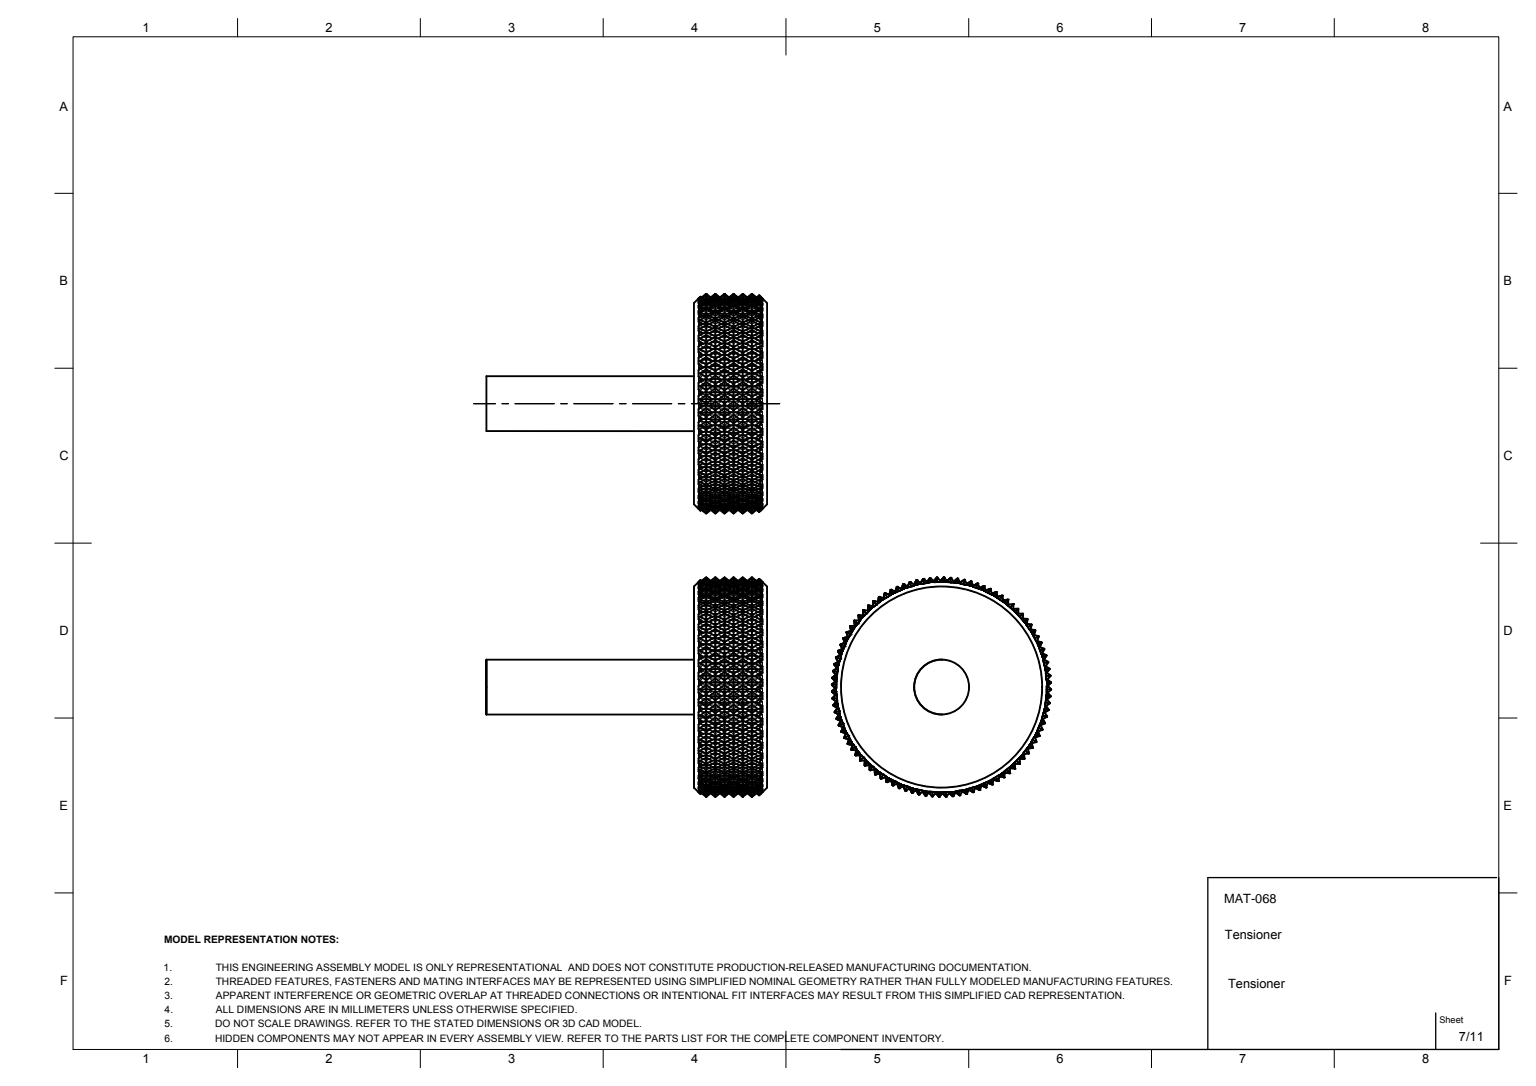
ISO-10303-21;
HEADER;
/* Generated by software containing ST-Developer
 * from STEP Tools, Inc. (www.steptools.com) 
 */

FILE_DESCRIPTION(
/* description */ ('CAx-IF Rec.Pracs.---Representation and Presentation of Product Manufa
cturing Information (PMI)---4.0---2014-10-13'),
/* implementation_level */ '2;1');

FILE_NAME(
/* name */ 'Tensioner.step',
/* time_stamp */ '2026-10-24T16:53:48-07:00',
/* author */ (''),
/* organization */ (''),
/* preprocessor_version */ 'ST-DEVELOPER v20.2',
/* originating_system */ 'Autodesk Translation Framework v15.17.0.0',
/* authorisation */ '');

FILE_SCHEMA (('AP242_MANAGED_MODEL_BASED_3D_ENGINEERING_MIM_LF { 1 0 10303 442 2 1 4 }'));
ENDSEC;

DATA;
#10=MECHANICAL_DESIGN_GEOMETRIC_PRESENTATION_REPRESENTATION('',(#3494),#107910);
#51=(
BOUNDED_CURVE()
B_SPLINE_CURVE(2,(#91091,#91092,#91093,#91094,#91095),.UNSPECIFIED.,.F.,
 .F.)
B_SPLINE_CURVE_WITH_KNOTS((3,2,3),(0.457349576892943,0.480683592164461,
0.539236617436895),.UNSPECIFIED.)
CURVE()
GEOMETRIC_REPRESENTATION_ITEM()
RATIONAL_B_SPLINE_CURVE((0.999326490452302,0.99964606396824,1.,0.999111853439226,
0.998440080679707))
REPRESENTATION_ITEM('')
);
#52=(
BOUNDED_CURVE()
B_SPLINE_CURVE(2,(#91384,#91385,#91386,#91387,#91388),.UNSPECIFIED.,.F.,
 .F.)
B_SPLINE_CURVE_WITH_KNOTS((3,2,3),(0.457349576892961,0.480683592164461,
0.539236615838568),.UNSPECIFIED.)
CURVE()
GEOMETRIC_REPRESENTATION_ITEM()
RATIONAL_B_SPLINE_CURVE((0.999326490452302,0.999646063968241,1.,0.99911185346347,
0.998440080716382))
REPRESENTATION_ITEM('')
);
#53=(
BOUNDED_CURVE()
B_SPLINE_CURVE(2,(#91904,#91905,#91906,#91907,#91908),.UNSPECIFIED.,.F.,
 .F.)
B_SPLINE_CURVE_WITH_KNOTS((3,2,3),(0.457349576892952,0.480683592164462,
0.539236618408897),.UNSPECIFIED.)
CURVE()
GEOMETRIC_REPRESENTATION_ITEM()
RATIONAL_B_SPLINE_CURVE((0.999326490452302,0.999646063968241,1.,0.999111853424483,
0.998440080657404))
REPRESENTATION_ITEM('')
);
#54=(
BOUNDED_CURVE()
B_SPLINE_CURVE(2,(#92179,#92180,#92181,#92182,#92183),.UNSPECIFIED.,.F.,
 .F.)
B_SPLINE_CURVE_WITH_KNOTS((3,2,3),(0.457349576892958,0.480683592164462,
0.539236618408893),.UNSPECIFIED.)
CURVE()
GEOMETRIC_REPRESENTATION_ITEM()
RATIONAL_B_SPLINE_CURVE((0.999326490452302,0.999646063968241,1.,0.999111853424483,
0.998440080657404))
REPRESENTATION_ITEM('')
);
#55=(
BOUNDED_CURVE()
B_SPLINE_CURVE(2,(#92403,#92404,#92405,#92406,#92407),.UNSPECIFIED.,.F.,
 .F.)
B_SPLINE_CURVE_WITH_KNOTS((3,2,3),(0.457349576892958,0.480683592164463,
0.539236618408894),.UNSPECIFIED.)
CURVE()
GEOMETRIC_REPRESENTATION_ITEM()
RATIONAL_B_SPLINE_CURVE((0.999326490452302,0.999646063968241,1.,0.999111853424483,
0.998440080657404))
REPRESENTATION_ITEM('')
);
#56=(
BOUNDED_CURVE()
B_SPLINE_CURVE(2,(#92707,#92708,#92709,#92710,#92711),.UNSPECIFIED.,.F.,
 .F.)
B_SPLINE_CURVE_WITH_KNOTS((3,2,3),(0.457349576892963,0.480683592164461,
0.539236618408894),.UNSPECIFIED.)
CURVE()
GEOMETRIC_REPRESENTATION_ITEM()
RATIONAL_B_SPLINE_CURVE((0.999326490452302,0.999646063968241,1.,0.999111853424483,
0.998440080657404))
REPRESENTATION_ITEM('')
);
#57=(
BOUNDED_CURVE()
B_SPLINE_CURVE(2,(#93011,#93012,#93013,#93014,#93015),.UNSPECIFIED.,.F.,
 .F.)
B_SPLINE_CURVE_WITH_KNOTS((3,2,3),(0.457349576892959,0.480683592164461,
0.539236618408895),.UNSPECIFIED.)
CURVE()
GEOMETRIC_REPRESENTATION_ITEM()
RATIONAL_B_SPLINE_CURVE((0.999326490452302,0.999646063968241,1.,0.999111853424483,
0.998440080657404))
REPRESENTATION_ITEM('')
);
#58=(
BOUNDED_CURVE()
B_SPLINE_CURVE(2,(#93315,#93316,#93317,#93318,#93319),.UNSPECIFIED.,.F.,
 .F.)
B_SPLINE_CURVE_WITH_KNOTS((3,2,3),(0.457349576892959,0.480683592164461,
0.539236615838582),.UNSPECIFIED.)
CURVE()
GEOMETRIC_REPRESENTATION_ITEM()
RATIONAL_B_SPLINE_CURVE((0.999326490452302,0.999646063968241,1.,0.99911185346347,
0.998440080716382))
REPRESENTATION_ITEM('')
);
#59=(
BOUNDED_CURVE()
B_SPLINE_CURVE(2,(#93619,#93620,#93621,#93622,#93623),.UNSPECIFIED.,.F.,
 .F.)
B_SPLINE_CURVE_WITH_KNOTS((3,2,3),(0.457349576892961,0.480683592164461,
0.539236618408892),.UNSPECIFIED.)
CURVE()
GEOMETRIC_REPRESENTATION_ITEM()
RATIONAL_B_SPLINE_CURVE((0.999326490452302,0.999646063968241,1.,0.999111853424483,
0.998440080657404))
REPRESENTATION_ITEM('')
);
#60=(
BOUNDED_CURVE()
B_SPLINE_CURVE(2,(#93923,#93924,#93925,#93926,#93927),.UNSPECIFIED.,.F.,
 .F.)
B_SPLINE_CURVE_WITH_KNOTS((3,2,3),(0.457349576892952,0.480683592164462,
0.539236615838583),.UNSPECIFIED.)
CURVE()
GEOMETRIC_REPRESENTATION_ITEM()
RATIONAL_B_SPLINE_CURVE((0.999326490452302,0.999646063968241,1.,0.99911185346347,
0.998440080716382))
REPRESENTATION_ITEM('')
);
#61=(
BOUNDED_CURVE()
B_SPLINE_CURVE(2,(#94227,#94228,#94229,#94230,#94231),.UNSPECIFIED.,.F.,
 .F.)
B_SPLINE_CURVE_WITH_KNOTS((3,2,3),(0.457349576892963,0.48068359216447,0.539236618408901),
 .UNSPECIFIED.)
CURVE()
GEOMETRIC_REPRESENTATION_ITEM()
RATIONAL_B_SPLINE_CURVE((0.999326490452302,0.999646063968241,1.,0.999111853424483,
0.998440080657404))
REPRESENTATION_ITEM('')
);
#62=(
BOUNDED_CURVE()
B_SPLINE_CURVE(2,(#94531,#94532,#94533,#94534,#94535),.UNSPECIFIED.,.F.,
 .F.)
B_SPLINE_CURVE_WITH_KNOTS((3,2,3),(0.457349576892948,0.48068359216446,0.539236618408892),
 .UNSPECIFIED.)
CURVE()
GEOMETRIC_REPRESENTATION_ITEM()
RATIONAL_B_SPLINE_CURVE((0.999326490452302,0.999646063968241,1.,0.999111853424483,
0.998440080657404))
REPRESENTATION_ITEM('')
);
#63=(
BOUNDED_CURVE()
B_SPLINE_CURVE(2,(#94835,#94836,#94837,#94838,#94839),.UNSPECIFIED.,.F.,
 .F.)
B_SPLINE_CURVE_WITH_KNOTS((3,2,3),(0.457349576892957,0.480683592164462,
0.539236618408896),.UNSPECIFIED.)
CURVE()
GEOMETRIC_REPRESENTATION_ITEM()
RATIONAL_B_SPLINE_CURVE((0.999326490452302,0.999646063968241,1.,0.999111853424483,
0.998440080657404))
REPRESENTATION_ITEM('')
);
#64=(
BOUNDED_CURVE()
B_SPLINE_CURVE(2,(#95139,#95140,#95141,#95142,#95143),.UNSPECIFIED.,.F.,
 .F.)
B_SPLINE_CURVE_WITH_KNOTS((3,2,3),(0.457349576892956,0.48068359216446,0.539236617436898),
 .UNSPECIFIED.)
CURVE()
GEOMETRIC_REPRESENTATION_ITEM()
RATIONAL_B_SPLINE_CURVE((0.999326490452302,0.999646063968241,1.,0.999111853439226,
0.998440080679707))
REPRESENTATION_ITEM('')
);
#65=(
BOUNDED_CURVE()
B_SPLINE_CURVE(2,(#95443,#95444,#95445,#95446,#95447),.UNSPECIFIED.,.F.,
 .F.)
B_SPLINE_CURVE_WITH_KNOTS((3,2,3),(0.457349576892961,0.480683592164473,
0.539236615838594),.UNSPECIFIED.)
CURVE()
GEOMETRIC_REPRESENTATION_ITEM()
RATIONAL_B_SPLINE_CURVE((0.999326490452302,0.999646063968241,1.,0.99911185346347,
0.998440080716382))
REPRESENTATION_ITEM('')
);
#66=(
BOUNDED_CURVE()
B_SPLINE_CURVE(2,(#95747,#95748,#95749,#95750,#95751),.UNSPECIFIED.,.F.,
 .F.)
B_SPLINE_CURVE_WITH_KNOTS((3,2,3),(0.457349576892959,0.480683592164459,
0.539236618408898),.UNSPECIFIED.)
CURVE()
GEOMETRIC_REPRESENTATION_ITEM()
RATIONAL_B_SPLINE_CURVE((0.999326490452302,0.999646063968241,1.,0.999111853424483,
0.998440080657404))
REPRESENTATION_ITEM('')
);
#67=(
BOUNDED_CURVE()
B_SPLINE_CURVE(2,(#96051,#96052,#96053,#96054,#96055),.UNSPECIFIED.,.F.,
 .F.)
B_SPLINE_CURVE_WITH_KNOTS((3,2,3),(0.457349576892962,0.480683592164469,
0.539236618408905),.UNSPECIFIED.)
CURVE()
GEOMETRIC_REPRESENTATION_ITEM()
RATIONAL_B_SPLINE_CURVE((0.999326490452302,0.999646063968241,1.,0.999111853424483,
0.998440080657404))
REPRESENTATION_ITEM('')
);
#68=(
BOUNDED_CURVE()
B_SPLINE_CURVE(2,(#96355,#96356,#96357,#96358,#96359),.UNSPECIFIED.,.F.,
 .F.)
B_SPLINE_CURVE_WITH_KNOTS((3,2,3),(0.457349576892966,0.480683592164469,
0.539236618408905),.UNSPECIFIED.)
CURVE()
GEOMETRIC_REPRESENTATION_ITEM()
RATIONAL_B_SPLINE_CURVE((0.999326490452302,0.999646063968241,1.,0.999111853424483,
0.998440080657404))
REPRESENTATION_ITEM('')
);
#69=(
BOUNDED_CURVE()
B_SPLINE_CURVE(2,(#96659,#96660,#96661,#96662,#96663),.UNSPECIFIED.,.F.,
 .F.)
B_SPLINE_CURVE_WITH_KNOTS((3,2,3),(0.457349576892951,0.48068359216446,0.539236618408896),
 .UNSPECIFIED.)
CURVE()
GEOMETRIC_REPRESENTATION_ITEM()
RATIONAL_B_SPLINE_CURVE((0.999326490452302,0.999646063968241,1.,0.999111853424483,
0.998440080657404))
REPRESENTATION_ITEM('')
);
#70=(
BOUNDED_CURVE()
B_SPLINE_CURVE(2,(#96963,#96964,#96965,#96966,#96967),.UNSPECIFIED.,.F.,
 .F.)
B_SPLINE_CURVE_WITH_KNOTS((3,2,3),(0.457349576892956,0.480683592164461,
0.539236618408896),.UNSPECIFIED.)
CURVE()
GEOMETRIC_REPRESENTATION_ITEM()
RATIONAL_B_SPLINE_CURVE((0.999326490452302,0.999646063968241,1.,0.999111853424483,
0.998440080657404))
REPRESENTATION_ITEM('')
);
#71=(
BOUNDED_CURVE()
B_SPLINE_CURVE(2,(#97267,#97268,#97269,#97270,#97271),.UNSPECIFIED.,.F.,
 .F.)
B_SPLINE_CURVE_WITH_KNOTS((3,2,3),(0.457349576892952,0.480683592164461,
0.539236618408892),.UNSPECIFIED.)
CURVE()
GEOMETRIC_REPRESENTATION_ITEM()
RATIONAL_B_SPLINE_CURVE((0.999326490452302,0.999646063968241,1.,0.999111853424483,
0.998440080657404))
REPRESENTATION_ITEM('')
);
#72=(
BOUNDED_CURVE()
B_SPLINE_CURVE(2,(#97571,#97572,#97573,#97574,#97575),.UNSPECIFIED.,.F.,
 .F.)
B_SPLINE_CURVE_WITH_KNOTS((3,2,3),(0.457349576892964,0.480683592164459,
0.539236618408898),.UNSPECIFIED.)
CURVE()
GEOMETRIC_REPRESENTATION_ITEM()
RATIONAL_B_SPLINE_CURVE((0.999326490452302,0.999646063968241,1.,0.999111853424483,
0.998440080657404))
REPRESENTATION_ITEM('')
);
#73=(
BOUNDED_CURVE()
B_SPLINE_CURVE(2,(#97875,#97876,#97877,#97878,#97879),.UNSPECIFIED.,.F.,
 .F.)
B_SPLINE_CURVE_WITH_KNOTS((3,2,3),(0.457349576892949,0.480683592164462,
0.539236618408898),.UNSPECIFIED.)
CURVE()
GEOMETRIC_REPRESENTATION_ITEM()
RATIONAL_B_SPLINE_CURVE((0.999326490452302,0.999646063968241,1.,0.999111853424483,
0.998440080657404))
REPRESENTATION_ITEM('')
);
#74=(
BOUNDED_CURVE()
B_SPLINE_CURVE(2,(#98179,#98180,#98181,#98182,#98183),.UNSPECIFIED.,.F.,
 .F.)
B_SPLINE_CURVE_WITH_KNOTS((3,2,3),(0.457349576892952,0.48068359216446,0.539236615838581),
 .UNSPECIFIED.)
CURVE()
GEOMETRIC_REPRESENTATION_ITEM()
RATIONAL_B_SPLINE_CURVE((0.999326490452302,0.999646063968241,1.,0.99911185346347,
0.998440080716382))
REPRESENTATION_ITEM('')
);
#75=(
BOUNDED_CURVE()
B_SPLINE_CURVE(2,(#98483,#98484,#98485,#98486,#98487),.UNSPECIFIED.,.F.,
 .F.)
B_SPLINE_CURVE_WITH_KNOTS((3,2,3),(0.457349576892958,0.48068359216446,0.539236618408894),
 .UNSPECIFIED.)
CURVE()
GEOMETRIC_REPRESENTATION_ITEM()
RATIONAL_B_SPLINE_CURVE((0.999326490452302,0.999646063968241,1.,0.999111853424483,
0.998440080657404))
REPRESENTATION_ITEM('')
);
#76=(
BOUNDED_CURVE()
B_SPLINE_CURVE(2,(#98787,#98788,#98789,#98790,#98791),.UNSPECIFIED.,.F.,
 .F.)
B_SPLINE_CURVE_WITH_KNOTS((3,2,3),(0.457349576892947,0.480683592164461,
0.539236617436902),.UNSPECIFIED.)
CURVE()
GEOMETRIC_REPRESENTATION_ITEM()
RATIONAL_B_SPLINE_CURVE((0.999326490452302,0.999646063968241,1.,0.999111853439226,
0.998440080679707))
REPRESENTATION_ITEM('')
);
#77=(
BOUNDED_CURVE()
B_SPLINE_CURVE(2,(#99091,#99092,#99093,#99094,#99095),.UNSPECIFIED.,.F.,
 .F.)
B_SPLINE_CURVE_WITH_KNOTS((3,2,3),(0.457349576892974,0.48068359216447,0.539236615838595),
 .UNSPECIFIED.)
CURVE()
GEOMETRIC_REPRESENTATION_ITEM()
RATIONAL_B_SPLINE_CURVE((0.999326490452302,0.999646063968241,1.,0.99911185346347,
0.998440080716382))
REPRESENTATION_ITEM('')
);
#78=(
BOUNDED_CURVE()
B_SPLINE_CURVE(2,(#99395,#99396,#99397,#99398,#99399),.UNSPECIFIED.,.F.,
 .F.)
B_SPLINE_CURVE_WITH_KNOTS((3,2,3),(0.457349576892952,0.480683592164461,
0.539236615838591),.UNSPECIFIED.)
CURVE()
GEOMETRIC_REPRESENTATION_ITEM()
RATIONAL_B_SPLINE_CURVE((0.999326490452302,0.999646063968241,1.,0.99911185346347,
0.998440080716382))
REPRESENTATION_ITEM('')
);
#79=(
BOUNDED_CURVE()
B_SPLINE_CURVE(2,(#99699,#99700,#99701,#99702,#99703),.UNSPECIFIED.,.F.,
 .F.)
B_SPLINE_CURVE_WITH_KNOTS((3,2,3),(0.457349576892966,0.480683592164471,
0.539236615838593),.UNSPECIFIED.)
CURVE()
GEOMETRIC_REPRESENTATION_ITEM()
RATIONAL_B_SPLINE_CURVE((0.999326490452302,0.999646063968241,1.,0.99911185346347,
0.998440080716382))
REPRESENTATION_ITEM('')
);
#80=(
BOUNDED_CURVE()
B_SPLINE_CURVE(2,(#100003,#100004,#100005,#100006,#100007),
 .UNSPECIFIED.,.F.,.F.)
B_SPLINE_CURVE_WITH_KNOTS((3,2,3),(0.457349576892955,0.48068359216446,0.539236618408892),
 .UNSPECIFIED.)
CURVE()
GEOMETRIC_REPRESENTATION_ITEM()
RATIONAL_B_SPLINE_CURVE((0.999326490452302,0.999646063968241,1.,0.999111853424483,
0.998440080657404))
REPRESENTATION_ITEM('')
);
#81=(
BOUNDED_CURVE()
B_SPLINE_CURVE(2,(#100307,#100308,#100309,#100310,#100311),
 .UNSPECIFIED.,.F.,.F.)
B_SPLINE_CURVE_WITH_KNOTS((3,2,3),(0.457349576892948,0.480683592164461,
0.539236618408894),.UNSPECIFIED.)
CURVE()
GEOMETRIC_REPRESENTATION_ITEM()
RATIONAL_B_SPLINE_CURVE((0.999326490452302,0.999646063968241,1.,0.999111853424483,
0.998440080657404))
REPRESENTATION_ITEM('')
);
#82=(
BOUNDED_CURVE()
B_SPLINE_CURVE(2,(#100611,#100612,#100613,#100614,#100615),
 .UNSPECIFIED.,.F.,.F.)
B_SPLINE_CURVE_WITH_KNOTS((3,2,3),(0.457349576892958,0.480683592164462,
0.539236615838579),.UNSPECIFIED.)
CURVE()
GEOMETRIC_REPRESENTATION_ITEM()
RATIONAL_B_SPLINE_CURVE((0.999326490452302,0.999646063968241,1.,0.99911185346347,
0.998440080716382))
REPRESENTATION_ITEM('')
);
#83=(
BOUNDED_CURVE()
B_SPLINE_CURVE(2,(#100915,#100916,#100917,#100918,#100919),
 .UNSPECIFIED.,.F.,.F.)
B_SPLINE_CURVE_WITH_KNOTS((3,2,3),(0.457349576892956,0.48068359216446,0.539236618408897),
 .UNSPECIFIED.)
CURVE()
GEOMETRIC_REPRESENTATION_ITEM()
RATIONAL_B_SPLINE_CURVE((0.999326490452302,0.999646063968241,1.,0.999111853424483,
0.998440080657404))
REPRESENTATION_ITEM('')
);
#84=(
BOUNDED_CURVE()
B_SPLINE_CURVE(2,(#101219,#101220,#101221,#101222,#101223),
 .UNSPECIFIED.,.F.,.F.)
B_SPLINE_CURVE_WITH_KNOTS((3,2,3),(0.457349576892958,0.480683592164462,
0.539236618408895),.UNSPECIFIED.)
CURVE()
GEOMETRIC_REPRESENTATION_ITEM()
RATIONAL_B_SPLINE_CURVE((0.999326490452302,0.999646063968241,1.,0.999111853424483,
0.998440080657404))
REPRESENTATION_ITEM('')
);
#85=(
BOUNDED_CURVE()
B_SPLINE_CURVE(2,(#101523,#101524,#101525,#101526,#101527),
 .UNSPECIFIED.,.F.,.F.)
B_SPLINE_CURVE_WITH_KNOTS((3,2,3),(0.457349576892956,0.480683592164458,
0.539236615838573),.UNSPECIFIED.)
CURVE()
GEOMETRIC_REPRESENTATION_ITEM()
RATIONAL_B_SPLINE_CURVE((0.999326490452302,0.999646063968241,1.,0.99911185346347,
0.998440080716382))
REPRESENTATION_ITEM('')
);
#86=(
BOUNDED_CURVE()
B_SPLINE_CURVE(2,(#101827,#101828,#101829,#101830,#101831),
 .UNSPECIFIED.,.F.,.F.)
B_SPLINE_CURVE_WITH_KNOTS((3,2,3),(0.457349576892953,0.48068359216446,0.539236618408898),
 .UNSPECIFIED.)
CURVE()
GEOMETRIC_REPRESENTATION_ITEM()
RATIONAL_B_SPLINE_CURVE((0.999326490452302,0.999646063968241,1.,0.999111853424483,
0.998440080657404))
REPRESENTATION_ITEM('')
);
#87=(
BOUNDED_CURVE()
B_SPLINE_CURVE(2,(#102131,#102132,#102133,#102134,#102135),
 .UNSPECIFIED.,.F.,.F.)
B_SPLINE_CURVE_WITH_KNOTS((3,2,3),(0.457349576892963,0.480683592164461,
0.539236618408896),.UNSPECIFIED.)
CURVE()
GEOMETRIC_REPRESENTATION_ITEM()
RATIONAL_B_SPLINE_CURVE((0.999326490452302,0.999646063968241,1.,0.999111853424483,
0.998440080657404))
REPRESENTATION_ITEM('')
);
#88=(
BOUNDED_CURVE()
B_SPLINE_CURVE(2,(#102435,#102436,#102437,#102438,#102439),
 .UNSPECIFIED.,.F.,.F.)
B_SPLINE_CURVE_WITH_KNOTS((3,2,3),(0.457349576892965,0.480683592164474,
0.539236615838598),.UNSPECIFIED.)
CURVE()
GEOMETRIC_REPRESENTATION_ITEM()
RATIONAL_B_SPLINE_CURVE((0.999326490452302,0.999646063968241,1.,0.99911185346347,
0.998440080716382))
REPRESENTATION_ITEM('')
);
#89=(
BOUNDED_CURVE()
B_SPLINE_CURVE(2,(#102739,#102740,#102741,#102742,#102743),
 .UNSPECIFIED.,.F.,.F.)
B_SPLINE_CURVE_WITH_KNOTS((3,2,3),(0.457349576892951,0.480683592164463,
0.5392366174369),.UNSPECIFIED.)
CURVE()
GEOMETRIC_REPRESENTATION_ITEM()
RATIONAL_B_SPLINE_CURVE((0.999326490452302,0.999646063968241,1.,0.999111853439226,
0.998440080679707))
REPRESENTATION_ITEM('')
);
#90=(
BOUNDED_CURVE()
B_SPLINE_CURVE(2,(#103043,#103044,#103045,#103046,#103047),
 .UNSPECIFIED.,.F.,.F.)
B_SPLINE_CURVE_WITH_KNOTS((3,2,3),(0.45734957689296,0.480683592164459,0.539236618408886),
 .UNSPECIFIED.)
CURVE()
GEOMETRIC_REPRESENTATION_ITEM()
RATIONAL_B_SPLINE_CURVE((0.999326490452302,0.999646063968241,1.,0.999111853424483,
0.998440080657404))
REPRESENTATION_ITEM('')
);
#91=(
BOUNDED_CURVE()
B_SPLINE_CURVE(2,(#103347,#103348,#103349,#103350,#103351),
 .UNSPECIFIED.,.F.,.F.)
B_SPLINE_CURVE_WITH_KNOTS((3,2,3),(0.457349576892963,0.48068359216447,0.5392366184089),
 .UNSPECIFIED.)
CURVE()
GEOMETRIC_REPRESENTATION_ITEM()
RATIONAL_B_SPLINE_CURVE((0.999326490452302,0.999646063968241,1.,0.999111853424483,
0.998440080657404))
REPRESENTATION_ITEM('')
);
#92=(
BOUNDED_CURVE()
B_SPLINE_CURVE(2,(#103651,#103652,#103653,#103654,#103655),
 .UNSPECIFIED.,.F.,.F.)
B_SPLINE_CURVE_WITH_KNOTS((3,2,3),(0.457349576892972,0.480683592164467,
0.539236618408904),.UNSPECIFIED.)
CURVE()
GEOMETRIC_REPRESENTATION_ITEM()
RATIONAL_B_SPLINE_CURVE((0.999326490452302,0.999646063968241,1.,0.999111853424483,
0.998440080657404))
REPRESENTATION_ITEM('')
);
#93=(
BOUNDED_CURVE()
B_SPLINE_CURVE(2,(#103955,#103956,#103957,#103958,#103959),
 .UNSPECIFIED.,.F.,.F.)
B_SPLINE_CURVE_WITH_KNOTS((3,2,3),(0.457349576892955,0.480683592164463,
0.539236618408902),.UNSPECIFIED.)
CURVE()
GEOMETRIC_REPRESENTATION_ITEM()
RATIONAL_B_SPLINE_CURVE((0.999326490452302,0.999646063968241,1.,0.999111853424483,
0.998440080657404))
REPRESENTATION_ITEM('')
);
#94=(
BOUNDED_CURVE()
B_SPLINE_CURVE(2,(#104259,#104260,#104261,#104262,#104263),
 .UNSPECIFIED.,.F.,.F.)
B_SPLINE_CURVE_WITH_KNOTS((3,2,3),(0.457349576892956,0.48068359216446,0.539236618408889),
 .UNSPECIFIED.)
CURVE()
GEOMETRIC_REPRESENTATION_ITEM()
RATIONAL_B_SPLINE_CURVE((0.999326490452302,0.999646063968241,1.,0.999111853424483,
0.998440080657404))
REPRESENTATION_ITEM('')
);
#95=(
BOUNDED_CURVE()
B_SPLINE_CURVE(2,(#104563,#104564,#104565,#104566,#104567),
 .UNSPECIFIED.,.F.,.F.)
B_SPLINE_CURVE_WITH_KNOTS((3,2,3),(0.457349576892965,0.480683592164471,
0.539236618408903),.UNSPECIFIED.)
CURVE()
GEOMETRIC_REPRESENTATION_ITEM()
RATIONAL_B_SPLINE_CURVE((0.999326490452302,0.999646063968241,1.,0.999111853424483,
0.998440080657404))
REPRESENTATION_ITEM('')
);
#96=(
BOUNDED_CURVE()
B_SPLINE_CURVE(2,(#104867,#104868,#104869,#104870,#104871),
 .UNSPECIFIED.,.F.,.F.)
B_SPLINE_CURVE_WITH_KNOTS((3,2,3),(0.457349576892956,0.480683592164462,
0.539236618408896),.UNSPECIFIED.)
CURVE()
GEOMETRIC_REPRESENTATION_ITEM()
RATIONAL_B_SPLINE_CURVE((0.999326490452302,0.999646063968241,1.,0.999111853424483,
0.998440080657404))
REPRESENTATION_ITEM('')
);
#97=(
BOUNDED_CURVE()
B_SPLINE_CURVE(2,(#105171,#105172,#105173,#105174,#105175),
 .UNSPECIFIED.,.F.,.F.)
B_SPLINE_CURVE_WITH_KNOTS((3,2,3),(0.45734957689296,0.480683592164462,0.539236618408894),
 .UNSPECIFIED.)
CURVE()
GEOMETRIC_REPRESENTATION_ITEM()
RATIONAL_B_SPLINE_CURVE((0.999326490452302,0.999646063968241,1.,0.999111853424483,
0.998440080657404))
REPRESENTATION_ITEM('')
);
#98=(
BOUNDED_CURVE()
B_SPLINE_CURVE(2,(#105475,#105476,#105477,#105478,#105479),
 .UNSPECIFIED.,.F.,.F.)
B_SPLINE_CURVE_WITH_KNOTS((3,2,3),(0.457349576892957,0.480683592164459,
0.539236618408901),.UNSPECIFIED.)
CURVE()
GEOMETRIC_REPRESENTATION_ITEM()
RATIONAL_B_SPLINE_CURVE((0.999326490452302,0.999646063968241,1.,0.999111853424483,
0.998440080657404))
REPRESENTATION_ITEM('')
);
#99=(
BOUNDED_CURVE()
B_SPLINE_CURVE(2,(#105779,#105780,#105781,#105782,#105783),
 .UNSPECIFIED.,.F.,.F.)
B_SPLINE_CURVE_WITH_KNOTS((3,2,3),(0.457349576892957,0.480683592164462,
0.539236615838586),.UNSPECIFIED.)
CURVE()
GEOMETRIC_REPRESENTATION_ITEM()
RATIONAL_B_SPLINE_CURVE((0.999326490452302,0.999646063968241,1.,0.99911185346347,
0.998440080716382))
REPRESENTATION_ITEM('')
);
#100=(
BOUNDED_CURVE()
B_SPLINE_CURVE(2,(#106083,#106084,#106085,#106086,#106087),
 .UNSPECIFIED.,.F.,.F.)
B_SPLINE_CURVE_WITH_KNOTS((3,2,3),(0.457349576892964,0.480683592164471,
0.539236615838594),.UNSPECIFIED.)
CURVE()
GEOMETRIC_REPRESENTATION_ITEM()
RATIONAL_B_SPLINE_CURVE((0.999326490452302,0.999646063968241,1.,0.99911185346347,
0.998440080716382))
REPRESENTATION_ITEM('')
);
#101=(
BOUNDED_SURFACE()
B_SPLINE_SURFACE(1,2,((#65259,#65260,#65261),(#65262,#65263,#65264)),
 .UNSPECIFIED.,.F.,.F.,.F.)
B_SPLINE_SURFACE_WITH_KNOTS((2,2),(3,3),(0.,1.),(0.0556006976418392,0.0675888856590501),
 .UNSPECIFIED.)
GEOMETRIC_REPRESENTATION_ITEM()
RATIONAL_B_SPLINE_SURFACE(((0.996397562408606,0.996150386832629,0.997319912843745),
(0.996397562408606,0.996150386832629,0.997319912843745)))
REPRESENTATION_ITEM('')
SURFACE()
);
#102=(
BOUNDED_SURFACE()
B_SPLINE_SURFACE(1,2,((#65277,#65278,#65279),(#65280,#65281,#65282),(#65283,
#65284,#65285)),.UNSPECIFIED.,.F.,.F.,.F.)
B_SPLINE_SURFACE_WITH_KNOTS((2,1,2),(3,3),(-0.000171761237665326,1.,1.00600020634817),
(0.066589869885605,0.0751324139155164),.UNSPECIFIED.)
GEOMETRIC_REPRESENTATION_ITEM()
RATIONAL_B_SPLINE_SURFACE(((0.997134830028878,0.997884084852412,0.999352698774608),
(0.997134830028878,0.997884084852412,0.999352698774608),(0.997134830028879,
0.997884084852412,0.999352698774608)))
REPRESENTATION_ITEM('')
SURFACE()
);
#103=(
BOUNDED_SURFACE()
B_SPLINE_SURFACE(1,2,((#65395,#65396,#65397),(#65398,#65399,#65400),(#65401,
#65402,#65403)),.UNSPECIFIED.,.F.,.F.,.F.)
B_SPLINE_SURFACE_WITH_KNOTS((2,1,2),(3,3),(0.,1.,1.01),(0.0456081671210044,
0.057598944781882),.UNSPECIFIED.)
GEOMETRIC_REPRESENTATION_ITEM()
RATIONAL_B_SPLINE_SURFACE(((0.997793907739636,0.996365558499688,0.996354522974128),
(0.997793907739636,0.996365558499688,0.996354522974128),(0.997793907739636,
0.996365558499688,0.996354522974128)))
REPRESENTATION_ITEM('')
SURFACE()
);
#104=(
BOUNDED_SURFACE()
B_SPLINE_SURFACE(1,2,((#65416,#65417,#65418),(#65419,#65420,#65421),(#65422,
#65423,#65424)),.UNSPECIFIED.,.F.,.F.,.F.)
B_SPLINE_SURFACE_WITH_KNOTS((2,1,2),(3,3),(0.,1.,1.01),(0.0556006976418428,
0.0675888856590486),.UNSPECIFIED.)
GEOMETRIC_REPRESENTATION_ITEM()
RATIONAL_B_SPLINE_SURFACE(((0.996397562408606,0.996150386832629,0.997319912843744),
(0.996397562408606,0.996150386832629,0.997319912843744),(0.996397562408606,
0.996150386832629,0.997319912843744)))
REPRESENTATION_ITEM('')
SURFACE()
);
#105=(
BOUNDED_SURFACE()
B_SPLINE_SURFACE(1,2,((#65482,#65483,#65484),(#65485,#65486,#65487),(#65488,
#65489,#65490)),.UNSPECIFIED.,.F.,.F.,.F.)
B_SPLINE_SURFACE_WITH_KNOTS((2,1,2),(3,3),(-0.00286810173538045,0.,0.477902879811279),
(0.0466073985929118,0.053183492915798),.UNSPECIFIED.)
GEOMETRIC_REPRESENTATION_ITEM()
RATIONAL_B_SPLINE_SURFACE(((0.997565691989291,0.996847118055594,0.996554836292953),
(0.997565691989291,0.996847118055594,0.996554836292953),(0.997565691989291,
0.996847118055594,0.996554836292953)))
REPRESENTATION_ITEM('')
SURFACE()
);
#106=(
BOUNDED_SURFACE()
B_SPLINE_SURFACE(1,2,((#65501,#65502,#65503),(#65504,#65505,#65506),(#65507,
#65508,#65509)),.UNSPECIFIED.,.F.,.F.,.F.)
B_SPLINE_SURFACE_WITH_KNOTS((2,1,2),(3,3),(-0.00286764392039102,0.,0.477902879807514),
(0.0565997133101203,0.0631721430887056),.UNSPECIFIED.)
GEOMETRIC_REPRESENTATION_ITEM()
RATIONAL_B_SPLINE_SURFACE(((0.996366204684738,0.996295417244646,0.996650447003324),
(0.996366204684738,0.996295417244646,0.996650447003324),(0.996366204684738,
0.996295417244646,0.996650447003324)))
REPRESENTATION_ITEM('')
SURFACE()
);
#107=(
BOUNDED_SURFACE()
B_SPLINE_SURFACE(1,2,((#65532,#65533,#65534,#65535,#65536),(#65537,#65538,
#65539,#65540,#65541),(#65542,#65543,#65544,#65545,#65546)),
 .UNSPECIFIED.,.F.,.F.,.F.)
B_SPLINE_SURFACE_WITH_KNOTS((2,1,2),(3,2,3),(0.,1.,1.01),(0.03559319327139,
0.0384615384615384,0.0476086899858148),.UNSPECIFIED.)
GEOMETRIC_REPRESENTATION_ITEM()
RATIONAL_B_SPLINE_SURFACE(((0.998993602249807,0.999456249886298,1.,0.9982659811314,
0.997356751596327),(0.998993602249807,0.999456249886298,1.,0.9982659811314,
0.997356751596327),(0.998993602249807,0.999456249886298,1.,0.9982659811314,
0.997356751596327)))
REPRESENTATION_ITEM('')
SURFACE()
);
#108=(
BOUNDED_SURFACE()
B_SPLINE_SURFACE(1,2,((#65572,#65573,#65574),(#65575,#65576,#65577)),
 .UNSPECIFIED.,.F.,.F.,.F.)
B_SPLINE_SURFACE_WITH_KNOTS((2,2),(3,3),(0.,1.),(0.0456081671210079,0.0575989447818804),
 .UNSPECIFIED.)
GEOMETRIC_REPRESENTATION_ITEM()
RATIONAL_B_SPLINE_SURFACE(((0.997793907739635,0.996365558499688,0.996354522974128),
(0.997793907739635,0.996365558499688,0.996354522974128)))
REPRESENTATION_ITEM('')
SURFACE()
);
#109=(
BOUNDED_SURFACE()
B_SPLINE_SURFACE(1,2,((#65635,#65636,#65637,#65638,#65639),(#65640,#65641,
#65642,#65643,#65644),(#65645,#65646,#65647,#65648,#65649)),
 .UNSPECIFIED.,.F.,.F.,.F.)
B_SPLINE_SURFACE_WITH_KNOTS((2,1,2),(3,2,3),(-0.00286743094908464,0.,0.480770297171449),
(0.0365944846643089,0.0384615384615384,0.0431859280915203),
 .UNSPECIFIED.)
GEOMETRIC_REPRESENTATION_ITEM()
RATIONAL_B_SPLINE_SURFACE(((0.999326490452167,0.999646063968166,1.,0.999104400890347,
0.9984288220563),(0.999326490452167,0.999646063968166,1.,0.999104400890347,
0.9984288220563),(0.999326490452167,0.999646063968166,1.,0.999104400890347,
0.9984288220563)))
REPRESENTATION_ITEM('')
SURFACE()
);
#110=(
BOUNDED_SURFACE()
B_SPLINE_SURFACE(1,2,((#65665,#65666,#65667),(#65668,#65669,#65670),(#65671,
#65672,#65673)),.UNSPECIFIED.,.F.,.F.,.F.)
B_SPLINE_SURFACE_WITH_KNOTS((2,1,2),(3,3),(-0.0028681017738025,0.,0.477902879812032),
(0.046607398592911,0.0531834933545499),.UNSPECIFIED.)
GEOMETRIC_REPRESENTATION_ITEM()
RATIONAL_B_SPLINE_SURFACE(((0.997565691989291,0.99684711800765,0.996554836253951),
(0.997565691989291,0.99684711800765,0.996554836253951),(0.997565691989291,
0.99684711800765,0.996554836253951)))
REPRESENTATION_ITEM('')
SURFACE()
);
#111=(
BOUNDED_SURFACE()
B_SPLINE_SURFACE(1,2,((#65701,#65702,#65703),(#65704,#65705,#65706)),
 .UNSPECIFIED.,.F.,.F.,.F.)
B_SPLINE_SURFACE_WITH_KNOTS((2,2),(3,3),(0.,1.),(0.0255903596131799,0.0375948596693886),
 .UNSPECIFIED.)
GEOMETRIC_REPRESENTATION_ITEM()
RATIONAL_B_SPLINE_SURFACE(((0.996753121755999,0.997505687613148,0.999678813023854),
(0.996753121755999,0.997505687613148,0.999678813023854)))
REPRESENTATION_ITEM('')
SURFACE()
);
#112=(
BOUNDED_SURFACE()
B_SPLINE_SURFACE(1,2,((#65719,#65720,#65721,#65722,#65723),(#65724,#65725,
#65726,#65727,#65728),(#65729,#65730,#65731,#65732,#65733)),
 .UNSPECIFIED.,.F.,.F.,.F.)
B_SPLINE_SURFACE_WITH_KNOTS((2,1,2),(3,2,3),(0.,1.,1.01),(0.0355931932713904,
0.0384615384615384,0.0476086899858121),.UNSPECIFIED.)
GEOMETRIC_REPRESENTATION_ITEM()
RATIONAL_B_SPLINE_SURFACE(((0.998993602249807,0.999456249886298,1.,0.998265981131401,
0.997356751596327),(0.998993602249807,0.999456249886298,1.,0.998265981131401,
0.997356751596327),(0.998993602249807,0.999456249886298,1.,0.998265981131401,
0.997356751596327)))
REPRESENTATION_ITEM('')
SURFACE()
);
#113=(
BOUNDED_SURFACE()
B_SPLINE_SURFACE(1,2,((#65830,#65831,#65832,#65833,#65834),(#65835,#65836,
#65837,#65838,#65839)),.UNSPECIFIED.,.F.,.F.,.F.)
B_SPLINE_SURFACE_WITH_KNOTS((2,2),(3,2,3),(0.,0.480770297146589),(0.0365944846642941,
0.0384615384615384,0.0431859280915188),.UNSPECIFIED.)
GEOMETRIC_REPRESENTATION_ITEM()
RATIONAL_B_SPLINE_SURFACE(((0.999326490452162,0.999646063968163,1.,0.999104400890347,
0.9984288220563),(0.999326490452162,0.999646063968163,1.,0.999104400890347,
0.9984288220563)))
REPRESENTATION_ITEM('')
SURFACE()
);
#114=(
BOUNDED_SURFACE()
B_SPLINE_SURFACE(1,2,((#65900,#65901,#65902),(#65903,#65904,#65905),(#65906,
#65907,#65908)),.UNSPECIFIED.,.F.,.F.,.F.)
B_SPLINE_SURFACE_WITH_KNOTS((2,1,2),(3,3),(-0.01,0.,1.),(0.0255903596131809,
0.0375948596693858),.UNSPECIFIED.)
GEOMETRIC_REPRESENTATION_ITEM()
RATIONAL_B_SPLINE_SURFACE(((0.996753121755999,0.997505687613148,0.999678813023853),
(0.996753121755999,0.997505687613148,0.999678813023853),(0.996753121755999,
0.997505687613148,0.999678813023853)))
REPRESENTATION_ITEM('')
SURFACE()
);
#115=(
BOUNDED_SURFACE()
B_SPLINE_SURFACE(1,2,((#66030,#66031,#66032),(#66033,#66034,#66035),(#66036,
#66037,#66038)),.UNSPECIFIED.,.F.,.F.,.F.)
B_SPLINE_SURFACE_WITH_KNOTS((2,1,2),(3,3),(-0.01,0.,1.00000001517992),(0.00560769168370699,
0.0176009700440532),.UNSPECIFIED.)
GEOMETRIC_REPRESENTATION_ITEM()
RATIONAL_B_SPLINE_SURFACE(((0.99818389211382,0.99657330421516,0.996380621259469),
(0.99818389211382,0.99657330421516,0.996380621259469),(0.99818389211382,
0.99657330421516,0.996380621259469)))
REPRESENTATION_ITEM('')
SURFACE()
);
#116=(
BOUNDED_SURFACE()
B_SPLINE_SURFACE(1,2,((#66180,#66181,#66182),(#66183,#66184,#66185),(#66186,
#66187,#66188)),.UNSPECIFIED.,.F.,.F.,.F.)
B_SPLINE_SURFACE_WITH_KNOTS((2,1,2),(3,3),(-0.01,0.,1.00000001523837),(0.0056076916836887,
0.0176009700440532),.UNSPECIFIED.)
GEOMETRIC_REPRESENTATION_ITEM()
RATIONAL_B_SPLINE_SURFACE(((0.998183892113825,0.99657330421516,0.996380621259469),
(0.998183892113825,0.99657330421516,0.996380621259469),(0.998183892113825,
0.99657330421516,0.996380621259469)))
REPRESENTATION_ITEM('')
SURFACE()
);
#117=(
BOUNDED_SURFACE()
B_SPLINE_SURFACE(1,2,((#66306,#66307,#66308),(#66309,#66310,#66311)),
 .UNSPECIFIED.,.F.,.F.,.F.)
B_SPLINE_SURFACE_WITH_KNOTS((2,2),(3,3),(0.,1.),(0.0556006976418416,0.0675888856590493),
 .UNSPECIFIED.)
GEOMETRIC_REPRESENTATION_ITEM()
RATIONAL_B_SPLINE_SURFACE(((0.996397562408606,0.996150386832629,0.997319912843745),
(0.996397562408606,0.996150386832629,0.997319912843745)))
REPRESENTATION_ITEM('')
SURFACE()
);
#118=(
BOUNDED_SURFACE()
B_SPLINE_SURFACE(1,2,((#66374,#66375,#66376),(#66377,#66378,#66379),(#66380,
#66381,#66382)),.UNSPECIFIED.,.F.,.F.,.F.)
B_SPLINE_SURFACE_WITH_KNOTS((2,1,2),(3,3),(0.,1.,1.01),(0.0456081671210036,
0.0575989447818809),.UNSPECIFIED.)
GEOMETRIC_REPRESENTATION_ITEM()
RATIONAL_B_SPLINE_SURFACE(((0.997793907739636,0.996365558499688,0.996354522974128),
(0.997793907739636,0.996365558499688,0.996354522974128),(0.997793907739636,
0.996365558499688,0.996354522974128)))
REPRESENTATION_ITEM('')
SURFACE()
);
#119=(
BOUNDED_SURFACE()
B_SPLINE_SURFACE(1,2,((#66394,#66395,#66396),(#66397,#66398,#66399),(#66400,
#66401,#66402)),.UNSPECIFIED.,.F.,.F.,.F.)
B_SPLINE_SURFACE_WITH_KNOTS((2,1,2),(3,3),(-0.00286810173540422,0.,0.477902879809766),
(0.0466073985929115,0.0531834929157974),.UNSPECIFIED.)
GEOMETRIC_REPRESENTATION_ITEM()
RATIONAL_B_SPLINE_SURFACE(((0.997565691989291,0.996847118055594,0.996554836292953),
(0.997565691989291,0.996847118055594,0.996554836292953),(0.997565691989291,
0.996847118055593,0.996554836292953)))
REPRESENTATION_ITEM('')
SURFACE()
);
#120=(
BOUNDED_SURFACE()
B_SPLINE_SURFACE(1,2,((#66448,#66449,#66450,#66451,#66452),(#66453,#66454,
#66455,#66456,#66457),(#66458,#66459,#66460,#66461,#66462)),
 .UNSPECIFIED.,.F.,.F.,.F.)
B_SPLINE_SURFACE_WITH_KNOTS((2,1,2),(3,2,3),(0.,1.,1.01),(0.0355931932713902,
0.0384615384615384,0.0476086899858131),.UNSPECIFIED.)
GEOMETRIC_REPRESENTATION_ITEM()
RATIONAL_B_SPLINE_SURFACE(((0.998993602249807,0.999456249886298,1.,0.998265981131401,
0.997356751596327),(0.998993602249807,0.999456249886298,1.,0.998265981131401,
0.997356751596327),(0.998993602249807,0.999456249886298,1.,0.998265981131401,
0.997356751596327)))
REPRESENTATION_ITEM('')
SURFACE()
);
#121=(
BOUNDED_SURFACE()
B_SPLINE_SURFACE(1,2,((#66510,#66511,#66512,#66513,#66514),(#66515,#66516,
#66517,#66518,#66519),(#66520,#66521,#66522,#66523,#66524)),
 .UNSPECIFIED.,.F.,.F.,.F.)
B_SPLINE_SURFACE_WITH_KNOTS((2,1,2),(3,2,3),(-0.00286743095031093,0.,0.480770297170425),
(0.0365944846643235,0.0384615384615384,0.0431859280915194),
 .UNSPECIFIED.)
GEOMETRIC_REPRESENTATION_ITEM()
RATIONAL_B_SPLINE_SURFACE(((0.999326490452172,0.999646063968169,1.,0.999104400890347,
0.9984288220563),(0.999326490452172,0.999646063968169,1.,0.999104400890347,
0.9984288220563),(0.999326490452172,0.999646063968169,1.,0.999104400890347,
0.9984288220563)))
REPRESENTATION_ITEM('')
SURFACE()
);
#122=(
BOUNDED_SURFACE()
B_SPLINE_SURFACE(1,2,((#66551,#66552,#66553),(#66554,#66555,#66556)),
 .UNSPECIFIED.,.F.,.F.,.F.)
B_SPLINE_SURFACE_WITH_KNOTS((2,2),(3,3),(0.,1.),(0.025590359613181,0.0375948596693881),
 .UNSPECIFIED.)
GEOMETRIC_REPRESENTATION_ITEM()
RATIONAL_B_SPLINE_SURFACE(((0.996753121755999,0.997505687613148,0.999678813023854),
(0.996753121755999,0.997505687613148,0.999678813023854)))
REPRESENTATION_ITEM('')
SURFACE()
);
#123=(
BOUNDED_SURFACE()
B_SPLINE_SURFACE(1,2,((#66591,#66592,#66593),(#66594,#66595,#66596),(#66597,
#66598,#66599)),.UNSPECIFIED.,.F.,.F.,.F.)
B_SPLINE_SURFACE_WITH_KNOTS((2,1,2),(3,3),(-0.00286823356222208,0.,0.477902879811012),
(0.0265907346180619,0.0331702037252919),.UNSPECIFIED.)
GEOMETRIC_REPRESENTATION_ITEM()
RATIONAL_B_SPLINE_SURFACE(((0.996888414395785,0.99736576547994,0.998269846384985),
(0.996888414395785,0.99736576547994,0.998269846384985),(0.996888414395785,
0.99736576547994,0.998269846384985)))
REPRESENTATION_ITEM('')
SURFACE()
);
#124=(
BOUNDED_SURFACE()
B_SPLINE_SURFACE(1,2,((#66698,#66699,#66700),(#66701,#66702,#66703),(#66704,
#66705,#66706),(#66707,#66708,#66709)),.UNSPECIFIED.,.F.,.F.,.F.)
B_SPLINE_SURFACE_WITH_KNOTS((2,1,1,2),(3,3),(-0.01,0.,1.,1.0101),(0.00560769168370619,
0.0176009700440517),.UNSPECIFIED.)
GEOMETRIC_REPRESENTATION_ITEM()
RATIONAL_B_SPLINE_SURFACE(((0.99818389211382,0.99657330421516,0.996380621259469),
(0.99818389211382,0.99657330421516,0.996380621259469),(0.99818389211382,
0.99657330421516,0.996380621259469),(0.99818389211382,0.99657330421516,
0.996380621259469)))
REPRESENTATION_ITEM('')
SURFACE()
);
#125=(
BOUNDED_SURFACE()
B_SPLINE_SURFACE(1,2,((#66832,#66833,#66834),(#66835,#66836,#66837)),
 .UNSPECIFIED.,.F.,.F.,.F.)
B_SPLINE_SURFACE_WITH_KNOTS((2,2),(3,3),(0.,1.),(0.0556006976418412,0.0675888856590511),
 .UNSPECIFIED.)
GEOMETRIC_REPRESENTATION_ITEM()
RATIONAL_B_SPLINE_SURFACE(((0.996397562408606,0.996150386832629,0.997319912843745),
(0.996397562408606,0.996150386832629,0.997319912843745)))
REPRESENTATION_ITEM('')
SURFACE()
);
#126=(
BOUNDED_SURFACE()
B_SPLINE_SURFACE(1,2,((#66906,#66907,#66908),(#66909,#66910,#66911),(#66912,
#66913,#66914)),.UNSPECIFIED.,.F.,.F.,.F.)
B_SPLINE_SURFACE_WITH_KNOTS((2,1,2),(3,3),(0.,1.,1.01),(0.0456081671210034,
0.0575989447818821),.UNSPECIFIED.)
GEOMETRIC_REPRESENTATION_ITEM()
RATIONAL_B_SPLINE_SURFACE(((0.997793907739636,0.996365558499688,0.996354522974128),
(0.997793907739636,0.996365558499688,0.996354522974128),(0.997793907739636,
0.996365558499688,0.996354522974128)))
REPRESENTATION_ITEM('')
SURFACE()
);
#127=(
BOUNDED_SURFACE()
B_SPLINE_SURFACE(1,2,((#66949,#66950,#66951),(#66952,#66953,#66954),(#66955,
#66956,#66957)),.UNSPECIFIED.,.F.,.F.,.F.)
B_SPLINE_SURFACE_WITH_KNOTS((2,1,2),(3,3),(-0.00286810173547451,0.,0.477902879808668),
(0.0466073985929113,0.0531834929157984),.UNSPECIFIED.)
GEOMETRIC_REPRESENTATION_ITEM()
RATIONAL_B_SPLINE_SURFACE(((0.997565691989291,0.996847118055593,0.996554836292953),
(0.997565691989291,0.996847118055593,0.996554836292953),(0.997565691989291,
0.996847118055593,0.996554836292953)))
REPRESENTATION_ITEM('')
SURFACE()
);
#128=(
BOUNDED_SURFACE()
B_SPLINE_SURFACE(1,2,((#66968,#66969,#66970,#66971,#66972),(#66973,#66974,
#66975,#66976,#66977),(#66978,#66979,#66980,#66981,#66982)),
 .UNSPECIFIED.,.F.,.F.,.F.)
B_SPLINE_SURFACE_WITH_KNOTS((2,1,2),(3,2,3),(0.,1.,1.01),(0.0355931932713904,
0.0384615384615384,0.0476086899858127),.UNSPECIFIED.)
GEOMETRIC_REPRESENTATION_ITEM()
RATIONAL_B_SPLINE_SURFACE(((0.998993602249807,0.999456249886298,1.,0.998265981131401,
0.997356751596327),(0.998993602249807,0.999456249886298,1.,0.998265981131401,
0.997356751596327),(0.998993602249807,0.999456249886298,1.,0.998265981131401,
0.997356751596327)))
REPRESENTATION_ITEM('')
SURFACE()
);
#129=(
BOUNDED_SURFACE()
B_SPLINE_SURFACE(1,2,((#67007,#67008,#67009,#67010,#67011),(#67012,#67013,
#67014,#67015,#67016),(#67017,#67018,#67019,#67020,#67021)),
 .UNSPECIFIED.,.F.,.F.,.F.)
B_SPLINE_SURFACE_WITH_KNOTS((2,1,2),(3,2,3),(-0.00141401191197287,0.,0.480770297102985),
(0.0365944846645793,0.0384615384615384,0.0431859280915182),
 .UNSPECIFIED.)
GEOMETRIC_REPRESENTATION_ITEM()
RATIONAL_B_SPLINE_SURFACE(((0.99932649045226,0.999646063968218,1.,0.999104400890347,
0.9984288220563),(0.99932649045226,0.999646063968218,1.,0.999104400890347,
0.9984288220563),(0.99932649045226,0.999646063968218,1.,0.999104400890347,
0.9984288220563)))
REPRESENTATION_ITEM('')
SURFACE()
);
#130=(
BOUNDED_SURFACE()
B_SPLINE_SURFACE(1,2,((#67077,#67078,#67079),(#67080,#67081,#67082),(#67083,
#67084,#67085)),.UNSPECIFIED.,.F.,.F.,.F.)
B_SPLINE_SURFACE_WITH_KNOTS((2,1,2),(3,3),(0.,1.,1.01),(0.0255903596131785,
0.0375948596693883),.UNSPECIFIED.)
GEOMETRIC_REPRESENTATION_ITEM()
RATIONAL_B_SPLINE_SURFACE(((0.996753121755999,0.997505687613148,0.999678813023854),
(0.996753121755999,0.997505687613148,0.999678813023854),(0.996753121755999,
0.997505687613148,0.999678813023854)))
REPRESENTATION_ITEM('')
SURFACE()
);
#131=(
BOUNDED_SURFACE()
B_SPLINE_SURFACE(1,2,((#67120,#67121,#67122),(#67123,#67124,#67125),(#67126,
#67127,#67128)),.UNSPECIFIED.,.F.,.F.,.F.)
B_SPLINE_SURFACE_WITH_KNOTS((2,1,2),(3,3),(-0.00286823356243391,0.,0.477902879809815),
(0.0265907346180619,0.0331702037252936),.UNSPECIFIED.)
GEOMETRIC_REPRESENTATION_ITEM()
RATIONAL_B_SPLINE_SURFACE(((0.996888414395785,0.997365765479939,0.998269846384985),
(0.996888414395785,0.997365765479939,0.998269846384985),(0.996888414395785,
0.997365765479939,0.998269846384985)))
REPRESENTATION_ITEM('')
SURFACE()
);
#132=(
BOUNDED_SURFACE()
B_SPLINE_SURFACE(1,2,((#67195,#67196,#67197),(#67198,#67199,#67200),(#67201,
#67202,#67203)),.UNSPECIFIED.,.F.,.F.,.F.)
B_SPLINE_SURFACE_WITH_KNOTS((2,1,2),(3,3),(-0.00286753128221124,0.,0.477902879810469),
(0.0166015299238957,0.023173678811188),.UNSPECIFIED.)
GEOMETRIC_REPRESENTATION_ITEM()
RATIONAL_B_SPLINE_SURFACE(((0.996422581660833,0.996252244737342,0.996507688616405),
(0.996422581660833,0.996252244737342,0.996507688616405),(0.996422581660833,
0.996252244737342,0.996507688616405)))
REPRESENTATION_ITEM('')
SURFACE()
);
#133=(
BOUNDED_SURFACE()
B_SPLINE_SURFACE(1,2,((#67220,#67221,#67222),(#67223,#67224,#67225),(#67226,
#67227,#67228),(#67229,#67230,#67231)),.UNSPECIFIED.,.F.,.F.,.F.)
B_SPLINE_SURFACE_WITH_KNOTS((2,1,1,2),(3,3),(-0.0101,0.,1.,1.01),(0.00560769168370512,
0.0176009700440517),.UNSPECIFIED.)
GEOMETRIC_REPRESENTATION_ITEM()
RATIONAL_B_SPLINE_SURFACE(((0.99818389211382,0.99657330421516,0.996380621259469),
(0.99818389211382,0.99657330421516,0.996380621259469),(0.99818389211382,
0.99657330421516,0.996380621259469),(0.99818389211382,0.99657330421516,
0.996380621259469)))
REPRESENTATION_ITEM('')
SURFACE()
);
#134=(
BOUNDED_SURFACE()
B_SPLINE_SURFACE(1,2,((#67354,#67355,#67356),(#67357,#67358,#67359)),
 .UNSPECIFIED.,.F.,.F.,.F.)
B_SPLINE_SURFACE_WITH_KNOTS((2,2),(3,3),(0.,1.),(0.0556006976418415,0.0675888856590488),
 .UNSPECIFIED.)
GEOMETRIC_REPRESENTATION_ITEM()
RATIONAL_B_SPLINE_SURFACE(((0.996397562408606,0.996150386832629,0.997319912843745),
(0.996397562408606,0.996150386832629,0.997319912843745)))
REPRESENTATION_ITEM('')
SURFACE()
);
#135=(
BOUNDED_SURFACE()
B_SPLINE_SURFACE(1,2,((#67428,#67429,#67430),(#67431,#67432,#67433),(#67434,
#67435,#67436)),.UNSPECIFIED.,.F.,.F.,.F.)
B_SPLINE_SURFACE_WITH_KNOTS((2,1,2),(3,3),(0.,1.,1.01),(0.0456081671210055,
0.0575989447818817),.UNSPECIFIED.)
GEOMETRIC_REPRESENTATION_ITEM()
RATIONAL_B_SPLINE_SURFACE(((0.997793907739636,0.996365558499688,0.996354522974128),
(0.997793907739636,0.996365558499688,0.996354522974128),(0.997793907739636,
0.996365558499688,0.996354522974128)))
REPRESENTATION_ITEM('')
SURFACE()
);
#136=(
BOUNDED_SURFACE()
B_SPLINE_SURFACE(1,2,((#67471,#67472,#67473),(#67474,#67475,#67476),(#67477,
#67478,#67479)),.UNSPECIFIED.,.F.,.F.,.F.)
B_SPLINE_SURFACE_WITH_KNOTS((2,1,2),(3,3),(-0.00286810173546857,0.,0.477902879806836),
(0.0466073985929116,0.0531834929157973),.UNSPECIFIED.)
GEOMETRIC_REPRESENTATION_ITEM()
RATIONAL_B_SPLINE_SURFACE(((0.997565691989291,0.996847118055594,0.996554836292953),
(0.997565691989291,0.996847118055594,0.996554836292953),(0.997565691989291,
0.996847118055594,0.996554836292953)))
REPRESENTATION_ITEM('')
SURFACE()
);
#137=(
BOUNDED_SURFACE()
B_SPLINE_SURFACE(1,2,((#67496,#67497,#67498,#67499,#67500),(#67501,#67502,
#67503,#67504,#67505),(#67506,#67507,#67508,#67509,#67510)),
 .UNSPECIFIED.,.F.,.F.,.F.)
B_SPLINE_SURFACE_WITH_KNOTS((2,1,2),(3,2,3),(0.,1.,1.01),(0.0355931932713903,
0.0384615384615384,0.0476086899858126),.UNSPECIFIED.)
GEOMETRIC_REPRESENTATION_ITEM()
RATIONAL_B_SPLINE_SURFACE(((0.998993602249807,0.999456249886298,1.,0.998265981131401,
0.997356751596327),(0.998993602249807,0.999456249886298,1.,0.998265981131401,
0.997356751596327),(0.998993602249807,0.999456249886298,1.,0.998265981131401,
0.997356751596327)))
REPRESENTATION_ITEM('')
SURFACE()
);
#138=(
BOUNDED_SURFACE()
B_SPLINE_SURFACE(1,2,((#67558,#67559,#67560,#67561,#67562),(#67563,#67564,
#67565,#67566,#67567),(#67568,#67569,#67570,#67571,#67572)),
 .UNSPECIFIED.,.F.,.F.,.F.)
B_SPLINE_SURFACE_WITH_KNOTS((2,1,2),(3,2,3),(-0.00141401191198394,0.,0.480770297101345),
(0.0365944846645757,0.0384615384615384,0.0431859280915184),
 .UNSPECIFIED.)
GEOMETRIC_REPRESENTATION_ITEM()
RATIONAL_B_SPLINE_SURFACE(((0.999326490452258,0.999646063968217,1.,0.999104400890347,
0.9984288220563),(0.999326490452258,0.999646063968217,1.,0.999104400890347,
0.9984288220563),(0.999326490452258,0.999646063968217,1.,0.999104400890347,
0.9984288220563)))
REPRESENTATION_ITEM('')
SURFACE()
);
#139=(
BOUNDED_SURFACE()
B_SPLINE_SURFACE(1,2,((#67588,#67589,#67590),(#67591,#67592,#67593),(#67594,
#67595,#67596)),.UNSPECIFIED.,.F.,.F.,.F.)
B_SPLINE_SURFACE_WITH_KNOTS((2,1,2),(3,3),(0.,1.,1.01),(0.0255903596131788,
0.0375948596693866),.UNSPECIFIED.)
GEOMETRIC_REPRESENTATION_ITEM()
RATIONAL_B_SPLINE_SURFACE(((0.996753121755999,0.997505687613147,0.999678813023853),
(0.996753121755999,0.997505687613147,0.999678813023853),(0.996753121755999,
0.997505687613147,0.999678813023853)))
REPRESENTATION_ITEM('')
SURFACE()
);
#140=(
BOUNDED_SURFACE()
B_SPLINE_SURFACE(1,2,((#67608,#67609,#67610),(#67611,#67612,#67613),(#67614,
#67615,#67616)),.UNSPECIFIED.,.F.,.F.,.F.)
B_SPLINE_SURFACE_WITH_KNOTS((2,1,2),(3,3),(-0.00286823356237821,0.,0.477902879808255),
(0.0265907346180626,0.0331702037252925),.UNSPECIFIED.)
GEOMETRIC_REPRESENTATION_ITEM()
RATIONAL_B_SPLINE_SURFACE(((0.996888414395785,0.997365765479939,0.998269846384986),
(0.996888414395785,0.997365765479939,0.998269846384986),(0.996888414395785,
0.997365765479939,0.998269846384986)))
REPRESENTATION_ITEM('')
SURFACE()
);
#141=(
BOUNDED_SURFACE()
B_SPLINE_SURFACE(1,2,((#67717,#67718,#67719),(#67720,#67721,#67722),(#67723,
#67724,#67725)),.UNSPECIFIED.,.F.,.F.,.F.)
B_SPLINE_SURFACE_WITH_KNOTS((2,1,2),(3,3),(-0.00286753128227487,0.,0.477902879809176),
(0.0166015299238962,0.0231736788111887),.UNSPECIFIED.)
GEOMETRIC_REPRESENTATION_ITEM()
RATIONAL_B_SPLINE_SURFACE(((0.996422581660833,0.996252244737342,0.996507688616405),
(0.996422581660833,0.996252244737342,0.996507688616404),(0.996422581660833,
0.996252244737342,0.996507688616404)))
REPRESENTATION_ITEM('')
SURFACE()
);
#142=(
BOUNDED_SURFACE()
B_SPLINE_SURFACE(1,2,((#67742,#67743,#67744),(#67745,#67746,#67747),(#67748,
#67749,#67750)),.UNSPECIFIED.,.F.,.F.,.F.)
B_SPLINE_SURFACE_WITH_KNOTS((2,1,2),(3,3),(-0.01,0.,1.),(0.00560769168370637,
0.0176009700440516),.UNSPECIFIED.)
GEOMETRIC_REPRESENTATION_ITEM()
RATIONAL_B_SPLINE_SURFACE(((0.99818389211382,0.99657330421516,0.996380621259469),
(0.99818389211382,0.99657330421516,0.996380621259469),(0.99818389211382,
0.99657330421516,0.996380621259469)))
REPRESENTATION_ITEM('')
SURFACE()
);
#143=(
BOUNDED_SURFACE()
B_SPLINE_SURFACE(1,2,((#67785,#67786,#67787),(#67788,#67789,#67790),(#67791,
#67792,#67793)),.UNSPECIFIED.,.F.,.F.,.F.)
B_SPLINE_SURFACE_WITH_KNOTS((2,1,2),(3,3),(-0.00206901892693671,0.,0.346769728509108),
(0.0066071315471312,0.0131849431468896),.UNSPECIFIED.)
GEOMETRIC_REPRESENTATION_ITEM()
RATIONAL_B_SPLINE_SURFACE(((0.997925307359465,0.997106772384946,0.996714752253861),
(0.997925307359465,0.997106772384946,0.996714752253861),(0.997925307359465,
0.997106772384946,0.996714752253861)))
REPRESENTATION_ITEM('')
SURFACE()
);
#144=(
BOUNDED_SURFACE()
B_SPLINE_SURFACE(1,2,((#67866,#67867,#67868),(#67869,#67870,#67871)),
 .UNSPECIFIED.,.F.,.F.,.F.)
B_SPLINE_SURFACE_WITH_KNOTS((2,2),(3,3),(0.,1.),(0.0556006976418457,0.0675888856590507),
 .UNSPECIFIED.)
GEOMETRIC_REPRESENTATION_ITEM()
RATIONAL_B_SPLINE_SURFACE(((0.996397562408606,0.996150386832629,0.997319912843745),
(0.996397562408606,0.996150386832629,0.997319912843745)))
REPRESENTATION_ITEM('')
SURFACE()
);
#145=(
BOUNDED_SURFACE()
B_SPLINE_SURFACE(1,2,((#67940,#67941,#67942),(#67943,#67944,#67945),(#67946,
#67947,#67948)),.UNSPECIFIED.,.F.,.F.,.F.)
B_SPLINE_SURFACE_WITH_KNOTS((2,1,2),(3,3),(0.,1.,1.01),(0.0456081671210043,
0.0575989447818814),.UNSPECIFIED.)
GEOMETRIC_REPRESENTATION_ITEM()
RATIONAL_B_SPLINE_SURFACE(((0.997793907739636,0.996365558499688,0.996354522974128),
(0.997793907739636,0.996365558499688,0.996354522974128),(0.997793907739636,
0.996365558499688,0.996354522974128)))
REPRESENTATION_ITEM('')
SURFACE()
);
#146=(
BOUNDED_SURFACE()
B_SPLINE_SURFACE(1,2,((#67983,#67984,#67985),(#67986,#67987,#67988),(#67989,
#67990,#67991)),.UNSPECIFIED.,.F.,.F.,.F.)
B_SPLINE_SURFACE_WITH_KNOTS((2,1,2),(3,3),(-0.00286810173237255,0.,0.477902879804808),
(0.0466073985929115,0.0531834929157976),.UNSPECIFIED.)
GEOMETRIC_REPRESENTATION_ITEM()
RATIONAL_B_SPLINE_SURFACE(((0.997565691989291,0.996847118055593,0.996554836292953),
(0.997565691989291,0.996847118055593,0.996554836292953),(0.997565691989291,
0.996847118055593,0.996554836292953)))
REPRESENTATION_ITEM('')
SURFACE()
);
#147=(
BOUNDED_SURFACE()
B_SPLINE_SURFACE(1,2,((#68008,#68009,#68010,#68011,#68012),(#68013,#68014,
#68015,#68016,#68017),(#68018,#68019,#68020,#68021,#68022)),
 .UNSPECIFIED.,.F.,.F.,.F.)
B_SPLINE_SURFACE_WITH_KNOTS((2,1,2),(3,2,3),(0.,1.,1.01),(0.0355931932713902,
0.0384615384615384,0.0476086899858139),.UNSPECIFIED.)
GEOMETRIC_REPRESENTATION_ITEM()
RATIONAL_B_SPLINE_SURFACE(((0.998993602249807,0.999456249886298,1.,0.998265981131401,
0.997356751596327),(0.998993602249807,0.999456249886298,1.,0.998265981131401,
0.997356751596327),(0.998993602249807,0.999456249886298,1.,0.998265981131401,
0.997356751596327)))
REPRESENTATION_ITEM('')
SURFACE()
);
#148=(
BOUNDED_SURFACE()
B_SPLINE_SURFACE(1,2,((#68070,#68071,#68072,#68073,#68074),(#68075,#68076,
#68077,#68078,#68079),(#68080,#68081,#68082,#68083,#68084)),
 .UNSPECIFIED.,.F.,.F.,.F.)
B_SPLINE_SURFACE_WITH_KNOTS((2,1,2),(3,2,3),(-0.00141401191198009,0.,0.480770297099536),
(0.0365944846645796,0.0384615384615384,0.0431859280915184),
 .UNSPECIFIED.)
GEOMETRIC_REPRESENTATION_ITEM()
RATIONAL_B_SPLINE_SURFACE(((0.99932649045226,0.999646063968218,1.,0.999104400890347,
0.9984288220563),(0.99932649045226,0.999646063968218,1.,0.999104400890347,
0.9984288220563),(0.99932649045226,0.999646063968218,1.,0.999104400890347,
0.9984288220563)))
REPRESENTATION_ITEM('')
SURFACE()
);
#149=(
BOUNDED_SURFACE()
B_SPLINE_SURFACE(1,2,((#68111,#68112,#68113),(#68114,#68115,#68116),(#68117,
#68118,#68119)),.UNSPECIFIED.,.F.,.F.,.F.)
B_SPLINE_SURFACE_WITH_KNOTS((2,1,2),(3,3),(0.,1.,1.01),(0.025590359613181,
0.0375948596693874),.UNSPECIFIED.)
GEOMETRIC_REPRESENTATION_ITEM()
RATIONAL_B_SPLINE_SURFACE(((0.996753121755999,0.997505687613148,0.999678813023853),
(0.996753121755999,0.997505687613148,0.999678813023853),(0.996753121755999,
0.997505687613148,0.999678813023853)))
REPRESENTATION_ITEM('')
SURFACE()
);
#150=(
BOUNDED_SURFACE()
B_SPLINE_SURFACE(1,2,((#68154,#68155,#68156),(#68157,#68158,#68159),(#68160,
#68161,#68162)),.UNSPECIFIED.,.F.,.F.,.F.)
B_SPLINE_SURFACE_WITH_KNOTS((2,1,2),(3,3),(-0.00286823045912087,0.,0.477902879806536),
(0.0265907346180616,0.0331702036774538),.UNSPECIFIED.)
GEOMETRIC_REPRESENTATION_ITEM()
RATIONAL_B_SPLINE_SURFACE(((0.996888414395785,0.997365765476469,0.998269846371838),
(0.996888414395785,0.997365765476469,0.998269846371838),(0.996888414395785,
0.997365765476469,0.998269846371838)))
REPRESENTATION_ITEM('')
SURFACE()
);
#151=(
BOUNDED_SURFACE()
B_SPLINE_SURFACE(1,2,((#68200,#68201,#68202),(#68203,#68204,#68205),(#68206,
#68207,#68208)),.UNSPECIFIED.,.F.,.F.,.F.)
B_SPLINE_SURFACE_WITH_KNOTS((2,1,2),(3,3),(-0.00286753128222655,0.,0.477902879807592),
(0.0166015299238958,0.0231736788111887),.UNSPECIFIED.)
GEOMETRIC_REPRESENTATION_ITEM()
RATIONAL_B_SPLINE_SURFACE(((0.996422581660833,0.996252244737342,0.996507688616404),
(0.996422581660833,0.996252244737342,0.996507688616404),(0.996422581660833,
0.996252244737342,0.996507688616404)))
REPRESENTATION_ITEM('')
SURFACE()
);
#152=(
BOUNDED_SURFACE()
B_SPLINE_SURFACE(1,2,((#68254,#68255,#68256),(#68257,#68258,#68259),(#68260,
#68261,#68262)),.UNSPECIFIED.,.F.,.F.,.F.)
B_SPLINE_SURFACE_WITH_KNOTS((2,1,2),(3,3),(0.,1.,1.01),(0.00560769170937608,
0.0176009697616828),.UNSPECIFIED.)
GEOMETRIC_REPRESENTATION_ITEM()
RATIONAL_B_SPLINE_SURFACE(((0.998183892106926,0.996573304252667,0.996380621268542),
(0.998183892106926,0.996573304252667,0.996380621268542),(0.998183892106926,
0.996573304252667,0.996380621268542)))
REPRESENTATION_ITEM('')
SURFACE()
);
#153=(
BOUNDED_SURFACE()
B_SPLINE_SURFACE(1,2,((#68297,#68298,#68299),(#68300,#68301,#68302),(#68303,
#68304,#68305)),.UNSPECIFIED.,.F.,.F.,.F.)
B_SPLINE_SURFACE_WITH_KNOTS((2,1,2),(3,3),(-0.00206901892698856,0.,0.346769728507897),
(0.00660713154714496,0.0131849431468368),.UNSPECIFIED.)
GEOMETRIC_REPRESENTATION_ITEM()
RATIONAL_B_SPLINE_SURFACE(((0.997925307359461,0.997106772384952,0.996714752253867),
(0.997925307359461,0.997106772384952,0.996714752253867),(0.997925307359461,
0.997106772384952,0.996714752253867)))
REPRESENTATION_ITEM('')
SURFACE()
);
#154=(
BOUNDED_SURFACE()
B_SPLINE_SURFACE(1,2,((#68378,#68379,#68380),(#68381,#68382,#68383)),
 .UNSPECIFIED.,.F.,.F.,.F.)
B_SPLINE_SURFACE_WITH_KNOTS((2,2),(3,3),(0.,1.),(0.0556006976418394,0.0675888856590502),
 .UNSPECIFIED.)
GEOMETRIC_REPRESENTATION_ITEM()
RATIONAL_B_SPLINE_SURFACE(((0.996397562408606,0.996150386832629,0.997319912843745),
(0.996397562408606,0.996150386832629,0.997319912843745)))
REPRESENTATION_ITEM('')
SURFACE()
);
#155=(
BOUNDED_SURFACE()
B_SPLINE_SURFACE(1,2,((#68452,#68453,#68454),(#68455,#68456,#68457),(#68458,
#68459,#68460)),.UNSPECIFIED.,.F.,.F.,.F.)
B_SPLINE_SURFACE_WITH_KNOTS((2,1,2),(3,3),(0.,1.,1.01),(0.0456081671210063,
0.0575989447818833),.UNSPECIFIED.)
GEOMETRIC_REPRESENTATION_ITEM()
RATIONAL_B_SPLINE_SURFACE(((0.997793907739636,0.996365558499688,0.996354522974128),
(0.997793907739636,0.996365558499688,0.996354522974128),(0.997793907739636,
0.996365558499688,0.996354522974128)))
REPRESENTATION_ITEM('')
SURFACE()
);
#156=(
BOUNDED_SURFACE()
B_SPLINE_SURFACE(1,2,((#68495,#68496,#68497),(#68498,#68499,#68500),(#68501,
#68502,#68503)),.UNSPECIFIED.,.F.,.F.,.F.)
B_SPLINE_SURFACE_WITH_KNOTS((2,1,2),(3,3),(-0.00286810173241533,0.,0.477902879802667),
(0.0466073985929121,0.053183492915798),.UNSPECIFIED.)
GEOMETRIC_REPRESENTATION_ITEM()
RATIONAL_B_SPLINE_SURFACE(((0.997565691989291,0.996847118055593,0.996554836292953),
(0.997565691989291,0.996847118055593,0.996554836292953),(0.997565691989291,
0.996847118055593,0.996554836292953)))
REPRESENTATION_ITEM('')
SURFACE()
);
#157=(
BOUNDED_SURFACE()
B_SPLINE_SURFACE(1,2,((#68520,#68521,#68522,#68523,#68524),(#68525,#68526,
#68527,#68528,#68529),(#68530,#68531,#68532,#68533,#68534)),
 .UNSPECIFIED.,.F.,.F.,.F.)
B_SPLINE_SURFACE_WITH_KNOTS((2,1,2),(3,2,3),(0.,1.,1.01),(0.0355931932713904,
0.0384615384615384,0.0476086899858132),.UNSPECIFIED.)
GEOMETRIC_REPRESENTATION_ITEM()
RATIONAL_B_SPLINE_SURFACE(((0.998993602249807,0.999456249886298,1.,0.998265981131401,
0.997356751596327),(0.998993602249807,0.999456249886298,1.,0.998265981131401,
0.997356751596327),(0.998993602249807,0.999456249886298,1.,0.998265981131401,
0.997356751596327)))
REPRESENTATION_ITEM('')
SURFACE()
);
#158=(
BOUNDED_SURFACE()
B_SPLINE_SURFACE(1,2,((#68582,#68583,#68584,#68585,#68586),(#68587,#68588,
#68589,#68590,#68591),(#68592,#68593,#68594,#68595,#68596)),
 .UNSPECIFIED.,.F.,.F.,.F.)
B_SPLINE_SURFACE_WITH_KNOTS((2,1,2),(3,2,3),(-0.00141401191198431,0.,0.480770297097393),
(0.0365944846645793,0.0384615384615384,0.043185928091518),.UNSPECIFIED.)
GEOMETRIC_REPRESENTATION_ITEM()
RATIONAL_B_SPLINE_SURFACE(((0.99932649045226,0.999646063968218,1.,0.999104400890347,
0.9984288220563),(0.99932649045226,0.999646063968218,1.,0.999104400890347,
0.9984288220563),(0.99932649045226,0.999646063968218,1.,0.999104400890347,
0.9984288220563)))
REPRESENTATION_ITEM('')
SURFACE()
);
#159=(
BOUNDED_SURFACE()
B_SPLINE_SURFACE(1,2,((#68623,#68624,#68625),(#68626,#68627,#68628),(#68629,
#68630,#68631)),.UNSPECIFIED.,.F.,.F.,.F.)
B_SPLINE_SURFACE_WITH_KNOTS((2,1,2),(3,3),(0.,1.,1.01),(0.0255903596131799,
0.0375948596693881),.UNSPECIFIED.)
GEOMETRIC_REPRESENTATION_ITEM()
RATIONAL_B_SPLINE_SURFACE(((0.996753121755999,0.997505687613148,0.999678813023854),
(0.996753121755999,0.997505687613148,0.999678813023854),(0.996753121755999,
0.997505687613148,0.999678813023854)))
REPRESENTATION_ITEM('')
SURFACE()
);
#160=(
BOUNDED_SURFACE()
B_SPLINE_SURFACE(1,2,((#68666,#68667,#68668),(#68669,#68670,#68671),(#68672,
#68673,#68674)),.UNSPECIFIED.,.F.,.F.,.F.)
B_SPLINE_SURFACE_WITH_KNOTS((2,1,2),(3,3),(-0.00286823356251491,0.,0.477902879804656),
(0.0265907346180619,0.0331702037252935),.UNSPECIFIED.)
GEOMETRIC_REPRESENTATION_ITEM()
RATIONAL_B_SPLINE_SURFACE(((0.996888414395785,0.997365765479939,0.998269846384986),
(0.996888414395785,0.997365765479939,0.998269846384986),(0.996888414395785,
0.997365765479939,0.998269846384986)))
REPRESENTATION_ITEM('')
SURFACE()
);
#161=(
BOUNDED_SURFACE()
B_SPLINE_SURFACE(1,2,((#68741,#68742,#68743),(#68744,#68745,#68746),(#68747,
#68748,#68749)),.UNSPECIFIED.,.F.,.F.,.F.)
B_SPLINE_SURFACE_WITH_KNOTS((2,1,2),(3,3),(-0.00286753128226436,0.,0.477902879805871),
(0.0166015299238958,0.0231736788111887),.UNSPECIFIED.)
GEOMETRIC_REPRESENTATION_ITEM()
RATIONAL_B_SPLINE_SURFACE(((0.996422581660833,0.996252244737342,0.996507688616404),
(0.996422581660833,0.996252244737342,0.996507688616404),(0.996422581660833,
0.996252244737342,0.996507688616404)))
REPRESENTATION_ITEM('')
SURFACE()
);
#162=(
BOUNDED_SURFACE()
B_SPLINE_SURFACE(1,2,((#68760,#68761,#68762),(#68763,#68764,#68765),(#68766,
#68767,#68768),(#68769,#68770,#68771)),.UNSPECIFIED.,.F.,.F.,.F.)
B_SPLINE_SURFACE_WITH_KNOTS((2,1,1,2),(3,3),(-0.0101,0.,1.,1.01),(0.00560769168370509,
0.0176009700440523),.UNSPECIFIED.)
GEOMETRIC_REPRESENTATION_ITEM()
RATIONAL_B_SPLINE_SURFACE(((0.998183892113821,0.99657330421516,0.996380621259469),
(0.998183892113821,0.99657330421516,0.996380621259469),(0.998183892113821,
0.99657330421516,0.996380621259469),(0.998183892113821,0.99657330421516,
0.996380621259469)))
REPRESENTATION_ITEM('')
SURFACE()
);
#163=(
BOUNDED_SURFACE()
B_SPLINE_SURFACE(1,2,((#68783,#68784,#68785),(#68786,#68787,#68788),(#68789,
#68790,#68791)),.UNSPECIFIED.,.F.,.F.,.F.)
B_SPLINE_SURFACE_WITH_KNOTS((2,1,2),(3,3),(-0.00206901892703507,0.,0.346769728506472),
(0.00660713154710819,0.0131849431468896),.UNSPECIFIED.)
GEOMETRIC_REPRESENTATION_ITEM()
RATIONAL_B_SPLINE_SURFACE(((0.997925307359471,0.997106772384947,0.99671475225386),
(0.997925307359471,0.997106772384947,0.99671475225386),(0.997925307359471,
0.997106772384947,0.99671475225386)))
REPRESENTATION_ITEM('')
SURFACE()
);
#164=(
BOUNDED_SURFACE()
B_SPLINE_SURFACE(1,2,((#68893,#68894,#68895),(#68896,#68897,#68898)),
 .UNSPECIFIED.,.F.,.F.,.F.)
B_SPLINE_SURFACE_WITH_KNOTS((2,2),(3,3),(0.,1.),(0.0556006976418427,0.0675888856590493),
 .UNSPECIFIED.)
GEOMETRIC_REPRESENTATION_ITEM()
RATIONAL_B_SPLINE_SURFACE(((0.996397562408606,0.996150386832629,0.997319912843745),
(0.996397562408606,0.996150386832629,0.997319912843745)))
REPRESENTATION_ITEM('')
SURFACE()
);
#165=(
BOUNDED_SURFACE()
B_SPLINE_SURFACE(1,2,((#68967,#68968,#68969),(#68970,#68971,#68972),(#68973,
#68974,#68975)),.UNSPECIFIED.,.F.,.F.,.F.)
B_SPLINE_SURFACE_WITH_KNOTS((2,1,2),(3,3),(0.,1.,1.01),(0.0456081671210056,
0.0575989447818805),.UNSPECIFIED.)
GEOMETRIC_REPRESENTATION_ITEM()
RATIONAL_B_SPLINE_SURFACE(((0.997793907739636,0.996365558499688,0.996354522974128),
(0.997793907739636,0.996365558499688,0.996354522974128),(0.997793907739636,
0.996365558499688,0.996354522974128)))
REPRESENTATION_ITEM('')
SURFACE()
);
#166=(
BOUNDED_SURFACE()
B_SPLINE_SURFACE(1,2,((#69010,#69011,#69012),(#69013,#69014,#69015),(#69016,
#69017,#69018)),.UNSPECIFIED.,.F.,.F.,.F.)
B_SPLINE_SURFACE_WITH_KNOTS((2,1,2),(3,3),(-0.00286810173213876,0.,0.477902879800509),
(0.0466073985929119,0.0531834929157981),.UNSPECIFIED.)
GEOMETRIC_REPRESENTATION_ITEM()
RATIONAL_B_SPLINE_SURFACE(((0.997565691989292,0.996847118055594,0.996554836292953),
(0.997565691989292,0.996847118055594,0.996554836292953),(0.997565691989292,
0.996847118055594,0.996554836292953)))
REPRESENTATION_ITEM('')
SURFACE()
);
#167=(
BOUNDED_SURFACE()
B_SPLINE_SURFACE(1,2,((#69035,#69036,#69037,#69038,#69039),(#69040,#69041,
#69042,#69043,#69044),(#69045,#69046,#69047,#69048,#69049)),
 .UNSPECIFIED.,.F.,.F.,.F.)
B_SPLINE_SURFACE_WITH_KNOTS((2,1,2),(3,2,3),(0.,1.,1.01),(0.0355931932713901,
0.0384615384615384,0.0476086899858143),.UNSPECIFIED.)
GEOMETRIC_REPRESENTATION_ITEM()
RATIONAL_B_SPLINE_SURFACE(((0.998993602249807,0.999456249886298,1.,0.998265981131401,
0.997356751596327),(0.998993602249807,0.999456249886298,1.,0.998265981131401,
0.997356751596327),(0.998993602249807,0.999456249886298,1.,0.998265981131401,
0.997356751596327)))
REPRESENTATION_ITEM('')
SURFACE()
);
#168=(
BOUNDED_SURFACE()
B_SPLINE_SURFACE(1,2,((#69097,#69098,#69099,#69100,#69101),(#69102,#69103,
#69104,#69105,#69106),(#69107,#69108,#69109,#69110,#69111)),
 .UNSPECIFIED.,.F.,.F.,.F.)
B_SPLINE_SURFACE_WITH_KNOTS((2,1,2),(3,2,3),(-0.00141401191198412,0.,0.480770297095169),
(0.0365944846645757,0.0384615384615384,0.0431859280915181),
 .UNSPECIFIED.)
GEOMETRIC_REPRESENTATION_ITEM()
RATIONAL_B_SPLINE_SURFACE(((0.999326490452259,0.999646063968217,1.,0.999104400890347,
0.9984288220563),(0.999326490452259,0.999646063968217,1.,0.999104400890347,
0.9984288220563),(0.999326490452259,0.999646063968217,1.,0.999104400890347,
0.9984288220563)))
REPRESENTATION_ITEM('')
SURFACE()
);
#169=(
BOUNDED_SURFACE()
B_SPLINE_SURFACE(1,2,((#69138,#69139,#69140),(#69141,#69142,#69143),(#69144,
#69145,#69146)),.UNSPECIFIED.,.F.,.F.,.F.)
B_SPLINE_SURFACE_WITH_KNOTS((2,1,2),(3,3),(0.,1.,1.01),(0.0255903596131801,
0.0375948596693865),.UNSPECIFIED.)
GEOMETRIC_REPRESENTATION_ITEM()
RATIONAL_B_SPLINE_SURFACE(((0.996753121755999,0.997505687613148,0.999678813023853),
(0.996753121755999,0.997505687613148,0.999678813023853),(0.996753121755999,
0.997505687613148,0.999678813023853)))
REPRESENTATION_ITEM('')
SURFACE()
);
#170=(
BOUNDED_SURFACE()
B_SPLINE_SURFACE(1,2,((#69181,#69182,#69183),(#69184,#69185,#69186),(#69187,
#69188,#69189)),.UNSPECIFIED.,.F.,.F.,.F.)
B_SPLINE_SURFACE_WITH_KNOTS((2,1,2),(3,3),(-0.00286823356233756,0.,0.477902879802539),
(0.0265907346180619,0.0331702037252928),.UNSPECIFIED.)
GEOMETRIC_REPRESENTATION_ITEM()
RATIONAL_B_SPLINE_SURFACE(((0.996888414395785,0.997365765479939,0.998269846384985),
(0.996888414395785,0.997365765479939,0.998269846384985),(0.996888414395785,
0.997365765479939,0.998269846384985)))
REPRESENTATION_ITEM('')
SURFACE()
);
#171=(
BOUNDED_SURFACE()
B_SPLINE_SURFACE(1,2,((#69256,#69257,#69258),(#69259,#69260,#69261),(#69262,
#69263,#69264)),.UNSPECIFIED.,.F.,.F.,.F.)
B_SPLINE_SURFACE_WITH_KNOTS((2,1,2),(3,3),(-0.0028675312823971,0.,0.47790287980379),
(0.016601529923896,0.0231736788111898),.UNSPECIFIED.)
GEOMETRIC_REPRESENTATION_ITEM()
RATIONAL_B_SPLINE_SURFACE(((0.996422581660833,0.996252244737342,0.996507688616404),
(0.996422581660833,0.996252244737342,0.996507688616404),(0.996422581660833,
0.996252244737342,0.996507688616404)))
REPRESENTATION_ITEM('')
SURFACE()
);
#172=(
BOUNDED_SURFACE()
B_SPLINE_SURFACE(1,2,((#69281,#69282,#69283),(#69284,#69285,#69286),(#69287,
#69288,#69289),(#69290,#69291,#69292)),.UNSPECIFIED.,.F.,.F.,.F.)
B_SPLINE_SURFACE_WITH_KNOTS((2,1,1,2),(3,3),(-0.0101,0.,1.,1.01),(0.00560769168370544,
0.0176009700440511),.UNSPECIFIED.)
GEOMETRIC_REPRESENTATION_ITEM()
RATIONAL_B_SPLINE_SURFACE(((0.99818389211382,0.99657330421516,0.996380621259469),
(0.99818389211382,0.99657330421516,0.996380621259469),(0.99818389211382,
0.99657330421516,0.996380621259469),(0.99818389211382,0.99657330421516,
0.996380621259469)))
REPRESENTATION_ITEM('')
SURFACE()
);
#173=(
BOUNDED_SURFACE()
B_SPLINE_SURFACE(1,2,((#69327,#69328,#69329),(#69330,#69331,#69332),(#69333,
#69334,#69335)),.UNSPECIFIED.,.F.,.F.,.F.)
B_SPLINE_SURFACE_WITH_KNOTS((2,1,2),(3,3),(-0.00206901892705003,0.,0.346769728504996),
(0.0066071315471665,0.0131849431468897),.UNSPECIFIED.)
GEOMETRIC_REPRESENTATION_ITEM()
RATIONAL_B_SPLINE_SURFACE(((0.997925307359456,0.997106772384944,0.99671475225386),
(0.997925307359456,0.997106772384944,0.99671475225386),(0.997925307359456,
0.997106772384944,0.99671475225386)))
REPRESENTATION_ITEM('')
SURFACE()
);
#174=(
BOUNDED_SURFACE()
B_SPLINE_SURFACE(1,2,((#69408,#69409,#69410),(#69411,#69412,#69413)),
 .UNSPECIFIED.,.F.,.F.,.F.)
B_SPLINE_SURFACE_WITH_KNOTS((2,2),(3,3),(0.,1.),(0.0556006976418448,0.0675888856590502),
 .UNSPECIFIED.)
GEOMETRIC_REPRESENTATION_ITEM()
RATIONAL_B_SPLINE_SURFACE(((0.996397562408606,0.996150386832629,0.997319912843745),
(0.996397562408606,0.996150386832629,0.997319912843745)))
REPRESENTATION_ITEM('')
SURFACE()
);
#175=(
BOUNDED_SURFACE()
B_SPLINE_SURFACE(1,2,((#69482,#69483,#69484),(#69485,#69486,#69487),(#69488,
#69489,#69490)),.UNSPECIFIED.,.F.,.F.,.F.)
B_SPLINE_SURFACE_WITH_KNOTS((2,1,2),(3,3),(0.,1.,1.01),(0.0456081671210065,
0.0575989447818822),.UNSPECIFIED.)
GEOMETRIC_REPRESENTATION_ITEM()
RATIONAL_B_SPLINE_SURFACE(((0.997793907739636,0.996365558499688,0.996354522974128),
(0.997793907739636,0.996365558499688,0.996354522974128),(0.997793907739636,
0.996365558499688,0.996354522974128)))
REPRESENTATION_ITEM('')
SURFACE()
);
#176=(
BOUNDED_SURFACE()
B_SPLINE_SURFACE(1,2,((#69525,#69526,#69527),(#69528,#69529,#69530),(#69531,
#69532,#69533)),.UNSPECIFIED.,.F.,.F.,.F.)
B_SPLINE_SURFACE_WITH_KNOTS((2,1,2),(3,3),(-0.0028681017353746,0.,0.477902879797914),
(0.0466073985929116,0.0531834929157982),.UNSPECIFIED.)
GEOMETRIC_REPRESENTATION_ITEM()
RATIONAL_B_SPLINE_SURFACE(((0.997565691989291,0.996847118055594,0.996554836292953),
(0.997565691989291,0.996847118055594,0.996554836292953),(0.997565691989291,
0.996847118055594,0.996554836292953)))
REPRESENTATION_ITEM('')
SURFACE()
);
#177=(
BOUNDED_SURFACE()
B_SPLINE_SURFACE(1,2,((#69550,#69551,#69552,#69553,#69554),(#69555,#69556,
#69557,#69558,#69559),(#69560,#69561,#69562,#69563,#69564)),
 .UNSPECIFIED.,.F.,.F.,.F.)
B_SPLINE_SURFACE_WITH_KNOTS((2,1,2),(3,2,3),(0.,1.,1.01),(0.0355931932713903,
0.0384615384615384,0.0476086899858138),.UNSPECIFIED.)
GEOMETRIC_REPRESENTATION_ITEM()
RATIONAL_B_SPLINE_SURFACE(((0.998993602249807,0.999456249886298,1.,0.998265981131401,
0.997356751596327),(0.998993602249807,0.999456249886298,1.,0.998265981131401,
0.997356751596327),(0.998993602249807,0.999456249886298,1.,0.998265981131401,
0.997356751596327)))
REPRESENTATION_ITEM('')
SURFACE()
);
#178=(
BOUNDED_SURFACE()
B_SPLINE_SURFACE(1,2,((#69612,#69613,#69614,#69615,#69616),(#69617,#69618,
#69619,#69620,#69621),(#69622,#69623,#69624,#69625,#69626)),
 .UNSPECIFIED.,.F.,.F.,.F.)
B_SPLINE_SURFACE_WITH_KNOTS((2,1,2),(3,2,3),(-0.0014140119119741,0.,0.480770297092789),
(0.0365944846645798,0.0384615384615384,0.0431859280915187),
 .UNSPECIFIED.)
GEOMETRIC_REPRESENTATION_ITEM()
RATIONAL_B_SPLINE_SURFACE(((0.99932649045226,0.999646063968218,1.,0.999104400890347,
0.9984288220563),(0.99932649045226,0.999646063968218,1.,0.999104400890347,
0.9984288220563),(0.99932649045226,0.999646063968218,1.,0.999104400890347,
0.9984288220563)))
REPRESENTATION_ITEM('')
SURFACE()
);
#179=(
BOUNDED_SURFACE()
B_SPLINE_SURFACE(1,2,((#69653,#69654,#69655),(#69656,#69657,#69658),(#69659,
#69660,#69661)),.UNSPECIFIED.,.F.,.F.,.F.)
B_SPLINE_SURFACE_WITH_KNOTS((2,1,2),(3,3),(0.,1.,1.01),(0.0255903596131829,
0.0375948596693895),.UNSPECIFIED.)
GEOMETRIC_REPRESENTATION_ITEM()
RATIONAL_B_SPLINE_SURFACE(((0.996753121755999,0.997505687613148,0.999678813023854),
(0.996753121755999,0.997505687613148,0.999678813023854),(0.996753121755999,
0.997505687613148,0.999678813023854)))
REPRESENTATION_ITEM('')
SURFACE()
);
#180=(
BOUNDED_SURFACE()
B_SPLINE_SURFACE(1,2,((#69696,#69697,#69698),(#69699,#69700,#69701),(#69702,
#69703,#69704)),.UNSPECIFIED.,.F.,.F.,.F.)
B_SPLINE_SURFACE_WITH_KNOTS((2,1,2),(3,3),(-0.0028682335623885,0.,0.477902879800222),
(0.0265907346180618,0.0331702037252924),.UNSPECIFIED.)
GEOMETRIC_REPRESENTATION_ITEM()
RATIONAL_B_SPLINE_SURFACE(((0.996888414395785,0.997365765479939,0.998269846384985),
(0.996888414395785,0.997365765479939,0.998269846384985),(0.996888414395785,
0.997365765479939,0.998269846384985)))
REPRESENTATION_ITEM('')
SURFACE()
);
#181=(
BOUNDED_SURFACE()
B_SPLINE_SURFACE(1,2,((#69771,#69772,#69773),(#69774,#69775,#69776),(#69777,
#69778,#69779)),.UNSPECIFIED.,.F.,.F.,.F.)
B_SPLINE_SURFACE_WITH_KNOTS((2,1,2),(3,3),(-0.00286753128209166,0.,0.477902879801465),
(0.0166015299238953,0.0231736788111885),.UNSPECIFIED.)
GEOMETRIC_REPRESENTATION_ITEM()
RATIONAL_B_SPLINE_SURFACE(((0.996422581660833,0.996252244737341,0.996507688616404),
(0.996422581660833,0.996252244737341,0.996507688616404),(0.996422581660833,
0.996252244737341,0.996507688616404)))
REPRESENTATION_ITEM('')
SURFACE()
);
#182=(
BOUNDED_SURFACE()
B_SPLINE_SURFACE(1,2,((#69796,#69797,#69798),(#69799,#69800,#69801),(#69802,
#69803,#69804),(#69805,#69806,#69807)),.UNSPECIFIED.,.F.,.F.,.F.)
B_SPLINE_SURFACE_WITH_KNOTS((2,1,1,2),(3,3),(-0.0101,0.,1.,1.01),(0.00560769168370701,
0.0176009700440521),.UNSPECIFIED.)
GEOMETRIC_REPRESENTATION_ITEM()
RATIONAL_B_SPLINE_SURFACE(((0.99818389211382,0.99657330421516,0.996380621259469),
(0.99818389211382,0.99657330421516,0.996380621259469),(0.99818389211382,
0.99657330421516,0.996380621259469),(0.99818389211382,0.99657330421516,
0.996380621259469)))
REPRESENTATION_ITEM('')
SURFACE()
);
#183=(
BOUNDED_SURFACE()
B_SPLINE_SURFACE(1,2,((#69842,#69843,#69844),(#69845,#69846,#69847),(#69848,
#69849,#69850)),.UNSPECIFIED.,.F.,.F.,.F.)
B_SPLINE_SURFACE_WITH_KNOTS((2,1,2),(3,3),(-0.00206901892700914,0.,0.346769728503543),
(0.00660713154717611,0.0131849431468889),.UNSPECIFIED.)
GEOMETRIC_REPRESENTATION_ITEM()
RATIONAL_B_SPLINE_SURFACE(((0.997925307359454,0.997106772384943,0.99671475225386),
(0.997925307359454,0.997106772384943,0.99671475225386),(0.997925307359454,
0.997106772384943,0.99671475225386)))
REPRESENTATION_ITEM('')
SURFACE()
);
#184=(
BOUNDED_SURFACE()
B_SPLINE_SURFACE(1,2,((#69923,#69924,#69925),(#69926,#69927,#69928)),
 .UNSPECIFIED.,.F.,.F.,.F.)
B_SPLINE_SURFACE_WITH_KNOTS((2,2),(3,3),(0.,1.),(0.0556006976418403,0.0675888856590522),
 .UNSPECIFIED.)
GEOMETRIC_REPRESENTATION_ITEM()
RATIONAL_B_SPLINE_SURFACE(((0.996397562408606,0.996150386832629,0.997319912843745),
(0.996397562408606,0.996150386832629,0.997319912843745)))
REPRESENTATION_ITEM('')
SURFACE()
);
#185=(
BOUNDED_SURFACE()
B_SPLINE_SURFACE(1,2,((#69997,#69998,#69999),(#70000,#70001,#70002),(#70003,
#70004,#70005)),.UNSPECIFIED.,.F.,.F.,.F.)
B_SPLINE_SURFACE_WITH_KNOTS((2,1,2),(3,3),(0.,1.,1.01),(0.0456081671210032,
0.0575989447818836),.UNSPECIFIED.)
GEOMETRIC_REPRESENTATION_ITEM()
RATIONAL_B_SPLINE_SURFACE(((0.997793907739636,0.996365558499688,0.996354522974128),
(0.997793907739636,0.996365558499688,0.996354522974128),(0.997793907739636,
0.996365558499688,0.996354522974128)))
REPRESENTATION_ITEM('')
SURFACE()
);
#186=(
BOUNDED_SURFACE()
B_SPLINE_SURFACE(1,2,((#70040,#70041,#70042),(#70043,#70044,#70045),(#70046,
#70047,#70048)),.UNSPECIFIED.,.F.,.F.,.F.)
B_SPLINE_SURFACE_WITH_KNOTS((2,1,2),(3,3),(-0.00286810173537214,0.,0.477902879795336),
(0.0466073985929122,0.0531834929157976),.UNSPECIFIED.)
GEOMETRIC_REPRESENTATION_ITEM()
RATIONAL_B_SPLINE_SURFACE(((0.997565691989291,0.996847118055594,0.996554836292953),
(0.997565691989291,0.996847118055594,0.996554836292953),(0.997565691989291,
0.996847118055594,0.996554836292953)))
REPRESENTATION_ITEM('')
SURFACE()
);
#187=(
BOUNDED_SURFACE()
B_SPLINE_SURFACE(1,2,((#70065,#70066,#70067,#70068,#70069),(#70070,#70071,
#70072,#70073,#70074),(#70075,#70076,#70077,#70078,#70079)),
 .UNSPECIFIED.,.F.,.F.,.F.)
B_SPLINE_SURFACE_WITH_KNOTS((2,1,2),(3,2,3),(0.,1.,1.01),(0.0355931932713903,
0.0384615384615384,0.0476086899858143),.UNSPECIFIED.)
GEOMETRIC_REPRESENTATION_ITEM()
RATIONAL_B_SPLINE_SURFACE(((0.998993602249807,0.999456249886298,1.,0.998265981131401,
0.997356751596327),(0.998993602249807,0.999456249886298,1.,0.998265981131401,
0.997356751596327),(0.998993602249807,0.999456249886298,1.,0.998265981131401,
0.997356751596327)))
REPRESENTATION_ITEM('')
SURFACE()
);
#188=(
BOUNDED_SURFACE()
B_SPLINE_SURFACE(1,2,((#70127,#70128,#70129,#70130,#70131),(#70132,#70133,
#70134,#70135,#70136),(#70137,#70138,#70139,#70140,#70141)),
 .UNSPECIFIED.,.F.,.F.,.F.)
B_SPLINE_SURFACE_WITH_KNOTS((2,1,2),(3,2,3),(-0.00141401191198383,0.,0.480770297090291),
(0.0365944846645756,0.0384615384615384,0.0431859280915189),
 .UNSPECIFIED.)
GEOMETRIC_REPRESENTATION_ITEM()
RATIONAL_B_SPLINE_SURFACE(((0.999326490452258,0.999646063968217,1.,0.999104400890347,
0.9984288220563),(0.999326490452258,0.999646063968217,1.,0.999104400890347,
0.9984288220563),(0.999326490452258,0.999646063968217,1.,0.999104400890347,
0.9984288220563)))
REPRESENTATION_ITEM('')
SURFACE()
);
#189=(
BOUNDED_SURFACE()
B_SPLINE_SURFACE(1,2,((#70168,#70169,#70170),(#70171,#70172,#70173),(#70174,
#70175,#70176)),.UNSPECIFIED.,.F.,.F.,.F.)
B_SPLINE_SURFACE_WITH_KNOTS((2,1,2),(3,3),(0.,1.,1.01),(0.0255903596131799,
0.0375948596693882),.UNSPECIFIED.)
GEOMETRIC_REPRESENTATION_ITEM()
RATIONAL_B_SPLINE_SURFACE(((0.996753121755999,0.997505687613148,0.999678813023854),
(0.996753121755999,0.997505687613148,0.999678813023854),(0.996753121755999,
0.997505687613148,0.999678813023854)))
REPRESENTATION_ITEM('')
SURFACE()
);
#190=(
BOUNDED_SURFACE()
B_SPLINE_SURFACE(1,2,((#70211,#70212,#70213),(#70214,#70215,#70216),(#70217,
#70218,#70219)),.UNSPECIFIED.,.F.,.F.,.F.)
B_SPLINE_SURFACE_WITH_KNOTS((2,1,2),(3,3),(-0.00286823356229767,0.,0.477902879797869),
(0.0265907346180625,0.0331702037252934),.UNSPECIFIED.)
GEOMETRIC_REPRESENTATION_ITEM()
RATIONAL_B_SPLINE_SURFACE(((0.996888414395785,0.997365765479939,0.998269846384985),
(0.996888414395785,0.997365765479939,0.998269846384985),(0.996888414395785,
0.997365765479939,0.998269846384985)))
REPRESENTATION_ITEM('')
SURFACE()
);
#191=(
BOUNDED_SURFACE()
B_SPLINE_SURFACE(1,2,((#70286,#70287,#70288),(#70289,#70290,#70291),(#70292,
#70293,#70294)),.UNSPECIFIED.,.F.,.F.,.F.)
B_SPLINE_SURFACE_WITH_KNOTS((2,1,2),(3,3),(-0.0028675312822896,0.,0.477902879799127),
(0.0166015299238957,0.0231736788111886),.UNSPECIFIED.)
GEOMETRIC_REPRESENTATION_ITEM()
RATIONAL_B_SPLINE_SURFACE(((0.996422581660833,0.996252244737342,0.996507688616404),
(0.996422581660833,0.996252244737342,0.996507688616404),(0.996422581660833,
0.996252244737342,0.996507688616404)))
REPRESENTATION_ITEM('')
SURFACE()
);
#192=(
BOUNDED_SURFACE()
B_SPLINE_SURFACE(1,2,((#70311,#70312,#70313),(#70314,#70315,#70316),(#70317,
#70318,#70319),(#70320,#70321,#70322)),.UNSPECIFIED.,.F.,.F.,.F.)
B_SPLINE_SURFACE_WITH_KNOTS((2,1,1,2),(3,3),(-0.0101,0.,1.,1.01),(0.00560769168370382,
0.0176009700440517),.UNSPECIFIED.)
GEOMETRIC_REPRESENTATION_ITEM()
RATIONAL_B_SPLINE_SURFACE(((0.998183892113821,0.99657330421516,0.996380621259469),
(0.998183892113821,0.99657330421516,0.996380621259469),(0.998183892113821,
0.99657330421516,0.996380621259469),(0.998183892113821,0.99657330421516,
0.996380621259469)))
REPRESENTATION_ITEM('')
SURFACE()
);
#193=(
BOUNDED_SURFACE()
B_SPLINE_SURFACE(1,2,((#70357,#70358,#70359),(#70360,#70361,#70362),(#70363,
#70364,#70365)),.UNSPECIFIED.,.F.,.F.,.F.)
B_SPLINE_SURFACE_WITH_KNOTS((2,1,2),(3,3),(-0.00206901892692145,0.,0.346769728502048),
(0.0066071315471865,0.0131849431468885),.UNSPECIFIED.)
GEOMETRIC_REPRESENTATION_ITEM()
RATIONAL_B_SPLINE_SURFACE(((0.997925307359452,0.997106772384943,0.996714752253861),
(0.997925307359452,0.997106772384943,0.996714752253861),(0.997925307359452,
0.997106772384943,0.996714752253861)))
REPRESENTATION_ITEM('')
SURFACE()
);
#194=(
BOUNDED_SURFACE()
B_SPLINE_SURFACE(1,2,((#70438,#70439,#70440),(#70441,#70442,#70443)),
 .UNSPECIFIED.,.F.,.F.,.F.)
B_SPLINE_SURFACE_WITH_KNOTS((2,2),(3,3),(0.,1.),(0.0556006976418414,0.0675888856590493),
 .UNSPECIFIED.)
GEOMETRIC_REPRESENTATION_ITEM()
RATIONAL_B_SPLINE_SURFACE(((0.996397562408606,0.996150386832629,0.997319912843745),
(0.996397562408606,0.996150386832629,0.997319912843745)))
REPRESENTATION_ITEM('')
SURFACE()
);
#195=(
BOUNDED_SURFACE()
B_SPLINE_SURFACE(1,2,((#70512,#70513,#70514),(#70515,#70516,#70517),(#70518,
#70519,#70520)),.UNSPECIFIED.,.F.,.F.,.F.)
B_SPLINE_SURFACE_WITH_KNOTS((2,1,2),(3,3),(0.,1.,1.01),(0.0456081671210046,
0.0575989447818808),.UNSPECIFIED.)
GEOMETRIC_REPRESENTATION_ITEM()
RATIONAL_B_SPLINE_SURFACE(((0.997793907739636,0.996365558499688,0.996354522974128),
(0.997793907739636,0.996365558499688,0.996354522974128),(0.997793907739636,
0.996365558499688,0.996354522974128)))
REPRESENTATION_ITEM('')
SURFACE()
);
#196=(
BOUNDED_SURFACE()
B_SPLINE_SURFACE(1,2,((#70555,#70556,#70557),(#70558,#70559,#70560),(#70561,
#70562,#70563)),.UNSPECIFIED.,.F.,.F.,.F.)
B_SPLINE_SURFACE_WITH_KNOTS((2,1,2),(3,3),(-0.00286810173532013,0.,0.477902879792973),
(0.0466073985929103,0.0531834929157972),.UNSPECIFIED.)
GEOMETRIC_REPRESENTATION_ITEM()
RATIONAL_B_SPLINE_SURFACE(((0.997565691989292,0.996847118055594,0.996554836292953),
(0.997565691989292,0.996847118055594,0.996554836292953),(0.997565691989292,
0.996847118055594,0.996554836292953)))
REPRESENTATION_ITEM('')
SURFACE()
);
#197=(
BOUNDED_SURFACE()
B_SPLINE_SURFACE(1,2,((#70580,#70581,#70582,#70583,#70584),(#70585,#70586,
#70587,#70588,#70589),(#70590,#70591,#70592,#70593,#70594)),
 .UNSPECIFIED.,.F.,.F.,.F.)
B_SPLINE_SURFACE_WITH_KNOTS((2,1,2),(3,2,3),(0.,1.,1.01),(0.0355931932713892,
0.0384615384615384,0.0476086899858129),.UNSPECIFIED.)
GEOMETRIC_REPRESENTATION_ITEM()
RATIONAL_B_SPLINE_SURFACE(((0.998993602249806,0.999456249886298,1.,0.998265981131401,
0.997356751596327),(0.998993602249806,0.999456249886298,1.,0.998265981131401,
0.997356751596327),(0.998993602249806,0.999456249886298,1.,0.998265981131401,
0.997356751596327)))
REPRESENTATION_ITEM('')
SURFACE()
);
#198=(
BOUNDED_SURFACE()
B_SPLINE_SURFACE(1,2,((#70642,#70643,#70644,#70645,#70646),(#70647,#70648,
#70649,#70650,#70651),(#70652,#70653,#70654,#70655,#70656)),
 .UNSPECIFIED.,.F.,.F.,.F.)
B_SPLINE_SURFACE_WITH_KNOTS((2,1,2),(3,2,3),(-0.00141401191198409,0.,0.480770297087816),
(0.0365944846645747,0.0384615384615384,0.0431859280915185),
 .UNSPECIFIED.)
GEOMETRIC_REPRESENTATION_ITEM()
RATIONAL_B_SPLINE_SURFACE(((0.999326490452258,0.999646063968217,1.,0.999104400890347,
0.9984288220563),(0.999326490452258,0.999646063968217,1.,0.999104400890347,
0.9984288220563),(0.999326490452258,0.999646063968217,1.,0.999104400890347,
0.9984288220563)))
REPRESENTATION_ITEM('')
SURFACE()
);
#199=(
BOUNDED_SURFACE()
B_SPLINE_SURFACE(1,2,((#70683,#70684,#70685),(#70686,#70687,#70688),(#70689,
#70690,#70691)),.UNSPECIFIED.,.F.,.F.,.F.)
B_SPLINE_SURFACE_WITH_KNOTS((2,1,2),(3,3),(0.,1.,1.01),(0.0255903596131799,
0.0375948596693877),.UNSPECIFIED.)
GEOMETRIC_REPRESENTATION_ITEM()
RATIONAL_B_SPLINE_SURFACE(((0.996753121755999,0.997505687613148,0.999678813023853),
(0.996753121755999,0.997505687613148,0.999678813023853),(0.996753121755999,
0.997505687613148,0.999678813023853)))
REPRESENTATION_ITEM('')
SURFACE()
);
#200=(
BOUNDED_SURFACE()
B_SPLINE_SURFACE(1,2,((#70726,#70727,#70728),(#70729,#70730,#70731),(#70732,
#70733,#70734)),.UNSPECIFIED.,.F.,.F.,.F.)
B_SPLINE_SURFACE_WITH_KNOTS((2,1,2),(3,3),(-0.00286823356226583,0.,0.477902879795317),
(0.0265907346180613,0.0331702037252919),.UNSPECIFIED.)
GEOMETRIC_REPRESENTATION_ITEM()
RATIONAL_B_SPLINE_SURFACE(((0.996888414395785,0.997365765479939,0.998269846384985),
(0.996888414395785,0.997365765479939,0.998269846384985),(0.996888414395785,
0.997365765479939,0.998269846384985)))
REPRESENTATION_ITEM('')
SURFACE()
);
#201=(
BOUNDED_SURFACE()
B_SPLINE_SURFACE(1,2,((#70801,#70802,#70803),(#70804,#70805,#70806),(#70807,
#70808,#70809)),.UNSPECIFIED.,.F.,.F.,.F.)
B_SPLINE_SURFACE_WITH_KNOTS((2,1,2),(3,3),(-0.00286753114057915,0.,0.477902879796716),
(0.0166015299238963,0.0231736788090048),.UNSPECIFIED.)
GEOMETRIC_REPRESENTATION_ITEM()
RATIONAL_B_SPLINE_SURFACE(((0.996422581660833,0.996252244737398,0.996507688616234),
(0.996422581660833,0.996252244737398,0.996507688616234),(0.996422581660833,
0.996252244737398,0.996507688616234)))
REPRESENTATION_ITEM('')
SURFACE()
);
#202=(
BOUNDED_SURFACE()
B_SPLINE_SURFACE(1,2,((#70826,#70827,#70828),(#70829,#70830,#70831),(#70832,
#70833,#70834),(#70835,#70836,#70837)),.UNSPECIFIED.,.F.,.F.,.F.)
B_SPLINE_SURFACE_WITH_KNOTS((2,1,1,2),(3,3),(-0.0101,0.,1.,1.01),(0.00560769168370605,
0.0176009700440523),.UNSPECIFIED.)
GEOMETRIC_REPRESENTATION_ITEM()
RATIONAL_B_SPLINE_SURFACE(((0.99818389211382,0.99657330421516,0.996380621259469),
(0.99818389211382,0.99657330421516,0.996380621259469),(0.99818389211382,
0.99657330421516,0.996380621259469),(0.99818389211382,0.99657330421516,
0.996380621259469)))
REPRESENTATION_ITEM('')
SURFACE()
);
#203=(
BOUNDED_SURFACE()
B_SPLINE_SURFACE(1,2,((#70872,#70873,#70874),(#70875,#70876,#70877),(#70878,
#70879,#70880)),.UNSPECIFIED.,.F.,.F.,.F.)
B_SPLINE_SURFACE_WITH_KNOTS((2,1,2),(3,3),(-0.00206901892691817,0.,0.346769728500459),
(0.00660713154719582,0.0131849431468882),.UNSPECIFIED.)
GEOMETRIC_REPRESENTATION_ITEM()
RATIONAL_B_SPLINE_SURFACE(((0.997925307359449,0.997106772384942,0.99671475225386),
(0.997925307359449,0.997106772384942,0.996714752253861),(0.997925307359449,
0.997106772384942,0.996714752253861)))
REPRESENTATION_ITEM('')
SURFACE()
);
#204=(
BOUNDED_SURFACE()
B_SPLINE_SURFACE(1,2,((#70953,#70954,#70955),(#70956,#70957,#70958)),
 .UNSPECIFIED.,.F.,.F.,.F.)
B_SPLINE_SURFACE_WITH_KNOTS((2,2),(3,3),(0.,1.),(0.0556006976418436,0.0675888856590503),
 .UNSPECIFIED.)
GEOMETRIC_REPRESENTATION_ITEM()
RATIONAL_B_SPLINE_SURFACE(((0.996397562408606,0.996150386832629,0.997319912843745),
(0.996397562408606,0.996150386832629,0.997319912843745)))
REPRESENTATION_ITEM('')
SURFACE()
);
#205=(
BOUNDED_SURFACE()
B_SPLINE_SURFACE(1,2,((#71027,#71028,#71029),(#71030,#71031,#71032),(#71033,
#71034,#71035)),.UNSPECIFIED.,.F.,.F.,.F.)
B_SPLINE_SURFACE_WITH_KNOTS((2,1,2),(3,3),(0.,1.,1.01),(0.0456081671210056,
0.0575989447818813),.UNSPECIFIED.)
GEOMETRIC_REPRESENTATION_ITEM()
RATIONAL_B_SPLINE_SURFACE(((0.997793907739636,0.996365558499688,0.996354522974128),
(0.997793907739636,0.996365558499688,0.996354522974128),(0.997793907739636,
0.996365558499688,0.996354522974128)))
REPRESENTATION_ITEM('')
SURFACE()
);
#206=(
BOUNDED_SURFACE()
B_SPLINE_SURFACE(1,2,((#71070,#71071,#71072),(#71073,#71074,#71075),(#71076,
#71077,#71078)),.UNSPECIFIED.,.F.,.F.,.F.)
B_SPLINE_SURFACE_WITH_KNOTS((2,1,2),(3,3),(-0.00286810173524515,0.,0.477902879790257),
(0.0466073985929112,0.0531834929157974),.UNSPECIFIED.)
GEOMETRIC_REPRESENTATION_ITEM()
RATIONAL_B_SPLINE_SURFACE(((0.997565691989291,0.996847118055594,0.996554836292953),
(0.997565691989291,0.996847118055594,0.996554836292953),(0.997565691989291,
0.996847118055594,0.996554836292953)))
REPRESENTATION_ITEM('')
SURFACE()
);
#207=(
BOUNDED_SURFACE()
B_SPLINE_SURFACE(1,2,((#71095,#71096,#71097,#71098,#71099),(#71100,#71101,
#71102,#71103,#71104),(#71105,#71106,#71107,#71108,#71109)),
 .UNSPECIFIED.,.F.,.F.,.F.)
B_SPLINE_SURFACE_WITH_KNOTS((2,1,2),(3,2,3),(0.,1.,1.01),(0.0355931932713904,
0.0384615384615384,0.0476086899858132),.UNSPECIFIED.)
GEOMETRIC_REPRESENTATION_ITEM()
RATIONAL_B_SPLINE_SURFACE(((0.998993602249807,0.999456249886298,1.,0.998265981131401,
0.997356751596327),(0.998993602249807,0.999456249886298,1.,0.998265981131401,
0.997356751596327),(0.998993602249807,0.999456249886298,1.,0.998265981131401,
0.997356751596327)))
REPRESENTATION_ITEM('')
SURFACE()
);
#208=(
BOUNDED_SURFACE()
B_SPLINE_SURFACE(1,2,((#71157,#71158,#71159,#71160,#71161),(#71162,#71163,
#71164,#71165,#71166),(#71167,#71168,#71169,#71170,#71171)),
 .UNSPECIFIED.,.F.,.F.,.F.)
B_SPLINE_SURFACE_WITH_KNOTS((2,1,2),(3,2,3),(-0.00141401191198426,0.,0.480770297085224),
(0.0365944846645756,0.0384615384615384,0.0431859280915178),
 .UNSPECIFIED.)
GEOMETRIC_REPRESENTATION_ITEM()
RATIONAL_B_SPLINE_SURFACE(((0.999326490452258,0.999646063968217,1.,0.999104400890347,
0.9984288220563),(0.999326490452258,0.999646063968217,1.,0.999104400890347,
0.9984288220563),(0.999326490452258,0.999646063968217,1.,0.999104400890347,
0.9984288220563)))
REPRESENTATION_ITEM('')
SURFACE()
);
#209=(
BOUNDED_SURFACE()
B_SPLINE_SURFACE(1,2,((#71198,#71199,#71200),(#71201,#71202,#71203),(#71204,
#71205,#71206)),.UNSPECIFIED.,.F.,.F.,.F.)
B_SPLINE_SURFACE_WITH_KNOTS((2,1,2),(3,3),(0.,1.,1.01),(0.0255903596131787,
0.0375948596693877),.UNSPECIFIED.)
GEOMETRIC_REPRESENTATION_ITEM()
RATIONAL_B_SPLINE_SURFACE(((0.996753121755999,0.997505687613148,0.999678813023853),
(0.996753121755999,0.997505687613148,0.999678813023853),(0.996753121755999,
0.997505687613148,0.999678813023853)))
REPRESENTATION_ITEM('')
SURFACE()
);
#210=(
BOUNDED_SURFACE()
B_SPLINE_SURFACE(1,2,((#71241,#71242,#71243),(#71244,#71245,#71246),(#71247,
#71248,#71249)),.UNSPECIFIED.,.F.,.F.,.F.)
B_SPLINE_SURFACE_WITH_KNOTS((2,1,2),(3,3),(-0.00286823356222536,0.,0.477902879792683),
(0.0265907346180612,0.0331702037252918),.UNSPECIFIED.)
GEOMETRIC_REPRESENTATION_ITEM()
RATIONAL_B_SPLINE_SURFACE(((0.996888414395785,0.997365765479939,0.998269846384985),
(0.996888414395785,0.997365765479939,0.998269846384985),(0.996888414395785,
0.997365765479939,0.998269846384985)))
REPRESENTATION_ITEM('')
SURFACE()
);
#211=(
BOUNDED_SURFACE()
B_SPLINE_SURFACE(1,2,((#71316,#71317,#71318),(#71319,#71320,#71321),(#71322,
#71323,#71324)),.UNSPECIFIED.,.F.,.F.,.F.)
B_SPLINE_SURFACE_WITH_KNOTS((2,1,2),(3,3),(-0.00286753074374937,0.,0.477902879794037),
(0.0166015299238958,0.023173678802883),.UNSPECIFIED.)
GEOMETRIC_REPRESENTATION_ITEM()
RATIONAL_B_SPLINE_SURFACE(((0.996422581660833,0.996252244737557,0.996507688615759),
(0.996422581660833,0.996252244737557,0.996507688615759),(0.996422581660833,
0.996252244737557,0.996507688615759)))
REPRESENTATION_ITEM('')
SURFACE()
);
#212=(
BOUNDED_SURFACE()
B_SPLINE_SURFACE(1,2,((#71341,#71342,#71343),(#71344,#71345,#71346),(#71347,
#71348,#71349),(#71350,#71351,#71352)),.UNSPECIFIED.,.F.,.F.,.F.)
B_SPLINE_SURFACE_WITH_KNOTS((2,1,1,2),(3,3),(-0.0101,0.,1.,1.01),(0.00560769168370419,
0.0176009700440507),.UNSPECIFIED.)
GEOMETRIC_REPRESENTATION_ITEM()
RATIONAL_B_SPLINE_SURFACE(((0.998183892113821,0.99657330421516,0.996380621259469),
(0.998183892113821,0.99657330421516,0.996380621259469),(0.998183892113821,
0.99657330421516,0.996380621259469),(0.998183892113821,0.99657330421516,
0.996380621259469)))
REPRESENTATION_ITEM('')
SURFACE()
);
#213=(
BOUNDED_SURFACE()
B_SPLINE_SURFACE(1,2,((#71387,#71388,#71389),(#71390,#71391,#71392),(#71393,
#71394,#71395)),.UNSPECIFIED.,.F.,.F.,.F.)
B_SPLINE_SURFACE_WITH_KNOTS((2,1,2),(3,3),(-0.00206901892690419,0.,0.346769728499074),
(0.00660713154720198,0.0131849431468887),.UNSPECIFIED.)
GEOMETRIC_REPRESENTATION_ITEM()
RATIONAL_B_SPLINE_SURFACE(((0.997925307359448,0.997106772384942,0.996714752253861),
(0.997925307359448,0.997106772384942,0.996714752253861),(0.997925307359448,
0.997106772384942,0.996714752253861)))
REPRESENTATION_ITEM('')
SURFACE()
);
#214=(
BOUNDED_SURFACE()
B_SPLINE_SURFACE(1,2,((#71468,#71469,#71470),(#71471,#71472,#71473)),
 .UNSPECIFIED.,.F.,.F.,.F.)
B_SPLINE_SURFACE_WITH_KNOTS((2,2),(3,3),(0.,1.),(0.0556006976418414,0.06758888565905),
 .UNSPECIFIED.)
GEOMETRIC_REPRESENTATION_ITEM()
RATIONAL_B_SPLINE_SURFACE(((0.996397562408606,0.996150386832629,0.997319912843745),
(0.996397562408606,0.996150386832629,0.997319912843745)))
REPRESENTATION_ITEM('')
SURFACE()
);
#215=(
BOUNDED_SURFACE()
B_SPLINE_SURFACE(1,2,((#71542,#71543,#71544),(#71545,#71546,#71547),(#71548,
#71549,#71550)),.UNSPECIFIED.,.F.,.F.,.F.)
B_SPLINE_SURFACE_WITH_KNOTS((2,1,2),(3,3),(0.,1.,1.01),(0.0456081671210075,
0.0575989447818828),.UNSPECIFIED.)
GEOMETRIC_REPRESENTATION_ITEM()
RATIONAL_B_SPLINE_SURFACE(((0.997793907739635,0.996365558499688,0.996354522974128),
(0.997793907739635,0.996365558499688,0.996354522974128),(0.997793907739635,
0.996365558499688,0.996354522974128)))
REPRESENTATION_ITEM('')
SURFACE()
);
#216=(
BOUNDED_SURFACE()
B_SPLINE_SURFACE(1,2,((#71585,#71586,#71587),(#71588,#71589,#71590),(#71591,
#71592,#71593)),.UNSPECIFIED.,.F.,.F.,.F.)
B_SPLINE_SURFACE_WITH_KNOTS((2,1,2),(3,3),(-0.00286810172002,0.,0.477902879787716),
(0.0466073985929109,0.0531834927425526),.UNSPECIFIED.)
GEOMETRIC_REPRESENTATION_ITEM()
RATIONAL_B_SPLINE_SURFACE(((0.997565691989291,0.996847118074524,0.996554836308353),
(0.997565691989291,0.996847118074524,0.996554836308353),(0.997565691989291,
0.996847118074524,0.996554836308353)))
REPRESENTATION_ITEM('')
SURFACE()
);
#217=(
BOUNDED_SURFACE()
B_SPLINE_SURFACE(1,2,((#71610,#71611,#71612,#71613,#71614),(#71615,#71616,
#71617,#71618,#71619),(#71620,#71621,#71622,#71623,#71624)),
 .UNSPECIFIED.,.F.,.F.,.F.)
B_SPLINE_SURFACE_WITH_KNOTS((2,1,2),(3,2,3),(0.,1.,1.01),(0.0355931932713914,
0.0384615384615384,0.0476086899858133),.UNSPECIFIED.)
GEOMETRIC_REPRESENTATION_ITEM()
RATIONAL_B_SPLINE_SURFACE(((0.998993602249807,0.999456249886298,1.,0.998265981131401,
0.997356751596327),(0.998993602249807,0.999456249886298,1.,0.998265981131401,
0.997356751596327),(0.998993602249807,0.999456249886298,1.,0.998265981131401,
0.997356751596327)))
REPRESENTATION_ITEM('')
SURFACE()
);
#218=(
BOUNDED_SURFACE()
B_SPLINE_SURFACE(1,2,((#71672,#71673,#71674,#71675,#71676),(#71677,#71678,
#71679,#71680,#71681),(#71682,#71683,#71684,#71685,#71686)),
 .UNSPECIFIED.,.F.,.F.,.F.)
B_SPLINE_SURFACE_WITH_KNOTS((2,1,2),(3,2,3),(-0.00286742666571506,0.,0.480770297123148),
(0.0365944846644088,0.0384615384615384,0.043185928091519),.UNSPECIFIED.)
GEOMETRIC_REPRESENTATION_ITEM()
RATIONAL_B_SPLINE_SURFACE(((0.999326490452201,0.999646063968185,1.,0.999104400890347,
0.9984288220563),(0.999326490452201,0.999646063968185,1.,0.999104400890347,
0.9984288220563),(0.999326490452201,0.999646063968185,1.,0.999104400890347,
0.9984288220563)))
REPRESENTATION_ITEM('')
SURFACE()
);
#219=(
BOUNDED_SURFACE()
B_SPLINE_SURFACE(1,2,((#71713,#71714,#71715),(#71716,#71717,#71718),(#71719,
#71720,#71721)),.UNSPECIFIED.,.F.,.F.,.F.)
B_SPLINE_SURFACE_WITH_KNOTS((2,1,2),(3,3),(0.,1.,1.01),(0.025590359613181,
0.0375948596693869),.UNSPECIFIED.)
GEOMETRIC_REPRESENTATION_ITEM()
RATIONAL_B_SPLINE_SURFACE(((0.996753121755999,0.997505687613148,0.999678813023853),
(0.996753121755999,0.997505687613148,0.999678813023853),(0.996753121755999,
0.997505687613148,0.999678813023853)))
REPRESENTATION_ITEM('')
SURFACE()
);
#220=(
BOUNDED_SURFACE()
B_SPLINE_SURFACE(1,2,((#71756,#71757,#71758),(#71759,#71760,#71761),(#71762,
#71763,#71764)),.UNSPECIFIED.,.F.,.F.,.F.)
B_SPLINE_SURFACE_WITH_KNOTS((2,1,2),(3,3),(-0.00286823257317966,0.,0.477902879790169),
(0.0265907346180612,0.0331702037100437),.UNSPECIFIED.)
GEOMETRIC_REPRESENTATION_ITEM()
RATIONAL_B_SPLINE_SURFACE(((0.996888414395785,0.997365765478833,0.998269846380795),
(0.996888414395785,0.997365765478833,0.998269846380795),(0.996888414395785,
0.997365765478833,0.998269846380795)))
REPRESENTATION_ITEM('')
SURFACE()
);
#221=(
BOUNDED_SURFACE()
B_SPLINE_SURFACE(1,2,((#71831,#71832,#71833),(#71834,#71835,#71836),(#71837,
#71838,#71839)),.UNSPECIFIED.,.F.,.F.,.F.)
B_SPLINE_SURFACE_WITH_KNOTS((2,1,2),(3,3),(-0.00286753114053279,0.,0.477902879791518),
(0.0166015299238948,0.0231736788090038),.UNSPECIFIED.)
GEOMETRIC_REPRESENTATION_ITEM()
RATIONAL_B_SPLINE_SURFACE(((0.996422581660833,0.996252244737398,0.996507688616235),
(0.996422581660833,0.996252244737398,0.996507688616234),(0.996422581660833,
0.996252244737398,0.996507688616235)))
REPRESENTATION_ITEM('')
SURFACE()
);
#222=(
BOUNDED_SURFACE()
B_SPLINE_SURFACE(1,2,((#71856,#71857,#71858),(#71859,#71860,#71861),(#71862,
#71863,#71864),(#71865,#71866,#71867)),.UNSPECIFIED.,.F.,.F.,.F.)
B_SPLINE_SURFACE_WITH_KNOTS((2,1,1,2),(3,3),(-0.0101,0.,1.,1.01),(0.00560769168370626,
0.0176009700440511),.UNSPECIFIED.)
GEOMETRIC_REPRESENTATION_ITEM()
RATIONAL_B_SPLINE_SURFACE(((0.99818389211382,0.99657330421516,0.996380621259469),
(0.99818389211382,0.99657330421516,0.996380621259469),(0.99818389211382,
0.99657330421516,0.996380621259469),(0.99818389211382,0.99657330421516,
0.996380621259469)))
REPRESENTATION_ITEM('')
SURFACE()
);
#223=(
BOUNDED_SURFACE()
B_SPLINE_SURFACE(1,2,((#71902,#71903,#71904),(#71905,#71906,#71907),(#71908,
#71909,#71910)),.UNSPECIFIED.,.F.,.F.,.F.)
B_SPLINE_SURFACE_WITH_KNOTS((2,1,2),(3,3),(-0.00206901892684705,0.,0.346769728497568),
(0.00660713154720629,0.0131849431468891),.UNSPECIFIED.)
GEOMETRIC_REPRESENTATION_ITEM()
RATIONAL_B_SPLINE_SURFACE(((0.997925307359447,0.997106772384942,0.996714752253861),
(0.997925307359447,0.997106772384942,0.996714752253861),(0.997925307359447,
0.997106772384942,0.996714752253861)))
REPRESENTATION_ITEM('')
SURFACE()
);
#224=(
BOUNDED_SURFACE()
B_SPLINE_SURFACE(1,2,((#71983,#71984,#71985),(#71986,#71987,#71988)),
 .UNSPECIFIED.,.F.,.F.,.F.)
B_SPLINE_SURFACE_WITH_KNOTS((2,2),(3,3),(0.,1.),(0.0556006976418414,0.0675888856590497),
 .UNSPECIFIED.)
GEOMETRIC_REPRESENTATION_ITEM()
RATIONAL_B_SPLINE_SURFACE(((0.996397562408606,0.996150386832629,0.997319912843745),
(0.996397562408606,0.996150386832629,0.997319912843745)))
REPRESENTATION_ITEM('')
SURFACE()
);
#225=(
BOUNDED_SURFACE()
B_SPLINE_SURFACE(1,2,((#72057,#72058,#72059),(#72060,#72061,#72062),(#72063,
#72064,#72065)),.UNSPECIFIED.,.F.,.F.,.F.)
B_SPLINE_SURFACE_WITH_KNOTS((2,1,2),(3,3),(0.,1.,1.01),(0.0456081671210055,
0.0575989447818817),.UNSPECIFIED.)
GEOMETRIC_REPRESENTATION_ITEM()
RATIONAL_B_SPLINE_SURFACE(((0.997793907739636,0.996365558499688,0.996354522974128),
(0.997793907739636,0.996365558499688,0.996354522974128),(0.997793907739636,
0.996365558499688,0.996354522974128)))
REPRESENTATION_ITEM('')
SURFACE()
);
#226=(
BOUNDED_SURFACE()
B_SPLINE_SURFACE(1,2,((#72100,#72101,#72102),(#72103,#72104,#72105),(#72106,
#72107,#72108)),.UNSPECIFIED.,.F.,.F.,.F.)
B_SPLINE_SURFACE_WITH_KNOTS((2,1,2),(3,3),(-0.00286810173515641,0.,0.477902879786463),
(0.0466073985929113,0.0531834929157985),.UNSPECIFIED.)
GEOMETRIC_REPRESENTATION_ITEM()
RATIONAL_B_SPLINE_SURFACE(((0.997565691989292,0.996847118055594,0.996554836292953),
(0.997565691989292,0.996847118055594,0.996554836292953),(0.997565691989292,
0.996847118055594,0.996554836292953)))
REPRESENTATION_ITEM('')
SURFACE()
);
#227=(
BOUNDED_SURFACE()
B_SPLINE_SURFACE(1,2,((#72125,#72126,#72127,#72128,#72129),(#72130,#72131,
#72132,#72133,#72134),(#72135,#72136,#72137,#72138,#72139)),
 .UNSPECIFIED.,.F.,.F.,.F.)
B_SPLINE_SURFACE_WITH_KNOTS((2,1,2),(3,2,3),(0.,1.,1.01),(0.0355931932713902,
0.0384615384615384,0.0476086899858155),.UNSPECIFIED.)
GEOMETRIC_REPRESENTATION_ITEM()
RATIONAL_B_SPLINE_SURFACE(((0.998993602249807,0.999456249886298,1.,0.9982659811314,
0.997356751596326),(0.998993602249807,0.999456249886298,1.,0.9982659811314,
0.997356751596326),(0.998993602249807,0.999456249886298,1.,0.9982659811314,
0.997356751596326)))
REPRESENTATION_ITEM('')
SURFACE()
);
#228=(
BOUNDED_SURFACE()
B_SPLINE_SURFACE(1,2,((#72187,#72188,#72189,#72190,#72191),(#72192,#72193,
#72194,#72195,#72196),(#72197,#72198,#72199,#72200,#72201)),
 .UNSPECIFIED.,.F.,.F.,.F.)
B_SPLINE_SURFACE_WITH_KNOTS((2,1,2),(3,2,3),(-0.00286743097398646,0.,0.480770297146974),
(0.0365944846644077,0.0384615384615384,0.0431859280915196),
 .UNSPECIFIED.)
GEOMETRIC_REPRESENTATION_ITEM()
RATIONAL_B_SPLINE_SURFACE(((0.999326490452201,0.999646063968185,1.,0.999104400890347,
0.9984288220563),(0.999326490452201,0.999646063968185,1.,0.999104400890347,
0.9984288220563),(0.999326490452201,0.999646063968185,1.,0.999104400890347,
0.9984288220563)))
REPRESENTATION_ITEM('')
SURFACE()
);
#229=(
BOUNDED_SURFACE()
B_SPLINE_SURFACE(1,2,((#72228,#72229,#72230),(#72231,#72232,#72233),(#72234,
#72235,#72236)),.UNSPECIFIED.,.F.,.F.,.F.)
B_SPLINE_SURFACE_WITH_KNOTS((2,1,2),(3,3),(0.,1.,1.01),(0.0255903596131818,
0.0375948596693897),.UNSPECIFIED.)
GEOMETRIC_REPRESENTATION_ITEM()
RATIONAL_B_SPLINE_SURFACE(((0.996753121755999,0.997505687613148,0.999678813023854),
(0.996753121755999,0.997505687613148,0.999678813023854),(0.996753121755999,
0.997505687613148,0.999678813023854)))
REPRESENTATION_ITEM('')
SURFACE()
);
#230=(
BOUNDED_SURFACE()
B_SPLINE_SURFACE(1,2,((#72271,#72272,#72273),(#72274,#72275,#72276),(#72277,
#72278,#72279)),.UNSPECIFIED.,.F.,.F.,.F.)
B_SPLINE_SURFACE_WITH_KNOTS((2,1,2),(3,3),(-0.00286823045902527,0.,0.477902879787612),
(0.0265907346180616,0.0331702036774543),.UNSPECIFIED.)
GEOMETRIC_REPRESENTATION_ITEM()
RATIONAL_B_SPLINE_SURFACE(((0.996888414395785,0.997365765476469,0.998269846371839),
(0.996888414395785,0.997365765476469,0.998269846371839),(0.996888414395785,
0.997365765476469,0.998269846371839)))
REPRESENTATION_ITEM('')
SURFACE()
);
#231=(
BOUNDED_SURFACE()
B_SPLINE_SURFACE(1,2,((#72346,#72347,#72348),(#72349,#72350,#72351),(#72352,
#72353,#72354)),.UNSPECIFIED.,.F.,.F.,.F.)
B_SPLINE_SURFACE_WITH_KNOTS((2,1,2),(3,3),(-0.00286753128207188,0.,0.477902879788894),
(0.0166015299238944,0.0231736788111879),.UNSPECIFIED.)
GEOMETRIC_REPRESENTATION_ITEM()
RATIONAL_B_SPLINE_SURFACE(((0.996422581660833,0.996252244737341,0.996507688616404),
(0.996422581660833,0.996252244737341,0.996507688616404),(0.996422581660833,
0.996252244737341,0.996507688616404)))
REPRESENTATION_ITEM('')
SURFACE()
);
#232=(
BOUNDED_SURFACE()
B_SPLINE_SURFACE(1,2,((#72371,#72372,#72373),(#72374,#72375,#72376),(#72377,
#72378,#72379),(#72380,#72381,#72382)),.UNSPECIFIED.,.F.,.F.,.F.)
B_SPLINE_SURFACE_WITH_KNOTS((2,1,1,2),(3,3),(-0.0101,0.,1.,1.01),(0.00560769168370511,
0.0176009700440523),.UNSPECIFIED.)
GEOMETRIC_REPRESENTATION_ITEM()
RATIONAL_B_SPLINE_SURFACE(((0.998183892113821,0.99657330421516,0.996380621259469),
(0.998183892113821,0.99657330421516,0.996380621259469),(0.998183892113821,
0.99657330421516,0.996380621259469),(0.998183892113821,0.99657330421516,
0.996380621259469)))
REPRESENTATION_ITEM('')
SURFACE()
);
#233=(
BOUNDED_SURFACE()
B_SPLINE_SURFACE(1,2,((#72417,#72418,#72419),(#72420,#72421,#72422),(#72423,
#72424,#72425)),.UNSPECIFIED.,.F.,.F.,.F.)
B_SPLINE_SURFACE_WITH_KNOTS((2,1,2),(3,3),(-0.00206901892682504,0.,0.346769728496379),
(0.0066071315472073,0.0131849431468888),.UNSPECIFIED.)
GEOMETRIC_REPRESENTATION_ITEM()
RATIONAL_B_SPLINE_SURFACE(((0.997925307359446,0.997106772384942,0.996714752253861),
(0.997925307359446,0.997106772384942,0.996714752253861),(0.997925307359446,
0.997106772384942,0.996714752253861)))
REPRESENTATION_ITEM('')
SURFACE()
);
#234=(
BOUNDED_SURFACE()
B_SPLINE_SURFACE(1,2,((#72498,#72499,#72500),(#72501,#72502,#72503)),
 .UNSPECIFIED.,.F.,.F.,.F.)
B_SPLINE_SURFACE_WITH_KNOTS((2,2),(3,3),(0.,1.),(0.0556006976418428,0.0675888856590498),
 .UNSPECIFIED.)
GEOMETRIC_REPRESENTATION_ITEM()
RATIONAL_B_SPLINE_SURFACE(((0.996397562408606,0.996150386832629,0.997319912843745),
(0.996397562408606,0.996150386832629,0.997319912843745)))
REPRESENTATION_ITEM('')
SURFACE()
);
#235=(
BOUNDED_SURFACE()
B_SPLINE_SURFACE(1,2,((#72572,#72573,#72574),(#72575,#72576,#72577),(#72578,
#72579,#72580)),.UNSPECIFIED.,.F.,.F.,.F.)
B_SPLINE_SURFACE_WITH_KNOTS((2,1,2),(3,3),(0.,1.,1.01),(0.0456081671210033,
0.057598944781882),.UNSPECIFIED.)
GEOMETRIC_REPRESENTATION_ITEM()
RATIONAL_B_SPLINE_SURFACE(((0.997793907739636,0.996365558499688,0.996354522974128),
(0.997793907739636,0.996365558499688,0.996354522974128),(0.997793907739636,
0.996365558499688,0.996354522974128)))
REPRESENTATION_ITEM('')
SURFACE()
);
#236=(
BOUNDED_SURFACE()
B_SPLINE_SURFACE(1,2,((#72615,#72616,#72617),(#72618,#72619,#72620),(#72621,
#72622,#72623)),.UNSPECIFIED.,.F.,.F.,.F.)
B_SPLINE_SURFACE_WITH_KNOTS((2,1,2),(3,3),(-0.00286810173510994,0.,0.477902879786495),
(0.0466073985929119,0.0531834929157975),.UNSPECIFIED.)
GEOMETRIC_REPRESENTATION_ITEM()
RATIONAL_B_SPLINE_SURFACE(((0.997565691989291,0.996847118055594,0.996554836292953),
(0.997565691989291,0.996847118055594,0.996554836292953),(0.997565691989291,
0.996847118055594,0.996554836292953)))
REPRESENTATION_ITEM('')
SURFACE()
);
#237=(
BOUNDED_SURFACE()
B_SPLINE_SURFACE(1,2,((#72640,#72641,#72642,#72643,#72644),(#72645,#72646,
#72647,#72648,#72649),(#72650,#72651,#72652,#72653,#72654)),
 .UNSPECIFIED.,.F.,.F.,.F.)
B_SPLINE_SURFACE_WITH_KNOTS((2,1,2),(3,2,3),(0.,1.,1.01),(0.0355931932713904,
0.0384615384615384,0.0476086899858138),.UNSPECIFIED.)
GEOMETRIC_REPRESENTATION_ITEM()
RATIONAL_B_SPLINE_SURFACE(((0.998993602249807,0.999456249886298,1.,0.998265981131401,
0.997356751596327),(0.998993602249807,0.999456249886298,1.,0.998265981131401,
0.997356751596327),(0.998993602249807,0.999456249886298,1.,0.998265981131401,
0.997356751596327)))
REPRESENTATION_ITEM('')
SURFACE()
);
#238=(
BOUNDED_SURFACE()
B_SPLINE_SURFACE(1,2,((#72702,#72703,#72704,#72705,#72706),(#72707,#72708,
#72709,#72710,#72711),(#72712,#72713,#72714,#72715,#72716)),
 .UNSPECIFIED.,.F.,.F.,.F.)
B_SPLINE_SURFACE_WITH_KNOTS((2,1,2),(3,2,3),(-0.00141401191198139,0.,0.480770297079875),
(0.0365944846645798,0.0384615384615384,0.0431859280915183),
 .UNSPECIFIED.)
GEOMETRIC_REPRESENTATION_ITEM()
RATIONAL_B_SPLINE_SURFACE(((0.99932649045226,0.999646063968218,1.,0.999104400890347,
0.9984288220563),(0.99932649045226,0.999646063968218,1.,0.999104400890347,
0.9984288220563),(0.99932649045226,0.999646063968218,1.,0.999104400890347,
0.9984288220563)))
REPRESENTATION_ITEM('')
SURFACE()
);
#239=(
BOUNDED_SURFACE()
B_SPLINE_SURFACE(1,2,((#72743,#72744,#72745),(#72746,#72747,#72748),(#72749,
#72750,#72751)),.UNSPECIFIED.,.F.,.F.,.F.)
B_SPLINE_SURFACE_WITH_KNOTS((2,1,2),(3,3),(0.,1.,1.01),(0.0255903596131808,
0.0375948596693885),.UNSPECIFIED.)
GEOMETRIC_REPRESENTATION_ITEM()
RATIONAL_B_SPLINE_SURFACE(((0.996753121755999,0.997505687613148,0.999678813023854),
(0.996753121755999,0.997505687613148,0.999678813023854),(0.996753121755999,
0.997505687613148,0.999678813023854)))
REPRESENTATION_ITEM('')
SURFACE()
);
#240=(
BOUNDED_SURFACE()
B_SPLINE_SURFACE(1,2,((#72786,#72787,#72788),(#72789,#72790,#72791),(#72792,
#72793,#72794)),.UNSPECIFIED.,.F.,.F.,.F.)
B_SPLINE_SURFACE_WITH_KNOTS((2,1,2),(3,3),(-0.00286823356224596,0.,0.47790287978649),
(0.0265907346180609,0.0331702037252913),.UNSPECIFIED.)
GEOMETRIC_REPRESENTATION_ITEM()
RATIONAL_B_SPLINE_SURFACE(((0.996888414395785,0.997365765479939,0.998269846384985),
(0.996888414395785,0.997365765479939,0.998269846384985),(0.996888414395785,
0.997365765479939,0.998269846384985)))
REPRESENTATION_ITEM('')
SURFACE()
);
#241=(
BOUNDED_SURFACE()
B_SPLINE_SURFACE(1,2,((#72861,#72862,#72863),(#72864,#72865,#72866),(#72867,
#72868,#72869)),.UNSPECIFIED.,.F.,.F.,.F.)
B_SPLINE_SURFACE_WITH_KNOTS((2,1,2),(3,3),(-0.00286753128217537,0.,0.477902879803344),
(0.0166015299238946,0.0231736788111885),.UNSPECIFIED.)
GEOMETRIC_REPRESENTATION_ITEM()
RATIONAL_B_SPLINE_SURFACE(((0.996422581660833,0.996252244737341,0.996507688616404),
(0.996422581660833,0.996252244737341,0.996507688616404),(0.996422581660833,
0.996252244737341,0.996507688616404)))
REPRESENTATION_ITEM('')
SURFACE()
);
#242=(
BOUNDED_SURFACE()
B_SPLINE_SURFACE(1,2,((#72886,#72887,#72888),(#72889,#72890,#72891),(#72892,
#72893,#72894),(#72895,#72896,#72897)),.UNSPECIFIED.,.F.,.F.,.F.)
B_SPLINE_SURFACE_WITH_KNOTS((2,1,1,2),(3,3),(-0.0101,0.,1.,1.01),(0.0056076916837073,
0.0176009700440516),.UNSPECIFIED.)
GEOMETRIC_REPRESENTATION_ITEM()
RATIONAL_B_SPLINE_SURFACE(((0.99818389211382,0.99657330421516,0.996380621259469),
(0.99818389211382,0.99657330421516,0.996380621259469),(0.99818389211382,
0.99657330421516,0.996380621259469),(0.99818389211382,0.99657330421516,
0.996380621259469)))
REPRESENTATION_ITEM('')
SURFACE()
);
#243=(
BOUNDED_SURFACE()
B_SPLINE_SURFACE(1,2,((#72932,#72933,#72934),(#72935,#72936,#72937),(#72938,
#72939,#72940)),.UNSPECIFIED.,.F.,.F.,.F.)
B_SPLINE_SURFACE_WITH_KNOTS((2,1,2),(3,3),(-0.00206901892514686,0.,0.346769728494917),
(0.00660713154720862,0.0131849431292488),.UNSPECIFIED.)
GEOMETRIC_REPRESENTATION_ITEM()
RATIONAL_B_SPLINE_SURFACE(((0.997925307359446,0.997106772387137,0.996714752255963),
(0.997925307359446,0.997106772387137,0.996714752255963),(0.997925307359446,
0.997106772387137,0.996714752255963)))
REPRESENTATION_ITEM('')
SURFACE()
);
#244=(
BOUNDED_SURFACE()
B_SPLINE_SURFACE(1,2,((#73013,#73014,#73015),(#73016,#73017,#73018)),
 .UNSPECIFIED.,.F.,.F.,.F.)
B_SPLINE_SURFACE_WITH_KNOTS((2,2),(3,3),(0.,1.),(0.0556006976418414,0.0675888856590506),
 .UNSPECIFIED.)
GEOMETRIC_REPRESENTATION_ITEM()
RATIONAL_B_SPLINE_SURFACE(((0.996397562408606,0.996150386832629,0.997319912843745),
(0.996397562408606,0.996150386832629,0.997319912843745)))
REPRESENTATION_ITEM('')
SURFACE()
);
#245=(
BOUNDED_SURFACE()
B_SPLINE_SURFACE(1,2,((#73087,#73088,#73089),(#73090,#73091,#73092)),
 .UNSPECIFIED.,.F.,.F.,.F.)
B_SPLINE_SURFACE_WITH_KNOTS((2,2),(3,3),(0.,1.),(0.0456081671210034,0.0575989447818825),
 .UNSPECIFIED.)
GEOMETRIC_REPRESENTATION_ITEM()
RATIONAL_B_SPLINE_SURFACE(((0.997793907739636,0.996365558499688,0.996354522974128),
(0.997793907739636,0.996365558499688,0.996354522974128)))
REPRESENTATION_ITEM('')
SURFACE()
);
#246=(
BOUNDED_SURFACE()
B_SPLINE_SURFACE(1,2,((#73159,#73160,#73161,#73162,#73163),(#73164,#73165,
#73166,#73167,#73168),(#73169,#73170,#73171,#73172,#73173)),
 .UNSPECIFIED.,.F.,.F.,.F.)
B_SPLINE_SURFACE_WITH_KNOTS((2,1,2),(3,2,3),(0.,1.,1.01),(0.0355931932713903,
0.0384615384615384,0.0476086899858127),.UNSPECIFIED.)
GEOMETRIC_REPRESENTATION_ITEM()
RATIONAL_B_SPLINE_SURFACE(((0.998993602249807,0.999456249886298,1.,0.998265981131401,
0.997356751596327),(0.998993602249807,0.999456249886298,1.,0.998265981131401,
0.997356751596327),(0.998993602249807,0.999456249886298,1.,0.998265981131401,
0.997356751596327)))
REPRESENTATION_ITEM('')
SURFACE()
);
#247=(
BOUNDED_SURFACE()
B_SPLINE_SURFACE(1,2,((#73221,#73222,#73223,#73224,#73225),(#73226,#73227,
#73228,#73229,#73230),(#73231,#73232,#73233,#73234,#73235)),
 .UNSPECIFIED.,.F.,.F.,.F.)
B_SPLINE_SURFACE_WITH_KNOTS((2,1,2),(3,2,3),(-0.00141401191198094,0.,0.480770297079957),
(0.0365944846645789,0.0384615384615384,0.0431859280915187),
 .UNSPECIFIED.)
GEOMETRIC_REPRESENTATION_ITEM()
RATIONAL_B_SPLINE_SURFACE(((0.99932649045226,0.999646063968218,1.,0.999104400890347,
0.9984288220563),(0.99932649045226,0.999646063968218,1.,0.999104400890347,
0.9984288220563),(0.99932649045226,0.999646063968218,1.,0.999104400890347,
0.9984288220563)))
REPRESENTATION_ITEM('')
SURFACE()
);
#248=(
BOUNDED_SURFACE()
B_SPLINE_SURFACE(1,2,((#73262,#73263,#73264),(#73265,#73266,#73267),(#73268,
#73269,#73270)),.UNSPECIFIED.,.F.,.F.,.F.)
B_SPLINE_SURFACE_WITH_KNOTS((2,1,2),(3,3),(0.,1.,1.01),(0.0255903596131778,
0.0375948596693862),.UNSPECIFIED.)
GEOMETRIC_REPRESENTATION_ITEM()
RATIONAL_B_SPLINE_SURFACE(((0.996753121755999,0.997505687613147,0.999678813023853),
(0.996753121755999,0.997505687613147,0.999678813023853),(0.996753121755999,
0.997505687613147,0.999678813023853)))
REPRESENTATION_ITEM('')
SURFACE()
);
#249=(
BOUNDED_SURFACE()
B_SPLINE_SURFACE(1,2,((#73305,#73306,#73307),(#73308,#73309,#73310),(#73311,
#73312,#73313)),.UNSPECIFIED.,.F.,.F.,.F.)
B_SPLINE_SURFACE_WITH_KNOTS((2,1,2),(3,3),(-0.00286823045909901,0.,0.477902879786441),
(0.0265907346180619,0.0331702036774536),.UNSPECIFIED.)
GEOMETRIC_REPRESENTATION_ITEM()
RATIONAL_B_SPLINE_SURFACE(((0.996888414395785,0.997365765476469,0.998269846371839),
(0.996888414395785,0.997365765476469,0.998269846371839),(0.996888414395785,
0.997365765476469,0.998269846371839)))
REPRESENTATION_ITEM('')
SURFACE()
);
#250=(
BOUNDED_SURFACE()
B_SPLINE_SURFACE(1,2,((#73380,#73381,#73382),(#73383,#73384,#73385),(#73386,
#73387,#73388)),.UNSPECIFIED.,.F.,.F.,.F.)
B_SPLINE_SURFACE_WITH_KNOTS((2,1,2),(3,3),(-0.00286753128207195,0.,0.477902879786496),
(0.0166015299238956,0.0231736788111879),.UNSPECIFIED.)
GEOMETRIC_REPRESENTATION_ITEM()
RATIONAL_B_SPLINE_SURFACE(((0.996422581660832,0.996252244737341,0.996507688616404),
(0.996422581660832,0.996252244737341,0.996507688616404),(0.996422581660832,
0.996252244737341,0.996507688616404)))
REPRESENTATION_ITEM('')
SURFACE()
);
#251=(
BOUNDED_SURFACE()
B_SPLINE_SURFACE(1,2,((#73405,#73406,#73407),(#73408,#73409,#73410),(#73411,
#73412,#73413),(#73414,#73415,#73416)),.UNSPECIFIED.,.F.,.F.,.F.)
B_SPLINE_SURFACE_WITH_KNOTS((2,1,1,2),(3,3),(-0.0101,0.,1.,1.01),(0.00560769168370627,
0.0176009700440521),.UNSPECIFIED.)
GEOMETRIC_REPRESENTATION_ITEM()
RATIONAL_B_SPLINE_SURFACE(((0.99818389211382,0.99657330421516,0.996380621259469),
(0.99818389211382,0.99657330421516,0.996380621259469),(0.99818389211382,
0.99657330421516,0.996380621259469),(0.99818389211382,0.99657330421516,
0.996380621259469)))
REPRESENTATION_ITEM('')
SURFACE()
);
#252=(
BOUNDED_SURFACE()
B_SPLINE_SURFACE(1,2,((#73451,#73452,#73453),(#73454,#73455,#73456),(#73457,
#73458,#73459)),.UNSPECIFIED.,.F.,.F.,.F.)
B_SPLINE_SURFACE_WITH_KNOTS((2,1,2),(3,3),(-0.0020690189250989,0.,0.346769728493813),
(0.00660713154720725,0.0131849431292534),.UNSPECIFIED.)
GEOMETRIC_REPRESENTATION_ITEM()
RATIONAL_B_SPLINE_SURFACE(((0.997925307359446,0.997106772387136,0.996714752255963),
(0.997925307359446,0.997106772387136,0.996714752255963),(0.997925307359446,
0.997106772387136,0.996714752255963)))
REPRESENTATION_ITEM('')
SURFACE()
);
#253=(
BOUNDED_SURFACE()
B_SPLINE_SURFACE(1,2,((#73532,#73533,#73534),(#73535,#73536,#73537)),
 .UNSPECIFIED.,.F.,.F.,.F.)
B_SPLINE_SURFACE_WITH_KNOTS((2,2),(3,3),(0.,1.),(0.0556006976418393,0.0675888856590512),
 .UNSPECIFIED.)
GEOMETRIC_REPRESENTATION_ITEM()
RATIONAL_B_SPLINE_SURFACE(((0.996397562408606,0.996150386832629,0.997319912843745),
(0.996397562408606,0.996150386832629,0.997319912843745)))
REPRESENTATION_ITEM('')
SURFACE()
);
#254=(
BOUNDED_SURFACE()
B_SPLINE_SURFACE(1,2,((#73606,#73607,#73608),(#73609,#73610,#73611),(#73612,
#73613,#73614)),.UNSPECIFIED.,.F.,.F.,.F.)
B_SPLINE_SURFACE_WITH_KNOTS((2,1,2),(3,3),(0.,1.,1.01),(0.0456081671210001,
0.0575989447818822),.UNSPECIFIED.)
GEOMETRIC_REPRESENTATION_ITEM()
RATIONAL_B_SPLINE_SURFACE(((0.997793907739637,0.996365558499688,0.996354522974128),
(0.997793907739637,0.996365558499688,0.996354522974128),(0.997793907739637,
0.996365558499688,0.996354522974128)))
REPRESENTATION_ITEM('')
SURFACE()
);
#255=(
BOUNDED_SURFACE()
B_SPLINE_SURFACE(1,2,((#73649,#73650,#73651),(#73652,#73653,#73654),(#73655,
#73656,#73657)),.UNSPECIFIED.,.F.,.F.,.F.)
B_SPLINE_SURFACE_WITH_KNOTS((2,1,2),(3,3),(-0.0028681017350075,0.,0.47790287978652),
(0.0466073985929105,0.0531834929157979),.UNSPECIFIED.)
GEOMETRIC_REPRESENTATION_ITEM()
RATIONAL_B_SPLINE_SURFACE(((0.997565691989291,0.996847118055594,0.996554836292953),
(0.997565691989291,0.996847118055594,0.996554836292953),(0.997565691989291,
0.996847118055594,0.996554836292953)))
REPRESENTATION_ITEM('')
SURFACE()
);
#256=(
BOUNDED_SURFACE()
B_SPLINE_SURFACE(1,2,((#73674,#73675,#73676,#73677,#73678),(#73679,#73680,
#73681,#73682,#73683),(#73684,#73685,#73686,#73687,#73688)),
 .UNSPECIFIED.,.F.,.F.,.F.)
B_SPLINE_SURFACE_WITH_KNOTS((2,1,2),(3,2,3),(0.,1.,1.01),(0.0355931932713903,
0.0384615384615384,0.0476086899858126),.UNSPECIFIED.)
GEOMETRIC_REPRESENTATION_ITEM()
RATIONAL_B_SPLINE_SURFACE(((0.998993602249807,0.999456249886298,1.,0.998265981131401,
0.997356751596327),(0.998993602249807,0.999456249886298,1.,0.998265981131401,
0.997356751596327),(0.998993602249807,0.999456249886298,1.,0.998265981131401,
0.997356751596327)))
REPRESENTATION_ITEM('')
SURFACE()
);
#257=(
BOUNDED_SURFACE()
B_SPLINE_SURFACE(1,2,((#73736,#73737,#73738,#73739,#73740),(#73741,#73742,
#73743,#73744,#73745),(#73746,#73747,#73748,#73749,#73750)),
 .UNSPECIFIED.,.F.,.F.,.F.)
B_SPLINE_SURFACE_WITH_KNOTS((2,1,2),(3,2,3),(-0.00286743098086898,0.,0.480770297146936),
(0.0365944846643956,0.0384615384615384,0.0431859280915195),
 .UNSPECIFIED.)
GEOMETRIC_REPRESENTATION_ITEM()
RATIONAL_B_SPLINE_SURFACE(((0.999326490452197,0.999646063968182,1.,0.999104400890347,
0.9984288220563),(0.999326490452197,0.999646063968182,1.,0.999104400890347,
0.9984288220563),(0.999326490452197,0.999646063968182,1.,0.999104400890347,
0.9984288220563)))
REPRESENTATION_ITEM('')
SURFACE()
);
#258=(
BOUNDED_SURFACE()
B_SPLINE_SURFACE(1,2,((#73777,#73778,#73779),(#73780,#73781,#73782),(#73783,
#73784,#73785)),.UNSPECIFIED.,.F.,.F.,.F.)
B_SPLINE_SURFACE_WITH_KNOTS((2,1,2),(3,3),(0.,1.,1.01),(0.0255903596131777,
0.0375948596693867),.UNSPECIFIED.)
GEOMETRIC_REPRESENTATION_ITEM()
RATIONAL_B_SPLINE_SURFACE(((0.996753121755999,0.997505687613147,0.999678813023853),
(0.996753121755999,0.997505687613147,0.999678813023853),(0.996753121755999,
0.997505687613147,0.999678813023853)))
REPRESENTATION_ITEM('')
SURFACE()
);
#259=(
BOUNDED_SURFACE()
B_SPLINE_SURFACE(1,2,((#73820,#73821,#73822),(#73823,#73824,#73825),(#73826,
#73827,#73828)),.UNSPECIFIED.,.F.,.F.,.F.)
B_SPLINE_SURFACE_WITH_KNOTS((2,1,2),(3,3),(-0.00286823356216264,0.,0.477902879786493),
(0.0265907346180615,0.0331702037252919),.UNSPECIFIED.)
GEOMETRIC_REPRESENTATION_ITEM()
RATIONAL_B_SPLINE_SURFACE(((0.996888414395785,0.997365765479939,0.998269846384985),
(0.996888414395785,0.997365765479939,0.998269846384985),(0.996888414395785,
0.997365765479939,0.998269846384985)))
REPRESENTATION_ITEM('')
SURFACE()
);
#260=(
BOUNDED_SURFACE()
B_SPLINE_SURFACE(1,2,((#73895,#73896,#73897),(#73898,#73899,#73900),(#73901,
#73902,#73903)),.UNSPECIFIED.,.F.,.F.,.F.)
B_SPLINE_SURFACE_WITH_KNOTS((2,1,2),(3,3),(-0.00286753128208516,0.,0.47790287978643),
(0.0166015299238966,0.0231736788111885),.UNSPECIFIED.)
GEOMETRIC_REPRESENTATION_ITEM()
RATIONAL_B_SPLINE_SURFACE(((0.996422581660833,0.996252244737341,0.996507688616404),
(0.996422581660833,0.996252244737341,0.996507688616404),(0.996422581660833,
0.996252244737341,0.996507688616404)))
REPRESENTATION_ITEM('')
SURFACE()
);
#261=(
BOUNDED_SURFACE()
B_SPLINE_SURFACE(1,2,((#73920,#73921,#73922),(#73923,#73924,#73925),(#73926,
#73927,#73928),(#73929,#73930,#73931)),.UNSPECIFIED.,.F.,.F.,.F.)
B_SPLINE_SURFACE_WITH_KNOTS((2,1,1,2),(3,3),(-0.0101,0.,1.,1.01),(0.00560769168370496,
0.0176009700440518),.UNSPECIFIED.)
GEOMETRIC_REPRESENTATION_ITEM()
RATIONAL_B_SPLINE_SURFACE(((0.998183892113821,0.99657330421516,0.996380621259469),
(0.998183892113821,0.99657330421516,0.996380621259469),(0.998183892113821,
0.99657330421516,0.996380621259469),(0.998183892113821,0.99657330421516,
0.996380621259469)))
REPRESENTATION_ITEM('')
SURFACE()
);
#262=(
BOUNDED_SURFACE()
B_SPLINE_SURFACE(1,2,((#73966,#73967,#73968),(#73969,#73970,#73971),(#73972,
#73973,#73974)),.UNSPECIFIED.,.F.,.F.,.F.)
B_SPLINE_SURFACE_WITH_KNOTS((2,1,2),(3,3),(-0.00206901892662539,0.,0.346769728493036),
(0.00660713154720504,0.013184943146903),.UNSPECIFIED.)
GEOMETRIC_REPRESENTATION_ITEM()
RATIONAL_B_SPLINE_SURFACE(((0.997925307359447,0.99710677238494,0.996714752253859),
(0.997925307359447,0.99710677238494,0.996714752253859),(0.997925307359447,
0.99710677238494,0.996714752253859)))
REPRESENTATION_ITEM('')
SURFACE()
);
#263=(
BOUNDED_SURFACE()
B_SPLINE_SURFACE(1,2,((#74047,#74048,#74049),(#74050,#74051,#74052)),
 .UNSPECIFIED.,.F.,.F.,.F.)
B_SPLINE_SURFACE_WITH_KNOTS((2,2),(3,3),(0.,1.),(0.0556006976418428,0.0675888856590492),
 .UNSPECIFIED.)
GEOMETRIC_REPRESENTATION_ITEM()
RATIONAL_B_SPLINE_SURFACE(((0.996397562408606,0.996150386832629,0.997319912843745),
(0.996397562408606,0.996150386832629,0.997319912843745)))
REPRESENTATION_ITEM('')
SURFACE()
);
#264=(
BOUNDED_SURFACE()
B_SPLINE_SURFACE(1,2,((#74121,#74122,#74123),(#74124,#74125,#74126),(#74127,
#74128,#74129)),.UNSPECIFIED.,.F.,.F.,.F.)
B_SPLINE_SURFACE_WITH_KNOTS((2,1,2),(3,3),(0.,1.,1.01),(0.0456081671210057,
0.0575989447818801),.UNSPECIFIED.)
GEOMETRIC_REPRESENTATION_ITEM()
RATIONAL_B_SPLINE_SURFACE(((0.997793907739636,0.996365558499688,0.996354522974128),
(0.997793907739636,0.996365558499688,0.996354522974128),(0.997793907739636,
0.996365558499688,0.996354522974128)))
REPRESENTATION_ITEM('')
SURFACE()
);
#265=(
BOUNDED_SURFACE()
B_SPLINE_SURFACE(1,2,((#74164,#74165,#74166),(#74167,#74168,#74169),(#74170,
#74171,#74172)),.UNSPECIFIED.,.F.,.F.,.F.)
B_SPLINE_SURFACE_WITH_KNOTS((2,1,2),(3,3),(-0.00286810173496387,0.,0.477902879786524),
(0.0466073985929113,0.0531834929157973),.UNSPECIFIED.)
GEOMETRIC_REPRESENTATION_ITEM()
RATIONAL_B_SPLINE_SURFACE(((0.997565691989291,0.996847118055594,0.996554836292953),
(0.997565691989291,0.996847118055594,0.996554836292953),(0.997565691989291,
0.996847118055594,0.996554836292953)))
REPRESENTATION_ITEM('')
SURFACE()
);
#266=(
BOUNDED_SURFACE()
B_SPLINE_SURFACE(1,2,((#74189,#74190,#74191,#74192,#74193),(#74194,#74195,
#74196,#74197,#74198),(#74199,#74200,#74201,#74202,#74203)),
 .UNSPECIFIED.,.F.,.F.,.F.)
B_SPLINE_SURFACE_WITH_KNOTS((2,1,2),(3,2,3),(0.,1.,1.01),(0.0355931932713904,
0.0384615384615384,0.047608689985811),.UNSPECIFIED.)
GEOMETRIC_REPRESENTATION_ITEM()
RATIONAL_B_SPLINE_SURFACE(((0.998993602249807,0.999456249886298,1.,0.998265981131401,
0.997356751596327),(0.998993602249807,0.999456249886298,1.,0.998265981131401,
0.997356751596327),(0.998993602249807,0.999456249886298,1.,0.998265981131401,
0.997356751596327)))
REPRESENTATION_ITEM('')
SURFACE()
);
#267=(
BOUNDED_SURFACE()
B_SPLINE_SURFACE(1,2,((#74251,#74252,#74253,#74254,#74255),(#74256,#74257,
#74258,#74259,#74260),(#74261,#74262,#74263,#74264,#74265)),
 .UNSPECIFIED.,.F.,.F.,.F.)
B_SPLINE_SURFACE_WITH_KNOTS((2,1,2),(3,2,3),(-0.00141401191198245,0.,0.48077029708073),
(0.0365944846645754,0.0384615384615384,0.0431859280915184),
 .UNSPECIFIED.)
GEOMETRIC_REPRESENTATION_ITEM()
RATIONAL_B_SPLINE_SURFACE(((0.999326490452258,0.999646063968217,1.,0.999104400890347,
0.9984288220563),(0.999326490452258,0.999646063968217,1.,0.999104400890347,
0.9984288220563),(0.999326490452258,0.999646063968217,1.,0.999104400890347,
0.9984288220563)))
REPRESENTATION_ITEM('')
SURFACE()
);
#268=(
BOUNDED_SURFACE()
B_SPLINE_SURFACE(1,2,((#74292,#74293,#74294),(#74295,#74296,#74297),(#74298,
#74299,#74300)),.UNSPECIFIED.,.F.,.F.,.F.)
B_SPLINE_SURFACE_WITH_KNOTS((2,1,2),(3,3),(0.,1.,1.01),(0.025590359613179,
0.0375948596693855),.UNSPECIFIED.)
GEOMETRIC_REPRESENTATION_ITEM()
RATIONAL_B_SPLINE_SURFACE(((0.996753121755999,0.997505687613147,0.999678813023853),
(0.996753121755999,0.997505687613147,0.999678813023853),(0.996753121755999,
0.997505687613147,0.999678813023853)))
REPRESENTATION_ITEM('')
SURFACE()
);
#269=(
BOUNDED_SURFACE()
B_SPLINE_SURFACE(1,2,((#74335,#74336,#74337),(#74338,#74339,#74340),(#74341,
#74342,#74343)),.UNSPECIFIED.,.F.,.F.,.F.)
B_SPLINE_SURFACE_WITH_KNOTS((2,1,2),(3,3),(-0.00286823356219737,0.,0.477902879786498),
(0.0265907346180618,0.0331702037252923),.UNSPECIFIED.)
GEOMETRIC_REPRESENTATION_ITEM()
RATIONAL_B_SPLINE_SURFACE(((0.996888414395785,0.997365765479939,0.998269846384985),
(0.996888414395785,0.997365765479939,0.998269846384985),(0.996888414395785,
0.997365765479939,0.998269846384985)))
REPRESENTATION_ITEM('')
SURFACE()
);
#270=(
BOUNDED_SURFACE()
B_SPLINE_SURFACE(1,2,((#74410,#74411,#74412),(#74413,#74414,#74415),(#74416,
#74417,#74418)),.UNSPECIFIED.,.F.,.F.,.F.)
B_SPLINE_SURFACE_WITH_KNOTS((2,1,2),(3,3),(-0.00286753128207131,0.,0.477902879786491),
(0.0166015299238959,0.0231736788111888),.UNSPECIFIED.)
GEOMETRIC_REPRESENTATION_ITEM()
RATIONAL_B_SPLINE_SURFACE(((0.996422581660833,0.996252244737342,0.996507688616404),
(0.996422581660833,0.996252244737342,0.996507688616404),(0.996422581660833,
0.996252244737342,0.996507688616404)))
REPRESENTATION_ITEM('')
SURFACE()
);
#271=(
BOUNDED_SURFACE()
B_SPLINE_SURFACE(1,2,((#74435,#74436,#74437),(#74438,#74439,#74440),(#74441,
#74442,#74443),(#74444,#74445,#74446)),.UNSPECIFIED.,.F.,.F.,.F.)
B_SPLINE_SURFACE_WITH_KNOTS((2,1,1,2),(3,3),(-0.0101,0.,1.,1.01),(0.00560769168370524,
0.0176009700440501),.UNSPECIFIED.)
GEOMETRIC_REPRESENTATION_ITEM()
RATIONAL_B_SPLINE_SURFACE(((0.998183892113821,0.99657330421516,0.996380621259469),
(0.998183892113821,0.99657330421516,0.996380621259469),(0.998183892113821,
0.99657330421516,0.996380621259469),(0.998183892113821,0.99657330421516,
0.996380621259469)))
REPRESENTATION_ITEM('')
SURFACE()
);
#272=(
BOUNDED_SURFACE()
B_SPLINE_SURFACE(1,2,((#74481,#74482,#74483),(#74484,#74485,#74486),(#74487,
#74488,#74489)),.UNSPECIFIED.,.F.,.F.,.F.)
B_SPLINE_SURFACE_WITH_KNOTS((2,1,2),(3,3),(-0.00206901892656846,0.,0.346769728493026),
(0.00660713154720006,0.0131849431469154),.UNSPECIFIED.)
GEOMETRIC_REPRESENTATION_ITEM()
RATIONAL_B_SPLINE_SURFACE(((0.997925307359448,0.997106772384939,0.996714752253857),
(0.997925307359448,0.997106772384939,0.996714752253857),(0.997925307359448,
0.997106772384939,0.996714752253857)))
REPRESENTATION_ITEM('')
SURFACE()
);
#273=(
BOUNDED_SURFACE()
B_SPLINE_SURFACE(1,2,((#74562,#74563,#74564),(#74565,#74566,#74567)),
 .UNSPECIFIED.,.F.,.F.,.F.)
B_SPLINE_SURFACE_WITH_KNOTS((2,2),(3,3),(0.,1.),(0.0556006976418415,0.0675888856590505),
 .UNSPECIFIED.)
GEOMETRIC_REPRESENTATION_ITEM()
RATIONAL_B_SPLINE_SURFACE(((0.996397562408606,0.996150386832629,0.997319912843745),
(0.996397562408606,0.996150386832629,0.997319912843745)))
REPRESENTATION_ITEM('')
SURFACE()
);
#274=(
BOUNDED_SURFACE()
B_SPLINE_SURFACE(1,2,((#74636,#74637,#74638),(#74639,#74640,#74641),(#74642,
#74643,#74644)),.UNSPECIFIED.,.F.,.F.,.F.)
B_SPLINE_SURFACE_WITH_KNOTS((2,1,2),(3,3),(0.,1.,1.01),(0.0456081671210066,
0.0575989447818817),.UNSPECIFIED.)
GEOMETRIC_REPRESENTATION_ITEM()
RATIONAL_B_SPLINE_SURFACE(((0.997793907739636,0.996365558499688,0.996354522974128),
(0.997793907739636,0.996365558499688,0.996354522974128),(0.997793907739636,
0.996365558499688,0.996354522974128)))
REPRESENTATION_ITEM('')
SURFACE()
);
#275=(
BOUNDED_SURFACE()
B_SPLINE_SURFACE(1,2,((#74679,#74680,#74681),(#74682,#74683,#74684),(#74685,
#74686,#74687)),.UNSPECIFIED.,.F.,.F.,.F.)
B_SPLINE_SURFACE_WITH_KNOTS((2,1,2),(3,3),(-0.00286810173489828,0.,0.477902879786517),
(0.0466073985929122,0.0531834929157977),.UNSPECIFIED.)
GEOMETRIC_REPRESENTATION_ITEM()
RATIONAL_B_SPLINE_SURFACE(((0.997565691989291,0.996847118055593,0.996554836292953),
(0.997565691989291,0.996847118055593,0.996554836292953),(0.997565691989291,
0.996847118055593,0.996554836292953)))
REPRESENTATION_ITEM('')
SURFACE()
);
#276=(
BOUNDED_SURFACE()
B_SPLINE_SURFACE(1,2,((#74704,#74705,#74706,#74707,#74708),(#74709,#74710,
#74711,#74712,#74713),(#74714,#74715,#74716,#74717,#74718)),
 .UNSPECIFIED.,.F.,.F.,.F.)
B_SPLINE_SURFACE_WITH_KNOTS((2,1,2),(3,2,3),(0.,1.,1.01),(0.0355931932713902,
0.0384615384615384,0.0476086899858138),.UNSPECIFIED.)
GEOMETRIC_REPRESENTATION_ITEM()
RATIONAL_B_SPLINE_SURFACE(((0.998993602249807,0.999456249886298,1.,0.998265981131401,
0.997356751596327),(0.998993602249807,0.999456249886298,1.,0.998265981131401,
0.997356751596327),(0.998993602249807,0.999456249886298,1.,0.998265981131401,
0.997356751596327)))
REPRESENTATION_ITEM('')
SURFACE()
);
#277=(
BOUNDED_SURFACE()
B_SPLINE_SURFACE(1,2,((#74766,#74767,#74768,#74769,#74770),(#74771,#74772,
#74773,#74774,#74775),(#74776,#74777,#74778,#74779,#74780)),
 .UNSPECIFIED.,.F.,.F.,.F.)
B_SPLINE_SURFACE_WITH_KNOTS((2,1,2),(3,2,3),(-0.00141401191198367,0.,0.480770297080774),
(0.0365944846645756,0.0384615384615384,0.0431859280915187),
 .UNSPECIFIED.)
GEOMETRIC_REPRESENTATION_ITEM()
RATIONAL_B_SPLINE_SURFACE(((0.999326490452259,0.999646063968217,1.,0.999104400890347,
0.9984288220563),(0.999326490452258,0.999646063968217,1.,0.999104400890347,
0.9984288220563),(0.999326490452258,0.999646063968217,1.,0.999104400890347,
0.9984288220563)))
REPRESENTATION_ITEM('')
SURFACE()
);
#278=(
BOUNDED_SURFACE()
B_SPLINE_SURFACE(1,2,((#74807,#74808,#74809),(#74810,#74811,#74812),(#74813,
#74814,#74815)),.UNSPECIFIED.,.F.,.F.,.F.)
B_SPLINE_SURFACE_WITH_KNOTS((2,1,2),(3,3),(0.,1.,1.01),(0.0255903596131811,
0.0375948596693875),.UNSPECIFIED.)
GEOMETRIC_REPRESENTATION_ITEM()
RATIONAL_B_SPLINE_SURFACE(((0.996753121755999,0.997505687613148,0.999678813023853),
(0.996753121755999,0.997505687613148,0.999678813023853),(0.996753121755999,
0.997505687613148,0.999678813023853)))
REPRESENTATION_ITEM('')
SURFACE()
);
#279=(
BOUNDED_SURFACE()
B_SPLINE_SURFACE(1,2,((#74850,#74851,#74852),(#74853,#74854,#74855),(#74856,
#74857,#74858)),.UNSPECIFIED.,.F.,.F.,.F.)
B_SPLINE_SURFACE_WITH_KNOTS((2,1,2),(3,3),(-0.00286823356220283,0.,0.477902879786487),
(0.0265907346180614,0.0331702037252926),.UNSPECIFIED.)
GEOMETRIC_REPRESENTATION_ITEM()
RATIONAL_B_SPLINE_SURFACE(((0.996888414395785,0.997365765479939,0.998269846384985),
(0.996888414395785,0.997365765479939,0.998269846384985),(0.996888414395785,
0.997365765479939,0.998269846384985)))
REPRESENTATION_ITEM('')
SURFACE()
);
#280=(
BOUNDED_SURFACE()
B_SPLINE_SURFACE(1,2,((#74925,#74926,#74927),(#74928,#74929,#74930),(#74931,
#74932,#74933)),.UNSPECIFIED.,.F.,.F.,.F.)
B_SPLINE_SURFACE_WITH_KNOTS((2,1,2),(3,3),(-0.00286753128207528,0.,0.477902879786539),
(0.0166015299238958,0.0231736788111881),.UNSPECIFIED.)
GEOMETRIC_REPRESENTATION_ITEM()
RATIONAL_B_SPLINE_SURFACE(((0.996422581660833,0.996252244737342,0.996507688616404),
(0.996422581660833,0.996252244737342,0.996507688616404),(0.996422581660833,
0.996252244737342,0.996507688616404)))
REPRESENTATION_ITEM('')
SURFACE()
);
#281=(
BOUNDED_SURFACE()
B_SPLINE_SURFACE(1,2,((#74950,#74951,#74952),(#74953,#74954,#74955),(#74956,
#74957,#74958),(#74959,#74960,#74961)),.UNSPECIFIED.,.F.,.F.,.F.)
B_SPLINE_SURFACE_WITH_KNOTS((2,1,1,2),(3,3),(-0.0101,0.,1.,1.01),(0.00560769168370515,
0.0176009700440511),.UNSPECIFIED.)
GEOMETRIC_REPRESENTATION_ITEM()
RATIONAL_B_SPLINE_SURFACE(((0.998183892113821,0.99657330421516,0.996380621259469),
(0.998183892113821,0.99657330421516,0.996380621259469),(0.998183892113821,
0.99657330421516,0.996380621259469),(0.998183892113821,0.99657330421516,
0.996380621259469)))
REPRESENTATION_ITEM('')
SURFACE()
);
#282=(
BOUNDED_SURFACE()
B_SPLINE_SURFACE(1,2,((#74996,#74997,#74998),(#74999,#75000,#75001),(#75002,
#75003,#75004)),.UNSPECIFIED.,.F.,.F.,.F.)
B_SPLINE_SURFACE_WITH_KNOTS((2,1,2),(3,3),(-0.00206901892653575,0.,0.346769728493005),
(0.00660713154719305,0.0131849431468706),.UNSPECIFIED.)
GEOMETRIC_REPRESENTATION_ITEM()
RATIONAL_B_SPLINE_SURFACE(((0.99792530735945,0.997106772384944,0.996714752253862),
(0.99792530735945,0.997106772384944,0.996714752253862),(0.99792530735945,
0.997106772384944,0.996714752253862)))
REPRESENTATION_ITEM('')
SURFACE()
);
#283=(
BOUNDED_SURFACE()
B_SPLINE_SURFACE(1,2,((#75077,#75078,#75079),(#75080,#75081,#75082)),
 .UNSPECIFIED.,.F.,.F.,.F.)
B_SPLINE_SURFACE_WITH_KNOTS((2,2),(3,3),(0.,1.),(0.0556006976418437,0.0675888856590508),
 .UNSPECIFIED.)
GEOMETRIC_REPRESENTATION_ITEM()
RATIONAL_B_SPLINE_SURFACE(((0.996397562408606,0.996150386832629,0.997319912843745),
(0.996397562408606,0.996150386832629,0.997319912843745)))
REPRESENTATION_ITEM('')
SURFACE()
);
#284=(
BOUNDED_SURFACE()
B_SPLINE_SURFACE(1,2,((#75151,#75152,#75153),(#75154,#75155,#75156),(#75157,
#75158,#75159)),.UNSPECIFIED.,.F.,.F.,.F.)
B_SPLINE_SURFACE_WITH_KNOTS((2,1,2),(3,3),(0.,1.,1.01),(0.0456081671210055,
0.0575989447818818),.UNSPECIFIED.)
GEOMETRIC_REPRESENTATION_ITEM()
RATIONAL_B_SPLINE_SURFACE(((0.997793907739636,0.996365558499688,0.996354522974128),
(0.997793907739636,0.996365558499688,0.996354522974128),(0.997793907739636,
0.996365558499688,0.996354522974128)))
REPRESENTATION_ITEM('')
SURFACE()
);
#285=(
BOUNDED_SURFACE()
B_SPLINE_SURFACE(1,2,((#75194,#75195,#75196),(#75197,#75198,#75199),(#75200,
#75201,#75202)),.UNSPECIFIED.,.F.,.F.,.F.)
B_SPLINE_SURFACE_WITH_KNOTS((2,1,2),(3,3),(-0.00286810173486603,0.,0.477902879786523),
(0.0466073985929115,0.0531834929157976),.UNSPECIFIED.)
GEOMETRIC_REPRESENTATION_ITEM()
RATIONAL_B_SPLINE_SURFACE(((0.997565691989291,0.996847118055594,0.996554836292953),
(0.997565691989291,0.996847118055594,0.996554836292953),(0.997565691989291,
0.996847118055594,0.996554836292953)))
REPRESENTATION_ITEM('')
SURFACE()
);
#286=(
BOUNDED_SURFACE()
B_SPLINE_SURFACE(1,2,((#75219,#75220,#75221,#75222,#75223),(#75224,#75225,
#75226,#75227,#75228),(#75229,#75230,#75231,#75232,#75233)),
 .UNSPECIFIED.,.F.,.F.,.F.)
B_SPLINE_SURFACE_WITH_KNOTS((2,1,2),(3,2,3),(0.,1.,1.01),(0.0355931932713902,
0.0384615384615384,0.0476086899858144),.UNSPECIFIED.)
GEOMETRIC_REPRESENTATION_ITEM()
RATIONAL_B_SPLINE_SURFACE(((0.998993602249807,0.999456249886298,1.,0.998265981131401,
0.997356751596327),(0.998993602249807,0.999456249886298,1.,0.998265981131401,
0.997356751596327),(0.998993602249807,0.999456249886298,1.,0.998265981131401,
0.997356751596327)))
REPRESENTATION_ITEM('')
SURFACE()
);
#287=(
BOUNDED_SURFACE()
B_SPLINE_SURFACE(1,2,((#75281,#75282,#75283,#75284,#75285),(#75286,#75287,
#75288,#75289,#75290),(#75291,#75292,#75293,#75294,#75295)),
 .UNSPECIFIED.,.F.,.F.,.F.)
B_SPLINE_SURFACE_WITH_KNOTS((2,1,2),(3,2,3),(-0.00286743098587475,0.,0.480770297146967),
(0.0365944846643704,0.0384615384615384,0.0431859280915192),
 .UNSPECIFIED.)
GEOMETRIC_REPRESENTATION_ITEM()
RATIONAL_B_SPLINE_SURFACE(((0.999326490452188,0.999646063968178,1.,0.999104400890346,
0.9984288220563),(0.999326490452188,0.999646063968178,1.,0.999104400890347,
0.9984288220563),(0.999326490452188,0.999646063968178,1.,0.999104400890347,
0.9984288220563)))
REPRESENTATION_ITEM('')
SURFACE()
);
#288=(
BOUNDED_SURFACE()
B_SPLINE_SURFACE(1,2,((#75322,#75323,#75324),(#75325,#75326,#75327),(#75328,
#75329,#75330)),.UNSPECIFIED.,.F.,.F.,.F.)
B_SPLINE_SURFACE_WITH_KNOTS((2,1,2),(3,3),(0.,1.,1.01),(0.025590359613181,
0.0375948596693885),.UNSPECIFIED.)
GEOMETRIC_REPRESENTATION_ITEM()
RATIONAL_B_SPLINE_SURFACE(((0.996753121755999,0.997505687613148,0.999678813023854),
(0.996753121755999,0.997505687613148,0.999678813023854),(0.996753121755999,
0.997505687613148,0.999678813023854)))
REPRESENTATION_ITEM('')
SURFACE()
);
#289=(
BOUNDED_SURFACE()
B_SPLINE_SURFACE(1,2,((#75365,#75366,#75367),(#75368,#75369,#75370),(#75371,
#75372,#75373)),.UNSPECIFIED.,.F.,.F.,.F.)
B_SPLINE_SURFACE_WITH_KNOTS((2,1,2),(3,3),(-0.00286823356216702,0.,0.477902879786504),
(0.0265907346180616,0.0331702037252923),.UNSPECIFIED.)
GEOMETRIC_REPRESENTATION_ITEM()
RATIONAL_B_SPLINE_SURFACE(((0.996888414395785,0.997365765479939,0.998269846384985),
(0.996888414395785,0.997365765479939,0.998269846384985),(0.996888414395785,
0.997365765479939,0.998269846384985)))
REPRESENTATION_ITEM('')
SURFACE()
);
#290=(
BOUNDED_SURFACE()
B_SPLINE_SURFACE(1,2,((#75440,#75441,#75442),(#75443,#75444,#75445),(#75446,
#75447,#75448)),.UNSPECIFIED.,.F.,.F.,.F.)
B_SPLINE_SURFACE_WITH_KNOTS((2,1,2),(3,3),(-0.00286753128206841,0.,0.477902879786505),
(0.0166015299238955,0.0231736788111888),.UNSPECIFIED.)
GEOMETRIC_REPRESENTATION_ITEM()
RATIONAL_B_SPLINE_SURFACE(((0.996422581660833,0.996252244737341,0.996507688616404),
(0.996422581660833,0.996252244737341,0.996507688616404),(0.996422581660833,
0.996252244737341,0.996507688616404)))
REPRESENTATION_ITEM('')
SURFACE()
);
#291=(
BOUNDED_SURFACE()
B_SPLINE_SURFACE(1,2,((#75465,#75466,#75467),(#75468,#75469,#75470),(#75471,
#75472,#75473),(#75474,#75475,#75476)),.UNSPECIFIED.,.F.,.F.,.F.)
B_SPLINE_SURFACE_WITH_KNOTS((2,1,1,2),(3,3),(-0.0101,0.,1.,1.01),(0.00560769168370622,
0.0176009700440522),.UNSPECIFIED.)
GEOMETRIC_REPRESENTATION_ITEM()
RATIONAL_B_SPLINE_SURFACE(((0.99818389211382,0.99657330421516,0.996380621259469),
(0.99818389211382,0.99657330421516,0.996380621259469),(0.99818389211382,
0.99657330421516,0.996380621259469),(0.99818389211382,0.99657330421516,
0.996380621259469)))
REPRESENTATION_ITEM('')
SURFACE()
);
#292=(
BOUNDED_SURFACE()
B_SPLINE_SURFACE(1,2,((#75511,#75512,#75513),(#75514,#75515,#75516),(#75517,
#75518,#75519)),.UNSPECIFIED.,.F.,.F.,.F.)
B_SPLINE_SURFACE_WITH_KNOTS((2,1,2),(3,3),(-0.00206901892646732,0.,0.346769728493036),
(0.00660713154718544,0.013184943146879),.UNSPECIFIED.)
GEOMETRIC_REPRESENTATION_ITEM()
RATIONAL_B_SPLINE_SURFACE(((0.997925307359452,0.997106772384944,0.996714752253861),
(0.997925307359452,0.997106772384944,0.996714752253861),(0.997925307359452,
0.997106772384944,0.996714752253861)))
REPRESENTATION_ITEM('')
SURFACE()
);
#293=(
BOUNDED_SURFACE()
B_SPLINE_SURFACE(1,2,((#75592,#75593,#75594),(#75595,#75596,#75597)),
 .UNSPECIFIED.,.F.,.F.,.F.)
B_SPLINE_SURFACE_WITH_KNOTS((2,2),(3,3),(0.,1.),(0.0556006976418415,0.0675888856590505),
 .UNSPECIFIED.)
GEOMETRIC_REPRESENTATION_ITEM()
RATIONAL_B_SPLINE_SURFACE(((0.996397562408606,0.996150386832629,0.997319912843745),
(0.996397562408606,0.996150386832629,0.997319912843745)))
REPRESENTATION_ITEM('')
SURFACE()
);
#294=(
BOUNDED_SURFACE()
B_SPLINE_SURFACE(1,2,((#75666,#75667,#75668),(#75669,#75670,#75671)),
 .UNSPECIFIED.,.F.,.F.,.F.)
B_SPLINE_SURFACE_WITH_KNOTS((2,2),(3,3),(0.,1.),(0.0456081671210054,0.0575989447818824),
 .UNSPECIFIED.)
GEOMETRIC_REPRESENTATION_ITEM()
RATIONAL_B_SPLINE_SURFACE(((0.997793907739636,0.996365558499688,0.996354522974128),
(0.997793907739636,0.996365558499688,0.996354522974128)))
REPRESENTATION_ITEM('')
SURFACE()
);
#295=(
BOUNDED_SURFACE()
B_SPLINE_SURFACE(1,2,((#75738,#75739,#75740,#75741,#75742),(#75743,#75744,
#75745,#75746,#75747),(#75748,#75749,#75750,#75751,#75752)),
 .UNSPECIFIED.,.F.,.F.,.F.)
B_SPLINE_SURFACE_WITH_KNOTS((2,1,2),(3,2,3),(0.,1.,1.01),(0.0355931932713902,
0.0384615384615384,0.0476086899858138),.UNSPECIFIED.)
GEOMETRIC_REPRESENTATION_ITEM()
RATIONAL_B_SPLINE_SURFACE(((0.998993602249807,0.999456249886298,1.,0.998265981131401,
0.997356751596327),(0.998993602249807,0.999456249886298,1.,0.998265981131401,
0.997356751596327),(0.998993602249807,0.999456249886298,1.,0.998265981131401,
0.997356751596327)))
REPRESENTATION_ITEM('')
SURFACE()
);
#296=(
BOUNDED_SURFACE()
B_SPLINE_SURFACE(1,2,((#75800,#75801,#75802,#75803,#75804),(#75805,#75806,
#75807,#75808,#75809),(#75810,#75811,#75812,#75813,#75814)),
 .UNSPECIFIED.,.F.,.F.,.F.)
B_SPLINE_SURFACE_WITH_KNOTS((2,1,2),(3,2,3),(-0.00141401191198346,0.,0.480770297080816),
(0.0365944846645752,0.0384615384615384,0.0431859280915184),
 .UNSPECIFIED.)
GEOMETRIC_REPRESENTATION_ITEM()
RATIONAL_B_SPLINE_SURFACE(((0.999326490452258,0.999646063968217,1.,0.999104400890347,
0.9984288220563),(0.999326490452258,0.999646063968217,1.,0.999104400890347,
0.9984288220563),(0.999326490452258,0.999646063968217,1.,0.999104400890347,
0.9984288220563)))
REPRESENTATION_ITEM('')
SURFACE()
);
#297=(
BOUNDED_SURFACE()
B_SPLINE_SURFACE(1,2,((#75841,#75842,#75843),(#75844,#75845,#75846),(#75847,
#75848,#75849)),.UNSPECIFIED.,.F.,.F.,.F.)
B_SPLINE_SURFACE_WITH_KNOTS((2,1,2),(3,3),(0.,1.,1.01),(0.025590359613181,
0.0375948596693879),.UNSPECIFIED.)
GEOMETRIC_REPRESENTATION_ITEM()
RATIONAL_B_SPLINE_SURFACE(((0.996753121755999,0.997505687613148,0.999678813023854),
(0.996753121755999,0.997505687613148,0.999678813023854),(0.996753121755999,
0.997505687613148,0.999678813023854)))
REPRESENTATION_ITEM('')
SURFACE()
);
#298=(
BOUNDED_SURFACE()
B_SPLINE_SURFACE(1,2,((#75884,#75885,#75886),(#75887,#75888,#75889),(#75890,
#75891,#75892)),.UNSPECIFIED.,.F.,.F.,.F.)
B_SPLINE_SURFACE_WITH_KNOTS((2,1,2),(3,3),(-0.00286823045904505,0.,0.477902879786501),
(0.0265907346180621,0.0331702036774533),.UNSPECIFIED.)
GEOMETRIC_REPRESENTATION_ITEM()
RATIONAL_B_SPLINE_SURFACE(((0.996888414395786,0.997365765476469,0.998269846371839),
(0.996888414395786,0.997365765476469,0.998269846371839),(0.996888414395786,
0.997365765476469,0.998269846371839)))
REPRESENTATION_ITEM('')
SURFACE()
);
#299=(
BOUNDED_SURFACE()
B_SPLINE_SURFACE(1,2,((#75959,#75960,#75961),(#75962,#75963,#75964),(#75965,
#75966,#75967)),.UNSPECIFIED.,.F.,.F.,.F.)
B_SPLINE_SURFACE_WITH_KNOTS((2,1,2),(3,3),(-0.00286753128206318,0.,0.477902879786521),
(0.0166015299238956,0.0231736788111887),.UNSPECIFIED.)
GEOMETRIC_REPRESENTATION_ITEM()
RATIONAL_B_SPLINE_SURFACE(((0.996422581660833,0.996252244737341,0.996507688616404),
(0.996422581660833,0.996252244737341,0.996507688616404),(0.996422581660833,
0.996252244737341,0.996507688616404)))
REPRESENTATION_ITEM('')
SURFACE()
);
#300=(
BOUNDED_SURFACE()
B_SPLINE_SURFACE(1,2,((#75984,#75985,#75986),(#75987,#75988,#75989),(#75990,
#75991,#75992),(#75993,#75994,#75995)),.UNSPECIFIED.,.F.,.F.,.F.)
B_SPLINE_SURFACE_WITH_KNOTS((2,1,1,2),(3,3),(-0.0101,0.,1.,1.01),(0.00560769168370531,
0.0176009700440517),.UNSPECIFIED.)
GEOMETRIC_REPRESENTATION_ITEM()
RATIONAL_B_SPLINE_SURFACE(((0.998183892113821,0.99657330421516,0.996380621259469),
(0.998183892113821,0.99657330421516,0.996380621259469),(0.998183892113821,
0.99657330421516,0.996380621259469),(0.998183892113821,0.99657330421516,
0.996380621259469)))
REPRESENTATION_ITEM('')
SURFACE()
);
#301=(
BOUNDED_SURFACE()
B_SPLINE_SURFACE(1,2,((#76030,#76031,#76032),(#76033,#76034,#76035),(#76036,
#76037,#76038)),.UNSPECIFIED.,.F.,.F.,.F.)
B_SPLINE_SURFACE_WITH_KNOTS((2,1,2),(3,3),(-0.00206901892640366,0.,0.346769728493003),
(0.00660713154717563,0.013184943146939),.UNSPECIFIED.)
GEOMETRIC_REPRESENTATION_ITEM()
RATIONAL_B_SPLINE_SURFACE(((0.997925307359454,0.997106772384937,0.996714752253855),
(0.997925307359454,0.997106772384937,0.996714752253855),(0.997925307359454,
0.997106772384937,0.996714752253854)))
REPRESENTATION_ITEM('')
SURFACE()
);
#302=(
BOUNDED_SURFACE()
B_SPLINE_SURFACE(1,2,((#76111,#76112,#76113),(#76114,#76115,#76116)),
 .UNSPECIFIED.,.F.,.F.,.F.)
B_SPLINE_SURFACE_WITH_KNOTS((2,2),(3,3),(0.,1.),(0.0556006976418414,0.0675888856590511),
 .UNSPECIFIED.)
GEOMETRIC_REPRESENTATION_ITEM()
RATIONAL_B_SPLINE_SURFACE(((0.996397562408606,0.996150386832629,0.997319912843745),
(0.996397562408606,0.996150386832629,0.997319912843745)))
REPRESENTATION_ITEM('')
SURFACE()
);
#303=(
BOUNDED_SURFACE()
B_SPLINE_SURFACE(1,2,((#76185,#76186,#76187),(#76188,#76189,#76190),(#76191,
#76192,#76193)),.UNSPECIFIED.,.F.,.F.,.F.)
B_SPLINE_SURFACE_WITH_KNOTS((2,1,2),(3,3),(0.,1.,1.01),(0.0456081671210045,
0.0575989447818814),.UNSPECIFIED.)
GEOMETRIC_REPRESENTATION_ITEM()
RATIONAL_B_SPLINE_SURFACE(((0.997793907739636,0.996365558499688,0.996354522974128),
(0.997793907739636,0.996365558499688,0.996354522974128),(0.997793907739636,
0.996365558499688,0.996354522974128)))
REPRESENTATION_ITEM('')
SURFACE()
);
#304=(
BOUNDED_SURFACE()
B_SPLINE_SURFACE(1,2,((#76228,#76229,#76230),(#76231,#76232,#76233),(#76234,
#76235,#76236)),.UNSPECIFIED.,.F.,.F.,.F.)
B_SPLINE_SURFACE_WITH_KNOTS((2,1,2),(3,3),(-0.00286810173474343,0.,0.477902879786529),
(0.0466073985929116,0.0531834929157972),.UNSPECIFIED.)
GEOMETRIC_REPRESENTATION_ITEM()
RATIONAL_B_SPLINE_SURFACE(((0.997565691989291,0.996847118055594,0.996554836292953),
(0.997565691989291,0.996847118055594,0.996554836292953),(0.997565691989291,
0.996847118055594,0.996554836292953)))
REPRESENTATION_ITEM('')
SURFACE()
);
#305=(
BOUNDED_SURFACE()
B_SPLINE_SURFACE(1,2,((#76314,#76315,#76316,#76317,#76318),(#76319,#76320,
#76321,#76322,#76323)),.UNSPECIFIED.,.F.,.F.,.F.)
B_SPLINE_SURFACE_WITH_KNOTS((2,2),(3,2,3),(0.,0.480770297080784),(0.0365944846645756,
0.0384615384615384,0.0431859280915184),.UNSPECIFIED.)
GEOMETRIC_REPRESENTATION_ITEM()
RATIONAL_B_SPLINE_SURFACE(((0.999326490452258,0.999646063968217,1.,0.999104400890347,
0.9984288220563),(0.999326490452258,0.999646063968217,1.,0.999104400890347,
0.9984288220563)))
REPRESENTATION_ITEM('')
SURFACE()
);
#306=(
BOUNDED_SURFACE()
B_SPLINE_SURFACE(1,2,((#76350,#76351,#76352),(#76353,#76354,#76355),(#76356,
#76357,#76358)),.UNSPECIFIED.,.F.,.F.,.F.)
B_SPLINE_SURFACE_WITH_KNOTS((2,1,2),(3,3),(0.,1.,1.01),(0.02559035961318,
0.0375948596693876),.UNSPECIFIED.)
GEOMETRIC_REPRESENTATION_ITEM()
RATIONAL_B_SPLINE_SURFACE(((0.996753121755999,0.997505687613148,0.999678813023853),
(0.996753121755999,0.997505687613148,0.999678813023853),(0.996753121755999,
0.997505687613148,0.999678813023853)))
REPRESENTATION_ITEM('')
SURFACE()
);
#307=(
BOUNDED_SURFACE()
B_SPLINE_SURFACE(1,2,((#76393,#76394,#76395),(#76396,#76397,#76398),(#76399,
#76400,#76401)),.UNSPECIFIED.,.F.,.F.,.F.)
B_SPLINE_SURFACE_WITH_KNOTS((2,1,2),(3,3),(-0.00286823045901626,0.,0.47790287978655),
(0.0265907346180616,0.0331702036774535),.UNSPECIFIED.)
GEOMETRIC_REPRESENTATION_ITEM()
RATIONAL_B_SPLINE_SURFACE(((0.996888414395785,0.997365765476469,0.998269846371839),
(0.996888414395785,0.997365765476469,0.998269846371838),(0.996888414395785,
0.997365765476469,0.998269846371838)))
REPRESENTATION_ITEM('')
SURFACE()
);
#308=(
BOUNDED_SURFACE()
B_SPLINE_SURFACE(1,2,((#76468,#76469,#76470),(#76471,#76472,#76473),(#76474,
#76475,#76476)),.UNSPECIFIED.,.F.,.F.,.F.)
B_SPLINE_SURFACE_WITH_KNOTS((2,1,2),(3,3),(-0.00286753128201114,0.,0.477902879786504),
(0.0166015299238954,0.0231736788111883),.UNSPECIFIED.)
GEOMETRIC_REPRESENTATION_ITEM()
RATIONAL_B_SPLINE_SURFACE(((0.996422581660833,0.996252244737342,0.996507688616404),
(0.996422581660833,0.996252244737342,0.996507688616404),(0.996422581660833,
0.996252244737342,0.996507688616404)))
REPRESENTATION_ITEM('')
SURFACE()
);
#309=(
BOUNDED_SURFACE()
B_SPLINE_SURFACE(1,2,((#76493,#76494,#76495),(#76496,#76497,#76498),(#76499,
#76500,#76501),(#76502,#76503,#76504)),.UNSPECIFIED.,.F.,.F.,.F.)
B_SPLINE_SURFACE_WITH_KNOTS((2,1,1,2),(3,3),(-0.0101,0.,1.,1.01),(0.00560769168370589,
0.0176009700440522),.UNSPECIFIED.)
GEOMETRIC_REPRESENTATION_ITEM()
RATIONAL_B_SPLINE_SURFACE(((0.99818389211382,0.99657330421516,0.996380621259469),
(0.99818389211382,0.99657330421516,0.996380621259469),(0.99818389211382,
0.99657330421516,0.996380621259469),(0.99818389211382,0.99657330421516,
0.996380621259469)))
REPRESENTATION_ITEM('')
SURFACE()
);
#310=(
BOUNDED_SURFACE()
B_SPLINE_SURFACE(1,2,((#76539,#76540,#76541),(#76542,#76543,#76544),(#76545,
#76546,#76547)),.UNSPECIFIED.,.F.,.F.,.F.)
B_SPLINE_SURFACE_WITH_KNOTS((2,1,2),(3,3),(-0.00206901892635118,0.,0.346769728493102),
(0.00660713154716551,0.0131849431469464),.UNSPECIFIED.)
GEOMETRIC_REPRESENTATION_ITEM()
RATIONAL_B_SPLINE_SURFACE(((0.997925307359457,0.997106772384937,0.996714752253854),
(0.997925307359457,0.997106772384937,0.996714752253854),(0.997925307359457,
0.997106772384937,0.996714752253854)))
REPRESENTATION_ITEM('')
SURFACE()
);
#311=(
BOUNDED_SURFACE()
B_SPLINE_SURFACE(1,2,((#76620,#76621,#76622),(#76623,#76624,#76625)),
 .UNSPECIFIED.,.F.,.F.,.F.)
B_SPLINE_SURFACE_WITH_KNOTS((2,2),(3,3),(0.,1.),(0.0556006976418414,0.0675888856590506),
 .UNSPECIFIED.)
GEOMETRIC_REPRESENTATION_ITEM()
RATIONAL_B_SPLINE_SURFACE(((0.996397562408606,0.996150386832629,0.997319912843745),
(0.996397562408606,0.996150386832629,0.997319912843745)))
REPRESENTATION_ITEM('')
SURFACE()
);
#312=(
BOUNDED_SURFACE()
B_SPLINE_SURFACE(1,2,((#76694,#76695,#76696),(#76697,#76698,#76699)),
 .UNSPECIFIED.,.F.,.F.,.F.)
B_SPLINE_SURFACE_WITH_KNOTS((2,2),(3,3),(0.,1.),(0.0456081671210044,0.0575989447818824),
 .UNSPECIFIED.)
GEOMETRIC_REPRESENTATION_ITEM()
RATIONAL_B_SPLINE_SURFACE(((0.997793907739636,0.996365558499688,0.996354522974128),
(0.997793907739636,0.996365558499688,0.996354522974128)))
REPRESENTATION_ITEM('')
SURFACE()
);
#313=(
BOUNDED_SURFACE()
B_SPLINE_SURFACE(1,2,((#76766,#76767,#76768,#76769,#76770),(#76771,#76772,
#76773,#76774,#76775),(#76776,#76777,#76778,#76779,#76780)),
 .UNSPECIFIED.,.F.,.F.,.F.)
B_SPLINE_SURFACE_WITH_KNOTS((2,1,2),(3,2,3),(0.,1.,1.01),(0.0355931932713903,
0.0384615384615384,0.0476086899858133),.UNSPECIFIED.)
GEOMETRIC_REPRESENTATION_ITEM()
RATIONAL_B_SPLINE_SURFACE(((0.998993602249807,0.999456249886298,1.,0.998265981131401,
0.997356751596327),(0.998993602249807,0.999456249886298,1.,0.998265981131401,
0.997356751596327),(0.998993602249807,0.999456249886298,1.,0.998265981131401,
0.997356751596327)))
REPRESENTATION_ITEM('')
SURFACE()
);
#314=(
BOUNDED_SURFACE()
B_SPLINE_SURFACE(1,2,((#76828,#76829,#76830,#76831,#76832),(#76833,#76834,
#76835,#76836,#76837),(#76838,#76839,#76840,#76841,#76842)),
 .UNSPECIFIED.,.F.,.F.,.F.)
B_SPLINE_SURFACE_WITH_KNOTS((2,1,2),(3,2,3),(-0.00286743098833038,0.,0.480770297147049),
(0.0365944846643319,0.0384615384615384,0.0431859280915196),
 .UNSPECIFIED.)
GEOMETRIC_REPRESENTATION_ITEM()
RATIONAL_B_SPLINE_SURFACE(((0.999326490452175,0.99964606396817,1.,0.999104400890347,
0.9984288220563),(0.999326490452175,0.99964606396817,1.,0.999104400890347,
0.9984288220563),(0.999326490452175,0.99964606396817,1.,0.999104400890347,
0.9984288220563)))
REPRESENTATION_ITEM('')
SURFACE()
);
#315=(
BOUNDED_SURFACE()
B_SPLINE_SURFACE(1,2,((#76869,#76870,#76871),(#76872,#76873,#76874)),
 .UNSPECIFIED.,.F.,.F.,.F.)
B_SPLINE_SURFACE_WITH_KNOTS((2,2),(3,3),(0.,1.),(0.0255903596131787,0.0375948596693877),
 .UNSPECIFIED.)
GEOMETRIC_REPRESENTATION_ITEM()
RATIONAL_B_SPLINE_SURFACE(((0.996753121755999,0.997505687613147,0.999678813023853),
(0.996753121755999,0.997505687613147,0.999678813023853)))
REPRESENTATION_ITEM('')
SURFACE()
);
#316=(
BOUNDED_SURFACE()
B_SPLINE_SURFACE(1,2,((#76991,#76992,#76993),(#76994,#76995,#76996),(#76997,
#76998,#76999)),.UNSPECIFIED.,.F.,.F.,.F.)
B_SPLINE_SURFACE_WITH_KNOTS((2,1,2),(3,3),(-0.00286753114038783,0.,0.477902879786557),
(0.0166015299238959,0.0231736788090033),.UNSPECIFIED.)
GEOMETRIC_REPRESENTATION_ITEM()
RATIONAL_B_SPLINE_SURFACE(((0.996422581660833,0.996252244737399,0.996507688616235),
(0.996422581660833,0.996252244737399,0.996507688616235),(0.996422581660833,
0.996252244737399,0.996507688616235)))
REPRESENTATION_ITEM('')
SURFACE()
);
#317=(
BOUNDED_SURFACE()
B_SPLINE_SURFACE(1,2,((#77016,#77017,#77018),(#77019,#77020,#77021),(#77022,
#77023,#77024),(#77025,#77026,#77027)),.UNSPECIFIED.,.F.,.F.,.F.)
B_SPLINE_SURFACE_WITH_KNOTS((2,1,1,2),(3,3),(-0.0101,0.,1.,1.01),(0.00560769168370523,
0.0176009700440517),.UNSPECIFIED.)
GEOMETRIC_REPRESENTATION_ITEM()
RATIONAL_B_SPLINE_SURFACE(((0.99818389211382,0.99657330421516,0.996380621259469),
(0.99818389211382,0.99657330421516,0.996380621259469),(0.99818389211382,
0.99657330421516,0.996380621259469),(0.99818389211382,0.99657330421516,
0.996380621259469)))
REPRESENTATION_ITEM('')
SURFACE()
);
#318=(
BOUNDED_SURFACE()
B_SPLINE_SURFACE(1,2,((#77062,#77063,#77064),(#77065,#77066,#77067),(#77068,
#77069,#77070)),.UNSPECIFIED.,.F.,.F.,.F.)
B_SPLINE_SURFACE_WITH_KNOTS((2,1,2),(3,3),(-0.0020690189263002,0.,0.346769728493041),
(0.00660713154715324,0.0131849431469514),.UNSPECIFIED.)
GEOMETRIC_REPRESENTATION_ITEM()
RATIONAL_B_SPLINE_SURFACE(((0.99792530735946,0.997106772384937,0.996714752253853),
(0.99792530735946,0.997106772384937,0.996714752253853),(0.99792530735946,
0.997106772384937,0.996714752253853)))
REPRESENTATION_ITEM('')
SURFACE()
);
#319=(
BOUNDED_SURFACE()
B_SPLINE_SURFACE(1,2,((#77143,#77144,#77145),(#77146,#77147,#77148)),
 .UNSPECIFIED.,.F.,.F.,.F.)
B_SPLINE_SURFACE_WITH_KNOTS((2,2),(3,3),(0.,1.),(0.0556006976418415,0.06758888565905),
 .UNSPECIFIED.)
GEOMETRIC_REPRESENTATION_ITEM()
RATIONAL_B_SPLINE_SURFACE(((0.996397562408606,0.996150386832629,0.997319912843745),
(0.996397562408606,0.996150386832629,0.997319912843745)))
REPRESENTATION_ITEM('')
SURFACE()
);
#320=(
BOUNDED_SURFACE()
B_SPLINE_SURFACE(1,2,((#77217,#77218,#77219),(#77220,#77221,#77222),(#77223,
#77224,#77225)),.UNSPECIFIED.,.F.,.F.,.F.)
B_SPLINE_SURFACE_WITH_KNOTS((2,1,2),(3,3),(0.,1.,1.01),(0.0456081671210055,
0.0575989447818818),.UNSPECIFIED.)
GEOMETRIC_REPRESENTATION_ITEM()
RATIONAL_B_SPLINE_SURFACE(((0.997793907739636,0.996365558499688,0.996354522974128),
(0.997793907739636,0.996365558499688,0.996354522974128),(0.997793907739636,
0.996365558499688,0.996354522974128)))
REPRESENTATION_ITEM('')
SURFACE()
);
#321=(
BOUNDED_SURFACE()
B_SPLINE_SURFACE(1,2,((#77260,#77261,#77262),(#77263,#77264,#77265),(#77266,
#77267,#77268)),.UNSPECIFIED.,.F.,.F.,.F.)
B_SPLINE_SURFACE_WITH_KNOTS((2,1,2),(3,3),(-0.00286810173465011,0.,0.477902879786603),
(0.0466073985929122,0.0531834929157972),.UNSPECIFIED.)
GEOMETRIC_REPRESENTATION_ITEM()
RATIONAL_B_SPLINE_SURFACE(((0.997565691989291,0.996847118055594,0.996554836292953),
(0.997565691989291,0.996847118055594,0.996554836292953),(0.997565691989291,
0.996847118055594,0.996554836292953)))
REPRESENTATION_ITEM('')
SURFACE()
);
#322=(
BOUNDED_SURFACE()
B_SPLINE_SURFACE(1,2,((#77285,#77286,#77287,#77288,#77289),(#77290,#77291,
#77292,#77293,#77294),(#77295,#77296,#77297,#77298,#77299)),
 .UNSPECIFIED.,.F.,.F.,.F.)
B_SPLINE_SURFACE_WITH_KNOTS((2,1,2),(3,2,3),(0.,1.,1.01),(0.0355931932713912,
0.0384615384615384,0.0476086899858135),.UNSPECIFIED.)
GEOMETRIC_REPRESENTATION_ITEM()
RATIONAL_B_SPLINE_SURFACE(((0.998993602249807,0.999456249886298,1.,0.998265981131401,
0.997356751596327),(0.998993602249807,0.999456249886298,1.,0.998265981131401,
0.997356751596327),(0.998993602249807,0.999456249886298,1.,0.998265981131401,
0.997356751596327)))
REPRESENTATION_ITEM('')
SURFACE()
);
#323=(
BOUNDED_SURFACE()
B_SPLINE_SURFACE(1,2,((#77347,#77348,#77349,#77350,#77351),(#77352,#77353,
#77354,#77355,#77356),(#77357,#77358,#77359,#77360,#77361)),
 .UNSPECIFIED.,.F.,.F.,.F.)
B_SPLINE_SURFACE_WITH_KNOTS((2,1,2),(3,2,3),(-0.00286743098864766,0.,0.480770297147027),
(0.0365944846643192,0.0384615384615384,0.0431859280915204),
 .UNSPECIFIED.)
GEOMETRIC_REPRESENTATION_ITEM()
RATIONAL_B_SPLINE_SURFACE(((0.999326490452171,0.999646063968168,1.,0.999104400890346,
0.998428822056299),(0.999326490452171,0.999646063968168,1.,0.999104400890346,
0.998428822056299),(0.999326490452171,0.999646063968168,1.,0.999104400890346,
0.998428822056299)))
REPRESENTATION_ITEM('')
SURFACE()
);
#324=(
BOUNDED_SURFACE()
B_SPLINE_SURFACE(1,2,((#77388,#77389,#77390),(#77391,#77392,#77393),(#77394,
#77395,#77396)),.UNSPECIFIED.,.F.,.F.,.F.)
B_SPLINE_SURFACE_WITH_KNOTS((2,1,2),(3,3),(0.,1.,1.01),(0.02559035961318,
0.0375948596693866),.UNSPECIFIED.)
GEOMETRIC_REPRESENTATION_ITEM()
RATIONAL_B_SPLINE_SURFACE(((0.996753121755999,0.997505687613148,0.999678813023853),
(0.996753121755999,0.997505687613148,0.999678813023853),(0.996753121755999,
0.997505687613148,0.999678813023853)))
REPRESENTATION_ITEM('')
SURFACE()
);
#325=(
BOUNDED_SURFACE()
B_SPLINE_SURFACE(1,2,((#77431,#77432,#77433),(#77434,#77435,#77436),(#77437,
#77438,#77439)),.UNSPECIFIED.,.F.,.F.,.F.)
B_SPLINE_SURFACE_WITH_KNOTS((2,1,2),(3,3),(-0.00286823356211481,0.,0.477902879786507),
(0.0265907346180626,0.0331702037252924),.UNSPECIFIED.)
GEOMETRIC_REPRESENTATION_ITEM()
RATIONAL_B_SPLINE_SURFACE(((0.996888414395785,0.997365765479939,0.998269846384985),
(0.996888414395785,0.997365765479939,0.998269846384985),(0.996888414395785,
0.997365765479939,0.998269846384985)))
REPRESENTATION_ITEM('')
SURFACE()
);
#326=(
BOUNDED_SURFACE()
B_SPLINE_SURFACE(1,2,((#77538,#77539,#77540),(#77541,#77542,#77543),(#77544,
#77545,#77546),(#77547,#77548,#77549)),.UNSPECIFIED.,.F.,.F.,.F.)
B_SPLINE_SURFACE_WITH_KNOTS((2,1,1,2),(3,3),(-0.0101,0.,1.,1.01),(0.00560769168370627,
0.0176009700440506),.UNSPECIFIED.)
GEOMETRIC_REPRESENTATION_ITEM()
RATIONAL_B_SPLINE_SURFACE(((0.99818389211382,0.99657330421516,0.996380621259469),
(0.99818389211382,0.99657330421516,0.996380621259469),(0.99818389211382,
0.99657330421516,0.996380621259469),(0.99818389211382,0.99657330421516,
0.996380621259469)))
REPRESENTATION_ITEM('')
SURFACE()
);
#327=(
BOUNDED_SURFACE()
B_SPLINE_SURFACE(1,2,((#77584,#77585,#77586),(#77587,#77588,#77589),(#77590,
#77591,#77592)),.UNSPECIFIED.,.F.,.F.,.F.)
B_SPLINE_SURFACE_WITH_KNOTS((2,1,2),(3,3),(-0.00206901892627739,0.,0.346769728493106),
(0.00660713154713986,0.013184943146955),.UNSPECIFIED.)
GEOMETRIC_REPRESENTATION_ITEM()
RATIONAL_B_SPLINE_SURFACE(((0.997925307359463,0.997106772384937,0.996714752253853),
(0.997925307359463,0.997106772384937,0.996714752253853),(0.997925307359463,
0.997106772384937,0.996714752253853)))
REPRESENTATION_ITEM('')
SURFACE()
);
#328=(
BOUNDED_SURFACE()
B_SPLINE_SURFACE(1,2,((#77665,#77666,#77667),(#77668,#77669,#77670)),
 .UNSPECIFIED.,.F.,.F.,.F.)
B_SPLINE_SURFACE_WITH_KNOTS((2,2),(3,3),(0.,1.),(0.0556006976418401,0.0675888856590505),
 .UNSPECIFIED.)
GEOMETRIC_REPRESENTATION_ITEM()
RATIONAL_B_SPLINE_SURFACE(((0.996397562408606,0.996150386832629,0.997319912843745),
(0.996397562408606,0.996150386832629,0.997319912843745)))
REPRESENTATION_ITEM('')
SURFACE()
);
#329=(
BOUNDED_SURFACE()
B_SPLINE_SURFACE(1,2,((#77739,#77740,#77741),(#77742,#77743,#77744),(#77745,
#77746,#77747)),.UNSPECIFIED.,.F.,.F.,.F.)
B_SPLINE_SURFACE_WITH_KNOTS((2,1,2),(3,3),(0.,1.,1.01),(0.0456081671210034,
0.0575989447818819),.UNSPECIFIED.)
GEOMETRIC_REPRESENTATION_ITEM()
RATIONAL_B_SPLINE_SURFACE(((0.997793907739636,0.996365558499688,0.996354522974128),
(0.997793907739636,0.996365558499688,0.996354522974128),(0.997793907739636,
0.996365558499688,0.996354522974128)))
REPRESENTATION_ITEM('')
SURFACE()
);
#330=(
BOUNDED_SURFACE()
B_SPLINE_SURFACE(1,2,((#77782,#77783,#77784),(#77785,#77786,#77787),(#77788,
#77789,#77790)),.UNSPECIFIED.,.F.,.F.,.F.)
B_SPLINE_SURFACE_WITH_KNOTS((2,1,2),(3,3),(-0.00286810173460448,0.,0.477902879786547),
(0.0466073985929112,0.0531834929157984),.UNSPECIFIED.)
GEOMETRIC_REPRESENTATION_ITEM()
RATIONAL_B_SPLINE_SURFACE(((0.997565691989291,0.996847118055593,0.996554836292953),
(0.997565691989291,0.996847118055593,0.996554836292953),(0.997565691989291,
0.996847118055593,0.996554836292953)))
REPRESENTATION_ITEM('')
SURFACE()
);
#331=(
BOUNDED_SURFACE()
B_SPLINE_SURFACE(1,2,((#77807,#77808,#77809,#77810,#77811),(#77812,#77813,
#77814,#77815,#77816),(#77817,#77818,#77819,#77820,#77821)),
 .UNSPECIFIED.,.F.,.F.,.F.)
B_SPLINE_SURFACE_WITH_KNOTS((2,1,2),(3,2,3),(0.,1.,1.01),(0.0355931932713902,
0.0384615384615384,0.0476086899858139),.UNSPECIFIED.)
GEOMETRIC_REPRESENTATION_ITEM()
RATIONAL_B_SPLINE_SURFACE(((0.998993602249807,0.999456249886298,1.,0.998265981131401,
0.997356751596327),(0.998993602249807,0.999456249886298,1.,0.998265981131401,
0.997356751596327),(0.998993602249807,0.999456249886298,1.,0.998265981131401,
0.997356751596327)))
REPRESENTATION_ITEM('')
SURFACE()
);
#332=(
BOUNDED_SURFACE()
B_SPLINE_SURFACE(1,2,((#77869,#77870,#77871,#77872,#77873),(#77874,#77875,
#77876,#77877,#77878),(#77879,#77880,#77881,#77882,#77883)),
 .UNSPECIFIED.,.F.,.F.,.F.)
B_SPLINE_SURFACE_WITH_KNOTS((2,1,2),(3,2,3),(-0.00286743098852175,0.,0.480770297147094),
(0.0365944846643036,0.0384615384615384,0.04318592809152),.UNSPECIFIED.)
GEOMETRIC_REPRESENTATION_ITEM()
RATIONAL_B_SPLINE_SURFACE(((0.999326490452165,0.999646063968165,1.,0.999104400890347,
0.9984288220563),(0.999326490452165,0.999646063968165,1.,0.999104400890347,
0.9984288220563),(0.999326490452165,0.999646063968165,1.,0.999104400890347,
0.9984288220563)))
REPRESENTATION_ITEM('')
SURFACE()
);
#333=(
BOUNDED_SURFACE()
B_SPLINE_SURFACE(1,2,((#77910,#77911,#77912),(#77913,#77914,#77915),(#77916,
#77917,#77918)),.UNSPECIFIED.,.F.,.F.,.F.)
B_SPLINE_SURFACE_WITH_KNOTS((2,1,2),(3,3),(0.,1.,1.01),(0.0255903596131798,
0.0375948596693887),.UNSPECIFIED.)
GEOMETRIC_REPRESENTATION_ITEM()
RATIONAL_B_SPLINE_SURFACE(((0.996753121755999,0.997505687613148,0.999678813023854),
(0.996753121755999,0.997505687613148,0.999678813023854),(0.996753121755999,
0.997505687613148,0.999678813023854)))
REPRESENTATION_ITEM('')
SURFACE()
);
#334=(
BOUNDED_SURFACE()
B_SPLINE_SURFACE(1,2,((#77953,#77954,#77955),(#77956,#77957,#77958),(#77959,
#77960,#77961)),.UNSPECIFIED.,.F.,.F.,.F.)
B_SPLINE_SURFACE_WITH_KNOTS((2,1,2),(3,3),(-0.0028682325730164,0.,0.477902879786577),
(0.0265907346180616,0.0331702037100451),.UNSPECIFIED.)
GEOMETRIC_REPRESENTATION_ITEM()
RATIONAL_B_SPLINE_SURFACE(((0.996888414395785,0.997365765478833,0.998269846380795),
(0.996888414395785,0.997365765478833,0.998269846380795),(0.996888414395785,
0.997365765478833,0.998269846380795)))
REPRESENTATION_ITEM('')
SURFACE()
);
#335=(
BOUNDED_SURFACE()
B_SPLINE_SURFACE(1,2,((#78028,#78029,#78030),(#78031,#78032,#78033),(#78034,
#78035,#78036)),.UNSPECIFIED.,.F.,.F.,.F.)
B_SPLINE_SURFACE_WITH_KNOTS((2,1,2),(3,3),(-0.0028675311404356,0.,0.47790287978656),
(0.0166015299238945,0.023173678809005),.UNSPECIFIED.)
GEOMETRIC_REPRESENTATION_ITEM()
RATIONAL_B_SPLINE_SURFACE(((0.996422581660833,0.996252244737399,0.996507688616235),
(0.996422581660833,0.996252244737399,0.996507688616235),(0.996422581660833,
0.996252244737399,0.996507688616235)))
REPRESENTATION_ITEM('')
SURFACE()
);
#336=(
BOUNDED_SURFACE()
B_SPLINE_SURFACE(1,2,((#78053,#78054,#78055),(#78056,#78057,#78058),(#78059,
#78060,#78061)),.UNSPECIFIED.,.F.,.F.,.F.)
B_SPLINE_SURFACE_WITH_KNOTS((2,1,2),(3,3),(-0.01,0.,1.00000001523966),(0.00560769168370504,
0.0176009700440523),.UNSPECIFIED.)
GEOMETRIC_REPRESENTATION_ITEM()
RATIONAL_B_SPLINE_SURFACE(((0.998183892113821,0.99657330421516,0.996380621259469),
(0.998183892113821,0.99657330421516,0.996380621259469),(0.998183892113821,
0.99657330421516,0.996380621259469)))
REPRESENTATION_ITEM('')
SURFACE()
);
#337=(
BOUNDED_SURFACE()
B_SPLINE_SURFACE(1,2,((#78184,#78185,#78186),(#78187,#78188,#78189)),
 .UNSPECIFIED.,.F.,.F.,.F.)
B_SPLINE_SURFACE_WITH_KNOTS((2,2),(3,3),(0.,1.),(0.0556006976418415,0.0675888856590494),
 .UNSPECIFIED.)
GEOMETRIC_REPRESENTATION_ITEM()
RATIONAL_B_SPLINE_SURFACE(((0.996397562408606,0.996150386832629,0.997319912843745),
(0.996397562408606,0.996150386832629,0.997319912843745)))
REPRESENTATION_ITEM('')
SURFACE()
);
#338=(
BOUNDED_SURFACE()
B_SPLINE_SURFACE(1,2,((#78258,#78259,#78260),(#78261,#78262,#78263),(#78264,
#78265,#78266)),.UNSPECIFIED.,.F.,.F.,.F.)
B_SPLINE_SURFACE_WITH_KNOTS((2,1,2),(3,3),(0.,1.,1.01),(0.0456081671210047,
0.0575989447818808),.UNSPECIFIED.)
GEOMETRIC_REPRESENTATION_ITEM()
RATIONAL_B_SPLINE_SURFACE(((0.997793907739636,0.996365558499688,0.996354522974128),
(0.997793907739636,0.996365558499688,0.996354522974128),(0.997793907739636,
0.996365558499688,0.996354522974128)))
REPRESENTATION_ITEM('')
SURFACE()
);
#339=(
BOUNDED_SURFACE()
B_SPLINE_SURFACE(1,2,((#78301,#78302,#78303),(#78304,#78305,#78306),(#78307,
#78308,#78309)),.UNSPECIFIED.,.F.,.F.,.F.)
B_SPLINE_SURFACE_WITH_KNOTS((2,1,2),(3,3),(-0.00286810171938679,0.,0.47790287978657),
(0.0466073985929119,0.0531834927425516),.UNSPECIFIED.)
GEOMETRIC_REPRESENTATION_ITEM()
RATIONAL_B_SPLINE_SURFACE(((0.997565691989291,0.996847118074524,0.996554836308353),
(0.997565691989291,0.996847118074524,0.996554836308353),(0.997565691989291,
0.996847118074524,0.996554836308353)))
REPRESENTATION_ITEM('')
SURFACE()
);
#340=(
BOUNDED_SURFACE()
B_SPLINE_SURFACE(1,2,((#78326,#78327,#78328,#78329,#78330),(#78331,#78332,
#78333,#78334,#78335),(#78336,#78337,#78338,#78339,#78340)),
 .UNSPECIFIED.,.F.,.F.,.F.)
B_SPLINE_SURFACE_WITH_KNOTS((2,1,2),(3,2,3),(0.,1.,1.01),(0.0355931932713914,
0.0384615384615384,0.0476086899858119),.UNSPECIFIED.)
GEOMETRIC_REPRESENTATION_ITEM()
RATIONAL_B_SPLINE_SURFACE(((0.998993602249807,0.999456249886298,1.,0.998265981131401,
0.997356751596327),(0.998993602249807,0.999456249886298,1.,0.998265981131401,
0.997356751596327),(0.998993602249807,0.999456249886298,1.,0.998265981131401,
0.997356751596327)))
REPRESENTATION_ITEM('')
SURFACE()
);
#341=(
BOUNDED_SURFACE()
B_SPLINE_SURFACE(1,2,((#78388,#78389,#78390,#78391,#78392),(#78393,#78394,
#78395,#78396,#78397),(#78398,#78399,#78400,#78401,#78402)),
 .UNSPECIFIED.,.F.,.F.,.F.)
B_SPLINE_SURFACE_WITH_KNOTS((2,1,2),(3,2,3),(-0.00286742668227491,0.,0.480770297121352),
(0.03659448466429,0.0384615384615384,0.0431859280915197),.UNSPECIFIED.)
GEOMETRIC_REPRESENTATION_ITEM()
RATIONAL_B_SPLINE_SURFACE(((0.99932649045216,0.999646063968162,1.,0.999104400890347,
0.9984288220563),(0.99932649045216,0.999646063968162,1.,0.999104400890347,
0.9984288220563),(0.99932649045216,0.999646063968162,1.,0.999104400890347,
0.9984288220563)))
REPRESENTATION_ITEM('')
SURFACE()
);
#342=(
BOUNDED_SURFACE()
B_SPLINE_SURFACE(1,2,((#78429,#78430,#78431),(#78432,#78433,#78434),(#78435,
#78436,#78437)),.UNSPECIFIED.,.F.,.F.,.F.)
B_SPLINE_SURFACE_WITH_KNOTS((2,1,2),(3,3),(0.,1.,1.01),(0.02559035961318,
0.0375948596693869),.UNSPECIFIED.)
GEOMETRIC_REPRESENTATION_ITEM()
RATIONAL_B_SPLINE_SURFACE(((0.996753121755999,0.997505687613148,0.999678813023853),
(0.996753121755999,0.997505687613148,0.999678813023853),(0.996753121755999,
0.997505687613148,0.999678813023853)))
REPRESENTATION_ITEM('')
SURFACE()
);
#343=(
BOUNDED_SURFACE()
B_SPLINE_SURFACE(1,2,((#78472,#78473,#78474),(#78475,#78476,#78477),(#78478,
#78479,#78480)),.UNSPECIFIED.,.F.,.F.,.F.)
B_SPLINE_SURFACE_WITH_KNOTS((2,1,2),(3,3),(-0.00286823257304667,0.,0.477902879786519),
(0.0265907346180622,0.0331702037100437),.UNSPECIFIED.)
GEOMETRIC_REPRESENTATION_ITEM()
RATIONAL_B_SPLINE_SURFACE(((0.996888414395785,0.997365765478833,0.998269846380795),
(0.996888414395785,0.997365765478833,0.998269846380795),(0.996888414395785,
0.997365765478833,0.998269846380795)))
REPRESENTATION_ITEM('')
SURFACE()
);
#344=(
BOUNDED_SURFACE()
B_SPLINE_SURFACE(1,2,((#78547,#78548,#78549),(#78550,#78551,#78552),(#78553,
#78554,#78555)),.UNSPECIFIED.,.F.,.F.,.F.)
B_SPLINE_SURFACE_WITH_KNOTS((2,1,2),(3,3),(-0.00286753114035171,0.,0.477902879786553),
(0.0166015299238961,0.0231736788090039),.UNSPECIFIED.)
GEOMETRIC_REPRESENTATION_ITEM()
RATIONAL_B_SPLINE_SURFACE(((0.996422581660833,0.996252244737399,0.996507688616235),
(0.996422581660833,0.996252244737399,0.996507688616235),(0.996422581660833,
0.996252244737398,0.996507688616234)))
REPRESENTATION_ITEM('')
SURFACE()
);
#345=(
BOUNDED_SURFACE()
B_SPLINE_SURFACE(1,2,((#78572,#78573,#78574),(#78575,#78576,#78577),(#78578,
#78579,#78580),(#78581,#78582,#78583)),.UNSPECIFIED.,.F.,.F.,.F.)
B_SPLINE_SURFACE_WITH_KNOTS((2,1,1,2),(3,3),(-0.0101,0.,1.,1.01),(0.00560769168370619,
0.0176009700440505),.UNSPECIFIED.)
GEOMETRIC_REPRESENTATION_ITEM()
RATIONAL_B_SPLINE_SURFACE(((0.99818389211382,0.99657330421516,0.996380621259469),
(0.99818389211382,0.99657330421516,0.996380621259469),(0.99818389211382,
0.99657330421516,0.996380621259469),(0.99818389211382,0.99657330421516,
0.996380621259469)))
REPRESENTATION_ITEM('')
SURFACE()
);
#346=(
BOUNDED_SURFACE()
B_SPLINE_SURFACE(1,2,((#78618,#78619,#78620),(#78621,#78622,#78623),(#78624,
#78625,#78626)),.UNSPECIFIED.,.F.,.F.,.F.)
B_SPLINE_SURFACE_WITH_KNOTS((2,1,2),(3,3),(-0.00206901892609941,0.,0.346769728493053),
(0.00660713154711239,0.0131849431469057),.UNSPECIFIED.)
GEOMETRIC_REPRESENTATION_ITEM()
RATIONAL_B_SPLINE_SURFACE(((0.99792530735947,0.997106772384945,0.996714752253859),
(0.99792530735947,0.997106772384945,0.996714752253859),(0.99792530735947,
0.997106772384945,0.996714752253859)))
REPRESENTATION_ITEM('')
SURFACE()
);
#347=(
BOUNDED_SURFACE()
B_SPLINE_SURFACE(1,2,((#78699,#78700,#78701),(#78702,#78703,#78704)),
 .UNSPECIFIED.,.F.,.F.,.F.)
B_SPLINE_SURFACE_WITH_KNOTS((2,2),(3,3),(0.,1.),(0.0556006976418415,0.0675888856590505),
 .UNSPECIFIED.)
GEOMETRIC_REPRESENTATION_ITEM()
RATIONAL_B_SPLINE_SURFACE(((0.996397562408606,0.996150386832629,0.997319912843745),
(0.996397562408606,0.996150386832629,0.997319912843745)))
REPRESENTATION_ITEM('')
SURFACE()
);
#348=(
BOUNDED_SURFACE()
B_SPLINE_SURFACE(1,2,((#78773,#78774,#78775),(#78776,#78777,#78778),(#78779,
#78780,#78781)),.UNSPECIFIED.,.F.,.F.,.F.)
B_SPLINE_SURFACE_WITH_KNOTS((2,1,2),(3,3),(0.,1.,1.01),(0.0456081671210044,
0.0575989447818814),.UNSPECIFIED.)
GEOMETRIC_REPRESENTATION_ITEM()
RATIONAL_B_SPLINE_SURFACE(((0.997793907739636,0.996365558499688,0.996354522974128),
(0.997793907739636,0.996365558499688,0.996354522974128),(0.997793907739636,
0.996365558499688,0.996354522974128)))
REPRESENTATION_ITEM('')
SURFACE()
);
#349=(
BOUNDED_SURFACE()
B_SPLINE_SURFACE(1,2,((#78816,#78817,#78818),(#78819,#78820,#78821),(#78822,
#78823,#78824)),.UNSPECIFIED.,.F.,.F.,.F.)
B_SPLINE_SURFACE_WITH_KNOTS((2,1,2),(3,3),(-0.00286810173453871,0.,0.477902879786588),
(0.0466073985929109,0.0531834929157976),.UNSPECIFIED.)
GEOMETRIC_REPRESENTATION_ITEM()
RATIONAL_B_SPLINE_SURFACE(((0.997565691989291,0.996847118055593,0.996554836292953),
(0.997565691989291,0.996847118055593,0.996554836292953),(0.997565691989291,
0.996847118055593,0.996554836292953)))
REPRESENTATION_ITEM('')
SURFACE()
);
#350=(
BOUNDED_SURFACE()
B_SPLINE_SURFACE(1,2,((#78841,#78842,#78843,#78844,#78845),(#78846,#78847,
#78848,#78849,#78850),(#78851,#78852,#78853,#78854,#78855)),
 .UNSPECIFIED.,.F.,.F.,.F.)
B_SPLINE_SURFACE_WITH_KNOTS((2,1,2),(3,2,3),(0.,1.,1.01),(0.0355931932713903,
0.0384615384615384,0.0476086899858134),.UNSPECIFIED.)
GEOMETRIC_REPRESENTATION_ITEM()
RATIONAL_B_SPLINE_SURFACE(((0.998993602249807,0.999456249886298,1.,0.998265981131401,
0.997356751596327),(0.998993602249807,0.999456249886298,1.,0.998265981131401,
0.997356751596327),(0.998993602249807,0.999456249886298,1.,0.998265981131401,
0.997356751596327)))
REPRESENTATION_ITEM('')
SURFACE()
);
#351=(
BOUNDED_SURFACE()
B_SPLINE_SURFACE(1,2,((#78903,#78904,#78905,#78906,#78907),(#78908,#78909,
#78910,#78911,#78912),(#78913,#78914,#78915,#78916,#78917)),
 .UNSPECIFIED.,.F.,.F.,.F.)
B_SPLINE_SURFACE_WITH_KNOTS((2,1,2),(3,2,3),(-0.00141401191198416,0.,0.480770297080041),
(0.0365944846645786,0.0384615384615384,0.0431859280915184),
 .UNSPECIFIED.)
GEOMETRIC_REPRESENTATION_ITEM()
RATIONAL_B_SPLINE_SURFACE(((0.999326490452259,0.999646063968217,1.,0.999104400890347,
0.9984288220563),(0.999326490452259,0.999646063968217,1.,0.999104400890347,
0.9984288220563),(0.999326490452259,0.999646063968217,1.,0.999104400890347,
0.9984288220563)))
REPRESENTATION_ITEM('')
SURFACE()
);
#352=(
BOUNDED_SURFACE()
B_SPLINE_SURFACE(1,2,((#78944,#78945,#78946),(#78947,#78948,#78949),(#78950,
#78951,#78952)),.UNSPECIFIED.,.F.,.F.,.F.)
B_SPLINE_SURFACE_WITH_KNOTS((2,1,2),(3,3),(0.,1.,1.01),(0.0255903596131787,
0.0375948596693877),.UNSPECIFIED.)
GEOMETRIC_REPRESENTATION_ITEM()
RATIONAL_B_SPLINE_SURFACE(((0.996753121755999,0.997505687613148,0.999678813023853),
(0.996753121755999,0.997505687613148,0.999678813023853),(0.996753121755999,
0.997505687613148,0.999678813023853)))
REPRESENTATION_ITEM('')
SURFACE()
);
#353=(
BOUNDED_SURFACE()
B_SPLINE_SURFACE(1,2,((#78987,#78988,#78989),(#78990,#78991,#78992),(#78993,
#78994,#78995)),.UNSPECIFIED.,.F.,.F.,.F.)
B_SPLINE_SURFACE_WITH_KNOTS((2,1,2),(3,3),(-0.00286823356215784,0.,0.477902879786496),
(0.0265907346180615,0.0331702037252929),.UNSPECIFIED.)
GEOMETRIC_REPRESENTATION_ITEM()
RATIONAL_B_SPLINE_SURFACE(((0.996888414395785,0.997365765479939,0.998269846384985),
(0.996888414395785,0.997365765479939,0.998269846384985),(0.996888414395785,
0.997365765479939,0.998269846384985)))
REPRESENTATION_ITEM('')
SURFACE()
);
#354=(
BOUNDED_SURFACE()
B_SPLINE_SURFACE(1,2,((#79062,#79063,#79064),(#79065,#79066,#79067),(#79068,
#79069,#79070)),.UNSPECIFIED.,.F.,.F.,.F.)
B_SPLINE_SURFACE_WITH_KNOTS((2,1,2),(3,3),(-0.00286753074356712,0.,0.47790287978649),
(0.0166015299238963,0.0231736788028835),.UNSPECIFIED.)
GEOMETRIC_REPRESENTATION_ITEM()
RATIONAL_B_SPLINE_SURFACE(((0.996422581660833,0.996252244737557,0.996507688615759),
(0.996422581660833,0.996252244737557,0.996507688615759),(0.996422581660833,
0.996252244737557,0.996507688615759)))
REPRESENTATION_ITEM('')
SURFACE()
);
#355=(
BOUNDED_SURFACE()
B_SPLINE_SURFACE(1,2,((#79087,#79088,#79089),(#79090,#79091,#79092),(#79093,
#79094,#79095),(#79096,#79097,#79098)),.UNSPECIFIED.,.F.,.F.,.F.)
B_SPLINE_SURFACE_WITH_KNOTS((2,1,1,2),(3,3),(-0.0101,0.,1.,1.01),(0.00560769168370609,
0.0176009700440527),.UNSPECIFIED.)
GEOMETRIC_REPRESENTATION_ITEM()
RATIONAL_B_SPLINE_SURFACE(((0.99818389211382,0.99657330421516,0.996380621259469),
(0.99818389211382,0.99657330421516,0.996380621259469),(0.99818389211382,
0.99657330421516,0.996380621259469),(0.99818389211382,0.99657330421516,
0.996380621259469)))
REPRESENTATION_ITEM('')
SURFACE()
);
#356=(
BOUNDED_SURFACE()
B_SPLINE_SURFACE(1,2,((#79133,#79134,#79135),(#79136,#79137,#79138),(#79139,
#79140,#79141)),.UNSPECIFIED.,.F.,.F.,.F.)
B_SPLINE_SURFACE_WITH_KNOTS((2,1,2),(3,3),(-0.00206901892446915,0.,0.346769728493051),
(0.00660713154709824,0.0131849431293194),.UNSPECIFIED.)
GEOMETRIC_REPRESENTATION_ITEM()
RATIONAL_B_SPLINE_SURFACE(((0.997925307359474,0.997106772387135,0.996714752255955),
(0.997925307359474,0.997106772387135,0.996714752255955),(0.997925307359474,
0.997106772387135,0.996714752255955)))
REPRESENTATION_ITEM('')
SURFACE()
);
#357=(
BOUNDED_SURFACE()
B_SPLINE_SURFACE(1,2,((#79214,#79215,#79216),(#79217,#79218,#79219)),
 .UNSPECIFIED.,.F.,.F.,.F.)
B_SPLINE_SURFACE_WITH_KNOTS((2,2),(3,3),(0.,1.),(0.0556006976418428,0.0675888856590498),
 .UNSPECIFIED.)
GEOMETRIC_REPRESENTATION_ITEM()
RATIONAL_B_SPLINE_SURFACE(((0.996397562408606,0.996150386832629,0.997319912843745),
(0.996397562408606,0.996150386832629,0.997319912843745)))
REPRESENTATION_ITEM('')
SURFACE()
);
#358=(
BOUNDED_SURFACE()
B_SPLINE_SURFACE(1,2,((#79288,#79289,#79290),(#79291,#79292,#79293),(#79294,
#79295,#79296)),.UNSPECIFIED.,.F.,.F.,.F.)
B_SPLINE_SURFACE_WITH_KNOTS((2,1,2),(3,3),(0.,1.,1.01),(0.0456081671210055,
0.0575989447818819),.UNSPECIFIED.)
GEOMETRIC_REPRESENTATION_ITEM()
RATIONAL_B_SPLINE_SURFACE(((0.997793907739636,0.996365558499688,0.996354522974128),
(0.997793907739636,0.996365558499688,0.996354522974128),(0.997793907739636,
0.996365558499688,0.996354522974128)))
REPRESENTATION_ITEM('')
SURFACE()
);
#359=(
BOUNDED_SURFACE()
B_SPLINE_SURFACE(1,2,((#79331,#79332,#79333),(#79334,#79335,#79336),(#79337,
#79338,#79339)),.UNSPECIFIED.,.F.,.F.,.F.)
B_SPLINE_SURFACE_WITH_KNOTS((2,1,2),(3,3),(-0.00286810173451702,0.,0.47790287978659),
(0.0466073985929117,0.0531834929157972),.UNSPECIFIED.)
GEOMETRIC_REPRESENTATION_ITEM()
RATIONAL_B_SPLINE_SURFACE(((0.997565691989291,0.996847118055593,0.996554836292953),
(0.997565691989291,0.996847118055593,0.996554836292953),(0.997565691989291,
0.996847118055594,0.996554836292953)))
REPRESENTATION_ITEM('')
SURFACE()
);
#360=(
BOUNDED_SURFACE()
B_SPLINE_SURFACE(1,2,((#79356,#79357,#79358,#79359,#79360),(#79361,#79362,
#79363,#79364,#79365),(#79366,#79367,#79368,#79369,#79370)),
 .UNSPECIFIED.,.F.,.F.,.F.)
B_SPLINE_SURFACE_WITH_KNOTS((2,1,2),(3,2,3),(0.,1.,1.01),(0.0355931932713904,
0.0384615384615384,0.0476086899858127),.UNSPECIFIED.)
GEOMETRIC_REPRESENTATION_ITEM()
RATIONAL_B_SPLINE_SURFACE(((0.998993602249807,0.999456249886298,1.,0.998265981131401,
0.997356751596327),(0.998993602249807,0.999456249886298,1.,0.998265981131401,
0.997356751596327),(0.998993602249807,0.999456249886298,1.,0.998265981131401,
0.997356751596327)))
REPRESENTATION_ITEM('')
SURFACE()
);
#361=(
BOUNDED_SURFACE()
B_SPLINE_SURFACE(1,2,((#79418,#79419,#79420,#79421,#79422),(#79423,#79424,
#79425,#79426,#79427),(#79428,#79429,#79430,#79431,#79432)),
 .UNSPECIFIED.,.F.,.F.,.F.)
B_SPLINE_SURFACE_WITH_KNOTS((2,1,2),(3,2,3),(-0.00286743098642913,0.,0.480770297146903),
(0.0365944846642603,0.0384615384615384,0.0431859280915195),
 .UNSPECIFIED.)
GEOMETRIC_REPRESENTATION_ITEM()
RATIONAL_B_SPLINE_SURFACE(((0.999326490452151,0.999646063968157,1.,0.999104400890347,
0.9984288220563),(0.999326490452151,0.999646063968157,1.,0.999104400890347,
0.9984288220563),(0.999326490452151,0.999646063968157,1.,0.999104400890347,
0.9984288220563)))
REPRESENTATION_ITEM('')
SURFACE()
);
#362=(
BOUNDED_SURFACE()
B_SPLINE_SURFACE(1,2,((#79459,#79460,#79461),(#79462,#79463,#79464),(#79465,
#79466,#79467)),.UNSPECIFIED.,.F.,.F.,.F.)
B_SPLINE_SURFACE_WITH_KNOTS((2,1,2),(3,3),(0.,1.,1.01),(0.0255903596131786,
0.0375948596693872),.UNSPECIFIED.)
GEOMETRIC_REPRESENTATION_ITEM()
RATIONAL_B_SPLINE_SURFACE(((0.996753121755999,0.997505687613147,0.999678813023853),
(0.996753121755999,0.997505687613147,0.999678813023853),(0.996753121755999,
0.997505687613147,0.999678813023853)))
REPRESENTATION_ITEM('')
SURFACE()
);
#363=(
BOUNDED_SURFACE()
B_SPLINE_SURFACE(1,2,((#79502,#79503,#79504),(#79505,#79506,#79507),(#79508,
#79509,#79510)),.UNSPECIFIED.,.F.,.F.,.F.)
B_SPLINE_SURFACE_WITH_KNOTS((2,1,2),(3,3),(-0.00286823356208571,0.,0.477902879786613),
(0.0265907346180613,0.0331702037252923),.UNSPECIFIED.)
GEOMETRIC_REPRESENTATION_ITEM()
RATIONAL_B_SPLINE_SURFACE(((0.996888414395785,0.997365765479939,0.998269846384985),
(0.996888414395785,0.997365765479939,0.998269846384985),(0.996888414395785,
0.997365765479939,0.998269846384985)))
REPRESENTATION_ITEM('')
SURFACE()
);
#364=(
BOUNDED_SURFACE()
B_SPLINE_SURFACE(1,2,((#79577,#79578,#79579),(#79580,#79581,#79582),(#79583,
#79584,#79585)),.UNSPECIFIED.,.F.,.F.,.F.)
B_SPLINE_SURFACE_WITH_KNOTS((2,1,2),(3,3),(-0.00286753128194045,0.,0.477902879786441),
(0.0166015299238959,0.0231736788111881),.UNSPECIFIED.)
GEOMETRIC_REPRESENTATION_ITEM()
RATIONAL_B_SPLINE_SURFACE(((0.996422581660833,0.996252244737342,0.996507688616404),
(0.996422581660833,0.996252244737342,0.996507688616404),(0.996422581660833,
0.996252244737342,0.996507688616404)))
REPRESENTATION_ITEM('')
SURFACE()
);
#365=(
BOUNDED_SURFACE()
B_SPLINE_SURFACE(1,2,((#79602,#79603,#79604),(#79605,#79606,#79607),(#79608,
#79609,#79610),(#79611,#79612,#79613)),.UNSPECIFIED.,.F.,.F.,.F.)
B_SPLINE_SURFACE_WITH_KNOTS((2,1,1,2),(3,3),(-0.0101,0.,1.,1.01),(0.00560769168370533,
0.0176009700440512),.UNSPECIFIED.)
GEOMETRIC_REPRESENTATION_ITEM()
RATIONAL_B_SPLINE_SURFACE(((0.998183892113821,0.99657330421516,0.996380621259469),
(0.998183892113821,0.99657330421516,0.996380621259469),(0.998183892113821,
0.99657330421516,0.996380621259469),(0.998183892113821,0.99657330421516,
0.996380621259469)))
REPRESENTATION_ITEM('')
SURFACE()
);
#366=(
BOUNDED_SURFACE()
B_SPLINE_SURFACE(1,2,((#79648,#79649,#79650),(#79651,#79652,#79653),(#79654,
#79655,#79656)),.UNSPECIFIED.,.F.,.F.,.F.)
B_SPLINE_SURFACE_WITH_KNOTS((2,1,2),(3,3),(-0.00206901892451206,0.,0.346769728493621),
(0.00660713154708297,0.0131849431293158),.UNSPECIFIED.)
GEOMETRIC_REPRESENTATION_ITEM()
RATIONAL_B_SPLINE_SURFACE(((0.997925307359477,0.997106772387136,0.996714752255955),
(0.997925307359477,0.997106772387136,0.996714752255955),(0.997925307359477,
0.997106772387136,0.996714752255955)))
REPRESENTATION_ITEM('')
SURFACE()
);
#367=(
BOUNDED_SURFACE()
B_SPLINE_SURFACE(1,2,((#79729,#79730,#79731),(#79732,#79733,#79734)),
 .UNSPECIFIED.,.F.,.F.,.F.)
B_SPLINE_SURFACE_WITH_KNOTS((2,2),(3,3),(0.,1.),(0.0556006976418427,0.0675888856590503),
 .UNSPECIFIED.)
GEOMETRIC_REPRESENTATION_ITEM()
RATIONAL_B_SPLINE_SURFACE(((0.996397562408606,0.996150386832629,0.997319912843745),
(0.996397562408606,0.996150386832629,0.997319912843745)))
REPRESENTATION_ITEM('')
SURFACE()
);
#368=(
BOUNDED_SURFACE()
B_SPLINE_SURFACE(1,2,((#79803,#79804,#79805),(#79806,#79807,#79808),(#79809,
#79810,#79811)),.UNSPECIFIED.,.F.,.F.,.F.)
B_SPLINE_SURFACE_WITH_KNOTS((2,1,2),(3,3),(0.,1.,1.01),(0.0456081671210046,
0.0575989447818824),.UNSPECIFIED.)
GEOMETRIC_REPRESENTATION_ITEM()
RATIONAL_B_SPLINE_SURFACE(((0.997793907739636,0.996365558499688,0.996354522974129),
(0.997793907739636,0.996365558499688,0.996354522974129),(0.997793907739636,
0.996365558499688,0.996354522974129)))
REPRESENTATION_ITEM('')
SURFACE()
);
#369=(
BOUNDED_SURFACE()
B_SPLINE_SURFACE(1,2,((#79846,#79847,#79848),(#79849,#79850,#79851),(#79852,
#79853,#79854)),.UNSPECIFIED.,.F.,.F.,.F.)
B_SPLINE_SURFACE_WITH_KNOTS((2,1,2),(3,3),(-0.00286810173448454,0.,0.477902879786614),
(0.0466073985929115,0.0531834929157978),.UNSPECIFIED.)
GEOMETRIC_REPRESENTATION_ITEM()
RATIONAL_B_SPLINE_SURFACE(((0.997565691989291,0.996847118055593,0.996554836292953),
(0.997565691989291,0.996847118055593,0.996554836292953),(0.997565691989291,
0.996847118055593,0.996554836292953)))
REPRESENTATION_ITEM('')
SURFACE()
);
#370=(
BOUNDED_SURFACE()
B_SPLINE_SURFACE(1,2,((#79871,#79872,#79873,#79874,#79875),(#79876,#79877,
#79878,#79879,#79880),(#79881,#79882,#79883,#79884,#79885)),
 .UNSPECIFIED.,.F.,.F.,.F.)
B_SPLINE_SURFACE_WITH_KNOTS((2,1,2),(3,2,3),(0.,1.,1.01),(0.0355931932713903,
0.0384615384615384,0.0476086899858137),.UNSPECIFIED.)
GEOMETRIC_REPRESENTATION_ITEM()
RATIONAL_B_SPLINE_SURFACE(((0.998993602249807,0.999456249886298,1.,0.998265981131401,
0.997356751596327),(0.998993602249807,0.999456249886298,1.,0.998265981131401,
0.997356751596327),(0.998993602249807,0.999456249886298,1.,0.998265981131401,
0.997356751596327)))
REPRESENTATION_ITEM('')
SURFACE()
);
#371=(
BOUNDED_SURFACE()
B_SPLINE_SURFACE(1,2,((#79933,#79934,#79935,#79936,#79937),(#79938,#79939,
#79940,#79941,#79942),(#79943,#79944,#79945,#79946,#79947)),
 .UNSPECIFIED.,.F.,.F.,.F.)
B_SPLINE_SURFACE_WITH_KNOTS((2,1,2),(3,2,3),(-0.00141401191197124,0.,0.48077029708092),
(0.0365944846645755,0.0384615384615384,0.0431859280915187),
 .UNSPECIFIED.)
GEOMETRIC_REPRESENTATION_ITEM()
RATIONAL_B_SPLINE_SURFACE(((0.999326490452259,0.999646063968217,1.,0.999104400890347,
0.9984288220563),(0.999326490452259,0.999646063968217,1.,0.999104400890347,
0.9984288220563),(0.999326490452259,0.999646063968217,1.,0.999104400890347,
0.9984288220563)))
REPRESENTATION_ITEM('')
SURFACE()
);
#372=(
BOUNDED_SURFACE()
B_SPLINE_SURFACE(1,2,((#79974,#79975,#79976),(#79977,#79978,#79979),(#79980,
#79981,#79982)),.UNSPECIFIED.,.F.,.F.,.F.)
B_SPLINE_SURFACE_WITH_KNOTS((2,1,2),(3,3),(0.,1.,1.01),(0.0255903596131801,
0.037594859669387),.UNSPECIFIED.)
GEOMETRIC_REPRESENTATION_ITEM()
RATIONAL_B_SPLINE_SURFACE(((0.996753121755999,0.997505687613148,0.999678813023853),
(0.996753121755999,0.997505687613148,0.999678813023853),(0.996753121755999,
0.997505687613148,0.999678813023853)))
REPRESENTATION_ITEM('')
SURFACE()
);
#373=(
BOUNDED_SURFACE()
B_SPLINE_SURFACE(1,2,((#80017,#80018,#80019),(#80020,#80021,#80022),(#80023,
#80024,#80025)),.UNSPECIFIED.,.F.,.F.,.F.)
B_SPLINE_SURFACE_WITH_KNOTS((2,1,2),(3,3),(-0.00286823356213617,0.,0.477902879786565),
(0.0265907346180619,0.0331702037252924),.UNSPECIFIED.)
GEOMETRIC_REPRESENTATION_ITEM()
RATIONAL_B_SPLINE_SURFACE(((0.996888414395785,0.997365765479939,0.998269846384985),
(0.996888414395785,0.997365765479939,0.998269846384985),(0.996888414395785,
0.997365765479939,0.998269846384985)))
REPRESENTATION_ITEM('')
SURFACE()
);
#374=(
BOUNDED_SURFACE()
B_SPLINE_SURFACE(1,2,((#80092,#80093,#80094),(#80095,#80096,#80097),(#80098,
#80099,#80100)),.UNSPECIFIED.,.F.,.F.,.F.)
B_SPLINE_SURFACE_WITH_KNOTS((2,1,2),(3,3),(-0.00286753128190398,0.,0.477902879786596),
(0.0166015299238956,0.0231736788111882),.UNSPECIFIED.)
GEOMETRIC_REPRESENTATION_ITEM()
RATIONAL_B_SPLINE_SURFACE(((0.996422581660833,0.996252244737342,0.996507688616404),
(0.996422581660833,0.996252244737342,0.996507688616404),(0.996422581660833,
0.996252244737342,0.996507688616404)))
REPRESENTATION_ITEM('')
SURFACE()
);
#375=(
BOUNDED_SURFACE()
B_SPLINE_SURFACE(1,2,((#80117,#80118,#80119),(#80120,#80121,#80122),(#80123,
#80124,#80125),(#80126,#80127,#80128)),.UNSPECIFIED.,.F.,.F.,.F.)
B_SPLINE_SURFACE_WITH_KNOTS((2,1,1,2),(3,3),(-0.0101,0.,1.,1.01),(0.00560769168370618,
0.0176009700440517),.UNSPECIFIED.)
GEOMETRIC_REPRESENTATION_ITEM()
RATIONAL_B_SPLINE_SURFACE(((0.99818389211382,0.99657330421516,0.996380621259469),
(0.99818389211382,0.99657330421516,0.996380621259469),(0.99818389211382,
0.99657330421516,0.996380621259469),(0.99818389211382,0.99657330421516,
0.996380621259469)))
REPRESENTATION_ITEM('')
SURFACE()
);
#376=(
BOUNDED_SURFACE()
B_SPLINE_SURFACE(1,2,((#80163,#80164,#80165),(#80166,#80167,#80168),(#80169,
#80170,#80171)),.UNSPECIFIED.,.F.,.F.,.F.)
B_SPLINE_SURFACE_WITH_KNOTS((2,1,2),(3,3),(-0.00206901892603345,0.,0.346769728494672),
(0.00660713154706902,0.013184943146953),.UNSPECIFIED.)
GEOMETRIC_REPRESENTATION_ITEM()
RATIONAL_B_SPLINE_SURFACE(((0.99792530735948,0.997106772384942,0.996714752253853),
(0.99792530735948,0.997106772384942,0.996714752253853),(0.99792530735948,
0.997106772384942,0.996714752253853)))
REPRESENTATION_ITEM('')
SURFACE()
);
#377=(
BOUNDED_SURFACE()
B_SPLINE_SURFACE(1,2,((#80244,#80245,#80246),(#80247,#80248,#80249)),
 .UNSPECIFIED.,.F.,.F.,.F.)
B_SPLINE_SURFACE_WITH_KNOTS((2,2),(3,3),(0.,1.),(0.0556006976418414,0.0675888856590506),
 .UNSPECIFIED.)
GEOMETRIC_REPRESENTATION_ITEM()
RATIONAL_B_SPLINE_SURFACE(((0.996397562408606,0.996150386832629,0.997319912843745),
(0.996397562408606,0.996150386832629,0.997319912843745)))
REPRESENTATION_ITEM('')
SURFACE()
);
#378=(
BOUNDED_SURFACE()
B_SPLINE_SURFACE(1,2,((#80318,#80319,#80320),(#80321,#80322,#80323),(#80324,
#80325,#80326)),.UNSPECIFIED.,.F.,.F.,.F.)
B_SPLINE_SURFACE_WITH_KNOTS((2,1,2),(3,3),(0.,1.,1.01),(0.0456081671210044,
0.0575989447818825),.UNSPECIFIED.)
GEOMETRIC_REPRESENTATION_ITEM()
RATIONAL_B_SPLINE_SURFACE(((0.997793907739636,0.996365558499688,0.996354522974128),
(0.997793907739636,0.996365558499688,0.996354522974128),(0.997793907739636,
0.996365558499688,0.996354522974128)))
REPRESENTATION_ITEM('')
SURFACE()
);
#379=(
BOUNDED_SURFACE()
B_SPLINE_SURFACE(1,2,((#80361,#80362,#80363),(#80364,#80365,#80366),(#80367,
#80368,#80369)),.UNSPECIFIED.,.F.,.F.,.F.)
B_SPLINE_SURFACE_WITH_KNOTS((2,1,2),(3,3),(-0.00286810173447193,0.,0.4779028797867),
(0.0466073985929119,0.0531834929157973),.UNSPECIFIED.)
GEOMETRIC_REPRESENTATION_ITEM()
RATIONAL_B_SPLINE_SURFACE(((0.997565691989291,0.996847118055594,0.996554836292953),
(0.997565691989291,0.996847118055594,0.996554836292953),(0.997565691989291,
0.996847118055594,0.996554836292953)))
REPRESENTATION_ITEM('')
SURFACE()
);
#380=(
BOUNDED_SURFACE()
B_SPLINE_SURFACE(1,2,((#80386,#80387,#80388,#80389,#80390),(#80391,#80392,
#80393,#80394,#80395),(#80396,#80397,#80398,#80399,#80400)),
 .UNSPECIFIED.,.F.,.F.,.F.)
B_SPLINE_SURFACE_WITH_KNOTS((2,1,2),(3,2,3),(0.,1.,1.01),(0.0355931932713903,
0.0384615384615384,0.0476086899858133),.UNSPECIFIED.)
GEOMETRIC_REPRESENTATION_ITEM()
RATIONAL_B_SPLINE_SURFACE(((0.998993602249807,0.999456249886298,1.,0.998265981131401,
0.997356751596327),(0.998993602249807,0.999456249886298,1.,0.998265981131401,
0.997356751596327),(0.998993602249807,0.999456249886298,1.,0.998265981131401,
0.997356751596327)))
REPRESENTATION_ITEM('')
SURFACE()
);
#381=(
BOUNDED_SURFACE()
B_SPLINE_SURFACE(1,2,((#80448,#80449,#80450,#80451,#80452),(#80453,#80454,
#80455,#80456,#80457),(#80458,#80459,#80460,#80461,#80462)),
 .UNSPECIFIED.,.F.,.F.,.F.)
B_SPLINE_SURFACE_WITH_KNOTS((2,1,2),(3,2,3),(-0.00141401191198348,0.,0.480770297080689),
(0.0365944846645759,0.0384615384615384,0.0431859280915187),
 .UNSPECIFIED.)
GEOMETRIC_REPRESENTATION_ITEM()
RATIONAL_B_SPLINE_SURFACE(((0.999326490452259,0.999646063968217,1.,0.999104400890347,
0.9984288220563),(0.999326490452259,0.999646063968217,1.,0.999104400890347,
0.9984288220563),(0.999326490452259,0.999646063968217,1.,0.999104400890347,
0.9984288220563)))
REPRESENTATION_ITEM('')
SURFACE()
);
#382=(
BOUNDED_SURFACE()
B_SPLINE_SURFACE(1,2,((#80489,#80490,#80491),(#80492,#80493,#80494),(#80495,
#80496,#80497)),.UNSPECIFIED.,.F.,.F.,.F.)
B_SPLINE_SURFACE_WITH_KNOTS((2,1,2),(3,3),(0.,1.,1.01),(0.0255903596131798,
0.0375948596693881),.UNSPECIFIED.)
GEOMETRIC_REPRESENTATION_ITEM()
RATIONAL_B_SPLINE_SURFACE(((0.996753121755999,0.997505687613148,0.999678813023854),
(0.996753121755999,0.997505687613148,0.999678813023854),(0.996753121755999,
0.997505687613148,0.999678813023854)))
REPRESENTATION_ITEM('')
SURFACE()
);
#383=(
BOUNDED_SURFACE()
B_SPLINE_SURFACE(1,2,((#80532,#80533,#80534),(#80535,#80536,#80537),(#80538,
#80539,#80540)),.UNSPECIFIED.,.F.,.F.,.F.)
B_SPLINE_SURFACE_WITH_KNOTS((2,1,2),(3,3),(-0.00286823045888591,0.,0.477902879786571),
(0.0265907346180616,0.0331702036774535),.UNSPECIFIED.)
GEOMETRIC_REPRESENTATION_ITEM()
RATIONAL_B_SPLINE_SURFACE(((0.996888414395785,0.997365765476469,0.998269846371838),
(0.996888414395785,0.997365765476469,0.998269846371838),(0.996888414395785,
0.997365765476469,0.998269846371838)))
REPRESENTATION_ITEM('')
SURFACE()
);
#384=(
BOUNDED_SURFACE()
B_SPLINE_SURFACE(1,2,((#80607,#80608,#80609),(#80610,#80611,#80612),(#80613,
#80614,#80615)),.UNSPECIFIED.,.F.,.F.,.F.)
B_SPLINE_SURFACE_WITH_KNOTS((2,1,2),(3,3),(-0.00286753128209032,0.,0.477902879786622),
(0.016601529923896,0.0231736788111887),.UNSPECIFIED.)
GEOMETRIC_REPRESENTATION_ITEM()
RATIONAL_B_SPLINE_SURFACE(((0.996422581660833,0.996252244737342,0.996507688616404),
(0.996422581660833,0.996252244737342,0.996507688616404),(0.996422581660833,
0.996252244737342,0.996507688616404)))
REPRESENTATION_ITEM('')
SURFACE()
);
#385=(
BOUNDED_SURFACE()
B_SPLINE_SURFACE(1,2,((#80632,#80633,#80634),(#80635,#80636,#80637),(#80638,
#80639,#80640),(#80641,#80642,#80643)),.UNSPECIFIED.,.F.,.F.,.F.)
B_SPLINE_SURFACE_WITH_KNOTS((2,1,1,2),(3,3),(-0.0101,0.,1.,1.01),(0.00560769168370516,
0.0176009700440517),.UNSPECIFIED.)
GEOMETRIC_REPRESENTATION_ITEM()
RATIONAL_B_SPLINE_SURFACE(((0.998183892113821,0.99657330421516,0.996380621259469),
(0.998183892113821,0.99657330421516,0.996380621259469),(0.998183892113821,
0.99657330421516,0.996380621259469),(0.998183892113821,0.99657330421516,
0.996380621259469)))
REPRESENTATION_ITEM('')
SURFACE()
);
#386=(
BOUNDED_SURFACE()
B_SPLINE_SURFACE(1,2,((#80678,#80679,#80680),(#80681,#80682,#80683),(#80684,
#80685,#80686)),.UNSPECIFIED.,.F.,.F.,.F.)
B_SPLINE_SURFACE_WITH_KNOTS((2,1,2),(3,3),(-0.00206901892596923,0.,0.346769728495858),
(0.00660713154705422,0.0131849431469467),.UNSPECIFIED.)
GEOMETRIC_REPRESENTATION_ITEM()
RATIONAL_B_SPLINE_SURFACE(((0.997925307359485,0.997106772384944,0.996714752253854),
(0.997925307359485,0.997106772384944,0.996714752253854),(0.997925307359485,
0.997106772384944,0.996714752253854)))
REPRESENTATION_ITEM('')
SURFACE()
);
#387=(
BOUNDED_SURFACE()
B_SPLINE_SURFACE(1,2,((#80759,#80760,#80761),(#80762,#80763,#80764)),
 .UNSPECIFIED.,.F.,.F.,.F.)
B_SPLINE_SURFACE_WITH_KNOTS((2,2),(3,3),(0.,1.),(0.0556006976418415,0.0675888856590506),
 .UNSPECIFIED.)
GEOMETRIC_REPRESENTATION_ITEM()
RATIONAL_B_SPLINE_SURFACE(((0.996397562408606,0.996150386832629,0.997319912843745),
(0.996397562408606,0.996150386832629,0.997319912843745)))
REPRESENTATION_ITEM('')
SURFACE()
);
#388=(
BOUNDED_SURFACE()
B_SPLINE_SURFACE(1,2,((#80833,#80834,#80835),(#80836,#80837,#80838),(#80839,
#80840,#80841)),.UNSPECIFIED.,.F.,.F.,.F.)
B_SPLINE_SURFACE_WITH_KNOTS((2,1,2),(3,3),(0.,1.,1.01),(0.0456081671210032,
0.0575989447818814),.UNSPECIFIED.)
GEOMETRIC_REPRESENTATION_ITEM()
RATIONAL_B_SPLINE_SURFACE(((0.997793907739636,0.996365558499688,0.996354522974128),
(0.997793907739636,0.996365558499688,0.996354522974128),(0.997793907739636,
0.996365558499688,0.996354522974128)))
REPRESENTATION_ITEM('')
SURFACE()
);
#389=(
BOUNDED_SURFACE()
B_SPLINE_SURFACE(1,2,((#80876,#80877,#80878),(#80879,#80880,#80881),(#80882,
#80883,#80884)),.UNSPECIFIED.,.F.,.F.,.F.)
B_SPLINE_SURFACE_WITH_KNOTS((2,1,2),(3,3),(-0.00286810173442196,0.,0.477902879786453),
(0.0466073985929114,0.0531834929157971),.UNSPECIFIED.)
GEOMETRIC_REPRESENTATION_ITEM()
RATIONAL_B_SPLINE_SURFACE(((0.997565691989291,0.996847118055594,0.996554836292953),
(0.997565691989291,0.996847118055594,0.996554836292953),(0.997565691989291,
0.996847118055594,0.996554836292953)))
REPRESENTATION_ITEM('')
SURFACE()
);
#390=(
BOUNDED_SURFACE()
B_SPLINE_SURFACE(1,2,((#80901,#80902,#80903,#80904,#80905),(#80906,#80907,
#80908,#80909,#80910),(#80911,#80912,#80913,#80914,#80915)),
 .UNSPECIFIED.,.F.,.F.,.F.)
B_SPLINE_SURFACE_WITH_KNOTS((2,1,2),(3,2,3),(0.,1.,1.01),(0.0355931932713903,
0.0384615384615384,0.0476086899858133),.UNSPECIFIED.)
GEOMETRIC_REPRESENTATION_ITEM()
RATIONAL_B_SPLINE_SURFACE(((0.998993602249807,0.999456249886298,1.,0.998265981131401,
0.997356751596327),(0.998993602249807,0.999456249886298,1.,0.998265981131401,
0.997356751596327),(0.998993602249807,0.999456249886298,1.,0.998265981131401,
0.997356751596327)))
REPRESENTATION_ITEM('')
SURFACE()
);
#391=(
BOUNDED_SURFACE()
B_SPLINE_SURFACE(1,2,((#80963,#80964,#80965,#80966,#80967),(#80968,#80969,
#80970,#80971,#80972),(#80973,#80974,#80975,#80976,#80977)),
 .UNSPECIFIED.,.F.,.F.,.F.)
B_SPLINE_SURFACE_WITH_KNOTS((2,1,2),(3,2,3),(-0.0014140119119804,0.,0.480770297080892),
(0.0365944846645756,0.0384615384615384,0.0431859280915182),
 .UNSPECIFIED.)
GEOMETRIC_REPRESENTATION_ITEM()
RATIONAL_B_SPLINE_SURFACE(((0.999326490452258,0.999646063968217,1.,0.999104400890347,
0.9984288220563),(0.999326490452258,0.999646063968217,1.,0.999104400890347,
0.9984288220563),(0.999326490452258,0.999646063968217,1.,0.999104400890347,
0.9984288220563)))
REPRESENTATION_ITEM('')
SURFACE()
);
#392=(
BOUNDED_SURFACE()
B_SPLINE_SURFACE(1,2,((#81004,#81005,#81006),(#81007,#81008,#81009),(#81010,
#81011,#81012)),.UNSPECIFIED.,.F.,.F.,.F.)
B_SPLINE_SURFACE_WITH_KNOTS((2,1,2),(3,3),(0.,1.,1.01),(0.0255903596131789,
0.0375948596693871),.UNSPECIFIED.)
GEOMETRIC_REPRESENTATION_ITEM()
RATIONAL_B_SPLINE_SURFACE(((0.996753121755999,0.997505687613148,0.999678813023853),
(0.996753121755999,0.997505687613148,0.999678813023853),(0.996753121755999,
0.997505687613148,0.999678813023853)))
REPRESENTATION_ITEM('')
SURFACE()
);
#393=(
BOUNDED_SURFACE()
B_SPLINE_SURFACE(1,2,((#81047,#81048,#81049),(#81050,#81051,#81052),(#81053,
#81054,#81055)),.UNSPECIFIED.,.F.,.F.,.F.)
B_SPLINE_SURFACE_WITH_KNOTS((2,1,2),(3,3),(-0.00286823356211971,0.,0.477902879786608),
(0.0265907346180618,0.0331702037252924),.UNSPECIFIED.)
GEOMETRIC_REPRESENTATION_ITEM()
RATIONAL_B_SPLINE_SURFACE(((0.996888414395785,0.997365765479939,0.998269846384985),
(0.996888414395785,0.997365765479939,0.998269846384985),(0.996888414395785,
0.997365765479939,0.998269846384985)))
REPRESENTATION_ITEM('')
SURFACE()
);
#394=(
BOUNDED_SURFACE()
B_SPLINE_SURFACE(1,2,((#81122,#81123,#81124),(#81125,#81126,#81127),(#81128,
#81129,#81130)),.UNSPECIFIED.,.F.,.F.,.F.)
B_SPLINE_SURFACE_WITH_KNOTS((2,1,2),(3,3),(-0.00286753128194112,0.,0.477902879786505),
(0.0166015299238958,0.0231736788111885),.UNSPECIFIED.)
GEOMETRIC_REPRESENTATION_ITEM()
RATIONAL_B_SPLINE_SURFACE(((0.996422581660833,0.996252244737342,0.996507688616404),
(0.996422581660833,0.996252244737342,0.996507688616404),(0.996422581660833,
0.996252244737342,0.996507688616404)))
REPRESENTATION_ITEM('')
SURFACE()
);
#395=(
BOUNDED_SURFACE()
B_SPLINE_SURFACE(1,2,((#81147,#81148,#81149),(#81150,#81151,#81152),(#81153,
#81154,#81155),(#81156,#81157,#81158)),.UNSPECIFIED.,.F.,.F.,.F.)
B_SPLINE_SURFACE_WITH_KNOTS((2,1,1,2),(3,3),(-0.0101,0.,1.,1.01),(0.00560769168370521,
0.0176009700440511),.UNSPECIFIED.)
GEOMETRIC_REPRESENTATION_ITEM()
RATIONAL_B_SPLINE_SURFACE(((0.998183892113821,0.99657330421516,0.996380621259469),
(0.998183892113821,0.99657330421516,0.996380621259469),(0.998183892113821,
0.99657330421516,0.996380621259469),(0.998183892113821,0.99657330421516,
0.996380621259469)))
REPRESENTATION_ITEM('')
SURFACE()
);
#396=(
BOUNDED_SURFACE()
B_SPLINE_SURFACE(1,2,((#81193,#81194,#81195),(#81196,#81197,#81198),(#81199,
#81200,#81201)),.UNSPECIFIED.,.F.,.F.,.F.)
B_SPLINE_SURFACE_WITH_KNOTS((2,1,2),(3,3),(-0.00206901892602457,0.,0.346769728497025),
(0.00660713154704112,0.0131849431469406),.UNSPECIFIED.)
GEOMETRIC_REPRESENTATION_ITEM()
RATIONAL_B_SPLINE_SURFACE(((0.997925307359487,0.997106772384945,0.996714752253855),
(0.997925307359487,0.997106772384945,0.996714752253855),(0.997925307359487,
0.997106772384945,0.996714752253855)))
REPRESENTATION_ITEM('')
SURFACE()
);
#397=(
BOUNDED_SURFACE()
B_SPLINE_SURFACE(1,2,((#81274,#81275,#81276),(#81277,#81278,#81279)),
 .UNSPECIFIED.,.F.,.F.,.F.)
B_SPLINE_SURFACE_WITH_KNOTS((2,2),(3,3),(0.,1.),(0.0556006976418426,0.067588885659051),
 .UNSPECIFIED.)
GEOMETRIC_REPRESENTATION_ITEM()
RATIONAL_B_SPLINE_SURFACE(((0.996397562408606,0.996150386832629,0.997319912843745),
(0.996397562408606,0.996150386832629,0.997319912843745)))
REPRESENTATION_ITEM('')
SURFACE()
);
#398=(
BOUNDED_SURFACE()
B_SPLINE_SURFACE(1,2,((#81348,#81349,#81350),(#81351,#81352,#81353)),
 .UNSPECIFIED.,.F.,.F.,.F.)
B_SPLINE_SURFACE_WITH_KNOTS((2,2),(3,3),(0.,1.),(0.0456081671210033,0.0575989447818814),
 .UNSPECIFIED.)
GEOMETRIC_REPRESENTATION_ITEM()
RATIONAL_B_SPLINE_SURFACE(((0.997793907739636,0.996365558499688,0.996354522974128),
(0.997793907739636,0.996365558499688,0.996354522974128)))
REPRESENTATION_ITEM('')
SURFACE()
);
#399=(
BOUNDED_SURFACE()
B_SPLINE_SURFACE(1,2,((#81420,#81421,#81422,#81423,#81424),(#81425,#81426,
#81427,#81428,#81429),(#81430,#81431,#81432,#81433,#81434)),
 .UNSPECIFIED.,.F.,.F.,.F.)
B_SPLINE_SURFACE_WITH_KNOTS((2,1,2),(3,2,3),(0.,1.,1.01),(0.0355931932713904,
0.0384615384615384,0.0476086899858126),.UNSPECIFIED.)
GEOMETRIC_REPRESENTATION_ITEM()
RATIONAL_B_SPLINE_SURFACE(((0.998993602249807,0.999456249886298,1.,0.998265981131401,
0.997356751596327),(0.998993602249807,0.999456249886298,1.,0.998265981131401,
0.997356751596327),(0.998993602249807,0.999456249886298,1.,0.998265981131401,
0.997356751596327)))
REPRESENTATION_ITEM('')
SURFACE()
);
#400=(
BOUNDED_SURFACE()
B_SPLINE_SURFACE(1,2,((#81482,#81483,#81484,#81485,#81486),(#81487,#81488,
#81489,#81490,#81491),(#81492,#81493,#81494,#81495,#81496)),
 .UNSPECIFIED.,.F.,.F.,.F.)
B_SPLINE_SURFACE_WITH_KNOTS((2,1,2),(3,2,3),(-0.00141401191198374,0.,0.480770297080743),
(0.0365944846645755,0.0384615384615384,0.0431859280915181),
 .UNSPECIFIED.)
GEOMETRIC_REPRESENTATION_ITEM()
RATIONAL_B_SPLINE_SURFACE(((0.999326490452259,0.999646063968217,1.,0.999104400890347,
0.9984288220563),(0.999326490452258,0.999646063968217,1.,0.999104400890347,
0.9984288220563),(0.999326490452258,0.999646063968217,1.,0.999104400890347,
0.9984288220563)))
REPRESENTATION_ITEM('')
SURFACE()
);
#401=(
BOUNDED_SURFACE()
B_SPLINE_SURFACE(1,2,((#81523,#81524,#81525),(#81526,#81527,#81528),(#81529,
#81530,#81531)),.UNSPECIFIED.,.F.,.F.,.F.)
B_SPLINE_SURFACE_WITH_KNOTS((2,1,2),(3,3),(0.,1.,1.01),(0.0255903596131787,
0.0375948596693867),.UNSPECIFIED.)
GEOMETRIC_REPRESENTATION_ITEM()
RATIONAL_B_SPLINE_SURFACE(((0.996753121755999,0.997505687613147,0.999678813023853),
(0.996753121755999,0.997505687613147,0.999678813023853),(0.996753121755999,
0.997505687613147,0.999678813023853)))
REPRESENTATION_ITEM('')
SURFACE()
);
#402=(
BOUNDED_SURFACE()
B_SPLINE_SURFACE(1,2,((#81566,#81567,#81568),(#81569,#81570,#81571),(#81572,
#81573,#81574)),.UNSPECIFIED.,.F.,.F.,.F.)
B_SPLINE_SURFACE_WITH_KNOTS((2,1,2),(3,3),(-0.00286823356207599,0.,0.477902879786576),
(0.0265907346180618,0.0331702037252926),.UNSPECIFIED.)
GEOMETRIC_REPRESENTATION_ITEM()
RATIONAL_B_SPLINE_SURFACE(((0.996888414395785,0.997365765479939,0.998269846384985),
(0.996888414395785,0.997365765479939,0.998269846384985),(0.996888414395785,
0.997365765479939,0.998269846384985)))
REPRESENTATION_ITEM('')
SURFACE()
);
#403=(
BOUNDED_SURFACE()
B_SPLINE_SURFACE(1,2,((#81641,#81642,#81643),(#81644,#81645,#81646),(#81647,
#81648,#81649)),.UNSPECIFIED.,.F.,.F.,.F.)
B_SPLINE_SURFACE_WITH_KNOTS((2,1,2),(3,3),(-0.00286753074348226,0.,0.477902879786661),
(0.0166015299238961,0.0231736788028833),.UNSPECIFIED.)
GEOMETRIC_REPRESENTATION_ITEM()
RATIONAL_B_SPLINE_SURFACE(((0.996422581660833,0.996252244737557,0.996507688615759),
(0.996422581660833,0.996252244737557,0.996507688615759),(0.996422581660833,
0.996252244737557,0.996507688615759)))
REPRESENTATION_ITEM('')
SURFACE()
);
#404=(
BOUNDED_SURFACE()
B_SPLINE_SURFACE(1,2,((#81666,#81667,#81668),(#81669,#81670,#81671),(#81672,
#81673,#81674),(#81675,#81676,#81677)),.UNSPECIFIED.,.F.,.F.,.F.)
B_SPLINE_SURFACE_WITH_KNOTS((2,1,1,2),(3,3),(-0.0101,0.,1.,1.01),(0.0056076916837051,
0.0176009700440511),.UNSPECIFIED.)
GEOMETRIC_REPRESENTATION_ITEM()
RATIONAL_B_SPLINE_SURFACE(((0.998183892113821,0.99657330421516,0.996380621259469),
(0.998183892113821,0.99657330421516,0.996380621259469),(0.998183892113821,
0.99657330421516,0.996380621259469),(0.998183892113821,0.99657330421516,
0.996380621259469)))
REPRESENTATION_ITEM('')
SURFACE()
);
#405=(
BOUNDED_SURFACE()
B_SPLINE_SURFACE(1,2,((#81712,#81713,#81714),(#81715,#81716,#81717),(#81718,
#81719,#81720)),.UNSPECIFIED.,.F.,.F.,.F.)
B_SPLINE_SURFACE_WITH_KNOTS((2,1,2),(3,3),(-0.0020690189259847,0.,0.346769728498705),
(0.00660713154702827,0.0131849431469338),.UNSPECIFIED.)
GEOMETRIC_REPRESENTATION_ITEM()
RATIONAL_B_SPLINE_SURFACE(((0.997925307359491,0.997106772384947,0.996714752253855),
(0.997925307359491,0.997106772384947,0.996714752253855),(0.997925307359491,
0.997106772384947,0.996714752253855)))
REPRESENTATION_ITEM('')
SURFACE()
);
#406=(
BOUNDED_SURFACE()
B_SPLINE_SURFACE(1,2,((#81793,#81794,#81795),(#81796,#81797,#81798)),
 .UNSPECIFIED.,.F.,.F.,.F.)
B_SPLINE_SURFACE_WITH_KNOTS((2,2),(3,3),(0.,1.),(0.0556006976418394,0.0675888856590496),
 .UNSPECIFIED.)
GEOMETRIC_REPRESENTATION_ITEM()
RATIONAL_B_SPLINE_SURFACE(((0.996397562408606,0.996150386832629,0.997319912843745),
(0.996397562408606,0.996150386832629,0.997319912843745)))
REPRESENTATION_ITEM('')
SURFACE()
);
#407=(
BOUNDED_SURFACE()
B_SPLINE_SURFACE(1,2,((#81867,#81868,#81869),(#81870,#81871,#81872),(#81873,
#81874,#81875)),.UNSPECIFIED.,.F.,.F.,.F.)
B_SPLINE_SURFACE_WITH_KNOTS((2,1,2),(3,3),(0.,1.,1.01),(0.0456081671210036,
0.0575989447818819),.UNSPECIFIED.)
GEOMETRIC_REPRESENTATION_ITEM()
RATIONAL_B_SPLINE_SURFACE(((0.997793907739636,0.996365558499688,0.996354522974128),
(0.997793907739636,0.996365558499688,0.996354522974128),(0.997793907739636,
0.996365558499688,0.996354522974128)))
REPRESENTATION_ITEM('')
SURFACE()
);
#408=(
BOUNDED_SURFACE()
B_SPLINE_SURFACE(1,2,((#81910,#81911,#81912),(#81913,#81914,#81915),(#81916,
#81917,#81918)),.UNSPECIFIED.,.F.,.F.,.F.)
B_SPLINE_SURFACE_WITH_KNOTS((2,1,2),(3,3),(-0.00286810173449685,0.,0.477902879786636),
(0.0466073985929117,0.0531834929157983),.UNSPECIFIED.)
GEOMETRIC_REPRESENTATION_ITEM()
RATIONAL_B_SPLINE_SURFACE(((0.997565691989291,0.996847118055593,0.996554836292953),
(0.997565691989291,0.996847118055593,0.996554836292953),(0.997565691989291,
0.996847118055593,0.996554836292953)))
REPRESENTATION_ITEM('')
SURFACE()
);
#409=(
BOUNDED_SURFACE()
B_SPLINE_SURFACE(1,2,((#81996,#81997,#81998,#81999,#82000),(#82001,#82002,
#82003,#82004,#82005)),.UNSPECIFIED.,.F.,.F.,.F.)
B_SPLINE_SURFACE_WITH_KNOTS((2,2),(3,2,3),(0.,0.480770297080763),(0.0365944846645756,
0.0384615384615384,0.0431859280915182),.UNSPECIFIED.)
GEOMETRIC_REPRESENTATION_ITEM()
RATIONAL_B_SPLINE_SURFACE(((0.999326490452258,0.999646063968217,1.,0.999104400890347,
0.9984288220563),(0.999326490452258,0.999646063968217,1.,0.999104400890347,
0.9984288220563)))
REPRESENTATION_ITEM('')
SURFACE()
);
#410=(
BOUNDED_SURFACE()
B_SPLINE_SURFACE(1,2,((#82032,#82033,#82034),(#82035,#82036,#82037),(#82038,
#82039,#82040)),.UNSPECIFIED.,.F.,.F.,.F.)
B_SPLINE_SURFACE_WITH_KNOTS((2,1,2),(3,3),(0.,1.,1.01),(0.0255903596131788,
0.0375948596693871),.UNSPECIFIED.)
GEOMETRIC_REPRESENTATION_ITEM()
RATIONAL_B_SPLINE_SURFACE(((0.996753121755999,0.997505687613148,0.999678813023853),
(0.996753121755999,0.997505687613148,0.999678813023853),(0.996753121755999,
0.997505687613148,0.999678813023853)))
REPRESENTATION_ITEM('')
SURFACE()
);
#411=(
BOUNDED_SURFACE()
B_SPLINE_SURFACE(1,2,((#82075,#82076,#82077),(#82078,#82079,#82080),(#82081,
#82082,#82083)),.UNSPECIFIED.,.F.,.F.,.F.)
B_SPLINE_SURFACE_WITH_KNOTS((2,1,2),(3,3),(-0.00286823356213975,0.,0.47790287978654),
(0.0265907346180619,0.0331702037252932),.UNSPECIFIED.)
GEOMETRIC_REPRESENTATION_ITEM()
RATIONAL_B_SPLINE_SURFACE(((0.996888414395785,0.997365765479939,0.998269846384986),
(0.996888414395785,0.997365765479939,0.998269846384986),(0.996888414395785,
0.997365765479939,0.998269846384986)))
REPRESENTATION_ITEM('')
SURFACE()
);
#412=(
BOUNDED_SURFACE()
B_SPLINE_SURFACE(1,2,((#82150,#82151,#82152),(#82153,#82154,#82155),(#82156,
#82157,#82158)),.UNSPECIFIED.,.F.,.F.,.F.)
B_SPLINE_SURFACE_WITH_KNOTS((2,1,2),(3,3),(-0.00286753128198799,0.,0.477902879786589),
(0.0166015299238963,0.023173678811189),.UNSPECIFIED.)
GEOMETRIC_REPRESENTATION_ITEM()
RATIONAL_B_SPLINE_SURFACE(((0.996422581660833,0.996252244737342,0.996507688616404),
(0.996422581660833,0.996252244737342,0.996507688616404),(0.996422581660833,
0.996252244737342,0.996507688616404)))
REPRESENTATION_ITEM('')
SURFACE()
);
#413=(
BOUNDED_SURFACE()
B_SPLINE_SURFACE(1,2,((#82175,#82176,#82177),(#82178,#82179,#82180),(#82181,
#82182,#82183),(#82184,#82185,#82186)),.UNSPECIFIED.,.F.,.F.,.F.)
B_SPLINE_SURFACE_WITH_KNOTS((2,1,1,2),(3,3),(-0.0101,0.,1.,1.01),(0.00560769168370525,
0.0176009700440511),.UNSPECIFIED.)
GEOMETRIC_REPRESENTATION_ITEM()
RATIONAL_B_SPLINE_SURFACE(((0.99818389211382,0.99657330421516,0.996380621259469),
(0.99818389211382,0.99657330421516,0.996380621259469),(0.99818389211382,
0.99657330421516,0.996380621259469),(0.99818389211382,0.99657330421516,
0.996380621259469)))
REPRESENTATION_ITEM('')
SURFACE()
);
#414=(
BOUNDED_SURFACE()
B_SPLINE_SURFACE(1,2,((#82221,#82222,#82223),(#82224,#82225,#82226),(#82227,
#82228,#82229)),.UNSPECIFIED.,.F.,.F.,.F.)
B_SPLINE_SURFACE_WITH_KNOTS((2,1,2),(3,3),(-0.00206901892598934,0.,0.346769728500098),
(0.00660713154701696,0.0131849431469243),.UNSPECIFIED.)
GEOMETRIC_REPRESENTATION_ITEM()
RATIONAL_B_SPLINE_SURFACE(((0.997925307359493,0.997106772384949,0.996714752253856),
(0.997925307359493,0.997106772384949,0.996714752253856),(0.997925307359494,
0.997106772384949,0.996714752253856)))
REPRESENTATION_ITEM('')
SURFACE()
);
#415=(
BOUNDED_SURFACE()
B_SPLINE_SURFACE(1,2,((#82302,#82303,#82304),(#82305,#82306,#82307)),
 .UNSPECIFIED.,.F.,.F.,.F.)
B_SPLINE_SURFACE_WITH_KNOTS((2,2),(3,3),(0.,1.),(0.0556006976418415,0.0675888856590506),
 .UNSPECIFIED.)
GEOMETRIC_REPRESENTATION_ITEM()
RATIONAL_B_SPLINE_SURFACE(((0.996397562408606,0.996150386832629,0.997319912843745),
(0.996397562408606,0.996150386832629,0.997319912843745)))
REPRESENTATION_ITEM('')
SURFACE()
);
#416=(
BOUNDED_SURFACE()
B_SPLINE_SURFACE(1,2,((#82376,#82377,#82378),(#82379,#82380,#82381),(#82382,
#82383,#82384)),.UNSPECIFIED.,.F.,.F.,.F.)
B_SPLINE_SURFACE_WITH_KNOTS((2,1,2),(3,3),(0.,1.,1.01),(0.0456081671210023,
0.057598944781881),.UNSPECIFIED.)
GEOMETRIC_REPRESENTATION_ITEM()
RATIONAL_B_SPLINE_SURFACE(((0.997793907739637,0.996365558499688,0.996354522974128),
(0.997793907739637,0.996365558499688,0.996354522974128),(0.997793907739637,
0.996365558499688,0.996354522974128)))
REPRESENTATION_ITEM('')
SURFACE()
);
#417=(
BOUNDED_SURFACE()
B_SPLINE_SURFACE(1,2,((#82419,#82420,#82421),(#82422,#82423,#82424),(#82425,
#82426,#82427)),.UNSPECIFIED.,.F.,.F.,.F.)
B_SPLINE_SURFACE_WITH_KNOTS((2,1,2),(3,3),(-0.00286810173498889,0.,0.477902879865112),
(0.0466073985929115,0.0531834929157973),.UNSPECIFIED.)
GEOMETRIC_REPRESENTATION_ITEM()
RATIONAL_B_SPLINE_SURFACE(((0.997565691989291,0.996847118055594,0.996554836292953),
(0.997565691989291,0.996847118055594,0.996554836292953),(0.997565691989291,
0.996847118055593,0.996554836292953)))
REPRESENTATION_ITEM('')
SURFACE()
);
#418=(
BOUNDED_SURFACE()
B_SPLINE_SURFACE(1,2,((#82444,#82445,#82446,#82447,#82448),(#82449,#82450,
#82451,#82452,#82453),(#82454,#82455,#82456,#82457,#82458)),
 .UNSPECIFIED.,.F.,.F.,.F.)
B_SPLINE_SURFACE_WITH_KNOTS((2,1,2),(3,2,3),(0.,1.,1.01),(0.0355931932713904,
0.0384615384615384,0.0476086899858127),.UNSPECIFIED.)
GEOMETRIC_REPRESENTATION_ITEM()
RATIONAL_B_SPLINE_SURFACE(((0.998993602249807,0.999456249886298,1.,0.998265981131401,
0.997356751596327),(0.998993602249807,0.999456249886298,1.,0.998265981131401,
0.997356751596327),(0.998993602249807,0.999456249886298,1.,0.998265981131401,
0.997356751596327)))
REPRESENTATION_ITEM('')
SURFACE()
);
#419=(
BOUNDED_SURFACE()
B_SPLINE_SURFACE(1,2,((#82506,#82507,#82508,#82509,#82510),(#82511,#82512,
#82513,#82514,#82515),(#82516,#82517,#82518,#82519,#82520)),
 .UNSPECIFIED.,.F.,.F.,.F.)
B_SPLINE_SURFACE_WITH_KNOTS((2,1,2),(3,2,3),(-0.00141401191196798,0.,0.480770297080667),
(0.0365944846645755,0.0384615384615384,0.0431859280915186),
 .UNSPECIFIED.)
GEOMETRIC_REPRESENTATION_ITEM()
RATIONAL_B_SPLINE_SURFACE(((0.999326490452258,0.999646063968217,1.,0.999104400890347,
0.9984288220563),(0.999326490452259,0.999646063968217,1.,0.999104400890347,
0.9984288220563),(0.999326490452259,0.999646063968217,1.,0.999104400890347,
0.9984288220563)))
REPRESENTATION_ITEM('')
SURFACE()
);
#420=(
BOUNDED_SURFACE()
B_SPLINE_SURFACE(1,2,((#82547,#82548,#82549),(#82550,#82551,#82552)),
 .UNSPECIFIED.,.F.,.F.,.F.)
B_SPLINE_SURFACE_WITH_KNOTS((2,2),(3,3),(0.,1.),(0.0255903596131801,0.0375948596693865),
 .UNSPECIFIED.)
GEOMETRIC_REPRESENTATION_ITEM()
RATIONAL_B_SPLINE_SURFACE(((0.996753121755999,0.997505687613148,0.999678813023853),
(0.996753121755999,0.997505687613148,0.999678813023853)))
REPRESENTATION_ITEM('')
SURFACE()
);
#421=(
BOUNDED_SURFACE()
B_SPLINE_SURFACE(1,2,((#82669,#82670,#82671),(#82672,#82673,#82674),(#82675,
#82676,#82677)),.UNSPECIFIED.,.F.,.F.,.F.)
B_SPLINE_SURFACE_WITH_KNOTS((2,1,2),(3,3),(-0.00286753074352407,0.,0.477902879786511),
(0.0166015299238963,0.0231736788028833),.UNSPECIFIED.)
GEOMETRIC_REPRESENTATION_ITEM()
RATIONAL_B_SPLINE_SURFACE(((0.996422581660833,0.996252244737557,0.996507688615759),
(0.996422581660833,0.996252244737557,0.996507688615759),(0.996422581660833,
0.996252244737557,0.996507688615759)))
REPRESENTATION_ITEM('')
SURFACE()
);
#422=(
BOUNDED_SURFACE()
B_SPLINE_SURFACE(1,2,((#82694,#82695,#82696),(#82697,#82698,#82699),(#82700,
#82701,#82702),(#82703,#82704,#82705)),.UNSPECIFIED.,.F.,.F.,.F.)
B_SPLINE_SURFACE_WITH_KNOTS((2,1,1,2),(3,3),(-0.0101,0.,1.,1.01),(0.00560769168370406,
0.0176009700440506),.UNSPECIFIED.)
GEOMETRIC_REPRESENTATION_ITEM()
RATIONAL_B_SPLINE_SURFACE(((0.998183892113821,0.99657330421516,0.996380621259469),
(0.998183892113821,0.99657330421516,0.996380621259469),(0.998183892113821,
0.99657330421516,0.996380621259469),(0.998183892113821,0.99657330421516,
0.996380621259469)))
REPRESENTATION_ITEM('')
SURFACE()
);
#423=(
BOUNDED_SURFACE()
B_SPLINE_SURFACE(1,2,((#82740,#82741,#82742),(#82743,#82744,#82745),(#82746,
#82747,#82748)),.UNSPECIFIED.,.F.,.F.,.F.)
B_SPLINE_SURFACE_WITH_KNOTS((2,1,2),(3,3),(-0.00206901892599668,0.,0.346769728501626),
(0.0066071315470067,0.013184943146863),.UNSPECIFIED.)
GEOMETRIC_REPRESENTATION_ITEM()
RATIONAL_B_SPLINE_SURFACE(((0.997925307359496,0.997106772384957,0.996714752253863),
(0.997925307359496,0.997106772384957,0.996714752253863),(0.997925307359496,
0.997106772384957,0.996714752253863)))
REPRESENTATION_ITEM('')
SURFACE()
);
#424=(
BOUNDED_SURFACE()
B_SPLINE_SURFACE(1,2,((#82821,#82822,#82823),(#82824,#82825,#82826)),
 .UNSPECIFIED.,.F.,.F.,.F.)
B_SPLINE_SURFACE_WITH_KNOTS((2,2),(3,3),(0.,1.),(0.0556006976418438,0.0675888856590503),
 .UNSPECIFIED.)
GEOMETRIC_REPRESENTATION_ITEM()
RATIONAL_B_SPLINE_SURFACE(((0.996397562408606,0.996150386832629,0.997319912843745),
(0.996397562408606,0.996150386832629,0.997319912843745)))
REPRESENTATION_ITEM('')
SURFACE()
);
#425=(
BOUNDED_SURFACE()
B_SPLINE_SURFACE(1,2,((#82895,#82896,#82897),(#82898,#82899,#82900),(#82901,
#82902,#82903)),.UNSPECIFIED.,.F.,.F.,.F.)
B_SPLINE_SURFACE_WITH_KNOTS((2,1,2),(3,3),(0.,1.,1.01),(0.0456081671210055,
0.0575989447818814),.UNSPECIFIED.)
GEOMETRIC_REPRESENTATION_ITEM()
RATIONAL_B_SPLINE_SURFACE(((0.997793907739636,0.996365558499688,0.996354522974128),
(0.997793907739636,0.996365558499688,0.996354522974128),(0.997793907739636,
0.996365558499688,0.996354522974128)))
REPRESENTATION_ITEM('')
SURFACE()
);
#426=(
BOUNDED_SURFACE()
B_SPLINE_SURFACE(1,2,((#82938,#82939,#82940),(#82941,#82942,#82943),(#82944,
#82945,#82946)),.UNSPECIFIED.,.F.,.F.,.F.)
B_SPLINE_SURFACE_WITH_KNOTS((2,1,2),(3,3),(-0.00286810173450747,0.,0.477902879789481),
(0.046607398592912,0.0531834929157981),.UNSPECIFIED.)
GEOMETRIC_REPRESENTATION_ITEM()
RATIONAL_B_SPLINE_SURFACE(((0.997565691989291,0.996847118055593,0.996554836292953),
(0.997565691989291,0.996847118055593,0.996554836292953),(0.997565691989291,
0.996847118055593,0.996554836292953)))
REPRESENTATION_ITEM('')
SURFACE()
);
#427=(
BOUNDED_SURFACE()
B_SPLINE_SURFACE(1,2,((#82963,#82964,#82965,#82966,#82967),(#82968,#82969,
#82970,#82971,#82972),(#82973,#82974,#82975,#82976,#82977)),
 .UNSPECIFIED.,.F.,.F.,.F.)
B_SPLINE_SURFACE_WITH_KNOTS((2,1,2),(3,2,3),(0.,1.,1.01),(0.0355931932713904,
0.0384615384615384,0.0476086899858121),.UNSPECIFIED.)
GEOMETRIC_REPRESENTATION_ITEM()
RATIONAL_B_SPLINE_SURFACE(((0.998993602249807,0.999456249886298,1.,0.998265981131401,
0.997356751596327),(0.998993602249807,0.999456249886298,1.,0.998265981131401,
0.997356751596327),(0.998993602249807,0.999456249886298,1.,0.998265981131401,
0.997356751596327)))
REPRESENTATION_ITEM('')
SURFACE()
);
#428=(
BOUNDED_SURFACE()
B_SPLINE_SURFACE(1,2,((#83025,#83026,#83027,#83028,#83029),(#83030,#83031,
#83032,#83033,#83034),(#83035,#83036,#83037,#83038,#83039)),
 .UNSPECIFIED.,.F.,.F.,.F.)
B_SPLINE_SURFACE_WITH_KNOTS((2,1,2),(3,2,3),(-0.00141401191198176,0.,0.480770297081945),
(0.0365944846645797,0.0384615384615384,0.0431859280915184),
 .UNSPECIFIED.)
GEOMETRIC_REPRESENTATION_ITEM()
RATIONAL_B_SPLINE_SURFACE(((0.99932649045226,0.999646063968218,1.,0.999104400890347,
0.9984288220563),(0.99932649045226,0.999646063968218,1.,0.999104400890347,
0.9984288220563),(0.99932649045226,0.999646063968218,1.,0.999104400890347,
0.9984288220563)))
REPRESENTATION_ITEM('')
SURFACE()
);
#429=(
BOUNDED_SURFACE()
B_SPLINE_SURFACE(1,2,((#83066,#83067,#83068),(#83069,#83070,#83071),(#83072,
#83073,#83074)),.UNSPECIFIED.,.F.,.F.,.F.)
B_SPLINE_SURFACE_WITH_KNOTS((2,1,2),(3,3),(0.,1.,1.01),(0.0255903596131819,
0.0375948596693879),.UNSPECIFIED.)
GEOMETRIC_REPRESENTATION_ITEM()
RATIONAL_B_SPLINE_SURFACE(((0.996753121755999,0.997505687613148,0.999678813023854),
(0.996753121755999,0.997505687613148,0.999678813023854),(0.996753121755999,
0.997505687613148,0.999678813023854)))
REPRESENTATION_ITEM('')
SURFACE()
);
#430=(
BOUNDED_SURFACE()
B_SPLINE_SURFACE(1,2,((#83109,#83110,#83111),(#83112,#83113,#83114),(#83115,
#83116,#83117)),.UNSPECIFIED.,.F.,.F.,.F.)
B_SPLINE_SURFACE_WITH_KNOTS((2,1,2),(3,3),(-0.00286823356200407,0.,0.477902879786893),
(0.0265907346180622,0.033170203725293),.UNSPECIFIED.)
GEOMETRIC_REPRESENTATION_ITEM()
RATIONAL_B_SPLINE_SURFACE(((0.996888414395785,0.997365765479939,0.998269846384985),
(0.996888414395785,0.997365765479939,0.998269846384985),(0.996888414395785,
0.997365765479939,0.998269846384985)))
REPRESENTATION_ITEM('')
SURFACE()
);
#431=(
BOUNDED_SURFACE()
B_SPLINE_SURFACE(1,2,((#83216,#83217,#83218),(#83219,#83220,#83221),(#83222,
#83223,#83224),(#83225,#83226,#83227)),.UNSPECIFIED.,.F.,.F.,.F.)
B_SPLINE_SURFACE_WITH_KNOTS((2,1,1,2),(3,3),(-0.0101,0.,1.,1.01),(0.00560769168370728,
0.0176009700440516),.UNSPECIFIED.)
GEOMETRIC_REPRESENTATION_ITEM()
RATIONAL_B_SPLINE_SURFACE(((0.99818389211382,0.99657330421516,0.996380621259469),
(0.99818389211382,0.99657330421516,0.996380621259469),(0.99818389211382,
0.99657330421516,0.996380621259469),(0.99818389211382,0.99657330421516,
0.996380621259469)))
REPRESENTATION_ITEM('')
SURFACE()
);
#432=(
BOUNDED_SURFACE()
B_SPLINE_SURFACE(1,2,((#83262,#83263,#83264),(#83265,#83266,#83267),(#83268,
#83269,#83270)),.UNSPECIFIED.,.F.,.F.,.F.)
B_SPLINE_SURFACE_WITH_KNOTS((2,1,2),(3,3),(-0.00206901892604864,0.,0.346769728503092),
(0.00660713154699752,0.0131849431469057),.UNSPECIFIED.)
GEOMETRIC_REPRESENTATION_ITEM()
RATIONAL_B_SPLINE_SURFACE(((0.997925307359498,0.997106772384952,0.996714752253859),
(0.997925307359498,0.997106772384952,0.996714752253859),(0.997925307359498,
0.997106772384952,0.996714752253858)))
REPRESENTATION_ITEM('')
SURFACE()
);
#433=(
BOUNDED_SURFACE()
B_SPLINE_SURFACE(1,2,((#83343,#83344,#83345),(#83346,#83347,#83348)),
 .UNSPECIFIED.,.F.,.F.,.F.)
B_SPLINE_SURFACE_WITH_KNOTS((2,2),(3,3),(0.,1.),(0.0556006976418438,0.0675888856590507),
 .UNSPECIFIED.)
GEOMETRIC_REPRESENTATION_ITEM()
RATIONAL_B_SPLINE_SURFACE(((0.996397562408606,0.996150386832629,0.997319912843745),
(0.996397562408606,0.996150386832629,0.997319912843745)))
REPRESENTATION_ITEM('')
SURFACE()
);
#434=(
BOUNDED_SURFACE()
B_SPLINE_SURFACE(1,2,((#83417,#83418,#83419),(#83420,#83421,#83422),(#83423,
#83424,#83425)),.UNSPECIFIED.,.F.,.F.,.F.)
B_SPLINE_SURFACE_WITH_KNOTS((2,1,2),(3,3),(0.,1.,1.01),(0.0456081671210054,
0.0575989447818828),.UNSPECIFIED.)
GEOMETRIC_REPRESENTATION_ITEM()
RATIONAL_B_SPLINE_SURFACE(((0.997793907739636,0.996365558499688,0.996354522974128),
(0.997793907739636,0.996365558499688,0.996354522974128),(0.997793907739636,
0.996365558499688,0.996354522974128)))
REPRESENTATION_ITEM('')
SURFACE()
);
#435=(
BOUNDED_SURFACE()
B_SPLINE_SURFACE(1,2,((#83460,#83461,#83462),(#83463,#83464,#83465),(#83466,
#83467,#83468)),.UNSPECIFIED.,.F.,.F.,.F.)
B_SPLINE_SURFACE_WITH_KNOTS((2,1,2),(3,3),(-0.00286810173452563,0.,0.477902879792037),
(0.0466073985929119,0.0531834929157979),.UNSPECIFIED.)
GEOMETRIC_REPRESENTATION_ITEM()
RATIONAL_B_SPLINE_SURFACE(((0.997565691989291,0.996847118055594,0.996554836292953),
(0.997565691989291,0.996847118055594,0.996554836292953),(0.997565691989291,
0.996847118055594,0.996554836292953)))
REPRESENTATION_ITEM('')
SURFACE()
);
#436=(
BOUNDED_SURFACE()
B_SPLINE_SURFACE(1,2,((#83485,#83486,#83487,#83488,#83489),(#83490,#83491,
#83492,#83493,#83494),(#83495,#83496,#83497,#83498,#83499)),
 .UNSPECIFIED.,.F.,.F.,.F.)
B_SPLINE_SURFACE_WITH_KNOTS((2,1,2),(3,2,3),(0.,1.,1.01),(0.0355931932713903,
0.0384615384615384,0.0476086899858139),.UNSPECIFIED.)
GEOMETRIC_REPRESENTATION_ITEM()
RATIONAL_B_SPLINE_SURFACE(((0.998993602249807,0.999456249886298,1.,0.998265981131401,
0.997356751596327),(0.998993602249807,0.999456249886298,1.,0.998265981131401,
0.997356751596327),(0.998993602249807,0.999456249886298,1.,0.998265981131401,
0.997356751596327)))
REPRESENTATION_ITEM('')
SURFACE()
);
#437=(
BOUNDED_SURFACE()
B_SPLINE_SURFACE(1,2,((#83547,#83548,#83549,#83550,#83551),(#83552,#83553,
#83554,#83555,#83556),(#83557,#83558,#83559,#83560,#83561)),
 .UNSPECIFIED.,.F.,.F.,.F.)
B_SPLINE_SURFACE_WITH_KNOTS((2,1,2),(3,2,3),(-0.00141401191198388,0.,0.480770297084423),
(0.0365944846645751,0.0384615384615384,0.0431859280915186),
 .UNSPECIFIED.)
GEOMETRIC_REPRESENTATION_ITEM()
RATIONAL_B_SPLINE_SURFACE(((0.999326490452258,0.999646063968217,1.,0.999104400890347,
0.9984288220563),(0.999326490452258,0.999646063968217,1.,0.999104400890347,
0.9984288220563),(0.999326490452258,0.999646063968217,1.,0.999104400890347,
0.9984288220563)))
REPRESENTATION_ITEM('')
SURFACE()
);
#438=(
BOUNDED_SURFACE()
B_SPLINE_SURFACE(1,2,((#83588,#83589,#83590),(#83591,#83592,#83593),(#83594,
#83595,#83596)),.UNSPECIFIED.,.F.,.F.,.F.)
B_SPLINE_SURFACE_WITH_KNOTS((2,1,2),(3,3),(0.,1.,1.01),(0.0255903596131801,
0.0375948596693865),.UNSPECIFIED.)
GEOMETRIC_REPRESENTATION_ITEM()
RATIONAL_B_SPLINE_SURFACE(((0.996753121755999,0.997505687613148,0.999678813023853),
(0.996753121755999,0.997505687613148,0.999678813023853),(0.996753121755999,
0.997505687613148,0.999678813023853)))
REPRESENTATION_ITEM('')
SURFACE()
);
#439=(
BOUNDED_SURFACE()
B_SPLINE_SURFACE(1,2,((#83631,#83632,#83633),(#83634,#83635,#83636),(#83637,
#83638,#83639)),.UNSPECIFIED.,.F.,.F.,.F.)
B_SPLINE_SURFACE_WITH_KNOTS((2,1,2),(3,3),(-0.00286823045906607,0.,0.477902879789481),
(0.0265907346180612,0.0331702036774533),.UNSPECIFIED.)
GEOMETRIC_REPRESENTATION_ITEM()
RATIONAL_B_SPLINE_SURFACE(((0.996888414395785,0.997365765476469,0.998269846371838),
(0.996888414395785,0.997365765476469,0.998269846371838),(0.996888414395785,
0.997365765476469,0.998269846371838)))
REPRESENTATION_ITEM('')
SURFACE()
);
#440=(
BOUNDED_SURFACE()
B_SPLINE_SURFACE(1,2,((#83706,#83707,#83708),(#83709,#83710,#83711),(#83712,
#83713,#83714)),.UNSPECIFIED.,.F.,.F.,.F.)
B_SPLINE_SURFACE_WITH_KNOTS((2,1,2),(3,3),(-0.00286753114037982,0.,0.47790287978806),
(0.016601529923896,0.0231736788090044),.UNSPECIFIED.)
GEOMETRIC_REPRESENTATION_ITEM()
RATIONAL_B_SPLINE_SURFACE(((0.996422581660833,0.996252244737399,0.996507688616235),
(0.996422581660833,0.996252244737399,0.996507688616235),(0.996422581660833,
0.996252244737399,0.996507688616235)))
REPRESENTATION_ITEM('')
SURFACE()
);
#441=(
BOUNDED_SURFACE()
B_SPLINE_SURFACE(1,2,((#83731,#83732,#83733),(#83734,#83735,#83736),(#83737,
#83738,#83739)),.UNSPECIFIED.,.F.,.F.,.F.)
B_SPLINE_SURFACE_WITH_KNOTS((2,1,2),(3,3),(-0.01,0.,1.00000001523928),(0.0056076916837061,
0.0176009700440528),.UNSPECIFIED.)
GEOMETRIC_REPRESENTATION_ITEM()
RATIONAL_B_SPLINE_SURFACE(((0.99818389211382,0.99657330421516,0.996380621259469),
(0.99818389211382,0.99657330421516,0.996380621259469),(0.99818389211382,
0.99657330421516,0.996380621259469)))
REPRESENTATION_ITEM('')
SURFACE()
);
#442=(
BOUNDED_SURFACE()
B_SPLINE_SURFACE(1,2,((#83862,#83863,#83864),(#83865,#83866,#83867)),
 .UNSPECIFIED.,.F.,.F.,.F.)
B_SPLINE_SURFACE_WITH_KNOTS((2,2),(3,3),(0.,1.),(0.0556006976418436,0.0675888856590519),
 .UNSPECIFIED.)
GEOMETRIC_REPRESENTATION_ITEM()
RATIONAL_B_SPLINE_SURFACE(((0.996397562408606,0.996150386832629,0.997319912843745),
(0.996397562408606,0.996150386832629,0.997319912843745)))
REPRESENTATION_ITEM('')
SURFACE()
);
#443=(
BOUNDED_SURFACE()
B_SPLINE_SURFACE(1,2,((#83936,#83937,#83938),(#83939,#83940,#83941),(#83942,
#83943,#83944)),.UNSPECIFIED.,.F.,.F.,.F.)
B_SPLINE_SURFACE_WITH_KNOTS((2,1,2),(3,3),(0.,1.,1.01),(0.0456081671210043,
0.057598944781883),.UNSPECIFIED.)
GEOMETRIC_REPRESENTATION_ITEM()
RATIONAL_B_SPLINE_SURFACE(((0.997793907739636,0.996365558499688,0.996354522974128),
(0.997793907739636,0.996365558499688,0.996354522974128),(0.997793907739636,
0.996365558499688,0.996354522974128)))
REPRESENTATION_ITEM('')
SURFACE()
);
#444=(
BOUNDED_SURFACE()
B_SPLINE_SURFACE(1,2,((#83979,#83980,#83981),(#83982,#83983,#83984),(#83985,
#83986,#83987)),.UNSPECIFIED.,.F.,.F.,.F.)
B_SPLINE_SURFACE_WITH_KNOTS((2,1,2),(3,3),(-0.00286810173457896,0.,0.477902879794604),
(0.0466073985929109,0.0531834929157975),.UNSPECIFIED.)
GEOMETRIC_REPRESENTATION_ITEM()
RATIONAL_B_SPLINE_SURFACE(((0.997565691989291,0.996847118055594,0.996554836292953),
(0.997565691989291,0.996847118055594,0.996554836292953),(0.997565691989291,
0.996847118055594,0.996554836292953)))
REPRESENTATION_ITEM('')
SURFACE()
);
#445=(
BOUNDED_SURFACE()
B_SPLINE_SURFACE(1,2,((#84004,#84005,#84006,#84007,#84008),(#84009,#84010,
#84011,#84012,#84013),(#84014,#84015,#84016,#84017,#84018)),
 .UNSPECIFIED.,.F.,.F.,.F.)
B_SPLINE_SURFACE_WITH_KNOTS((2,1,2),(3,2,3),(0.,1.,1.01),(0.0355931932713903,
0.0384615384615384,0.0476086899858138),.UNSPECIFIED.)
GEOMETRIC_REPRESENTATION_ITEM()
RATIONAL_B_SPLINE_SURFACE(((0.998993602249807,0.999456249886298,1.,0.998265981131401,
0.997356751596327),(0.998993602249807,0.999456249886298,1.,0.998265981131401,
0.997356751596327),(0.998993602249807,0.999456249886298,1.,0.998265981131401,
0.997356751596327)))
REPRESENTATION_ITEM('')
SURFACE()
);
#446=(
BOUNDED_SURFACE()
B_SPLINE_SURFACE(1,2,((#84066,#84067,#84068,#84069,#84070),(#84071,#84072,
#84073,#84074,#84075),(#84076,#84077,#84078,#84079,#84080)),
 .UNSPECIFIED.,.F.,.F.,.F.)
B_SPLINE_SURFACE_WITH_KNOTS((2,1,2),(3,2,3),(-0.00286743096746644,0.,0.480770297153185),
(0.0365944846641764,0.0384615384615384,0.0431859280915206),
 .UNSPECIFIED.)
GEOMETRIC_REPRESENTATION_ITEM()
RATIONAL_B_SPLINE_SURFACE(((0.999326490452122,0.999646063968141,1.,0.999104400890346,
0.998428822056299),(0.999326490452122,0.999646063968141,1.,0.999104400890346,
0.998428822056299),(0.999326490452122,0.999646063968141,1.,0.999104400890346,
0.998428822056299)))
REPRESENTATION_ITEM('')
SURFACE()
);
#447=(
BOUNDED_SURFACE()
B_SPLINE_SURFACE(1,2,((#84107,#84108,#84109),(#84110,#84111,#84112),(#84113,
#84114,#84115)),.UNSPECIFIED.,.F.,.F.,.F.)
B_SPLINE_SURFACE_WITH_KNOTS((2,1,2),(3,3),(0.,1.,1.01),(0.0255903596131786,
0.0375948596693872),.UNSPECIFIED.)
GEOMETRIC_REPRESENTATION_ITEM()
RATIONAL_B_SPLINE_SURFACE(((0.996753121755999,0.997505687613147,0.999678813023853),
(0.996753121755999,0.997505687613147,0.999678813023853),(0.996753121755999,
0.997505687613147,0.999678813023853)))
REPRESENTATION_ITEM('')
SURFACE()
);
#448=(
BOUNDED_SURFACE()
B_SPLINE_SURFACE(1,2,((#84150,#84151,#84152),(#84153,#84154,#84155),(#84156,
#84157,#84158)),.UNSPECIFIED.,.F.,.F.,.F.)
B_SPLINE_SURFACE_WITH_KNOTS((2,1,2),(3,3),(-0.00286823356217506,0.,0.477902879792038),
(0.0265907346180622,0.0331702037252929),.UNSPECIFIED.)
GEOMETRIC_REPRESENTATION_ITEM()
RATIONAL_B_SPLINE_SURFACE(((0.996888414395785,0.997365765479939,0.998269846384985),
(0.996888414395785,0.997365765479939,0.998269846384985),(0.996888414395785,
0.997365765479939,0.998269846384985)))
REPRESENTATION_ITEM('')
SURFACE()
);
#449=(
BOUNDED_SURFACE()
B_SPLINE_SURFACE(1,2,((#84225,#84226,#84227),(#84228,#84229,#84230),(#84231,
#84232,#84233)),.UNSPECIFIED.,.F.,.F.,.F.)
B_SPLINE_SURFACE_WITH_KNOTS((2,1,2),(3,3),(-0.00286753114037473,0.,0.477902879790725),
(0.0166015299238962,0.0231736788090045),.UNSPECIFIED.)
GEOMETRIC_REPRESENTATION_ITEM()
RATIONAL_B_SPLINE_SURFACE(((0.996422581660833,0.996252244737398,0.996507688616234),
(0.996422581660833,0.996252244737398,0.996507688616234),(0.996422581660833,
0.996252244737399,0.996507688616235)))
REPRESENTATION_ITEM('')
SURFACE()
);
#450=(
BOUNDED_SURFACE()
B_SPLINE_SURFACE(1,2,((#84250,#84251,#84252),(#84253,#84254,#84255),(#84256,
#84257,#84258),(#84259,#84260,#84261)),.UNSPECIFIED.,.F.,.F.,.F.)
B_SPLINE_SURFACE_WITH_KNOTS((2,1,1,2),(3,3),(-0.0101,0.,1.,1.01),(0.00560769168370621,
0.0176009700440521),.UNSPECIFIED.)
GEOMETRIC_REPRESENTATION_ITEM()
RATIONAL_B_SPLINE_SURFACE(((0.99818389211382,0.99657330421516,0.996380621259469),
(0.99818389211382,0.99657330421516,0.996380621259469),(0.99818389211382,
0.99657330421516,0.996380621259469),(0.99818389211382,0.99657330421516,
0.996380621259469)))
REPRESENTATION_ITEM('')
SURFACE()
);
#451=(
BOUNDED_SURFACE()
B_SPLINE_SURFACE(1,2,((#84296,#84297,#84298),(#84299,#84300,#84301),(#84302,
#84303,#84304)),.UNSPECIFIED.,.F.,.F.,.F.)
B_SPLINE_SURFACE_WITH_KNOTS((2,1,2),(3,3),(-0.0020690189260231,0.,0.346769728505991),
(0.00660713154698392,0.0131849431468902),.UNSPECIFIED.)
GEOMETRIC_REPRESENTATION_ITEM()
RATIONAL_B_SPLINE_SURFACE(((0.997925307359502,0.997106772384955,0.996714752253861),
(0.997925307359502,0.997106772384955,0.996714752253861),(0.997925307359502,
0.997106772384955,0.996714752253861)))
REPRESENTATION_ITEM('')
SURFACE()
);
#452=(
BOUNDED_SURFACE()
B_SPLINE_SURFACE(1,2,((#84377,#84378,#84379),(#84380,#84381,#84382)),
 .UNSPECIFIED.,.F.,.F.,.F.)
B_SPLINE_SURFACE_WITH_KNOTS((2,2),(3,3),(0.,1.),(0.0556006976418385,0.0675888856590485),
 .UNSPECIFIED.)
GEOMETRIC_REPRESENTATION_ITEM()
RATIONAL_B_SPLINE_SURFACE(((0.996397562408606,0.996150386832629,0.997319912843744),
(0.996397562408606,0.996150386832629,0.997319912843744)))
REPRESENTATION_ITEM('')
SURFACE()
);
#453=(
BOUNDED_SURFACE()
B_SPLINE_SURFACE(1,2,((#84451,#84452,#84453),(#84454,#84455,#84456),(#84457,
#84458,#84459)),.UNSPECIFIED.,.F.,.F.,.F.)
B_SPLINE_SURFACE_WITH_KNOTS((2,1,2),(3,3),(0.,1.,1.01),(0.0456081671210087,
0.057598944781882),.UNSPECIFIED.)
GEOMETRIC_REPRESENTATION_ITEM()
RATIONAL_B_SPLINE_SURFACE(((0.997793907739635,0.996365558499688,0.996354522974128),
(0.997793907739635,0.996365558499688,0.996354522974128),(0.997793907739635,
0.996365558499688,0.996354522974128)))
REPRESENTATION_ITEM('')
SURFACE()
);
#454=(
BOUNDED_SURFACE()
B_SPLINE_SURFACE(1,2,((#84494,#84495,#84496),(#84497,#84498,#84499),(#84500,
#84501,#84502)),.UNSPECIFIED.,.F.,.F.,.F.)
B_SPLINE_SURFACE_WITH_KNOTS((2,1,2),(3,3),(-0.0028681017194608,0.,0.477902879797066),
(0.046607398592912,0.0531834927425532),.UNSPECIFIED.)
GEOMETRIC_REPRESENTATION_ITEM()
RATIONAL_B_SPLINE_SURFACE(((0.997565691989291,0.996847118074524,0.996554836308353),
(0.997565691989291,0.996847118074524,0.996554836308353),(0.997565691989291,
0.996847118074524,0.996554836308353)))
REPRESENTATION_ITEM('')
SURFACE()
);
#455=(
BOUNDED_SURFACE()
B_SPLINE_SURFACE(1,2,((#84519,#84520,#84521,#84522,#84523),(#84524,#84525,
#84526,#84527,#84528),(#84529,#84530,#84531,#84532,#84533)),
 .UNSPECIFIED.,.F.,.F.,.F.)
B_SPLINE_SURFACE_WITH_KNOTS((2,1,2),(3,2,3),(0.,1.,1.01),(0.0355931932713903,
0.0384615384615384,0.0476086899858133),.UNSPECIFIED.)
GEOMETRIC_REPRESENTATION_ITEM()
RATIONAL_B_SPLINE_SURFACE(((0.998993602249807,0.999456249886298,1.,0.998265981131401,
0.997356751596327),(0.998993602249807,0.999456249886298,1.,0.998265981131401,
0.997356751596327),(0.998993602249807,0.999456249886298,1.,0.998265981131401,
0.997356751596327)))
REPRESENTATION_ITEM('')
SURFACE()
);
#456=(
BOUNDED_SURFACE()
B_SPLINE_SURFACE(1,2,((#84581,#84582,#84583,#84584,#84585),(#84586,#84587,
#84588,#84589,#84590),(#84591,#84592,#84593,#84594,#84595)),
 .UNSPECIFIED.,.F.,.F.,.F.)
B_SPLINE_SURFACE_WITH_KNOTS((2,1,2),(3,2,3),(-0.00286742665919738,0.,0.480770297130077),
(0.036594484664175,0.0384615384615384,0.0431859280915206),.UNSPECIFIED.)
GEOMETRIC_REPRESENTATION_ITEM()
RATIONAL_B_SPLINE_SURFACE(((0.999326490452121,0.99964606396814,1.,0.999104400890346,
0.998428822056299),(0.999326490452121,0.99964606396814,1.,0.999104400890346,
0.998428822056299),(0.999326490452121,0.99964606396814,1.,0.999104400890346,
0.998428822056299)))
REPRESENTATION_ITEM('')
SURFACE()
);
#457=(
BOUNDED_SURFACE()
B_SPLINE_SURFACE(1,2,((#84622,#84623,#84624),(#84625,#84626,#84627),(#84628,
#84629,#84630)),.UNSPECIFIED.,.F.,.F.,.F.)
B_SPLINE_SURFACE_WITH_KNOTS((2,1,2),(3,3),(0.,1.,1.01),(0.02559035961318,
0.0375948596693871),.UNSPECIFIED.)
GEOMETRIC_REPRESENTATION_ITEM()
RATIONAL_B_SPLINE_SURFACE(((0.996753121755999,0.997505687613148,0.999678813023853),
(0.996753121755999,0.997505687613148,0.999678813023853),(0.996753121755999,
0.997505687613148,0.999678813023853)))
REPRESENTATION_ITEM('')
SURFACE()
);
#458=(
BOUNDED_SURFACE()
B_SPLINE_SURFACE(1,2,((#84665,#84666,#84667),(#84668,#84669,#84670),(#84671,
#84672,#84673)),.UNSPECIFIED.,.F.,.F.,.F.)
B_SPLINE_SURFACE_WITH_KNOTS((2,1,2),(3,3),(-0.00286823257315062,0.,0.477902879794566),
(0.0265907346180623,0.0331702037100443),.UNSPECIFIED.)
GEOMETRIC_REPRESENTATION_ITEM()
RATIONAL_B_SPLINE_SURFACE(((0.996888414395785,0.997365765478833,0.998269846380795),
(0.996888414395785,0.997365765478833,0.998269846380795),(0.996888414395785,
0.997365765478833,0.998269846380795)))
REPRESENTATION_ITEM('')
SURFACE()
);
#459=(
BOUNDED_SURFACE()
B_SPLINE_SURFACE(1,2,((#84740,#84741,#84742),(#84743,#84744,#84745),(#84746,
#84747,#84748)),.UNSPECIFIED.,.F.,.F.,.F.)
B_SPLINE_SURFACE_WITH_KNOTS((2,1,2),(3,3),(-0.00286753114032031,0.,0.477902879793208),
(0.0166015299238958,0.0231736788090044),.UNSPECIFIED.)
GEOMETRIC_REPRESENTATION_ITEM()
RATIONAL_B_SPLINE_SURFACE(((0.996422581660833,0.996252244737398,0.996507688616235),
(0.996422581660833,0.996252244737398,0.996507688616235),(0.996422581660833,
0.996252244737399,0.996507688616235)))
REPRESENTATION_ITEM('')
SURFACE()
);
#460=(
BOUNDED_SURFACE()
B_SPLINE_SURFACE(1,2,((#84765,#84766,#84767),(#84768,#84769,#84770),(#84771,
#84772,#84773),(#84774,#84775,#84776)),.UNSPECIFIED.,.F.,.F.,.F.)
B_SPLINE_SURFACE_WITH_KNOTS((2,1,1,2),(3,3),(-0.0101,0.,1.,1.01),(0.00560769168370516,
0.0176009700440511),.UNSPECIFIED.)
GEOMETRIC_REPRESENTATION_ITEM()
RATIONAL_B_SPLINE_SURFACE(((0.998183892113821,0.99657330421516,0.996380621259469),
(0.998183892113821,0.99657330421516,0.996380621259469),(0.998183892113821,
0.99657330421516,0.996380621259469),(0.998183892113821,0.99657330421516,
0.996380621259469)))
REPRESENTATION_ITEM('')
SURFACE()
);
#461=(
BOUNDED_SURFACE()
B_SPLINE_SURFACE(1,2,((#84811,#84812,#84813),(#84814,#84815,#84816),(#84817,
#84818,#84819)),.UNSPECIFIED.,.F.,.F.,.F.)
B_SPLINE_SURFACE_WITH_KNOTS((2,1,2),(3,3),(-0.00206901892615475,0.,0.346769728507453),
(0.00660713154697986,0.0131849431468375),.UNSPECIFIED.)
GEOMETRIC_REPRESENTATION_ITEM()
RATIONAL_B_SPLINE_SURFACE(((0.997925307359503,0.997106772384962,0.996714752253866),
(0.997925307359503,0.997106772384962,0.996714752253866),(0.997925307359503,
0.997106772384962,0.996714752253866)))
REPRESENTATION_ITEM('')
SURFACE()
);
#462=(
BOUNDED_SURFACE()
B_SPLINE_SURFACE(1,2,((#84892,#84893,#84894),(#84895,#84896,#84897)),
 .UNSPECIFIED.,.F.,.F.,.F.)
B_SPLINE_SURFACE_WITH_KNOTS((2,2),(3,3),(0.,1.),(0.0556006976418427,0.0675888856590499),
 .UNSPECIFIED.)
GEOMETRIC_REPRESENTATION_ITEM()
RATIONAL_B_SPLINE_SURFACE(((0.996397562408606,0.996150386832629,0.997319912843745),
(0.996397562408606,0.996150386832629,0.997319912843745)))
REPRESENTATION_ITEM('')
SURFACE()
);
#463=(
BOUNDED_SURFACE()
B_SPLINE_SURFACE(1,2,((#84966,#84967,#84968),(#84969,#84970,#84971),(#84972,
#84973,#84974)),.UNSPECIFIED.,.F.,.F.,.F.)
B_SPLINE_SURFACE_WITH_KNOTS((2,1,2),(3,3),(0.,1.,1.01),(0.0456081671210024,
0.0575989447818799),.UNSPECIFIED.)
GEOMETRIC_REPRESENTATION_ITEM()
RATIONAL_B_SPLINE_SURFACE(((0.997793907739637,0.996365558499689,0.996354522974128),
(0.997793907739637,0.996365558499689,0.996354522974128),(0.997793907739637,
0.996365558499689,0.996354522974128)))
REPRESENTATION_ITEM('')
SURFACE()
);
#464=(
BOUNDED_SURFACE()
B_SPLINE_SURFACE(1,2,((#85009,#85010,#85011),(#85012,#85013,#85014),(#85015,
#85016,#85017)),.UNSPECIFIED.,.F.,.F.,.F.)
B_SPLINE_SURFACE_WITH_KNOTS((2,1,2),(3,3),(-0.00286810173468854,0.,0.47790287979959),
(0.0466073985929113,0.0531834929157972),.UNSPECIFIED.)
GEOMETRIC_REPRESENTATION_ITEM()
RATIONAL_B_SPLINE_SURFACE(((0.997565691989291,0.996847118055593,0.996554836292953),
(0.997565691989291,0.996847118055593,0.996554836292953),(0.997565691989291,
0.996847118055593,0.996554836292953)))
REPRESENTATION_ITEM('')
SURFACE()
);
#465=(
BOUNDED_SURFACE()
B_SPLINE_SURFACE(1,2,((#85034,#85035,#85036,#85037,#85038),(#85039,#85040,
#85041,#85042,#85043),(#85044,#85045,#85046,#85047,#85048)),
 .UNSPECIFIED.,.F.,.F.,.F.)
B_SPLINE_SURFACE_WITH_KNOTS((2,1,2),(3,2,3),(0.,1.,1.01),(0.0355931932713903,
0.0384615384615384,0.0476086899858149),.UNSPECIFIED.)
GEOMETRIC_REPRESENTATION_ITEM()
RATIONAL_B_SPLINE_SURFACE(((0.998993602249807,0.999456249886298,1.,0.9982659811314,
0.997356751596327),(0.998993602249807,0.999456249886298,1.,0.9982659811314,
0.997356751596327),(0.998993602249807,0.999456249886298,1.,0.9982659811314,
0.997356751596327)))
REPRESENTATION_ITEM('')
SURFACE()
);
#466=(
BOUNDED_SURFACE()
B_SPLINE_SURFACE(1,2,((#85096,#85097,#85098,#85099,#85100),(#85101,#85102,
#85103,#85104,#85105),(#85106,#85107,#85108,#85109,#85110)),
 .UNSPECIFIED.,.F.,.F.,.F.)
B_SPLINE_SURFACE_WITH_KNOTS((2,1,2),(3,2,3),(-0.00141401191198397,0.,0.480770297092029),
(0.0365944846645762,0.0384615384615384,0.043185928091518),.UNSPECIFIED.)
GEOMETRIC_REPRESENTATION_ITEM()
RATIONAL_B_SPLINE_SURFACE(((0.999326490452258,0.999646063968217,1.,0.999104400890347,
0.9984288220563),(0.999326490452259,0.999646063968217,1.,0.999104400890347,
0.9984288220563),(0.999326490452259,0.999646063968217,1.,0.999104400890347,
0.9984288220563)))
REPRESENTATION_ITEM('')
SURFACE()
);
#467=(
BOUNDED_SURFACE()
B_SPLINE_SURFACE(1,2,((#85137,#85138,#85139),(#85140,#85141,#85142),(#85143,
#85144,#85145)),.UNSPECIFIED.,.F.,.F.,.F.)
B_SPLINE_SURFACE_WITH_KNOTS((2,1,2),(3,3),(0.,1.,1.01),(0.025590359613181,
0.0375948596693886),.UNSPECIFIED.)
GEOMETRIC_REPRESENTATION_ITEM()
RATIONAL_B_SPLINE_SURFACE(((0.996753121755999,0.997505687613148,0.999678813023854),
(0.996753121755999,0.997505687613148,0.999678813023854),(0.996753121755999,
0.997505687613148,0.999678813023854)))
REPRESENTATION_ITEM('')
SURFACE()
);
#468=(
BOUNDED_SURFACE()
B_SPLINE_SURFACE(1,2,((#85180,#85181,#85182),(#85183,#85184,#85185),(#85186,
#85187,#85188)),.UNSPECIFIED.,.F.,.F.,.F.)
B_SPLINE_SURFACE_WITH_KNOTS((2,1,2),(3,3),(-0.00286823356219242,0.,0.477902879797069),
(0.0265907346180625,0.0331702037252923),.UNSPECIFIED.)
GEOMETRIC_REPRESENTATION_ITEM()
RATIONAL_B_SPLINE_SURFACE(((0.996888414395785,0.997365765479939,0.998269846384986),
(0.996888414395785,0.997365765479939,0.998269846384985),(0.996888414395786,
0.997365765479939,0.998269846384985)))
REPRESENTATION_ITEM('')
SURFACE()
);
#469=(
BOUNDED_SURFACE()
B_SPLINE_SURFACE(1,2,((#85255,#85256,#85257),(#85258,#85259,#85260),(#85261,
#85262,#85263)),.UNSPECIFIED.,.F.,.F.,.F.)
B_SPLINE_SURFACE_WITH_KNOTS((2,1,2),(3,3),(-0.00286753128209527,0.,0.477902879795792),
(0.016601529923896,0.0231736788111884),.UNSPECIFIED.)
GEOMETRIC_REPRESENTATION_ITEM()
RATIONAL_B_SPLINE_SURFACE(((0.996422581660833,0.996252244737341,0.996507688616404),
(0.996422581660833,0.996252244737341,0.996507688616404),(0.996422581660833,
0.996252244737341,0.996507688616404)))
REPRESENTATION_ITEM('')
SURFACE()
);
#470=(
BOUNDED_SURFACE()
B_SPLINE_SURFACE(1,2,((#85280,#85281,#85282),(#85283,#85284,#85285),(#85286,
#85287,#85288),(#85289,#85290,#85291)),.UNSPECIFIED.,.F.,.F.,.F.)
B_SPLINE_SURFACE_WITH_KNOTS((2,1,1,2),(3,3),(-0.0101,0.,1.,1.01),(0.00560769168370618,
0.0176009700440511),.UNSPECIFIED.)
GEOMETRIC_REPRESENTATION_ITEM()
RATIONAL_B_SPLINE_SURFACE(((0.99818389211382,0.99657330421516,0.996380621259469),
(0.99818389211382,0.99657330421516,0.996380621259469),(0.99818389211382,
0.99657330421516,0.996380621259469),(0.99818389211382,0.99657330421516,
0.996380621259469)))
REPRESENTATION_ITEM('')
SURFACE()
);
#471=(
BOUNDED_SURFACE()
B_SPLINE_SURFACE(1,2,((#85326,#85327,#85328),(#85329,#85330,#85331),(#85332,
#85333,#85334)),.UNSPECIFIED.,.F.,.F.,.F.)
B_SPLINE_SURFACE_WITH_KNOTS((2,1,2),(3,3),(-0.00206901892616219,0.,0.346769728508837),
(0.0066071315469777,0.0131849431468903),.UNSPECIFIED.)
GEOMETRIC_REPRESENTATION_ITEM()
RATIONAL_B_SPLINE_SURFACE(((0.997925307359503,0.997106772384955,0.996714752253861),
(0.997925307359503,0.997106772384955,0.99671475225386),(0.997925307359504,
0.997106772384955,0.99671475225386)))
REPRESENTATION_ITEM('')
SURFACE()
);
#472=(
BOUNDED_SURFACE()
B_SPLINE_SURFACE(1,2,((#85407,#85408,#85409),(#85410,#85411,#85412)),
 .UNSPECIFIED.,.F.,.F.,.F.)
B_SPLINE_SURFACE_WITH_KNOTS((2,2),(3,3),(0.,1.),(0.0556006976418383,0.0675888856590508),
 .UNSPECIFIED.)
GEOMETRIC_REPRESENTATION_ITEM()
RATIONAL_B_SPLINE_SURFACE(((0.996397562408606,0.996150386832629,0.997319912843745),
(0.996397562408606,0.996150386832629,0.997319912843745)))
REPRESENTATION_ITEM('')
SURFACE()
);
#473=(
BOUNDED_SURFACE()
B_SPLINE_SURFACE(1,2,((#85481,#85482,#85483),(#85484,#85485,#85486),(#85487,
#85488,#85489)),.UNSPECIFIED.,.F.,.F.,.F.)
B_SPLINE_SURFACE_WITH_KNOTS((2,1,2),(3,3),(0.,1.,1.01),(0.0456081671210034,
0.057598944781882),.UNSPECIFIED.)
GEOMETRIC_REPRESENTATION_ITEM()
RATIONAL_B_SPLINE_SURFACE(((0.997793907739636,0.996365558499688,0.996354522974128),
(0.997793907739636,0.996365558499688,0.996354522974128),(0.997793907739636,
0.996365558499688,0.996354522974128)))
REPRESENTATION_ITEM('')
SURFACE()
);
#474=(
BOUNDED_SURFACE()
B_SPLINE_SURFACE(1,2,((#85524,#85525,#85526),(#85527,#85528,#85529),(#85530,
#85531,#85532)),.UNSPECIFIED.,.F.,.F.,.F.)
B_SPLINE_SURFACE_WITH_KNOTS((2,1,2),(3,3),(-0.00286810173476254,0.,0.477902879801921),
(0.0466073985929117,0.0531834929157977),.UNSPECIFIED.)
GEOMETRIC_REPRESENTATION_ITEM()
RATIONAL_B_SPLINE_SURFACE(((0.997565691989291,0.996847118055594,0.996554836292953),
(0.997565691989291,0.996847118055594,0.996554836292953),(0.997565691989291,
0.996847118055594,0.996554836292953)))
REPRESENTATION_ITEM('')
SURFACE()
);
#475=(
BOUNDED_SURFACE()
B_SPLINE_SURFACE(1,2,((#85549,#85550,#85551,#85552,#85553),(#85554,#85555,
#85556,#85557,#85558),(#85559,#85560,#85561,#85562,#85563)),
 .UNSPECIFIED.,.F.,.F.,.F.)
B_SPLINE_SURFACE_WITH_KNOTS((2,1,2),(3,2,3),(0.,1.,1.01),(0.0355931932713904,
0.0384615384615384,0.0476086899858116),.UNSPECIFIED.)
GEOMETRIC_REPRESENTATION_ITEM()
RATIONAL_B_SPLINE_SURFACE(((0.998993602249807,0.999456249886298,1.,0.998265981131401,
0.997356751596327),(0.998993602249807,0.999456249886298,1.,0.998265981131401,
0.997356751596327),(0.998993602249807,0.999456249886298,1.,0.998265981131401,
0.997356751596327)))
REPRESENTATION_ITEM('')
SURFACE()
);
#476=(
BOUNDED_SURFACE()
B_SPLINE_SURFACE(1,2,((#85611,#85612,#85613,#85614,#85615),(#85616,#85617,
#85618,#85619,#85620),(#85621,#85622,#85623,#85624,#85625)),
 .UNSPECIFIED.,.F.,.F.,.F.)
B_SPLINE_SURFACE_WITH_KNOTS((2,1,2),(3,2,3),(-0.00141401191198296,0.,0.480770297094429),
(0.0365944846645748,0.0384615384615384,0.0431859280915183),
 .UNSPECIFIED.)
GEOMETRIC_REPRESENTATION_ITEM()
RATIONAL_B_SPLINE_SURFACE(((0.999326490452258,0.999646063968217,1.,0.999104400890347,
0.9984288220563),(0.999326490452258,0.999646063968217,1.,0.999104400890347,
0.9984288220563),(0.999326490452258,0.999646063968217,1.,0.999104400890347,
0.9984288220563)))
REPRESENTATION_ITEM('')
SURFACE()
);
#477=(
BOUNDED_SURFACE()
B_SPLINE_SURFACE(1,2,((#85652,#85653,#85654),(#85655,#85656,#85657),(#85658,
#85659,#85660)),.UNSPECIFIED.,.F.,.F.,.F.)
B_SPLINE_SURFACE_WITH_KNOTS((2,1,2),(3,3),(0.,1.,1.01),(0.0255903596131811,
0.0375948596693879),.UNSPECIFIED.)
GEOMETRIC_REPRESENTATION_ITEM()
RATIONAL_B_SPLINE_SURFACE(((0.996753121755999,0.997505687613148,0.999678813023854),
(0.996753121755999,0.997505687613148,0.999678813023854),(0.996753121755999,
0.997505687613148,0.999678813023854)))
REPRESENTATION_ITEM('')
SURFACE()
);
#478=(
BOUNDED_SURFACE()
B_SPLINE_SURFACE(1,2,((#85695,#85696,#85697),(#85698,#85699,#85700),(#85701,
#85702,#85703)),.UNSPECIFIED.,.F.,.F.,.F.)
B_SPLINE_SURFACE_WITH_KNOTS((2,1,2),(3,3),(-0.00286823356221668,0.,0.477902879799528),
(0.0265907346180627,0.0331702037252926),.UNSPECIFIED.)
GEOMETRIC_REPRESENTATION_ITEM()
RATIONAL_B_SPLINE_SURFACE(((0.996888414395785,0.997365765479939,0.998269846384985),
(0.996888414395785,0.997365765479939,0.998269846384985),(0.996888414395785,
0.997365765479939,0.998269846384985)))
REPRESENTATION_ITEM('')
SURFACE()
);
#479=(
BOUNDED_SURFACE()
B_SPLINE_SURFACE(1,2,((#85770,#85771,#85772),(#85773,#85774,#85775),(#85776,
#85777,#85778)),.UNSPECIFIED.,.F.,.F.,.F.)
B_SPLINE_SURFACE_WITH_KNOTS((2,1,2),(3,3),(-0.00286753128205672,0.,0.477902879798263),
(0.0166015299238967,0.0231736788111887),.UNSPECIFIED.)
GEOMETRIC_REPRESENTATION_ITEM()
RATIONAL_B_SPLINE_SURFACE(((0.996422581660833,0.996252244737342,0.996507688616404),
(0.996422581660833,0.996252244737342,0.996507688616404),(0.996422581660833,
0.996252244737342,0.996507688616404)))
REPRESENTATION_ITEM('')
SURFACE()
);
#480=(
BOUNDED_SURFACE()
B_SPLINE_SURFACE(1,2,((#85795,#85796,#85797),(#85798,#85799,#85800),(#85801,
#85802,#85803),(#85804,#85805,#85806)),.UNSPECIFIED.,.F.,.F.,.F.)
B_SPLINE_SURFACE_WITH_KNOTS((2,1,1,2),(3,3),(-0.0101,0.,1.,1.01),(0.00560769168370501,
0.0176009700440522),.UNSPECIFIED.)
GEOMETRIC_REPRESENTATION_ITEM()
RATIONAL_B_SPLINE_SURFACE(((0.998183892113821,0.99657330421516,0.996380621259469),
(0.998183892113821,0.99657330421516,0.996380621259469),(0.998183892113821,
0.99657330421516,0.996380621259469),(0.998183892113821,0.99657330421516,
0.996380621259469)))
REPRESENTATION_ITEM('')
SURFACE()
);
#481=(
BOUNDED_SURFACE()
B_SPLINE_SURFACE(1,2,((#85841,#85842,#85843),(#85844,#85845,#85846),(#85847,
#85848,#85849)),.UNSPECIFIED.,.F.,.F.,.F.)
B_SPLINE_SURFACE_WITH_KNOTS((2,1,2),(3,3),(-0.00206901892463095,0.,0.346769728509987),
(0.00660713154697685,0.0131849431292506),.UNSPECIFIED.)
GEOMETRIC_REPRESENTATION_ITEM()
RATIONAL_B_SPLINE_SURFACE(((0.997925307359503,0.99710677238715,0.996714752255963),
(0.997925307359503,0.99710677238715,0.996714752255963),(0.997925307359503,
0.99710677238715,0.996714752255963)))
REPRESENTATION_ITEM('')
SURFACE()
);
#482=(
BOUNDED_SURFACE()
B_SPLINE_SURFACE(1,2,((#85922,#85923,#85924),(#85925,#85926,#85927)),
 .UNSPECIFIED.,.F.,.F.,.F.)
B_SPLINE_SURFACE_WITH_KNOTS((2,2),(3,3),(0.,1.),(0.0556006976418437,0.0675888856590492),
 .UNSPECIFIED.)
GEOMETRIC_REPRESENTATION_ITEM()
RATIONAL_B_SPLINE_SURFACE(((0.996397562408606,0.996150386832629,0.997319912843745),
(0.996397562408606,0.996150386832629,0.997319912843745)))
REPRESENTATION_ITEM('')
SURFACE()
);
#483=(
BOUNDED_SURFACE()
B_SPLINE_SURFACE(1,2,((#85996,#85997,#85998),(#85999,#86000,#86001),(#86002,
#86003,#86004)),.UNSPECIFIED.,.F.,.F.,.F.)
B_SPLINE_SURFACE_WITH_KNOTS((2,1,2),(3,3),(0.,1.,1.01),(0.0456081671210057,
0.0575989447818802),.UNSPECIFIED.)
GEOMETRIC_REPRESENTATION_ITEM()
RATIONAL_B_SPLINE_SURFACE(((0.997793907739636,0.996365558499688,0.996354522974128),
(0.997793907739636,0.996365558499688,0.996354522974128),(0.997793907739636,
0.996365558499688,0.996354522974128)))
REPRESENTATION_ITEM('')
SURFACE()
);
#484=(
BOUNDED_SURFACE()
B_SPLINE_SURFACE(1,2,((#86039,#86040,#86041),(#86042,#86043,#86044),(#86045,
#86046,#86047)),.UNSPECIFIED.,.F.,.F.,.F.)
B_SPLINE_SURFACE_WITH_KNOTS((2,1,2),(3,3),(-0.00286810173481973,0.,0.477902879804097),
(0.0466073985929127,0.053183492915797),.UNSPECIFIED.)
GEOMETRIC_REPRESENTATION_ITEM()
RATIONAL_B_SPLINE_SURFACE(((0.997565691989291,0.996847118055594,0.996554836292953),
(0.997565691989291,0.996847118055594,0.996554836292953),(0.997565691989291,
0.996847118055594,0.996554836292953)))
REPRESENTATION_ITEM('')
SURFACE()
);
#485=(
BOUNDED_SURFACE()
B_SPLINE_SURFACE(1,2,((#86064,#86065,#86066,#86067,#86068),(#86069,#86070,
#86071,#86072,#86073),(#86074,#86075,#86076,#86077,#86078)),
 .UNSPECIFIED.,.F.,.F.,.F.)
B_SPLINE_SURFACE_WITH_KNOTS((2,1,2),(3,2,3),(0.,1.,1.01),(0.0355931932713904,
0.0384615384615384,0.0476086899858128),.UNSPECIFIED.)
GEOMETRIC_REPRESENTATION_ITEM()
RATIONAL_B_SPLINE_SURFACE(((0.998993602249807,0.999456249886298,1.,0.998265981131401,
0.997356751596327),(0.998993602249807,0.999456249886298,1.,0.998265981131401,
0.997356751596327),(0.998993602249807,0.999456249886298,1.,0.998265981131401,
0.997356751596327)))
REPRESENTATION_ITEM('')
SURFACE()
);
#486=(
BOUNDED_SURFACE()
B_SPLINE_SURFACE(1,2,((#86126,#86127,#86128,#86129,#86130),(#86131,#86132,
#86133,#86134,#86135),(#86136,#86137,#86138,#86139,#86140)),
 .UNSPECIFIED.,.F.,.F.,.F.)
B_SPLINE_SURFACE_WITH_KNOTS((2,1,2),(3,2,3),(-0.00141401191198409,0.,0.4807702970967),
(0.0365944846645792,0.0384615384615384,0.043185928091518),.UNSPECIFIED.)
GEOMETRIC_REPRESENTATION_ITEM()
RATIONAL_B_SPLINE_SURFACE(((0.999326490452259,0.999646063968217,1.,0.999104400890347,
0.9984288220563),(0.999326490452259,0.999646063968217,1.,0.999104400890347,
0.9984288220563),(0.999326490452259,0.999646063968217,1.,0.999104400890347,
0.9984288220563)))
REPRESENTATION_ITEM('')
SURFACE()
);
#487=(
BOUNDED_SURFACE()
B_SPLINE_SURFACE(1,2,((#86167,#86168,#86169),(#86170,#86171,#86172),(#86173,
#86174,#86175)),.UNSPECIFIED.,.F.,.F.,.F.)
B_SPLINE_SURFACE_WITH_KNOTS((2,1,2),(3,3),(0.,1.,1.01),(0.0255903596131777,
0.0375948596693867),.UNSPECIFIED.)
GEOMETRIC_REPRESENTATION_ITEM()
RATIONAL_B_SPLINE_SURFACE(((0.996753121755999,0.997505687613147,0.999678813023853),
(0.996753121755999,0.997505687613147,0.999678813023853),(0.996753121755999,
0.997505687613147,0.999678813023853)))
REPRESENTATION_ITEM('')
SURFACE()
);
#488=(
BOUNDED_SURFACE()
B_SPLINE_SURFACE(1,2,((#86210,#86211,#86212),(#86213,#86214,#86215),(#86216,
#86217,#86218)),.UNSPECIFIED.,.F.,.F.,.F.)
B_SPLINE_SURFACE_WITH_KNOTS((2,1,2),(3,3),(-0.00286823356225374,0.,0.477902879801828),
(0.0265907346180626,0.0331702037252923),.UNSPECIFIED.)
GEOMETRIC_REPRESENTATION_ITEM()
RATIONAL_B_SPLINE_SURFACE(((0.996888414395785,0.997365765479939,0.998269846384985),
(0.996888414395785,0.997365765479939,0.998269846384985),(0.996888414395785,
0.997365765479939,0.998269846384985)))
REPRESENTATION_ITEM('')
SURFACE()
);
#489=(
BOUNDED_SURFACE()
B_SPLINE_SURFACE(1,2,((#86285,#86286,#86287),(#86288,#86289,#86290),(#86291,
#86292,#86293)),.UNSPECIFIED.,.F.,.F.,.F.)
B_SPLINE_SURFACE_WITH_KNOTS((2,1,2),(3,3),(-0.00286753128208184,0.,0.477902879800619),
(0.0166015299238959,0.0231736788111884),.UNSPECIFIED.)
GEOMETRIC_REPRESENTATION_ITEM()
RATIONAL_B_SPLINE_SURFACE(((0.996422581660833,0.996252244737341,0.996507688616404),
(0.996422581660833,0.996252244737341,0.996507688616404),(0.996422581660833,
0.996252244737341,0.996507688616404)))
REPRESENTATION_ITEM('')
SURFACE()
);
#490=(
BOUNDED_SURFACE()
B_SPLINE_SURFACE(1,2,((#86310,#86311,#86312),(#86313,#86314,#86315),(#86316,
#86317,#86318),(#86319,#86320,#86321)),.UNSPECIFIED.,.F.,.F.,.F.)
B_SPLINE_SURFACE_WITH_KNOTS((2,1,1,2),(3,3),(-0.0101,0.,1.,1.01),(0.00560769168370726,
0.0176009700440521),.UNSPECIFIED.)
GEOMETRIC_REPRESENTATION_ITEM()
RATIONAL_B_SPLINE_SURFACE(((0.99818389211382,0.99657330421516,0.996380621259469),
(0.99818389211382,0.99657330421516,0.996380621259469),(0.99818389211382,
0.99657330421516,0.996380621259469),(0.99818389211382,0.99657330421516,
0.996380621259469)))
REPRESENTATION_ITEM('')
SURFACE()
);
#491=(
BOUNDED_SURFACE()
B_SPLINE_SURFACE(1,2,((#86356,#86357,#86358),(#86359,#86360,#86361),(#86362,
#86363,#86364)),.UNSPECIFIED.,.F.,.F.,.F.)
B_SPLINE_SURFACE_WITH_KNOTS((2,1,2),(3,3),(-0.00206901892625295,0.,0.346769728511189),
(0.00660713154697812,0.013184943146838),.UNSPECIFIED.)
GEOMETRIC_REPRESENTATION_ITEM()
RATIONAL_B_SPLINE_SURFACE(((0.997925307359503,0.997106772384961,0.996714752253866),
(0.997925307359503,0.997106772384961,0.996714752253866),(0.997925307359503,
0.997106772384961,0.996714752253866)))
REPRESENTATION_ITEM('')
SURFACE()
);
#492=(
BOUNDED_SURFACE()
B_SPLINE_SURFACE(1,2,((#86437,#86438,#86439),(#86440,#86441,#86442)),
 .UNSPECIFIED.,.F.,.F.,.F.)
B_SPLINE_SURFACE_WITH_KNOTS((2,2),(3,3),(0.,1.),(0.0556006976418426,0.0675888856590519),
 .UNSPECIFIED.)
GEOMETRIC_REPRESENTATION_ITEM()
RATIONAL_B_SPLINE_SURFACE(((0.996397562408606,0.996150386832629,0.997319912843745),
(0.996397562408606,0.996150386832629,0.997319912843745)))
REPRESENTATION_ITEM('')
SURFACE()
);
#493=(
BOUNDED_SURFACE()
B_SPLINE_SURFACE(1,2,((#86511,#86512,#86513),(#86514,#86515,#86516),(#86517,
#86518,#86519)),.UNSPECIFIED.,.F.,.F.,.F.)
B_SPLINE_SURFACE_WITH_KNOTS((2,1,2),(3,3),(0.,1.,1.01),(0.0456081671210031,
0.0575989447818832),.UNSPECIFIED.)
GEOMETRIC_REPRESENTATION_ITEM()
RATIONAL_B_SPLINE_SURFACE(((0.997793907739636,0.996365558499688,0.996354522974128),
(0.997793907739636,0.996365558499688,0.996354522974128),(0.997793907739636,
0.996365558499688,0.996354522974128)))
REPRESENTATION_ITEM('')
SURFACE()
);
#494=(
BOUNDED_SURFACE()
B_SPLINE_SURFACE(1,2,((#86554,#86555,#86556),(#86557,#86558,#86559),(#86560,
#86561,#86562)),.UNSPECIFIED.,.F.,.F.,.F.)
B_SPLINE_SURFACE_WITH_KNOTS((2,1,2),(3,3),(-0.00286810173489927,0.,0.477902879806116),
(0.046607398592912,0.0531834929157973),.UNSPECIFIED.)
GEOMETRIC_REPRESENTATION_ITEM()
RATIONAL_B_SPLINE_SURFACE(((0.997565691989291,0.996847118055593,0.996554836292953),
(0.997565691989291,0.996847118055593,0.996554836292953),(0.997565691989291,
0.996847118055593,0.996554836292953)))
REPRESENTATION_ITEM('')
SURFACE()
);
#495=(
BOUNDED_SURFACE()
B_SPLINE_SURFACE(1,2,((#86579,#86580,#86581,#86582,#86583),(#86584,#86585,
#86586,#86587,#86588),(#86589,#86590,#86591,#86592,#86593)),
 .UNSPECIFIED.,.F.,.F.,.F.)
B_SPLINE_SURFACE_WITH_KNOTS((2,1,2),(3,2,3),(0.,1.,1.01),(0.0355931932713903,
0.0384615384615384,0.0476086899858138),.UNSPECIFIED.)
GEOMETRIC_REPRESENTATION_ITEM()
RATIONAL_B_SPLINE_SURFACE(((0.998993602249807,0.999456249886298,1.,0.998265981131401,
0.997356751596327),(0.998993602249807,0.999456249886298,1.,0.998265981131401,
0.997356751596327),(0.998993602249807,0.999456249886298,1.,0.998265981131401,
0.997356751596327)))
REPRESENTATION_ITEM('')
SURFACE()
);
#496=(
BOUNDED_SURFACE()
B_SPLINE_SURFACE(1,2,((#86641,#86642,#86643,#86644,#86645),(#86646,#86647,
#86648,#86649,#86650),(#86651,#86652,#86653,#86654,#86655)),
 .UNSPECIFIED.,.F.,.F.,.F.)
B_SPLINE_SURFACE_WITH_KNOTS((2,1,2),(3,2,3),(-0.00286743095560886,0.,0.480770297165012),
(0.0365944846641869,0.0384615384615384,0.0431859280915204),
 .UNSPECIFIED.)
GEOMETRIC_REPRESENTATION_ITEM()
RATIONAL_B_SPLINE_SURFACE(((0.999326490452125,0.999646063968143,1.,0.999104400890347,
0.9984288220563),(0.999326490452125,0.999646063968143,1.,0.999104400890347,
0.9984288220563),(0.999326490452125,0.999646063968143,1.,0.999104400890347,
0.9984288220563)))
REPRESENTATION_ITEM('')
SURFACE()
);
#497=(
BOUNDED_SURFACE()
B_SPLINE_SURFACE(1,2,((#86682,#86683,#86684),(#86685,#86686,#86687),(#86688,
#86689,#86690)),.UNSPECIFIED.,.F.,.F.,.F.)
B_SPLINE_SURFACE_WITH_KNOTS((2,1,2),(3,3),(0.,1.,1.01),(0.0255903596131801,
0.0375948596693875),.UNSPECIFIED.)
GEOMETRIC_REPRESENTATION_ITEM()
RATIONAL_B_SPLINE_SURFACE(((0.996753121755999,0.997505687613148,0.999678813023853),
(0.996753121755999,0.997505687613148,0.999678813023853),(0.996753121755999,
0.997505687613148,0.999678813023853)))
REPRESENTATION_ITEM('')
SURFACE()
);
#498=(
BOUNDED_SURFACE()
B_SPLINE_SURFACE(1,2,((#86725,#86726,#86727),(#86728,#86729,#86730),(#86731,
#86732,#86733)),.UNSPECIFIED.,.F.,.F.,.F.)
B_SPLINE_SURFACE_WITH_KNOTS((2,1,2),(3,3),(-0.00286823356225963,0.,0.477902879804001),
(0.0265907346180617,0.0331702037252925),.UNSPECIFIED.)
GEOMETRIC_REPRESENTATION_ITEM()
RATIONAL_B_SPLINE_SURFACE(((0.996888414395785,0.997365765479939,0.998269846384985),
(0.996888414395785,0.997365765479939,0.998269846384985),(0.996888414395785,
0.997365765479939,0.998269846384985)))
REPRESENTATION_ITEM('')
SURFACE()
);
#499=(
BOUNDED_SURFACE()
B_SPLINE_SURFACE(1,2,((#86800,#86801,#86802),(#86803,#86804,#86805),(#86806,
#86807,#86808)),.UNSPECIFIED.,.F.,.F.,.F.)
B_SPLINE_SURFACE_WITH_KNOTS((2,1,2),(3,3),(-0.0028675312820472,0.,0.477902879803021),
(0.0166015299238958,0.023173678811189),.UNSPECIFIED.)
GEOMETRIC_REPRESENTATION_ITEM()
RATIONAL_B_SPLINE_SURFACE(((0.996422581660833,0.996252244737342,0.996507688616404),
(0.996422581660833,0.996252244737342,0.996507688616404),(0.996422581660833,
0.996252244737342,0.996507688616404)))
REPRESENTATION_ITEM('')
SURFACE()
);
#500=(
BOUNDED_SURFACE()
B_SPLINE_SURFACE(1,2,((#86825,#86826,#86827),(#86828,#86829,#86830),(#86831,
#86832,#86833),(#86834,#86835,#86836)),.UNSPECIFIED.,.F.,.F.,.F.)
B_SPLINE_SURFACE_WITH_KNOTS((2,1,1,2),(3,3),(-0.0101,0.,1.,1.01),(0.00560769168370729,
0.0176009700440515),.UNSPECIFIED.)
GEOMETRIC_REPRESENTATION_ITEM()
RATIONAL_B_SPLINE_SURFACE(((0.99818389211382,0.99657330421516,0.996380621259469),
(0.99818389211382,0.99657330421516,0.996380621259469),(0.99818389211382,
0.99657330421516,0.996380621259469),(0.99818389211382,0.99657330421516,
0.996380621259469)))
REPRESENTATION_ITEM('')
SURFACE()
);
#501=(
BOUNDED_SURFACE()
B_SPLINE_SURFACE(1,2,((#86871,#86872,#86873),(#86874,#86875,#86876),(#86877,
#86878,#86879)),.UNSPECIFIED.,.F.,.F.,.F.)
B_SPLINE_SURFACE_WITH_KNOTS((2,1,2),(3,3),(-0.00206901892633123,0.,0.346769728512148),
(0.00660713154698074,0.0131849431468902),.UNSPECIFIED.)
GEOMETRIC_REPRESENTATION_ITEM()
RATIONAL_B_SPLINE_SURFACE(((0.997925307359502,0.997106772384955,0.99671475225386),
(0.997925307359502,0.997106772384955,0.99671475225386),(0.997925307359502,
0.997106772384955,0.99671475225386)))
REPRESENTATION_ITEM('')
SURFACE()
);
#502=(
BOUNDED_SURFACE()
B_SPLINE_SURFACE(1,2,((#86952,#86953,#86954),(#86955,#86956,#86957)),
 .UNSPECIFIED.,.F.,.F.,.F.)
B_SPLINE_SURFACE_WITH_KNOTS((2,2),(3,3),(0.,1.),(0.0556006976418428,0.0675888856590498),
 .UNSPECIFIED.)
GEOMETRIC_REPRESENTATION_ITEM()
RATIONAL_B_SPLINE_SURFACE(((0.996397562408606,0.996150386832629,0.997319912843745),
(0.996397562408606,0.996150386832629,0.997319912843745)))
REPRESENTATION_ITEM('')
SURFACE()
);
#503=(
BOUNDED_SURFACE()
B_SPLINE_SURFACE(1,2,((#87026,#87027,#87028),(#87029,#87030,#87031),(#87032,
#87033,#87034)),.UNSPECIFIED.,.F.,.F.,.F.)
B_SPLINE_SURFACE_WITH_KNOTS((2,1,2),(3,3),(0.,1.,1.01),(0.0456081671210065,
0.0575989447818823),.UNSPECIFIED.)
GEOMETRIC_REPRESENTATION_ITEM()
RATIONAL_B_SPLINE_SURFACE(((0.997793907739636,0.996365558499688,0.996354522974128),
(0.997793907739636,0.996365558499688,0.996354522974128),(0.997793907739636,
0.996365558499688,0.996354522974128)))
REPRESENTATION_ITEM('')
SURFACE()
);
#504=(
BOUNDED_SURFACE()
B_SPLINE_SURFACE(1,2,((#87069,#87070,#87071),(#87072,#87073,#87074),(#87075,
#87076,#87077)),.UNSPECIFIED.,.F.,.F.,.F.)
B_SPLINE_SURFACE_WITH_KNOTS((2,1,2),(3,3),(-0.00286810173493617,0.,0.477902879807942),
(0.046607398592912,0.0531834929157968),.UNSPECIFIED.)
GEOMETRIC_REPRESENTATION_ITEM()
RATIONAL_B_SPLINE_SURFACE(((0.997565691989291,0.996847118055594,0.996554836292953),
(0.997565691989291,0.996847118055594,0.996554836292953),(0.997565691989291,
0.996847118055594,0.996554836292953)))
REPRESENTATION_ITEM('')
SURFACE()
);
#505=(
BOUNDED_SURFACE()
B_SPLINE_SURFACE(1,2,((#87094,#87095,#87096,#87097,#87098),(#87099,#87100,
#87101,#87102,#87103),(#87104,#87105,#87106,#87107,#87108)),
 .UNSPECIFIED.,.F.,.F.,.F.)
B_SPLINE_SURFACE_WITH_KNOTS((2,1,2),(3,2,3),(0.,1.,1.01),(0.0355931932713904,
0.0384615384615384,0.0476086899858133),.UNSPECIFIED.)
GEOMETRIC_REPRESENTATION_ITEM()
RATIONAL_B_SPLINE_SURFACE(((0.998993602249807,0.999456249886298,1.,0.998265981131401,
0.997356751596327),(0.998993602249807,0.999456249886298,1.,0.998265981131401,
0.997356751596327),(0.998993602249807,0.999456249886298,1.,0.998265981131401,
0.997356751596327)))
REPRESENTATION_ITEM('')
SURFACE()
);
#506=(
BOUNDED_SURFACE()
B_SPLINE_SURFACE(1,2,((#87156,#87157,#87158,#87159,#87160),(#87161,#87162,
#87163,#87164,#87165),(#87166,#87167,#87168,#87169,#87170)),
 .UNSPECIFIED.,.F.,.F.,.F.)
B_SPLINE_SURFACE_WITH_KNOTS((2,1,2),(3,2,3),(-0.00141401191198266,0.,0.48077029710071),
(0.0365944846645759,0.0384615384615384,0.0431859280915189),
 .UNSPECIFIED.)
GEOMETRIC_REPRESENTATION_ITEM()
RATIONAL_B_SPLINE_SURFACE(((0.999326490452258,0.999646063968217,1.,0.999104400890347,
0.9984288220563),(0.999326490452258,0.999646063968217,1.,0.999104400890347,
0.9984288220563),(0.999326490452258,0.999646063968217,1.,0.999104400890347,
0.9984288220563)))
REPRESENTATION_ITEM('')
SURFACE()
);
#507=(
BOUNDED_SURFACE()
B_SPLINE_SURFACE(1,2,((#87197,#87198,#87199),(#87200,#87201,#87202),(#87203,
#87204,#87205)),.UNSPECIFIED.,.F.,.F.,.F.)
B_SPLINE_SURFACE_WITH_KNOTS((2,1,2),(3,3),(0.,1.,1.01),(0.0255903596131819,
0.0375948596693869),.UNSPECIFIED.)
GEOMETRIC_REPRESENTATION_ITEM()
RATIONAL_B_SPLINE_SURFACE(((0.996753121755999,0.997505687613148,0.999678813023853),
(0.996753121755999,0.997505687613148,0.999678813023853),(0.996753121755999,
0.997505687613148,0.999678813023853)))
REPRESENTATION_ITEM('')
SURFACE()
);
#508=(
BOUNDED_SURFACE()
B_SPLINE_SURFACE(1,2,((#87240,#87241,#87242),(#87243,#87244,#87245),(#87246,
#87247,#87248)),.UNSPECIFIED.,.F.,.F.,.F.)
B_SPLINE_SURFACE_WITH_KNOTS((2,1,2),(3,3),(-0.00286823356225022,0.,0.477902879806047),
(0.0265907346180628,0.0331702037252935),.UNSPECIFIED.)
GEOMETRIC_REPRESENTATION_ITEM()
RATIONAL_B_SPLINE_SURFACE(((0.996888414395785,0.997365765479939,0.998269846384985),
(0.996888414395785,0.997365765479939,0.998269846384985),(0.996888414395785,
0.997365765479939,0.998269846384985)))
REPRESENTATION_ITEM('')
SURFACE()
);
#509=(
BOUNDED_SURFACE()
B_SPLINE_SURFACE(1,2,((#87315,#87316,#87317),(#87318,#87319,#87320),(#87321,
#87322,#87323)),.UNSPECIFIED.,.F.,.F.,.F.)
B_SPLINE_SURFACE_WITH_KNOTS((2,1,2),(3,3),(-0.00286753074368029,0.,0.47790287980504),
(0.0166015299238948,0.0231736788028833),.UNSPECIFIED.)
GEOMETRIC_REPRESENTATION_ITEM()
RATIONAL_B_SPLINE_SURFACE(((0.996422581660833,0.996252244737556,0.996507688615758),
(0.996422581660833,0.996252244737556,0.996507688615758),(0.996422581660833,
0.996252244737556,0.996507688615758)))
REPRESENTATION_ITEM('')
SURFACE()
);
#510=(
BOUNDED_SURFACE()
B_SPLINE_SURFACE(1,2,((#87340,#87341,#87342),(#87343,#87344,#87345),(#87346,
#87347,#87348),(#87349,#87350,#87351)),.UNSPECIFIED.,.F.,.F.,.F.)
B_SPLINE_SURFACE_WITH_KNOTS((2,1,1,2),(3,3),(-0.0101,0.,1.,1.01),(0.00560769168370531,
0.0176009700440506),.UNSPECIFIED.)
GEOMETRIC_REPRESENTATION_ITEM()
RATIONAL_B_SPLINE_SURFACE(((0.99818389211382,0.99657330421516,0.996380621259469),
(0.99818389211382,0.99657330421516,0.996380621259469),(0.99818389211382,
0.99657330421516,0.996380621259469),(0.99818389211382,0.99657330421516,
0.996380621259469)))
REPRESENTATION_ITEM('')
SURFACE()
);
#511=(
BOUNDED_SURFACE()
B_SPLINE_SURFACE(1,2,((#87386,#87387,#87388),(#87389,#87390,#87391),(#87392,
#87393,#87394)),.UNSPECIFIED.,.F.,.F.,.F.)
B_SPLINE_SURFACE_WITH_KNOTS((2,1,2),(3,3),(-0.00206901892636993,0.,0.346769728513067),
(0.00660713154698595,0.0131849431468901),.UNSPECIFIED.)
GEOMETRIC_REPRESENTATION_ITEM()
RATIONAL_B_SPLINE_SURFACE(((0.997925307359501,0.997106772384955,0.99671475225386),
(0.997925307359501,0.997106772384955,0.99671475225386),(0.997925307359501,
0.997106772384955,0.99671475225386)))
REPRESENTATION_ITEM('')
SURFACE()
);
#512=(
BOUNDED_SURFACE()
B_SPLINE_SURFACE(1,2,((#87467,#87468,#87469),(#87470,#87471,#87472)),
 .UNSPECIFIED.,.F.,.F.,.F.)
B_SPLINE_SURFACE_WITH_KNOTS((2,2),(3,3),(0.,1.),(0.0556006976418437,0.0675888856590502),
 .UNSPECIFIED.)
GEOMETRIC_REPRESENTATION_ITEM()
RATIONAL_B_SPLINE_SURFACE(((0.996397562408606,0.996150386832629,0.997319912843745),
(0.996397562408606,0.996150386832629,0.997319912843745)))
REPRESENTATION_ITEM('')
SURFACE()
);
#513=(
BOUNDED_SURFACE()
B_SPLINE_SURFACE(1,2,((#87541,#87542,#87543),(#87544,#87545,#87546),(#87547,
#87548,#87549)),.UNSPECIFIED.,.F.,.F.,.F.)
B_SPLINE_SURFACE_WITH_KNOTS((2,1,2),(3,3),(0.,1.,1.01),(0.0456081671210055,
0.0575989447818823),.UNSPECIFIED.)
GEOMETRIC_REPRESENTATION_ITEM()
RATIONAL_B_SPLINE_SURFACE(((0.997793907739636,0.996365558499688,0.996354522974128),
(0.997793907739636,0.996365558499688,0.996354522974128),(0.997793907739636,
0.996365558499688,0.996354522974128)))
REPRESENTATION_ITEM('')
SURFACE()
);
#514=(
BOUNDED_SURFACE()
B_SPLINE_SURFACE(1,2,((#87584,#87585,#87586),(#87587,#87588,#87589),(#87590,
#87591,#87592)),.UNSPECIFIED.,.F.,.F.,.F.)
B_SPLINE_SURFACE_WITH_KNOTS((2,1,2),(3,3),(-0.00286810173500546,0.,0.477902879809462),
(0.0466073985929117,0.0531834929157977),.UNSPECIFIED.)
GEOMETRIC_REPRESENTATION_ITEM()
RATIONAL_B_SPLINE_SURFACE(((0.997565691989291,0.996847118055593,0.996554836292953),
(0.997565691989291,0.996847118055593,0.996554836292953),(0.997565691989291,
0.996847118055593,0.996554836292953)))
REPRESENTATION_ITEM('')
SURFACE()
);
#515=(
BOUNDED_SURFACE()
B_SPLINE_SURFACE(1,2,((#87609,#87610,#87611,#87612,#87613),(#87614,#87615,
#87616,#87617,#87618),(#87619,#87620,#87621,#87622,#87623)),
 .UNSPECIFIED.,.F.,.F.,.F.)
B_SPLINE_SURFACE_WITH_KNOTS((2,1,2),(3,2,3),(0.,1.,1.01),(0.0355931932713903,
0.0384615384615384,0.0476086899858143),.UNSPECIFIED.)
GEOMETRIC_REPRESENTATION_ITEM()
RATIONAL_B_SPLINE_SURFACE(((0.998993602249807,0.999456249886298,1.,0.998265981131401,
0.997356751596327),(0.998993602249807,0.999456249886298,1.,0.998265981131401,
0.997356751596327),(0.998993602249807,0.999456249886298,1.,0.998265981131401,
0.997356751596327)))
REPRESENTATION_ITEM('')
SURFACE()
);
#516=(
BOUNDED_SURFACE()
B_SPLINE_SURFACE(1,2,((#87671,#87672,#87673,#87674,#87675),(#87676,#87677,
#87678,#87679,#87680),(#87681,#87682,#87683,#87684,#87685)),
 .UNSPECIFIED.,.F.,.F.,.F.)
B_SPLINE_SURFACE_WITH_KNOTS((2,1,2),(3,2,3),(-0.00286743095205352,0.,0.480770297168586),
(0.0365944846642022,0.0384615384615384,0.04318592809152),.UNSPECIFIED.)
GEOMETRIC_REPRESENTATION_ITEM()
RATIONAL_B_SPLINE_SURFACE(((0.999326490452131,0.999646063968146,1.,0.999104400890347,
0.9984288220563),(0.999326490452131,0.999646063968146,1.,0.999104400890347,
0.998428822056299),(0.999326490452131,0.999646063968146,1.,0.999104400890347,
0.998428822056299)))
REPRESENTATION_ITEM('')
SURFACE()
);
#517=(
BOUNDED_SURFACE()
B_SPLINE_SURFACE(1,2,((#87712,#87713,#87714),(#87715,#87716,#87717),(#87718,
#87719,#87720)),.UNSPECIFIED.,.F.,.F.,.F.)
B_SPLINE_SURFACE_WITH_KNOTS((2,1,2),(3,3),(0.,1.,1.01),(0.025590359613181,
0.0375948596693874),.UNSPECIFIED.)
GEOMETRIC_REPRESENTATION_ITEM()
RATIONAL_B_SPLINE_SURFACE(((0.996753121755999,0.997505687613148,0.999678813023853),
(0.996753121755999,0.997505687613148,0.999678813023853),(0.996753121755999,
0.997505687613148,0.999678813023853)))
REPRESENTATION_ITEM('')
SURFACE()
);
#518=(
BOUNDED_SURFACE()
B_SPLINE_SURFACE(1,2,((#87755,#87756,#87757),(#87758,#87759,#87760),(#87761,
#87762,#87763)),.UNSPECIFIED.,.F.,.F.,.F.)
B_SPLINE_SURFACE_WITH_KNOTS((2,1,2),(3,3),(-0.00286823356227653,0.,0.477902879807841),
(0.0265907346180622,0.0331702037252924),.UNSPECIFIED.)
GEOMETRIC_REPRESENTATION_ITEM()
RATIONAL_B_SPLINE_SURFACE(((0.996888414395785,0.997365765479939,0.998269846384985),
(0.996888414395785,0.997365765479939,0.998269846384985),(0.996888414395785,
0.997365765479939,0.998269846384985)))
REPRESENTATION_ITEM('')
SURFACE()
);
#519=(
BOUNDED_SURFACE()
B_SPLINE_SURFACE(1,2,((#87830,#87831,#87832),(#87833,#87834,#87835),(#87836,
#87837,#87838)),.UNSPECIFIED.,.F.,.F.,.F.)
B_SPLINE_SURFACE_WITH_KNOTS((2,1,2),(3,3),(-0.00286753128216935,0.,0.477902879807046),
(0.0166015299238956,0.0231736788111884),.UNSPECIFIED.)
GEOMETRIC_REPRESENTATION_ITEM()
RATIONAL_B_SPLINE_SURFACE(((0.996422581660833,0.996252244737342,0.996507688616404),
(0.996422581660833,0.996252244737342,0.996507688616404),(0.996422581660833,
0.996252244737342,0.996507688616404)))
REPRESENTATION_ITEM('')
SURFACE()
);
#520=(
BOUNDED_SURFACE()
B_SPLINE_SURFACE(1,2,((#87855,#87856,#87857),(#87858,#87859,#87860),(#87861,
#87862,#87863),(#87864,#87865,#87866)),.UNSPECIFIED.,.F.,.F.,.F.)
B_SPLINE_SURFACE_WITH_KNOTS((2,1,1,2),(3,3),(-0.0101,0.,1.,1.01),(0.00560769168370714,
0.0176009700440521),.UNSPECIFIED.)
GEOMETRIC_REPRESENTATION_ITEM()
RATIONAL_B_SPLINE_SURFACE(((0.99818389211382,0.99657330421516,0.996380621259469),
(0.99818389211382,0.99657330421516,0.996380621259469),(0.99818389211382,
0.99657330421516,0.996380621259469),(0.99818389211382,0.99657330421516,
0.996380621259469)))
REPRESENTATION_ITEM('')
SURFACE()
);
#521=(
BOUNDED_SURFACE()
B_SPLINE_SURFACE(1,2,((#87901,#87902,#87903),(#87904,#87905,#87906),(#87907,
#87908,#87909)),.UNSPECIFIED.,.F.,.F.,.F.)
B_SPLINE_SURFACE_WITH_KNOTS((2,1,2),(3,3),(-0.00206901892643086,0.,0.346769728513646),
(0.00660713154699298,0.0131849431468898),.UNSPECIFIED.)
GEOMETRIC_REPRESENTATION_ITEM()
RATIONAL_B_SPLINE_SURFACE(((0.997925307359499,0.997106772384954,0.99671475225386),
(0.997925307359499,0.997106772384954,0.99671475225386),(0.997925307359499,
0.997106772384954,0.99671475225386)))
REPRESENTATION_ITEM('')
SURFACE()
);
#522=(
BOUNDED_SURFACE()
B_SPLINE_SURFACE(1,2,((#87982,#87983,#87984),(#87985,#87986,#87987)),
 .UNSPECIFIED.,.F.,.F.,.F.)
B_SPLINE_SURFACE_WITH_KNOTS((2,2),(3,3),(0.,1.),(0.0556006976418426,0.0675888856590509),
 .UNSPECIFIED.)
GEOMETRIC_REPRESENTATION_ITEM()
RATIONAL_B_SPLINE_SURFACE(((0.996397562408606,0.996150386832629,0.997319912843745),
(0.996397562408606,0.996150386832629,0.997319912843745)))
REPRESENTATION_ITEM('')
SURFACE()
);
#523=(
BOUNDED_SURFACE()
B_SPLINE_SURFACE(1,2,((#88056,#88057,#88058),(#88059,#88060,#88061),(#88062,
#88063,#88064)),.UNSPECIFIED.,.F.,.F.,.F.)
B_SPLINE_SURFACE_WITH_KNOTS((2,1,2),(3,3),(0.,1.,1.01),(0.0456081671207015,
0.0575989447852278),.UNSPECIFIED.)
GEOMETRIC_REPRESENTATION_ITEM()
RATIONAL_B_SPLINE_SURFACE(((0.997793907739708,0.99636555849929,0.996354522974122),
(0.997793907739708,0.99636555849929,0.996354522974122),(0.997793907739708,
0.99636555849929,0.996354522974122)))
REPRESENTATION_ITEM('')
SURFACE()
);
#524=(
BOUNDED_SURFACE()
B_SPLINE_SURFACE(1,2,((#88099,#88100,#88101),(#88102,#88103,#88104),(#88105,
#88106,#88107)),.UNSPECIFIED.,.F.,.F.,.F.)
B_SPLINE_SURFACE_WITH_KNOTS((2,1,2),(3,3),(-0.00286810173509,0.,0.477902879810816),
(0.0466073985929116,0.053183492915798),.UNSPECIFIED.)
GEOMETRIC_REPRESENTATION_ITEM()
RATIONAL_B_SPLINE_SURFACE(((0.997565691989291,0.996847118055594,0.996554836292953),
(0.997565691989291,0.996847118055594,0.996554836292953),(0.997565691989291,
0.996847118055594,0.996554836292953)))
REPRESENTATION_ITEM('')
SURFACE()
);
#525=(
BOUNDED_SURFACE()
B_SPLINE_SURFACE(1,2,((#88124,#88125,#88126,#88127,#88128),(#88129,#88130,
#88131,#88132,#88133),(#88134,#88135,#88136,#88137,#88138)),
 .UNSPECIFIED.,.F.,.F.,.F.)
B_SPLINE_SURFACE_WITH_KNOTS((2,1,2),(3,2,3),(0.,1.,1.01),(0.0355931932713903,
0.0384615384615384,0.0476086899858139),.UNSPECIFIED.)
GEOMETRIC_REPRESENTATION_ITEM()
RATIONAL_B_SPLINE_SURFACE(((0.998993602249807,0.999456249886298,1.,0.998265981131401,
0.997356751596327),(0.998993602249807,0.999456249886298,1.,0.998265981131401,
0.997356751596327),(0.998993602249807,0.999456249886298,1.,0.998265981131401,
0.997356751596327)))
REPRESENTATION_ITEM('')
SURFACE()
);
#526=(
BOUNDED_SURFACE()
B_SPLINE_SURFACE(1,2,((#88186,#88187,#88188,#88189,#88190),(#88191,#88192,
#88193,#88194,#88195),(#88196,#88197,#88198,#88199,#88200)),
 .UNSPECIFIED.,.F.,.F.,.F.)
B_SPLINE_SURFACE_WITH_KNOTS((2,1,2),(3,2,3),(-0.00141401191198401,0.,0.480770297103859),
(0.0365944846645752,0.0384615384615384,0.0431859280915187),
 .UNSPECIFIED.)
GEOMETRIC_REPRESENTATION_ITEM()
RATIONAL_B_SPLINE_SURFACE(((0.999326490452258,0.999646063968217,1.,0.999104400890347,
0.9984288220563),(0.999326490452258,0.999646063968217,1.,0.999104400890347,
0.9984288220563),(0.999326490452258,0.999646063968217,1.,0.999104400890347,
0.9984288220563)))
REPRESENTATION_ITEM('')
SURFACE()
);
#527=(
BOUNDED_SURFACE()
B_SPLINE_SURFACE(1,2,((#88227,#88228,#88229),(#88230,#88231,#88232),(#88233,
#88234,#88235)),.UNSPECIFIED.,.F.,.F.,.F.)
B_SPLINE_SURFACE_WITH_KNOTS((2,1,2),(3,3),(0.,1.,1.01),(0.0255903596131799,
0.0375948596693882),.UNSPECIFIED.)
GEOMETRIC_REPRESENTATION_ITEM()
RATIONAL_B_SPLINE_SURFACE(((0.996753121755999,0.997505687613148,0.999678813023854),
(0.996753121755999,0.997505687613148,0.999678813023854),(0.996753121755999,
0.997505687613148,0.999678813023854)))
REPRESENTATION_ITEM('')
SURFACE()
);
#528=(
BOUNDED_SURFACE()
B_SPLINE_SURFACE(1,2,((#88270,#88271,#88272),(#88273,#88274,#88275),(#88276,
#88277,#88278)),.UNSPECIFIED.,.F.,.F.,.F.)
B_SPLINE_SURFACE_WITH_KNOTS((2,1,2),(3,3),(-0.00286823356231214,0.,0.477902879809393),
(0.0265907346180619,0.033170203725292),.UNSPECIFIED.)
GEOMETRIC_REPRESENTATION_ITEM()
RATIONAL_B_SPLINE_SURFACE(((0.996888414395785,0.997365765479939,0.998269846384985),
(0.996888414395785,0.997365765479939,0.998269846384985),(0.996888414395785,
0.997365765479939,0.998269846384985)))
REPRESENTATION_ITEM('')
SURFACE()
);
#529=(
BOUNDED_SURFACE()
B_SPLINE_SURFACE(1,2,((#88345,#88346,#88347),(#88348,#88349,#88350),(#88351,
#88352,#88353)),.UNSPECIFIED.,.F.,.F.,.F.)
B_SPLINE_SURFACE_WITH_KNOTS((2,1,2),(3,3),(-0.00286753074372667,0.,0.477902879808682),
(0.0166015299238963,0.023173678802884),.UNSPECIFIED.)
GEOMETRIC_REPRESENTATION_ITEM()
RATIONAL_B_SPLINE_SURFACE(((0.996422581660833,0.996252244737557,0.996507688615759),
(0.996422581660833,0.996252244737557,0.996507688615759),(0.996422581660833,
0.996252244737557,0.996507688615759)))
REPRESENTATION_ITEM('')
SURFACE()
);
#530=(
BOUNDED_SURFACE()
B_SPLINE_SURFACE(1,2,((#88370,#88371,#88372),(#88373,#88374,#88375),(#88376,
#88377,#88378),(#88379,#88380,#88381)),.UNSPECIFIED.,.F.,.F.,.F.)
B_SPLINE_SURFACE_WITH_KNOTS((2,1,1,2),(3,3),(-0.0101,0.,1.,1.01),(0.00560769168370498,
0.0176009700440528),.UNSPECIFIED.)
GEOMETRIC_REPRESENTATION_ITEM()
RATIONAL_B_SPLINE_SURFACE(((0.998183892113821,0.99657330421516,0.996380621259469),
(0.998183892113821,0.99657330421516,0.996380621259469),(0.998183892113821,
0.99657330421516,0.996380621259469),(0.998183892113821,0.99657330421516,
0.996380621259469)))
REPRESENTATION_ITEM('')
SURFACE()
);
#531=(
BOUNDED_SURFACE()
B_SPLINE_SURFACE(1,2,((#88416,#88417,#88418),(#88419,#88420,#88421),(#88422,
#88423,#88424)),.UNSPECIFIED.,.F.,.F.,.F.)
B_SPLINE_SURFACE_WITH_KNOTS((2,1,2),(3,3),(-0.00206901892651131,0.,0.346769728514169),
(0.00660713154700106,0.0131849431468915),.UNSPECIFIED.)
GEOMETRIC_REPRESENTATION_ITEM()
RATIONAL_B_SPLINE_SURFACE(((0.997925307359498,0.997106772384953,0.99671475225386),
(0.997925307359498,0.997106772384953,0.99671475225386),(0.997925307359498,
0.997106772384953,0.99671475225386)))
REPRESENTATION_ITEM('')
SURFACE()
);
#532=(
BOUNDED_SURFACE()
B_SPLINE_SURFACE(1,2,((#88506,#88507,#88508),(#88509,#88510,#88511),(#88512,
#88513,#88514)),.UNSPECIFIED.,.F.,.F.,.F.)
B_SPLINE_SURFACE_WITH_KNOTS((2,1,2),(3,3),(-0.01,0.,1.),(0.0556006976418415,
0.0675888856590499),.UNSPECIFIED.)
GEOMETRIC_REPRESENTATION_ITEM()
RATIONAL_B_SPLINE_SURFACE(((0.996397562408606,0.996150386832629,0.997319912843745),
(0.996397562408606,0.996150386832629,0.997319912843745),(0.996397562408606,
0.996150386832629,0.997319912843745)))
REPRESENTATION_ITEM('')
SURFACE()
);
#533=(
BOUNDED_SURFACE()
B_SPLINE_SURFACE(1,2,((#88574,#88575,#88576),(#88577,#88578,#88579)),
 .UNSPECIFIED.,.F.,.F.,.F.)
B_SPLINE_SURFACE_WITH_KNOTS((2,2),(3,3),(0.,1.),(0.0456081671210044,0.0575989447818823),
 .UNSPECIFIED.)
GEOMETRIC_REPRESENTATION_ITEM()
RATIONAL_B_SPLINE_SURFACE(((0.997793907739636,0.996365558499688,0.996354522974128),
(0.997793907739636,0.996365558499688,0.996354522974128)))
REPRESENTATION_ITEM('')
SURFACE()
);
#534=(
BOUNDED_SURFACE()
B_SPLINE_SURFACE(1,2,((#88646,#88647,#88648,#88649,#88650),(#88651,#88652,
#88653,#88654,#88655),(#88656,#88657,#88658,#88659,#88660)),
 .UNSPECIFIED.,.F.,.F.,.F.)
B_SPLINE_SURFACE_WITH_KNOTS((2,1,2),(3,2,3),(0.,1.,1.01),(0.0355931932713903,
0.0384615384615384,0.0476086899858139),.UNSPECIFIED.)
GEOMETRIC_REPRESENTATION_ITEM()
RATIONAL_B_SPLINE_SURFACE(((0.998993602249807,0.999456249886298,1.,0.998265981131401,
0.997356751596327),(0.998993602249807,0.999456249886298,1.,0.998265981131401,
0.997356751596327),(0.998993602249807,0.999456249886298,1.,0.998265981131401,
0.997356751596327)))
REPRESENTATION_ITEM('')
SURFACE()
);
#535=(
BOUNDED_SURFACE()
B_SPLINE_SURFACE(1,2,((#88708,#88709,#88710,#88711,#88712),(#88713,#88714,
#88715,#88716,#88717),(#88718,#88719,#88720,#88721,#88722)),
 .UNSPECIFIED.,.F.,.F.,.F.)
B_SPLINE_SURFACE_WITH_KNOTS((2,1,2),(3,2,3),(-0.0014140119119827,0.,0.480770297104947),
(0.0365944846645793,0.0384615384615384,0.0431859280915189),
 .UNSPECIFIED.)
GEOMETRIC_REPRESENTATION_ITEM()
RATIONAL_B_SPLINE_SURFACE(((0.99932649045226,0.999646063968218,1.,0.999104400890347,
0.9984288220563),(0.99932649045226,0.999646063968218,1.,0.999104400890347,
0.9984288220563),(0.99932649045226,0.999646063968218,1.,0.999104400890347,
0.9984288220563)))
REPRESENTATION_ITEM('')
SURFACE()
);
#536=(
BOUNDED_SURFACE()
B_SPLINE_SURFACE(1,2,((#88749,#88750,#88751),(#88752,#88753,#88754),(#88755,
#88756,#88757)),.UNSPECIFIED.,.F.,.F.,.F.)
B_SPLINE_SURFACE_WITH_KNOTS((2,1,2),(3,3),(0.,1.,1.01),(0.0255903596131785,
0.0375948596693877),.UNSPECIFIED.)
GEOMETRIC_REPRESENTATION_ITEM()
RATIONAL_B_SPLINE_SURFACE(((0.996753121755999,0.997505687613148,0.999678813023853),
(0.996753121755999,0.997505687613148,0.999678813023853),(0.996753121755999,
0.997505687613148,0.999678813023853)))
REPRESENTATION_ITEM('')
SURFACE()
);
#537=(
BOUNDED_SURFACE()
B_SPLINE_SURFACE(1,2,((#88792,#88793,#88794),(#88795,#88796,#88797),(#88798,
#88799,#88800)),.UNSPECIFIED.,.F.,.F.,.F.)
B_SPLINE_SURFACE_WITH_KNOTS((2,1,2),(3,3),(-0.00286823356223954,0.,0.477902879810711),
(0.0265907346180618,0.0331702037252911),.UNSPECIFIED.)
GEOMETRIC_REPRESENTATION_ITEM()
RATIONAL_B_SPLINE_SURFACE(((0.996888414395785,0.997365765479939,0.998269846384985),
(0.996888414395785,0.997365765479939,0.998269846384985),(0.996888414395785,
0.997365765479939,0.998269846384985)))
REPRESENTATION_ITEM('')
SURFACE()
);
#538=(
BOUNDED_SURFACE()
B_SPLINE_SURFACE(1,2,((#88867,#88868,#88869),(#88870,#88871,#88872),(#88873,
#88874,#88875)),.UNSPECIFIED.,.F.,.F.,.F.)
B_SPLINE_SURFACE_WITH_KNOTS((2,1,2),(3,3),(-0.00286753128216343,0.,0.477902879810108),
(0.0166015299238955,0.0231736788111875),.UNSPECIFIED.)
GEOMETRIC_REPRESENTATION_ITEM()
RATIONAL_B_SPLINE_SURFACE(((0.996422581660833,0.996252244737342,0.996507688616404),
(0.996422581660833,0.996252244737342,0.996507688616404),(0.996422581660833,
0.996252244737342,0.996507688616404)))
REPRESENTATION_ITEM('')
SURFACE()
);
#539=(
BOUNDED_SURFACE()
B_SPLINE_SURFACE(1,2,((#88892,#88893,#88894),(#88895,#88896,#88897),(#88898,
#88899,#88900),(#88901,#88902,#88903)),.UNSPECIFIED.,.F.,.F.,.F.)
B_SPLINE_SURFACE_WITH_KNOTS((2,1,1,2),(3,3),(-0.0101,0.,1.,1.01),(0.00560769168370538,
0.0176009700440511),.UNSPECIFIED.)
GEOMETRIC_REPRESENTATION_ITEM()
RATIONAL_B_SPLINE_SURFACE(((0.99818389211382,0.99657330421516,0.996380621259469),
(0.99818389211382,0.99657330421516,0.996380621259469),(0.99818389211382,
0.99657330421516,0.996380621259469),(0.99818389211382,0.99657330421516,
0.996380621259469)))
REPRESENTATION_ITEM('')
SURFACE()
);
#540=(
BOUNDED_SURFACE()
B_SPLINE_SURFACE(1,2,((#88938,#88939,#88940),(#88941,#88942,#88943),(#88944,
#88945,#88946)),.UNSPECIFIED.,.F.,.F.,.F.)
B_SPLINE_SURFACE_WITH_KNOTS((2,1,2),(3,3),(-0.00206901892655097,0.,0.346769728514504),
(0.00660713154700985,0.0131849431468903),.UNSPECIFIED.)
GEOMETRIC_REPRESENTATION_ITEM()
RATIONAL_B_SPLINE_SURFACE(((0.997925307359495,0.997106772384953,0.99671475225386),
(0.997925307359495,0.997106772384953,0.99671475225386),(0.997925307359495,
0.997106772384953,0.99671475225386)))
REPRESENTATION_ITEM('')
SURFACE()
);
#541=(
BOUNDED_SURFACE()
B_SPLINE_SURFACE(1,2,((#88983,#88984,#88985),(#88986,#88987,#88988)),
 .UNSPECIFIED.,.F.,.F.,.F.)
B_SPLINE_SURFACE_WITH_KNOTS((2,2),(3,3),(0.,1.),(0.0556006976418414,0.0675888856590499),
 .UNSPECIFIED.)
GEOMETRIC_REPRESENTATION_ITEM()
RATIONAL_B_SPLINE_SURFACE(((0.996397562408606,0.996150386832629,0.997319912843745),
(0.996397562408606,0.996150386832629,0.997319912843745)))
REPRESENTATION_ITEM('')
SURFACE()
);
#542=(
BOUNDED_SURFACE()
B_SPLINE_SURFACE(1,2,((#89048,#89049,#89050),(#89051,#89052,#89053),(#89054,
#89055,#89056),(#89057,#89058,#89059)),.UNSPECIFIED.,.F.,.F.,.F.)
B_SPLINE_SURFACE_WITH_KNOTS((2,1,1,2),(3,3),(-0.01,0.,1.,1.0101),(0.0456081671210032,
0.0575989447818821),.UNSPECIFIED.)
GEOMETRIC_REPRESENTATION_ITEM()
RATIONAL_B_SPLINE_SURFACE(((0.997793907739636,0.996365558499688,0.996354522974128),
(0.997793907739636,0.996365558499688,0.996354522974128),(0.997793907739636,
0.996365558499688,0.996354522974128),(0.997793907739636,0.996365558499688,
0.996354522974128)))
REPRESENTATION_ITEM('')
SURFACE()
);
#543=(
BOUNDED_SURFACE()
B_SPLINE_SURFACE(1,2,((#89094,#89095,#89096),(#89097,#89098,#89099),(#89100,
#89101,#89102)),.UNSPECIFIED.,.F.,.F.,.F.)
B_SPLINE_SURFACE_WITH_KNOTS((2,1,2),(3,3),(-0.00286810173515549,0.,0.477902879812476),
(0.0466073985929118,0.0531834929157986),.UNSPECIFIED.)
GEOMETRIC_REPRESENTATION_ITEM()
RATIONAL_B_SPLINE_SURFACE(((0.997565691989291,0.996847118055593,0.996554836292953),
(0.997565691989291,0.996847118055593,0.996554836292953),(0.997565691989291,
0.996847118055593,0.996554836292953)))
REPRESENTATION_ITEM('')
SURFACE()
);
#544=(
BOUNDED_SURFACE()
B_SPLINE_SURFACE(1,2,((#89171,#89172,#89173,#89174,#89175),(#89176,#89177,
#89178,#89179,#89180)),.UNSPECIFIED.,.F.,.F.,.F.)
B_SPLINE_SURFACE_WITH_KNOTS((2,2),(3,2,3),(0.,0.480770297105795),(0.0365944846645799,
0.0384615384615384,0.0431859280915184),.UNSPECIFIED.)
GEOMETRIC_REPRESENTATION_ITEM()
RATIONAL_B_SPLINE_SURFACE(((0.99932649045226,0.999646063968218,1.,0.999104400890347,
0.9984288220563),(0.99932649045226,0.999646063968218,1.,0.999104400890347,
0.9984288220563)))
REPRESENTATION_ITEM('')
SURFACE()
);
#545=(
BOUNDED_SURFACE()
B_SPLINE_SURFACE(1,2,((#89196,#89197,#89198),(#89199,#89200,#89201),(#89202,
#89203,#89204)),.UNSPECIFIED.,.F.,.F.,.F.)
B_SPLINE_SURFACE_WITH_KNOTS((2,1,2),(3,3),(-0.000171761234198046,1.,1.00600020634825),
(0.066589869885604,0.0751324139120509),.UNSPECIFIED.)
GEOMETRIC_REPRESENTATION_ITEM()
RATIONAL_B_SPLINE_SURFACE(((0.997134830028879,0.997884084852109,0.999352698773416),
(0.997134830028879,0.997884084852109,0.999352698773416),(0.997134830028878,
0.997884084852109,0.999352698773416)))
REPRESENTATION_ITEM('')
SURFACE()
);
#546=(
BOUNDED_SURFACE()
B_SPLINE_SURFACE(1,2,((#89254,#89255,#89256),(#89257,#89258,#89259),(#89260,
#89261,#89262)),.UNSPECIFIED.,.F.,.F.,.F.)
B_SPLINE_SURFACE_WITH_KNOTS((2,1,2),(3,3),(0.,1.,1.01),(0.0255903596131786,
0.0375948596693877),.UNSPECIFIED.)
GEOMETRIC_REPRESENTATION_ITEM()
RATIONAL_B_SPLINE_SURFACE(((0.996753121755999,0.997505687613148,0.999678813023853),
(0.996753121755999,0.997505687613148,0.999678813023853),(0.996753121755999,
0.997505687613148,0.999678813023853)))
REPRESENTATION_ITEM('')
SURFACE()
);
#547=(
BOUNDED_SURFACE()
B_SPLINE_SURFACE(1,2,((#89297,#89298,#89299),(#89300,#89301,#89302),(#89303,
#89304,#89305)),.UNSPECIFIED.,.F.,.F.,.F.)
B_SPLINE_SURFACE_WITH_KNOTS((2,1,2),(3,3),(-0.00286823356227599,0.,0.477902879811651),
(0.0265907346180628,0.033170203725292),.UNSPECIFIED.)
GEOMETRIC_REPRESENTATION_ITEM()
RATIONAL_B_SPLINE_SURFACE(((0.996888414395785,0.997365765479939,0.998269846384985),
(0.996888414395785,0.997365765479939,0.998269846384985),(0.996888414395785,
0.997365765479939,0.998269846384985)))
REPRESENTATION_ITEM('')
SURFACE()
);
#548=(
BOUNDED_SURFACE()
B_SPLINE_SURFACE(1,2,((#89372,#89373,#89374),(#89375,#89376,#89377),(#89378,
#89379,#89380)),.UNSPECIFIED.,.F.,.F.,.F.)
B_SPLINE_SURFACE_WITH_KNOTS((2,1,2),(3,3),(-0.00286753074369785,0.,0.477902879811209),
(0.0166015299238962,0.0231736788028824),.UNSPECIFIED.)
GEOMETRIC_REPRESENTATION_ITEM()
RATIONAL_B_SPLINE_SURFACE(((0.996422581660833,0.996252244737557,0.996507688615759),
(0.996422581660833,0.996252244737557,0.996507688615759),(0.996422581660833,
0.996252244737558,0.996507688615759)))
REPRESENTATION_ITEM('')
SURFACE()
);
#549=(
BOUNDED_SURFACE()
B_SPLINE_SURFACE(1,2,((#89397,#89398,#89399),(#89400,#89401,#89402),(#89403,
#89404,#89405),(#89406,#89407,#89408)),.UNSPECIFIED.,.F.,.F.,.F.)
B_SPLINE_SURFACE_WITH_KNOTS((2,1,1,2),(3,3),(-0.0101,0.,1.,1.01),(0.00560769168370639,
0.0176009700440511),.UNSPECIFIED.)
GEOMETRIC_REPRESENTATION_ITEM()
RATIONAL_B_SPLINE_SURFACE(((0.99818389211382,0.99657330421516,0.996380621259469),
(0.99818389211382,0.99657330421516,0.996380621259469),(0.99818389211382,
0.99657330421516,0.996380621259469),(0.99818389211382,0.99657330421516,
0.996380621259469)))
REPRESENTATION_ITEM('')
SURFACE()
);
#550=(
BOUNDED_SURFACE()
B_SPLINE_SURFACE(1,2,((#89443,#89444,#89445),(#89446,#89447,#89448),(#89449,
#89450,#89451)),.UNSPECIFIED.,.F.,.F.,.F.)
B_SPLINE_SURFACE_WITH_KNOTS((2,1,2),(3,3),(-0.00206901892662418,0.,0.346769728514616),
(0.00660713154702066,0.0131849431468895),.UNSPECIFIED.)
GEOMETRIC_REPRESENTATION_ITEM()
RATIONAL_B_SPLINE_SURFACE(((0.997925307359492,0.997106772384953,0.99671475225386),
(0.997925307359492,0.997106772384953,0.99671475225386),(0.997925307359492,
0.997106772384953,0.99671475225386)))
REPRESENTATION_ITEM('')
SURFACE()
);
#551=(
BOUNDED_SURFACE()
B_SPLINE_SURFACE(1,2,((#89507,#89508,#89509),(#89510,#89511,#89512)),
 .UNSPECIFIED.,.F.,.F.,.F.)
B_SPLINE_SURFACE_WITH_KNOTS((2,2),(3,3),(0.,1.),(0.0456081671210045,0.0575989447818819),
 .UNSPECIFIED.)
GEOMETRIC_REPRESENTATION_ITEM()
RATIONAL_B_SPLINE_SURFACE(((0.997793907739636,0.996365558499688,0.996354522974128),
(0.997793907739636,0.996365558499688,0.996354522974128)))
REPRESENTATION_ITEM('')
SURFACE()
);
#552=(
BOUNDED_SURFACE()
B_SPLINE_SURFACE(1,2,((#89570,#89571,#89572,#89573,#89574),(#89575,#89576,
#89577,#89578,#89579),(#89580,#89581,#89582,#89583,#89584),(#89585,#89586,
#89587,#89588,#89589)),.UNSPECIFIED.,.F.,.F.,.F.)
B_SPLINE_SURFACE_WITH_KNOTS((2,1,1,2),(3,2,3),(-0.01,0.,1.,1.0101),(0.0355931932713904,
0.0384615384615384,0.0476086899858126),.UNSPECIFIED.)
GEOMETRIC_REPRESENTATION_ITEM()
RATIONAL_B_SPLINE_SURFACE(((0.998993602249807,0.999456249886298,1.,0.998265981131401,
0.997356751596327),(0.998993602249807,0.999456249886298,1.,0.998265981131401,
0.997356751596327),(0.998993602249807,0.999456249886298,1.,0.998265981131401,
0.997356751596327),(0.998993602249807,0.999456249886298,1.,0.998265981131401,
0.997356751596327)))
REPRESENTATION_ITEM('')
SURFACE()
);
#553=(
BOUNDED_SURFACE()
B_SPLINE_SURFACE(1,2,((#89637,#89638,#89639,#89640,#89641),(#89642,#89643,
#89644,#89645,#89646),(#89647,#89648,#89649,#89650,#89651)),
 .UNSPECIFIED.,.F.,.F.,.F.)
B_SPLINE_SURFACE_WITH_KNOTS((2,1,2),(3,2,3),(-0.00141401191197939,0.,0.480770297106305),
(0.0365944846645761,0.0384615384615384,0.0431859280915181),
 .UNSPECIFIED.)
GEOMETRIC_REPRESENTATION_ITEM()
RATIONAL_B_SPLINE_SURFACE(((0.999326490452259,0.999646063968217,1.,0.999104400890347,
0.9984288220563),(0.999326490452259,0.999646063968217,1.,0.999104400890347,
0.9984288220563),(0.999326490452259,0.999646063968217,1.,0.999104400890347,
0.9984288220563)))
REPRESENTATION_ITEM('')
SURFACE()
);
#554=(
BOUNDED_SURFACE()
B_SPLINE_SURFACE(1,2,((#89659,#89660,#89661),(#89662,#89663,#89664)),
 .UNSPECIFIED.,.F.,.F.,.F.)
B_SPLINE_SURFACE_WITH_KNOTS((2,2),(3,3),(0.,1.),(0.02559035961318,0.0375948596693869),
 .UNSPECIFIED.)
GEOMETRIC_REPRESENTATION_ITEM()
RATIONAL_B_SPLINE_SURFACE(((0.996753121755999,0.997505687613148,0.999678813023853),
(0.996753121755999,0.997505687613148,0.999678813023853)))
REPRESENTATION_ITEM('')
SURFACE()
);
#555=(
BOUNDED_SURFACE()
B_SPLINE_SURFACE(1,2,((#89725,#89726,#89727),(#89728,#89729,#89730),(#89731,
#89732,#89733)),.UNSPECIFIED.,.F.,.F.,.F.)
B_SPLINE_SURFACE_WITH_KNOTS((2,1,2),(3,3),(-0.000171761234875073,1.,1.00600020634811),
(0.0665898698856039,0.0751324139127276),.UNSPECIFIED.)
GEOMETRIC_REPRESENTATION_ITEM()
RATIONAL_B_SPLINE_SURFACE(((0.997134830028879,0.997884084852167,0.999352698773649),
(0.997134830028879,0.997884084852167,0.999352698773649),(0.997134830028879,
0.997884084852167,0.999352698773649)))
REPRESENTATION_ITEM('')
SURFACE()
);
#556=(
BOUNDED_SURFACE()
B_SPLINE_SURFACE(1,2,((#89772,#89773,#89774),(#89775,#89776,#89777),(#89778,
#89779,#89780),(#89781,#89782,#89783)),.UNSPECIFIED.,.F.,.F.,.F.)
B_SPLINE_SURFACE_WITH_KNOTS((2,1,1,2),(3,3),(-0.01,0.,1.,1.0101),(0.0556006976418396,
0.0675888856590483),.UNSPECIFIED.)
GEOMETRIC_REPRESENTATION_ITEM()
RATIONAL_B_SPLINE_SURFACE(((0.996397562408606,0.996150386832629,0.997319912843744),
(0.996397562408606,0.996150386832629,0.997319912843744),(0.996397562408606,
0.996150386832629,0.997319912843744),(0.996397562408606,0.996150386832629,
0.997319912843744)))
REPRESENTATION_ITEM('')
SURFACE()
);
#557=(
BOUNDED_SURFACE()
B_SPLINE_SURFACE(1,2,((#89899,#89900,#89901),(#89902,#89903,#89904),(#89905,
#89906,#89907)),.UNSPECIFIED.,.F.,.F.,.F.)
B_SPLINE_SURFACE_WITH_KNOTS((2,1,2),(3,3),(-0.00286753114067742,0.,0.477902879812045),
(0.0166015299238962,0.0231736788090054),.UNSPECIFIED.)
GEOMETRIC_REPRESENTATION_ITEM()
RATIONAL_B_SPLINE_SURFACE(((0.996422581660833,0.996252244737399,0.996507688616235),
(0.996422581660833,0.996252244737399,0.996507688616235),(0.996422581660833,
0.996252244737399,0.996507688616235)))
REPRESENTATION_ITEM('')
SURFACE()
);
#558=(
BOUNDED_SURFACE()
B_SPLINE_SURFACE(1,2,((#89924,#89925,#89926),(#89927,#89928,#89929),(#89930,
#89931,#89932),(#89933,#89934,#89935)),.UNSPECIFIED.,.F.,.F.,.F.)
B_SPLINE_SURFACE_WITH_KNOTS((2,1,1,2),(3,3),(-0.0101,0.,1.,1.01),(0.00560769168370519,
0.0176009700440511),.UNSPECIFIED.)
GEOMETRIC_REPRESENTATION_ITEM()
RATIONAL_B_SPLINE_SURFACE(((0.998183892113821,0.99657330421516,0.996380621259469),
(0.998183892113821,0.99657330421516,0.996380621259469),(0.998183892113821,
0.99657330421516,0.996380621259469),(0.998183892113821,0.99657330421516,
0.996380621259469)))
REPRESENTATION_ITEM('')
SURFACE()
);
#559=(
BOUNDED_SURFACE()
B_SPLINE_SURFACE(1,2,((#89970,#89971,#89972),(#89973,#89974,#89975),(#89976,
#89977,#89978)),.UNSPECIFIED.,.F.,.F.,.F.)
B_SPLINE_SURFACE_WITH_KNOTS((2,1,2),(3,3),(-0.00206901892668318,0.,0.346769728514577),
(0.00660713154703276,0.0131849431468903),.UNSPECIFIED.)
GEOMETRIC_REPRESENTATION_ITEM()
RATIONAL_B_SPLINE_SURFACE(((0.99792530735949,0.997106772384952,0.996714752253861),
(0.99792530735949,0.997106772384952,0.996714752253861),(0.99792530735949,
0.997106772384952,0.996714752253861)))
REPRESENTATION_ITEM('')
SURFACE()
);
#560=(
BOUNDED_SURFACE()
B_SPLINE_SURFACE(1,2,((#90104,#90105,#90106,#90107,#90108),(#90109,#90110,
#90111,#90112,#90113)),.UNSPECIFIED.,.F.,.F.,.F.)
B_SPLINE_SURFACE_WITH_KNOTS((2,2),(3,2,3),(0.,0.480770297106543),(0.0365944846645797,
0.0384615384615384,0.0431859280915183),.UNSPECIFIED.)
GEOMETRIC_REPRESENTATION_ITEM()
RATIONAL_B_SPLINE_SURFACE(((0.999326490452259,0.999646063968217,1.,0.999104400890347,
0.9984288220563),(0.999326490452259,0.999646063968217,1.,0.999104400890347,
0.9984288220563)))
REPRESENTATION_ITEM('')
SURFACE()
);
#561=(
BOUNDED_SURFACE()
B_SPLINE_SURFACE(1,2,((#90121,#90122,#90123),(#90124,#90125,#90126),(#90127,
#90128,#90129),(#90130,#90131,#90132)),.UNSPECIFIED.,.F.,.F.,.F.)
B_SPLINE_SURFACE_WITH_KNOTS((2,1,1,2),(3,3),(-0.01,0.,1.,1.0101),(0.0255903596131811,
0.0375948596693868),.UNSPECIFIED.)
GEOMETRIC_REPRESENTATION_ITEM()
RATIONAL_B_SPLINE_SURFACE(((0.996753121755999,0.997505687613148,0.999678813023853),
(0.996753121755999,0.997505687613148,0.999678813023853),(0.996753121755999,
0.997505687613148,0.999678813023853),(0.996753121755999,0.997505687613148,
0.999678813023853)))
REPRESENTATION_ITEM('')
SURFACE()
);
#562=(
BOUNDED_SURFACE()
B_SPLINE_SURFACE(1,2,((#90167,#90168,#90169),(#90170,#90171,#90172),(#90173,
#90174,#90175)),.UNSPECIFIED.,.F.,.F.,.F.)
B_SPLINE_SURFACE_WITH_KNOTS((2,1,2),(3,3),(-0.00286823356239707,0.,0.47790287981273),
(0.0265907346180625,0.033170203725292),.UNSPECIFIED.)
GEOMETRIC_REPRESENTATION_ITEM()
RATIONAL_B_SPLINE_SURFACE(((0.996888414395785,0.997365765479939,0.998269846384985),
(0.996888414395785,0.997365765479939,0.998269846384985),(0.996888414395785,
0.997365765479939,0.998269846384985)))
REPRESENTATION_ITEM('')
SURFACE()
);
#563=(
BOUNDED_SURFACE()
B_SPLINE_SURFACE(1,2,((#90290,#90291,#90292),(#90293,#90294,#90295),(#90296,
#90297,#90298)),.UNSPECIFIED.,.F.,.F.,.F.)
B_SPLINE_SURFACE_WITH_KNOTS((2,1,2),(3,3),(-0.00286833998609553,0.,0.477902879812572),
(0.0665898698862494,0.073171619874849),.UNSPECIFIED.)
GEOMETRIC_REPRESENTATION_ITEM()
RATIONAL_B_SPLINE_SURFACE(((0.997134830028992,0.997712106295797,0.998716408300625),
(0.997134830028992,0.997712106295797,0.998716408300625),(0.997134830028992,
0.997712106295797,0.998716408300625)))
REPRESENTATION_ITEM('')
SURFACE()
);
#564=(
BOUNDED_SURFACE()
B_SPLINE_SURFACE(1,2,((#90306,#90307,#90308),(#90309,#90310,#90311),(#90312,
#90313,#90314),(#90315,#90316,#90317)),.UNSPECIFIED.,.F.,.F.,.F.)
B_SPLINE_SURFACE_WITH_KNOTS((2,1,1,2),(3,3),(-0.0101,0.,1.,1.01),(0.0556006976418405,
0.0675888856590483),.UNSPECIFIED.)
GEOMETRIC_REPRESENTATION_ITEM()
RATIONAL_B_SPLINE_SURFACE(((0.996397562408606,0.996150386832629,0.997319912843744),
(0.996397562408606,0.996150386832629,0.997319912843744),(0.996397562408606,
0.996150386832629,0.997319912843744),(0.996397562408606,0.996150386832629,
0.997319912843744)))
REPRESENTATION_ITEM('')
SURFACE()
);
#565=(
BOUNDED_SURFACE()
B_SPLINE_SURFACE(1,2,((#90377,#90378,#90379),(#90380,#90381,#90382),(#90383,
#90384,#90385),(#90386,#90387,#90388)),.UNSPECIFIED.,.F.,.F.,.F.)
B_SPLINE_SURFACE_WITH_KNOTS((2,1,1,2),(3,3),(-0.01,0.,1.,1.0101),(0.0456081671210023,
0.0575989447818803),.UNSPECIFIED.)
GEOMETRIC_REPRESENTATION_ITEM()
RATIONAL_B_SPLINE_SURFACE(((0.997793907739637,0.996365558499688,0.996354522974128),
(0.997793907739637,0.996365558499688,0.996354522974128),(0.997793907739637,
0.996365558499688,0.996354522974128),(0.997793907739637,0.996365558499688,
0.996354522974128)))
REPRESENTATION_ITEM('')
SURFACE()
);
#566=(
BOUNDED_SURFACE()
B_SPLINE_SURFACE(1,2,((#90423,#90424,#90425),(#90426,#90427,#90428),(#90429,
#90430,#90431)),.UNSPECIFIED.,.F.,.F.,.F.)
B_SPLINE_SURFACE_WITH_KNOTS((2,1,2),(3,3),(-0.0028681017353273,0.,0.477902879815827),
(0.0466073985929115,0.0531834929157966),.UNSPECIFIED.)
GEOMETRIC_REPRESENTATION_ITEM()
RATIONAL_B_SPLINE_SURFACE(((0.997565691989291,0.996847118055594,0.996554836292953),
(0.997565691989291,0.996847118055594,0.996554836292953),(0.997565691989291,
0.996847118055594,0.996554836292953)))
REPRESENTATION_ITEM('')
SURFACE()
);
#567=(
BOUNDED_SURFACE()
B_SPLINE_SURFACE(1,2,((#90445,#90446,#90447),(#90448,#90449,#90450),(#90451,
#90452,#90453),(#90454,#90455,#90456)),.UNSPECIFIED.,.F.,.F.,.F.)
B_SPLINE_SURFACE_WITH_KNOTS((2,1,1,2),(3,3),(-0.0101,0.,1.,1.01),(0.0056076916837051,
0.0176009700440511),.UNSPECIFIED.)
GEOMETRIC_REPRESENTATION_ITEM()
RATIONAL_B_SPLINE_SURFACE(((0.998183892113821,0.99657330421516,0.996380621259469),
(0.998183892113821,0.99657330421516,0.996380621259469),(0.998183892113821,
0.99657330421516,0.996380621259469),(0.998183892113821,0.99657330421516,
0.996380621259469)))
REPRESENTATION_ITEM('')
SURFACE()
);
#568=(
BOUNDED_SURFACE()
B_SPLINE_SURFACE(1,2,((#90491,#90492,#90493),(#90494,#90495,#90496),(#90497,
#90498,#90499)),.UNSPECIFIED.,.F.,.F.,.F.)
B_SPLINE_SURFACE_WITH_KNOTS((2,1,2),(3,3),(-0.00206901892672331,0.,0.346769728514296),
(0.00660713154704671,0.0131849431468893),.UNSPECIFIED.)
GEOMETRIC_REPRESENTATION_ITEM()
RATIONAL_B_SPLINE_SURFACE(((0.997925307359486,0.997106772384951,0.99671475225386),
(0.997925307359486,0.997106772384951,0.99671475225386),(0.997925307359486,
0.997106772384951,0.99671475225386)))
REPRESENTATION_ITEM('')
SURFACE()
);
#569=(
BOUNDED_SURFACE()
B_SPLINE_SURFACE(1,2,((#90573,#90574,#90575),(#90576,#90577,#90578)),
 .UNSPECIFIED.,.F.,.F.,.F.)
B_SPLINE_SURFACE_WITH_KNOTS((2,2),(3,3),(0.,1.),(0.0255903596131799,0.0375948596693882),
 .UNSPECIFIED.)
GEOMETRIC_REPRESENTATION_ITEM()
RATIONAL_B_SPLINE_SURFACE(((0.996753121755999,0.997505687613148,0.999678813023854),
(0.996753121755999,0.997505687613148,0.999678813023854)))
REPRESENTATION_ITEM('')
SURFACE()
);
#570=(
BOUNDED_SURFACE()
B_SPLINE_SURFACE(1,2,((#90635,#90636,#90637),(#90638,#90639,#90640),(#90641,
#90642,#90643),(#90644,#90645,#90646)),.UNSPECIFIED.,.F.,.F.,.F.)
B_SPLINE_SURFACE_WITH_KNOTS((2,1,1,2),(3,3),(-0.00600004466592092,0.,1.,
1.00399715809618),(0.0166015299238287,0.0265907346180642),.UNSPECIFIED.)
GEOMETRIC_REPRESENTATION_ITEM()
RATIONAL_B_SPLINE_SURFACE(((0.996422581660836,0.996163681501244,0.996888414395786),
(0.996422581660836,0.996163681501244,0.996888414395786),(0.996422581660836,
0.996163681501244,0.996888414395786),(0.996422581660836,0.996163681501244,
0.996888414395786)))
REPRESENTATION_ITEM('')
SURFACE()
);
#571=(
BOUNDED_SURFACE()
B_SPLINE_SURFACE(1,2,((#90680,#90681,#90682),(#90683,#90684,#90685),(#90686,
#90687,#90688)),.UNSPECIFIED.,.F.,.F.,.F.)
B_SPLINE_SURFACE_WITH_KNOTS((2,1,2),(3,3),(-0.00286753114071372,0.,0.477902879812748),
(0.0166015299238963,0.0231736788090055),.UNSPECIFIED.)
GEOMETRIC_REPRESENTATION_ITEM()
RATIONAL_B_SPLINE_SURFACE(((0.996422581660833,0.996252244737399,0.996507688616235),
(0.996422581660833,0.996252244737399,0.996507688616235),(0.996422581660833,
0.996252244737399,0.996507688616235)))
REPRESENTATION_ITEM('')
SURFACE()
);
#572=(
BOUNDED_SURFACE()
B_SPLINE_SURFACE(1,2,((#90696,#90697,#90698),(#90699,#90700,#90701),(#90702,
#90703,#90704)),.UNSPECIFIED.,.F.,.F.,.F.)
B_SPLINE_SURFACE_WITH_KNOTS((2,1,2),(3,3),(-0.01,0.,1.00000001523839),(0.00560769168370637,
0.0176009700440516),.UNSPECIFIED.)
GEOMETRIC_REPRESENTATION_ITEM()
RATIONAL_B_SPLINE_SURFACE(((0.99818389211382,0.99657330421516,0.996380621259469),
(0.99818389211382,0.99657330421516,0.996380621259469),(0.99818389211382,
0.99657330421516,0.996380621259469)))
REPRESENTATION_ITEM('')
SURFACE()
);
#573=(
BOUNDED_SURFACE()
B_SPLINE_SURFACE(1,2,((#90757,#90758,#90759),(#90760,#90761,#90762),(#90763,
#90764,#90765)),.UNSPECIFIED.,.F.,.F.,.F.)
B_SPLINE_SURFACE_WITH_KNOTS((2,1,2),(3,3),(-0.000171761236754886,1.,1.00600020634818),
(0.0665898698856032,0.0751324139146066),.UNSPECIFIED.)
GEOMETRIC_REPRESENTATION_ITEM()
RATIONAL_B_SPLINE_SURFACE(((0.997134830028878,0.997884084852332,0.999352698774295),
(0.997134830028878,0.997884084852332,0.999352698774295),(0.997134830028878,
0.997884084852332,0.999352698774295)))
REPRESENTATION_ITEM('')
SURFACE()
);
#574=(
BOUNDED_SURFACE()
B_SPLINE_SURFACE(1,2,((#90780,#90781,#90782),(#90783,#90784,#90785),(#90786,
#90787,#90788)),.UNSPECIFIED.,.F.,.F.,.F.)
B_SPLINE_SURFACE_WITH_KNOTS((2,1,2),(3,3),(-0.00286833998615812,0.,0.477902879812017),
(0.0665898698862492,0.07317161987485),.UNSPECIFIED.)
GEOMETRIC_REPRESENTATION_ITEM()
RATIONAL_B_SPLINE_SURFACE(((0.997134830028992,0.997712106295797,0.998716408300625),
(0.997134830028992,0.997712106295797,0.998716408300625),(0.997134830028992,
0.997712106295797,0.998716408300625)))
REPRESENTATION_ITEM('')
SURFACE()
);
#575=(
BOUNDED_SURFACE()
B_SPLINE_SURFACE(1,2,((#90796,#90797,#90798),(#90799,#90800,#90801),(#90802,
#90803,#90804)),.UNSPECIFIED.,.F.,.F.,.F.)
B_SPLINE_SURFACE_WITH_KNOTS((2,1,2),(3,3),(-0.01,0.,1.),(0.0556006976418417,
0.0675888856590487),.UNSPECIFIED.)
GEOMETRIC_REPRESENTATION_ITEM()
RATIONAL_B_SPLINE_SURFACE(((0.996397562408606,0.996150386832629,0.997319912843744),
(0.996397562408606,0.996150386832629,0.997319912843744),(0.996397562408606,
0.996150386832629,0.997319912843744)))
REPRESENTATION_ITEM('')
SURFACE()
);
#576=(
BOUNDED_SURFACE()
B_SPLINE_SURFACE(1,2,((#90840,#90841,#90842),(#90843,#90844,#90845),(#90846,
#90847,#90848)),.UNSPECIFIED.,.F.,.F.,.F.)
B_SPLINE_SURFACE_WITH_KNOTS((2,1,2),(3,3),(-0.00286764392049501,0.,0.47790287980793),
(0.0565997133101191,0.0631721430887064),.UNSPECIFIED.)
GEOMETRIC_REPRESENTATION_ITEM()
RATIONAL_B_SPLINE_SURFACE(((0.996366204684739,0.996295417244646,0.996650447003323),
(0.996366204684739,0.996295417244646,0.996650447003323),(0.996366204684738,
0.996295417244646,0.996650447003323)))
REPRESENTATION_ITEM('')
SURFACE()
);
#577=(
BOUNDED_SURFACE()
B_SPLINE_SURFACE(1,2,((#90856,#90857,#90858),(#90859,#90860,#90861),(#90862,
#90863,#90864),(#90865,#90866,#90867)),.UNSPECIFIED.,.F.,.F.,.F.)
B_SPLINE_SURFACE_WITH_KNOTS((2,1,1,2),(3,3),(-0.0101,0.,1.,1.01),(0.0456081671210031,
0.057598944781881),.UNSPECIFIED.)
GEOMETRIC_REPRESENTATION_ITEM()
RATIONAL_B_SPLINE_SURFACE(((0.997793907739636,0.996365558499688,0.996354522974128),
(0.997793907739636,0.996365558499688,0.996354522974128),(0.997793907739636,
0.996365558499688,0.996354522974128),(0.997793907739636,0.996365558499688,
0.996354522974128)))
REPRESENTATION_ITEM('')
SURFACE()
);
#578=(
BOUNDED_SURFACE()
B_SPLINE_SURFACE(1,2,((#90901,#90902,#90903),(#90904,#90905,#90906),(#90907,
#90908,#90909)),.UNSPECIFIED.,.F.,.F.,.F.)
B_SPLINE_SURFACE_WITH_KNOTS((2,1,2),(3,3),(-0.00286810173531933,0.,0.477902879812644),
(0.046607398592911,0.0531834929157964),.UNSPECIFIED.)
GEOMETRIC_REPRESENTATION_ITEM()
RATIONAL_B_SPLINE_SURFACE(((0.997565691989291,0.996847118055594,0.996554836292953),
(0.997565691989291,0.996847118055594,0.996554836292953),(0.997565691989291,
0.996847118055594,0.996554836292953)))
REPRESENTATION_ITEM('')
SURFACE()
);
#579=(
BOUNDED_SURFACE()
B_SPLINE_SURFACE(1,2,((#90917,#90918,#90919,#90920,#90921),(#90922,#90923,
#90924,#90925,#90926),(#90927,#90928,#90929,#90930,#90931),(#90932,#90933,
#90934,#90935,#90936)),.UNSPECIFIED.,.F.,.F.,.F.)
B_SPLINE_SURFACE_WITH_KNOTS((2,1,1,2),(3,2,3),(-0.01,0.,1.,1.0101),(0.0355931932713894,
0.0384615384615384,0.0476086899858116),.UNSPECIFIED.)
GEOMETRIC_REPRESENTATION_ITEM()
RATIONAL_B_SPLINE_SURFACE(((0.998993602249806,0.999456249886298,1.,0.998265981131401,
0.997356751596327),(0.998993602249806,0.999456249886298,1.,0.998265981131401,
0.997356751596327),(0.998993602249806,0.999456249886298,1.,0.998265981131401,
0.997356751596327),(0.998993602249806,0.999456249886298,1.,0.998265981131401,
0.997356751596327)))
REPRESENTATION_ITEM('')
SURFACE()
);
#580=(
BOUNDED_SURFACE()
B_SPLINE_SURFACE(1,2,((#90983,#90984,#90985,#90986,#90987),(#90988,#90989,
#90990,#90991,#90992),(#90993,#90994,#90995,#90996,#90997)),
 .UNSPECIFIED.,.F.,.F.,.F.)
B_SPLINE_SURFACE_WITH_KNOTS((2,1,2),(3,2,3),(-0.00286743094794425,0.,0.48077029717846),
(0.0365944846642787,0.0384615384615384,0.0431859280915192),
 .UNSPECIFIED.)
GEOMETRIC_REPRESENTATION_ITEM()
RATIONAL_B_SPLINE_SURFACE(((0.999326490452157,0.99964606396816,1.,0.999104400890347,
0.998428822056299),(0.999326490452157,0.99964606396816,1.,0.999104400890347,
0.998428822056299),(0.999326490452157,0.99964606396816,1.,0.999104400890347,
0.998428822056299)))
REPRESENTATION_ITEM('')
SURFACE()
);
#581=(
BOUNDED_SURFACE()
B_SPLINE_SURFACE(1,2,((#91058,#91059,#91060),(#91061,#91062,#91063)),
 .UNSPECIFIED.,.F.,.F.,.F.)
B_SPLINE_SURFACE_WITH_KNOTS((2,2),(3,3),(0.,1.),(0.0255903596132002,0.0375948596691635),
 .UNSPECIFIED.)
GEOMETRIC_REPRESENTATION_ITEM()
RATIONAL_B_SPLINE_SURFACE(((0.996753121756002,0.997505687613137,0.999678813023772),
(0.996753121756002,0.997505687613137,0.999678813023772)))
REPRESENTATION_ITEM('')
SURFACE()
);
#582=(
BOUNDED_SURFACE()
B_SPLINE_SURFACE(1,2,((#91081,#91082,#91083,#91084,#91085),(#91086,#91087,
#91088,#91089,#91090)),.UNSPECIFIED.,.F.,.F.,.F.)
B_SPLINE_SURFACE_WITH_KNOTS((2,2),(3,2,3),(0.519229702917177,1.),(0.0365944846644287,
0.0384615384615384,0.0431859278099541),.UNSPECIFIED.)
GEOMETRIC_REPRESENTATION_ITEM()
RATIONAL_B_SPLINE_SURFACE(((0.999326490452208,0.999646063968189,1.,0.999104400943723,
0.998428822136826),(0.999326490452208,0.999646063968189,1.,0.999104400943723,
0.998428822136826)))
REPRESENTATION_ITEM('')
SURFACE()
);
#583=(
BOUNDED_SURFACE()
B_SPLINE_SURFACE(1,2,((#91146,#91147,#91148),(#91149,#91150,#91151)),
 .UNSPECIFIED.,.F.,.F.,.F.)
B_SPLINE_SURFACE_WITH_KNOTS((2,2),(3,3),(0.,1.),(0.0456081671210052,0.0575989447818612),
 .UNSPECIFIED.)
GEOMETRIC_REPRESENTATION_ITEM()
RATIONAL_B_SPLINE_SURFACE(((0.997793907739636,0.996365558499691,0.996354522974128),
(0.997793907739636,0.996365558499691,0.996354522974128)))
REPRESENTATION_ITEM('')
SURFACE()
);
#584=(
BOUNDED_SURFACE()
B_SPLINE_SURFACE(1,2,((#91186,#91187,#91188),(#91189,#91190,#91191)),
 .UNSPECIFIED.,.F.,.F.,.F.)
B_SPLINE_SURFACE_WITH_KNOTS((2,2),(3,3),(0.,1.),(0.0556006976522449,0.067588885544615),
 .UNSPECIFIED.)
GEOMETRIC_REPRESENTATION_ITEM()
RATIONAL_B_SPLINE_SURFACE(((0.996397562408177,0.996150386836003,0.997319912821417),
(0.996397562408177,0.996150386836003,0.997319912821417)))
REPRESENTATION_ITEM('')
SURFACE()
);
#585=(
BOUNDED_SURFACE()
B_SPLINE_SURFACE(1,2,((#91226,#91227,#91228),(#91229,#91230,#91231)),
 .UNSPECIFIED.,.F.,.F.,.F.)
B_SPLINE_SURFACE_WITH_KNOTS((2,2),(3,3),(0.,1.),(0.0657448619281078,0.0758849574338243),
 .UNSPECIFIED.)
GEOMETRIC_REPRESENTATION_ITEM()
RATIONAL_B_SPLINE_SURFACE(((0.996993639757276,0.997798549146192,0.999617032345115),
(0.996993639757276,0.997798549146192,0.999617032345115)))
REPRESENTATION_ITEM('')
SURFACE()
);
#586=(
BOUNDED_SURFACE()
B_SPLINE_SURFACE(1,2,((#91272,#91273,#91274),(#91275,#91276,#91277)),
 .UNSPECIFIED.,.F.,.F.,.F.)
B_SPLINE_SURFACE_WITH_KNOTS((2,2),(3,3),(0.,1.),(0.00560769170938426,0.0176009697615929),
 .UNSPECIFIED.)
GEOMETRIC_REPRESENTATION_ITEM()
RATIONAL_B_SPLINE_SURFACE(((0.998183892106924,0.996573304252679,0.996380621268545),
(0.998183892106924,0.996573304252679,0.996380621268545)))
REPRESENTATION_ITEM('')
SURFACE()
);
#587=(
BOUNDED_SURFACE()
B_SPLINE_SURFACE(1,2,((#91368,#91369,#91370),(#91371,#91372,#91373)),
 .UNSPECIFIED.,.F.,.F.,.F.)
B_SPLINE_SURFACE_WITH_KNOTS((2,2),(3,3),(0.,1.),(0.00560769170938315,0.0176009697615924),
 .UNSPECIFIED.)
GEOMETRIC_REPRESENTATION_ITEM()
RATIONAL_B_SPLINE_SURFACE(((0.998183892106924,0.996573304252679,0.996380621268545),
(0.998183892106924,0.996573304252679,0.996380621268545)))
REPRESENTATION_ITEM('')
SURFACE()
);
#588=(
BOUNDED_SURFACE()
B_SPLINE_SURFACE(1,2,((#91374,#91375,#91376,#91377,#91378),(#91379,#91380,
#91381,#91382,#91383)),.UNSPECIFIED.,.F.,.F.,.F.)
B_SPLINE_SURFACE_WITH_KNOTS((2,2),(3,2,3),(0.519229702914946,1.),(0.0365944846644327,
0.0384615384615384,0.0431859276813001),.UNSPECIFIED.)
GEOMETRIC_REPRESENTATION_ITEM()
RATIONAL_B_SPLINE_SURFACE(((0.999326490452209,0.999646063968189,1.,0.999104400968112,
0.998428822173621),(0.999326490452209,0.999646063968189,1.,0.999104400968112,
0.998428822173621)))
REPRESENTATION_ITEM('')
SURFACE()
);
#589=(
BOUNDED_SURFACE()
B_SPLINE_SURFACE(1,2,((#91456,#91457,#91458),(#91459,#91460,#91461)),
 .UNSPECIFIED.,.F.,.F.,.F.)
B_SPLINE_SURFACE_WITH_KNOTS((2,2),(3,3),(0.,1.),(0.045608167121004,0.0575989447818607),
 .UNSPECIFIED.)
GEOMETRIC_REPRESENTATION_ITEM()
RATIONAL_B_SPLINE_SURFACE(((0.997793907739636,0.996365558499691,0.996354522974128),
(0.997793907739636,0.996365558499691,0.996354522974128)))
REPRESENTATION_ITEM('')
SURFACE()
);
#590=(
BOUNDED_SURFACE()
B_SPLINE_SURFACE(1,2,((#91496,#91497,#91498),(#91499,#91500,#91501)),
 .UNSPECIFIED.,.F.,.F.,.F.)
B_SPLINE_SURFACE_WITH_KNOTS((2,2),(3,3),(0.,1.),(0.0556006976522436,0.0675888855446153),
 .UNSPECIFIED.)
GEOMETRIC_REPRESENTATION_ITEM()
RATIONAL_B_SPLINE_SURFACE(((0.996397562408177,0.996150386836003,0.997319912821417),
(0.996397562408177,0.996150386836003,0.997319912821417)))
REPRESENTATION_ITEM('')
SURFACE()
);
#591=(
BOUNDED_SURFACE()
B_SPLINE_SURFACE(1,2,((#91536,#91537,#91538),(#91539,#91540,#91541)),
 .UNSPECIFIED.,.F.,.F.,.F.)
B_SPLINE_SURFACE_WITH_KNOTS((2,2),(3,3),(0.,1.),(0.0657450014656856,0.0758834225204709),
 .UNSPECIFIED.)
GEOMETRIC_REPRESENTATION_ITEM()
RATIONAL_B_SPLINE_SURFACE(((0.99699366191014,0.997798452328481,0.99961648183819),
(0.99699366191014,0.997798452328481,0.99961648183819)))
REPRESENTATION_ITEM('')
SURFACE()
);
#592=(
BOUNDED_SURFACE()
B_SPLINE_SURFACE(1,2,((#91592,#91593,#91594),(#91595,#91596,#91597)),
 .UNSPECIFIED.,.F.,.F.,.F.)
B_SPLINE_SURFACE_WITH_KNOTS((2,2),(3,3),(0.,1.),(0.0255903596132011,0.037594859669167),
 .UNSPECIFIED.)
GEOMETRIC_REPRESENTATION_ITEM()
RATIONAL_B_SPLINE_SURFACE(((0.996753121756002,0.997505687613138,0.999678813023773),
(0.996753121756002,0.997505687613138,0.999678813023773)))
REPRESENTATION_ITEM('')
SURFACE()
);
#593=(
BOUNDED_SURFACE()
B_SPLINE_SURFACE(1,2,((#91672,#91673,#91674),(#91675,#91676,#91677)),
 .UNSPECIFIED.,.F.,.F.,.F.)
B_SPLINE_SURFACE_WITH_KNOTS((2,2),(3,3),(0.,1.),(0.00560769170938355,0.0176009697615912),
 .UNSPECIFIED.)
GEOMETRIC_REPRESENTATION_ITEM()
RATIONAL_B_SPLINE_SURFACE(((0.998183892106924,0.996573304252679,0.996380621268545),
(0.998183892106924,0.996573304252679,0.996380621268545)))
REPRESENTATION_ITEM('')
SURFACE()
);
#594=(
BOUNDED_SURFACE()
B_SPLINE_SURFACE(1,2,((#91762,#91763,#91764),(#91765,#91766,#91767)),
 .UNSPECIFIED.,.F.,.F.,.F.)
B_SPLINE_SURFACE_WITH_KNOTS((2,2),(3,3),(0.,1.),(0.0456081671210064,0.0575989447818599),
 .UNSPECIFIED.)
GEOMETRIC_REPRESENTATION_ITEM()
RATIONAL_B_SPLINE_SURFACE(((0.997793907739636,0.996365558499691,0.996354522974128),
(0.997793907739636,0.996365558499691,0.996354522974128)))
REPRESENTATION_ITEM('')
SURFACE()
);
#595=(
BOUNDED_SURFACE()
B_SPLINE_SURFACE(1,2,((#91802,#91803,#91804),(#91805,#91806,#91807)),
 .UNSPECIFIED.,.F.,.F.,.F.)
B_SPLINE_SURFACE_WITH_KNOTS((2,2),(3,3),(0.,1.),(0.0556006976522427,0.0675888855446155),
 .UNSPECIFIED.)
GEOMETRIC_REPRESENTATION_ITEM()
RATIONAL_B_SPLINE_SURFACE(((0.996397562408177,0.996150386836003,0.997319912821417),
(0.996397562408177,0.996150386836003,0.997319912821417)))
REPRESENTATION_ITEM('')
SURFACE()
);
#596=(
BOUNDED_SURFACE()
B_SPLINE_SURFACE(1,2,((#91842,#91843,#91844),(#91845,#91846,#91847)),
 .UNSPECIFIED.,.F.,.F.,.F.)
B_SPLINE_SURFACE_WITH_KNOTS((2,2),(3,3),(0.,1.),(0.065744861928108,0.0758849574338245),
 .UNSPECIFIED.)
GEOMETRIC_REPRESENTATION_ITEM()
RATIONAL_B_SPLINE_SURFACE(((0.996993639757276,0.997798549146192,0.999617032345115),
(0.996993639757276,0.997798549146192,0.999617032345115)))
REPRESENTATION_ITEM('')
SURFACE()
);
#597=(
BOUNDED_SURFACE()
B_SPLINE_SURFACE(1,2,((#91882,#91883,#91884),(#91885,#91886,#91887)),
 .UNSPECIFIED.,.F.,.F.,.F.)
B_SPLINE_SURFACE_WITH_KNOTS((2,2),(3,3),(0.,1.),(0.0255903596131999,0.0375948596691669),
 .UNSPECIFIED.)
GEOMETRIC_REPRESENTATION_ITEM()
RATIONAL_B_SPLINE_SURFACE(((0.996753121756002,0.997505687613138,0.999678813023773),
(0.996753121756002,0.997505687613138,0.999678813023773)))
REPRESENTATION_ITEM('')
SURFACE()
);
#598=(
BOUNDED_SURFACE()
B_SPLINE_SURFACE(1,2,((#91910,#91911,#91912,#91913,#91914),(#91915,#91916,
#91917,#91918,#91919)),.UNSPECIFIED.,.F.,.F.,.F.)
B_SPLINE_SURFACE_WITH_KNOTS((2,2),(3,2,3),(0.519229702917952,1.),(0.0365944846644359,
0.0384615384615384,0.0431859278882002),.UNSPECIFIED.)
GEOMETRIC_REPRESENTATION_ITEM()
RATIONAL_B_SPLINE_SURFACE(((0.99932649045221,0.99964606396819,1.,0.99910440092889,
0.998428822114449),(0.99932649045221,0.99964606396819,1.,0.99910440092889,
0.998428822114449)))
REPRESENTATION_ITEM('')
SURFACE()
);
#599=(
BOUNDED_SURFACE()
B_SPLINE_SURFACE(1,2,((#91976,#91977,#91978),(#91979,#91980,#91981)),
 .UNSPECIFIED.,.F.,.F.,.F.)
B_SPLINE_SURFACE_WITH_KNOTS((2,2),(3,3),(0.,1.),(0.00560769170938407,0.0176009697615916),
 .UNSPECIFIED.)
GEOMETRIC_REPRESENTATION_ITEM()
RATIONAL_B_SPLINE_SURFACE(((0.998183892106924,0.996573304252679,0.996380621268545),
(0.998183892106924,0.996573304252679,0.996380621268545)))
REPRESENTATION_ITEM('')
SURFACE()
);
#600=(
BOUNDED_SURFACE()
B_SPLINE_SURFACE(1,2,((#92066,#92067,#92068),(#92069,#92070,#92071)),
 .UNSPECIFIED.,.F.,.F.,.F.)
B_SPLINE_SURFACE_WITH_KNOTS((2,2),(3,3),(0.,1.),(0.0255903596131989,0.0375948596691652),
 .UNSPECIFIED.)
GEOMETRIC_REPRESENTATION_ITEM()
RATIONAL_B_SPLINE_SURFACE(((0.996753121756001,0.997505687613137,0.999678813023773),
(0.996753121756001,0.997505687613137,0.999678813023773)))
REPRESENTATION_ITEM('')
SURFACE()
);
#601=(
BOUNDED_SURFACE()
B_SPLINE_SURFACE(1,2,((#92106,#92107,#92108),(#92109,#92110,#92111)),
 .UNSPECIFIED.,.F.,.F.,.F.)
B_SPLINE_SURFACE_WITH_KNOTS((2,2),(3,3),(0.,1.),(0.0556006976522448,0.0675888855446141),
 .UNSPECIFIED.)
GEOMETRIC_REPRESENTATION_ITEM()
RATIONAL_B_SPLINE_SURFACE(((0.996397562408177,0.996150386836003,0.997319912821417),
(0.996397562408177,0.996150386836003,0.997319912821417)))
REPRESENTATION_ITEM('')
SURFACE()
);
#602=(
BOUNDED_SURFACE()
B_SPLINE_SURFACE(1,2,((#92146,#92147,#92148),(#92149,#92150,#92151)),
 .UNSPECIFIED.,.F.,.F.,.F.)
B_SPLINE_SURFACE_WITH_KNOTS((2,2),(3,3),(0.,1.),(0.0657448619281069,0.0758849574338248),
 .UNSPECIFIED.)
GEOMETRIC_REPRESENTATION_ITEM()
RATIONAL_B_SPLINE_SURFACE(((0.996993639757276,0.997798549146192,0.999617032345115),
(0.996993639757276,0.997798549146192,0.999617032345115)))
REPRESENTATION_ITEM('')
SURFACE()
);
#603=(
BOUNDED_SURFACE()
B_SPLINE_SURFACE(1,2,((#92169,#92170,#92171,#92172,#92173),(#92174,#92175,
#92176,#92177,#92178)),.UNSPECIFIED.,.F.,.F.,.F.)
B_SPLINE_SURFACE_WITH_KNOTS((2,2),(3,2,3),(0.519229702915815,1.),(0.0365944846644425,
0.0384615384615384,0.0431859278882058),.UNSPECIFIED.)
GEOMETRIC_REPRESENTATION_ITEM()
RATIONAL_B_SPLINE_SURFACE(((0.999326490452213,0.999646063968191,1.,0.999104400928889,
0.998428822114447),(0.999326490452213,0.999646063968191,1.,0.999104400928889,
0.998428822114447)))
REPRESENTATION_ITEM('')
SURFACE()
);
#604=(
BOUNDED_SURFACE()
B_SPLINE_SURFACE(1,2,((#92200,#92201,#92202),(#92203,#92204,#92205)),
 .UNSPECIFIED.,.F.,.F.,.F.)
B_SPLINE_SURFACE_WITH_KNOTS((2,2),(3,3),(0.,1.),(0.0456081671210052,0.0575989447818616),
 .UNSPECIFIED.)
GEOMETRIC_REPRESENTATION_ITEM()
RATIONAL_B_SPLINE_SURFACE(((0.997793907739636,0.996365558499691,0.996354522974128),
(0.997793907739636,0.996365558499691,0.996354522974128)))
REPRESENTATION_ITEM('')
SURFACE()
);
#605=(
BOUNDED_SURFACE()
B_SPLINE_SURFACE(1,2,((#92280,#92281,#92282),(#92283,#92284,#92285)),
 .UNSPECIFIED.,.F.,.F.,.F.)
B_SPLINE_SURFACE_WITH_KNOTS((2,2),(3,3),(0.,1.),(0.00560769170938321,0.0176009697615924),
 .UNSPECIFIED.)
GEOMETRIC_REPRESENTATION_ITEM()
RATIONAL_B_SPLINE_SURFACE(((0.998183892106924,0.996573304252679,0.996380621268545),
(0.998183892106924,0.996573304252679,0.996380621268545)))
REPRESENTATION_ITEM('')
SURFACE()
);
#606=(
BOUNDED_SURFACE()
B_SPLINE_SURFACE(1,2,((#92370,#92371,#92372),(#92373,#92374,#92375)),
 .UNSPECIFIED.,.F.,.F.,.F.)
B_SPLINE_SURFACE_WITH_KNOTS((2,2),(3,3),(0.,1.),(0.0255903596131988,0.0375948596691661),
 .UNSPECIFIED.)
GEOMETRIC_REPRESENTATION_ITEM()
RATIONAL_B_SPLINE_SURFACE(((0.996753121756001,0.997505687613137,0.999678813023773),
(0.996753121756001,0.997505687613137,0.999678813023773)))
REPRESENTATION_ITEM('')
SURFACE()
);
#607=(
BOUNDED_SURFACE()
B_SPLINE_SURFACE(1,2,((#92393,#92394,#92395,#92396,#92397),(#92398,#92399,
#92400,#92401,#92402)),.UNSPECIFIED.,.F.,.F.,.F.)
B_SPLINE_SURFACE_WITH_KNOTS((2,2),(3,2,3),(0.519229702913765,1.),(0.0365944846644499,
0.0384615384615384,0.0431859278882126),.UNSPECIFIED.)
GEOMETRIC_REPRESENTATION_ITEM()
RATIONAL_B_SPLINE_SURFACE(((0.999326490452215,0.999646063968193,1.,0.999104400928888,
0.998428822114445),(0.999326490452215,0.999646063968193,1.,0.999104400928888,
0.998428822114445)))
REPRESENTATION_ITEM('')
SURFACE()
);
#608=(
BOUNDED_SURFACE()
B_SPLINE_SURFACE(1,2,((#92441,#92442,#92443),(#92444,#92445,#92446)),
 .UNSPECIFIED.,.F.,.F.,.F.)
B_SPLINE_SURFACE_WITH_KNOTS((2,2),(3,3),(0.,1.),(0.0657448619281088,0.0758849574338248),
 .UNSPECIFIED.)
GEOMETRIC_REPRESENTATION_ITEM()
RATIONAL_B_SPLINE_SURFACE(((0.996993639757276,0.997798549146193,0.999617032345115),
(0.996993639757276,0.997798549146193,0.999617032345115)))
REPRESENTATION_ITEM('')
SURFACE()
);
#609=(
BOUNDED_SURFACE()
B_SPLINE_SURFACE(1,2,((#92498,#92499,#92500),(#92501,#92502,#92503)),
 .UNSPECIFIED.,.F.,.F.,.F.)
B_SPLINE_SURFACE_WITH_KNOTS((2,2),(3,3),(0.,1.),(0.0456081671210064,0.0575989447818615),
 .UNSPECIFIED.)
GEOMETRIC_REPRESENTATION_ITEM()
RATIONAL_B_SPLINE_SURFACE(((0.997793907739636,0.996365558499691,0.996354522974128),
(0.997793907739636,0.996365558499691,0.996354522974128)))
REPRESENTATION_ITEM('')
SURFACE()
);
#610=(
BOUNDED_SURFACE()
B_SPLINE_SURFACE(1,2,((#92504,#92505,#92506),(#92507,#92508,#92509)),
 .UNSPECIFIED.,.F.,.F.,.F.)
B_SPLINE_SURFACE_WITH_KNOTS((2,2),(3,3),(0.,1.),(0.0556006976522447,0.0675888855446161),
 .UNSPECIFIED.)
GEOMETRIC_REPRESENTATION_ITEM()
RATIONAL_B_SPLINE_SURFACE(((0.996397562408177,0.996150386836003,0.997319912821417),
(0.996397562408177,0.996150386836003,0.997319912821417)))
REPRESENTATION_ITEM('')
SURFACE()
);
#611=(
BOUNDED_SURFACE()
B_SPLINE_SURFACE(1,2,((#92584,#92585,#92586),(#92587,#92588,#92589)),
 .UNSPECIFIED.,.F.,.F.,.F.)
B_SPLINE_SURFACE_WITH_KNOTS((2,2),(3,3),(0.,1.),(0.00560769170938333,0.0176009697615919),
 .UNSPECIFIED.)
GEOMETRIC_REPRESENTATION_ITEM()
RATIONAL_B_SPLINE_SURFACE(((0.998183892106924,0.996573304252679,0.996380621268545),
(0.998183892106924,0.996573304252679,0.996380621268545)))
REPRESENTATION_ITEM('')
SURFACE()
);
#612=(
BOUNDED_SURFACE()
B_SPLINE_SURFACE(1,2,((#92674,#92675,#92676),(#92677,#92678,#92679)),
 .UNSPECIFIED.,.F.,.F.,.F.)
B_SPLINE_SURFACE_WITH_KNOTS((2,2),(3,3),(0.,1.),(0.0255903596131999,0.037594859669166),
 .UNSPECIFIED.)
GEOMETRIC_REPRESENTATION_ITEM()
RATIONAL_B_SPLINE_SURFACE(((0.996753121756002,0.997505687613138,0.999678813023773),
(0.996753121756002,0.997505687613138,0.999678813023773)))
REPRESENTATION_ITEM('')
SURFACE()
);
#613=(
BOUNDED_SURFACE()
B_SPLINE_SURFACE(1,2,((#92697,#92698,#92699,#92700,#92701),(#92702,#92703,
#92704,#92705,#92706)),.UNSPECIFIED.,.F.,.F.,.F.)
B_SPLINE_SURFACE_WITH_KNOTS((2,2),(3,2,3),(0.519229702912058,1.),(0.0365944846644593,
0.0384615384615384,0.0431859278882214),.UNSPECIFIED.)
GEOMETRIC_REPRESENTATION_ITEM()
RATIONAL_B_SPLINE_SURFACE(((0.999326490452218,0.999646063968195,1.,0.999104400928886,
0.998428822114442),(0.999326490452218,0.999646063968195,1.,0.999104400928886,
0.998428822114442)))
REPRESENTATION_ITEM('')
SURFACE()
);
#614=(
BOUNDED_SURFACE()
B_SPLINE_SURFACE(1,2,((#92762,#92763,#92764),(#92765,#92766,#92767)),
 .UNSPECIFIED.,.F.,.F.,.F.)
B_SPLINE_SURFACE_WITH_KNOTS((2,2),(3,3),(0.,1.),(0.0456081671210073,0.057598944781862),
 .UNSPECIFIED.)
GEOMETRIC_REPRESENTATION_ITEM()
RATIONAL_B_SPLINE_SURFACE(((0.997793907739635,0.99636555849969,0.996354522974128),
(0.997793907739635,0.99636555849969,0.996354522974128)))
REPRESENTATION_ITEM('')
SURFACE()
);
#615=(
BOUNDED_SURFACE()
B_SPLINE_SURFACE(1,2,((#92802,#92803,#92804),(#92805,#92806,#92807)),
 .UNSPECIFIED.,.F.,.F.,.F.)
B_SPLINE_SURFACE_WITH_KNOTS((2,2),(3,3),(0.,1.),(0.0556006976522459,0.0675888855446161),
 .UNSPECIFIED.)
GEOMETRIC_REPRESENTATION_ITEM()
RATIONAL_B_SPLINE_SURFACE(((0.996397562408177,0.996150386836003,0.997319912821417),
(0.996397562408177,0.996150386836003,0.997319912821417)))
REPRESENTATION_ITEM('')
SURFACE()
);
#616=(
BOUNDED_SURFACE()
B_SPLINE_SURFACE(1,2,((#92808,#92809,#92810),(#92811,#92812,#92813)),
 .UNSPECIFIED.,.F.,.F.,.F.)
B_SPLINE_SURFACE_WITH_KNOTS((2,2),(3,3),(0.,1.),(0.0657448619281089,0.0758849574338248),
 .UNSPECIFIED.)
GEOMETRIC_REPRESENTATION_ITEM()
RATIONAL_B_SPLINE_SURFACE(((0.996993639757276,0.997798549146193,0.999617032345115),
(0.996993639757276,0.997798549146193,0.999617032345115)))
REPRESENTATION_ITEM('')
SURFACE()
);
#617=(
BOUNDED_SURFACE()
B_SPLINE_SURFACE(1,2,((#92888,#92889,#92890),(#92891,#92892,#92893)),
 .UNSPECIFIED.,.F.,.F.,.F.)
B_SPLINE_SURFACE_WITH_KNOTS((2,2),(3,3),(0.,1.),(0.00560769170938518,0.0176009697615933),
 .UNSPECIFIED.)
GEOMETRIC_REPRESENTATION_ITEM()
RATIONAL_B_SPLINE_SURFACE(((0.998183892106923,0.996573304252679,0.996380621268545),
(0.998183892106923,0.996573304252679,0.996380621268545)))
REPRESENTATION_ITEM('')
SURFACE()
);
#618=(
BOUNDED_SURFACE()
B_SPLINE_SURFACE(1,2,((#92978,#92979,#92980),(#92981,#92982,#92983)),
 .UNSPECIFIED.,.F.,.F.,.F.)
B_SPLINE_SURFACE_WITH_KNOTS((2,2),(3,3),(0.,1.),(0.025590359613201,0.0375948596691667),
 .UNSPECIFIED.)
GEOMETRIC_REPRESENTATION_ITEM()
RATIONAL_B_SPLINE_SURFACE(((0.996753121756002,0.997505687613138,0.999678813023773),
(0.996753121756002,0.997505687613138,0.999678813023773)))
REPRESENTATION_ITEM('')
SURFACE()
);
#619=(
BOUNDED_SURFACE()
B_SPLINE_SURFACE(1,2,((#93001,#93002,#93003,#93004,#93005),(#93006,#93007,
#93008,#93009,#93010)),.UNSPECIFIED.,.F.,.F.,.F.)
B_SPLINE_SURFACE_WITH_KNOTS((2,2),(3,2,3),(0.519229702910745,1.),(0.0365944846644696,
0.0384615384615384,0.0431859278882312),.UNSPECIFIED.)
GEOMETRIC_REPRESENTATION_ITEM()
RATIONAL_B_SPLINE_SURFACE(((0.999326490452223,0.999646063968197,1.,0.999104400928884,
0.998428822114439),(0.999326490452222,0.999646063968197,1.,0.999104400928884,
0.998428822114439)))
REPRESENTATION_ITEM('')
SURFACE()
);
#620=(
BOUNDED_SURFACE()
B_SPLINE_SURFACE(1,2,((#93066,#93067,#93068),(#93069,#93070,#93071)),
 .UNSPECIFIED.,.F.,.F.,.F.)
B_SPLINE_SURFACE_WITH_KNOTS((2,2),(3,3),(0.,1.),(0.045608167121007,0.0575989447818626),
 .UNSPECIFIED.)
GEOMETRIC_REPRESENTATION_ITEM()
RATIONAL_B_SPLINE_SURFACE(((0.997793907739636,0.996365558499691,0.996354522974128),
(0.997793907739636,0.996365558499691,0.996354522974128)))
REPRESENTATION_ITEM('')
SURFACE()
);
#621=(
BOUNDED_SURFACE()
B_SPLINE_SURFACE(1,2,((#93106,#93107,#93108),(#93109,#93110,#93111)),
 .UNSPECIFIED.,.F.,.F.,.F.)
B_SPLINE_SURFACE_WITH_KNOTS((2,2),(3,3),(0.,1.),(0.0556006976522467,0.0675888855446182),
 .UNSPECIFIED.)
GEOMETRIC_REPRESENTATION_ITEM()
RATIONAL_B_SPLINE_SURFACE(((0.996397562408177,0.996150386836003,0.997319912821418),
(0.996397562408177,0.996150386836003,0.997319912821418)))
REPRESENTATION_ITEM('')
SURFACE()
);
#622=(
BOUNDED_SURFACE()
B_SPLINE_SURFACE(1,2,((#93112,#93113,#93114),(#93115,#93116,#93117)),
 .UNSPECIFIED.,.F.,.F.,.F.)
B_SPLINE_SURFACE_WITH_KNOTS((2,2),(3,3),(0.,1.),(0.0657448619281111,0.0758849574338245),
 .UNSPECIFIED.)
GEOMETRIC_REPRESENTATION_ITEM()
RATIONAL_B_SPLINE_SURFACE(((0.996993639757276,0.997798549146193,0.999617032345115),
(0.996993639757276,0.997798549146193,0.999617032345115)))
REPRESENTATION_ITEM('')
SURFACE()
);
#623=(
BOUNDED_SURFACE()
B_SPLINE_SURFACE(1,2,((#93192,#93193,#93194),(#93195,#93196,#93197)),
 .UNSPECIFIED.,.F.,.F.,.F.)
B_SPLINE_SURFACE_WITH_KNOTS((2,2),(3,3),(0.,1.),(0.00560769170938328,0.0176009697615929),
 .UNSPECIFIED.)
GEOMETRIC_REPRESENTATION_ITEM()
RATIONAL_B_SPLINE_SURFACE(((0.998183892106924,0.996573304252679,0.996380621268545),
(0.998183892106924,0.996573304252679,0.996380621268545)))
REPRESENTATION_ITEM('')
SURFACE()
);
#624=(
BOUNDED_SURFACE()
B_SPLINE_SURFACE(1,2,((#93282,#93283,#93284),(#93285,#93286,#93287)),
 .UNSPECIFIED.,.F.,.F.,.F.)
B_SPLINE_SURFACE_WITH_KNOTS((2,2),(3,3),(0.,1.),(0.0255903596132023,0.0375948596691656),
 .UNSPECIFIED.)
GEOMETRIC_REPRESENTATION_ITEM()
RATIONAL_B_SPLINE_SURFACE(((0.996753121756002,0.997505687613138,0.999678813023773),
(0.996753121756002,0.997505687613138,0.999678813023773)))
REPRESENTATION_ITEM('')
SURFACE()
);
#625=(
BOUNDED_SURFACE()
B_SPLINE_SURFACE(1,2,((#93305,#93306,#93307,#93308,#93309),(#93310,#93311,
#93312,#93313,#93314)),.UNSPECIFIED.,.F.,.F.,.F.)
B_SPLINE_SURFACE_WITH_KNOTS((2,2),(3,2,3),(0.519229702909494,1.),(0.0365944846644814,
0.0384615384615384,0.0431859276813475),.UNSPECIFIED.)
GEOMETRIC_REPRESENTATION_ITEM()
RATIONAL_B_SPLINE_SURFACE(((0.999326490452226,0.999646063968199,1.,0.999104400968103,
0.998428822173607),(0.999326490452226,0.999646063968199,1.,0.999104400968103,
0.998428822173607)))
REPRESENTATION_ITEM('')
SURFACE()
);
#626=(
BOUNDED_SURFACE()
B_SPLINE_SURFACE(1,2,((#93370,#93371,#93372),(#93373,#93374,#93375)),
 .UNSPECIFIED.,.F.,.F.,.F.)
B_SPLINE_SURFACE_WITH_KNOTS((2,2),(3,3),(0.,1.),(0.0456081671210083,0.0575989447818618),
 .UNSPECIFIED.)
GEOMETRIC_REPRESENTATION_ITEM()
RATIONAL_B_SPLINE_SURFACE(((0.997793907739635,0.996365558499691,0.996354522974128),
(0.997793907739635,0.996365558499691,0.996354522974128)))
REPRESENTATION_ITEM('')
SURFACE()
);
#627=(
BOUNDED_SURFACE()
B_SPLINE_SURFACE(1,2,((#93410,#93411,#93412),(#93413,#93414,#93415)),
 .UNSPECIFIED.,.F.,.F.,.F.)
B_SPLINE_SURFACE_WITH_KNOTS((2,2),(3,3),(0.,1.),(0.0556006976522459,0.067588885544616),
 .UNSPECIFIED.)
GEOMETRIC_REPRESENTATION_ITEM()
RATIONAL_B_SPLINE_SURFACE(((0.996397562408177,0.996150386836003,0.997319912821417),
(0.996397562408177,0.996150386836003,0.997319912821417)))
REPRESENTATION_ITEM('')
SURFACE()
);
#628=(
BOUNDED_SURFACE()
B_SPLINE_SURFACE(1,2,((#93416,#93417,#93418),(#93419,#93420,#93421)),
 .UNSPECIFIED.,.F.,.F.,.F.)
B_SPLINE_SURFACE_WITH_KNOTS((2,2),(3,3),(0.,1.),(0.0657448619281089,0.0758849574338248),
 .UNSPECIFIED.)
GEOMETRIC_REPRESENTATION_ITEM()
RATIONAL_B_SPLINE_SURFACE(((0.996993639757276,0.997798549146193,0.999617032345115),
(0.996993639757276,0.997798549146193,0.999617032345115)))
REPRESENTATION_ITEM('')
SURFACE()
);
#629=(
BOUNDED_SURFACE()
B_SPLINE_SURFACE(1,2,((#93496,#93497,#93498),(#93499,#93500,#93501)),
 .UNSPECIFIED.,.F.,.F.,.F.)
B_SPLINE_SURFACE_WITH_KNOTS((2,2),(3,3),(0.,1.),(0.00560769170938487,0.0176009697615911),
 .UNSPECIFIED.)
GEOMETRIC_REPRESENTATION_ITEM()
RATIONAL_B_SPLINE_SURFACE(((0.998183892106923,0.996573304252679,0.996380621268545),
(0.998183892106923,0.996573304252679,0.996380621268545)))
REPRESENTATION_ITEM('')
SURFACE()
);
#630=(
BOUNDED_SURFACE()
B_SPLINE_SURFACE(1,2,((#93586,#93587,#93588),(#93589,#93590,#93591)),
 .UNSPECIFIED.,.F.,.F.,.F.)
B_SPLINE_SURFACE_WITH_KNOTS((2,2),(3,3),(0.,1.),(0.0255903596132002,0.0375948596691649),
 .UNSPECIFIED.)
GEOMETRIC_REPRESENTATION_ITEM()
RATIONAL_B_SPLINE_SURFACE(((0.996753121756002,0.997505687613138,0.999678813023773),
(0.996753121756002,0.997505687613138,0.999678813023773)))
REPRESENTATION_ITEM('')
SURFACE()
);
#631=(
BOUNDED_SURFACE()
B_SPLINE_SURFACE(1,2,((#93609,#93610,#93611,#93612,#93613),(#93614,#93615,
#93616,#93617,#93618)),.UNSPECIFIED.,.F.,.F.,.F.)
B_SPLINE_SURFACE_WITH_KNOTS((2,2),(3,2,3),(0.519229702908737,1.),(0.0365944846644944,
0.0384615384615384,0.0431859278882546),.UNSPECIFIED.)
GEOMETRIC_REPRESENTATION_ITEM()
RATIONAL_B_SPLINE_SURFACE(((0.999326490452231,0.999646063968201,1.,0.99910440092888,
0.998428822114433),(0.999326490452231,0.999646063968201,1.,0.99910440092888,
0.998428822114433)))
REPRESENTATION_ITEM('')
SURFACE()
);
#632=(
BOUNDED_SURFACE()
B_SPLINE_SURFACE(1,2,((#93674,#93675,#93676),(#93677,#93678,#93679)),
 .UNSPECIFIED.,.F.,.F.,.F.)
B_SPLINE_SURFACE_WITH_KNOTS((2,2),(3,3),(0.,1.),(0.0456081671210051,0.0575989447818623),
 .UNSPECIFIED.)
GEOMETRIC_REPRESENTATION_ITEM()
RATIONAL_B_SPLINE_SURFACE(((0.997793907739636,0.99636555849969,0.996354522974128),
(0.997793907739636,0.99636555849969,0.996354522974128)))
REPRESENTATION_ITEM('')
SURFACE()
);
#633=(
BOUNDED_SURFACE()
B_SPLINE_SURFACE(1,2,((#93714,#93715,#93716),(#93717,#93718,#93719)),
 .UNSPECIFIED.,.F.,.F.,.F.)
B_SPLINE_SURFACE_WITH_KNOTS((2,2),(3,3),(0.,1.),(0.0556006976522459,0.067588885544615),
 .UNSPECIFIED.)
GEOMETRIC_REPRESENTATION_ITEM()
RATIONAL_B_SPLINE_SURFACE(((0.996397562408177,0.996150386836003,0.997319912821417),
(0.996397562408177,0.996150386836003,0.997319912821417)))
REPRESENTATION_ITEM('')
SURFACE()
);
#634=(
BOUNDED_SURFACE()
B_SPLINE_SURFACE(1,2,((#93720,#93721,#93722),(#93723,#93724,#93725)),
 .UNSPECIFIED.,.F.,.F.,.F.)
B_SPLINE_SURFACE_WITH_KNOTS((2,2),(3,3),(0.,1.),(0.0657448619281078,0.0758849574338246),
 .UNSPECIFIED.)
GEOMETRIC_REPRESENTATION_ITEM()
RATIONAL_B_SPLINE_SURFACE(((0.996993639757276,0.997798549146192,0.999617032345115),
(0.996993639757276,0.997798549146192,0.999617032345115)))
REPRESENTATION_ITEM('')
SURFACE()
);
#635=(
BOUNDED_SURFACE()
B_SPLINE_SURFACE(1,2,((#93800,#93801,#93802),(#93803,#93804,#93805)),
 .UNSPECIFIED.,.F.,.F.,.F.)
B_SPLINE_SURFACE_WITH_KNOTS((2,2),(3,3),(0.,1.),(0.00560769170938445,0.0176009697615928),
 .UNSPECIFIED.)
GEOMETRIC_REPRESENTATION_ITEM()
RATIONAL_B_SPLINE_SURFACE(((0.998183892106924,0.996573304252679,0.996380621268545),
(0.998183892106924,0.996573304252679,0.996380621268545)))
REPRESENTATION_ITEM('')
SURFACE()
);
#636=(
BOUNDED_SURFACE()
B_SPLINE_SURFACE(1,2,((#93890,#93891,#93892),(#93893,#93894,#93895)),
 .UNSPECIFIED.,.F.,.F.,.F.)
B_SPLINE_SURFACE_WITH_KNOTS((2,2),(3,3),(0.,1.),(0.0255903596131976,0.037594859669167),
 .UNSPECIFIED.)
GEOMETRIC_REPRESENTATION_ITEM()
RATIONAL_B_SPLINE_SURFACE(((0.996753121756001,0.997505687613137,0.999678813023773),
(0.996753121756001,0.997505687613137,0.999678813023773)))
REPRESENTATION_ITEM('')
SURFACE()
);
#637=(
BOUNDED_SURFACE()
B_SPLINE_SURFACE(1,2,((#93913,#93914,#93915,#93916,#93917),(#93918,#93919,
#93920,#93921,#93922)),.UNSPECIFIED.,.F.,.F.,.F.)
B_SPLINE_SURFACE_WITH_KNOTS((2,2),(3,2,3),(0.519229702908059,1.),(0.0365944846645068,
0.0384615384615384,0.0431859276813725),.UNSPECIFIED.)
GEOMETRIC_REPRESENTATION_ITEM()
RATIONAL_B_SPLINE_SURFACE(((0.999326490452235,0.999646063968204,1.,0.999104400968098,
0.9984288221736),(0.999326490452235,0.999646063968204,1.,0.999104400968098,
0.9984288221736)))
REPRESENTATION_ITEM('')
SURFACE()
);
#638=(
BOUNDED_SURFACE()
B_SPLINE_SURFACE(1,2,((#93978,#93979,#93980),(#93981,#93982,#93983)),
 .UNSPECIFIED.,.F.,.F.,.F.)
B_SPLINE_SURFACE_WITH_KNOTS((2,2),(3,3),(0.,1.),(0.0456081671210074,0.0575989447818625),
 .UNSPECIFIED.)
GEOMETRIC_REPRESENTATION_ITEM()
RATIONAL_B_SPLINE_SURFACE(((0.997793907739636,0.996365558499691,0.996354522974128),
(0.997793907739636,0.996365558499691,0.996354522974128)))
REPRESENTATION_ITEM('')
SURFACE()
);
#639=(
BOUNDED_SURFACE()
B_SPLINE_SURFACE(1,2,((#94018,#94019,#94020),(#94021,#94022,#94023)),
 .UNSPECIFIED.,.F.,.F.,.F.)
B_SPLINE_SURFACE_WITH_KNOTS((2,2),(3,3),(0.,1.),(0.0556006976522466,0.0675888855446203),
 .UNSPECIFIED.)
GEOMETRIC_REPRESENTATION_ITEM()
RATIONAL_B_SPLINE_SURFACE(((0.996397562408177,0.996150386836003,0.997319912821418),
(0.996397562408177,0.996150386836003,0.997319912821418)))
REPRESENTATION_ITEM('')
SURFACE()
);
#640=(
BOUNDED_SURFACE()
B_SPLINE_SURFACE(1,2,((#94024,#94025,#94026),(#94027,#94028,#94029)),
 .UNSPECIFIED.,.F.,.F.,.F.)
B_SPLINE_SURFACE_WITH_KNOTS((2,2),(3,3),(0.,1.),(0.0657448619281133,0.0758849574338239),
 .UNSPECIFIED.)
GEOMETRIC_REPRESENTATION_ITEM()
RATIONAL_B_SPLINE_SURFACE(((0.996993639757277,0.997798549146193,0.999617032345115),
(0.996993639757277,0.997798549146193,0.999617032345115)))
REPRESENTATION_ITEM('')
SURFACE()
);
#641=(
BOUNDED_SURFACE()
B_SPLINE_SURFACE(1,2,((#94104,#94105,#94106),(#94107,#94108,#94109)),
 .UNSPECIFIED.,.F.,.F.,.F.)
B_SPLINE_SURFACE_WITH_KNOTS((2,2),(3,3),(0.,1.),(0.00560769170938316,0.0176009697615929),
 .UNSPECIFIED.)
GEOMETRIC_REPRESENTATION_ITEM()
RATIONAL_B_SPLINE_SURFACE(((0.998183892106924,0.996573304252679,0.996380621268545),
(0.998183892106924,0.996573304252679,0.996380621268545)))
REPRESENTATION_ITEM('')
SURFACE()
);
#642=(
BOUNDED_SURFACE()
B_SPLINE_SURFACE(1,2,((#94194,#94195,#94196),(#94197,#94198,#94199)),
 .UNSPECIFIED.,.F.,.F.,.F.)
B_SPLINE_SURFACE_WITH_KNOTS((2,2),(3,3),(0.,1.),(0.0255903596132013,0.0375948596691634),
 .UNSPECIFIED.)
GEOMETRIC_REPRESENTATION_ITEM()
RATIONAL_B_SPLINE_SURFACE(((0.996753121756002,0.997505687613138,0.999678813023772),
(0.996753121756002,0.997505687613138,0.999678813023772)))
REPRESENTATION_ITEM('')
SURFACE()
);
#643=(
BOUNDED_SURFACE()
B_SPLINE_SURFACE(1,2,((#94217,#94218,#94219,#94220,#94221),(#94222,#94223,
#94224,#94225,#94226)),.UNSPECIFIED.,.F.,.F.,.F.)
B_SPLINE_SURFACE_WITH_KNOTS((2,2),(3,2,3),(0.519229702907959,1.),(0.0365944846645215,
0.0384615384615384,0.0431859278882817),.UNSPECIFIED.)
GEOMETRIC_REPRESENTATION_ITEM()
RATIONAL_B_SPLINE_SURFACE(((0.99932649045224,0.999646063968206,1.,0.999104400928875,
0.998428822114425),(0.99932649045224,0.999646063968206,1.,0.999104400928875,
0.998428822114425)))
REPRESENTATION_ITEM('')
SURFACE()
);
#644=(
BOUNDED_SURFACE()
B_SPLINE_SURFACE(1,2,((#94282,#94283,#94284),(#94285,#94286,#94287)),
 .UNSPECIFIED.,.F.,.F.,.F.)
B_SPLINE_SURFACE_WITH_KNOTS((2,2),(3,3),(0.,1.),(0.0456081671210053,0.0575989447818599),
 .UNSPECIFIED.)
GEOMETRIC_REPRESENTATION_ITEM()
RATIONAL_B_SPLINE_SURFACE(((0.997793907739636,0.996365558499691,0.996354522974128),
(0.997793907739636,0.996365558499691,0.996354522974128)))
REPRESENTATION_ITEM('')
SURFACE()
);
#645=(
BOUNDED_SURFACE()
B_SPLINE_SURFACE(1,2,((#94322,#94323,#94324),(#94325,#94326,#94327)),
 .UNSPECIFIED.,.F.,.F.,.F.)
B_SPLINE_SURFACE_WITH_KNOTS((2,2),(3,3),(0.,1.),(0.0556006976522416,0.0675888855446144),
 .UNSPECIFIED.)
GEOMETRIC_REPRESENTATION_ITEM()
RATIONAL_B_SPLINE_SURFACE(((0.996397562408177,0.996150386836003,0.997319912821417),
(0.996397562408177,0.996150386836003,0.997319912821417)))
REPRESENTATION_ITEM('')
SURFACE()
);
#646=(
BOUNDED_SURFACE()
B_SPLINE_SURFACE(1,2,((#94328,#94329,#94330),(#94331,#94332,#94333)),
 .UNSPECIFIED.,.F.,.F.,.F.)
B_SPLINE_SURFACE_WITH_KNOTS((2,2),(3,3),(0.,1.),(0.0657448619281068,0.0758849574338251),
 .UNSPECIFIED.)
GEOMETRIC_REPRESENTATION_ITEM()
RATIONAL_B_SPLINE_SURFACE(((0.996993639757276,0.997798549146192,0.999617032345115),
(0.996993639757276,0.997798549146192,0.999617032345115)))
REPRESENTATION_ITEM('')
SURFACE()
);
#647=(
BOUNDED_SURFACE()
B_SPLINE_SURFACE(1,2,((#94408,#94409,#94410),(#94411,#94412,#94413)),
 .UNSPECIFIED.,.F.,.F.,.F.)
B_SPLINE_SURFACE_WITH_KNOTS((2,2),(3,3),(0.,1.),(0.00560769170938346,0.0176009697615929),
 .UNSPECIFIED.)
GEOMETRIC_REPRESENTATION_ITEM()
RATIONAL_B_SPLINE_SURFACE(((0.998183892106924,0.996573304252679,0.996380621268545),
(0.998183892106924,0.996573304252679,0.996380621268545)))
REPRESENTATION_ITEM('')
SURFACE()
);
#648=(
BOUNDED_SURFACE()
B_SPLINE_SURFACE(1,2,((#94498,#94499,#94500),(#94501,#94502,#94503)),
 .UNSPECIFIED.,.F.,.F.,.F.)
B_SPLINE_SURFACE_WITH_KNOTS((2,2),(3,3),(0.,1.),(0.0255903596132008,0.0375948596691676),
 .UNSPECIFIED.)
GEOMETRIC_REPRESENTATION_ITEM()
RATIONAL_B_SPLINE_SURFACE(((0.996753121756002,0.997505687613138,0.999678813023774),
(0.996753121756002,0.997505687613138,0.999678813023774)))
REPRESENTATION_ITEM('')
SURFACE()
);
#649=(
BOUNDED_SURFACE()
B_SPLINE_SURFACE(1,2,((#94521,#94522,#94523,#94524,#94525),(#94526,#94527,
#94528,#94529,#94530)),.UNSPECIFIED.,.F.,.F.,.F.)
B_SPLINE_SURFACE_WITH_KNOTS((2,2),(3,2,3),(0.519229702908038,1.),(0.0365944846645354,
0.0384615384615384,0.0431859278882965),.UNSPECIFIED.)
GEOMETRIC_REPRESENTATION_ITEM()
RATIONAL_B_SPLINE_SURFACE(((0.999326490452245,0.999646063968209,1.,0.999104400928872,
0.998428822114421),(0.999326490452245,0.999646063968209,1.,0.999104400928872,
0.998428822114421)))
REPRESENTATION_ITEM('')
SURFACE()
);
#650=(
BOUNDED_SURFACE()
B_SPLINE_SURFACE(1,2,((#94586,#94587,#94588),(#94589,#94590,#94591)),
 .UNSPECIFIED.,.F.,.F.,.F.)
B_SPLINE_SURFACE_WITH_KNOTS((2,2),(3,3),(0.,1.),(0.0456081671210039,0.0575989447818623),
 .UNSPECIFIED.)
GEOMETRIC_REPRESENTATION_ITEM()
RATIONAL_B_SPLINE_SURFACE(((0.997793907739636,0.996365558499691,0.996354522974129),
(0.997793907739636,0.996365558499691,0.996354522974129)))
REPRESENTATION_ITEM('')
SURFACE()
);
#651=(
BOUNDED_SURFACE()
B_SPLINE_SURFACE(1,2,((#94626,#94627,#94628),(#94629,#94630,#94631)),
 .UNSPECIFIED.,.F.,.F.,.F.)
B_SPLINE_SURFACE_WITH_KNOTS((2,2),(3,3),(0.,1.),(0.0556006976522458,0.0675888855446171),
 .UNSPECIFIED.)
GEOMETRIC_REPRESENTATION_ITEM()
RATIONAL_B_SPLINE_SURFACE(((0.996397562408177,0.996150386836003,0.997319912821417),
(0.996397562408177,0.996150386836003,0.997319912821417)))
REPRESENTATION_ITEM('')
SURFACE()
);
#652=(
BOUNDED_SURFACE()
B_SPLINE_SURFACE(1,2,((#94632,#94633,#94634),(#94635,#94636,#94637)),
 .UNSPECIFIED.,.F.,.F.,.F.)
B_SPLINE_SURFACE_WITH_KNOTS((2,2),(3,3),(0.,1.),(0.06574486192811,0.0758849574338243),
 .UNSPECIFIED.)
GEOMETRIC_REPRESENTATION_ITEM()
RATIONAL_B_SPLINE_SURFACE(((0.996993639757276,0.997798549146193,0.999617032345115),
(0.996993639757276,0.997798549146193,0.999617032345115)))
REPRESENTATION_ITEM('')
SURFACE()
);
#653=(
BOUNDED_SURFACE()
B_SPLINE_SURFACE(1,2,((#94712,#94713,#94714),(#94715,#94716,#94717)),
 .UNSPECIFIED.,.F.,.F.,.F.)
B_SPLINE_SURFACE_WITH_KNOTS((2,2),(3,3),(0.,1.),(0.00560769170938328,0.0176009697615924),
 .UNSPECIFIED.)
GEOMETRIC_REPRESENTATION_ITEM()
RATIONAL_B_SPLINE_SURFACE(((0.998183892106924,0.996573304252679,0.996380621268545),
(0.998183892106924,0.996573304252679,0.996380621268545)))
REPRESENTATION_ITEM('')
SURFACE()
);
#654=(
BOUNDED_SURFACE()
B_SPLINE_SURFACE(1,2,((#94802,#94803,#94804),(#94805,#94806,#94807)),
 .UNSPECIFIED.,.F.,.F.,.F.)
B_SPLINE_SURFACE_WITH_KNOTS((2,2),(3,3),(0.,1.),(0.0255903596131998,0.0375948596691678),
 .UNSPECIFIED.)
GEOMETRIC_REPRESENTATION_ITEM()
RATIONAL_B_SPLINE_SURFACE(((0.996753121756002,0.997505687613138,0.999678813023774),
(0.996753121756002,0.997505687613138,0.999678813023774)))
REPRESENTATION_ITEM('')
SURFACE()
);
#655=(
BOUNDED_SURFACE()
B_SPLINE_SURFACE(1,2,((#94825,#94826,#94827,#94828,#94829),(#94830,#94831,
#94832,#94833,#94834)),.UNSPECIFIED.,.F.,.F.,.F.)
B_SPLINE_SURFACE_WITH_KNOTS((2,2),(3,2,3),(0.519229702908415,1.),(0.0365944846645497,
0.0384615384615384,0.0431859278883109),.UNSPECIFIED.)
GEOMETRIC_REPRESENTATION_ITEM()
RATIONAL_B_SPLINE_SURFACE(((0.99932649045225,0.999646063968212,1.,0.999104400928869,
0.998428822114416),(0.99932649045225,0.999646063968212,1.,0.999104400928869,
0.998428822114416)))
REPRESENTATION_ITEM('')
SURFACE()
);
#656=(
BOUNDED_SURFACE()
B_SPLINE_SURFACE(1,2,((#94890,#94891,#94892),(#94893,#94894,#94895)),
 .UNSPECIFIED.,.F.,.F.,.F.)
B_SPLINE_SURFACE_WITH_KNOTS((2,2),(3,3),(0.,1.),(0.045608167121011,0.0575989447818594),
 .UNSPECIFIED.)
GEOMETRIC_REPRESENTATION_ITEM()
RATIONAL_B_SPLINE_SURFACE(((0.997793907739635,0.996365558499691,0.996354522974128),
(0.997793907739635,0.996365558499691,0.996354522974128)))
REPRESENTATION_ITEM('')
SURFACE()
);
#657=(
BOUNDED_SURFACE()
B_SPLINE_SURFACE(1,2,((#94930,#94931,#94932),(#94933,#94934,#94935)),
 .UNSPECIFIED.,.F.,.F.,.F.)
B_SPLINE_SURFACE_WITH_KNOTS((2,2),(3,3),(0.,1.),(0.0556006976522414,0.0675888855446165),
 .UNSPECIFIED.)
GEOMETRIC_REPRESENTATION_ITEM()
RATIONAL_B_SPLINE_SURFACE(((0.996397562408177,0.996150386836003,0.997319912821417),
(0.996397562408177,0.996150386836003,0.997319912821417)))
REPRESENTATION_ITEM('')
SURFACE()
);
#658=(
BOUNDED_SURFACE()
B_SPLINE_SURFACE(1,2,((#94936,#94937,#94938),(#94939,#94940,#94941)),
 .UNSPECIFIED.,.F.,.F.,.F.)
B_SPLINE_SURFACE_WITH_KNOTS((2,2),(3,3),(0.,1.),(0.0657448619281089,0.0758849574338246),
 .UNSPECIFIED.)
GEOMETRIC_REPRESENTATION_ITEM()
RATIONAL_B_SPLINE_SURFACE(((0.996993639757276,0.997798549146193,0.999617032345115),
(0.996993639757276,0.997798549146193,0.999617032345115)))
REPRESENTATION_ITEM('')
SURFACE()
);
#659=(
BOUNDED_SURFACE()
B_SPLINE_SURFACE(1,2,((#95016,#95017,#95018),(#95019,#95020,#95021)),
 .UNSPECIFIED.,.F.,.F.,.F.)
B_SPLINE_SURFACE_WITH_KNOTS((2,2),(3,3),(0.,1.),(0.00560769170938354,0.0176009697615918),
 .UNSPECIFIED.)
GEOMETRIC_REPRESENTATION_ITEM()
RATIONAL_B_SPLINE_SURFACE(((0.998183892106924,0.996573304252679,0.996380621268545),
(0.998183892106924,0.996573304252679,0.996380621268545)))
REPRESENTATION_ITEM('')
SURFACE()
);
#660=(
BOUNDED_SURFACE()
B_SPLINE_SURFACE(1,2,((#95106,#95107,#95108),(#95109,#95110,#95111)),
 .UNSPECIFIED.,.F.,.F.,.F.)
B_SPLINE_SURFACE_WITH_KNOTS((2,2),(3,3),(0.,1.),(0.0255903596131989,0.037594859669165),
 .UNSPECIFIED.)
GEOMETRIC_REPRESENTATION_ITEM()
RATIONAL_B_SPLINE_SURFACE(((0.996753121756001,0.997505687613137,0.999678813023773),
(0.996753121756001,0.997505687613137,0.999678813023773)))
REPRESENTATION_ITEM('')
SURFACE()
);
#661=(
BOUNDED_SURFACE()
B_SPLINE_SURFACE(1,2,((#95129,#95130,#95131,#95132,#95133),(#95134,#95135,
#95136,#95137,#95138)),.UNSPECIFIED.,.F.,.F.,.F.)
B_SPLINE_SURFACE_WITH_KNOTS((2,2),(3,2,3),(0.519229702909028,1.),(0.036594484664565,
0.0384615384615384,0.0431859278100856),.UNSPECIFIED.)
GEOMETRIC_REPRESENTATION_ITEM()
RATIONAL_B_SPLINE_SURFACE(((0.999326490452255,0.999646063968215,1.,0.999104400943698,
0.998428822136789),(0.999326490452255,0.999646063968215,1.,0.999104400943698,
0.998428822136789)))
REPRESENTATION_ITEM('')
SURFACE()
);
#662=(
BOUNDED_SURFACE()
B_SPLINE_SURFACE(1,2,((#95194,#95195,#95196),(#95197,#95198,#95199)),
 .UNSPECIFIED.,.F.,.F.,.F.)
B_SPLINE_SURFACE_WITH_KNOTS((2,2),(3,3),(0.,1.),(0.0456081671210063,0.0575989447818626),
 .UNSPECIFIED.)
GEOMETRIC_REPRESENTATION_ITEM()
RATIONAL_B_SPLINE_SURFACE(((0.997793907739636,0.99636555849969,0.996354522974128),
(0.997793907739636,0.99636555849969,0.996354522974128)))
REPRESENTATION_ITEM('')
SURFACE()
);
#663=(
BOUNDED_SURFACE()
B_SPLINE_SURFACE(1,2,((#95234,#95235,#95236),(#95237,#95238,#95239)),
 .UNSPECIFIED.,.F.,.F.,.F.)
B_SPLINE_SURFACE_WITH_KNOTS((2,2),(3,3),(0.,1.),(0.0556006976522473,0.0675888855446128),
 .UNSPECIFIED.)
GEOMETRIC_REPRESENTATION_ITEM()
RATIONAL_B_SPLINE_SURFACE(((0.996397562408177,0.996150386836004,0.997319912821417),
(0.996397562408177,0.996150386836004,0.997319912821417)))
REPRESENTATION_ITEM('')
SURFACE()
);
#664=(
BOUNDED_SURFACE()
B_SPLINE_SURFACE(1,2,((#95240,#95241,#95242),(#95243,#95244,#95245)),
 .UNSPECIFIED.,.F.,.F.,.F.)
B_SPLINE_SURFACE_WITH_KNOTS((2,2),(3,3),(0.,1.),(0.0657448619281057,0.0758849574338256),
 .UNSPECIFIED.)
GEOMETRIC_REPRESENTATION_ITEM()
RATIONAL_B_SPLINE_SURFACE(((0.996993639757275,0.997798549146192,0.999617032345116),
(0.996993639757275,0.997798549146192,0.999617032345116)))
REPRESENTATION_ITEM('')
SURFACE()
);
#665=(
BOUNDED_SURFACE()
B_SPLINE_SURFACE(1,2,((#95320,#95321,#95322),(#95323,#95324,#95325)),
 .UNSPECIFIED.,.F.,.F.,.F.)
B_SPLINE_SURFACE_WITH_KNOTS((2,2),(3,3),(0.,1.),(0.00560769170938434,0.0176009697615933),
 .UNSPECIFIED.)
GEOMETRIC_REPRESENTATION_ITEM()
RATIONAL_B_SPLINE_SURFACE(((0.998183892106924,0.996573304252679,0.996380621268545),
(0.998183892106924,0.996573304252679,0.996380621268545)))
REPRESENTATION_ITEM('')
SURFACE()
);
#666=(
BOUNDED_SURFACE()
B_SPLINE_SURFACE(1,2,((#95410,#95411,#95412),(#95413,#95414,#95415)),
 .UNSPECIFIED.,.F.,.F.,.F.)
B_SPLINE_SURFACE_WITH_KNOTS((2,2),(3,3),(0.,1.),(0.0255903596132,0.037594859669166),
 .UNSPECIFIED.)
GEOMETRIC_REPRESENTATION_ITEM()
RATIONAL_B_SPLINE_SURFACE(((0.996753121756002,0.997505687613138,0.999678813023773),
(0.996753121756002,0.997505687613138,0.999678813023773)))
REPRESENTATION_ITEM('')
SURFACE()
);
#667=(
BOUNDED_SURFACE()
B_SPLINE_SURFACE(1,2,((#95433,#95434,#95435,#95436,#95437),(#95438,#95439,
#95440,#95441,#95442)),.UNSPECIFIED.,.F.,.F.,.F.)
B_SPLINE_SURFACE_WITH_KNOTS((2,2),(3,2,3),(0.519229702909967,1.),(0.0365944846645798,
0.0384615384615384,0.0431859276814445),.UNSPECIFIED.)
GEOMETRIC_REPRESENTATION_ITEM()
RATIONAL_B_SPLINE_SURFACE(((0.99932649045226,0.999646063968218,1.,0.999104400968085,
0.99842882217358),(0.99932649045226,0.999646063968218,1.,0.999104400968085,
0.99842882217358)))
REPRESENTATION_ITEM('')
SURFACE()
);
#668=(
BOUNDED_SURFACE()
B_SPLINE_SURFACE(1,2,((#95498,#95499,#95500),(#95501,#95502,#95503)),
 .UNSPECIFIED.,.F.,.F.,.F.)
B_SPLINE_SURFACE_WITH_KNOTS((2,2),(3,3),(0.,1.),(0.0456081671210074,0.0575989447818626),
 .UNSPECIFIED.)
GEOMETRIC_REPRESENTATION_ITEM()
RATIONAL_B_SPLINE_SURFACE(((0.997793907739635,0.996365558499691,0.996354522974128),
(0.997793907739635,0.996365558499691,0.996354522974128)))
REPRESENTATION_ITEM('')
SURFACE()
);
#669=(
BOUNDED_SURFACE()
B_SPLINE_SURFACE(1,2,((#95538,#95539,#95540),(#95541,#95542,#95543)),
 .UNSPECIFIED.,.F.,.F.,.F.)
B_SPLINE_SURFACE_WITH_KNOTS((2,2),(3,3),(0.,1.),(0.0556006976522466,0.0675888855446202),
 .UNSPECIFIED.)
GEOMETRIC_REPRESENTATION_ITEM()
RATIONAL_B_SPLINE_SURFACE(((0.996397562408177,0.996150386836003,0.997319912821418),
(0.996397562408177,0.996150386836003,0.997319912821418)))
REPRESENTATION_ITEM('')
SURFACE()
);
#670=(
BOUNDED_SURFACE()
B_SPLINE_SURFACE(1,2,((#95544,#95545,#95546),(#95547,#95548,#95549)),
 .UNSPECIFIED.,.F.,.F.,.F.)
B_SPLINE_SURFACE_WITH_KNOTS((2,2),(3,3),(0.,1.),(0.0657448619281132,0.0758849574338236),
 .UNSPECIFIED.)
GEOMETRIC_REPRESENTATION_ITEM()
RATIONAL_B_SPLINE_SURFACE(((0.996993639757277,0.997798549146193,0.999617032345115),
(0.996993639757277,0.997798549146193,0.999617032345115)))
REPRESENTATION_ITEM('')
SURFACE()
);
#671=(
BOUNDED_SURFACE()
B_SPLINE_SURFACE(1,2,((#95624,#95625,#95626),(#95627,#95628,#95629)),
 .UNSPECIFIED.,.F.,.F.,.F.)
B_SPLINE_SURFACE_WITH_KNOTS((2,2),(3,3),(0.,1.),(0.00560769170938474,0.0176009697615934),
 .UNSPECIFIED.)
GEOMETRIC_REPRESENTATION_ITEM()
RATIONAL_B_SPLINE_SURFACE(((0.998183892106924,0.996573304252679,0.996380621268545),
(0.998183892106924,0.996573304252679,0.996380621268545)))
REPRESENTATION_ITEM('')
SURFACE()
);
#672=(
BOUNDED_SURFACE()
B_SPLINE_SURFACE(1,2,((#95714,#95715,#95716),(#95717,#95718,#95719)),
 .UNSPECIFIED.,.F.,.F.,.F.)
B_SPLINE_SURFACE_WITH_KNOTS((2,2),(3,3),(0.,1.),(0.0255903596132025,0.0375948596691633),
 .UNSPECIFIED.)
GEOMETRIC_REPRESENTATION_ITEM()
RATIONAL_B_SPLINE_SURFACE(((0.996753121756002,0.997505687613138,0.999678813023772),
(0.996753121756002,0.997505687613138,0.999678813023772)))
REPRESENTATION_ITEM('')
SURFACE()
);
#673=(
BOUNDED_SURFACE()
B_SPLINE_SURFACE(1,2,((#95737,#95738,#95739,#95740,#95741),(#95742,#95743,
#95744,#95745,#95746)),.UNSPECIFIED.,.F.,.F.,.F.)
B_SPLINE_SURFACE_WITH_KNOTS((2,2),(3,2,3),(0.519229702911282,1.),(0.036594484664593,
0.0384615384615384,0.0431859278883545),.UNSPECIFIED.)
GEOMETRIC_REPRESENTATION_ITEM()
RATIONAL_B_SPLINE_SURFACE(((0.999326490452264,0.99964606396822,1.,0.999104400928861,
0.998428822114404),(0.999326490452264,0.99964606396822,1.,0.999104400928861,
0.998428822114404)))
REPRESENTATION_ITEM('')
SURFACE()
);
#674=(
BOUNDED_SURFACE()
B_SPLINE_SURFACE(1,2,((#95802,#95803,#95804),(#95805,#95806,#95807)),
 .UNSPECIFIED.,.F.,.F.,.F.)
B_SPLINE_SURFACE_WITH_KNOTS((2,2),(3,3),(0.,1.),(0.045608167121007,0.0575989447818626),
 .UNSPECIFIED.)
GEOMETRIC_REPRESENTATION_ITEM()
RATIONAL_B_SPLINE_SURFACE(((0.997793907739636,0.996365558499691,0.996354522974128),
(0.997793907739636,0.996365558499691,0.996354522974128)))
REPRESENTATION_ITEM('')
SURFACE()
);
#675=(
BOUNDED_SURFACE()
B_SPLINE_SURFACE(1,2,((#95842,#95843,#95844),(#95845,#95846,#95847)),
 .UNSPECIFIED.,.F.,.F.,.F.)
B_SPLINE_SURFACE_WITH_KNOTS((2,2),(3,3),(0.,1.),(0.0556006976522468,0.067588885544617),
 .UNSPECIFIED.)
GEOMETRIC_REPRESENTATION_ITEM()
RATIONAL_B_SPLINE_SURFACE(((0.996397562408177,0.996150386836003,0.997319912821417),
(0.996397562408177,0.996150386836003,0.997319912821417)))
REPRESENTATION_ITEM('')
SURFACE()
);
#676=(
BOUNDED_SURFACE()
B_SPLINE_SURFACE(1,2,((#95848,#95849,#95850),(#95851,#95852,#95853)),
 .UNSPECIFIED.,.F.,.F.,.F.)
B_SPLINE_SURFACE_WITH_KNOTS((2,2),(3,3),(0.,1.),(0.06574486192811,0.0758849574338238),
 .UNSPECIFIED.)
GEOMETRIC_REPRESENTATION_ITEM()
RATIONAL_B_SPLINE_SURFACE(((0.996993639757276,0.997798549146193,0.999617032345115),
(0.996993639757276,0.997798549146193,0.999617032345115)))
REPRESENTATION_ITEM('')
SURFACE()
);
#677=(
BOUNDED_SURFACE()
B_SPLINE_SURFACE(1,2,((#95928,#95929,#95930),(#95931,#95932,#95933)),
 .UNSPECIFIED.,.F.,.F.,.F.)
B_SPLINE_SURFACE_WITH_KNOTS((2,2),(3,3),(0.,1.),(0.00560769170938203,0.017600969761593),
 .UNSPECIFIED.)
GEOMETRIC_REPRESENTATION_ITEM()
RATIONAL_B_SPLINE_SURFACE(((0.998183892106924,0.996573304252679,0.996380621268545),
(0.998183892106924,0.996573304252679,0.996380621268545)))
REPRESENTATION_ITEM('')
SURFACE()
);
#678=(
BOUNDED_SURFACE()
B_SPLINE_SURFACE(1,2,((#96018,#96019,#96020),(#96021,#96022,#96023)),
 .UNSPECIFIED.,.F.,.F.,.F.)
B_SPLINE_SURFACE_WITH_KNOTS((2,2),(3,3),(0.,1.),(0.0255903596131999,0.0375948596691669),
 .UNSPECIFIED.)
GEOMETRIC_REPRESENTATION_ITEM()
RATIONAL_B_SPLINE_SURFACE(((0.996753121756002,0.997505687613138,0.999678813023773),
(0.996753121756002,0.997505687613138,0.999678813023773)))
REPRESENTATION_ITEM('')
SURFACE()
);
#679=(
BOUNDED_SURFACE()
B_SPLINE_SURFACE(1,2,((#96041,#96042,#96043,#96044,#96045),(#96046,#96047,
#96048,#96049,#96050)),.UNSPECIFIED.,.F.,.F.,.F.)
B_SPLINE_SURFACE_WITH_KNOTS((2,2),(3,2,3),(0.51922970291275,1.),(0.036594484664607,
0.0384615384615384,0.0431859278883671),.UNSPECIFIED.)
GEOMETRIC_REPRESENTATION_ITEM()
RATIONAL_B_SPLINE_SURFACE(((0.999326490452269,0.999646063968222,1.,0.999104400928858,
0.998428822114401),(0.999326490452269,0.999646063968222,1.,0.999104400928858,
0.998428822114401)))
REPRESENTATION_ITEM('')
SURFACE()
);
#680=(
BOUNDED_SURFACE()
B_SPLINE_SURFACE(1,2,((#96106,#96107,#96108),(#96109,#96110,#96111)),
 .UNSPECIFIED.,.F.,.F.,.F.)
B_SPLINE_SURFACE_WITH_KNOTS((2,2),(3,3),(0.,1.),(0.0456081671210039,0.0575989447818618),
 .UNSPECIFIED.)
GEOMETRIC_REPRESENTATION_ITEM()
RATIONAL_B_SPLINE_SURFACE(((0.997793907739636,0.996365558499691,0.996354522974128),
(0.997793907739636,0.996365558499691,0.996354522974128)))
REPRESENTATION_ITEM('')
SURFACE()
);
#681=(
BOUNDED_SURFACE()
B_SPLINE_SURFACE(1,2,((#96146,#96147,#96148),(#96149,#96150,#96151)),
 .UNSPECIFIED.,.F.,.F.,.F.)
B_SPLINE_SURFACE_WITH_KNOTS((2,2),(3,3),(0.,1.),(0.0556006976522446,0.0675888855446173),
 .UNSPECIFIED.)
GEOMETRIC_REPRESENTATION_ITEM()
RATIONAL_B_SPLINE_SURFACE(((0.996397562408177,0.996150386836003,0.997319912821418),
(0.996397562408177,0.996150386836003,0.997319912821418)))
REPRESENTATION_ITEM('')
SURFACE()
);
#682=(
BOUNDED_SURFACE()
B_SPLINE_SURFACE(1,2,((#96152,#96153,#96154),(#96155,#96156,#96157)),
 .UNSPECIFIED.,.F.,.F.,.F.)
B_SPLINE_SURFACE_WITH_KNOTS((2,2),(3,3),(0.,1.),(0.0657448619281101,0.0758849574338239),
 .UNSPECIFIED.)
GEOMETRIC_REPRESENTATION_ITEM()
RATIONAL_B_SPLINE_SURFACE(((0.996993639757276,0.997798549146193,0.999617032345115),
(0.996993639757276,0.997798549146193,0.999617032345115)))
REPRESENTATION_ITEM('')
SURFACE()
);
#683=(
BOUNDED_SURFACE()
B_SPLINE_SURFACE(1,2,((#96232,#96233,#96234),(#96235,#96236,#96237)),
 .UNSPECIFIED.,.F.,.F.,.F.)
B_SPLINE_SURFACE_WITH_KNOTS((2,2),(3,3),(0.,1.),(0.00560769170938346,0.0176009697615912),
 .UNSPECIFIED.)
GEOMETRIC_REPRESENTATION_ITEM()
RATIONAL_B_SPLINE_SURFACE(((0.998183892106924,0.996573304252679,0.996380621268545),
(0.998183892106924,0.996573304252679,0.996380621268545)))
REPRESENTATION_ITEM('')
SURFACE()
);
#684=(
BOUNDED_SURFACE()
B_SPLINE_SURFACE(1,2,((#96322,#96323,#96324),(#96325,#96326,#96327)),
 .UNSPECIFIED.,.F.,.F.,.F.)
B_SPLINE_SURFACE_WITH_KNOTS((2,2),(3,3),(0.,1.),(0.0255903596131992,0.0375948596691636),
 .UNSPECIFIED.)
GEOMETRIC_REPRESENTATION_ITEM()
RATIONAL_B_SPLINE_SURFACE(((0.996753121756001,0.997505687613137,0.999678813023772),
(0.996753121756001,0.997505687613137,0.999678813023772)))
REPRESENTATION_ITEM('')
SURFACE()
);
#685=(
BOUNDED_SURFACE()
B_SPLINE_SURFACE(1,2,((#96345,#96346,#96347,#96348,#96349),(#96350,#96351,
#96352,#96353,#96354)),.UNSPECIFIED.,.F.,.F.,.F.)
B_SPLINE_SURFACE_WITH_KNOTS((2,2),(3,2,3),(0.51922970291459,1.),(0.0365944846646184,
0.0384615384615384,0.0431859278883792),.UNSPECIFIED.)
GEOMETRIC_REPRESENTATION_ITEM()
RATIONAL_B_SPLINE_SURFACE(((0.999326490452273,0.999646063968225,1.,0.999104400928856,
0.998428822114397),(0.999326490452273,0.999646063968225,1.,0.999104400928856,
0.998428822114397)))
REPRESENTATION_ITEM('')
SURFACE()
);
#686=(
BOUNDED_SURFACE()
B_SPLINE_SURFACE(1,2,((#96410,#96411,#96412),(#96413,#96414,#96415)),
 .UNSPECIFIED.,.F.,.F.,.F.)
B_SPLINE_SURFACE_WITH_KNOTS((2,2),(3,3),(0.,1.),(0.0456081671210053,0.0575989447818604),
 .UNSPECIFIED.)
GEOMETRIC_REPRESENTATION_ITEM()
RATIONAL_B_SPLINE_SURFACE(((0.997793907739636,0.996365558499691,0.996354522974128),
(0.997793907739636,0.996365558499691,0.996354522974128)))
REPRESENTATION_ITEM('')
SURFACE()
);
#687=(
BOUNDED_SURFACE()
B_SPLINE_SURFACE(1,2,((#96450,#96451,#96452),(#96453,#96454,#96455)),
 .UNSPECIFIED.,.F.,.F.,.F.)
B_SPLINE_SURFACE_WITH_KNOTS((2,2),(3,3),(0.,1.),(0.0556006976522424,0.0675888855446163),
 .UNSPECIFIED.)
GEOMETRIC_REPRESENTATION_ITEM()
RATIONAL_B_SPLINE_SURFACE(((0.996397562408177,0.996150386836003,0.997319912821417),
(0.996397562408177,0.996150386836003,0.997319912821417)))
REPRESENTATION_ITEM('')
SURFACE()
);
#688=(
BOUNDED_SURFACE()
B_SPLINE_SURFACE(1,2,((#96456,#96457,#96458),(#96459,#96460,#96461)),
 .UNSPECIFIED.,.F.,.F.,.F.)
B_SPLINE_SURFACE_WITH_KNOTS((2,2),(3,3),(0.,1.),(0.065744861928109,0.0758849574338236),
 .UNSPECIFIED.)
GEOMETRIC_REPRESENTATION_ITEM()
RATIONAL_B_SPLINE_SURFACE(((0.996993639757276,0.997798549146192,0.999617032345115),
(0.996993639757276,0.997798549146192,0.999617032345115)))
REPRESENTATION_ITEM('')
SURFACE()
);
#689=(
BOUNDED_SURFACE()
B_SPLINE_SURFACE(1,2,((#96536,#96537,#96538),(#96539,#96540,#96541)),
 .UNSPECIFIED.,.F.,.F.,.F.)
B_SPLINE_SURFACE_WITH_KNOTS((2,2),(3,3),(0.,1.),(0.00560769170938321,0.0176009697615924),
 .UNSPECIFIED.)
GEOMETRIC_REPRESENTATION_ITEM()
RATIONAL_B_SPLINE_SURFACE(((0.998183892106924,0.996573304252679,0.996380621268545),
(0.998183892106924,0.996573304252679,0.996380621268545)))
REPRESENTATION_ITEM('')
SURFACE()
);
#690=(
BOUNDED_SURFACE()
B_SPLINE_SURFACE(1,2,((#96626,#96627,#96628),(#96629,#96630,#96631)),
 .UNSPECIFIED.,.F.,.F.,.F.)
B_SPLINE_SURFACE_WITH_KNOTS((2,2),(3,3),(0.,1.),(0.0255903596131988,0.0375948596691661),
 .UNSPECIFIED.)
GEOMETRIC_REPRESENTATION_ITEM()
RATIONAL_B_SPLINE_SURFACE(((0.996753121756001,0.997505687613137,0.999678813023773),
(0.996753121756001,0.997505687613137,0.999678813023773)))
REPRESENTATION_ITEM('')
SURFACE()
);
#691=(
BOUNDED_SURFACE()
B_SPLINE_SURFACE(1,2,((#96649,#96650,#96651,#96652,#96653),(#96654,#96655,
#96656,#96657,#96658)),.UNSPECIFIED.,.F.,.F.,.F.)
B_SPLINE_SURFACE_WITH_KNOTS((2,2),(3,2,3),(0.519229702916504,1.),(0.036594484664629,
0.0384615384615384,0.0431859278883907),.UNSPECIFIED.)
GEOMETRIC_REPRESENTATION_ITEM()
RATIONAL_B_SPLINE_SURFACE(((0.999326490452277,0.999646063968227,1.,0.999104400928854,
0.998428822114394),(0.999326490452277,0.999646063968227,1.,0.999104400928854,
0.998428822114394)))
REPRESENTATION_ITEM('')
SURFACE()
);
#692=(
BOUNDED_SURFACE()
B_SPLINE_SURFACE(1,2,((#96714,#96715,#96716),(#96717,#96718,#96719)),
 .UNSPECIFIED.,.F.,.F.,.F.)
B_SPLINE_SURFACE_WITH_KNOTS((2,2),(3,3),(0.,1.),(0.0456081671210051,0.0575989447818622),
 .UNSPECIFIED.)
GEOMETRIC_REPRESENTATION_ITEM()
RATIONAL_B_SPLINE_SURFACE(((0.997793907739636,0.996365558499691,0.996354522974128),
(0.997793907739636,0.996365558499691,0.996354522974128)))
REPRESENTATION_ITEM('')
SURFACE()
);
#693=(
BOUNDED_SURFACE()
B_SPLINE_SURFACE(1,2,((#96754,#96755,#96756),(#96757,#96758,#96759)),
 .UNSPECIFIED.,.F.,.F.,.F.)
B_SPLINE_SURFACE_WITH_KNOTS((2,2),(3,3),(0.,1.),(0.0556006976522459,0.0675888855446151),
 .UNSPECIFIED.)
GEOMETRIC_REPRESENTATION_ITEM()
RATIONAL_B_SPLINE_SURFACE(((0.996397562408177,0.996150386836003,0.997319912821417),
(0.996397562408177,0.996150386836003,0.997319912821417)))
REPRESENTATION_ITEM('')
SURFACE()
);
#694=(
BOUNDED_SURFACE()
B_SPLINE_SURFACE(1,2,((#96760,#96761,#96762),(#96763,#96764,#96765)),
 .UNSPECIFIED.,.F.,.F.,.F.)
B_SPLINE_SURFACE_WITH_KNOTS((2,2),(3,3),(0.,1.),(0.065744861928108,0.0758849574338239),
 .UNSPECIFIED.)
GEOMETRIC_REPRESENTATION_ITEM()
RATIONAL_B_SPLINE_SURFACE(((0.996993639757276,0.997798549146192,0.999617032345115),
(0.996993639757276,0.997798549146192,0.999617032345115)))
REPRESENTATION_ITEM('')
SURFACE()
);
#695=(
BOUNDED_SURFACE()
B_SPLINE_SURFACE(1,2,((#96840,#96841,#96842),(#96843,#96844,#96845)),
 .UNSPECIFIED.,.F.,.F.,.F.)
B_SPLINE_SURFACE_WITH_KNOTS((2,2),(3,3),(0.,1.),(0.0056076917093823,0.0176009697615919),
 .UNSPECIFIED.)
GEOMETRIC_REPRESENTATION_ITEM()
RATIONAL_B_SPLINE_SURFACE(((0.998183892106924,0.996573304252679,0.996380621268545),
(0.998183892106924,0.996573304252679,0.996380621268545)))
REPRESENTATION_ITEM('')
SURFACE()
);
#696=(
BOUNDED_SURFACE()
B_SPLINE_SURFACE(1,2,((#96930,#96931,#96932),(#96933,#96934,#96935)),
 .UNSPECIFIED.,.F.,.F.,.F.)
B_SPLINE_SURFACE_WITH_KNOTS((2,2),(3,3),(0.,1.),(0.0255903596131989,0.0375948596691636),
 .UNSPECIFIED.)
GEOMETRIC_REPRESENTATION_ITEM()
RATIONAL_B_SPLINE_SURFACE(((0.996753121756001,0.997505687613137,0.999678813023772),
(0.996753121756001,0.997505687613137,0.999678813023772)))
REPRESENTATION_ITEM('')
SURFACE()
);
#697=(
BOUNDED_SURFACE()
B_SPLINE_SURFACE(1,2,((#96953,#96954,#96955,#96956,#96957),(#96958,#96959,
#96960,#96961,#96962)),.UNSPECIFIED.,.F.,.F.,.F.)
B_SPLINE_SURFACE_WITH_KNOTS((2,2),(3,2,3),(0.519229702918739,1.),(0.0365944846646386,
0.0384615384615384,0.0431859278884007),.UNSPECIFIED.)
GEOMETRIC_REPRESENTATION_ITEM()
RATIONAL_B_SPLINE_SURFACE(((0.99932649045228,0.999646063968229,1.,0.999104400928852,
0.998428822114391),(0.99932649045228,0.999646063968229,1.,0.999104400928852,
0.998428822114391)))
REPRESENTATION_ITEM('')
SURFACE()
);
#698=(
BOUNDED_SURFACE()
B_SPLINE_SURFACE(1,2,((#97018,#97019,#97020),(#97021,#97022,#97023)),
 .UNSPECIFIED.,.F.,.F.,.F.)
B_SPLINE_SURFACE_WITH_KNOTS((2,2),(3,3),(0.,1.),(0.0456081671210051,0.0575989447818617),
 .UNSPECIFIED.)
GEOMETRIC_REPRESENTATION_ITEM()
RATIONAL_B_SPLINE_SURFACE(((0.997793907739636,0.996365558499691,0.996354522974128),
(0.997793907739636,0.996365558499691,0.996354522974128)))
REPRESENTATION_ITEM('')
SURFACE()
);
#699=(
BOUNDED_SURFACE()
B_SPLINE_SURFACE(1,2,((#97058,#97059,#97060),(#97061,#97062,#97063)),
 .UNSPECIFIED.,.F.,.F.,.F.)
B_SPLINE_SURFACE_WITH_KNOTS((2,2),(3,3),(0.,1.),(0.0556006976522445,0.0675888855446183),
 .UNSPECIFIED.)
GEOMETRIC_REPRESENTATION_ITEM()
RATIONAL_B_SPLINE_SURFACE(((0.996397562408177,0.996150386836003,0.997319912821418),
(0.996397562408177,0.996150386836003,0.997319912821418)))
REPRESENTATION_ITEM('')
SURFACE()
);
#700=(
BOUNDED_SURFACE()
B_SPLINE_SURFACE(1,2,((#97064,#97065,#97066),(#97067,#97068,#97069)),
 .UNSPECIFIED.,.F.,.F.,.F.)
B_SPLINE_SURFACE_WITH_KNOTS((2,2),(3,3),(0.,1.),(0.0657448619281112,0.0758849574338233),
 .UNSPECIFIED.)
GEOMETRIC_REPRESENTATION_ITEM()
RATIONAL_B_SPLINE_SURFACE(((0.996993639757276,0.997798549146193,0.999617032345115),
(0.996993639757276,0.997798549146193,0.999617032345115)))
REPRESENTATION_ITEM('')
SURFACE()
);
#701=(
BOUNDED_SURFACE()
B_SPLINE_SURFACE(1,2,((#97144,#97145,#97146),(#97147,#97148,#97149)),
 .UNSPECIFIED.,.F.,.F.,.F.)
B_SPLINE_SURFACE_WITH_KNOTS((2,2),(3,3),(0.,1.),(0.00560769170938328,0.0176009697615924),
 .UNSPECIFIED.)
GEOMETRIC_REPRESENTATION_ITEM()
RATIONAL_B_SPLINE_SURFACE(((0.998183892106924,0.996573304252679,0.996380621268545),
(0.998183892106924,0.996573304252679,0.996380621268545)))
REPRESENTATION_ITEM('')
SURFACE()
);
#702=(
BOUNDED_SURFACE()
B_SPLINE_SURFACE(1,2,((#97234,#97235,#97236),(#97237,#97238,#97239)),
 .UNSPECIFIED.,.F.,.F.,.F.)
B_SPLINE_SURFACE_WITH_KNOTS((2,2),(3,3),(0.,1.),(0.0255903596132,0.0375948596691669),
 .UNSPECIFIED.)
GEOMETRIC_REPRESENTATION_ITEM()
RATIONAL_B_SPLINE_SURFACE(((0.996753121756002,0.997505687613138,0.999678813023773),
(0.996753121756002,0.997505687613138,0.999678813023773)))
REPRESENTATION_ITEM('')
SURFACE()
);
#703=(
BOUNDED_SURFACE()
B_SPLINE_SURFACE(1,2,((#97257,#97258,#97259,#97260,#97261),(#97262,#97263,
#97264,#97265,#97266)),.UNSPECIFIED.,.F.,.F.,.F.)
B_SPLINE_SURFACE_WITH_KNOTS((2,2),(3,2,3),(0.519229702920879,1.),(0.0365944846646469,
0.0384615384615384,0.0431859278884089),.UNSPECIFIED.)
GEOMETRIC_REPRESENTATION_ITEM()
RATIONAL_B_SPLINE_SURFACE(((0.999326490452283,0.99964606396823,1.,0.99910440092885,
0.998428822114389),(0.999326490452283,0.99964606396823,1.,0.99910440092885,
0.998428822114389)))
REPRESENTATION_ITEM('')
SURFACE()
);
#704=(
BOUNDED_SURFACE()
B_SPLINE_SURFACE(1,2,((#97322,#97323,#97324),(#97325,#97326,#97327)),
 .UNSPECIFIED.,.F.,.F.,.F.)
B_SPLINE_SURFACE_WITH_KNOTS((2,2),(3,3),(0.,1.),(0.0456081671210064,0.0575989447818616),
 .UNSPECIFIED.)
GEOMETRIC_REPRESENTATION_ITEM()
RATIONAL_B_SPLINE_SURFACE(((0.997793907739636,0.996365558499691,0.996354522974128),
(0.997793907739636,0.996365558499691,0.996354522974128)))
REPRESENTATION_ITEM('')
SURFACE()
);
#705=(
BOUNDED_SURFACE()
B_SPLINE_SURFACE(1,2,((#97362,#97363,#97364),(#97365,#97366,#97367)),
 .UNSPECIFIED.,.F.,.F.,.F.)
B_SPLINE_SURFACE_WITH_KNOTS((2,2),(3,3),(0.,1.),(0.0556006976522447,0.0675888855446172),
 .UNSPECIFIED.)
GEOMETRIC_REPRESENTATION_ITEM()
RATIONAL_B_SPLINE_SURFACE(((0.996397562408177,0.996150386836003,0.997319912821417),
(0.996397562408177,0.996150386836003,0.997319912821417)))
REPRESENTATION_ITEM('')
SURFACE()
);
#706=(
BOUNDED_SURFACE()
B_SPLINE_SURFACE(1,2,((#97368,#97369,#97370),(#97371,#97372,#97373)),
 .UNSPECIFIED.,.F.,.F.,.F.)
B_SPLINE_SURFACE_WITH_KNOTS((2,2),(3,3),(0.,1.),(0.0657448619281101,0.0758849574338232),
 .UNSPECIFIED.)
GEOMETRIC_REPRESENTATION_ITEM()
RATIONAL_B_SPLINE_SURFACE(((0.996993639757276,0.997798549146193,0.999617032345115),
(0.996993639757276,0.997798549146193,0.999617032345115)))
REPRESENTATION_ITEM('')
SURFACE()
);
#707=(
BOUNDED_SURFACE()
B_SPLINE_SURFACE(1,2,((#97448,#97449,#97450),(#97451,#97452,#97453)),
 .UNSPECIFIED.,.F.,.F.,.F.)
B_SPLINE_SURFACE_WITH_KNOTS((2,2),(3,3),(0.,1.),(0.00560769170938317,0.0176009697615924),
 .UNSPECIFIED.)
GEOMETRIC_REPRESENTATION_ITEM()
RATIONAL_B_SPLINE_SURFACE(((0.998183892106924,0.996573304252679,0.996380621268545),
(0.998183892106924,0.996573304252679,0.996380621268545)))
REPRESENTATION_ITEM('')
SURFACE()
);
#708=(
BOUNDED_SURFACE()
B_SPLINE_SURFACE(1,2,((#97538,#97539,#97540),(#97541,#97542,#97543)),
 .UNSPECIFIED.,.F.,.F.,.F.)
B_SPLINE_SURFACE_WITH_KNOTS((2,2),(3,3),(0.,1.),(0.0255903596132,0.0375948596691668),
 .UNSPECIFIED.)
GEOMETRIC_REPRESENTATION_ITEM()
RATIONAL_B_SPLINE_SURFACE(((0.996753121756002,0.997505687613138,0.999678813023773),
(0.996753121756002,0.997505687613138,0.999678813023773)))
REPRESENTATION_ITEM('')
SURFACE()
);
#709=(
BOUNDED_SURFACE()
B_SPLINE_SURFACE(1,2,((#97561,#97562,#97563,#97564,#97565),(#97566,#97567,
#97568,#97569,#97570)),.UNSPECIFIED.,.F.,.F.,.F.)
B_SPLINE_SURFACE_WITH_KNOTS((2,2),(3,2,3),(0.519229702923312,1.),(0.0365944846646546,
0.0384615384615384,0.0431859278884165),.UNSPECIFIED.)
GEOMETRIC_REPRESENTATION_ITEM()
RATIONAL_B_SPLINE_SURFACE(((0.999326490452285,0.999646063968232,1.,0.999104400928849,
0.998428822114386),(0.999326490452285,0.999646063968232,1.,0.999104400928849,
0.998428822114386)))
REPRESENTATION_ITEM('')
SURFACE()
);
#710=(
BOUNDED_SURFACE()
B_SPLINE_SURFACE(1,2,((#97626,#97627,#97628),(#97629,#97630,#97631)),
 .UNSPECIFIED.,.F.,.F.,.F.)
B_SPLINE_SURFACE_WITH_KNOTS((2,2),(3,3),(0.,1.),(0.0456081671210064,0.057598944781862),
 .UNSPECIFIED.)
GEOMETRIC_REPRESENTATION_ITEM()
RATIONAL_B_SPLINE_SURFACE(((0.997793907739636,0.996365558499691,0.996354522974128),
(0.997793907739636,0.996365558499691,0.996354522974128)))
REPRESENTATION_ITEM('')
SURFACE()
);
#711=(
BOUNDED_SURFACE()
B_SPLINE_SURFACE(1,2,((#97666,#97667,#97668),(#97669,#97670,#97671)),
 .UNSPECIFIED.,.F.,.F.,.F.)
B_SPLINE_SURFACE_WITH_KNOTS((2,2),(3,3),(0.,1.),(0.0556006976522457,0.0675888855446172),
 .UNSPECIFIED.)
GEOMETRIC_REPRESENTATION_ITEM()
RATIONAL_B_SPLINE_SURFACE(((0.996397562408177,0.996150386836003,0.997319912821417),
(0.996397562408177,0.996150386836003,0.997319912821417)))
REPRESENTATION_ITEM('')
SURFACE()
);
#712=(
BOUNDED_SURFACE()
B_SPLINE_SURFACE(1,2,((#97672,#97673,#97674),(#97675,#97676,#97677)),
 .UNSPECIFIED.,.F.,.F.,.F.)
B_SPLINE_SURFACE_WITH_KNOTS((2,2),(3,3),(0.,1.),(0.0657448619281102,0.0758849574338228),
 .UNSPECIFIED.)
GEOMETRIC_REPRESENTATION_ITEM()
RATIONAL_B_SPLINE_SURFACE(((0.996993639757276,0.997798549146193,0.999617032345115),
(0.996993639757276,0.997798549146193,0.999617032345115)))
REPRESENTATION_ITEM('')
SURFACE()
);
#713=(
BOUNDED_SURFACE()
B_SPLINE_SURFACE(1,2,((#97752,#97753,#97754),(#97755,#97756,#97757)),
 .UNSPECIFIED.,.F.,.F.,.F.)
B_SPLINE_SURFACE_WITH_KNOTS((2,2),(3,3),(0.,1.),(0.00560769170938325,0.0176009697615924),
 .UNSPECIFIED.)
GEOMETRIC_REPRESENTATION_ITEM()
RATIONAL_B_SPLINE_SURFACE(((0.998183892106924,0.996573304252679,0.996380621268545),
(0.998183892106924,0.996573304252679,0.996380621268545)))
REPRESENTATION_ITEM('')
SURFACE()
);
#714=(
BOUNDED_SURFACE()
B_SPLINE_SURFACE(1,2,((#97842,#97843,#97844),(#97845,#97846,#97847)),
 .UNSPECIFIED.,.F.,.F.,.F.)
B_SPLINE_SURFACE_WITH_KNOTS((2,2),(3,3),(0.,1.),(0.0255903596131989,0.0375948596691661),
 .UNSPECIFIED.)
GEOMETRIC_REPRESENTATION_ITEM()
RATIONAL_B_SPLINE_SURFACE(((0.996753121756001,0.997505687613137,0.999678813023773),
(0.996753121756001,0.997505687613137,0.999678813023773)))
REPRESENTATION_ITEM('')
SURFACE()
);
#715=(
BOUNDED_SURFACE()
B_SPLINE_SURFACE(1,2,((#97865,#97866,#97867,#97868,#97869),(#97870,#97871,
#97872,#97873,#97874)),.UNSPECIFIED.,.F.,.F.,.F.)
B_SPLINE_SURFACE_WITH_KNOTS((2,2),(3,2,3),(0.519229702925686,1.),(0.0365944846646577,
0.0384615384615384,0.0431859278884218),.UNSPECIFIED.)
GEOMETRIC_REPRESENTATION_ITEM()
RATIONAL_B_SPLINE_SURFACE(((0.999326490452286,0.999646063968232,1.,0.999104400928848,
0.998428822114385),(0.999326490452286,0.999646063968232,1.,0.999104400928848,
0.998428822114385)))
REPRESENTATION_ITEM('')
SURFACE()
);
#716=(
BOUNDED_SURFACE()
B_SPLINE_SURFACE(1,2,((#97930,#97931,#97932),(#97933,#97934,#97935)),
 .UNSPECIFIED.,.F.,.F.,.F.)
B_SPLINE_SURFACE_WITH_KNOTS((2,2),(3,3),(0.,1.),(0.0456081671210071,0.057598944781862),
 .UNSPECIFIED.)
GEOMETRIC_REPRESENTATION_ITEM()
RATIONAL_B_SPLINE_SURFACE(((0.997793907739636,0.996365558499691,0.996354522974128),
(0.997793907739636,0.996365558499691,0.996354522974128)))
REPRESENTATION_ITEM('')
SURFACE()
);
#717=(
BOUNDED_SURFACE()
B_SPLINE_SURFACE(1,2,((#97970,#97971,#97972),(#97973,#97974,#97975)),
 .UNSPECIFIED.,.F.,.F.,.F.)
B_SPLINE_SURFACE_WITH_KNOTS((2,2),(3,3),(0.,1.),(0.0556006976522457,0.0675888855446172),
 .UNSPECIFIED.)
GEOMETRIC_REPRESENTATION_ITEM()
RATIONAL_B_SPLINE_SURFACE(((0.996397562408177,0.996150386836003,0.997319912821417),
(0.996397562408177,0.996150386836003,0.997319912821417)))
REPRESENTATION_ITEM('')
SURFACE()
);
#718=(
BOUNDED_SURFACE()
B_SPLINE_SURFACE(1,2,((#97976,#97977,#97978),(#97979,#97980,#97981)),
 .UNSPECIFIED.,.F.,.F.,.F.)
B_SPLINE_SURFACE_WITH_KNOTS((2,2),(3,3),(0.,1.),(0.0657448619281102,0.0758849574338228),
 .UNSPECIFIED.)
GEOMETRIC_REPRESENTATION_ITEM()
RATIONAL_B_SPLINE_SURFACE(((0.996993639757276,0.997798549146193,0.999617032345115),
(0.996993639757276,0.997798549146193,0.999617032345115)))
REPRESENTATION_ITEM('')
SURFACE()
);
#719=(
BOUNDED_SURFACE()
B_SPLINE_SURFACE(1,2,((#98056,#98057,#98058),(#98059,#98060,#98061)),
 .UNSPECIFIED.,.F.,.F.,.F.)
B_SPLINE_SURFACE_WITH_KNOTS((2,2),(3,3),(0.,1.),(0.0056076917093843,0.0176009697615923),
 .UNSPECIFIED.)
GEOMETRIC_REPRESENTATION_ITEM()
RATIONAL_B_SPLINE_SURFACE(((0.998183892106924,0.996573304252679,0.996380621268545),
(0.998183892106924,0.996573304252679,0.996380621268545)))
REPRESENTATION_ITEM('')
SURFACE()
);
#720=(
BOUNDED_SURFACE()
B_SPLINE_SURFACE(1,2,((#98146,#98147,#98148),(#98149,#98150,#98151)),
 .UNSPECIFIED.,.F.,.F.,.F.)
B_SPLINE_SURFACE_WITH_KNOTS((2,2),(3,3),(0.,1.),(0.0255903596131988,0.037594859669166),
 .UNSPECIFIED.)
GEOMETRIC_REPRESENTATION_ITEM()
RATIONAL_B_SPLINE_SURFACE(((0.996753121756001,0.997505687613137,0.999678813023773),
(0.996753121756001,0.997505687613137,0.999678813023773)))
REPRESENTATION_ITEM('')
SURFACE()
);
#721=(
BOUNDED_SURFACE()
B_SPLINE_SURFACE(1,2,((#98169,#98170,#98171,#98172,#98173),(#98174,#98175,
#98176,#98177,#98178)),.UNSPECIFIED.,.F.,.F.,.F.)
B_SPLINE_SURFACE_WITH_KNOTS((2,2),(3,2,3),(0.519229702928186,1.),(0.0365944846646617,
0.0384615384615384,0.0431859276815302),.UNSPECIFIED.)
GEOMETRIC_REPRESENTATION_ITEM()
RATIONAL_B_SPLINE_SURFACE(((0.999326490452288,0.999646063968233,1.,0.999104400968069,
0.998428822173555),(0.999326490452288,0.999646063968233,1.,0.999104400968069,
0.998428822173555)))
REPRESENTATION_ITEM('')
SURFACE()
);
#722=(
BOUNDED_SURFACE()
B_SPLINE_SURFACE(1,2,((#98234,#98235,#98236),(#98237,#98238,#98239)),
 .UNSPECIFIED.,.F.,.F.,.F.)
B_SPLINE_SURFACE_WITH_KNOTS((2,2),(3,3),(0.,1.),(0.0456081671210064,0.0575989447818616),
 .UNSPECIFIED.)
GEOMETRIC_REPRESENTATION_ITEM()
RATIONAL_B_SPLINE_SURFACE(((0.997793907739636,0.996365558499691,0.996354522974128),
(0.997793907739636,0.996365558499691,0.996354522974128)))
REPRESENTATION_ITEM('')
SURFACE()
);
#723=(
BOUNDED_SURFACE()
B_SPLINE_SURFACE(1,2,((#98274,#98275,#98276),(#98277,#98278,#98279)),
 .UNSPECIFIED.,.F.,.F.,.F.)
B_SPLINE_SURFACE_WITH_KNOTS((2,2),(3,3),(0.,1.),(0.0556006976522447,0.0675888855446151),
 .UNSPECIFIED.)
GEOMETRIC_REPRESENTATION_ITEM()
RATIONAL_B_SPLINE_SURFACE(((0.996397562408177,0.996150386836003,0.997319912821417),
(0.996397562408177,0.996150386836003,0.997319912821417)))
REPRESENTATION_ITEM('')
SURFACE()
);
#724=(
BOUNDED_SURFACE()
B_SPLINE_SURFACE(1,2,((#98280,#98281,#98282),(#98283,#98284,#98285)),
 .UNSPECIFIED.,.F.,.F.,.F.)
B_SPLINE_SURFACE_WITH_KNOTS((2,2),(3,3),(0.,1.),(0.065744861928108,0.075884957433823),
 .UNSPECIFIED.)
GEOMETRIC_REPRESENTATION_ITEM()
RATIONAL_B_SPLINE_SURFACE(((0.996993639757276,0.997798549146192,0.999617032345115),
(0.996993639757276,0.997798549146192,0.999617032345115)))
REPRESENTATION_ITEM('')
SURFACE()
);
#725=(
BOUNDED_SURFACE()
B_SPLINE_SURFACE(1,2,((#98360,#98361,#98362),(#98363,#98364,#98365)),
 .UNSPECIFIED.,.F.,.F.,.F.)
B_SPLINE_SURFACE_WITH_KNOTS((2,2),(3,3),(0.,1.),(0.00560769170938324,0.017600969761593),
 .UNSPECIFIED.)
GEOMETRIC_REPRESENTATION_ITEM()
RATIONAL_B_SPLINE_SURFACE(((0.998183892106924,0.996573304252679,0.996380621268545),
(0.998183892106924,0.996573304252679,0.996380621268545)))
REPRESENTATION_ITEM('')
SURFACE()
);
#726=(
BOUNDED_SURFACE()
B_SPLINE_SURFACE(1,2,((#98450,#98451,#98452),(#98453,#98454,#98455)),
 .UNSPECIFIED.,.F.,.F.,.F.)
B_SPLINE_SURFACE_WITH_KNOTS((2,2),(3,3),(0.,1.),(0.0255903596132001,0.0375948596691658),
 .UNSPECIFIED.)
GEOMETRIC_REPRESENTATION_ITEM()
RATIONAL_B_SPLINE_SURFACE(((0.996753121756002,0.997505687613138,0.999678813023773),
(0.996753121756002,0.997505687613138,0.999678813023773)))
REPRESENTATION_ITEM('')
SURFACE()
);
#727=(
BOUNDED_SURFACE()
B_SPLINE_SURFACE(1,2,((#98473,#98474,#98475,#98476,#98477),(#98478,#98479,
#98480,#98481,#98482)),.UNSPECIFIED.,.F.,.F.,.F.)
B_SPLINE_SURFACE_WITH_KNOTS((2,2),(3,2,3),(0.519229702930507,1.),(0.0365944846646633,
0.0384615384615384,0.0431859278884275),.UNSPECIFIED.)
GEOMETRIC_REPRESENTATION_ITEM()
RATIONAL_B_SPLINE_SURFACE(((0.999326490452288,0.999646063968233,1.,0.999104400928847,
0.998428822114384),(0.999326490452288,0.999646063968233,1.,0.999104400928847,
0.998428822114384)))
REPRESENTATION_ITEM('')
SURFACE()
);
#728=(
BOUNDED_SURFACE()
B_SPLINE_SURFACE(1,2,((#98538,#98539,#98540),(#98541,#98542,#98543)),
 .UNSPECIFIED.,.F.,.F.,.F.)
B_SPLINE_SURFACE_WITH_KNOTS((2,2),(3,3),(0.,1.),(0.0456081671210063,0.0575989447818616),
 .UNSPECIFIED.)
GEOMETRIC_REPRESENTATION_ITEM()
RATIONAL_B_SPLINE_SURFACE(((0.997793907739636,0.996365558499691,0.996354522974128),
(0.997793907739636,0.996365558499691,0.996354522974128)))
REPRESENTATION_ITEM('')
SURFACE()
);
#729=(
BOUNDED_SURFACE()
B_SPLINE_SURFACE(1,2,((#98578,#98579,#98580),(#98581,#98582,#98583)),
 .UNSPECIFIED.,.F.,.F.,.F.)
B_SPLINE_SURFACE_WITH_KNOTS((2,2),(3,3),(0.,1.),(0.0556006976522446,0.0675888855446162),
 .UNSPECIFIED.)
GEOMETRIC_REPRESENTATION_ITEM()
RATIONAL_B_SPLINE_SURFACE(((0.996397562408177,0.996150386836003,0.997319912821417),
(0.996397562408177,0.996150386836003,0.997319912821417)))
REPRESENTATION_ITEM('')
SURFACE()
);
#730=(
BOUNDED_SURFACE()
B_SPLINE_SURFACE(1,2,((#98584,#98585,#98586),(#98587,#98588,#98589)),
 .UNSPECIFIED.,.F.,.F.,.F.)
B_SPLINE_SURFACE_WITH_KNOTS((2,2),(3,3),(0.,1.),(0.0657448619281091,0.0758849574338227),
 .UNSPECIFIED.)
GEOMETRIC_REPRESENTATION_ITEM()
RATIONAL_B_SPLINE_SURFACE(((0.996993639757276,0.997798549146192,0.999617032345115),
(0.996993639757276,0.997798549146192,0.999617032345115)))
REPRESENTATION_ITEM('')
SURFACE()
);
#731=(
BOUNDED_SURFACE()
B_SPLINE_SURFACE(1,2,((#98664,#98665,#98666),(#98667,#98668,#98669)),
 .UNSPECIFIED.,.F.,.F.,.F.)
B_SPLINE_SURFACE_WITH_KNOTS((2,2),(3,3),(0.,1.),(0.00560769170938338,0.0176009697615912),
 .UNSPECIFIED.)
GEOMETRIC_REPRESENTATION_ITEM()
RATIONAL_B_SPLINE_SURFACE(((0.998183892106924,0.996573304252679,0.996380621268545),
(0.998183892106924,0.996573304252679,0.996380621268545)))
REPRESENTATION_ITEM('')
SURFACE()
);
#732=(
BOUNDED_SURFACE()
B_SPLINE_SURFACE(1,2,((#98754,#98755,#98756),(#98757,#98758,#98759)),
 .UNSPECIFIED.,.F.,.F.,.F.)
B_SPLINE_SURFACE_WITH_KNOTS((2,2),(3,3),(0.,1.),(0.0255903596132001,0.037594859669166),
 .UNSPECIFIED.)
GEOMETRIC_REPRESENTATION_ITEM()
RATIONAL_B_SPLINE_SURFACE(((0.996753121756002,0.997505687613138,0.999678813023773),
(0.996753121756002,0.997505687613138,0.999678813023773)))
REPRESENTATION_ITEM('')
SURFACE()
);
#733=(
BOUNDED_SURFACE()
B_SPLINE_SURFACE(1,2,((#98777,#98778,#98779,#98780,#98781),(#98782,#98783,
#98784,#98785,#98786)),.UNSPECIFIED.,.F.,.F.,.F.)
B_SPLINE_SURFACE_WITH_KNOTS((2,2),(3,2,3),(0.519229702931999,1.),(0.0365944846646612,
0.0384615384615384,0.0431859278101874),.UNSPECIFIED.)
GEOMETRIC_REPRESENTATION_ITEM()
RATIONAL_B_SPLINE_SURFACE(((0.999326490452287,0.999646063968233,1.,0.999104400943679,
0.998428822136759),(0.999326490452287,0.999646063968233,1.,0.999104400943679,
0.998428822136759)))
REPRESENTATION_ITEM('')
SURFACE()
);
#734=(
BOUNDED_SURFACE()
B_SPLINE_SURFACE(1,2,((#98842,#98843,#98844),(#98845,#98846,#98847)),
 .UNSPECIFIED.,.F.,.F.,.F.)
B_SPLINE_SURFACE_WITH_KNOTS((2,2),(3,3),(0.,1.),(0.0456081671210053,0.0575989447818606),
 .UNSPECIFIED.)
GEOMETRIC_REPRESENTATION_ITEM()
RATIONAL_B_SPLINE_SURFACE(((0.997793907739636,0.996365558499691,0.996354522974128),
(0.997793907739636,0.996365558499691,0.996354522974128)))
REPRESENTATION_ITEM('')
SURFACE()
);
#735=(
BOUNDED_SURFACE()
B_SPLINE_SURFACE(1,2,((#98882,#98883,#98884),(#98885,#98886,#98887)),
 .UNSPECIFIED.,.F.,.F.,.F.)
B_SPLINE_SURFACE_WITH_KNOTS((2,2),(3,3),(0.,1.),(0.0556006976522437,0.0675888855446153),
 .UNSPECIFIED.)
GEOMETRIC_REPRESENTATION_ITEM()
RATIONAL_B_SPLINE_SURFACE(((0.996397562408177,0.996150386836003,0.997319912821417),
(0.996397562408177,0.996150386836003,0.997319912821417)))
REPRESENTATION_ITEM('')
SURFACE()
);
#736=(
BOUNDED_SURFACE()
B_SPLINE_SURFACE(1,2,((#98888,#98889,#98890),(#98891,#98892,#98893)),
 .UNSPECIFIED.,.F.,.F.,.F.)
B_SPLINE_SURFACE_WITH_KNOTS((2,2),(3,3),(0.,1.),(0.0657448619281082,0.0758849574338225),
 .UNSPECIFIED.)
GEOMETRIC_REPRESENTATION_ITEM()
RATIONAL_B_SPLINE_SURFACE(((0.996993639757276,0.997798549146192,0.999617032345115),
(0.996993639757276,0.997798549146192,0.999617032345115)))
REPRESENTATION_ITEM('')
SURFACE()
);
#737=(
BOUNDED_SURFACE()
B_SPLINE_SURFACE(1,2,((#98968,#98969,#98970),(#98971,#98972,#98973)),
 .UNSPECIFIED.,.F.,.F.,.F.)
B_SPLINE_SURFACE_WITH_KNOTS((2,2),(3,3),(0.,1.),(0.00560769170938422,0.0176009697615929),
 .UNSPECIFIED.)
GEOMETRIC_REPRESENTATION_ITEM()
RATIONAL_B_SPLINE_SURFACE(((0.998183892106924,0.996573304252679,0.996380621268545),
(0.998183892106924,0.996573304252679,0.996380621268545)))
REPRESENTATION_ITEM('')
SURFACE()
);
#738=(
BOUNDED_SURFACE()
B_SPLINE_SURFACE(1,2,((#99058,#99059,#99060),(#99061,#99062,#99063)),
 .UNSPECIFIED.,.F.,.F.,.F.)
B_SPLINE_SURFACE_WITH_KNOTS((2,2),(3,3),(0.,1.),(0.0255903596131999,0.037594859669168),
 .UNSPECIFIED.)
GEOMETRIC_REPRESENTATION_ITEM()
RATIONAL_B_SPLINE_SURFACE(((0.996753121756002,0.997505687613138,0.999678813023774),
(0.996753121756002,0.997505687613138,0.999678813023774)))
REPRESENTATION_ITEM('')
SURFACE()
);
#739=(
BOUNDED_SURFACE()
B_SPLINE_SURFACE(1,2,((#99081,#99082,#99083,#99084,#99085),(#99086,#99087,
#99088,#99089,#99090)),.UNSPECIFIED.,.F.,.F.,.F.)
B_SPLINE_SURFACE_WITH_KNOTS((2,2),(3,2,3),(0.519229702931916,1.),(0.0365944846646506,
0.0384615384615384,0.0431859276815304),.UNSPECIFIED.)
GEOMETRIC_REPRESENTATION_ITEM()
RATIONAL_B_SPLINE_SURFACE(((0.999326490452284,0.999646063968231,1.,0.999104400968068,
0.998428822173555),(0.999326490452284,0.999646063968231,1.,0.999104400968068,
0.998428822173555)))
REPRESENTATION_ITEM('')
SURFACE()
);
#740=(
BOUNDED_SURFACE()
B_SPLINE_SURFACE(1,2,((#99146,#99147,#99148),(#99149,#99150,#99151)),
 .UNSPECIFIED.,.F.,.F.,.F.)
B_SPLINE_SURFACE_WITH_KNOTS((2,2),(3,3),(0.,1.),(0.0456081671210071,0.057598944781862),
 .UNSPECIFIED.)
GEOMETRIC_REPRESENTATION_ITEM()
RATIONAL_B_SPLINE_SURFACE(((0.997793907739636,0.996365558499691,0.996354522974128),
(0.997793907739636,0.996365558499691,0.996354522974128)))
REPRESENTATION_ITEM('')
SURFACE()
);
#741=(
BOUNDED_SURFACE()
B_SPLINE_SURFACE(1,2,((#99186,#99187,#99188),(#99189,#99190,#99191)),
 .UNSPECIFIED.,.F.,.F.,.F.)
B_SPLINE_SURFACE_WITH_KNOTS((2,2),(3,3),(0.,1.),(0.0556006976522447,0.0675888855446163),
 .UNSPECIFIED.)
GEOMETRIC_REPRESENTATION_ITEM()
RATIONAL_B_SPLINE_SURFACE(((0.996397562408177,0.996150386836003,0.997319912821417),
(0.996397562408177,0.996150386836003,0.997319912821417)))
REPRESENTATION_ITEM('')
SURFACE()
);
#742=(
BOUNDED_SURFACE()
B_SPLINE_SURFACE(1,2,((#99192,#99193,#99194),(#99195,#99196,#99197)),
 .UNSPECIFIED.,.F.,.F.,.F.)
B_SPLINE_SURFACE_WITH_KNOTS((2,2),(3,3),(0.,1.),(0.0657450014656867,0.0758834225204695),
 .UNSPECIFIED.)
GEOMETRIC_REPRESENTATION_ITEM()
RATIONAL_B_SPLINE_SURFACE(((0.99699366191014,0.997798452328481,0.99961648183819),
(0.99699366191014,0.997798452328481,0.99961648183819)))
REPRESENTATION_ITEM('')
SURFACE()
);
#743=(
BOUNDED_SURFACE()
B_SPLINE_SURFACE(1,2,((#99272,#99273,#99274),(#99275,#99276,#99277)),
 .UNSPECIFIED.,.F.,.F.,.F.)
B_SPLINE_SURFACE_WITH_KNOTS((2,2),(3,3),(0.,1.),(0.0056076917093829,0.0176009697615918),
 .UNSPECIFIED.)
GEOMETRIC_REPRESENTATION_ITEM()
RATIONAL_B_SPLINE_SURFACE(((0.998183892106924,0.996573304252679,0.996380621268545),
(0.998183892106924,0.996573304252679,0.996380621268545)))
REPRESENTATION_ITEM('')
SURFACE()
);
#744=(
BOUNDED_SURFACE()
B_SPLINE_SURFACE(1,2,((#99362,#99363,#99364),(#99365,#99366,#99367)),
 .UNSPECIFIED.,.F.,.F.,.F.)
B_SPLINE_SURFACE_WITH_KNOTS((2,2),(3,3),(0.,1.),(0.0255903596131988,0.037594859669165),
 .UNSPECIFIED.)
GEOMETRIC_REPRESENTATION_ITEM()
RATIONAL_B_SPLINE_SURFACE(((0.996753121756001,0.997505687613137,0.999678813023773),
(0.996753121756001,0.997505687613137,0.999678813023773)))
REPRESENTATION_ITEM('')
SURFACE()
);
#745=(
BOUNDED_SURFACE()
B_SPLINE_SURFACE(1,2,((#99385,#99386,#99387,#99388,#99389),(#99390,#99391,
#99392,#99393,#99394)),.UNSPECIFIED.,.F.,.F.,.F.)
B_SPLINE_SURFACE_WITH_KNOTS((2,2),(3,2,3),(0.519229702931731,1.),(0.0365944846646451,
0.0384615384615384,0.0431859276815275),.UNSPECIFIED.)
GEOMETRIC_REPRESENTATION_ITEM()
RATIONAL_B_SPLINE_SURFACE(((0.999326490452282,0.99964606396823,1.,0.999104400968069,
0.998428822173556),(0.999326490452282,0.99964606396823,1.,0.999104400968069,
0.998428822173556)))
REPRESENTATION_ITEM('')
SURFACE()
);
#746=(
BOUNDED_SURFACE()
B_SPLINE_SURFACE(1,2,((#99450,#99451,#99452),(#99453,#99454,#99455)),
 .UNSPECIFIED.,.F.,.F.,.F.)
B_SPLINE_SURFACE_WITH_KNOTS((2,2),(3,3),(0.,1.),(0.0456081671210062,0.0575989447818616),
 .UNSPECIFIED.)
GEOMETRIC_REPRESENTATION_ITEM()
RATIONAL_B_SPLINE_SURFACE(((0.997793907739636,0.996365558499691,0.996354522974128),
(0.997793907739636,0.996365558499691,0.996354522974128)))
REPRESENTATION_ITEM('')
SURFACE()
);
#747=(
BOUNDED_SURFACE()
B_SPLINE_SURFACE(1,2,((#99490,#99491,#99492),(#99493,#99494,#99495)),
 .UNSPECIFIED.,.F.,.F.,.F.)
B_SPLINE_SURFACE_WITH_KNOTS((2,2),(3,3),(0.,1.),(0.0556006976522447,0.0675888855446162),
 .UNSPECIFIED.)
GEOMETRIC_REPRESENTATION_ITEM()
RATIONAL_B_SPLINE_SURFACE(((0.996397562408177,0.996150386836003,0.997319912821417),
(0.996397562408177,0.996150386836003,0.997319912821417)))
REPRESENTATION_ITEM('')
SURFACE()
);
#748=(
BOUNDED_SURFACE()
B_SPLINE_SURFACE(1,2,((#99496,#99497,#99498),(#99499,#99500,#99501)),
 .UNSPECIFIED.,.F.,.F.,.F.)
B_SPLINE_SURFACE_WITH_KNOTS((2,2),(3,3),(0.,1.),(0.0657448619281091,0.0758849574338226),
 .UNSPECIFIED.)
GEOMETRIC_REPRESENTATION_ITEM()
RATIONAL_B_SPLINE_SURFACE(((0.996993639757276,0.997798549146192,0.999617032345115),
(0.996993639757276,0.997798549146192,0.999617032345115)))
REPRESENTATION_ITEM('')
SURFACE()
);
#749=(
BOUNDED_SURFACE()
B_SPLINE_SURFACE(1,2,((#99576,#99577,#99578),(#99579,#99580,#99581)),
 .UNSPECIFIED.,.F.,.F.,.F.)
B_SPLINE_SURFACE_WITH_KNOTS((2,2),(3,3),(0.,1.),(0.00560769170938373,0.0176009697615924),
 .UNSPECIFIED.)
GEOMETRIC_REPRESENTATION_ITEM()
RATIONAL_B_SPLINE_SURFACE(((0.998183892106924,0.996573304252679,0.996380621268545),
(0.998183892106924,0.996573304252679,0.996380621268545)))
REPRESENTATION_ITEM('')
SURFACE()
);
#750=(
BOUNDED_SURFACE()
B_SPLINE_SURFACE(1,2,((#99666,#99667,#99668),(#99669,#99670,#99671)),
 .UNSPECIFIED.,.F.,.F.,.F.)
B_SPLINE_SURFACE_WITH_KNOTS((2,2),(3,3),(0.,1.),(0.0255903596132,0.037594859669166),
 .UNSPECIFIED.)
GEOMETRIC_REPRESENTATION_ITEM()
RATIONAL_B_SPLINE_SURFACE(((0.996753121756002,0.997505687613138,0.999678813023773),
(0.996753121756002,0.997505687613138,0.999678813023773)))
REPRESENTATION_ITEM('')
SURFACE()
);
#751=(
BOUNDED_SURFACE()
B_SPLINE_SURFACE(1,2,((#99689,#99690,#99691,#99692,#99693),(#99694,#99695,
#99696,#99697,#99698)),.UNSPECIFIED.,.F.,.F.,.F.)
B_SPLINE_SURFACE_WITH_KNOTS((2,2),(3,2,3),(0.519229702931711,1.),(0.036594484664649,
0.0384615384615384,0.043185927681521),.UNSPECIFIED.)
GEOMETRIC_REPRESENTATION_ITEM()
RATIONAL_B_SPLINE_SURFACE(((0.999326490452283,0.999646063968231,1.,0.99910440096807,
0.998428822173557),(0.999326490452283,0.999646063968231,1.,0.99910440096807,
0.998428822173557)))
REPRESENTATION_ITEM('')
SURFACE()
);
#752=(
BOUNDED_SURFACE()
B_SPLINE_SURFACE(1,2,((#99754,#99755,#99756),(#99757,#99758,#99759)),
 .UNSPECIFIED.,.F.,.F.,.F.)
B_SPLINE_SURFACE_WITH_KNOTS((2,2),(3,3),(0.,1.),(0.0456081671210063,0.0575989447818621),
 .UNSPECIFIED.)
GEOMETRIC_REPRESENTATION_ITEM()
RATIONAL_B_SPLINE_SURFACE(((0.997793907739636,0.996365558499691,0.996354522974128),
(0.997793907739636,0.996365558499691,0.996354522974128)))
REPRESENTATION_ITEM('')
SURFACE()
);
#753=(
BOUNDED_SURFACE()
B_SPLINE_SURFACE(1,2,((#99794,#99795,#99796),(#99797,#99798,#99799)),
 .UNSPECIFIED.,.F.,.F.,.F.)
B_SPLINE_SURFACE_WITH_KNOTS((2,2),(3,3),(0.,1.),(0.0556006976522445,0.0675888855446172),
 .UNSPECIFIED.)
GEOMETRIC_REPRESENTATION_ITEM()
RATIONAL_B_SPLINE_SURFACE(((0.996397562408177,0.996150386836003,0.997319912821417),
(0.996397562408177,0.996150386836003,0.997319912821417)))
REPRESENTATION_ITEM('')
SURFACE()
);
#754=(
BOUNDED_SURFACE()
B_SPLINE_SURFACE(1,2,((#99800,#99801,#99802),(#99803,#99804,#99805)),
 .UNSPECIFIED.,.F.,.F.,.F.)
B_SPLINE_SURFACE_WITH_KNOTS((2,2),(3,3),(0.,1.),(0.0657448619281102,0.0758849574338218),
 .UNSPECIFIED.)
GEOMETRIC_REPRESENTATION_ITEM()
RATIONAL_B_SPLINE_SURFACE(((0.996993639757276,0.997798549146192,0.999617032345114),
(0.996993639757276,0.997798549146192,0.999617032345114)))
REPRESENTATION_ITEM('')
SURFACE()
);
#755=(
BOUNDED_SURFACE()
B_SPLINE_SURFACE(1,2,((#99880,#99881,#99882),(#99883,#99884,#99885)),
 .UNSPECIFIED.,.F.,.F.,.F.)
B_SPLINE_SURFACE_WITH_KNOTS((2,2),(3,3),(0.,1.),(0.0056076917093831,0.017600969761593),
 .UNSPECIFIED.)
GEOMETRIC_REPRESENTATION_ITEM()
RATIONAL_B_SPLINE_SURFACE(((0.998183892106924,0.996573304252679,0.996380621268545),
(0.998183892106924,0.996573304252679,0.996380621268545)))
REPRESENTATION_ITEM('')
SURFACE()
);
#756=(
BOUNDED_SURFACE()
B_SPLINE_SURFACE(1,2,((#99970,#99971,#99972),(#99973,#99974,#99975)),
 .UNSPECIFIED.,.F.,.F.,.F.)
B_SPLINE_SURFACE_WITH_KNOTS((2,2),(3,3),(0.,1.),(0.025590359613201,0.0375948596691668),
 .UNSPECIFIED.)
GEOMETRIC_REPRESENTATION_ITEM()
RATIONAL_B_SPLINE_SURFACE(((0.996753121756002,0.997505687613138,0.999678813023773),
(0.996753121756002,0.997505687613138,0.999678813023773)))
REPRESENTATION_ITEM('')
SURFACE()
);
#757=(
BOUNDED_SURFACE()
B_SPLINE_SURFACE(1,2,((#99993,#99994,#99995,#99996,#99997),(#99998,#99999,
#100000,#100001,#100002)),.UNSPECIFIED.,.F.,.F.,.F.)
B_SPLINE_SURFACE_WITH_KNOTS((2,2),(3,2,3),(0.519229702931684,1.),(0.0365944846646416,
0.0384615384615384,0.0431859278884089),.UNSPECIFIED.)
GEOMETRIC_REPRESENTATION_ITEM()
RATIONAL_B_SPLINE_SURFACE(((0.999326490452281,0.999646063968229,1.,0.99910440092885,
0.998428822114388),(0.999326490452281,0.999646063968229,1.,0.99910440092885,
0.998428822114388)))
REPRESENTATION_ITEM('')
SURFACE()
);
#758=(
BOUNDED_SURFACE()
B_SPLINE_SURFACE(1,2,((#100058,#100059,#100060),(#100061,#100062,#100063)),
 .UNSPECIFIED.,.F.,.F.,.F.)
B_SPLINE_SURFACE_WITH_KNOTS((2,2),(3,3),(0.,1.),(0.0456081671210073,0.0575989447818615),
 .UNSPECIFIED.)
GEOMETRIC_REPRESENTATION_ITEM()
RATIONAL_B_SPLINE_SURFACE(((0.997793907739636,0.996365558499691,0.996354522974128),
(0.997793907739636,0.996365558499691,0.996354522974128)))
REPRESENTATION_ITEM('')
SURFACE()
);
#759=(
BOUNDED_SURFACE()
B_SPLINE_SURFACE(1,2,((#100098,#100099,#100100),(#100101,#100102,#100103)),
 .UNSPECIFIED.,.F.,.F.,.F.)
B_SPLINE_SURFACE_WITH_KNOTS((2,2),(3,3),(0.,1.),(0.0556006976522446,0.0675888855446172),
 .UNSPECIFIED.)
GEOMETRIC_REPRESENTATION_ITEM()
RATIONAL_B_SPLINE_SURFACE(((0.996397562408177,0.996150386836003,0.997319912821418),
(0.996397562408177,0.996150386836003,0.997319912821418)))
REPRESENTATION_ITEM('')
SURFACE()
);
#760=(
BOUNDED_SURFACE()
B_SPLINE_SURFACE(1,2,((#100104,#100105,#100106),(#100107,#100108,#100109)),
 .UNSPECIFIED.,.F.,.F.,.F.)
B_SPLINE_SURFACE_WITH_KNOTS((2,2),(3,3),(0.,1.),(0.0657448619281101,0.0758849574338219),
 .UNSPECIFIED.)
GEOMETRIC_REPRESENTATION_ITEM()
RATIONAL_B_SPLINE_SURFACE(((0.996993639757276,0.997798549146193,0.999617032345114),
(0.996993639757276,0.997798549146193,0.999617032345114)))
REPRESENTATION_ITEM('')
SURFACE()
);
#761=(
BOUNDED_SURFACE()
B_SPLINE_SURFACE(1,2,((#100184,#100185,#100186),(#100187,#100188,#100189)),
 .UNSPECIFIED.,.F.,.F.,.F.)
B_SPLINE_SURFACE_WITH_KNOTS((2,2),(3,3),(0.,1.),(0.00560769170938418,0.0176009697615923),
 .UNSPECIFIED.)
GEOMETRIC_REPRESENTATION_ITEM()
RATIONAL_B_SPLINE_SURFACE(((0.998183892106923,0.996573304252679,0.996380621268545),
(0.998183892106923,0.996573304252679,0.996380621268545)))
REPRESENTATION_ITEM('')
SURFACE()
);
#762=(
BOUNDED_SURFACE()
B_SPLINE_SURFACE(1,2,((#100274,#100275,#100276),(#100277,#100278,#100279)),
 .UNSPECIFIED.,.F.,.F.,.F.)
B_SPLINE_SURFACE_WITH_KNOTS((2,2),(3,3),(0.,1.),(0.025590359613201,0.0375948596691677),
 .UNSPECIFIED.)
GEOMETRIC_REPRESENTATION_ITEM()
RATIONAL_B_SPLINE_SURFACE(((0.996753121756002,0.997505687613138,0.999678813023774),
(0.996753121756002,0.997505687613138,0.999678813023774)))
REPRESENTATION_ITEM('')
SURFACE()
);
#763=(
BOUNDED_SURFACE()
B_SPLINE_SURFACE(1,2,((#100297,#100298,#100299,#100300,#100301),(#100302,
#100303,#100304,#100305,#100306)),.UNSPECIFIED.,.F.,.F.,.F.)
B_SPLINE_SURFACE_WITH_KNOTS((2,2),(3,2,3),(0.519229702931402,1.),(0.0365944846646318,
0.0384615384615384,0.0431859278884006),.UNSPECIFIED.)
GEOMETRIC_REPRESENTATION_ITEM()
RATIONAL_B_SPLINE_SURFACE(((0.999326490452278,0.999646063968227,1.,0.999104400928852,
0.998428822114391),(0.999326490452278,0.999646063968227,1.,0.999104400928852,
0.998428822114391)))
REPRESENTATION_ITEM('')
SURFACE()
);
#764=(
BOUNDED_SURFACE()
B_SPLINE_SURFACE(1,2,((#100362,#100363,#100364),(#100365,#100366,#100367)),
 .UNSPECIFIED.,.F.,.F.,.F.)
B_SPLINE_SURFACE_WITH_KNOTS((2,2),(3,3),(0.,1.),(0.045608167121007,0.0575989447818626),
 .UNSPECIFIED.)
GEOMETRIC_REPRESENTATION_ITEM()
RATIONAL_B_SPLINE_SURFACE(((0.997793907739636,0.996365558499691,0.996354522974128),
(0.997793907739636,0.996365558499691,0.996354522974128)))
REPRESENTATION_ITEM('')
SURFACE()
);
#765=(
BOUNDED_SURFACE()
B_SPLINE_SURFACE(1,2,((#100402,#100403,#100404),(#100405,#100406,#100407)),
 .UNSPECIFIED.,.F.,.F.,.F.)
B_SPLINE_SURFACE_WITH_KNOTS((2,2),(3,3),(0.,1.),(0.0556006976522468,0.0675888855446172),
 .UNSPECIFIED.)
GEOMETRIC_REPRESENTATION_ITEM()
RATIONAL_B_SPLINE_SURFACE(((0.996397562408177,0.996150386836004,0.997319912821418),
(0.996397562408177,0.996150386836004,0.997319912821418)))
REPRESENTATION_ITEM('')
SURFACE()
);
#766=(
BOUNDED_SURFACE()
B_SPLINE_SURFACE(1,2,((#100408,#100409,#100410),(#100411,#100412,#100413)),
 .UNSPECIFIED.,.F.,.F.,.F.)
B_SPLINE_SURFACE_WITH_KNOTS((2,2),(3,3),(0.,1.),(0.0657448619281104,0.075884957433822),
 .UNSPECIFIED.)
GEOMETRIC_REPRESENTATION_ITEM()
RATIONAL_B_SPLINE_SURFACE(((0.996993639757276,0.997798549146193,0.999617032345114),
(0.996993639757276,0.997798549146193,0.999617032345114)))
REPRESENTATION_ITEM('')
SURFACE()
);
#767=(
BOUNDED_SURFACE()
B_SPLINE_SURFACE(1,2,((#100488,#100489,#100490),(#100491,#100492,#100493)),
 .UNSPECIFIED.,.F.,.F.,.F.)
B_SPLINE_SURFACE_WITH_KNOTS((2,2),(3,3),(0.,1.),(0.00560769170938319,0.0176009697615929),
 .UNSPECIFIED.)
GEOMETRIC_REPRESENTATION_ITEM()
RATIONAL_B_SPLINE_SURFACE(((0.998183892106924,0.996573304252679,0.996380621268545),
(0.998183892106924,0.996573304252679,0.996380621268545)))
REPRESENTATION_ITEM('')
SURFACE()
);
#768=(
BOUNDED_SURFACE()
B_SPLINE_SURFACE(1,2,((#100578,#100579,#100580),(#100581,#100582,#100583)),
 .UNSPECIFIED.,.F.,.F.,.F.)
B_SPLINE_SURFACE_WITH_KNOTS((2,2),(3,3),(0.,1.),(0.0255903596132008,0.037594859669168),
 .UNSPECIFIED.)
GEOMETRIC_REPRESENTATION_ITEM()
RATIONAL_B_SPLINE_SURFACE(((0.996753121756002,0.997505687613138,0.999678813023774),
(0.996753121756002,0.997505687613138,0.999678813023774)))
REPRESENTATION_ITEM('')
SURFACE()
);
#769=(
BOUNDED_SURFACE()
B_SPLINE_SURFACE(1,2,((#100601,#100602,#100603,#100604,#100605),(#100606,
#100607,#100608,#100609,#100610)),.UNSPECIFIED.,.F.,.F.,.F.)
B_SPLINE_SURFACE_WITH_KNOTS((2,2),(3,2,3),(0.519229702931324,1.),(0.0365944846646224,
0.0384615384615384,0.0431859276814949),.UNSPECIFIED.)
GEOMETRIC_REPRESENTATION_ITEM()
RATIONAL_B_SPLINE_SURFACE(((0.999326490452275,0.999646063968226,1.,0.999104400968075,
0.998428822173566),(0.999326490452275,0.999646063968226,1.,0.999104400968075,
0.998428822173566)))
REPRESENTATION_ITEM('')
SURFACE()
);
#770=(
BOUNDED_SURFACE()
B_SPLINE_SURFACE(1,2,((#100666,#100667,#100668),(#100669,#100670,#100671)),
 .UNSPECIFIED.,.F.,.F.,.F.)
B_SPLINE_SURFACE_WITH_KNOTS((2,2),(3,3),(0.,1.),(0.0456081671210084,0.0575989447818613),
 .UNSPECIFIED.)
GEOMETRIC_REPRESENTATION_ITEM()
RATIONAL_B_SPLINE_SURFACE(((0.997793907739635,0.996365558499691,0.996354522974128),
(0.997793907739635,0.996365558499691,0.996354522974128)))
REPRESENTATION_ITEM('')
SURFACE()
);
#771=(
BOUNDED_SURFACE()
B_SPLINE_SURFACE(1,2,((#100706,#100707,#100708),(#100709,#100710,#100711)),
 .UNSPECIFIED.,.F.,.F.,.F.)
B_SPLINE_SURFACE_WITH_KNOTS((2,2),(3,3),(0.,1.),(0.0556006976522446,0.0675888855446172),
 .UNSPECIFIED.)
GEOMETRIC_REPRESENTATION_ITEM()
RATIONAL_B_SPLINE_SURFACE(((0.996397562408177,0.996150386836003,0.997319912821417),
(0.996397562408177,0.996150386836003,0.997319912821417)))
REPRESENTATION_ITEM('')
SURFACE()
);
#772=(
BOUNDED_SURFACE()
B_SPLINE_SURFACE(1,2,((#100712,#100713,#100714),(#100715,#100716,#100717)),
 .UNSPECIFIED.,.F.,.F.,.F.)
B_SPLINE_SURFACE_WITH_KNOTS((2,2),(3,3),(0.,1.),(0.0657448619281102,0.0758849574338218),
 .UNSPECIFIED.)
GEOMETRIC_REPRESENTATION_ITEM()
RATIONAL_B_SPLINE_SURFACE(((0.996993639757276,0.997798549146193,0.999617032345114),
(0.996993639757276,0.997798549146193,0.999617032345114)))
REPRESENTATION_ITEM('')
SURFACE()
);
#773=(
BOUNDED_SURFACE()
B_SPLINE_SURFACE(1,2,((#100792,#100793,#100794),(#100795,#100796,#100797)),
 .UNSPECIFIED.,.F.,.F.,.F.)
B_SPLINE_SURFACE_WITH_KNOTS((2,2),(3,3),(0.,1.),(0.00560769170938338,0.0176009697615918),
 .UNSPECIFIED.)
GEOMETRIC_REPRESENTATION_ITEM()
RATIONAL_B_SPLINE_SURFACE(((0.998183892106924,0.996573304252679,0.996380621268545),
(0.998183892106924,0.996573304252679,0.996380621268545)))
REPRESENTATION_ITEM('')
SURFACE()
);
#774=(
BOUNDED_SURFACE()
B_SPLINE_SURFACE(1,2,((#100882,#100883,#100884),(#100885,#100886,#100887)),
 .UNSPECIFIED.,.F.,.F.,.F.)
B_SPLINE_SURFACE_WITH_KNOTS((2,2),(3,3),(0.,1.),(0.0255903596131989,0.0375948596691661),
 .UNSPECIFIED.)
GEOMETRIC_REPRESENTATION_ITEM()
RATIONAL_B_SPLINE_SURFACE(((0.996753121756001,0.997505687613137,0.999678813023773),
(0.996753121756001,0.997505687613137,0.999678813023773)))
REPRESENTATION_ITEM('')
SURFACE()
);
#775=(
BOUNDED_SURFACE()
B_SPLINE_SURFACE(1,2,((#100905,#100906,#100907,#100908,#100909),(#100910,
#100911,#100912,#100913,#100914)),.UNSPECIFIED.,.F.,.F.,.F.)
B_SPLINE_SURFACE_WITH_KNOTS((2,2),(3,2,3),(0.519229702931156,1.),(0.0365944846646104,
0.0384615384615384,0.0431859278883797),.UNSPECIFIED.)
GEOMETRIC_REPRESENTATION_ITEM()
RATIONAL_B_SPLINE_SURFACE(((0.99932649045227,0.999646063968223,1.,0.999104400928856,
0.998428822114396),(0.99932649045227,0.999646063968223,1.,0.999104400928856,
0.998428822114396)))
REPRESENTATION_ITEM('')
SURFACE()
);
#776=(
BOUNDED_SURFACE()
B_SPLINE_SURFACE(1,2,((#100970,#100971,#100972),(#100973,#100974,#100975)),
 .UNSPECIFIED.,.F.,.F.,.F.)
B_SPLINE_SURFACE_WITH_KNOTS((2,2),(3,3),(0.,1.),(0.0456081671210071,0.0575989447818621),
 .UNSPECIFIED.)
GEOMETRIC_REPRESENTATION_ITEM()
RATIONAL_B_SPLINE_SURFACE(((0.997793907739635,0.996365558499691,0.996354522974128),
(0.997793907739635,0.996365558499691,0.996354522974128)))
REPRESENTATION_ITEM('')
SURFACE()
);
#777=(
BOUNDED_SURFACE()
B_SPLINE_SURFACE(1,2,((#101010,#101011,#101012),(#101013,#101014,#101015)),
 .UNSPECIFIED.,.F.,.F.,.F.)
B_SPLINE_SURFACE_WITH_KNOTS((2,2),(3,3),(0.,1.),(0.0556006976522457,0.0675888855446171),
 .UNSPECIFIED.)
GEOMETRIC_REPRESENTATION_ITEM()
RATIONAL_B_SPLINE_SURFACE(((0.996397562408177,0.996150386836003,0.997319912821417),
(0.996397562408177,0.996150386836003,0.997319912821417)))
REPRESENTATION_ITEM('')
SURFACE()
);
#778=(
BOUNDED_SURFACE()
B_SPLINE_SURFACE(1,2,((#101016,#101017,#101018),(#101019,#101020,#101021)),
 .UNSPECIFIED.,.F.,.F.,.F.)
B_SPLINE_SURFACE_WITH_KNOTS((2,2),(3,3),(0.,1.),(0.0657448619281101,0.0758849574338219),
 .UNSPECIFIED.)
GEOMETRIC_REPRESENTATION_ITEM()
RATIONAL_B_SPLINE_SURFACE(((0.996993639757276,0.997798549146193,0.999617032345114),
(0.996993639757276,0.997798549146193,0.999617032345114)))
REPRESENTATION_ITEM('')
SURFACE()
);
#779=(
BOUNDED_SURFACE()
B_SPLINE_SURFACE(1,2,((#101096,#101097,#101098),(#101099,#101100,#101101)),
 .UNSPECIFIED.,.F.,.F.,.F.)
B_SPLINE_SURFACE_WITH_KNOTS((2,2),(3,3),(0.,1.),(0.00560769170938345,0.0176009697615912),
 .UNSPECIFIED.)
GEOMETRIC_REPRESENTATION_ITEM()
RATIONAL_B_SPLINE_SURFACE(((0.998183892106924,0.996573304252679,0.996380621268545),
(0.998183892106924,0.996573304252679,0.996380621268545)))
REPRESENTATION_ITEM('')
SURFACE()
);
#780=(
BOUNDED_SURFACE()
B_SPLINE_SURFACE(1,2,((#101186,#101187,#101188),(#101189,#101190,#101191)),
 .UNSPECIFIED.,.F.,.F.,.F.)
B_SPLINE_SURFACE_WITH_KNOTS((2,2),(3,3),(0.,1.),(0.0255903596131981,0.0375948596691614),
 .UNSPECIFIED.)
GEOMETRIC_REPRESENTATION_ITEM()
RATIONAL_B_SPLINE_SURFACE(((0.996753121756001,0.997505687613137,0.999678813023771),
(0.996753121756001,0.997505687613137,0.999678813023771)))
REPRESENTATION_ITEM('')
SURFACE()
);
#781=(
BOUNDED_SURFACE()
B_SPLINE_SURFACE(1,2,((#101209,#101210,#101211,#101212,#101213),(#101214,
#101215,#101216,#101217,#101218)),.UNSPECIFIED.,.F.,.F.,.F.)
B_SPLINE_SURFACE_WITH_KNOTS((2,2),(3,2,3),(0.519229702931099,1.),(0.0365944846645983,
0.0384615384615384,0.0431859278883673),.UNSPECIFIED.)
GEOMETRIC_REPRESENTATION_ITEM()
RATIONAL_B_SPLINE_SURFACE(((0.999326490452266,0.999646063968221,1.,0.999104400928858,
0.998428822114401),(0.999326490452266,0.999646063968221,1.,0.999104400928858,
0.998428822114401)))
REPRESENTATION_ITEM('')
SURFACE()
);
#782=(
BOUNDED_SURFACE()
B_SPLINE_SURFACE(1,2,((#101274,#101275,#101276),(#101277,#101278,#101279)),
 .UNSPECIFIED.,.F.,.F.,.F.)
B_SPLINE_SURFACE_WITH_KNOTS((2,2),(3,3),(0.,1.),(0.0456081671210021,0.0575989447818602),
 .UNSPECIFIED.)
GEOMETRIC_REPRESENTATION_ITEM()
RATIONAL_B_SPLINE_SURFACE(((0.997793907739637,0.996365558499691,0.996354522974128),
(0.997793907739637,0.996365558499691,0.996354522974128)))
REPRESENTATION_ITEM('')
SURFACE()
);
#783=(
BOUNDED_SURFACE()
B_SPLINE_SURFACE(1,2,((#101314,#101315,#101316),(#101317,#101318,#101319)),
 .UNSPECIFIED.,.F.,.F.,.F.)
B_SPLINE_SURFACE_WITH_KNOTS((2,2),(3,3),(0.,1.),(0.0556006976522425,0.0675888855446155),
 .UNSPECIFIED.)
GEOMETRIC_REPRESENTATION_ITEM()
RATIONAL_B_SPLINE_SURFACE(((0.996397562408177,0.996150386836003,0.997319912821417),
(0.996397562408177,0.996150386836003,0.997319912821417)))
REPRESENTATION_ITEM('')
SURFACE()
);
#784=(
BOUNDED_SURFACE()
B_SPLINE_SURFACE(1,2,((#101320,#101321,#101322),(#101323,#101324,#101325)),
 .UNSPECIFIED.,.F.,.F.,.F.)
B_SPLINE_SURFACE_WITH_KNOTS((2,2),(3,3),(0.,1.),(0.0657448619281082,0.0758849574338231),
 .UNSPECIFIED.)
GEOMETRIC_REPRESENTATION_ITEM()
RATIONAL_B_SPLINE_SURFACE(((0.996993639757276,0.997798549146192,0.999617032345115),
(0.996993639757276,0.997798549146192,0.999617032345115)))
REPRESENTATION_ITEM('')
SURFACE()
);
#785=(
BOUNDED_SURFACE()
B_SPLINE_SURFACE(1,2,((#101400,#101401,#101402),(#101403,#101404,#101405)),
 .UNSPECIFIED.,.F.,.F.,.F.)
B_SPLINE_SURFACE_WITH_KNOTS((2,2),(3,3),(0.,1.),(0.00560769170938436,0.0176009697615923),
 .UNSPECIFIED.)
GEOMETRIC_REPRESENTATION_ITEM()
RATIONAL_B_SPLINE_SURFACE(((0.998183892106924,0.996573304252679,0.996380621268545),
(0.998183892106924,0.996573304252679,0.996380621268545)))
REPRESENTATION_ITEM('')
SURFACE()
);
#786=(
BOUNDED_SURFACE()
B_SPLINE_SURFACE(1,2,((#101490,#101491,#101492),(#101493,#101494,#101495)),
 .UNSPECIFIED.,.F.,.F.,.F.)
B_SPLINE_SURFACE_WITH_KNOTS((2,2),(3,3),(0.,1.),(0.0255903596131979,0.0375948596691638),
 .UNSPECIFIED.)
GEOMETRIC_REPRESENTATION_ITEM()
RATIONAL_B_SPLINE_SURFACE(((0.996753121756001,0.997505687613137,0.999678813023772),
(0.996753121756001,0.997505687613137,0.999678813023772)))
REPRESENTATION_ITEM('')
SURFACE()
);
#787=(
BOUNDED_SURFACE()
B_SPLINE_SURFACE(1,2,((#101513,#101514,#101515,#101516,#101517),(#101518,
#101519,#101520,#101521,#101522)),.UNSPECIFIED.,.F.,.F.,.F.)
B_SPLINE_SURFACE_WITH_KNOTS((2,2),(3,2,3),(0.519229702930943,1.),(0.0365944846645846,
0.0384615384615384,0.0431859276814578),.UNSPECIFIED.)
GEOMETRIC_REPRESENTATION_ITEM()
RATIONAL_B_SPLINE_SURFACE(((0.999326490452261,0.999646063968218,1.,0.999104400968082,
0.998428822173576),(0.999326490452261,0.999646063968218,1.,0.999104400968082,
0.998428822173576)))
REPRESENTATION_ITEM('')
SURFACE()
);
#788=(
BOUNDED_SURFACE()
B_SPLINE_SURFACE(1,2,((#101578,#101579,#101580),(#101581,#101582,#101583)),
 .UNSPECIFIED.,.F.,.F.,.F.)
B_SPLINE_SURFACE_WITH_KNOTS((2,2),(3,3),(0.,1.),(0.0456081671210052,0.0575989447818616),
 .UNSPECIFIED.)
GEOMETRIC_REPRESENTATION_ITEM()
RATIONAL_B_SPLINE_SURFACE(((0.997793907739636,0.996365558499691,0.996354522974128),
(0.997793907739636,0.996365558499691,0.996354522974128)))
REPRESENTATION_ITEM('')
SURFACE()
);
#789=(
BOUNDED_SURFACE()
B_SPLINE_SURFACE(1,2,((#101618,#101619,#101620),(#101621,#101622,#101623)),
 .UNSPECIFIED.,.F.,.F.,.F.)
B_SPLINE_SURFACE_WITH_KNOTS((2,2),(3,3),(0.,1.),(0.0556006976522446,0.0675888855446172),
 .UNSPECIFIED.)
GEOMETRIC_REPRESENTATION_ITEM()
RATIONAL_B_SPLINE_SURFACE(((0.996397562408177,0.996150386836003,0.997319912821417),
(0.996397562408177,0.996150386836003,0.997319912821417)))
REPRESENTATION_ITEM('')
SURFACE()
);
#790=(
BOUNDED_SURFACE()
B_SPLINE_SURFACE(1,2,((#101624,#101625,#101626),(#101627,#101628,#101629)),
 .UNSPECIFIED.,.F.,.F.,.F.)
B_SPLINE_SURFACE_WITH_KNOTS((2,2),(3,3),(0.,1.),(0.0657448619281102,0.0758849574338215),
 .UNSPECIFIED.)
GEOMETRIC_REPRESENTATION_ITEM()
RATIONAL_B_SPLINE_SURFACE(((0.996993639757276,0.997798549146193,0.999617032345114),
(0.996993639757276,0.997798549146193,0.999617032345114)))
REPRESENTATION_ITEM('')
SURFACE()
);
#791=(
BOUNDED_SURFACE()
B_SPLINE_SURFACE(1,2,((#101704,#101705,#101706),(#101707,#101708,#101709)),
 .UNSPECIFIED.,.F.,.F.,.F.)
B_SPLINE_SURFACE_WITH_KNOTS((2,2),(3,3),(0.,1.),(0.00560769170938512,0.0176009697615927),
 .UNSPECIFIED.)
GEOMETRIC_REPRESENTATION_ITEM()
RATIONAL_B_SPLINE_SURFACE(((0.998183892106923,0.996573304252679,0.996380621268545),
(0.998183892106923,0.996573304252679,0.996380621268545)))
REPRESENTATION_ITEM('')
SURFACE()
);
#792=(
BOUNDED_SURFACE()
B_SPLINE_SURFACE(1,2,((#101794,#101795,#101796),(#101797,#101798,#101799)),
 .UNSPECIFIED.,.F.,.F.,.F.)
B_SPLINE_SURFACE_WITH_KNOTS((2,2),(3,3),(0.,1.),(0.0255903596132013,0.0375948596691634),
 .UNSPECIFIED.)
GEOMETRIC_REPRESENTATION_ITEM()
RATIONAL_B_SPLINE_SURFACE(((0.996753121756002,0.997505687613138,0.999678813023772),
(0.996753121756002,0.997505687613138,0.999678813023772)))
REPRESENTATION_ITEM('')
SURFACE()
);
#793=(
BOUNDED_SURFACE()
B_SPLINE_SURFACE(1,2,((#101817,#101818,#101819,#101820,#101821),(#101822,
#101823,#101824,#101825,#101826)),.UNSPECIFIED.,.F.,.F.,.F.)
B_SPLINE_SURFACE_WITH_KNOTS((2,2),(3,2,3),(0.519229702930844,1.),(0.0365944846645699,
0.0384615384615384,0.0431859278883406),.UNSPECIFIED.)
GEOMETRIC_REPRESENTATION_ITEM()
RATIONAL_B_SPLINE_SURFACE(((0.999326490452256,0.999646063968215,1.,0.999104400928863,
0.998428822114408),(0.999326490452256,0.999646063968215,1.,0.999104400928863,
0.998428822114408)))
REPRESENTATION_ITEM('')
SURFACE()
);
#794=(
BOUNDED_SURFACE()
B_SPLINE_SURFACE(1,2,((#101882,#101883,#101884),(#101885,#101886,#101887)),
 .UNSPECIFIED.,.F.,.F.,.F.)
B_SPLINE_SURFACE_WITH_KNOTS((2,2),(3,3),(0.,1.),(0.0456081671210051,0.0575989447818622),
 .UNSPECIFIED.)
GEOMETRIC_REPRESENTATION_ITEM()
RATIONAL_B_SPLINE_SURFACE(((0.997793907739636,0.996365558499691,0.996354522974128),
(0.997793907739636,0.996365558499691,0.996354522974128)))
REPRESENTATION_ITEM('')
SURFACE()
);
#795=(
BOUNDED_SURFACE()
B_SPLINE_SURFACE(1,2,((#101922,#101923,#101924),(#101925,#101926,#101927)),
 .UNSPECIFIED.,.F.,.F.,.F.)
B_SPLINE_SURFACE_WITH_KNOTS((2,2),(3,3),(0.,1.),(0.0556006976522459,0.0675888855446171),
 .UNSPECIFIED.)
GEOMETRIC_REPRESENTATION_ITEM()
RATIONAL_B_SPLINE_SURFACE(((0.996397562408177,0.996150386836003,0.997319912821417),
(0.996397562408177,0.996150386836003,0.997319912821417)))
REPRESENTATION_ITEM('')
SURFACE()
);
#796=(
BOUNDED_SURFACE()
B_SPLINE_SURFACE(1,2,((#101928,#101929,#101930),(#101931,#101932,#101933)),
 .UNSPECIFIED.,.F.,.F.,.F.)
B_SPLINE_SURFACE_WITH_KNOTS((2,2),(3,3),(0.,1.),(0.0657448619281102,0.0758849574338221),
 .UNSPECIFIED.)
GEOMETRIC_REPRESENTATION_ITEM()
RATIONAL_B_SPLINE_SURFACE(((0.996993639757276,0.997798549146193,0.999617032345114),
(0.996993639757276,0.997798549146193,0.999617032345114)))
REPRESENTATION_ITEM('')
SURFACE()
);
#797=(
BOUNDED_SURFACE()
B_SPLINE_SURFACE(1,2,((#102008,#102009,#102010),(#102011,#102012,#102013)),
 .UNSPECIFIED.,.F.,.F.,.F.)
B_SPLINE_SURFACE_WITH_KNOTS((2,2),(3,3),(0.,1.),(0.00560769170938337,0.0176009697615918),
 .UNSPECIFIED.)
GEOMETRIC_REPRESENTATION_ITEM()
RATIONAL_B_SPLINE_SURFACE(((0.998183892106924,0.996573304252679,0.996380621268545),
(0.998183892106924,0.996573304252679,0.996380621268545)))
REPRESENTATION_ITEM('')
SURFACE()
);
#798=(
BOUNDED_SURFACE()
B_SPLINE_SURFACE(1,2,((#102098,#102099,#102100),(#102101,#102102,#102103)),
 .UNSPECIFIED.,.F.,.F.,.F.)
B_SPLINE_SURFACE_WITH_KNOTS((2,2),(3,3),(0.,1.),(0.0255903596132021,0.0375948596691676),
 .UNSPECIFIED.)
GEOMETRIC_REPRESENTATION_ITEM()
RATIONAL_B_SPLINE_SURFACE(((0.996753121756002,0.997505687613138,0.999678813023774),
(0.996753121756002,0.997505687613138,0.999678813023774)))
REPRESENTATION_ITEM('')
SURFACE()
);
#799=(
BOUNDED_SURFACE()
B_SPLINE_SURFACE(1,2,((#102121,#102122,#102123,#102124,#102125),(#102126,
#102127,#102128,#102129,#102130)),.UNSPECIFIED.,.F.,.F.,.F.)
B_SPLINE_SURFACE_WITH_KNOTS((2,2),(3,2,3),(0.519229702930734,1.),(0.0365944846645561,
0.0384615384615384,0.0431859278883255),.UNSPECIFIED.)
GEOMETRIC_REPRESENTATION_ITEM()
RATIONAL_B_SPLINE_SURFACE(((0.999326490452252,0.999646063968213,1.,0.999104400928866,
0.998428822114412),(0.999326490452252,0.999646063968213,1.,0.999104400928866,
0.998428822114412)))
REPRESENTATION_ITEM('')
SURFACE()
);
#800=(
BOUNDED_SURFACE()
B_SPLINE_SURFACE(1,2,((#102186,#102187,#102188),(#102189,#102190,#102191)),
 .UNSPECIFIED.,.F.,.F.,.F.)
B_SPLINE_SURFACE_WITH_KNOTS((2,2),(3,3),(0.,1.),(0.0456081671210071,0.0575989447818615),
 .UNSPECIFIED.)
GEOMETRIC_REPRESENTATION_ITEM()
RATIONAL_B_SPLINE_SURFACE(((0.997793907739636,0.996365558499691,0.996354522974128),
(0.997793907739636,0.996365558499691,0.996354522974128)))
REPRESENTATION_ITEM('')
SURFACE()
);
#801=(
BOUNDED_SURFACE()
B_SPLINE_SURFACE(1,2,((#102226,#102227,#102228),(#102229,#102230,#102231)),
 .UNSPECIFIED.,.F.,.F.,.F.)
B_SPLINE_SURFACE_WITH_KNOTS((2,2),(3,3),(0.,1.),(0.0556006976522447,0.0675888855446152),
 .UNSPECIFIED.)
GEOMETRIC_REPRESENTATION_ITEM()
RATIONAL_B_SPLINE_SURFACE(((0.996397562408177,0.996150386836003,0.997319912821417),
(0.996397562408177,0.996150386836003,0.997319912821417)))
REPRESENTATION_ITEM('')
SURFACE()
);
#802=(
BOUNDED_SURFACE()
B_SPLINE_SURFACE(1,2,((#102232,#102233,#102234),(#102235,#102236,#102237)),
 .UNSPECIFIED.,.F.,.F.,.F.)
B_SPLINE_SURFACE_WITH_KNOTS((2,2),(3,3),(0.,1.),(0.0657448619281081,0.0758849574338218),
 .UNSPECIFIED.)
GEOMETRIC_REPRESENTATION_ITEM()
RATIONAL_B_SPLINE_SURFACE(((0.996993639757276,0.997798549146192,0.999617032345114),
(0.996993639757276,0.997798549146192,0.999617032345114)))
REPRESENTATION_ITEM('')
SURFACE()
);
#803=(
BOUNDED_SURFACE()
B_SPLINE_SURFACE(1,2,((#102312,#102313,#102314),(#102315,#102316,#102317)),
 .UNSPECIFIED.,.F.,.F.,.F.)
B_SPLINE_SURFACE_WITH_KNOTS((2,2),(3,3),(0.,1.),(0.00560769170938437,0.0176009697615918),
 .UNSPECIFIED.)
GEOMETRIC_REPRESENTATION_ITEM()
RATIONAL_B_SPLINE_SURFACE(((0.998183892106924,0.996573304252679,0.996380621268545),
(0.998183892106924,0.996573304252679,0.996380621268545)))
REPRESENTATION_ITEM('')
SURFACE()
);
#804=(
BOUNDED_SURFACE()
B_SPLINE_SURFACE(1,2,((#102402,#102403,#102404),(#102405,#102406,#102407)),
 .UNSPECIFIED.,.F.,.F.,.F.)
B_SPLINE_SURFACE_WITH_KNOTS((2,2),(3,3),(0.,1.),(0.0255903596132008,0.0375948596691702),
 .UNSPECIFIED.)
GEOMETRIC_REPRESENTATION_ITEM()
RATIONAL_B_SPLINE_SURFACE(((0.996753121756002,0.997505687613138,0.999678813023775),
(0.996753121756002,0.997505687613138,0.999678813023775)))
REPRESENTATION_ITEM('')
SURFACE()
);
#805=(
BOUNDED_SURFACE()
B_SPLINE_SURFACE(1,2,((#102425,#102426,#102427,#102428,#102429),(#102430,
#102431,#102432,#102433,#102434)),.UNSPECIFIED.,.F.,.F.,.F.)
B_SPLINE_SURFACE_WITH_KNOTS((2,2),(3,2,3),(0.519229702930626,1.),(0.0365944846645412,
0.0384615384615384,0.0431859276814168),.UNSPECIFIED.)
GEOMETRIC_REPRESENTATION_ITEM()
RATIONAL_B_SPLINE_SURFACE(((0.999326490452246,0.99964606396821,1.,0.99910440096809,
0.998428822173588),(0.999326490452246,0.99964606396821,1.,0.99910440096809,
0.998428822173588)))
REPRESENTATION_ITEM('')
SURFACE()
);
#806=(
BOUNDED_SURFACE()
B_SPLINE_SURFACE(1,2,((#102490,#102491,#102492),(#102493,#102494,#102495)),
 .UNSPECIFIED.,.F.,.F.,.F.)
B_SPLINE_SURFACE_WITH_KNOTS((2,2),(3,3),(0.,1.),(0.0456081671210094,0.0575989447818618),
 .UNSPECIFIED.)
GEOMETRIC_REPRESENTATION_ITEM()
RATIONAL_B_SPLINE_SURFACE(((0.997793907739635,0.996365558499691,0.996354522974128),
(0.997793907739635,0.996365558499691,0.996354522974128)))
REPRESENTATION_ITEM('')
SURFACE()
);
#807=(
BOUNDED_SURFACE()
B_SPLINE_SURFACE(1,2,((#102530,#102531,#102532),(#102533,#102534,#102535)),
 .UNSPECIFIED.,.F.,.F.,.F.)
B_SPLINE_SURFACE_WITH_KNOTS((2,2),(3,3),(0.,1.),(0.0556006976522449,0.0675888855446151),
 .UNSPECIFIED.)
GEOMETRIC_REPRESENTATION_ITEM()
RATIONAL_B_SPLINE_SURFACE(((0.996397562408177,0.996150386836003,0.997319912821417),
(0.996397562408177,0.996150386836003,0.997319912821417)))
REPRESENTATION_ITEM('')
SURFACE()
);
#808=(
BOUNDED_SURFACE()
B_SPLINE_SURFACE(1,2,((#102536,#102537,#102538),(#102539,#102540,#102541)),
 .UNSPECIFIED.,.F.,.F.,.F.)
B_SPLINE_SURFACE_WITH_KNOTS((2,2),(3,3),(0.,1.),(0.0657448619281081,0.0758849574338224),
 .UNSPECIFIED.)
GEOMETRIC_REPRESENTATION_ITEM()
RATIONAL_B_SPLINE_SURFACE(((0.996993639757276,0.997798549146192,0.999617032345114),
(0.996993639757276,0.997798549146192,0.999617032345114)))
REPRESENTATION_ITEM('')
SURFACE()
);
#809=(
BOUNDED_SURFACE()
B_SPLINE_SURFACE(1,2,((#102616,#102617,#102618),(#102619,#102620,#102621)),
 .UNSPECIFIED.,.F.,.F.,.F.)
B_SPLINE_SURFACE_WITH_KNOTS((2,2),(3,3),(0.,1.),(0.00560769170938164,0.0176009697615925),
 .UNSPECIFIED.)
GEOMETRIC_REPRESENTATION_ITEM()
RATIONAL_B_SPLINE_SURFACE(((0.998183892106924,0.996573304252679,0.996380621268545),
(0.998183892106924,0.996573304252679,0.996380621268545)))
REPRESENTATION_ITEM('')
SURFACE()
);
#810=(
BOUNDED_SURFACE()
B_SPLINE_SURFACE(1,2,((#102706,#102707,#102708),(#102709,#102710,#102711)),
 .UNSPECIFIED.,.F.,.F.,.F.)
B_SPLINE_SURFACE_WITH_KNOTS((2,2),(3,3),(0.,1.),(0.0255903596131988,0.0375948596691661),
 .UNSPECIFIED.)
GEOMETRIC_REPRESENTATION_ITEM()
RATIONAL_B_SPLINE_SURFACE(((0.996753121756001,0.997505687613137,0.999678813023773),
(0.996753121756001,0.997505687613137,0.999678813023773)))
REPRESENTATION_ITEM('')
SURFACE()
);
#811=(
BOUNDED_SURFACE()
B_SPLINE_SURFACE(1,2,((#102729,#102730,#102731,#102732,#102733),(#102734,
#102735,#102736,#102737,#102738)),.UNSPECIFIED.,.F.,.F.,.F.)
B_SPLINE_SURFACE_WITH_KNOTS((2,2),(3,2,3),(0.519229702930531,1.),(0.0365944846645262,
0.0384615384615384,0.0431859278100564),.UNSPECIFIED.)
GEOMETRIC_REPRESENTATION_ITEM()
RATIONAL_B_SPLINE_SURFACE(((0.999326490452241,0.999646063968207,1.,0.999104400943704,
0.998428822136797),(0.999326490452241,0.999646063968207,1.,0.999104400943704,
0.998428822136797)))
REPRESENTATION_ITEM('')
SURFACE()
);
#812=(
BOUNDED_SURFACE()
B_SPLINE_SURFACE(1,2,((#102794,#102795,#102796),(#102797,#102798,#102799)),
 .UNSPECIFIED.,.F.,.F.,.F.)
B_SPLINE_SURFACE_WITH_KNOTS((2,2),(3,3),(0.,1.),(0.0456081671210071,0.0575989447818625),
 .UNSPECIFIED.)
GEOMETRIC_REPRESENTATION_ITEM()
RATIONAL_B_SPLINE_SURFACE(((0.997793907739635,0.99636555849969,0.996354522974128),
(0.997793907739635,0.99636555849969,0.996354522974128)))
REPRESENTATION_ITEM('')
SURFACE()
);
#813=(
BOUNDED_SURFACE()
B_SPLINE_SURFACE(1,2,((#102834,#102835,#102836),(#102837,#102838,#102839)),
 .UNSPECIFIED.,.F.,.F.,.F.)
B_SPLINE_SURFACE_WITH_KNOTS((2,2),(3,3),(0.,1.),(0.0556006976522469,0.067588885544616),
 .UNSPECIFIED.)
GEOMETRIC_REPRESENTATION_ITEM()
RATIONAL_B_SPLINE_SURFACE(((0.996397562408177,0.996150386836004,0.997319912821417),
(0.996397562408177,0.996150386836004,0.997319912821417)))
REPRESENTATION_ITEM('')
SURFACE()
);
#814=(
BOUNDED_SURFACE()
B_SPLINE_SURFACE(1,2,((#102840,#102841,#102842),(#102843,#102844,#102845)),
 .UNSPECIFIED.,.F.,.F.,.F.)
B_SPLINE_SURFACE_WITH_KNOTS((2,2),(3,3),(0.,1.),(0.0657448619281091,0.0758849574338235),
 .UNSPECIFIED.)
GEOMETRIC_REPRESENTATION_ITEM()
RATIONAL_B_SPLINE_SURFACE(((0.996993639757276,0.997798549146192,0.999617032345115),
(0.996993639757276,0.997798549146192,0.999617032345115)))
REPRESENTATION_ITEM('')
SURFACE()
);
#815=(
BOUNDED_SURFACE()
B_SPLINE_SURFACE(1,2,((#102920,#102921,#102922),(#102923,#102924,#102925)),
 .UNSPECIFIED.,.F.,.F.,.F.)
B_SPLINE_SURFACE_WITH_KNOTS((2,2),(3,3),(0.,1.),(0.00560769170938326,0.0176009697615917),
 .UNSPECIFIED.)
GEOMETRIC_REPRESENTATION_ITEM()
RATIONAL_B_SPLINE_SURFACE(((0.998183892106924,0.996573304252679,0.996380621268545),
(0.998183892106924,0.996573304252679,0.996380621268545)))
REPRESENTATION_ITEM('')
SURFACE()
);
#816=(
BOUNDED_SURFACE()
B_SPLINE_SURFACE(1,2,((#103010,#103011,#103012),(#103013,#103014,#103015)),
 .UNSPECIFIED.,.F.,.F.,.F.)
B_SPLINE_SURFACE_WITH_KNOTS((2,2),(3,3),(0.,1.),(0.0255903596132,0.0375948596691658),
 .UNSPECIFIED.)
GEOMETRIC_REPRESENTATION_ITEM()
RATIONAL_B_SPLINE_SURFACE(((0.996753121756002,0.997505687613138,0.999678813023773),
(0.996753121756002,0.997505687613138,0.999678813023773)))
REPRESENTATION_ITEM('')
SURFACE()
);
#817=(
BOUNDED_SURFACE()
B_SPLINE_SURFACE(1,2,((#103033,#103034,#103035,#103036,#103037),(#103038,
#103039,#103040,#103041,#103042)),.UNSPECIFIED.,.F.,.F.,.F.)
B_SPLINE_SURFACE_WITH_KNOTS((2,2),(3,2,3),(0.519229702930332,1.),(0.0365944846645122,
0.0384615384615384,0.0431859278882811),.UNSPECIFIED.)
GEOMETRIC_REPRESENTATION_ITEM()
RATIONAL_B_SPLINE_SURFACE(((0.999326490452237,0.999646063968205,1.,0.999104400928875,
0.998428822114426),(0.999326490452237,0.999646063968205,1.,0.999104400928875,
0.998428822114426)))
REPRESENTATION_ITEM('')
SURFACE()
);
#818=(
BOUNDED_SURFACE()
B_SPLINE_SURFACE(1,2,((#103098,#103099,#103100),(#103101,#103102,#103103)),
 .UNSPECIFIED.,.F.,.F.,.F.)
B_SPLINE_SURFACE_WITH_KNOTS((2,2),(3,3),(0.,1.),(0.0456081671210064,0.0575989447818616),
 .UNSPECIFIED.)
GEOMETRIC_REPRESENTATION_ITEM()
RATIONAL_B_SPLINE_SURFACE(((0.997793907739636,0.996365558499691,0.996354522974128),
(0.997793907739636,0.996365558499691,0.996354522974128)))
REPRESENTATION_ITEM('')
SURFACE()
);
#819=(
BOUNDED_SURFACE()
B_SPLINE_SURFACE(1,2,((#103138,#103139,#103140),(#103141,#103142,#103143)),
 .UNSPECIFIED.,.F.,.F.,.F.)
B_SPLINE_SURFACE_WITH_KNOTS((2,2),(3,3),(0.,1.),(0.0556006976522446,0.067588885544616),
 .UNSPECIFIED.)
GEOMETRIC_REPRESENTATION_ITEM()
RATIONAL_B_SPLINE_SURFACE(((0.996397562408177,0.996150386836003,0.997319912821417),
(0.996397562408177,0.996150386836003,0.997319912821417)))
REPRESENTATION_ITEM('')
SURFACE()
);
#820=(
BOUNDED_SURFACE()
B_SPLINE_SURFACE(1,2,((#103144,#103145,#103146),(#103147,#103148,#103149)),
 .UNSPECIFIED.,.F.,.F.,.F.)
B_SPLINE_SURFACE_WITH_KNOTS((2,2),(3,3),(0.,1.),(0.0657448619281089,0.0758849574338229),
 .UNSPECIFIED.)
GEOMETRIC_REPRESENTATION_ITEM()
RATIONAL_B_SPLINE_SURFACE(((0.996993639757276,0.997798549146192,0.999617032345115),
(0.996993639757276,0.997798549146192,0.999617032345115)))
REPRESENTATION_ITEM('')
SURFACE()
);
#821=(
BOUNDED_SURFACE()
B_SPLINE_SURFACE(1,2,((#103224,#103225,#103226),(#103227,#103228,#103229)),
 .UNSPECIFIED.,.F.,.F.,.F.)
B_SPLINE_SURFACE_WITH_KNOTS((2,2),(3,3),(0.,1.),(0.005607691709382,0.0176009697615936),
 .UNSPECIFIED.)
GEOMETRIC_REPRESENTATION_ITEM()
RATIONAL_B_SPLINE_SURFACE(((0.998183892106924,0.996573304252679,0.996380621268545),
(0.998183892106924,0.996573304252679,0.996380621268545)))
REPRESENTATION_ITEM('')
SURFACE()
);
#822=(
BOUNDED_SURFACE()
B_SPLINE_SURFACE(1,2,((#103314,#103315,#103316),(#103317,#103318,#103319)),
 .UNSPECIFIED.,.F.,.F.,.F.)
B_SPLINE_SURFACE_WITH_KNOTS((2,2),(3,3),(0.,1.),(0.0255903596132,0.037594859669166),
 .UNSPECIFIED.)
GEOMETRIC_REPRESENTATION_ITEM()
RATIONAL_B_SPLINE_SURFACE(((0.996753121756002,0.997505687613138,0.999678813023773),
(0.996753121756002,0.997505687613138,0.999678813023773)))
REPRESENTATION_ITEM('')
SURFACE()
);
#823=(
BOUNDED_SURFACE()
B_SPLINE_SURFACE(1,2,((#103337,#103338,#103339,#103340,#103341),(#103342,
#103343,#103344,#103345,#103346)),.UNSPECIFIED.,.F.,.F.,.F.)
B_SPLINE_SURFACE_WITH_KNOTS((2,2),(3,2,3),(0.519229702930221,1.),(0.0365944846644977,
0.0384615384615384,0.0431859278882677),.UNSPECIFIED.)
GEOMETRIC_REPRESENTATION_ITEM()
RATIONAL_B_SPLINE_SURFACE(((0.999326490452232,0.999646063968202,1.,0.999104400928877,
0.998428822114429),(0.999326490452232,0.999646063968202,1.,0.999104400928877,
0.998428822114429)))
REPRESENTATION_ITEM('')
SURFACE()
);
#824=(
BOUNDED_SURFACE()
B_SPLINE_SURFACE(1,2,((#103402,#103403,#103404),(#103405,#103406,#103407)),
 .UNSPECIFIED.,.F.,.F.,.F.)
B_SPLINE_SURFACE_WITH_KNOTS((2,2),(3,3),(0.,1.),(0.0456081671210053,0.0575989447818605),
 .UNSPECIFIED.)
GEOMETRIC_REPRESENTATION_ITEM()
RATIONAL_B_SPLINE_SURFACE(((0.997793907739636,0.996365558499691,0.996354522974128),
(0.997793907739636,0.996365558499691,0.996354522974128)))
REPRESENTATION_ITEM('')
SURFACE()
);
#825=(
BOUNDED_SURFACE()
B_SPLINE_SURFACE(1,2,((#103442,#103443,#103444),(#103445,#103446,#103447)),
 .UNSPECIFIED.,.F.,.F.,.F.)
B_SPLINE_SURFACE_WITH_KNOTS((2,2),(3,3),(0.,1.),(0.0556006976522437,0.0675888855446152),
 .UNSPECIFIED.)
GEOMETRIC_REPRESENTATION_ITEM()
RATIONAL_B_SPLINE_SURFACE(((0.996397562408177,0.996150386836003,0.997319912821417),
(0.996397562408177,0.996150386836003,0.997319912821417)))
REPRESENTATION_ITEM('')
SURFACE()
);
#826=(
BOUNDED_SURFACE()
B_SPLINE_SURFACE(1,2,((#103448,#103449,#103450),(#103451,#103452,#103453)),
 .UNSPECIFIED.,.F.,.F.,.F.)
B_SPLINE_SURFACE_WITH_KNOTS((2,2),(3,3),(0.,1.),(0.065744861928108,0.0758849574338232),
 .UNSPECIFIED.)
GEOMETRIC_REPRESENTATION_ITEM()
RATIONAL_B_SPLINE_SURFACE(((0.996993639757276,0.997798549146192,0.999617032345115),
(0.996993639757276,0.997798549146192,0.999617032345115)))
REPRESENTATION_ITEM('')
SURFACE()
);
#827=(
BOUNDED_SURFACE()
B_SPLINE_SURFACE(1,2,((#103528,#103529,#103530),(#103531,#103532,#103533)),
 .UNSPECIFIED.,.F.,.F.,.F.)
B_SPLINE_SURFACE_WITH_KNOTS((2,2),(3,3),(0.,1.),(0.00560769170938538,0.0176009697615917),
 .UNSPECIFIED.)
GEOMETRIC_REPRESENTATION_ITEM()
RATIONAL_B_SPLINE_SURFACE(((0.998183892106923,0.996573304252679,0.996380621268545),
(0.998183892106923,0.996573304252679,0.996380621268545)))
REPRESENTATION_ITEM('')
SURFACE()
);
#828=(
BOUNDED_SURFACE()
B_SPLINE_SURFACE(1,2,((#103618,#103619,#103620),(#103621,#103622,#103623)),
 .UNSPECIFIED.,.F.,.F.,.F.)
B_SPLINE_SURFACE_WITH_KNOTS((2,2),(3,3),(0.,1.),(0.0255903596132031,0.0375948596691665),
 .UNSPECIFIED.)
GEOMETRIC_REPRESENTATION_ITEM()
RATIONAL_B_SPLINE_SURFACE(((0.996753121756002,0.997505687613138,0.999678813023773),
(0.996753121756002,0.997505687613138,0.999678813023773)))
REPRESENTATION_ITEM('')
SURFACE()
);
#829=(
BOUNDED_SURFACE()
B_SPLINE_SURFACE(1,2,((#103641,#103642,#103643,#103644,#103645),(#103646,
#103647,#103648,#103649,#103650)),.UNSPECIFIED.,.F.,.F.,.F.)
B_SPLINE_SURFACE_WITH_KNOTS((2,2),(3,2,3),(0.519229702930174,1.),(0.0365944846644854,
0.0384615384615384,0.0431859278882548),.UNSPECIFIED.)
GEOMETRIC_REPRESENTATION_ITEM()
RATIONAL_B_SPLINE_SURFACE(((0.999326490452227,0.999646063968199,1.,0.99910440092888,
0.998428822114433),(0.999326490452227,0.999646063968199,1.,0.99910440092888,
0.998428822114433)))
REPRESENTATION_ITEM('')
SURFACE()
);
#830=(
BOUNDED_SURFACE()
B_SPLINE_SURFACE(1,2,((#103706,#103707,#103708),(#103709,#103710,#103711)),
 .UNSPECIFIED.,.F.,.F.,.F.)
B_SPLINE_SURFACE_WITH_KNOTS((2,2),(3,3),(0.,1.),(0.0456081671210082,0.057598944781862),
 .UNSPECIFIED.)
GEOMETRIC_REPRESENTATION_ITEM()
RATIONAL_B_SPLINE_SURFACE(((0.997793907739635,0.996365558499691,0.996354522974128),
(0.997793907739635,0.996365558499691,0.996354522974128)))
REPRESENTATION_ITEM('')
SURFACE()
);
#831=(
BOUNDED_SURFACE()
B_SPLINE_SURFACE(1,2,((#103746,#103747,#103748),(#103749,#103750,#103751)),
 .UNSPECIFIED.,.F.,.F.,.F.)
B_SPLINE_SURFACE_WITH_KNOTS((2,2),(3,3),(0.,1.),(0.0556006976522477,0.067588885544619),
 .UNSPECIFIED.)
GEOMETRIC_REPRESENTATION_ITEM()
RATIONAL_B_SPLINE_SURFACE(((0.996397562408177,0.996150386836004,0.997319912821418),
(0.996397562408177,0.996150386836004,0.997319912821418)))
REPRESENTATION_ITEM('')
SURFACE()
);
#832=(
BOUNDED_SURFACE()
B_SPLINE_SURFACE(1,2,((#103752,#103753,#103754),(#103755,#103756,#103757)),
 .UNSPECIFIED.,.F.,.F.,.F.)
B_SPLINE_SURFACE_WITH_KNOTS((2,2),(3,3),(0.,1.),(0.0657448619281122,0.0758849574338225),
 .UNSPECIFIED.)
GEOMETRIC_REPRESENTATION_ITEM()
RATIONAL_B_SPLINE_SURFACE(((0.996993639757277,0.997798549146193,0.999617032345115),
(0.996993639757277,0.997798549146193,0.999617032345115)))
REPRESENTATION_ITEM('')
SURFACE()
);
#833=(
BOUNDED_SURFACE()
B_SPLINE_SURFACE(1,2,((#103832,#103833,#103834),(#103835,#103836,#103837)),
 .UNSPECIFIED.,.F.,.F.,.F.)
B_SPLINE_SURFACE_WITH_KNOTS((2,2),(3,3),(0.,1.),(0.00560769170938322,0.0176009697615935),
 .UNSPECIFIED.)
GEOMETRIC_REPRESENTATION_ITEM()
RATIONAL_B_SPLINE_SURFACE(((0.998183892106924,0.996573304252679,0.996380621268545),
(0.998183892106924,0.996573304252679,0.996380621268545)))
REPRESENTATION_ITEM('')
SURFACE()
);
#834=(
BOUNDED_SURFACE()
B_SPLINE_SURFACE(1,2,((#103922,#103923,#103924),(#103925,#103926,#103927)),
 .UNSPECIFIED.,.F.,.F.,.F.)
B_SPLINE_SURFACE_WITH_KNOTS((2,2),(3,3),(0.,1.),(0.0255903596131996,0.0375948596691703),
 .UNSPECIFIED.)
GEOMETRIC_REPRESENTATION_ITEM()
RATIONAL_B_SPLINE_SURFACE(((0.996753121756002,0.997505687613138,0.999678813023775),
(0.996753121756002,0.997505687613138,0.999678813023775)))
REPRESENTATION_ITEM('')
SURFACE()
);
#835=(
BOUNDED_SURFACE()
B_SPLINE_SURFACE(1,2,((#103945,#103946,#103947,#103948,#103949),(#103950,
#103951,#103952,#103953,#103954)),.UNSPECIFIED.,.F.,.F.,.F.)
B_SPLINE_SURFACE_WITH_KNOTS((2,2),(3,2,3),(0.519229702929906,1.),(0.036594484664473,
0.0384615384615384,0.043185927888243),.UNSPECIFIED.)
GEOMETRIC_REPRESENTATION_ITEM()
RATIONAL_B_SPLINE_SURFACE(((0.999326490452223,0.999646063968197,1.,0.999104400928882,
0.998428822114436),(0.999326490452223,0.999646063968197,1.,0.999104400928882,
0.998428822114436)))
REPRESENTATION_ITEM('')
SURFACE()
);
#836=(
BOUNDED_SURFACE()
B_SPLINE_SURFACE(1,2,((#104010,#104011,#104012),(#104013,#104014,#104015)),
 .UNSPECIFIED.,.F.,.F.,.F.)
B_SPLINE_SURFACE_WITH_KNOTS((2,2),(3,3),(0.,1.),(0.0456081671210071,0.0575989447818621),
 .UNSPECIFIED.)
GEOMETRIC_REPRESENTATION_ITEM()
RATIONAL_B_SPLINE_SURFACE(((0.997793907739636,0.996365558499691,0.996354522974128),
(0.997793907739636,0.996365558499691,0.996354522974128)))
REPRESENTATION_ITEM('')
SURFACE()
);
#837=(
BOUNDED_SURFACE()
B_SPLINE_SURFACE(1,2,((#104050,#104051,#104052),(#104053,#104054,#104055)),
 .UNSPECIFIED.,.F.,.F.,.F.)
B_SPLINE_SURFACE_WITH_KNOTS((2,2),(3,3),(0.,1.),(0.055600697652246,0.0675888855446162),
 .UNSPECIFIED.)
GEOMETRIC_REPRESENTATION_ITEM()
RATIONAL_B_SPLINE_SURFACE(((0.996397562408177,0.996150386836003,0.997319912821417),
(0.996397562408177,0.996150386836003,0.997319912821417)))
REPRESENTATION_ITEM('')
SURFACE()
);
#838=(
BOUNDED_SURFACE()
B_SPLINE_SURFACE(1,2,((#104056,#104057,#104058),(#104059,#104060,#104061)),
 .UNSPECIFIED.,.F.,.F.,.F.)
B_SPLINE_SURFACE_WITH_KNOTS((2,2),(3,3),(0.,1.),(0.0657448619281092,0.0758849574338239),
 .UNSPECIFIED.)
GEOMETRIC_REPRESENTATION_ITEM()
RATIONAL_B_SPLINE_SURFACE(((0.996993639757276,0.997798549146193,0.999617032345115),
(0.996993639757276,0.997798549146193,0.999617032345115)))
REPRESENTATION_ITEM('')
SURFACE()
);
#839=(
BOUNDED_SURFACE()
B_SPLINE_SURFACE(1,2,((#104130,#104131,#104132),(#104133,#104134,#104135)),
 .UNSPECIFIED.,.F.,.F.,.F.)
B_SPLINE_SURFACE_WITH_KNOTS((2,2),(3,3),(0.,1.),(0.00560769170938336,0.0176009697615918),
 .UNSPECIFIED.)
GEOMETRIC_REPRESENTATION_ITEM()
RATIONAL_B_SPLINE_SURFACE(((0.998183892106924,0.996573304252679,0.996380621268545),
(0.998183892106924,0.996573304252679,0.996380621268545)))
REPRESENTATION_ITEM('')
SURFACE()
);
#840=(
BOUNDED_SURFACE()
B_SPLINE_SURFACE(1,2,((#104226,#104227,#104228),(#104229,#104230,#104231)),
 .UNSPECIFIED.,.F.,.F.,.F.)
B_SPLINE_SURFACE_WITH_KNOTS((2,2),(3,3),(0.,1.),(0.0255903596132001,0.0375948596691636),
 .UNSPECIFIED.)
GEOMETRIC_REPRESENTATION_ITEM()
RATIONAL_B_SPLINE_SURFACE(((0.996753121756002,0.997505687613137,0.999678813023772),
(0.996753121756002,0.997505687613137,0.999678813023772)))
REPRESENTATION_ITEM('')
SURFACE()
);
#841=(
BOUNDED_SURFACE()
B_SPLINE_SURFACE(1,2,((#104249,#104250,#104251,#104252,#104253),(#104254,
#104255,#104256,#104257,#104258)),.UNSPECIFIED.,.F.,.F.,.F.)
B_SPLINE_SURFACE_WITH_KNOTS((2,2),(3,2,3),(0.519229702929822,1.),(0.0365944846644523,
0.0384615384615384,0.0431859278882314),.UNSPECIFIED.)
GEOMETRIC_REPRESENTATION_ITEM()
RATIONAL_B_SPLINE_SURFACE(((0.999326490452216,0.999646063968193,1.,0.999104400928884,
0.998428822114439),(0.999326490452216,0.999646063968193,1.,0.999104400928884,
0.998428822114439)))
REPRESENTATION_ITEM('')
SURFACE()
);
#842=(
BOUNDED_SURFACE()
B_SPLINE_SURFACE(1,2,((#104314,#104315,#104316),(#104317,#104318,#104319)),
 .UNSPECIFIED.,.F.,.F.,.F.)
B_SPLINE_SURFACE_WITH_KNOTS((2,2),(3,3),(0.,1.),(0.0456081671210085,0.0575989447818603),
 .UNSPECIFIED.)
GEOMETRIC_REPRESENTATION_ITEM()
RATIONAL_B_SPLINE_SURFACE(((0.997793907739635,0.996365558499691,0.996354522974128),
(0.997793907739635,0.996365558499691,0.996354522974128)))
REPRESENTATION_ITEM('')
SURFACE()
);
#843=(
BOUNDED_SURFACE()
B_SPLINE_SURFACE(1,2,((#104354,#104355,#104356),(#104357,#104358,#104359)),
 .UNSPECIFIED.,.F.,.F.,.F.)
B_SPLINE_SURFACE_WITH_KNOTS((2,2),(3,3),(0.,1.),(0.0556006976522427,0.0675888855446153),
 .UNSPECIFIED.)
GEOMETRIC_REPRESENTATION_ITEM()
RATIONAL_B_SPLINE_SURFACE(((0.996397562408177,0.996150386836003,0.997319912821417),
(0.996397562408177,0.996150386836003,0.997319912821417)))
REPRESENTATION_ITEM('')
SURFACE()
);
#844=(
BOUNDED_SURFACE()
B_SPLINE_SURFACE(1,2,((#104360,#104361,#104362),(#104363,#104364,#104365)),
 .UNSPECIFIED.,.F.,.F.,.F.)
B_SPLINE_SURFACE_WITH_KNOTS((2,2),(3,3),(0.,1.),(0.065744861928108,0.0758849574338233),
 .UNSPECIFIED.)
GEOMETRIC_REPRESENTATION_ITEM()
RATIONAL_B_SPLINE_SURFACE(((0.996993639757276,0.997798549146192,0.999617032345115),
(0.996993639757276,0.997798549146192,0.999617032345115)))
REPRESENTATION_ITEM('')
SURFACE()
);
#845=(
BOUNDED_SURFACE()
B_SPLINE_SURFACE(1,2,((#104440,#104441,#104442),(#104443,#104444,#104445)),
 .UNSPECIFIED.,.F.,.F.,.F.)
B_SPLINE_SURFACE_WITH_KNOTS((2,2),(3,3),(0.,1.),(0.00560769170938435,0.0176009697615927),
 .UNSPECIFIED.)
GEOMETRIC_REPRESENTATION_ITEM()
RATIONAL_B_SPLINE_SURFACE(((0.998183892106924,0.996573304252679,0.996380621268545),
(0.998183892106924,0.996573304252679,0.996380621268545)))
REPRESENTATION_ITEM('')
SURFACE()
);
#846=(
BOUNDED_SURFACE()
B_SPLINE_SURFACE(1,2,((#104530,#104531,#104532),(#104533,#104534,#104535)),
 .UNSPECIFIED.,.F.,.F.,.F.)
B_SPLINE_SURFACE_WITH_KNOTS((2,2),(3,3),(0.,1.),(0.025590359613201,0.0375948596691668),
 .UNSPECIFIED.)
GEOMETRIC_REPRESENTATION_ITEM()
RATIONAL_B_SPLINE_SURFACE(((0.996753121756002,0.997505687613138,0.999678813023773),
(0.996753121756002,0.997505687613138,0.999678813023773)))
REPRESENTATION_ITEM('')
SURFACE()
);
#847=(
BOUNDED_SURFACE()
B_SPLINE_SURFACE(1,2,((#104553,#104554,#104555,#104556,#104557),(#104558,
#104559,#104560,#104561,#104562)),.UNSPECIFIED.,.F.,.F.,.F.)
B_SPLINE_SURFACE_WITH_KNOTS((2,2),(3,2,3),(0.519229702929727,1.),(0.0365944846644431,
0.0384615384615384,0.0431859278882212),.UNSPECIFIED.)
GEOMETRIC_REPRESENTATION_ITEM()
RATIONAL_B_SPLINE_SURFACE(((0.999326490452213,0.999646063968191,1.,0.999104400928886,
0.998428822114442),(0.999326490452213,0.999646063968191,1.,0.999104400928886,
0.998428822114442)))
REPRESENTATION_ITEM('')
SURFACE()
);
#848=(
BOUNDED_SURFACE()
B_SPLINE_SURFACE(1,2,((#104618,#104619,#104620),(#104621,#104622,#104623)),
 .UNSPECIFIED.,.F.,.F.,.F.)
B_SPLINE_SURFACE_WITH_KNOTS((2,2),(3,3),(0.,1.),(0.0456081671210059,0.0575989447818637),
 .UNSPECIFIED.)
GEOMETRIC_REPRESENTATION_ITEM()
RATIONAL_B_SPLINE_SURFACE(((0.997793907739636,0.99636555849969,0.996354522974128),
(0.997793907739636,0.99636555849969,0.996354522974128)))
REPRESENTATION_ITEM('')
SURFACE()
);
#849=(
BOUNDED_SURFACE()
B_SPLINE_SURFACE(1,2,((#104658,#104659,#104660),(#104661,#104662,#104663)),
 .UNSPECIFIED.,.F.,.F.,.F.)
B_SPLINE_SURFACE_WITH_KNOTS((2,2),(3,3),(0.,1.),(0.055600697652249,0.0675888855446156),
 .UNSPECIFIED.)
GEOMETRIC_REPRESENTATION_ITEM()
RATIONAL_B_SPLINE_SURFACE(((0.996397562408177,0.996150386836004,0.997319912821417),
(0.996397562408177,0.996150386836004,0.997319912821417)))
REPRESENTATION_ITEM('')
SURFACE()
);
#850=(
BOUNDED_SURFACE()
B_SPLINE_SURFACE(1,2,((#104664,#104665,#104666),(#104667,#104668,#104669)),
 .UNSPECIFIED.,.F.,.F.,.F.)
B_SPLINE_SURFACE_WITH_KNOTS((2,2),(3,3),(0.,1.),(0.0657448619281089,0.0758849574338234),
 .UNSPECIFIED.)
GEOMETRIC_REPRESENTATION_ITEM()
RATIONAL_B_SPLINE_SURFACE(((0.996993639757276,0.997798549146192,0.999617032345115),
(0.996993639757276,0.997798549146192,0.999617032345115)))
REPRESENTATION_ITEM('')
SURFACE()
);
#851=(
BOUNDED_SURFACE()
B_SPLINE_SURFACE(1,2,((#104744,#104745,#104746),(#104747,#104748,#104749)),
 .UNSPECIFIED.,.F.,.F.,.F.)
B_SPLINE_SURFACE_WITH_KNOTS((2,2),(3,3),(0.,1.),(0.00560769170938427,0.0176009697615923),
 .UNSPECIFIED.)
GEOMETRIC_REPRESENTATION_ITEM()
RATIONAL_B_SPLINE_SURFACE(((0.998183892106924,0.996573304252679,0.996380621268545),
(0.998183892106924,0.996573304252679,0.996380621268545)))
REPRESENTATION_ITEM('')
SURFACE()
);
#852=(
BOUNDED_SURFACE()
B_SPLINE_SURFACE(1,2,((#104834,#104835,#104836),(#104837,#104838,#104839)),
 .UNSPECIFIED.,.F.,.F.,.F.)
B_SPLINE_SURFACE_WITH_KNOTS((2,2),(3,3),(0.,1.),(0.0255903596131988,0.0375948596691661),
 .UNSPECIFIED.)
GEOMETRIC_REPRESENTATION_ITEM()
RATIONAL_B_SPLINE_SURFACE(((0.996753121756001,0.997505687613137,0.999678813023773),
(0.996753121756001,0.997505687613137,0.999678813023773)))
REPRESENTATION_ITEM('')
SURFACE()
);
#853=(
BOUNDED_SURFACE()
B_SPLINE_SURFACE(1,2,((#104857,#104858,#104859,#104860,#104861),(#104862,
#104863,#104864,#104865,#104866)),.UNSPECIFIED.,.F.,.F.,.F.)
B_SPLINE_SURFACE_WITH_KNOTS((2,2),(3,2,3),(0.519229702929575,1.),(0.0365944846644434,
0.0384615384615384,0.0431859278882126),.UNSPECIFIED.)
GEOMETRIC_REPRESENTATION_ITEM()
RATIONAL_B_SPLINE_SURFACE(((0.999326490452213,0.999646063968191,1.,0.999104400928888,
0.998428822114445),(0.999326490452213,0.999646063968191,1.,0.999104400928888,
0.998428822114445)))
REPRESENTATION_ITEM('')
SURFACE()
);
#854=(
BOUNDED_SURFACE()
B_SPLINE_SURFACE(1,2,((#104922,#104923,#104924),(#104925,#104926,#104927)),
 .UNSPECIFIED.,.F.,.F.,.F.)
B_SPLINE_SURFACE_WITH_KNOTS((2,2),(3,3),(0.,1.),(0.0456081671210072,0.0575989447818615),
 .UNSPECIFIED.)
GEOMETRIC_REPRESENTATION_ITEM()
RATIONAL_B_SPLINE_SURFACE(((0.997793907739636,0.996365558499691,0.996354522974128),
(0.997793907739636,0.996365558499691,0.996354522974128)))
REPRESENTATION_ITEM('')
SURFACE()
);
#855=(
BOUNDED_SURFACE()
B_SPLINE_SURFACE(1,2,((#104962,#104963,#104964),(#104965,#104966,#104967)),
 .UNSPECIFIED.,.F.,.F.,.F.)
B_SPLINE_SURFACE_WITH_KNOTS((2,2),(3,3),(0.,1.),(0.0556006976522444,0.0675888855446182),
 .UNSPECIFIED.)
GEOMETRIC_REPRESENTATION_ITEM()
RATIONAL_B_SPLINE_SURFACE(((0.996397562408177,0.996150386836003,0.997319912821418),
(0.996397562408177,0.996150386836003,0.997319912821418)))
REPRESENTATION_ITEM('')
SURFACE()
);
#856=(
BOUNDED_SURFACE()
B_SPLINE_SURFACE(1,2,((#104968,#104969,#104970),(#104971,#104972,#104973)),
 .UNSPECIFIED.,.F.,.F.,.F.)
B_SPLINE_SURFACE_WITH_KNOTS((2,2),(3,3),(0.,1.),(0.0657448619281111,0.0758849574338232),
 .UNSPECIFIED.)
GEOMETRIC_REPRESENTATION_ITEM()
RATIONAL_B_SPLINE_SURFACE(((0.996993639757276,0.997798549146193,0.999617032345115),
(0.996993639757276,0.997798549146193,0.999617032345115)))
REPRESENTATION_ITEM('')
SURFACE()
);
#857=(
BOUNDED_SURFACE()
B_SPLINE_SURFACE(1,2,((#105048,#105049,#105050),(#105051,#105052,#105053)),
 .UNSPECIFIED.,.F.,.F.,.F.)
B_SPLINE_SURFACE_WITH_KNOTS((2,2),(3,3),(0.,1.),(0.00560769170938328,0.0176009697615924),
 .UNSPECIFIED.)
GEOMETRIC_REPRESENTATION_ITEM()
RATIONAL_B_SPLINE_SURFACE(((0.998183892106924,0.996573304252679,0.996380621268545),
(0.998183892106924,0.996573304252679,0.996380621268545)))
REPRESENTATION_ITEM('')
SURFACE()
);
#858=(
BOUNDED_SURFACE()
B_SPLINE_SURFACE(1,2,((#105138,#105139,#105140),(#105141,#105142,#105143)),
 .UNSPECIFIED.,.F.,.F.,.F.)
B_SPLINE_SURFACE_WITH_KNOTS((2,2),(3,3),(0.,1.),(0.025590359613199,0.0375948596691636),
 .UNSPECIFIED.)
GEOMETRIC_REPRESENTATION_ITEM()
RATIONAL_B_SPLINE_SURFACE(((0.996753121756001,0.997505687613137,0.999678813023772),
(0.996753121756001,0.997505687613137,0.999678813023772)))
REPRESENTATION_ITEM('')
SURFACE()
);
#859=(
BOUNDED_SURFACE()
B_SPLINE_SURFACE(1,2,((#105161,#105162,#105163,#105164,#105165),(#105166,
#105167,#105168,#105169,#105170)),.UNSPECIFIED.,.F.,.F.,.F.)
B_SPLINE_SURFACE_WITH_KNOTS((2,2),(3,2,3),(0.519229702927906,1.),(0.0365944846644382,
0.0384615384615384,0.0431859278882051),.UNSPECIFIED.)
GEOMETRIC_REPRESENTATION_ITEM()
RATIONAL_B_SPLINE_SURFACE(((0.999326490452211,0.999646063968191,1.,0.999104400928889,
0.998428822114447),(0.999326490452211,0.999646063968191,1.,0.999104400928889,
0.998428822114447)))
REPRESENTATION_ITEM('')
SURFACE()
);
#860=(
BOUNDED_SURFACE()
B_SPLINE_SURFACE(1,2,((#105226,#105227,#105228),(#105229,#105230,#105231)),
 .UNSPECIFIED.,.F.,.F.,.F.)
B_SPLINE_SURFACE_WITH_KNOTS((2,2),(3,3),(0.,1.),(0.0456081671210052,0.0575989447818616),
 .UNSPECIFIED.)
GEOMETRIC_REPRESENTATION_ITEM()
RATIONAL_B_SPLINE_SURFACE(((0.997793907739636,0.996365558499691,0.996354522974128),
(0.997793907739636,0.996365558499691,0.996354522974128)))
REPRESENTATION_ITEM('')
SURFACE()
);
#861=(
BOUNDED_SURFACE()
B_SPLINE_SURFACE(1,2,((#105266,#105267,#105268),(#105269,#105270,#105271)),
 .UNSPECIFIED.,.F.,.F.,.F.)
B_SPLINE_SURFACE_WITH_KNOTS((2,2),(3,3),(0.,1.),(0.0556006976522447,0.0675888855446152),
 .UNSPECIFIED.)
GEOMETRIC_REPRESENTATION_ITEM()
RATIONAL_B_SPLINE_SURFACE(((0.996397562408177,0.996150386836003,0.997319912821417),
(0.996397562408177,0.996150386836003,0.997319912821417)))
REPRESENTATION_ITEM('')
SURFACE()
);
#862=(
BOUNDED_SURFACE()
B_SPLINE_SURFACE(1,2,((#105272,#105273,#105274),(#105275,#105276,#105277)),
 .UNSPECIFIED.,.F.,.F.,.F.)
B_SPLINE_SURFACE_WITH_KNOTS((2,2),(3,3),(0.,1.),(0.065744861928108,0.0758849574338236),
 .UNSPECIFIED.)
GEOMETRIC_REPRESENTATION_ITEM()
RATIONAL_B_SPLINE_SURFACE(((0.996993639757276,0.997798549146192,0.999617032345115),
(0.996993639757276,0.997798549146192,0.999617032345115)))
REPRESENTATION_ITEM('')
SURFACE()
);
#863=(
BOUNDED_SURFACE()
B_SPLINE_SURFACE(1,2,((#105352,#105353,#105354),(#105355,#105356,#105357)),
 .UNSPECIFIED.,.F.,.F.,.F.)
B_SPLINE_SURFACE_WITH_KNOTS((2,2),(3,3),(0.,1.),(0.00560769170938434,0.0176009697615923),
 .UNSPECIFIED.)
GEOMETRIC_REPRESENTATION_ITEM()
RATIONAL_B_SPLINE_SURFACE(((0.998183892106924,0.996573304252679,0.996380621268545),
(0.998183892106924,0.996573304252679,0.996380621268545)))
REPRESENTATION_ITEM('')
SURFACE()
);
#864=(
BOUNDED_SURFACE()
B_SPLINE_SURFACE(1,2,((#105442,#105443,#105444),(#105445,#105446,#105447)),
 .UNSPECIFIED.,.F.,.F.,.F.)
B_SPLINE_SURFACE_WITH_KNOTS((2,2),(3,3),(0.,1.),(0.0255903596132011,0.0375948596691667),
 .UNSPECIFIED.)
GEOMETRIC_REPRESENTATION_ITEM()
RATIONAL_B_SPLINE_SURFACE(((0.996753121756002,0.997505687613138,0.999678813023773),
(0.996753121756002,0.997505687613138,0.999678813023773)))
REPRESENTATION_ITEM('')
SURFACE()
);
#865=(
BOUNDED_SURFACE()
B_SPLINE_SURFACE(1,2,((#105465,#105466,#105467,#105468,#105469),(#105470,
#105471,#105472,#105473,#105474)),.UNSPECIFIED.,.F.,.F.,.F.)
B_SPLINE_SURFACE_WITH_KNOTS((2,2),(3,2,3),(0.519229702925083,1.),(0.0365944846644329,
0.0384615384615384,0.0431859278882006),.UNSPECIFIED.)
GEOMETRIC_REPRESENTATION_ITEM()
RATIONAL_B_SPLINE_SURFACE(((0.99932649045221,0.99964606396819,1.,0.99910440092889,
0.998428822114448),(0.99932649045221,0.99964606396819,1.,0.99910440092889,
0.998428822114448)))
REPRESENTATION_ITEM('')
SURFACE()
);
#866=(
BOUNDED_SURFACE()
B_SPLINE_SURFACE(1,2,((#105530,#105531,#105532),(#105533,#105534,#105535)),
 .UNSPECIFIED.,.F.,.F.,.F.)
B_SPLINE_SURFACE_WITH_KNOTS((2,2),(3,3),(0.,1.),(0.0456081671210051,0.0575989447818617),
 .UNSPECIFIED.)
GEOMETRIC_REPRESENTATION_ITEM()
RATIONAL_B_SPLINE_SURFACE(((0.997793907739636,0.996365558499691,0.996354522974128),
(0.997793907739636,0.996365558499691,0.996354522974128)))
REPRESENTATION_ITEM('')
SURFACE()
);
#867=(
BOUNDED_SURFACE()
B_SPLINE_SURFACE(1,2,((#105570,#105571,#105572),(#105573,#105574,#105575)),
 .UNSPECIFIED.,.F.,.F.,.F.)
B_SPLINE_SURFACE_WITH_KNOTS((2,2),(3,3),(0.,1.),(0.0556006976522446,0.0675888855446173),
 .UNSPECIFIED.)
GEOMETRIC_REPRESENTATION_ITEM()
RATIONAL_B_SPLINE_SURFACE(((0.996397562408177,0.996150386836003,0.997319912821418),
(0.996397562408177,0.996150386836003,0.997319912821418)))
REPRESENTATION_ITEM('')
SURFACE()
);
#868=(
BOUNDED_SURFACE()
B_SPLINE_SURFACE(1,2,((#105576,#105577,#105578),(#105579,#105580,#105581)),
 .UNSPECIFIED.,.F.,.F.,.F.)
B_SPLINE_SURFACE_WITH_KNOTS((2,2),(3,3),(0.,1.),(0.0657448619281101,0.0758849574338238),
 .UNSPECIFIED.)
GEOMETRIC_REPRESENTATION_ITEM()
RATIONAL_B_SPLINE_SURFACE(((0.996993639757276,0.997798549146193,0.999617032345115),
(0.996993639757276,0.997798549146193,0.999617032345115)))
REPRESENTATION_ITEM('')
SURFACE()
);
#869=(
BOUNDED_SURFACE()
B_SPLINE_SURFACE(1,2,((#105656,#105657,#105658),(#105659,#105660,#105661)),
 .UNSPECIFIED.,.F.,.F.,.F.)
B_SPLINE_SURFACE_WITH_KNOTS((2,2),(3,3),(0.,1.),(0.00560769170938528,0.0176009697615926),
 .UNSPECIFIED.)
GEOMETRIC_REPRESENTATION_ITEM()
RATIONAL_B_SPLINE_SURFACE(((0.998183892106923,0.996573304252679,0.996380621268545),
(0.998183892106923,0.996573304252679,0.996380621268545)))
REPRESENTATION_ITEM('')
SURFACE()
);
#870=(
BOUNDED_SURFACE()
B_SPLINE_SURFACE(1,2,((#105746,#105747,#105748),(#105749,#105750,#105751)),
 .UNSPECIFIED.,.F.,.F.,.F.)
B_SPLINE_SURFACE_WITH_KNOTS((2,2),(3,3),(0.,1.),(0.0255903596132,0.0375948596691668),
 .UNSPECIFIED.)
GEOMETRIC_REPRESENTATION_ITEM()
RATIONAL_B_SPLINE_SURFACE(((0.996753121756002,0.997505687613138,0.999678813023773),
(0.996753121756002,0.997505687613138,0.999678813023773)))
REPRESENTATION_ITEM('')
SURFACE()
);
#871=(
BOUNDED_SURFACE()
B_SPLINE_SURFACE(1,2,((#105769,#105770,#105771,#105772,#105773),(#105774,
#105775,#105776,#105777,#105778)),.UNSPECIFIED.,.F.,.F.,.F.)
B_SPLINE_SURFACE_WITH_KNOTS((2,2),(3,2,3),(0.5192297029227,1.),(0.0365944846644306,
0.0384615384615384,0.0431859276813022),.UNSPECIFIED.)
GEOMETRIC_REPRESENTATION_ITEM()
RATIONAL_B_SPLINE_SURFACE(((0.999326490452209,0.999646063968189,1.,0.999104400968112,
0.99842882217362),(0.999326490452208,0.999646063968189,1.,0.999104400968112,
0.99842882217362)))
REPRESENTATION_ITEM('')
SURFACE()
);
#872=(
BOUNDED_SURFACE()
B_SPLINE_SURFACE(1,2,((#105834,#105835,#105836),(#105837,#105838,#105839)),
 .UNSPECIFIED.,.F.,.F.,.F.)
B_SPLINE_SURFACE_WITH_KNOTS((2,2),(3,3),(0.,1.),(0.0456081671210065,0.0575989447818604),
 .UNSPECIFIED.)
GEOMETRIC_REPRESENTATION_ITEM()
RATIONAL_B_SPLINE_SURFACE(((0.997793907739636,0.996365558499691,0.996354522974128),
(0.997793907739636,0.996365558499691,0.996354522974128)))
REPRESENTATION_ITEM('')
SURFACE()
);
#873=(
BOUNDED_SURFACE()
B_SPLINE_SURFACE(1,2,((#105874,#105875,#105876),(#105877,#105878,#105879)),
 .UNSPECIFIED.,.F.,.F.,.F.)
B_SPLINE_SURFACE_WITH_KNOTS((2,2),(3,3),(0.,1.),(0.0556006976522425,0.0675888855446154),
 .UNSPECIFIED.)
GEOMETRIC_REPRESENTATION_ITEM()
RATIONAL_B_SPLINE_SURFACE(((0.996397562408177,0.996150386836003,0.997319912821417),
(0.996397562408177,0.996150386836003,0.997319912821417)))
REPRESENTATION_ITEM('')
SURFACE()
);
#874=(
BOUNDED_SURFACE()
B_SPLINE_SURFACE(1,2,((#105880,#105881,#105882),(#105883,#105884,#105885)),
 .UNSPECIFIED.,.F.,.F.,.F.)
B_SPLINE_SURFACE_WITH_KNOTS((2,2),(3,3),(0.,1.),(0.065744861928108,0.075884957433824),
 .UNSPECIFIED.)
GEOMETRIC_REPRESENTATION_ITEM()
RATIONAL_B_SPLINE_SURFACE(((0.996993639757276,0.997798549146192,0.999617032345115),
(0.996993639757276,0.997798549146192,0.999617032345115)))
REPRESENTATION_ITEM('')
SURFACE()
);
#875=(
BOUNDED_SURFACE()
B_SPLINE_SURFACE(1,2,((#105960,#105961,#105962),(#105963,#105964,#105965)),
 .UNSPECIFIED.,.F.,.F.,.F.)
B_SPLINE_SURFACE_WITH_KNOTS((2,2),(3,3),(0.,1.),(0.00560769170938643,0.0176009697615936),
 .UNSPECIFIED.)
GEOMETRIC_REPRESENTATION_ITEM()
RATIONAL_B_SPLINE_SURFACE(((0.998183892106923,0.996573304252679,0.996380621268545),
(0.998183892106923,0.996573304252679,0.996380621268545)))
REPRESENTATION_ITEM('')
SURFACE()
);
#876=(
BOUNDED_SURFACE()
B_SPLINE_SURFACE(1,2,((#106050,#106051,#106052),(#106053,#106054,#106055)),
 .UNSPECIFIED.,.F.,.F.,.F.)
B_SPLINE_SURFACE_WITH_KNOTS((2,2),(3,3),(0.,1.),(0.025590359613201,0.037594859669168),
 .UNSPECIFIED.)
GEOMETRIC_REPRESENTATION_ITEM()
RATIONAL_B_SPLINE_SURFACE(((0.996753121756002,0.997505687613138,0.999678813023774),
(0.996753121756002,0.997505687613138,0.999678813023774)))
REPRESENTATION_ITEM('')
SURFACE()
);
#877=(
BOUNDED_SURFACE()
B_SPLINE_SURFACE(1,2,((#106073,#106074,#106075,#106076,#106077),(#106078,
#106079,#106080,#106081,#106082)),.UNSPECIFIED.,.F.,.F.,.F.)
B_SPLINE_SURFACE_WITH_KNOTS((2,2),(3,2,3),(0.519229702919849,1.),(0.0365944846644282,
0.0384615384615384,0.043185927681299),.UNSPECIFIED.)
GEOMETRIC_REPRESENTATION_ITEM()
RATIONAL_B_SPLINE_SURFACE(((0.999326490452208,0.999646063968189,1.,0.999104400968112,
0.998428822173621),(0.999326490452208,0.999646063968189,1.,0.999104400968112,
0.998428822173621)))
REPRESENTATION_ITEM('')
SURFACE()
);
#878=(
BOUNDED_SURFACE()
B_SPLINE_SURFACE(1,2,((#106138,#106139,#106140),(#106141,#106142,#106143)),
 .UNSPECIFIED.,.F.,.F.,.F.)
B_SPLINE_SURFACE_WITH_KNOTS((2,2),(3,3),(0.,1.),(0.0456081671210094,0.0575989447818618),
 .UNSPECIFIED.)
GEOMETRIC_REPRESENTATION_ITEM()
RATIONAL_B_SPLINE_SURFACE(((0.997793907739635,0.996365558499691,0.996354522974128),
(0.997793907739635,0.996365558499691,0.996354522974128)))
REPRESENTATION_ITEM('')
SURFACE()
);
#879=(
BOUNDED_SURFACE()
B_SPLINE_SURFACE(1,2,((#106178,#106179,#106180),(#106181,#106182,#106183)),
 .UNSPECIFIED.,.F.,.F.,.F.)
B_SPLINE_SURFACE_WITH_KNOTS((2,2),(3,3),(0.,1.),(0.0556006976522459,0.067588885544616),
 .UNSPECIFIED.)
GEOMETRIC_REPRESENTATION_ITEM()
RATIONAL_B_SPLINE_SURFACE(((0.996397562408177,0.996150386836004,0.997319912821417),
(0.996397562408177,0.996150386836004,0.997319912821417)))
REPRESENTATION_ITEM('')
SURFACE()
);
#880=(
BOUNDED_SURFACE()
B_SPLINE_SURFACE(1,2,((#106184,#106185,#106186),(#106187,#106188,#106189)),
 .UNSPECIFIED.,.F.,.F.,.F.)
B_SPLINE_SURFACE_WITH_KNOTS((2,2),(3,3),(0.,1.),(0.0657448619281089,0.0758849574338248),
 .UNSPECIFIED.)
GEOMETRIC_REPRESENTATION_ITEM()
RATIONAL_B_SPLINE_SURFACE(((0.996993639757276,0.997798549146193,0.999617032345115),
(0.996993639757276,0.997798549146193,0.999617032345115)))
REPRESENTATION_ITEM('')
SURFACE()
);
#881=CONICAL_SURFACE('',#45721,0.006,0.78539816339745);
#882=CONICAL_SURFACE('',#45823,0.0055,0.78539816339746);
#886=ELLIPSE('',#46076,0.00505204240379114,0.00230472370237008);
#887=ELLIPSE('',#46082,0.00460880147227119,0.00192167872360598);
#888=ELLIPSE('',#46092,0.00865509473932915,0.00758557668119749);
#889=ELLIPSE('',#46180,0.00621516716548231,0.00601620425193647);
#890=ELLIPSE('',#46181,0.00648423822157093,0.00593239723153129);
#891=ELLIPSE('',#46187,0.0070905986611636,0.0012893204637363);
#892=ELLIPSE('',#46191,0.0050534643241034,0.00230601081969104);
#893=ELLIPSE('',#46202,0.00865512552606261,0.00758560652833544);
#894=ELLIPSE('',#46246,0.00621537602140178,0.00601630533451007);
#895=ELLIPSE('',#46247,0.00648435333080737,0.00593260142270717);
#896=ELLIPSE('',#46249,0.00709129851600952,0.00128949452168959);
#897=ELLIPSE('',#46252,0.00505210470082459,0.00230478008540994);
#898=ELLIPSE('',#46263,0.00865513528145594,0.00758561599623131);
#899=ELLIPSE('',#46307,0.00621524391851374,0.00601624139928821);
#900=ELLIPSE('',#46308,0.0064843122029582,0.00593252852474117);
#901=ELLIPSE('',#46310,0.00709039114265013,0.00128926885533352);
#902=ELLIPSE('',#46313,0.00505390723859556,0.00230641180953775);
#903=ELLIPSE('',#46324,0.00865509821766808,0.00758558009748805);
#904=ELLIPSE('',#46368,0.00621529545248987,0.00601626634096811);
#905=ELLIPSE('',#46369,0.0064843319772775,0.00593256359853056);
#906=ELLIPSE('',#46371,0.00709065821253241,0.0012893352089985);
#907=ELLIPSE('',#46374,0.0050890313490455,0.00233831897377822);
#908=ELLIPSE('',#46385,0.00865510845069279,0.00758559005407188);
#909=ELLIPSE('',#46429,0.00621534731034554,0.0060162914392953);
#910=ELLIPSE('',#46430,0.00648437887335218,0.00593264681892162);
#911=ELLIPSE('',#46432,0.00709002873922731,0.00128917846438477);
#912=ELLIPSE('',#46435,0.0050520856182914,0.00230476281589073);
#913=ELLIPSE('',#46446,0.00865511426296996,0.00758559562353494);
#914=ELLIPSE('',#46490,0.00621521803085549,0.00601622887006362);
#915=ELLIPSE('',#46491,0.00648442221515968,0.00593272364388297);
#916=ELLIPSE('',#46493,0.00709090319602856,0.00128939616487807);
#917=ELLIPSE('',#46496,0.00505269719487927,0.00230531637340278);
#918=ELLIPSE('',#46507,0.00865513573468569,0.00758561645123289);
#919=ELLIPSE('',#46551,0.00621526992760936,0.00601625398735536);
#920=ELLIPSE('',#46552,0.00648433724962787,0.00593257294843176);
#921=ELLIPSE('',#46554,0.00709023333512276,0.00128922949570934);
#922=ELLIPSE('',#46557,0.0050526446036089,0.00230526876880624);
#923=ELLIPSE('',#46568,0.00865513735985754,0.00758561798170201);
#924=ELLIPSE('',#46612,0.00621519248449229,0.00601621650592652);
#925=ELLIPSE('',#46613,0.00648435975442786,0.00593261285788805);
#926=ELLIPSE('',#46615,0.00709078687884672,0.00128936725092669);
#927=ELLIPSE('',#46618,0.00505218071000825,0.00230484888152921);
#928=ELLIPSE('',#46629,0.00865511153964906,0.0075855930117702);
#929=ELLIPSE('',#46673,0.00621521819686636,0.00601622895043552);
#930=ELLIPSE('',#46674,0.00648435621900189,0.0059326065851825);
#931=ELLIPSE('',#46676,0.00709157095271754,0.00128956239099297);
#932=ELLIPSE('',#46679,0.00505287260556312,0.00230547515433253);
#933=ELLIPSE('',#46690,0.00865512124916736,0.00758560240185387);
#934=ELLIPSE('',#46734,0.00621534747320918,0.00601629151811313);
#935=ELLIPSE('',#46735,0.00648436926222662,0.00593262969405175);
#936=ELLIPSE('',#46737,0.00709121156280895,0.00128947288156415);
#937=ELLIPSE('',#46740,0.00505234254805064,0.00230499536293981);
#938=ELLIPSE('',#46751,0.00865510577377427,0.00758558737369668);
#939=ELLIPSE('',#46795,0.0062152056610705,0.00601622288331262);
#940=ELLIPSE('',#46796,0.00648437614788083,0.00593264193050572);
#941=ELLIPSE('',#46798,0.00709079551933392,0.00128936945124519);
#942=ELLIPSE('',#46801,0.00505308063550296,0.00230566346961813);
#943=ELLIPSE('',#46812,0.00865516464328738,0.00758564444626258);
#944=ELLIPSE('',#46856,0.00621525717507994,0.00601624781537191);
#945=ELLIPSE('',#46857,0.00648435399756577,0.00593260264617468);
#946=ELLIPSE('',#46859,0.00709125807572499,0.00128948456247621);
#947=ELLIPSE('',#46862,0.00505407572626888,0.00230656436075209);
#948=ELLIPSE('',#46873,0.00865507611239517,0.00758555855456918);
#949=ELLIPSE('',#46917,0.00621529569567966,0.00601626645859758);
#950=ELLIPSE('',#46918,0.00648434122881266,0.00593257999422627);
#951=ELLIPSE('',#46920,0.00709052630964259,0.00128930239034199);
#952=ELLIPSE('',#46923,0.00505216738260241,0.00230483681883502);
#953=ELLIPSE('',#46934,0.0086551013472187,0.00758558314017204);
#954=ELLIPSE('',#46978,0.00621523480011978,0.0060162369862471);
#955=ELLIPSE('',#46979,0.00648435210818557,0.00593259930385406);
#956=ELLIPSE('',#46981,0.00709110677776559,0.0012894465833154);
#957=ELLIPSE('',#46984,0.00505386286247069,0.00230637163389658);
#958=ELLIPSE('',#46995,0.00865508082772966,0.00758556319306449);
#959=ELLIPSE('',#47039,0.00621524583016535,0.00601624232453474);
#960=ELLIPSE('',#47040,0.00648433993340202,0.00593257769459382);
#961=ELLIPSE('',#47042,0.00709064233112991,0.0012893311074234);
#962=ELLIPSE('',#47045,0.00497700215010779,0.00223729133900348);
#963=ELLIPSE('',#47056,0.0086551050322695,0.00758558656708154);
#964=ELLIPSE('',#47100,0.00621523774150067,0.0060162384097202);
#965=ELLIPSE('',#47101,0.0064843246995372,0.00593255066143694);
#966=ELLIPSE('',#47103,0.00709045075792868,0.00128928348314944);
#967=ELLIPSE('',#47106,0.0049942788104379,0.00225273055972324);
#968=ELLIPSE('',#47117,0.00865514878432738,0.00758562908741592);
#969=ELLIPSE('',#47161,0.00621525709474776,0.00601624777632549);
#970=ELLIPSE('',#47162,0.00648435246172703,0.00593259993727655);
#971=ELLIPSE('',#47164,0.00709029022462916,0.00128924346647885);
#972=ELLIPSE('',#47167,0.00505405294220357,0.00230654373401579);
#973=ELLIPSE('',#47178,0.00865514566750678,0.00758562601058983);
#974=ELLIPSE('',#47222,0.00621520533038221,0.00601622272323379);
#975=ELLIPSE('',#47223,0.00648434821407422,0.00593259239188297);
#976=ELLIPSE('',#47225,0.00709096491369054,0.00128941161665014);
#977=ELLIPSE('',#47228,0.00505353081443679,0.00230607101122026);
#978=ELLIPSE('',#47239,0.00865505354911252,0.00758553677638153);
#979=ELLIPSE('',#47283,0.00621527010598489,0.00601625407364374);
#980=ELLIPSE('',#47284,0.00648438806646418,0.00593266310364782);
#981=ELLIPSE('',#47286,0.00709071191997087,0.0012893485270995);
#982=ELLIPSE('',#47289,0.00505346384021596,0.00230601037853248);
#983=ELLIPSE('',#47300,0.00865510202610495,0.00758558385576672);
#984=ELLIPSE('',#47344,0.00621524420609326,0.00601624153854915);
#985=ELLIPSE('',#47345,0.00648436364018349,0.00593261972706044);
#986=ELLIPSE('',#47347,0.00709069660148338,0.0012893447619227);
#987=ELLIPSE('',#47350,0.00505505780866651,0.00230745364042269);
#988=ELLIPSE('',#47361,0.00865515793670053,0.0075856380555555);
#989=ELLIPSE('',#47405,0.00621521863585752,0.00601622916295315);
#990=ELLIPSE('',#47406,0.00648436189412657,0.0059326166804513);
#991=ELLIPSE('',#47408,0.00709088846227213,0.00128939245022837);
#992=ELLIPSE('',#47411,0.00504563136550804,0.00229892492076941);
#993=ELLIPSE('',#47422,0.00865510725747081,0.00758558883147086);
#994=ELLIPSE('',#47466,0.00621519257981388,0.00601621655201505);
#995=ELLIPSE('',#47467,0.0064843435728204,0.00593258411188729);
#996=ELLIPSE('',#47469,0.00709119685945131,0.00128946934905443);
#997=ELLIPSE('',#47472,0.00505391488108627,0.00230641873073941);
#998=ELLIPSE('',#47483,0.00865515520019524,0.00758563531672948);
#999=ELLIPSE('',#47527,0.00621537347876877,0.00601630410400769);
#1000=ELLIPSE('',#47528,0.0064843388243652,0.00593257571394916);
#1001=ELLIPSE('',#47530,0.00709076450352905,0.00128936161857139);
#1002=ELLIPSE('',#47533,0.005053948238314,0.00230644893380194);
#1003=ELLIPSE('',#47544,0.00865509653169551,0.00758557854237256);
#1004=ELLIPSE('',#47588,0.00621514106793808,0.00601619162089527);
#1005=ELLIPSE('',#47589,0.00648424807037612,0.00593241469410971);
#1006=ELLIPSE('',#47591,0.00709079105844187,0.00128936836893104);
#1007=ELLIPSE('',#47594,0.00505231057978,0.00230496642628584);
#1008=ELLIPSE('',#47605,0.00865508149523495,0.00758556383848639);
#1009=ELLIPSE('',#47649,0.00621539900993303,0.00601631646068148);
#1010=ELLIPSE('',#47650,0.00648433706096967,0.00593257260494097);
#1011=ELLIPSE('',#47652,0.00709114959659087,0.0012894575414131);
#1012=ELLIPSE('',#47655,0.00505417128153103,0.00230665088079652);
#1013=ELLIPSE('',#47666,0.00865512007154011,0.00758560124867166);
#1014=ELLIPSE('',#47710,0.0062153221253105,0.00601627925005241);
#1015=ELLIPSE('',#47711,0.00648437107278222,0.00593263291279239);
#1016=ELLIPSE('',#47713,0.00709055276537754,0.00128930892171807);
#1017=ELLIPSE('',#47716,0.00504571052979579,0.00229899647725242);
#1018=ELLIPSE('',#47727,0.00865515831542652,0.00758563843237898);
#1019=ELLIPSE('',#47771,0.00621504059289944,0.00601614299178234);
#1020=ELLIPSE('',#47772,0.00648435366732346,0.00593260206262849);
#1021=ELLIPSE('',#47774,0.00709067179251568,0.00128933848534169);
#1022=ELLIPSE('',#47777,0.0049748455941374,0.00223536775184007);
#1023=ELLIPSE('',#47788,0.00865512077413154,0.00758560196280287);
#1024=ELLIPSE('',#47832,0.00621529596421664,0.00601626658841289);
#1025=ELLIPSE('',#47833,0.00648438623642478,0.00593265985810756);
#1026=ELLIPSE('',#47835,0.0070908495799914,0.00128938276638011);
#1027=ELLIPSE('',#47838,0.00498598901432705,0.00224531598960363);
#1028=ELLIPSE('',#47849,0.00865514380798239,0.00758562431463873);
#1029=ELLIPSE('',#47893,0.00621521820687037,0.00601622895494);
#1030=ELLIPSE('',#47894,0.00648432613400307,0.00593255322684216);
#1031=ELLIPSE('',#47896,0.00709071216078011,0.00128934845297877);
#1032=ELLIPSE('',#47899,0.00505220961919958,0.00230487504732119);
#1033=ELLIPSE('',#47910,0.00865515886241701,0.00758563894485504);
#1034=ELLIPSE('',#47954,0.00621539897200116,0.00601631644192197);
#1035=ELLIPSE('',#47955,0.00648429433668458,0.00593249679273564);
#1036=ELLIPSE('',#47957,0.00709092653210478,0.00128940198033132);
#1037=ELLIPSE('',#47960,0.00505363409789085,0.00230616451930728);
#1038=ELLIPSE('',#47971,0.00865511993115791,0.00758560120699035);
#1039=ELLIPSE('',#48015,0.00621534716993814,0.00601629137100437);
#1040=ELLIPSE('',#48016,0.00648432509643861,0.0059325513838022);
#1041=ELLIPSE('',#48018,0.0070912200594845,0.00128947495864189);
#1042=ELLIPSE('',#48021,0.00505222431865997,0.00230488835088698);
#1043=ELLIPSE('',#48032,0.00865506890500387,0.00758555170092938);
#1044=ELLIPSE('',#48076,0.00621514063419339,0.00601619141091768);
#1045=ELLIPSE('',#48077,0.00648435306981849,0.00593260099471013);
#1046=ELLIPSE('',#48079,0.00709071025182221,0.00128934820887216);
#1047=ELLIPSE('',#48082,0.00505327809031931,0.00230584221748581);
#1048=ELLIPSE('',#48093,0.00865515228595944,0.00758563259983201);
#1049=ELLIPSE('',#48137,0.00621534746386843,0.00601629151335203);
#1050=ELLIPSE('',#48138,0.00648433641997979,0.00593257147747394);
#1051=ELLIPSE('',#48140,0.00709090941811193,0.00128939770831554);
#1052=ELLIPSE('',#48143,0.00505253275184091,0.00230516752406919);
#1053=ELLIPSE('',#48154,0.00865507528679423,0.00758555773898941);
#1054=ELLIPSE('',#48198,0.00621533449362357,0.00601628523588446);
#1055=ELLIPSE('',#48199,0.00648433275812308,0.0059325649596866);
#1056=ELLIPSE('',#48201,0.00709058807553439,0.00128931769610372);
#1057=ELLIPSE('',#48204,0.00505264582740208,0.00230526987582819);
#1058=ELLIPSE('',#48215,0.00865516225075192,0.00758564219542599);
#1059=ELLIPSE('',#48259,0.00621532149524689,0.00601627894494369);
#1060=ELLIPSE('',#48260,0.00648439073664356,0.00593266783283331);
#1061=ELLIPSE('',#48262,0.00709118291446364,0.00128946573593998);
#1062=ELLIPSE('',#48265,0.00505239964645357,0.00230504704486186);
#1063=ELLIPSE('',#48276,0.0086550935418262,0.00758557553418211);
#1064=ELLIPSE('',#48320,0.00621523121561208,0.00601623525106577);
#1065=ELLIPSE('',#48321,0.0064843641048612,0.00593262058267339);
#1066=ELLIPSE('',#48323,0.00709104236502589,0.00128943077820424);
#1067=ELLIPSE('',#48326,0.0050525425659858,0.0023051764069886);
#1068=ELLIPSE('',#48337,0.00865508682964421,0.00758556902181305);
#1069=ELLIPSE('',#48381,0.00621523116343429,0.00601623522580888);
#1070=ELLIPSE('',#48382,0.0064843477615119,0.00593259158809656);
#1071=ELLIPSE('',#48384,0.00709066162127243,0.0012893359428282);
#1072=ELLIPSE('',#48387,0.00498500862158727,0.00224443989119654);
#1073=ELLIPSE('',#48398,0.00865510656953884,0.00758558822009033);
#1074=ELLIPSE('',#48442,0.00621517946931786,0.0060162102065265);
#1075=ELLIPSE('',#48443,0.00648435291446554,0.00593260071268177);
#1076=ELLIPSE('',#48445,0.00709069939164397,0.00128934538239027);
#1077=ELLIPSE('',#48448,0.00505387585032357,0.00230638339351009);
#1078=ELLIPSE('',#48459,0.00865517106043899,0.00758565079628095);
#1079=ELLIPSE('',#48503,0.00621524417632009,0.00601624152393858);
#1080=ELLIPSE('',#48504,0.00648433396300445,0.00593256709201826);
#1081=ELLIPSE('',#48506,0.00709056942096103,0.00128931313168986);
#1082=ELLIPSE('',#48509,0.00505243006869415,0.00230507457996915);
#1083=ELLIPSE('',#48520,0.00865518739164197,0.00758566662396141);
#1084=ELLIPSE('',#48564,0.00621526384282503,0.00601625104227291);
#1085=ELLIPSE('',#48565,0.00648434251869749,0.00593258228049829);
#1086=ELLIPSE('',#48567,0.00709045845399877,0.00128928544995619);
#1087=ELLIPSE('',#48570,0.00505342198852363,0.00230597248826897);
#1088=ELLIPSE('',#48581,0.00865509832858885,0.00758558021126826);
#1089=ELLIPSE('',#48625,0.00621520544883468,0.00601622278028145);
#1090=ELLIPSE('',#48626,0.00648436223366202,0.00593261726583697);
#1091=ELLIPSE('',#48628,0.00709066606273037,0.0012893371910688);
#1092=ELLIPSE('',#48631,0.00505290596600244,0.00230550535243315);
#1093=ELLIPSE('',#48642,0.00865511613860218,0.00758559749223903);
#1094=ELLIPSE('',#48686,0.00621524420773405,0.0060162415391342);
#1095=ELLIPSE('',#48687,0.00648436382412113,0.00593262008351636);
#1096=ELLIPSE('',#48689,0.00709084298865159,0.00128938119659501);
#1097=ELLIPSE('',#48692,0.00505273138252932,0.00230534731942932);
#1098=ELLIPSE('',#48703,0.00865515121971655,0.00758563144244627);
#1099=ELLIPSE('',#48747,0.00621534729708559,0.00601629143262738);
#1100=ELLIPSE('',#48748,0.00648437791316611,0.0059326450846128);
#1101=ELLIPSE('',#48750,0.00709077396930198,0.00128936401951887);
#1102=ELLIPSE('',#48758,0.0050525152800079,0.00230515170877071);
#1103=ELLIPSE('',#48764,0.00865510594678074,0.00758558765394751);
#1104=ELLIPSE('',#48808,0.00621537342646163,0.00601630407875128);
#1105=ELLIPSE('',#48809,0.00648430341187163,0.00593251290911168);
#1106=ELLIPSE('',#48811,0.00709066882204238,0.00128933789968135);
#1107=ELLIPSE('',#48824,0.00505237134147902,0.0023050214260488);
#1108=ELLIPSE('',#48830,0.00865513889575835,0.00758561962224155);
#1109=ELLIPSE('',#48869,0.00621527020298751,0.00601625412034941);
#1110=ELLIPSE('',#48870,0.00648435578149643,0.00593260581661072);
#1111=ELLIPSE('',#48872,0.00709059988545386,0.00128932076398224);
#1112=ELLIPSE('',#48893,0.00865512097604794,0.00758560212593767);
#1113=ELLIPSE('',#48902,0.00460921634661896,0.00192202285706926);
#1114=ELLIPSE('',#48930,0.00621514084277246,0.00601619151211962);
#1115=ELLIPSE('',#48931,0.0064843629627248,0.00593261855117462);
#1116=ELLIPSE('',#48933,0.00709081214989054,0.00128937362404988);
#1117=ELLIPSE('',#48965,0.00461178042656441,0.00192415041839508);
#1118=ELLIPSE('',#48971,0.00865515359670422,0.00758563388640994);
#1119=ELLIPSE('',#48991,0.00621526986242424,0.0060162539556225);
#1120=ELLIPSE('',#48992,0.00648432994839084,0.00593255998262295);
#1121=ELLIPSE('',#48994,0.00709045362965754,0.00128928441829338);
#1122=ELLIPSE('',#49031,0.00505250516664137,0.00230514255651931);
#1123=ELLIPSE('',#49037,0.00865516221802523,0.00758564206595745);
#1124=ELLIPSE('',#49052,0.00621521875625456,0.00601622922104769);
#1125=ELLIPSE('',#49053,0.0064843251186602,0.00593255145155149);
#1126=ELLIPSE('',#49055,0.00709092921434546,0.00128940267805035);
#1127=ELLIPSE('',#49099,0.00460883271893841,0.00192170463706111);
#1128=ELLIPSE('',#49105,0.00865514794548704,0.00758562834632257);
#1129=ELLIPSE('',#49113,0.00621529595082828,0.00601626658192771);
#1130=ELLIPSE('',#49114,0.00648438224890444,0.00593265271232124);
#1131=ELLIPSE('',#49116,0.00709044419804569,0.00128928198746711);
#1132=ELLIPSE('',#49118,0.00621547662594353,0.00601635402501883);
#1133=ELLIPSE('',#49119,0.00648431602834799,0.00593253527427483);
#1134=ELLIPSE('',#49121,0.00709091596384868,0.00128939945197051);
#1135=ELLIPSE('',#49123,0.00865512107813427,0.00758560229656082);
#1142=B_SPLINE_CURVE_WITH_KNOTS('',3,(#63532,#63533,#63534,#63535,#63536,
#63537),.UNSPECIFIED.,.F.,.F.,(4,2,4),(0.00611332411698155,0.00920174751816869,
0.0184034950186372),.UNSPECIFIED.);
#1143=B_SPLINE_CURVE_WITH_KNOTS('',3,(#63542,#63543,#63544,#63545),
 .UNSPECIFIED.,.F.,.F.,(4,4),(0.,0.00611332411698155),.UNSPECIFIED.);
#1144=B_SPLINE_CURVE_WITH_KNOTS('',3,(#63551,#63552,#63553,#63554,#63555,
#63556),.UNSPECIFIED.,.F.,.F.,(4,2,4),(-0.0184046527946452,-0.00920271228272339,
-9.99999999399051E-7),.UNSPECIFIED.);
#1145=B_SPLINE_CURVE_WITH_KNOTS('',3,(#63558,#63559,#63560,#63561,#63562,
#63563),.UNSPECIFIED.,.F.,.F.,(4,2,4),(-0.0184034950181132,-0.00920121908066632,
0.),.UNSPECIFIED.);
#1146=B_SPLINE_CURVE_WITH_KNOTS('',3,(#63569,#63570,#63571,#63572,#63573,
#63574),.UNSPECIFIED.,.F.,.F.,(4,2,4),(-0.0184046552084519,-0.00920271305813145,
-9.99999998350369E-7),.UNSPECIFIED.);
#1147=B_SPLINE_CURVE_WITH_KNOTS('',3,(#63576,#63577,#63578,#63579,#63580,
#63581),.UNSPECIFIED.,.F.,.F.,(4,2,4),(-0.0184034950162585,-0.00920171905417117,
0.),.UNSPECIFIED.);
#1148=B_SPLINE_CURVE_WITH_KNOTS('',3,(#63587,#63588,#63589,#63590,#63591,
#63592),.UNSPECIFIED.,.F.,.F.,(4,2,4),(-0.0184046525439867,-0.00920271218195336,
-9.99999998588597E-7),.UNSPECIFIED.);
#1149=B_SPLINE_CURVE_WITH_KNOTS('',3,(#63594,#63595,#63596,#63597,#63598,
#63599),.UNSPECIFIED.,.F.,.F.,(4,2,4),(-0.0184034950137807,-0.0092012190782782,
0.),.UNSPECIFIED.);
#1150=B_SPLINE_CURVE_WITH_KNOTS('',3,(#63605,#63606,#63607,#63608,#63609,
#63610),.UNSPECIFIED.,.F.,.F.,(4,2,4),(-0.0184046538139259,-0.0092027126177381,
-9.99999998292297E-7),.UNSPECIFIED.);
#1151=B_SPLINE_CURVE_WITH_KNOTS('',3,(#63612,#63613,#63614,#63615,#63616,
#63617),.UNSPECIFIED.,.F.,.F.,(4,2,4),(-0.0184034922219404,-0.00920171720053826,
0.),.UNSPECIFIED.);
#1152=B_SPLINE_CURVE_WITH_KNOTS('',3,(#63623,#63624,#63625,#63626,#63627,
#63628),.UNSPECIFIED.,.F.,.F.,(4,2,4),(-0.0184046552625379,-0.00920321307301659,
-9.99999997544632E-7),.UNSPECIFIED.);
#1153=B_SPLINE_CURVE_WITH_KNOTS('',3,(#63630,#63631,#63632,#63633,#63634,
#63635),.UNSPECIFIED.,.F.,.F.,(4,2,4),(-0.0184034934971486,-0.00920171804671571,
0.),.UNSPECIFIED.);
#1154=B_SPLINE_CURVE_WITH_KNOTS('',3,(#63641,#63642,#63643,#63644,#63645,
#63646),.UNSPECIFIED.,.F.,.F.,(4,2,4),(-0.0184046527956429,-0.00920271228294938,
-9.9999999874853E-7),.UNSPECIFIED.);
#1155=B_SPLINE_CURVE_WITH_KNOTS('',3,(#63648,#63649,#63650,#63651,#63652,
#63653),.UNSPECIFIED.,.F.,.F.,(4,2,4),(-0.0184034934960222,-0.00920121807191662,
0.),.UNSPECIFIED.);
#1156=B_SPLINE_CURVE_WITH_KNOTS('',3,(#63659,#63660,#63661,#63662,#63663,
#63664),.UNSPECIFIED.,.F.,.F.,(4,2,4),(-0.0184046552623352,-0.00920321307304284,
-9.99999995192347E-7),.UNSPECIFIED.);
#1157=B_SPLINE_CURVE_WITH_KNOTS('',3,(#63666,#63667,#63668,#63669,#63670,
#63671),.UNSPECIFIED.,.F.,.F.,(4,2,4),(-0.0184034950209319,-0.00920171905609732,
0.),.UNSPECIFIED.);
#1158=B_SPLINE_CURVE_WITH_KNOTS('',3,(#63677,#63678,#63679,#63680,#63681,
#63682),.UNSPECIFIED.,.F.,.F.,(4,2,4),(-0.0184046552624292,-0.00920321307301334,
-9.99999998405054E-7),.UNSPECIFIED.);
#1159=B_SPLINE_CURVE_WITH_KNOTS('',3,(#63684,#63685,#63686,#63687,#63688,
#63689),.UNSPECIFIED.,.F.,.F.,(4,2,4),(-0.0184034922316533,-0.00920121723059212,
0.),.UNSPECIFIED.);
#1160=B_SPLINE_CURVE_WITH_KNOTS('',3,(#63695,#63696,#63697,#63698,#63699,
#63700),.UNSPECIFIED.,.F.,.F.,(4,2,4),(-0.0184046538159848,-0.00920321259746976,
-9.99999995355411E-7),.UNSPECIFIED.);
#1161=B_SPLINE_CURVE_WITH_KNOTS('',3,(#63702,#63703,#63704,#63705,#63706,
#63707),.UNSPECIFIED.,.F.,.F.,(4,2,4),(-0.0184034935073226,-0.00920121807649925,
0.),.UNSPECIFIED.);
#1162=B_SPLINE_CURVE_WITH_KNOTS('',3,(#63713,#63714,#63715,#63716,#63717,
#63718),.UNSPECIFIED.,.F.,.F.,(4,2,4),(-0.0184046538140245,-0.00920321259680655,
-9.99999999765078E-7),.UNSPECIFIED.);
#1163=B_SPLINE_CURVE_WITH_KNOTS('',3,(#63720,#63721,#63722,#63723,#63724,
#63725),.UNSPECIFIED.,.F.,.F.,(4,2,4),(-0.0184034922241276,-0.0092017172013849,
0.),.UNSPECIFIED.);
#1164=B_SPLINE_CURVE_WITH_KNOTS('',3,(#63731,#63732,#63733,#63734,#63735,
#63736),.UNSPECIFIED.,.F.,.F.,(4,2,4),(-0.0184046552624612,-0.009203213073035,
-9.99999994151513E-7),.UNSPECIFIED.);
#1165=B_SPLINE_CURVE_WITH_KNOTS('',3,(#63738,#63739,#63740,#63741,#63742,
#63743),.UNSPECIFIED.,.F.,.F.,(4,2,4),(-0.018403495013842,-0.00920171905315888,
0.),.UNSPECIFIED.);
#1166=B_SPLINE_CURVE_WITH_KNOTS('',3,(#63749,#63750,#63751,#63752,#63753,
#63754),.UNSPECIFIED.,.F.,.F.,(4,2,4),(-0.0184046538158014,-0.00920321259735261,
-9.99999998127499E-7),.UNSPECIFIED.);
#1167=B_SPLINE_CURVE_WITH_KNOTS('',3,(#63756,#63757,#63758,#63759,#63760,
#63761),.UNSPECIFIED.,.F.,.F.,(4,2,4),(-0.0184034935026953,-0.00920121807403472,
0.),.UNSPECIFIED.);
#1168=B_SPLINE_CURVE_WITH_KNOTS('',3,(#63767,#63768,#63769,#63770,#63771,
#63772),.UNSPECIFIED.,.F.,.F.,(4,2,4),(-0.018404655262374,-0.00920271309393877,
-1.00000000437944E-6),.UNSPECIFIED.);
#1169=B_SPLINE_CURVE_WITH_KNOTS('',3,(#63774,#63775,#63776,#63777,#63778,
#63779),.UNSPECIFIED.,.F.,.F.,(4,2,4),(-0.0184034922298959,-0.00920171720445481,
0.),.UNSPECIFIED.);
#1170=B_SPLINE_CURVE_WITH_KNOTS('',3,(#63785,#63786,#63787,#63788,#63789,
#63790),.UNSPECIFIED.,.F.,.F.,(4,2,4),(-0.0184046538164437,-0.00920321259763748,
-9.99999998085865E-7),.UNSPECIFIED.);
#1171=B_SPLINE_CURVE_WITH_KNOTS('',3,(#63792,#63793,#63794,#63795,#63796,
#63797),.UNSPECIFIED.,.F.,.F.,(4,2,4),(-0.0184034922283115,-0.00920121722873323,
0.),.UNSPECIFIED.);
#1172=B_SPLINE_CURVE_WITH_KNOTS('',3,(#63803,#63804,#63805,#63806,#63807,
#63808),.UNSPECIFIED.,.F.,.F.,(4,2,4),(-0.0184046552620133,-0.0092027130938019,
-1.00000000659958E-6),.UNSPECIFIED.);
#1173=B_SPLINE_CURVE_WITH_KNOTS('',3,(#63810,#63811,#63812,#63813,#63814,
#63815),.UNSPECIFIED.,.F.,.F.,(4,2,4),(-0.0184034950211358,-0.00920121908139663,
0.),.UNSPECIFIED.);
#1174=B_SPLINE_CURVE_WITH_KNOTS('',3,(#63821,#63822,#63823,#63824,#63825,
#63826),.UNSPECIFIED.,.F.,.F.,(4,2,4),(-0.0184046552623167,-0.00920321307295721,
-9.99999992049028E-7),.UNSPECIFIED.);
#1175=B_SPLINE_CURVE_WITH_KNOTS('',3,(#63828,#63829,#63830,#63831,#63832,
#63833),.UNSPECIFIED.,.F.,.F.,(4,2,4),(-0.018403495020376,-0.00920171905578727,
0.),.UNSPECIFIED.);
#1176=B_SPLINE_CURVE_WITH_KNOTS('',3,(#63839,#63840,#63841,#63842,#63843,
#63844),.UNSPECIFIED.,.F.,.F.,(4,2,4),(-0.0184046552623086,-0.00920321307293521,
-9.99999992045558E-7),.UNSPECIFIED.);
#1177=B_SPLINE_CURVE_WITH_KNOTS('',3,(#63846,#63847,#63848,#63849,#63850,
#63851),.UNSPECIFIED.,.F.,.F.,(4,2,4),(-0.0184034950217447,-0.00920121908163889,
0.),.UNSPECIFIED.);
#1178=B_SPLINE_CURVE_WITH_KNOTS('',3,(#63857,#63858,#63859,#63860,#63861,
#63862),.UNSPECIFIED.,.F.,.F.,(4,2,4),(-0.0184046538153619,-0.00920321259730723,
-9.99999998842205E-7),.UNSPECIFIED.);
#1179=B_SPLINE_CURVE_WITH_KNOTS('',3,(#63864,#63865,#63866,#63867,#63868,
#63869),.UNSPECIFIED.,.F.,.F.,(4,2,4),(-0.018403492225561,-0.00920171720238882,
0.),.UNSPECIFIED.);
#1180=B_SPLINE_CURVE_WITH_KNOTS('',3,(#63875,#63876,#63877,#63878,#63879,
#63880),.UNSPECIFIED.,.F.,.F.,(4,2,4),(-0.0184046552621458,-0.00920321307288206,
-9.99999994595602E-7),.UNSPECIFIED.);
#1181=B_SPLINE_CURVE_WITH_KNOTS('',3,(#63882,#63883,#63884,#63885,#63886,
#63887),.UNSPECIFIED.,.F.,.F.,(4,2,4),(-0.0184034922345392,-0.0092017172066897,
0.),.UNSPECIFIED.);
#1182=B_SPLINE_CURVE_WITH_KNOTS('',3,(#63893,#63894,#63895,#63896,#63897,
#63898),.UNSPECIFIED.,.F.,.F.,(4,2,4),(-0.0184046552622753,-0.00920321307294581,
-9.9999999906078E-7),.UNSPECIFIED.);
#1183=B_SPLINE_CURVE_WITH_KNOTS('',3,(#63900,#63901,#63902,#63903,#63904,
#63905),.UNSPECIFIED.,.F.,.F.,(4,2,4),(-0.0184034950134852,-0.00920121907819735,
0.),.UNSPECIFIED.);
#1184=B_SPLINE_CURVE_WITH_KNOTS('',3,(#63911,#63912,#63913,#63914,#63915,
#63916),.UNSPECIFIED.,.F.,.F.,(4,2,4),(-0.0184046552618532,-0.0092032130728355,
-9.99999998443218E-7),.UNSPECIFIED.);
#1185=B_SPLINE_CURVE_WITH_KNOTS('',3,(#63918,#63919,#63920,#63921,#63922,
#63923),.UNSPECIFIED.,.F.,.F.,(4,2,4),(-0.0184034950182595,-0.00920121908026001,
0.),.UNSPECIFIED.);
#1186=B_SPLINE_CURVE_WITH_KNOTS('',3,(#63929,#63930,#63931,#63932,#63933,
#63934),.UNSPECIFIED.,.F.,.F.,(4,2,4),(-0.0184046552615148,-0.00920321307277643,
-9.9999999743014E-7),.UNSPECIFIED.);
#1187=B_SPLINE_CURVE_WITH_KNOTS('',3,(#63936,#63937,#63938,#63939,#63940,
#63941),.UNSPECIFIED.,.F.,.F.,(4,2,4),(-0.0184034935070808,-0.00920121807681914,
0.),.UNSPECIFIED.);
#1188=B_SPLINE_CURVE_WITH_KNOTS('',3,(#63947,#63948,#63949,#63950,#63951,
#63952),.UNSPECIFIED.,.F.,.F.,(4,2,4),(-0.0184046538151697,-0.0092027126181944,
-9.99999999591605E-7),.UNSPECIFIED.);
#1189=B_SPLINE_CURVE_WITH_KNOTS('',3,(#63954,#63955,#63956,#63957,#63958,
#63959),.UNSPECIFIED.,.F.,.F.,(4,2,4),(-0.0184034935055579,-0.00920171805030441,
0.),.UNSPECIFIED.);
#1190=B_SPLINE_CURVE_WITH_KNOTS('',3,(#63965,#63966,#63967,#63968,#63969,
#63970),.UNSPECIFIED.,.F.,.F.,(4,2,4),(-0.0184046552616214,-0.00920321307281472,
-9.99999998259338E-7),.UNSPECIFIED.);
#1191=B_SPLINE_CURVE_WITH_KNOTS('',3,(#63972,#63973,#63974,#63975,#63976,
#63977),.UNSPECIFIED.,.F.,.F.,(4,2,4),(-0.0184034950180823,-0.00920171905488093,
0.),.UNSPECIFIED.);
#1192=B_SPLINE_CURVE_WITH_KNOTS('',3,(#63983,#63984,#63985,#63986,#63987,
#63988),.UNSPECIFIED.,.F.,.F.,(4,2,4),(-0.0184046552617036,-0.00920321307280033,
-9.99999998373829E-7),.UNSPECIFIED.);
#1193=B_SPLINE_CURVE_WITH_KNOTS('',3,(#63990,#63991,#63992,#63993,#63994,
#63995),.UNSPECIFIED.,.F.,.F.,(4,2,4),(-0.018403495017296,-0.00920171905455372,
0.),.UNSPECIFIED.);
#1194=B_SPLINE_CURVE_WITH_KNOTS('',3,(#64001,#64002,#64003,#64004,#64005,
#64006),.UNSPECIFIED.,.F.,.F.,(4,2,4),(-0.018404652798285,-0.0092027122837556,
-9.99999999265477E-7),.UNSPECIFIED.);
#1195=B_SPLINE_CURVE_WITH_KNOTS('',3,(#64008,#64009,#64010,#64011,#64012,
#64013),.UNSPECIFIED.,.F.,.F.,(4,2,4),(-0.0184034950141069,-0.00920121907865255,
0.),.UNSPECIFIED.);
#1196=B_SPLINE_CURVE_WITH_KNOTS('',3,(#64019,#64020,#64021,#64022,#64023,
#64024),.UNSPECIFIED.,.F.,.F.,(4,2,4),(-0.018404655262912,-0.00920271309410598,
-9.9999999990559E-7),.UNSPECIFIED.);
#1197=B_SPLINE_CURVE_WITH_KNOTS('',3,(#64026,#64027,#64028,#64029,#64030,
#64031),.UNSPECIFIED.,.F.,.F.,(4,2,4),(-0.0184034935030653,-0.00920121807424569,
0.),.UNSPECIFIED.);
#1198=B_SPLINE_CURVE_WITH_KNOTS('',3,(#64037,#64038,#64039,#64040,#64041,
#64042),.UNSPECIFIED.,.F.,.F.,(4,2,4),(-0.0184046538166818,-0.00920321259763074,
-9.99999998269746E-7),.UNSPECIFIED.);
#1199=B_SPLINE_CURVE_WITH_KNOTS('',3,(#64044,#64045,#64046,#64047,#64048,
#64049),.UNSPECIFIED.,.F.,.F.,(4,2,4),(-0.0184034935060984,-0.00920171805076214,
0.),.UNSPECIFIED.);
#1200=B_SPLINE_CURVE_WITH_KNOTS('',3,(#64055,#64056,#64057,#64058,#64059,
#64060),.UNSPECIFIED.,.F.,.F.,(4,2,4),(-0.0184046552627787,-0.00920271309404019,
-1.00000000020223E-6),.UNSPECIFIED.);
#1201=B_SPLINE_CURVE_WITH_KNOTS('',3,(#64062,#64063,#64064,#64065,#64066,
#64067),.UNSPECIFIED.,.F.,.F.,(4,2,4),(-0.0184034950154033,-0.00920121907917747,
0.),.UNSPECIFIED.);
#1202=B_SPLINE_CURVE_WITH_KNOTS('',3,(#64073,#64074,#64075,#64076,#64077,
#64078),.UNSPECIFIED.,.F.,.F.,(4,2,4),(-0.0184046527954837,-0.00920271228290404,
-9.99999998804041E-7),.UNSPECIFIED.);
#1203=B_SPLINE_CURVE_WITH_KNOTS('',3,(#64080,#64081,#64082,#64083,#64084,
#64085),.UNSPECIFIED.,.F.,.F.,(4,2,4),(-0.0184034922305112,-0.00920171720460419,
0.),.UNSPECIFIED.);
#1204=B_SPLINE_CURVE_WITH_KNOTS('',3,(#64091,#64092,#64093,#64094,#64095,
#64096),.UNSPECIFIED.,.F.,.F.,(4,2,4),(-0.0184046538149872,-0.00920271261810088,
-9.99999999161394E-7),.UNSPECIFIED.);
#1205=B_SPLINE_CURVE_WITH_KNOTS('',3,(#64098,#64099,#64100,#64101,#64102,
#64103),.UNSPECIFIED.,.F.,.F.,(4,2,4),(-0.0184034950171307,-0.00920121907998442,
0.),.UNSPECIFIED.);
#1206=B_SPLINE_CURVE_WITH_KNOTS('',3,(#64109,#64110,#64111,#64112,#64113,
#64114),.UNSPECIFIED.,.F.,.F.,(4,2,4),(-0.0184046552620757,-0.00920271309386517,
-9.99999998351278E-7),.UNSPECIFIED.);
#1207=B_SPLINE_CURVE_WITH_KNOTS('',3,(#64116,#64117,#64118,#64119,#64120,
#64121),.UNSPECIFIED.,.F.,.F.,(4,2,4),(-0.0184034950179269,-0.00920121908024188,
0.),.UNSPECIFIED.);
#1208=B_SPLINE_CURVE_WITH_KNOTS('',3,(#64127,#64128,#64129,#64130,#64131,
#64132),.UNSPECIFIED.,.F.,.F.,(4,2,4),(-0.0184046552620944,-0.00920321307293593,
-9.99999996004197E-7),.UNSPECIFIED.);
#1209=B_SPLINE_CURVE_WITH_KNOTS('',3,(#64134,#64135,#64136,#64137,#64138,
#64139),.UNSPECIFIED.,.F.,.F.,(4,2,4),(-0.018403495018241,-0.00920121908043562,
0.),.UNSPECIFIED.);
#1210=B_SPLINE_CURVE_WITH_KNOTS('',3,(#64145,#64146,#64147,#64148,#64149,
#64150),.UNSPECIFIED.,.F.,.F.,(4,2,4),(-0.0184046552624699,-0.00920271309392275,
-9.99999999333132E-7),.UNSPECIFIED.);
#1211=B_SPLINE_CURVE_WITH_KNOTS('',3,(#64152,#64153,#64154,#64155,#64156,
#64157),.UNSPECIFIED.,.F.,.F.,(4,2,4),(-0.0184034935021887,-0.00920171804868947,
0.),.UNSPECIFIED.);
#1212=B_SPLINE_CURVE_WITH_KNOTS('',3,(#64163,#64164,#64165,#64166,#64167,
#64168),.UNSPECIFIED.,.F.,.F.,(4,2,4),(-0.018404655261847,-0.00920321307284733,
-9.9999999673972E-7),.UNSPECIFIED.);
#1213=B_SPLINE_CURVE_WITH_KNOTS('',3,(#64170,#64171,#64172,#64173,#64174,
#64175),.UNSPECIFIED.,.F.,.F.,(4,2,4),(-0.0184034950156038,-0.00920171905399093,
0.),.UNSPECIFIED.);
#1214=B_SPLINE_CURVE_WITH_KNOTS('',3,(#64181,#64182,#64183,#64184,#64185,
#64186),.UNSPECIFIED.,.F.,.F.,(4,2,4),(-0.0184046552619265,-0.00920271309381794,
-1.00000000422852E-6),.UNSPECIFIED.);
#1215=B_SPLINE_CURVE_WITH_KNOTS('',3,(#64188,#64189,#64190,#64191,#64192,
#64193),.UNSPECIFIED.,.F.,.F.,(4,2,4),(-0.0184034935053294,-0.00920171805006122,
0.),.UNSPECIFIED.);
#1216=B_SPLINE_CURVE_WITH_KNOTS('',3,(#64199,#64200,#64201,#64202,#64203,
#64204),.UNSPECIFIED.,.F.,.F.,(4,2,4),(-0.0184046552617174,-0.0092027130937688,
-1.0000000028737E-6),.UNSPECIFIED.);
#1217=B_SPLINE_CURVE_WITH_KNOTS('',3,(#64206,#64207,#64208,#64209,#64210,
#64211),.UNSPECIFIED.,.F.,.F.,(4,2,4),(-0.0184034935071716,-0.00920121807651139,
0.),.UNSPECIFIED.);
#1218=B_SPLINE_CURVE_WITH_KNOTS('',3,(#64217,#64218,#64219,#64220,#64221,
#64222),.UNSPECIFIED.,.F.,.F.,(4,2,4),(-0.0184046552619574,-0.00920321307285213,
-9.99999993825385E-7),.UNSPECIFIED.);
#1219=B_SPLINE_CURVE_WITH_KNOTS('',3,(#64224,#64225,#64226,#64227,#64228,
#64229),.UNSPECIFIED.,.F.,.F.,(4,2,4),(-0.0184034950150159,-0.0092012190789793,
0.),.UNSPECIFIED.);
#1220=B_SPLINE_CURVE_WITH_KNOTS('',3,(#64235,#64236,#64237,#64238,#64239,
#64240),.UNSPECIFIED.,.F.,.F.,(4,2,4),(-0.0184046538169765,-0.00920321259774155,
-9.99999998980983E-7),.UNSPECIFIED.);
#1221=B_SPLINE_CURVE_WITH_KNOTS('',3,(#64242,#64243,#64244,#64245,#64246,
#64247),.UNSPECIFIED.,.F.,.F.,(4,2,4),(-0.0184034922295949,-0.00920171720370545,
0.),.UNSPECIFIED.);
#1222=B_SPLINE_CURVE_WITH_KNOTS('',3,(#64253,#64254,#64255,#64256,#64257,
#64258),.UNSPECIFIED.,.F.,.F.,(4,2,4),(-0.0184046552619846,-0.00920321307289419,
-9.99999994213963E-7),.UNSPECIFIED.);
#1223=B_SPLINE_CURVE_WITH_KNOTS('',3,(#64260,#64261,#64262,#64263,#64264,
#64265),.UNSPECIFIED.,.F.,.F.,(4,2,4),(-0.0184034950135014,-0.00920121907842531,
0.),.UNSPECIFIED.);
#1224=B_SPLINE_CURVE_WITH_KNOTS('',3,(#64271,#64272,#64273,#64274,#64275,
#64276),.UNSPECIFIED.,.F.,.F.,(4,2,4),(-0.0184046552620079,-0.00920321307288379,
-9.99999996600942E-7),.UNSPECIFIED.);
#1225=B_SPLINE_CURVE_WITH_KNOTS('',3,(#64278,#64279,#64280,#64281,#64282,
#64283),.UNSPECIFIED.,.F.,.F.,(4,2,4),(-0.0184034934973619,-0.00920121807230492,
0.),.UNSPECIFIED.);
#1226=B_SPLINE_CURVE_WITH_KNOTS('',3,(#64289,#64290,#64291,#64292,#64293,
#64294),.UNSPECIFIED.,.F.,.F.,(4,2,4),(-0.0184046552621581,-0.00920271309384943,
-1.00000000408974E-6),.UNSPECIFIED.);
#1227=B_SPLINE_CURVE_WITH_KNOTS('',3,(#64296,#64297,#64298,#64299,#64300,
#64301),.UNSPECIFIED.,.F.,.F.,(4,2,4),(-0.0184034935033682,-0.00920171804998622,
0.),.UNSPECIFIED.);
#1228=B_SPLINE_CURVE_WITH_KNOTS('',3,(#64307,#64308,#64309,#64310,#64311,
#64312),.UNSPECIFIED.,.F.,.F.,(4,2,4),(-0.0184046552616837,-0.00920271309374225,
-1.0000000056235E-6),.UNSPECIFIED.);
#1229=B_SPLINE_CURVE_WITH_KNOTS('',3,(#64314,#64315,#64316,#64317,#64318,
#64319),.UNSPECIFIED.,.F.,.F.,(4,2,4),(-0.0184034922272409,-0.0092012172282045,
0.),.UNSPECIFIED.);
#1230=B_SPLINE_CURVE_WITH_KNOTS('',3,(#64325,#64326,#64327,#64328,#64329,
#64330),.UNSPECIFIED.,.F.,.F.,(4,2,4),(-0.01840465526186,-0.00920321307287029,
-9.99999999317519E-7),.UNSPECIFIED.);
#1231=B_SPLINE_CURVE_WITH_KNOTS('',3,(#64332,#64333,#64334,#64335,#64336,
#64337),.UNSPECIFIED.,.F.,.F.,(4,2,4),(-0.0184034950163261,-0.00920121907951736,
0.),.UNSPECIFIED.);
#1232=B_SPLINE_CURVE_WITH_KNOTS('',3,(#64343,#64344,#64345,#64346,#64347,
#64348),.UNSPECIFIED.,.F.,.F.,(4,2,4),(-0.0184046527928335,-0.00920321226108215,
-9.99999998651385E-7),.UNSPECIFIED.);
#1233=B_SPLINE_CURVE_WITH_KNOTS('',3,(#64350,#64351,#64352,#64353,#64354,
#64355),.UNSPECIFIED.,.F.,.F.,(4,2,4),(-0.0184034935007121,-0.0092012180734001,
0.),.UNSPECIFIED.);
#1234=B_SPLINE_CURVE_WITH_KNOTS('',3,(#64361,#64362,#64363,#64364,#64365,
#64366),.UNSPECIFIED.,.F.,.F.,(4,2,4),(-0.01840465526219,-0.00920271309386883,
-1.0000000022093E-6),.UNSPECIFIED.);
#1235=B_SPLINE_CURVE_WITH_KNOTS('',3,(#64368,#64369,#64370,#64371,#64372,
#64373),.UNSPECIFIED.,.F.,.F.,(4,2,4),(-0.0184034950219852,-0.00920171905652633,
0.),.UNSPECIFIED.);
#1236=B_SPLINE_CURVE_WITH_KNOTS('',3,(#64379,#64380,#64381,#64382,#64383,
#64384),.UNSPECIFIED.,.F.,.F.,(4,2,4),(-0.0184046538120481,-0.00920321259614537,
-9.9999999918915E-7),.UNSPECIFIED.);
#1237=B_SPLINE_CURVE_WITH_KNOTS('',3,(#64386,#64387,#64388,#64389,#64390,
#64391),.UNSPECIFIED.,.F.,.F.,(4,2,4),(-0.0184034950175798,-0.00920171905480655,
0.),.UNSPECIFIED.);
#1238=B_SPLINE_CURVE_WITH_KNOTS('',3,(#64397,#64398,#64399,#64400,#64401,
#64402),.UNSPECIFIED.,.F.,.F.,(4,2,4),(-0.0184046552618216,-0.00920271309381456,
-9.99999998805776E-7),.UNSPECIFIED.);
#1239=B_SPLINE_CURVE_WITH_KNOTS('',3,(#64404,#64405,#64406,#64407,#64408,
#64409),.UNSPECIFIED.,.F.,.F.,(4,2,4),(-0.0184034950228819,-0.00920171905700514,
0.),.UNSPECIFIED.);
#1240=B_SPLINE_CURVE_WITH_KNOTS('',3,(#64415,#64416,#64417,#64418,#64419,
#64420),.UNSPECIFIED.,.F.,.F.,(4,2,4),(-0.0184046552095742,-0.00920271305842647,
-9.9999999915099E-7),.UNSPECIFIED.);
#1241=B_SPLINE_CURVE_WITH_KNOTS('',3,(#64422,#64423,#64424,#64425,#64426,
#64427),.UNSPECIFIED.,.F.,.F.,(4,2,4),(-0.0184034935059472,-0.00920171805058506,
0.),.UNSPECIFIED.);
#1242=B_SPLINE_CURVE_WITH_KNOTS('',3,(#64432,#64433,#64434,#64435,#64436,
#64437),.UNSPECIFIED.,.F.,.F.,(4,2,4),(-0.01840465254103,-0.00920271218116683,
-9.99999999315784E-7),.UNSPECIFIED.);
#1243=B_SPLINE_CURVE_WITH_KNOTS('',3,(#64441,#64442,#64443,#64444),
 .UNSPECIFIED.,.F.,.F.,(4,4),(0.0165621619175432,0.0219133296771791),
 .UNSPECIFIED.);
#1244=B_SPLINE_CURVE_WITH_KNOTS('',3,(#64449,#64450,#64451,#64452,#64453,
#64454),.UNSPECIFIED.,.F.,.F.,(4,2,4),(9.99962477529338E-7,0.0105693184169416,
0.0165621619175432),.UNSPECIFIED.);
#1245=B_SPLINE_CURVE_WITH_KNOTS('',3,(#64464,#64465,#64466,#64467),
 .UNSPECIFIED.,.F.,.F.,(4,4),(4.75255497207553,4.76308887897647),
 .UNSPECIFIED.);
#1246=B_SPLINE_CURVE_WITH_KNOTS('',3,(#64479,#64480,#64481,#64482),
 .UNSPECIFIED.,.F.,.F.,(4,4),(4.75255497207216,4.76308887897314),
 .UNSPECIFIED.);
#1247=B_SPLINE_CURVE_WITH_KNOTS('',3,(#64494,#64495,#64496,#64497),
 .UNSPECIFIED.,.F.,.F.,(4,4),(4.75255497206109,4.7630888789621),
 .UNSPECIFIED.);
#1248=B_SPLINE_CURVE_WITH_KNOTS('',3,(#64509,#64510,#64511,#64512),
 .UNSPECIFIED.,.F.,.F.,(4,4),(4.75255497207336,4.76308887897441),
 .UNSPECIFIED.);
#1249=B_SPLINE_CURVE_WITH_KNOTS('',3,(#64524,#64525,#64526,#64527),
 .UNSPECIFIED.,.F.,.F.,(4,4),(4.7525549721169,4.763088879018),
 .UNSPECIFIED.);
#1250=B_SPLINE_CURVE_WITH_KNOTS('',3,(#64539,#64540,#64541,#64542),
 .UNSPECIFIED.,.F.,.F.,(4,4),(4.75255497216149,4.76308887906267),
 .UNSPECIFIED.);
#1251=B_SPLINE_CURVE_WITH_KNOTS('',3,(#64554,#64555,#64556,#64557),
 .UNSPECIFIED.,.F.,.F.,(4,4),(4.75255497220882,4.76308887911007),
 .UNSPECIFIED.);
#1252=B_SPLINE_CURVE_WITH_KNOTS('',3,(#64569,#64570,#64571,#64572),
 .UNSPECIFIED.,.F.,.F.,(4,4),(4.75255497220738,4.76308887910871),
 .UNSPECIFIED.);
#1253=B_SPLINE_CURVE_WITH_KNOTS('',3,(#64584,#64585,#64586,#64587),
 .UNSPECIFIED.,.F.,.F.,(4,4),(4.75255497208619,4.7630888789876),
 .UNSPECIFIED.);
#1254=B_SPLINE_CURVE_WITH_KNOTS('',3,(#64599,#64600,#64601,#64602),
 .UNSPECIFIED.,.F.,.F.,(4,4),(4.75255497206892,4.76308887897041),
 .UNSPECIFIED.);
#1255=B_SPLINE_CURVE_WITH_KNOTS('',3,(#64614,#64615,#64616,#64617),
 .UNSPECIFIED.,.F.,.F.,(4,4),(4.75255497207531,4.7630888789769),
 .UNSPECIFIED.);
#1256=B_SPLINE_CURVE_WITH_KNOTS('',3,(#64629,#64630,#64631,#64632),
 .UNSPECIFIED.,.F.,.F.,(4,4),(4.75255497209236,4.76308887899405),
 .UNSPECIFIED.);
#1257=B_SPLINE_CURVE_WITH_KNOTS('',3,(#64644,#64645,#64646,#64647),
 .UNSPECIFIED.,.F.,.F.,(4,4),(4.75255497206474,4.76308887896652),
 .UNSPECIFIED.);
#1258=B_SPLINE_CURVE_WITH_KNOTS('',3,(#64659,#64660,#64661,#64662),
 .UNSPECIFIED.,.F.,.F.,(4,4),(4.75255497207158,4.76308887897344),
 .UNSPECIFIED.);
#1259=B_SPLINE_CURVE_WITH_KNOTS('',3,(#64674,#64675,#64676,#64677),
 .UNSPECIFIED.,.F.,.F.,(4,4),(4.75255497208885,4.76308887899078),
 .UNSPECIFIED.);
#1260=B_SPLINE_CURVE_WITH_KNOTS('',3,(#64689,#64690,#64691,#64692),
 .UNSPECIFIED.,.F.,.F.,(4,4),(4.75255497206809,4.76308887897013),
 .UNSPECIFIED.);
#1261=B_SPLINE_CURVE_WITH_KNOTS('',3,(#64704,#64705,#64706,#64707),
 .UNSPECIFIED.,.F.,.F.,(4,4),(4.75255497207646,4.76308887897857),
 .UNSPECIFIED.);
#1262=B_SPLINE_CURVE_WITH_KNOTS('',3,(#64719,#64720,#64721,#64722),
 .UNSPECIFIED.,.F.,.F.,(4,4),(4.75255497207436,4.76308887897653),
 .UNSPECIFIED.);
#1263=B_SPLINE_CURVE_WITH_KNOTS('',3,(#64734,#64735,#64736,#64737),
 .UNSPECIFIED.,.F.,.F.,(4,4),(4.75255497208078,4.763088878983),
 .UNSPECIFIED.);
#1264=B_SPLINE_CURVE_WITH_KNOTS('',3,(#64749,#64750,#64751,#64752),
 .UNSPECIFIED.,.F.,.F.,(4,4),(4.75255497227339,4.76308887917565),
 .UNSPECIFIED.);
#1265=B_SPLINE_CURVE_WITH_KNOTS('',3,(#64764,#64765,#64766,#64767),
 .UNSPECIFIED.,.F.,.F.,(4,4),(4.75255497224816,4.76308887915048),
 .UNSPECIFIED.);
#1266=B_SPLINE_CURVE_WITH_KNOTS('',3,(#64779,#64780,#64781,#64782),
 .UNSPECIFIED.,.F.,.F.,(4,4),(4.75255497220241,4.76308887910477),
 .UNSPECIFIED.);
#1267=B_SPLINE_CURVE_WITH_KNOTS('',3,(#64794,#64795,#64796,#64797),
 .UNSPECIFIED.,.F.,.F.,(4,4),(4.75255497215918,4.76308887906153),
 .UNSPECIFIED.);
#1268=B_SPLINE_CURVE_WITH_KNOTS('',3,(#64809,#64810,#64811,#64812),
 .UNSPECIFIED.,.F.,.F.,(4,4),(4.752554972119,4.7630888790214),
 .UNSPECIFIED.);
#1269=B_SPLINE_CURVE_WITH_KNOTS('',3,(#64824,#64825,#64826,#64827),
 .UNSPECIFIED.,.F.,.F.,(4,4),(4.75255497209406,4.76308887915569),
 .UNSPECIFIED.);
#1270=B_SPLINE_CURVE_WITH_KNOTS('',3,(#64839,#64840,#64841,#64842),
 .UNSPECIFIED.,.F.,.F.,(4,4),(4.75255497213315,4.76308887903548),
 .UNSPECIFIED.);
#1271=B_SPLINE_CURVE_WITH_KNOTS('',3,(#64854,#64855,#64856,#64857),
 .UNSPECIFIED.,.F.,.F.,(4,4),(4.75255497214093,4.76308887904322),
 .UNSPECIFIED.);
#1272=B_SPLINE_CURVE_WITH_KNOTS('',3,(#64869,#64870,#64871,#64872),
 .UNSPECIFIED.,.F.,.F.,(4,4),(4.75255497222018,4.76308887912243),
 .UNSPECIFIED.);
#1273=B_SPLINE_CURVE_WITH_KNOTS('',3,(#64884,#64885,#64886,#64887),
 .UNSPECIFIED.,.F.,.F.,(4,4),(4.75255497202817,4.76308887893043),
 .UNSPECIFIED.);
#1274=B_SPLINE_CURVE_WITH_KNOTS('',3,(#64899,#64900,#64901,#64902),
 .UNSPECIFIED.,.F.,.F.,(4,4),(4.75255497204426,4.76308887894642),
 .UNSPECIFIED.);
#1275=B_SPLINE_CURVE_WITH_KNOTS('',3,(#64914,#64915,#64916,#64917),
 .UNSPECIFIED.,.F.,.F.,(4,4),(4.75255497203009,4.76308887893217),
 .UNSPECIFIED.);
#1276=B_SPLINE_CURVE_WITH_KNOTS('',3,(#64929,#64930,#64931,#64932),
 .UNSPECIFIED.,.F.,.F.,(4,4),(4.7525549720349,4.76308887893693),
 .UNSPECIFIED.);
#1277=B_SPLINE_CURVE_WITH_KNOTS('',3,(#64944,#64945,#64946,#64947),
 .UNSPECIFIED.,.F.,.F.,(4,4),(4.75255497200156,4.76308887890348),
 .UNSPECIFIED.);
#1278=B_SPLINE_CURVE_WITH_KNOTS('',3,(#64959,#64960,#64961,#64962),
 .UNSPECIFIED.,.F.,.F.,(4,4),(4.75255497203018,4.76308887893203),
 .UNSPECIFIED.);
#1279=B_SPLINE_CURVE_WITH_KNOTS('',3,(#64974,#64975,#64976,#64977),
 .UNSPECIFIED.,.F.,.F.,(4,4),(4.75255497199264,4.7630888788944),
 .UNSPECIFIED.);
#1280=B_SPLINE_CURVE_WITH_KNOTS('',3,(#64989,#64990,#64991,#64992),
 .UNSPECIFIED.,.F.,.F.,(4,4),(4.75255497198854,4.76308887889023),
 .UNSPECIFIED.);
#1281=B_SPLINE_CURVE_WITH_KNOTS('',3,(#65004,#65005,#65006,#65007),
 .UNSPECIFIED.,.F.,.F.,(4,4),(4.75255497197651,4.76308887887812),
 .UNSPECIFIED.);
#1282=B_SPLINE_CURVE_WITH_KNOTS('',3,(#65019,#65020,#65021,#65022),
 .UNSPECIFIED.,.F.,.F.,(4,4),(4.75255497195996,4.76308887886144),
 .UNSPECIFIED.);
#1283=B_SPLINE_CURVE_WITH_KNOTS('',3,(#65034,#65035,#65036,#65037),
 .UNSPECIFIED.,.F.,.F.,(4,4),(4.75255497195405,4.76308887885545),
 .UNSPECIFIED.);
#1284=B_SPLINE_CURVE_WITH_KNOTS('',3,(#65049,#65050,#65051,#65052),
 .UNSPECIFIED.,.F.,.F.,(4,4),(4.75255497194695,4.76308887884825),
 .UNSPECIFIED.);
#1285=B_SPLINE_CURVE_WITH_KNOTS('',3,(#65064,#65065,#65066,#65067),
 .UNSPECIFIED.,.F.,.F.,(4,4),(4.7525549719234,4.76308887882463),
 .UNSPECIFIED.);
#1286=B_SPLINE_CURVE_WITH_KNOTS('',3,(#65079,#65080,#65081,#65082),
 .UNSPECIFIED.,.F.,.F.,(4,4),(4.75255497193489,4.76308887883606),
 .UNSPECIFIED.);
#1287=B_SPLINE_CURVE_WITH_KNOTS('',3,(#65094,#65095,#65096,#65097),
 .UNSPECIFIED.,.F.,.F.,(4,4),(4.75255497192173,4.76308887882284),
 .UNSPECIFIED.);
#1288=B_SPLINE_CURVE_WITH_KNOTS('',3,(#65109,#65110,#65111,#65112),
 .UNSPECIFIED.,.F.,.F.,(4,4),(4.75255497191409,4.76308887881513),
 .UNSPECIFIED.);
#1289=B_SPLINE_CURVE_WITH_KNOTS('',3,(#65124,#65125,#65126,#65127),
 .UNSPECIFIED.,.F.,.F.,(4,4),(4.75255497190642,4.76308887880743),
 .UNSPECIFIED.);
#1290=B_SPLINE_CURVE_WITH_KNOTS('',3,(#65139,#65140,#65141,#65142),
 .UNSPECIFIED.,.F.,.F.,(4,4),(4.75255497190071,4.76308887880165),
 .UNSPECIFIED.);
#1291=B_SPLINE_CURVE_WITH_KNOTS('',3,(#65154,#65155,#65156,#65157),
 .UNSPECIFIED.,.F.,.F.,(4,4),(4.75255497189559,4.76308887879652),
 .UNSPECIFIED.);
#1292=B_SPLINE_CURVE_WITH_KNOTS('',3,(#65169,#65170,#65171,#65172),
 .UNSPECIFIED.,.F.,.F.,(4,4),(4.75255497189571,4.76308887879664),
 .UNSPECIFIED.);
#1293=B_SPLINE_CURVE_WITH_KNOTS('',3,(#65184,#65185,#65186,#65187),
 .UNSPECIFIED.,.F.,.F.,(4,4),(4.75255497188971,4.76308887879064),
 .UNSPECIFIED.);
#1294=B_SPLINE_CURVE_WITH_KNOTS('',3,(#65198,#65199,#65200,#65201),
 .UNSPECIFIED.,.F.,.F.,(4,4),(4.75255497186513,4.76308887897258),
 .UNSPECIFIED.);
#1295=B_SPLINE_CURVE_WITH_KNOTS('',3,(#65223,#65224,#65225,#65226,#65227,
#65228,#65229),.UNSPECIFIED.,.F.,.F.,(4,3,4),(0.,0.5,0.999990117119694),
 .UNSPECIFIED.);
#1296=B_SPLINE_CURVE_WITH_KNOTS('',3,(#65252,#65253,#65254,#65255,#65256,
#65257),.UNSPECIFIED.,.F.,.F.,(4,2,4),(0.,0.0198677118939269,0.039736333875931),
 .UNSPECIFIED.);
#1297=B_SPLINE_CURVE_WITH_KNOTS('',3,(#65287,#65288,#65289,#65290,#65291,
#65292,#65293),.UNSPECIFIED.,.F.,.F.,(4,3,4),(0.,0.5,0.999990115107466),
 .UNSPECIFIED.);
#1298=B_SPLINE_CURVE_WITH_KNOTS('',3,(#65319,#65320,#65321,#65322,#65323,
#65324),.UNSPECIFIED.,.F.,.F.,(4,2,4),(0.,0.019903067966103,0.0398070346017422),
 .UNSPECIFIED.);
#1299=B_SPLINE_CURVE_WITH_KNOTS('',3,(#65346,#65347,#65348,#65349,#65350,
#65351),.UNSPECIFIED.,.F.,.F.,(4,2,4),(0.,0.0198677117249203,0.0397363335964693),
 .UNSPECIFIED.);
#1300=B_SPLINE_CURVE_WITH_KNOTS('',3,(#65375,#65376,#65377,#65378,#65379,
#65380),.UNSPECIFIED.,.F.,.F.,(4,2,4),(0.,0.0198973966006019,0.0397956843350417),
 .UNSPECIFIED.);
#1301=B_SPLINE_CURVE_WITH_KNOTS('',3,(#65453,#65454,#65455,#65456,#65457,
#65458),.UNSPECIFIED.,.F.,.F.,(4,2,4),(0.,0.0198994178811908,0.0397997368662755),
 .UNSPECIFIED.);
#1302=B_SPLINE_CURVE_WITH_KNOTS('',3,(#65475,#65476,#65477,#65478,#65479,
#65480),.UNSPECIFIED.,.F.,.F.,(4,2,4),(0.,0.0198973966005004,0.039795684334322),
 .UNSPECIFIED.);
#1303=B_SPLINE_CURVE_WITH_KNOTS('',3,(#65494,#65495,#65496,#65497,#65498,
#65499),.UNSPECIFIED.,.F.,.F.,(4,2,4),(0.,0.0198905179568995,0.0397819072566626),
 .UNSPECIFIED.);
#1304=B_SPLINE_CURVE_WITH_KNOTS('',3,(#65514,#65515,#65516,#65517,#65518,
#65519),.UNSPECIFIED.,.F.,.F.,(4,2,4),(0.,0.0199030098319572,0.0398069010941151),
 .UNSPECIFIED.);
#1305=B_SPLINE_CURVE_WITH_KNOTS('',3,(#65549,#65550,#65551,#65552,#65553,
#65554,#65555),.UNSPECIFIED.,.F.,.F.,(4,3,4),(0.0365944846647011,0.0384615384615384,
0.0431466153076602),.UNSPECIFIED.);
#1306=B_SPLINE_CURVE_WITH_KNOTS('',3,(#65557,#65558,#65559,#65560,#65561,
#65562,#65563,#65564),.UNSPECIFIED.,.F.,.F.,(4,2,2,4),(1.77350755374016E-6,
0.00863675573580245,0.0171409052851941,0.0172810535282736),
 .UNSPECIFIED.);
#1307=B_SPLINE_CURVE_WITH_KNOTS('',3,(#65606,#65607,#65608,#65609,#65610,
#65611),.UNSPECIFIED.,.F.,.F.,(4,2,4),(0.,0.0198536183249784,0.0397081496300452),
 .UNSPECIFIED.);
#1308=B_SPLINE_CURVE_WITH_KNOTS('',3,(#65628,#65629,#65630,#65631,#65632,
#65633),.UNSPECIFIED.,.F.,.F.,(4,2,4),(0.,0.0198994178801103,0.039799736862051),
 .UNSPECIFIED.);
#1309=B_SPLINE_CURVE_WITH_KNOTS('',3,(#65652,#65653,#65654,#65655,#65656,
#65657),.UNSPECIFIED.,.F.,.F.,(4,2,4),(-0.00212389296650024,-0.00106194370310601,
0.),.UNSPECIFIED.);
#1310=B_SPLINE_CURVE_WITH_KNOTS('',3,(#65658,#65659,#65660,#65661,#65662,
#65663),.UNSPECIFIED.,.F.,.F.,(4,2,4),(9.99998418911506E-7,0.0193527846137979,
0.0387045795163393),.UNSPECIFIED.);
#1311=B_SPLINE_CURVE_WITH_KNOTS('',3,(#65678,#65679,#65680,#65681,#65682,
#65683),.UNSPECIFIED.,.F.,.F.,(4,2,4),(0.,0.0198905190016668,0.0397819091577267),
 .UNSPECIFIED.);
#1312=B_SPLINE_CURVE_WITH_KNOTS('',3,(#65688,#65689,#65690,#65691,#65692,
#65693),.UNSPECIFIED.,.F.,.F.,(4,2,4),(-0.00212486200559533,-0.00106293275925874,
-9.99999998182793E-7),.UNSPECIFIED.);
#1313=B_SPLINE_CURVE_WITH_KNOTS('',3,(#65741,#65742,#65743,#65744,#65745,
#65746,#65747),.UNSPECIFIED.,.F.,.F.,(4,3,4),(0.0365944846647015,0.0384615384615384,
0.0431466153076587),.UNSPECIFIED.);
#1314=B_SPLINE_CURVE_WITH_KNOTS('',3,(#65749,#65750,#65751,#65752,#65753,
#65754,#65755,#65756),.UNSPECIFIED.,.F.,.F.,(4,2,2,4),(1.77292721144812E-6,
0.00863675579268646,0.0171409291098449,0.0172810748822113),
 .UNSPECIFIED.);
#1315=B_SPLINE_CURVE_WITH_KNOTS('',3,(#65775,#65776,#65777,#65778,#65779,
#65780),.UNSPECIFIED.,.F.,.F.,(4,2,4),(0.,0.0198583386697715,0.0397175618272593),
 .UNSPECIFIED.);
#1316=B_SPLINE_CURVE_WITH_KNOTS('',3,(#65797,#65798,#65799,#65800,#65801,
#65802),.UNSPECIFIED.,.F.,.F.,(4,2,4),(0.,0.0198536183213069,0.0397081496154716),
 .UNSPECIFIED.);
#1317=B_SPLINE_CURVE_WITH_KNOTS('',3,(#65823,#65824,#65825,#65826,#65827,
#65828),.UNSPECIFIED.,.F.,.F.,(4,2,4),(0.,0.019876258198358,0.0397534246592788),
 .UNSPECIFIED.);
#1318=B_SPLINE_CURVE_WITH_KNOTS('',3,(#65843,#65844,#65845,#65846,#65847,
#65848),.UNSPECIFIED.,.F.,.F.,(4,2,4),(-0.00212389454210504,-0.00106194431286647,
0.),.UNSPECIFIED.);
#1319=B_SPLINE_CURVE_WITH_KNOTS('',3,(#65849,#65850,#65851,#65852,#65853,
#65854),.UNSPECIFIED.,.F.,.F.,(4,2,4),(9.99998417577743E-7,0.0193522748428586,
0.038704569289107),.UNSPECIFIED.);
#1320=B_SPLINE_CURVE_WITH_KNOTS('',3,(#65866,#65867,#65868,#65869,#65870,
#65871),.UNSPECIFIED.,.F.,.F.,(4,2,4),(-0.00212486139194619,-0.00106293275903844,
-1.00000000112337E-6),.UNSPECIFIED.);
#1321=B_SPLINE_CURVE_WITH_KNOTS('',3,(#65937,#65938,#65939,#65940,#65941,
#65942),.UNSPECIFIED.,.F.,.F.,(4,2,4),(0.,0.0199008240806452,0.0398025406855435),
 .UNSPECIFIED.);
#1322=B_SPLINE_CURVE_WITH_KNOTS('',3,(#65959,#65960,#65961,#65962,#65963,
#65964),.UNSPECIFIED.,.F.,.F.,(4,2,4),(0.,0.0198583386680412,0.0397175618203158),
 .UNSPECIFIED.);
#1323=B_SPLINE_CURVE_WITH_KNOTS('',3,(#65985,#65986,#65987,#65988,#65989,
#65990),.UNSPECIFIED.,.F.,.F.,(4,2,4),(0.,0.0199042621693574,0.0398094213946847),
 .UNSPECIFIED.);
#1324=B_SPLINE_CURVE_WITH_KNOTS('',3,(#66012,#66013,#66014,#66015,#66016,
#66017),.UNSPECIFIED.,.F.,.F.,(4,2,4),(0.,0.0198762582949225,0.0397534248643712),
 .UNSPECIFIED.);
#1325=B_SPLINE_CURVE_WITH_KNOTS('',3,(#66095,#66096,#66097,#66098,#66099,
#66100),.UNSPECIFIED.,.F.,.F.,(4,2,4),(0.,0.019895479367571,0.0397918615427886),
 .UNSPECIFIED.);
#1326=B_SPLINE_CURVE_WITH_KNOTS('',3,(#66117,#66118,#66119,#66120,#66121,
#66122),.UNSPECIFIED.,.F.,.F.,(4,2,4),(0.,0.0199008240758206,0.0398025406664044),
 .UNSPECIFIED.);
#1327=B_SPLINE_CURVE_WITH_KNOTS('',3,(#66162,#66163,#66164,#66165,#66166,
#66167),.UNSPECIFIED.,.F.,.F.,(4,2,4),(0.,0.0199042621633849,0.0398094213825159),
 .UNSPECIFIED.);
#1328=B_SPLINE_CURVE_WITH_KNOTS('',3,(#66218,#66219,#66220,#66221,#66222,
#66223),.UNSPECIFIED.,.F.,.F.,(4,2,4),(0.,0.0198954793631272,0.0397918615243005),
 .UNSPECIFIED.);
#1329=B_SPLINE_CURVE_WITH_KNOTS('',3,(#66264,#66265,#66266,#66267,#66268,
#66269,#66270),.UNSPECIFIED.,.F.,.F.,(4,3,4),(0.,0.5,0.99999011712143),
 .UNSPECIFIED.);
#1330=B_SPLINE_CURVE_WITH_KNOTS('',3,(#66293,#66294,#66295,#66296,#66297,
#66298),.UNSPECIFIED.,.F.,.F.,(4,2,4),(0.,0.0198677118963707,0.0397363338857673),
 .UNSPECIFIED.);
#1331=B_SPLINE_CURVE_WITH_KNOTS('',3,(#66340,#66341,#66342,#66343,#66344,
#66345),.UNSPECIFIED.,.F.,.F.,(4,2,4),(0.,0.0198973966012806,0.0397956843374697),
 .UNSPECIFIED.);
#1332=B_SPLINE_CURVE_WITH_KNOTS('',3,(#66367,#66368,#66369,#66370,#66371,
#66372),.UNSPECIFIED.,.F.,.F.,(4,2,4),(0.,0.0199030679677246,0.0398070346083461),
 .UNSPECIFIED.);
#1333=B_SPLINE_CURVE_WITH_KNOTS('',3,(#66406,#66407,#66408,#66409,#66410,
#66411),.UNSPECIFIED.,.F.,.F.,(4,2,4),(0.,0.0198905179566254,0.039781907255294),
 .UNSPECIFIED.);
#1334=B_SPLINE_CURVE_WITH_KNOTS('',3,(#66436,#66437,#66438,#66439,#66440,
#66441),.UNSPECIFIED.,.F.,.F.,(4,2,4),(0.,0.0198994178826517,0.0397997368722785),
 .UNSPECIFIED.);
#1335=B_SPLINE_CURVE_WITH_KNOTS('',3,(#66465,#66466,#66467,#66468,#66469,
#66470,#66471),.UNSPECIFIED.,.F.,.F.,(4,3,4),(0.0365944846647268,0.0384615384615384,
0.0431466153076594),.UNSPECIFIED.);
#1336=B_SPLINE_CURVE_WITH_KNOTS('',3,(#66472,#66473,#66474,#66475,#66476,
#66477,#66478,#66479),.UNSPECIFIED.,.F.,.F.,(4,2,2,4),(1.77350715213377E-6,
0.0086367558589756,0.0171409489082422,0.0172810924755889),.UNSPECIFIED.);
#1337=B_SPLINE_CURVE_WITH_KNOTS('',3,(#66504,#66505,#66506,#66507,#66508,
#66509),.UNSPECIFIED.,.F.,.F.,(4,2,4),(0.,0.0198536183240437,0.0397081496263899),
 .UNSPECIFIED.);
#1338=B_SPLINE_CURVE_WITH_KNOTS('',3,(#66527,#66528,#66529,#66530,#66531,
#66532),.UNSPECIFIED.,.F.,.F.,(4,2,4),(-0.0021238913584622,-0.00106194304649518,
0.),.UNSPECIFIED.);
#1339=B_SPLINE_CURVE_WITH_KNOTS('',3,(#66533,#66534,#66535,#66536,#66537,
#66538),.UNSPECIFIED.,.F.,.F.,(4,2,4),(9.99998417920556E-7,0.0193527846142068,
0.0387045795170656),.UNSPECIFIED.);
#1340=B_SPLINE_CURVE_WITH_KNOTS('',3,(#66544,#66545,#66546,#66547,#66548,
#66549),.UNSPECIFIED.,.F.,.F.,(4,2,4),(-0.00212486263447062,-0.00106293275266832,
-9.99999998948673E-7),.UNSPECIFIED.);
#1341=B_SPLINE_CURVE_WITH_KNOTS('',3,(#66585,#66586,#66587,#66588,#66589,
#66590),.UNSPECIFIED.,.F.,.F.,(4,2,4),(0.,0.0198583386708035,0.0397175618316024),
 .UNSPECIFIED.);
#1342=B_SPLINE_CURVE_WITH_KNOTS('',3,(#66603,#66604,#66605,#66606,#66607,
#66608),.UNSPECIFIED.,.F.,.F.,(4,2,4),(0.,0.0198761967030548,0.0397532849661016),
 .UNSPECIFIED.);
#1343=B_SPLINE_CURVE_WITH_KNOTS('',3,(#66660,#66661,#66662,#66663,#66664,
#66665),.UNSPECIFIED.,.F.,.F.,(4,2,4),(0.,0.0199008240827659,0.0398025406936002),
 .UNSPECIFIED.);
#1344=B_SPLINE_CURVE_WITH_KNOTS('',3,(#66685,#66686,#66687,#66688,#66689,
#66690),.UNSPECIFIED.,.F.,.F.,(4,2,4),(0.,0.0199042621706517,0.0398094213994398),
 .UNSPECIFIED.);
#1345=B_SPLINE_CURVE_WITH_KNOTS('',3,(#66738,#66739,#66740,#66741,#66742,
#66743),.UNSPECIFIED.,.F.,.F.,(4,2,4),(0.,0.0198954793707845,0.0397918615553697),
 .UNSPECIFIED.);
#1346=B_SPLINE_CURVE_WITH_KNOTS('',3,(#66790,#66791,#66792,#66793,#66794,
#66795,#66796),.UNSPECIFIED.,.F.,.F.,(4,3,4),(0.,0.5,0.999990117122412),
 .UNSPECIFIED.);
#1347=B_SPLINE_CURVE_WITH_KNOTS('',3,(#66819,#66820,#66821,#66822,#66823,
#66824),.UNSPECIFIED.,.F.,.F.,(4,2,4),(0.,0.019867711898593,0.0397363338947165),
 .UNSPECIFIED.);
#1348=B_SPLINE_CURVE_WITH_KNOTS('',3,(#66866,#66867,#66868,#66869,#66870,
#66871),.UNSPECIFIED.,.F.,.F.,(4,2,4),(0.,0.0198973966022289,0.0397956843415848),
 .UNSPECIFIED.);
#1349=B_SPLINE_CURVE_WITH_KNOTS('',3,(#66893,#66894,#66895,#66896,#66897,
#66898),.UNSPECIFIED.,.F.,.F.,(4,2,4),(0.,0.0199030679688408,0.03980703461301),
 .UNSPECIFIED.);
#1350=B_SPLINE_CURVE_WITH_KNOTS('',3,(#66943,#66944,#66945,#66946,#66947,
#66948),.UNSPECIFIED.,.F.,.F.,(4,2,4),(0.,0.0198994178838214,0.0397997368769709),
 .UNSPECIFIED.);
#1351=B_SPLINE_CURVE_WITH_KNOTS('',3,(#66961,#66962,#66963,#66964,#66965,
#66966),.UNSPECIFIED.,.F.,.F.,(4,2,4),(0.,0.0198905179566607,0.0397819072561946),
 .UNSPECIFIED.);
#1352=B_SPLINE_CURVE_WITH_KNOTS('',3,(#66985,#66986,#66987,#66988,#66989,
#66990,#66991),.UNSPECIFIED.,.F.,.F.,(4,3,4),(0.036594484664701,0.0384615384615384,
0.0431466153076598),.UNSPECIFIED.);
#1353=B_SPLINE_CURVE_WITH_KNOTS('',3,(#66992,#66993,#66994,#66995,#66996,
#66997,#66998,#66999),.UNSPECIFIED.,.F.,.F.,(4,2,2,4),(1.77257448215108E-6,
0.00863675575236804,0.0171409239383189,0.0172810702978924),
 .UNSPECIFIED.);
#1354=B_SPLINE_CURVE_WITH_KNOTS('',3,(#67024,#67025,#67026,#67027,#67028,
#67029),.UNSPECIFIED.,.F.,.F.,(4,2,4),(-0.00212388996317658,-0.00106194249137579,
0.),.UNSPECIFIED.);
#1355=B_SPLINE_CURVE_WITH_KNOTS('',3,(#67030,#67031,#67032,#67033,#67034,
#67035),.UNSPECIFIED.,.F.,.F.,(4,2,4),(9.99998418160754E-7,0.0193522753881725,
0.0387045692982265),.UNSPECIFIED.);
#1356=B_SPLINE_CURVE_WITH_KNOTS('',3,(#67060,#67061,#67062,#67063,#67064,
#67065),.UNSPECIFIED.,.F.,.F.,(4,2,4),(0.,0.0198536183256091,0.039708149632394),
 .UNSPECIFIED.);
#1357=B_SPLINE_CURVE_WITH_KNOTS('',3,(#67070,#67071,#67072,#67073,#67074,
#67075),.UNSPECIFIED.,.F.,.F.,(4,2,4),(-0.00212486323669885,-0.00106293276579889,
-9.99999996992874E-7),.UNSPECIFIED.);
#1358=B_SPLINE_CURVE_WITH_KNOTS('',3,(#67114,#67115,#67116,#67117,#67118,
#67119),.UNSPECIFIED.,.F.,.F.,(4,2,4),(0.,0.0198583386720477,0.0397175618366298),
 .UNSPECIFIED.);
#1359=B_SPLINE_CURVE_WITH_KNOTS('',3,(#67132,#67133,#67134,#67135,#67136,
#67137),.UNSPECIFIED.,.F.,.F.,(4,2,4),(0.,0.0198761966979935,0.0397532849518538),
 .UNSPECIFIED.);
#1360=B_SPLINE_CURVE_WITH_KNOTS('',3,(#67189,#67190,#67191,#67192,#67193,
#67194),.UNSPECIFIED.,.F.,.F.,(4,2,4),(0.,0.0199008240838985,0.039802540698102),
 .UNSPECIFIED.);
#1361=B_SPLINE_CURVE_WITH_KNOTS('',3,(#67207,#67208,#67209,#67210,#67211,
#67212),.UNSPECIFIED.,.F.,.F.,(4,2,4),(0.,0.0199042047183892,0.039809289175465),
 .UNSPECIFIED.);
#1362=B_SPLINE_CURVE_WITH_KNOTS('',3,(#67260,#67261,#67262,#67263,#67264,
#67265),.UNSPECIFIED.,.F.,.F.,(4,2,4),(0.,0.0198954793043815,0.0397918613553301),
 .UNSPECIFIED.);
#1363=B_SPLINE_CURVE_WITH_KNOTS('',3,(#67312,#67313,#67314,#67315,#67316,
#67317,#67318),.UNSPECIFIED.,.F.,.F.,(4,3,4),(0.,0.5,0.999990117123793),
 .UNSPECIFIED.);
#1364=B_SPLINE_CURVE_WITH_KNOTS('',3,(#67341,#67342,#67343,#67344,#67345,
#67346),.UNSPECIFIED.,.F.,.F.,(4,2,4),(0.,0.0198677119029657,0.039736333911811),
 .UNSPECIFIED.);
#1365=B_SPLINE_CURVE_WITH_KNOTS('',3,(#67388,#67389,#67390,#67391,#67392,
#67393),.UNSPECIFIED.,.F.,.F.,(4,2,4),(0.,0.0198973966033577,0.0397956843461078),
 .UNSPECIFIED.);
#1366=B_SPLINE_CURVE_WITH_KNOTS('',3,(#67415,#67416,#67417,#67418,#67419,
#67420),.UNSPECIFIED.,.F.,.F.,(4,2,4),(0.,0.0199030679707897,0.0398070346211267),
 .UNSPECIFIED.);
#1367=B_SPLINE_CURVE_WITH_KNOTS('',3,(#67465,#67466,#67467,#67468,#67469,
#67470),.UNSPECIFIED.,.F.,.F.,(4,2,4),(0.,0.0198994178847544,0.0397997368809266),
 .UNSPECIFIED.);
#1368=B_SPLINE_CURVE_WITH_KNOTS('',3,(#67483,#67484,#67485,#67486,#67487,
#67488),.UNSPECIFIED.,.F.,.F.,(4,2,4),(0.,0.0198905179563737,0.0397819072583148),
 .UNSPECIFIED.);
#1369=B_SPLINE_CURVE_WITH_KNOTS('',3,(#67513,#67514,#67515,#67516,#67517,
#67518,#67519),.UNSPECIFIED.,.F.,.F.,(4,3,4),(0.0365944846647015,0.0384615384615384,
0.0431466153076599),.UNSPECIFIED.);
#1370=B_SPLINE_CURVE_WITH_KNOTS('',3,(#67520,#67521,#67522,#67523,#67524,
#67525,#67526,#67527),.UNSPECIFIED.,.F.,.F.,(4,2,2,4),(1.77257433175202E-6,
0.00863675581122146,0.0171409325034123,0.0172810779526648),
 .UNSPECIFIED.);
#1371=B_SPLINE_CURVE_WITH_KNOTS('',3,(#67552,#67553,#67554,#67555,#67556,
#67557),.UNSPECIFIED.,.F.,.F.,(4,2,4),(0.,0.0198536183270368,0.0397081496382176),
 .UNSPECIFIED.);
#1372=B_SPLINE_CURVE_WITH_KNOTS('',3,(#67575,#67576,#67577,#67578,#67579,
#67580),.UNSPECIFIED.,.F.,.F.,(4,2,4),(-0.00212388914888901,-0.00106194216549549,
0.),.UNSPECIFIED.);
#1373=B_SPLINE_CURVE_WITH_KNOTS('',3,(#67581,#67582,#67583,#67584,#67585,
#67586),.UNSPECIFIED.,.F.,.F.,(4,2,4),(9.99998418999774E-7,0.019352785409166,
0.0387045795316142),.UNSPECIFIED.);
#1374=B_SPLINE_CURVE_WITH_KNOTS('',3,(#67620,#67621,#67622,#67623,#67624,
#67625),.UNSPECIFIED.,.F.,.F.,(4,2,4),(0.,0.0198761967017776,0.0397532849566243),
 .UNSPECIFIED.);
#1375=B_SPLINE_CURVE_WITH_KNOTS('',3,(#67631,#67632,#67633,#67634,#67635,
#67636),.UNSPECIFIED.,.F.,.F.,(4,2,4),(-0.00212486385494385,-0.00106293276454614,
-1.00000000456354E-6),.UNSPECIFIED.);
#1376=B_SPLINE_CURVE_WITH_KNOTS('',3,(#67655,#67656,#67657,#67658,#67659,
#67660),.UNSPECIFIED.,.F.,.F.,(4,2,4),(0.,0.0198583386741828,0.0397175618451867),
 .UNSPECIFIED.);
#1377=B_SPLINE_CURVE_WITH_KNOTS('',3,(#67711,#67712,#67713,#67714,#67715,
#67716),.UNSPECIFIED.,.F.,.F.,(4,2,4),(0.,0.0199008240853172,0.0398025407040322),
 .UNSPECIFIED.);
#1378=B_SPLINE_CURVE_WITH_KNOTS('',3,(#67729,#67730,#67731,#67732,#67733,
#67734),.UNSPECIFIED.,.F.,.F.,(4,2,4),(0.,0.0199042047179996,0.0398092891748803),
 .UNSPECIFIED.);
#1379=B_SPLINE_CURVE_WITH_KNOTS('',3,(#67779,#67780,#67781,#67782,#67783,
#67784),.UNSPECIFIED.,.F.,.F.,(4,2,4),(0.,0.0198954793727932,0.0397918615634901),
 .UNSPECIFIED.);
#1380=B_SPLINE_CURVE_WITH_KNOTS('',3,(#67824,#67825,#67826,#67827,#67828,
#67829,#67830),.UNSPECIFIED.,.F.,.F.,(4,3,4),(0.,0.5,0.999990117126542),
 .UNSPECIFIED.);
#1381=B_SPLINE_CURVE_WITH_KNOTS('',3,(#67853,#67854,#67855,#67856,#67857,
#67858),.UNSPECIFIED.,.F.,.F.,(4,2,4),(0.,0.0198677119061941,0.0397363339249417),
 .UNSPECIFIED.);
#1382=B_SPLINE_CURVE_WITH_KNOTS('',3,(#67900,#67901,#67902,#67903,#67904,
#67905),.UNSPECIFIED.,.F.,.F.,(4,2,4),(0.,0.0198973966042074,0.0397956843497479),
 .UNSPECIFIED.);
#1383=B_SPLINE_CURVE_WITH_KNOTS('',3,(#67927,#67928,#67929,#67930,#67931,
#67932),.UNSPECIFIED.,.F.,.F.,(4,2,4),(0.,0.0199030679727059,0.0398070346286982),
 .UNSPECIFIED.);
#1384=B_SPLINE_CURVE_WITH_KNOTS('',3,(#67977,#67978,#67979,#67980,#67981,
#67982),.UNSPECIFIED.,.F.,.F.,(4,2,4),(0.,0.0198994178163347,0.0397997366745588),
 .UNSPECIFIED.);
#1385=B_SPLINE_CURVE_WITH_KNOTS('',3,(#67995,#67996,#67997,#67998,#67999,
#68000),.UNSPECIFIED.,.F.,.F.,(4,2,4),(0.,0.0198905179567855,0.0397819072575837),
 .UNSPECIFIED.);
#1386=B_SPLINE_CURVE_WITH_KNOTS('',3,(#68025,#68026,#68027,#68028,#68029,
#68030,#68031),.UNSPECIFIED.,.F.,.F.,(4,3,4),(0.0365944846647011,0.0384615384615384,
0.0431466153076599),.UNSPECIFIED.);
#1387=B_SPLINE_CURVE_WITH_KNOTS('',3,(#68032,#68033,#68034,#68035,#68036,
#68037,#68038,#68039),.UNSPECIFIED.,.F.,.F.,(4,2,2,4),(1.77256723985765E-6,
0.00863675584772395,0.017140965275147,0.0172811072181662),.UNSPECIFIED.);
#1388=B_SPLINE_CURVE_WITH_KNOTS('',3,(#68064,#68065,#68066,#68067,#68068,
#68069),.UNSPECIFIED.,.F.,.F.,(4,2,4),(0.,0.0198536183277256,0.0397081496406794),
 .UNSPECIFIED.);
#1389=B_SPLINE_CURVE_WITH_KNOTS('',3,(#68087,#68088,#68089,#68090,#68091,
#68092),.UNSPECIFIED.,.F.,.F.,(4,2,4),(-0.00212388605083564,-0.00106194091765259,
0.),.UNSPECIFIED.);
#1390=B_SPLINE_CURVE_WITH_KNOTS('',3,(#68093,#68094,#68095,#68096,#68097,
#68098),.UNSPECIFIED.,.F.,.F.,(4,2,4),(9.99998419401124E-7,0.0193527854087786,
0.0387045795309009),.UNSPECIFIED.);
#1391=B_SPLINE_CURVE_WITH_KNOTS('',3,(#68104,#68105,#68106,#68107,#68108,
#68109),.UNSPECIFIED.,.F.,.F.,(4,2,4),(-0.00212486447982969,-0.00106293277044209,
-9.99999998075674E-7),.UNSPECIFIED.);
#1392=B_SPLINE_CURVE_WITH_KNOTS('',3,(#68148,#68149,#68150,#68151,#68152,
#68153),.UNSPECIFIED.,.F.,.F.,(4,2,4),(0.,0.0198583386755922,0.0397175618510719),
 .UNSPECIFIED.);
#1393=B_SPLINE_CURVE_WITH_KNOTS('',3,(#68166,#68167,#68168,#68169,#68170,
#68171),.UNSPECIFIED.,.F.,.F.,(4,2,4),(0.,0.0198761965810603,0.039753284719404),
 .UNSPECIFIED.);
#1394=B_SPLINE_CURVE_WITH_KNOTS('',3,(#68212,#68213,#68214,#68215,#68216,
#68217),.UNSPECIFIED.,.F.,.F.,(4,2,4),(0.,0.0199042047183857,0.0398092891790922),
 .UNSPECIFIED.);
#1395=B_SPLINE_CURVE_WITH_KNOTS('',3,(#68242,#68243,#68244,#68245,#68246,
#68247),.UNSPECIFIED.,.F.,.F.,(4,2,4),(0.,0.0199008240861043,0.0398025407072504),
 .UNSPECIFIED.);
#1396=B_SPLINE_CURVE_WITH_KNOTS('',3,(#68291,#68292,#68293,#68294,#68295,
#68296),.UNSPECIFIED.,.F.,.F.,(4,2,4),(0.,0.0198954793743314,0.0397918615697323),
 .UNSPECIFIED.);
#1397=B_SPLINE_CURVE_WITH_KNOTS('',3,(#68336,#68337,#68338,#68339,#68340,
#68341,#68342),.UNSPECIFIED.,.F.,.F.,(4,3,4),(0.,0.5,0.9999901171293),
 .UNSPECIFIED.);
#1398=B_SPLINE_CURVE_WITH_KNOTS('',3,(#68365,#68366,#68367,#68368,#68369,
#68370),.UNSPECIFIED.,.F.,.F.,(4,2,4),(0.,0.0198677119105387,0.0397363339423693),
 .UNSPECIFIED.);
#1399=B_SPLINE_CURVE_WITH_KNOTS('',3,(#68412,#68413,#68414,#68415,#68416,
#68417),.UNSPECIFIED.,.F.,.F.,(4,2,4),(0.,0.019897396605077,0.0397956843531935),
 .UNSPECIFIED.);
#1400=B_SPLINE_CURVE_WITH_KNOTS('',3,(#68439,#68440,#68441,#68442,#68443,
#68444),.UNSPECIFIED.,.F.,.F.,(4,2,4),(0.,0.0199030679766039,0.0398070346443927),
 .UNSPECIFIED.);
#1401=B_SPLINE_CURVE_WITH_KNOTS('',3,(#68489,#68490,#68491,#68492,#68493,
#68494),.UNSPECIFIED.,.F.,.F.,(4,2,4),(0.,0.0198994178865019,0.0397997368880701),
 .UNSPECIFIED.);
#1402=B_SPLINE_CURVE_WITH_KNOTS('',3,(#68507,#68508,#68509,#68510,#68511,
#68512),.UNSPECIFIED.,.F.,.F.,(4,2,4),(0.,0.0198905179569301,0.0397819072590209),
 .UNSPECIFIED.);
#1403=B_SPLINE_CURVE_WITH_KNOTS('',3,(#68537,#68538,#68539,#68540,#68541,
#68542,#68543),.UNSPECIFIED.,.F.,.F.,(4,3,4),(0.0365944846647007,0.0384615384615384,
0.0431466153076595),.UNSPECIFIED.);
#1404=B_SPLINE_CURVE_WITH_KNOTS('',3,(#68544,#68545,#68546,#68547,#68548,
#68549,#68550,#68551),.UNSPECIFIED.,.F.,.F.,(4,2,2,4),(1.77256358031356E-6,
0.00863675581093288,0.017140951289934,0.0172810947306584),.UNSPECIFIED.);
#1405=B_SPLINE_CURVE_WITH_KNOTS('',3,(#68576,#68577,#68578,#68579,#68580,
#68581),.UNSPECIFIED.,.F.,.F.,(4,2,4),(0.,0.0198536183285242,0.0397081496440867),
 .UNSPECIFIED.);
#1406=B_SPLINE_CURVE_WITH_KNOTS('',3,(#68599,#68600,#68601,#68602,#68603,
#68604),.UNSPECIFIED.,.F.,.F.,(4,2,4),(-0.00212388353492024,-0.00106193992386253,
0.),.UNSPECIFIED.);
#1407=B_SPLINE_CURVE_WITH_KNOTS('',3,(#68605,#68606,#68607,#68608,#68609,
#68610),.UNSPECIFIED.,.F.,.F.,(4,2,4),(9.99998415477424E-7,0.0193522803902194,
0.0387045693967639),.UNSPECIFIED.);
#1408=B_SPLINE_CURVE_WITH_KNOTS('',3,(#68616,#68617,#68618,#68619,#68620,
#68621),.UNSPECIFIED.,.F.,.F.,(4,2,4),(-0.00212486501284603,-0.00106293275806993,
-9.99999997913477E-7),.UNSPECIFIED.);
#1409=B_SPLINE_CURVE_WITH_KNOTS('',3,(#68660,#68661,#68662,#68663,#68664,
#68665),.UNSPECIFIED.,.F.,.F.,(4,2,4),(0.,0.0198583386762458,0.0397175618534314),
 .UNSPECIFIED.);
#1410=B_SPLINE_CURVE_WITH_KNOTS('',3,(#68678,#68679,#68680,#68681,#68682,
#68683),.UNSPECIFIED.,.F.,.F.,(4,2,4),(0.,0.019876196696537,0.0397532849500752),
 .UNSPECIFIED.);
#1411=B_SPLINE_CURVE_WITH_KNOTS('',3,(#68735,#68736,#68737,#68738,#68739,
#68740),.UNSPECIFIED.,.F.,.F.,(4,2,4),(0.,0.0199008240870978,0.039802540710855),
 .UNSPECIFIED.);
#1412=B_SPLINE_CURVE_WITH_KNOTS('',3,(#68753,#68754,#68755,#68756,#68757,
#68758),.UNSPECIFIED.,.F.,.F.,(4,2,4),(0.,0.019904204718409,0.0398092891761761),
 .UNSPECIFIED.);
#1413=B_SPLINE_CURVE_WITH_KNOTS('',3,(#68817,#68818,#68819,#68820,#68821,
#68822),.UNSPECIFIED.,.F.,.F.,(4,2,4),(0.,0.0198954793770109,0.039791861578122),
 .UNSPECIFIED.);
#1414=B_SPLINE_CURVE_WITH_KNOTS('',3,(#68851,#68852,#68853,#68854,#68855,
#68856,#68857),.UNSPECIFIED.,.F.,.F.,(4,3,4),(0.,0.5,0.999990117130999),
 .UNSPECIFIED.);
#1415=B_SPLINE_CURVE_WITH_KNOTS('',3,(#68880,#68881,#68882,#68883,#68884,
#68885),.UNSPECIFIED.,.F.,.F.,(4,2,4),(0.,0.0198677119151675,0.0397363339609174),
 .UNSPECIFIED.);
#1416=B_SPLINE_CURVE_WITH_KNOTS('',3,(#68927,#68928,#68929,#68930,#68931,
#68932),.UNSPECIFIED.,.F.,.F.,(4,2,4),(0.,0.0198973966056516,0.039795684355372),
 .UNSPECIFIED.);
#1417=B_SPLINE_CURVE_WITH_KNOTS('',3,(#68954,#68955,#68956,#68957,#68958,
#68959),.UNSPECIFIED.,.F.,.F.,(4,2,4),(0.,0.0199030679802205,0.0398070346592923),
 .UNSPECIFIED.);
#1418=B_SPLINE_CURVE_WITH_KNOTS('',3,(#69004,#69005,#69006,#69007,#69008,
#69009),.UNSPECIFIED.,.F.,.F.,(4,2,4),(0.,0.0198994178870172,0.0397997368900241),
 .UNSPECIFIED.);
#1419=B_SPLINE_CURVE_WITH_KNOTS('',3,(#69022,#69023,#69024,#69025,#69026,
#69027),.UNSPECIFIED.,.F.,.F.,(4,2,4),(0.,0.0198905179567028,0.039781907256152),
 .UNSPECIFIED.);
#1420=B_SPLINE_CURVE_WITH_KNOTS('',3,(#69052,#69053,#69054,#69055,#69056,
#69057,#69058),.UNSPECIFIED.,.F.,.F.,(4,3,4),(0.0365944846647009,0.0384615384615384,
0.0431466153076596),.UNSPECIFIED.);
#1421=B_SPLINE_CURVE_WITH_KNOTS('',3,(#69059,#69060,#69061,#69062,#69063,
#69064,#69065,#69066),.UNSPECIFIED.,.F.,.F.,(4,2,2,4),(1.77256703655956E-6,
0.00863675592193242,0.017140984838655,0.0172811247032637),.UNSPECIFIED.);
#1422=B_SPLINE_CURVE_WITH_KNOTS('',3,(#69091,#69092,#69093,#69094,#69095,
#69096),.UNSPECIFIED.,.F.,.F.,(4,2,4),(0.,0.0198536183299061,0.0397081496493331),
 .UNSPECIFIED.);
#1423=B_SPLINE_CURVE_WITH_KNOTS('',3,(#69114,#69115,#69116,#69117,#69118,
#69119),.UNSPECIFIED.,.F.,.F.,(4,2,4),(-0.00212388200777003,-0.0010619393097638,
0.),.UNSPECIFIED.);
#1424=B_SPLINE_CURVE_WITH_KNOTS('',3,(#69120,#69121,#69122,#69123,#69124,
#69125),.UNSPECIFIED.,.F.,.F.,(4,2,4),(9.99998423274043E-7,0.01935278540972,
0.0387045795326976),.UNSPECIFIED.);
#1425=B_SPLINE_CURVE_WITH_KNOTS('',3,(#69131,#69132,#69133,#69134,#69135,
#69136),.UNSPECIFIED.,.F.,.F.,(4,2,4),(-0.0021248655886198,-0.00106293276740361,
-9.99999997247777E-7),.UNSPECIFIED.);
#1426=B_SPLINE_CURVE_WITH_KNOTS('',3,(#69175,#69176,#69177,#69178,#69179,
#69180),.UNSPECIFIED.,.F.,.F.,(4,2,4),(0.,0.0198583386771501,0.0397175618572917),
 .UNSPECIFIED.);
#1427=B_SPLINE_CURVE_WITH_KNOTS('',3,(#69193,#69194,#69195,#69196,#69197,
#69198),.UNSPECIFIED.,.F.,.F.,(4,2,4),(0.,0.0198761966897326,0.0397532849443772),
 .UNSPECIFIED.);
#1428=B_SPLINE_CURVE_WITH_KNOTS('',3,(#69250,#69251,#69252,#69253,#69254,
#69255),.UNSPECIFIED.,.F.,.F.,(4,2,4),(0.,0.0199008240880666,0.0398025407146116),
 .UNSPECIFIED.);
#1429=B_SPLINE_CURVE_WITH_KNOTS('',3,(#69268,#69269,#69270,#69271,#69272,
#69273),.UNSPECIFIED.,.F.,.F.,(4,2,4),(0.,0.0199042047186014,0.0398092891759251),
 .UNSPECIFIED.);
#1430=B_SPLINE_CURVE_WITH_KNOTS('',3,(#69321,#69322,#69323,#69324,#69325,
#69326),.UNSPECIFIED.,.F.,.F.,(4,2,4),(0.,0.019895479376471,0.039791861578371),
 .UNSPECIFIED.);
#1431=B_SPLINE_CURVE_WITH_KNOTS('',3,(#69366,#69367,#69368,#69369,#69370,
#69371,#69372),.UNSPECIFIED.,.F.,.F.,(4,3,4),(0.,0.5,0.999990117134267),
 .UNSPECIFIED.);
#1432=B_SPLINE_CURVE_WITH_KNOTS('',3,(#69395,#69396,#69397,#69398,#69399,
#69400),.UNSPECIFIED.,.F.,.F.,(4,2,4),(0.,0.0198677119197326,0.0397363339795572),
 .UNSPECIFIED.);
#1433=B_SPLINE_CURVE_WITH_KNOTS('',3,(#69442,#69443,#69444,#69445,#69446,
#69447),.UNSPECIFIED.,.F.,.F.,(4,2,4),(0.,0.0198973966056449,0.0397956843554118),
 .UNSPECIFIED.);
#1434=B_SPLINE_CURVE_WITH_KNOTS('',3,(#69469,#69470,#69471,#69472,#69473,
#69474),.UNSPECIFIED.,.F.,.F.,(4,2,4),(0.,0.0199030679854828,0.0398070346804227),
 .UNSPECIFIED.);
#1435=B_SPLINE_CURVE_WITH_KNOTS('',3,(#69519,#69520,#69521,#69522,#69523,
#69524),.UNSPECIFIED.,.F.,.F.,(4,2,4),(0.,0.0198994178876402,0.0397997368926258),
 .UNSPECIFIED.);
#1436=B_SPLINE_CURVE_WITH_KNOTS('',3,(#69537,#69538,#69539,#69540,#69541,
#69542),.UNSPECIFIED.,.F.,.F.,(4,2,4),(0.,0.019890517957229,0.0397819072577925),
 .UNSPECIFIED.);
#1437=B_SPLINE_CURVE_WITH_KNOTS('',3,(#69567,#69568,#69569,#69570,#69571,
#69572,#69573),.UNSPECIFIED.,.F.,.F.,(4,3,4),(0.036594484664701,0.0384615384615384,
0.0431466153076602),.UNSPECIFIED.);
#1438=B_SPLINE_CURVE_WITH_KNOTS('',3,(#69574,#69575,#69576,#69577,#69578,
#69579,#69580,#69581),.UNSPECIFIED.,.F.,.F.,(4,2,2,4),(1.77256732140101E-6,
0.00863675581872223,0.0171409391189963,0.0172810838451956),
 .UNSPECIFIED.);
#1439=B_SPLINE_CURVE_WITH_KNOTS('',3,(#69606,#69607,#69608,#69609,#69610,
#69611),.UNSPECIFIED.,.F.,.F.,(4,2,4),(0.,0.0198536183299362,0.0397081496494468),
 .UNSPECIFIED.);
#1440=B_SPLINE_CURVE_WITH_KNOTS('',3,(#69629,#69630,#69631,#69632,#69633,
#69634),.UNSPECIFIED.,.F.,.F.,(4,2,4),(-0.00212387831185543,-0.00106193782572264,
0.),.UNSPECIFIED.);
#1441=B_SPLINE_CURVE_WITH_KNOTS('',3,(#69635,#69636,#69637,#69638,#69639,
#69640),.UNSPECIFIED.,.F.,.F.,(4,2,4),(9.99998423982381E-7,0.0193522753882191,
0.038704569298396),.UNSPECIFIED.);
#1442=B_SPLINE_CURVE_WITH_KNOTS('',3,(#69646,#69647,#69648,#69649,#69650,
#69651),.UNSPECIFIED.,.F.,.F.,(4,2,4),(-0.00212486605241449,-0.00106293275969741,
-9.99999995914859E-7),.UNSPECIFIED.);
#1443=B_SPLINE_CURVE_WITH_KNOTS('',3,(#69690,#69691,#69692,#69693,#69694,
#69695),.UNSPECIFIED.,.F.,.F.,(4,2,4),(0.,0.019858338677387,0.0397175618584201),
 .UNSPECIFIED.);
#1444=B_SPLINE_CURVE_WITH_KNOTS('',3,(#69708,#69709,#69710,#69711,#69712,
#69713),.UNSPECIFIED.,.F.,.F.,(4,2,4),(0.,0.0198761967027802,0.0397532849636417),
 .UNSPECIFIED.);
#1445=B_SPLINE_CURVE_WITH_KNOTS('',3,(#69765,#69766,#69767,#69768,#69769,
#69770),.UNSPECIFIED.,.F.,.F.,(4,2,4),(0.,0.0199008240889834,0.039802540718122),
 .UNSPECIFIED.);
#1446=B_SPLINE_CURVE_WITH_KNOTS('',3,(#69783,#69784,#69785,#69786,#69787,
#69788),.UNSPECIFIED.,.F.,.F.,(4,2,4),(0.,0.0199042047184434,0.0398092891758487),
 .UNSPECIFIED.);
#1447=B_SPLINE_CURVE_WITH_KNOTS('',3,(#69836,#69837,#69838,#69839,#69840,
#69841),.UNSPECIFIED.,.F.,.F.,(4,2,4),(0.,0.0198954793771532,0.0397918615810156),
 .UNSPECIFIED.);
#1448=B_SPLINE_CURVE_WITH_KNOTS('',3,(#69881,#69882,#69883,#69884,#69885,
#69886,#69887),.UNSPECIFIED.,.F.,.F.,(4,3,4),(0.,0.5,0.999990117136375),
 .UNSPECIFIED.);
#1449=B_SPLINE_CURVE_WITH_KNOTS('',3,(#69910,#69911,#69912,#69913,#69914,
#69915),.UNSPECIFIED.,.F.,.F.,(4,2,4),(0.,0.0198677119243952,0.0397363339986725),
 .UNSPECIFIED.);
#1450=B_SPLINE_CURVE_WITH_KNOTS('',3,(#69957,#69958,#69959,#69960,#69961,
#69962),.UNSPECIFIED.,.F.,.F.,(4,2,4),(0.,0.0198973966060797,0.0397956843571033),
 .UNSPECIFIED.);
#1451=B_SPLINE_CURVE_WITH_KNOTS('',3,(#69984,#69985,#69986,#69987,#69988,
#69989),.UNSPECIFIED.,.F.,.F.,(4,2,4),(0.,0.0199030679898499,0.0398070346983652),
 .UNSPECIFIED.);
#1452=B_SPLINE_CURVE_WITH_KNOTS('',3,(#70034,#70035,#70036,#70037,#70038,
#70039),.UNSPECIFIED.,.F.,.F.,(4,2,4),(0.,0.0198994178878564,0.03979973689336),
 .UNSPECIFIED.);
#1453=B_SPLINE_CURVE_WITH_KNOTS('',3,(#70052,#70053,#70054,#70055,#70056,
#70057),.UNSPECIFIED.,.F.,.F.,(4,2,4),(0.,0.0198905179571636,0.0397819072599618),
 .UNSPECIFIED.);
#1454=B_SPLINE_CURVE_WITH_KNOTS('',3,(#70082,#70083,#70084,#70085,#70086,
#70087,#70088),.UNSPECIFIED.,.F.,.F.,(4,3,4),(0.0365944846647013,0.0384615384615384,
0.0431466153076604),.UNSPECIFIED.);
#1455=B_SPLINE_CURVE_WITH_KNOTS('',3,(#70089,#70090,#70091,#70092,#70093,
#70094,#70095,#70096),.UNSPECIFIED.,.F.,.F.,(4,2,2,4),(1.7725671724742E-6,
0.00863675585766041,0.0171409671998102,0.0172811089329915),
 .UNSPECIFIED.);
#1456=B_SPLINE_CURVE_WITH_KNOTS('',3,(#70121,#70122,#70123,#70124,#70125,
#70126),.UNSPECIFIED.,.F.,.F.,(4,2,4),(0.,0.0198536183343959,0.0397081496659324),
 .UNSPECIFIED.);
#1457=B_SPLINE_CURVE_WITH_KNOTS('',3,(#70144,#70145,#70146,#70147,#70148,
#70149),.UNSPECIFIED.,.F.,.F.,(4,2,4),(-0.00212387641773327,-0.0010619370665021,
0.),.UNSPECIFIED.);
#1458=B_SPLINE_CURVE_WITH_KNOTS('',3,(#70150,#70151,#70152,#70153,#70154,
#70155),.UNSPECIFIED.,.F.,.F.,(4,2,4),(9.99998414701243E-7,0.0193527803906903,
0.0387045693989795),.UNSPECIFIED.);
#1459=B_SPLINE_CURVE_WITH_KNOTS('',3,(#70161,#70162,#70163,#70164,#70165,
#70166),.UNSPECIFIED.,.F.,.F.,(4,2,4),(-0.00212486654942059,-0.00106293276399481,
-9.99999993921228E-7),.UNSPECIFIED.);
#1460=B_SPLINE_CURVE_WITH_KNOTS('',3,(#70205,#70206,#70207,#70208,#70209,
#70210),.UNSPECIFIED.,.F.,.F.,(4,2,4),(0.,0.0198583386780391,0.0397175618608395),
 .UNSPECIFIED.);
#1461=B_SPLINE_CURVE_WITH_KNOTS('',3,(#70223,#70224,#70225,#70226,#70227,
#70228),.UNSPECIFIED.,.F.,.F.,(4,2,4),(0.,0.0198761967007073,0.0397532849594556),
 .UNSPECIFIED.);
#1462=B_SPLINE_CURVE_WITH_KNOTS('',3,(#70280,#70281,#70282,#70283,#70284,
#70285),.UNSPECIFIED.,.F.,.F.,(4,2,4),(0.,0.0199008240893237,0.0398025407191679),
 .UNSPECIFIED.);
#1463=B_SPLINE_CURVE_WITH_KNOTS('',3,(#70298,#70299,#70300,#70301,#70302,
#70303),.UNSPECIFIED.,.F.,.F.,(4,2,4),(0.,0.0199042047187462,0.0398092891746098),
 .UNSPECIFIED.);
#1464=B_SPLINE_CURVE_WITH_KNOTS('',3,(#70351,#70352,#70353,#70354,#70355,
#70356),.UNSPECIFIED.,.F.,.F.,(4,2,4),(0.,0.019895479377941,0.0397918615841521),
 .UNSPECIFIED.);
#1465=B_SPLINE_CURVE_WITH_KNOTS('',3,(#70396,#70397,#70398,#70399,#70400,
#70401,#70402),.UNSPECIFIED.,.F.,.F.,(4,3,4),(0.,0.5,0.999990117139493),
 .UNSPECIFIED.);
#1466=B_SPLINE_CURVE_WITH_KNOTS('',3,(#70425,#70426,#70427,#70428,#70429,
#70430),.UNSPECIFIED.,.F.,.F.,(4,2,4),(0.,0.0198677119298734,0.0397363340203713),
 .UNSPECIFIED.);
#1467=B_SPLINE_CURVE_WITH_KNOTS('',3,(#70472,#70473,#70474,#70475,#70476,
#70477),.UNSPECIFIED.,.F.,.F.,(4,2,4),(0.,0.019897396605761,0.0397956843558467),
 .UNSPECIFIED.);
#1468=B_SPLINE_CURVE_WITH_KNOTS('',3,(#70499,#70500,#70501,#70502,#70503,
#70504),.UNSPECIFIED.,.F.,.F.,(4,2,4),(0.,0.0199030679943856,0.0398070347169293),
 .UNSPECIFIED.);
#1469=B_SPLINE_CURVE_WITH_KNOTS('',3,(#70549,#70550,#70551,#70552,#70553,
#70554),.UNSPECIFIED.,.F.,.F.,(4,2,4),(0.,0.0198994178880039,0.0397997368943815),
 .UNSPECIFIED.);
#1470=B_SPLINE_CURVE_WITH_KNOTS('',3,(#70567,#70568,#70569,#70570,#70571,
#70572),.UNSPECIFIED.,.F.,.F.,(4,2,4),(0.,0.0198905179572561,0.039781907255197),
 .UNSPECIFIED.);
#1471=B_SPLINE_CURVE_WITH_KNOTS('',3,(#70597,#70598,#70599,#70600,#70601,
#70602,#70603),.UNSPECIFIED.,.F.,.F.,(4,3,4),(0.0365944846647005,0.0384615384615384,
0.04314661530766),.UNSPECIFIED.);
#1472=B_SPLINE_CURVE_WITH_KNOTS('',3,(#70604,#70605,#70606,#70607,#70608,
#70609,#70610,#70611),.UNSPECIFIED.,.F.,.F.,(4,2,2,4),(1.77256358748408E-6,
0.00863675582048878,0.0171409428335954,0.0172810871701512),
 .UNSPECIFIED.);
#1473=B_SPLINE_CURVE_WITH_KNOTS('',3,(#70636,#70637,#70638,#70639,#70640,
#70641),.UNSPECIFIED.,.F.,.F.,(4,2,4),(0.,0.0198536183313603,0.0397081496548265),
 .UNSPECIFIED.);
#1474=B_SPLINE_CURVE_WITH_KNOTS('',3,(#70659,#70660,#70661,#70662,#70663,
#70664),.UNSPECIFIED.,.F.,.F.,(4,2,4),(-0.00212387341997532,-0.00106193587239301,
0.),.UNSPECIFIED.);
#1475=B_SPLINE_CURVE_WITH_KNOTS('',3,(#70665,#70666,#70667,#70668,#70669,
#70670),.UNSPECIFIED.,.F.,.F.,(4,2,4),(9.99998417067894E-7,0.0193527854098381,
0.0387045795330794),.UNSPECIFIED.);
#1476=B_SPLINE_CURVE_WITH_KNOTS('',3,(#70676,#70677,#70678,#70679,#70680,
#70681),.UNSPECIFIED.,.F.,.F.,(4,2,4),(-0.00212486691426954,-0.00106293276048919,
-9.99999995782153E-7),.UNSPECIFIED.);
#1477=B_SPLINE_CURVE_WITH_KNOTS('',3,(#70720,#70721,#70722,#70723,#70724,
#70725),.UNSPECIFIED.,.F.,.F.,(4,2,4),(0.,0.0198583386780509,0.0397175618608029),
 .UNSPECIFIED.);
#1478=B_SPLINE_CURVE_WITH_KNOTS('',3,(#70738,#70739,#70740,#70741,#70742,
#70743),.UNSPECIFIED.,.F.,.F.,(4,2,4),(0.,0.019876196698291,0.0397532849502144),
 .UNSPECIFIED.);
#1479=B_SPLINE_CURVE_WITH_KNOTS('',3,(#70795,#70796,#70797,#70798,#70799,
#70800),.UNSPECIFIED.,.F.,.F.,(4,2,4),(0.,0.0199008240898987,0.0398025407215578),
 .UNSPECIFIED.);
#1480=B_SPLINE_CURVE_WITH_KNOTS('',3,(#70813,#70814,#70815,#70816,#70817,
#70818),.UNSPECIFIED.,.F.,.F.,(4,2,4),(0.,0.0199042047126661,0.0398092891636698),
 .UNSPECIFIED.);
#1481=B_SPLINE_CURVE_WITH_KNOTS('',3,(#70866,#70867,#70868,#70869,#70870,
#70871),.UNSPECIFIED.,.F.,.F.,(4,2,4),(0.,0.0198954793785179,0.0397918615868151),
 .UNSPECIFIED.);
#1482=B_SPLINE_CURVE_WITH_KNOTS('',3,(#70911,#70912,#70913,#70914,#70915,
#70916,#70917),.UNSPECIFIED.,.F.,.F.,(4,3,4),(0.,0.5,0.99999011714245),
 .UNSPECIFIED.);
#1483=B_SPLINE_CURVE_WITH_KNOTS('',3,(#70940,#70941,#70942,#70943,#70944,
#70945),.UNSPECIFIED.,.F.,.F.,(4,2,4),(0.,0.0198677119349441,0.0397363340407095),
 .UNSPECIFIED.);
#1484=B_SPLINE_CURVE_WITH_KNOTS('',3,(#70987,#70988,#70989,#70990,#70991,
#70992),.UNSPECIFIED.,.F.,.F.,(4,2,4),(0.,0.0198973966055972,0.0397956843554853),
 .UNSPECIFIED.);
#1485=B_SPLINE_CURVE_WITH_KNOTS('',3,(#71014,#71015,#71016,#71017,#71018,
#71019),.UNSPECIFIED.,.F.,.F.,(4,2,4),(0.,0.0199030680000759,0.0398070347395109),
 .UNSPECIFIED.);
#1486=B_SPLINE_CURVE_WITH_KNOTS('',3,(#71064,#71065,#71066,#71067,#71068,
#71069),.UNSPECIFIED.,.F.,.F.,(4,2,4),(0.,0.0198994178881233,0.0397997368947557),
 .UNSPECIFIED.);
#1487=B_SPLINE_CURVE_WITH_KNOTS('',3,(#71082,#71083,#71084,#71085,#71086,
#71087),.UNSPECIFIED.,.F.,.F.,(4,2,4),(0.,0.0198905179572044,0.039781907261386),
 .UNSPECIFIED.);
#1488=B_SPLINE_CURVE_WITH_KNOTS('',3,(#71112,#71113,#71114,#71115,#71116,
#71117,#71118),.UNSPECIFIED.,.F.,.F.,(4,3,4),(0.0365944846647007,0.0384615384615384,
0.0431466153076593),.UNSPECIFIED.);
#1489=B_SPLINE_CURVE_WITH_KNOTS('',3,(#71119,#71120,#71121,#71122,#71123,
#71124,#71125,#71126),.UNSPECIFIED.,.F.,.F.,(4,2,2,4),(1.77256357976421E-6,
0.00863675581873873,0.017140945662596,0.0172810896980204),.UNSPECIFIED.);
#1490=B_SPLINE_CURVE_WITH_KNOTS('',3,(#71151,#71152,#71153,#71154,#71155,
#71156),.UNSPECIFIED.,.F.,.F.,(4,2,4),(0.,0.0198536183310732,0.03970814965373),
 .UNSPECIFIED.);
#1491=B_SPLINE_CURVE_WITH_KNOTS('',3,(#71174,#71175,#71176,#71177,#71178,
#71179),.UNSPECIFIED.,.F.,.F.,(4,2,4),(-0.00212387063254784,-0.00106193475602023,
0.),.UNSPECIFIED.);
#1492=B_SPLINE_CURVE_WITH_KNOTS('',3,(#71180,#71181,#71182,#71183,#71184,
#71185),.UNSPECIFIED.,.F.,.F.,(4,2,4),(9.99998414999011E-7,0.0193527753884389,
0.0387045692999441),.UNSPECIFIED.);
#1493=B_SPLINE_CURVE_WITH_KNOTS('',3,(#71191,#71192,#71193,#71194,#71195,
#71196),.UNSPECIFIED.,.F.,.F.,(4,2,4),(-0.00212486729427008,-0.00106293276111579,
-9.99999993211292E-7),.UNSPECIFIED.);
#1494=B_SPLINE_CURVE_WITH_KNOTS('',3,(#71235,#71236,#71237,#71238,#71239,
#71240),.UNSPECIFIED.,.F.,.F.,(4,2,4),(0.,0.019858338678372,0.0397175618622352),
 .UNSPECIFIED.);
#1495=B_SPLINE_CURVE_WITH_KNOTS('',3,(#71253,#71254,#71255,#71256,#71257,
#71258),.UNSPECIFIED.,.F.,.F.,(4,2,4),(0.,0.0198761967066437,0.0397532849678352),
 .UNSPECIFIED.);
#1496=B_SPLINE_CURVE_WITH_KNOTS('',3,(#71310,#71311,#71312,#71313,#71314,
#71315),.UNSPECIFIED.,.F.,.F.,(4,2,4),(0.,0.0199008240895588,0.0398025407203014),
 .UNSPECIFIED.);
#1497=B_SPLINE_CURVE_WITH_KNOTS('',3,(#71328,#71329,#71330,#71331,#71332,
#71333),.UNSPECIFIED.,.F.,.F.,(4,2,4),(0.,0.0199042046961962,0.0398092891330403),
 .UNSPECIFIED.);
#1498=B_SPLINE_CURVE_WITH_KNOTS('',3,(#71381,#71382,#71383,#71384,#71385,
#71386),.UNSPECIFIED.,.F.,.F.,(4,2,4),(0.,0.0198954793788172,0.0397918615878541),
 .UNSPECIFIED.);
#1499=B_SPLINE_CURVE_WITH_KNOTS('',3,(#71426,#71427,#71428,#71429,#71430,
#71431,#71432),.UNSPECIFIED.,.F.,.F.,(4,3,4),(0.,0.5,0.999990117145692),
 .UNSPECIFIED.);
#1500=B_SPLINE_CURVE_WITH_KNOTS('',3,(#71455,#71456,#71457,#71458,#71459,
#71460),.UNSPECIFIED.,.F.,.F.,(4,2,4),(0.,0.0198677119382913,0.0397363340538751),
 .UNSPECIFIED.);
#1501=B_SPLINE_CURVE_WITH_KNOTS('',3,(#71502,#71503,#71504,#71505,#71506,
#71507),.UNSPECIFIED.,.F.,.F.,(4,2,4),(0.,0.0198973966054705,0.0397956843550537),
 .UNSPECIFIED.);
#1502=B_SPLINE_CURVE_WITH_KNOTS('',3,(#71529,#71530,#71531,#71532,#71533,
#71534),.UNSPECIFIED.,.F.,.F.,(4,2,4),(0.,0.019903068003928,0.0398070347549453),
 .UNSPECIFIED.);
#1503=B_SPLINE_CURVE_WITH_KNOTS('',3,(#71579,#71580,#71581,#71582,#71583,
#71584),.UNSPECIFIED.,.F.,.F.,(4,2,4),(0.,0.0198994178874679,0.0397997368920064),
 .UNSPECIFIED.);
#1504=B_SPLINE_CURVE_WITH_KNOTS('',3,(#71597,#71598,#71599,#71600,#71601,
#71602),.UNSPECIFIED.,.F.,.F.,(4,2,4),(0.,0.0198905174414553,0.0397819062199287),
 .UNSPECIFIED.);
#1505=B_SPLINE_CURVE_WITH_KNOTS('',3,(#71627,#71628,#71629,#71630,#71631,
#71632,#71633),.UNSPECIFIED.,.F.,.F.,(4,3,4),(0.0365944846647015,0.0384615384615384,
0.0431466153076595),.UNSPECIFIED.);
#1506=B_SPLINE_CURVE_WITH_KNOTS('',3,(#71634,#71635,#71636,#71637,#71638,
#71639,#71640,#71641),.UNSPECIFIED.,.F.,.F.,(4,2,2,4),(1.77291495321644E-6,
0.00863675579526595,0.0171409306756836,0.0172810762685451),
 .UNSPECIFIED.);
#1507=B_SPLINE_CURVE_WITH_KNOTS('',3,(#71666,#71667,#71668,#71669,#71670,
#71671),.UNSPECIFIED.,.F.,.F.,(4,2,4),(0.,0.0198536183312814,0.0397081496542885),
 .UNSPECIFIED.);
#1508=B_SPLINE_CURVE_WITH_KNOTS('',3,(#71689,#71690,#71691,#71692,#71693,
#71694),.UNSPECIFIED.,.F.,.F.,(4,2,4),(-0.00212386760957224,-0.00106193354766672,
0.),.UNSPECIFIED.);
#1509=B_SPLINE_CURVE_WITH_KNOTS('',3,(#71695,#71696,#71697,#71698,#71699,
#71700),.UNSPECIFIED.,.F.,.F.,(4,2,4),(9.99998413909848E-7,0.0193527748421895,
0.038704569287749),.UNSPECIFIED.);
#1510=B_SPLINE_CURVE_WITH_KNOTS('',3,(#71706,#71707,#71708,#71709,#71710,
#71711),.UNSPECIFIED.,.F.,.F.,(4,2,4),(-0.0021248675435194,-0.00106293275918252,
-1.00000000268332E-6),.UNSPECIFIED.);
#1511=B_SPLINE_CURVE_WITH_KNOTS('',3,(#71750,#71751,#71752,#71753,#71754,
#71755),.UNSPECIFIED.,.F.,.F.,(4,2,4),(0.,0.0198583386782803,0.0397175618619299),
 .UNSPECIFIED.);
#1512=B_SPLINE_CURVE_WITH_KNOTS('',3,(#71768,#71769,#71770,#71771,#71772,
#71773),.UNSPECIFIED.,.F.,.F.,(4,2,4),(0.,0.0198761966619282,0.0397532848848484),
 .UNSPECIFIED.);
#1513=B_SPLINE_CURVE_WITH_KNOTS('',3,(#71825,#71826,#71827,#71828,#71829,
#71830),.UNSPECIFIED.,.F.,.F.,(4,2,4),(0.,0.0199008240900917,0.0398025407223278),
 .UNSPECIFIED.);
#1514=B_SPLINE_CURVE_WITH_KNOTS('',3,(#71843,#71844,#71845,#71846,#71847,
#71848),.UNSPECIFIED.,.F.,.F.,(4,2,4),(0.,0.0199042047128343,0.0398092891614523),
 .UNSPECIFIED.);
#1515=B_SPLINE_CURVE_WITH_KNOTS('',3,(#71896,#71897,#71898,#71899,#71900,
#71901),.UNSPECIFIED.,.F.,.F.,(4,2,4),(0.,0.0198954793788647,0.0397918615880732),
 .UNSPECIFIED.);
#1516=B_SPLINE_CURVE_WITH_KNOTS('',3,(#71941,#71942,#71943,#71944,#71945,
#71946,#71947),.UNSPECIFIED.,.F.,.F.,(4,3,4),(0.,0.5,0.999990117148444),
 .UNSPECIFIED.);
#1517=B_SPLINE_CURVE_WITH_KNOTS('',3,(#71970,#71971,#71972,#71973,#71974,
#71975),.UNSPECIFIED.,.F.,.F.,(4,2,4),(0.,0.0198677119395526,0.0397363340592826),
 .UNSPECIFIED.);
#1518=B_SPLINE_CURVE_WITH_KNOTS('',3,(#72017,#72018,#72019,#72020,#72021,
#72022),.UNSPECIFIED.,.F.,.F.,(4,2,4),(0.,0.0198973966050765,0.0397956843534938),
 .UNSPECIFIED.);
#1519=B_SPLINE_CURVE_WITH_KNOTS('',3,(#72044,#72045,#72046,#72047,#72048,
#72049),.UNSPECIFIED.,.F.,.F.,(4,2,4),(0.,0.0199030680059554,0.0398070347632472),
 .UNSPECIFIED.);
#1520=B_SPLINE_CURVE_WITH_KNOTS('',3,(#72094,#72095,#72096,#72097,#72098,
#72099),.UNSPECIFIED.,.F.,.F.,(4,2,4),(0.,0.0198994178873714,0.0397997368914788),
 .UNSPECIFIED.);
#1521=B_SPLINE_CURVE_WITH_KNOTS('',3,(#72112,#72113,#72114,#72115,#72116,
#72117),.UNSPECIFIED.,.F.,.F.,(4,2,4),(0.,0.0198905179568428,0.0397819072611588),
 .UNSPECIFIED.);
#1522=B_SPLINE_CURVE_WITH_KNOTS('',3,(#72142,#72143,#72144,#72145,#72146,
#72147,#72148),.UNSPECIFIED.,.F.,.F.,(4,3,4),(0.0365944846647007,0.0384615384615384,
0.0431466153076601),.UNSPECIFIED.);
#1523=B_SPLINE_CURVE_WITH_KNOTS('',3,(#72149,#72150,#72151,#72152,#72153,
#72154,#72155,#72156),.UNSPECIFIED.,.F.,.F.,(4,2,2,4),(1.77349251834674E-6,
0.00863675583297312,0.017140940164705,0.0172810846677369),.UNSPECIFIED.);
#1524=B_SPLINE_CURVE_WITH_KNOTS('',3,(#72181,#72182,#72183,#72184,#72185,
#72186),.UNSPECIFIED.,.F.,.F.,(4,2,4),(0.,0.0198536183306229,0.0397081496516829),
 .UNSPECIFIED.);
#1525=B_SPLINE_CURVE_WITH_KNOTS('',3,(#72204,#72205,#72206,#72207,#72208,
#72209),.UNSPECIFIED.,.F.,.F.,(4,2,4),(-0.00212386483367974,-0.00106193243731324,
0.),.UNSPECIFIED.);
#1526=B_SPLINE_CURVE_WITH_KNOTS('',3,(#72210,#72211,#72212,#72213,#72214,
#72215),.UNSPECIFIED.,.F.,.F.,(4,2,4),(9.99998414062903E-7,0.0193527795959641,
0.0387045693836927),.UNSPECIFIED.);
#1527=B_SPLINE_CURVE_WITH_KNOTS('',3,(#72221,#72222,#72223,#72224,#72225,
#72226),.UNSPECIFIED.,.F.,.F.,(4,2,4),(-0.0021248677897174,-0.00106293276009572,
-1.0000000007246E-6),.UNSPECIFIED.);
#1528=B_SPLINE_CURVE_WITH_KNOTS('',3,(#72265,#72266,#72267,#72268,#72269,
#72270),.UNSPECIFIED.,.F.,.F.,(4,2,4),(0.,0.0198583386780633,0.0397175618609683),
 .UNSPECIFIED.);
#1529=B_SPLINE_CURVE_WITH_KNOTS('',3,(#72283,#72284,#72285,#72286,#72287,
#72288),.UNSPECIFIED.,.F.,.F.,(4,2,4),(0.,0.0198761965838071,0.0397532847185604),
 .UNSPECIFIED.);
#1530=B_SPLINE_CURVE_WITH_KNOTS('',3,(#72340,#72341,#72342,#72343,#72344,
#72345),.UNSPECIFIED.,.F.,.F.,(4,2,4),(0.,0.0199008240900329,0.0398025407218782),
 .UNSPECIFIED.);
#1531=B_SPLINE_CURVE_WITH_KNOTS('',3,(#72358,#72359,#72360,#72361,#72362,
#72363),.UNSPECIFIED.,.F.,.F.,(4,2,4),(0.,0.0199042047189754,0.0398092891731179),
 .UNSPECIFIED.);
#1532=B_SPLINE_CURVE_WITH_KNOTS('',3,(#72411,#72412,#72413,#72414,#72415,
#72416),.UNSPECIFIED.,.F.,.F.,(4,2,4),(0.,0.0198954793789966,0.0397918615887045),
 .UNSPECIFIED.);
#1533=B_SPLINE_CURVE_WITH_KNOTS('',3,(#72456,#72457,#72458,#72459,#72460,
#72461,#72462),.UNSPECIFIED.,.F.,.F.,(4,3,4),(0.,0.5,0.999990117151347),
 .UNSPECIFIED.);
#1534=B_SPLINE_CURVE_WITH_KNOTS('',3,(#72485,#72486,#72487,#72488,#72489,
#72490),.UNSPECIFIED.,.F.,.F.,(4,2,4),(0.,0.0198677119409769,0.0397363340651177),
 .UNSPECIFIED.);
#1535=B_SPLINE_CURVE_WITH_KNOTS('',3,(#72532,#72533,#72534,#72535,#72536,
#72537),.UNSPECIFIED.,.F.,.F.,(4,2,4),(0.,0.0198973966047253,0.0397956843521631),
 .UNSPECIFIED.);
#1536=B_SPLINE_CURVE_WITH_KNOTS('',3,(#72559,#72560,#72561,#72562,#72563,
#72564),.UNSPECIFIED.,.F.,.F.,(4,2,4),(0.,0.0199030680072161,0.0398070347685307),
 .UNSPECIFIED.);
#1537=B_SPLINE_CURVE_WITH_KNOTS('',3,(#72609,#72610,#72611,#72612,#72613,
#72614),.UNSPECIFIED.,.F.,.F.,(4,2,4),(0.,0.0198994178862985,0.0397997368875154),
 .UNSPECIFIED.);
#1538=B_SPLINE_CURVE_WITH_KNOTS('',3,(#72627,#72628,#72629,#72630,#72631,
#72632),.UNSPECIFIED.,.F.,.F.,(4,2,4),(0.,0.0198905179568695,0.0397819072595301),
 .UNSPECIFIED.);
#1539=B_SPLINE_CURVE_WITH_KNOTS('',3,(#72657,#72658,#72659,#72660,#72661,
#72662,#72663),.UNSPECIFIED.,.F.,.F.,(4,3,4),(0.0365944846647013,0.0384615384615384,
0.0431466153076599),.UNSPECIFIED.);
#1540=B_SPLINE_CURVE_WITH_KNOTS('',3,(#72664,#72665,#72666,#72667,#72668,
#72669,#72670,#72671),.UNSPECIFIED.,.F.,.F.,(4,2,2,4),(1.77256738873533E-6,
0.00863675579260533,0.0171409324946532,0.0172810779368845),
 .UNSPECIFIED.);
#1541=B_SPLINE_CURVE_WITH_KNOTS('',3,(#72696,#72697,#72698,#72699,#72700,
#72701),.UNSPECIFIED.,.F.,.F.,(4,2,4),(0.,0.0198536183302958,0.0397081496500012),
 .UNSPECIFIED.);
#1542=B_SPLINE_CURVE_WITH_KNOTS('',3,(#72719,#72720,#72721,#72722,#72723,
#72724),.UNSPECIFIED.,.F.,.F.,(4,2,4),(-0.00212386114999187,-0.00106193096416825,
0.),.UNSPECIFIED.);
#1543=B_SPLINE_CURVE_WITH_KNOTS('',3,(#72725,#72726,#72727,#72728,#72729,
#72730),.UNSPECIFIED.,.F.,.F.,(4,2,4),(9.99998414494249E-7,0.0193527803897854,
0.0387045693971851),.UNSPECIFIED.);
#1544=B_SPLINE_CURVE_WITH_KNOTS('',3,(#72736,#72737,#72738,#72739,#72740,
#72741),.UNSPECIFIED.,.F.,.F.,(4,2,4),(-0.00212486788589273,-0.00106293275882422,
-1.00000000009728E-6),.UNSPECIFIED.);
#1545=B_SPLINE_CURVE_WITH_KNOTS('',3,(#72780,#72781,#72782,#72783,#72784,
#72785),.UNSPECIFIED.,.F.,.F.,(4,2,4),(0.,0.0198583386778968,0.0397175618601019),
 .UNSPECIFIED.);
#1546=B_SPLINE_CURVE_WITH_KNOTS('',3,(#72798,#72799,#72800,#72801,#72802,
#72803),.UNSPECIFIED.,.F.,.F.,(4,2,4),(0.,0.0198761967018805,0.0397532849590274),
 .UNSPECIFIED.);
#1547=B_SPLINE_CURVE_WITH_KNOTS('',3,(#72855,#72856,#72857,#72858,#72859,
#72860),.UNSPECIFIED.,.F.,.F.,(4,2,4),(0.,0.0199008240895138,0.0398025407194746),
 .UNSPECIFIED.);
#1548=B_SPLINE_CURVE_WITH_KNOTS('',3,(#72873,#72874,#72875,#72876,#72877,
#72878),.UNSPECIFIED.,.F.,.F.,(4,2,4),(0.,0.0199042047188044,0.0398092891658421),
 .UNSPECIFIED.);
#1549=B_SPLINE_CURVE_WITH_KNOTS('',3,(#72926,#72927,#72928,#72929,#72930,
#72931),.UNSPECIFIED.,.F.,.F.,(4,2,4),(0.,0.0198954793786522,0.0397918615872593),
 .UNSPECIFIED.);
#1550=B_SPLINE_CURVE_WITH_KNOTS('',3,(#72971,#72972,#72973,#72974,#72975,
#72976,#72977),.UNSPECIFIED.,.F.,.F.,(4,3,4),(0.,0.5,0.99999011715422),
 .UNSPECIFIED.);
#1551=B_SPLINE_CURVE_WITH_KNOTS('',3,(#73000,#73001,#73002,#73003,#73004,
#73005),.UNSPECIFIED.,.F.,.F.,(4,2,4),(0.,0.0198677119426146,0.0397363340713369),
 .UNSPECIFIED.);
#1552=B_SPLINE_CURVE_WITH_KNOTS('',3,(#73047,#73048,#73049,#73050,#73051,
#73052),.UNSPECIFIED.,.F.,.F.,(4,2,4),(0.,0.0198973966035302,0.0397956843468986),
 .UNSPECIFIED.);
#1553=B_SPLINE_CURVE_WITH_KNOTS('',3,(#73074,#73075,#73076,#73077,#73078,
#73079),.UNSPECIFIED.,.F.,.F.,(4,2,4),(0.,0.0199030680084652,0.0398070347735349),
 .UNSPECIFIED.);
#1554=B_SPLINE_CURVE_WITH_KNOTS('',3,(#73121,#73122,#73123,#73124,#73125,
#73126),.UNSPECIFIED.,.F.,.F.,(4,2,4),(0.,0.0198994178853394,0.0397997368837477),
 .UNSPECIFIED.);
#1555=B_SPLINE_CURVE_WITH_KNOTS('',3,(#73146,#73147,#73148,#73149,#73150,
#73151),.UNSPECIFIED.,.F.,.F.,(4,2,4),(0.,0.0198905727746721,0.0397820348055632),
 .UNSPECIFIED.);
#1556=B_SPLINE_CURVE_WITH_KNOTS('',3,(#73176,#73177,#73178,#73179,#73180,
#73181,#73182),.UNSPECIFIED.,.F.,.F.,(4,3,4),(0.0365944846647006,0.0384615384615384,
0.0431466153076602),.UNSPECIFIED.);
#1557=B_SPLINE_CURVE_WITH_KNOTS('',3,(#73183,#73184,#73185,#73186,#73187,
#73188,#73189,#73190),.UNSPECIFIED.,.F.,.F.,(4,2,2,4),(1.77256368440199E-6,
0.00863675579558576,0.0171409356063339,0.0172810807143027),
 .UNSPECIFIED.);
#1558=B_SPLINE_CURVE_WITH_KNOTS('',3,(#73215,#73216,#73217,#73218,#73219,
#73220),.UNSPECIFIED.,.F.,.F.,(4,2,4),(0.,0.0198536183296266,0.0397081496475667),
 .UNSPECIFIED.);
#1559=B_SPLINE_CURVE_WITH_KNOTS('',3,(#73238,#73239,#73240,#73241,#73242,
#73243),.UNSPECIFIED.,.F.,.F.,(4,2,4),(-0.0021238584746236,-0.00106192989366009,
0.),.UNSPECIFIED.);
#1560=B_SPLINE_CURVE_WITH_KNOTS('',3,(#73244,#73245,#73246,#73247,#73248,
#73249),.UNSPECIFIED.,.F.,.F.,(4,2,4),(9.99998415229336E-7,0.0193527803903097,
0.0387045693981831),.UNSPECIFIED.);
#1561=B_SPLINE_CURVE_WITH_KNOTS('',3,(#73255,#73256,#73257,#73258,#73259,
#73260),.UNSPECIFIED.,.F.,.F.,(4,2,4),(-0.00212486797083145,-0.00106293275865109,
-9.99999996147095E-7),.UNSPECIFIED.);
#1562=B_SPLINE_CURVE_WITH_KNOTS('',3,(#73299,#73300,#73301,#73302,#73303,
#73304),.UNSPECIFIED.,.F.,.F.,(4,2,4),(0.,0.0198583386770375,0.0397175618570197),
 .UNSPECIFIED.);
#1563=B_SPLINE_CURVE_WITH_KNOTS('',3,(#73317,#73318,#73319,#73320,#73321,
#73322),.UNSPECIFIED.,.F.,.F.,(4,2,4),(0.,0.0198761965570183,0.039753284662268),
 .UNSPECIFIED.);
#1564=B_SPLINE_CURVE_WITH_KNOTS('',3,(#73374,#73375,#73376,#73377,#73378,
#73379),.UNSPECIFIED.,.F.,.F.,(4,2,4),(0.,0.0199008240890413,0.0398025407175076),
 .UNSPECIFIED.);
#1565=B_SPLINE_CURVE_WITH_KNOTS('',3,(#73392,#73393,#73394,#73395,#73396,
#73397),.UNSPECIFIED.,.F.,.F.,(4,2,4),(0.,0.0199042047190454,0.0398092891796812),
 .UNSPECIFIED.);
#1566=B_SPLINE_CURVE_WITH_KNOTS('',3,(#73445,#73446,#73447,#73448,#73449,
#73450),.UNSPECIFIED.,.F.,.F.,(4,2,4),(0.,0.019895479378126,0.0397918615851958),
 .UNSPECIFIED.);
#1567=B_SPLINE_CURVE_WITH_KNOTS('',3,(#73490,#73491,#73492,#73493,#73494,
#73495,#73496),.UNSPECIFIED.,.F.,.F.,(4,3,4),(0.,0.5,0.999990117157017),
 .UNSPECIFIED.);
#1568=B_SPLINE_CURVE_WITH_KNOTS('',3,(#73519,#73520,#73521,#73522,#73523,
#73524),.UNSPECIFIED.,.F.,.F.,(4,2,4),(0.,0.0198677119443712,0.0397363340782618),
 .UNSPECIFIED.);
#1569=B_SPLINE_CURVE_WITH_KNOTS('',3,(#73566,#73567,#73568,#73569,#73570,
#73571),.UNSPECIFIED.,.F.,.F.,(4,2,4),(0.,0.0198973966024781,0.0397956843428114),
 .UNSPECIFIED.);
#1570=B_SPLINE_CURVE_WITH_KNOTS('',3,(#73593,#73594,#73595,#73596,#73597,
#73598),.UNSPECIFIED.,.F.,.F.,(4,2,4),(0.,0.0199030680104709,0.0398070347819283),
 .UNSPECIFIED.);
#1571=B_SPLINE_CURVE_WITH_KNOTS('',3,(#73643,#73644,#73645,#73646,#73647,
#73648),.UNSPECIFIED.,.F.,.F.,(4,2,4),(0.,0.0198994178844569,0.0397997368800826),
 .UNSPECIFIED.);
#1572=B_SPLINE_CURVE_WITH_KNOTS('',3,(#73661,#73662,#73663,#73664,#73665,
#73666),.UNSPECIFIED.,.F.,.F.,(4,2,4),(0.,0.0198905179569914,0.0397819072575795),
 .UNSPECIFIED.);
#1573=B_SPLINE_CURVE_WITH_KNOTS('',3,(#73691,#73692,#73693,#73694,#73695,
#73696,#73697),.UNSPECIFIED.,.F.,.F.,(4,3,4),(0.0365944846647009,0.0384615384615384,
0.04314661530766),.UNSPECIFIED.);
#1574=B_SPLINE_CURVE_WITH_KNOTS('',3,(#73698,#73699,#73700,#73701,#73702,
#73703,#73704,#73705),.UNSPECIFIED.,.F.,.F.,(4,2,2,4),(1.77349250019423E-6,
0.00863675584712622,0.017140946030412,0.0172810899018738),.UNSPECIFIED.);
#1575=B_SPLINE_CURVE_WITH_KNOTS('',3,(#73730,#73731,#73732,#73733,#73734,
#73735),.UNSPECIFIED.,.F.,.F.,(4,2,4),(0.,0.0198536183292936,0.0397081496458144),
 .UNSPECIFIED.);
#1576=B_SPLINE_CURVE_WITH_KNOTS('',3,(#73753,#73754,#73755,#73756,#73757,
#73758),.UNSPECIFIED.,.F.,.F.,(4,2,4),(-0.00212385697820441,-0.00106192928909173,
0.),.UNSPECIFIED.);
#1577=B_SPLINE_CURVE_WITH_KNOTS('',3,(#73759,#73760,#73761,#73762,#73763,
#73764),.UNSPECIFIED.,.F.,.F.,(4,2,4),(9.99998411255266E-7,0.0193532896046044,
0.0387045796181942),.UNSPECIFIED.);
#1578=B_SPLINE_CURVE_WITH_KNOTS('',3,(#73770,#73771,#73772,#73773,#73774,
#73775),.UNSPECIFIED.,.F.,.F.,(4,2,4),(-0.00212486795133422,-0.0010629327604503,
-9.99999996965017E-7),.UNSPECIFIED.);
#1579=B_SPLINE_CURVE_WITH_KNOTS('',3,(#73814,#73815,#73816,#73817,#73818,
#73819),.UNSPECIFIED.,.F.,.F.,(4,2,4),(0.,0.0198583386764475,0.0397175618547699),
 .UNSPECIFIED.);
#1580=B_SPLINE_CURVE_WITH_KNOTS('',3,(#73832,#73833,#73834,#73835,#73836,
#73837),.UNSPECIFIED.,.F.,.F.,(4,2,4),(0.,0.0198761967067316,0.0397532849617256),
 .UNSPECIFIED.);
#1581=B_SPLINE_CURVE_WITH_KNOTS('',3,(#73889,#73890,#73891,#73892,#73893,
#73894),.UNSPECIFIED.,.F.,.F.,(4,2,4),(0.,0.0199008240884147,0.0398025407150453),
 .UNSPECIFIED.);
#1582=B_SPLINE_CURVE_WITH_KNOTS('',3,(#73907,#73908,#73909,#73910,#73911,
#73912),.UNSPECIFIED.,.F.,.F.,(4,2,4),(0.,0.0199042047189995,0.0398092891650532),
 .UNSPECIFIED.);
#1583=B_SPLINE_CURVE_WITH_KNOTS('',3,(#73960,#73961,#73962,#73963,#73964,
#73965),.UNSPECIFIED.,.F.,.F.,(4,2,4),(0.,0.0198954793777621,0.0397918615838469),
 .UNSPECIFIED.);
#1584=B_SPLINE_CURVE_WITH_KNOTS('',3,(#74005,#74006,#74007,#74008,#74009,
#74010,#74011),.UNSPECIFIED.,.F.,.F.,(4,3,4),(0.,0.5,0.99999011715892),
 .UNSPECIFIED.);
#1585=B_SPLINE_CURVE_WITH_KNOTS('',3,(#74034,#74035,#74036,#74037,#74038,
#74039),.UNSPECIFIED.,.F.,.F.,(4,2,4),(0.,0.0198677119454309,0.0397363340830025),
 .UNSPECIFIED.);
#1586=B_SPLINE_CURVE_WITH_KNOTS('',3,(#74081,#74082,#74083,#74084,#74085,
#74086),.UNSPECIFIED.,.F.,.F.,(4,2,4),(0.,0.0198973966015896,0.0397956843389232),
 .UNSPECIFIED.);
#1587=B_SPLINE_CURVE_WITH_KNOTS('',3,(#74108,#74109,#74110,#74111,#74112,
#74113),.UNSPECIFIED.,.F.,.F.,(4,2,4),(0.,0.0199030680114917,0.0398070347856482),
 .UNSPECIFIED.);
#1588=B_SPLINE_CURVE_WITH_KNOTS('',3,(#74158,#74159,#74160,#74161,#74162,
#74163),.UNSPECIFIED.,.F.,.F.,(4,2,4),(0.,0.0198994178840687,0.0397997368781493),
 .UNSPECIFIED.);
#1589=B_SPLINE_CURVE_WITH_KNOTS('',3,(#74176,#74177,#74178,#74179,#74180,
#74181),.UNSPECIFIED.,.F.,.F.,(4,2,4),(0.,0.019890517957065,0.0397819072698597),
 .UNSPECIFIED.);
#1590=B_SPLINE_CURVE_WITH_KNOTS('',3,(#74206,#74207,#74208,#74209,#74210,
#74211,#74212),.UNSPECIFIED.,.F.,.F.,(4,3,4),(0.0365944846647012,0.0384615384615384,
0.0431466153076599),.UNSPECIFIED.);
#1591=B_SPLINE_CURVE_WITH_KNOTS('',3,(#74213,#74214,#74215,#74216,#74217,
#74218,#74219,#74220),.UNSPECIFIED.,.F.,.F.,(4,2,2,4),(1.7725636922617E-6,
0.00863675577788347,0.0171409340540784,0.0172810793308343),
 .UNSPECIFIED.);
#1592=B_SPLINE_CURVE_WITH_KNOTS('',3,(#74245,#74246,#74247,#74248,#74249,
#74250),.UNSPECIFIED.,.F.,.F.,(4,2,4),(0.,0.0198536183279069,0.0397081496402279),
 .UNSPECIFIED.);
#1593=B_SPLINE_CURVE_WITH_KNOTS('',3,(#74268,#74269,#74270,#74271,#74272,
#74273),.UNSPECIFIED.,.F.,.F.,(4,2,4),(-0.00212385473939844,-0.00106192839292651,
0.),.UNSPECIFIED.);
#1594=B_SPLINE_CURVE_WITH_KNOTS('',3,(#74274,#74275,#74276,#74277,#74278,
#74279),.UNSPECIFIED.,.F.,.F.,(4,2,4),(9.99998421610724E-7,0.0193522803912436,
0.0387045693987194),.UNSPECIFIED.);
#1595=B_SPLINE_CURVE_WITH_KNOTS('',3,(#74285,#74286,#74287,#74288,#74289,
#74290),.UNSPECIFIED.,.F.,.F.,(4,2,4),(-0.0021248678892231,-0.00106293275681277,
-1.00000000261284E-6),.UNSPECIFIED.);
#1596=B_SPLINE_CURVE_WITH_KNOTS('',3,(#74329,#74330,#74331,#74332,#74333,
#74334),.UNSPECIFIED.,.F.,.F.,(4,2,4),(0.,0.0198583386753345,0.039717561849955),
 .UNSPECIFIED.);
#1597=B_SPLINE_CURVE_WITH_KNOTS('',3,(#74347,#74348,#74349,#74350,#74351,
#74352),.UNSPECIFIED.,.F.,.F.,(4,2,4),(0.,0.0198761967127292,0.0397532849960256),
 .UNSPECIFIED.);
#1598=B_SPLINE_CURVE_WITH_KNOTS('',3,(#74404,#74405,#74406,#74407,#74408,
#74409),.UNSPECIFIED.,.F.,.F.,(4,2,4),(0.,0.0199008240880627,0.0398025407135643),
 .UNSPECIFIED.);
#1599=B_SPLINE_CURVE_WITH_KNOTS('',3,(#74422,#74423,#74424,#74425,#74426,
#74427),.UNSPECIFIED.,.F.,.F.,(4,2,4),(0.,0.0199042047187738,0.0398092891784042),
 .UNSPECIFIED.);
#1600=B_SPLINE_CURVE_WITH_KNOTS('',3,(#74475,#74476,#74477,#74478,#74479,
#74480),.UNSPECIFIED.,.F.,.F.,(4,2,4),(0.,0.0198954793773227,0.0397918615821683),
 .UNSPECIFIED.);
#1601=B_SPLINE_CURVE_WITH_KNOTS('',3,(#74520,#74521,#74522,#74523,#74524,
#74525,#74526),.UNSPECIFIED.,.F.,.F.,(4,3,4),(0.,0.5,0.99999011716107),
 .UNSPECIFIED.);
#1602=B_SPLINE_CURVE_WITH_KNOTS('',3,(#74549,#74550,#74551,#74552,#74553,
#74554),.UNSPECIFIED.,.F.,.F.,(4,2,4),(0.,0.0198677119468207,0.0397363340885719),
 .UNSPECIFIED.);
#1603=B_SPLINE_CURVE_WITH_KNOTS('',3,(#74596,#74597,#74598,#74599,#74600,
#74601),.UNSPECIFIED.,.F.,.F.,(4,2,4),(0.,0.0198973966000579,0.0397956843329122),
 .UNSPECIFIED.);
#1604=B_SPLINE_CURVE_WITH_KNOTS('',3,(#74623,#74624,#74625,#74626,#74627,
#74628),.UNSPECIFIED.,.F.,.F.,(4,2,4),(0.,0.01990306801314,0.0398070347925831),
 .UNSPECIFIED.);
#1605=B_SPLINE_CURVE_WITH_KNOTS('',3,(#74673,#74674,#74675,#74676,#74677,
#74678),.UNSPECIFIED.,.F.,.F.,(4,2,4),(0.,0.0198994178828134,0.0397997368733775),
 .UNSPECIFIED.);
#1606=B_SPLINE_CURVE_WITH_KNOTS('',3,(#74691,#74692,#74693,#74694,#74695,
#74696),.UNSPECIFIED.,.F.,.F.,(4,2,4),(0.,0.0198905179570001,0.0397819072527676),
 .UNSPECIFIED.);
#1607=B_SPLINE_CURVE_WITH_KNOTS('',3,(#74721,#74722,#74723,#74724,#74725,
#74726,#74727),.UNSPECIFIED.,.F.,.F.,(4,3,4),(0.0365944846647015,0.0384615384615384,
0.0431466153076602),.UNSPECIFIED.);
#1608=B_SPLINE_CURVE_WITH_KNOTS('',3,(#74728,#74729,#74730,#74731,#74732,
#74733,#74734,#74735),.UNSPECIFIED.,.F.,.F.,(4,2,2,4),(1.77256369998672E-6,
0.00863675578444654,0.0171409282122659,0.0172810740976024),
 .UNSPECIFIED.);
#1609=B_SPLINE_CURVE_WITH_KNOTS('',3,(#74760,#74761,#74762,#74763,#74764,
#74765),.UNSPECIFIED.,.F.,.F.,(4,2,4),(0.,0.0198536183267392,0.039708149635655),
 .UNSPECIFIED.);
#1610=B_SPLINE_CURVE_WITH_KNOTS('',3,(#74783,#74784,#74785,#74786,#74787,
#74788),.UNSPECIFIED.,.F.,.F.,(4,2,4),(-0.00212385284338186,-0.00106192763760952,
0.),.UNSPECIFIED.);
#1611=B_SPLINE_CURVE_WITH_KNOTS('',3,(#74789,#74790,#74791,#74792,#74793,
#74794),.UNSPECIFIED.,.F.,.F.,(4,2,4),(9.99998414498686E-7,0.0193532903994283,
0.0387045796339771),.UNSPECIFIED.);
#1612=B_SPLINE_CURVE_WITH_KNOTS('',3,(#74800,#74801,#74802,#74803,#74804,
#74805),.UNSPECIFIED.,.F.,.F.,(4,2,4),(-0.00212486777295456,-0.00106293276548707,
-1.00000000054809E-6),.UNSPECIFIED.);
#1613=B_SPLINE_CURVE_WITH_KNOTS('',3,(#74844,#74845,#74846,#74847,#74848,
#74849),.UNSPECIFIED.,.F.,.F.,(4,2,4),(0.,0.0198583386744434,0.0397175618466529),
 .UNSPECIFIED.);
#1614=B_SPLINE_CURVE_WITH_KNOTS('',3,(#74862,#74863,#74864,#74865,#74866,
#74867),.UNSPECIFIED.,.F.,.F.,(4,2,4),(0.,0.0198761967069154,0.0397532849758011),
 .UNSPECIFIED.);
#1615=B_SPLINE_CURVE_WITH_KNOTS('',3,(#74919,#74920,#74921,#74922,#74923,
#74924),.UNSPECIFIED.,.F.,.F.,(4,2,4),(0.,0.0199008240869926,0.0398025407092003),
 .UNSPECIFIED.);
#1616=B_SPLINE_CURVE_WITH_KNOTS('',3,(#74937,#74938,#74939,#74940,#74941,
#74942),.UNSPECIFIED.,.F.,.F.,(4,2,4),(0.,0.0199042047190074,0.0398092891779339),
 .UNSPECIFIED.);
#1617=B_SPLINE_CURVE_WITH_KNOTS('',3,(#74990,#74991,#74992,#74993,#74994,
#74995),.UNSPECIFIED.,.F.,.F.,(4,2,4),(0.,0.0198954793762232,0.0397918615774369),
 .UNSPECIFIED.);
#1618=B_SPLINE_CURVE_WITH_KNOTS('',3,(#75035,#75036,#75037,#75038,#75039,
#75040,#75041),.UNSPECIFIED.,.F.,.F.,(4,3,4),(0.,0.5,0.999990117163183),
 .UNSPECIFIED.);
#1619=B_SPLINE_CURVE_WITH_KNOTS('',3,(#75064,#75065,#75066,#75067,#75068,
#75069),.UNSPECIFIED.,.F.,.F.,(4,2,4),(0.,0.0198677119479282,0.0397363340928585),
 .UNSPECIFIED.);
#1620=B_SPLINE_CURVE_WITH_KNOTS('',3,(#75111,#75112,#75113,#75114,#75115,
#75116),.UNSPECIFIED.,.F.,.F.,(4,2,4),(0.,0.0198973965989467,0.039795684329128),
 .UNSPECIFIED.);
#1621=B_SPLINE_CURVE_WITH_KNOTS('',3,(#75138,#75139,#75140,#75141,#75142,
#75143),.UNSPECIFIED.,.F.,.F.,(4,2,4),(0.,0.0199030680141118,0.0398070347963341),
 .UNSPECIFIED.);
#1622=B_SPLINE_CURVE_WITH_KNOTS('',3,(#75188,#75189,#75190,#75191,#75192,
#75193),.UNSPECIFIED.,.F.,.F.,(4,2,4),(0.,0.0198994178815675,0.0397997368683613),
 .UNSPECIFIED.);
#1623=B_SPLINE_CURVE_WITH_KNOTS('',3,(#75206,#75207,#75208,#75209,#75210,
#75211),.UNSPECIFIED.,.F.,.F.,(4,2,4),(0.,0.0198905179569802,0.0397819072620881),
 .UNSPECIFIED.);
#1624=B_SPLINE_CURVE_WITH_KNOTS('',3,(#75236,#75237,#75238,#75239,#75240,
#75241,#75242),.UNSPECIFIED.,.F.,.F.,(4,3,4),(0.0365944846647007,0.0384615384615384,
0.0431466153076595),.UNSPECIFIED.);
#1625=B_SPLINE_CURVE_WITH_KNOTS('',3,(#75243,#75244,#75245,#75246,#75247,
#75248,#75249,#75250),.UNSPECIFIED.,.F.,.F.,(4,2,2,4),(1.77349269128769E-6,
0.00863675576722594,0.0171409186233939,0.0172810654209329),
 .UNSPECIFIED.);
#1626=B_SPLINE_CURVE_WITH_KNOTS('',3,(#75275,#75276,#75277,#75278,#75279,
#75280),.UNSPECIFIED.,.F.,.F.,(4,2,4),(0.,0.0198536183260036,0.0397081496324284),
 .UNSPECIFIED.);
#1627=B_SPLINE_CURVE_WITH_KNOTS('',3,(#75298,#75299,#75300,#75301,#75302,
#75303),.UNSPECIFIED.,.F.,.F.,(4,2,4),(-0.00212385118147093,-0.00106192697594493,
0.),.UNSPECIFIED.);
#1628=B_SPLINE_CURVE_WITH_KNOTS('',3,(#75304,#75305,#75306,#75307,#75308,
#75309),.UNSPECIFIED.,.F.,.F.,(4,2,4),(9.99998416995636E-7,0.0193522795956267,
0.0387045693813799),.UNSPECIFIED.);
#1629=B_SPLINE_CURVE_WITH_KNOTS('',3,(#75315,#75316,#75317,#75318,#75319,
#75320),.UNSPECIFIED.,.F.,.F.,(4,2,4),(-0.00212486747589103,-0.00106293275719458,
-9.99999997170799E-7),.UNSPECIFIED.);
#1630=B_SPLINE_CURVE_WITH_KNOTS('',3,(#75359,#75360,#75361,#75362,#75363,
#75364),.UNSPECIFIED.,.F.,.F.,(4,2,4),(0.,0.0198583386732508,0.0397175618416976),
 .UNSPECIFIED.);
#1631=B_SPLINE_CURVE_WITH_KNOTS('',3,(#75377,#75378,#75379,#75380,#75381,
#75382),.UNSPECIFIED.,.F.,.F.,(4,2,4),(0.,0.019876196698315,0.0397532849596158),
 .UNSPECIFIED.);
#1632=B_SPLINE_CURVE_WITH_KNOTS('',3,(#75434,#75435,#75436,#75437,#75438,
#75439),.UNSPECIFIED.,.F.,.F.,(4,2,4),(0.,0.0199008240858154,0.0398025407041441),
 .UNSPECIFIED.);
#1633=B_SPLINE_CURVE_WITH_KNOTS('',3,(#75452,#75453,#75454,#75455,#75456,
#75457),.UNSPECIFIED.,.F.,.F.,(4,2,4),(0.,0.019904204718824,0.0398092891828929),
 .UNSPECIFIED.);
#1634=B_SPLINE_CURVE_WITH_KNOTS('',3,(#75505,#75506,#75507,#75508,#75509,
#75510),.UNSPECIFIED.,.F.,.F.,(4,2,4),(0.,0.0198954793749717,0.0397918615725202),
 .UNSPECIFIED.);
#1635=B_SPLINE_CURVE_WITH_KNOTS('',3,(#75550,#75551,#75552,#75553,#75554,
#75555,#75556),.UNSPECIFIED.,.F.,.F.,(4,3,4),(0.,0.5,0.999990117164291),
 .UNSPECIFIED.);
#1636=B_SPLINE_CURVE_WITH_KNOTS('',3,(#75579,#75580,#75581,#75582,#75583,
#75584),.UNSPECIFIED.,.F.,.F.,(4,2,4),(0.,0.0198677119492189,0.0397363340978274),
 .UNSPECIFIED.);
#1637=B_SPLINE_CURVE_WITH_KNOTS('',3,(#75626,#75627,#75628,#75629,#75630,
#75631),.UNSPECIFIED.,.F.,.F.,(4,2,4),(0.,0.0198973965974829,0.0397956843228074),
 .UNSPECIFIED.);
#1638=B_SPLINE_CURVE_WITH_KNOTS('',3,(#75653,#75654,#75655,#75656,#75657,
#75658),.UNSPECIFIED.,.F.,.F.,(4,2,4),(0.,0.0199030680152636,0.0398070348010775),
 .UNSPECIFIED.);
#1639=B_SPLINE_CURVE_WITH_KNOTS('',3,(#75700,#75701,#75702,#75703,#75704,
#75705),.UNSPECIFIED.,.F.,.F.,(4,2,4),(0.,0.0198994178801307,0.0397997368625414),
 .UNSPECIFIED.);
#1640=B_SPLINE_CURVE_WITH_KNOTS('',3,(#75725,#75726,#75727,#75728,#75729,
#75730),.UNSPECIFIED.,.F.,.F.,(4,2,4),(0.,0.019890572780449,0.0397820348288668),
 .UNSPECIFIED.);
#1641=B_SPLINE_CURVE_WITH_KNOTS('',3,(#75755,#75756,#75757,#75758,#75759,
#75760,#75761),.UNSPECIFIED.,.F.,.F.,(4,3,4),(0.0365944846647011,0.0384615384615384,
0.0431466153076599),.UNSPECIFIED.);
#1642=B_SPLINE_CURVE_WITH_KNOTS('',3,(#75762,#75763,#75764,#75765,#75766,
#75767,#75768,#75769),.UNSPECIFIED.,.F.,.F.,(4,2,2,4),(1.77256738234578E-6,
0.00863675579810489,0.0171409372906893,0.0172810822319369),
 .UNSPECIFIED.);
#1643=B_SPLINE_CURVE_WITH_KNOTS('',3,(#75794,#75795,#75796,#75797,#75798,
#75799),.UNSPECIFIED.,.F.,.F.,(4,2,4),(0.,0.019853618324023,0.0397081496247761),
 .UNSPECIFIED.);
#1644=B_SPLINE_CURVE_WITH_KNOTS('',3,(#75817,#75818,#75819,#75820,#75821,
#75822),.UNSPECIFIED.,.F.,.F.,(4,2,4),(-0.00212384980647466,-0.00106192642804374,
0.),.UNSPECIFIED.);
#1645=B_SPLINE_CURVE_WITH_KNOTS('',3,(#75823,#75824,#75825,#75826,#75827,
#75828),.UNSPECIFIED.,.F.,.F.,(4,2,4),(9.99998416490131E-7,0.0193522803905122,
0.0387045693972246),.UNSPECIFIED.);
#1646=B_SPLINE_CURVE_WITH_KNOTS('',3,(#75834,#75835,#75836,#75837,#75838,
#75839),.UNSPECIFIED.,.F.,.F.,(4,2,4),(-0.00212486726074812,-0.00106293276493776,
-9.99999998992909E-7),.UNSPECIFIED.);
#1647=B_SPLINE_CURVE_WITH_KNOTS('',3,(#75878,#75879,#75880,#75881,#75882,
#75883),.UNSPECIFIED.,.F.,.F.,(4,2,4),(0.,0.0198583386718413,0.0397175618360036),
 .UNSPECIFIED.);
#1648=B_SPLINE_CURVE_WITH_KNOTS('',3,(#75896,#75897,#75898,#75899,#75900,
#75901),.UNSPECIFIED.,.F.,.F.,(4,2,4),(0.,0.0198761965659768,0.0397532846823463),
 .UNSPECIFIED.);
#1649=B_SPLINE_CURVE_WITH_KNOTS('',3,(#75953,#75954,#75955,#75956,#75957,
#75958),.UNSPECIFIED.,.F.,.F.,(4,2,4),(0.,0.0199008240845495,0.0398025406993579),
 .UNSPECIFIED.);
#1650=B_SPLINE_CURVE_WITH_KNOTS('',3,(#75971,#75972,#75973,#75974,#75975,
#75976),.UNSPECIFIED.,.F.,.F.,(4,2,4),(0.,0.0199042047188238,0.0398092891624507),
 .UNSPECIFIED.);
#1651=B_SPLINE_CURVE_WITH_KNOTS('',3,(#76024,#76025,#76026,#76027,#76028,
#76029),.UNSPECIFIED.,.F.,.F.,(4,2,4),(0.,0.0198954793737053,0.0397918615673638),
 .UNSPECIFIED.);
#1652=B_SPLINE_CURVE_WITH_KNOTS('',3,(#76069,#76070,#76071,#76072,#76073,
#76074,#76075),.UNSPECIFIED.,.F.,.F.,(4,3,4),(0.,0.5,0.999990117165551),
 .UNSPECIFIED.);
#1653=B_SPLINE_CURVE_WITH_KNOTS('',3,(#76098,#76099,#76100,#76101,#76102,
#76103),.UNSPECIFIED.,.F.,.F.,(4,2,4),(0.,0.0198677119501225,0.0397363341016526),
 .UNSPECIFIED.);
#1654=B_SPLINE_CURVE_WITH_KNOTS('',3,(#76145,#76146,#76147,#76148,#76149,
#76150),.UNSPECIFIED.,.F.,.F.,(4,2,4),(0.,0.0198973965964354,0.0397956843184013),
 .UNSPECIFIED.);
#1655=B_SPLINE_CURVE_WITH_KNOTS('',3,(#76172,#76173,#76174,#76175,#76176,
#76177),.UNSPECIFIED.,.F.,.F.,(4,2,4),(0.,0.0199030680160421,0.0398070348041842),
 .UNSPECIFIED.);
#1656=B_SPLINE_CURVE_WITH_KNOTS('',3,(#76222,#76223,#76224,#76225,#76226,
#76227),.UNSPECIFIED.,.F.,.F.,(4,2,4),(0.,0.0198994178785787,0.0397997368562093),
 .UNSPECIFIED.);
#1657=B_SPLINE_CURVE_WITH_KNOTS('',3,(#76240,#76241,#76242,#76243,#76244,
#76245),.UNSPECIFIED.,.F.,.F.,(4,2,4),(0.,0.019890517956938,0.0397819072549784),
 .UNSPECIFIED.);
#1658=B_SPLINE_CURVE_WITH_KNOTS('',3,(#76271,#76272,#76273,#76274,#76275,
#76276),.UNSPECIFIED.,.F.,.F.,(4,2,4),(0.036594484664701,0.0384615384615384,
0.0431466153076599),.UNSPECIFIED.);
#1659=B_SPLINE_CURVE_WITH_KNOTS('',3,(#76277,#76278,#76279,#76280,#76281,
#76282,#76283),.UNSPECIFIED.,.F.,.F.,(4,3,4),(0.,0.00863415824006578,0.0172757258251161),
 .UNSPECIFIED.);
#1660=B_SPLINE_CURVE_WITH_KNOTS('',3,(#76308,#76309,#76310,#76311,#76312,
#76313),.UNSPECIFIED.,.F.,.F.,(4,2,4),(0.,0.0198541182823923,0.0397081495471127),
 .UNSPECIFIED.);
#1661=B_SPLINE_CURVE_WITH_KNOTS('',3,(#76326,#76327,#76328,#76329,#76330,
#76331),.UNSPECIFIED.,.F.,.F.,(4,2,4),(-0.00212384884036098,-0.00106192603334971,
0.),.UNSPECIFIED.);
#1662=B_SPLINE_CURVE_WITH_KNOTS('',3,(#76332,#76333,#76334,#76335,#76336,
#76337),.UNSPECIFIED.,.F.,.F.,(4,2,4),(9.99998417286137E-7,0.0193522803914762,
0.0387045693990307),.UNSPECIFIED.);
#1663=B_SPLINE_CURVE_WITH_KNOTS('',3,(#76343,#76344,#76345,#76346,#76347,
#76348),.UNSPECIFIED.,.F.,.F.,(4,2,4),(-0.00212486683933188,-0.0010629327524213,
-9.99999998585899E-7),.UNSPECIFIED.);
#1664=B_SPLINE_CURVE_WITH_KNOTS('',3,(#76387,#76388,#76389,#76390,#76391,
#76392),.UNSPECIFIED.,.F.,.F.,(4,2,4),(0.,0.0198583386710425,0.0397175618327234),
 .UNSPECIFIED.);
#1665=B_SPLINE_CURVE_WITH_KNOTS('',3,(#76405,#76406,#76407,#76408,#76409,
#76410),.UNSPECIFIED.,.F.,.F.,(4,2,4),(0.,0.0198761965784973,0.0397532847182389),
 .UNSPECIFIED.);
#1666=B_SPLINE_CURVE_WITH_KNOTS('',3,(#76462,#76463,#76464,#76465,#76466,
#76467),.UNSPECIFIED.,.F.,.F.,(4,2,4),(0.,0.0199008240829753,0.0398025406932351),
 .UNSPECIFIED.);
#1667=B_SPLINE_CURVE_WITH_KNOTS('',3,(#76480,#76481,#76482,#76483,#76484,
#76485),.UNSPECIFIED.,.F.,.F.,(4,2,4),(0.,0.0199047046187306,0.0398092889177888),
 .UNSPECIFIED.);
#1668=B_SPLINE_CURVE_WITH_KNOTS('',3,(#76533,#76534,#76535,#76536,#76537,
#76538),.UNSPECIFIED.,.F.,.F.,(4,2,4),(0.,0.0198954793723645,0.0397918615620052),
 .UNSPECIFIED.);
#1669=B_SPLINE_CURVE_WITH_KNOTS('',3,(#76578,#76579,#76580,#76581,#76582,
#76583,#76584),.UNSPECIFIED.,.F.,.F.,(4,3,4),(0.,0.5,0.999990117166381),
 .UNSPECIFIED.);
#1670=B_SPLINE_CURVE_WITH_KNOTS('',3,(#76607,#76608,#76609,#76610,#76611,
#76612),.UNSPECIFIED.,.F.,.F.,(4,2,4),(0.,0.0198677119506905,0.0397363341039637),
 .UNSPECIFIED.);
#1671=B_SPLINE_CURVE_WITH_KNOTS('',3,(#76654,#76655,#76656,#76657,#76658,
#76659),.UNSPECIFIED.,.F.,.F.,(4,2,4),(0.,0.0198973965943807,0.0397956843103301),
 .UNSPECIFIED.);
#1672=B_SPLINE_CURVE_WITH_KNOTS('',3,(#76681,#76682,#76683,#76684,#76685,
#76686),.UNSPECIFIED.,.F.,.F.,(4,2,4),(0.,0.0199030680172143,0.0398070348088722),
 .UNSPECIFIED.);
#1673=B_SPLINE_CURVE_WITH_KNOTS('',3,(#76728,#76729,#76730,#76731,#76732,
#76733),.UNSPECIFIED.,.F.,.F.,(4,2,4),(0.,0.0198994178771943,0.0397997368507428),
 .UNSPECIFIED.);
#1674=B_SPLINE_CURVE_WITH_KNOTS('',3,(#76753,#76754,#76755,#76756,#76757,
#76758),.UNSPECIFIED.,.F.,.F.,(4,2,4),(0.,0.0198905727828279,0.0397820348383145),
 .UNSPECIFIED.);
#1675=B_SPLINE_CURVE_WITH_KNOTS('',3,(#76783,#76784,#76785,#76786,#76787,
#76788,#76789),.UNSPECIFIED.,.F.,.F.,(4,3,4),(0.0365944846647011,0.0384615384615384,
0.0431466153076597),.UNSPECIFIED.);
#1676=B_SPLINE_CURVE_WITH_KNOTS('',3,(#76790,#76791,#76792,#76793,#76794,
#76795,#76796,#76797),.UNSPECIFIED.,.F.,.F.,(4,2,2,4),(1.77349269003237E-6,
0.00863675577167021,0.0171409216007662,0.0172810680711004),
 .UNSPECIFIED.);
#1677=B_SPLINE_CURVE_WITH_KNOTS('',3,(#76822,#76823,#76824,#76825,#76826,
#76827),.UNSPECIFIED.,.F.,.F.,(4,2,4),(0.,0.0198536183208147,0.0397081496118954),
 .UNSPECIFIED.);
#1678=B_SPLINE_CURVE_WITH_KNOTS('',3,(#76845,#76846,#76847,#76848,#76849,
#76850),.UNSPECIFIED.,.F.,.F.,(4,2,4),(-0.00212384825724064,-0.00106192581024466,
0.),.UNSPECIFIED.);
#1679=B_SPLINE_CURVE_WITH_KNOTS('',3,(#76851,#76852,#76853,#76854,#76855,
#76856),.UNSPECIFIED.,.F.,.F.,(4,2,4),(9.99998417360777E-7,0.0193522795962004,
0.0387045693826146),.UNSPECIFIED.);
#1680=B_SPLINE_CURVE_WITH_KNOTS('',3,(#76862,#76863,#76864,#76865,#76866,
#76867),.UNSPECIFIED.,.F.,.F.,(4,2,4),(-0.00212486648408312,-0.00106293275900954,
-9.99999996604845E-7),.UNSPECIFIED.);
#1681=B_SPLINE_CURVE_WITH_KNOTS('',3,(#76903,#76904,#76905,#76906,#76907,
#76908),.UNSPECIFIED.,.F.,.F.,(4,2,4),(0.,0.0198583386697237,0.0397175618277278),
 .UNSPECIFIED.);
#1682=B_SPLINE_CURVE_WITH_KNOTS('',3,(#76928,#76929,#76930,#76931,#76932,
#76933),.UNSPECIFIED.,.F.,.F.,(4,2,4),(0.,0.0198762582556093,0.0397534248900765),
 .UNSPECIFIED.);
#1683=B_SPLINE_CURVE_WITH_KNOTS('',3,(#76985,#76986,#76987,#76988,#76989,
#76990),.UNSPECIFIED.,.F.,.F.,(4,2,4),(0.,0.019901323992909,0.0398025404511413),
 .UNSPECIFIED.);
#1684=B_SPLINE_CURVE_WITH_KNOTS('',3,(#77003,#77004,#77005,#77006,#77007,
#77008),.UNSPECIFIED.,.F.,.F.,(4,2,4),(0.,0.019904204713085,0.0398092891717569),
 .UNSPECIFIED.);
#1685=B_SPLINE_CURVE_WITH_KNOTS('',3,(#77056,#77057,#77058,#77059,#77060,
#77061),.UNSPECIFIED.,.F.,.F.,(4,2,4),(0.,0.0198954793706761,0.0397918615552283),
 .UNSPECIFIED.);
#1686=B_SPLINE_CURVE_WITH_KNOTS('',3,(#77101,#77102,#77103,#77104,#77105,
#77106,#77107),.UNSPECIFIED.,.F.,.F.,(4,3,4),(0.,0.5,0.999990117166621),
 .UNSPECIFIED.);
#1687=B_SPLINE_CURVE_WITH_KNOTS('',3,(#77130,#77131,#77132,#77133,#77134,
#77135),.UNSPECIFIED.,.F.,.F.,(4,2,4),(0.,0.0198677119511838,0.0397363341058345),
 .UNSPECIFIED.);
#1688=B_SPLINE_CURVE_WITH_KNOTS('',3,(#77177,#77178,#77179,#77180,#77181,
#77182),.UNSPECIFIED.,.F.,.F.,(4,2,4),(0.,0.0198973965935688,0.0397956843067912),
 .UNSPECIFIED.);
#1689=B_SPLINE_CURVE_WITH_KNOTS('',3,(#77204,#77205,#77206,#77207,#77208,
#77209),.UNSPECIFIED.,.F.,.F.,(4,2,4),(0.,0.0199030680177893,0.0398070348110941),
 .UNSPECIFIED.);
#1690=B_SPLINE_CURVE_WITH_KNOTS('',3,(#77254,#77255,#77256,#77257,#77258,
#77259),.UNSPECIFIED.,.F.,.F.,(4,2,4),(0.,0.0198994178756067,0.0397997368447963),
 .UNSPECIFIED.);
#1691=B_SPLINE_CURVE_WITH_KNOTS('',3,(#77272,#77273,#77274,#77275,#77276,
#77277),.UNSPECIFIED.,.F.,.F.,(4,2,4),(0.,0.0198905179569198,0.039781907258255),
 .UNSPECIFIED.);
#1692=B_SPLINE_CURVE_WITH_KNOTS('',3,(#77302,#77303,#77304,#77305,#77306,
#77307,#77308),.UNSPECIFIED.,.F.,.F.,(4,3,4),(0.0365944846647018,0.0384615384615384,
0.0431466153076603),.UNSPECIFIED.);
#1693=B_SPLINE_CURVE_WITH_KNOTS('',3,(#77309,#77310,#77311,#77312,#77313,
#77314,#77315,#77316),.UNSPECIFIED.,.F.,.F.,(4,2,2,4),(1.7734928133057E-6,
0.00863675575681659,0.0171409114737263,0.017281059029724),.UNSPECIFIED.);
#1694=B_SPLINE_CURVE_WITH_KNOTS('',3,(#77341,#77342,#77343,#77344,#77345,
#77346),.UNSPECIFIED.,.F.,.F.,(4,2,4),(0.,0.0198536183197665,0.0397081496077481),
 .UNSPECIFIED.);
#1695=B_SPLINE_CURVE_WITH_KNOTS('',3,(#77364,#77365,#77366,#77367,#77368,
#77369),.UNSPECIFIED.,.F.,.F.,(4,2,4),(-0.0021238480623822,-0.00106192573417119,
0.),.UNSPECIFIED.);
#1696=B_SPLINE_CURVE_WITH_KNOTS('',3,(#77370,#77371,#77372,#77373,#77374,
#77375),.UNSPECIFIED.,.F.,.F.,(4,2,4),(9.99998409595905E-7,0.0193532896051288,
0.0387045796195939),.UNSPECIFIED.);
#1697=B_SPLINE_CURVE_WITH_KNOTS('',3,(#77381,#77382,#77383,#77384,#77385,
#77386),.UNSPECIFIED.,.F.,.F.,(4,2,4),(-0.00212486601988817,-0.00106293275364175,
-1.00000000020982E-6),.UNSPECIFIED.);
#1698=B_SPLINE_CURVE_WITH_KNOTS('',3,(#77425,#77426,#77427,#77428,#77429,
#77430),.UNSPECIFIED.,.F.,.F.,(4,2,4),(0.,0.0198583386674524,0.0397175618184792),
 .UNSPECIFIED.);
#1699=B_SPLINE_CURVE_WITH_KNOTS('',3,(#77443,#77444,#77445,#77446,#77447,
#77448),.UNSPECIFIED.,.F.,.F.,(4,2,4),(0.,0.0198761967044215,0.039753284959996),
 .UNSPECIFIED.);
#1700=B_SPLINE_CURVE_WITH_KNOTS('',3,(#77500,#77501,#77502,#77503,#77504,
#77505),.UNSPECIFIED.,.F.,.F.,(4,2,4),(0.,0.0199008240805986,0.0398025406833724),
 .UNSPECIFIED.);
#1701=B_SPLINE_CURVE_WITH_KNOTS('',3,(#77525,#77526,#77527,#77528,#77529,
#77530),.UNSPECIFIED.,.F.,.F.,(4,2,4),(0.,0.0199042622206626,0.039809421612776),
 .UNSPECIFIED.);
#1702=B_SPLINE_CURVE_WITH_KNOTS('',3,(#77578,#77579,#77580,#77581,#77582,
#77583),.UNSPECIFIED.,.F.,.F.,(4,2,4),(0.,0.0198954793698275,0.0397918615516674),
 .UNSPECIFIED.);
#1703=B_SPLINE_CURVE_WITH_KNOTS('',3,(#77623,#77624,#77625,#77626,#77627,
#77628,#77629),.UNSPECIFIED.,.F.,.F.,(4,3,4),(0.,0.5,0.999990117166003),
 .UNSPECIFIED.);
#1704=B_SPLINE_CURVE_WITH_KNOTS('',3,(#77652,#77653,#77654,#77655,#77656,
#77657),.UNSPECIFIED.,.F.,.F.,(4,2,4),(0.,0.0198677119515248,0.0397363341074989),
 .UNSPECIFIED.);
#1705=B_SPLINE_CURVE_WITH_KNOTS('',3,(#77699,#77700,#77701,#77702,#77703,
#77704),.UNSPECIFIED.,.F.,.F.,(4,2,4),(0.,0.0198973965915467,0.0397956842989783),
 .UNSPECIFIED.);
#1706=B_SPLINE_CURVE_WITH_KNOTS('',3,(#77726,#77727,#77728,#77729,#77730,
#77731),.UNSPECIFIED.,.F.,.F.,(4,2,4),(0.,0.0199030680180883,0.0398070348124307),
 .UNSPECIFIED.);
#1707=B_SPLINE_CURVE_WITH_KNOTS('',3,(#77776,#77777,#77778,#77779,#77780,
#77781),.UNSPECIFIED.,.F.,.F.,(4,2,4),(0.,0.0198994178738356,0.0397997368373613),
 .UNSPECIFIED.);
#1708=B_SPLINE_CURVE_WITH_KNOTS('',3,(#77794,#77795,#77796,#77797,#77798,
#77799),.UNSPECIFIED.,.F.,.F.,(4,2,4),(0.,0.0198905179569007,0.0397819072607639),
 .UNSPECIFIED.);
#1709=B_SPLINE_CURVE_WITH_KNOTS('',3,(#77824,#77825,#77826,#77827,#77828,
#77829,#77830),.UNSPECIFIED.,.F.,.F.,(4,3,4),(0.0365944846647006,0.0384615384615384,
0.0431466153076599),.UNSPECIFIED.);
#1710=B_SPLINE_CURVE_WITH_KNOTS('',3,(#77831,#77832,#77833,#77834,#77835,
#77836,#77837,#77838),.UNSPECIFIED.,.F.,.F.,(4,2,2,4),(1.77349264648523E-6,
0.00863675580432023,0.017140932899279,0.0172810781627562),.UNSPECIFIED.);
#1711=B_SPLINE_CURVE_WITH_KNOTS('',3,(#77863,#77864,#77865,#77866,#77867,
#77868),.UNSPECIFIED.,.F.,.F.,(4,2,4),(0.,0.0198536183179197,0.0397081496007127),
 .UNSPECIFIED.);
#1712=B_SPLINE_CURVE_WITH_KNOTS('',3,(#77886,#77887,#77888,#77889,#77890,
#77891),.UNSPECIFIED.,.F.,.F.,(4,2,4),(-0.00212384826848124,-0.00106192580172268,
0.),.UNSPECIFIED.);
#1713=B_SPLINE_CURVE_WITH_KNOTS('',3,(#77892,#77893,#77894,#77895,#77896,
#77897),.UNSPECIFIED.,.F.,.F.,(4,2,4),(9.99998409484697E-7,0.0193527745925596,
0.0387045692823788),.UNSPECIFIED.);
#1714=B_SPLINE_CURVE_WITH_KNOTS('',3,(#77903,#77904,#77905,#77906,#77907,
#77908),.UNSPECIFIED.,.F.,.F.,(4,2,4),(-0.00212486549577526,-0.00106293274763414,
-9.99999999081163E-7),.UNSPECIFIED.);
#1715=B_SPLINE_CURVE_WITH_KNOTS('',3,(#77947,#77948,#77949,#77950,#77951,
#77952),.UNSPECIFIED.,.F.,.F.,(4,2,4),(0.,0.0198583386666685,0.0397175618153152),
 .UNSPECIFIED.);
#1716=B_SPLINE_CURVE_WITH_KNOTS('',3,(#77965,#77966,#77967,#77968,#77969,
#77970),.UNSPECIFIED.,.F.,.F.,(4,2,4),(0.,0.0198761966603836,0.0397532848690265),
 .UNSPECIFIED.);
#1717=B_SPLINE_CURVE_WITH_KNOTS('',3,(#78022,#78023,#78024,#78025,#78026,
#78027),.UNSPECIFIED.,.F.,.F.,(4,2,4),(0.,0.0199008240786792,0.039802540676266),
 .UNSPECIFIED.);
#1718=B_SPLINE_CURVE_WITH_KNOTS('',3,(#78040,#78041,#78042,#78043,#78044,
#78045),.UNSPECIFIED.,.F.,.F.,(4,2,4),(0.,0.0199042047132145,0.0398092891672759),
 .UNSPECIFIED.);
#1719=B_SPLINE_CURVE_WITH_KNOTS('',3,(#78090,#78091,#78092,#78093,#78094,
#78095),.UNSPECIFIED.,.F.,.F.,(4,2,4),(0.,0.0198954793679848,0.0397918615443618),
 .UNSPECIFIED.);
#1720=B_SPLINE_CURVE_WITH_KNOTS('',3,(#78142,#78143,#78144,#78145,#78146,
#78147,#78148),.UNSPECIFIED.,.F.,.F.,(4,3,4),(0.,0.5,0.999990117166367),
 .UNSPECIFIED.);
#1721=B_SPLINE_CURVE_WITH_KNOTS('',3,(#78171,#78172,#78173,#78174,#78175,
#78176),.UNSPECIFIED.,.F.,.F.,(4,2,4),(0.,0.0198677119512784,0.039736334106876),
 .UNSPECIFIED.);
#1722=B_SPLINE_CURVE_WITH_KNOTS('',3,(#78218,#78219,#78220,#78221,#78222,
#78223),.UNSPECIFIED.,.F.,.F.,(4,2,4),(0.,0.019897396590471,0.0397956842942256),
 .UNSPECIFIED.);
#1723=B_SPLINE_CURVE_WITH_KNOTS('',3,(#78245,#78246,#78247,#78248,#78249,
#78250),.UNSPECIFIED.,.F.,.F.,(4,2,4),(0.,0.0199030680183993,0.0398070348136018),
 .UNSPECIFIED.);
#1724=B_SPLINE_CURVE_WITH_KNOTS('',3,(#78295,#78296,#78297,#78298,#78299,
#78300),.UNSPECIFIED.,.F.,.F.,(4,2,4),(0.,0.0198994178727326,0.0397997368327952),
 .UNSPECIFIED.);
#1725=B_SPLINE_CURVE_WITH_KNOTS('',3,(#78313,#78314,#78315,#78316,#78317,
#78318),.UNSPECIFIED.,.F.,.F.,(4,2,4),(0.,0.0198905174670392,0.0397819062735446),
 .UNSPECIFIED.);
#1726=B_SPLINE_CURVE_WITH_KNOTS('',3,(#78343,#78344,#78345,#78346,#78347,
#78348,#78349),.UNSPECIFIED.,.F.,.F.,(4,3,4),(0.0365944846647016,0.0384615384615384,
0.0431466153076595),.UNSPECIFIED.);
#1727=B_SPLINE_CURVE_WITH_KNOTS('',3,(#78350,#78351,#78352,#78353,#78354,
#78355,#78356,#78357),.UNSPECIFIED.,.F.,.F.,(4,2,2,4),(1.77292731488234E-6,
0.00863675577096559,0.0171409248953735,0.0172810711148425),
 .UNSPECIFIED.);
#1728=B_SPLINE_CURVE_WITH_KNOTS('',3,(#78382,#78383,#78384,#78385,#78386,
#78387),.UNSPECIFIED.,.F.,.F.,(4,2,4),(0.,0.0198536183160875,0.0397081495930974),
 .UNSPECIFIED.);
#1729=B_SPLINE_CURVE_WITH_KNOTS('',3,(#78405,#78406,#78407,#78408,#78409,
#78410),.UNSPECIFIED.,.F.,.F.,(4,2,4),(-0.00212384862416112,-0.00106192594848514,
0.),.UNSPECIFIED.);
#1730=B_SPLINE_CURVE_WITH_KNOTS('',3,(#78411,#78412,#78413,#78414,#78415,
#78416),.UNSPECIFIED.,.F.,.F.,(4,2,4),(9.9999841687486E-7,0.0193527898667748,
0.0387045796213571),.UNSPECIFIED.);
#1731=B_SPLINE_CURVE_WITH_KNOTS('',3,(#78422,#78423,#78424,#78425,#78426,
#78427),.UNSPECIFIED.,.F.,.F.,(4,2,4),(-0.00212486503056007,-0.00106293275801356,
-1.00000000012482E-6),.UNSPECIFIED.);
#1732=B_SPLINE_CURVE_WITH_KNOTS('',3,(#78466,#78467,#78468,#78469,#78470,
#78471),.UNSPECIFIED.,.F.,.F.,(4,2,4),(0.,0.0198583386648012,0.0397175618073442),
 .UNSPECIFIED.);
#1733=B_SPLINE_CURVE_WITH_KNOTS('',3,(#78484,#78485,#78486,#78487,#78488,
#78489),.UNSPECIFIED.,.F.,.F.,(4,2,4),(0.,0.0198761966601199,0.0397532848749042),
 .UNSPECIFIED.);
#1734=B_SPLINE_CURVE_WITH_KNOTS('',3,(#78541,#78542,#78543,#78544,#78545,
#78546),.UNSPECIFIED.,.F.,.F.,(4,2,4),(0.,0.0199008240773645,0.0398025406710212),
 .UNSPECIFIED.);
#1735=B_SPLINE_CURVE_WITH_KNOTS('',3,(#78559,#78560,#78561,#78562,#78563,
#78564),.UNSPECIFIED.,.F.,.F.,(4,2,4),(0.,0.0199042047128573,0.0398092891591882),
 .UNSPECIFIED.);
#1736=B_SPLINE_CURVE_WITH_KNOTS('',3,(#78612,#78613,#78614,#78615,#78616,
#78617),.UNSPECIFIED.,.F.,.F.,(4,2,4),(0.,0.0198954793664142,0.0397918615380289),
 .UNSPECIFIED.);
#1737=B_SPLINE_CURVE_WITH_KNOTS('',3,(#78657,#78658,#78659,#78660,#78661,
#78662,#78663),.UNSPECIFIED.,.F.,.F.,(4,3,4),(0.,0.5,0.999990117164971),
 .UNSPECIFIED.);
#1738=B_SPLINE_CURVE_WITH_KNOTS('',3,(#78686,#78687,#78688,#78689,#78690,
#78691),.UNSPECIFIED.,.F.,.F.,(4,2,4),(0.,0.0198677119514339,0.0397363341070424),
 .UNSPECIFIED.);
#1739=B_SPLINE_CURVE_WITH_KNOTS('',3,(#78733,#78734,#78735,#78736,#78737,
#78738),.UNSPECIFIED.,.F.,.F.,(4,2,4),(0.,0.0198973965889047,0.0397956842881278),
 .UNSPECIFIED.);
#1740=B_SPLINE_CURVE_WITH_KNOTS('',3,(#78760,#78761,#78762,#78763,#78764,
#78765),.UNSPECIFIED.,.F.,.F.,(4,2,4),(0.,0.0199030680184938,0.0398070348140193),
 .UNSPECIFIED.);
#1741=B_SPLINE_CURVE_WITH_KNOTS('',3,(#78810,#78811,#78812,#78813,#78814,
#78815),.UNSPECIFIED.,.F.,.F.,(4,2,4),(0.,0.0198994178707068,0.0397997368248638),
 .UNSPECIFIED.);
#1742=B_SPLINE_CURVE_WITH_KNOTS('',3,(#78828,#78829,#78830,#78831,#78832,
#78833),.UNSPECIFIED.,.F.,.F.,(4,2,4),(0.,0.0198905179572786,0.0397819072688436),
 .UNSPECIFIED.);
#1743=B_SPLINE_CURVE_WITH_KNOTS('',3,(#78858,#78859,#78860,#78861,#78862,
#78863,#78864),.UNSPECIFIED.,.F.,.F.,(4,3,4),(0.0365944846647006,0.0384615384615384,
0.0431466153076599),.UNSPECIFIED.);
#1744=B_SPLINE_CURVE_WITH_KNOTS('',3,(#78865,#78866,#78867,#78868,#78869,
#78870,#78871,#78872),.UNSPECIFIED.,.F.,.F.,(4,2,2,4),(1.77258020099164E-6,
0.00863675570858734,0.0171409061550788,0.0172810544018275),
 .UNSPECIFIED.);
#1745=B_SPLINE_CURVE_WITH_KNOTS('',3,(#78897,#78898,#78899,#78900,#78901,
#78902),.UNSPECIFIED.,.F.,.F.,(4,2,4),(0.,0.0198536183145067,0.0397081495869588),
 .UNSPECIFIED.);
#1746=B_SPLINE_CURVE_WITH_KNOTS('',3,(#78920,#78921,#78922,#78923,#78924,
#78925),.UNSPECIFIED.,.F.,.F.,(4,2,4),(-0.00212384856218078,-0.00106192592379002,
0.),.UNSPECIFIED.);
#1747=B_SPLINE_CURVE_WITH_KNOTS('',3,(#78926,#78927,#78928,#78929,#78930,
#78931),.UNSPECIFIED.,.F.,.F.,(4,2,4),(9.99998415920771E-7,0.0193527803902452,
0.0387045693980609),.UNSPECIFIED.);
#1748=B_SPLINE_CURVE_WITH_KNOTS('',3,(#78937,#78938,#78939,#78940,#78941,
#78942),.UNSPECIFIED.,.F.,.F.,(4,2,4),(-0.00212486443485167,-0.00106293275784374,
-9.99999999056443E-7),.UNSPECIFIED.);
#1749=B_SPLINE_CURVE_WITH_KNOTS('',3,(#78981,#78982,#78983,#78984,#78985,
#78986),.UNSPECIFIED.,.F.,.F.,(4,2,4),(0.,0.0198583386637869,0.0397175618035615),
 .UNSPECIFIED.);
#1750=B_SPLINE_CURVE_WITH_KNOTS('',3,(#78999,#79000,#79001,#79002,#79003,
#79004),.UNSPECIFIED.,.F.,.F.,(4,2,4),(0.,0.0198761967104589,0.0397532849902813),
 .UNSPECIFIED.);
#1751=B_SPLINE_CURVE_WITH_KNOTS('',3,(#79056,#79057,#79058,#79059,#79060,
#79061),.UNSPECIFIED.,.F.,.F.,(4,2,4),(0.,0.0199008240757587,0.0398025406643214),
 .UNSPECIFIED.);
#1752=B_SPLINE_CURVE_WITH_KNOTS('',3,(#79074,#79075,#79076,#79077,#79078,
#79079),.UNSPECIFIED.,.F.,.F.,(4,2,4),(0.,0.0199042046967123,0.0398092891327804),
 .UNSPECIFIED.);
#1753=B_SPLINE_CURVE_WITH_KNOTS('',3,(#79127,#79128,#79129,#79130,#79131,
#79132),.UNSPECIFIED.,.F.,.F.,(4,2,4),(0.,0.0198954793650519,0.039791861532841),
 .UNSPECIFIED.);
#1754=B_SPLINE_CURVE_WITH_KNOTS('',3,(#79172,#79173,#79174,#79175,#79176,
#79177,#79178),.UNSPECIFIED.,.F.,.F.,(4,3,4),(0.,0.5,0.999990117164572),
 .UNSPECIFIED.);
#1755=B_SPLINE_CURVE_WITH_KNOTS('',3,(#79201,#79202,#79203,#79204,#79205,
#79206),.UNSPECIFIED.,.F.,.F.,(4,2,4),(0.,0.019867711951081,0.0397363341059826),
 .UNSPECIFIED.);
#1756=B_SPLINE_CURVE_WITH_KNOTS('',3,(#79248,#79249,#79250,#79251,#79252,
#79253),.UNSPECIFIED.,.F.,.F.,(4,2,4),(0.,0.0198973965879299,0.0397956842843274),
 .UNSPECIFIED.);
#1757=B_SPLINE_CURVE_WITH_KNOTS('',3,(#79275,#79276,#79277,#79278,#79279,
#79280),.UNSPECIFIED.,.F.,.F.,(4,2,4),(0.,0.0199030680185526,0.0398070348141684),
 .UNSPECIFIED.);
#1758=B_SPLINE_CURVE_WITH_KNOTS('',3,(#79325,#79326,#79327,#79328,#79329,
#79330),.UNSPECIFIED.,.F.,.F.,(4,2,4),(0.,0.0198994178698969,0.0397997368217084),
 .UNSPECIFIED.);
#1759=B_SPLINE_CURVE_WITH_KNOTS('',3,(#79343,#79344,#79345,#79346,#79347,
#79348),.UNSPECIFIED.,.F.,.F.,(4,2,4),(0.,0.0198905179572962,0.039781907256784),
 .UNSPECIFIED.);
#1760=B_SPLINE_CURVE_WITH_KNOTS('',3,(#79373,#79374,#79375,#79376,#79377,
#79378,#79379),.UNSPECIFIED.,.F.,.F.,(4,3,4),(0.0365944846647006,0.0384615384615384,
0.0431466153076591),.UNSPECIFIED.);
#1761=B_SPLINE_CURVE_WITH_KNOTS('',3,(#79380,#79381,#79382,#79383,#79384,
#79385,#79386,#79387),.UNSPECIFIED.,.F.,.F.,(4,2,2,4),(1.77350751380791E-6,
0.0086367557881011,0.0171409177879644,0.0172810646875839),.UNSPECIFIED.);
#1762=B_SPLINE_CURVE_WITH_KNOTS('',3,(#79412,#79413,#79414,#79415,#79416,
#79417),.UNSPECIFIED.,.F.,.F.,(4,2,4),(0.,0.0198536183132773,0.0397081495822158),
 .UNSPECIFIED.);
#1763=B_SPLINE_CURVE_WITH_KNOTS('',3,(#79435,#79436,#79437,#79438,#79439,
#79440),.UNSPECIFIED.,.F.,.F.,(4,2,4),(-0.00212385087314715,-0.00106192684123349,
0.),.UNSPECIFIED.);
#1764=B_SPLINE_CURVE_WITH_KNOTS('',3,(#79441,#79442,#79443,#79444,#79445,
#79446),.UNSPECIFIED.,.F.,.F.,(4,2,4),(9.99998417712879E-7,0.0193527846157326,
0.0387045795193881),.UNSPECIFIED.);
#1765=B_SPLINE_CURVE_WITH_KNOTS('',3,(#79452,#79453,#79454,#79455,#79456,
#79457),.UNSPECIFIED.,.F.,.F.,(4,2,4),(-0.00212486389546323,-0.0010629327504673,
-9.99999998651385E-7),.UNSPECIFIED.);
#1766=B_SPLINE_CURVE_WITH_KNOTS('',3,(#79496,#79497,#79498,#79499,#79500,
#79501),.UNSPECIFIED.,.F.,.F.,(4,2,4),(0.,0.0198583386619873,0.0397175617964205),
 .UNSPECIFIED.);
#1767=B_SPLINE_CURVE_WITH_KNOTS('',3,(#79514,#79515,#79516,#79517,#79518,
#79519),.UNSPECIFIED.,.F.,.F.,(4,2,4),(0.,0.0198761967014612,0.0397532849518429),
 .UNSPECIFIED.);
#1768=B_SPLINE_CURVE_WITH_KNOTS('',3,(#79571,#79572,#79573,#79574,#79575,
#79576),.UNSPECIFIED.,.F.,.F.,(4,2,4),(0.,0.0199008240741428,0.0398025406583395),
 .UNSPECIFIED.);
#1769=B_SPLINE_CURVE_WITH_KNOTS('',3,(#79589,#79590,#79591,#79592,#79593,
#79594),.UNSPECIFIED.,.F.,.F.,(4,2,4),(0.,0.0199042047186291,0.0398092891745138),
 .UNSPECIFIED.);
#1770=B_SPLINE_CURVE_WITH_KNOTS('',3,(#79642,#79643,#79644,#79645,#79646,
#79647),.UNSPECIFIED.,.F.,.F.,(4,2,4),(0.,0.0198954793632857,0.0397918615254757),
 .UNSPECIFIED.);
#1771=B_SPLINE_CURVE_WITH_KNOTS('',3,(#79687,#79688,#79689,#79690,#79691,
#79692,#79693),.UNSPECIFIED.,.F.,.F.,(4,3,4),(0.,0.5,0.999990117162871),
 .UNSPECIFIED.);
#1772=B_SPLINE_CURVE_WITH_KNOTS('',3,(#79716,#79717,#79718,#79719,#79720,
#79721),.UNSPECIFIED.,.F.,.F.,(4,2,4),(0.,0.0198677119513824,0.0397363341067771),
 .UNSPECIFIED.);
#1773=B_SPLINE_CURVE_WITH_KNOTS('',3,(#79763,#79764,#79765,#79766,#79767,
#79768),.UNSPECIFIED.,.F.,.F.,(4,2,4),(0.,0.019897396586304,0.0397956842776212),
 .UNSPECIFIED.);
#1774=B_SPLINE_CURVE_WITH_KNOTS('',3,(#79790,#79791,#79792,#79793,#79794,
#79795),.UNSPECIFIED.,.F.,.F.,(4,2,4),(0.,0.0199030680185807,0.0398070348140608),
 .UNSPECIFIED.);
#1775=B_SPLINE_CURVE_WITH_KNOTS('',3,(#79840,#79841,#79842,#79843,#79844,
#79845),.UNSPECIFIED.,.F.,.F.,(4,2,4),(0.,0.0198994178679604,0.0397997368137069),
 .UNSPECIFIED.);
#1776=B_SPLINE_CURVE_WITH_KNOTS('',3,(#79858,#79859,#79860,#79861,#79862,
#79863),.UNSPECIFIED.,.F.,.F.,(4,2,4),(0.,0.0198905179567476,0.0397819072467453),
 .UNSPECIFIED.);
#1777=B_SPLINE_CURVE_WITH_KNOTS('',3,(#79888,#79889,#79890,#79891,#79892,
#79893,#79894),.UNSPECIFIED.,.F.,.F.,(4,3,4),(0.0365944846647015,0.0384615384615384,
0.0431466153076602),.UNSPECIFIED.);
#1778=B_SPLINE_CURVE_WITH_KNOTS('',3,(#79895,#79896,#79897,#79898,#79899,
#79900,#79901,#79902),.UNSPECIFIED.,.F.,.F.,(4,2,2,4),(1.77257984617272E-6,
0.00863675584960567,0.0171409478371716,0.0172810916427102),
 .UNSPECIFIED.);
#1779=B_SPLINE_CURVE_WITH_KNOTS('',3,(#79927,#79928,#79929,#79930,#79931,
#79932),.UNSPECIFIED.,.F.,.F.,(4,2,4),(0.,0.0198536183117049,0.0397081495761841),
 .UNSPECIFIED.);
#1780=B_SPLINE_CURVE_WITH_KNOTS('',3,(#79950,#79951,#79952,#79953,#79954,
#79955),.UNSPECIFIED.,.F.,.F.,(4,2,4),(-0.00212385226401534,-0.00106192740973201,
0.),.UNSPECIFIED.);
#1781=B_SPLINE_CURVE_WITH_KNOTS('',3,(#79956,#79957,#79958,#79959,#79960,
#79961),.UNSPECIFIED.,.F.,.F.,(4,2,4),(9.99998417825365E-7,0.0193527904136142,
0.0387045796348744),.UNSPECIFIED.);
#1782=B_SPLINE_CURVE_WITH_KNOTS('',3,(#79967,#79968,#79969,#79970,#79971,
#79972),.UNSPECIFIED.,.F.,.F.,(4,2,4),(-0.00212486331074845,-0.00106293275284134,
-1.00000000155683E-6),.UNSPECIFIED.);
#1783=B_SPLINE_CURVE_WITH_KNOTS('',3,(#80011,#80012,#80013,#80014,#80015,
#80016),.UNSPECIFIED.,.F.,.F.,(4,2,4),(0.,0.0198583386611987,0.0397175617931082),
 .UNSPECIFIED.);
#1784=B_SPLINE_CURVE_WITH_KNOTS('',3,(#80029,#80030,#80031,#80032,#80033,
#80034),.UNSPECIFIED.,.F.,.F.,(4,2,4),(0.,0.0198761966899037,0.039753284941563),
 .UNSPECIFIED.);
#1785=B_SPLINE_CURVE_WITH_KNOTS('',3,(#80086,#80087,#80088,#80089,#80090,
#80091),.UNSPECIFIED.,.F.,.F.,(4,2,4),(0.,0.0199008240728521,0.0398025406528661),
 .UNSPECIFIED.);
#1786=B_SPLINE_CURVE_WITH_KNOTS('',3,(#80104,#80105,#80106,#80107,#80108,
#80109),.UNSPECIFIED.,.F.,.F.,(4,2,4),(0.,0.0199042047187496,0.03980928917477),
 .UNSPECIFIED.);
#1787=B_SPLINE_CURVE_WITH_KNOTS('',3,(#80157,#80158,#80159,#80160,#80161,
#80162),.UNSPECIFIED.,.F.,.F.,(4,2,4),(0.,0.0198954793619581,0.0397918615199839),
 .UNSPECIFIED.);
#1788=B_SPLINE_CURVE_WITH_KNOTS('',3,(#80202,#80203,#80204,#80205,#80206,
#80207,#80208),.UNSPECIFIED.,.F.,.F.,(4,3,4),(0.,0.5,0.999990117160646),
 .UNSPECIFIED.);
#1789=B_SPLINE_CURVE_WITH_KNOTS('',3,(#80231,#80232,#80233,#80234,#80235,
#80236),.UNSPECIFIED.,.F.,.F.,(4,2,4),(0.,0.0198677119502807,0.039736334103427),
 .UNSPECIFIED.);
#1790=B_SPLINE_CURVE_WITH_KNOTS('',3,(#80278,#80279,#80280,#80281,#80282,
#80283),.UNSPECIFIED.,.F.,.F.,(4,2,4),(0.,0.0198973965839471,0.0397956842684524),
 .UNSPECIFIED.);
#1791=B_SPLINE_CURVE_WITH_KNOTS('',3,(#80305,#80306,#80307,#80308,#80309,
#80310),.UNSPECIFIED.,.F.,.F.,(4,2,4),(0.,0.0199030680177332,0.0398070348109682),
 .UNSPECIFIED.);
#1792=B_SPLINE_CURVE_WITH_KNOTS('',3,(#80355,#80356,#80357,#80358,#80359,
#80360),.UNSPECIFIED.,.F.,.F.,(4,2,4),(0.,0.0198994178663628,0.0397997368074939),
 .UNSPECIFIED.);
#1793=B_SPLINE_CURVE_WITH_KNOTS('',3,(#80373,#80374,#80375,#80376,#80377,
#80378),.UNSPECIFIED.,.F.,.F.,(4,2,4),(0.,0.0198905179571887,0.0397819072607149),
 .UNSPECIFIED.);
#1794=B_SPLINE_CURVE_WITH_KNOTS('',3,(#80403,#80404,#80405,#80406,#80407,
#80408,#80409),.UNSPECIFIED.,.F.,.F.,(4,3,4),(0.0365944846647005,0.0384615384615384,
0.0431466153076602),.UNSPECIFIED.);
#1795=B_SPLINE_CURVE_WITH_KNOTS('',3,(#80410,#80411,#80412,#80413,#80414,
#80415,#80416,#80417),.UNSPECIFIED.,.F.,.F.,(4,2,2,4),(1.77257993802502E-6,
0.00863675581682755,0.0171409344827175,0.0172810797173663),
 .UNSPECIFIED.);
#1796=B_SPLINE_CURVE_WITH_KNOTS('',3,(#80442,#80443,#80444,#80445,#80446,
#80447),.UNSPECIFIED.,.F.,.F.,(4,2,4),(0.,0.0198536183101753,0.0397081495702501),
 .UNSPECIFIED.);
#1797=B_SPLINE_CURVE_WITH_KNOTS('',3,(#80465,#80466,#80467,#80468,#80469,
#80470),.UNSPECIFIED.,.F.,.F.,(4,2,4),(-0.0021238541167507,-0.00106192814372196,
0.),.UNSPECIFIED.);
#1798=B_SPLINE_CURVE_WITH_KNOTS('',3,(#80471,#80472,#80473,#80474,#80475,
#80476),.UNSPECIFIED.,.F.,.F.,(4,2,4),(9.99998419123142E-7,0.0193527904127871,
0.0387045796331662),.UNSPECIFIED.);
#1799=B_SPLINE_CURVE_WITH_KNOTS('',3,(#80482,#80483,#80484,#80485,#80486,
#80487),.UNSPECIFIED.,.F.,.F.,(4,2,4),(-0.00212486283058553,-0.00106293276585407,
-1.00000000193045E-6),.UNSPECIFIED.);
#1800=B_SPLINE_CURVE_WITH_KNOTS('',3,(#80526,#80527,#80528,#80529,#80530,
#80531),.UNSPECIFIED.,.F.,.F.,(4,2,4),(0.,0.0198583386596414,0.0397175617869763),
 .UNSPECIFIED.);
#1801=B_SPLINE_CURVE_WITH_KNOTS('',3,(#80544,#80545,#80546,#80547,#80548,
#80549),.UNSPECIFIED.,.F.,.F.,(4,2,4),(0.,0.0198761965688489,0.0397532846844471),
 .UNSPECIFIED.);
#1802=B_SPLINE_CURVE_WITH_KNOTS('',3,(#80601,#80602,#80603,#80604,#80605,
#80606),.UNSPECIFIED.,.F.,.F.,(4,2,4),(0.,0.0199008240713145,0.0398025406471834),
 .UNSPECIFIED.);
#1803=B_SPLINE_CURVE_WITH_KNOTS('',3,(#80619,#80620,#80621,#80622,#80623,
#80624),.UNSPECIFIED.,.F.,.F.,(4,2,4),(0.,0.0199042047187008,0.0398092891715554),
 .UNSPECIFIED.);
#1804=B_SPLINE_CURVE_WITH_KNOTS('',3,(#80672,#80673,#80674,#80675,#80676,
#80677),.UNSPECIFIED.,.F.,.F.,(4,2,4),(0.,0.019895979281645,0.0397918613086002),
 .UNSPECIFIED.);
#1805=B_SPLINE_CURVE_WITH_KNOTS('',3,(#80717,#80718,#80719,#80720,#80721,
#80722,#80723),.UNSPECIFIED.,.F.,.F.,(4,3,4),(0.,0.5,0.99999011715943),
 .UNSPECIFIED.);
#1806=B_SPLINE_CURVE_WITH_KNOTS('',3,(#80746,#80747,#80748,#80749,#80750,
#80751),.UNSPECIFIED.,.F.,.F.,(4,2,4),(0.,0.0198677119493813,0.0397363340992066),
 .UNSPECIFIED.);
#1807=B_SPLINE_CURVE_WITH_KNOTS('',3,(#80793,#80794,#80795,#80796,#80797,
#80798),.UNSPECIFIED.,.F.,.F.,(4,2,4),(0.,0.0198973965800523,0.0397956842522655),
 .UNSPECIFIED.);
#1808=B_SPLINE_CURVE_WITH_KNOTS('',3,(#80820,#80821,#80822,#80823,#80824,
#80825),.UNSPECIFIED.,.F.,.F.,(4,2,4),(0.,0.0199030680179019,0.0398070348114157),
 .UNSPECIFIED.);
#1809=B_SPLINE_CURVE_WITH_KNOTS('',3,(#80870,#80871,#80872,#80873,#80874,
#80875),.UNSPECIFIED.,.F.,.F.,(4,2,4),(0.,0.0198994178626952,0.0397997367921896),
 .UNSPECIFIED.);
#1810=B_SPLINE_CURVE_WITH_KNOTS('',3,(#80888,#80889,#80890,#80891,#80892,
#80893),.UNSPECIFIED.,.F.,.F.,(4,2,4),(0.,0.0198905179575111,0.0397819072674916),
 .UNSPECIFIED.);
#1811=B_SPLINE_CURVE_WITH_KNOTS('',3,(#80918,#80919,#80920,#80921,#80922,
#80923,#80924),.UNSPECIFIED.,.F.,.F.,(4,3,4),(0.0365944846647006,0.0384615384615384,
0.0431466153076597),.UNSPECIFIED.);
#1812=B_SPLINE_CURVE_WITH_KNOTS('',3,(#80925,#80926,#80927,#80928,#80929,
#80930,#80931,#80932),.UNSPECIFIED.,.F.,.F.,(4,2,2,4),(1.77257997374341E-6,
0.00863675581523217,0.0171409311328255,0.0172810767227047),
 .UNSPECIFIED.);
#1813=B_SPLINE_CURVE_WITH_KNOTS('',3,(#80957,#80958,#80959,#80960,#80961,
#80962),.UNSPECIFIED.,.F.,.F.,(4,2,4),(0.,0.0198536183074313,0.0397081495588918),
 .UNSPECIFIED.);
#1814=B_SPLINE_CURVE_WITH_KNOTS('',3,(#80980,#80981,#80982,#80983,#80984,
#80985),.UNSPECIFIED.,.F.,.F.,(4,2,4),(-0.00212385633540368,-0.00106192904131713,
0.),.UNSPECIFIED.);
#1815=B_SPLINE_CURVE_WITH_KNOTS('',3,(#80986,#80987,#80988,#80989,#80990,
#80991),.UNSPECIFIED.,.F.,.F.,(4,2,4),(9.99998410553807E-7,0.0193527753876696,
0.0387045692985089),.UNSPECIFIED.);
#1816=B_SPLINE_CURVE_WITH_KNOTS('',3,(#80997,#80998,#80999,#81000,#81001,
#81002),.UNSPECIFIED.,.F.,.F.,(4,2,4),(-0.0021248622707656,-0.00106293276671975,
-1.00000000055655E-6),.UNSPECIFIED.);
#1817=B_SPLINE_CURVE_WITH_KNOTS('',3,(#81041,#81042,#81043,#81044,#81045,
#81046),.UNSPECIFIED.,.F.,.F.,(4,2,4),(0.,0.0198583386584655,0.0397175617823022),
 .UNSPECIFIED.);
#1818=B_SPLINE_CURVE_WITH_KNOTS('',3,(#81059,#81060,#81061,#81062,#81063,
#81064),.UNSPECIFIED.,.F.,.F.,(4,2,4),(0.,0.0198761967007967,0.0397532849597277),
 .UNSPECIFIED.);
#1819=B_SPLINE_CURVE_WITH_KNOTS('',3,(#81116,#81117,#81118,#81119,#81120,
#81121),.UNSPECIFIED.,.F.,.F.,(4,2,4),(0.,0.0199008240701687,0.0398025406425139),
 .UNSPECIFIED.);
#1820=B_SPLINE_CURVE_WITH_KNOTS('',3,(#81134,#81135,#81136,#81137,#81138,
#81139),.UNSPECIFIED.,.F.,.F.,(4,2,4),(0.,0.0199042047188792,0.0398092891791789),
 .UNSPECIFIED.);
#1821=B_SPLINE_CURVE_WITH_KNOTS('',3,(#81187,#81188,#81189,#81190,#81191,
#81192),.UNSPECIFIED.,.F.,.F.,(4,2,4),(0.,0.0198954793595894,0.0397918615110356),
 .UNSPECIFIED.);
#1822=B_SPLINE_CURVE_WITH_KNOTS('',3,(#81232,#81233,#81234,#81235,#81236,
#81237,#81238),.UNSPECIFIED.,.F.,.F.,(4,3,4),(0.,0.5,0.999990117156445),
 .UNSPECIFIED.);
#1823=B_SPLINE_CURVE_WITH_KNOTS('',3,(#81261,#81262,#81263,#81264,#81265,
#81266),.UNSPECIFIED.,.F.,.F.,(4,2,4),(0.,0.0198677119497614,0.0397363341009546),
 .UNSPECIFIED.);
#1824=B_SPLINE_CURVE_WITH_KNOTS('',3,(#81308,#81309,#81310,#81311,#81312,
#81313),.UNSPECIFIED.,.F.,.F.,(4,2,4),(0.,0.0198973965760269,0.0397956842361046),
 .UNSPECIFIED.);
#1825=B_SPLINE_CURVE_WITH_KNOTS('',3,(#81335,#81336,#81337,#81338,#81339,
#81340),.UNSPECIFIED.,.F.,.F.,(4,2,4),(0.,0.0199030680172686,0.0398070348086195),
 .UNSPECIFIED.);
#1826=B_SPLINE_CURVE_WITH_KNOTS('',3,(#81382,#81383,#81384,#81385,#81386,
#81387),.UNSPECIFIED.,.F.,.F.,(4,2,4),(0.,0.0198994178579901,0.0397997367735032),
 .UNSPECIFIED.);
#1827=B_SPLINE_CURVE_WITH_KNOTS('',3,(#81407,#81408,#81409,#81410,#81411,
#81412),.UNSPECIFIED.,.F.,.F.,(4,2,4),(0.,0.0198905727828699,0.0397820348380782),
 .UNSPECIFIED.);
#1828=B_SPLINE_CURVE_WITH_KNOTS('',3,(#81437,#81438,#81439,#81440,#81441,
#81442,#81443),.UNSPECIFIED.,.F.,.F.,(4,3,4),(0.0365944846647011,0.0384615384615384,
0.0431466153076595),.UNSPECIFIED.);
#1829=B_SPLINE_CURVE_WITH_KNOTS('',3,(#81444,#81445,#81446,#81447,#81448,
#81449,#81450,#81451),.UNSPECIFIED.,.F.,.F.,(4,2,2,4),(1.77258011691398E-6,
0.00863675577077701,0.0171409165754082,0.017281063727439),.UNSPECIFIED.);
#1830=B_SPLINE_CURVE_WITH_KNOTS('',3,(#81476,#81477,#81478,#81479,#81480,
#81481),.UNSPECIFIED.,.F.,.F.,(4,2,4),(0.,0.0198536183030717,0.039708149541506),
 .UNSPECIFIED.);
#1831=B_SPLINE_CURVE_WITH_KNOTS('',3,(#81499,#81500,#81501,#81502,#81503,
#81504),.UNSPECIFIED.,.F.,.F.,(4,2,4),(-0.00212385871063614,-0.00106192998404695,
0.),.UNSPECIFIED.);
#1832=B_SPLINE_CURVE_WITH_KNOTS('',3,(#81505,#81506,#81507,#81508,#81509,
#81510),.UNSPECIFIED.,.F.,.F.,(4,2,4),(9.99998418614826E-7,0.0193527904140548,
0.0387045796357254),.UNSPECIFIED.);
#1833=B_SPLINE_CURVE_WITH_KNOTS('',3,(#81516,#81517,#81518,#81519,#81520,
#81521),.UNSPECIFIED.,.F.,.F.,(4,2,4),(-0.00212486175378365,-0.00106293276587914,
-1.00000000015431E-6),.UNSPECIFIED.);
#1834=B_SPLINE_CURVE_WITH_KNOTS('',3,(#81560,#81561,#81562,#81563,#81564,
#81565),.UNSPECIFIED.,.F.,.F.,(4,2,4),(0.,0.0198583386549503,0.0397175617682779),
 .UNSPECIFIED.);
#1835=B_SPLINE_CURVE_WITH_KNOTS('',3,(#81578,#81579,#81580,#81581,#81582,
#81583),.UNSPECIFIED.,.F.,.F.,(4,2,4),(0.,0.0198761966973816,0.0397532849399191),
 .UNSPECIFIED.);
#1836=B_SPLINE_CURVE_WITH_KNOTS('',3,(#81635,#81636,#81637,#81638,#81639,
#81640),.UNSPECIFIED.,.F.,.F.,(4,2,4),(0.,0.0199008240672371,0.0398025406305121),
 .UNSPECIFIED.);
#1837=B_SPLINE_CURVE_WITH_KNOTS('',3,(#81653,#81654,#81655,#81656,#81657,
#81658),.UNSPECIFIED.,.F.,.F.,(4,2,4),(0.,0.0199042046967335,0.0398092891201385),
 .UNSPECIFIED.);
#1838=B_SPLINE_CURVE_WITH_KNOTS('',3,(#81706,#81707,#81708,#81709,#81710,
#81711),.UNSPECIFIED.,.F.,.F.,(4,2,4),(0.,0.0198954793574705,0.0397918615025454),
 .UNSPECIFIED.);
#1839=B_SPLINE_CURVE_WITH_KNOTS('',3,(#81751,#81752,#81753,#81754,#81755,
#81756,#81757),.UNSPECIFIED.,.F.,.F.,(4,3,4),(0.,0.5,0.999990117154057),
 .UNSPECIFIED.);
#1840=B_SPLINE_CURVE_WITH_KNOTS('',3,(#81780,#81781,#81782,#81783,#81784,
#81785),.UNSPECIFIED.,.F.,.F.,(4,2,4),(0.,0.0198677119483035,0.0397363340951872),
 .UNSPECIFIED.);
#1841=B_SPLINE_CURVE_WITH_KNOTS('',3,(#81827,#81828,#81829,#81830,#81831,
#81832),.UNSPECIFIED.,.F.,.F.,(4,2,4),(0.,0.0198973965729276,0.0397956842231821),
 .UNSPECIFIED.);
#1842=B_SPLINE_CURVE_WITH_KNOTS('',3,(#81854,#81855,#81856,#81857,#81858,
#81859),.UNSPECIFIED.,.F.,.F.,(4,2,4),(0.,0.0199030680155105,0.0398070348020406),
 .UNSPECIFIED.);
#1843=B_SPLINE_CURVE_WITH_KNOTS('',3,(#81904,#81905,#81906,#81907,#81908,
#81909),.UNSPECIFIED.,.F.,.F.,(4,2,4),(0.,0.0198994178544206,0.0397997367588171),
 .UNSPECIFIED.);
#1844=B_SPLINE_CURVE_WITH_KNOTS('',3,(#81922,#81923,#81924,#81925,#81926,
#81927),.UNSPECIFIED.,.F.,.F.,(4,2,4),(0.,0.0198905179573927,0.0397819072603145),
 .UNSPECIFIED.);
#1845=B_SPLINE_CURVE_WITH_KNOTS('',3,(#81953,#81954,#81955,#81956,#81957,
#81958),.UNSPECIFIED.,.F.,.F.,(4,2,4),(0.0365944846647007,0.0384615384615384,
0.0431466153076597),.UNSPECIFIED.);
#1846=B_SPLINE_CURVE_WITH_KNOTS('',3,(#81959,#81960,#81961,#81962,#81963,
#81964,#81965),.UNSPECIFIED.,.F.,.F.,(4,3,4),(0.,0.00863415824062196,0.0172757271482925),
 .UNSPECIFIED.);
#1847=B_SPLINE_CURVE_WITH_KNOTS('',3,(#81990,#81991,#81992,#81993,#81994,
#81995),.UNSPECIFIED.,.F.,.F.,(4,2,4),(0.,0.0198536182496097,0.0397081494264778),
 .UNSPECIFIED.);
#1848=B_SPLINE_CURVE_WITH_KNOTS('',3,(#82008,#82009,#82010,#82011,#82012,
#82013),.UNSPECIFIED.,.F.,.F.,(4,2,4),(-0.00212386114214876,-0.00106193095631279,
0.),.UNSPECIFIED.);
#1849=B_SPLINE_CURVE_WITH_KNOTS('',3,(#82014,#82015,#82016,#82017,#82018,
#82019),.UNSPECIFIED.,.F.,.F.,(4,2,4),(9.99998416295649E-7,0.0193522753878931,
0.0387045692978022),.UNSPECIFIED.);
#1850=B_SPLINE_CURVE_WITH_KNOTS('',3,(#82025,#82026,#82027,#82028,#82029,
#82030),.UNSPECIFIED.,.F.,.F.,(4,2,4),(-0.00212486125230607,-0.00106293276248913,
-9.99999999050588E-7),.UNSPECIFIED.);
#1851=B_SPLINE_CURVE_WITH_KNOTS('',3,(#82069,#82070,#82071,#82072,#82073,
#82074),.UNSPECIFIED.,.F.,.F.,(4,2,4),(0.,0.0198583386509932,0.0397175617519128),
 .UNSPECIFIED.);
#1852=B_SPLINE_CURVE_WITH_KNOTS('',3,(#82087,#82088,#82089,#82090,#82091,
#82092),.UNSPECIFIED.,.F.,.F.,(4,2,4),(0.,0.0198761967152631,0.0397532849904637),
 .UNSPECIFIED.);
#1853=B_SPLINE_CURVE_WITH_KNOTS('',3,(#82144,#82145,#82146,#82147,#82148,
#82149),.UNSPECIFIED.,.F.,.F.,(4,2,4),(0.,0.0199008240626534,0.0398025406124932),
 .UNSPECIFIED.);
#1854=B_SPLINE_CURVE_WITH_KNOTS('',3,(#82162,#82163,#82164,#82165,#82166,
#82167),.UNSPECIFIED.,.F.,.F.,(4,2,4),(0.,0.0199042047190279,0.0398092891738967),
 .UNSPECIFIED.);
#1855=B_SPLINE_CURVE_WITH_KNOTS('',3,(#82215,#82216,#82217,#82218,#82219,
#82220),.UNSPECIFIED.,.F.,.F.,(4,2,4),(0.,0.019895479353864,0.039791861487405),
 .UNSPECIFIED.);
#1856=B_SPLINE_CURVE_WITH_KNOTS('',3,(#82260,#82261,#82262,#82263,#82264,
#82265,#82266),.UNSPECIFIED.,.F.,.F.,(4,3,4),(0.,0.5,0.999990117151758),
 .UNSPECIFIED.);
#1857=B_SPLINE_CURVE_WITH_KNOTS('',3,(#82289,#82290,#82291,#82292,#82293,
#82294),.UNSPECIFIED.,.F.,.F.,(4,2,4),(0.,0.0198677119425251,0.0397363340720499),
 .UNSPECIFIED.);
#1858=B_SPLINE_CURVE_WITH_KNOTS('',3,(#82336,#82337,#82338,#82339,#82340,
#82341),.UNSPECIFIED.,.F.,.F.,(4,2,4),(0.,0.019897396570235,0.03979568421255),
 .UNSPECIFIED.);
#1859=B_SPLINE_CURVE_WITH_KNOTS('',3,(#82363,#82364,#82365,#82366,#82367,
#82368),.UNSPECIFIED.,.F.,.F.,(4,2,4),(0.,0.0199030680124401,0.039807034789456),
 .UNSPECIFIED.);
#1860=B_SPLINE_CURVE_WITH_KNOTS('',3,(#82413,#82414,#82415,#82416,#82417,
#82418),.UNSPECIFIED.,.F.,.F.,(4,2,4),(0.,0.0198994177390595,0.0397997364069847),
 .UNSPECIFIED.);
#1861=B_SPLINE_CURVE_WITH_KNOTS('',3,(#82431,#82432,#82433,#82434,#82435,
#82436),.UNSPECIFIED.,.F.,.F.,(4,2,4),(0.,0.0198905179574466,0.0397819072636344),
 .UNSPECIFIED.);
#1862=B_SPLINE_CURVE_WITH_KNOTS('',3,(#82461,#82462,#82463,#82464,#82465,
#82466,#82467),.UNSPECIFIED.,.F.,.F.,(4,3,4),(0.036594484664701,0.0384615384615384,
0.0431466153076601),.UNSPECIFIED.);
#1863=B_SPLINE_CURVE_WITH_KNOTS('',3,(#82468,#82469,#82470,#82471,#82472,
#82473,#82474,#82475),.UNSPECIFIED.,.F.,.F.,(4,2,2,4),(1.7725796662609E-6,
0.00863675589283121,0.0171409825398772,0.017281122632475),.UNSPECIFIED.);
#1864=B_SPLINE_CURVE_WITH_KNOTS('',3,(#82500,#82501,#82502,#82503,#82504,
#82505),.UNSPECIFIED.,.F.,.F.,(4,2,4),(0.,0.0198536182960252,0.0397081495129872),
 .UNSPECIFIED.);
#1865=B_SPLINE_CURVE_WITH_KNOTS('',3,(#82523,#82524,#82525,#82526,#82527,
#82528),.UNSPECIFIED.,.F.,.F.,(4,2,4),(-0.00212386406946142,-0.00106193213051581,
0.),.UNSPECIFIED.);
#1866=B_SPLINE_CURVE_WITH_KNOTS('',3,(#82529,#82530,#82531,#82532,#82533,
#82534),.UNSPECIFIED.,.F.,.F.,(4,2,4),(9.999984119248E-7,0.0193527803903459,
0.0387045693982159),.UNSPECIFIED.);
#1867=B_SPLINE_CURVE_WITH_KNOTS('',3,(#82540,#82541,#82542,#82543,#82544,
#82545),.UNSPECIFIED.,.F.,.F.,(4,2,4),(-0.00212486080361574,-0.0010629327631662,
-9.9999995856301E-7),.UNSPECIFIED.);
#1868=B_SPLINE_CURVE_WITH_KNOTS('',3,(#82581,#82582,#82583,#82584,#82585,
#82586),.UNSPECIFIED.,.F.,.F.,(4,2,4),(0.,0.0198583386475972,0.0397175617382976),
 .UNSPECIFIED.);
#1869=B_SPLINE_CURVE_WITH_KNOTS('',3,(#82606,#82607,#82608,#82609,#82610,
#82611),.UNSPECIFIED.,.F.,.F.,(4,2,4),(0.,0.0198762583887502,0.0397534251573493),
 .UNSPECIFIED.);
#1870=B_SPLINE_CURVE_WITH_KNOTS('',3,(#82663,#82664,#82665,#82666,#82667,
#82668),.UNSPECIFIED.,.F.,.F.,(4,2,4),(0.,0.0199008240587804,0.0398025405967764),
 .UNSPECIFIED.);
#1871=B_SPLINE_CURVE_WITH_KNOTS('',3,(#82681,#82682,#82683,#82684,#82685,
#82686),.UNSPECIFIED.,.F.,.F.,(4,2,4),(0.,0.0199042046968128,0.0398092891349481),
 .UNSPECIFIED.);
#1872=B_SPLINE_CURVE_WITH_KNOTS('',3,(#82734,#82735,#82736,#82737,#82738,
#82739),.UNSPECIFIED.,.F.,.F.,(4,2,4),(0.,0.0198954793496364,0.0397918614699736),
 .UNSPECIFIED.);
#1873=B_SPLINE_CURVE_WITH_KNOTS('',3,(#82779,#82780,#82781,#82782,#82783,
#82784,#82785),.UNSPECIFIED.,.F.,.F.,(4,3,4),(0.,0.5,0.999990117148265),
 .UNSPECIFIED.);
#1874=B_SPLINE_CURVE_WITH_KNOTS('',3,(#82808,#82809,#82810,#82811,#82812,
#82813),.UNSPECIFIED.,.F.,.F.,(4,2,4),(0.,0.0198677119379566,0.0397363340538177),
 .UNSPECIFIED.);
#1875=B_SPLINE_CURVE_WITH_KNOTS('',3,(#82855,#82856,#82857,#82858,#82859,
#82860),.UNSPECIFIED.,.F.,.F.,(4,2,4),(0.,0.0198973965677259,0.039795684202283),
 .UNSPECIFIED.);
#1876=B_SPLINE_CURVE_WITH_KNOTS('',3,(#82882,#82883,#82884,#82885,#82886,
#82887),.UNSPECIFIED.,.F.,.F.,(4,2,4),(0.,0.0199030680078316,0.0398070347704704),
 .UNSPECIFIED.);
#1877=B_SPLINE_CURVE_WITH_KNOTS('',3,(#82932,#82933,#82934,#82935,#82936,
#82937),.UNSPECIFIED.,.F.,.F.,(4,2,4),(0.,0.0198994178487356,0.0397997367357689),
 .UNSPECIFIED.);
#1878=B_SPLINE_CURVE_WITH_KNOTS('',3,(#82950,#82951,#82952,#82953,#82954,
#82955),.UNSPECIFIED.,.F.,.F.,(4,2,4),(0.,0.0198905179573299,0.0397819072639096),
 .UNSPECIFIED.);
#1879=B_SPLINE_CURVE_WITH_KNOTS('',3,(#82980,#82981,#82982,#82983,#82984,
#82985,#82986),.UNSPECIFIED.,.F.,.F.,(4,3,4),(0.0365944846647014,0.0384615384615384,
0.04314661530766),.UNSPECIFIED.);
#1880=B_SPLINE_CURVE_WITH_KNOTS('',3,(#82987,#82988,#82989,#82990,#82991,
#82992,#82993,#82994),.UNSPECIFIED.,.F.,.F.,(4,2,2,4),(1.77257983382598E-6,
0.00863675586255013,0.0171409553449648,0.0172810983525703),
 .UNSPECIFIED.);
#1881=B_SPLINE_CURVE_WITH_KNOTS('',3,(#83019,#83020,#83021,#83022,#83023,
#83024),.UNSPECIFIED.,.F.,.F.,(4,2,4),(0.,0.0198536182927432,0.0397081495002002),
 .UNSPECIFIED.);
#1882=B_SPLINE_CURVE_WITH_KNOTS('',3,(#83042,#83043,#83044,#83045,#83046,
#83047),.UNSPECIFIED.,.F.,.F.,(4,2,4),(-0.00212386589842508,-0.00106193285457721,
0.),.UNSPECIFIED.);
#1883=B_SPLINE_CURVE_WITH_KNOTS('',3,(#83048,#83049,#83050,#83051,#83052,
#83053),.UNSPECIFIED.,.F.,.F.,(4,2,4),(9.999984136454E-7,0.0193527803893325,
0.0387045693968282),.UNSPECIFIED.);
#1884=B_SPLINE_CURVE_WITH_KNOTS('',3,(#83059,#83060,#83061,#83062,#83063,
#83064),.UNSPECIFIED.,.F.,.F.,(4,2,4),(-0.00212486040271112,-0.00106293276267297,
-9.99999999499947E-7),.UNSPECIFIED.);
#1885=B_SPLINE_CURVE_WITH_KNOTS('',3,(#83103,#83104,#83105,#83106,#83107,
#83108),.UNSPECIFIED.,.F.,.F.,(4,2,4),(0.,0.0198583386450044,0.0397175617275022),
 .UNSPECIFIED.);
#1886=B_SPLINE_CURVE_WITH_KNOTS('',3,(#83121,#83122,#83123,#83124,#83125,
#83126),.UNSPECIFIED.,.F.,.F.,(4,2,4),(0.,0.0198761966898207,0.0397532849432792),
 .UNSPECIFIED.);
#1887=B_SPLINE_CURVE_WITH_KNOTS('',3,(#83178,#83179,#83180,#83181,#83182,
#83183),.UNSPECIFIED.,.F.,.F.,(4,2,4),(0.,0.0199008240557302,0.0398025405845411),
 .UNSPECIFIED.);
#1888=B_SPLINE_CURVE_WITH_KNOTS('',3,(#83203,#83204,#83205,#83206,#83207,
#83208),.UNSPECIFIED.,.F.,.F.,(4,2,4),(0.,0.0199042622253509,0.0398094216210589),
 .UNSPECIFIED.);
#1889=B_SPLINE_CURVE_WITH_KNOTS('',3,(#83256,#83257,#83258,#83259,#83260,
#83261),.UNSPECIFIED.,.F.,.F.,(4,2,4),(0.,0.0198954793460365,0.039791861455587),
 .UNSPECIFIED.);
#1890=B_SPLINE_CURVE_WITH_KNOTS('',3,(#83301,#83302,#83303,#83304,#83305,
#83306,#83307),.UNSPECIFIED.,.F.,.F.,(4,3,4),(0.,0.5,0.999990117145585),
 .UNSPECIFIED.);
#1891=B_SPLINE_CURVE_WITH_KNOTS('',3,(#83330,#83331,#83332,#83333,#83334,
#83335),.UNSPECIFIED.,.F.,.F.,(4,2,4),(0.,0.0198677119330699,0.0397363340341339),
 .UNSPECIFIED.);
#1892=B_SPLINE_CURVE_WITH_KNOTS('',3,(#83377,#83378,#83379,#83380,#83381,
#83382),.UNSPECIFIED.,.F.,.F.,(4,2,4),(0.,0.0198973965657402,0.0397956841946094),
 .UNSPECIFIED.);
#1893=B_SPLINE_CURVE_WITH_KNOTS('',3,(#83404,#83405,#83406,#83407,#83408,
#83409),.UNSPECIFIED.,.F.,.F.,(4,2,4),(0.,0.0199030680030106,0.0398070347510793),
 .UNSPECIFIED.);
#1894=B_SPLINE_CURVE_WITH_KNOTS('',3,(#83454,#83455,#83456,#83457,#83458,
#83459),.UNSPECIFIED.,.F.,.F.,(4,2,4),(0.,0.0198994178466467,0.0397997367273577),
 .UNSPECIFIED.);
#1895=B_SPLINE_CURVE_WITH_KNOTS('',3,(#83472,#83473,#83474,#83475,#83476,
#83477),.UNSPECIFIED.,.F.,.F.,(4,2,4),(0.,0.0198905179575656,0.0397819072622247),
 .UNSPECIFIED.);
#1896=B_SPLINE_CURVE_WITH_KNOTS('',3,(#83502,#83503,#83504,#83505,#83506,
#83507,#83508),.UNSPECIFIED.,.F.,.F.,(4,3,4),(0.0365944846647009,0.0384615384615384,
0.0431466153076601),.UNSPECIFIED.);
#1897=B_SPLINE_CURVE_WITH_KNOTS('',3,(#83509,#83510,#83511,#83512,#83513,
#83514,#83515,#83516),.UNSPECIFIED.,.F.,.F.,(4,2,2,4),(1.77257991476566E-6,
0.00863675580737219,0.017140944467863,0.017281088627107),.UNSPECIFIED.);
#1898=B_SPLINE_CURVE_WITH_KNOTS('',3,(#83541,#83542,#83543,#83544,#83545,
#83546),.UNSPECIFIED.,.F.,.F.,(4,2,4),(0.,0.0198536182901603,0.0397081494900814),
 .UNSPECIFIED.);
#1899=B_SPLINE_CURVE_WITH_KNOTS('',3,(#83564,#83565,#83566,#83567,#83568,
#83569),.UNSPECIFIED.,.F.,.F.,(4,2,4),(-0.00212386958331815,-0.0010619343358337,
0.),.UNSPECIFIED.);
#1900=B_SPLINE_CURVE_WITH_KNOTS('',3,(#83570,#83571,#83572,#83573,#83574,
#83575),.UNSPECIFIED.,.F.,.F.,(4,2,4),(9.99998417085594E-7,0.0193527904138238,
0.0387045796352013),.UNSPECIFIED.);
#1901=B_SPLINE_CURVE_WITH_KNOTS('',3,(#83581,#83582,#83583,#83584,#83585,
#83586),.UNSPECIFIED.,.F.,.F.,(4,2,4),(-0.00212486007883822,-0.00106293276263092,
-1.00000000208484E-6),.UNSPECIFIED.);
#1902=B_SPLINE_CURVE_WITH_KNOTS('',3,(#83625,#83626,#83627,#83628,#83629,
#83630),.UNSPECIFIED.,.F.,.F.,(4,2,4),(0.,0.0198583386419039,0.0397175617148195),
 .UNSPECIFIED.);
#1903=B_SPLINE_CURVE_WITH_KNOTS('',3,(#83643,#83644,#83645,#83646,#83647,
#83648),.UNSPECIFIED.,.F.,.F.,(4,2,4),(0.,0.0198761965843594,0.0397532847208746),
 .UNSPECIFIED.);
#1904=B_SPLINE_CURVE_WITH_KNOTS('',3,(#83700,#83701,#83702,#83703,#83704,
#83705),.UNSPECIFIED.,.F.,.F.,(4,2,4),(0.,0.0199008240528343,0.0398025405727771),
 .UNSPECIFIED.);
#1905=B_SPLINE_CURVE_WITH_KNOTS('',3,(#83718,#83719,#83720,#83721,#83722,
#83723),.UNSPECIFIED.,.F.,.F.,(4,2,4),(0.,0.0199042047135222,0.039809289172212),
 .UNSPECIFIED.);
#1906=B_SPLINE_CURVE_WITH_KNOTS('',3,(#83768,#83769,#83770,#83771,#83772,
#83773),.UNSPECIFIED.,.F.,.F.,(4,2,4),(0.,0.0198954793428837,0.0397918614431882),
 .UNSPECIFIED.);
#1907=B_SPLINE_CURVE_WITH_KNOTS('',3,(#83820,#83821,#83822,#83823,#83824,
#83825,#83826),.UNSPECIFIED.,.F.,.F.,(4,3,4),(0.,0.5,0.999990117143057),
 .UNSPECIFIED.);
#1908=B_SPLINE_CURVE_WITH_KNOTS('',3,(#83849,#83850,#83851,#83852,#83853,
#83854),.UNSPECIFIED.,.F.,.F.,(4,2,4),(0.,0.0198677119280884,0.0397363340135476),
 .UNSPECIFIED.);
#1909=B_SPLINE_CURVE_WITH_KNOTS('',3,(#83896,#83897,#83898,#83899,#83900,
#83901),.UNSPECIFIED.,.F.,.F.,(4,2,4),(0.,0.0198973965647451,0.0397956841902401),
 .UNSPECIFIED.);
#1910=B_SPLINE_CURVE_WITH_KNOTS('',3,(#83923,#83924,#83925,#83926,#83927,
#83928),.UNSPECIFIED.,.F.,.F.,(4,2,4),(0.,0.0199030679985029,0.0398070347325486),
 .UNSPECIFIED.);
#1911=B_SPLINE_CURVE_WITH_KNOTS('',3,(#83973,#83974,#83975,#83976,#83977,
#83978),.UNSPECIFIED.,.F.,.F.,(4,2,4),(0.,0.0198994178454141,0.0397997367225458),
 .UNSPECIFIED.);
#1912=B_SPLINE_CURVE_WITH_KNOTS('',3,(#83991,#83992,#83993,#83994,#83995,
#83996),.UNSPECIFIED.,.F.,.F.,(4,2,4),(0.,0.0198905179578417,0.039781907267824),
 .UNSPECIFIED.);
#1913=B_SPLINE_CURVE_WITH_KNOTS('',3,(#84021,#84022,#84023,#84024,#84025,
#84026,#84027),.UNSPECIFIED.,.F.,.F.,(4,3,4),(0.0365944846647011,0.0384615384615384,
0.0431466153076598),.UNSPECIFIED.);
#1914=B_SPLINE_CURVE_WITH_KNOTS('',3,(#84028,#84029,#84030,#84031,#84032,
#84033,#84034,#84035),.UNSPECIFIED.,.F.,.F.,(4,2,2,4),(1.77350747916397E-6,
0.00863675580036768,0.017140922315829,0.0172810687295207),.UNSPECIFIED.);
#1915=B_SPLINE_CURVE_WITH_KNOTS('',3,(#84060,#84061,#84062,#84063,#84064,
#84065),.UNSPECIFIED.,.F.,.F.,(4,2,4),(0.,0.0198536182877321,0.0397081494798666),
 .UNSPECIFIED.);
#1916=B_SPLINE_CURVE_WITH_KNOTS('',3,(#84083,#84084,#84085,#84086,#84087,
#84088),.UNSPECIFIED.,.F.,.F.,(4,2,4),(-0.00212387260142457,-0.00106193554358744,
0.),.UNSPECIFIED.);
#1917=B_SPLINE_CURVE_WITH_KNOTS('',3,(#84089,#84090,#84091,#84092,#84093,
#84094),.UNSPECIFIED.,.F.,.F.,(4,2,4),(9.99998417845244E-7,0.0193527896159823,
0.0387045796147699),.UNSPECIFIED.);
#1918=B_SPLINE_CURVE_WITH_KNOTS('',3,(#84100,#84101,#84102,#84103,#84104,
#84105),.UNSPECIFIED.,.F.,.F.,(4,2,4),(-0.00212485975597055,-0.00106293275863081,
-1.00000000247038E-6),.UNSPECIFIED.);
#1919=B_SPLINE_CURVE_WITH_KNOTS('',3,(#84144,#84145,#84146,#84147,#84148,
#84149),.UNSPECIFIED.,.F.,.F.,(4,2,4),(0.,0.0198583386395679,0.0397175617056758),
 .UNSPECIFIED.);
#1920=B_SPLINE_CURVE_WITH_KNOTS('',3,(#84162,#84163,#84164,#84165,#84166,
#84167),.UNSPECIFIED.,.F.,.F.,(4,2,4),(0.,0.0198761966924393,0.0397532849423359),
 .UNSPECIFIED.);
#1921=B_SPLINE_CURVE_WITH_KNOTS('',3,(#84219,#84220,#84221,#84222,#84223,
#84224),.UNSPECIFIED.,.F.,.F.,(4,2,4),(0.,0.0199008240503633,0.0398025405628424),
 .UNSPECIFIED.);
#1922=B_SPLINE_CURVE_WITH_KNOTS('',3,(#84237,#84238,#84239,#84240,#84241,
#84242),.UNSPECIFIED.,.F.,.F.,(4,2,4),(0.,0.0199042047129859,0.0398092891685953),
 .UNSPECIFIED.);
#1923=B_SPLINE_CURVE_WITH_KNOTS('',3,(#84290,#84291,#84292,#84293,#84294,
#84295),.UNSPECIFIED.,.F.,.F.,(4,2,4),(0.,0.0198954793400186,0.0397918614313439),
 .UNSPECIFIED.);
#1924=B_SPLINE_CURVE_WITH_KNOTS('',3,(#84335,#84336,#84337,#84338,#84339,
#84340,#84341),.UNSPECIFIED.,.F.,.F.,(4,3,4),(0.,0.5,0.999990117139736),
 .UNSPECIFIED.);
#1925=B_SPLINE_CURVE_WITH_KNOTS('',3,(#84364,#84365,#84366,#84367,#84368,
#84369),.UNSPECIFIED.,.F.,.F.,(4,2,4),(0.,0.0198677119226095,0.0397363339916417),
 .UNSPECIFIED.);
#1926=B_SPLINE_CURVE_WITH_KNOTS('',3,(#84411,#84412,#84413,#84414,#84415,
#84416),.UNSPECIFIED.,.F.,.F.,(4,2,4),(0.,0.0198973965640123,0.0397956841869985),
 .UNSPECIFIED.);
#1927=B_SPLINE_CURVE_WITH_KNOTS('',3,(#84438,#84439,#84440,#84441,#84442,
#84443),.UNSPECIFIED.,.F.,.F.,(4,2,4),(0.,0.0199030679932799,0.0398070347114654),
 .UNSPECIFIED.);
#1928=B_SPLINE_CURVE_WITH_KNOTS('',3,(#84488,#84489,#84490,#84491,#84492,
#84493),.UNSPECIFIED.,.F.,.F.,(4,2,4),(0.,0.0198994178439414,0.0397997367162081),
 .UNSPECIFIED.);
#1929=B_SPLINE_CURVE_WITH_KNOTS('',3,(#84506,#84507,#84508,#84509,#84510,
#84511),.UNSPECIFIED.,.F.,.F.,(4,2,4),(0.,0.019890517442833,0.0397819062338529),
 .UNSPECIFIED.);
#1930=B_SPLINE_CURVE_WITH_KNOTS('',3,(#84536,#84537,#84538,#84539,#84540,
#84541,#84542),.UNSPECIFIED.,.F.,.F.,(4,3,4),(0.0365944846647008,0.0384615384615384,
0.0431466153076597),.UNSPECIFIED.);
#1931=B_SPLINE_CURVE_WITH_KNOTS('',3,(#84543,#84544,#84545,#84546,#84547,
#84548,#84549,#84550),.UNSPECIFIED.,.F.,.F.,(4,2,2,4),(1.77292709988644E-6,
0.0086367558366745,0.0171409573179643,0.0172811000564802),.UNSPECIFIED.);
#1932=B_SPLINE_CURVE_WITH_KNOTS('',3,(#84575,#84576,#84577,#84578,#84579,
#84580),.UNSPECIFIED.,.F.,.F.,(4,2,4),(0.,0.0198536182904639,0.0397081494895467),
 .UNSPECIFIED.);
#1933=B_SPLINE_CURVE_WITH_KNOTS('',3,(#84598,#84599,#84600,#84601,#84602,
#84603),.UNSPECIFIED.,.F.,.F.,(4,2,4),(-0.00212387561594626,-0.00106193674627472,
0.),.UNSPECIFIED.);
#1934=B_SPLINE_CURVE_WITH_KNOTS('',3,(#84604,#84605,#84606,#84607,#84608,
#84609),.UNSPECIFIED.,.F.,.F.,(4,2,4),(9.99998416488062E-7,0.0193532848499299,
0.0387045795217607),.UNSPECIFIED.);
#1935=B_SPLINE_CURVE_WITH_KNOTS('',3,(#84615,#84616,#84617,#84618,#84619,
#84620),.UNSPECIFIED.,.F.,.F.,(4,2,4),(-0.00212485951467819,-0.00106293276219924,
-1.00000000035185E-6),.UNSPECIFIED.);
#1936=B_SPLINE_CURVE_WITH_KNOTS('',3,(#84659,#84660,#84661,#84662,#84663,
#84664),.UNSPECIFIED.,.F.,.F.,(4,2,4),(0.,0.0198583386383744,0.0397175617010874),
 .UNSPECIFIED.);
#1937=B_SPLINE_CURVE_WITH_KNOTS('',3,(#84677,#84678,#84679,#84680,#84681,
#84682),.UNSPECIFIED.,.F.,.F.,(4,2,4),(0.,0.0198761966567487,0.0397532848798819),
 .UNSPECIFIED.);
#1938=B_SPLINE_CURVE_WITH_KNOTS('',3,(#84734,#84735,#84736,#84737,#84738,
#84739),.UNSPECIFIED.,.F.,.F.,(4,2,4),(0.,0.0199008240483616,0.0398025405546555),
 .UNSPECIFIED.);
#1939=B_SPLINE_CURVE_WITH_KNOTS('',3,(#84752,#84753,#84754,#84755,#84756,
#84757),.UNSPECIFIED.,.F.,.F.,(4,2,4),(0.,0.0199042047130261,0.0398092891574592),
 .UNSPECIFIED.);
#1940=B_SPLINE_CURVE_WITH_KNOTS('',3,(#84805,#84806,#84807,#84808,#84809,
#84810),.UNSPECIFIED.,.F.,.F.,(4,2,4),(0.,0.0198954793377787,0.0397918614218809),
 .UNSPECIFIED.);
#1941=B_SPLINE_CURVE_WITH_KNOTS('',3,(#84850,#84851,#84852,#84853,#84854,
#84855,#84856),.UNSPECIFIED.,.F.,.F.,(4,3,4),(0.,0.5,0.999990117136952),
 .UNSPECIFIED.);
#1942=B_SPLINE_CURVE_WITH_KNOTS('',3,(#84879,#84880,#84881,#84882,#84883,
#84884),.UNSPECIFIED.,.F.,.F.,(4,2,4),(0.,0.0198677119178716,0.0397363339724512),
 .UNSPECIFIED.);
#1943=B_SPLINE_CURVE_WITH_KNOTS('',3,(#84926,#84927,#84928,#84929,#84930,
#84931),.UNSPECIFIED.,.F.,.F.,(4,2,4),(0.,0.019897396564037,0.0397956841876327),
 .UNSPECIFIED.);
#1944=B_SPLINE_CURVE_WITH_KNOTS('',3,(#84953,#84954,#84955,#84956,#84957,
#84958),.UNSPECIFIED.,.F.,.F.,(4,2,4),(0.,0.0199030679169175,0.0398070344753143),
 .UNSPECIFIED.);
#1945=B_SPLINE_CURVE_WITH_KNOTS('',3,(#85003,#85004,#85005,#85006,#85007,
#85008),.UNSPECIFIED.,.F.,.F.,(4,2,4),(0.,0.0198994178439266,0.0397997367162002),
 .UNSPECIFIED.);
#1946=B_SPLINE_CURVE_WITH_KNOTS('',3,(#85021,#85022,#85023,#85024,#85025,
#85026),.UNSPECIFIED.,.F.,.F.,(4,2,4),(0.,0.0198905179576396,0.0397819072528401),
 .UNSPECIFIED.);
#1947=B_SPLINE_CURVE_WITH_KNOTS('',3,(#85051,#85052,#85053,#85054,#85055,
#85056,#85057),.UNSPECIFIED.,.F.,.F.,(4,3,4),(0.0365944846647013,0.0384615384615384,
0.0431466153076595),.UNSPECIFIED.);
#1948=B_SPLINE_CURVE_WITH_KNOTS('',3,(#85058,#85059,#85060,#85061,#85062,
#85063,#85064,#85065),.UNSPECIFIED.,.F.,.F.,(4,2,2,4),(1.77257998041709E-6,
0.00863675581017835,0.0171409340093189,0.0172810792958315),
 .UNSPECIFIED.);
#1949=B_SPLINE_CURVE_WITH_KNOTS('',3,(#85090,#85091,#85092,#85093,#85094,
#85095),.UNSPECIFIED.,.F.,.F.,(4,2,4),(0.,0.0198536182858879,0.0397081494725743),
 .UNSPECIFIED.);
#1950=B_SPLINE_CURVE_WITH_KNOTS('',3,(#85113,#85114,#85115,#85116,#85117,
#85118),.UNSPECIFIED.,.F.,.F.,(4,2,4),(-0.00212387854594797,-0.00106193791950009,
0.),.UNSPECIFIED.);
#1951=B_SPLINE_CURVE_WITH_KNOTS('',3,(#85119,#85120,#85121,#85122,#85123,
#85124),.UNSPECIFIED.,.F.,.F.,(4,2,4),(9.9999841885959E-7,0.019352785410249,
0.0387045795338068),.UNSPECIFIED.);
#1952=B_SPLINE_CURVE_WITH_KNOTS('',3,(#85130,#85131,#85132,#85133,#85134,
#85135),.UNSPECIFIED.,.F.,.F.,(4,2,4),(-0.00212485939877907,-0.00106293275771695,
-1.0000000009139E-6),.UNSPECIFIED.);
#1953=B_SPLINE_CURVE_WITH_KNOTS('',3,(#85174,#85175,#85176,#85177,#85178,
#85179),.UNSPECIFIED.,.F.,.F.,(4,2,4),(0.,0.0198583386375086,0.0397175616972905),
 .UNSPECIFIED.);
#1954=B_SPLINE_CURVE_WITH_KNOTS('',3,(#85192,#85193,#85194,#85195,#85196,
#85197),.UNSPECIFIED.,.F.,.F.,(4,2,4),(0.,0.0198761967049228,0.0397532849789576),
 .UNSPECIFIED.);
#1955=B_SPLINE_CURVE_WITH_KNOTS('',3,(#85249,#85250,#85251,#85252,#85253,
#85254),.UNSPECIFIED.,.F.,.F.,(4,2,4),(0.,0.0199008240467533,0.0398025405489657),
 .UNSPECIFIED.);
#1956=B_SPLINE_CURVE_WITH_KNOTS('',3,(#85267,#85268,#85269,#85270,#85271,
#85272),.UNSPECIFIED.,.F.,.F.,(4,2,4),(0.,0.0199042047189651,0.0398092891742666),
 .UNSPECIFIED.);
#1957=B_SPLINE_CURVE_WITH_KNOTS('',3,(#85320,#85321,#85322,#85323,#85324,
#85325),.UNSPECIFIED.,.F.,.F.,(4,2,4),(0.,0.0198954793358551,0.0397918614147188),
 .UNSPECIFIED.);
#1958=B_SPLINE_CURVE_WITH_KNOTS('',3,(#85365,#85366,#85367,#85368,#85369,
#85370,#85371),.UNSPECIFIED.,.F.,.F.,(4,3,4),(0.,0.5,0.999990117133631),
 .UNSPECIFIED.);
#1959=B_SPLINE_CURVE_WITH_KNOTS('',3,(#85394,#85395,#85396,#85397,#85398,
#85399),.UNSPECIFIED.,.F.,.F.,(4,2,4),(0.,0.0198677119133151,0.0397363339545231),
 .UNSPECIFIED.);
#1960=B_SPLINE_CURVE_WITH_KNOTS('',3,(#85441,#85442,#85443,#85444,#85445,
#85446),.UNSPECIFIED.,.F.,.F.,(4,2,4),(0.,0.019897396565073,0.0397956841914982),
 .UNSPECIFIED.);
#1961=B_SPLINE_CURVE_WITH_KNOTS('',3,(#85468,#85469,#85470,#85471,#85472,
#85473),.UNSPECIFIED.,.F.,.F.,(4,2,4),(0.,0.019903067983549,0.0398070346719),
 .UNSPECIFIED.);
#1962=B_SPLINE_CURVE_WITH_KNOTS('',3,(#85518,#85519,#85520,#85521,#85522,
#85523),.UNSPECIFIED.,.F.,.F.,(4,2,4),(0.,0.0198994178443784,0.0397997367178181),
 .UNSPECIFIED.);
#1963=B_SPLINE_CURVE_WITH_KNOTS('',3,(#85536,#85537,#85538,#85539,#85540,
#85541),.UNSPECIFIED.,.F.,.F.,(4,2,4),(0.,0.0198905179573494,0.0397819072555251),
 .UNSPECIFIED.);
#1964=B_SPLINE_CURVE_WITH_KNOTS('',3,(#85566,#85567,#85568,#85569,#85570,
#85571,#85572),.UNSPECIFIED.,.F.,.F.,(4,3,4),(0.0365944846647011,0.0384615384615384,
0.0431466153076598),.UNSPECIFIED.);
#1965=B_SPLINE_CURVE_WITH_KNOTS('',3,(#85573,#85574,#85575,#85576,#85577,
#85578,#85579,#85580),.UNSPECIFIED.,.F.,.F.,(4,2,2,4),(1.77257445604461E-6,
0.0086367557856313,0.017140932747332,0.0172810781644652),.UNSPECIFIED.);
#1966=B_SPLINE_CURVE_WITH_KNOTS('',3,(#85605,#85606,#85607,#85608,#85609,
#85610),.UNSPECIFIED.,.F.,.F.,(4,2,4),(0.,0.0198536182864876,0.0397081494752219),
 .UNSPECIFIED.);
#1967=B_SPLINE_CURVE_WITH_KNOTS('',3,(#85628,#85629,#85630,#85631,#85632,
#85633),.UNSPECIFIED.,.F.,.F.,(4,2,4),(-0.00212388115337583,-0.00106193896363325,
0.),.UNSPECIFIED.);
#1968=B_SPLINE_CURVE_WITH_KNOTS('',3,(#85634,#85635,#85636,#85637,#85638,
#85639),.UNSPECIFIED.,.F.,.F.,(4,2,4),(9.99998415348017E-7,0.0193527753883658,
0.0387045692997803),.UNSPECIFIED.);
#1969=B_SPLINE_CURVE_WITH_KNOTS('',3,(#85645,#85646,#85647,#85648,#85649,
#85650),.UNSPECIFIED.,.F.,.F.,(4,2,4),(-0.00212485930517326,-0.00106293276164361,
-9.99999999790814E-7),.UNSPECIFIED.);
#1970=B_SPLINE_CURVE_WITH_KNOTS('',3,(#85689,#85690,#85691,#85692,#85693,
#85694),.UNSPECIFIED.,.F.,.F.,(4,2,4),(0.,0.0198583386372447,0.0397175616961046),
 .UNSPECIFIED.);
#1971=B_SPLINE_CURVE_WITH_KNOTS('',3,(#85707,#85708,#85709,#85710,#85711,
#85712),.UNSPECIFIED.,.F.,.F.,(4,2,4),(0.,0.0198761967024035,0.0397532849668273),
 .UNSPECIFIED.);
#1972=B_SPLINE_CURVE_WITH_KNOTS('',3,(#85764,#85765,#85766,#85767,#85768,
#85769),.UNSPECIFIED.,.F.,.F.,(4,2,4),(0.,0.0199008240468501,0.0398025405488885),
 .UNSPECIFIED.);
#1973=B_SPLINE_CURVE_WITH_KNOTS('',3,(#85782,#85783,#85784,#85785,#85786,
#85787),.UNSPECIFIED.,.F.,.F.,(4,2,4),(0.,0.0199042047191258,0.0398092891768156),
 .UNSPECIFIED.);
#1974=B_SPLINE_CURVE_WITH_KNOTS('',3,(#85835,#85836,#85837,#85838,#85839,
#85840),.UNSPECIFIED.,.F.,.F.,(4,2,4),(0.,0.0198954793351462,0.0397918614117019),
 .UNSPECIFIED.);
#1975=B_SPLINE_CURVE_WITH_KNOTS('',3,(#85880,#85881,#85882,#85883,#85884,
#85885,#85886),.UNSPECIFIED.,.F.,.F.,(4,3,4),(0.,0.5,0.999990117130729),
 .UNSPECIFIED.);
#1976=B_SPLINE_CURVE_WITH_KNOTS('',3,(#85909,#85910,#85911,#85912,#85913,
#85914),.UNSPECIFIED.,.F.,.F.,(4,2,4),(0.,0.0198677119088387,0.039736333935962),
 .UNSPECIFIED.);
#1977=B_SPLINE_CURVE_WITH_KNOTS('',3,(#85956,#85957,#85958,#85959,#85960,
#85961),.UNSPECIFIED.,.F.,.F.,(4,2,4),(0.,0.0198973965662461,0.0397956841962341),
 .UNSPECIFIED.);
#1978=B_SPLINE_CURVE_WITH_KNOTS('',3,(#85983,#85984,#85985,#85986,#85987,
#85988),.UNSPECIFIED.,.F.,.F.,(4,2,4),(0.,0.0199030679089294,0.0398070344430507),
 .UNSPECIFIED.);
#1979=B_SPLINE_CURVE_WITH_KNOTS('',3,(#86033,#86034,#86035,#86036,#86037,
#86038),.UNSPECIFIED.,.F.,.F.,(4,2,4),(0.,0.0198994178459843,0.0397997367240867),
 .UNSPECIFIED.);
#1980=B_SPLINE_CURVE_WITH_KNOTS('',3,(#86051,#86052,#86053,#86054,#86055,
#86056),.UNSPECIFIED.,.F.,.F.,(4,2,4),(0.,0.0198905179578903,0.0397819072560775),
 .UNSPECIFIED.);
#1981=B_SPLINE_CURVE_WITH_KNOTS('',3,(#86081,#86082,#86083,#86084,#86085,
#86086,#86087),.UNSPECIFIED.,.F.,.F.,(4,3,4),(0.0365944846647006,0.0384615384615384,
0.0431466153076595),.UNSPECIFIED.);
#1982=B_SPLINE_CURVE_WITH_KNOTS('',3,(#86088,#86089,#86090,#86091,#86092,
#86093,#86094,#86095),.UNSPECIFIED.,.F.,.F.,(4,2,2,4),(1.77257423772781E-6,
0.00863675585116524,0.0171409641324324,0.0172811061893529),
 .UNSPECIFIED.);
#1983=B_SPLINE_CURVE_WITH_KNOTS('',3,(#86120,#86121,#86122,#86123,#86124,
#86125),.UNSPECIFIED.,.F.,.F.,(4,2,4),(0.,0.019853618287136,0.03970814947742),
 .UNSPECIFIED.);
#1984=B_SPLINE_CURVE_WITH_KNOTS('',3,(#86143,#86144,#86145,#86146,#86147,
#86148),.UNSPECIFIED.,.F.,.F.,(4,2,4),(-0.00212388284445759,-0.00106193963809625,
0.),.UNSPECIFIED.);
#1985=B_SPLINE_CURVE_WITH_KNOTS('',3,(#86149,#86150,#86151,#86152,#86153,
#86154),.UNSPECIFIED.,.F.,.F.,(4,2,4),(9.99998416549644E-7,0.019353285396123,
0.0387045795327764),.UNSPECIFIED.);
#1986=B_SPLINE_CURVE_WITH_KNOTS('',3,(#86160,#86161,#86162,#86163,#86164,
#86165),.UNSPECIFIED.,.F.,.F.,(4,2,4),(-0.00212485927854704,-0.00106293275914596,
-1.00000000017165E-6),.UNSPECIFIED.);
#1987=B_SPLINE_CURVE_WITH_KNOTS('',3,(#86204,#86205,#86206,#86207,#86208,
#86209),.UNSPECIFIED.,.F.,.F.,(4,2,4),(0.,0.0198583386380477,0.0397175616990257),
 .UNSPECIFIED.);
#1988=B_SPLINE_CURVE_WITH_KNOTS('',3,(#86222,#86223,#86224,#86225,#86226,
#86227),.UNSPECIFIED.,.F.,.F.,(4,2,4),(0.,0.0198761967031353,0.0397532849810569),
 .UNSPECIFIED.);
#1989=B_SPLINE_CURVE_WITH_KNOTS('',3,(#86279,#86280,#86281,#86282,#86283,
#86284),.UNSPECIFIED.,.F.,.F.,(4,2,4),(0.,0.0199008240464419,0.0398025405473232),
 .UNSPECIFIED.);
#1990=B_SPLINE_CURVE_WITH_KNOTS('',3,(#86297,#86298,#86299,#86300,#86301,
#86302),.UNSPECIFIED.,.F.,.F.,(4,2,4),(0.,0.0199042047190527,0.039809289180571),
 .UNSPECIFIED.);
#1991=B_SPLINE_CURVE_WITH_KNOTS('',3,(#86350,#86351,#86352,#86353,#86354,
#86355),.UNSPECIFIED.,.F.,.F.,(4,2,4),(0.,0.0198954793351661,0.0397918614116676),
 .UNSPECIFIED.);
#1992=B_SPLINE_CURVE_WITH_KNOTS('',3,(#86395,#86396,#86397,#86398,#86399,
#86400,#86401),.UNSPECIFIED.,.F.,.F.,(4,3,4),(0.,0.5,0.999990117128898),
 .UNSPECIFIED.);
#1993=B_SPLINE_CURVE_WITH_KNOTS('',3,(#86424,#86425,#86426,#86427,#86428,
#86429),.UNSPECIFIED.,.F.,.F.,(4,2,4),(0.,0.0198677119052138,0.0397363339218776),
 .UNSPECIFIED.);
#1994=B_SPLINE_CURVE_WITH_KNOTS('',3,(#86471,#86472,#86473,#86474,#86475,
#86476),.UNSPECIFIED.,.F.,.F.,(4,2,4),(0.,0.0198973965680208,0.0397956842029936),
 .UNSPECIFIED.);
#1995=B_SPLINE_CURVE_WITH_KNOTS('',3,(#86498,#86499,#86500,#86501,#86502,
#86503),.UNSPECIFIED.,.F.,.F.,(4,2,4),(0.,0.0199030679777334,0.0398070346486175),
 .UNSPECIFIED.);
#1996=B_SPLINE_CURVE_WITH_KNOTS('',3,(#86548,#86549,#86550,#86551,#86552,
#86553),.UNSPECIFIED.,.F.,.F.,(4,2,4),(0.,0.0198994178470161,0.0397997367286354),
 .UNSPECIFIED.);
#1997=B_SPLINE_CURVE_WITH_KNOTS('',3,(#86566,#86567,#86568,#86569,#86570,
#86571),.UNSPECIFIED.,.F.,.F.,(4,2,4),(0.,0.0198905179576503,0.0397819072501323),
 .UNSPECIFIED.);
#1998=B_SPLINE_CURVE_WITH_KNOTS('',3,(#86596,#86597,#86598,#86599,#86600,
#86601,#86602),.UNSPECIFIED.,.F.,.F.,(4,3,4),(0.0365944846647007,0.0384615384615384,
0.0431466153076595),.UNSPECIFIED.);
#1999=B_SPLINE_CURVE_WITH_KNOTS('',3,(#86603,#86604,#86605,#86606,#86607,
#86608,#86609,#86610),.UNSPECIFIED.,.F.,.F.,(4,2,2,4),(1.77350725314824E-6,
0.00863675587077613,0.0171409468521658,0.0172810906422092),
 .UNSPECIFIED.);
#2000=B_SPLINE_CURVE_WITH_KNOTS('',3,(#86635,#86636,#86637,#86638,#86639,
#86640),.UNSPECIFIED.,.F.,.F.,(4,2,4),(0.,0.0198536182885339,0.0397081494834228),
 .UNSPECIFIED.);
#2001=B_SPLINE_CURVE_WITH_KNOTS('',3,(#86658,#86659,#86660,#86661,#86662,
#86663),.UNSPECIFIED.,.F.,.F.,(4,2,4),(-0.00212388622566706,-0.00106194099469101,
0.),.UNSPECIFIED.);
#2002=B_SPLINE_CURVE_WITH_KNOTS('',3,(#86664,#86665,#86666,#86667,#86668,
#86669),.UNSPECIFIED.,.F.,.F.,(4,2,4),(9.99998417676033E-7,0.0193527846155029,
0.0387045795199078),.UNSPECIFIED.);
#2003=B_SPLINE_CURVE_WITH_KNOTS('',3,(#86675,#86676,#86677,#86678,#86679,
#86680),.UNSPECIFIED.,.F.,.F.,(4,2,4),(-0.00212485935732975,-0.00106293275849113,
-9.9999999990987E-7),.UNSPECIFIED.);
#2004=B_SPLINE_CURVE_WITH_KNOTS('',3,(#86719,#86720,#86721,#86722,#86723,
#86724),.UNSPECIFIED.,.F.,.F.,(4,2,4),(0.,0.0198583386387385,0.0397175617020387),
 .UNSPECIFIED.);
#2005=B_SPLINE_CURVE_WITH_KNOTS('',3,(#86737,#86738,#86739,#86740,#86741,
#86742),.UNSPECIFIED.,.F.,.F.,(4,2,4),(0.,0.0198761966976469,0.0397532849454558),
 .UNSPECIFIED.);
#2006=B_SPLINE_CURVE_WITH_KNOTS('',3,(#86794,#86795,#86796,#86797,#86798,
#86799),.UNSPECIFIED.,.F.,.F.,(4,2,4),(0.,0.0199008240470287,0.0398025405500045),
 .UNSPECIFIED.);
#2007=B_SPLINE_CURVE_WITH_KNOTS('',3,(#86812,#86813,#86814,#86815,#86816,
#86817),.UNSPECIFIED.,.F.,.F.,(4,2,4),(0.,0.0199042047189135,0.0398092891728897),
 .UNSPECIFIED.);
#2008=B_SPLINE_CURVE_WITH_KNOTS('',3,(#86865,#86866,#86867,#86868,#86869,
#86870),.UNSPECIFIED.,.F.,.F.,(4,2,4),(0.,0.0198954793353804,0.0397918614125083),
 .UNSPECIFIED.);
#2009=B_SPLINE_CURVE_WITH_KNOTS('',3,(#86910,#86911,#86912,#86913,#86914,
#86915,#86916),.UNSPECIFIED.,.F.,.F.,(4,3,4),(0.,0.5,0.99999011712649),
 .UNSPECIFIED.);
#2010=B_SPLINE_CURVE_WITH_KNOTS('',3,(#86939,#86940,#86941,#86942,#86943,
#86944),.UNSPECIFIED.,.F.,.F.,(4,2,4),(0.,0.0198677119013193,0.0397363339055224),
 .UNSPECIFIED.);
#2011=B_SPLINE_CURVE_WITH_KNOTS('',3,(#86986,#86987,#86988,#86989,#86990,
#86991),.UNSPECIFIED.,.F.,.F.,(4,2,4),(0.,0.0198973965708148,0.0397956842143026),
 .UNSPECIFIED.);
#2012=B_SPLINE_CURVE_WITH_KNOTS('',3,(#87013,#87014,#87015,#87016,#87017,
#87018),.UNSPECIFIED.,.F.,.F.,(4,2,4),(0.,0.019903067974991,0.039807034637192),
 .UNSPECIFIED.);
#2013=B_SPLINE_CURVE_WITH_KNOTS('',3,(#87063,#87064,#87065,#87066,#87067,
#87068),.UNSPECIFIED.,.F.,.F.,(4,2,4),(0.,0.019899417849379,0.039799736737851),
 .UNSPECIFIED.);
#2014=B_SPLINE_CURVE_WITH_KNOTS('',3,(#87081,#87082,#87083,#87084,#87085,
#87086),.UNSPECIFIED.,.F.,.F.,(4,2,4),(0.,0.0198905179576478,0.0397819072520095),
 .UNSPECIFIED.);
#2015=B_SPLINE_CURVE_WITH_KNOTS('',3,(#87111,#87112,#87113,#87114,#87115,
#87116,#87117),.UNSPECIFIED.,.F.,.F.,(4,3,4),(0.0365944846647008,0.0384615384615384,
0.0431466153076604),.UNSPECIFIED.);
#2016=B_SPLINE_CURVE_WITH_KNOTS('',3,(#87118,#87119,#87120,#87121,#87122,
#87123,#87124,#87125),.UNSPECIFIED.,.F.,.F.,(4,2,2,4),(1.77257424359709E-6,
0.00863675585403953,0.0171409617643079,0.0172811040803507),
 .UNSPECIFIED.);
#2017=B_SPLINE_CURVE_WITH_KNOTS('',3,(#87150,#87151,#87152,#87153,#87154,
#87155),.UNSPECIFIED.,.F.,.F.,(4,2,4),(0.,0.0198536182903914,0.0397081494910964),
 .UNSPECIFIED.);
#2018=B_SPLINE_CURVE_WITH_KNOTS('',3,(#87173,#87174,#87175,#87176,#87177,
#87178),.UNSPECIFIED.,.F.,.F.,(4,2,4),(-0.00212388840135336,-0.00106194186675072,
0.),.UNSPECIFIED.);
#2019=B_SPLINE_CURVE_WITH_KNOTS('',3,(#87179,#87180,#87181,#87182,#87183,
#87184),.UNSPECIFIED.,.F.,.F.,(4,2,4),(9.99998422430955E-7,0.0193522803908578,
0.0387045693979158),.UNSPECIFIED.);
#2020=B_SPLINE_CURVE_WITH_KNOTS('',3,(#87190,#87191,#87192,#87193,#87194,
#87195),.UNSPECIFIED.,.F.,.F.,(4,2,4),(-0.00212485944936608,-0.00106293276036146,
-9.99999998619293E-7),.UNSPECIFIED.);
#2021=B_SPLINE_CURVE_WITH_KNOTS('',3,(#87234,#87235,#87236,#87237,#87238,
#87239),.UNSPECIFIED.,.F.,.F.,(4,2,4),(0.,0.0198583386404155,0.0397175617084474),
 .UNSPECIFIED.);
#2022=B_SPLINE_CURVE_WITH_KNOTS('',3,(#87252,#87253,#87254,#87255,#87256,
#87257),.UNSPECIFIED.,.F.,.F.,(4,2,4),(0.,0.0198761967052115,0.039753284964214),
 .UNSPECIFIED.);
#2023=B_SPLINE_CURVE_WITH_KNOTS('',3,(#87309,#87310,#87311,#87312,#87313,
#87314),.UNSPECIFIED.,.F.,.F.,(4,2,4),(0.,0.0199008240486882,0.0398025405564813),
 .UNSPECIFIED.);
#2024=B_SPLINE_CURVE_WITH_KNOTS('',3,(#87327,#87328,#87329,#87330,#87331,
#87332),.UNSPECIFIED.,.F.,.F.,(4,2,4),(0.,0.0199042046968269,0.0398092891377679),
 .UNSPECIFIED.);
#2025=B_SPLINE_CURVE_WITH_KNOTS('',3,(#87380,#87381,#87382,#87383,#87384,
#87385),.UNSPECIFIED.,.F.,.F.,(4,2,4),(0.,0.0198954793366912,0.0397918614176109),
 .UNSPECIFIED.);
#2026=B_SPLINE_CURVE_WITH_KNOTS('',3,(#87425,#87426,#87427,#87428,#87429,
#87430,#87431),.UNSPECIFIED.,.F.,.F.,(4,3,4),(0.,0.5,0.999990117124345),
 .UNSPECIFIED.);
#2027=B_SPLINE_CURVE_WITH_KNOTS('',3,(#87454,#87455,#87456,#87457,#87458,
#87459),.UNSPECIFIED.,.F.,.F.,(4,2,4),(0.,0.0198677118984356,0.0397363338941566),
 .UNSPECIFIED.);
#2028=B_SPLINE_CURVE_WITH_KNOTS('',3,(#87501,#87502,#87503,#87504,#87505,
#87506),.UNSPECIFIED.,.F.,.F.,(4,2,4),(0.,0.0198973965734549,0.0397956842251395),
 .UNSPECIFIED.);
#2029=B_SPLINE_CURVE_WITH_KNOTS('',3,(#87528,#87529,#87530,#87531,#87532,
#87533),.UNSPECIFIED.,.F.,.F.,(4,2,4),(0.,0.0199030679732815,0.0398070346300929),
 .UNSPECIFIED.);
#2030=B_SPLINE_CURVE_WITH_KNOTS('',3,(#87578,#87579,#87580,#87581,#87582,
#87583),.UNSPECIFIED.,.F.,.F.,(4,2,4),(0.,0.0198994178519258,0.0397997367485529),
 .UNSPECIFIED.);
#2031=B_SPLINE_CURVE_WITH_KNOTS('',3,(#87596,#87597,#87598,#87599,#87600,
#87601),.UNSPECIFIED.,.F.,.F.,(4,2,4),(0.,0.0198905179577305,0.0397819072604309),
 .UNSPECIFIED.);
#2032=B_SPLINE_CURVE_WITH_KNOTS('',3,(#87626,#87627,#87628,#87629,#87630,
#87631,#87632),.UNSPECIFIED.,.F.,.F.,(4,3,4),(0.0365944846647008,0.0384615384615384,
0.0431466153076593),.UNSPECIFIED.);
#2033=B_SPLINE_CURVE_WITH_KNOTS('',3,(#87633,#87634,#87635,#87636,#87637,
#87638,#87639,#87640),.UNSPECIFIED.,.F.,.F.,(4,2,2,4),(1.77350726836409E-6,
0.00863675583502219,0.0171409422935184,0.0172810865614791),
 .UNSPECIFIED.);
#2034=B_SPLINE_CURVE_WITH_KNOTS('',3,(#87665,#87666,#87667,#87668,#87669,
#87670),.UNSPECIFIED.,.F.,.F.,(4,2,4),(0.,0.0198536182928153,0.0397081495005046),
 .UNSPECIFIED.);
#2035=B_SPLINE_CURVE_WITH_KNOTS('',3,(#87688,#87689,#87690,#87691,#87692,
#87693),.UNSPECIFIED.,.F.,.F.,(4,2,4),(-0.00212389023527468,-0.00106194259666521,
0.),.UNSPECIFIED.);
#2036=B_SPLINE_CURVE_WITH_KNOTS('',3,(#87694,#87695,#87696,#87697,#87698,
#87699),.UNSPECIFIED.,.F.,.F.,(4,2,4),(9.9999841659296E-7,0.0193527846149201,
0.0387045795187982),.UNSPECIFIED.);
#2037=B_SPLINE_CURVE_WITH_KNOTS('',3,(#87705,#87706,#87707,#87708,#87709,
#87710),.UNSPECIFIED.,.F.,.F.,(4,2,4),(-0.0021248596145857,-0.0010629327539674,
-9.9999999555859E-7),.UNSPECIFIED.);
#2038=B_SPLINE_CURVE_WITH_KNOTS('',3,(#87749,#87750,#87751,#87752,#87753,
#87754),.UNSPECIFIED.,.F.,.F.,(4,2,4),(0.,0.01985833864266,0.0397175617172488),
 .UNSPECIFIED.);
#2039=B_SPLINE_CURVE_WITH_KNOTS('',3,(#87767,#87768,#87769,#87770,#87771,
#87772),.UNSPECIFIED.,.F.,.F.,(4,2,4),(0.,0.0198761966927882,0.0397532849301295),
 .UNSPECIFIED.);
#2040=B_SPLINE_CURVE_WITH_KNOTS('',3,(#87824,#87825,#87826,#87827,#87828,
#87829),.UNSPECIFIED.,.F.,.F.,(4,2,4),(0.,0.0199008240501793,0.0398025405623191),
 .UNSPECIFIED.);
#2041=B_SPLINE_CURVE_WITH_KNOTS('',3,(#87842,#87843,#87844,#87845,#87846,
#87847),.UNSPECIFIED.,.F.,.F.,(4,2,4),(0.,0.0199042047187131,0.0398092891818602),
 .UNSPECIFIED.);
#2042=B_SPLINE_CURVE_WITH_KNOTS('',3,(#87895,#87896,#87897,#87898,#87899,
#87900),.UNSPECIFIED.,.F.,.F.,(4,2,4),(0.,0.0198954793377096,0.0397918614217478),
 .UNSPECIFIED.);
#2043=B_SPLINE_CURVE_WITH_KNOTS('',3,(#87949,#87950,#87951,#87952,#87953,
#87954,#87955),.UNSPECIFIED.,.F.,.F.,(4,3,4),(0.,0.5,0.999990117122682),
 .UNSPECIFIED.);
#2044=B_SPLINE_CURVE_WITH_KNOTS('',3,(#87975,#87976,#87977,#87978,#87979,
#87980),.UNSPECIFIED.,.F.,.F.,(4,2,4),(0.,0.0198677118957237,0.0397363338827323),
 .UNSPECIFIED.);
#2045=B_SPLINE_CURVE_WITH_KNOTS('',3,(#88016,#88017,#88018,#88019,#88020,
#88021),.UNSPECIFIED.,.F.,.F.,(4,2,4),(0.,0.019897396576599,0.0397956842383687),
 .UNSPECIFIED.);
#2046=B_SPLINE_CURVE_WITH_KNOTS('',3,(#88043,#88044,#88045,#88046,#88047,
#88048),.UNSPECIFIED.,.F.,.F.,(4,2,4),(0.,0.0199030679703947,0.0398070346186951),
 .UNSPECIFIED.);
#2047=B_SPLINE_CURVE_WITH_KNOTS('',3,(#88093,#88094,#88095,#88096,#88097,
#88098),.UNSPECIFIED.,.F.,.F.,(4,2,4),(0.,0.0198994178551836,0.0397997367613937),
 .UNSPECIFIED.);
#2048=B_SPLINE_CURVE_WITH_KNOTS('',3,(#88111,#88112,#88113,#88114,#88115,
#88116),.UNSPECIFIED.,.F.,.F.,(4,2,4),(0.,0.0198905179579926,0.0397819072597309),
 .UNSPECIFIED.);
#2049=B_SPLINE_CURVE_WITH_KNOTS('',3,(#88141,#88142,#88143,#88144,#88145,
#88146,#88147),.UNSPECIFIED.,.F.,.F.,(4,3,4),(0.0365944846647007,0.0384615384615384,
0.0431466153076602),.UNSPECIFIED.);
#2050=B_SPLINE_CURVE_WITH_KNOTS('',3,(#88148,#88149,#88150,#88151,#88152,
#88153,#88154,#88155),.UNSPECIFIED.,.F.,.F.,(4,2,2,4),(1.77257431379691E-6,
0.00863675585003615,0.0171409480655562,0.0172810918447234),
 .UNSPECIFIED.);
#2051=B_SPLINE_CURVE_WITH_KNOTS('',3,(#88180,#88181,#88182,#88183,#88184,
#88185),.UNSPECIFIED.,.F.,.F.,(4,2,4),(0.,0.0198536182957362,0.0397081495124057),
 .UNSPECIFIED.);
#2052=B_SPLINE_CURVE_WITH_KNOTS('',3,(#88203,#88204,#88205,#88206,#88207,
#88208),.UNSPECIFIED.,.F.,.F.,(4,2,4),(-0.00212389196723753,-0.00106194329372377,
0.),.UNSPECIFIED.);
#2053=B_SPLINE_CURVE_WITH_KNOTS('',3,(#88209,#88210,#88211,#88212,#88213,
#88214),.UNSPECIFIED.,.F.,.F.,(4,2,4),(9.99998415913432E-7,0.0193532903992515,
0.0387045796335792),.UNSPECIFIED.);
#2054=B_SPLINE_CURVE_WITH_KNOTS('',3,(#88220,#88221,#88222,#88223,#88224,
#88225),.UNSPECIFIED.,.F.,.F.,(4,2,4),(-0.00212485993964147,-0.00106293276514982,
-9.99999999241842E-7),.UNSPECIFIED.);
#2055=B_SPLINE_CURVE_WITH_KNOTS('',3,(#88264,#88265,#88266,#88267,#88268,
#88269),.UNSPECIFIED.,.F.,.F.,(4,2,4),(0.,0.0198583386451148,0.0397175617274757),
 .UNSPECIFIED.);
#2056=B_SPLINE_CURVE_WITH_KNOTS('',3,(#88282,#88283,#88284,#88285,#88286,
#88287),.UNSPECIFIED.,.F.,.F.,(4,2,4),(0.,0.0198761967052751,0.0397532849527076),
 .UNSPECIFIED.);
#2057=B_SPLINE_CURVE_WITH_KNOTS('',3,(#88339,#88340,#88341,#88342,#88343,
#88344),.UNSPECIFIED.,.F.,.F.,(4,2,4),(0.,0.0199008240526954,0.0398025405729508),
 .UNSPECIFIED.);
#2058=B_SPLINE_CURVE_WITH_KNOTS('',3,(#88357,#88358,#88359,#88360,#88361,
#88362),.UNSPECIFIED.,.F.,.F.,(4,2,4),(0.,0.0199042046062945,0.03980928886621),
 .UNSPECIFIED.);
#2059=B_SPLINE_CURVE_WITH_KNOTS('',3,(#88410,#88411,#88412,#88413,#88414,
#88415),.UNSPECIFIED.,.F.,.F.,(4,2,4),(0.,0.0198954793402216,0.0397918614318321),
 .UNSPECIFIED.);
#2060=B_SPLINE_CURVE_WITH_KNOTS('',3,(#88473,#88474,#88475,#88476,#88477,
#88478,#88479),.UNSPECIFIED.,.F.,.F.,(4,3,4),(0.,0.5,0.999990117121439),
 .UNSPECIFIED.);
#2061=B_SPLINE_CURVE_WITH_KNOTS('',3,(#88499,#88500,#88501,#88502,#88503,
#88504),.UNSPECIFIED.,.F.,.F.,(4,2,4),(0.,0.0198677118935691,0.0397363338743666),
 .UNSPECIFIED.);
#2062=B_SPLINE_CURVE_WITH_KNOTS('',3,(#88543,#88544,#88545,#88546,#88547,
#88548),.UNSPECIFIED.,.F.,.F.,(4,2,4),(0.,0.0198973965805586,0.0397956842538152),
 .UNSPECIFIED.);
#2063=B_SPLINE_CURVE_WITH_KNOTS('',3,(#88567,#88568,#88569,#88570,#88571,
#88572),.UNSPECIFIED.,.F.,.F.,(4,2,4),(0.,0.0199030679694276,0.0398070346147848),
 .UNSPECIFIED.);
#2064=B_SPLINE_CURVE_WITH_KNOTS('',3,(#88608,#88609,#88610,#88611,#88612,
#88613),.UNSPECIFIED.,.F.,.F.,(4,2,4),(0.,0.0198994178595983,0.039799736779155),
 .UNSPECIFIED.);
#2065=B_SPLINE_CURVE_WITH_KNOTS('',3,(#88633,#88634,#88635,#88636,#88637,
#88638),.UNSPECIFIED.,.F.,.F.,(4,2,4),(0.,0.0198905727313931,0.0397820346291919),
 .UNSPECIFIED.);
#2066=B_SPLINE_CURVE_WITH_KNOTS('',3,(#88663,#88664,#88665,#88666,#88667,
#88668,#88669),.UNSPECIFIED.,.F.,.F.,(4,3,4),(0.0365944846647009,0.0384615384615384,
0.0431466153076604),.UNSPECIFIED.);
#2067=B_SPLINE_CURVE_WITH_KNOTS('',3,(#88670,#88671,#88672,#88673,#88674,
#88675,#88676,#88677),.UNSPECIFIED.,.F.,.F.,(4,2,2,4),(1.77257444760541E-6,
0.00863675578236859,0.0171409366166497,0.0172810816176936),
 .UNSPECIFIED.);
#2068=B_SPLINE_CURVE_WITH_KNOTS('',3,(#88702,#88703,#88704,#88705,#88706,
#88707),.UNSPECIFIED.,.F.,.F.,(4,2,4),(0.,0.0198536182988451,0.0397081495254481),
 .UNSPECIFIED.);
#2069=B_SPLINE_CURVE_WITH_KNOTS('',3,(#88725,#88726,#88727,#88728,#88729,
#88730),.UNSPECIFIED.,.F.,.F.,(4,2,4),(-0.0021238923472171,-0.00106194344129639,
0.),.UNSPECIFIED.);
#2070=B_SPLINE_CURVE_WITH_KNOTS('',3,(#88731,#88732,#88733,#88734,#88735,
#88736),.UNSPECIFIED.,.F.,.F.,(4,2,4),(9.99998416362877E-7,0.0193527803909816,
0.0387045693995249),.UNSPECIFIED.);
#2071=B_SPLINE_CURVE_WITH_KNOTS('',3,(#88742,#88743,#88744,#88745,#88746,
#88747),.UNSPECIFIED.,.F.,.F.,(4,2,4),(-0.00212486022885731,-0.00106293276487756,
-9.99999998945638E-7),.UNSPECIFIED.);
#2072=B_SPLINE_CURVE_WITH_KNOTS('',3,(#88786,#88787,#88788,#88789,#88790,
#88791),.UNSPECIFIED.,.F.,.F.,(4,2,4),(0.,0.0198583386481131,0.0397175617395592),
 .UNSPECIFIED.);
#2073=B_SPLINE_CURVE_WITH_KNOTS('',3,(#88804,#88805,#88806,#88807,#88808,
#88809),.UNSPECIFIED.,.F.,.F.,(4,2,4),(0.,0.0198761966972832,0.0397532849531587),
 .UNSPECIFIED.);
#2074=B_SPLINE_CURVE_WITH_KNOTS('',3,(#88861,#88862,#88863,#88864,#88865,
#88866),.UNSPECIFIED.,.F.,.F.,(4,2,4),(0.,0.0199008240549723,0.0398025405821787),
 .UNSPECIFIED.);
#2075=B_SPLINE_CURVE_WITH_KNOTS('',3,(#88879,#88880,#88881,#88882,#88883,
#88884),.UNSPECIFIED.,.F.,.F.,(4,2,4),(0.,0.0199042047186047,0.0398092891806177),
 .UNSPECIFIED.);
#2076=B_SPLINE_CURVE_WITH_KNOTS('',3,(#88932,#88933,#88934,#88935,#88936,
#88937),.UNSPECIFIED.,.F.,.F.,(4,2,4),(0.,0.0198954793430153,0.039791861443219),
 .UNSPECIFIED.);
#2077=B_SPLINE_CURVE_WITH_KNOTS('',3,(#89017,#89018,#89019,#89020,#89021,
#89022),.UNSPECIFIED.,.F.,.F.,(4,2,4),(0.,0.0198973965846368,0.0397956842709046),
 .UNSPECIFIED.);
#2078=B_SPLINE_CURVE_WITH_KNOTS('',3,(#89041,#89042,#89043,#89044,#89045,
#89046),.UNSPECIFIED.,.F.,.F.,(4,2,4),(0.,0.01990306796779,0.0398070346084726),
 .UNSPECIFIED.);
#2079=B_SPLINE_CURVE_WITH_KNOTS('',3,(#89088,#89089,#89090,#89091,#89092,
#89093),.UNSPECIFIED.,.F.,.F.,(4,2,4),(0.,0.0198994178631783,0.0397997367937552),
 .UNSPECIFIED.);
#2080=B_SPLINE_CURVE_WITH_KNOTS('',3,(#89103,#89104,#89105,#89106,#89107,
#89108),.UNSPECIFIED.,.F.,.F.,(4,2,4),(0.,0.0198905179573968,0.0397819072752402),
 .UNSPECIFIED.);
#2081=B_SPLINE_CURVE_WITH_KNOTS('',3,(#89128,#89129,#89130,#89131,#89132,
#89133),.UNSPECIFIED.,.F.,.F.,(4,2,4),(0.0365944846647011,0.0384615384615384,
0.0431466153076599),.UNSPECIFIED.);
#2082=B_SPLINE_CURVE_WITH_KNOTS('',3,(#89134,#89135,#89136,#89137,#89138,
#89139,#89140),.UNSPECIFIED.,.F.,.F.,(4,3,4),(0.,0.00863415824051205,0.0172757293265222),
 .UNSPECIFIED.);
#2083=B_SPLINE_CURVE_WITH_KNOTS('',3,(#89165,#89166,#89167,#89168,#89169,
#89170),.UNSPECIFIED.,.F.,.F.,(4,2,4),(0.,0.0198536182040679,0.0397081492848769),
 .UNSPECIFIED.);
#2084=B_SPLINE_CURVE_WITH_KNOTS('',3,(#89183,#89184,#89185,#89186,#89187,
#89188),.UNSPECIFIED.,.F.,.F.,(4,2,4),(-0.00212389330288763,-0.00106194382034054,
0.),.UNSPECIFIED.);
#2085=B_SPLINE_CURVE_WITH_KNOTS('',3,(#89189,#89190,#89191,#89192,#89193,
#89194),.UNSPECIFIED.,.F.,.F.,(4,2,4),(9.99998421535138E-7,0.0193527854095481,
0.0387045795324334),.UNSPECIFIED.);
#2086=B_SPLINE_CURVE_WITH_KNOTS('',3,(#89210,#89211,#89212,#89213,#89214,
#89215,#89216),.UNSPECIFIED.,.F.,.F.,(4,3,4),(0.,0.5,0.999990115097979),
 .UNSPECIFIED.);
#2087=B_SPLINE_CURVE_WITH_KNOTS('',3,(#89236,#89237,#89238,#89239,#89240,
#89241),.UNSPECIFIED.,.F.,.F.,(4,2,4),(0.,0.0198677117286434,0.0397363336110727),
 .UNSPECIFIED.);
#2088=B_SPLINE_CURVE_WITH_KNOTS('',3,(#89247,#89248,#89249,#89250,#89251,
#89252),.UNSPECIFIED.,.F.,.F.,(4,2,4),(-0.00212486061334155,-0.00106293276465332,
-9.99999994678421E-7),.UNSPECIFIED.);
#2089=B_SPLINE_CURVE_WITH_KNOTS('',3,(#89291,#89292,#89293,#89294,#89295,
#89296),.UNSPECIFIED.,.F.,.F.,(4,2,4),(0.,0.0198583386511999,0.0397175617526615),
 .UNSPECIFIED.);
#2090=B_SPLINE_CURVE_WITH_KNOTS('',3,(#89309,#89310,#89311,#89312,#89313,
#89314),.UNSPECIFIED.,.F.,.F.,(4,2,4),(0.,0.0198761967019296,0.0397532849637006),
 .UNSPECIFIED.);
#2091=B_SPLINE_CURVE_WITH_KNOTS('',3,(#89366,#89367,#89368,#89369,#89370,
#89371),.UNSPECIFIED.,.F.,.F.,(4,2,4),(0.,0.0199008240588883,0.0398025405977883),
 .UNSPECIFIED.);
#2092=B_SPLINE_CURVE_WITH_KNOTS('',3,(#89384,#89385,#89386,#89387,#89388,
#89389),.UNSPECIFIED.,.F.,.F.,(4,2,4),(0.,0.0199042046965285,0.039809289131505),
 .UNSPECIFIED.);
#2093=B_SPLINE_CURVE_WITH_KNOTS('',3,(#89437,#89438,#89439,#89440,#89441,
#89442),.UNSPECIFIED.,.F.,.F.,(4,2,4),(0.,0.0198954793465745,0.0397918614572659),
 .UNSPECIFIED.);
#2094=B_SPLINE_CURVE_WITH_KNOTS('',3,(#89484,#89485,#89486,#89487,#89488,
#89489),.UNSPECIFIED.,.F.,.F.,(4,2,4),(-0.00212486106831169,-0.00106293275660098,
-9.99999994408878E-7),.UNSPECIFIED.);
#2095=B_SPLINE_CURVE_WITH_KNOTS('',3,(#89491,#89492,#89493,#89494,#89495,
#89496),.UNSPECIFIED.,.F.,.F.,(4,2,4),(-0.00212389479901396,-0.00106194442085412,
0.),.UNSPECIFIED.);
#2096=B_SPLINE_CURVE_WITH_KNOTS('',3,(#89541,#89542,#89543,#89544,#89545,
#89546),.UNSPECIFIED.,.F.,.F.,(4,2,4),(0.,0.0198994178670901,0.0397997368094576),
 .UNSPECIFIED.);
#2097=B_SPLINE_CURVE_WITH_KNOTS('',3,(#89563,#89564,#89565,#89566,#89567,
#89568),.UNSPECIFIED.,.F.,.F.,(4,2,4),(0.,0.0198905727281448,0.0397820346162575),
 .UNSPECIFIED.);
#2098=B_SPLINE_CURVE_WITH_KNOTS('',3,(#89592,#89593,#89594,#89595,#89596,
#89597,#89598),.UNSPECIFIED.,.F.,.F.,(4,3,4),(0.036594484664701,0.0384615384615384,
0.0431466153076596),.UNSPECIFIED.);
#2099=B_SPLINE_CURVE_WITH_KNOTS('',3,(#89599,#89600,#89601,#89602,#89603,
#89604,#89605,#89606),.UNSPECIFIED.,.F.,.F.,(4,2,2,4),(1.7725797502064E-6,
0.00863675584056385,0.0171399056837115,0.0172810927018386),
 .UNSPECIFIED.);
#2100=B_SPLINE_CURVE_WITH_KNOTS('',3,(#89631,#89632,#89633,#89634,#89635,
#89636),.UNSPECIFIED.,.F.,.F.,(4,2,4),(0.,0.0198536183073532,0.0397081495597498),
 .UNSPECIFIED.);
#2101=B_SPLINE_CURVE_WITH_KNOTS('',3,(#89652,#89653,#89654,#89655,#89656,
#89657),.UNSPECIFIED.,.F.,.F.,(4,2,4),(9.99998420096059E-7,0.0193522753886915,
0.0387045692994476),.UNSPECIFIED.);
#2102=B_SPLINE_CURVE_WITH_KNOTS('',3,(#89693,#89694,#89695,#89696,#89697,
#89698),.UNSPECIFIED.,.F.,.F.,(4,2,4),(0.,0.019858338655085,0.0397175617676976),
 .UNSPECIFIED.);
#2103=B_SPLINE_CURVE_WITH_KNOTS('',3,(#89718,#89719,#89720,#89721,#89722,
#89723),.UNSPECIFIED.,.F.,.F.,(4,2,4),(0.,0.0198762583335164,0.0397534249341096),
 .UNSPECIFIED.);
#2104=B_SPLINE_CURVE_WITH_KNOTS('',3,(#89739,#89740,#89741,#89742,#89743,
#89744,#89745),.UNSPECIFIED.,.F.,.F.,(4,3,4),(0.,0.5,0.999990115106081),
 .UNSPECIFIED.);
#2105=B_SPLINE_CURVE_WITH_KNOTS('',3,(#89765,#89766,#89767,#89768,#89769,
#89770),.UNSPECIFIED.,.F.,.F.,(4,2,4),(0.,0.0198677117239206,0.0397363335921476),
 .UNSPECIFIED.);
#2106=B_SPLINE_CURVE_WITH_KNOTS('',3,(#89812,#89813,#89814,#89815,#89816,
#89817),.UNSPECIFIED.,.F.,.F.,(4,2,4),(0.,0.0198973965928252,0.0397956843034983),
 .UNSPECIFIED.);
#2107=B_SPLINE_CURVE_WITH_KNOTS('',3,(#89836,#89837,#89838,#89839,#89840,
#89841),.UNSPECIFIED.,.F.,.F.,(4,2,4),(0.,0.0199030679705157,0.0398070346190355),
 .UNSPECIFIED.);
#2108=B_SPLINE_CURVE_WITH_KNOTS('',3,(#89893,#89894,#89895,#89896,#89897,
#89898),.UNSPECIFIED.,.F.,.F.,(4,2,4),(0.,0.0199008240622871,0.0398025406117409),
 .UNSPECIFIED.);
#2109=B_SPLINE_CURVE_WITH_KNOTS('',3,(#89911,#89912,#89913,#89914,#89915,
#89916),.UNSPECIFIED.,.F.,.F.,(4,2,4),(0.,0.0199042047128084,0.0398092891706494),
 .UNSPECIFIED.);
#2110=B_SPLINE_CURVE_WITH_KNOTS('',3,(#89964,#89965,#89966,#89967,#89968,
#89969),.UNSPECIFIED.,.F.,.F.,(4,2,4),(0.,0.0198954793500795,0.0397918614720059),
 .UNSPECIFIED.);
#2111=B_SPLINE_CURVE_WITH_KNOTS('',3,(#90029,#90030,#90031,#90032,#90033,
#90034),.UNSPECIFIED.,.F.,.F.,(4,2,4),(-0.00212486151725449,-0.00106293276451091,
-9.99999995882767E-7),.UNSPECIFIED.);
#2112=B_SPLINE_CURVE_WITH_KNOTS('',3,(#90036,#90037,#90038,#90039,#90040,
#90041),.UNSPECIFIED.,.F.,.F.,(4,2,4),(-0.00212389433155121,-0.00106194422672578,
0.),.UNSPECIFIED.);
#2113=B_SPLINE_CURVE_WITH_KNOTS('',3,(#90061,#90062,#90063,#90064,#90065,
#90066),.UNSPECIFIED.,.F.,.F.,(4,2,4),(0.0365944846647011,0.0384615384615384,
0.0431466153076599),.UNSPECIFIED.);
#2114=B_SPLINE_CURVE_WITH_KNOTS('',3,(#90067,#90068,#90069,#90070,#90071,
#90072,#90073),.UNSPECIFIED.,.F.,.F.,(4,3,4),(0.,0.00863415823997989,0.0172757326529418),
 .UNSPECIFIED.);
#2115=B_SPLINE_CURVE_WITH_KNOTS('',3,(#90098,#90099,#90100,#90101,#90102,
#90103),.UNSPECIFIED.,.F.,.F.,(4,2,4),(0.,0.0198541182711426,0.039708149503461),
 .UNSPECIFIED.);
#2116=B_SPLINE_CURVE_WITH_KNOTS('',3,(#90114,#90115,#90116,#90117,#90118,
#90119),.UNSPECIFIED.,.F.,.F.,(4,2,4),(9.9999842080534E-7,0.0193527904135635,
0.0387045796346496),.UNSPECIFIED.);
#2117=B_SPLINE_CURVE_WITH_KNOTS('',3,(#90161,#90162,#90163,#90164,#90165,
#90166),.UNSPECIFIED.,.F.,.F.,(4,2,4),(0.,0.0198583386593065,0.0397175617852667),
 .UNSPECIFIED.);
#2118=B_SPLINE_CURVE_WITH_KNOTS('',3,(#90176,#90177,#90178,#90179,#90180,
#90181),.UNSPECIFIED.,.F.,.F.,(4,2,4),(0.,0.0198761967046,0.0397532849569533),
 .UNSPECIFIED.);
#2119=B_SPLINE_CURVE_WITH_KNOTS('',3,(#90227,#90228,#90229,#90230,#90231,
#90232),.UNSPECIFIED.,.F.,.F.,(4,2,4),(0.,0.0199008240664257,0.0398025406285198),
 .UNSPECIFIED.);
#2120=B_SPLINE_CURVE_WITH_KNOTS('',3,(#90252,#90253,#90254,#90255,#90256,
#90257),.UNSPECIFIED.,.F.,.F.,(4,2,4),(0.,0.0199042621650074,0.0398094213886953),
 .UNSPECIFIED.);
#2121=B_SPLINE_CURVE_WITH_KNOTS('',3,(#90280,#90281,#90282,#90283,#90284,
#90285,#90286),.UNSPECIFIED.,.F.,.F.,(4,3,4),(0.,0.5,0.999990117119127),
 .UNSPECIFIED.);
#2122=B_SPLINE_CURVE_WITH_KNOTS('',3,(#90299,#90300,#90301,#90302,#90303,
#90304),.UNSPECIFIED.,.F.,.F.,(4,2,4),(0.,0.0198676496451984,0.0397361927455519),
 .UNSPECIFIED.);
#2123=B_SPLINE_CURVE_WITH_KNOTS('',3,(#90346,#90347,#90348,#90349,#90350,
#90351),.UNSPECIFIED.,.F.,.F.,(4,2,4),(0.,0.0198973965961517,0.0397956843169669),
 .UNSPECIFIED.);
#2124=B_SPLINE_CURVE_WITH_KNOTS('',3,(#90370,#90371,#90372,#90373,#90374,
#90375),.UNSPECIFIED.,.F.,.F.,(4,2,4),(0.,0.019903067966377,0.0398070346026983),
 .UNSPECIFIED.);
#2125=B_SPLINE_CURVE_WITH_KNOTS('',3,(#90417,#90418,#90419,#90420,#90421,
#90422),.UNSPECIFIED.,.F.,.F.,(4,2,4),(0.,0.0198994178758511,0.039799736844854),
 .UNSPECIFIED.);
#2126=B_SPLINE_CURVE_WITH_KNOTS('',3,(#90432,#90433,#90434,#90435,#90436,
#90437),.UNSPECIFIED.,.F.,.F.,(4,2,4),(0.,0.0198905179572641,0.0397819072592456),
 .UNSPECIFIED.);
#2127=B_SPLINE_CURVE_WITH_KNOTS('',3,(#90485,#90486,#90487,#90488,#90489,
#90490),.UNSPECIFIED.,.F.,.F.,(4,2,4),(0.,0.0198954793536976,0.0397918614864844),
 .UNSPECIFIED.);
#2128=B_SPLINE_CURVE_WITH_KNOTS('',3,(#90523,#90524,#90525,#90526,#90527,
#90528),.UNSPECIFIED.,.F.,.F.,(4,2,4),(-0.00212486217399669,-0.0010629327504893,
-9.99999997006E-7),.UNSPECIFIED.);
#2129=B_SPLINE_CURVE_WITH_KNOTS('',3,(#90530,#90531,#90532,#90533,#90534,
#90535),.UNSPECIFIED.,.F.,.F.,(4,2,4),(-0.00212389488246331,-0.00106194445546336,
0.),.UNSPECIFIED.);
#2130=B_SPLINE_CURVE_WITH_KNOTS('',3,(#90606,#90607,#90608,#90609,#90610,
#90611),.UNSPECIFIED.,.F.,.F.,(4,2,4),(0.,0.0198583386615053,0.0397175617941277),
 .UNSPECIFIED.);
#2131=B_SPLINE_CURVE_WITH_KNOTS('',3,(#90628,#90629,#90630,#90631,#90632,
#90633),.UNSPECIFIED.,.F.,.F.,(4,2,4),(0.,0.019876258198031,0.0397534246582595),
 .UNSPECIFIED.);
#2132=B_SPLINE_CURVE_WITH_KNOTS('',3,(#90674,#90675,#90676,#90677,#90678,
#90679),.UNSPECIFIED.,.F.,.F.,(4,2,4),(0.,0.0199013242067181,0.0398025408594927),
 .UNSPECIFIED.);
#2133=B_SPLINE_CURVE_WITH_KNOTS('',3,(#90689,#90690,#90691,#90692,#90693,
#90694),.UNSPECIFIED.,.F.,.F.,(4,2,4),(0.,0.019904704836476,0.0398092893406518),
 .UNSPECIFIED.);
#2134=B_SPLINE_CURVE_WITH_KNOTS('',3,(#90733,#90734,#90735,#90736,#90737,
#90738),.UNSPECIFIED.,.F.,.F.,(4,2,4),(0.,0.0198954793582144,0.0397918615045159),
 .UNSPECIFIED.);
#2135=B_SPLINE_CURVE_WITH_KNOTS('',3,(#90771,#90772,#90773,#90774,#90775,
#90776,#90777),.UNSPECIFIED.,.F.,.F.,(4,3,4),(0.,0.5,0.999990115106096),
 .UNSPECIFIED.);
#2136=B_SPLINE_CURVE_WITH_KNOTS('',3,(#90789,#90790,#90791,#90792,#90793,
#90794),.UNSPECIFIED.,.F.,.F.,(4,2,4),(0.,0.0198676494907608,0.0397361925123579),
 .UNSPECIFIED.);
#2137=B_SPLINE_CURVE_WITH_KNOTS('',3,(#90832,#90833,#90834,#90835,#90836,
#90837),.UNSPECIFIED.,.F.,.F.,(4,2,4),(0.,0.0198973965979104,0.0397956843240261),
 .UNSPECIFIED.);
#2138=B_SPLINE_CURVE_WITH_KNOTS('',3,(#90849,#90850,#90851,#90852,#90853,
#90854),.UNSPECIFIED.,.F.,.F.,(4,2,4),(0.,0.0199030098322562,0.0398069010987286),
 .UNSPECIFIED.);
#2139=B_SPLINE_CURVE_WITH_KNOTS('',3,(#90895,#90896,#90897,#90898,#90899,
#90900),.UNSPECIFIED.,.F.,.F.,(4,2,4),(0.,0.0198994178785925,0.0397997368562008),
 .UNSPECIFIED.);
#2140=B_SPLINE_CURVE_WITH_KNOTS('',3,(#90910,#90911,#90912,#90913,#90914,
#90915),.UNSPECIFIED.,.F.,.F.,(4,2,4),(0.,0.0198905179570912,0.0397819072622904),
 .UNSPECIFIED.);
#2141=B_SPLINE_CURVE_WITH_KNOTS('',3,(#90939,#90940,#90941,#90942,#90943,
#90944,#90945),.UNSPECIFIED.,.F.,.F.,(4,3,4),(0.0365944846647076,0.0384615384615384,
0.043146615307659),.UNSPECIFIED.);
#2142=B_SPLINE_CURVE_WITH_KNOTS('',3,(#90946,#90947,#90948,#90949,#90950,
#90951,#90952,#90953),.UNSPECIFIED.,.F.,.F.,(4,2,2,4),(1.77350714240743E-6,
0.00863675589070899,0.0171399223480672,0.0172811074735198),
 .UNSPECIFIED.);
#2143=B_SPLINE_CURVE_WITH_KNOTS('',3,(#90977,#90978,#90979,#90980,#90981,
#90982),.UNSPECIFIED.,.F.,.F.,(4,2,4),(0.,0.0198536183202665,0.0397081496113208),
 .UNSPECIFIED.);
#2144=B_SPLINE_CURVE_WITH_KNOTS('',3,(#90998,#90999,#91000,#91001,#91002,
#91003),.UNSPECIFIED.,.F.,.F.,(4,2,4),(9.99998420192272E-7,0.0193527896174958,
0.0387045796181448),.UNSPECIFIED.);
#2145=B_SPLINE_CURVE_WITH_KNOTS('',3,(#91233,#91234,#91235,#91236),
 .UNSPECIFIED.,.F.,.F.,(4,4),(3.44076343139105E-7,9.58822346085573E-5),
 .UNSPECIFIED.);
#2146=B_SPLINE_CURVE_WITH_KNOTS('',3,(#91329,#91330,#91331,#91332),
 .UNSPECIFIED.,.F.,.F.,(4,4),(3.44076343937661E-7,9.58822346085479E-5),
 .UNSPECIFIED.);
#2147=B_SPLINE_CURVE_WITH_KNOTS('',3,(#91633,#91634,#91635,#91636),
 .UNSPECIFIED.,.F.,.F.,(4,4),(3.44076344756528E-7,9.58822346085586E-5),
 .UNSPECIFIED.);
#2148=B_SPLINE_CURVE_WITH_KNOTS('',3,(#91937,#91938,#91939,#91940),
 .UNSPECIFIED.,.F.,.F.,(4,4),(3.44076345613438E-7,9.5882234608549E-5),
 .UNSPECIFIED.);
#2149=B_SPLINE_CURVE_WITH_KNOTS('',3,(#92241,#92242,#92243,#92244),
 .UNSPECIFIED.,.F.,.F.,(4,4),(3.44076346610602E-7,9.5882234608586E-5),
 .UNSPECIFIED.);
#2150=B_SPLINE_CURVE_WITH_KNOTS('',3,(#92545,#92546,#92547,#92548),
 .UNSPECIFIED.,.F.,.F.,(4,4),(3.44076347442387E-7,9.58822346085427E-5),
 .UNSPECIFIED.);
#2151=B_SPLINE_CURVE_WITH_KNOTS('',3,(#92849,#92850,#92851,#92852),
 .UNSPECIFIED.,.F.,.F.,(4,4),(3.4407634849255E-7,9.58822346085551E-5),
 .UNSPECIFIED.);
#2152=B_SPLINE_CURVE_WITH_KNOTS('',3,(#93153,#93154,#93155,#93156),
 .UNSPECIFIED.,.F.,.F.,(4,4),(3.44076349385464E-7,9.58822346085304E-5),
 .UNSPECIFIED.);
#2153=B_SPLINE_CURVE_WITH_KNOTS('',3,(#93457,#93458,#93459,#93460),
 .UNSPECIFIED.,.F.,.F.,(4,4),(3.44076350325311E-7,9.5882234608509E-5),
 .UNSPECIFIED.);
#2154=B_SPLINE_CURVE_WITH_KNOTS('',3,(#93761,#93762,#93763,#93764),
 .UNSPECIFIED.,.F.,.F.,(4,4),(3.44076351419414E-7,9.58822346086072E-5),
 .UNSPECIFIED.);
#2155=B_SPLINE_CURVE_WITH_KNOTS('',3,(#94065,#94066,#94067,#94068),
 .UNSPECIFIED.,.F.,.F.,(4,4),(3.44076352242797E-7,9.58822346085252E-5),
 .UNSPECIFIED.);
#2156=B_SPLINE_CURVE_WITH_KNOTS('',3,(#94369,#94370,#94371,#94372),
 .UNSPECIFIED.,.F.,.F.,(4,4),(3.44076353092136E-7,9.58822346085853E-5),
 .UNSPECIFIED.);
#2157=B_SPLINE_CURVE_WITH_KNOTS('',3,(#94673,#94674,#94675,#94676),
 .UNSPECIFIED.,.F.,.F.,(4,4),(3.44076353913147E-7,9.58822346085855E-5),
 .UNSPECIFIED.);
#2158=B_SPLINE_CURVE_WITH_KNOTS('',3,(#94977,#94978,#94979,#94980),
 .UNSPECIFIED.,.F.,.F.,(4,4),(3.44076354603741E-7,9.58822346086191E-5),
 .UNSPECIFIED.);
#2159=B_SPLINE_CURVE_WITH_KNOTS('',3,(#95281,#95282,#95283,#95284),
 .UNSPECIFIED.,.F.,.F.,(4,4),(3.440763552087E-7,9.58822346085434E-5),
 .UNSPECIFIED.);
#2160=B_SPLINE_CURVE_WITH_KNOTS('',3,(#95585,#95586,#95587,#95588),
 .UNSPECIFIED.,.F.,.F.,(4,4),(3.44076355662546E-7,9.5882234608571E-5),
 .UNSPECIFIED.);
#2161=B_SPLINE_CURVE_WITH_KNOTS('',3,(#95889,#95890,#95891,#95892),
 .UNSPECIFIED.,.F.,.F.,(4,4),(3.44076356005326E-7,9.58822346085531E-5),
 .UNSPECIFIED.);
#2162=B_SPLINE_CURVE_WITH_KNOTS('',3,(#96193,#96194,#96195,#96196),
 .UNSPECIFIED.,.F.,.F.,(4,4),(3.44076356300518E-7,9.58822346085333E-5),
 .UNSPECIFIED.);
#2163=B_SPLINE_CURVE_WITH_KNOTS('',3,(#96497,#96498,#96499,#96500),
 .UNSPECIFIED.,.F.,.F.,(4,4),(3.44076356438746E-7,9.58822346085612E-5),
 .UNSPECIFIED.);
#2164=B_SPLINE_CURVE_WITH_KNOTS('',3,(#96801,#96802,#96803,#96804),
 .UNSPECIFIED.,.F.,.F.,(4,4),(3.44076356391263E-7,9.58822346085676E-5),
 .UNSPECIFIED.);
#2165=B_SPLINE_CURVE_WITH_KNOTS('',3,(#97105,#97106,#97107,#97108),
 .UNSPECIFIED.,.F.,.F.,(4,4),(3.44076356413286E-7,9.58822346085746E-5),
 .UNSPECIFIED.);
#2166=B_SPLINE_CURVE_WITH_KNOTS('',3,(#97409,#97410,#97411,#97412),
 .UNSPECIFIED.,.F.,.F.,(4,4),(3.44076356099639E-7,9.58822346086219E-5),
 .UNSPECIFIED.);
#2167=B_SPLINE_CURVE_WITH_KNOTS('',3,(#97713,#97714,#97715,#97716),
 .UNSPECIFIED.,.F.,.F.,(4,4),(3.44076355765E-7,9.58822346085517E-5),
 .UNSPECIFIED.);
#2168=B_SPLINE_CURVE_WITH_KNOTS('',3,(#98017,#98018,#98019,#98020),
 .UNSPECIFIED.,.F.,.F.,(4,4),(3.44076355331457E-7,9.58822346085816E-5),
 .UNSPECIFIED.);
#2169=B_SPLINE_CURVE_WITH_KNOTS('',3,(#98321,#98322,#98323,#98324),
 .UNSPECIFIED.,.F.,.F.,(4,4),(3.44076354721354E-7,9.58822346085665E-5),
 .UNSPECIFIED.);
#2170=B_SPLINE_CURVE_WITH_KNOTS('',3,(#98625,#98626,#98627,#98628),
 .UNSPECIFIED.,.F.,.F.,(4,4),(3.44076354108817E-7,9.5882234608515E-5),
 .UNSPECIFIED.);
#2171=B_SPLINE_CURVE_WITH_KNOTS('',3,(#98929,#98930,#98931,#98932),
 .UNSPECIFIED.,.F.,.F.,(4,4),(3.44076353460809E-7,9.58822346085927E-5),
 .UNSPECIFIED.);
#2172=B_SPLINE_CURVE_WITH_KNOTS('',3,(#99233,#99234,#99235,#99236),
 .UNSPECIFIED.,.F.,.F.,(4,4),(3.44076352635546E-7,9.58822346085778E-5),
 .UNSPECIFIED.);
#2173=B_SPLINE_CURVE_WITH_KNOTS('',3,(#99537,#99538,#99539,#99540),
 .UNSPECIFIED.,.F.,.F.,(4,4),(3.44076351743482E-7,9.58822346085721E-5),
 .UNSPECIFIED.);
#2174=B_SPLINE_CURVE_WITH_KNOTS('',3,(#99841,#99842,#99843,#99844),
 .UNSPECIFIED.,.F.,.F.,(4,4),(3.44076350748374E-7,9.58822346085306E-5),
 .UNSPECIFIED.);
#2175=B_SPLINE_CURVE_WITH_KNOTS('',3,(#100145,#100146,#100147,#100148),
 .UNSPECIFIED.,.F.,.F.,(4,4),(3.44076349811527E-7,9.58822346085378E-5),
 .UNSPECIFIED.);
#2176=B_SPLINE_CURVE_WITH_KNOTS('',3,(#100449,#100450,#100451,#100452),
 .UNSPECIFIED.,.F.,.F.,(4,4),(3.44076348755265E-7,9.58822346085592E-5),
 .UNSPECIFIED.);
#2177=B_SPLINE_CURVE_WITH_KNOTS('',3,(#100753,#100754,#100755,#100756),
 .UNSPECIFIED.,.F.,.F.,(4,4),(3.44076347719767E-7,9.58822346085908E-5),
 .UNSPECIFIED.);
#2178=B_SPLINE_CURVE_WITH_KNOTS('',3,(#101057,#101058,#101059,#101060),
 .UNSPECIFIED.,.F.,.F.,(4,4),(3.44076346912447E-7,9.588223460854E-5),
 .UNSPECIFIED.);
#2179=B_SPLINE_CURVE_WITH_KNOTS('',3,(#101361,#101362,#101363,#101364),
 .UNSPECIFIED.,.F.,.F.,(4,4),(3.44076345873186E-7,9.58822346084459E-5),
 .UNSPECIFIED.);
#2180=B_SPLINE_CURVE_WITH_KNOTS('',3,(#101665,#101666,#101667,#101668),
 .UNSPECIFIED.,.F.,.F.,(4,4),(3.44076345035861E-7,9.58822346085724E-5),
 .UNSPECIFIED.);
#2181=B_SPLINE_CURVE_WITH_KNOTS('',3,(#101969,#101970,#101971,#101972),
 .UNSPECIFIED.,.F.,.F.,(4,4),(3.4407634418853E-7,9.58822346084491E-5),
 .UNSPECIFIED.);
#2182=B_SPLINE_CURVE_WITH_KNOTS('',3,(#102273,#102274,#102275,#102276),
 .UNSPECIFIED.,.F.,.F.,(4,4),(3.44076343458719E-7,9.58822346085829E-5),
 .UNSPECIFIED.);
#2183=B_SPLINE_CURVE_WITH_KNOTS('',3,(#102577,#102578,#102579,#102580),
 .UNSPECIFIED.,.F.,.F.,(4,4),(3.4407634265707E-7,9.58822346085594E-5),
 .UNSPECIFIED.);
#2184=B_SPLINE_CURVE_WITH_KNOTS('',3,(#102881,#102882,#102883,#102884),
 .UNSPECIFIED.,.F.,.F.,(4,4),(3.44076342139102E-7,9.5882234608581E-5),
 .UNSPECIFIED.);
#2185=B_SPLINE_CURVE_WITH_KNOTS('',3,(#103185,#103186,#103187,#103188),
 .UNSPECIFIED.,.F.,.F.,(4,4),(3.44076341609194E-7,9.58822346085673E-5),
 .UNSPECIFIED.);
#2186=B_SPLINE_CURVE_WITH_KNOTS('',3,(#103489,#103490,#103491,#103492),
 .UNSPECIFIED.,.F.,.F.,(4,4),(3.44076341299288E-7,9.58822346085517E-5),
 .UNSPECIFIED.);
#2187=B_SPLINE_CURVE_WITH_KNOTS('',3,(#103793,#103794,#103795,#103796),
 .UNSPECIFIED.,.F.,.F.,(4,4),(3.44076341018736E-7,9.5882234608553E-5),
 .UNSPECIFIED.);
#2188=B_SPLINE_CURVE_WITH_KNOTS('',3,(#104137,#104138,#104139,#104140),
 .UNSPECIFIED.,.F.,.F.,(4,4),(3.44076340792074E-7,9.58822346085118E-5),
 .UNSPECIFIED.);
#2189=B_SPLINE_CURVE_WITH_KNOTS('',3,(#104401,#104402,#104403,#104404),
 .UNSPECIFIED.,.F.,.F.,(4,4),(3.44076340724659E-7,9.58822346085855E-5),
 .UNSPECIFIED.);
#2190=B_SPLINE_CURVE_WITH_KNOTS('',3,(#104705,#104706,#104707,#104708),
 .UNSPECIFIED.,.F.,.F.,(4,4),(3.44076340891315E-7,9.58822346085796E-5),
 .UNSPECIFIED.);
#2191=B_SPLINE_CURVE_WITH_KNOTS('',3,(#105009,#105010,#105011,#105012),
 .UNSPECIFIED.,.F.,.F.,(4,4),(3.4407634120523E-7,9.5882234608577E-5),
 .UNSPECIFIED.);
#2192=B_SPLINE_CURVE_WITH_KNOTS('',3,(#105313,#105314,#105315,#105316),
 .UNSPECIFIED.,.F.,.F.,(4,4),(3.44076341566053E-7,9.5882234608583E-5),
 .UNSPECIFIED.);
#2193=B_SPLINE_CURVE_WITH_KNOTS('',3,(#105617,#105618,#105619,#105620),
 .UNSPECIFIED.,.F.,.F.,(4,4),(3.44076341947078E-7,9.58822346086343E-5),
 .UNSPECIFIED.);
#2194=B_SPLINE_CURVE_WITH_KNOTS('',3,(#105921,#105922,#105923,#105924),
 .UNSPECIFIED.,.F.,.F.,(4,4),(3.44076342475543E-7,9.58822346086365E-5),
 .UNSPECIFIED.);
#2199=B_SPLINE_SURFACE_WITH_KNOTS('',3,3,((#65202,#65203,#65204,#65205),
(#65206,#65207,#65208,#65209),(#65210,#65211,#65212,#65213),(#65214,#65215,
#65216,#65217)),.UNSPECIFIED.,.F.,.F.,.F.,(4,4),(4,4),(-0.000171895435141639,
1.00600020634823),(0.0665898698856052,0.0751325481130375),.UNSPECIFIED.);
#2200=B_SPLINE_SURFACE_WITH_KNOTS('',3,3,((#65233,#65234,#65235,#65236),
(#65237,#65238,#65239,#65240),(#65241,#65242,#65243,#65244),(#65245,#65246,
#65247,#65248)),.UNSPECIFIED.,.F.,.F.,.F.,(4,4),(4,4),(-0.00286833998603604,
0.477902879809884),(0.0665898698862512,0.0731716198748498),
 .UNSPECIFIED.);
#2201=B_SPLINE_SURFACE_WITH_KNOTS('',3,3,((#65300,#65301,#65302,#65303),
(#65304,#65305,#65306,#65307),(#65308,#65309,#65310,#65311),(#65312,#65313,
#65314,#65315)),.UNSPECIFIED.,.F.,.F.,.F.,(4,4),(4,4),(-0.00286764392048215,
0.477902879806999),(0.0565997133101203,0.0631721430887071),
 .UNSPECIFIED.);
#2202=B_SPLINE_SURFACE_WITH_KNOTS('',3,3,((#65326,#65327,#65328,#65329),
(#65330,#65331,#65332,#65333),(#65334,#65335,#65336,#65337),(#65338,#65339,
#65340,#65341)),.UNSPECIFIED.,.F.,.F.,.F.,(4,4),(4,4),(-0.00286833998604881,
0.477902879811004),(0.0665898698862518,0.0731716198748491),
 .UNSPECIFIED.);
#2203=B_SPLINE_SURFACE_WITH_KNOTS('',3,3,((#65358,#65359,#65360,#65361),
(#65362,#65363,#65364,#65365),(#65366,#65367,#65368,#65369),(#65370,#65371,
#65372,#65373)),.UNSPECIFIED.,.F.,.F.,.F.,(4,4),(4,4),(0.522097120207134,
1.00286791825535),(0.0600156865486949,0.0665898700060146),.UNSPECIFIED.);
#2204=B_SPLINE_SURFACE_WITH_KNOTS('',3,3,((#65436,#65437,#65438,#65439),
(#65440,#65441,#65442,#65443),(#65444,#65445,#65446,#65447),(#65448,#65449,
#65450,#65451)),.UNSPECIFIED.,.F.,.F.,.F.,(4,4),(4,4),(0.52209712020793,
1.00286780122186),(0.050026355085867,0.056599713310142),.UNSPECIFIED.);
#2205=B_SPLINE_SURFACE_WITH_KNOTS('',3,3,((#65459,#65460,#65461,#65462),
(#65463,#65464,#65465,#65466),(#65467,#65468,#65469,#65470),(#65471,#65472,
#65473,#65474)),.UNSPECIFIED.,.F.,.F.,.F.,(4,4),(4,4),(0.522097120207881,
1.0028679182553),(0.0600156865486941,0.0665898700060137),.UNSPECIFIED.);
#2206=B_SPLINE_SURFACE_WITH_KNOTS('',3,3,((#65589,#65590,#65591,#65592),
(#65593,#65594,#65595,#65596),(#65597,#65598,#65599,#65600),(#65601,#65602,
#65603,#65604)),.UNSPECIFIED.,.F.,.F.,.F.,(4,4),(4,4),(0.522097120205934,
1.00286848452567),(0.0400218729465712,0.0466073985929453),.UNSPECIFIED.);
#2207=B_SPLINE_SURFACE_WITH_KNOTS('',3,3,((#65612,#65613,#65614,#65615),
(#65616,#65617,#65618,#65619),(#65620,#65621,#65622,#65623),(#65624,#65625,
#65626,#65627)),.UNSPECIFIED.,.F.,.F.,.F.,(4,4),(4,4),(0.522097120207841,
1.0028678012217),(0.0500263550858681,0.0565997133101407),.UNSPECIFIED.);
#2208=B_SPLINE_SURFACE_WITH_KNOTS('',3,3,((#65758,#65759,#65760,#65761),
(#65762,#65763,#65764,#65765),(#65766,#65767,#65768,#65769),(#65770,#65771,
#65772,#65773)),.UNSPECIFIED.,.F.,.F.,.F.,(4,4),(4,4),(0.52209712020777,
1.0028686220115),(0.0300094532292152,0.0365944846647039),.UNSPECIFIED.);
#2209=B_SPLINE_SURFACE_WITH_KNOTS('',3,3,((#65781,#65782,#65783,#65784),
(#65785,#65786,#65787,#65788),(#65789,#65790,#65791,#65792),(#65793,#65794,
#65795,#65796)),.UNSPECIFIED.,.F.,.F.,.F.,(4,4),(4,4),(0.522097120207815,
1.00286848452581),(0.0400218729465705,0.0466073985929441),.UNSPECIFIED.);
#2210=B_SPLINE_SURFACE_WITH_KNOTS('',3,3,((#65804,#65805,#65806,#65807),
(#65808,#65809,#65810,#65811),(#65812,#65813,#65814,#65815),(#65816,#65817,
#65818,#65819)),.UNSPECIFIED.,.F.,.F.,.F.,(4,4),(4,4),(-0.00286823045918448,
0.477902879812007),(0.0265907346180622,0.0331702036774535),
 .UNSPECIFIED.);
#2211=B_SPLINE_SURFACE_WITH_KNOTS('',3,3,((#65872,#65873,#65874,#65875),
(#65876,#65877,#65878,#65879),(#65880,#65881,#65882,#65883),(#65884,#65885,
#65886,#65887)),.UNSPECIFIED.,.F.,.F.,.F.,(4,4),(4,4),(-0.00600003960325622,
1.),(0.0166015299238292,0.0265907346494256),.UNSPECIFIED.);
#2212=B_SPLINE_SURFACE_WITH_KNOTS('',3,3,((#65920,#65921,#65922,#65923),
(#65924,#65925,#65926,#65927),(#65928,#65929,#65930,#65931),(#65932,#65933,
#65934,#65935)),.UNSPECIFIED.,.F.,.F.,.F.,(4,4),(4,4),(0.522097120207639,
1.00286780293604),(0.0200175229645447,0.0265907346360307),.UNSPECIFIED.);
#2213=B_SPLINE_SURFACE_WITH_KNOTS('',3,3,((#65943,#65944,#65945,#65946),
(#65947,#65948,#65949,#65950),(#65951,#65952,#65953,#65954),(#65955,#65956,
#65957,#65958)),.UNSPECIFIED.,.F.,.F.,.F.,(4,4),(4,4),(0.522097120207691,
1.00286862201147),(0.0300094532292164,0.0365944846647027),.UNSPECIFIED.);
#2214=B_SPLINE_SURFACE_WITH_KNOTS('',3,3,((#65966,#65967,#65968,#65969),
(#65970,#65971,#65972,#65973),(#65974,#65975,#65976,#65977),(#65978,#65979,
#65980,#65981)),.UNSPECIFIED.,.F.,.F.,.F.,(4,4),(4,4),(-0.00286753128226228,
0.477902879812248),(0.0166015299238962,0.0231736788111887),
 .UNSPECIFIED.);
#2215=B_SPLINE_SURFACE_WITH_KNOTS('',3,3,((#65992,#65993,#65994,#65995),
(#65996,#65997,#65998,#65999),(#66000,#66001,#66002,#66003),(#66004,#66005,
#66006,#66007)),.UNSPECIFIED.,.F.,.F.,.F.,(4,4),(4,4),(-0.00286823257327278,
0.477902879814032),(0.0265907346180614,0.0331702037100441),
 .UNSPECIFIED.);
#2216=B_SPLINE_SURFACE_WITH_KNOTS('',3,3,((#66051,#66052,#66053,#66054),
(#66055,#66056,#66057,#66058),(#66059,#66060,#66061,#66062),(#66063,#66064,
#66065,#66066)),.UNSPECIFIED.,.F.,.F.,.F.,(4,4),(4,4),(-0.00600003960402798,
1.),(0.0166015299238298,0.0265907346180636),.UNSPECIFIED.);
#2217=B_SPLINE_SURFACE_WITH_KNOTS('',3,3,((#66078,#66079,#66080,#66081),
(#66082,#66083,#66084,#66085),(#66086,#66087,#66088,#66089),(#66090,#66091,
#66092,#66093)),.UNSPECIFIED.,.F.,.F.,.F.,(4,4),(4,4),(0.522097120211835,
1.00286791014268),(0.0100271466749328,0.0166015302184286),.UNSPECIFIED.);
#2218=B_SPLINE_SURFACE_WITH_KNOTS('',3,3,((#66101,#66102,#66103,#66104),
(#66105,#66106,#66107,#66108),(#66109,#66110,#66111,#66112),(#66113,#66114,
#66115,#66116)),.UNSPECIFIED.,.F.,.F.,.F.,(4,4),(4,4),(0.522097120210755,
1.00286780410477),(0.0200175229646526,0.0265907346180628),.UNSPECIFIED.);
#2219=B_SPLINE_SURFACE_WITH_KNOTS('',3,3,((#66124,#66125,#66126,#66127),
(#66128,#66129,#66130,#66131),(#66132,#66133,#66134,#66135),(#66136,#66137,
#66138,#66139)),.UNSPECIFIED.,.F.,.F.,.F.,(4,4),(4,4),(-0.00206901892528682,
0.346769728512502),(0.00660713154708869,0.0131849431292509),
 .UNSPECIFIED.);
#2220=B_SPLINE_SURFACE_WITH_KNOTS('',3,3,((#66142,#66143,#66144,#66145),
(#66146,#66147,#66148,#66149),(#66150,#66151,#66152,#66153),(#66154,#66155,
#66156,#66157)),.UNSPECIFIED.,.F.,.F.,.F.,(4,4),(4,4),(-0.00286753114059943,
0.477902879812669),(0.0166015299238967,0.0231736788090041),
 .UNSPECIFIED.);
#2221=B_SPLINE_SURFACE_WITH_KNOTS('',3,3,((#66202,#66203,#66204,#66205),
(#66206,#66207,#66208,#66209),(#66210,#66211,#66212,#66213),(#66214,#66215,
#66216,#66217)),.UNSPECIFIED.,.F.,.F.,.F.,(4,4),(4,4),(0.522097120209506,
1.00286791014276),(0.0100271466749321,0.0166015302184266),.UNSPECIFIED.);
#2222=B_SPLINE_SURFACE_WITH_KNOTS('',3,3,((#66225,#66226,#66227,#66228),
(#66229,#66230,#66231,#66232),(#66233,#66234,#66235,#66236),(#66237,#66238,
#66239,#66240)),.UNSPECIFIED.,.F.,.F.,.F.,(4,4),(4,4),(-0.00206901892681215,
0.346769728513212),(0.00660713154707451,0.0131849431468889),
 .UNSPECIFIED.);
#2223=B_SPLINE_SURFACE_WITH_KNOTS('',3,3,((#66243,#66244,#66245,#66246),
(#66247,#66248,#66249,#66250),(#66251,#66252,#66253,#66254),(#66255,#66256,
#66257,#66258)),.UNSPECIFIED.,.F.,.F.,.F.,(4,4),(4,4),(-0.00017189543604345,
1.00600020634822),(0.0665898698856049,0.0751325481139401),.UNSPECIFIED.);
#2224=B_SPLINE_SURFACE_WITH_KNOTS('',3,3,((#66274,#66275,#66276,#66277),
(#66278,#66279,#66280,#66281),(#66282,#66283,#66284,#66285),(#66286,#66287,
#66288,#66289)),.UNSPECIFIED.,.F.,.F.,.F.,(4,4),(4,4),(-0.00286833998606733,
0.477902879808364),(0.0665898698862513,0.0731716198748499),
 .UNSPECIFIED.);
#2225=B_SPLINE_SURFACE_WITH_KNOTS('',3,3,((#66323,#66324,#66325,#66326),
(#66327,#66328,#66329,#66330),(#66331,#66332,#66333,#66334),(#66335,#66336,
#66337,#66338)),.UNSPECIFIED.,.F.,.F.,.F.,(4,4),(4,4),(0.522097120207237,
1.00286791825536),(0.060015686548694,0.0665898700060145),.UNSPECIFIED.);
#2226=B_SPLINE_SURFACE_WITH_KNOTS('',3,3,((#66348,#66349,#66350,#66351),
(#66352,#66353,#66354,#66355),(#66356,#66357,#66358,#66359),(#66360,#66361,
#66362,#66363)),.UNSPECIFIED.,.F.,.F.,.F.,(4,4),(4,4),(-0.00286764392041053,
0.477902879806332),(0.0565997133101199,0.0631721430887065),
 .UNSPECIFIED.);
#2227=B_SPLINE_SURFACE_WITH_KNOTS('',3,3,((#66419,#66420,#66421,#66422),
(#66423,#66424,#66425,#66426),(#66427,#66428,#66429,#66430),(#66431,#66432,
#66433,#66434)),.UNSPECIFIED.,.F.,.F.,.F.,(4,4),(4,4),(0.522097120208047,
1.00286780122186),(0.0500263550858671,0.0565997133101429),.UNSPECIFIED.);
#2228=B_SPLINE_SURFACE_WITH_KNOTS('',3,3,((#66487,#66488,#66489,#66490),
(#66491,#66492,#66493,#66494),(#66495,#66496,#66497,#66498),(#66499,#66500,
#66501,#66502)),.UNSPECIFIED.,.F.,.F.,.F.,(4,4),(4,4),(0.522097120207861,
1.00286848452579),(0.04002187294657,0.0466073985929448),.UNSPECIFIED.);
#2229=B_SPLINE_SURFACE_WITH_KNOTS('',3,3,((#66568,#66569,#66570,#66571),
(#66572,#66573,#66574,#66575),(#66576,#66577,#66578,#66579),(#66580,#66581,
#66582,#66583)),.UNSPECIFIED.,.F.,.F.,.F.,(4,4),(4,4),(0.522097120207821,
1.00286862201146),(0.0300094532292163,0.0365944846647042),.UNSPECIFIED.);
#2230=B_SPLINE_SURFACE_WITH_KNOTS('',3,3,((#66616,#66617,#66618,#66619),
(#66620,#66621,#66622,#66623),(#66624,#66625,#66626,#66627),(#66628,#66629,
#66630,#66631)),.UNSPECIFIED.,.F.,.F.,.F.,(4,4),(4,4),(-0.00600003961893236,
1.00000000246922),(0.0166015299238283,0.0265907346180639),.UNSPECIFIED.);
#2231=B_SPLINE_SURFACE_WITH_KNOTS('',3,3,((#66643,#66644,#66645,#66646),
(#66647,#66648,#66649,#66650),(#66651,#66652,#66653,#66654),(#66655,#66656,
#66657,#66658)),.UNSPECIFIED.,.F.,.F.,.F.,(4,4),(4,4),(0.522097120207632,
1.00286780410469),(0.0200175229646513,0.0265907346180639),.UNSPECIFIED.);
#2232=B_SPLINE_SURFACE_WITH_KNOTS('',3,3,((#66666,#66667,#66668,#66669),
(#66670,#66671,#66672,#66673),(#66674,#66675,#66676,#66677),(#66678,#66679,
#66680,#66681)),.UNSPECIFIED.,.F.,.F.,.F.,(4,4),(4,4),(-0.00286753128237169,
0.477902879811433),(0.0166015299238964,0.0231736788111891),
 .UNSPECIFIED.);
#2233=B_SPLINE_SURFACE_WITH_KNOTS('',3,3,((#66721,#66722,#66723,#66724),
(#66725,#66726,#66727,#66728),(#66729,#66730,#66731,#66732),(#66733,#66734,
#66735,#66736)),.UNSPECIFIED.,.F.,.F.,.F.,(4,4),(4,4),(0.52209712020752,
1.00286791014276),(0.0100271466749314,0.0166015302184266),.UNSPECIFIED.);
#2234=B_SPLINE_SURFACE_WITH_KNOTS('',3,3,((#66744,#66745,#66746,#66747),
(#66748,#66749,#66750,#66751),(#66752,#66753,#66754,#66755),(#66756,#66757,
#66758,#66759)),.UNSPECIFIED.,.F.,.F.,.F.,(4,4),(4,4),(-0.00206901892532922,
0.346769728511554),(0.006607131547103,0.0131849431292508),.UNSPECIFIED.);
#2235=B_SPLINE_SURFACE_WITH_KNOTS('',3,3,((#66769,#66770,#66771,#66772),
(#66773,#66774,#66775,#66776),(#66777,#66778,#66779,#66780),(#66781,#66782,
#66783,#66784)),.UNSPECIFIED.,.F.,.F.,.F.,(4,4),(4,4),(-0.000171895436876361,
1.0060002063483),(0.0665898698856048,0.0751325481147718),.UNSPECIFIED.);
#2236=B_SPLINE_SURFACE_WITH_KNOTS('',3,3,((#66800,#66801,#66802,#66803),
(#66804,#66805,#66806,#66807),(#66808,#66809,#66810,#66811),(#66812,#66813,
#66814,#66815)),.UNSPECIFIED.,.F.,.F.,.F.,(4,4),(4,4),(-0.00286833998598439,
0.477902879806776),(0.0665898698862512,0.0731716198748508),
 .UNSPECIFIED.);
#2237=B_SPLINE_SURFACE_WITH_KNOTS('',3,3,((#66849,#66850,#66851,#66852),
(#66853,#66854,#66855,#66856),(#66857,#66858,#66859,#66860),(#66861,#66862,
#66863,#66864)),.UNSPECIFIED.,.F.,.F.,.F.,(4,4),(4,4),(0.52209712020747,
1.00286791825534),(0.0600156865486935,0.0665898700060149),.UNSPECIFIED.);
#2238=B_SPLINE_SURFACE_WITH_KNOTS('',3,3,((#66874,#66875,#66876,#66877),
(#66878,#66879,#66880,#66881),(#66882,#66883,#66884,#66885),(#66886,#66887,
#66888,#66889)),.UNSPECIFIED.,.F.,.F.,.F.,(4,4),(4,4),(-0.00286764392048183,
0.477902879805442),(0.0565997133101207,0.0631721430887071),
 .UNSPECIFIED.);
#2239=B_SPLINE_SURFACE_WITH_KNOTS('',3,3,((#66926,#66927,#66928,#66929),
(#66930,#66931,#66932,#66933),(#66934,#66935,#66936,#66937),(#66938,#66939,
#66940,#66941)),.UNSPECIFIED.,.F.,.F.,.F.,(4,4),(4,4),(0.52209712020814,
1.00286780122194),(0.0500263550858672,0.0565997133101429),.UNSPECIFIED.);
#2240=B_SPLINE_SURFACE_WITH_KNOTS('',3,3,((#67043,#67044,#67045,#67046),
(#67047,#67048,#67049,#67050),(#67051,#67052,#67053,#67054),(#67055,#67056,
#67057,#67058)),.UNSPECIFIED.,.F.,.F.,.F.,(4,4),(4,4),(0.522097120207753,
1.00286848452573),(0.0400218729465699,0.0466073985929442),.UNSPECIFIED.);
#2241=B_SPLINE_SURFACE_WITH_KNOTS('',3,3,((#67097,#67098,#67099,#67100),
(#67101,#67102,#67103,#67104),(#67105,#67106,#67107,#67108),(#67109,#67110,
#67111,#67112)),.UNSPECIFIED.,.F.,.F.,.F.,(4,4),(4,4),(0.522097120207934,
1.00286862201156),(0.0300094532292163,0.0365944846647036),.UNSPECIFIED.);
#2242=B_SPLINE_SURFACE_WITH_KNOTS('',3,3,((#67145,#67146,#67147,#67148),
(#67149,#67150,#67151,#67152),(#67153,#67154,#67155,#67156),(#67157,#67158,
#67159,#67160)),.UNSPECIFIED.,.F.,.F.,.F.,(4,4),(4,4),(-0.00600003960417136,
1.),(0.0166015299238285,0.0265907346180639),.UNSPECIFIED.);
#2243=B_SPLINE_SURFACE_WITH_KNOTS('',3,3,((#67172,#67173,#67174,#67175),
(#67176,#67177,#67178,#67179),(#67180,#67181,#67182,#67183),(#67184,#67185,
#67186,#67187)),.UNSPECIFIED.,.F.,.F.,.F.,(4,4),(4,4),(0.522097120207778,
1.00286780410464),(0.0200175229646509,0.0265907346180637),.UNSPECIFIED.);
#2244=B_SPLINE_SURFACE_WITH_KNOTS('',3,3,((#67243,#67244,#67245,#67246),
(#67247,#67248,#67249,#67250),(#67251,#67252,#67253,#67254),(#67255,#67256,
#67257,#67258)),.UNSPECIFIED.,.F.,.F.,.F.,(4,4),(4,4),(0.522097120207468,
1.00286791014282),(0.0100271466749307,0.0166015302184274),.UNSPECIFIED.);
#2245=B_SPLINE_SURFACE_WITH_KNOTS('',3,3,((#67266,#67267,#67268,#67269),
(#67270,#67271,#67272,#67273),(#67274,#67275,#67276,#67277),(#67278,#67279,
#67280,#67281)),.UNSPECIFIED.,.F.,.F.,.F.,(4,4),(4,4),(-0.00206901892691836,
0.346769728510449),(0.0066071315471172,0.01318494314689),.UNSPECIFIED.);
#2246=B_SPLINE_SURFACE_WITH_KNOTS('',3,3,((#67291,#67292,#67293,#67294),
(#67295,#67296,#67297,#67298),(#67299,#67300,#67301,#67302),(#67303,#67304,
#67305,#67306)),.UNSPECIFIED.,.F.,.F.,.F.,(4,4),(4,4),(-0.000171895437594373,
1.00600020634835),(0.0665898698856038,0.0751325481154914),.UNSPECIFIED.);
#2247=B_SPLINE_SURFACE_WITH_KNOTS('',3,3,((#67322,#67323,#67324,#67325),
(#67326,#67327,#67328,#67329),(#67330,#67331,#67332,#67333),(#67334,#67335,
#67336,#67337)),.UNSPECIFIED.,.F.,.F.,.F.,(4,4),(4,4),(-0.00286833998596821,
0.477902879804721),(0.0665898698862504,0.0731716198748499),
 .UNSPECIFIED.);
#2248=B_SPLINE_SURFACE_WITH_KNOTS('',3,3,((#67371,#67372,#67373,#67374),
(#67375,#67376,#67377,#67378),(#67379,#67380,#67381,#67382),(#67383,#67384,
#67385,#67386)),.UNSPECIFIED.,.F.,.F.,.F.,(4,4),(4,4),(0.522097120207427,
1.00286791825535),(0.0600156865486936,0.0665898700060144),.UNSPECIFIED.);
#2249=B_SPLINE_SURFACE_WITH_KNOTS('',3,3,((#67396,#67397,#67398,#67399),
(#67400,#67401,#67402,#67403),(#67404,#67405,#67406,#67407),(#67408,#67409,
#67410,#67411)),.UNSPECIFIED.,.F.,.F.,.F.,(4,4),(4,4),(-0.0028676439203989,
0.477902879804634),(0.0565997133101206,0.0631721430887066),
 .UNSPECIFIED.);
#2250=B_SPLINE_SURFACE_WITH_KNOTS('',3,3,((#67448,#67449,#67450,#67451),
(#67452,#67453,#67454,#67455),(#67456,#67457,#67458,#67459),(#67460,#67461,
#67462,#67463)),.UNSPECIFIED.,.F.,.F.,.F.,(4,4),(4,4),(0.522097120208323,
1.00286780122187),(0.0500263550858673,0.0565997133101427),.UNSPECIFIED.);
#2251=B_SPLINE_SURFACE_WITH_KNOTS('',3,3,((#67535,#67536,#67537,#67538),
(#67539,#67540,#67541,#67542),(#67543,#67544,#67545,#67546),(#67547,#67548,
#67549,#67550)),.UNSPECIFIED.,.F.,.F.,.F.,(4,4),(4,4),(0.522097120207898,
1.00286848452575),(0.0400218729465706,0.0466073985929453),.UNSPECIFIED.);
#2252=B_SPLINE_SURFACE_WITH_KNOTS('',3,3,((#67638,#67639,#67640,#67641),
(#67642,#67643,#67644,#67645),(#67646,#67647,#67648,#67649),(#67650,#67651,
#67652,#67653)),.UNSPECIFIED.,.F.,.F.,.F.,(4,4),(4,4),(0.52209712020705,
1.00286862201153),(0.0300094532292157,0.0365944846647043),.UNSPECIFIED.);
#2253=B_SPLINE_SURFACE_WITH_KNOTS('',3,3,((#67667,#67668,#67669,#67670),
(#67671,#67672,#67673,#67674),(#67675,#67676,#67677,#67678),(#67679,#67680,
#67681,#67682)),.UNSPECIFIED.,.F.,.F.,.F.,(4,4),(4,4),(-0.00600003961898803,
1.00000000246933),(0.0166015299238284,0.0265907346180633),.UNSPECIFIED.);
#2254=B_SPLINE_SURFACE_WITH_KNOTS('',3,3,((#67694,#67695,#67696,#67697),
(#67698,#67699,#67700,#67701),(#67702,#67703,#67704,#67705),(#67706,#67707,
#67708,#67709)),.UNSPECIFIED.,.F.,.F.,.F.,(4,4),(4,4),(0.522097120207611,
1.00286780410466),(0.0200175229646512,0.026590734618064),.UNSPECIFIED.);
#2255=B_SPLINE_SURFACE_WITH_KNOTS('',3,3,((#67762,#67763,#67764,#67765),
(#67766,#67767,#67768,#67769),(#67770,#67771,#67772,#67773),(#67774,#67775,
#67776,#67777)),.UNSPECIFIED.,.F.,.F.,.F.,(4,4),(4,4),(0.522097120207844,
1.00286791014275),(0.010027146674931,0.0166015302184281),.UNSPECIFIED.);
#2256=B_SPLINE_SURFACE_WITH_KNOTS('',3,3,((#67803,#67804,#67805,#67806),
(#67807,#67808,#67809,#67810),(#67811,#67812,#67813,#67814),(#67815,#67816,
#67817,#67818)),.UNSPECIFIED.,.F.,.F.,.F.,(4,4),(4,4),(-0.000171895438429025,
1.00600020634782),(0.0665898698856051,0.0751325481163243),.UNSPECIFIED.);
#2257=B_SPLINE_SURFACE_WITH_KNOTS('',3,3,((#67834,#67835,#67836,#67837),
(#67838,#67839,#67840,#67841),(#67842,#67843,#67844,#67845),(#67846,#67847,
#67848,#67849)),.UNSPECIFIED.,.F.,.F.,.F.,(4,4),(4,4),(-0.00286833998609855,
0.477902879802562),(0.0665898698862514,0.0731716198748506),
 .UNSPECIFIED.);
#2258=B_SPLINE_SURFACE_WITH_KNOTS('',3,3,((#67883,#67884,#67885,#67886),
(#67887,#67888,#67889,#67890),(#67891,#67892,#67893,#67894),(#67895,#67896,
#67897,#67898)),.UNSPECIFIED.,.F.,.F.,.F.,(4,4),(4,4),(0.522097120207539,
1.00286791825532),(0.0600156865486929,0.0665898700060141),.UNSPECIFIED.);
#2259=B_SPLINE_SURFACE_WITH_KNOTS('',3,3,((#67908,#67909,#67910,#67911),
(#67912,#67913,#67914,#67915),(#67916,#67917,#67918,#67919),(#67920,#67921,
#67922,#67923)),.UNSPECIFIED.,.F.,.F.,.F.,(4,4),(4,4),(-0.00286764392058903,
0.477902879803589),(0.0565997133101206,0.0631721430887071),
 .UNSPECIFIED.);
#2260=B_SPLINE_SURFACE_WITH_KNOTS('',3,3,((#67960,#67961,#67962,#67963),
(#67964,#67965,#67966,#67967),(#67968,#67969,#67970,#67971),(#67972,#67973,
#67974,#67975)),.UNSPECIFIED.,.F.,.F.,.F.,(4,4),(4,4),(0.522097120208424,
1.00286780122193),(0.0500263550858662,0.0565997133101414),.UNSPECIFIED.);
#2261=B_SPLINE_SURFACE_WITH_KNOTS('',3,3,((#68047,#68048,#68049,#68050),
(#68051,#68052,#68053,#68054),(#68055,#68056,#68057,#68058),(#68059,#68060,
#68061,#68062)),.UNSPECIFIED.,.F.,.F.,.F.,(4,4),(4,4),(0.522097120208083,
1.00286848452576),(0.0400218729465703,0.046607398592945),.UNSPECIFIED.);
#2262=B_SPLINE_SURFACE_WITH_KNOTS('',3,3,((#68131,#68132,#68133,#68134),
(#68135,#68136,#68137,#68138),(#68139,#68140,#68141,#68142),(#68143,#68144,
#68145,#68146)),.UNSPECIFIED.,.F.,.F.,.F.,(4,4),(4,4),(0.522097120207127,
1.00286862201156),(0.0300094532292159,0.0365944846647045),.UNSPECIFIED.);
#2263=B_SPLINE_SURFACE_WITH_KNOTS('',3,3,((#68173,#68174,#68175,#68176),
(#68177,#68178,#68179,#68180),(#68181,#68182,#68183,#68184),(#68185,#68186,
#68187,#68188)),.UNSPECIFIED.,.F.,.F.,.F.,(4,4),(4,4),(-0.00600003961897224,
1.00000000246921),(0.0166015299238289,0.0265907346180631),.UNSPECIFIED.);
#2264=B_SPLINE_SURFACE_WITH_KNOTS('',3,3,((#68225,#68226,#68227,#68228),
(#68229,#68230,#68231,#68232),(#68233,#68234,#68235,#68236),(#68237,#68238,
#68239,#68240)),.UNSPECIFIED.,.F.,.F.,.F.,(4,4),(4,4),(0.522097120208025,
1.0028678041047),(0.0200175229646515,0.0265907346180654),.UNSPECIFIED.);
#2265=B_SPLINE_SURFACE_WITH_KNOTS('',3,3,((#68274,#68275,#68276,#68277),
(#68278,#68279,#68280,#68281),(#68282,#68283,#68284,#68285),(#68286,#68287,
#68288,#68289)),.UNSPECIFIED.,.F.,.F.,.F.,(4,4),(4,4),(0.522097120207859,
1.0028679101242),(0.0100271466766969,0.0166015299239905),.UNSPECIFIED.);
#2266=B_SPLINE_SURFACE_WITH_KNOTS('',3,3,((#68315,#68316,#68317,#68318),
(#68319,#68320,#68321,#68322),(#68323,#68324,#68325,#68326),(#68327,#68328,
#68329,#68330)),.UNSPECIFIED.,.F.,.F.,.F.,(4,4),(4,4),(-0.000171895439399329,
1.00600020634824),(0.0665898698856054,0.075132548117295),.UNSPECIFIED.);
#2267=B_SPLINE_SURFACE_WITH_KNOTS('',3,3,((#68346,#68347,#68348,#68349),
(#68350,#68351,#68352,#68353),(#68354,#68355,#68356,#68357),(#68358,#68359,
#68360,#68361)),.UNSPECIFIED.,.F.,.F.,.F.,(4,4),(4,4),(-0.00286833998591409,
0.477902879800245),(0.0665898698862516,0.0731716198748497),
 .UNSPECIFIED.);
#2268=B_SPLINE_SURFACE_WITH_KNOTS('',3,3,((#68395,#68396,#68397,#68398),
(#68399,#68400,#68401,#68402),(#68403,#68404,#68405,#68406),(#68407,#68408,
#68409,#68410)),.UNSPECIFIED.,.F.,.F.,.F.,(4,4),(4,4),(0.522097120207782,
1.00286791825533),(0.0600156865486934,0.0665898700060146),.UNSPECIFIED.);
#2269=B_SPLINE_SURFACE_WITH_KNOTS('',3,3,((#68420,#68421,#68422,#68423),
(#68424,#68425,#68426,#68427),(#68428,#68429,#68430,#68431),(#68432,#68433,
#68434,#68435)),.UNSPECIFIED.,.F.,.F.,.F.,(4,4),(4,4),(-0.00286764392045514,
0.477902879801544),(0.0565997133101201,0.0631721430887063),
 .UNSPECIFIED.);
#2270=B_SPLINE_SURFACE_WITH_KNOTS('',3,3,((#68472,#68473,#68474,#68475),
(#68476,#68477,#68478,#68479),(#68480,#68481,#68482,#68483),(#68484,#68485,
#68486,#68487)),.UNSPECIFIED.,.F.,.F.,.F.,(4,4),(4,4),(0.522097120208516,
1.00286780122182),(0.0500263550858674,0.056599713310142),.UNSPECIFIED.);
#2271=B_SPLINE_SURFACE_WITH_KNOTS('',3,3,((#68559,#68560,#68561,#68562),
(#68563,#68564,#68565,#68566),(#68567,#68568,#68569,#68570),(#68571,#68572,
#68573,#68574)),.UNSPECIFIED.,.F.,.F.,.F.,(4,4),(4,4),(0.522097120208114,
1.00286848452572),(0.04002187294657,0.0466073985929447),.UNSPECIFIED.);
#2272=B_SPLINE_SURFACE_WITH_KNOTS('',3,3,((#68643,#68644,#68645,#68646),
(#68647,#68648,#68649,#68650),(#68651,#68652,#68653,#68654),(#68655,#68656,
#68657,#68658)),.UNSPECIFIED.,.F.,.F.,.F.,(4,4),(4,4),(0.522097120207307,
1.00286862201159),(0.0300094532292165,0.036594484664703),.UNSPECIFIED.);
#2273=B_SPLINE_SURFACE_WITH_KNOTS('',3,3,((#68691,#68692,#68693,#68694),
(#68695,#68696,#68697,#68698),(#68699,#68700,#68701,#68702),(#68703,#68704,
#68705,#68706)),.UNSPECIFIED.,.F.,.F.,.F.,(4,4),(4,4),(-0.00600003961900311,
1.00000000246904),(0.0166015299238284,0.0265907346180639),.UNSPECIFIED.);
#2274=B_SPLINE_SURFACE_WITH_KNOTS('',3,3,((#68718,#68719,#68720,#68721),
(#68722,#68723,#68724,#68725),(#68726,#68727,#68728,#68729),(#68730,#68731,
#68732,#68733)),.UNSPECIFIED.,.F.,.F.,.F.,(4,4),(4,4),(0.522097120208122,
1.00286780410469),(0.0200175229646511,0.0265907346180648),.UNSPECIFIED.);
#2275=B_SPLINE_SURFACE_WITH_KNOTS('',3,3,((#68800,#68801,#68802,#68803),
(#68804,#68805,#68806,#68807),(#68808,#68809,#68810,#68811),(#68812,#68813,
#68814,#68815)),.UNSPECIFIED.,.F.,.F.,.F.,(4,4),(4,4),(0.522097120208081,
1.00286791016343),(0.0100271466746118,0.0166015302184275),.UNSPECIFIED.);
#2276=B_SPLINE_SURFACE_WITH_KNOTS('',3,3,((#68830,#68831,#68832,#68833),
(#68834,#68835,#68836,#68837),(#68838,#68839,#68840,#68841),(#68842,#68843,
#68844,#68845)),.UNSPECIFIED.,.F.,.F.,.F.,(4,4),(4,4),(-0.000171895439914325,
1.00600020634824),(0.0665898698856042,0.0751325481178124),.UNSPECIFIED.);
#2277=B_SPLINE_SURFACE_WITH_KNOTS('',3,3,((#68861,#68862,#68863,#68864),
(#68865,#68866,#68867,#68868),(#68869,#68870,#68871,#68872),(#68873,#68874,
#68875,#68876)),.UNSPECIFIED.,.F.,.F.,.F.,(4,4),(4,4),(-0.00286833998599997,
0.477902879797889),(0.0665898698862502,0.0731716198748498),
 .UNSPECIFIED.);
#2278=B_SPLINE_SURFACE_WITH_KNOTS('',3,3,((#68910,#68911,#68912,#68913),
(#68914,#68915,#68916,#68917),(#68918,#68919,#68920,#68921),(#68922,#68923,
#68924,#68925)),.UNSPECIFIED.,.F.,.F.,.F.,(4,4),(4,4),(0.522097120207876,
1.00286791825534),(0.0600156865486929,0.0665898700060145),.UNSPECIFIED.);
#2279=B_SPLINE_SURFACE_WITH_KNOTS('',3,3,((#68935,#68936,#68937,#68938),
(#68939,#68940,#68941,#68942),(#68943,#68944,#68945,#68946),(#68947,#68948,
#68949,#68950)),.UNSPECIFIED.,.F.,.F.,.F.,(4,4),(4,4),(-0.00286764392042158,
0.477902879799075),(0.0565997133101205,0.0631721430887066),
 .UNSPECIFIED.);
#2280=B_SPLINE_SURFACE_WITH_KNOTS('',3,3,((#68987,#68988,#68989,#68990),
(#68991,#68992,#68993,#68994),(#68995,#68996,#68997,#68998),(#68999,#69000,
#69001,#69002)),.UNSPECIFIED.,.F.,.F.,.F.,(4,4),(4,4),(0.522097120208699,
1.0028678012219),(0.0500263550858663,0.056599713310142),.UNSPECIFIED.);
#2281=B_SPLINE_SURFACE_WITH_KNOTS('',3,3,((#69074,#69075,#69076,#69077),
(#69078,#69079,#69080,#69081),(#69082,#69083,#69084,#69085),(#69086,#69087,
#69088,#69089)),.UNSPECIFIED.,.F.,.F.,.F.,(4,4),(4,4),(0.522097120208235,
1.00286848452568),(0.0400218729465703,0.0466073985929451),.UNSPECIFIED.);
#2282=B_SPLINE_SURFACE_WITH_KNOTS('',3,3,((#69158,#69159,#69160,#69161),
(#69162,#69163,#69164,#69165),(#69166,#69167,#69168,#69169),(#69170,#69171,
#69172,#69173)),.UNSPECIFIED.,.F.,.F.,.F.,(4,4),(4,4),(0.522097120207369,
1.00286862201154),(0.0300094532292155,0.0365944846647039),.UNSPECIFIED.);
#2283=B_SPLINE_SURFACE_WITH_KNOTS('',3,3,((#69206,#69207,#69208,#69209),
(#69210,#69211,#69212,#69213),(#69214,#69215,#69216,#69217),(#69218,#69219,
#69220,#69221)),.UNSPECIFIED.,.F.,.F.,.F.,(4,4),(4,4),(-0.00600003961895626,
1.00000000246898),(0.0166015299238287,0.0265907346180638),.UNSPECIFIED.);
#2284=B_SPLINE_SURFACE_WITH_KNOTS('',3,3,((#69233,#69234,#69235,#69236),
(#69237,#69238,#69239,#69240),(#69241,#69242,#69243,#69244),(#69245,#69246,
#69247,#69248)),.UNSPECIFIED.,.F.,.F.,.F.,(4,4),(4,4),(0.52209712020829,
1.00286780410469),(0.0200175229646519,0.0265907346180654),.UNSPECIFIED.);
#2285=B_SPLINE_SURFACE_WITH_KNOTS('',3,3,((#69304,#69305,#69306,#69307),
(#69308,#69309,#69310,#69311),(#69312,#69313,#69314,#69315),(#69316,#69317,
#69318,#69319)),.UNSPECIFIED.,.F.,.F.,.F.,(4,4),(4,4),(0.522097120208155,
1.00286791014275),(0.0100271466749312,0.0166015302184278),.UNSPECIFIED.);
#2286=B_SPLINE_SURFACE_WITH_KNOTS('',3,3,((#69345,#69346,#69347,#69348),
(#69349,#69350,#69351,#69352),(#69353,#69354,#69355,#69356),(#69357,#69358,
#69359,#69360)),.UNSPECIFIED.,.F.,.F.,.F.,(4,4),(4,4),(-0.000171895440587519,
1.00600020634826),(0.0665898698856032,0.075132548118484),.UNSPECIFIED.);
#2287=B_SPLINE_SURFACE_WITH_KNOTS('',3,3,((#69376,#69377,#69378,#69379),
(#69380,#69381,#69382,#69383),(#69384,#69385,#69386,#69387),(#69388,#69389,
#69390,#69391)),.UNSPECIFIED.,.F.,.F.,.F.,(4,4),(4,4),(-0.00286833998609265,
0.477902879795302),(0.0665898698862507,0.0731716198748496),
 .UNSPECIFIED.);
#2288=B_SPLINE_SURFACE_WITH_KNOTS('',3,3,((#69425,#69426,#69427,#69428),
(#69429,#69430,#69431,#69432),(#69433,#69434,#69435,#69436),(#69437,#69438,
#69439,#69440)),.UNSPECIFIED.,.F.,.F.,.F.,(4,4),(4,4),(0.522097120207918,
1.0028679182553),(0.0600156865486945,0.0665898700060156),.UNSPECIFIED.);
#2289=B_SPLINE_SURFACE_WITH_KNOTS('',3,3,((#69450,#69451,#69452,#69453),
(#69454,#69455,#69456,#69457),(#69458,#69459,#69460,#69461),(#69462,#69463,
#69464,#69465)),.UNSPECIFIED.,.F.,.F.,.F.,(4,4),(4,4),(-0.00286764392026509,
0.477902879796714),(0.0565997133101197,0.0631721430887055),
 .UNSPECIFIED.);
#2290=B_SPLINE_SURFACE_WITH_KNOTS('',3,3,((#69502,#69503,#69504,#69505),
(#69506,#69507,#69508,#69509),(#69510,#69511,#69512,#69513),(#69514,#69515,
#69516,#69517)),.UNSPECIFIED.,.F.,.F.,.F.,(4,4),(4,4),(0.522097120208835,
1.00286780122186),(0.0500263550858674,0.0565997133101427),.UNSPECIFIED.);
#2291=B_SPLINE_SURFACE_WITH_KNOTS('',3,3,((#69589,#69590,#69591,#69592),
(#69593,#69594,#69595,#69596),(#69597,#69598,#69599,#69600),(#69601,#69602,
#69603,#69604)),.UNSPECIFIED.,.F.,.F.,.F.,(4,4),(4,4),(0.522097120208443,
1.00286848452571),(0.0400218729465707,0.0466073985929442),.UNSPECIFIED.);
#2292=B_SPLINE_SURFACE_WITH_KNOTS('',3,3,((#69673,#69674,#69675,#69676),
(#69677,#69678,#69679,#69680),(#69681,#69682,#69683,#69684),(#69685,#69686,
#69687,#69688)),.UNSPECIFIED.,.F.,.F.,.F.,(4,4),(4,4),(0.522097120207526,
1.00286862201152),(0.0300094532292168,0.0365944846647034),.UNSPECIFIED.);
#2293=B_SPLINE_SURFACE_WITH_KNOTS('',3,3,((#69721,#69722,#69723,#69724),
(#69725,#69726,#69727,#69728),(#69729,#69730,#69731,#69732),(#69733,#69734,
#69735,#69736)),.UNSPECIFIED.,.F.,.F.,.F.,(4,4),(4,4),(-0.00600003961890225,
1.00000000246947),(0.0166015299238274,0.0265907346180638),.UNSPECIFIED.);
#2294=B_SPLINE_SURFACE_WITH_KNOTS('',3,3,((#69748,#69749,#69750,#69751),
(#69752,#69753,#69754,#69755),(#69756,#69757,#69758,#69759),(#69760,#69761,
#69762,#69763)),.UNSPECIFIED.,.F.,.F.,.F.,(4,4),(4,4),(0.522097120208393,
1.00286780410469),(0.0200175229646505,0.0265907346180638),.UNSPECIFIED.);
#2295=B_SPLINE_SURFACE_WITH_KNOTS('',3,3,((#69819,#69820,#69821,#69822),
(#69823,#69824,#69825,#69826),(#69827,#69828,#69829,#69830),(#69831,#69832,
#69833,#69834)),.UNSPECIFIED.,.F.,.F.,.F.,(4,4),(4,4),(0.522097120208245,
1.00286791014273),(0.0100271466749314,0.0166015302184273),.UNSPECIFIED.);
#2296=B_SPLINE_SURFACE_WITH_KNOTS('',3,3,((#69860,#69861,#69862,#69863),
(#69864,#69865,#69866,#69867),(#69868,#69869,#69870,#69871),(#69872,#69873,
#69874,#69875)),.UNSPECIFIED.,.F.,.F.,.F.,(4,4),(4,4),(-0.000171895440979682,
1.00600020634811),(0.0665898698856036,0.0751325481188771),.UNSPECIFIED.);
#2297=B_SPLINE_SURFACE_WITH_KNOTS('',3,3,((#69891,#69892,#69893,#69894),
(#69895,#69896,#69897,#69898),(#69899,#69900,#69901,#69902),(#69903,#69904,
#69905,#69906)),.UNSPECIFIED.,.F.,.F.,.F.,(4,4),(4,4),(-0.00286833998597401,
0.477902879792813),(0.0665898698862506,0.0731716198748496),
 .UNSPECIFIED.);
#2298=B_SPLINE_SURFACE_WITH_KNOTS('',3,3,((#69940,#69941,#69942,#69943),
(#69944,#69945,#69946,#69947),(#69948,#69949,#69950,#69951),(#69952,#69953,
#69954,#69955)),.UNSPECIFIED.,.F.,.F.,.F.,(4,4),(4,4),(0.522097120208123,
1.0028679182553),(0.0600156865486942,0.0665898700060151),.UNSPECIFIED.);
#2299=B_SPLINE_SURFACE_WITH_KNOTS('',3,3,((#69965,#69966,#69967,#69968),
(#69969,#69970,#69971,#69972),(#69973,#69974,#69975,#69976),(#69977,#69978,
#69979,#69980)),.UNSPECIFIED.,.F.,.F.,.F.,(4,4),(4,4),(-0.00286764392041422,
0.477902879794138),(0.0565997133101191,0.0631721430887055),
 .UNSPECIFIED.);
#2300=B_SPLINE_SURFACE_WITH_KNOTS('',3,3,((#70017,#70018,#70019,#70020),
(#70021,#70022,#70023,#70024),(#70025,#70026,#70027,#70028),(#70029,#70030,
#70031,#70032)),.UNSPECIFIED.,.F.,.F.,.F.,(4,4),(4,4),(0.522097120208892,
1.00286780122189),(0.0500263550858667,0.0565997133101436),.UNSPECIFIED.);
#2301=B_SPLINE_SURFACE_WITH_KNOTS('',3,3,((#70104,#70105,#70106,#70107),
(#70108,#70109,#70110,#70111),(#70112,#70113,#70114,#70115),(#70116,#70117,
#70118,#70119)),.UNSPECIFIED.,.F.,.F.,.F.,(4,4),(4,4),(0.522097120208542,
1.00286848452571),(0.04002187294657,0.046607398592945),.UNSPECIFIED.);
#2302=B_SPLINE_SURFACE_WITH_KNOTS('',3,3,((#70188,#70189,#70190,#70191),
(#70192,#70193,#70194,#70195),(#70196,#70197,#70198,#70199),(#70200,#70201,
#70202,#70203)),.UNSPECIFIED.,.F.,.F.,.F.,(4,4),(4,4),(0.522097120207708,
1.00286862201152),(0.0300094532292153,0.0365944846647039),.UNSPECIFIED.);
#2303=B_SPLINE_SURFACE_WITH_KNOTS('',3,3,((#70236,#70237,#70238,#70239),
(#70240,#70241,#70242,#70243),(#70244,#70245,#70246,#70247),(#70248,#70249,
#70250,#70251)),.UNSPECIFIED.,.F.,.F.,.F.,(4,4),(4,4),(-0.0060000396189727,
1.00000000246903),(0.0166015299238285,0.0265907346180665),.UNSPECIFIED.);
#2304=B_SPLINE_SURFACE_WITH_KNOTS('',3,3,((#70263,#70264,#70265,#70266),
(#70267,#70268,#70269,#70270),(#70271,#70272,#70273,#70274),(#70275,#70276,
#70277,#70278)),.UNSPECIFIED.,.F.,.F.,.F.,(4,4),(4,4),(0.522097120208515,
1.0028678041046),(0.0200175229646511,0.0265907346180649),.UNSPECIFIED.);
#2305=B_SPLINE_SURFACE_WITH_KNOTS('',3,3,((#70334,#70335,#70336,#70337),
(#70338,#70339,#70340,#70341),(#70342,#70343,#70344,#70345),(#70346,#70347,
#70348,#70349)),.UNSPECIFIED.,.F.,.F.,.F.,(4,4),(4,4),(0.522097120208354,
1.00286791014275),(0.0100271466749302,0.0166015302184277),.UNSPECIFIED.);
#2306=B_SPLINE_SURFACE_WITH_KNOTS('',3,3,((#70375,#70376,#70377,#70378),
(#70379,#70380,#70381,#70382),(#70383,#70384,#70385,#70386),(#70387,#70388,
#70389,#70390)),.UNSPECIFIED.,.F.,.F.,.F.,(4,4),(4,4),(-0.000171895441186971,
1.00600020634811),(0.0665898698856045,0.0751325481190837),.UNSPECIFIED.);
#2307=B_SPLINE_SURFACE_WITH_KNOTS('',3,3,((#70406,#70407,#70408,#70409),
(#70410,#70411,#70412,#70413),(#70414,#70415,#70416,#70417),(#70418,#70419,
#70420,#70421)),.UNSPECIFIED.,.F.,.F.,.F.,(4,4),(4,4),(-0.00286833998595339,
0.477902879790259),(0.0665898698862505,0.0731716198748495),
 .UNSPECIFIED.);
#2308=B_SPLINE_SURFACE_WITH_KNOTS('',3,3,((#70455,#70456,#70457,#70458),
(#70459,#70460,#70461,#70462),(#70463,#70464,#70465,#70466),(#70467,#70468,
#70469,#70470)),.UNSPECIFIED.,.F.,.F.,.F.,(4,4),(4,4),(0.52209712020833,
1.00286791825539),(0.060015686548694,0.0665898700060138),.UNSPECIFIED.);
#2309=B_SPLINE_SURFACE_WITH_KNOTS('',3,3,((#70480,#70481,#70482,#70483),
(#70484,#70485,#70486,#70487),(#70488,#70489,#70490,#70491),(#70492,#70493,
#70494,#70495)),.UNSPECIFIED.,.F.,.F.,.F.,(4,4),(4,4),(-0.0028676439203935,
0.47790287979146),(0.0565997133101203,0.0631721430887067),.UNSPECIFIED.);
#2310=B_SPLINE_SURFACE_WITH_KNOTS('',3,3,((#70532,#70533,#70534,#70535),
(#70536,#70537,#70538,#70539),(#70540,#70541,#70542,#70543),(#70544,#70545,
#70546,#70547)),.UNSPECIFIED.,.F.,.F.,.F.,(4,4),(4,4),(0.522097120209094,
1.00286780122184),(0.0500263550858663,0.0565997133101416),.UNSPECIFIED.);
#2311=B_SPLINE_SURFACE_WITH_KNOTS('',3,3,((#70619,#70620,#70621,#70622),
(#70623,#70624,#70625,#70626),(#70627,#70628,#70629,#70630),(#70631,#70632,
#70633,#70634)),.UNSPECIFIED.,.F.,.F.,.F.,(4,4),(4,4),(0.522097120208589,
1.0028684845257),(0.0400218729465704,0.0466073985929445),.UNSPECIFIED.);
#2312=B_SPLINE_SURFACE_WITH_KNOTS('',3,3,((#70703,#70704,#70705,#70706),
(#70707,#70708,#70709,#70710),(#70711,#70712,#70713,#70714),(#70715,#70716,
#70717,#70718)),.UNSPECIFIED.,.F.,.F.,.F.,(4,4),(4,4),(0.522097120207781,
1.00286862201155),(0.0300094532292166,0.0365944846647042),.UNSPECIFIED.);
#2313=B_SPLINE_SURFACE_WITH_KNOTS('',3,3,((#70751,#70752,#70753,#70754),
(#70755,#70756,#70757,#70758),(#70759,#70760,#70761,#70762),(#70763,#70764,
#70765,#70766)),.UNSPECIFIED.,.F.,.F.,.F.,(4,4),(4,4),(-0.00600003962552284,
1.00000000356504),(0.0166015299238284,0.0265907346180639),.UNSPECIFIED.);
#2314=B_SPLINE_SURFACE_WITH_KNOTS('',3,3,((#70778,#70779,#70780,#70781),
(#70782,#70783,#70784,#70785),(#70786,#70787,#70788,#70789),(#70790,#70791,
#70792,#70793)),.UNSPECIFIED.,.F.,.F.,.F.,(4,4),(4,4),(0.522097120208704,
1.0028678041047),(0.0200175229646511,0.0265907346180645),.UNSPECIFIED.);
#2315=B_SPLINE_SURFACE_WITH_KNOTS('',3,3,((#70849,#70850,#70851,#70852),
(#70853,#70854,#70855,#70856),(#70857,#70858,#70859,#70860),(#70861,#70862,
#70863,#70864)),.UNSPECIFIED.,.F.,.F.,.F.,(4,4),(4,4),(0.522097120208485,
1.00286791014268),(0.0100271466749304,0.0166015302184274),.UNSPECIFIED.);
#2316=B_SPLINE_SURFACE_WITH_KNOTS('',3,3,((#70890,#70891,#70892,#70893),
(#70894,#70895,#70896,#70897),(#70898,#70899,#70900,#70901),(#70902,#70903,
#70904,#70905)),.UNSPECIFIED.,.F.,.F.,.F.,(4,4),(4,4),(-0.000171895441305832,
1.0060002063484),(0.0665898698856052,0.0751325481192021),.UNSPECIFIED.);
#2317=B_SPLINE_SURFACE_WITH_KNOTS('',3,3,((#70921,#70922,#70923,#70924),
(#70925,#70926,#70927,#70928),(#70929,#70930,#70931,#70932),(#70933,#70934,
#70935,#70936)),.UNSPECIFIED.,.F.,.F.,.F.,(4,4),(4,4),(-0.00286833998590792,
0.47790287978769),(0.0665898698862517,0.0731716198748515),.UNSPECIFIED.);
#2318=B_SPLINE_SURFACE_WITH_KNOTS('',3,3,((#70970,#70971,#70972,#70973),
(#70974,#70975,#70976,#70977),(#70978,#70979,#70980,#70981),(#70982,#70983,
#70984,#70985)),.UNSPECIFIED.,.F.,.F.,.F.,(4,4),(4,4),(0.522097120208308,
1.00286791825531),(0.0600156865486945,0.0665898700060152),.UNSPECIFIED.);
#2319=B_SPLINE_SURFACE_WITH_KNOTS('',3,3,((#70995,#70996,#70997,#70998),
(#70999,#71000,#71001,#71002),(#71003,#71004,#71005,#71006),(#71007,#71008,
#71009,#71010)),.UNSPECIFIED.,.F.,.F.,.F.,(4,4),(4,4),(-0.00286764392030075,
0.477902879788978),(0.0565997133101198,0.0631721430887066),
 .UNSPECIFIED.);
#2320=B_SPLINE_SURFACE_WITH_KNOTS('',3,3,((#71047,#71048,#71049,#71050),
(#71051,#71052,#71053,#71054),(#71055,#71056,#71057,#71058),(#71059,#71060,
#71061,#71062)),.UNSPECIFIED.,.F.,.F.,.F.,(4,4),(4,4),(0.522097120209165,
1.00286780122187),(0.0500263550858667,0.0565997133101418),.UNSPECIFIED.);
#2321=B_SPLINE_SURFACE_WITH_KNOTS('',3,3,((#71134,#71135,#71136,#71137),
(#71138,#71139,#71140,#71141),(#71142,#71143,#71144,#71145),(#71146,#71147,
#71148,#71149)),.UNSPECIFIED.,.F.,.F.,.F.,(4,4),(4,4),(0.522097120208777,
1.00286848452568),(0.0400218729465703,0.0466073985929443),.UNSPECIFIED.);
#2322=B_SPLINE_SURFACE_WITH_KNOTS('',3,3,((#71218,#71219,#71220,#71221),
(#71222,#71223,#71224,#71225),(#71226,#71227,#71228,#71229),(#71230,#71231,
#71232,#71233)),.UNSPECIFIED.,.F.,.F.,.F.,(4,4),(4,4),(0.522097120207874,
1.00286862201151),(0.030009453229216,0.0365944846647041),.UNSPECIFIED.);
#2323=B_SPLINE_SURFACE_WITH_KNOTS('',3,3,((#71266,#71267,#71268,#71269),
(#71270,#71271,#71272,#71273),(#71274,#71275,#71276,#71277),(#71278,#71279,
#71280,#71281)),.UNSPECIFIED.,.F.,.F.,.F.,(4,4),(4,4),(-0.00600003964383708,
1.00000000663581),(0.0166015299238285,0.0265907346180638),.UNSPECIFIED.);
#2324=B_SPLINE_SURFACE_WITH_KNOTS('',3,3,((#71293,#71294,#71295,#71296),
(#71297,#71298,#71299,#71300),(#71301,#71302,#71303,#71304),(#71305,#71306,
#71307,#71308)),.UNSPECIFIED.,.F.,.F.,.F.,(4,4),(4,4),(0.522097120208762,
1.00286780410467),(0.0200175229646509,0.0265907346180652),.UNSPECIFIED.);
#2325=B_SPLINE_SURFACE_WITH_KNOTS('',3,3,((#71364,#71365,#71366,#71367),
(#71368,#71369,#71370,#71371),(#71372,#71373,#71374,#71375),(#71376,#71377,
#71378,#71379)),.UNSPECIFIED.,.F.,.F.,.F.,(4,4),(4,4),(0.522097120208637,
1.0028679101427),(0.0100271466749316,0.016601530218427),.UNSPECIFIED.);
#2326=B_SPLINE_SURFACE_WITH_KNOTS('',3,3,((#71405,#71406,#71407,#71408),
(#71409,#71410,#71411,#71412),(#71413,#71414,#71415,#71416),(#71417,#71418,
#71419,#71420)),.UNSPECIFIED.,.F.,.F.,.F.,(4,4),(4,4),(-0.000171895441813873,
1.00600020634879),(0.0665898698856054,0.0751325481197112),.UNSPECIFIED.);
#2327=B_SPLINE_SURFACE_WITH_KNOTS('',3,3,((#71436,#71437,#71438,#71439),
(#71440,#71441,#71442,#71443),(#71444,#71445,#71446,#71447),(#71448,#71449,
#71450,#71451)),.UNSPECIFIED.,.F.,.F.,.F.,(4,4),(4,4),(-0.00286833998582016,
0.47790287978653),(0.0665898698862516,0.0731716198748501),.UNSPECIFIED.);
#2328=B_SPLINE_SURFACE_WITH_KNOTS('',3,3,((#71485,#71486,#71487,#71488),
(#71489,#71490,#71491,#71492),(#71493,#71494,#71495,#71496),(#71497,#71498,
#71499,#71500)),.UNSPECIFIED.,.F.,.F.,.F.,(4,4),(4,4),(0.52209712020856,
1.00286791825536),(0.0600156865486949,0.0665898700060146),.UNSPECIFIED.);
#2329=B_SPLINE_SURFACE_WITH_KNOTS('',3,3,((#71510,#71511,#71512,#71513),
(#71514,#71515,#71516,#71517),(#71518,#71519,#71520,#71521),(#71522,#71523,
#71524,#71525)),.UNSPECIFIED.,.F.,.F.,.F.,(4,4),(4,4),(-0.00286764392030322,
0.477902879786523),(0.0565997133101207,0.0631721430887062),
 .UNSPECIFIED.);
#2330=B_SPLINE_SURFACE_WITH_KNOTS('',3,3,((#71562,#71563,#71564,#71565),
(#71566,#71567,#71568,#71569),(#71570,#71571,#71572,#71573),(#71574,#71575,
#71576,#71577)),.UNSPECIFIED.,.F.,.F.,.F.,(4,4),(4,4),(0.522097120209218,
1.00286780122187),(0.0500263550858677,0.0565997133101425),.UNSPECIFIED.);
#2331=B_SPLINE_SURFACE_WITH_KNOTS('',3,3,((#71649,#71650,#71651,#71652),
(#71653,#71654,#71655,#71656),(#71657,#71658,#71659,#71660),(#71661,#71662,
#71663,#71664)),.UNSPECIFIED.,.F.,.F.,.F.,(4,4),(4,4),(0.522097120208972,
1.00286848452572),(0.0400218729465709,0.046607398592944),.UNSPECIFIED.);
#2332=B_SPLINE_SURFACE_WITH_KNOTS('',3,3,((#71733,#71734,#71735,#71736),
(#71737,#71738,#71739,#71740),(#71741,#71742,#71743,#71744),(#71745,#71746,
#71747,#71748)),.UNSPECIFIED.,.F.,.F.,.F.,(4,4),(4,4),(0.522097120207987,
1.00286862201156),(0.0300094532292159,0.0365944846647027),.UNSPECIFIED.);
#2333=B_SPLINE_SURFACE_WITH_KNOTS('',3,3,((#71781,#71782,#71783,#71784),
(#71785,#71786,#71787,#71788),(#71789,#71790,#71791,#71792),(#71793,#71794,
#71795,#71796)),.UNSPECIFIED.,.F.,.F.,.F.,(4,4),(4,4),(-0.00600003962543891,
1.00000000356508),(0.0166015299238274,0.0265907346180633),.UNSPECIFIED.);
#2334=B_SPLINE_SURFACE_WITH_KNOTS('',3,3,((#71808,#71809,#71810,#71811),
(#71812,#71813,#71814,#71815),(#71816,#71817,#71818,#71819),(#71820,#71821,
#71822,#71823)),.UNSPECIFIED.,.F.,.F.,.F.,(4,4),(4,4),(0.522097120208868,
1.00286780410463),(0.0200175229646521,0.0265907346180646),.UNSPECIFIED.);
#2335=B_SPLINE_SURFACE_WITH_KNOTS('',3,3,((#71879,#71880,#71881,#71882),
(#71883,#71884,#71885,#71886),(#71887,#71888,#71889,#71890),(#71891,#71892,
#71893,#71894)),.UNSPECIFIED.,.F.,.F.,.F.,(4,4),(4,4),(0.522097120208733,
1.00286791014268),(0.0100271466749324,0.0166015302184277),.UNSPECIFIED.);
#2336=B_SPLINE_SURFACE_WITH_KNOTS('',3,3,((#71920,#71921,#71922,#71923),
(#71924,#71925,#71926,#71927),(#71928,#71929,#71930,#71931),(#71932,#71933,
#71934,#71935)),.UNSPECIFIED.,.F.,.F.,.F.,(4,4),(4,4),(-0.000171895441749836,
1.00600020634798),(0.0665898698856038,0.0751325481196475),.UNSPECIFIED.);
#2337=B_SPLINE_SURFACE_WITH_KNOTS('',3,3,((#71951,#71952,#71953,#71954),
(#71955,#71956,#71957,#71958),(#71959,#71960,#71961,#71962),(#71963,#71964,
#71965,#71966)),.UNSPECIFIED.,.F.,.F.,.F.,(4,4),(4,4),(-0.00286833998593411,
0.477902879786537),(0.0665898698862503,0.0731716198748497),
 .UNSPECIFIED.);
#2338=B_SPLINE_SURFACE_WITH_KNOTS('',3,3,((#72000,#72001,#72002,#72003),
(#72004,#72005,#72006,#72007),(#72008,#72009,#72010,#72011),(#72012,#72013,
#72014,#72015)),.UNSPECIFIED.,.F.,.F.,.F.,(4,4),(4,4),(0.5220971202086,
1.00286791825529),(0.0600156865486942,0.0665898700060152),.UNSPECIFIED.);
#2339=B_SPLINE_SURFACE_WITH_KNOTS('',3,3,((#72025,#72026,#72027,#72028),
(#72029,#72030,#72031,#72032),(#72033,#72034,#72035,#72036),(#72037,#72038,
#72039,#72040)),.UNSPECIFIED.,.F.,.F.,.F.,(4,4),(4,4),(-0.00286764392031674,
0.477902879786535),(0.05659971331012,0.0631721430887066),.UNSPECIFIED.);
#2340=B_SPLINE_SURFACE_WITH_KNOTS('',3,3,((#72077,#72078,#72079,#72080),
(#72081,#72082,#72083,#72084),(#72085,#72086,#72087,#72088),(#72089,#72090,
#72091,#72092)),.UNSPECIFIED.,.F.,.F.,.F.,(4,4),(4,4),(0.522097120209359,
1.00286780122188),(0.0500263550858677,0.0565997133101425),.UNSPECIFIED.);
#2341=B_SPLINE_SURFACE_WITH_KNOTS('',3,3,((#72164,#72165,#72166,#72167),
(#72168,#72169,#72170,#72171),(#72172,#72173,#72174,#72175),(#72176,#72177,
#72178,#72179)),.UNSPECIFIED.,.F.,.F.,.F.,(4,4),(4,4),(0.522097120208958,
1.00286848452566),(0.0400218729465711,0.0466073985929456),.UNSPECIFIED.);
#2342=B_SPLINE_SURFACE_WITH_KNOTS('',3,3,((#72248,#72249,#72250,#72251),
(#72252,#72253,#72254,#72255),(#72256,#72257,#72258,#72259),(#72260,#72261,
#72262,#72263)),.UNSPECIFIED.,.F.,.F.,.F.,(4,4),(4,4),(0.52209712020823,
1.00286862201158),(0.0300094532292163,0.0365944846647038),.UNSPECIFIED.);
#2343=B_SPLINE_SURFACE_WITH_KNOTS('',3,3,((#72296,#72297,#72298,#72299),
(#72300,#72301,#72302,#72303),(#72304,#72305,#72306,#72307),(#72308,#72309,
#72310,#72311)),.UNSPECIFIED.,.F.,.F.,.F.,(4,4),(4,4),(-0.00600003961876303,
1.00000000246915),(0.0166015299238274,0.0265907346180639),.UNSPECIFIED.);
#2344=B_SPLINE_SURFACE_WITH_KNOTS('',3,3,((#72323,#72324,#72325,#72326),
(#72327,#72328,#72329,#72330),(#72331,#72332,#72333,#72334),(#72335,#72336,
#72337,#72338)),.UNSPECIFIED.,.F.,.F.,.F.,(4,4),(4,4),(0.52209712020903,
1.00286780410459),(0.0200175229646514,0.0265907346180651),.UNSPECIFIED.);
#2345=B_SPLINE_SURFACE_WITH_KNOTS('',3,3,((#72394,#72395,#72396,#72397),
(#72398,#72399,#72400,#72401),(#72402,#72403,#72404,#72405),(#72406,#72407,
#72408,#72409)),.UNSPECIFIED.,.F.,.F.,.F.,(4,4),(4,4),(0.522097120208794,
1.00286791014255),(0.0100271466749329,0.0166015302184292),.UNSPECIFIED.);
#2346=B_SPLINE_SURFACE_WITH_KNOTS('',3,3,((#72435,#72436,#72437,#72438),
(#72439,#72440,#72441,#72442),(#72443,#72444,#72445,#72446),(#72447,#72448,
#72449,#72450)),.UNSPECIFIED.,.F.,.F.,.F.,(4,4),(4,4),(-0.000171895441761731,
1.00600020634806),(0.0665898698856041,0.0751325481196596),.UNSPECIFIED.);
#2347=B_SPLINE_SURFACE_WITH_KNOTS('',3,3,((#72466,#72467,#72468,#72469),
(#72470,#72471,#72472,#72473),(#72474,#72475,#72476,#72477),(#72478,#72479,
#72480,#72481)),.UNSPECIFIED.,.F.,.F.,.F.,(4,4),(4,4),(-0.00286833998590083,
0.477902879786522),(0.0665898698862503,0.0731716198748499),
 .UNSPECIFIED.);
#2348=B_SPLINE_SURFACE_WITH_KNOTS('',3,3,((#72515,#72516,#72517,#72518),
(#72519,#72520,#72521,#72522),(#72523,#72524,#72525,#72526),(#72527,#72528,
#72529,#72530)),.UNSPECIFIED.,.F.,.F.,.F.,(4,4),(4,4),(0.522097120208708,
1.00286791825529),(0.060015686548694,0.0665898700060155),.UNSPECIFIED.);
#2349=B_SPLINE_SURFACE_WITH_KNOTS('',3,3,((#72540,#72541,#72542,#72543),
(#72544,#72545,#72546,#72547),(#72548,#72549,#72550,#72551),(#72552,#72553,
#72554,#72555)),.UNSPECIFIED.,.F.,.F.,.F.,(4,4),(4,4),(-0.00286764392027188,
0.477902879786551),(0.0565997133101198,0.0631721430887068),
 .UNSPECIFIED.);
#2350=B_SPLINE_SURFACE_WITH_KNOTS('',3,3,((#72592,#72593,#72594,#72595),
(#72596,#72597,#72598,#72599),(#72600,#72601,#72602,#72603),(#72604,#72605,
#72606,#72607)),.UNSPECIFIED.,.F.,.F.,.F.,(4,4),(4,4),(0.522097120209487,
1.00286780122187),(0.0500263550858668,0.0565997133101425),.UNSPECIFIED.);
#2351=B_SPLINE_SURFACE_WITH_KNOTS('',3,3,((#72679,#72680,#72681,#72682),
(#72683,#72684,#72685,#72686),(#72687,#72688,#72689,#72690),(#72691,#72692,
#72693,#72694)),.UNSPECIFIED.,.F.,.F.,.F.,(4,4),(4,4),(0.522097120209154,
1.00286848452568),(0.04002187294657,0.0466073985929447),.UNSPECIFIED.);
#2352=B_SPLINE_SURFACE_WITH_KNOTS('',3,3,((#72763,#72764,#72765,#72766),
(#72767,#72768,#72769,#72770),(#72771,#72772,#72773,#72774),(#72775,#72776,
#72777,#72778)),.UNSPECIFIED.,.F.,.F.,.F.,(4,4),(4,4),(0.522097120208207,
1.00286862201156),(0.0300094532292159,0.0365944846647044),.UNSPECIFIED.);
#2353=B_SPLINE_SURFACE_WITH_KNOTS('',3,3,((#72811,#72812,#72813,#72814),
(#72815,#72816,#72817,#72818),(#72819,#72820,#72821,#72822),(#72823,#72824,
#72825,#72826)),.UNSPECIFIED.,.F.,.F.,.F.,(4,4),(4,4),(-0.00600003961874595,
1.00000000246929),(0.0166015299238277,0.0265907346180653),.UNSPECIFIED.);
#2354=B_SPLINE_SURFACE_WITH_KNOTS('',3,3,((#72838,#72839,#72840,#72841),
(#72842,#72843,#72844,#72845),(#72846,#72847,#72848,#72849),(#72850,#72851,
#72852,#72853)),.UNSPECIFIED.,.F.,.F.,.F.,(4,4),(4,4),(0.522097120209191,
1.00286780410462),(0.0200175229646514,0.026590734618065),.UNSPECIFIED.);
#2355=B_SPLINE_SURFACE_WITH_KNOTS('',3,3,((#72909,#72910,#72911,#72912),
(#72913,#72914,#72915,#72916),(#72917,#72918,#72919,#72920),(#72921,#72922,
#72923,#72924)),.UNSPECIFIED.,.F.,.F.,.F.,(4,4),(4,4),(0.522097120208983,
1.00286791014259),(0.0100271466749312,0.0166015302184277),.UNSPECIFIED.);
#2356=B_SPLINE_SURFACE_WITH_KNOTS('',3,3,((#72950,#72951,#72952,#72953),
(#72954,#72955,#72956,#72957),(#72958,#72959,#72960,#72961),(#72962,#72963,
#72964,#72965)),.UNSPECIFIED.,.F.,.F.,.F.,(4,4),(4,4),(-0.000171895441537365,
1.00600020634792),(0.0665898698856057,0.0751325481194348),.UNSPECIFIED.);
#2357=B_SPLINE_SURFACE_WITH_KNOTS('',3,3,((#72981,#72982,#72983,#72984),
(#72985,#72986,#72987,#72988),(#72989,#72990,#72991,#72992),(#72993,#72994,
#72995,#72996)),.UNSPECIFIED.,.F.,.F.,.F.,(4,4),(4,4),(-0.00286833998593498,
0.477902879786539),(0.0665898698862505,0.073171619874851),.UNSPECIFIED.);
#2358=B_SPLINE_SURFACE_WITH_KNOTS('',3,3,((#73030,#73031,#73032,#73033),
(#73034,#73035,#73036,#73037),(#73038,#73039,#73040,#73041),(#73042,#73043,
#73044,#73045)),.UNSPECIFIED.,.F.,.F.,.F.,(4,4),(4,4),(0.52209712020883,
1.00286791825528),(0.0600156865486942,0.0665898700060142),.UNSPECIFIED.);
#2359=B_SPLINE_SURFACE_WITH_KNOTS('',3,3,((#73055,#73056,#73057,#73058),
(#73059,#73060,#73061,#73062),(#73063,#73064,#73065,#73066),(#73067,#73068,
#73069,#73070)),.UNSPECIFIED.,.F.,.F.,.F.,(4,4),(4,4),(-0.00286764392029753,
0.47790287978651),(0.0565997133101198,0.0631721430887059),.UNSPECIFIED.);
#2360=B_SPLINE_SURFACE_WITH_KNOTS('',3,3,((#73104,#73105,#73106,#73107),
(#73108,#73109,#73110,#73111),(#73112,#73113,#73114,#73115),(#73116,#73117,
#73118,#73119)),.UNSPECIFIED.,.F.,.F.,.F.,(4,4),(4,4),(0.522097120209604,
1.0028678012218),(0.0500263550858673,0.0565997133101429),.UNSPECIFIED.);
#2361=B_SPLINE_SURFACE_WITH_KNOTS('',3,3,((#73127,#73128,#73129,#73130),
(#73131,#73132,#73133,#73134),(#73135,#73136,#73137,#73138),(#73139,#73140,
#73141,#73142)),.UNSPECIFIED.,.F.,.F.,.F.,(4,4),(4,4),(-0.00286810177351708,
0.477902879786512),(0.0466073985929107,0.0531834933545498),
 .UNSPECIFIED.);
#2362=B_SPLINE_SURFACE_WITH_KNOTS('',3,3,((#73198,#73199,#73200,#73201),
(#73202,#73203,#73204,#73205),(#73206,#73207,#73208,#73209),(#73210,#73211,
#73212,#73213)),.UNSPECIFIED.,.F.,.F.,.F.,(4,4),(4,4),(0.522097120209231,
1.00286848452578),(0.0400218729465709,0.0466073985929455),.UNSPECIFIED.);
#2363=B_SPLINE_SURFACE_WITH_KNOTS('',3,3,((#73282,#73283,#73284,#73285),
(#73286,#73287,#73288,#73289),(#73290,#73291,#73292,#73293),(#73294,#73295,
#73296,#73297)),.UNSPECIFIED.,.F.,.F.,.F.,(4,4),(4,4),(0.522097120208532,
1.00286862201161),(0.0300094532292161,0.0365944846647031),.UNSPECIFIED.);
#2364=B_SPLINE_SURFACE_WITH_KNOTS('',3,3,((#73330,#73331,#73332,#73333),
(#73334,#73335,#73336,#73337),(#73338,#73339,#73340,#73341),(#73342,#73343,
#73344,#73345)),.UNSPECIFIED.,.F.,.F.,.F.,(4,4),(4,4),(-0.00600003961854877,
1.0000000024688),(0.0166015299238285,0.0265907346180647),.UNSPECIFIED.);
#2365=B_SPLINE_SURFACE_WITH_KNOTS('',3,3,((#73357,#73358,#73359,#73360),
(#73361,#73362,#73363,#73364),(#73365,#73366,#73367,#73368),(#73369,#73370,
#73371,#73372)),.UNSPECIFIED.,.F.,.F.,.F.,(4,4),(4,4),(0.522097120209233,
1.00286780410459),(0.020017522964652,0.026590734618065),.UNSPECIFIED.);
#2366=B_SPLINE_SURFACE_WITH_KNOTS('',3,3,((#73428,#73429,#73430,#73431),
(#73432,#73433,#73434,#73435),(#73436,#73437,#73438,#73439),(#73440,#73441,
#73442,#73443)),.UNSPECIFIED.,.F.,.F.,.F.,(4,4),(4,4),(0.522097120209193,
1.00286791014268),(0.0100271466749299,0.0166015302184267),.UNSPECIFIED.);
#2367=B_SPLINE_SURFACE_WITH_KNOTS('',3,3,((#73469,#73470,#73471,#73472),
(#73473,#73474,#73475,#73476),(#73477,#73478,#73479,#73480),(#73481,#73482,
#73483,#73484)),.UNSPECIFIED.,.F.,.F.,.F.,(4,4),(4,4),(-0.000171895441178554,
1.00600020634866),(0.0665898698856039,0.0751325481190739),.UNSPECIFIED.);
#2368=B_SPLINE_SURFACE_WITH_KNOTS('',3,3,((#73500,#73501,#73502,#73503),
(#73504,#73505,#73506,#73507),(#73508,#73509,#73510,#73511),(#73512,#73513,
#73514,#73515)),.UNSPECIFIED.,.F.,.F.,.F.,(4,4),(4,4),(-0.00286833998589992,
0.477902879786536),(0.066589869886251,0.0731716198748508),.UNSPECIFIED.);
#2369=B_SPLINE_SURFACE_WITH_KNOTS('',3,3,((#73549,#73550,#73551,#73552),
(#73553,#73554,#73555,#73556),(#73557,#73558,#73559,#73560),(#73561,#73562,
#73563,#73564)),.UNSPECIFIED.,.F.,.F.,.F.,(4,4),(4,4),(0.522097120208903,
1.00286791825528),(0.0600156865486934,0.0665898700060148),.UNSPECIFIED.);
#2370=B_SPLINE_SURFACE_WITH_KNOTS('',3,3,((#73574,#73575,#73576,#73577),
(#73578,#73579,#73580,#73581),(#73582,#73583,#73584,#73585),(#73586,#73587,
#73588,#73589)),.UNSPECIFIED.,.F.,.F.,.F.,(4,4),(4,4),(-0.00286764392025972,
0.477902879786554),(0.0565997133101205,0.0631721430887069),
 .UNSPECIFIED.);
#2371=B_SPLINE_SURFACE_WITH_KNOTS('',3,3,((#73626,#73627,#73628,#73629),
(#73630,#73631,#73632,#73633),(#73634,#73635,#73636,#73637),(#73638,#73639,
#73640,#73641)),.UNSPECIFIED.,.F.,.F.,.F.,(4,4),(4,4),(0.52209712020971,
1.00286780122195),(0.0500263550858671,0.0565997133101426),.UNSPECIFIED.);
#2372=B_SPLINE_SURFACE_WITH_KNOTS('',3,3,((#73713,#73714,#73715,#73716),
(#73717,#73718,#73719,#73720),(#73721,#73722,#73723,#73724),(#73725,#73726,
#73727,#73728)),.UNSPECIFIED.,.F.,.F.,.F.,(4,4),(4,4),(0.522097120209253,
1.0028684845256),(0.0400218729465702,0.046607398592945),.UNSPECIFIED.);
#2373=B_SPLINE_SURFACE_WITH_KNOTS('',3,3,((#73797,#73798,#73799,#73800),
(#73801,#73802,#73803,#73804),(#73805,#73806,#73807,#73808),(#73809,#73810,
#73811,#73812)),.UNSPECIFIED.,.F.,.F.,.F.,(4,4),(4,4),(0.52209712020847,
1.00286862201149),(0.0300094532292159,0.0365944846647042),.UNSPECIFIED.);
#2374=B_SPLINE_SURFACE_WITH_KNOTS('',3,3,((#73845,#73846,#73847,#73848),
(#73849,#73850,#73851,#73852),(#73853,#73854,#73855,#73856),(#73857,#73858,
#73859,#73860)),.UNSPECIFIED.,.F.,.F.,.F.,(4,4),(4,4),(-0.00600003961872756,
1.00000000246921),(0.0166015299238287,0.026590734618063),.UNSPECIFIED.);
#2375=B_SPLINE_SURFACE_WITH_KNOTS('',3,3,((#73872,#73873,#73874,#73875),
(#73876,#73877,#73878,#73879),(#73880,#73881,#73882,#73883),(#73884,#73885,
#73886,#73887)),.UNSPECIFIED.,.F.,.F.,.F.,(4,4),(4,4),(0.522097120209441,
1.00286780410464),(0.0200175229646508,0.0265907346180652),.UNSPECIFIED.);
#2376=B_SPLINE_SURFACE_WITH_KNOTS('',3,3,((#73943,#73944,#73945,#73946),
(#73947,#73948,#73949,#73950),(#73951,#73952,#73953,#73954),(#73955,#73956,
#73957,#73958)),.UNSPECIFIED.,.F.,.F.,.F.,(4,4),(4,4),(0.522097120209274,
1.00286791014271),(0.0100271466749308,0.0166015302184272),.UNSPECIFIED.);
#2377=B_SPLINE_SURFACE_WITH_KNOTS('',3,3,((#73984,#73985,#73986,#73987),
(#73988,#73989,#73990,#73991),(#73992,#73993,#73994,#73995),(#73996,#73997,
#73998,#73999)),.UNSPECIFIED.,.F.,.F.,.F.,(4,4),(4,4),(-0.000171895440844185,
1.00600020634819),(0.0665898698856036,0.0751325481187421),.UNSPECIFIED.);
#2378=B_SPLINE_SURFACE_WITH_KNOTS('',3,3,((#74015,#74016,#74017,#74018),
(#74019,#74020,#74021,#74022),(#74023,#74024,#74025,#74026),(#74027,#74028,
#74029,#74030)),.UNSPECIFIED.,.F.,.F.,.F.,(4,4),(4,4),(-0.00286833998589259,
0.477902879786537),(0.0665898698862502,0.0731716198748502),
 .UNSPECIFIED.);
#2379=B_SPLINE_SURFACE_WITH_KNOTS('',3,3,((#74064,#74065,#74066,#74067),
(#74068,#74069,#74070,#74071),(#74072,#74073,#74074,#74075),(#74076,#74077,
#74078,#74079)),.UNSPECIFIED.,.F.,.F.,.F.,(4,4),(4,4),(0.522097120208998,
1.0028679182553),(0.0600156865486937,0.0665898700060142),.UNSPECIFIED.);
#2380=B_SPLINE_SURFACE_WITH_KNOTS('',3,3,((#74089,#74090,#74091,#74092),
(#74093,#74094,#74095,#74096),(#74097,#74098,#74099,#74100),(#74101,#74102,
#74103,#74104)),.UNSPECIFIED.,.F.,.F.,.F.,(4,4),(4,4),(-0.00286764392026813,
0.477902879786526),(0.0565997133101208,0.0631721430887064),
 .UNSPECIFIED.);
#2381=B_SPLINE_SURFACE_WITH_KNOTS('',3,3,((#74141,#74142,#74143,#74144),
(#74145,#74146,#74147,#74148),(#74149,#74150,#74151,#74152),(#74153,#74154,
#74155,#74156)),.UNSPECIFIED.,.F.,.F.,.F.,(4,4),(4,4),(0.522097120209777,
1.00286780122189),(0.0500263550858672,0.0565997133101431),.UNSPECIFIED.);
#2382=B_SPLINE_SURFACE_WITH_KNOTS('',3,3,((#74228,#74229,#74230,#74231),
(#74232,#74233,#74234,#74235),(#74236,#74237,#74238,#74239),(#74240,#74241,
#74242,#74243)),.UNSPECIFIED.,.F.,.F.,.F.,(4,4),(4,4),(0.522097120209504,
1.00286848452574),(0.0400218729465704,0.046607398592945),.UNSPECIFIED.);
#2383=B_SPLINE_SURFACE_WITH_KNOTS('',3,3,((#74312,#74313,#74314,#74315),
(#74316,#74317,#74318,#74319),(#74320,#74321,#74322,#74323),(#74324,#74325,
#74326,#74327)),.UNSPECIFIED.,.F.,.F.,.F.,(4,4),(4,4),(0.52209712020866,
1.00286862201146),(0.0300094532292161,0.0365944846647038),.UNSPECIFIED.);
#2384=B_SPLINE_SURFACE_WITH_KNOTS('',3,3,((#74360,#74361,#74362,#74363),
(#74364,#74365,#74366,#74367),(#74368,#74369,#74370,#74371),(#74372,#74373,
#74374,#74375)),.UNSPECIFIED.,.F.,.F.,.F.,(4,4),(4,4),(-0.00600003961858661,
1.00000000246924),(0.0166015299238286,0.0265907346180638),.UNSPECIFIED.);
#2385=B_SPLINE_SURFACE_WITH_KNOTS('',3,3,((#74387,#74388,#74389,#74390),
(#74391,#74392,#74393,#74394),(#74395,#74396,#74397,#74398),(#74399,#74400,
#74401,#74402)),.UNSPECIFIED.,.F.,.F.,.F.,(4,4),(4,4),(0.522097120209524,
1.00286780410468),(0.020017522964651,0.0265907346180651),.UNSPECIFIED.);
#2386=B_SPLINE_SURFACE_WITH_KNOTS('',3,3,((#74458,#74459,#74460,#74461),
(#74462,#74463,#74464,#74465),(#74466,#74467,#74468,#74469),(#74470,#74471,
#74472,#74473)),.UNSPECIFIED.,.F.,.F.,.F.,(4,4),(4,4),(0.522097120209415,
1.00286791014287),(0.0100271466749306,0.0166015302184268),.UNSPECIFIED.);
#2387=B_SPLINE_SURFACE_WITH_KNOTS('',3,3,((#74499,#74500,#74501,#74502),
(#74503,#74504,#74505,#74506),(#74507,#74508,#74509,#74510),(#74511,#74512,
#74513,#74514)),.UNSPECIFIED.,.F.,.F.,.F.,(4,4),(4,4),(-0.000171895440408026,
1.0060002063483),(0.0665898698856056,0.0751325481183052),.UNSPECIFIED.);
#2388=B_SPLINE_SURFACE_WITH_KNOTS('',3,3,((#74530,#74531,#74532,#74533),
(#74534,#74535,#74536,#74537),(#74538,#74539,#74540,#74541),(#74542,#74543,
#74544,#74545)),.UNSPECIFIED.,.F.,.F.,.F.,(4,4),(4,4),(-0.00286833998588494,
0.477902879786516),(0.0665898698862518,0.0731716198748496),
 .UNSPECIFIED.);
#2389=B_SPLINE_SURFACE_WITH_KNOTS('',3,3,((#74579,#74580,#74581,#74582),
(#74583,#74584,#74585,#74586),(#74587,#74588,#74589,#74590),(#74591,#74592,
#74593,#74594)),.UNSPECIFIED.,.F.,.F.,.F.,(4,4),(4,4),(0.522097120209113,
1.00286791825532),(0.0600156865486933,0.066589870006014),.UNSPECIFIED.);
#2390=B_SPLINE_SURFACE_WITH_KNOTS('',3,3,((#74604,#74605,#74606,#74607),
(#74608,#74609,#74610,#74611),(#74612,#74613,#74614,#74615),(#74616,#74617,
#74618,#74619)),.UNSPECIFIED.,.F.,.F.,.F.,(4,4),(4,4),(-0.00286764392025136,
0.47790287978653),(0.0565997133101204,0.0631721430887062),.UNSPECIFIED.);
#2391=B_SPLINE_SURFACE_WITH_KNOTS('',3,3,((#74656,#74657,#74658,#74659),
(#74660,#74661,#74662,#74663),(#74664,#74665,#74666,#74667),(#74668,#74669,
#74670,#74671)),.UNSPECIFIED.,.F.,.F.,.F.,(4,4),(4,4),(0.52209712020994,
1.0028678012219),(0.0500263550858669,0.0565997133101416),.UNSPECIFIED.);
#2392=B_SPLINE_SURFACE_WITH_KNOTS('',3,3,((#74743,#74744,#74745,#74746),
(#74747,#74748,#74749,#74750),(#74751,#74752,#74753,#74754),(#74755,#74756,
#74757,#74758)),.UNSPECIFIED.,.F.,.F.,.F.,(4,4),(4,4),(0.522097120209583,
1.00286848452588),(0.0400218729465702,0.0466073985929453),.UNSPECIFIED.);
#2393=B_SPLINE_SURFACE_WITH_KNOTS('',3,3,((#74827,#74828,#74829,#74830),
(#74831,#74832,#74833,#74834),(#74835,#74836,#74837,#74838),(#74839,#74840,
#74841,#74842)),.UNSPECIFIED.,.F.,.F.,.F.,(4,4),(4,4),(0.522097120208653,
1.0028686220115),(0.0300094532292165,0.0365944846647038),.UNSPECIFIED.);
#2394=B_SPLINE_SURFACE_WITH_KNOTS('',3,3,((#74875,#74876,#74877,#74878),
(#74879,#74880,#74881,#74882),(#74883,#74884,#74885,#74886),(#74887,#74888,
#74889,#74890)),.UNSPECIFIED.,.F.,.F.,.F.,(4,4),(4,4),(-0.00600003961854107,
1.00000000246902),(0.0166015299238288,0.0265907346180632),.UNSPECIFIED.);
#2395=B_SPLINE_SURFACE_WITH_KNOTS('',3,3,((#74902,#74903,#74904,#74905),
(#74906,#74907,#74908,#74909),(#74910,#74911,#74912,#74913),(#74914,#74915,
#74916,#74917)),.UNSPECIFIED.,.F.,.F.,.F.,(4,4),(4,4),(0.522097120209538,
1.00286780410455),(0.0200175229646514,0.0265907346180652),.UNSPECIFIED.);
#2396=B_SPLINE_SURFACE_WITH_KNOTS('',3,3,((#74973,#74974,#74975,#74976),
(#74977,#74978,#74979,#74980),(#74981,#74982,#74983,#74984),(#74985,#74986,
#74987,#74988)),.UNSPECIFIED.,.F.,.F.,.F.,(4,4),(4,4),(0.522097120209429,
1.00286791014269),(0.0100271466749311,0.0166015302184276),.UNSPECIFIED.);
#2397=B_SPLINE_SURFACE_WITH_KNOTS('',3,3,((#75014,#75015,#75016,#75017),
(#75018,#75019,#75020,#75021),(#75022,#75023,#75024,#75025),(#75026,#75027,
#75028,#75029)),.UNSPECIFIED.,.F.,.F.,.F.,(4,4),(4,4),(-0.000171895439675098,
1.00600020634843),(0.0665898698856039,0.0751325481175709),.UNSPECIFIED.);
#2398=B_SPLINE_SURFACE_WITH_KNOTS('',3,3,((#75045,#75046,#75047,#75048),
(#75049,#75050,#75051,#75052),(#75053,#75054,#75055,#75056),(#75057,#75058,
#75059,#75060)),.UNSPECIFIED.,.F.,.F.,.F.,(4,4),(4,4),(-0.00286833998592894,
0.477902879786575),(0.0665898698862504,0.0731716198748503),
 .UNSPECIFIED.);
#2399=B_SPLINE_SURFACE_WITH_KNOTS('',3,3,((#75094,#75095,#75096,#75097),
(#75098,#75099,#75100,#75101),(#75102,#75103,#75104,#75105),(#75106,#75107,
#75108,#75109)),.UNSPECIFIED.,.F.,.F.,.F.,(4,4),(4,4),(0.52209712020939,
1.00286791825516),(0.0600156865486937,0.0665898700060151),.UNSPECIFIED.);
#2400=B_SPLINE_SURFACE_WITH_KNOTS('',3,3,((#75119,#75120,#75121,#75122),
(#75123,#75124,#75125,#75126),(#75127,#75128,#75129,#75130),(#75131,#75132,
#75133,#75134)),.UNSPECIFIED.,.F.,.F.,.F.,(4,4),(4,4),(-0.00286764392024561,
0.47790287978655),(0.0565997133101205,0.0631721430887062),.UNSPECIFIED.);
#2401=B_SPLINE_SURFACE_WITH_KNOTS('',3,3,((#75171,#75172,#75173,#75174),
(#75175,#75176,#75177,#75178),(#75179,#75180,#75181,#75182),(#75183,#75184,
#75185,#75186)),.UNSPECIFIED.,.F.,.F.,.F.,(4,4),(4,4),(0.522097120210138,
1.00286780122168),(0.0500263550858672,0.0565997133101423),.UNSPECIFIED.);
#2402=B_SPLINE_SURFACE_WITH_KNOTS('',3,3,((#75258,#75259,#75260,#75261),
(#75262,#75263,#75264,#75265),(#75266,#75267,#75268,#75269),(#75270,#75271,
#75272,#75273)),.UNSPECIFIED.,.F.,.F.,.F.,(4,4),(4,4),(0.522097120209848,
1.00286848452586),(0.0400218729465692,0.0466073985929449),.UNSPECIFIED.);
#2403=B_SPLINE_SURFACE_WITH_KNOTS('',3,3,((#75342,#75343,#75344,#75345),
(#75346,#75347,#75348,#75349),(#75350,#75351,#75352,#75353),(#75354,#75355,
#75356,#75357)),.UNSPECIFIED.,.F.,.F.,.F.,(4,4),(4,4),(0.52209712020886,
1.00286862201148),(0.0300094532292159,0.0365944846647037),.UNSPECIFIED.);
#2404=B_SPLINE_SURFACE_WITH_KNOTS('',3,3,((#75390,#75391,#75392,#75393),
(#75394,#75395,#75396,#75397),(#75398,#75399,#75400,#75401),(#75402,#75403,
#75404,#75405)),.UNSPECIFIED.,.F.,.F.,.F.,(4,4),(4,4),(-0.00600003961852695,
1.0000000024693),(0.0166015299238276,0.0265907346180643),.UNSPECIFIED.);
#2405=B_SPLINE_SURFACE_WITH_KNOTS('',3,3,((#75417,#75418,#75419,#75420),
(#75421,#75422,#75423,#75424),(#75425,#75426,#75427,#75428),(#75429,#75430,
#75431,#75432)),.UNSPECIFIED.,.F.,.F.,.F.,(4,4),(4,4),(0.522097120209692,
1.00286780410451),(0.0200175229646511,0.0265907346180654),.UNSPECIFIED.);
#2406=B_SPLINE_SURFACE_WITH_KNOTS('',3,3,((#75488,#75489,#75490,#75491),
(#75492,#75493,#75494,#75495),(#75496,#75497,#75498,#75499),(#75500,#75501,
#75502,#75503)),.UNSPECIFIED.,.F.,.F.,.F.,(4,4),(4,4),(0.522097120209553,
1.00286791014263),(0.0100271466749314,0.0166015302184278),.UNSPECIFIED.);
#2407=B_SPLINE_SURFACE_WITH_KNOTS('',3,3,((#75529,#75530,#75531,#75532),
(#75533,#75534,#75535,#75536),(#75537,#75538,#75539,#75540),(#75541,#75542,
#75543,#75544)),.UNSPECIFIED.,.F.,.F.,.F.,(4,4),(4,4),(-0.000171895438814887,
1.00600020634805),(0.0665898698856055,0.0751325481167114),.UNSPECIFIED.);
#2408=B_SPLINE_SURFACE_WITH_KNOTS('',3,3,((#75560,#75561,#75562,#75563),
(#75564,#75565,#75566,#75567),(#75568,#75569,#75570,#75571),(#75572,#75573,
#75574,#75575)),.UNSPECIFIED.,.F.,.F.,.F.,(4,4),(4,4),(-0.00286833998585249,
0.477902879786554),(0.0665898698862516,0.0731716198748504),
 .UNSPECIFIED.);
#2409=B_SPLINE_SURFACE_WITH_KNOTS('',3,3,((#75609,#75610,#75611,#75612),
(#75613,#75614,#75615,#75616),(#75617,#75618,#75619,#75620),(#75621,#75622,
#75623,#75624)),.UNSPECIFIED.,.F.,.F.,.F.,(4,4),(4,4),(0.522097120209408,
1.00286791825511),(0.0600156865486939,0.0665898700060147),.UNSPECIFIED.);
#2410=B_SPLINE_SURFACE_WITH_KNOTS('',3,3,((#75634,#75635,#75636,#75637),
(#75638,#75639,#75640,#75641),(#75642,#75643,#75644,#75645),(#75646,#75647,
#75648,#75649)),.UNSPECIFIED.,.F.,.F.,.F.,(4,4),(4,4),(-0.00286764392030078,
0.477902879786555),(0.0565997133101203,0.0631721430887069),
 .UNSPECIFIED.);
#2411=B_SPLINE_SURFACE_WITH_KNOTS('',3,3,((#75683,#75684,#75685,#75686),
(#75687,#75688,#75689,#75690),(#75691,#75692,#75693,#75694),(#75695,#75696,
#75697,#75698)),.UNSPECIFIED.,.F.,.F.,.F.,(4,4),(4,4),(0.522097120210099,
1.00286780122183),(0.050026355085867,0.0565997133101419),.UNSPECIFIED.);
#2412=B_SPLINE_SURFACE_WITH_KNOTS('',3,3,((#75706,#75707,#75708,#75709),
(#75710,#75711,#75712,#75713),(#75714,#75715,#75716,#75717),(#75718,#75719,
#75720,#75721)),.UNSPECIFIED.,.F.,.F.,.F.,(4,4),(4,4),(-0.00286810177325765,
0.477902879786541),(0.0466073985929107,0.05318349335455),.UNSPECIFIED.);
#2413=B_SPLINE_SURFACE_WITH_KNOTS('',3,3,((#75777,#75778,#75779,#75780),
(#75781,#75782,#75783,#75784),(#75785,#75786,#75787,#75788),(#75789,#75790,
#75791,#75792)),.UNSPECIFIED.,.F.,.F.,.F.,(4,4),(4,4),(0.522097120209848,
1.00286848452562),(0.0400218729465703,0.0466073985929447),.UNSPECIFIED.);
#2414=B_SPLINE_SURFACE_WITH_KNOTS('',3,3,((#75861,#75862,#75863,#75864),
(#75865,#75866,#75867,#75868),(#75869,#75870,#75871,#75872),(#75873,#75874,
#75875,#75876)),.UNSPECIFIED.,.F.,.F.,.F.,(4,4),(4,4),(0.522097120209105,
1.00286862201146),(0.0300094532292165,0.0365944846647027),.UNSPECIFIED.);
#2415=B_SPLINE_SURFACE_WITH_KNOTS('',3,3,((#75909,#75910,#75911,#75912),
(#75913,#75914,#75915,#75916),(#75917,#75918,#75919,#75920),(#75921,#75922,
#75923,#75924)),.UNSPECIFIED.,.F.,.F.,.F.,(4,4),(4,4),(-0.006000039618303,
1.00000000246901),(0.0166015299238286,0.026590734618064),.UNSPECIFIED.);
#2416=B_SPLINE_SURFACE_WITH_KNOTS('',3,3,((#75936,#75937,#75938,#75939),
(#75940,#75941,#75942,#75943),(#75944,#75945,#75946,#75947),(#75948,#75949,
#75950,#75951)),.UNSPECIFIED.,.F.,.F.,.F.,(4,4),(4,4),(0.522097120209899,
1.00286780410473),(0.0200175229646523,0.0265907346180642),.UNSPECIFIED.);
#2417=B_SPLINE_SURFACE_WITH_KNOTS('',3,3,((#76007,#76008,#76009,#76010),
(#76011,#76012,#76013,#76014),(#76015,#76016,#76017,#76018),(#76019,#76020,
#76021,#76022)),.UNSPECIFIED.,.F.,.F.,.F.,(4,4),(4,4),(0.5220971202096,
1.00286791014285),(0.0100271466749314,0.0166015302184275),.UNSPECIFIED.);
#2418=B_SPLINE_SURFACE_WITH_KNOTS('',3,3,((#76048,#76049,#76050,#76051),
(#76052,#76053,#76054,#76055),(#76056,#76057,#76058,#76059),(#76060,#76061,
#76062,#76063)),.UNSPECIFIED.,.F.,.F.,.F.,(4,4),(4,4),(-0.000171895438212527,
1.00600020634832),(0.0665898698856039,0.0751325481161105),.UNSPECIFIED.);
#2419=B_SPLINE_SURFACE_WITH_KNOTS('',3,3,((#76079,#76080,#76081,#76082),
(#76083,#76084,#76085,#76086),(#76087,#76088,#76089,#76090),(#76091,#76092,
#76093,#76094)),.UNSPECIFIED.,.F.,.F.,.F.,(4,4),(4,4),(-0.00286833998582986,
0.477902879786545),(0.0665898698862504,0.0731716198748493),
 .UNSPECIFIED.);
#2420=B_SPLINE_SURFACE_WITH_KNOTS('',3,3,((#76128,#76129,#76130,#76131),
(#76132,#76133,#76134,#76135),(#76136,#76137,#76138,#76139),(#76140,#76141,
#76142,#76143)),.UNSPECIFIED.,.F.,.F.,.F.,(4,4),(4,4),(0.522097120209601,
1.00286791825518),(0.060015686548695,0.0665898700060147),.UNSPECIFIED.);
#2421=B_SPLINE_SURFACE_WITH_KNOTS('',3,3,((#76153,#76154,#76155,#76156),
(#76157,#76158,#76159,#76160),(#76161,#76162,#76163,#76164),(#76165,#76166,
#76167,#76168)),.UNSPECIFIED.,.F.,.F.,.F.,(4,4),(4,4),(-0.00286764392023406,
0.477902879786583),(0.0565997133101206,0.0631721430887068),
 .UNSPECIFIED.);
#2422=B_SPLINE_SURFACE_WITH_KNOTS('',3,3,((#76205,#76206,#76207,#76208),
(#76209,#76210,#76211,#76212),(#76213,#76214,#76215,#76216),(#76217,#76218,
#76219,#76220)),.UNSPECIFIED.,.F.,.F.,.F.,(4,4),(4,4),(0.522097120210378,
1.00286780122182),(0.0500263550858676,0.0565997133101427),.UNSPECIFIED.);
#2423=B_SPLINE_SURFACE_WITH_KNOTS('',3,3,((#76253,#76254,#76255,#76256),
(#76257,#76258,#76259,#76260),(#76261,#76262,#76263,#76264),(#76265,#76266,
#76267,#76268)),.UNSPECIFIED.,.F.,.F.,.F.,(4,4),(4,4),(-0.0060001464356663,
1.),(0.0365944846640624,0.0466073985929451),.UNSPECIFIED.);
#2424=B_SPLINE_SURFACE_WITH_KNOTS('',3,3,((#76291,#76292,#76293,#76294),
(#76295,#76296,#76297,#76298),(#76299,#76300,#76301,#76302),(#76303,#76304,
#76305,#76306)),.UNSPECIFIED.,.F.,.F.,.F.,(4,4),(4,4),(0.522097120210012,
1.0028684845257),(0.0400218729465707,0.0466073985929451),.UNSPECIFIED.);
#2425=B_SPLINE_SURFACE_WITH_KNOTS('',3,3,((#76370,#76371,#76372,#76373),
(#76374,#76375,#76376,#76377),(#76378,#76379,#76380,#76381),(#76382,#76383,
#76384,#76385)),.UNSPECIFIED.,.F.,.F.,.F.,(4,4),(4,4),(0.522097120209054,
1.00286862201138),(0.0300094532292158,0.0365944846647039),.UNSPECIFIED.);
#2426=B_SPLINE_SURFACE_WITH_KNOTS('',3,3,((#76418,#76419,#76420,#76421),
(#76422,#76423,#76424,#76425),(#76426,#76427,#76428,#76429),(#76430,#76431,
#76432,#76433)),.UNSPECIFIED.,.F.,.F.,.F.,(4,4),(4,4),(-0.00600003961845795,
1.00000000246918),(0.0166015299238286,0.0265907346180636),.UNSPECIFIED.);
#2427=B_SPLINE_SURFACE_WITH_KNOTS('',3,3,((#76445,#76446,#76447,#76448),
(#76449,#76450,#76451,#76452),(#76453,#76454,#76455,#76456),(#76457,#76458,
#76459,#76460)),.UNSPECIFIED.,.F.,.F.,.F.,(4,4),(4,4),(0.522097120210085,
1.0028678041046),(0.0200175229646512,0.026590734618065),.UNSPECIFIED.);
#2428=B_SPLINE_SURFACE_WITH_KNOTS('',3,3,((#76516,#76517,#76518,#76519),
(#76520,#76521,#76522,#76523),(#76524,#76525,#76526,#76527),(#76528,#76529,
#76530,#76531)),.UNSPECIFIED.,.F.,.F.,.F.,(4,4),(4,4),(0.522097120209799,
1.00286791014274),(0.0100271466749313,0.0166015302184278),.UNSPECIFIED.);
#2429=B_SPLINE_SURFACE_WITH_KNOTS('',3,3,((#76557,#76558,#76559,#76560),
(#76561,#76562,#76563,#76564),(#76565,#76566,#76567,#76568),(#76569,#76570,
#76571,#76572)),.UNSPECIFIED.,.F.,.F.,.F.,(4,4),(4,4),(-0.000171895437403129,
1.00600020634821),(0.0665898698856045,0.0751325481152999),.UNSPECIFIED.);
#2430=B_SPLINE_SURFACE_WITH_KNOTS('',3,3,((#76588,#76589,#76590,#76591),
(#76592,#76593,#76594,#76595),(#76596,#76597,#76598,#76599),(#76600,#76601,
#76602,#76603)),.UNSPECIFIED.,.F.,.F.,.F.,(4,4),(4,4),(-0.00286833998592427,
0.477902879786586),(0.0665898698862519,0.0731716198748508),
 .UNSPECIFIED.);
#2431=B_SPLINE_SURFACE_WITH_KNOTS('',3,3,((#76637,#76638,#76639,#76640),
(#76641,#76642,#76643,#76644),(#76645,#76646,#76647,#76648),(#76649,#76650,
#76651,#76652)),.UNSPECIFIED.,.F.,.F.,.F.,(4,4),(4,4),(0.522097120209579,
1.00286791825534),(0.0600156865486934,0.0665898700060136),.UNSPECIFIED.);
#2432=B_SPLINE_SURFACE_WITH_KNOTS('',3,3,((#76662,#76663,#76664,#76665),
(#76666,#76667,#76668,#76669),(#76670,#76671,#76672,#76673),(#76674,#76675,
#76676,#76677)),.UNSPECIFIED.,.F.,.F.,.F.,(4,4),(4,4),(-0.00286764392025056,
0.477902879786533),(0.0565997133101202,0.0631721430887066),
 .UNSPECIFIED.);
#2433=B_SPLINE_SURFACE_WITH_KNOTS('',3,3,((#76711,#76712,#76713,#76714),
(#76715,#76716,#76717,#76718),(#76719,#76720,#76721,#76722),(#76723,#76724,
#76725,#76726)),.UNSPECIFIED.,.F.,.F.,.F.,(4,4),(4,4),(0.522097120210524,
1.00286780122199),(0.0500263550858677,0.0565997133101438),.UNSPECIFIED.);
#2434=B_SPLINE_SURFACE_WITH_KNOTS('',3,3,((#76734,#76735,#76736,#76737),
(#76738,#76739,#76740,#76741),(#76742,#76743,#76744,#76745),(#76746,#76747,
#76748,#76749)),.UNSPECIFIED.,.F.,.F.,.F.,(4,4),(4,4),(-0.00286810177311321,
0.477902879786528),(0.0466073985929115,0.0531834933545508),
 .UNSPECIFIED.);
#2435=B_SPLINE_SURFACE_WITH_KNOTS('',3,3,((#76805,#76806,#76807,#76808),
(#76809,#76810,#76811,#76812),(#76813,#76814,#76815,#76816),(#76817,#76818,
#76819,#76820)),.UNSPECIFIED.,.F.,.F.,.F.,(4,4),(4,4),(0.522097120210016,
1.00286848452579),(0.0400218729465696,0.0466073985929448),.UNSPECIFIED.);
#2436=B_SPLINE_SURFACE_WITH_KNOTS('',3,3,((#76886,#76887,#76888,#76889),
(#76890,#76891,#76892,#76893),(#76894,#76895,#76896,#76897),(#76898,#76899,
#76900,#76901)),.UNSPECIFIED.,.F.,.F.,.F.,(4,4),(4,4),(0.522097120209344,
1.00286862201151),(0.0300094532292164,0.0365944846647039),.UNSPECIFIED.);
#2437=B_SPLINE_SURFACE_WITH_KNOTS('',3,3,((#76909,#76910,#76911,#76912),
(#76913,#76914,#76915,#76916),(#76917,#76918,#76919,#76920),(#76921,#76922,
#76923,#76924)),.UNSPECIFIED.,.F.,.F.,.F.,(4,4),(4,4),(-0.00286823045904117,
0.477902879786487),(0.0265907346180614,0.0331702036774536),
 .UNSPECIFIED.);
#2438=B_SPLINE_SURFACE_WITH_KNOTS('',3,3,((#76941,#76942,#76943,#76944),
(#76945,#76946,#76947,#76948),(#76949,#76950,#76951,#76952),(#76953,#76954,
#76955,#76956)),.UNSPECIFIED.,.F.,.F.,.F.,(4,4),(4,4),(-0.00600003962494949,
1.00000000356517),(0.0166015299238284,0.0265907346180641),.UNSPECIFIED.);
#2439=B_SPLINE_SURFACE_WITH_KNOTS('',3,3,((#76968,#76969,#76970,#76971),
(#76972,#76973,#76974,#76975),(#76976,#76977,#76978,#76979),(#76980,#76981,
#76982,#76983)),.UNSPECIFIED.,.F.,.F.,.F.,(4,4),(4,4),(0.522097120210132,
1.00286780410458),(0.0200175229646515,0.0265907346180646),.UNSPECIFIED.);
#2440=B_SPLINE_SURFACE_WITH_KNOTS('',3,3,((#77039,#77040,#77041,#77042),
(#77043,#77044,#77045,#77046),(#77047,#77048,#77049,#77050),(#77051,#77052,
#77053,#77054)),.UNSPECIFIED.,.F.,.F.,.F.,(4,4),(4,4),(0.522097120209969,
1.00286791014268),(0.0100271466749314,0.0166015302184277),.UNSPECIFIED.);
#2441=B_SPLINE_SURFACE_WITH_KNOTS('',3,3,((#77080,#77081,#77082,#77083),
(#77084,#77085,#77086,#77087),(#77088,#77089,#77090,#77091),(#77092,#77093,
#77094,#77095)),.UNSPECIFIED.,.F.,.F.,.F.,(4,4),(4,4),(-0.000171895436535362,
1.00600020634832),(0.0665898698856043,0.075132548114432),.UNSPECIFIED.);
#2442=B_SPLINE_SURFACE_WITH_KNOTS('',3,3,((#77111,#77112,#77113,#77114),
(#77115,#77116,#77117,#77118),(#77119,#77120,#77121,#77122),(#77123,#77124,
#77125,#77126)),.UNSPECIFIED.,.F.,.F.,.F.,(4,4),(4,4),(-0.00286833998596488,
0.477902879786617),(0.0665898698862506,0.0731716198748498),
 .UNSPECIFIED.);
#2443=B_SPLINE_SURFACE_WITH_KNOTS('',3,3,((#77160,#77161,#77162,#77163),
(#77164,#77165,#77166,#77167),(#77168,#77169,#77170,#77171),(#77172,#77173,
#77174,#77175)),.UNSPECIFIED.,.F.,.F.,.F.,(4,4),(4,4),(0.522097120209847,
1.00286791825524),(0.0600156865486933,0.0665898700060139),.UNSPECIFIED.);
#2444=B_SPLINE_SURFACE_WITH_KNOTS('',3,3,((#77185,#77186,#77187,#77188),
(#77189,#77190,#77191,#77192),(#77193,#77194,#77195,#77196),(#77197,#77198,
#77199,#77200)),.UNSPECIFIED.,.F.,.F.,.F.,(4,4),(4,4),(-0.00286764392028603,
0.477902879786574),(0.0565997133101217,0.063172143088707),.UNSPECIFIED.);
#2445=B_SPLINE_SURFACE_WITH_KNOTS('',3,3,((#77237,#77238,#77239,#77240),
(#77241,#77242,#77243,#77244),(#77245,#77246,#77247,#77248),(#77249,#77250,
#77251,#77252)),.UNSPECIFIED.,.F.,.F.,.F.,(4,4),(4,4),(0.522097120210472,
1.00286780122192),(0.0500263550858672,0.0565997133101425),.UNSPECIFIED.);
#2446=B_SPLINE_SURFACE_WITH_KNOTS('',3,3,((#77324,#77325,#77326,#77327),
(#77328,#77329,#77330,#77331),(#77332,#77333,#77334,#77335),(#77336,#77337,
#77338,#77339)),.UNSPECIFIED.,.F.,.F.,.F.,(4,4),(4,4),(0.522097120210281,
1.00286848452586),(0.0400218729465702,0.0466073985929454),.UNSPECIFIED.);
#2447=B_SPLINE_SURFACE_WITH_KNOTS('',3,3,((#77408,#77409,#77410,#77411),
(#77412,#77413,#77414,#77415),(#77416,#77417,#77418,#77419),(#77420,#77421,
#77422,#77423)),.UNSPECIFIED.,.F.,.F.,.F.,(4,4),(4,4),(0.522097120209377,
1.00286862201145),(0.0300094532292159,0.0365944846647033),.UNSPECIFIED.);
#2448=B_SPLINE_SURFACE_WITH_KNOTS('',3,3,((#77456,#77457,#77458,#77459),
(#77460,#77461,#77462,#77463),(#77464,#77465,#77466,#77467),(#77468,#77469,
#77470,#77471)),.UNSPECIFIED.,.F.,.F.,.F.,(4,4),(4,4),(-0.00600003960349703,
1.),(0.0166015299238287,0.0265907346180644),.UNSPECIFIED.);
#2449=B_SPLINE_SURFACE_WITH_KNOTS('',3,3,((#77483,#77484,#77485,#77486),
(#77487,#77488,#77489,#77490),(#77491,#77492,#77493,#77494),(#77495,#77496,
#77497,#77498)),.UNSPECIFIED.,.F.,.F.,.F.,(4,4),(4,4),(0.522097120210262,
1.00286780410451),(0.0200175229646517,0.0265907346180652),.UNSPECIFIED.);
#2450=B_SPLINE_SURFACE_WITH_KNOTS('',3,3,((#77506,#77507,#77508,#77509),
(#77510,#77511,#77512,#77513),(#77514,#77515,#77516,#77517),(#77518,#77519,
#77520,#77521)),.UNSPECIFIED.,.F.,.F.,.F.,(4,4),(4,4),(-0.00286753114042522,
0.477902879786509),(0.0166015299238958,0.0231736788090039),
 .UNSPECIFIED.);
#2451=B_SPLINE_SURFACE_WITH_KNOTS('',3,3,((#77561,#77562,#77563,#77564),
(#77565,#77566,#77567,#77568),(#77569,#77570,#77571,#77572),(#77573,#77574,
#77575,#77576)),.UNSPECIFIED.,.F.,.F.,.F.,(4,4),(4,4),(0.522097120210089,
1.00286791014277),(0.0100271466749312,0.0166015302184273),.UNSPECIFIED.);
#2452=B_SPLINE_SURFACE_WITH_KNOTS('',3,3,((#77602,#77603,#77604,#77605),
(#77606,#77607,#77608,#77609),(#77610,#77611,#77612,#77613),(#77614,#77615,
#77616,#77617)),.UNSPECIFIED.,.F.,.F.,.F.,(4,4),(4,4),(-0.000171895435626065,
1.00600020634828),(0.0665898698856039,0.0751325481135236),.UNSPECIFIED.);
#2453=B_SPLINE_SURFACE_WITH_KNOTS('',3,3,((#77633,#77634,#77635,#77636),
(#77637,#77638,#77639,#77640),(#77641,#77642,#77643,#77644),(#77645,#77646,
#77647,#77648)),.UNSPECIFIED.,.F.,.F.,.F.,(4,4),(4,4),(-0.00286833998592586,
0.477902879786536),(0.0665898698862503,0.0731716198748495),
 .UNSPECIFIED.);
#2454=B_SPLINE_SURFACE_WITH_KNOTS('',3,3,((#77682,#77683,#77684,#77685),
(#77686,#77687,#77688,#77689),(#77690,#77691,#77692,#77693),(#77694,#77695,
#77696,#77697)),.UNSPECIFIED.,.F.,.F.,.F.,(4,4),(4,4),(0.522097120209945,
1.0028679182552),(0.0600156865486939,0.0665898700060147),.UNSPECIFIED.);
#2455=B_SPLINE_SURFACE_WITH_KNOTS('',3,3,((#77707,#77708,#77709,#77710),
(#77711,#77712,#77713,#77714),(#77715,#77716,#77717,#77718),(#77719,#77720,
#77721,#77722)),.UNSPECIFIED.,.F.,.F.,.F.,(4,4),(4,4),(-0.00286764392026067,
0.477902879786611),(0.0565997133101195,0.0631721430887069),
 .UNSPECIFIED.);
#2456=B_SPLINE_SURFACE_WITH_KNOTS('',3,3,((#77759,#77760,#77761,#77762),
(#77763,#77764,#77765,#77766),(#77767,#77768,#77769,#77770),(#77771,#77772,
#77773,#77774)),.UNSPECIFIED.,.F.,.F.,.F.,(4,4),(4,4),(0.522097120210691,
1.00286780122204),(0.0500263550858657,0.0565997133101437),.UNSPECIFIED.);
#2457=B_SPLINE_SURFACE_WITH_KNOTS('',3,3,((#77846,#77847,#77848,#77849),
(#77850,#77851,#77852,#77853),(#77854,#77855,#77856,#77857),(#77858,#77859,
#77860,#77861)),.UNSPECIFIED.,.F.,.F.,.F.,(4,4),(4,4),(0.522097120210333,
1.00286848452579),(0.0400218729465701,0.0466073985929457),.UNSPECIFIED.);
#2458=B_SPLINE_SURFACE_WITH_KNOTS('',3,3,((#77930,#77931,#77932,#77933),
(#77934,#77935,#77936,#77937),(#77938,#77939,#77940,#77941),(#77942,#77943,
#77944,#77945)),.UNSPECIFIED.,.F.,.F.,.F.,(4,4),(4,4),(0.522097120209519,
1.00286862201157),(0.0300094532292161,0.0365944846647038),.UNSPECIFIED.);
#2459=B_SPLINE_SURFACE_WITH_KNOTS('',3,3,((#77978,#77979,#77980,#77981),
(#77982,#77983,#77984,#77985),(#77986,#77987,#77988,#77989),(#77990,#77991,
#77992,#77993)),.UNSPECIFIED.,.F.,.F.,.F.,(4,4),(4,4),(-0.0060000396247669,
1.00000000356511),(0.0166015299238272,0.0265907346180642),.UNSPECIFIED.);
#2460=B_SPLINE_SURFACE_WITH_KNOTS('',3,3,((#78005,#78006,#78007,#78008),
(#78009,#78010,#78011,#78012),(#78013,#78014,#78015,#78016),(#78017,#78018,
#78019,#78020)),.UNSPECIFIED.,.F.,.F.,.F.,(4,4),(4,4),(0.522097120210314,
1.00286780410453),(0.0200175229646511,0.0265907346180649),.UNSPECIFIED.);
#2461=B_SPLINE_SURFACE_WITH_KNOTS('',3,3,((#78073,#78074,#78075,#78076),
(#78077,#78078,#78079,#78080),(#78081,#78082,#78083,#78084),(#78085,#78086,
#78087,#78088)),.UNSPECIFIED.,.F.,.F.,.F.,(4,4),(4,4),(0.522097120210105,
1.0028679101425),(0.0100271466749325,0.0166015302184282),.UNSPECIFIED.);
#2462=B_SPLINE_SURFACE_WITH_KNOTS('',3,3,((#78096,#78097,#78098,#78099),
(#78100,#78101,#78102,#78103),(#78104,#78105,#78106,#78107),(#78108,#78109,
#78110,#78111)),.UNSPECIFIED.,.F.,.F.,.F.,(4,4),(4,4),(-0.00206901892618064,
0.346769728493059),(0.00660713154712627,0.0131849431469577),
 .UNSPECIFIED.);
#2463=B_SPLINE_SURFACE_WITH_KNOTS('',3,3,((#78121,#78122,#78123,#78124),
(#78125,#78126,#78127,#78128),(#78129,#78130,#78131,#78132),(#78133,#78134,
#78135,#78136)),.UNSPECIFIED.,.F.,.F.,.F.,(4,4),(4,4),(-0.000171895434855279,
1.00600020634832),(0.0665898698856049,0.0751325481127517),.UNSPECIFIED.);
#2464=B_SPLINE_SURFACE_WITH_KNOTS('',3,3,((#78152,#78153,#78154,#78155),
(#78156,#78157,#78158,#78159),(#78160,#78161,#78162,#78163),(#78164,#78165,
#78166,#78167)),.UNSPECIFIED.,.F.,.F.,.F.,(4,4),(4,4),(-0.00286833998594799,
0.477902879786575),(0.066589869886252,0.0731716198748501),.UNSPECIFIED.);
#2465=B_SPLINE_SURFACE_WITH_KNOTS('',3,3,((#78201,#78202,#78203,#78204),
(#78205,#78206,#78207,#78208),(#78209,#78210,#78211,#78212),(#78213,#78214,
#78215,#78216)),.UNSPECIFIED.,.F.,.F.,.F.,(4,4),(4,4),(0.522097120210037,
1.00286791825517),(0.0600156865486943,0.0665898700060142),.UNSPECIFIED.);
#2466=B_SPLINE_SURFACE_WITH_KNOTS('',3,3,((#78226,#78227,#78228,#78229),
(#78230,#78231,#78232,#78233),(#78234,#78235,#78236,#78237),(#78238,#78239,
#78240,#78241)),.UNSPECIFIED.,.F.,.F.,.F.,(4,4),(4,4),(-0.00286764392024655,
0.477902879786472),(0.0565997133101204,0.0631721430887056),
 .UNSPECIFIED.);
#2467=B_SPLINE_SURFACE_WITH_KNOTS('',3,3,((#78278,#78279,#78280,#78281),
(#78282,#78283,#78284,#78285),(#78286,#78287,#78288,#78289),(#78290,#78291,
#78292,#78293)),.UNSPECIFIED.,.F.,.F.,.F.,(4,4),(4,4),(0.522097120210844,
1.0028678012219),(0.050026355085867,0.0565997133101422),.UNSPECIFIED.);
#2468=B_SPLINE_SURFACE_WITH_KNOTS('',3,3,((#78365,#78366,#78367,#78368),
(#78369,#78370,#78371,#78372),(#78373,#78374,#78375,#78376),(#78377,#78378,
#78379,#78380)),.UNSPECIFIED.,.F.,.F.,.F.,(4,4),(4,4),(0.522097120210373,
1.00286848452577),(0.0400218729465708,0.0466073985929444),.UNSPECIFIED.);
#2469=B_SPLINE_SURFACE_WITH_KNOTS('',3,3,((#78449,#78450,#78451,#78452),
(#78453,#78454,#78455,#78456),(#78457,#78458,#78459,#78460),(#78461,#78462,
#78463,#78464)),.UNSPECIFIED.,.F.,.F.,.F.,(4,4),(4,4),(0.522097120209569,
1.0028686220114),(0.0300094532292161,0.0365944846647028),.UNSPECIFIED.);
#2470=B_SPLINE_SURFACE_WITH_KNOTS('',3,3,((#78497,#78498,#78499,#78500),
(#78501,#78502,#78503,#78504),(#78505,#78506,#78507,#78508),(#78509,#78510,
#78511,#78512)),.UNSPECIFIED.,.F.,.F.,.F.,(4,4),(4,4),(-0.00600003962476691,
1.00000000356515),(0.016601529923829,0.0265907346180638),.UNSPECIFIED.);
#2471=B_SPLINE_SURFACE_WITH_KNOTS('',3,3,((#78524,#78525,#78526,#78527),
(#78528,#78529,#78530,#78531),(#78532,#78533,#78534,#78535),(#78536,#78537,
#78538,#78539)),.UNSPECIFIED.,.F.,.F.,.F.,(4,4),(4,4),(0.522097120210578,
1.0028678041046),(0.0200175229646522,0.0265907346180645),.UNSPECIFIED.);
#2472=B_SPLINE_SURFACE_WITH_KNOTS('',3,3,((#78595,#78596,#78597,#78598),
(#78599,#78600,#78601,#78602),(#78603,#78604,#78605,#78606),(#78607,#78608,
#78609,#78610)),.UNSPECIFIED.,.F.,.F.,.F.,(4,4),(4,4),(0.52209712021034,
1.00286791014272),(0.0100271466749315,0.0166015302184262),.UNSPECIFIED.);
#2473=B_SPLINE_SURFACE_WITH_KNOTS('',3,3,((#78636,#78637,#78638,#78639),
(#78640,#78641,#78642,#78643),(#78644,#78645,#78646,#78647),(#78648,#78649,
#78650,#78651)),.UNSPECIFIED.,.F.,.F.,.F.,(4,4),(4,4),(-0.000171895433735589,
1.00600020634835),(0.0665898698856037,0.0751325481116349),.UNSPECIFIED.);
#2474=B_SPLINE_SURFACE_WITH_KNOTS('',3,3,((#78667,#78668,#78669,#78670),
(#78671,#78672,#78673,#78674),(#78675,#78676,#78677,#78678),(#78679,#78680,
#78681,#78682)),.UNSPECIFIED.,.F.,.F.,.F.,(4,4),(4,4),(-0.00286833998586006,
0.477902879786518),(0.0665898698862502,0.0731716198748497),
 .UNSPECIFIED.);
#2475=B_SPLINE_SURFACE_WITH_KNOTS('',3,3,((#78716,#78717,#78718,#78719),
(#78720,#78721,#78722,#78723),(#78724,#78725,#78726,#78727),(#78728,#78729,
#78730,#78731)),.UNSPECIFIED.,.F.,.F.,.F.,(4,4),(4,4),(0.52209712021009,
1.00286791825523),(0.0600156865486944,0.0665898700060149),.UNSPECIFIED.);
#2476=B_SPLINE_SURFACE_WITH_KNOTS('',3,3,((#78741,#78742,#78743,#78744),
(#78745,#78746,#78747,#78748),(#78749,#78750,#78751,#78752),(#78753,#78754,
#78755,#78756)),.UNSPECIFIED.,.F.,.F.,.F.,(4,4),(4,4),(-0.00286764392027115,
0.477902879786605),(0.0565997133101205,0.0631721430887074),
 .UNSPECIFIED.);
#2477=B_SPLINE_SURFACE_WITH_KNOTS('',3,3,((#78793,#78794,#78795,#78796),
(#78797,#78798,#78799,#78800),(#78801,#78802,#78803,#78804),(#78805,#78806,
#78807,#78808)),.UNSPECIFIED.,.F.,.F.,.F.,(4,4),(4,4),(0.522097120210832,
1.00286780122184),(0.0500263550858676,0.0565997133101431),.UNSPECIFIED.);
#2478=B_SPLINE_SURFACE_WITH_KNOTS('',3,3,((#78880,#78881,#78882,#78883),
(#78884,#78885,#78886,#78887),(#78888,#78889,#78890,#78891),(#78892,#78893,
#78894,#78895)),.UNSPECIFIED.,.F.,.F.,.F.,(4,4),(4,4),(0.522097120210514,
1.00286848452574),(0.0400218729465704,0.0466073985929453),.UNSPECIFIED.);
#2479=B_SPLINE_SURFACE_WITH_KNOTS('',3,3,((#78964,#78965,#78966,#78967),
(#78968,#78969,#78970,#78971),(#78972,#78973,#78974,#78975),(#78976,#78977,
#78978,#78979)),.UNSPECIFIED.,.F.,.F.,.F.,(4,4),(4,4),(0.522097120209706,
1.00286862201148),(0.030009453229216,0.0365944846647038),.UNSPECIFIED.);
#2480=B_SPLINE_SURFACE_WITH_KNOTS('',3,3,((#79012,#79013,#79014,#79015),
(#79016,#79017,#79018,#79019),(#79020,#79021,#79022,#79023),(#79024,#79025,
#79026,#79027)),.UNSPECIFIED.,.F.,.F.,.F.,(4,4),(4,4),(-0.00600003964311649,
1.00000000663621),(0.0166015299238286,0.0265907346180639),.UNSPECIFIED.);
#2481=B_SPLINE_SURFACE_WITH_KNOTS('',3,3,((#79039,#79040,#79041,#79042),
(#79043,#79044,#79045,#79046),(#79047,#79048,#79049,#79050),(#79051,#79052,
#79053,#79054)),.UNSPECIFIED.,.F.,.F.,.F.,(4,4),(4,4),(0.522097120210579,
1.00286780410459),(0.0200175229646512,0.026590734618065),.UNSPECIFIED.);
#2482=B_SPLINE_SURFACE_WITH_KNOTS('',3,3,((#79110,#79111,#79112,#79113),
(#79114,#79115,#79116,#79117),(#79118,#79119,#79120,#79121),(#79122,#79123,
#79124,#79125)),.UNSPECIFIED.,.F.,.F.,.F.,(4,4),(4,4),(0.522097120210466,
1.00286791014274),(0.0100271466749329,0.0166015302184284),.UNSPECIFIED.);
#2483=B_SPLINE_SURFACE_WITH_KNOTS('',3,3,((#79151,#79152,#79153,#79154),
(#79155,#79156,#79157,#79158),(#79159,#79160,#79161,#79162),(#79163,#79164,
#79165,#79166)),.UNSPECIFIED.,.F.,.F.,.F.,(4,4),(4,4),(-0.000171895432979033,
1.00600020634818),(0.0665898698856052,0.0751325481108763),.UNSPECIFIED.);
#2484=B_SPLINE_SURFACE_WITH_KNOTS('',3,3,((#79182,#79183,#79184,#79185),
(#79186,#79187,#79188,#79189),(#79190,#79191,#79192,#79193),(#79194,#79195,
#79196,#79197)),.UNSPECIFIED.,.F.,.F.,.F.,(4,4),(4,4),(-0.00286833998587121,
0.477902879786704),(0.0665898698862514,0.0731716198748496),
 .UNSPECIFIED.);
#2485=B_SPLINE_SURFACE_WITH_KNOTS('',3,3,((#79231,#79232,#79233,#79234),
(#79235,#79236,#79237,#79238),(#79239,#79240,#79241,#79242),(#79243,#79244,
#79245,#79246)),.UNSPECIFIED.,.F.,.F.,.F.,(4,4),(4,4),(0.522097120210201,
1.0028679182551),(0.0600156865486941,0.0665898700060154),.UNSPECIFIED.);
#2486=B_SPLINE_SURFACE_WITH_KNOTS('',3,3,((#79256,#79257,#79258,#79259),
(#79260,#79261,#79262,#79263),(#79264,#79265,#79266,#79267),(#79268,#79269,
#79270,#79271)),.UNSPECIFIED.,.F.,.F.,.F.,(4,4),(4,4),(-0.00286764392018088,
0.477902879786574),(0.0565997133101201,0.0631721430887063),
 .UNSPECIFIED.);
#2487=B_SPLINE_SURFACE_WITH_KNOTS('',3,3,((#79308,#79309,#79310,#79311),
(#79312,#79313,#79314,#79315),(#79316,#79317,#79318,#79319),(#79320,#79321,
#79322,#79323)),.UNSPECIFIED.,.F.,.F.,.F.,(4,4),(4,4),(0.522097120211028,
1.00286780122187),(0.0500263550858676,0.0565997133101434),.UNSPECIFIED.);
#2488=B_SPLINE_SURFACE_WITH_KNOTS('',3,3,((#79395,#79396,#79397,#79398),
(#79399,#79400,#79401,#79402),(#79403,#79404,#79405,#79406),(#79407,#79408,
#79409,#79410)),.UNSPECIFIED.,.F.,.F.,.F.,(4,4),(4,4),(0.522097120210638,
1.00286848452575),(0.0400218729465699,0.046607398592945),.UNSPECIFIED.);
#2489=B_SPLINE_SURFACE_WITH_KNOTS('',3,3,((#79479,#79480,#79481,#79482),
(#79483,#79484,#79485,#79486),(#79487,#79488,#79489,#79490),(#79491,#79492,
#79493,#79494)),.UNSPECIFIED.,.F.,.F.,.F.,(4,4),(4,4),(0.522097120209859,
1.00286862201151),(0.0300094532292154,0.0365944846647027),.UNSPECIFIED.);
#2490=B_SPLINE_SURFACE_WITH_KNOTS('',3,3,((#79527,#79528,#79529,#79530),
(#79531,#79532,#79533,#79534),(#79535,#79536,#79537,#79538),(#79539,#79540,
#79541,#79542)),.UNSPECIFIED.,.F.,.F.,.F.,(4,4),(4,4),(-0.00600003961813093,
1.00000000246938),(0.0166015299238286,0.0265907346180632),.UNSPECIFIED.);
#2491=B_SPLINE_SURFACE_WITH_KNOTS('',3,3,((#79554,#79555,#79556,#79557),
(#79558,#79559,#79560,#79561),(#79562,#79563,#79564,#79565),(#79566,#79567,
#79568,#79569)),.UNSPECIFIED.,.F.,.F.,.F.,(4,4),(4,4),(0.522097120210637,
1.00286780410452),(0.0200175229646505,0.0265907346180656),.UNSPECIFIED.);
#2492=B_SPLINE_SURFACE_WITH_KNOTS('',3,3,((#79625,#79626,#79627,#79628),
(#79629,#79630,#79631,#79632),(#79633,#79634,#79635,#79636),(#79637,#79638,
#79639,#79640)),.UNSPECIFIED.,.F.,.F.,.F.,(4,4),(4,4),(0.522097120210457,
1.0028679101428),(0.0100271466749311,0.0166015302184272),.UNSPECIFIED.);
#2493=B_SPLINE_SURFACE_WITH_KNOTS('',3,3,((#79666,#79667,#79668,#79669),
(#79670,#79671,#79672,#79673),(#79674,#79675,#79676,#79677),(#79678,#79679,
#79680,#79681)),.UNSPECIFIED.,.F.,.F.,.F.,(4,4),(4,4),(-0.00017189543205102,
1.00600020634805),(0.0665898698856059,0.0751325481099475),.UNSPECIFIED.);
#2494=B_SPLINE_SURFACE_WITH_KNOTS('',3,3,((#79697,#79698,#79699,#79700),
(#79701,#79702,#79703,#79704),(#79705,#79706,#79707,#79708),(#79709,#79710,
#79711,#79712)),.UNSPECIFIED.,.F.,.F.,.F.,(4,4),(4,4),(-0.0028683399860157,
0.477902879786574),(0.0665898698862513,0.0731716198748509),
 .UNSPECIFIED.);
#2495=B_SPLINE_SURFACE_WITH_KNOTS('',3,3,((#79746,#79747,#79748,#79749),
(#79750,#79751,#79752,#79753),(#79754,#79755,#79756,#79757),(#79758,#79759,
#79760,#79761)),.UNSPECIFIED.,.F.,.F.,.F.,(4,4),(4,4),(0.522097120210386,
1.00286791825519),(0.0600156865486944,0.0665898700060139),.UNSPECIFIED.);
#2496=B_SPLINE_SURFACE_WITH_KNOTS('',3,3,((#79771,#79772,#79773,#79774),
(#79775,#79776,#79777,#79778),(#79779,#79780,#79781,#79782),(#79783,#79784,
#79785,#79786)),.UNSPECIFIED.,.F.,.F.,.F.,(4,4),(4,4),(-0.00286764392010482,
0.477902879786664),(0.0565997133101203,0.0631721430887056),
 .UNSPECIFIED.);
#2497=B_SPLINE_SURFACE_WITH_KNOTS('',3,3,((#79823,#79824,#79825,#79826),
(#79827,#79828,#79829,#79830),(#79831,#79832,#79833,#79834),(#79835,#79836,
#79837,#79838)),.UNSPECIFIED.,.F.,.F.,.F.,(4,4),(4,4),(0.522097120211212,
1.00286780122197),(0.0500263550858661,0.0565997133101428),.UNSPECIFIED.);
#2498=B_SPLINE_SURFACE_WITH_KNOTS('',3,3,((#79910,#79911,#79912,#79913),
(#79914,#79915,#79916,#79917),(#79918,#79919,#79920,#79921),(#79922,#79923,
#79924,#79925)),.UNSPECIFIED.,.F.,.F.,.F.,(4,4),(4,4),(0.522097120210728,
1.00286848452584),(0.04002187294657,0.0466073985929452),.UNSPECIFIED.);
#2499=B_SPLINE_SURFACE_WITH_KNOTS('',3,3,((#79994,#79995,#79996,#79997),
(#79998,#79999,#80000,#80001),(#80002,#80003,#80004,#80005),(#80006,#80007,
#80008,#80009)),.UNSPECIFIED.,.F.,.F.,.F.,(4,4),(4,4),(0.522097120209888,
1.00286862201144),(0.0300094532292169,0.0365944846647038),.UNSPECIFIED.);
#2500=B_SPLINE_SURFACE_WITH_KNOTS('',3,3,((#80042,#80043,#80044,#80045),
(#80046,#80047,#80048,#80049),(#80050,#80051,#80052,#80053),(#80054,#80055,
#80056,#80057)),.UNSPECIFIED.,.F.,.F.,.F.,(4,4),(4,4),(-0.00600003961812457,
1.00000000246936),(0.0166015299238285,0.0265907346180632),.UNSPECIFIED.);
#2501=B_SPLINE_SURFACE_WITH_KNOTS('',3,3,((#80069,#80070,#80071,#80072),
(#80073,#80074,#80075,#80076),(#80077,#80078,#80079,#80080),(#80081,#80082,
#80083,#80084)),.UNSPECIFIED.,.F.,.F.,.F.,(4,4),(4,4),(0.522097120210843,
1.00286780410462),(0.0200175229646514,0.026590734618064),.UNSPECIFIED.);
#2502=B_SPLINE_SURFACE_WITH_KNOTS('',3,3,((#80140,#80141,#80142,#80143),
(#80144,#80145,#80146,#80147),(#80148,#80149,#80150,#80151),(#80152,#80153,
#80154,#80155)),.UNSPECIFIED.,.F.,.F.,.F.,(4,4),(4,4),(0.522097120210691,
1.00286791014268),(0.0100271466749321,0.0166015302184286),.UNSPECIFIED.);
#2503=B_SPLINE_SURFACE_WITH_KNOTS('',3,3,((#80181,#80182,#80183,#80184),
(#80185,#80186,#80187,#80188),(#80189,#80190,#80191,#80192),(#80193,#80194,
#80195,#80196)),.UNSPECIFIED.,.F.,.F.,.F.,(4,4),(4,4),(-0.00017189543133579,
1.00600020634815),(0.0665898698856047,0.0751325481092326),.UNSPECIFIED.);
#2504=B_SPLINE_SURFACE_WITH_KNOTS('',3,3,((#80212,#80213,#80214,#80215),
(#80216,#80217,#80218,#80219),(#80220,#80221,#80222,#80223),(#80224,#80225,
#80226,#80227)),.UNSPECIFIED.,.F.,.F.,.F.,(4,4),(4,4),(-0.00286833998587508,
0.477902879786664),(0.0665898698862506,0.0731716198748496),
 .UNSPECIFIED.);
#2505=B_SPLINE_SURFACE_WITH_KNOTS('',3,3,((#80261,#80262,#80263,#80264),
(#80265,#80266,#80267,#80268),(#80269,#80270,#80271,#80272),(#80273,#80274,
#80275,#80276)),.UNSPECIFIED.,.F.,.F.,.F.,(4,4),(4,4),(0.522097120209475,
1.00286791825523),(0.0600156865486928,0.0665898700060142),.UNSPECIFIED.);
#2506=B_SPLINE_SURFACE_WITH_KNOTS('',3,3,((#80286,#80287,#80288,#80289),
(#80290,#80291,#80292,#80293),(#80294,#80295,#80296,#80297),(#80298,#80299,
#80300,#80301)),.UNSPECIFIED.,.F.,.F.,.F.,(4,4),(4,4),(-0.0028676439202061,
0.477902879786615),(0.0565997133101201,0.0631721430887064),
 .UNSPECIFIED.);
#2507=B_SPLINE_SURFACE_WITH_KNOTS('',3,3,((#80338,#80339,#80340,#80341),
(#80342,#80343,#80344,#80345),(#80346,#80347,#80348,#80349),(#80350,#80351,
#80352,#80353)),.UNSPECIFIED.,.F.,.F.,.F.,(4,4),(4,4),(0.522097120210878,
1.00286780122192),(0.0500263550858677,0.0565997133101427),.UNSPECIFIED.);
#2508=B_SPLINE_SURFACE_WITH_KNOTS('',3,3,((#80425,#80426,#80427,#80428),
(#80429,#80430,#80431,#80432),(#80433,#80434,#80435,#80436),(#80437,#80438,
#80439,#80440)),.UNSPECIFIED.,.F.,.F.,.F.,(4,4),(4,4),(0.522097120210891,
1.00286848452579),(0.0400218729465691,0.0466073985929451),.UNSPECIFIED.);
#2509=B_SPLINE_SURFACE_WITH_KNOTS('',3,3,((#80509,#80510,#80511,#80512),
(#80513,#80514,#80515,#80516),(#80517,#80518,#80519,#80520),(#80521,#80522,
#80523,#80524)),.UNSPECIFIED.,.F.,.F.,.F.,(4,4),(4,4),(0.522097120209977,
1.00286862201146),(0.0300094532292159,0.0365944846647041),.UNSPECIFIED.);
#2510=B_SPLINE_SURFACE_WITH_KNOTS('',3,3,((#80557,#80558,#80559,#80560),
(#80561,#80562,#80563,#80564),(#80565,#80566,#80567,#80568),(#80569,#80570,
#80571,#80572)),.UNSPECIFIED.,.F.,.F.,.F.,(4,4),(4,4),(-0.00600003961813121,
1.0000000024693),(0.0166015299238285,0.0265907346180638),.UNSPECIFIED.);
#2511=B_SPLINE_SURFACE_WITH_KNOTS('',3,3,((#80584,#80585,#80586,#80587),
(#80588,#80589,#80590,#80591),(#80592,#80593,#80594,#80595),(#80596,#80597,
#80598,#80599)),.UNSPECIFIED.,.F.,.F.,.F.,(4,4),(4,4),(0.522097120210981,
1.00286780410451),(0.0200175229646507,0.026590734618064),.UNSPECIFIED.);
#2512=B_SPLINE_SURFACE_WITH_KNOTS('',3,3,((#80655,#80656,#80657,#80658),
(#80659,#80660,#80661,#80662),(#80663,#80664,#80665,#80666),(#80667,#80668,
#80669,#80670)),.UNSPECIFIED.,.F.,.F.,.F.,(4,4),(4,4),(0.522097120210828,
1.00286791014284),(0.0100271466749304,0.0166015302184278),.UNSPECIFIED.);
#2513=B_SPLINE_SURFACE_WITH_KNOTS('',3,3,((#80696,#80697,#80698,#80699),
(#80700,#80701,#80702,#80703),(#80704,#80705,#80706,#80707),(#80708,#80709,
#80710,#80711)),.UNSPECIFIED.,.F.,.F.,.F.,(4,4),(4,4),(-0.00017189543037276,
1.00600020634836),(0.0665898698856047,0.0751325481082702),.UNSPECIFIED.);
#2514=B_SPLINE_SURFACE_WITH_KNOTS('',3,3,((#80727,#80728,#80729,#80730),
(#80731,#80732,#80733,#80734),(#80735,#80736,#80737,#80738),(#80739,#80740,
#80741,#80742)),.UNSPECIFIED.,.F.,.F.,.F.,(4,4),(4,4),(-0.00286833998584599,
0.477902879786607),(0.0665898698862517,0.07317161987485),.UNSPECIFIED.);
#2515=B_SPLINE_SURFACE_WITH_KNOTS('',3,3,((#80776,#80777,#80778,#80779),
(#80780,#80781,#80782,#80783),(#80784,#80785,#80786,#80787),(#80788,#80789,
#80790,#80791)),.UNSPECIFIED.,.F.,.F.,.F.,(4,4),(4,4),(0.522097120207303,
1.00286791825526),(0.0600156865486934,0.0665898700060142),.UNSPECIFIED.);
#2516=B_SPLINE_SURFACE_WITH_KNOTS('',3,3,((#80801,#80802,#80803,#80804),
(#80805,#80806,#80807,#80808),(#80809,#80810,#80811,#80812),(#80813,#80814,
#80815,#80816)),.UNSPECIFIED.,.F.,.F.,.F.,(4,4),(4,4),(-0.00286764392024303,
0.477902879786695),(0.0565997133101202,0.0631721430887064),
 .UNSPECIFIED.);
#2517=B_SPLINE_SURFACE_WITH_KNOTS('',3,3,((#80853,#80854,#80855,#80856),
(#80857,#80858,#80859,#80860),(#80861,#80862,#80863,#80864),(#80865,#80866,
#80867,#80868)),.UNSPECIFIED.,.F.,.F.,.F.,(4,4),(4,4),(0.522097120208596,
1.00286780122191),(0.0500263550858673,0.0565997133101421),.UNSPECIFIED.);
#2518=B_SPLINE_SURFACE_WITH_KNOTS('',3,3,((#80940,#80941,#80942,#80943),
(#80944,#80945,#80946,#80947),(#80948,#80949,#80950,#80951),(#80952,#80953,
#80954,#80955)),.UNSPECIFIED.,.F.,.F.,.F.,(4,4),(4,4),(0.522097120209593,
1.00286848452575),(0.0400218729465712,0.0466073985929449),.UNSPECIFIED.);
#2519=B_SPLINE_SURFACE_WITH_KNOTS('',3,3,((#81024,#81025,#81026,#81027),
(#81028,#81029,#81030,#81031),(#81032,#81033,#81034,#81035),(#81036,#81037,
#81038,#81039)),.UNSPECIFIED.,.F.,.F.,.F.,(4,4),(4,4),(0.522097120210169,
1.00286862201142),(0.0300094532292164,0.036594484664704),.UNSPECIFIED.);
#2520=B_SPLINE_SURFACE_WITH_KNOTS('',3,3,((#81072,#81073,#81074,#81075),
(#81076,#81077,#81078,#81079),(#81080,#81081,#81082,#81083),(#81084,#81085,
#81086,#81087)),.UNSPECIFIED.,.F.,.F.,.F.,(4,4),(4,4),(-0.00600003961800698,
1.00000000246934),(0.0166015299238286,0.0265907346180639),.UNSPECIFIED.);
#2521=B_SPLINE_SURFACE_WITH_KNOTS('',3,3,((#81099,#81100,#81101,#81102),
(#81103,#81104,#81105,#81106),(#81107,#81108,#81109,#81110),(#81111,#81112,
#81113,#81114)),.UNSPECIFIED.,.F.,.F.,.F.,(4,4),(4,4),(0.522097120210999,
1.0028678041046),(0.020017522964652,0.0265907346180649),.UNSPECIFIED.);
#2522=B_SPLINE_SURFACE_WITH_KNOTS('',3,3,((#81170,#81171,#81172,#81173),
(#81174,#81175,#81176,#81177),(#81178,#81179,#81180,#81181),(#81182,#81183,
#81184,#81185)),.UNSPECIFIED.,.F.,.F.,.F.,(4,4),(4,4),(0.522097120210868,
1.00286791014275),(0.0100271466749306,0.0166015302184266),.UNSPECIFIED.);
#2523=B_SPLINE_SURFACE_WITH_KNOTS('',3,3,((#81211,#81212,#81213,#81214),
(#81215,#81216,#81217,#81218),(#81219,#81220,#81221,#81222),(#81223,#81224,
#81225,#81226)),.UNSPECIFIED.,.F.,.F.,.F.,(4,4),(4,4),(-0.0001718954296519,
1.00600020634795),(0.0665898698856053,0.0751325481075477),.UNSPECIFIED.);
#2524=B_SPLINE_SURFACE_WITH_KNOTS('',3,3,((#81242,#81243,#81244,#81245),
(#81246,#81247,#81248,#81249),(#81250,#81251,#81252,#81253),(#81254,#81255,
#81256,#81257)),.UNSPECIFIED.,.F.,.F.,.F.,(4,4),(4,4),(-0.00286833998595421,
0.477902879786473),(0.0665898698862515,0.0731716198748503),
 .UNSPECIFIED.);
#2525=B_SPLINE_SURFACE_WITH_KNOTS('',3,3,((#81291,#81292,#81293,#81294),
(#81295,#81296,#81297,#81298),(#81299,#81300,#81301,#81302),(#81303,#81304,
#81305,#81306)),.UNSPECIFIED.,.F.,.F.,.F.,(4,4),(4,4),(0.522097120205134,
1.00286791825525),(0.060015686548694,0.0665898700060144),.UNSPECIFIED.);
#2526=B_SPLINE_SURFACE_WITH_KNOTS('',3,3,((#81316,#81317,#81318,#81319),
(#81320,#81321,#81322,#81323),(#81324,#81325,#81326,#81327),(#81328,#81329,
#81330,#81331)),.UNSPECIFIED.,.F.,.F.,.F.,(4,4),(4,4),(-0.00286764392015422,
0.477902879786423),(0.0565997133101208,0.0631721430887068),
 .UNSPECIFIED.);
#2527=B_SPLINE_SURFACE_WITH_KNOTS('',3,3,((#81365,#81366,#81367,#81368),
(#81369,#81370,#81371,#81372),(#81373,#81374,#81375,#81376),(#81377,#81378,
#81379,#81380)),.UNSPECIFIED.,.F.,.F.,.F.,(4,4),(4,4),(0.522097120206487,
1.00286780122197),(0.0500263550858671,0.0565997133101411),.UNSPECIFIED.);
#2528=B_SPLINE_SURFACE_WITH_KNOTS('',3,3,((#81388,#81389,#81390,#81391),
(#81392,#81393,#81394,#81395),(#81396,#81397,#81398,#81399),(#81400,#81401,
#81402,#81403)),.UNSPECIFIED.,.F.,.F.,.F.,(4,4),(4,4),(-0.00286810177283975,
0.477902879786577),(0.0466073985929119,0.0531834933545505),
 .UNSPECIFIED.);
#2529=B_SPLINE_SURFACE_WITH_KNOTS('',3,3,((#81459,#81460,#81461,#81462),
(#81463,#81464,#81465,#81466),(#81467,#81468,#81469,#81470),(#81471,#81472,
#81473,#81474)),.UNSPECIFIED.,.F.,.F.,.F.,(4,4),(4,4),(0.522097120207441,
1.00286848452585),(0.0400218729465689,0.0466073985929454),.UNSPECIFIED.);
#2530=B_SPLINE_SURFACE_WITH_KNOTS('',3,3,((#81543,#81544,#81545,#81546),
(#81547,#81548,#81549,#81550),(#81551,#81552,#81553,#81554),(#81555,#81556,
#81557,#81558)),.UNSPECIFIED.,.F.,.F.,.F.,(4,4),(4,4),(0.522097120208268,
1.00286862201145),(0.0300094532292153,0.0365944846647042),.UNSPECIFIED.);
#2531=B_SPLINE_SURFACE_WITH_KNOTS('',3,3,((#81591,#81592,#81593,#81594),
(#81595,#81596,#81597,#81598),(#81599,#81600,#81601,#81602),(#81603,#81604,
#81605,#81606)),.UNSPECIFIED.,.F.,.F.,.F.,(4,4),(4,4),(-0.00600003964319226,
1.00000000663601),(0.0166015299238287,0.0265907346180634),.UNSPECIFIED.);
#2532=B_SPLINE_SURFACE_WITH_KNOTS('',3,3,((#81618,#81619,#81620,#81621),
(#81622,#81623,#81624,#81625),(#81626,#81627,#81628,#81629),(#81630,#81631,
#81632,#81633)),.UNSPECIFIED.,.F.,.F.,.F.,(4,4),(4,4),(0.522097120209615,
1.00286780410456),(0.0200175229646514,0.0265907346180652),.UNSPECIFIED.);
#2533=B_SPLINE_SURFACE_WITH_KNOTS('',3,3,((#81689,#81690,#81691,#81692),
(#81693,#81694,#81695,#81696),(#81697,#81698,#81699,#81700),(#81701,#81702,
#81703,#81704)),.UNSPECIFIED.,.F.,.F.,.F.,(4,4),(4,4),(0.522097120210727,
1.0028679101428),(0.0100271466749319,0.0166015302184276),.UNSPECIFIED.);
#2534=B_SPLINE_SURFACE_WITH_KNOTS('',3,3,((#81730,#81731,#81732,#81733),
(#81734,#81735,#81736,#81737),(#81738,#81739,#81740,#81741),(#81742,#81743,
#81744,#81745)),.UNSPECIFIED.,.F.,.F.,.F.,(4,4),(4,4),(-0.00017189542896064,
1.00600020634802),(0.0665898698856043,0.0751325481068571),.UNSPECIFIED.);
#2535=B_SPLINE_SURFACE_WITH_KNOTS('',3,3,((#81761,#81762,#81763,#81764),
(#81765,#81766,#81767,#81768),(#81769,#81770,#81771,#81772),(#81773,#81774,
#81775,#81776)),.UNSPECIFIED.,.F.,.F.,.F.,(4,4),(4,4),(-0.00286833998593375,
0.47790287978645),(0.0665898698862501,0.07317161987485),.UNSPECIFIED.);
#2536=B_SPLINE_SURFACE_WITH_KNOTS('',3,3,((#81810,#81811,#81812,#81813),
(#81814,#81815,#81816,#81817),(#81818,#81819,#81820,#81821),(#81822,#81823,
#81824,#81825)),.UNSPECIFIED.,.F.,.F.,.F.,(4,4),(4,4),(0.522097120203271,
1.00286791825529),(0.0600156865486934,0.0665898700060131),.UNSPECIFIED.);
#2537=B_SPLINE_SURFACE_WITH_KNOTS('',3,3,((#81835,#81836,#81837,#81838),
(#81839,#81840,#81841,#81842),(#81843,#81844,#81845,#81846),(#81847,#81848,
#81849,#81850)),.UNSPECIFIED.,.F.,.F.,.F.,(4,4),(4,4),(-0.00286764392023632,
0.477902879786599),(0.0565997133101197,0.0631721430887068),
 .UNSPECIFIED.);
#2538=B_SPLINE_SURFACE_WITH_KNOTS('',3,3,((#81887,#81888,#81889,#81890),
(#81891,#81892,#81893,#81894),(#81895,#81896,#81897,#81898),(#81899,#81900,
#81901,#81902)),.UNSPECIFIED.,.F.,.F.,.F.,(4,4),(4,4),(0.522097120204332,
1.00286780122196),(0.0500263550858673,0.0565997133101428),.UNSPECIFIED.);
#2539=B_SPLINE_SURFACE_WITH_KNOTS('',3,3,((#81935,#81936,#81937,#81938),
(#81939,#81940,#81941,#81942),(#81943,#81944,#81945,#81946),(#81947,#81948,
#81949,#81950)),.UNSPECIFIED.,.F.,.F.,.F.,(4,4),(4,4),(-0.00600014643533104,
1.),(0.0365944846640577,0.046607398592944),.UNSPECIFIED.);
#2540=B_SPLINE_SURFACE_WITH_KNOTS('',3,3,((#81973,#81974,#81975,#81976),
(#81977,#81978,#81979,#81980),(#81981,#81982,#81983,#81984),(#81985,#81986,
#81987,#81988)),.UNSPECIFIED.,.F.,.F.,.F.,(4,4),(4,4),(0.522097120205363,
1.00286848452578),(0.0400218729465698,0.0466073985929445),.UNSPECIFIED.);
#2541=B_SPLINE_SURFACE_WITH_KNOTS('',3,3,((#82052,#82053,#82054,#82055),
(#82056,#82057,#82058,#82059),(#82060,#82061,#82062,#82063),(#82064,#82065,
#82066,#82067)),.UNSPECIFIED.,.F.,.F.,.F.,(4,4),(4,4),(0.522097120206,1.00286862201151),
(0.0300094532292161,0.0365944846647034),.UNSPECIFIED.);
#2542=B_SPLINE_SURFACE_WITH_KNOTS('',3,3,((#82100,#82101,#82102,#82103),
(#82104,#82105,#82106,#82107),(#82108,#82109,#82110,#82111),(#82112,#82113,
#82114,#82115)),.UNSPECIFIED.,.F.,.F.,.F.,(4,4),(4,4),(-0.00600003961801213,
1.00000000246949),(0.0166015299238286,0.0265907346180633),.UNSPECIFIED.);
#2543=B_SPLINE_SURFACE_WITH_KNOTS('',3,3,((#82127,#82128,#82129,#82130),
(#82131,#82132,#82133,#82134),(#82135,#82136,#82137,#82138),(#82139,#82140,
#82141,#82142)),.UNSPECIFIED.,.F.,.F.,.F.,(4,4),(4,4),(0.522097120207366,
1.00286780410456),(0.0200175229646512,0.0265907346180654),.UNSPECIFIED.);
#2544=B_SPLINE_SURFACE_WITH_KNOTS('',3,3,((#82198,#82199,#82200,#82201),
(#82202,#82203,#82204,#82205),(#82206,#82207,#82208,#82209),(#82210,#82211,
#82212,#82213)),.UNSPECIFIED.,.F.,.F.,.F.,(4,4),(4,4),(0.522097120208367,
1.00286791014273),(0.0100271466749317,0.0166015302184278),.UNSPECIFIED.);
#2545=B_SPLINE_SURFACE_WITH_KNOTS('',3,3,((#82239,#82240,#82241,#82242),
(#82243,#82244,#82245,#82246),(#82247,#82248,#82249,#82250),(#82251,#82252,
#82253,#82254)),.UNSPECIFIED.,.F.,.F.,.F.,(4,4),(4,4),(-0.000171895428571592,
1.00600020634813),(0.0665898698856047,0.0751325481064681),.UNSPECIFIED.);
#2546=B_SPLINE_SURFACE_WITH_KNOTS('',3,3,((#82270,#82271,#82272,#82273),
(#82274,#82275,#82276,#82277),(#82278,#82279,#82280,#82281),(#82282,#82283,
#82284,#82285)),.UNSPECIFIED.,.F.,.F.,.F.,(4,4),(4,4),(-0.00286833998598749,
0.477902879789405),(0.0665898698862508,0.0731716198748509),
 .UNSPECIFIED.);
#2547=B_SPLINE_SURFACE_WITH_KNOTS('',3,3,((#82319,#82320,#82321,#82322),
(#82323,#82324,#82325,#82326),(#82327,#82328,#82329,#82330),(#82331,#82332,
#82333,#82334)),.UNSPECIFIED.,.F.,.F.,.F.,(4,4),(4,4),(0.52209712020154,
1.00286791825529),(0.0600156865486932,0.0665898700060148),.UNSPECIFIED.);
#2548=B_SPLINE_SURFACE_WITH_KNOTS('',3,3,((#82344,#82345,#82346,#82347),
(#82348,#82349,#82350,#82351),(#82352,#82353,#82354,#82355),(#82356,#82357,
#82358,#82359)),.UNSPECIFIED.,.F.,.F.,.F.,(4,4),(4,4),(-0.00286764392027554,
0.477902879788135),(0.0565997133101202,0.0631721430887068),
 .UNSPECIFIED.);
#2549=B_SPLINE_SURFACE_WITH_KNOTS('',3,3,((#82396,#82397,#82398,#82399),
(#82400,#82401,#82402,#82403),(#82404,#82405,#82406,#82407),(#82408,#82409,
#82410,#82411)),.UNSPECIFIED.,.F.,.F.,.F.,(4,4),(4,4),(0.522097120202531,
1.00286780122197),(0.050026355085867,0.0565997133101419),.UNSPECIFIED.);
#2550=B_SPLINE_SURFACE_WITH_KNOTS('',3,3,((#82483,#82484,#82485,#82486),
(#82487,#82488,#82489,#82490),(#82491,#82492,#82493,#82494),(#82495,#82496,
#82497,#82498)),.UNSPECIFIED.,.F.,.F.,.F.,(4,4),(4,4),(0.522097120203339,
1.00286848452584),(0.0400218729465689,0.0466073985929463),.UNSPECIFIED.);
#2551=B_SPLINE_SURFACE_WITH_KNOTS('',3,3,((#82564,#82565,#82566,#82567),
(#82568,#82569,#82570,#82571),(#82572,#82573,#82574,#82575),(#82576,#82577,
#82578,#82579)),.UNSPECIFIED.,.F.,.F.,.F.,(4,4),(4,4),(0.522097120204001,
1.00286862201145),(0.0300094532292154,0.0365944846647039),.UNSPECIFIED.);
#2552=B_SPLINE_SURFACE_WITH_KNOTS('',3,3,((#82587,#82588,#82589,#82590),
(#82591,#82592,#82593,#82594),(#82595,#82596,#82597,#82598),(#82599,#82600,
#82601,#82602)),.UNSPECIFIED.,.F.,.F.,.F.,(4,4),(4,4),(-0.0028682335621104,
0.477902879786601),(0.026590734618062,0.0331702037252921),.UNSPECIFIED.);
#2553=B_SPLINE_SURFACE_WITH_KNOTS('',3,3,((#82619,#82620,#82621,#82622),
(#82623,#82624,#82625,#82626),(#82627,#82628,#82629,#82630),(#82631,#82632,
#82633,#82634)),.UNSPECIFIED.,.F.,.F.,.F.,(4,4),(4,4),(-0.00600003964307988,
1.00000000663629),(0.0166015299238289,0.0265907346180633),.UNSPECIFIED.);
#2554=B_SPLINE_SURFACE_WITH_KNOTS('',3,3,((#82646,#82647,#82648,#82649),
(#82650,#82651,#82652,#82653),(#82654,#82655,#82656,#82657),(#82658,#82659,
#82660,#82661)),.UNSPECIFIED.,.F.,.F.,.F.,(4,4),(4,4),(0.522097120205243,
1.00286780410455),(0.0200175229646507,0.0265907346180654),.UNSPECIFIED.);
#2555=B_SPLINE_SURFACE_WITH_KNOTS('',3,3,((#82717,#82718,#82719,#82720),
(#82721,#82722,#82723,#82724),(#82725,#82726,#82727,#82728),(#82729,#82730,
#82731,#82732)),.UNSPECIFIED.,.F.,.F.,.F.,(4,4),(4,4),(0.522097120206236,
1.00286791014282),(0.0100271466749313,0.0166015302184277),.UNSPECIFIED.);
#2556=B_SPLINE_SURFACE_WITH_KNOTS('',3,3,((#82758,#82759,#82760,#82761),
(#82762,#82763,#82764,#82765),(#82766,#82767,#82768,#82769),(#82770,#82771,
#82772,#82773)),.UNSPECIFIED.,.F.,.F.,.F.,(4,4),(4,4),(-0.000171895428076154,
1.00600020634796),(0.0665898698856047,0.0751325481059748),.UNSPECIFIED.);
#2557=B_SPLINE_SURFACE_WITH_KNOTS('',3,3,((#82789,#82790,#82791,#82792),
(#82793,#82794,#82795,#82796),(#82797,#82798,#82799,#82800),(#82801,#82802,
#82803,#82804)),.UNSPECIFIED.,.F.,.F.,.F.,(4,4),(4,4),(-0.002868339985951,
0.477902879791939),(0.0665898698862501,0.0731716198748492),
 .UNSPECIFIED.);
#2558=B_SPLINE_SURFACE_WITH_KNOTS('',3,3,((#82838,#82839,#82840,#82841),
(#82842,#82843,#82844,#82845),(#82846,#82847,#82848,#82849),(#82850,#82851,
#82852,#82853)),.UNSPECIFIED.,.F.,.F.,.F.,(4,4),(4,4),(0.522097120200109,
1.00286791825532),(0.0600156865486933,0.0665898700060144),.UNSPECIFIED.);
#2559=B_SPLINE_SURFACE_WITH_KNOTS('',3,3,((#82863,#82864,#82865,#82866),
(#82867,#82868,#82869,#82870),(#82871,#82872,#82873,#82874),(#82875,#82876,
#82877,#82878)),.UNSPECIFIED.,.F.,.F.,.F.,(4,4),(4,4),(-0.00286764392029188,
0.477902879790651),(0.0565997133101211,0.0631721430887068),
 .UNSPECIFIED.);
#2560=B_SPLINE_SURFACE_WITH_KNOTS('',3,3,((#82915,#82916,#82917,#82918),
(#82919,#82920,#82921,#82922),(#82923,#82924,#82925,#82926),(#82927,#82928,
#82929,#82930)),.UNSPECIFIED.,.F.,.F.,.F.,(4,4),(4,4),(0.522097120201025,
1.00286780122203),(0.0500263550858673,0.0565997133101423),.UNSPECIFIED.);
#2561=B_SPLINE_SURFACE_WITH_KNOTS('',3,3,((#83002,#83003,#83004,#83005),
(#83006,#83007,#83008,#83009),(#83010,#83011,#83012,#83013),(#83014,#83015,
#83016,#83017)),.UNSPECIFIED.,.F.,.F.,.F.,(4,4),(4,4),(0.522097120201695,
1.00286848452585),(0.0400218729465699,0.0466073985929445),.UNSPECIFIED.);
#2562=B_SPLINE_SURFACE_WITH_KNOTS('',3,3,((#83086,#83087,#83088,#83089),
(#83090,#83091,#83092,#83093),(#83094,#83095,#83096,#83097),(#83098,#83099,
#83100,#83101)),.UNSPECIFIED.,.F.,.F.,.F.,(4,4),(4,4),(0.522097120202243,
1.00286862201148),(0.0300094532292163,0.0365944846647038),.UNSPECIFIED.);
#2563=B_SPLINE_SURFACE_WITH_KNOTS('',3,3,((#83134,#83135,#83136,#83137),
(#83138,#83139,#83140,#83141),(#83142,#83143,#83144,#83145),(#83146,#83147,
#83148,#83149)),.UNSPECIFIED.,.F.,.F.,.F.,(4,4),(4,4),(-0.00600003960321525,
1.),(0.0166015299238289,0.0265907346180637),.UNSPECIFIED.);
#2564=B_SPLINE_SURFACE_WITH_KNOTS('',3,3,((#83161,#83162,#83163,#83164),
(#83165,#83166,#83167,#83168),(#83169,#83170,#83171,#83172),(#83173,#83174,
#83175,#83176)),.UNSPECIFIED.,.F.,.F.,.F.,(4,4),(4,4),(0.52209712020337,
1.00286780410461),(0.0200175229646522,0.0265907346180655),.UNSPECIFIED.);
#2565=B_SPLINE_SURFACE_WITH_KNOTS('',3,3,((#83184,#83185,#83186,#83187),
(#83188,#83189,#83190,#83191),(#83192,#83193,#83194,#83195),(#83196,#83197,
#83198,#83199)),.UNSPECIFIED.,.F.,.F.,.F.,(4,4),(4,4),(-0.00286753128207834,
0.477902879786653),(0.0166015299238961,0.0231736788111887),
 .UNSPECIFIED.);
#2566=B_SPLINE_SURFACE_WITH_KNOTS('',3,3,((#83239,#83240,#83241,#83242),
(#83243,#83244,#83245,#83246),(#83247,#83248,#83249,#83250),(#83251,#83252,
#83253,#83254)),.UNSPECIFIED.,.F.,.F.,.F.,(4,4),(4,4),(0.522097120204273,
1.00286791014282),(0.0100271466749313,0.0166015302184272),.UNSPECIFIED.);
#2567=B_SPLINE_SURFACE_WITH_KNOTS('',3,3,((#83280,#83281,#83282,#83283),
(#83284,#83285,#83286,#83287),(#83288,#83289,#83290,#83291),(#83292,#83293,
#83294,#83295)),.UNSPECIFIED.,.F.,.F.,.F.,(4,4),(4,4),(-0.000171895427606127,
1.006000206348),(0.0665898698856038,0.0751325481055029),.UNSPECIFIED.);
#2568=B_SPLINE_SURFACE_WITH_KNOTS('',3,3,((#83311,#83312,#83313,#83314),
(#83315,#83316,#83317,#83318),(#83319,#83320,#83321,#83322),(#83323,#83324,
#83325,#83326)),.UNSPECIFIED.,.F.,.F.,.F.,(4,4),(4,4),(-0.00286833998596085,
0.477902879794542),(0.0665898698862505,0.0731716198748491),
 .UNSPECIFIED.);
#2569=B_SPLINE_SURFACE_WITH_KNOTS('',3,3,((#83360,#83361,#83362,#83363),
(#83364,#83365,#83366,#83367),(#83368,#83369,#83370,#83371),(#83372,#83373,
#83374,#83375)),.UNSPECIFIED.,.F.,.F.,.F.,(4,4),(4,4),(0.522097120198851,
1.00286791825524),(0.060015686548694,0.0665898700060149),.UNSPECIFIED.);
#2570=B_SPLINE_SURFACE_WITH_KNOTS('',3,3,((#83385,#83386,#83387,#83388),
(#83389,#83390,#83391,#83392),(#83393,#83394,#83395,#83396),(#83397,#83398,
#83399,#83400)),.UNSPECIFIED.,.F.,.F.,.F.,(4,4),(4,4),(-0.00286764392021428,
0.477902879793322),(0.0565997133101211,0.063172143088707),.UNSPECIFIED.);
#2571=B_SPLINE_SURFACE_WITH_KNOTS('',3,3,((#83437,#83438,#83439,#83440),
(#83441,#83442,#83443,#83444),(#83445,#83446,#83447,#83448),(#83449,#83450,
#83451,#83452)),.UNSPECIFIED.,.F.,.F.,.F.,(4,4),(4,4),(0.522097120199709,
1.00286780122204),(0.0500263550858672,0.056599713310143),.UNSPECIFIED.);
#2572=B_SPLINE_SURFACE_WITH_KNOTS('',3,3,((#83524,#83525,#83526,#83527),
(#83528,#83529,#83530,#83531),(#83532,#83533,#83534,#83535),(#83536,#83537,
#83538,#83539)),.UNSPECIFIED.,.F.,.F.,.F.,(4,4),(4,4),(0.52209712020022,
1.00286848452585),(0.0400218729465699,0.0466073985929449),.UNSPECIFIED.);
#2573=B_SPLINE_SURFACE_WITH_KNOTS('',3,3,((#83608,#83609,#83610,#83611),
(#83612,#83613,#83614,#83615),(#83616,#83617,#83618,#83619),(#83620,#83621,
#83622,#83623)),.UNSPECIFIED.,.F.,.F.,.F.,(4,4),(4,4),(0.522097120200653,
1.00286862201151),(0.0300094532292151,0.0365944846647036),.UNSPECIFIED.);
#2574=B_SPLINE_SURFACE_WITH_KNOTS('',3,3,((#83656,#83657,#83658,#83659),
(#83660,#83661,#83662,#83663),(#83664,#83665,#83666,#83667),(#83668,#83669,
#83670,#83671)),.UNSPECIFIED.,.F.,.F.,.F.,(4,4),(4,4),(-0.0060000396247756,
1.00000000356517),(0.0166015299238288,0.0265907346180661),.UNSPECIFIED.);
#2575=B_SPLINE_SURFACE_WITH_KNOTS('',3,3,((#83683,#83684,#83685,#83686),
(#83687,#83688,#83689,#83690),(#83691,#83692,#83693,#83694),(#83695,#83696,
#83697,#83698)),.UNSPECIFIED.,.F.,.F.,.F.,(4,4),(4,4),(0.522097120201635,
1.0028678041046),(0.020017522964651,0.0265907346180654),.UNSPECIFIED.);
#2576=B_SPLINE_SURFACE_WITH_KNOTS('',3,3,((#83751,#83752,#83753,#83754),
(#83755,#83756,#83757,#83758),(#83759,#83760,#83761,#83762),(#83763,#83764,
#83765,#83766)),.UNSPECIFIED.,.F.,.F.,.F.,(4,4),(4,4),(0.522097120202428,
1.00286791014283),(0.0100271466749307,0.0166015302184278),.UNSPECIFIED.);
#2577=B_SPLINE_SURFACE_WITH_KNOTS('',3,3,((#83774,#83775,#83776,#83777),
(#83778,#83779,#83780,#83781),(#83782,#83783,#83784,#83785),(#83786,#83787,
#83788,#83789)),.UNSPECIFIED.,.F.,.F.,.F.,(4,4),(4,4),(-0.00206901892602344,
0.346769728504638),(0.00660713154698981,0.0131849431468423),
 .UNSPECIFIED.);
#2578=B_SPLINE_SURFACE_WITH_KNOTS('',3,3,((#83799,#83800,#83801,#83802),
(#83803,#83804,#83805,#83806),(#83807,#83808,#83809,#83810),(#83811,#83812,
#83813,#83814)),.UNSPECIFIED.,.F.,.F.,.F.,(4,4),(4,4),(-0.000171895427410773,
1.00600020634837),(0.0665898698856052,0.0751325481053073),.UNSPECIFIED.);
#2579=B_SPLINE_SURFACE_WITH_KNOTS('',3,3,((#83830,#83831,#83832,#83833),
(#83834,#83835,#83836,#83837),(#83838,#83839,#83840,#83841),(#83842,#83843,
#83844,#83845)),.UNSPECIFIED.,.F.,.F.,.F.,(4,4),(4,4),(-0.00286833998591909,
0.477902879796992),(0.0665898698862512,0.0731716198748501),
 .UNSPECIFIED.);
#2580=B_SPLINE_SURFACE_WITH_KNOTS('',3,3,((#83879,#83880,#83881,#83882),
(#83883,#83884,#83885,#83886),(#83887,#83888,#83889,#83890),(#83891,#83892,
#83893,#83894)),.UNSPECIFIED.,.F.,.F.,.F.,(4,4),(4,4),(0.522097120197966,
1.00286791825531),(0.0600156865486934,0.0665898700060137),.UNSPECIFIED.);
#2581=B_SPLINE_SURFACE_WITH_KNOTS('',3,3,((#83904,#83905,#83906,#83907),
(#83908,#83909,#83910,#83911),(#83912,#83913,#83914,#83915),(#83916,#83917,
#83918,#83919)),.UNSPECIFIED.,.F.,.F.,.F.,(4,4),(4,4),(-0.00286764392030516,
0.477902879795798),(0.0565997133101207,0.0631721430887073),
 .UNSPECIFIED.);
#2582=B_SPLINE_SURFACE_WITH_KNOTS('',3,3,((#83956,#83957,#83958,#83959),
(#83960,#83961,#83962,#83963),(#83964,#83965,#83966,#83967),(#83968,#83969,
#83970,#83971)),.UNSPECIFIED.,.F.,.F.,.F.,(4,4),(4,4),(0.522097120198643,
1.00286780122203),(0.0500263550858678,0.0565997133101423),.UNSPECIFIED.);
#2583=B_SPLINE_SURFACE_WITH_KNOTS('',3,3,((#84043,#84044,#84045,#84046),
(#84047,#84048,#84049,#84050),(#84051,#84052,#84053,#84054),(#84055,#84056,
#84057,#84058)),.UNSPECIFIED.,.F.,.F.,.F.,(4,4),(4,4),(0.52209712019902,
1.00286848452579),(0.0400218729465707,0.0466073985929451),.UNSPECIFIED.);
#2584=B_SPLINE_SURFACE_WITH_KNOTS('',3,3,((#84127,#84128,#84129,#84130),
(#84131,#84132,#84133,#84134),(#84135,#84136,#84137,#84138),(#84139,#84140,
#84141,#84142)),.UNSPECIFIED.,.F.,.F.,.F.,(4,4),(4,4),(0.522097120199269,
1.00286862201159),(0.0300094532292162,0.0365944846647032),.UNSPECIFIED.);
#2585=B_SPLINE_SURFACE_WITH_KNOTS('',3,3,((#84175,#84176,#84177,#84178),
(#84179,#84180,#84181,#84182),(#84183,#84184,#84185,#84186),(#84187,#84188,
#84189,#84190)),.UNSPECIFIED.,.F.,.F.,.F.,(4,4),(4,4),(-0.00600003962464963,
1.00000000356543),(0.0166015299238286,0.026590734618064),.UNSPECIFIED.);
#2586=B_SPLINE_SURFACE_WITH_KNOTS('',3,3,((#84202,#84203,#84204,#84205),
(#84206,#84207,#84208,#84209),(#84210,#84211,#84212,#84213),(#84214,#84215,
#84216,#84217)),.UNSPECIFIED.,.F.,.F.,.F.,(4,4),(4,4),(0.522097120200225,
1.00286780410463),(0.0200175229646515,0.0265907346180643),.UNSPECIFIED.);
#2587=B_SPLINE_SURFACE_WITH_KNOTS('',3,3,((#84273,#84274,#84275,#84276),
(#84277,#84278,#84279,#84280),(#84281,#84282,#84283,#84284),(#84285,#84286,
#84287,#84288)),.UNSPECIFIED.,.F.,.F.,.F.,(4,4),(4,4),(0.522097120200841,
1.00286791014282),(0.0100271466749316,0.0166015302184268),.UNSPECIFIED.);
#2588=B_SPLINE_SURFACE_WITH_KNOTS('',3,3,((#84314,#84315,#84316,#84317),
(#84318,#84319,#84320,#84321),(#84322,#84323,#84324,#84325),(#84326,#84327,
#84328,#84329)),.UNSPECIFIED.,.F.,.F.,.F.,(4,4),(4,4),(-0.00017189542728392,
1.00600020634822),(0.0665898698856043,0.0751325481051806),.UNSPECIFIED.);
#2589=B_SPLINE_SURFACE_WITH_KNOTS('',3,3,((#84345,#84346,#84347,#84348),
(#84349,#84350,#84351,#84352),(#84353,#84354,#84355,#84356),(#84357,#84358,
#84359,#84360)),.UNSPECIFIED.,.F.,.F.,.F.,(4,4),(4,4),(-0.00286833998600279,
0.47790287979949),(0.0665898698862503,0.0731716198748491),.UNSPECIFIED.);
#2590=B_SPLINE_SURFACE_WITH_KNOTS('',3,3,((#84394,#84395,#84396,#84397),
(#84398,#84399,#84400,#84401),(#84402,#84403,#84404,#84405),(#84406,#84407,
#84408,#84409)),.UNSPECIFIED.,.F.,.F.,.F.,(4,4),(4,4),(0.522097120197419,
1.00286791825534),(0.0600156865486943,0.0665898700060139),.UNSPECIFIED.);
#2591=B_SPLINE_SURFACE_WITH_KNOTS('',3,3,((#84419,#84420,#84421,#84422),
(#84423,#84424,#84425,#84426),(#84427,#84428,#84429,#84430),(#84431,#84432,
#84433,#84434)),.UNSPECIFIED.,.F.,.F.,.F.,(4,4),(4,4),(-0.00286764392029051,
0.477902879798242),(0.0565997133101205,0.0631721430887056),
 .UNSPECIFIED.);
#2592=B_SPLINE_SURFACE_WITH_KNOTS('',3,3,((#84471,#84472,#84473,#84474),
(#84475,#84476,#84477,#84478),(#84479,#84480,#84481,#84482),(#84483,#84484,
#84485,#84486)),.UNSPECIFIED.,.F.,.F.,.F.,(4,4),(4,4),(0.522097120197909,
1.00286780122208),(0.0500263550858677,0.0565997133101417),.UNSPECIFIED.);
#2593=B_SPLINE_SURFACE_WITH_KNOTS('',3,3,((#84558,#84559,#84560,#84561),
(#84562,#84563,#84564,#84565),(#84566,#84567,#84568,#84569),(#84570,#84571,
#84572,#84573)),.UNSPECIFIED.,.F.,.F.,.F.,(4,4),(4,4),(0.522097120198037,
1.00286848452582),(0.0400218729465713,0.0466073985929447),.UNSPECIFIED.);
#2594=B_SPLINE_SURFACE_WITH_KNOTS('',3,3,((#84642,#84643,#84644,#84645),
(#84646,#84647,#84648,#84649),(#84650,#84651,#84652,#84653),(#84654,#84655,
#84656,#84657)),.UNSPECIFIED.,.F.,.F.,.F.,(4,4),(4,4),(0.522097120198327,
1.00286862201147),(0.0300094532292163,0.0365944846647041),.UNSPECIFIED.);
#2595=B_SPLINE_SURFACE_WITH_KNOTS('',3,3,((#84690,#84691,#84692,#84693),
(#84694,#84695,#84696,#84697),(#84698,#84699,#84700,#84701),(#84702,#84703,
#84704,#84705)),.UNSPECIFIED.,.F.,.F.,.F.,(4,4),(4,4),(-0.00600003962474401,
1.00000000356551),(0.0166015299238287,0.0265907346180634),.UNSPECIFIED.);
#2596=B_SPLINE_SURFACE_WITH_KNOTS('',3,3,((#84717,#84718,#84719,#84720),
(#84721,#84722,#84723,#84724),(#84725,#84726,#84727,#84728),(#84729,#84730,
#84731,#84732)),.UNSPECIFIED.,.F.,.F.,.F.,(4,4),(4,4),(0.522097120199008,
1.00286780410468),(0.020017522964651,0.0265907346180643),.UNSPECIFIED.);
#2597=B_SPLINE_SURFACE_WITH_KNOTS('',3,3,((#84788,#84789,#84790,#84791),
(#84792,#84793,#84794,#84795),(#84796,#84797,#84798,#84799),(#84800,#84801,
#84802,#84803)),.UNSPECIFIED.,.F.,.F.,.F.,(4,4),(4,4),(0.522097120199533,
1.00286791014275),(0.0100271466749321,0.0166015302184269),.UNSPECIFIED.);
#2598=B_SPLINE_SURFACE_WITH_KNOTS('',3,3,((#84829,#84830,#84831,#84832),
(#84833,#84834,#84835,#84836),(#84837,#84838,#84839,#84840),(#84841,#84842,
#84843,#84844)),.UNSPECIFIED.,.F.,.F.,.F.,(4,4),(4,4),(-0.000171895427232253,
1.00600020634838),(0.0665898698856038,0.0751325481051289),.UNSPECIFIED.);
#2599=B_SPLINE_SURFACE_WITH_KNOTS('',3,3,((#84860,#84861,#84862,#84863),
(#84864,#84865,#84866,#84867),(#84868,#84869,#84870,#84871),(#84872,#84873,
#84874,#84875)),.UNSPECIFIED.,.F.,.F.,.F.,(4,4),(4,4),(-0.00286833998594681,
0.477902879801946),(0.0665898698862508,0.0731716198748497),
 .UNSPECIFIED.);
#2600=B_SPLINE_SURFACE_WITH_KNOTS('',3,3,((#84909,#84910,#84911,#84912),
(#84913,#84914,#84915,#84916),(#84917,#84918,#84919,#84920),(#84921,#84922,
#84923,#84924)),.UNSPECIFIED.,.F.,.F.,.F.,(4,4),(4,4),(0.522097120197177,
1.00286791825534),(0.0600156865486938,0.0665898700060139),.UNSPECIFIED.);
#2601=B_SPLINE_SURFACE_WITH_KNOTS('',3,3,((#84934,#84935,#84936,#84937),
(#84938,#84939,#84940,#84941),(#84942,#84943,#84944,#84945),(#84946,#84947,
#84948,#84949)),.UNSPECIFIED.,.F.,.F.,.F.,(4,4),(4,4),(-0.00286764392033648,
0.477902879800479),(0.056599713310121,0.0631721430887073),.UNSPECIFIED.);
#2602=B_SPLINE_SURFACE_WITH_KNOTS('',3,3,((#84986,#84987,#84988,#84989),
(#84990,#84991,#84992,#84993),(#84994,#84995,#84996,#84997),(#84998,#84999,
#85000,#85001)),.UNSPECIFIED.,.F.,.F.,.F.,(4,4),(4,4),(0.522097120197487,
1.00286780122204),(0.0500263550858663,0.0565997133101417),.UNSPECIFIED.);
#2603=B_SPLINE_SURFACE_WITH_KNOTS('',3,3,((#85073,#85074,#85075,#85076),
(#85077,#85078,#85079,#85080),(#85081,#85082,#85083,#85084),(#85085,#85086,
#85087,#85088)),.UNSPECIFIED.,.F.,.F.,.F.,(4,4),(4,4),(0.522097120197465,
1.00286848452583),(0.0400218729465712,0.0466073985929438),.UNSPECIFIED.);
#2604=B_SPLINE_SURFACE_WITH_KNOTS('',3,3,((#85157,#85158,#85159,#85160),
(#85161,#85162,#85163,#85164),(#85165,#85166,#85167,#85168),(#85169,#85170,
#85171,#85172)),.UNSPECIFIED.,.F.,.F.,.F.,(4,4),(4,4),(0.52209712019751,
1.00286862201153),(0.030009453229217,0.0365944846647047),.UNSPECIFIED.);
#2605=B_SPLINE_SURFACE_WITH_KNOTS('',3,3,((#85205,#85206,#85207,#85208),
(#85209,#85210,#85211,#85212),(#85213,#85214,#85215,#85216),(#85217,#85218,
#85219,#85220)),.UNSPECIFIED.,.F.,.F.,.F.,(4,4),(4,4),(-0.00600003961810723,
1.00000000246924),(0.0166015299238289,0.0265907346180637),.UNSPECIFIED.);
#2606=B_SPLINE_SURFACE_WITH_KNOTS('',3,3,((#85232,#85233,#85234,#85235),
(#85236,#85237,#85238,#85239),(#85240,#85241,#85242,#85243),(#85244,#85245,
#85246,#85247)),.UNSPECIFIED.,.F.,.F.,.F.,(4,4),(4,4),(0.522097120198131,
1.00286780410467),(0.020017522964652,0.0265907346180655),.UNSPECIFIED.);
#2607=B_SPLINE_SURFACE_WITH_KNOTS('',3,3,((#85303,#85304,#85305,#85306),
(#85307,#85308,#85309,#85310),(#85311,#85312,#85313,#85314),(#85315,#85316,
#85317,#85318)),.UNSPECIFIED.,.F.,.F.,.F.,(4,4),(4,4),(0.522097120198457,
1.00286791014282),(0.0100271466749326,0.0166015302184268),.UNSPECIFIED.);
#2608=B_SPLINE_SURFACE_WITH_KNOTS('',3,3,((#85344,#85345,#85346,#85347),
(#85348,#85349,#85350,#85351),(#85352,#85353,#85354,#85355),(#85356,#85357,
#85358,#85359)),.UNSPECIFIED.,.F.,.F.,.F.,(4,4),(4,4),(-0.000171895427308574,
1.00600020634819),(0.0665898698856039,0.075132548105205),.UNSPECIFIED.);
#2609=B_SPLINE_SURFACE_WITH_KNOTS('',3,3,((#85375,#85376,#85377,#85378),
(#85379,#85380,#85381,#85382),(#85383,#85384,#85385,#85386),(#85387,#85388,
#85389,#85390)),.UNSPECIFIED.,.F.,.F.,.F.,(4,4),(4,4),(-0.00286833998600449,
0.477902879804012),(0.0665898698862502,0.0731716198748502),
 .UNSPECIFIED.);
#2610=B_SPLINE_SURFACE_WITH_KNOTS('',3,3,((#85424,#85425,#85426,#85427),
(#85428,#85429,#85430,#85431),(#85432,#85433,#85434,#85435),(#85436,#85437,
#85438,#85439)),.UNSPECIFIED.,.F.,.F.,.F.,(4,4),(4,4),(0.522097120197181,
1.00286791825527),(0.060015686548694,0.0665898700060143),.UNSPECIFIED.);
#2611=B_SPLINE_SURFACE_WITH_KNOTS('',3,3,((#85449,#85450,#85451,#85452),
(#85453,#85454,#85455,#85456),(#85457,#85458,#85459,#85460),(#85461,#85462,
#85463,#85464)),.UNSPECIFIED.,.F.,.F.,.F.,(4,4),(4,4),(-0.0028676439203597,
0.477902879802986),(0.0565997133101214,0.0631721430887067),
 .UNSPECIFIED.);
#2612=B_SPLINE_SURFACE_WITH_KNOTS('',3,3,((#85501,#85502,#85503,#85504),
(#85505,#85506,#85507,#85508),(#85509,#85510,#85511,#85512),(#85513,#85514,
#85515,#85516)),.UNSPECIFIED.,.F.,.F.,.F.,(4,4),(4,4),(0.522097120197347,
1.00286780122201),(0.050026355085867,0.0565997133101426),.UNSPECIFIED.);
#2613=B_SPLINE_SURFACE_WITH_KNOTS('',3,3,((#85588,#85589,#85590,#85591),
(#85592,#85593,#85594,#85595),(#85596,#85597,#85598,#85599),(#85600,#85601,
#85602,#85603)),.UNSPECIFIED.,.F.,.F.,.F.,(4,4),(4,4),(0.522097120197233,
1.00286848452581),(0.0400218729465715,0.0466073985929451),.UNSPECIFIED.);
#2614=B_SPLINE_SURFACE_WITH_KNOTS('',3,3,((#85672,#85673,#85674,#85675),
(#85676,#85677,#85678,#85679),(#85680,#85681,#85682,#85683),(#85684,#85685,
#85686,#85687)),.UNSPECIFIED.,.F.,.F.,.F.,(4,4),(4,4),(0.522097120197018,
1.0028686220116),(0.0300094532292167,0.0365944846647034),.UNSPECIFIED.);
#2615=B_SPLINE_SURFACE_WITH_KNOTS('',3,3,((#85720,#85721,#85722,#85723),
(#85724,#85725,#85726,#85727),(#85728,#85729,#85730,#85731),(#85732,#85733,
#85734,#85735)),.UNSPECIFIED.,.F.,.F.,.F.,(4,4),(4,4),(-0.00600003961809443,
1.00000000246919),(0.0166015299238287,0.0265907346180648),.UNSPECIFIED.);
#2616=B_SPLINE_SURFACE_WITH_KNOTS('',3,3,((#85747,#85748,#85749,#85750),
(#85751,#85752,#85753,#85754),(#85755,#85756,#85757,#85758),(#85759,#85760,
#85761,#85762)),.UNSPECIFIED.,.F.,.F.,.F.,(4,4),(4,4),(0.522097120197489,
1.00286780410464),(0.020017522964652,0.0265907346180644),.UNSPECIFIED.);
#2617=B_SPLINE_SURFACE_WITH_KNOTS('',3,3,((#85818,#85819,#85820,#85821),
(#85822,#85823,#85824,#85825),(#85826,#85827,#85828,#85829),(#85830,#85831,
#85832,#85833)),.UNSPECIFIED.,.F.,.F.,.F.,(4,4),(4,4),(0.522097120197819,
1.00286791014287),(0.010027146674932,0.0166015302184279),.UNSPECIFIED.);
#2618=B_SPLINE_SURFACE_WITH_KNOTS('',3,3,((#85859,#85860,#85861,#85862),
(#85863,#85864,#85865,#85866),(#85867,#85868,#85869,#85870),(#85871,#85872,
#85873,#85874)),.UNSPECIFIED.,.F.,.F.,.F.,(4,4),(4,4),(-0.000171895427393694,
1.00600020634845),(0.0665898698856037,0.0751325481052895),.UNSPECIFIED.);
#2619=B_SPLINE_SURFACE_WITH_KNOTS('',3,3,((#85890,#85891,#85892,#85893),
(#85894,#85895,#85896,#85897),(#85898,#85899,#85900,#85901),(#85902,#85903,
#85904,#85905)),.UNSPECIFIED.,.F.,.F.,.F.,(4,4),(4,4),(-0.00286833998598056,
0.47790287980605),(0.0665898698862503,0.07317161987485),.UNSPECIFIED.);
#2620=B_SPLINE_SURFACE_WITH_KNOTS('',3,3,((#85939,#85940,#85941,#85942),
(#85943,#85944,#85945,#85946),(#85947,#85948,#85949,#85950),(#85951,#85952,
#85953,#85954)),.UNSPECIFIED.,.F.,.F.,.F.,(4,4),(4,4),(0.522097120197503,
1.00286791825538),(0.0600156865486932,0.066589870006015),.UNSPECIFIED.);
#2621=B_SPLINE_SURFACE_WITH_KNOTS('',3,3,((#85964,#85965,#85966,#85967),
(#85968,#85969,#85970,#85971),(#85972,#85973,#85974,#85975),(#85976,#85977,
#85978,#85979)),.UNSPECIFIED.,.F.,.F.,.F.,(4,4),(4,4),(-0.00286764392038191,
0.477902879804341),(0.0565997133101219,0.063172143088707),.UNSPECIFIED.);
#2622=B_SPLINE_SURFACE_WITH_KNOTS('',3,3,((#86016,#86017,#86018,#86019),
(#86020,#86021,#86022,#86023),(#86024,#86025,#86026,#86027),(#86028,#86029,
#86030,#86031)),.UNSPECIFIED.,.F.,.F.,.F.,(4,4),(4,4),(0.522097120197698,
1.00286780122194),(0.0500263550858669,0.0565997133101426),.UNSPECIFIED.);
#2623=B_SPLINE_SURFACE_WITH_KNOTS('',3,3,((#86103,#86104,#86105,#86106),
(#86107,#86108,#86109,#86110),(#86111,#86112,#86113,#86114),(#86115,#86116,
#86117,#86118)),.UNSPECIFIED.,.F.,.F.,.F.,(4,4),(4,4),(0.522097120197408,
1.00286848452587),(0.0400218729465692,0.0466073985929454),.UNSPECIFIED.);
#2624=B_SPLINE_SURFACE_WITH_KNOTS('',3,3,((#86187,#86188,#86189,#86190),
(#86191,#86192,#86193,#86194),(#86195,#86196,#86197,#86198),(#86199,#86200,
#86201,#86202)),.UNSPECIFIED.,.F.,.F.,.F.,(4,4),(4,4),(0.522097120197092,
1.00286862201155),(0.0300094532292162,0.0365944846647039),.UNSPECIFIED.);
#2625=B_SPLINE_SURFACE_WITH_KNOTS('',3,3,((#86235,#86236,#86237,#86238),
(#86239,#86240,#86241,#86242),(#86243,#86244,#86245,#86246),(#86247,#86248,
#86249,#86250)),.UNSPECIFIED.,.F.,.F.,.F.,(4,4),(4,4),(-0.00600003961847192,
1.00000000246937),(0.0166015299238286,0.0265907346180649),.UNSPECIFIED.);
#2626=B_SPLINE_SURFACE_WITH_KNOTS('',3,3,((#86262,#86263,#86264,#86265),
(#86266,#86267,#86268,#86269),(#86270,#86271,#86272,#86273),(#86274,#86275,
#86276,#86277)),.UNSPECIFIED.,.F.,.F.,.F.,(4,4),(4,4),(0.522097120197192,
1.00286780410466),(0.020017522964651,0.0265907346180642),.UNSPECIFIED.);
#2627=B_SPLINE_SURFACE_WITH_KNOTS('',3,3,((#86333,#86334,#86335,#86336),
(#86337,#86338,#86339,#86340),(#86341,#86342,#86343,#86344),(#86345,#86346,
#86347,#86348)),.UNSPECIFIED.,.F.,.F.,.F.,(4,4),(4,4),(0.522097120197277,
1.00286791014289),(0.0100271466749306,0.0166015302184277),.UNSPECIFIED.);
#2628=B_SPLINE_SURFACE_WITH_KNOTS('',3,3,((#86374,#86375,#86376,#86377),
(#86378,#86379,#86380,#86381),(#86382,#86383,#86384,#86385),(#86386,#86387,
#86388,#86389)),.UNSPECIFIED.,.F.,.F.,.F.,(4,4),(4,4),(-0.000171895427889023,
1.00600020634831),(0.0665898698856037,0.0751325481057876),.UNSPECIFIED.);
#2629=B_SPLINE_SURFACE_WITH_KNOTS('',3,3,((#86405,#86406,#86407,#86408),
(#86409,#86410,#86411,#86412),(#86413,#86414,#86415,#86416),(#86417,#86418,
#86419,#86420)),.UNSPECIFIED.,.F.,.F.,.F.,(4,4),(4,4),(-0.00286833998599298,
0.477902879807884),(0.0665898698862499,0.0731716198748494),
 .UNSPECIFIED.);
#2630=B_SPLINE_SURFACE_WITH_KNOTS('',3,3,((#86454,#86455,#86456,#86457),
(#86458,#86459,#86460,#86461),(#86462,#86463,#86464,#86465),(#86466,#86467,
#86468,#86469)),.UNSPECIFIED.,.F.,.F.,.F.,(4,4),(4,4),(0.522097120198093,
1.00286791825529),(0.0600156865486939,0.0665898700060143),.UNSPECIFIED.);
#2631=B_SPLINE_SURFACE_WITH_KNOTS('',3,3,((#86479,#86480,#86481,#86482),
(#86483,#86484,#86485,#86486),(#86487,#86488,#86489,#86490),(#86491,#86492,
#86493,#86494)),.UNSPECIFIED.,.F.,.F.,.F.,(4,4),(4,4),(-0.00286764392039988,
0.477902879805311),(0.0565997133101209,0.0631721430887081),
 .UNSPECIFIED.);
#2632=B_SPLINE_SURFACE_WITH_KNOTS('',3,3,((#86531,#86532,#86533,#86534),
(#86535,#86536,#86537,#86538),(#86539,#86540,#86541,#86542),(#86543,#86544,
#86545,#86546)),.UNSPECIFIED.,.F.,.F.,.F.,(4,4),(4,4),(0.522097120198022,
1.00286780122197),(0.0500263550858675,0.0565997133101425),.UNSPECIFIED.);
#2633=B_SPLINE_SURFACE_WITH_KNOTS('',3,3,((#86618,#86619,#86620,#86621),
(#86622,#86623,#86624,#86625),(#86626,#86627,#86628,#86629),(#86630,#86631,
#86632,#86633)),.UNSPECIFIED.,.F.,.F.,.F.,(4,4),(4,4),(0.522097120197733,
1.00286848452573),(0.0400218729465702,0.046607398592945),.UNSPECIFIED.);
#2634=B_SPLINE_SURFACE_WITH_KNOTS('',3,3,((#86702,#86703,#86704,#86705),
(#86706,#86707,#86708,#86709),(#86710,#86711,#86712,#86713),(#86714,#86715,
#86716,#86717)),.UNSPECIFIED.,.F.,.F.,.F.,(4,4),(4,4),(0.522097120197201,
1.00286862201148),(0.0300094532292163,0.0365944846647032),.UNSPECIFIED.);
#2635=B_SPLINE_SURFACE_WITH_KNOTS('',3,3,((#86750,#86751,#86752,#86753),
(#86754,#86755,#86756,#86757),(#86758,#86759,#86760,#86761),(#86762,#86763,
#86764,#86765)),.UNSPECIFIED.,.F.,.F.,.F.,(4,4),(4,4),(-0.006000039618272,
1.00000000246948),(0.0166015299238286,0.0265907346180638),.UNSPECIFIED.);
#2636=B_SPLINE_SURFACE_WITH_KNOTS('',3,3,((#86777,#86778,#86779,#86780),
(#86781,#86782,#86783,#86784),(#86785,#86786,#86787,#86788),(#86789,#86790,
#86791,#86792)),.UNSPECIFIED.,.F.,.F.,.F.,(4,4),(4,4),(0.522097120197316,
1.00286780410477),(0.0200175229646532,0.0265907346180642),.UNSPECIFIED.);
#2637=B_SPLINE_SURFACE_WITH_KNOTS('',3,3,((#86848,#86849,#86850,#86851),
(#86852,#86853,#86854,#86855),(#86856,#86857,#86858,#86859),(#86860,#86861,
#86862,#86863)),.UNSPECIFIED.,.F.,.F.,.F.,(4,4),(4,4),(0.522097120197198,
1.00286791014281),(0.0100271466749316,0.0166015302184268),.UNSPECIFIED.);
#2638=B_SPLINE_SURFACE_WITH_KNOTS('',3,3,((#86889,#86890,#86891,#86892),
(#86893,#86894,#86895,#86896),(#86897,#86898,#86899,#86900),(#86901,#86902,
#86903,#86904)),.UNSPECIFIED.,.F.,.F.,.F.,(4,4),(4,4),(-0.000171895428070672,
1.00600020634857),(0.0665898698856042,0.0751325481059675),.UNSPECIFIED.);
#2639=B_SPLINE_SURFACE_WITH_KNOTS('',3,3,((#86920,#86921,#86922,#86923),
(#86924,#86925,#86926,#86927),(#86928,#86929,#86930,#86931),(#86932,#86933,
#86934,#86935)),.UNSPECIFIED.,.F.,.F.,.F.,(4,4),(4,4),(-0.00286833998598336,
0.47790287980941),(0.0665898698862507,0.0731716198748504),.UNSPECIFIED.);
#2640=B_SPLINE_SURFACE_WITH_KNOTS('',3,3,((#86969,#86970,#86971,#86972),
(#86973,#86974,#86975,#86976),(#86977,#86978,#86979,#86980),(#86981,#86982,
#86983,#86984)),.UNSPECIFIED.,.F.,.F.,.F.,(4,4),(4,4),(0.522097120199068,
1.00286791825529),(0.0600156865486931,0.0665898700060154),.UNSPECIFIED.);
#2641=B_SPLINE_SURFACE_WITH_KNOTS('',3,3,((#86994,#86995,#86996,#86997),
(#86998,#86999,#87000,#87001),(#87002,#87003,#87004,#87005),(#87006,#87007,
#87008,#87009)),.UNSPECIFIED.,.F.,.F.,.F.,(4,4),(4,4),(-0.00286764392030641,
0.477902879806162),(0.0565997133101207,0.0631721430887058),
 .UNSPECIFIED.);
#2642=B_SPLINE_SURFACE_WITH_KNOTS('',3,3,((#87046,#87047,#87048,#87049),
(#87050,#87051,#87052,#87053),(#87054,#87055,#87056,#87057),(#87058,#87059,
#87060,#87061)),.UNSPECIFIED.,.F.,.F.,.F.,(4,4),(4,4),(0.522097120198757,
1.00286780122195),(0.0500263550858673,0.0565997133101423),.UNSPECIFIED.);
#2643=B_SPLINE_SURFACE_WITH_KNOTS('',3,3,((#87133,#87134,#87135,#87136),
(#87137,#87138,#87139,#87140),(#87141,#87142,#87143,#87144),(#87145,#87146,
#87147,#87148)),.UNSPECIFIED.,.F.,.F.,.F.,(4,4),(4,4),(0.52209712019838,
1.00286848452582),(0.0400218729465696,0.046607398592946),.UNSPECIFIED.);
#2644=B_SPLINE_SURFACE_WITH_KNOTS('',3,3,((#87217,#87218,#87219,#87220),
(#87221,#87222,#87223,#87224),(#87225,#87226,#87227,#87228),(#87229,#87230,
#87231,#87232)),.UNSPECIFIED.,.F.,.F.,.F.,(4,4),(4,4),(0.522097120197711,
1.00286862201152),(0.0300094532292164,0.0365944846647043),.UNSPECIFIED.);
#2645=B_SPLINE_SURFACE_WITH_KNOTS('',3,3,((#87265,#87266,#87267,#87268),
(#87269,#87270,#87271,#87272),(#87273,#87274,#87275,#87276),(#87277,#87278,
#87279,#87280)),.UNSPECIFIED.,.F.,.F.,.F.,(4,4),(4,4),(-0.00600003964343286,
1.00000000663609),(0.0166015299238276,0.0265907346180635),.UNSPECIFIED.);
#2646=B_SPLINE_SURFACE_WITH_KNOTS('',3,3,((#87292,#87293,#87294,#87295),
(#87296,#87297,#87298,#87299),(#87300,#87301,#87302,#87303),(#87304,#87305,
#87306,#87307)),.UNSPECIFIED.,.F.,.F.,.F.,(4,4),(4,4),(0.522097120197779,
1.0028678041047),(0.0200175229646511,0.0265907346180654),.UNSPECIFIED.);
#2647=B_SPLINE_SURFACE_WITH_KNOTS('',3,3,((#87363,#87364,#87365,#87366),
(#87367,#87368,#87369,#87370),(#87371,#87372,#87373,#87374),(#87375,#87376,
#87377,#87378)),.UNSPECIFIED.,.F.,.F.,.F.,(4,4),(4,4),(0.52209712019753,
1.00286791014286),(0.0100271466749306,0.0166015302184279),.UNSPECIFIED.);
#2648=B_SPLINE_SURFACE_WITH_KNOTS('',3,3,((#87404,#87405,#87406,#87407),
(#87408,#87409,#87410,#87411),(#87412,#87413,#87414,#87415),(#87416,#87417,
#87418,#87419)),.UNSPECIFIED.,.F.,.F.,.F.,(4,4),(4,4),(-0.000171895428638224,
1.00600020634821),(0.0665898698856058,0.0751325481065355),.UNSPECIFIED.);
#2649=B_SPLINE_SURFACE_WITH_KNOTS('',3,3,((#87435,#87436,#87437,#87438),
(#87439,#87440,#87441,#87442),(#87443,#87444,#87445,#87446),(#87447,#87448,
#87449,#87450)),.UNSPECIFIED.,.F.,.F.,.F.,(4,4),(4,4),(-0.00286833998602934,
0.477902879810758),(0.0665898698862525,0.0731716198748499),
 .UNSPECIFIED.);
#2650=B_SPLINE_SURFACE_WITH_KNOTS('',3,3,((#87484,#87485,#87486,#87487),
(#87488,#87489,#87490,#87491),(#87492,#87493,#87494,#87495),(#87496,#87497,
#87498,#87499)),.UNSPECIFIED.,.F.,.F.,.F.,(4,4),(4,4),(0.522097120200412,
1.00286791825534),(0.0600156865486936,0.0665898700060149),.UNSPECIFIED.);
#2651=B_SPLINE_SURFACE_WITH_KNOTS('',3,3,((#87509,#87510,#87511,#87512),
(#87513,#87514,#87515,#87516),(#87517,#87518,#87519,#87520),(#87521,#87522,
#87523,#87524)),.UNSPECIFIED.,.F.,.F.,.F.,(4,4),(4,4),(-0.00286764392033235,
0.477902879806884),(0.0565997133101206,0.0631721430887058),
 .UNSPECIFIED.);
#2652=B_SPLINE_SURFACE_WITH_KNOTS('',3,3,((#87561,#87562,#87563,#87564),
(#87565,#87566,#87567,#87568),(#87569,#87570,#87571,#87572),(#87573,#87574,
#87575,#87576)),.UNSPECIFIED.,.F.,.F.,.F.,(4,4),(4,4),(0.522097120200083,
1.00286780122198),(0.0500263550858671,0.0565997133101428),.UNSPECIFIED.);
#2653=B_SPLINE_SURFACE_WITH_KNOTS('',3,3,((#87648,#87649,#87650,#87651),
(#87652,#87653,#87654,#87655),(#87656,#87657,#87658,#87659),(#87660,#87661,
#87662,#87663)),.UNSPECIFIED.,.F.,.F.,.F.,(4,4),(4,4),(0.522097120199211,
1.00286848452593),(0.0400218729465695,0.0466073985929449),.UNSPECIFIED.);
#2654=B_SPLINE_SURFACE_WITH_KNOTS('',3,3,((#87732,#87733,#87734,#87735),
(#87736,#87737,#87738,#87739),(#87740,#87741,#87742,#87743),(#87744,#87745,
#87746,#87747)),.UNSPECIFIED.,.F.,.F.,.F.,(4,4),(4,4),(0.522097120198449,
1.00286862201144),(0.0300094532292165,0.0365944846647043),.UNSPECIFIED.);
#2655=B_SPLINE_SURFACE_WITH_KNOTS('',3,3,((#87780,#87781,#87782,#87783),
(#87784,#87785,#87786,#87787),(#87788,#87789,#87790,#87791),(#87792,#87793,
#87794,#87795)),.UNSPECIFIED.,.F.,.F.,.F.,(4,4),(4,4),(-0.00600003961843867,
1.00000000246921),(0.0166015299238294,0.0265907346180654),.UNSPECIFIED.);
#2656=B_SPLINE_SURFACE_WITH_KNOTS('',3,3,((#87807,#87808,#87809,#87810),
(#87811,#87812,#87813,#87814),(#87815,#87816,#87817,#87818),(#87819,#87820,
#87821,#87822)),.UNSPECIFIED.,.F.,.F.,.F.,(4,4),(4,4),(0.522097120198335,
1.00286780410464),(0.020017522964651,0.0265907346180648),.UNSPECIFIED.);
#2657=B_SPLINE_SURFACE_WITH_KNOTS('',3,3,((#87878,#87879,#87880,#87881),
(#87882,#87883,#87884,#87885),(#87886,#87887,#87888,#87889),(#87890,#87891,
#87892,#87893)),.UNSPECIFIED.,.F.,.F.,.F.,(4,4),(4,4),(0.522097120198003,
1.00286791014296),(0.0100271466749305,0.0166015302184264),.UNSPECIFIED.);
#2658=B_SPLINE_SURFACE_WITH_KNOTS('',3,3,((#87928,#87929,#87930,#87931),
(#87932,#87933,#87934,#87935),(#87936,#87937,#87938,#87939),(#87940,#87941,
#87942,#87943)),.UNSPECIFIED.,.F.,.F.,.F.,(4,4),(4,4),(-0.000171895430464311,
1.00600020634802),(0.0665898698856059,0.075132548107472),.UNSPECIFIED.);
#2659=B_SPLINE_SURFACE_WITH_KNOTS('',3,3,((#87959,#87960,#87961,#87962),
(#87963,#87964,#87965,#87966),(#87967,#87968,#87969,#87970),(#87971,#87972,
#87973,#87974)),.UNSPECIFIED.,.F.,.F.,.F.,(4,4),(4,4),(-0.00286833998604501,
0.477902879811737),(0.0665898698862518,0.0731716198748509),
 .UNSPECIFIED.);
#2660=B_SPLINE_SURFACE_WITH_KNOTS('',3,3,((#87999,#88000,#88001,#88002),
(#88003,#88004,#88005,#88006),(#88007,#88008,#88009,#88010),(#88011,#88012,
#88013,#88014)),.UNSPECIFIED.,.F.,.F.,.F.,(4,4),(4,4),(0.522097120201955,
1.00286791825535),(0.060015686548694,0.0665898700060146),.UNSPECIFIED.);
#2661=B_SPLINE_SURFACE_WITH_KNOTS('',3,3,((#88024,#88025,#88026,#88027),
(#88028,#88029,#88030,#88031),(#88032,#88033,#88034,#88035),(#88036,#88037,
#88038,#88039)),.UNSPECIFIED.,.F.,.F.,.F.,(4,4),(4,4),(-0.00286764392031658,
0.477902879807482),(0.0565997133101202,0.0631721430887052),
 .UNSPECIFIED.);
#2662=B_SPLINE_SURFACE_WITH_KNOTS('',3,3,((#88076,#88077,#88078,#88079),
(#88080,#88081,#88082,#88083),(#88084,#88085,#88086,#88087),(#88088,#88089,
#88090,#88091)),.UNSPECIFIED.,.F.,.F.,.F.,(4,4),(4,4),(0.522097120201401,
1.00286780122214),(0.050026355085846,0.0565997133136308),.UNSPECIFIED.);
#2663=B_SPLINE_SURFACE_WITH_KNOTS('',3,3,((#88163,#88164,#88165,#88166),
(#88167,#88168,#88169,#88170),(#88171,#88172,#88173,#88174),(#88175,#88176,
#88177,#88178)),.UNSPECIFIED.,.F.,.F.,.F.,(4,4),(4,4),(0.522097120200645,
1.0028684845258),(0.0400218729465706,0.046607398592945),.UNSPECIFIED.);
#2664=B_SPLINE_SURFACE_WITH_KNOTS('',3,3,((#88247,#88248,#88249,#88250),
(#88251,#88252,#88253,#88254),(#88255,#88256,#88257,#88258),(#88259,#88260,
#88261,#88262)),.UNSPECIFIED.,.F.,.F.,.F.,(4,4),(4,4),(0.52209712019984,
1.00286862201161),(0.030009453229216,0.0365944846647042),.UNSPECIFIED.);
#2665=B_SPLINE_SURFACE_WITH_KNOTS('',3,3,((#88295,#88296,#88297,#88298),
(#88299,#88300,#88301,#88302),(#88303,#88304,#88305,#88306),(#88307,#88308,
#88309,#88310)),.UNSPECIFIED.,.F.,.F.,.F.,(4,4),(4,4),(-0.00600003964349658,
1.00000000663616),(0.0166015299238282,0.0265907346180646),.UNSPECIFIED.);
#2666=B_SPLINE_SURFACE_WITH_KNOTS('',3,3,((#88322,#88323,#88324,#88325),
(#88326,#88327,#88328,#88329),(#88330,#88331,#88332,#88333),(#88334,#88335,
#88336,#88337)),.UNSPECIFIED.,.F.,.F.,.F.,(4,4),(4,4),(0.522097120199433,
1.00286780410456),(0.0200175229646522,0.0265907346180651),.UNSPECIFIED.);
#2667=B_SPLINE_SURFACE_WITH_KNOTS('',3,3,((#88393,#88394,#88395,#88396),
(#88397,#88398,#88399,#88400),(#88401,#88402,#88403,#88404),(#88405,#88406,
#88407,#88408)),.UNSPECIFIED.,.F.,.F.,.F.,(4,4),(4,4),(0.522097120198737,
1.00286791014283),(0.0100271466749313,0.0166015302184274),.UNSPECIFIED.);
#2668=B_SPLINE_SURFACE_WITH_KNOTS('',3,3,((#88452,#88453,#88454,#88455),
(#88456,#88457,#88458,#88459),(#88460,#88461,#88462,#88463),(#88464,#88465,
#88466,#88467)),.UNSPECIFIED.,.F.,.F.,.F.,(4,4),(4,4),(-0.00017189543000408,
1.00600020634828),(0.0665898698856059,0.0751325481078998),.UNSPECIFIED.);
#2669=B_SPLINE_SURFACE_WITH_KNOTS('',3,3,((#88483,#88484,#88485,#88486),
(#88487,#88488,#88489,#88490),(#88491,#88492,#88493,#88494),(#88495,#88496,
#88497,#88498)),.UNSPECIFIED.,.F.,.F.,.F.,(4,4),(4,4),(-0.00286833998600284,
0.47790287981238),(0.0665898698862513,0.0731716198748498),.UNSPECIFIED.);
#2670=B_SPLINE_SURFACE_WITH_KNOTS('',3,3,((#88526,#88527,#88528,#88529),
(#88530,#88531,#88532,#88533),(#88534,#88535,#88536,#88537),(#88538,#88539,
#88540,#88541)),.UNSPECIFIED.,.F.,.F.,.F.,(4,4),(4,4),(0.522097120203743,
1.00286791825528),(0.0600156865486936,0.0665898700060145),.UNSPECIFIED.);
#2671=B_SPLINE_SURFACE_WITH_KNOTS('',3,3,((#88551,#88552,#88553,#88554),
(#88555,#88556,#88557,#88558),(#88559,#88560,#88561,#88562),(#88563,#88564,
#88565,#88566)),.UNSPECIFIED.,.F.,.F.,.F.,(4,4),(4,4),(-0.00286764392046435,
0.477902879807759),(0.0565997133101208,0.0631721430887072),
 .UNSPECIFIED.);
#2672=B_SPLINE_SURFACE_WITH_KNOTS('',3,3,((#88591,#88592,#88593,#88594),
(#88595,#88596,#88597,#88598),(#88599,#88600,#88601,#88602),(#88603,#88604,
#88605,#88606)),.UNSPECIFIED.,.F.,.F.,.F.,(4,4),(4,4),(0.522097120203084,
1.00286780122204),(0.0500263550858665,0.0565997133101422),.UNSPECIFIED.);
#2673=B_SPLINE_SURFACE_WITH_KNOTS('',3,3,((#88614,#88615,#88616,#88617),
(#88618,#88619,#88620,#88621),(#88622,#88623,#88624,#88625),(#88626,#88627,
#88628,#88629)),.UNSPECIFIED.,.F.,.F.,.F.,(4,4),(4,4),(-0.00286810177351089,
0.477902879811734),(0.046607398592912,0.0531834933545505),.UNSPECIFIED.);
#2674=B_SPLINE_SURFACE_WITH_KNOTS('',3,3,((#88685,#88686,#88687,#88688),
(#88689,#88690,#88691,#88692),(#88693,#88694,#88695,#88696),(#88697,#88698,
#88699,#88700)),.UNSPECIFIED.,.F.,.F.,.F.,(4,4),(4,4),(0.522097120202046,
1.00286848452576),(0.0400218729465706,0.046607398592945),.UNSPECIFIED.);
#2675=B_SPLINE_SURFACE_WITH_KNOTS('',3,3,((#88769,#88770,#88771,#88772),
(#88773,#88774,#88775,#88776),(#88777,#88778,#88779,#88780),(#88781,#88782,
#88783,#88784)),.UNSPECIFIED.,.F.,.F.,.F.,(4,4),(4,4),(0.522097120201246,
1.0028686220115),(0.0300094532292166,0.0365944846647037),.UNSPECIFIED.);
#2676=B_SPLINE_SURFACE_WITH_KNOTS('',3,3,((#88817,#88818,#88819,#88820),
(#88821,#88822,#88823,#88824),(#88825,#88826,#88827,#88828),(#88829,#88830,
#88831,#88832)),.UNSPECIFIED.,.F.,.F.,.F.,(4,4),(4,4),(-0.00600003961857937,
1.00000000246931),(0.0166015299238284,0.0265907346180637),.UNSPECIFIED.);
#2677=B_SPLINE_SURFACE_WITH_KNOTS('',3,3,((#88844,#88845,#88846,#88847),
(#88848,#88849,#88850,#88851),(#88852,#88853,#88854,#88855),(#88856,#88857,
#88858,#88859)),.UNSPECIFIED.,.F.,.F.,.F.,(4,4),(4,4),(0.522097120200689,
1.00286780410456),(0.0200175229646513,0.0265907346180651),.UNSPECIFIED.);
#2678=B_SPLINE_SURFACE_WITH_KNOTS('',3,3,((#88915,#88916,#88917,#88918),
(#88919,#88920,#88921,#88922),(#88923,#88924,#88925,#88926),(#88927,#88928,
#88929,#88930)),.UNSPECIFIED.,.F.,.F.,.F.,(4,4),(4,4),(0.522097120199946,
1.00286791014292),(0.0100271466749312,0.0166015302184281),.UNSPECIFIED.);
#2679=B_SPLINE_SURFACE_WITH_KNOTS('',3,3,((#89000,#89001,#89002,#89003),
(#89004,#89005,#89006,#89007),(#89008,#89009,#89010,#89011),(#89012,#89013,
#89014,#89015)),.UNSPECIFIED.,.F.,.F.,.F.,(4,4),(4,4),(0.522097120206275,
1.00286791825534),(0.0600156865486935,0.0665898700060147),.UNSPECIFIED.);
#2680=B_SPLINE_SURFACE_WITH_KNOTS('',3,3,((#89025,#89026,#89027,#89028),
(#89029,#89030,#89031,#89032),(#89033,#89034,#89035,#89036),(#89037,#89038,
#89039,#89040)),.UNSPECIFIED.,.F.,.F.,.F.,(4,4),(4,4),(-0.00286764392045874,
0.477902879808112),(0.0565997133101205,0.0631721430887073),
 .UNSPECIFIED.);
#2681=B_SPLINE_SURFACE_WITH_KNOTS('',3,3,((#89071,#89072,#89073,#89074),
(#89075,#89076,#89077,#89078),(#89079,#89080,#89081,#89082),(#89083,#89084,
#89085,#89086)),.UNSPECIFIED.,.F.,.F.,.F.,(4,4),(4,4),(0.522097120204885,
1.00286780122186),(0.0500263550858663,0.0565997133101424),.UNSPECIFIED.);
#2682=B_SPLINE_SURFACE_WITH_KNOTS('',3,3,((#89110,#89111,#89112,#89113),
(#89114,#89115,#89116,#89117),(#89118,#89119,#89120,#89121),(#89122,#89123,
#89124,#89125)),.UNSPECIFIED.,.F.,.F.,.F.,(4,4),(4,4),(-0.00600014643596561,
1.),(0.036594484664054,0.0466073985929448),.UNSPECIFIED.);
#2683=B_SPLINE_SURFACE_WITH_KNOTS('',3,3,((#89148,#89149,#89150,#89151),
(#89152,#89153,#89154,#89155),(#89156,#89157,#89158,#89159),(#89160,#89161,
#89162,#89163)),.UNSPECIFIED.,.F.,.F.,.F.,(4,4),(4,4),(0.522097120203888,
1.00286848452563),(0.0400218729465705,0.046607398592945),.UNSPECIFIED.);
#2684=B_SPLINE_SURFACE_WITH_KNOTS('',3,3,((#89220,#89221,#89222,#89223),
(#89224,#89225,#89226,#89227),(#89228,#89229,#89230,#89231),(#89232,#89233,
#89234,#89235)),.UNSPECIFIED.,.F.,.F.,.F.,(4,4),(4,4),(-0.00286833998611542,
0.477902879815673),(0.0665898698862504,0.0731716198748485),
 .UNSPECIFIED.);
#2685=B_SPLINE_SURFACE_WITH_KNOTS('',3,3,((#89274,#89275,#89276,#89277),
(#89278,#89279,#89280,#89281),(#89282,#89283,#89284,#89285),(#89286,#89287,
#89288,#89289)),.UNSPECIFIED.,.F.,.F.,.F.,(4,4),(4,4),(0.52209712020296,
1.00286862201167),(0.0300094532292166,0.0365944846647042),.UNSPECIFIED.);
#2686=B_SPLINE_SURFACE_WITH_KNOTS('',3,3,((#89322,#89323,#89324,#89325),
(#89326,#89327,#89328,#89329),(#89330,#89331,#89332,#89333),(#89334,#89335,
#89336,#89337)),.UNSPECIFIED.,.F.,.F.,.F.,(4,4),(4,4),(-0.00600003964364205,
1.00000000663609),(0.0166015299238285,0.0265907346180648),.UNSPECIFIED.);
#2687=B_SPLINE_SURFACE_WITH_KNOTS('',3,3,((#89349,#89350,#89351,#89352),
(#89353,#89354,#89355,#89356),(#89357,#89358,#89359,#89360),(#89361,#89362,
#89363,#89364)),.UNSPECIFIED.,.F.,.F.,.F.,(4,4),(4,4),(0.522097120202179,
1.00286780410463),(0.020017522964651,0.026590734618065),.UNSPECIFIED.);
#2688=B_SPLINE_SURFACE_WITH_KNOTS('',3,3,((#89420,#89421,#89422,#89423),
(#89424,#89425,#89426,#89427),(#89428,#89429,#89430,#89431),(#89432,#89433,
#89434,#89435)),.UNSPECIFIED.,.F.,.F.,.F.,(4,4),(4,4),(0.522097120201302,
1.00286791014286),(0.0100271466749303,0.0166015302184269),.UNSPECIFIED.);
#2689=B_SPLINE_SURFACE_WITH_KNOTS('',3,3,((#89524,#89525,#89526,#89527),
(#89528,#89529,#89530,#89531),(#89532,#89533,#89534,#89535),(#89536,#89537,
#89538,#89539)),.UNSPECIFIED.,.F.,.F.,.F.,(4,4),(4,4),(0.52209712020732,
1.00286780122193),(0.050026355085867,0.0565997133101424),.UNSPECIFIED.);
#2690=B_SPLINE_SURFACE_WITH_KNOTS('',3,3,((#89547,#89548,#89549,#89550),
(#89551,#89552,#89553,#89554),(#89555,#89556,#89557,#89558),(#89559,#89560,
#89561,#89562)),.UNSPECIFIED.,.F.,.F.,.F.,(4,4),(4,4),(-0.00286810177367121,
0.477902879812735),(0.046607398592912,0.0531834933545511),.UNSPECIFIED.);
#2691=B_SPLINE_SURFACE_WITH_KNOTS('',3,3,((#89614,#89615,#89616,#89617),
(#89618,#89619,#89620,#89621),(#89622,#89623,#89624,#89625),(#89626,#89627,
#89628,#89629)),.UNSPECIFIED.,.F.,.F.,.F.,(4,4),(4,4),(0.522097120205853,
1.00286848452572),(0.0400218729465696,0.0466073985929448),.UNSPECIFIED.);
#2692=B_SPLINE_SURFACE_WITH_KNOTS('',3,3,((#89676,#89677,#89678,#89679),
(#89680,#89681,#89682,#89683),(#89684,#89685,#89686,#89687),(#89688,#89689,
#89690,#89691)),.UNSPECIFIED.,.F.,.F.,.F.,(4,4),(4,4),(0.52209712020468,
1.0028686220115),(0.0300094532292157,0.0365944846647038),.UNSPECIFIED.);
#2693=B_SPLINE_SURFACE_WITH_KNOTS('',3,3,((#89699,#89700,#89701,#89702),
(#89703,#89704,#89705,#89706),(#89707,#89708,#89709,#89710),(#89711,#89712,
#89713,#89714)),.UNSPECIFIED.,.F.,.F.,.F.,(4,4),(4,4),(-0.00286823356233573,
0.477902879812311),(0.0265907346180621,0.0331702037252922),
 .UNSPECIFIED.);
#2694=B_SPLINE_SURFACE_WITH_KNOTS('',3,3,((#89749,#89750,#89751,#89752),
(#89753,#89754,#89755,#89756),(#89757,#89758,#89759,#89760),(#89761,#89762,
#89763,#89764)),.UNSPECIFIED.,.F.,.F.,.F.,(4,4),(4,4),(-0.00286833998610001,
0.477902879812836),(0.0665898698862507,0.0731716198748494),
 .UNSPECIFIED.);
#2695=B_SPLINE_SURFACE_WITH_KNOTS('',3,3,((#89795,#89796,#89797,#89798),
(#89799,#89800,#89801,#89802),(#89803,#89804,#89805,#89806),(#89807,#89808,
#89809,#89810)),.UNSPECIFIED.,.F.,.F.,.F.,(4,4),(4,4),(0.522097120205365,
1.00286791825533),(0.0600156865486915,0.0665898700060128),.UNSPECIFIED.);
#2696=B_SPLINE_SURFACE_WITH_KNOTS('',3,3,((#89820,#89821,#89822,#89823),
(#89824,#89825,#89826,#89827),(#89828,#89829,#89830,#89831),(#89832,#89833,
#89834,#89835)),.UNSPECIFIED.,.F.,.F.,.F.,(4,4),(4,4),(-0.00286764392040503,
0.477902879811564),(0.0565997133101196,0.0631721430887057),
 .UNSPECIFIED.);
#2697=B_SPLINE_SURFACE_WITH_KNOTS('',3,3,((#89849,#89850,#89851,#89852),
(#89853,#89854,#89855,#89856),(#89857,#89858,#89859,#89860),(#89861,#89862,
#89863,#89864)),.UNSPECIFIED.,.F.,.F.,.F.,(4,4),(4,4),(-0.00600003962528381,
1.00000000356522),(0.0166015299238274,0.0265907346180631),.UNSPECIFIED.);
#2698=B_SPLINE_SURFACE_WITH_KNOTS('',3,3,((#89876,#89877,#89878,#89879),
(#89880,#89881,#89882,#89883),(#89884,#89885,#89886,#89887),(#89888,#89889,
#89890,#89891)),.UNSPECIFIED.,.F.,.F.,.F.,(4,4),(4,4),(0.522097120203962,
1.00286780410476),(0.0200175229646509,0.0265907346180654),.UNSPECIFIED.);
#2699=B_SPLINE_SURFACE_WITH_KNOTS('',3,3,((#89947,#89948,#89949,#89950),
(#89951,#89952,#89953,#89954),(#89955,#89956,#89957,#89958),(#89959,#89960,
#89961,#89962)),.UNSPECIFIED.,.F.,.F.,.F.,(4,4),(4,4),(0.52209712020327,
1.00286791014279),(0.0100271466749304,0.0166015302184271),.UNSPECIFIED.);
#2700=B_SPLINE_SURFACE_WITH_KNOTS('',3,3,((#90043,#90044,#90045,#90046),
(#90047,#90048,#90049,#90050),(#90051,#90052,#90053,#90054),(#90055,#90056,
#90057,#90058)),.UNSPECIFIED.,.F.,.F.,.F.,(4,4),(4,4),(-0.0060001464360308,
1.),(0.0365944846640544,0.0466073985929448),.UNSPECIFIED.);
#2701=B_SPLINE_SURFACE_WITH_KNOTS('',3,3,((#90081,#90082,#90083,#90084),
(#90085,#90086,#90087,#90088),(#90089,#90090,#90091,#90092),(#90093,#90094,
#90095,#90096)),.UNSPECIFIED.,.F.,.F.,.F.,(4,4),(4,4),(0.522097120208598,
1.00286848452568),(0.0400218729465714,0.0466073985929447),.UNSPECIFIED.);
#2702=B_SPLINE_SURFACE_WITH_KNOTS('',3,3,((#90144,#90145,#90146,#90147),
(#90148,#90149,#90150,#90151),(#90152,#90153,#90154,#90155),(#90156,#90157,
#90158,#90159)),.UNSPECIFIED.,.F.,.F.,.F.,(4,4),(4,4),(0.522097120206756,
1.00286862201145),(0.0300094532292163,0.0365944846647035),.UNSPECIFIED.);
#2703=B_SPLINE_SURFACE_WITH_KNOTS('',3,3,((#90183,#90184,#90185,#90186),
(#90187,#90188,#90189,#90190),(#90191,#90192,#90193,#90194),(#90195,#90196,
#90197,#90198)),.UNSPECIFIED.,.F.,.F.,.F.,(4,4),(4,4),(-0.00600003960396672,
1.),(0.0166015299238285,0.0265907346180638),.UNSPECIFIED.);
#2704=B_SPLINE_SURFACE_WITH_KNOTS('',3,3,((#90210,#90211,#90212,#90213),
(#90214,#90215,#90216,#90217),(#90218,#90219,#90220,#90221),(#90222,#90223,
#90224,#90225)),.UNSPECIFIED.,.F.,.F.,.F.,(4,4),(4,4),(0.522097120206069,
1.0028678041047),(0.0200175229646512,0.026590734618065),.UNSPECIFIED.);
#2705=B_SPLINE_SURFACE_WITH_KNOTS('',3,3,((#90233,#90234,#90235,#90236),
(#90237,#90238,#90239,#90240),(#90241,#90242,#90243,#90244),(#90245,#90246,
#90247,#90248)),.UNSPECIFIED.,.F.,.F.,.F.,(4,4),(4,4),(-0.00286753114062764,
0.477902879812649),(0.0166015299238962,0.0231736788090045),
 .UNSPECIFIED.);
#2706=B_SPLINE_SURFACE_WITH_KNOTS('',3,3,((#90259,#90260,#90261,#90262),
(#90263,#90264,#90265,#90266),(#90267,#90268,#90269,#90270),(#90271,#90272,
#90273,#90274)),.UNSPECIFIED.,.F.,.F.,.F.,(4,4),(4,4),(-0.000171895434491828,
1.00600020634819),(0.0665898698856031,0.0751325481108773),.UNSPECIFIED.);
#2707=B_SPLINE_SURFACE_WITH_KNOTS('',3,3,((#90329,#90330,#90331,#90332),
(#90333,#90334,#90335,#90336),(#90337,#90338,#90339,#90340),(#90341,#90342,
#90343,#90344)),.UNSPECIFIED.,.F.,.F.,.F.,(4,4),(4,4),(0.522097120206893,
1.00286791825543),(0.060015686548693,0.0665898700060125),.UNSPECIFIED.);
#2708=B_SPLINE_SURFACE_WITH_KNOTS('',3,3,((#90354,#90355,#90356,#90357),
(#90358,#90359,#90360,#90361),(#90362,#90363,#90364,#90365),(#90366,#90367,
#90368,#90369)),.UNSPECIFIED.,.F.,.F.,.F.,(4,4),(4,4),(-0.00286764392048026,
0.477902879808188),(0.056599713310119,0.0631721430887063),.UNSPECIFIED.);
#2709=B_SPLINE_SURFACE_WITH_KNOTS('',3,3,((#90400,#90401,#90402,#90403),
(#90404,#90405,#90406,#90407),(#90408,#90409,#90410,#90411),(#90412,#90413,
#90414,#90415)),.UNSPECIFIED.,.F.,.F.,.F.,(4,4),(4,4),(0.522097120206727,
1.00286780122188),(0.0500263550858663,0.0565997133101412),.UNSPECIFIED.);
#2710=B_SPLINE_SURFACE_WITH_KNOTS('',3,3,((#90468,#90469,#90470,#90471),
(#90472,#90473,#90474,#90475),(#90476,#90477,#90478,#90479),(#90480,#90481,
#90482,#90483)),.UNSPECIFIED.,.F.,.F.,.F.,(4,4),(4,4),(0.522097120204994,
1.0028679101427),(0.0100271466749314,0.0166015302184274),.UNSPECIFIED.);
#2711=B_SPLINE_SURFACE_WITH_KNOTS('',3,3,((#90589,#90590,#90591,#90592),
(#90593,#90594,#90595,#90596),(#90597,#90598,#90599,#90600),(#90601,#90602,
#90603,#90604)),.UNSPECIFIED.,.F.,.F.,.F.,(4,4),(4,4),(0.522097120209516,
1.00286862201142),(0.0300094532292164,0.0365944846647041),.UNSPECIFIED.);
#2712=B_SPLINE_SURFACE_WITH_KNOTS('',3,3,((#90612,#90613,#90614,#90615),
(#90616,#90617,#90618,#90619),(#90620,#90621,#90622,#90623),(#90624,#90625,
#90626,#90627)),.UNSPECIFIED.,.F.,.F.,.F.,(4,4),(4,4),(-0.00286823045920498,
0.477902879812828),(0.026590734618062,0.0331702036774536),.UNSPECIFIED.);
#2713=B_SPLINE_SURFACE_WITH_KNOTS('',3,3,((#90657,#90658,#90659,#90660),
(#90661,#90662,#90663,#90664),(#90665,#90666,#90667,#90668),(#90669,#90670,
#90671,#90672)),.UNSPECIFIED.,.F.,.F.,.F.,(4,4),(4,4),(0.522097120208285,
1.00286780410462),(0.0200175229646509,0.0265907346180644),.UNSPECIFIED.);
#2714=B_SPLINE_SURFACE_WITH_KNOTS('',3,3,((#90716,#90717,#90718,#90719),
(#90720,#90721,#90722,#90723),(#90724,#90725,#90726,#90727),(#90728,#90729,
#90730,#90731)),.UNSPECIFIED.,.F.,.F.,.F.,(4,4),(4,4),(0.522097120207253,
1.00286791014264),(0.0100271466749324,0.0166015302184276),.UNSPECIFIED.);
#2715=B_SPLINE_SURFACE_WITH_KNOTS('',3,3,((#90739,#90740,#90741,#90742),
(#90743,#90744,#90745,#90746),(#90747,#90748,#90749,#90750),(#90751,#90752,
#90753,#90754)),.UNSPECIFIED.,.F.,.F.,.F.,(4,4),(4,4),(-0.00206901892678166,
0.34676972851382),(0.00660713154702252,0.0131849431468904),
 .UNSPECIFIED.);
#2716=B_SPLINE_SURFACE_WITH_KNOTS('',3,3,((#90815,#90816,#90817,#90818),
(#90819,#90820,#90821,#90822),(#90823,#90824,#90825,#90826),(#90827,#90828,
#90829,#90830)),.UNSPECIFIED.,.F.,.F.,.F.,(4,4),(4,4),(0.522097120206813,
1.00286791825532),(0.0600156865486929,0.0665898700060134),.UNSPECIFIED.);
#2717=B_SPLINE_SURFACE_WITH_KNOTS('',3,3,((#90878,#90879,#90880,#90881),
(#90882,#90883,#90884,#90885),(#90886,#90887,#90888,#90889),(#90890,#90891,
#90892,#90893)),.UNSPECIFIED.,.F.,.F.,.F.,(4,4),(4,4),(0.522097120207726,
1.00286780122191),(0.0500263550858662,0.0565997133101415),.UNSPECIFIED.);
#2718=B_SPLINE_SURFACE_WITH_KNOTS('',3,3,((#90960,#90961,#90962,#90963),
(#90964,#90965,#90966,#90967),(#90968,#90969,#90970,#90971),(#90972,#90973,
#90974,#90975)),.UNSPECIFIED.,.F.,.F.,.F.,(4,4),(4,4),(0.522097120207574,
1.00286848452577),(0.0400218729465695,0.0466073985929437),.UNSPECIFIED.);
#2719=B_SPLINE_SURFACE_WITH_KNOTS('',3,3,((#91024,#91025,#91026,#91027),
(#91028,#91029,#91030,#91031),(#91032,#91033,#91034,#91035),(#91036,#91037,
#91038,#91039)),.UNSPECIFIED.,.F.,.F.,.F.,(4,4),(4,4),(0.522097120198755,
1.00286823669301),(0.0265907346180633,0.0331702036622765),.UNSPECIFIED.);
#2720=B_SPLINE_SURFACE_WITH_KNOTS('',3,3,((#91041,#91042,#91043,#91044),
(#91045,#91046,#91047,#91048),(#91049,#91050,#91051,#91052),(#91053,#91054,
#91055,#91056)),.UNSPECIFIED.,.F.,.F.,.F.,(4,4),(4,4),(-0.00286862201165793,
0.477902879801984),(0.0300094532292788,0.0365944846647005),
 .UNSPECIFIED.);
#2721=B_SPLINE_SURFACE_WITH_KNOTS('',3,3,((#91064,#91065,#91066,#91067),
(#91068,#91069,#91070,#91071),(#91072,#91073,#91074,#91075),(#91076,#91077,
#91078,#91079)),.UNSPECIFIED.,.F.,.F.,.F.,(4,4),(4,4),(-0.00286848453285561,
0.47790287980318),(0.0400218729466597,0.0466073985929426),.UNSPECIFIED.);
#2722=B_SPLINE_SURFACE_WITH_KNOTS('',3,3,((#91096,#91097,#91098,#91099),
(#91100,#91101,#91102,#91103),(#91104,#91105,#91106,#91107),(#91108,#91109,
#91110,#91111)),.UNSPECIFIED.,.F.,.F.,.F.,(4,4),(4,4),(0.,1.00600014639747),
(0.0365944846644987,0.046607398592915),.UNSPECIFIED.);
#2723=B_SPLINE_SURFACE_WITH_KNOTS('',3,3,((#91112,#91113,#91114,#91115),
(#91116,#91117,#91118,#91119),(#91120,#91121,#91122,#91123),(#91124,#91125,
#91126,#91127)),.UNSPECIFIED.,.F.,.F.,.F.,(4,4),(4,4),(-0.00286780122415295,
0.477902879802985),(0.0500263550858989,0.0565997133101389),
 .UNSPECIFIED.);
#2724=B_SPLINE_SURFACE_WITH_KNOTS('',3,3,((#91129,#91130,#91131,#91132),
(#91133,#91134,#91135,#91136),(#91137,#91138,#91139,#91140),(#91141,#91142,
#91143,#91144)),.UNSPECIFIED.,.F.,.F.,.F.,(4,4),(4,4),(0.522097120201262,
1.00286810177284),(0.0466073985929439,0.0531834933545494),.UNSPECIFIED.);
#2725=B_SPLINE_SURFACE_WITH_KNOTS('',3,3,((#91152,#91153,#91154,#91155),
(#91156,#91157,#91158,#91159),(#91160,#91161,#91162,#91163),(#91164,#91165,
#91166,#91167)),.UNSPECIFIED.,.F.,.F.,.F.,(4,4),(4,4),(-0.00286792598902313,
0.477902879802582),(0.0600156865494597,0.0665898698871158),
 .UNSPECIFIED.);
#2726=B_SPLINE_SURFACE_WITH_KNOTS('',3,3,((#91169,#91170,#91171,#91172),
(#91173,#91174,#91175,#91176),(#91177,#91178,#91179,#91180),(#91181,#91182,
#91183,#91184)),.UNSPECIFIED.,.F.,.F.,.F.,(4,4),(4,4),(0.522097120202546,
1.00286764392041),(0.0565997133101403,0.0631721430887051),.UNSPECIFIED.);
#2727=B_SPLINE_SURFACE_WITH_KNOTS('',3,3,((#91192,#91193,#91194,#91195),
(#91196,#91197,#91198,#91199),(#91200,#91201,#91202,#91203),(#91204,#91205,
#91206,#91207)),.UNSPECIFIED.,.F.,.F.,.F.,(4,4),(4,4),(0.522097120203716,
1.00286833998597),(0.0665898698871153,0.0731716198748442),.UNSPECIFIED.);
#2728=B_SPLINE_SURFACE_WITH_KNOTS('',3,3,((#91209,#91210,#91211,#91212),
(#91213,#91214,#91215,#91216),(#91217,#91218,#91219,#91220),(#91221,#91222,
#91223,#91224)),.UNSPECIFIED.,.F.,.F.,.F.,(4,4),(4,4),(-0.0012473153074531,
0.209045111704136),(0.0700194292965939,0.0749900982978269),
 .UNSPECIFIED.);
#2729=B_SPLINE_SURFACE_WITH_KNOTS('',3,3,((#91238,#91239,#91240,#91241),
(#91242,#91243,#91244,#91245),(#91246,#91247,#91248,#91249),(#91250,#91251,
#91252,#91253)),.UNSPECIFIED.,.F.,.F.,.F.,(4,4),(4,4),(-0.00286791014417758,
0.477902879802125),(0.0100271466769369,0.0166015299239865),
 .UNSPECIFIED.);
#2730=B_SPLINE_SURFACE_WITH_KNOTS('',3,3,((#91255,#91256,#91257,#91258),
(#91259,#91260,#91261,#91262),(#91263,#91264,#91265,#91266),(#91267,#91268,
#91269,#91270)),.UNSPECIFIED.,.F.,.F.,.F.,(4,4),(4,4),(0.653230271487925,
1.00206901891114),(0.00656788395392195,0.0131849432429873),
 .UNSPECIFIED.);
#2731=B_SPLINE_SURFACE_WITH_KNOTS('',3,3,((#91278,#91279,#91280,#91281),
(#91282,#91283,#91284,#91285),(#91286,#91287,#91288,#91289),(#91290,#91291,
#91292,#91293)),.UNSPECIFIED.,.F.,.F.,.F.,(4,4),(4,4),(0.,1.00600003961375),
(0.0166015299239895,0.0265907346180635),.UNSPECIFIED.);
#2732=B_SPLINE_SURFACE_WITH_KNOTS('',3,3,((#91296,#91297,#91298,#91299),
(#91300,#91301,#91302,#91303),(#91304,#91305,#91306,#91307),(#91308,#91309,
#91310,#91311)),.UNSPECIFIED.,.F.,.F.,.F.,(4,4),(4,4),(0.522097120198875,
1.0028675316012),(0.0166015299239866,0.0231736788037103),.UNSPECIFIED.);
#2733=B_SPLINE_SURFACE_WITH_KNOTS('',3,3,((#91312,#91313,#91314,#91315),
(#91316,#91317,#91318,#91319),(#91320,#91321,#91322,#91323),(#91324,#91325,
#91326,#91327)),.UNSPECIFIED.,.F.,.F.,.F.,(4,4),(4,4),(-0.00286780410483755,
0.47790287980203),(0.0200175229646903,0.0265907346180618),.UNSPECIFIED.);
#2734=B_SPLINE_SURFACE_WITH_KNOTS('',3,3,((#91334,#91335,#91336,#91337),
(#91338,#91339,#91340,#91341),(#91342,#91343,#91344,#91345),(#91346,#91347,
#91348,#91349)),.UNSPECIFIED.,.F.,.F.,.F.,(4,4),(4,4),(-0.00286791014425298,
0.477902879801941),(0.0100271466769356,0.0166015299239881),
 .UNSPECIFIED.);
#2735=B_SPLINE_SURFACE_WITH_KNOTS('',3,3,((#91351,#91352,#91353,#91354),
(#91355,#91356,#91357,#91358),(#91359,#91360,#91361,#91362),(#91363,#91364,
#91365,#91366)),.UNSPECIFIED.,.F.,.F.,.F.,(4,4),(4,4),(0.653230271487142,
1.002069018909),(0.00656788395391975,0.0131849432429877),.UNSPECIFIED.);
#2736=B_SPLINE_SURFACE_WITH_KNOTS('',3,3,((#91389,#91390,#91391,#91392),
(#91393,#91394,#91395,#91396),(#91397,#91398,#91399,#91400),(#91401,#91402,
#91403,#91404)),.UNSPECIFIED.,.F.,.F.,.F.,(4,4),(4,4),(-0.00286848453293753,
0.477902879803458),(0.0400218729466608,0.0466073985929422),
 .UNSPECIFIED.);
#2737=B_SPLINE_SURFACE_WITH_KNOTS('',3,3,((#91406,#91407,#91408,#91409),
(#91410,#91411,#91412,#91413),(#91414,#91415,#91416,#91417),(#91418,#91419,
#91420,#91421)),.UNSPECIFIED.,.F.,.F.,.F.,(4,4),(4,4),(0.,1.00600014639741),
(0.0365944846644992,0.0466073985929148),.UNSPECIFIED.);
#2738=B_SPLINE_SURFACE_WITH_KNOTS('',3,3,((#91422,#91423,#91424,#91425),
(#91426,#91427,#91428,#91429),(#91430,#91431,#91432,#91433),(#91434,#91435,
#91436,#91437)),.UNSPECIFIED.,.F.,.F.,.F.,(4,4),(4,4),(-0.00286780122418116,
0.477902879803416),(0.050026355085899,0.056599713310139),.UNSPECIFIED.);
#2739=B_SPLINE_SURFACE_WITH_KNOTS('',3,3,((#91439,#91440,#91441,#91442),
(#91443,#91444,#91445,#91446),(#91447,#91448,#91449,#91450),(#91451,#91452,
#91453,#91454)),.UNSPECIFIED.,.F.,.F.,.F.,(4,4),(4,4),(0.52209712019881,
1.00286810177268),(0.0466073985929444,0.053183492588891),.UNSPECIFIED.);
#2740=B_SPLINE_SURFACE_WITH_KNOTS('',3,3,((#91462,#91463,#91464,#91465),
(#91466,#91467,#91468,#91469),(#91470,#91471,#91472,#91473),(#91474,#91475,
#91476,#91477)),.UNSPECIFIED.,.F.,.F.,.F.,(4,4),(4,4),(-0.00286792598894552,
0.477902879803265),(0.0600156865494594,0.0665898698871161),
 .UNSPECIFIED.);
#2741=B_SPLINE_SURFACE_WITH_KNOTS('',3,3,((#91479,#91480,#91481,#91482),
(#91483,#91484,#91485,#91486),(#91487,#91488,#91489,#91490),(#91491,#91492,
#91493,#91494)),.UNSPECIFIED.,.F.,.F.,.F.,(4,4),(4,4),(0.522097120200067,
1.00286764392044),(0.0565997133101416,0.0631721430887055),.UNSPECIFIED.);
#2742=B_SPLINE_SURFACE_WITH_KNOTS('',3,3,((#91502,#91503,#91504,#91505),
(#91506,#91507,#91508,#91509),(#91510,#91511,#91512,#91513),(#91514,#91515,
#91516,#91517)),.UNSPECIFIED.,.F.,.F.,.F.,(4,4),(4,4),(0.522097120201106,
1.00286833998596),(0.0665898698871184,0.0731716198748444),.UNSPECIFIED.);
#2743=B_SPLINE_SURFACE_WITH_KNOTS('',3,3,((#91519,#91520,#91521,#91522),
(#91523,#91524,#91525,#91526),(#91527,#91528,#91529,#91530),(#91531,#91532,
#91533,#91534)),.UNSPECIFIED.,.F.,.F.,.F.,(4,4),(4,4),(-0.00124731530673201,
0.209045111704814),(0.0700194292966092,0.0749900982978298),
 .UNSPECIFIED.);
#2744=B_SPLINE_SURFACE_WITH_KNOTS('',3,3,((#91542,#91543,#91544,#91545),
(#91546,#91547,#91548,#91549),(#91550,#91551,#91552,#91553),(#91554,#91555,
#91556,#91557)),.UNSPECIFIED.,.F.,.F.,.F.,(4,4),(4,4),(-0.00286780410483184,
0.477902879802143),(0.0200175229646905,0.0265907346180623),
 .UNSPECIFIED.);
#2745=B_SPLINE_SURFACE_WITH_KNOTS('',3,3,((#91559,#91560,#91561,#91562),
(#91563,#91564,#91565,#91566),(#91567,#91568,#91569,#91570),(#91571,#91572,
#91573,#91574)),.UNSPECIFIED.,.F.,.F.,.F.,(4,4),(4,4),(0.5220971201967,
1.00286753160129),(0.0166015299239878,0.0231736788037118),.UNSPECIFIED.);
#2746=B_SPLINE_SURFACE_WITH_KNOTS('',3,3,((#91576,#91577,#91578,#91579),
(#91580,#91581,#91582,#91583),(#91584,#91585,#91586,#91587),(#91588,#91589,
#91590,#91591)),.UNSPECIFIED.,.F.,.F.,.F.,(4,4),(4,4),(0.,1.00600003961372),
(0.0166015299239882,0.0265907346180641),.UNSPECIFIED.);
#2747=B_SPLINE_SURFACE_WITH_KNOTS('',3,3,((#91600,#91601,#91602,#91603),
(#91604,#91605,#91606,#91607),(#91608,#91609,#91610,#91611),(#91612,#91613,
#91614,#91615)),.UNSPECIFIED.,.F.,.F.,.F.,(4,4),(4,4),(0.522097120197952,
1.00286823669295),(0.0265907346180637,0.0331702036051741),.UNSPECIFIED.);
#2748=B_SPLINE_SURFACE_WITH_KNOTS('',3,3,((#91616,#91617,#91618,#91619),
(#91620,#91621,#91622,#91623),(#91624,#91625,#91626,#91627),(#91628,#91629,
#91630,#91631)),.UNSPECIFIED.,.F.,.F.,.F.,(4,4),(4,4),(-0.00286862201161512,
0.477902879802719),(0.0300094532292791,0.0365944846647173),
 .UNSPECIFIED.);
#2749=B_SPLINE_SURFACE_WITH_KNOTS('',3,3,((#91638,#91639,#91640,#91641),
(#91642,#91643,#91644,#91645),(#91646,#91647,#91648,#91649),(#91650,#91651,
#91652,#91653)),.UNSPECIFIED.,.F.,.F.,.F.,(4,4),(4,4),(-0.00286791014429398,
0.477902879801375),(0.0100271466769348,0.0166015299239883),
 .UNSPECIFIED.);
#2750=B_SPLINE_SURFACE_WITH_KNOTS('',3,3,((#91655,#91656,#91657,#91658),
(#91659,#91660,#91661,#91662),(#91663,#91664,#91665,#91666),(#91667,#91668,
#91669,#91670)),.UNSPECIFIED.,.F.,.F.,.F.,(4,4),(4,4),(0.653230271486491,
1.00206901890709),(0.00656788395391518,0.013184943242987),.UNSPECIFIED.);
#2751=B_SPLINE_SURFACE_WITH_KNOTS('',3,3,((#91678,#91679,#91680,#91681),
(#91682,#91683,#91684,#91685),(#91686,#91687,#91688,#91689),(#91690,#91691,
#91692,#91693)),.UNSPECIFIED.,.F.,.F.,.F.,(4,4),(4,4),(-0.00286780410483956,
0.477902879801899),(0.0200175229646901,0.0265907346180625),
 .UNSPECIFIED.);
#2752=B_SPLINE_SURFACE_WITH_KNOTS('',3,3,((#91695,#91696,#91697,#91698),
(#91699,#91700,#91701,#91702),(#91703,#91704,#91705,#91706),(#91707,#91708,
#91709,#91710)),.UNSPECIFIED.,.F.,.F.,.F.,(4,4),(4,4),(0.52209712019461,
1.00286753160142),(0.0166015299239879,0.0231736788037111),.UNSPECIFIED.);
#2753=B_SPLINE_SURFACE_WITH_KNOTS('',3,3,((#91712,#91713,#91714,#91715),
(#91716,#91717,#91718,#91719),(#91720,#91721,#91722,#91723),(#91724,#91725,
#91726,#91727)),.UNSPECIFIED.,.F.,.F.,.F.,(4,4),(4,4),(0.,1.00600003961387),
(0.0166015299239869,0.0265907346180636),.UNSPECIFIED.);
#2754=B_SPLINE_SURFACE_WITH_KNOTS('',3,3,((#91728,#91729,#91730,#91731),
(#91732,#91733,#91734,#91735),(#91736,#91737,#91738,#91739),(#91740,#91741,
#91742,#91743)),.UNSPECIFIED.,.F.,.F.,.F.,(4,4),(4,4),(0.522097120196459,
1.00286810177292),(0.0466073985929452,0.0531834925888918),.UNSPECIFIED.);
#2755=B_SPLINE_SURFACE_WITH_KNOTS('',3,3,((#91745,#91746,#91747,#91748),
(#91749,#91750,#91751,#91752),(#91753,#91754,#91755,#91756),(#91757,#91758,
#91759,#91760)),.UNSPECIFIED.,.F.,.F.,.F.,(4,4),(4,4),(-0.00286780122426028,
0.477902879803546),(0.0500263550859001,0.056599713310138),.UNSPECIFIED.);
#2756=B_SPLINE_SURFACE_WITH_KNOTS('',3,3,((#91768,#91769,#91770,#91771),
(#91772,#91773,#91774,#91775),(#91776,#91777,#91778,#91779),(#91780,#91781,
#91782,#91783)),.UNSPECIFIED.,.F.,.F.,.F.,(4,4),(4,4),(-0.00286792598905476,
0.477902879803487),(0.0600156865494573,0.0665898698871151),
 .UNSPECIFIED.);
#2757=B_SPLINE_SURFACE_WITH_KNOTS('',3,3,((#91785,#91786,#91787,#91788),
(#91789,#91790,#91791,#91792),(#91793,#91794,#91795,#91796),(#91797,#91798,
#91799,#91800)),.UNSPECIFIED.,.F.,.F.,.F.,(4,4),(4,4),(0.522097120197693,
1.00286764392045),(0.0565997133101411,0.063172143088705),.UNSPECIFIED.);
#2758=B_SPLINE_SURFACE_WITH_KNOTS('',3,3,((#91808,#91809,#91810,#91811),
(#91812,#91813,#91814,#91815),(#91816,#91817,#91818,#91819),(#91820,#91821,
#91822,#91823)),.UNSPECIFIED.,.F.,.F.,.F.,(4,4),(4,4),(0.522097120198564,
1.002868339986),(0.0665898698871173,0.0731716198748439),.UNSPECIFIED.);
#2759=B_SPLINE_SURFACE_WITH_KNOTS('',3,3,((#91825,#91826,#91827,#91828),
(#91829,#91830,#91831,#91832),(#91833,#91834,#91835,#91836),(#91837,#91838,
#91839,#91840)),.UNSPECIFIED.,.F.,.F.,.F.,(4,4),(4,4),(-0.00124731530626188,
0.209045111705136),(0.0700194292966233,0.0749900982978318),
 .UNSPECIFIED.);
#2760=B_SPLINE_SURFACE_WITH_KNOTS('',3,3,((#91848,#91849,#91850,#91851),
(#91852,#91853,#91854,#91855),(#91856,#91857,#91858,#91859),(#91860,#91861,
#91862,#91863)),.UNSPECIFIED.,.F.,.F.,.F.,(4,4),(4,4),(-0.00286862201161757,
0.4779028798025),(0.0300094532292784,0.0365944846647023),.UNSPECIFIED.);
#2761=B_SPLINE_SURFACE_WITH_KNOTS('',3,3,((#91865,#91866,#91867,#91868),
(#91869,#91870,#91871,#91872),(#91873,#91874,#91875,#91876),(#91877,#91878,
#91879,#91880)),.UNSPECIFIED.,.F.,.F.,.F.,(4,4),(4,4),(0.522097120195729,
1.00286823669305),(0.0265907346180635,0.0331702036889927),.UNSPECIFIED.);
#2762=B_SPLINE_SURFACE_WITH_KNOTS('',3,3,((#91888,#91889,#91890,#91891),
(#91892,#91893,#91894,#91895),(#91896,#91897,#91898,#91899),(#91900,#91901,
#91902,#91903)),.UNSPECIFIED.,.F.,.F.,.F.,(4,4),(4,4),(0.,1.00600014639748),
(0.0365944846644978,0.0466073985929161),.UNSPECIFIED.);
#2763=B_SPLINE_SURFACE_WITH_KNOTS('',3,3,((#91920,#91921,#91922,#91923),
(#91924,#91925,#91926,#91927),(#91928,#91929,#91930,#91931),(#91932,#91933,
#91934,#91935)),.UNSPECIFIED.,.F.,.F.,.F.,(4,4),(4,4),(-0.00286848453299392,
0.47790287980232),(0.0400218729466594,0.046607398592943),.UNSPECIFIED.);
#2764=B_SPLINE_SURFACE_WITH_KNOTS('',3,3,((#91942,#91943,#91944,#91945),
(#91946,#91947,#91948,#91949),(#91950,#91951,#91952,#91953),(#91954,#91955,
#91956,#91957)),.UNSPECIFIED.,.F.,.F.,.F.,(4,4),(4,4),(-0.00286791014432967,
0.477902879800558),(0.0100271466769341,0.0166015299239865),
 .UNSPECIFIED.);
#2765=B_SPLINE_SURFACE_WITH_KNOTS('',3,3,((#91959,#91960,#91961,#91962),
(#91963,#91964,#91965,#91966),(#91967,#91968,#91969,#91970),(#91971,#91972,
#91973,#91974)),.UNSPECIFIED.,.F.,.F.,.F.,(4,4),(4,4),(0.65323027148601,
1.00206901890512),(0.00656788395390979,0.0131849432429878),
 .UNSPECIFIED.);
#2766=B_SPLINE_SURFACE_WITH_KNOTS('',3,3,((#91982,#91983,#91984,#91985),
(#91986,#91987,#91988,#91989),(#91990,#91991,#91992,#91993),(#91994,#91995,
#91996,#91997)),.UNSPECIFIED.,.F.,.F.,.F.,(4,4),(4,4),(-0.00286780410483655,
0.477902879801139),(0.0200175229646906,0.0265907346180617),
 .UNSPECIFIED.);
#2767=B_SPLINE_SURFACE_WITH_KNOTS('',3,3,((#91999,#92000,#92001,#92002),
(#92003,#92004,#92005,#92006),(#92007,#92008,#92009,#92010),(#92011,#92012,
#92013,#92014)),.UNSPECIFIED.,.F.,.F.,.F.,(4,4),(4,4),(0.522097120192733,
1.00286753160138),(0.016601529923988,0.0231736788037116),.UNSPECIFIED.);
#2768=B_SPLINE_SURFACE_WITH_KNOTS('',3,3,((#92016,#92017,#92018,#92019),
(#92020,#92021,#92022,#92023),(#92024,#92025,#92026,#92027),(#92028,#92029,
#92030,#92031)),.UNSPECIFIED.,.F.,.F.,.F.,(4,4),(4,4),(0.,1.00600003961361),
(0.0166015299239868,0.0265907346180624),.UNSPECIFIED.);
#2769=B_SPLINE_SURFACE_WITH_KNOTS('',3,3,((#92032,#92033,#92034,#92035),
(#92036,#92037,#92038,#92039),(#92040,#92041,#92042,#92043),(#92044,#92045,
#92046,#92047)),.UNSPECIFIED.,.F.,.F.,.F.,(4,4),(4,4),(-0.00286862201160953,
0.477902879801959),(0.0300094532292791,0.0365944846647172),
 .UNSPECIFIED.);
#2770=B_SPLINE_SURFACE_WITH_KNOTS('',3,3,((#92049,#92050,#92051,#92052),
(#92053,#92054,#92055,#92056),(#92057,#92058,#92059,#92060),(#92061,#92062,
#92063,#92064)),.UNSPECIFIED.,.F.,.F.,.F.,(4,4),(4,4),(0.522097120193524,
1.00286823669304),(0.026590734618063,0.0331702036889923),.UNSPECIFIED.);
#2771=B_SPLINE_SURFACE_WITH_KNOTS('',3,3,((#92072,#92073,#92074,#92075),
(#92076,#92077,#92078,#92079),(#92080,#92081,#92082,#92083),(#92084,#92085,
#92086,#92087)),.UNSPECIFIED.,.F.,.F.,.F.,(4,4),(4,4),(0.522097120195503,
1.00286764392042),(0.0565997133101417,0.0631721430887048),.UNSPECIFIED.);
#2772=B_SPLINE_SURFACE_WITH_KNOTS('',3,3,((#92089,#92090,#92091,#92092),
(#92093,#92094,#92095,#92096),(#92097,#92098,#92099,#92100),(#92101,#92102,
#92103,#92104)),.UNSPECIFIED.,.F.,.F.,.F.,(4,4),(4,4),(-0.00286792598905419,
0.477902879803423),(0.0600156865494597,0.0665898698871165),
 .UNSPECIFIED.);
#2773=B_SPLINE_SURFACE_WITH_KNOTS('',3,3,((#92112,#92113,#92114,#92115),
(#92116,#92117,#92118,#92119),(#92120,#92121,#92122,#92123),(#92124,#92125,
#92126,#92127)),.UNSPECIFIED.,.F.,.F.,.F.,(4,4),(4,4),(0.522097120196121,
1.00286833998585),(0.0665898698871173,0.073171619874844),.UNSPECIFIED.);
#2774=B_SPLINE_SURFACE_WITH_KNOTS('',3,3,((#92129,#92130,#92131,#92132),
(#92133,#92134,#92135,#92136),(#92137,#92138,#92139,#92140),(#92141,#92142,
#92143,#92144)),.UNSPECIFIED.,.F.,.F.,.F.,(4,4),(4,4),(-0.00124731530620073,
0.209045111705207),(0.0700194292966371,0.0749900982978334),
 .UNSPECIFIED.);
#2775=B_SPLINE_SURFACE_WITH_KNOTS('',3,3,((#92152,#92153,#92154,#92155),
(#92156,#92157,#92158,#92159),(#92160,#92161,#92162,#92163),(#92164,#92165,
#92166,#92167)),.UNSPECIFIED.,.F.,.F.,.F.,(4,4),(4,4),(-0.00286848453302246,
0.477902879801834),(0.0400218729466601,0.046607398592943),.UNSPECIFIED.);
#2776=B_SPLINE_SURFACE_WITH_KNOTS('',3,3,((#92184,#92185,#92186,#92187),
(#92188,#92189,#92190,#92191),(#92192,#92193,#92194,#92195),(#92196,#92197,
#92198,#92199)),.UNSPECIFIED.,.F.,.F.,.F.,(4,4),(4,4),(0.,1.00600014639736),
(0.0365944846644989,0.0466073985929157),.UNSPECIFIED.);
#2777=B_SPLINE_SURFACE_WITH_KNOTS('',3,3,((#92208,#92209,#92210,#92211),
(#92212,#92213,#92214,#92215),(#92216,#92217,#92218,#92219),(#92220,#92221,
#92222,#92223)),.UNSPECIFIED.,.F.,.F.,.F.,(4,4),(4,4),(0.522097120195486,
1.00286810177294),(0.0466073985929438,0.0531834933545495),.UNSPECIFIED.);
#2778=B_SPLINE_SURFACE_WITH_KNOTS('',3,3,((#92224,#92225,#92226,#92227),
(#92228,#92229,#92230,#92231),(#92232,#92233,#92234,#92235),(#92236,#92237,
#92238,#92239)),.UNSPECIFIED.,.F.,.F.,.F.,(4,4),(4,4),(-0.00286780122428723,
0.477902879802085),(0.0500263550858992,0.0565997133101407),
 .UNSPECIFIED.);
#2779=B_SPLINE_SURFACE_WITH_KNOTS('',3,3,((#92246,#92247,#92248,#92249),
(#92250,#92251,#92252,#92253),(#92254,#92255,#92256,#92257),(#92258,#92259,
#92260,#92261)),.UNSPECIFIED.,.F.,.F.,.F.,(4,4),(4,4),(-0.00286791014439694,
0.477902879799415),(0.0100271466769345,0.0166015299239855),
 .UNSPECIFIED.);
#2780=B_SPLINE_SURFACE_WITH_KNOTS('',3,3,((#92263,#92264,#92265,#92266),
(#92267,#92268,#92269,#92270),(#92271,#92272,#92273,#92274),(#92275,#92276,
#92277,#92278)),.UNSPECIFIED.,.F.,.F.,.F.,(4,4),(4,4),(0.653230271485745,
1.00206901890371),(0.00656788395390478,0.0131849432429869),
 .UNSPECIFIED.);
#2781=B_SPLINE_SURFACE_WITH_KNOTS('',3,3,((#92286,#92287,#92288,#92289),
(#92290,#92291,#92292,#92293),(#92294,#92295,#92296,#92297),(#92298,#92299,
#92300,#92301)),.UNSPECIFIED.,.F.,.F.,.F.,(4,4),(4,4),(-0.00286780410478452,
0.477902879800153),(0.0200175229646906,0.0265907346180619),
 .UNSPECIFIED.);
#2782=B_SPLINE_SURFACE_WITH_KNOTS('',3,3,((#92303,#92304,#92305,#92306),
(#92307,#92308,#92309,#92310),(#92311,#92312,#92313,#92314),(#92315,#92316,
#92317,#92318)),.UNSPECIFIED.,.F.,.F.,.F.,(4,4),(4,4),(0.522097120191154,
1.00286753160141),(0.016601529923988,0.0231736787930311),.UNSPECIFIED.);
#2783=B_SPLINE_SURFACE_WITH_KNOTS('',3,3,((#92320,#92321,#92322,#92323),
(#92324,#92325,#92326,#92327),(#92328,#92329,#92330,#92331),(#92332,#92333,
#92334,#92335)),.UNSPECIFIED.,.F.,.F.,.F.,(4,4),(4,4),(0.,1.00600003961398),
(0.0166015299239882,0.0265907346180622),.UNSPECIFIED.);
#2784=B_SPLINE_SURFACE_WITH_KNOTS('',3,3,((#92336,#92337,#92338,#92339),
(#92340,#92341,#92342,#92343),(#92344,#92345,#92346,#92347),(#92348,#92349,
#92350,#92351)),.UNSPECIFIED.,.F.,.F.,.F.,(4,4),(4,4),(-0.00286862201161503,
0.477902879801108),(0.0300094532292788,0.0365944846647166),
 .UNSPECIFIED.);
#2785=B_SPLINE_SURFACE_WITH_KNOTS('',3,3,((#92353,#92354,#92355,#92356),
(#92357,#92358,#92359,#92360),(#92361,#92362,#92363,#92364),(#92365,#92366,
#92367,#92368)),.UNSPECIFIED.,.F.,.F.,.F.,(4,4),(4,4),(0.522097120191805,
1.00286823669312),(0.0265907346180641,0.0331702036889924),.UNSPECIFIED.);
#2786=B_SPLINE_SURFACE_WITH_KNOTS('',3,3,((#92376,#92377,#92378,#92379),
(#92380,#92381,#92382,#92383),(#92384,#92385,#92386,#92387),(#92388,#92389,
#92390,#92391)),.UNSPECIFIED.,.F.,.F.,.F.,(4,4),(4,4),(-0.0028684845330722,
0.477902879801392),(0.0400218729466607,0.0466073985929435),
 .UNSPECIFIED.);
#2787=B_SPLINE_SURFACE_WITH_KNOTS('',3,3,((#92408,#92409,#92410,#92411),
(#92412,#92413,#92414,#92415),(#92416,#92417,#92418,#92419),(#92420,#92421,
#92422,#92423)),.UNSPECIFIED.,.F.,.F.,.F.,(4,4),(4,4),(0.,1.00600014639735),
(0.0365944846644988,0.0466073985929162),.UNSPECIFIED.);
#2788=B_SPLINE_SURFACE_WITH_KNOTS('',3,3,((#92424,#92425,#92426,#92427),
(#92428,#92429,#92430,#92431),(#92432,#92433,#92434,#92435),(#92436,#92437,
#92438,#92439)),.UNSPECIFIED.,.F.,.F.,.F.,(4,4),(4,4),(0.52209712019443,
1.00286833998601),(0.0665898698871202,0.073171619874844),.UNSPECIFIED.);
#2789=B_SPLINE_SURFACE_WITH_KNOTS('',3,3,((#92448,#92449,#92450,#92451),
(#92452,#92453,#92454,#92455),(#92456,#92457,#92458,#92459),(#92460,#92461,
#92462,#92463)),.UNSPECIFIED.,.F.,.F.,.F.,(4,4),(4,4),(-0.00124731530661292,
0.209045111704791),(0.0700194292966529,0.0749900982978302),
 .UNSPECIFIED.);
#2790=B_SPLINE_SURFACE_WITH_KNOTS('',3,3,((#92464,#92465,#92466,#92467),
(#92468,#92469,#92470,#92471),(#92472,#92473,#92474,#92475),(#92476,#92477,
#92478,#92479)),.UNSPECIFIED.,.F.,.F.,.F.,(4,4),(4,4),(-0.00286780122435983,
0.477902879801441),(0.0500263550858991,0.05659971331014),.UNSPECIFIED.);
#2791=B_SPLINE_SURFACE_WITH_KNOTS('',3,3,((#92481,#92482,#92483,#92484),
(#92485,#92486,#92487,#92488),(#92489,#92490,#92491,#92492),(#92493,#92494,
#92495,#92496)),.UNSPECIFIED.,.F.,.F.,.F.,(4,4),(4,4),(0.522097120193469,
1.00286810177265),(0.0466073985929449,0.0531834925888935),.UNSPECIFIED.);
#2792=B_SPLINE_SURFACE_WITH_KNOTS('',3,3,((#92512,#92513,#92514,#92515),
(#92516,#92517,#92518,#92519),(#92520,#92521,#92522,#92523),(#92524,#92525,
#92526,#92527)),.UNSPECIFIED.,.F.,.F.,.F.,(4,4),(4,4),(0.522097120195661,
1.00286764392054),(0.0565997133101417,0.0631721430887064),.UNSPECIFIED.);
#2793=B_SPLINE_SURFACE_WITH_KNOTS('',3,3,((#92528,#92529,#92530,#92531),
(#92532,#92533,#92534,#92535),(#92536,#92537,#92538,#92539),(#92540,#92541,
#92542,#92543)),.UNSPECIFIED.,.F.,.F.,.F.,(4,4),(4,4),(-0.00286792598902705,
0.477902879801742),(0.06001568654946,0.0665898698871169),.UNSPECIFIED.);
#2794=B_SPLINE_SURFACE_WITH_KNOTS('',3,3,((#92550,#92551,#92552,#92553),
(#92554,#92555,#92556,#92557),(#92558,#92559,#92560,#92561),(#92562,#92563,
#92564,#92565)),.UNSPECIFIED.,.F.,.F.,.F.,(4,4),(4,4),(-0.00286791014444834,
0.477902879798085),(0.0100271466769347,0.0166015299239865),
 .UNSPECIFIED.);
#2795=B_SPLINE_SURFACE_WITH_KNOTS('',3,3,((#92567,#92568,#92569,#92570),
(#92571,#92572,#92573,#92574),(#92575,#92576,#92577,#92578),(#92579,#92580,
#92581,#92582)),.UNSPECIFIED.,.F.,.F.,.F.,(4,4),(4,4),(0.653230271485697,
1.00206901890237),(0.00656788395389881,0.0131849432429867),
 .UNSPECIFIED.);
#2796=B_SPLINE_SURFACE_WITH_KNOTS('',3,3,((#92590,#92591,#92592,#92593),
(#92594,#92595,#92596,#92597),(#92598,#92599,#92600,#92601),(#92602,#92603,
#92604,#92605)),.UNSPECIFIED.,.F.,.F.,.F.,(4,4),(4,4),(-0.002867804104808,
0.477902879798951),(0.020017522964691,0.0265907346180616),.UNSPECIFIED.);
#2797=B_SPLINE_SURFACE_WITH_KNOTS('',3,3,((#92607,#92608,#92609,#92610),
(#92611,#92612,#92613,#92614),(#92615,#92616,#92617,#92618),(#92619,#92620,
#92621,#92622)),.UNSPECIFIED.,.F.,.F.,.F.,(4,4),(4,4),(0.52209712018981,
1.00286753160131),(0.0166015299239889,0.0231736788075213),.UNSPECIFIED.);
#2798=B_SPLINE_SURFACE_WITH_KNOTS('',3,3,((#92624,#92625,#92626,#92627),
(#92628,#92629,#92630,#92631),(#92632,#92633,#92634,#92635),(#92636,#92637,
#92638,#92639)),.UNSPECIFIED.,.F.,.F.,.F.,(4,4),(4,4),(0.,1.00600003961366),
(0.0166015299239869,0.0265907346180631),.UNSPECIFIED.);
#2799=B_SPLINE_SURFACE_WITH_KNOTS('',3,3,((#92640,#92641,#92642,#92643),
(#92644,#92645,#92646,#92647),(#92648,#92649,#92650,#92651),(#92652,#92653,
#92654,#92655)),.UNSPECIFIED.,.F.,.F.,.F.,(4,4),(4,4),(-0.00286862201162927,
0.477902879800058),(0.0300094532292786,0.0365944846647019),
 .UNSPECIFIED.);
#2800=B_SPLINE_SURFACE_WITH_KNOTS('',3,3,((#92657,#92658,#92659,#92660),
(#92661,#92662,#92663,#92664),(#92665,#92666,#92667,#92668),(#92669,#92670,
#92671,#92672)),.UNSPECIFIED.,.F.,.F.,.F.,(4,4),(4,4),(0.522097120190289,
1.00286823669302),(0.026590734618063,0.0331702036889927),.UNSPECIFIED.);
#2801=B_SPLINE_SURFACE_WITH_KNOTS('',3,3,((#92680,#92681,#92682,#92683),
(#92684,#92685,#92686,#92687),(#92688,#92689,#92690,#92691),(#92692,#92693,
#92694,#92695)),.UNSPECIFIED.,.F.,.F.,.F.,(4,4),(4,4),(-0.00286848453311717,
0.477902879800286),(0.0400218729466604,0.0466073985929421),
 .UNSPECIFIED.);
#2802=B_SPLINE_SURFACE_WITH_KNOTS('',3,3,((#92712,#92713,#92714,#92715),
(#92716,#92717,#92718,#92719),(#92720,#92721,#92722,#92723),(#92724,#92725,
#92726,#92727)),.UNSPECIFIED.,.F.,.F.,.F.,(4,4),(4,4),(0.,1.0060001463975),
(0.0365944846644987,0.0466073985929169),.UNSPECIFIED.);
#2803=B_SPLINE_SURFACE_WITH_KNOTS('',3,3,((#92728,#92729,#92730,#92731),
(#92732,#92733,#92734,#92735),(#92736,#92737,#92738,#92739),(#92740,#92741,
#92742,#92743)),.UNSPECIFIED.,.F.,.F.,.F.,(4,4),(4,4),(-0.00286780122439779,
0.477902879800689),(0.0500263550859002,0.0565997133101411),
 .UNSPECIFIED.);
#2804=B_SPLINE_SURFACE_WITH_KNOTS('',3,3,((#92745,#92746,#92747,#92748),
(#92749,#92750,#92751,#92752),(#92753,#92754,#92755,#92756),(#92757,#92758,
#92759,#92760)),.UNSPECIFIED.,.F.,.F.,.F.,(4,4),(4,4),(0.522097120191868,
1.00286810177297),(0.0466073985929451,0.0531834933545502),.UNSPECIFIED.);
#2805=B_SPLINE_SURFACE_WITH_KNOTS('',3,3,((#92768,#92769,#92770,#92771),
(#92772,#92773,#92774,#92775),(#92776,#92777,#92778,#92779),(#92780,#92781,
#92782,#92783)),.UNSPECIFIED.,.F.,.F.,.F.,(4,4),(4,4),(-0.00286792598900614,
0.47790287980102),(0.0600156865494604,0.0665898698871169),.UNSPECIFIED.);
#2806=B_SPLINE_SURFACE_WITH_KNOTS('',3,3,((#92785,#92786,#92787,#92788),
(#92789,#92790,#92791,#92792),(#92793,#92794,#92795,#92796),(#92797,#92798,
#92799,#92800)),.UNSPECIFIED.,.F.,.F.,.F.,(4,4),(4,4),(0.522097120194769,
1.00286764392045),(0.0565997133101423,0.0631721430887064),.UNSPECIFIED.);
#2807=B_SPLINE_SURFACE_WITH_KNOTS('',3,3,((#92816,#92817,#92818,#92819),
(#92820,#92821,#92822,#92823),(#92824,#92825,#92826,#92827),(#92828,#92829,
#92830,#92831)),.UNSPECIFIED.,.F.,.F.,.F.,(4,4),(4,4),(0.522097120193573,
1.00286833998603),(0.066589869887119,0.0731716198748446),.UNSPECIFIED.);
#2808=B_SPLINE_SURFACE_WITH_KNOTS('',3,3,((#92832,#92833,#92834,#92835),
(#92836,#92837,#92838,#92839),(#92840,#92841,#92842,#92843),(#92844,#92845,
#92846,#92847)),.UNSPECIFIED.,.F.,.F.,.F.,(4,4),(4,4),(-0.00124731530708468,
0.209045111704209),(0.070019429296666,0.0749900982978293),.UNSPECIFIED.);
#2809=B_SPLINE_SURFACE_WITH_KNOTS('',3,3,((#92854,#92855,#92856,#92857),
(#92858,#92859,#92860,#92861),(#92862,#92863,#92864,#92865),(#92866,#92867,
#92868,#92869)),.UNSPECIFIED.,.F.,.F.,.F.,(4,4),(4,4),(-0.00286791014448215,
0.477902879796417),(0.0100271466769337,0.0166015299239869),
 .UNSPECIFIED.);
#2810=B_SPLINE_SURFACE_WITH_KNOTS('',3,3,((#92871,#92872,#92873,#92874),
(#92875,#92876,#92877,#92878),(#92879,#92880,#92881,#92882),(#92883,#92884,
#92885,#92886)),.UNSPECIFIED.,.F.,.F.,.F.,(4,4),(4,4),(0.653230271485805,
1.00206901890132),(0.00656788395389165,0.0131849432429875),
 .UNSPECIFIED.);
#2811=B_SPLINE_SURFACE_WITH_KNOTS('',3,3,((#92894,#92895,#92896,#92897),
(#92898,#92899,#92900,#92901),(#92902,#92903,#92904,#92905),(#92906,#92907,
#92908,#92909)),.UNSPECIFIED.,.F.,.F.,.F.,(4,4),(4,4),(-0.00286780410477404,
0.477902879797415),(0.0200175229646904,0.0265907346180627),
 .UNSPECIFIED.);
#2812=B_SPLINE_SURFACE_WITH_KNOTS('',3,3,((#92911,#92912,#92913,#92914),
(#92915,#92916,#92917,#92918),(#92919,#92920,#92921,#92922),(#92923,#92924,
#92925,#92926)),.UNSPECIFIED.,.F.,.F.,.F.,(4,4),(4,4),(0.522097120188512,
1.00286753160135),(0.0166015299239885,0.0231736787930316),.UNSPECIFIED.);
#2813=B_SPLINE_SURFACE_WITH_KNOTS('',3,3,((#92928,#92929,#92930,#92931),
(#92932,#92933,#92934,#92935),(#92936,#92937,#92938,#92939),(#92940,#92941,
#92942,#92943)),.UNSPECIFIED.,.F.,.F.,.F.,(4,4),(4,4),(0.,1.00600003961351),
(0.0166015299239904,0.0265907346180641),.UNSPECIFIED.);
#2814=B_SPLINE_SURFACE_WITH_KNOTS('',3,3,((#92944,#92945,#92946,#92947),
(#92948,#92949,#92950,#92951),(#92952,#92953,#92954,#92955),(#92956,#92957,
#92958,#92959)),.UNSPECIFIED.,.F.,.F.,.F.,(4,4),(4,4),(-0.00286862201164203,
0.477902879798625),(0.0300094532292783,0.0365944846647018),
 .UNSPECIFIED.);
#2815=B_SPLINE_SURFACE_WITH_KNOTS('',3,3,((#92961,#92962,#92963,#92964),
(#92965,#92966,#92967,#92968),(#92969,#92970,#92971,#92972),(#92973,#92974,
#92975,#92976)),.UNSPECIFIED.,.F.,.F.,.F.,(4,4),(4,4),(0.522097120188926,
1.00286823669299),(0.0265907346180644,0.0331702036889922),.UNSPECIFIED.);
#2816=B_SPLINE_SURFACE_WITH_KNOTS('',3,3,((#92984,#92985,#92986,#92987),
(#92988,#92989,#92990,#92991),(#92992,#92993,#92994,#92995),(#92996,#92997,
#92998,#92999)),.UNSPECIFIED.,.F.,.F.,.F.,(4,4),(4,4),(-0.00286848453316085,
0.477902879799002),(0.0400218729466581,0.0466073985929425),
 .UNSPECIFIED.);
#2817=B_SPLINE_SURFACE_WITH_KNOTS('',3,3,((#93016,#93017,#93018,#93019),
(#93020,#93021,#93022,#93023),(#93024,#93025,#93026,#93027),(#93028,#93029,
#93030,#93031)),.UNSPECIFIED.,.F.,.F.,.F.,(4,4),(4,4),(0.,1.0060001463976),
(0.0365944846644989,0.0466073985929171),.UNSPECIFIED.);
#2818=B_SPLINE_SURFACE_WITH_KNOTS('',3,3,((#93032,#93033,#93034,#93035),
(#93036,#93037,#93038,#93039),(#93040,#93041,#93042,#93043),(#93044,#93045,
#93046,#93047)),.UNSPECIFIED.,.F.,.F.,.F.,(4,4),(4,4),(-0.00286780122443639,
0.477902879799573),(0.0500263550858993,0.0565997133101408),
 .UNSPECIFIED.);
#2819=B_SPLINE_SURFACE_WITH_KNOTS('',3,3,((#93049,#93050,#93051,#93052),
(#93053,#93054,#93055,#93056),(#93057,#93058,#93059,#93060),(#93061,#93062,
#93063,#93064)),.UNSPECIFIED.,.F.,.F.,.F.,(4,4),(4,4),(0.522097120190254,
1.00286810177252),(0.0466073985929451,0.0531834925888939),.UNSPECIFIED.);
#2820=B_SPLINE_SURFACE_WITH_KNOTS('',3,3,((#93072,#93073,#93074,#93075),
(#93076,#93077,#93078,#93079),(#93080,#93081,#93082,#93083),(#93084,#93085,
#93086,#93087)),.UNSPECIFIED.,.F.,.F.,.F.,(4,4),(4,4),(-0.00286792598898738,
0.477902879800105),(0.0600156865494592,0.0665898698871172),
 .UNSPECIFIED.);
#2821=B_SPLINE_SURFACE_WITH_KNOTS('',3,3,((#93089,#93090,#93091,#93092),
(#93093,#93094,#93095,#93096),(#93097,#93098,#93099,#93100),(#93101,#93102,
#93103,#93104)),.UNSPECIFIED.,.F.,.F.,.F.,(4,4),(4,4),(0.522097120193723,
1.00286764392043),(0.0565997133101425,0.0631721430887051),.UNSPECIFIED.);
#2822=B_SPLINE_SURFACE_WITH_KNOTS('',3,3,((#93120,#93121,#93122,#93123),
(#93124,#93125,#93126,#93127),(#93128,#93129,#93130,#93131),(#93132,#93133,
#93134,#93135)),.UNSPECIFIED.,.F.,.F.,.F.,(4,4),(4,4),(0.522097120191563,
1.00286833998597),(0.0665898698871186,0.0731716198748454),.UNSPECIFIED.);
#2823=B_SPLINE_SURFACE_WITH_KNOTS('',3,3,((#93136,#93137,#93138,#93139),
(#93140,#93141,#93142,#93143),(#93144,#93145,#93146,#93147),(#93148,#93149,
#93150,#93151)),.UNSPECIFIED.,.F.,.F.,.F.,(4,4),(4,4),(-0.00124731530803454,
0.209045111703296),(0.0700194292966781,0.0749900982978239),
 .UNSPECIFIED.);
#2824=B_SPLINE_SURFACE_WITH_KNOTS('',3,3,((#93158,#93159,#93160,#93161),
(#93162,#93163,#93164,#93165),(#93166,#93167,#93168,#93169),(#93170,#93171,
#93172,#93173)),.UNSPECIFIED.,.F.,.F.,.F.,(4,4),(4,4),(-0.00286791014452394,
0.477902879794564),(0.0100271466769348,0.0166015299239866),
 .UNSPECIFIED.);
#2825=B_SPLINE_SURFACE_WITH_KNOTS('',3,3,((#93175,#93176,#93177,#93178),
(#93179,#93180,#93181,#93182),(#93183,#93184,#93185,#93186),(#93187,#93188,
#93189,#93190)),.UNSPECIFIED.,.F.,.F.,.F.,(4,4),(4,4),(0.653230271486075,
1.00206901890076),(0.00656788395388381,0.0131849432429868),
 .UNSPECIFIED.);
#2826=B_SPLINE_SURFACE_WITH_KNOTS('',3,3,((#93198,#93199,#93200,#93201),
(#93202,#93203,#93204,#93205),(#93206,#93207,#93208,#93209),(#93210,#93211,
#93212,#93213)),.UNSPECIFIED.,.F.,.F.,.F.,(4,4),(4,4),(-0.002867804104759,
0.477902879795688),(0.0200175229646897,0.0265907346180626),
 .UNSPECIFIED.);
#2827=B_SPLINE_SURFACE_WITH_KNOTS('',3,3,((#93215,#93216,#93217,#93218),
(#93219,#93220,#93221,#93222),(#93223,#93224,#93225,#93226),(#93227,#93228,
#93229,#93230)),.UNSPECIFIED.,.F.,.F.,.F.,(4,4),(4,4),(0.522097120187777,
1.00286753160138),(0.0166015299239877,0.0231736788075219),.UNSPECIFIED.);
#2828=B_SPLINE_SURFACE_WITH_KNOTS('',3,3,((#93232,#93233,#93234,#93235),
(#93236,#93237,#93238,#93239),(#93240,#93241,#93242,#93243),(#93244,#93245,
#93246,#93247)),.UNSPECIFIED.,.F.,.F.,.F.,(4,4),(4,4),(0.,1.00600003961393),
(0.0166015299239902,0.0265907346180655),.UNSPECIFIED.);
#2829=B_SPLINE_SURFACE_WITH_KNOTS('',3,3,((#93248,#93249,#93250,#93251),
(#93252,#93253,#93254,#93255),(#93256,#93257,#93258,#93259),(#93260,#93261,
#93262,#93263)),.UNSPECIFIED.,.F.,.F.,.F.,(4,4),(4,4),(-0.0028686220116367,
0.477902879796942),(0.0300094532292783,0.0365944846647026),
 .UNSPECIFIED.);
#2830=B_SPLINE_SURFACE_WITH_KNOTS('',3,3,((#93265,#93266,#93267,#93268),
(#93269,#93270,#93271,#93272),(#93273,#93274,#93275,#93276),(#93277,#93278,
#93279,#93280)),.UNSPECIFIED.,.F.,.F.,.F.,(4,4),(4,4),(0.522097120188087,
1.00286823669321),(0.0265907346180629,0.0331702036889928),.UNSPECIFIED.);
#2831=B_SPLINE_SURFACE_WITH_KNOTS('',3,3,((#93288,#93289,#93290,#93291),
(#93292,#93293,#93294,#93295),(#93296,#93297,#93298,#93299),(#93300,#93301,
#93302,#93303)),.UNSPECIFIED.,.F.,.F.,.F.,(4,4),(4,4),(-0.00286848453322405,
0.477902879797452),(0.0400218729466589,0.0466073985929433),
 .UNSPECIFIED.);
#2832=B_SPLINE_SURFACE_WITH_KNOTS('',3,3,((#93320,#93321,#93322,#93323),
(#93324,#93325,#93326,#93327),(#93328,#93329,#93330,#93331),(#93332,#93333,
#93334,#93335)),.UNSPECIFIED.,.F.,.F.,.F.,(4,4),(4,4),(0.,1.00600014639746),
(0.0365944846644991,0.046607398592917),.UNSPECIFIED.);
#2833=B_SPLINE_SURFACE_WITH_KNOTS('',3,3,((#93336,#93337,#93338,#93339),
(#93340,#93341,#93342,#93343),(#93344,#93345,#93346,#93347),(#93348,#93349,
#93350,#93351)),.UNSPECIFIED.,.F.,.F.,.F.,(4,4),(4,4),(-0.00286780122450092,
0.477902879798157),(0.0500263550858995,0.0565997133101396),
 .UNSPECIFIED.);
#2834=B_SPLINE_SURFACE_WITH_KNOTS('',3,3,((#93353,#93354,#93355,#93356),
(#93357,#93358,#93359,#93360),(#93361,#93362,#93363,#93364),(#93365,#93366,
#93367,#93368)),.UNSPECIFIED.,.F.,.F.,.F.,(4,4),(4,4),(0.522097120189125,
1.00286810177271),(0.0466073985929443,0.0531834925888927),.UNSPECIFIED.);
#2835=B_SPLINE_SURFACE_WITH_KNOTS('',3,3,((#93376,#93377,#93378,#93379),
(#93380,#93381,#93382,#93383),(#93384,#93385,#93386,#93387),(#93388,#93389,
#93390,#93391)),.UNSPECIFIED.,.F.,.F.,.F.,(4,4),(4,4),(-0.00286792598902637,
0.477902879798802),(0.0600156865494596,0.0665898698871163),
 .UNSPECIFIED.);
#2836=B_SPLINE_SURFACE_WITH_KNOTS('',3,3,((#93393,#93394,#93395,#93396),
(#93397,#93398,#93399,#93400),(#93401,#93402,#93403,#93404),(#93405,#93406,
#93407,#93408)),.UNSPECIFIED.,.F.,.F.,.F.,(4,4),(4,4),(0.522097120193084,
1.00286764392051),(0.0565997133101423,0.0631721430887053),.UNSPECIFIED.);
#2837=B_SPLINE_SURFACE_WITH_KNOTS('',3,3,((#93424,#93425,#93426,#93427),
(#93428,#93429,#93430,#93431),(#93432,#93433,#93434,#93435),(#93436,#93437,
#93438,#93439)),.UNSPECIFIED.,.F.,.F.,.F.,(4,4),(4,4),(0.52209712019007,
1.00286833998607),(0.0665898698871196,0.0731716198748448),.UNSPECIFIED.);
#2838=B_SPLINE_SURFACE_WITH_KNOTS('',3,3,((#93440,#93441,#93442,#93443),
(#93444,#93445,#93446,#93447),(#93448,#93449,#93450,#93451),(#93452,#93453,
#93454,#93455)),.UNSPECIFIED.,.F.,.F.,.F.,(4,4),(4,4),(-0.00124731530915548,
0.209045111702115),(0.07001942929669,0.0749900982978186),.UNSPECIFIED.);
#2839=B_SPLINE_SURFACE_WITH_KNOTS('',3,3,((#93462,#93463,#93464,#93465),
(#93466,#93467,#93468,#93469),(#93470,#93471,#93472,#93473),(#93474,#93475,
#93476,#93477)),.UNSPECIFIED.,.F.,.F.,.F.,(4,4),(4,4),(-0.00286791014454036,
0.477902879792387),(0.0100271466769345,0.0166015299239863),
 .UNSPECIFIED.);
#2840=B_SPLINE_SURFACE_WITH_KNOTS('',3,3,((#93479,#93480,#93481,#93482),
(#93483,#93484,#93485,#93486),(#93487,#93488,#93489,#93490),(#93491,#93492,
#93493,#93494)),.UNSPECIFIED.,.F.,.F.,.F.,(4,4),(4,4),(0.653230271486586,
1.00206901890025),(0.00656788395387618,0.0131849432429879),
 .UNSPECIFIED.);
#2841=B_SPLINE_SURFACE_WITH_KNOTS('',3,3,((#93502,#93503,#93504,#93505),
(#93506,#93507,#93508,#93509),(#93510,#93511,#93512,#93513),(#93514,#93515,
#93516,#93517)),.UNSPECIFIED.,.F.,.F.,.F.,(4,4),(4,4),(-0.00286780410473863,
0.477902879793642),(0.0200175229646915,0.0265907346180612),
 .UNSPECIFIED.);
#2842=B_SPLINE_SURFACE_WITH_KNOTS('',3,3,((#93519,#93520,#93521,#93522),
(#93523,#93524,#93525,#93526),(#93527,#93528,#93529,#93530),(#93531,#93532,
#93533,#93534)),.UNSPECIFIED.,.F.,.F.,.F.,(4,4),(4,4),(0.522097120187455,
1.00286753160133),(0.0166015299239889,0.0231736787930312),.UNSPECIFIED.);
#2843=B_SPLINE_SURFACE_WITH_KNOTS('',3,3,((#93536,#93537,#93538,#93539),
(#93540,#93541,#93542,#93543),(#93544,#93545,#93546,#93547),(#93548,#93549,
#93550,#93551)),.UNSPECIFIED.,.F.,.F.,.F.,(4,4),(4,4),(0.,1.00600003961403),
(0.0166015299239862,0.0265907346180637),.UNSPECIFIED.);
#2844=B_SPLINE_SURFACE_WITH_KNOTS('',3,3,((#93552,#93553,#93554,#93555),
(#93556,#93557,#93558,#93559),(#93560,#93561,#93562,#93563),(#93564,#93565,
#93566,#93567)),.UNSPECIFIED.,.F.,.F.,.F.,(4,4),(4,4),(-0.00286862201162951,
0.477902879795088),(0.0300094532292795,0.0365944846647016),
 .UNSPECIFIED.);
#2845=B_SPLINE_SURFACE_WITH_KNOTS('',3,3,((#93569,#93570,#93571,#93572),
(#93573,#93574,#93575,#93576),(#93577,#93578,#93579,#93580),(#93581,#93582,
#93583,#93584)),.UNSPECIFIED.,.F.,.F.,.F.,(4,4),(4,4),(0.52209712018746,
1.00286823669317),(0.026590734618063,0.0331702036889934),.UNSPECIFIED.);
#2846=B_SPLINE_SURFACE_WITH_KNOTS('',3,3,((#93592,#93593,#93594,#93595),
(#93596,#93597,#93598,#93599),(#93600,#93601,#93602,#93603),(#93604,#93605,
#93606,#93607)),.UNSPECIFIED.,.F.,.F.,.F.,(4,4),(4,4),(-0.00286848453325639,
0.477902879795614),(0.0400218729466603,0.0466073985929429),
 .UNSPECIFIED.);
#2847=B_SPLINE_SURFACE_WITH_KNOTS('',3,3,((#93624,#93625,#93626,#93627),
(#93628,#93629,#93630,#93631),(#93632,#93633,#93634,#93635),(#93636,#93637,
#93638,#93639)),.UNSPECIFIED.,.F.,.F.,.F.,(4,4),(4,4),(0.,1.00600014639741),
(0.036594484664499,0.0466073985929158),.UNSPECIFIED.);
#2848=B_SPLINE_SURFACE_WITH_KNOTS('',3,3,((#93640,#93641,#93642,#93643),
(#93644,#93645,#93646,#93647),(#93648,#93649,#93650,#93651),(#93652,#93653,
#93654,#93655)),.UNSPECIFIED.,.F.,.F.,.F.,(4,4),(4,4),(-0.00286780122453885,
0.477902879796429),(0.0500263550859007,0.0565997133101406),
 .UNSPECIFIED.);
#2849=B_SPLINE_SURFACE_WITH_KNOTS('',3,3,((#93657,#93658,#93659,#93660),
(#93661,#93662,#93663,#93664),(#93665,#93666,#93667,#93668),(#93669,#93670,
#93671,#93672)),.UNSPECIFIED.,.F.,.F.,.F.,(4,4),(4,4),(0.522097120188107,
1.00286810177272),(0.0466073985929452,0.0531834925888921),.UNSPECIFIED.);
#2850=B_SPLINE_SURFACE_WITH_KNOTS('',3,3,((#93680,#93681,#93682,#93683),
(#93684,#93685,#93686,#93687),(#93688,#93689,#93690,#93691),(#93692,#93693,
#93694,#93695)),.UNSPECIFIED.,.F.,.F.,.F.,(4,4),(4,4),(-0.00286792598897243,
0.477902879797169),(0.0600156865494596,0.0665898698871175),
 .UNSPECIFIED.);
#2851=B_SPLINE_SURFACE_WITH_KNOTS('',3,3,((#93697,#93698,#93699,#93700),
(#93701,#93702,#93703,#93704),(#93705,#93706,#93707,#93708),(#93709,#93710,
#93711,#93712)),.UNSPECIFIED.,.F.,.F.,.F.,(4,4),(4,4),(0.522097120192675,
1.0028676439205),(0.0565997133101423,0.0631721430887056),.UNSPECIFIED.);
#2852=B_SPLINE_SURFACE_WITH_KNOTS('',3,3,((#93728,#93729,#93730,#93731),
(#93732,#93733,#93734,#93735),(#93736,#93737,#93738,#93739),(#93740,#93741,
#93742,#93743)),.UNSPECIFIED.,.F.,.F.,.F.,(4,4),(4,4),(0.522097120188981,
1.00286833998611),(0.0665898698871197,0.0731716198748445),.UNSPECIFIED.);
#2853=B_SPLINE_SURFACE_WITH_KNOTS('',3,3,((#93744,#93745,#93746,#93747),
(#93748,#93749,#93750,#93751),(#93752,#93753,#93754,#93755),(#93756,#93757,
#93758,#93759)),.UNSPECIFIED.,.F.,.F.,.F.,(4,4),(4,4),(-0.00124731531066159,
0.209045111700583),(0.0700194292967009,0.0749900982978111),
 .UNSPECIFIED.);
#2854=B_SPLINE_SURFACE_WITH_KNOTS('',3,3,((#93766,#93767,#93768,#93769),
(#93770,#93771,#93772,#93773),(#93774,#93775,#93776,#93777),(#93778,#93779,
#93780,#93781)),.UNSPECIFIED.,.F.,.F.,.F.,(4,4),(4,4),(-0.00286791014456512,
0.477902879790222),(0.0100271466769336,0.0166015299239865),
 .UNSPECIFIED.);
#2855=B_SPLINE_SURFACE_WITH_KNOTS('',3,3,((#93783,#93784,#93785,#93786),
(#93787,#93788,#93789,#93790),(#93791,#93792,#93793,#93794),(#93795,#93796,
#93797,#93798)),.UNSPECIFIED.,.F.,.F.,.F.,(4,4),(4,4),(0.653230271487221,
1.00206901890035),(0.00656788395386757,0.0131849432429867),
 .UNSPECIFIED.);
#2856=B_SPLINE_SURFACE_WITH_KNOTS('',3,3,((#93806,#93807,#93808,#93809),
(#93810,#93811,#93812,#93813),(#93814,#93815,#93816,#93817),(#93818,#93819,
#93820,#93821)),.UNSPECIFIED.,.F.,.F.,.F.,(4,4),(4,4),(-0.00286780410471625,
0.477902879791447),(0.0200175229646886,0.0265907346180621),
 .UNSPECIFIED.);
#2857=B_SPLINE_SURFACE_WITH_KNOTS('',3,3,((#93823,#93824,#93825,#93826),
(#93827,#93828,#93829,#93830),(#93831,#93832,#93833,#93834),(#93835,#93836,
#93837,#93838)),.UNSPECIFIED.,.F.,.F.,.F.,(4,4),(4,4),(0.522097120186926,
1.00286753160134),(0.0166015299239881,0.0231736788075218),.UNSPECIFIED.);
#2858=B_SPLINE_SURFACE_WITH_KNOTS('',3,3,((#93840,#93841,#93842,#93843),
(#93844,#93845,#93846,#93847),(#93848,#93849,#93850,#93851),(#93852,#93853,
#93854,#93855)),.UNSPECIFIED.,.F.,.F.,.F.,(4,4),(4,4),(0.,1.00600003961439),
(0.0166015299239894,0.0265907346180612),.UNSPECIFIED.);
#2859=B_SPLINE_SURFACE_WITH_KNOTS('',3,3,((#93856,#93857,#93858,#93859),
(#93860,#93861,#93862,#93863),(#93864,#93865,#93866,#93867),(#93868,#93869,
#93870,#93871)),.UNSPECIFIED.,.F.,.F.,.F.,(4,4),(4,4),(-0.00286862201160481,
0.477902879793087),(0.0300094532292791,0.0365944846647159),
 .UNSPECIFIED.);
#2860=B_SPLINE_SURFACE_WITH_KNOTS('',3,3,((#93873,#93874,#93875,#93876),
(#93877,#93878,#93879,#93880),(#93881,#93882,#93883,#93884),(#93885,#93886,
#93887,#93888)),.UNSPECIFIED.,.F.,.F.,.F.,(4,4),(4,4),(0.522097120186975,
1.00286823669319),(0.026590734618063,0.0331702036889921),.UNSPECIFIED.);
#2861=B_SPLINE_SURFACE_WITH_KNOTS('',3,3,((#93896,#93897,#93898,#93899),
(#93900,#93901,#93902,#93903),(#93904,#93905,#93906,#93907),(#93908,#93909,
#93910,#93911)),.UNSPECIFIED.,.F.,.F.,.F.,(4,4),(4,4),(-0.00286848453329562,
0.477902879793674),(0.0400218729466592,0.0466073985929428),
 .UNSPECIFIED.);
#2862=B_SPLINE_SURFACE_WITH_KNOTS('',3,3,((#93928,#93929,#93930,#93931),
(#93932,#93933,#93934,#93935),(#93936,#93937,#93938,#93939),(#93940,#93941,
#93942,#93943)),.UNSPECIFIED.,.F.,.F.,.F.,(4,4),(4,4),(0.,1.00600014639722),
(0.036594484664498,0.0466073985929171),.UNSPECIFIED.);
#2863=B_SPLINE_SURFACE_WITH_KNOTS('',3,3,((#93944,#93945,#93946,#93947),
(#93948,#93949,#93950,#93951),(#93952,#93953,#93954,#93955),(#93956,#93957,
#93958,#93959)),.UNSPECIFIED.,.F.,.F.,.F.,(4,4),(4,4),(-0.00286780122455666,
0.477902879794515),(0.0500263550858996,0.0565997133101404),
 .UNSPECIFIED.);
#2864=B_SPLINE_SURFACE_WITH_KNOTS('',3,3,((#93961,#93962,#93963,#93964),
(#93965,#93966,#93967,#93968),(#93969,#93970,#93971,#93972),(#93973,#93974,
#93975,#93976)),.UNSPECIFIED.,.F.,.F.,.F.,(4,4),(4,4),(0.522097120187377,
1.00286810177268),(0.046607398592944,0.0531834925888931),.UNSPECIFIED.);
#2865=B_SPLINE_SURFACE_WITH_KNOTS('',3,3,((#93984,#93985,#93986,#93987),
(#93988,#93989,#93990,#93991),(#93992,#93993,#93994,#93995),(#93996,#93997,
#93998,#93999)),.UNSPECIFIED.,.F.,.F.,.F.,(4,4),(4,4),(-0.00286792598896508,
0.477902879795425),(0.06001568654946,0.0665898698871157),.UNSPECIFIED.);
#2866=B_SPLINE_SURFACE_WITH_KNOTS('',3,3,((#94001,#94002,#94003,#94004),
(#94005,#94006,#94007,#94008),(#94009,#94010,#94011,#94012),(#94013,#94014,
#94015,#94016)),.UNSPECIFIED.,.F.,.F.,.F.,(4,4),(4,4),(0.522097120192157,
1.00286764392065),(0.056599713310142,0.0631721430887059),.UNSPECIFIED.);
#2867=B_SPLINE_SURFACE_WITH_KNOTS('',3,3,((#94032,#94033,#94034,#94035),
(#94036,#94037,#94038,#94039),(#94040,#94041,#94042,#94043),(#94044,#94045,
#94046,#94047)),.UNSPECIFIED.,.F.,.F.,.F.,(4,4),(4,4),(0.522097120187888,
1.00286833998592),(0.0665898698871188,0.0731716198748451),.UNSPECIFIED.);
#2868=B_SPLINE_SURFACE_WITH_KNOTS('',3,3,((#94048,#94049,#94050,#94051),
(#94052,#94053,#94054,#94055),(#94056,#94057,#94058,#94059),(#94060,#94061,
#94062,#94063)),.UNSPECIFIED.,.F.,.F.,.F.,(4,4),(4,4),(-0.0012473153123853,
0.20904511169894),(0.0700194292967067,0.0749900982978036),.UNSPECIFIED.);
#2869=B_SPLINE_SURFACE_WITH_KNOTS('',3,3,((#94070,#94071,#94072,#94073),
(#94074,#94075,#94076,#94077),(#94078,#94079,#94080,#94081),(#94082,#94083,
#94084,#94085)),.UNSPECIFIED.,.F.,.F.,.F.,(4,4),(4,4),(-0.00286791014463769,
0.477902879787847),(0.0100271466769354,0.0166015299239863),
 .UNSPECIFIED.);
#2870=B_SPLINE_SURFACE_WITH_KNOTS('',3,3,((#94087,#94088,#94089,#94090),
(#94091,#94092,#94093,#94094),(#94095,#94096,#94097,#94098),(#94099,#94100,
#94101,#94102)),.UNSPECIFIED.,.F.,.F.,.F.,(4,4),(4,4),(0.653230271487996,
1.00206901890057),(0.0065678839538601,0.0131849432428959),.UNSPECIFIED.);
#2871=B_SPLINE_SURFACE_WITH_KNOTS('',3,3,((#94110,#94111,#94112,#94113),
(#94114,#94115,#94116,#94117),(#94118,#94119,#94120,#94121),(#94122,#94123,
#94124,#94125)),.UNSPECIFIED.,.F.,.F.,.F.,(4,4),(4,4),(-0.00286780410470499,
0.477902879789078),(0.0200175229646918,0.0265907346180623),
 .UNSPECIFIED.);
#2872=B_SPLINE_SURFACE_WITH_KNOTS('',3,3,((#94127,#94128,#94129,#94130),
(#94131,#94132,#94133,#94134),(#94135,#94136,#94137,#94138),(#94139,#94140,
#94141,#94142)),.UNSPECIFIED.,.F.,.F.,.F.,(4,4),(4,4),(0.522097120187148,
1.00286753160136),(0.0166015299239889,0.023173678807522),.UNSPECIFIED.);
#2873=B_SPLINE_SURFACE_WITH_KNOTS('',3,3,((#94144,#94145,#94146,#94147),
(#94148,#94149,#94150,#94151),(#94152,#94153,#94154,#94155),(#94156,#94157,
#94158,#94159)),.UNSPECIFIED.,.F.,.F.,.F.,(4,4),(4,4),(0.,1.00600003961348),
(0.0166015299239894,0.0265907346180641),.UNSPECIFIED.);
#2874=B_SPLINE_SURFACE_WITH_KNOTS('',3,3,((#94160,#94161,#94162,#94163),
(#94164,#94165,#94166,#94167),(#94168,#94169,#94170,#94171),(#94172,#94173,
#94174,#94175)),.UNSPECIFIED.,.F.,.F.,.F.,(4,4),(4,4),(-0.00286862201164332,
0.47790287979074),(0.0300094532292789,0.0365944846647017),.UNSPECIFIED.);
#2875=B_SPLINE_SURFACE_WITH_KNOTS('',3,3,((#94177,#94178,#94179,#94180),
(#94181,#94182,#94183,#94184),(#94185,#94186,#94187,#94188),(#94189,#94190,
#94191,#94192)),.UNSPECIFIED.,.F.,.F.,.F.,(4,4),(4,4),(0.522097120187057,
1.00286823669314),(0.0265907346180631,0.0331702036889925),.UNSPECIFIED.);
#2876=B_SPLINE_SURFACE_WITH_KNOTS('',3,3,((#94200,#94201,#94202,#94203),
(#94204,#94205,#94206,#94207),(#94208,#94209,#94210,#94211),(#94212,#94213,
#94214,#94215)),.UNSPECIFIED.,.F.,.F.,.F.,(4,4),(4,4),(-0.00286848453332952,
0.477902879791493),(0.0400218729466608,0.0466073985929421),
 .UNSPECIFIED.);
#2877=B_SPLINE_SURFACE_WITH_KNOTS('',3,3,((#94232,#94233,#94234,#94235),
(#94236,#94237,#94238,#94239),(#94240,#94241,#94242,#94243),(#94244,#94245,
#94246,#94247)),.UNSPECIFIED.,.F.,.F.,.F.,(4,4),(4,4),(0.,1.00600014639748),
(0.0365944846644985,0.0466073985929158),.UNSPECIFIED.);
#2878=B_SPLINE_SURFACE_WITH_KNOTS('',3,3,((#94248,#94249,#94250,#94251),
(#94252,#94253,#94254,#94255),(#94256,#94257,#94258,#94259),(#94260,#94261,
#94262,#94263)),.UNSPECIFIED.,.F.,.F.,.F.,(4,4),(4,4),(-0.00286780122465239,
0.477902879792368),(0.0500263550858997,0.0565997133101407),
 .UNSPECIFIED.);
#2879=B_SPLINE_SURFACE_WITH_KNOTS('',3,3,((#94265,#94266,#94267,#94268),
(#94269,#94270,#94271,#94272),(#94273,#94274,#94275,#94276),(#94277,#94278,
#94279,#94280)),.UNSPECIFIED.,.F.,.F.,.F.,(4,4),(4,4),(0.522097120187087,
1.00286810177271),(0.046607398592944,0.0531834925888927),.UNSPECIFIED.);
#2880=B_SPLINE_SURFACE_WITH_KNOTS('',3,3,((#94288,#94289,#94290,#94291),
(#94292,#94293,#94294,#94295),(#94296,#94297,#94298,#94299),(#94300,#94301,
#94302,#94303)),.UNSPECIFIED.,.F.,.F.,.F.,(4,4),(4,4),(-0.00286792598898423,
0.477902879793432),(0.0600156865494613,0.0665898698871174),
 .UNSPECIFIED.);
#2881=B_SPLINE_SURFACE_WITH_KNOTS('',3,3,((#94305,#94306,#94307,#94308),
(#94309,#94310,#94311,#94312),(#94313,#94314,#94315,#94316),(#94317,#94318,
#94319,#94320)),.UNSPECIFIED.,.F.,.F.,.F.,(4,4),(4,4),(0.522097120191966,
1.00286764392046),(0.0565997133101417,0.0631721430887065),.UNSPECIFIED.);
#2882=B_SPLINE_SURFACE_WITH_KNOTS('',3,3,((#94336,#94337,#94338,#94339),
(#94340,#94341,#94342,#94343),(#94344,#94345,#94346,#94347),(#94348,#94349,
#94350,#94351)),.UNSPECIFIED.,.F.,.F.,.F.,(4,4),(4,4),(0.522097120187141,
1.00286833998606),(0.0665898698871199,0.0731716198748447),.UNSPECIFIED.);
#2883=B_SPLINE_SURFACE_WITH_KNOTS('',3,3,((#94352,#94353,#94354,#94355),
(#94356,#94357,#94358,#94359),(#94360,#94361,#94362,#94363),(#94364,#94365,
#94366,#94367)),.UNSPECIFIED.,.F.,.F.,.F.,(4,4),(4,4),(-0.00124731531428327,
0.20904511169693),(0.0700194292967153,0.0749900982977941),.UNSPECIFIED.);
#2884=B_SPLINE_SURFACE_WITH_KNOTS('',3,3,((#94374,#94375,#94376,#94377),
(#94378,#94379,#94380,#94381),(#94382,#94383,#94384,#94385),(#94386,#94387,
#94388,#94389)),.UNSPECIFIED.,.F.,.F.,.F.,(4,4),(4,4),(-0.00286791014465478,
0.47790287978797),(0.010027146676937,0.0166015299239869),.UNSPECIFIED.);
#2885=B_SPLINE_SURFACE_WITH_KNOTS('',3,3,((#94391,#94392,#94393,#94394),
(#94395,#94396,#94397,#94398),(#94399,#94400,#94401,#94402),(#94403,#94404,
#94405,#94406)),.UNSPECIFIED.,.F.,.F.,.F.,(4,4),(4,4),(0.653230271488951,
1.00206901890119),(0.00656788395403398,0.0131849432121938),
 .UNSPECIFIED.);
#2886=B_SPLINE_SURFACE_WITH_KNOTS('',3,3,((#94414,#94415,#94416,#94417),
(#94418,#94419,#94420,#94421),(#94422,#94423,#94424,#94425),(#94426,#94427,
#94428,#94429)),.UNSPECIFIED.,.F.,.F.,.F.,(4,4),(4,4),(-0.00286780410476047,
0.477902879787733),(0.0200175229646912,0.0265907346180626),
 .UNSPECIFIED.);
#2887=B_SPLINE_SURFACE_WITH_KNOTS('',3,3,((#94431,#94432,#94433,#94434),
(#94435,#94436,#94437,#94438),(#94439,#94440,#94441,#94442),(#94443,#94444,
#94445,#94446)),.UNSPECIFIED.,.F.,.F.,.F.,(4,4),(4,4),(0.522097120187582,
1.00286753160139),(0.016601529923988,0.0231736788075219),.UNSPECIFIED.);
#2888=B_SPLINE_SURFACE_WITH_KNOTS('',3,3,((#94448,#94449,#94450,#94451),
(#94452,#94453,#94454,#94455),(#94456,#94457,#94458,#94459),(#94460,#94461,
#94462,#94463)),.UNSPECIFIED.,.F.,.F.,.F.,(4,4),(4,4),(0.,1.00600003961397),
(0.0166015299239893,0.0265907346180646),.UNSPECIFIED.);
#2889=B_SPLINE_SURFACE_WITH_KNOTS('',3,3,((#94464,#94465,#94466,#94467),
(#94468,#94469,#94470,#94471),(#94472,#94473,#94474,#94475),(#94476,#94477,
#94478,#94479)),.UNSPECIFIED.,.F.,.F.,.F.,(4,4),(4,4),(-0.00286862201159924,
0.477902879789508),(0.0300094532292792,0.036594484664703),.UNSPECIFIED.);
#2890=B_SPLINE_SURFACE_WITH_KNOTS('',3,3,((#94481,#94482,#94483,#94484),
(#94485,#94486,#94487,#94488),(#94489,#94490,#94491,#94492),(#94493,#94494,
#94495,#94496)),.UNSPECIFIED.,.F.,.F.,.F.,(4,4),(4,4),(0.522097120187338,
1.00286823669316),(0.0265907346180638,0.0331702036889928),.UNSPECIFIED.);
#2891=B_SPLINE_SURFACE_WITH_KNOTS('',3,3,((#94504,#94505,#94506,#94507),
(#94508,#94509,#94510,#94511),(#94512,#94513,#94514,#94515),(#94516,#94517,
#94518,#94519)),.UNSPECIFIED.,.F.,.F.,.F.,(4,4),(4,4),(-0.0028684845333738,
0.477902879789181),(0.0400218729466608,0.0466073985929428),
 .UNSPECIFIED.);
#2892=B_SPLINE_SURFACE_WITH_KNOTS('',3,3,((#94536,#94537,#94538,#94539),
(#94540,#94541,#94542,#94543),(#94544,#94545,#94546,#94547),(#94548,#94549,
#94550,#94551)),.UNSPECIFIED.,.F.,.F.,.F.,(4,4),(4,4),(0.,1.00600014639733),
(0.0365944846644987,0.0466073985929149),.UNSPECIFIED.);
#2893=B_SPLINE_SURFACE_WITH_KNOTS('',3,3,((#94552,#94553,#94554,#94555),
(#94556,#94557,#94558,#94559),(#94560,#94561,#94562,#94563),(#94564,#94565,
#94566,#94567)),.UNSPECIFIED.,.F.,.F.,.F.,(4,4),(4,4),(-0.0028678012246552,
0.477902879790202),(0.0500263550859005,0.0565997133101566),
 .UNSPECIFIED.);
#2894=B_SPLINE_SURFACE_WITH_KNOTS('',3,3,((#94569,#94570,#94571,#94572),
(#94573,#94574,#94575,#94576),(#94577,#94578,#94579,#94580),(#94581,#94582,
#94583,#94584)),.UNSPECIFIED.,.F.,.F.,.F.,(4,4),(4,4),(0.522097120187115,
1.00286810177277),(0.0466073985929444,0.0531834925888919),.UNSPECIFIED.);
#2895=B_SPLINE_SURFACE_WITH_KNOTS('',3,3,((#94592,#94593,#94594,#94595),
(#94596,#94597,#94598,#94599),(#94600,#94601,#94602,#94603),(#94604,#94605,
#94606,#94607)),.UNSPECIFIED.,.F.,.F.,.F.,(4,4),(4,4),(-0.00286792598901002,
0.477902879791329),(0.0600156865494609,0.0665898698871177),
 .UNSPECIFIED.);
#2896=B_SPLINE_SURFACE_WITH_KNOTS('',3,3,((#94609,#94610,#94611,#94612),
(#94613,#94614,#94615,#94616),(#94617,#94618,#94619,#94620),(#94621,#94622,
#94623,#94624)),.UNSPECIFIED.,.F.,.F.,.F.,(4,4),(4,4),(0.522097120191972,
1.00286764392054),(0.0565997133101411,0.0631721430887067),.UNSPECIFIED.);
#2897=B_SPLINE_SURFACE_WITH_KNOTS('',3,3,((#94640,#94641,#94642,#94643),
(#94644,#94645,#94646,#94647),(#94648,#94649,#94650,#94651),(#94652,#94653,
#94654,#94655)),.UNSPECIFIED.,.F.,.F.,.F.,(4,4),(4,4),(0.522097120186964,
1.00286833998601),(0.0665898698871194,0.073171619874845),.UNSPECIFIED.);
#2898=B_SPLINE_SURFACE_WITH_KNOTS('',3,3,((#94656,#94657,#94658,#94659),
(#94660,#94661,#94662,#94663),(#94664,#94665,#94666,#94667),(#94668,#94669,
#94670,#94671)),.UNSPECIFIED.,.F.,.F.,.F.,(4,4),(4,4),(-0.00124731531647025,
0.209045111694821),(0.0700194292967201,0.0749900982977851),
 .UNSPECIFIED.);
#2899=B_SPLINE_SURFACE_WITH_KNOTS('',3,3,((#94678,#94679,#94680,#94681),
(#94682,#94683,#94684,#94685),(#94686,#94687,#94688,#94689),(#94690,#94691,
#94692,#94693)),.UNSPECIFIED.,.F.,.F.,.F.,(4,4),(4,4),(-0.00286791014469107,
0.477902879787991),(0.0100271466769376,0.0166015299239867),
 .UNSPECIFIED.);
#2900=B_SPLINE_SURFACE_WITH_KNOTS('',3,3,((#94695,#94696,#94697,#94698),
(#94699,#94700,#94701,#94702),(#94703,#94704,#94705,#94706),(#94707,#94708,
#94709,#94710)),.UNSPECIFIED.,.F.,.F.,.F.,(4,4),(4,4),(0.653230271490066,
1.00206901890208),(0.00656788395384224,0.013184943242989),.UNSPECIFIED.);
#2901=B_SPLINE_SURFACE_WITH_KNOTS('',3,3,((#94718,#94719,#94720,#94721),
(#94722,#94723,#94724,#94725),(#94726,#94727,#94728,#94729),(#94730,#94731,
#94732,#94733)),.UNSPECIFIED.,.F.,.F.,.F.,(4,4),(4,4),(-0.00286780410467914,
0.47790287978789),(0.0200175229646906,0.0265907346180624),.UNSPECIFIED.);
#2902=B_SPLINE_SURFACE_WITH_KNOTS('',3,3,((#94735,#94736,#94737,#94738),
(#94739,#94740,#94741,#94742),(#94743,#94744,#94745,#94746),(#94747,#94748,
#94749,#94750)),.UNSPECIFIED.,.F.,.F.,.F.,(4,4),(4,4),(0.522097120188421,
1.0028675316014),(0.0166015299239883,0.0231736788075223),.UNSPECIFIED.);
#2903=B_SPLINE_SURFACE_WITH_KNOTS('',3,3,((#94752,#94753,#94754,#94755),
(#94756,#94757,#94758,#94759),(#94760,#94761,#94762,#94763),(#94764,#94765,
#94766,#94767)),.UNSPECIFIED.,.F.,.F.,.F.,(4,4),(4,4),(0.,1.00600003961381),
(0.0166015299239883,0.0265907346180636),.UNSPECIFIED.);
#2904=B_SPLINE_SURFACE_WITH_KNOTS('',3,3,((#94768,#94769,#94770,#94771),
(#94772,#94773,#94774,#94775),(#94776,#94777,#94778,#94779),(#94780,#94781,
#94782,#94783)),.UNSPECIFIED.,.F.,.F.,.F.,(4,4),(4,4),(-0.00286862201160178,
0.477902879789629),(0.030009453229279,0.0365944846647018),.UNSPECIFIED.);
#2905=B_SPLINE_SURFACE_WITH_KNOTS('',3,3,((#94785,#94786,#94787,#94788),
(#94789,#94790,#94791,#94792),(#94793,#94794,#94795,#94796),(#94797,#94798,
#94799,#94800)),.UNSPECIFIED.,.F.,.F.,.F.,(4,4),(4,4),(0.522097120187916,
1.00286823669319),(0.0265907346180628,0.0331702036889921),.UNSPECIFIED.);
#2906=B_SPLINE_SURFACE_WITH_KNOTS('',3,3,((#94808,#94809,#94810,#94811),
(#94812,#94813,#94814,#94815),(#94816,#94817,#94818,#94819),(#94820,#94821,
#94822,#94823)),.UNSPECIFIED.,.F.,.F.,.F.,(4,4),(4,4),(-0.00286848453385445,
0.47790287986132),(0.0400218729466611,0.0466073985929426),.UNSPECIFIED.);
#2907=B_SPLINE_SURFACE_WITH_KNOTS('',3,3,((#94840,#94841,#94842,#94843),
(#94844,#94845,#94846,#94847),(#94848,#94849,#94850,#94851),(#94852,#94853,
#94854,#94855)),.UNSPECIFIED.,.F.,.F.,.F.,(4,4),(4,4),(0.,1.00600014639724),
(0.0365944846644992,0.0466073985929183),.UNSPECIFIED.);
#2908=B_SPLINE_SURFACE_WITH_KNOTS('',3,3,((#94856,#94857,#94858,#94859),
(#94860,#94861,#94862,#94863),(#94864,#94865,#94866,#94867),(#94868,#94869,
#94870,#94871)),.UNSPECIFIED.,.F.,.F.,.F.,(4,4),(4,4),(-0.00286780122466993,
0.477902879787799),(0.0500263550859,0.0565997133101405),.UNSPECIFIED.);
#2909=B_SPLINE_SURFACE_WITH_KNOTS('',3,3,((#94873,#94874,#94875,#94876),
(#94877,#94878,#94879,#94880),(#94881,#94882,#94883,#94884),(#94885,#94886,
#94887,#94888)),.UNSPECIFIED.,.F.,.F.,.F.,(4,4),(4,4),(0.522097120187333,
1.00286810177263),(0.0466073985929444,0.0531834925888926),.UNSPECIFIED.);
#2910=B_SPLINE_SURFACE_WITH_KNOTS('',3,3,((#94896,#94897,#94898,#94899),
(#94900,#94901,#94902,#94903),(#94904,#94905,#94906,#94907),(#94908,#94909,
#94910,#94911)),.UNSPECIFIED.,.F.,.F.,.F.,(4,4),(4,4),(-0.00286792598906402,
0.477902879788954),(0.0600156865494604,0.0665898698871162),
 .UNSPECIFIED.);
#2911=B_SPLINE_SURFACE_WITH_KNOTS('',3,3,((#94913,#94914,#94915,#94916),
(#94917,#94918,#94919,#94920),(#94921,#94922,#94923,#94924),(#94925,#94926,
#94927,#94928)),.UNSPECIFIED.,.F.,.F.,.F.,(4,4),(4,4),(0.52209712019194,
1.00286764392053),(0.0565997133101412,0.0631721430887059),.UNSPECIFIED.);
#2912=B_SPLINE_SURFACE_WITH_KNOTS('',3,3,((#94944,#94945,#94946,#94947),
(#94948,#94949,#94950,#94951),(#94952,#94953,#94954,#94955),(#94956,#94957,
#94958,#94959)),.UNSPECIFIED.,.F.,.F.,.F.,(4,4),(4,4),(0.522097120186829,
1.00286833998607),(0.0665898698871188,0.073171619874845),.UNSPECIFIED.);
#2913=B_SPLINE_SURFACE_WITH_KNOTS('',3,3,((#94960,#94961,#94962,#94963),
(#94964,#94965,#94966,#94967),(#94968,#94969,#94970,#94971),(#94972,#94973,
#94974,#94975)),.UNSPECIFIED.,.F.,.F.,.F.,(4,4),(4,4),(-0.00124731531869756,
0.209045111692496),(0.0700194292967225,0.0749900982977736),
 .UNSPECIFIED.);
#2914=B_SPLINE_SURFACE_WITH_KNOTS('',3,3,((#94982,#94983,#94984,#94985),
(#94986,#94987,#94988,#94989),(#94990,#94991,#94992,#94993),(#94994,#94995,
#94996,#94997)),.UNSPECIFIED.,.F.,.F.,.F.,(4,4),(4,4),(-0.00286791014473155,
0.477902879788205),(0.0100271466769362,0.0166015299239883),
 .UNSPECIFIED.);
#2915=B_SPLINE_SURFACE_WITH_KNOTS('',3,3,((#94999,#95000,#95001,#95002),
(#95003,#95004,#95005,#95006),(#95007,#95008,#95009,#95010),(#95011,#95012,
#95013,#95014)),.UNSPECIFIED.,.F.,.F.,.F.,(4,4),(4,4),(0.653230271491342,
1.00206901890342),(0.00656788395383524,0.0131849432428966),
 .UNSPECIFIED.);
#2916=B_SPLINE_SURFACE_WITH_KNOTS('',3,3,((#95022,#95023,#95024,#95025),
(#95026,#95027,#95028,#95029),(#95030,#95031,#95032,#95033),(#95034,#95035,
#95036,#95037)),.UNSPECIFIED.,.F.,.F.,.F.,(4,4),(4,4),(-0.00286780410464737,
0.477902879787977),(0.0200175229646909,0.0265907346180625),
 .UNSPECIFIED.);
#2917=B_SPLINE_SURFACE_WITH_KNOTS('',3,3,((#95039,#95040,#95041,#95042),
(#95043,#95044,#95045,#95046),(#95047,#95048,#95049,#95050),(#95051,#95052,
#95053,#95054)),.UNSPECIFIED.,.F.,.F.,.F.,(4,4),(4,4),(0.522097120189436,
1.0028675316014),(0.0166015299239882,0.0231736788037103),.UNSPECIFIED.);
#2918=B_SPLINE_SURFACE_WITH_KNOTS('',3,3,((#95056,#95057,#95058,#95059),
(#95060,#95061,#95062,#95063),(#95064,#95065,#95066,#95067),(#95068,#95069,
#95070,#95071)),.UNSPECIFIED.,.F.,.F.,.F.,(4,4),(4,4),(0.,1.00600003961361),
(0.0166015299239868,0.0265907346180623),.UNSPECIFIED.);
#2919=B_SPLINE_SURFACE_WITH_KNOTS('',3,3,((#95072,#95073,#95074,#95075),
(#95076,#95077,#95078,#95079),(#95080,#95081,#95082,#95083),(#95084,#95085,
#95086,#95087)),.UNSPECIFIED.,.F.,.F.,.F.,(4,4),(4,4),(-0.00286862201168353,
0.477902879789614),(0.0300094532292789,0.036594484664702),.UNSPECIFIED.);
#2920=B_SPLINE_SURFACE_WITH_KNOTS('',3,3,((#95089,#95090,#95091,#95092),
(#95093,#95094,#95095,#95096),(#95097,#95098,#95099,#95100),(#95101,#95102,
#95103,#95104)),.UNSPECIFIED.,.F.,.F.,.F.,(4,4),(4,4),(0.522097120188798,
1.00286823669314),(0.0265907346180632,0.0331702036622774),.UNSPECIFIED.);
#2921=B_SPLINE_SURFACE_WITH_KNOTS('',3,3,((#95112,#95113,#95114,#95115),
(#95116,#95117,#95118,#95119),(#95120,#95121,#95122,#95123),(#95124,#95125,
#95126,#95127)),.UNSPECIFIED.,.F.,.F.,.F.,(4,4),(4,4),(-0.00286848453343133,
0.477902879788268),(0.0400218729466607,0.046607398592943),.UNSPECIFIED.);
#2922=B_SPLINE_SURFACE_WITH_KNOTS('',3,3,((#95144,#95145,#95146,#95147),
(#95148,#95149,#95150,#95151),(#95152,#95153,#95154,#95155),(#95156,#95157,
#95158,#95159)),.UNSPECIFIED.,.F.,.F.,.F.,(4,4),(4,4),(0.,1.00600014639763),
(0.0365944846644997,0.0466073985929161),.UNSPECIFIED.);
#2923=B_SPLINE_SURFACE_WITH_KNOTS('',3,3,((#95160,#95161,#95162,#95163),
(#95164,#95165,#95166,#95167),(#95168,#95169,#95170,#95171),(#95172,#95173,
#95174,#95175)),.UNSPECIFIED.,.F.,.F.,.F.,(4,4),(4,4),(-0.00286780122468948,
0.477902879787664),(0.0500263550858997,0.0565997133101402),
 .UNSPECIFIED.);
#2924=B_SPLINE_SURFACE_WITH_KNOTS('',3,3,((#95177,#95178,#95179,#95180),
(#95181,#95182,#95183,#95184),(#95185,#95186,#95187,#95188),(#95189,#95190,
#95191,#95192)),.UNSPECIFIED.,.F.,.F.,.F.,(4,4),(4,4),(0.522097120187869,
1.00286810177258),(0.0466073985929447,0.0531834922865672),.UNSPECIFIED.);
#2925=B_SPLINE_SURFACE_WITH_KNOTS('',3,3,((#95200,#95201,#95202,#95203),
(#95204,#95205,#95206,#95207),(#95208,#95209,#95210,#95211),(#95212,#95213,
#95214,#95215)),.UNSPECIFIED.,.F.,.F.,.F.,(4,4),(4,4),(-0.00286792598893663,
0.477902879787536),(0.0600156865494607,0.0665898698871167),
 .UNSPECIFIED.);
#2926=B_SPLINE_SURFACE_WITH_KNOTS('',3,3,((#95217,#95218,#95219,#95220),
(#95221,#95222,#95223,#95224),(#95225,#95226,#95227,#95228),(#95229,#95230,
#95231,#95232)),.UNSPECIFIED.,.F.,.F.,.F.,(4,4),(4,4),(0.522097120192148,
1.00286764392044),(0.0565997133101418,0.0631721430887059),.UNSPECIFIED.);
#2927=B_SPLINE_SURFACE_WITH_KNOTS('',3,3,((#95248,#95249,#95250,#95251),
(#95252,#95253,#95254,#95255),(#95256,#95257,#95258,#95259),(#95260,#95261,
#95262,#95263)),.UNSPECIFIED.,.F.,.F.,.F.,(4,4),(4,4),(0.52209712018707,
1.00286833998598),(0.0665898698871193,0.0731716198748453),.UNSPECIFIED.);
#2928=B_SPLINE_SURFACE_WITH_KNOTS('',3,3,((#95264,#95265,#95266,#95267),
(#95268,#95269,#95270,#95271),(#95272,#95273,#95274,#95275),(#95276,#95277,
#95278,#95279)),.UNSPECIFIED.,.F.,.F.,.F.,(4,4),(4,4),(-0.00124731532117962,
0.209045111690077),(0.0700194292967239,0.0749900982977618),
 .UNSPECIFIED.);
#2929=B_SPLINE_SURFACE_WITH_KNOTS('',3,3,((#95286,#95287,#95288,#95289),
(#95290,#95291,#95292,#95293),(#95294,#95295,#95296,#95297),(#95298,#95299,
#95300,#95301)),.UNSPECIFIED.,.F.,.F.,.F.,(4,4),(4,4),(-0.00286791014476839,
0.477902879788331),(0.010027146676934,0.0166015299239869),.UNSPECIFIED.);
#2930=B_SPLINE_SURFACE_WITH_KNOTS('',3,3,((#95303,#95304,#95305,#95306),
(#95307,#95308,#95309,#95310),(#95311,#95312,#95313,#95314),(#95315,#95316,
#95317,#95318)),.UNSPECIFIED.,.F.,.F.,.F.,(4,4),(4,4),(0.653230271492636,
1.00206901890481),(0.00656788395382744,0.0131849432429878),
 .UNSPECIFIED.);
#2931=B_SPLINE_SURFACE_WITH_KNOTS('',3,3,((#95326,#95327,#95328,#95329),
(#95330,#95331,#95332,#95333),(#95334,#95335,#95336,#95337),(#95338,#95339,
#95340,#95341)),.UNSPECIFIED.,.F.,.F.,.F.,(4,4),(4,4),(-0.00286780410474824,
0.477902879788205),(0.0200175229646895,0.0265907346180613),
 .UNSPECIFIED.);
#2932=B_SPLINE_SURFACE_WITH_KNOTS('',3,3,((#95343,#95344,#95345,#95346),
(#95347,#95348,#95349,#95350),(#95351,#95352,#95353,#95354),(#95355,#95356,
#95357,#95358)),.UNSPECIFIED.,.F.,.F.,.F.,(4,4),(4,4),(0.522097120190702,
1.00286753160135),(0.0166015299239877,0.0231736788037103),.UNSPECIFIED.);
#2933=B_SPLINE_SURFACE_WITH_KNOTS('',3,3,((#95360,#95361,#95362,#95363),
(#95364,#95365,#95366,#95367),(#95368,#95369,#95370,#95371),(#95372,#95373,
#95374,#95375)),.UNSPECIFIED.,.F.,.F.,.F.,(4,4),(4,4),(0.,1.00600003961362),
(0.0166015299239903,0.0265907346180637),.UNSPECIFIED.);
#2934=B_SPLINE_SURFACE_WITH_KNOTS('',3,3,((#95376,#95377,#95378,#95379),
(#95380,#95381,#95382,#95383),(#95384,#95385,#95386,#95387),(#95388,#95389,
#95390,#95391)),.UNSPECIFIED.,.F.,.F.,.F.,(4,4),(4,4),(-0.0028686220116881,
0.477902879789794),(0.0300094532292792,0.0365944846647018),
 .UNSPECIFIED.);
#2935=B_SPLINE_SURFACE_WITH_KNOTS('',3,3,((#95393,#95394,#95395,#95396),
(#95397,#95398,#95399,#95400),(#95401,#95402,#95403,#95404),(#95405,#95406,
#95407,#95408)),.UNSPECIFIED.,.F.,.F.,.F.,(4,4),(4,4),(0.522097120190027,
1.00286823669311),(0.0265907346180631,0.0331702036889928),.UNSPECIFIED.);
#2936=B_SPLINE_SURFACE_WITH_KNOTS('',3,3,((#95416,#95417,#95418,#95419),
(#95420,#95421,#95422,#95423),(#95424,#95425,#95426,#95427),(#95428,#95429,
#95430,#95431)),.UNSPECIFIED.,.F.,.F.,.F.,(4,4),(4,4),(-0.00286848453347387,
0.477902879788492),(0.0400218729466595,0.0466073985929424),
 .UNSPECIFIED.);
#2937=B_SPLINE_SURFACE_WITH_KNOTS('',3,3,((#95448,#95449,#95450,#95451),
(#95452,#95453,#95454,#95455),(#95456,#95457,#95458,#95459),(#95460,#95461,
#95462,#95463)),.UNSPECIFIED.,.F.,.F.,.F.,(4,4),(4,4),(0.,1.00600014639749),
(0.0365944846644999,0.0466073985929169),.UNSPECIFIED.);
#2938=B_SPLINE_SURFACE_WITH_KNOTS('',3,3,((#95464,#95465,#95466,#95467),
(#95468,#95469,#95470,#95471),(#95472,#95473,#95474,#95475),(#95476,#95477,
#95478,#95479)),.UNSPECIFIED.,.F.,.F.,.F.,(4,4),(4,4),(-0.00286780122467789,
0.477902879787799),(0.0500263550858996,0.0565997133101406),
 .UNSPECIFIED.);
#2939=B_SPLINE_SURFACE_WITH_KNOTS('',3,3,((#95481,#95482,#95483,#95484),
(#95485,#95486,#95487,#95488),(#95489,#95490,#95491,#95492),(#95493,#95494,
#95495,#95496)),.UNSPECIFIED.,.F.,.F.,.F.,(4,4),(4,4),(0.522097120188824,
1.00286810177264),(0.0466073985929438,0.0531834925888932),.UNSPECIFIED.);
#2940=B_SPLINE_SURFACE_WITH_KNOTS('',3,3,((#95504,#95505,#95506,#95507),
(#95508,#95509,#95510,#95511),(#95512,#95513,#95514,#95515),(#95516,#95517,
#95518,#95519)),.UNSPECIFIED.,.F.,.F.,.F.,(4,4),(4,4),(-0.0028679259889164,
0.477902879787716),(0.0600156865494595,0.066589869887117),.UNSPECIFIED.);
#2941=B_SPLINE_SURFACE_WITH_KNOTS('',3,3,((#95521,#95522,#95523,#95524),
(#95525,#95526,#95527,#95528),(#95529,#95530,#95531,#95532),(#95533,#95534,
#95535,#95536)),.UNSPECIFIED.,.F.,.F.,.F.,(4,4),(4,4),(0.522097120192599,
1.00286764392051),(0.0565997133101417,0.0631721430887069),.UNSPECIFIED.);
#2942=B_SPLINE_SURFACE_WITH_KNOTS('',3,3,((#95552,#95553,#95554,#95555),
(#95556,#95557,#95558,#95559),(#95560,#95561,#95562,#95563),(#95564,#95565,
#95566,#95567)),.UNSPECIFIED.,.F.,.F.,.F.,(4,4),(4,4),(0.522097120187818,
1.00286833998607),(0.0665898698871186,0.0731716198748448),.UNSPECIFIED.);
#2943=B_SPLINE_SURFACE_WITH_KNOTS('',3,3,((#95568,#95569,#95570,#95571),
(#95572,#95573,#95574,#95575),(#95576,#95577,#95578,#95579),(#95580,#95581,
#95582,#95583)),.UNSPECIFIED.,.F.,.F.,.F.,(4,4),(4,4),(-0.0012473153236173,
0.209045111687613),(0.0700194292967237,0.0749900982977506),
 .UNSPECIFIED.);
#2944=B_SPLINE_SURFACE_WITH_KNOTS('',3,3,((#95590,#95591,#95592,#95593),
(#95594,#95595,#95596,#95597),(#95598,#95599,#95600,#95601),(#95602,#95603,
#95604,#95605)),.UNSPECIFIED.,.F.,.F.,.F.,(4,4),(4,4),(-0.00286791014474091,
0.477902879788312),(0.0100271466769347,0.0166015299239868),
 .UNSPECIFIED.);
#2945=B_SPLINE_SURFACE_WITH_KNOTS('',3,3,((#95607,#95608,#95609,#95610),
(#95611,#95612,#95613,#95614),(#95615,#95616,#95617,#95618),(#95619,#95620,
#95621,#95622)),.UNSPECIFIED.,.F.,.F.,.F.,(4,4),(4,4),(0.653230271494008,
1.00206901890662),(0.00656788395382045,0.0131849432428963),
 .UNSPECIFIED.);
#2946=B_SPLINE_SURFACE_WITH_KNOTS('',3,3,((#95630,#95631,#95632,#95633),
(#95634,#95635,#95636,#95637),(#95638,#95639,#95640,#95641),(#95642,#95643,
#95644,#95645)),.UNSPECIFIED.,.F.,.F.,.F.,(4,4),(4,4),(-0.00286780410476748,
0.477902879788327),(0.0200175229646906,0.0265907346180623),
 .UNSPECIFIED.);
#2947=B_SPLINE_SURFACE_WITH_KNOTS('',3,3,((#95647,#95648,#95649,#95650),
(#95651,#95652,#95653,#95654),(#95655,#95656,#95657,#95658),(#95659,#95660,
#95661,#95662)),.UNSPECIFIED.,.F.,.F.,.F.,(4,4),(4,4),(0.522097120192319,
1.00286753160135),(0.016601529923988,0.0231736788037106),.UNSPECIFIED.);
#2948=B_SPLINE_SURFACE_WITH_KNOTS('',3,3,((#95664,#95665,#95666,#95667),
(#95668,#95669,#95670,#95671),(#95672,#95673,#95674,#95675),(#95676,#95677,
#95678,#95679)),.UNSPECIFIED.,.F.,.F.,.F.,(4,4),(4,4),(0.,1.00600003961367),
(0.0166015299239903,0.0265907346180654),.UNSPECIFIED.);
#2949=B_SPLINE_SURFACE_WITH_KNOTS('',3,3,((#95680,#95681,#95682,#95683),
(#95684,#95685,#95686,#95687),(#95688,#95689,#95690,#95691),(#95692,#95693,
#95694,#95695)),.UNSPECIFIED.,.F.,.F.,.F.,(4,4),(4,4),(-0.00286862201167118,
0.477902879789893),(0.0300094532292783,0.0365944846647164),
 .UNSPECIFIED.);
#2950=B_SPLINE_SURFACE_WITH_KNOTS('',3,3,((#95697,#95698,#95699,#95700),
(#95701,#95702,#95703,#95704),(#95705,#95706,#95707,#95708),(#95709,#95710,
#95711,#95712)),.UNSPECIFIED.,.F.,.F.,.F.,(4,4),(4,4),(0.522097120191619,
1.0028682366931),(0.026590734618064,0.0331702036051744),.UNSPECIFIED.);
#2951=B_SPLINE_SURFACE_WITH_KNOTS('',3,3,((#95720,#95721,#95722,#95723),
(#95724,#95725,#95726,#95727),(#95728,#95729,#95730,#95731),(#95732,#95733,
#95734,#95735)),.UNSPECIFIED.,.F.,.F.,.F.,(4,4),(4,4),(-0.00286848453356115,
0.477902879788435),(0.0400218729466602,0.0466073985929428),
 .UNSPECIFIED.);
#2952=B_SPLINE_SURFACE_WITH_KNOTS('',3,3,((#95752,#95753,#95754,#95755),
(#95756,#95757,#95758,#95759),(#95760,#95761,#95762,#95763),(#95764,#95765,
#95766,#95767)),.UNSPECIFIED.,.F.,.F.,.F.,(4,4),(4,4),(0.,1.00600014639742),
(0.0365944846645018,0.046607398592917),.UNSPECIFIED.);
#2953=B_SPLINE_SURFACE_WITH_KNOTS('',3,3,((#95768,#95769,#95770,#95771),
(#95772,#95773,#95774,#95775),(#95776,#95777,#95778,#95779),(#95780,#95781,
#95782,#95783)),.UNSPECIFIED.,.F.,.F.,.F.,(4,4),(4,4),(-0.00286780122470004,
0.477902879787953),(0.0500263550858998,0.0565997133101408),
 .UNSPECIFIED.);
#2954=B_SPLINE_SURFACE_WITH_KNOTS('',3,3,((#95785,#95786,#95787,#95788),
(#95789,#95790,#95791,#95792),(#95793,#95794,#95795,#95796),(#95797,#95798,
#95799,#95800)),.UNSPECIFIED.,.F.,.F.,.F.,(4,4),(4,4),(0.522097120190077,
1.00286810177263),(0.0466073985929447,0.0531834925888939),.UNSPECIFIED.);
#2955=B_SPLINE_SURFACE_WITH_KNOTS('',3,3,((#95808,#95809,#95810,#95811),
(#95812,#95813,#95814,#95815),(#95816,#95817,#95818,#95819),(#95820,#95821,
#95822,#95823)),.UNSPECIFIED.,.F.,.F.,.F.,(4,4),(4,4),(-0.00286792598895217,
0.477902879787812),(0.0600156865494599,0.0665898698871171),
 .UNSPECIFIED.);
#2956=B_SPLINE_SURFACE_WITH_KNOTS('',3,3,((#95825,#95826,#95827,#95828),
(#95829,#95830,#95831,#95832),(#95833,#95834,#95835,#95836),(#95837,#95838,
#95839,#95840)),.UNSPECIFIED.,.F.,.F.,.F.,(4,4),(4,4),(0.522097120193104,
1.0028676439205),(0.0565997133101426,0.0631721430887066),.UNSPECIFIED.);
#2957=B_SPLINE_SURFACE_WITH_KNOTS('',3,3,((#95856,#95857,#95858,#95859),
(#95860,#95861,#95862,#95863),(#95864,#95865,#95866,#95867),(#95868,#95869,
#95870,#95871)),.UNSPECIFIED.,.F.,.F.,.F.,(4,4),(4,4),(0.522097120188608,
1.00286833998595),(0.0665898698871196,0.073171619874845),.UNSPECIFIED.);
#2958=B_SPLINE_SURFACE_WITH_KNOTS('',3,3,((#95872,#95873,#95874,#95875),
(#95876,#95877,#95878,#95879),(#95880,#95881,#95882,#95883),(#95884,#95885,
#95886,#95887)),.UNSPECIFIED.,.F.,.F.,.F.,(4,4),(4,4),(-0.00124731532625225,
0.209045111685989),(0.0700194292967225,0.0749900982977378),
 .UNSPECIFIED.);
#2959=B_SPLINE_SURFACE_WITH_KNOTS('',3,3,((#95894,#95895,#95896,#95897),
(#95898,#95899,#95900,#95901),(#95902,#95903,#95904,#95905),(#95906,#95907,
#95908,#95909)),.UNSPECIFIED.,.F.,.F.,.F.,(4,4),(4,4),(-0.00286791014464121,
0.477902879788685),(0.0100271466769344,0.0166015299239869),
 .UNSPECIFIED.);
#2960=B_SPLINE_SURFACE_WITH_KNOTS('',3,3,((#95911,#95912,#95913,#95914),
(#95915,#95916,#95917,#95918),(#95919,#95920,#95921,#95922),(#95923,#95924,
#95925,#95926)),.UNSPECIFIED.,.F.,.F.,.F.,(4,4),(4,4),(0.653230271495439,
1.00206901890855),(0.00656788395381374,0.0131849432429887),
 .UNSPECIFIED.);
#2961=B_SPLINE_SURFACE_WITH_KNOTS('',3,3,((#95934,#95935,#95936,#95937),
(#95938,#95939,#95940,#95941),(#95942,#95943,#95944,#95945),(#95946,#95947,
#95948,#95949)),.UNSPECIFIED.,.F.,.F.,.F.,(4,4),(4,4),(-0.00286780410480697,
0.477902879788339),(0.0200175229646895,0.026590734618062),.UNSPECIFIED.);
#2962=B_SPLINE_SURFACE_WITH_KNOTS('',3,3,((#95951,#95952,#95953,#95954),
(#95955,#95956,#95957,#95958),(#95959,#95960,#95961,#95962),(#95963,#95964,
#95965,#95966)),.UNSPECIFIED.,.F.,.F.,.F.,(4,4),(4,4),(0.522097120194227,
1.00286753160135),(0.0166015299239885,0.0231736788075229),.UNSPECIFIED.);
#2963=B_SPLINE_SURFACE_WITH_KNOTS('',3,3,((#95968,#95969,#95970,#95971),
(#95972,#95973,#95974,#95975),(#95976,#95977,#95978,#95979),(#95980,#95981,
#95982,#95983)),.UNSPECIFIED.,.F.,.F.,.F.,(4,4),(4,4),(0.,1.0060000396139),
(0.0166015299239893,0.0265907346180634),.UNSPECIFIED.);
#2964=B_SPLINE_SURFACE_WITH_KNOTS('',3,3,((#95984,#95985,#95986,#95987),
(#95988,#95989,#95990,#95991),(#95992,#95993,#95994,#95995),(#95996,#95997,
#95998,#95999)),.UNSPECIFIED.,.F.,.F.,.F.,(4,4),(4,4),(-0.00286862201168709,
0.477902879790105),(0.030009453229278,0.0365944846647019),.UNSPECIFIED.);
#2965=B_SPLINE_SURFACE_WITH_KNOTS('',3,3,((#96001,#96002,#96003,#96004),
(#96005,#96006,#96007,#96008),(#96009,#96010,#96011,#96012),(#96013,#96014,
#96015,#96016)),.UNSPECIFIED.,.F.,.F.,.F.,(4,4),(4,4),(0.522097120193262,
1.00286823669315),(0.0265907346180635,0.0331702036889921),.UNSPECIFIED.);
#2966=B_SPLINE_SURFACE_WITH_KNOTS('',3,3,((#96024,#96025,#96026,#96027),
(#96028,#96029,#96030,#96031),(#96032,#96033,#96034,#96035),(#96036,#96037,
#96038,#96039)),.UNSPECIFIED.,.F.,.F.,.F.,(4,4),(4,4),(-0.00286848453346161,
0.477902879788731),(0.0400218729466591,0.046607398592943),.UNSPECIFIED.);
#2967=B_SPLINE_SURFACE_WITH_KNOTS('',3,3,((#96056,#96057,#96058,#96059),
(#96060,#96061,#96062,#96063),(#96064,#96065,#96066,#96067),(#96068,#96069,
#96070,#96071)),.UNSPECIFIED.,.F.,.F.,.F.,(4,4),(4,4),(0.,1.00600014639745),
(0.0365944846645014,0.046607398592915),.UNSPECIFIED.);
#2968=B_SPLINE_SURFACE_WITH_KNOTS('',3,3,((#96072,#96073,#96074,#96075),
(#96076,#96077,#96078,#96079),(#96080,#96081,#96082,#96083),(#96084,#96085,
#96086,#96087)),.UNSPECIFIED.,.F.,.F.,.F.,(4,4),(4,4),(-0.00286780122479215,
0.477902879787963),(0.0500263550858996,0.0565997133101403),
 .UNSPECIFIED.);
#2969=B_SPLINE_SURFACE_WITH_KNOTS('',3,3,((#96089,#96090,#96091,#96092),
(#96093,#96094,#96095,#96096),(#96097,#96098,#96099,#96100),(#96101,#96102,
#96103,#96104)),.UNSPECIFIED.,.F.,.F.,.F.,(4,4),(4,4),(0.522097120191531,
1.00286810177261),(0.0466073985929444,0.0531834925888928),.UNSPECIFIED.);
#2970=B_SPLINE_SURFACE_WITH_KNOTS('',3,3,((#96112,#96113,#96114,#96115),
(#96116,#96117,#96118,#96119),(#96120,#96121,#96122,#96123),(#96124,#96125,
#96126,#96127)),.UNSPECIFIED.,.F.,.F.,.F.,(4,4),(4,4),(-0.0028679259889122,
0.47790287978794),(0.0600156865494595,0.0665898698871168),.UNSPECIFIED.);
#2971=B_SPLINE_SURFACE_WITH_KNOTS('',3,3,((#96129,#96130,#96131,#96132),
(#96133,#96134,#96135,#96136),(#96137,#96138,#96139,#96140),(#96141,#96142,
#96143,#96144)),.UNSPECIFIED.,.F.,.F.,.F.,(4,4),(4,4),(0.522097120193808,
1.00286764392049),(0.0565997133101416,0.0631721430887065),.UNSPECIFIED.);
#2972=B_SPLINE_SURFACE_WITH_KNOTS('',3,3,((#96160,#96161,#96162,#96163),
(#96164,#96165,#96166,#96167),(#96168,#96169,#96170,#96171),(#96172,#96173,
#96174,#96175)),.UNSPECIFIED.,.F.,.F.,.F.,(4,4),(4,4),(0.522097120189876,
1.00286833998599),(0.0665898698871201,0.073171619874845),.UNSPECIFIED.);
#2973=B_SPLINE_SURFACE_WITH_KNOTS('',3,3,((#96176,#96177,#96178,#96179),
(#96180,#96181,#96182,#96183),(#96184,#96185,#96186,#96187),(#96188,#96189,
#96190,#96191)),.UNSPECIFIED.,.F.,.F.,.F.,(4,4),(4,4),(-0.00124731532879475,
0.209045111684705),(0.070019429296718,0.0749900982977259),.UNSPECIFIED.);
#2974=B_SPLINE_SURFACE_WITH_KNOTS('',3,3,((#96198,#96199,#96200,#96201),
(#96202,#96203,#96204,#96205),(#96206,#96207,#96208,#96209),(#96210,#96211,
#96212,#96213)),.UNSPECIFIED.,.F.,.F.,.F.,(4,4),(4,4),(-0.00286791014460047,
0.477902879788786),(0.0100271466769346,0.0166015299239869),
 .UNSPECIFIED.);
#2975=B_SPLINE_SURFACE_WITH_KNOTS('',3,3,((#96215,#96216,#96217,#96218),
(#96219,#96220,#96221,#96222),(#96223,#96224,#96225,#96226),(#96227,#96228,
#96229,#96230)),.UNSPECIFIED.,.F.,.F.,.F.,(4,4),(4,4),(0.65323027149697,
1.00206901891073),(0.00656788395380929,0.0131849432428967),
 .UNSPECIFIED.);
#2976=B_SPLINE_SURFACE_WITH_KNOTS('',3,3,((#96238,#96239,#96240,#96241),
(#96242,#96243,#96244,#96245),(#96246,#96247,#96248,#96249),(#96250,#96251,
#96252,#96253)),.UNSPECIFIED.,.F.,.F.,.F.,(4,4),(4,4),(-0.0028678041047042,
0.477902879788517),(0.0200175229646909,0.0265907346180623),
 .UNSPECIFIED.);
#2977=B_SPLINE_SURFACE_WITH_KNOTS('',3,3,((#96255,#96256,#96257,#96258),
(#96259,#96260,#96261,#96262),(#96263,#96264,#96265,#96266),(#96267,#96268,
#96269,#96270)),.UNSPECIFIED.,.F.,.F.,.F.,(4,4),(4,4),(0.522097120196316,
1.00286753160137),(0.0166015299239891,0.0231736787930315),.UNSPECIFIED.);
#2978=B_SPLINE_SURFACE_WITH_KNOTS('',3,3,((#96272,#96273,#96274,#96275),
(#96276,#96277,#96278,#96279),(#96280,#96281,#96282,#96283),(#96284,#96285,
#96286,#96287)),.UNSPECIFIED.,.F.,.F.,.F.,(4,4),(4,4),(0.,1.00600003961326),
(0.016601529923986,0.0265907346180621),.UNSPECIFIED.);
#2979=B_SPLINE_SURFACE_WITH_KNOTS('',3,3,((#96288,#96289,#96290,#96291),
(#96292,#96293,#96294,#96295),(#96296,#96297,#96298,#96299),(#96300,#96301,
#96302,#96303)),.UNSPECIFIED.,.F.,.F.,.F.,(4,4),(4,4),(-0.002868622011607,
0.477902879790175),(0.0300094532292789,0.0365944846647016),
 .UNSPECIFIED.);
#2980=B_SPLINE_SURFACE_WITH_KNOTS('',3,3,((#96305,#96306,#96307,#96308),
(#96309,#96310,#96311,#96312),(#96313,#96314,#96315,#96316),(#96317,#96318,
#96319,#96320)),.UNSPECIFIED.,.F.,.F.,.F.,(4,4),(4,4),(0.522097120195324,
1.00286823669309),(0.0265907346180643,0.0331702036889928),.UNSPECIFIED.);
#2981=B_SPLINE_SURFACE_WITH_KNOTS('',3,3,((#96328,#96329,#96330,#96331),
(#96332,#96333,#96334,#96335),(#96336,#96337,#96338,#96339),(#96340,#96341,
#96342,#96343)),.UNSPECIFIED.,.F.,.F.,.F.,(4,4),(4,4),(-0.00286848453336819,
0.477902879788819),(0.0400218729466601,0.0466073985929425),
 .UNSPECIFIED.);
#2982=B_SPLINE_SURFACE_WITH_KNOTS('',3,3,((#96360,#96361,#96362,#96363),
(#96364,#96365,#96366,#96367),(#96368,#96369,#96370,#96371),(#96372,#96373,
#96374,#96375)),.UNSPECIFIED.,.F.,.F.,.F.,(4,4),(4,4),(0.,1.00600014639738),
(0.0365944846645024,0.0466073985929158),.UNSPECIFIED.);
#2983=B_SPLINE_SURFACE_WITH_KNOTS('',3,3,((#96376,#96377,#96378,#96379),
(#96380,#96381,#96382,#96383),(#96384,#96385,#96386,#96387),(#96388,#96389,
#96390,#96391)),.UNSPECIFIED.,.F.,.F.,.F.,(4,4),(4,4),(-0.00286780122472916,
0.477902879788083),(0.0500263550859002,0.0565997133101401),
 .UNSPECIFIED.);
#2984=B_SPLINE_SURFACE_WITH_KNOTS('',3,3,((#96393,#96394,#96395,#96396),
(#96397,#96398,#96399,#96400),(#96401,#96402,#96403,#96404),(#96405,#96406,
#96407,#96408)),.UNSPECIFIED.,.F.,.F.,.F.,(4,4),(4,4),(0.522097120193348,
1.0028681017726),(0.0466073985929442,0.0531834925888927),.UNSPECIFIED.);
#2985=B_SPLINE_SURFACE_WITH_KNOTS('',3,3,((#96416,#96417,#96418,#96419),
(#96420,#96421,#96422,#96423),(#96424,#96425,#96426,#96427),(#96428,#96429,
#96430,#96431)),.UNSPECIFIED.,.F.,.F.,.F.,(4,4),(4,4),(-0.00286792598894037,
0.477902879787975),(0.0600156865494599,0.0665898698871175),
 .UNSPECIFIED.);
#2986=B_SPLINE_SURFACE_WITH_KNOTS('',3,3,((#96433,#96434,#96435,#96436),
(#96437,#96438,#96439,#96440),(#96441,#96442,#96443,#96444),(#96445,#96446,
#96447,#96448)),.UNSPECIFIED.,.F.,.F.,.F.,(4,4),(4,4),(0.522097120194627,
1.00286764392052),(0.0565997133101422,0.0631721430887062),.UNSPECIFIED.);
#2987=B_SPLINE_SURFACE_WITH_KNOTS('',3,3,((#96464,#96465,#96466,#96467),
(#96468,#96469,#96470,#96471),(#96472,#96473,#96474,#96475),(#96476,#96477,
#96478,#96479)),.UNSPECIFIED.,.F.,.F.,.F.,(4,4),(4,4),(0.522097120191363,
1.00286833998609),(0.0665898698871185,0.0731716198748452),.UNSPECIFIED.);
#2988=B_SPLINE_SURFACE_WITH_KNOTS('',3,3,((#96480,#96481,#96482,#96483),
(#96484,#96485,#96486,#96487),(#96488,#96489,#96490,#96491),(#96492,#96493,
#96494,#96495)),.UNSPECIFIED.,.F.,.F.,.F.,(4,4),(4,4),(-0.00124731532115134,
0.209045111683166),(0.0700194292967135,0.0749900982977138),
 .UNSPECIFIED.);
#2989=B_SPLINE_SURFACE_WITH_KNOTS('',3,3,((#96502,#96503,#96504,#96505),
(#96506,#96507,#96508,#96509),(#96510,#96511,#96512,#96513),(#96514,#96515,
#96516,#96517)),.UNSPECIFIED.,.F.,.F.,.F.,(4,4),(4,4),(-0.00286791014476116,
0.477902879789011),(0.0100271466769342,0.0166015299239867),
 .UNSPECIFIED.);
#2990=B_SPLINE_SURFACE_WITH_KNOTS('',3,3,((#96519,#96520,#96521,#96522),
(#96523,#96524,#96525,#96526),(#96527,#96528,#96529,#96530),(#96531,#96532,
#96533,#96534)),.UNSPECIFIED.,.F.,.F.,.F.,(4,4),(4,4),(0.653230271498448,
1.00206901891297),(0.00656788395380222,0.013184943242988),.UNSPECIFIED.);
#2991=B_SPLINE_SURFACE_WITH_KNOTS('',3,3,((#96542,#96543,#96544,#96545),
(#96546,#96547,#96548,#96549),(#96550,#96551,#96552,#96553),(#96554,#96555,
#96556,#96557)),.UNSPECIFIED.,.F.,.F.,.F.,(4,4),(4,4),(-0.00286780410469616,
0.477902879788752),(0.0200175229646897,0.0265907346180627),
 .UNSPECIFIED.);
#2992=B_SPLINE_SURFACE_WITH_KNOTS('',3,3,((#96559,#96560,#96561,#96562),
(#96563,#96564,#96565,#96566),(#96567,#96568,#96569,#96570),(#96571,#96572,
#96573,#96574)),.UNSPECIFIED.,.F.,.F.,.F.,(4,4),(4,4),(0.522097120198486,
1.00286753160131),(0.0166015299239886,0.0231736788075218),.UNSPECIFIED.);
#2993=B_SPLINE_SURFACE_WITH_KNOTS('',3,3,((#96576,#96577,#96578,#96579),
(#96580,#96581,#96582,#96583),(#96584,#96585,#96586,#96587),(#96588,#96589,
#96590,#96591)),.UNSPECIFIED.,.F.,.F.,.F.,(4,4),(4,4),(0.,1.00600003961412),
(0.0166015299239884,0.0265907346180622),.UNSPECIFIED.);
#2994=B_SPLINE_SURFACE_WITH_KNOTS('',3,3,((#96592,#96593,#96594,#96595),
(#96596,#96597,#96598,#96599),(#96600,#96601,#96602,#96603),(#96604,#96605,
#96606,#96607)),.UNSPECIFIED.,.F.,.F.,.F.,(4,4),(4,4),(-0.00286862201157625,
0.477902879790364),(0.0300094532292792,0.0365944846647022),
 .UNSPECIFIED.);
#2995=B_SPLINE_SURFACE_WITH_KNOTS('',3,3,((#96609,#96610,#96611,#96612),
(#96613,#96614,#96615,#96616),(#96617,#96618,#96619,#96620),(#96621,#96622,
#96623,#96624)),.UNSPECIFIED.,.F.,.F.,.F.,(4,4),(4,4),(0.522097120197417,
1.0028682366931),(0.0265907346180633,0.0331702036889933),.UNSPECIFIED.);
#2996=B_SPLINE_SURFACE_WITH_KNOTS('',3,3,((#96632,#96633,#96634,#96635),
(#96636,#96637,#96638,#96639),(#96640,#96641,#96642,#96643),(#96644,#96645,
#96646,#96647)),.UNSPECIFIED.,.F.,.F.,.F.,(4,4),(4,4),(-0.00286848453359728,
0.477902879788827),(0.0400218729466586,0.0466073985929424),
 .UNSPECIFIED.);
#2997=B_SPLINE_SURFACE_WITH_KNOTS('',3,3,((#96664,#96665,#96666,#96667),
(#96668,#96669,#96670,#96671),(#96672,#96673,#96674,#96675),(#96676,#96677,
#96678,#96679)),.UNSPECIFIED.,.F.,.F.,.F.,(4,4),(4,4),(0.,1.00600014639725),
(0.0365944846645025,0.0466073985929155),.UNSPECIFIED.);
#2998=B_SPLINE_SURFACE_WITH_KNOTS('',3,3,((#96680,#96681,#96682,#96683),
(#96684,#96685,#96686,#96687),(#96688,#96689,#96690,#96691),(#96692,#96693,
#96694,#96695)),.UNSPECIFIED.,.F.,.F.,.F.,(4,4),(4,4),(-0.00286780122481621,
0.477902879788107),(0.0500263550858988,0.0565997133101405),
 .UNSPECIFIED.);
#2999=B_SPLINE_SURFACE_WITH_KNOTS('',3,3,((#96697,#96698,#96699,#96700),
(#96701,#96702,#96703,#96704),(#96705,#96706,#96707,#96708),(#96709,#96710,
#96711,#96712)),.UNSPECIFIED.,.F.,.F.,.F.,(4,4),(4,4),(0.5220971201952,
1.0028681017726),(0.0466073985929438,0.0531834925888936),.UNSPECIFIED.);
#3000=B_SPLINE_SURFACE_WITH_KNOTS('',3,3,((#96720,#96721,#96722,#96723),
(#96724,#96725,#96726,#96727),(#96728,#96729,#96730,#96731),(#96732,#96733,
#96734,#96735)),.UNSPECIFIED.,.F.,.F.,.F.,(4,4),(4,4),(-0.0028679259890384,
0.477902879788142),(0.0600156865494599,0.0665898698871172),
 .UNSPECIFIED.);
#3001=B_SPLINE_SURFACE_WITH_KNOTS('',3,3,((#96737,#96738,#96739,#96740),
(#96741,#96742,#96743,#96744),(#96745,#96746,#96747,#96748),(#96749,#96750,
#96751,#96752)),.UNSPECIFIED.,.F.,.F.,.F.,(4,4),(4,4),(0.522097120195508,
1.00286764392054),(0.0565997133101409,0.0631721430887068),.UNSPECIFIED.);
#3002=B_SPLINE_SURFACE_WITH_KNOTS('',3,3,((#96768,#96769,#96770,#96771),
(#96772,#96773,#96774,#96775),(#96776,#96777,#96778,#96779),(#96780,#96781,
#96782,#96783)),.UNSPECIFIED.,.F.,.F.,.F.,(4,4),(4,4),(0.52209712019312,
1.00286833998605),(0.066589869887118,0.0731716198748457),.UNSPECIFIED.);
#3003=B_SPLINE_SURFACE_WITH_KNOTS('',3,3,((#96784,#96785,#96786,#96787),
(#96788,#96789,#96790,#96791),(#96792,#96793,#96794,#96795),(#96796,#96797,
#96798,#96799)),.UNSPECIFIED.,.F.,.F.,.F.,(4,4),(4,4),(-0.0012473153211076,
0.209045111681666),(0.0700194292967032,0.0749900982977026),
 .UNSPECIFIED.);
#3004=B_SPLINE_SURFACE_WITH_KNOTS('',3,3,((#96806,#96807,#96808,#96809),
(#96810,#96811,#96812,#96813),(#96814,#96815,#96816,#96817),(#96818,#96819,
#96820,#96821)),.UNSPECIFIED.,.F.,.F.,.F.,(4,4),(4,4),(-0.00286791014473917,
0.477902879789097),(0.0100271466769336,0.0166015299239868),
 .UNSPECIFIED.);
#3005=B_SPLINE_SURFACE_WITH_KNOTS('',3,3,((#96823,#96824,#96825,#96826),
(#96827,#96828,#96829,#96830),(#96831,#96832,#96833,#96834),(#96835,#96836,
#96837,#96838)),.UNSPECIFIED.,.F.,.F.,.F.,(4,4),(4,4),(0.653230271499908,
1.00206901891551),(0.00656788395379813,0.0131849432429885),
 .UNSPECIFIED.);
#3006=B_SPLINE_SURFACE_WITH_KNOTS('',3,3,((#96846,#96847,#96848,#96849),
(#96850,#96851,#96852,#96853),(#96854,#96855,#96856,#96857),(#96858,#96859,
#96860,#96861)),.UNSPECIFIED.,.F.,.F.,.F.,(4,4),(4,4),(-0.00286780410476446,
0.477902879788805),(0.0200175229646903,0.0265907346180629),
 .UNSPECIFIED.);
#3007=B_SPLINE_SURFACE_WITH_KNOTS('',3,3,((#96863,#96864,#96865,#96866),
(#96867,#96868,#96869,#96870),(#96871,#96872,#96873,#96874),(#96875,#96876,
#96877,#96878)),.UNSPECIFIED.,.F.,.F.,.F.,(4,4),(4,4),(0.522097120200814,
1.00286753160131),(0.0166015299239891,0.0231736787930312),.UNSPECIFIED.);
#3008=B_SPLINE_SURFACE_WITH_KNOTS('',3,3,((#96880,#96881,#96882,#96883),
(#96884,#96885,#96886,#96887),(#96888,#96889,#96890,#96891),(#96892,#96893,
#96894,#96895)),.UNSPECIFIED.,.F.,.F.,.F.,(4,4),(4,4),(0.,1.00600003961374),
(0.0166015299239868,0.0265907346180621),.UNSPECIFIED.);
#3009=B_SPLINE_SURFACE_WITH_KNOTS('',3,3,((#96896,#96897,#96898,#96899),
(#96900,#96901,#96902,#96903),(#96904,#96905,#96906,#96907),(#96908,#96909,
#96910,#96911)),.UNSPECIFIED.,.F.,.F.,.F.,(4,4),(4,4),(-0.00286862201174504,
0.477902879790358),(0.0300094532292793,0.0365944846647016),
 .UNSPECIFIED.);
#3010=B_SPLINE_SURFACE_WITH_KNOTS('',3,3,((#96913,#96914,#96915,#96916),
(#96917,#96918,#96919,#96920),(#96921,#96922,#96923,#96924),(#96925,#96926,
#96927,#96928)),.UNSPECIFIED.,.F.,.F.,.F.,(4,4),(4,4),(0.522097120199715,
1.00286823669304),(0.0265907346180626,0.0331702036889934),.UNSPECIFIED.);
#3011=B_SPLINE_SURFACE_WITH_KNOTS('',3,3,((#96936,#96937,#96938,#96939),
(#96940,#96941,#96942,#96943),(#96944,#96945,#96946,#96947),(#96948,#96949,
#96950,#96951)),.UNSPECIFIED.,.F.,.F.,.F.,(4,4),(4,4),(-0.00286848453345688,
0.477902879788998),(0.0400218729466602,0.0466073985929435),
 .UNSPECIFIED.);
#3012=B_SPLINE_SURFACE_WITH_KNOTS('',3,3,((#96968,#96969,#96970,#96971),
(#96972,#96973,#96974,#96975),(#96976,#96977,#96978,#96979),(#96980,#96981,
#96982,#96983)),.UNSPECIFIED.,.F.,.F.,.F.,(4,4),(4,4),(0.,1.0060001463976),
(0.0365944846645024,0.0466073985929158),.UNSPECIFIED.);
#3013=B_SPLINE_SURFACE_WITH_KNOTS('',3,3,((#96984,#96985,#96986,#96987),
(#96988,#96989,#96990,#96991),(#96992,#96993,#96994,#96995),(#96996,#96997,
#96998,#96999)),.UNSPECIFIED.,.F.,.F.,.F.,(4,4),(4,4),(-0.00286780122472176,
0.47790287978859),(0.0500263550858996,0.0565997133101399),.UNSPECIFIED.);
#3014=B_SPLINE_SURFACE_WITH_KNOTS('',3,3,((#97001,#97002,#97003,#97004),
(#97005,#97006,#97007,#97008),(#97009,#97010,#97011,#97012),(#97013,#97014,
#97015,#97016)),.UNSPECIFIED.,.F.,.F.,.F.,(4,4),(4,4),(0.522097120197378,
1.00286810177282),(0.0466073985929436,0.0531834933545503),.UNSPECIFIED.);
#3015=B_SPLINE_SURFACE_WITH_KNOTS('',3,3,((#97024,#97025,#97026,#97027),
(#97028,#97029,#97030,#97031),(#97032,#97033,#97034,#97035),(#97036,#97037,
#97038,#97039)),.UNSPECIFIED.,.F.,.F.,.F.,(4,4),(4,4),(-0.00286792598899008,
0.477902879788161),(0.0600156865494598,0.0665898698871171),
 .UNSPECIFIED.);
#3016=B_SPLINE_SURFACE_WITH_KNOTS('',3,3,((#97041,#97042,#97043,#97044),
(#97045,#97046,#97047,#97048),(#97049,#97050,#97051,#97052),(#97053,#97054,
#97055,#97056)),.UNSPECIFIED.,.F.,.F.,.F.,(4,4),(4,4),(0.522097120196579,
1.00286764392047),(0.056599713310142,0.0631721430887062),.UNSPECIFIED.);
#3017=B_SPLINE_SURFACE_WITH_KNOTS('',3,3,((#97072,#97073,#97074,#97075),
(#97076,#97077,#97078,#97079),(#97080,#97081,#97082,#97083),(#97084,#97085,
#97086,#97087)),.UNSPECIFIED.,.F.,.F.,.F.,(4,4),(4,4),(0.522097120195032,
1.00286833998602),(0.0665898698871187,0.0731716198748464),.UNSPECIFIED.);
#3018=B_SPLINE_SURFACE_WITH_KNOTS('',3,3,((#97088,#97089,#97090,#97091),
(#97092,#97093,#97094,#97095),(#97096,#97097,#97098,#97099),(#97100,#97101,
#97102,#97103)),.UNSPECIFIED.,.F.,.F.,.F.,(4,4),(4,4),(-0.00124731532104556,
0.209045111680193),(0.0700194292966934,0.0749900982976918),
 .UNSPECIFIED.);
#3019=B_SPLINE_SURFACE_WITH_KNOTS('',3,3,((#97110,#97111,#97112,#97113),
(#97114,#97115,#97116,#97117),(#97118,#97119,#97120,#97121),(#97122,#97123,
#97124,#97125)),.UNSPECIFIED.,.F.,.F.,.F.,(4,4),(4,4),(-0.00286791014469159,
0.477902879789153),(0.0100271466769335,0.0166015299239866),
 .UNSPECIFIED.);
#3020=B_SPLINE_SURFACE_WITH_KNOTS('',3,3,((#97127,#97128,#97129,#97130),
(#97131,#97132,#97133,#97134),(#97135,#97136,#97137,#97138),(#97139,#97140,
#97141,#97142)),.UNSPECIFIED.,.F.,.F.,.F.,(4,4),(4,4),(0.65323027150149,
1.00206901891795),(0.0065678839537943,0.0131849432429871),.UNSPECIFIED.);
#3021=B_SPLINE_SURFACE_WITH_KNOTS('',3,3,((#97150,#97151,#97152,#97153),
(#97154,#97155,#97156,#97157),(#97158,#97159,#97160,#97161),(#97162,#97163,
#97164,#97165)),.UNSPECIFIED.,.F.,.F.,.F.,(4,4),(4,4),(-0.00286780410462738,
0.477902879788914),(0.0200175229646893,0.0265907346180623),
 .UNSPECIFIED.);
#3022=B_SPLINE_SURFACE_WITH_KNOTS('',3,3,((#97167,#97168,#97169,#97170),
(#97171,#97172,#97173,#97174),(#97175,#97176,#97177,#97178),(#97179,#97180,
#97181,#97182)),.UNSPECIFIED.,.F.,.F.,.F.,(4,4),(4,4),(0.522097120203192,
1.00286753160128),(0.0166015299239873,0.0231736788075223),.UNSPECIFIED.);
#3023=B_SPLINE_SURFACE_WITH_KNOTS('',3,3,((#97184,#97185,#97186,#97187),
(#97188,#97189,#97190,#97191),(#97192,#97193,#97194,#97195),(#97196,#97197,
#97198,#97199)),.UNSPECIFIED.,.F.,.F.,.F.,(4,4),(4,4),(0.,1.00600003961393),
(0.0166015299239881,0.0265907346180636),.UNSPECIFIED.);
#3024=B_SPLINE_SURFACE_WITH_KNOTS('',3,3,((#97200,#97201,#97202,#97203),
(#97204,#97205,#97206,#97207),(#97208,#97209,#97210,#97211),(#97212,#97213,
#97214,#97215)),.UNSPECIFIED.,.F.,.F.,.F.,(4,4),(4,4),(-0.00286862201168659,
0.477902879790677),(0.0300094532292788,0.0365944846647015),
 .UNSPECIFIED.);
#3025=B_SPLINE_SURFACE_WITH_KNOTS('',3,3,((#97217,#97218,#97219,#97220),
(#97221,#97222,#97223,#97224),(#97225,#97226,#97227,#97228),(#97229,#97230,
#97231,#97232)),.UNSPECIFIED.,.F.,.F.,.F.,(4,4),(4,4),(0.522097120202095,
1.00286823669305),(0.0265907346180628,0.0331702036889925),.UNSPECIFIED.);
#3026=B_SPLINE_SURFACE_WITH_KNOTS('',3,3,((#97240,#97241,#97242,#97243),
(#97244,#97245,#97246,#97247),(#97248,#97249,#97250,#97251),(#97252,#97253,
#97254,#97255)),.UNSPECIFIED.,.F.,.F.,.F.,(4,4),(4,4),(-0.00286848453351476,
0.47790287978917),(0.0400218729466592,0.0466073985929419),.UNSPECIFIED.);
#3027=B_SPLINE_SURFACE_WITH_KNOTS('',3,3,((#97272,#97273,#97274,#97275),
(#97276,#97277,#97278,#97279),(#97280,#97281,#97282,#97283),(#97284,#97285,
#97286,#97287)),.UNSPECIFIED.,.F.,.F.,.F.,(4,4),(4,4),(0.,1.00600014639755),
(0.0365944846645033,0.0466073985929164),.UNSPECIFIED.);
#3028=B_SPLINE_SURFACE_WITH_KNOTS('',3,3,((#97288,#97289,#97290,#97291),
(#97292,#97293,#97294,#97295),(#97296,#97297,#97298,#97299),(#97300,#97301,
#97302,#97303)),.UNSPECIFIED.,.F.,.F.,.F.,(4,4),(4,4),(-0.00286780122478771,
0.477902879788463),(0.0500263550858998,0.0565997133101397),
 .UNSPECIFIED.);
#3029=B_SPLINE_SURFACE_WITH_KNOTS('',3,3,((#97305,#97306,#97307,#97308),
(#97309,#97310,#97311,#97312),(#97313,#97314,#97315,#97316),(#97317,#97318,
#97319,#97320)),.UNSPECIFIED.,.F.,.F.,.F.,(4,4),(4,4),(0.522097120199638,
1.00286810177254),(0.0466073985929435,0.0531834925888921),.UNSPECIFIED.);
#3030=B_SPLINE_SURFACE_WITH_KNOTS('',3,3,((#97328,#97329,#97330,#97331),
(#97332,#97333,#97334,#97335),(#97336,#97337,#97338,#97339),(#97340,#97341,
#97342,#97343)),.UNSPECIFIED.,.F.,.F.,.F.,(4,4),(4,4),(-0.00286792598894184,
0.477902879788324),(0.0600156865494592,0.0665898698871167),
 .UNSPECIFIED.);
#3031=B_SPLINE_SURFACE_WITH_KNOTS('',3,3,((#97345,#97346,#97347,#97348),
(#97349,#97350,#97351,#97352),(#97353,#97354,#97355,#97356),(#97357,#97358,
#97359,#97360)),.UNSPECIFIED.,.F.,.F.,.F.,(4,4),(4,4),(0.522097120198475,
1.0028676439205),(0.0565997133101411,0.0631721430887063),.UNSPECIFIED.);
#3032=B_SPLINE_SURFACE_WITH_KNOTS('',3,3,((#97376,#97377,#97378,#97379),
(#97380,#97381,#97382,#97383),(#97384,#97385,#97386,#97387),(#97388,#97389,
#97390,#97391)),.UNSPECIFIED.,.F.,.F.,.F.,(4,4),(4,4),(0.522097120197217,
1.00286833998599),(0.0665898698871181,0.0731716198748449),.UNSPECIFIED.);
#3033=B_SPLINE_SURFACE_WITH_KNOTS('',3,3,((#97392,#97393,#97394,#97395),
(#97396,#97397,#97398,#97399),(#97400,#97401,#97402,#97403),(#97404,#97405,
#97406,#97407)),.UNSPECIFIED.,.F.,.F.,.F.,(4,4),(4,4),(-0.00124731532105012,
0.209045111678836),(0.0700194292966838,0.0749900982976822),
 .UNSPECIFIED.);
#3034=B_SPLINE_SURFACE_WITH_KNOTS('',3,3,((#97414,#97415,#97416,#97417),
(#97418,#97419,#97420,#97421),(#97422,#97423,#97424,#97425),(#97426,#97427,
#97428,#97429)),.UNSPECIFIED.,.F.,.F.,.F.,(4,4),(4,4),(-0.0028679101447297,
0.477902879789159),(0.0100271466769351,0.0166015299239871),
 .UNSPECIFIED.);
#3035=B_SPLINE_SURFACE_WITH_KNOTS('',3,3,((#97431,#97432,#97433,#97434),
(#97435,#97436,#97437,#97438),(#97439,#97440,#97441,#97442),(#97443,#97444,
#97445,#97446)),.UNSPECIFIED.,.F.,.F.,.F.,(4,4),(4,4),(0.653230271502837,
1.00206901892052),(0.00656788395379318,0.0131849432429889),
 .UNSPECIFIED.);
#3036=B_SPLINE_SURFACE_WITH_KNOTS('',3,3,((#97454,#97455,#97456,#97457),
(#97458,#97459,#97460,#97461),(#97462,#97463,#97464,#97465),(#97466,#97467,
#97468,#97469)),.UNSPECIFIED.,.F.,.F.,.F.,(4,4),(4,4),(-0.00286780410467987,
0.477902879789059),(0.0200175229646905,0.0265907346180626),
 .UNSPECIFIED.);
#3037=B_SPLINE_SURFACE_WITH_KNOTS('',3,3,((#97471,#97472,#97473,#97474),
(#97475,#97476,#97477,#97478),(#97479,#97480,#97481,#97482),(#97483,#97484,
#97485,#97486)),.UNSPECIFIED.,.F.,.F.,.F.,(4,4),(4,4),(0.522097120205828,
1.00286753160122),(0.016601529923988,0.0231736788075224),.UNSPECIFIED.);
#3038=B_SPLINE_SURFACE_WITH_KNOTS('',3,3,((#97488,#97489,#97490,#97491),
(#97492,#97493,#97494,#97495),(#97496,#97497,#97498,#97499),(#97500,#97501,
#97502,#97503)),.UNSPECIFIED.,.F.,.F.,.F.,(4,4),(4,4),(0.,1.00600003961379),
(0.016601529923988,0.0265907346180635),.UNSPECIFIED.);
#3039=B_SPLINE_SURFACE_WITH_KNOTS('',3,3,((#97504,#97505,#97506,#97507),
(#97508,#97509,#97510,#97511),(#97512,#97513,#97514,#97515),(#97516,#97517,
#97518,#97519)),.UNSPECIFIED.,.F.,.F.,.F.,(4,4),(4,4),(-0.00286862201166983,
0.477902879790738),(0.0300094532292793,0.0365944846647023),
 .UNSPECIFIED.);
#3040=B_SPLINE_SURFACE_WITH_KNOTS('',3,3,((#97521,#97522,#97523,#97524),
(#97525,#97526,#97527,#97528),(#97529,#97530,#97531,#97532),(#97533,#97534,
#97535,#97536)),.UNSPECIFIED.,.F.,.F.,.F.,(4,4),(4,4),(0.522097120204583,
1.00286823669297),(0.0265907346180627,0.0331702036051738),.UNSPECIFIED.);
#3041=B_SPLINE_SURFACE_WITH_KNOTS('',3,3,((#97544,#97545,#97546,#97547),
(#97548,#97549,#97550,#97551),(#97552,#97553,#97554,#97555),(#97556,#97557,
#97558,#97559)),.UNSPECIFIED.,.F.,.F.,.F.,(4,4),(4,4),(-0.0028684845334923,
0.477902879789434),(0.04002187294666,0.0466073985929439),.UNSPECIFIED.);
#3042=B_SPLINE_SURFACE_WITH_KNOTS('',3,3,((#97576,#97577,#97578,#97579),
(#97580,#97581,#97582,#97583),(#97584,#97585,#97586,#97587),(#97588,#97589,
#97590,#97591)),.UNSPECIFIED.,.F.,.F.,.F.,(4,4),(4,4),(0.,1.00600014639746),
(0.0365944846645047,0.0466073985929165),.UNSPECIFIED.);
#3043=B_SPLINE_SURFACE_WITH_KNOTS('',3,3,((#97592,#97593,#97594,#97595),
(#97596,#97597,#97598,#97599),(#97600,#97601,#97602,#97603),(#97604,#97605,
#97606,#97607)),.UNSPECIFIED.,.F.,.F.,.F.,(4,4),(4,4),(-0.00286780122482743,
0.477902879788715),(0.0500263550859003,0.0565997133101399),
 .UNSPECIFIED.);
#3044=B_SPLINE_SURFACE_WITH_KNOTS('',3,3,((#97609,#97610,#97611,#97612),
(#97613,#97614,#97615,#97616),(#97617,#97618,#97619,#97620),(#97621,#97622,
#97623,#97624)),.UNSPECIFIED.,.F.,.F.,.F.,(4,4),(4,4),(0.522097120202103,
1.00286810177252),(0.0466073985929445,0.0531834925888931),.UNSPECIFIED.);
#3045=B_SPLINE_SURFACE_WITH_KNOTS('',3,3,((#97632,#97633,#97634,#97635),
(#97636,#97637,#97638,#97639),(#97640,#97641,#97642,#97643),(#97644,#97645,
#97646,#97647)),.UNSPECIFIED.,.F.,.F.,.F.,(4,4),(4,4),(-0.00286792598910059,
0.477902879788515),(0.0600156865494612,0.0665898698871175),
 .UNSPECIFIED.);
#3046=B_SPLINE_SURFACE_WITH_KNOTS('',3,3,((#97649,#97650,#97651,#97652),
(#97653,#97654,#97655,#97656),(#97657,#97658,#97659,#97660),(#97661,#97662,
#97663,#97664)),.UNSPECIFIED.,.F.,.F.,.F.,(4,4),(4,4),(0.522097120200887,
1.0028676439205),(0.0565997133101418,0.0631721430887064),.UNSPECIFIED.);
#3047=B_SPLINE_SURFACE_WITH_KNOTS('',3,3,((#97680,#97681,#97682,#97683),
(#97684,#97685,#97686,#97687),(#97688,#97689,#97690,#97691),(#97692,#97693,
#97694,#97695)),.UNSPECIFIED.,.F.,.F.,.F.,(4,4),(4,4),(0.522097120199466,
1.00286833998596),(0.0665898698871184,0.0731716198748447),.UNSPECIFIED.);
#3048=B_SPLINE_SURFACE_WITH_KNOTS('',3,3,((#97696,#97697,#97698,#97699),
(#97700,#97701,#97702,#97703),(#97704,#97705,#97706,#97707),(#97708,#97709,
#97710,#97711)),.UNSPECIFIED.,.F.,.F.,.F.,(4,4),(4,4),(-0.0012473153211035,
0.2090451116773),(0.0700194292966747,0.0749900982976723),.UNSPECIFIED.);
#3049=B_SPLINE_SURFACE_WITH_KNOTS('',3,3,((#97718,#97719,#97720,#97721),
(#97722,#97723,#97724,#97725),(#97726,#97727,#97728,#97729),(#97730,#97731,
#97732,#97733)),.UNSPECIFIED.,.F.,.F.,.F.,(4,4),(4,4),(-0.00286791014464772,
0.477902879789483),(0.0100271466769355,0.0166015299239867),
 .UNSPECIFIED.);
#3050=B_SPLINE_SURFACE_WITH_KNOTS('',3,3,((#97735,#97736,#97737,#97738),
(#97739,#97740,#97741,#97742),(#97743,#97744,#97745,#97746),(#97747,#97748,
#97749,#97750)),.UNSPECIFIED.,.F.,.F.,.F.,(4,4),(4,4),(0.653230271504001,
1.00206901892309),(0.00656788395379142,0.0131849432429884),
 .UNSPECIFIED.);
#3051=B_SPLINE_SURFACE_WITH_KNOTS('',3,3,((#97758,#97759,#97760,#97761),
(#97762,#97763,#97764,#97765),(#97766,#97767,#97768,#97769),(#97770,#97771,
#97772,#97773)),.UNSPECIFIED.,.F.,.F.,.F.,(4,4),(4,4),(-0.00286780410480499,
0.477902879789146),(0.0200175229646898,0.0265907346180605),
 .UNSPECIFIED.);
#3052=B_SPLINE_SURFACE_WITH_KNOTS('',3,3,((#97775,#97776,#97777,#97778),
(#97779,#97780,#97781,#97782),(#97783,#97784,#97785,#97786),(#97787,#97788,
#97789,#97790)),.UNSPECIFIED.,.F.,.F.,.F.,(4,4),(4,4),(0.522097120208367,
1.0028675316012),(0.016601529923988,0.023173678807522),.UNSPECIFIED.);
#3053=B_SPLINE_SURFACE_WITH_KNOTS('',3,3,((#97792,#97793,#97794,#97795),
(#97796,#97797,#97798,#97799),(#97800,#97801,#97802,#97803),(#97804,#97805,
#97806,#97807)),.UNSPECIFIED.,.F.,.F.,.F.,(4,4),(4,4),(0.,1.0060000396137),
(0.016601529923988,0.0265907346180622),.UNSPECIFIED.);
#3054=B_SPLINE_SURFACE_WITH_KNOTS('',3,3,((#97808,#97809,#97810,#97811),
(#97812,#97813,#97814,#97815),(#97816,#97817,#97818,#97819),(#97820,#97821,
#97822,#97823)),.UNSPECIFIED.,.F.,.F.,.F.,(4,4),(4,4),(-0.00286862201158081,
0.47790287979081),(0.0300094532292784,0.0365944846647014),.UNSPECIFIED.);
#3055=B_SPLINE_SURFACE_WITH_KNOTS('',3,3,((#97825,#97826,#97827,#97828),
(#97829,#97830,#97831,#97832),(#97833,#97834,#97835,#97836),(#97837,#97838,
#97839,#97840)),.UNSPECIFIED.,.F.,.F.,.F.,(4,4),(4,4),(0.522097120207176,
1.00286823669295),(0.026590734618063,0.033170203688992),.UNSPECIFIED.);
#3056=B_SPLINE_SURFACE_WITH_KNOTS('',3,3,((#97848,#97849,#97850,#97851),
(#97852,#97853,#97854,#97855),(#97856,#97857,#97858,#97859),(#97860,#97861,
#97862,#97863)),.UNSPECIFIED.,.F.,.F.,.F.,(4,4),(4,4),(-0.00286848453347558,
0.477902879789301),(0.0400218729466597,0.0466073985929426),
 .UNSPECIFIED.);
#3057=B_SPLINE_SURFACE_WITH_KNOTS('',3,3,((#97880,#97881,#97882,#97883),
(#97884,#97885,#97886,#97887),(#97888,#97889,#97890,#97891),(#97892,#97893,
#97894,#97895)),.UNSPECIFIED.,.F.,.F.,.F.,(4,4),(4,4),(0.,1.00600014639744),
(0.0365944846645046,0.0466073985929167),.UNSPECIFIED.);
#3058=B_SPLINE_SURFACE_WITH_KNOTS('',3,3,((#97896,#97897,#97898,#97899),
(#97900,#97901,#97902,#97903),(#97904,#97905,#97906,#97907),(#97908,#97909,
#97910,#97911)),.UNSPECIFIED.,.F.,.F.,.F.,(4,4),(4,4),(-0.00286780122479574,
0.477902879788766),(0.0500263550859,0.0565997133101406),.UNSPECIFIED.);
#3059=B_SPLINE_SURFACE_WITH_KNOTS('',3,3,((#97913,#97914,#97915,#97916),
(#97917,#97918,#97919,#97920),(#97921,#97922,#97923,#97924),(#97925,#97926,
#97927,#97928)),.UNSPECIFIED.,.F.,.F.,.F.,(4,4),(4,4),(0.522097120204506,
1.00286810177246),(0.0466073985929448,0.0531834925888934),.UNSPECIFIED.);
#3060=B_SPLINE_SURFACE_WITH_KNOTS('',3,3,((#97936,#97937,#97938,#97939),
(#97940,#97941,#97942,#97943),(#97944,#97945,#97946,#97947),(#97948,#97949,
#97950,#97951)),.UNSPECIFIED.,.F.,.F.,.F.,(4,4),(4,4),(-0.00286792598892555,
0.477902879788712),(0.0600156865494599,0.0665898698871178),
 .UNSPECIFIED.);
#3061=B_SPLINE_SURFACE_WITH_KNOTS('',3,3,((#97953,#97954,#97955,#97956),
(#97957,#97958,#97959,#97960),(#97961,#97962,#97963,#97964),(#97965,#97966,
#97967,#97968)),.UNSPECIFIED.,.F.,.F.,.F.,(4,4),(4,4),(0.522097120203374,
1.00286764392044),(0.0565997133101419,0.0631721430887051),.UNSPECIFIED.);
#3062=B_SPLINE_SURFACE_WITH_KNOTS('',3,3,((#97984,#97985,#97986,#97987),
(#97988,#97989,#97990,#97991),(#97992,#97993,#97994,#97995),(#97996,#97997,
#97998,#97999)),.UNSPECIFIED.,.F.,.F.,.F.,(4,4),(4,4),(0.522097120201856,
1.00286833998603),(0.0665898698871177,0.0731716198748464),.UNSPECIFIED.);
#3063=B_SPLINE_SURFACE_WITH_KNOTS('',3,3,((#98000,#98001,#98002,#98003),
(#98004,#98005,#98006,#98007),(#98008,#98009,#98010,#98011),(#98012,#98013,
#98014,#98015)),.UNSPECIFIED.,.F.,.F.,.F.,(4,4),(4,4),(-0.00124731532103314,
0.209045111675863),(0.0700194292966633,0.074990098297664),.UNSPECIFIED.);
#3064=B_SPLINE_SURFACE_WITH_KNOTS('',3,3,((#98022,#98023,#98024,#98025),
(#98026,#98027,#98028,#98029),(#98030,#98031,#98032,#98033),(#98034,#98035,
#98036,#98037)),.UNSPECIFIED.,.F.,.F.,.F.,(4,4),(4,4),(-0.00286791014461308,
0.477902879789457),(0.0100271466769381,0.0166015299239867),
 .UNSPECIFIED.);
#3065=B_SPLINE_SURFACE_WITH_KNOTS('',3,3,((#98039,#98040,#98041,#98042),
(#98043,#98044,#98045,#98046),(#98047,#98048,#98049,#98050),(#98051,#98052,
#98053,#98054)),.UNSPECIFIED.,.F.,.F.,.F.,(4,4),(4,4),(0.653230271507036,
1.00206901892555),(0.00656788395397564,0.0131849432121935),
 .UNSPECIFIED.);
#3066=B_SPLINE_SURFACE_WITH_KNOTS('',3,3,((#98062,#98063,#98064,#98065),
(#98066,#98067,#98068,#98069),(#98070,#98071,#98072,#98073),(#98074,#98075,
#98076,#98077)),.UNSPECIFIED.,.F.,.F.,.F.,(4,4),(4,4),(-0.00286780410475934,
0.477902879789225),(0.02001752296469,0.026590734618062),.UNSPECIFIED.);
#3067=B_SPLINE_SURFACE_WITH_KNOTS('',3,3,((#98079,#98080,#98081,#98082),
(#98083,#98084,#98085,#98086),(#98087,#98088,#98089,#98090),(#98091,#98092,
#98093,#98094)),.UNSPECIFIED.,.F.,.F.,.F.,(4,4),(4,4),(0.522097120210828,
1.00286753160118),(0.0166015299239881,0.0231736788075221),.UNSPECIFIED.);
#3068=B_SPLINE_SURFACE_WITH_KNOTS('',3,3,((#98096,#98097,#98098,#98099),
(#98100,#98101,#98102,#98103),(#98104,#98105,#98106,#98107),(#98108,#98109,
#98110,#98111)),.UNSPECIFIED.,.F.,.F.,.F.,(4,4),(4,4),(0.,1.00600003961384),
(0.016601529923988,0.0265907346180622),.UNSPECIFIED.);
#3069=B_SPLINE_SURFACE_WITH_KNOTS('',3,3,((#98112,#98113,#98114,#98115),
(#98116,#98117,#98118,#98119),(#98120,#98121,#98122,#98123),(#98124,#98125,
#98126,#98127)),.UNSPECIFIED.,.F.,.F.,.F.,(4,4),(4,4),(-0.00286862201159159,
0.477902879791095),(0.0300094532292787,0.0365944846647163),
 .UNSPECIFIED.);
#3070=B_SPLINE_SURFACE_WITH_KNOTS('',3,3,((#98129,#98130,#98131,#98132),
(#98133,#98134,#98135,#98136),(#98137,#98138,#98139,#98140),(#98141,#98142,
#98143,#98144)),.UNSPECIFIED.,.F.,.F.,.F.,(4,4),(4,4),(0.522097120209687,
1.00286823669294),(0.0265907346180634,0.0331702036889921),.UNSPECIFIED.);
#3071=B_SPLINE_SURFACE_WITH_KNOTS('',3,3,((#98152,#98153,#98154,#98155),
(#98156,#98157,#98158,#98159),(#98160,#98161,#98162,#98163),(#98164,#98165,
#98166,#98167)),.UNSPECIFIED.,.F.,.F.,.F.,(4,4),(4,4),(-0.0028684845334302,
0.477902879789558),(0.0400218729466606,0.0466073985929422),
 .UNSPECIFIED.);
#3072=B_SPLINE_SURFACE_WITH_KNOTS('',3,3,((#98184,#98185,#98186,#98187),
(#98188,#98189,#98190,#98191),(#98192,#98193,#98194,#98195),(#98196,#98197,
#98198,#98199)),.UNSPECIFIED.,.F.,.F.,.F.,(4,4),(4,4),(0.,1.00600014639751),
(0.0365944846645049,0.0466073985929156),.UNSPECIFIED.);
#3073=B_SPLINE_SURFACE_WITH_KNOTS('',3,3,((#98200,#98201,#98202,#98203),
(#98204,#98205,#98206,#98207),(#98208,#98209,#98210,#98211),(#98212,#98213,
#98214,#98215)),.UNSPECIFIED.,.F.,.F.,.F.,(4,4),(4,4),(-0.00286780122473538,
0.477902879789028),(0.0500263550859005,0.0565997133101408),
 .UNSPECIFIED.);
#3074=B_SPLINE_SURFACE_WITH_KNOTS('',3,3,((#98217,#98218,#98219,#98220),
(#98221,#98222,#98223,#98224),(#98225,#98226,#98227,#98228),(#98229,#98230,
#98231,#98232)),.UNSPECIFIED.,.F.,.F.,.F.,(4,4),(4,4),(0.522097120207056,
1.00286810177249),(0.0466073985929443,0.0531834925888928),.UNSPECIFIED.);
#3075=B_SPLINE_SURFACE_WITH_KNOTS('',3,3,((#98240,#98241,#98242,#98243),
(#98244,#98245,#98246,#98247),(#98248,#98249,#98250,#98251),(#98252,#98253,
#98254,#98255)),.UNSPECIFIED.,.F.,.F.,.F.,(4,4),(4,4),(-0.00286792598897873,
0.47790287978871),(0.0600156865494609,0.0665898698871172),.UNSPECIFIED.);
#3076=B_SPLINE_SURFACE_WITH_KNOTS('',3,3,((#98257,#98258,#98259,#98260),
(#98261,#98262,#98263,#98264),(#98265,#98266,#98267,#98268),(#98269,#98270,
#98271,#98272)),.UNSPECIFIED.,.F.,.F.,.F.,(4,4),(4,4),(0.522097120205968,
1.00286764392047),(0.0565997133101421,0.0631721430887068),.UNSPECIFIED.);
#3077=B_SPLINE_SURFACE_WITH_KNOTS('',3,3,((#98288,#98289,#98290,#98291),
(#98292,#98293,#98294,#98295),(#98296,#98297,#98298,#98299),(#98300,#98301,
#98302,#98303)),.UNSPECIFIED.,.F.,.F.,.F.,(4,4),(4,4),(0.522097120204424,
1.00286833998594),(0.0665898698871185,0.073171619874845),.UNSPECIFIED.);
#3078=B_SPLINE_SURFACE_WITH_KNOTS('',3,3,((#98304,#98305,#98306,#98307),
(#98308,#98309,#98310,#98311),(#98312,#98313,#98314,#98315),(#98316,#98317,
#98318,#98319)),.UNSPECIFIED.,.F.,.F.,.F.,(4,4),(4,4),(-0.00124731532105512,
0.209045111674549),(0.0700194292966487,0.074990098297657),.UNSPECIFIED.);
#3079=B_SPLINE_SURFACE_WITH_KNOTS('',3,3,((#98326,#98327,#98328,#98329),
(#98330,#98331,#98332,#98333),(#98334,#98335,#98336,#98337),(#98338,#98339,
#98340,#98341)),.UNSPECIFIED.,.F.,.F.,.F.,(4,4),(4,4),(-0.00286791014458099,
0.477902879789525),(0.0100271466769368,0.0166015299239868),
 .UNSPECIFIED.);
#3080=B_SPLINE_SURFACE_WITH_KNOTS('',3,3,((#98343,#98344,#98345,#98346),
(#98347,#98348,#98349,#98350),(#98351,#98352,#98353,#98354),(#98355,#98356,
#98357,#98358)),.UNSPECIFIED.,.F.,.F.,.F.,(4,4),(4,4),(0.653230271506329,
1.00206901892807),(0.00656788395397555,0.0131849432122001),
 .UNSPECIFIED.);
#3081=B_SPLINE_SURFACE_WITH_KNOTS('',3,3,((#98366,#98367,#98368,#98369),
(#98370,#98371,#98372,#98373),(#98374,#98375,#98376,#98377),(#98378,#98379,
#98380,#98381)),.UNSPECIFIED.,.F.,.F.,.F.,(4,4),(4,4),(-0.00286780410469745,
0.477902879789348),(0.0200175229646915,0.026590734618063),.UNSPECIFIED.);
#3082=B_SPLINE_SURFACE_WITH_KNOTS('',3,3,((#98383,#98384,#98385,#98386),
(#98387,#98388,#98389,#98390),(#98391,#98392,#98393,#98394),(#98395,#98396,
#98397,#98398)),.UNSPECIFIED.,.F.,.F.,.F.,(4,4),(4,4),(0.522097120210687,
1.00286753160123),(0.016601529923989,0.023173678793031),.UNSPECIFIED.);
#3083=B_SPLINE_SURFACE_WITH_KNOTS('',3,3,((#98400,#98401,#98402,#98403),
(#98404,#98405,#98406,#98407),(#98408,#98409,#98410,#98411),(#98412,#98413,
#98414,#98415)),.UNSPECIFIED.,.F.,.F.,.F.,(4,4),(4,4),(0.,1.00600003961384),
(0.0166015299239892,0.0265907346180636),.UNSPECIFIED.);
#3084=B_SPLINE_SURFACE_WITH_KNOTS('',3,3,((#98416,#98417,#98418,#98419),
(#98420,#98421,#98422,#98423),(#98424,#98425,#98426,#98427),(#98428,#98429,
#98430,#98431)),.UNSPECIFIED.,.F.,.F.,.F.,(4,4),(4,4),(-0.00286862201150934,
0.477902879791048),(0.0300094532292786,0.0365944846647024),
 .UNSPECIFIED.);
#3085=B_SPLINE_SURFACE_WITH_KNOTS('',3,3,((#98433,#98434,#98435,#98436),
(#98437,#98438,#98439,#98440),(#98441,#98442,#98443,#98444),(#98445,#98446,
#98447,#98448)),.UNSPECIFIED.,.F.,.F.,.F.,(4,4),(4,4),(0.522097120210921,
1.00286823669297),(0.0265907346180638,0.0331702036889932),.UNSPECIFIED.);
#3086=B_SPLINE_SURFACE_WITH_KNOTS('',3,3,((#98456,#98457,#98458,#98459),
(#98460,#98461,#98462,#98463),(#98464,#98465,#98466,#98467),(#98468,#98469,
#98470,#98471)),.UNSPECIFIED.,.F.,.F.,.F.,(4,4),(4,4),(-0.00286848453340593,
0.47790287978974),(0.0400218729466611,0.0466073985929437),.UNSPECIFIED.);
#3087=B_SPLINE_SURFACE_WITH_KNOTS('',3,3,((#98488,#98489,#98490,#98491),
(#98492,#98493,#98494,#98495),(#98496,#98497,#98498,#98499),(#98500,#98501,
#98502,#98503)),.UNSPECIFIED.,.F.,.F.,.F.,(4,4),(4,4),(0.,1.00600014639748),
(0.0365944846645065,0.0466073985929166),.UNSPECIFIED.);
#3088=B_SPLINE_SURFACE_WITH_KNOTS('',3,3,((#98504,#98505,#98506,#98507),
(#98508,#98509,#98510,#98511),(#98512,#98513,#98514,#98515),(#98516,#98517,
#98518,#98519)),.UNSPECIFIED.,.F.,.F.,.F.,(4,4),(4,4),(-0.00286780122467488,
0.477902879789109),(0.0500263550859008,0.0565997133101401),
 .UNSPECIFIED.);
#3089=B_SPLINE_SURFACE_WITH_KNOTS('',3,3,((#98521,#98522,#98523,#98524),
(#98525,#98526,#98527,#98528),(#98529,#98530,#98531,#98532),(#98533,#98534,
#98535,#98536)),.UNSPECIFIED.,.F.,.F.,.F.,(4,4),(4,4),(0.522097120209639,
1.0028681017725),(0.0466073985929444,0.0531834925888927),.UNSPECIFIED.);
#3090=B_SPLINE_SURFACE_WITH_KNOTS('',3,3,((#98544,#98545,#98546,#98547),
(#98548,#98549,#98550,#98551),(#98552,#98553,#98554,#98555),(#98556,#98557,
#98558,#98559)),.UNSPECIFIED.,.F.,.F.,.F.,(4,4),(4,4),(-0.00286792598901557,
0.477902879789036),(0.0600156865494605,0.0665898698871177),
 .UNSPECIFIED.);
#3091=B_SPLINE_SURFACE_WITH_KNOTS('',3,3,((#98561,#98562,#98563,#98564),
(#98565,#98566,#98567,#98568),(#98569,#98570,#98571,#98572),(#98573,#98574,
#98575,#98576)),.UNSPECIFIED.,.F.,.F.,.F.,(4,4),(4,4),(0.522097120208366,
1.00286764392047),(0.056599713310141,0.0631721430887066),.UNSPECIFIED.);
#3092=B_SPLINE_SURFACE_WITH_KNOTS('',3,3,((#98592,#98593,#98594,#98595),
(#98596,#98597,#98598,#98599),(#98600,#98601,#98602,#98603),(#98604,#98605,
#98606,#98607)),.UNSPECIFIED.,.F.,.F.,.F.,(4,4),(4,4),(0.522097120206995,
1.00286833998595),(0.0665898698871194,0.0731716198748452),.UNSPECIFIED.);
#3093=B_SPLINE_SURFACE_WITH_KNOTS('',3,3,((#98608,#98609,#98610,#98611),
(#98612,#98613,#98614,#98615),(#98616,#98617,#98618,#98619),(#98620,#98621,
#98622,#98623)),.UNSPECIFIED.,.F.,.F.,.F.,(4,4),(4,4),(-0.00124731532103649,
0.209045111673288),(0.070019429296636,0.074990098297651),.UNSPECIFIED.);
#3094=B_SPLINE_SURFACE_WITH_KNOTS('',3,3,((#98630,#98631,#98632,#98633),
(#98634,#98635,#98636,#98637),(#98638,#98639,#98640,#98641),(#98642,#98643,
#98644,#98645)),.UNSPECIFIED.,.F.,.F.,.F.,(4,4),(4,4),(-0.00286791014454375,
0.477902879789698),(0.0100271466769373,0.0166015299239864),
 .UNSPECIFIED.);
#3095=B_SPLINE_SURFACE_WITH_KNOTS('',3,3,((#98647,#98648,#98649,#98650),
(#98651,#98652,#98653,#98654),(#98655,#98656,#98657,#98658),(#98659,#98660,
#98661,#98662)),.UNSPECIFIED.,.F.,.F.,.F.,(4,4),(4,4),(0.653230271507101,
1.00206901893051),(0.00656788395379447,0.0131849432429115),
 .UNSPECIFIED.);
#3096=B_SPLINE_SURFACE_WITH_KNOTS('',3,3,((#98670,#98671,#98672,#98673),
(#98674,#98675,#98676,#98677),(#98678,#98679,#98680,#98681),(#98682,#98683,
#98684,#98685)),.UNSPECIFIED.,.F.,.F.,.F.,(4,4),(4,4),(-0.00286780410484465,
0.47790287978942),(0.0200175229646894,0.0265907346180617),.UNSPECIFIED.);
#3097=B_SPLINE_SURFACE_WITH_KNOTS('',3,3,((#98687,#98688,#98689,#98690),
(#98691,#98692,#98693,#98694),(#98695,#98696,#98697,#98698),(#98699,#98700,
#98701,#98702)),.UNSPECIFIED.,.F.,.F.,.F.,(4,4),(4,4),(0.522097120210559,
1.00286753160123),(0.0166015299239872,0.0231736788037107),.UNSPECIFIED.);
#3098=B_SPLINE_SURFACE_WITH_KNOTS('',3,3,((#98704,#98705,#98706,#98707),
(#98708,#98709,#98710,#98711),(#98712,#98713,#98714,#98715),(#98716,#98717,
#98718,#98719)),.UNSPECIFIED.,.F.,.F.,.F.,(4,4),(4,4),(0.,1.00600003961392),
(0.016601529923987,0.0265907346180635),.UNSPECIFIED.);
#3099=B_SPLINE_SURFACE_WITH_KNOTS('',3,3,((#98720,#98721,#98722,#98723),
(#98724,#98725,#98726,#98727),(#98728,#98729,#98730,#98731),(#98732,#98733,
#98734,#98735)),.UNSPECIFIED.,.F.,.F.,.F.,(4,4),(4,4),(-0.00286862201165759,
0.477902879791254),(0.0300094532292787,0.0365944846647016),
 .UNSPECIFIED.);
#3100=B_SPLINE_SURFACE_WITH_KNOTS('',3,3,((#98737,#98738,#98739,#98740),
(#98741,#98742,#98743,#98744),(#98745,#98746,#98747,#98748),(#98749,#98750,
#98751,#98752)),.UNSPECIFIED.,.F.,.F.,.F.,(4,4),(4,4),(0.522097120210765,
1.00286823669301),(0.0265907346180635,0.0331702036622759),.UNSPECIFIED.);
#3101=B_SPLINE_SURFACE_WITH_KNOTS('',3,3,((#98760,#98761,#98762,#98763),
(#98764,#98765,#98766,#98767),(#98768,#98769,#98770,#98771),(#98772,#98773,
#98774,#98775)),.UNSPECIFIED.,.F.,.F.,.F.,(4,4),(4,4),(-0.00286848453341356,
0.477902879789721),(0.0400218729466614,0.0466073985929431),
 .UNSPECIFIED.);
#3102=B_SPLINE_SURFACE_WITH_KNOTS('',3,3,((#98792,#98793,#98794,#98795),
(#98796,#98797,#98798,#98799),(#98800,#98801,#98802,#98803),(#98804,#98805,
#98806,#98807)),.UNSPECIFIED.,.F.,.F.,.F.,(4,4),(4,4),(0.,1.00600014639744),
(0.0365944846645058,0.0466073985929154),.UNSPECIFIED.);
#3103=B_SPLINE_SURFACE_WITH_KNOTS('',3,3,((#98808,#98809,#98810,#98811),
(#98812,#98813,#98814,#98815),(#98816,#98817,#98818,#98819),(#98820,#98821,
#98822,#98823)),.UNSPECIFIED.,.F.,.F.,.F.,(4,4),(4,4),(-0.00286780122470342,
0.477902879789203),(0.0500263550858997,0.0565997133101398),
 .UNSPECIFIED.);
#3104=B_SPLINE_SURFACE_WITH_KNOTS('',3,3,((#98825,#98826,#98827,#98828),
(#98829,#98830,#98831,#98832),(#98833,#98834,#98835,#98836),(#98837,#98838,
#98839,#98840)),.UNSPECIFIED.,.F.,.F.,.F.,(4,4),(4,4),(0.522097120210796,
1.00286810177246),(0.0466073985929437,0.0531834922865657),.UNSPECIFIED.);
#3105=B_SPLINE_SURFACE_WITH_KNOTS('',3,3,((#98848,#98849,#98850,#98851),
(#98852,#98853,#98854,#98855),(#98856,#98857,#98858,#98859),(#98860,#98861,
#98862,#98863)),.UNSPECIFIED.,.F.,.F.,.F.,(4,4),(4,4),(-0.00286792598889512,
0.477902879788943),(0.060015686549461,0.0665898698871167),.UNSPECIFIED.);
#3106=B_SPLINE_SURFACE_WITH_KNOTS('',3,3,((#98865,#98866,#98867,#98868),
(#98869,#98870,#98871,#98872),(#98873,#98874,#98875,#98876),(#98877,#98878,
#98879,#98880)),.UNSPECIFIED.,.F.,.F.,.F.,(4,4),(4,4),(0.522097120210891,
1.0028676439204),(0.0565997133101416,0.0631721430887053),.UNSPECIFIED.);
#3107=B_SPLINE_SURFACE_WITH_KNOTS('',3,3,((#98896,#98897,#98898,#98899),
(#98900,#98901,#98902,#98903),(#98904,#98905,#98906,#98907),(#98908,#98909,
#98910,#98911)),.UNSPECIFIED.,.F.,.F.,.F.,(4,4),(4,4),(0.522097120209503,
1.00286833998596),(0.0665898698871188,0.073171619874845),.UNSPECIFIED.);
#3108=B_SPLINE_SURFACE_WITH_KNOTS('',3,3,((#98912,#98913,#98914,#98915),
(#98916,#98917,#98918,#98919),(#98920,#98921,#98922,#98923),(#98924,#98925,
#98926,#98927)),.UNSPECIFIED.,.F.,.F.,.F.,(4,4),(4,4),(-0.00124731532102576,
0.209045111672193),(0.0700194292966195,0.0749900982976457),
 .UNSPECIFIED.);
#3109=B_SPLINE_SURFACE_WITH_KNOTS('',3,3,((#98934,#98935,#98936,#98937),
(#98938,#98939,#98940,#98941),(#98942,#98943,#98944,#98945),(#98946,#98947,
#98948,#98949)),.UNSPECIFIED.,.F.,.F.,.F.,(4,4),(4,4),(-0.00286791014449015,
0.47790287978987),(0.0100271466769346,0.0166015299239873),.UNSPECIFIED.);
#3110=B_SPLINE_SURFACE_WITH_KNOTS('',3,3,((#98951,#98952,#98953,#98954),
(#98955,#98956,#98957,#98958),(#98959,#98960,#98961,#98962),(#98963,#98964,
#98965,#98966)),.UNSPECIFIED.,.F.,.F.,.F.,(4,4),(4,4),(0.653230271506975,
1.00206901893248),(0.00656788395379699,0.0131849432430145),
 .UNSPECIFIED.);
#3111=B_SPLINE_SURFACE_WITH_KNOTS('',3,3,((#98974,#98975,#98976,#98977),
(#98978,#98979,#98980,#98981),(#98982,#98983,#98984,#98985),(#98986,#98987,
#98988,#98989)),.UNSPECIFIED.,.F.,.F.,.F.,(4,4),(4,4),(-0.00286780410469933,
0.477902879789596),(0.0200175229646896,0.026590734618062),.UNSPECIFIED.);
#3112=B_SPLINE_SURFACE_WITH_KNOTS('',3,3,((#98991,#98992,#98993,#98994),
(#98995,#98996,#98997,#98998),(#98999,#99000,#99001,#99002),(#99003,#99004,
#99005,#99006)),.UNSPECIFIED.,.F.,.F.,.F.,(4,4),(4,4),(0.522097120210308,
1.00286753160123),(0.0166015299239883,0.0231736788037113),.UNSPECIFIED.);
#3113=B_SPLINE_SURFACE_WITH_KNOTS('',3,3,((#99008,#99009,#99010,#99011),
(#99012,#99013,#99014,#99015),(#99016,#99017,#99018,#99019),(#99020,#99021,
#99022,#99023)),.UNSPECIFIED.,.F.,.F.,.F.,(4,4),(4,4),(0.,1.0060000396139),
(0.0166015299239893,0.0265907346180633),.UNSPECIFIED.);
#3114=B_SPLINE_SURFACE_WITH_KNOTS('',3,3,((#99024,#99025,#99026,#99027),
(#99028,#99029,#99030,#99031),(#99032,#99033,#99034,#99035),(#99036,#99037,
#99038,#99039)),.UNSPECIFIED.,.F.,.F.,.F.,(4,4),(4,4),(-0.00286862201163364,
0.477902879791346),(0.030009453229279,0.0365944846647037),.UNSPECIFIED.);
#3115=B_SPLINE_SURFACE_WITH_KNOTS('',3,3,((#99041,#99042,#99043,#99044),
(#99045,#99046,#99047,#99048),(#99049,#99050,#99051,#99052),(#99053,#99054,
#99055,#99056)),.UNSPECIFIED.,.F.,.F.,.F.,(4,4),(4,4),(0.522097120210626,
1.00286823669299),(0.0265907346180645,0.0331702036622782),.UNSPECIFIED.);
#3116=B_SPLINE_SURFACE_WITH_KNOTS('',3,3,((#99064,#99065,#99066,#99067),
(#99068,#99069,#99070,#99071),(#99072,#99073,#99074,#99075),(#99076,#99077,
#99078,#99079)),.UNSPECIFIED.,.F.,.F.,.F.,(4,4),(4,4),(-0.00286848453330232,
0.47790287978981),(0.0400218729466605,0.0466073985929431),.UNSPECIFIED.);
#3117=B_SPLINE_SURFACE_WITH_KNOTS('',3,3,((#99096,#99097,#99098,#99099),
(#99100,#99101,#99102,#99103),(#99104,#99105,#99106,#99107),(#99108,#99109,
#99110,#99111)),.UNSPECIFIED.,.F.,.F.,.F.,(4,4),(4,4),(0.,1.0060001463974),
(0.036594484664507,0.0466073985929166),.UNSPECIFIED.);
#3118=B_SPLINE_SURFACE_WITH_KNOTS('',3,3,((#99112,#99113,#99114,#99115),
(#99116,#99117,#99118,#99119),(#99120,#99121,#99122,#99123),(#99124,#99125,
#99126,#99127)),.UNSPECIFIED.,.F.,.F.,.F.,(4,4),(4,4),(-0.00286780122463184,
0.477902879789366),(0.0500263550859003,0.0565997133101415),
 .UNSPECIFIED.);
#3119=B_SPLINE_SURFACE_WITH_KNOTS('',3,3,((#99129,#99130,#99131,#99132),
(#99133,#99134,#99135,#99136),(#99137,#99138,#99139,#99140),(#99141,#99142,
#99143,#99144)),.UNSPECIFIED.,.F.,.F.,.F.,(4,4),(4,4),(0.522097120210698,
1.0028681017726),(0.0466073985929441,0.0531834925888937),.UNSPECIFIED.);
#3120=B_SPLINE_SURFACE_WITH_KNOTS('',3,3,((#99152,#99153,#99154,#99155),
(#99156,#99157,#99158,#99159),(#99160,#99161,#99162,#99163),(#99164,#99165,
#99166,#99167)),.UNSPECIFIED.,.F.,.F.,.F.,(4,4),(4,4),(-0.00286792598895932,
0.477902879789034),(0.0600156865494597,0.0665898698871171),
 .UNSPECIFIED.);
#3121=B_SPLINE_SURFACE_WITH_KNOTS('',3,3,((#99169,#99170,#99171,#99172),
(#99173,#99174,#99175,#99176),(#99177,#99178,#99179,#99180),(#99181,#99182,
#99183,#99184)),.UNSPECIFIED.,.F.,.F.,.F.,(4,4),(4,4),(0.522097120210928,
1.00286764392042),(0.0565997133101425,0.0631721430887067),.UNSPECIFIED.);
#3122=B_SPLINE_SURFACE_WITH_KNOTS('',3,3,((#99200,#99201,#99202,#99203),
(#99204,#99205,#99206,#99207),(#99208,#99209,#99210,#99211),(#99212,#99213,
#99214,#99215)),.UNSPECIFIED.,.F.,.F.,.F.,(4,4),(4,4),(0.522097120210139,
1.002868339986),(0.0665898698871195,0.0731716198748449),.UNSPECIFIED.);
#3123=B_SPLINE_SURFACE_WITH_KNOTS('',3,3,((#99216,#99217,#99218,#99219),
(#99220,#99221,#99222,#99223),(#99224,#99225,#99226,#99227),(#99228,#99229,
#99230,#99231)),.UNSPECIFIED.,.F.,.F.,.F.,(4,4),(4,4),(-0.0012473153210028,
0.209045111671177),(0.0700194292966059,0.0749900982976427),
 .UNSPECIFIED.);
#3124=B_SPLINE_SURFACE_WITH_KNOTS('',3,3,((#99238,#99239,#99240,#99241),
(#99242,#99243,#99244,#99245),(#99246,#99247,#99248,#99249),(#99250,#99251,
#99252,#99253)),.UNSPECIFIED.,.F.,.F.,.F.,(4,4),(4,4),(-0.00286791014442176,
0.477902879789923),(0.0100271466769339,0.0166015299239868),
 .UNSPECIFIED.);
#3125=B_SPLINE_SURFACE_WITH_KNOTS('',3,3,((#99255,#99256,#99257,#99258),
(#99259,#99260,#99261,#99262),(#99263,#99264,#99265,#99266),(#99267,#99268,
#99269,#99270)),.UNSPECIFIED.,.F.,.F.,.F.,(4,4),(4,4),(0.653230271506902,
1.00206901893463),(0.00656788395380054,0.0131849432430249),
 .UNSPECIFIED.);
#3126=B_SPLINE_SURFACE_WITH_KNOTS('',3,3,((#99278,#99279,#99280,#99281),
(#99282,#99283,#99284,#99285),(#99286,#99287,#99288,#99289),(#99290,#99291,
#99292,#99293)),.UNSPECIFIED.,.F.,.F.,.F.,(4,4),(4,4),(-0.00286780410473915,
0.477902879789725),(0.0200175229646895,0.0265907346180625),
 .UNSPECIFIED.);
#3127=B_SPLINE_SURFACE_WITH_KNOTS('',3,3,((#99295,#99296,#99297,#99298),
(#99299,#99300,#99301,#99302),(#99303,#99304,#99305,#99306),(#99307,#99308,
#99309,#99310)),.UNSPECIFIED.,.F.,.F.,.F.,(4,4),(4,4),(0.522097120210315,
1.00286753160118),(0.0166015299239891,0.0231736788037108),.UNSPECIFIED.);
#3128=B_SPLINE_SURFACE_WITH_KNOTS('',3,3,((#99312,#99313,#99314,#99315),
(#99316,#99317,#99318,#99319),(#99320,#99321,#99322,#99323),(#99324,#99325,
#99326,#99327)),.UNSPECIFIED.,.F.,.F.,.F.,(4,4),(4,4),(0.,1.0060000396137),
(0.0166015299239869,0.0265907346180621),.UNSPECIFIED.);
#3129=B_SPLINE_SURFACE_WITH_KNOTS('',3,3,((#99328,#99329,#99330,#99331),
(#99332,#99333,#99334,#99335),(#99336,#99337,#99338,#99339),(#99340,#99341,
#99342,#99343)),.UNSPECIFIED.,.F.,.F.,.F.,(4,4),(4,4),(-0.00286862201153849,
0.477902879791419),(0.0300094532292795,0.0365944846647028),
 .UNSPECIFIED.);
#3130=B_SPLINE_SURFACE_WITH_KNOTS('',3,3,((#99345,#99346,#99347,#99348),
(#99349,#99350,#99351,#99352),(#99353,#99354,#99355,#99356),(#99357,#99358,
#99359,#99360)),.UNSPECIFIED.,.F.,.F.,.F.,(4,4),(4,4),(0.522097120210556,
1.00286823669293),(0.0265907346180642,0.0331702036889928),.UNSPECIFIED.);
#3131=B_SPLINE_SURFACE_WITH_KNOTS('',3,3,((#99368,#99369,#99370,#99371),
(#99372,#99373,#99374,#99375),(#99376,#99377,#99378,#99379),(#99380,#99381,
#99382,#99383)),.UNSPECIFIED.,.F.,.F.,.F.,(4,4),(4,4),(-0.00286848453325725,
0.477902879790036),(0.0400218729466594,0.0466073985929445),
 .UNSPECIFIED.);
#3132=B_SPLINE_SURFACE_WITH_KNOTS('',3,3,((#99400,#99401,#99402,#99403),
(#99404,#99405,#99406,#99407),(#99408,#99409,#99410,#99411),(#99412,#99413,
#99414,#99415)),.UNSPECIFIED.,.F.,.F.,.F.,(4,4),(4,4),(0.,1.00600014639735),
(0.0365944846645063,0.046607398592916),.UNSPECIFIED.);
#3133=B_SPLINE_SURFACE_WITH_KNOTS('',3,3,((#99416,#99417,#99418,#99419),
(#99420,#99421,#99422,#99423),(#99424,#99425,#99426,#99427),(#99428,#99429,
#99430,#99431)),.UNSPECIFIED.,.F.,.F.,.F.,(4,4),(4,4),(-0.00286780122456139,
0.477902879789289),(0.0500263550859003,0.0565997133101399),
 .UNSPECIFIED.);
#3134=B_SPLINE_SURFACE_WITH_KNOTS('',3,3,((#99433,#99434,#99435,#99436),
(#99437,#99438,#99439,#99440),(#99441,#99442,#99443,#99444),(#99445,#99446,
#99447,#99448)),.UNSPECIFIED.,.F.,.F.,.F.,(4,4),(4,4),(0.522097120210739,
1.00286810177251),(0.046607398592945,0.0531834925888924),.UNSPECIFIED.);
#3135=B_SPLINE_SURFACE_WITH_KNOTS('',3,3,((#99456,#99457,#99458,#99459),
(#99460,#99461,#99462,#99463),(#99464,#99465,#99466,#99467),(#99468,#99469,
#99470,#99471)),.UNSPECIFIED.,.F.,.F.,.F.,(4,4),(4,4),(-0.00286792598899,
0.477902879789314),(0.0600156865494594,0.0665898698871176),
 .UNSPECIFIED.);
#3136=B_SPLINE_SURFACE_WITH_KNOTS('',3,3,((#99473,#99474,#99475,#99476),
(#99477,#99478,#99479,#99480),(#99481,#99482,#99483,#99484),(#99485,#99486,
#99487,#99488)),.UNSPECIFIED.,.F.,.F.,.F.,(4,4),(4,4),(0.522097120210747,
1.00286764392045),(0.0565997133101418,0.0631721430887066),.UNSPECIFIED.);
#3137=B_SPLINE_SURFACE_WITH_KNOTS('',3,3,((#99504,#99505,#99506,#99507),
(#99508,#99509,#99510,#99511),(#99512,#99513,#99514,#99515),(#99516,#99517,
#99518,#99519)),.UNSPECIFIED.,.F.,.F.,.F.,(4,4),(4,4),(0.522097120209877,
1.00286833998603),(0.0665898698871188,0.0731716198748456),.UNSPECIFIED.);
#3138=B_SPLINE_SURFACE_WITH_KNOTS('',3,3,((#99520,#99521,#99522,#99523),
(#99524,#99525,#99526,#99527),(#99528,#99529,#99530,#99531),(#99532,#99533,
#99534,#99535)),.UNSPECIFIED.,.F.,.F.,.F.,(4,4),(4,4),(-0.00124731532106721,
0.209045111670196),(0.0700194292965919,0.0749900982976401),
 .UNSPECIFIED.);
#3139=B_SPLINE_SURFACE_WITH_KNOTS('',3,3,((#99542,#99543,#99544,#99545),
(#99546,#99547,#99548,#99549),(#99550,#99551,#99552,#99553),(#99554,#99555,
#99556,#99557)),.UNSPECIFIED.,.F.,.F.,.F.,(4,4),(4,4),(-0.00286791014437286,
0.477902879790058),(0.010027146676935,0.0166015299239852),.UNSPECIFIED.);
#3140=B_SPLINE_SURFACE_WITH_KNOTS('',3,3,((#99559,#99560,#99561,#99562),
(#99563,#99564,#99565,#99566),(#99567,#99568,#99569,#99570),(#99571,#99572,
#99573,#99574)),.UNSPECIFIED.,.F.,.F.,.F.,(4,4),(4,4),(0.653230271507036,
1.00206901892628),(0.00656788395380599,0.0131849432430315),
 .UNSPECIFIED.);
#3141=B_SPLINE_SURFACE_WITH_KNOTS('',3,3,((#99582,#99583,#99584,#99585),
(#99586,#99587,#99588,#99589),(#99590,#99591,#99592,#99593),(#99594,#99595,
#99596,#99597)),.UNSPECIFIED.,.F.,.F.,.F.,(4,4),(4,4),(-0.00286780410475729,
0.477902879789832),(0.02001752296469,0.026590734618062),.UNSPECIFIED.);
#3142=B_SPLINE_SURFACE_WITH_KNOTS('',3,3,((#99599,#99600,#99601,#99602),
(#99603,#99604,#99605,#99606),(#99607,#99608,#99609,#99610),(#99611,#99612,
#99613,#99614)),.UNSPECIFIED.,.F.,.F.,.F.,(4,4),(4,4),(0.52209712021033,
1.00286753160121),(0.0166015299239888,0.0231736788037107),.UNSPECIFIED.);
#3143=B_SPLINE_SURFACE_WITH_KNOTS('',3,3,((#99616,#99617,#99618,#99619),
(#99620,#99621,#99622,#99623),(#99624,#99625,#99626,#99627),(#99628,#99629,
#99630,#99631)),.UNSPECIFIED.,.F.,.F.,.F.,(4,4),(4,4),(0.,1.00600003961385),
(0.0166015299239882,0.0265907346180635),.UNSPECIFIED.);
#3144=B_SPLINE_SURFACE_WITH_KNOTS('',3,3,((#99632,#99633,#99634,#99635),
(#99636,#99637,#99638,#99639),(#99640,#99641,#99642,#99643),(#99644,#99645,
#99646,#99647)),.UNSPECIFIED.,.F.,.F.,.F.,(4,4),(4,4),(-0.00286862201164465,
0.477902879791502),(0.0300094532292795,0.0365944846647017),
 .UNSPECIFIED.);
#3145=B_SPLINE_SURFACE_WITH_KNOTS('',3,3,((#99649,#99650,#99651,#99652),
(#99653,#99654,#99655,#99656),(#99657,#99658,#99659,#99660),(#99661,#99662,
#99663,#99664)),.UNSPECIFIED.,.F.,.F.,.F.,(4,4),(4,4),(0.52209712021055,
1.00286823669298),(0.0265907346180646,0.0331702036051747),.UNSPECIFIED.);
#3146=B_SPLINE_SURFACE_WITH_KNOTS('',3,3,((#99672,#99673,#99674,#99675),
(#99676,#99677,#99678,#99679),(#99680,#99681,#99682,#99683),(#99684,#99685,
#99686,#99687)),.UNSPECIFIED.,.F.,.F.,.F.,(4,4),(4,4),(-0.00286848453320442,
0.477902879790044),(0.0400218729466604,0.0466073985929431),
 .UNSPECIFIED.);
#3147=B_SPLINE_SURFACE_WITH_KNOTS('',3,3,((#99704,#99705,#99706,#99707),
(#99708,#99709,#99710,#99711),(#99712,#99713,#99714,#99715),(#99716,#99717,
#99718,#99719)),.UNSPECIFIED.,.F.,.F.,.F.,(4,4),(4,4),(0.,1.00600014639742),
(0.0365944846645066,0.0466073985929164),.UNSPECIFIED.);
#3148=B_SPLINE_SURFACE_WITH_KNOTS('',3,3,((#99720,#99721,#99722,#99723),
(#99724,#99725,#99726,#99727),(#99728,#99729,#99730,#99731),(#99732,#99733,
#99734,#99735)),.UNSPECIFIED.,.F.,.F.,.F.,(4,4),(4,4),(-0.00286780122448064,
0.47790287978947),(0.0500263550859002,0.0565997133101405),.UNSPECIFIED.);
#3149=B_SPLINE_SURFACE_WITH_KNOTS('',3,3,((#99737,#99738,#99739,#99740),
(#99741,#99742,#99743,#99744),(#99745,#99746,#99747,#99748),(#99749,#99750,
#99751,#99752)),.UNSPECIFIED.,.F.,.F.,.F.,(4,4),(4,4),(0.522097120210521,
1.00286810177273),(0.0466073985929442,0.0531834933545511),.UNSPECIFIED.);
#3150=B_SPLINE_SURFACE_WITH_KNOTS('',3,3,((#99760,#99761,#99762,#99763),
(#99764,#99765,#99766,#99767),(#99768,#99769,#99770,#99771),(#99772,#99773,
#99774,#99775)),.UNSPECIFIED.,.F.,.F.,.F.,(4,4),(4,4),(-0.00286792598884402,
0.47790287978941),(0.0600156865494606,0.0665898698871172),.UNSPECIFIED.);
#3151=B_SPLINE_SURFACE_WITH_KNOTS('',3,3,((#99777,#99778,#99779,#99780),
(#99781,#99782,#99783,#99784),(#99785,#99786,#99787,#99788),(#99789,#99790,
#99791,#99792)),.UNSPECIFIED.,.F.,.F.,.F.,(4,4),(4,4),(0.522097120210711,
1.00286764392047),(0.0565997133101428,0.0631721430887067),.UNSPECIFIED.);
#3152=B_SPLINE_SURFACE_WITH_KNOTS('',3,3,((#99808,#99809,#99810,#99811),
(#99812,#99813,#99814,#99815),(#99816,#99817,#99818,#99819),(#99820,#99821,
#99822,#99823)),.UNSPECIFIED.,.F.,.F.,.F.,(4,4),(4,4),(0.522097120209842,
1.00286833998597),(0.0665898698871195,0.0731716198748457),.UNSPECIFIED.);
#3153=B_SPLINE_SURFACE_WITH_KNOTS('',3,3,((#99824,#99825,#99826,#99827),
(#99828,#99829,#99830,#99831),(#99832,#99833,#99834,#99835),(#99836,#99837,
#99838,#99839)),.UNSPECIFIED.,.F.,.F.,.F.,(4,4),(4,4),(-0.0012473153210368,
0.209045111669589),(0.0700194292965764,0.0749900982976409),
 .UNSPECIFIED.);
#3154=B_SPLINE_SURFACE_WITH_KNOTS('',3,3,((#99846,#99847,#99848,#99849),
(#99850,#99851,#99852,#99853),(#99854,#99855,#99856,#99857),(#99858,#99859,
#99860,#99861)),.UNSPECIFIED.,.F.,.F.,.F.,(4,4),(4,4),(-0.00286791014430819,
0.477902879790145),(0.0100271466769347,0.0166015299239866),
 .UNSPECIFIED.);
#3155=B_SPLINE_SURFACE_WITH_KNOTS('',3,3,((#99863,#99864,#99865,#99866),
(#99867,#99868,#99869,#99870),(#99871,#99872,#99873,#99874),(#99875,#99876,
#99877,#99878)),.UNSPECIFIED.,.F.,.F.,.F.,(4,4),(4,4),(0.65323027150708,
1.00206901892629),(0.00656788395381101,0.0131849432430403),
 .UNSPECIFIED.);
#3156=B_SPLINE_SURFACE_WITH_KNOTS('',3,3,((#99886,#99887,#99888,#99889),
(#99890,#99891,#99892,#99893),(#99894,#99895,#99896,#99897),(#99898,#99899,
#99900,#99901)),.UNSPECIFIED.,.F.,.F.,.F.,(4,4),(4,4),(-0.00286780410471765,
0.477902879789932),(0.0200175229646929,0.026590734618062),.UNSPECIFIED.);
#3157=B_SPLINE_SURFACE_WITH_KNOTS('',3,3,((#99903,#99904,#99905,#99906),
(#99907,#99908,#99909,#99910),(#99911,#99912,#99913,#99914),(#99915,#99916,
#99917,#99918)),.UNSPECIFIED.,.F.,.F.,.F.,(4,4),(4,4),(0.522097120210158,
1.00286753160114),(0.0166015299239891,0.0231736788075221),.UNSPECIFIED.);
#3158=B_SPLINE_SURFACE_WITH_KNOTS('',3,3,((#99920,#99921,#99922,#99923),
(#99924,#99925,#99926,#99927),(#99928,#99929,#99930,#99931),(#99932,#99933,
#99934,#99935)),.UNSPECIFIED.,.F.,.F.,.F.,(4,4),(4,4),(0.,1.00600003961369),
(0.0166015299239894,0.0265907346180634),.UNSPECIFIED.);
#3159=B_SPLINE_SURFACE_WITH_KNOTS('',3,3,((#99936,#99937,#99938,#99939),
(#99940,#99941,#99942,#99943),(#99944,#99945,#99946,#99947),(#99948,#99949,
#99950,#99951)),.UNSPECIFIED.,.F.,.F.,.F.,(4,4),(4,4),(-0.00286862201159803,
0.47790287979161),(0.0300094532292792,0.0365944846647022),.UNSPECIFIED.);
#3160=B_SPLINE_SURFACE_WITH_KNOTS('',3,3,((#99953,#99954,#99955,#99956),
(#99957,#99958,#99959,#99960),(#99961,#99962,#99963,#99964),(#99965,#99966,
#99967,#99968)),.UNSPECIFIED.,.F.,.F.,.F.,(4,4),(4,4),(0.52209712021027,
1.00286823669294),(0.0265907346180636,0.0331702036051739),.UNSPECIFIED.);
#3161=B_SPLINE_SURFACE_WITH_KNOTS('',3,3,((#99976,#99977,#99978,#99979),
(#99980,#99981,#99982,#99983),(#99984,#99985,#99986,#99987),(#99988,#99989,
#99990,#99991)),.UNSPECIFIED.,.F.,.F.,.F.,(4,4),(4,4),(-0.00286848453316211,
0.477902879790156),(0.0400218729466606,0.0466073985929427),
 .UNSPECIFIED.);
#3162=B_SPLINE_SURFACE_WITH_KNOTS('',3,3,((#100008,#100009,#100010,#100011),
(#100012,#100013,#100014,#100015),(#100016,#100017,#100018,#100019),(#100020,
#100021,#100022,#100023)),.UNSPECIFIED.,.F.,.F.,.F.,(4,4),(4,4),(0.,1.00600014639725),
(0.0365944846645068,0.0466073985929167),.UNSPECIFIED.);
#3163=B_SPLINE_SURFACE_WITH_KNOTS('',3,3,((#100024,#100025,#100026,#100027),
(#100028,#100029,#100030,#100031),(#100032,#100033,#100034,#100035),(#100036,
#100037,#100038,#100039)),.UNSPECIFIED.,.F.,.F.,.F.,(4,4),(4,4),(-0.00286780122448816,
0.477902879789605),(0.0500263550859002,0.0565997133101408),
 .UNSPECIFIED.);
#3164=B_SPLINE_SURFACE_WITH_KNOTS('',3,3,((#100041,#100042,#100043,#100044),
(#100045,#100046,#100047,#100048),(#100049,#100050,#100051,#100052),(#100053,
#100054,#100055,#100056)),.UNSPECIFIED.,.F.,.F.,.F.,(4,4),(4,4),(0.522097120210515,
1.00286810177255),(0.0466073985929452,0.0531834925888926),.UNSPECIFIED.);
#3165=B_SPLINE_SURFACE_WITH_KNOTS('',3,3,((#100064,#100065,#100066,#100067),
(#100068,#100069,#100070,#100071),(#100072,#100073,#100074,#100075),(#100076,
#100077,#100078,#100079)),.UNSPECIFIED.,.F.,.F.,.F.,(4,4),(4,4),(-0.00286792598896076,
0.477902879789448),(0.0600156865494602,0.0665898698871176),
 .UNSPECIFIED.);
#3166=B_SPLINE_SURFACE_WITH_KNOTS('',3,3,((#100081,#100082,#100083,#100084),
(#100085,#100086,#100087,#100088),(#100089,#100090,#100091,#100092),(#100093,
#100094,#100095,#100096)),.UNSPECIFIED.,.F.,.F.,.F.,(4,4),(4,4),(0.522097120210527,
1.00286764392044),(0.0565997133101414,0.0631721430887068),.UNSPECIFIED.);
#3167=B_SPLINE_SURFACE_WITH_KNOTS('',3,3,((#100112,#100113,#100114,#100115),
(#100116,#100117,#100118,#100119),(#100120,#100121,#100122,#100123),(#100124,
#100125,#100126,#100127)),.UNSPECIFIED.,.F.,.F.,.F.,(4,4),(4,4),(0.522097120209726,
1.00286833998588),(0.0665898698871198,0.0731716198748447),.UNSPECIFIED.);
#3168=B_SPLINE_SURFACE_WITH_KNOTS('',3,3,((#100128,#100129,#100130,#100131),
(#100132,#100133,#100134,#100135),(#100136,#100137,#100138,#100139),(#100140,
#100141,#100142,#100143)),.UNSPECIFIED.,.F.,.F.,.F.,(4,4),(4,4),(-0.00124731532101478,
0.209045111669004),(0.0700194292965637,0.0749900982976416),
 .UNSPECIFIED.);
#3169=B_SPLINE_SURFACE_WITH_KNOTS('',3,3,((#100150,#100151,#100152,#100153),
(#100154,#100155,#100156,#100157),(#100158,#100159,#100160,#100161),(#100162,
#100163,#100164,#100165)),.UNSPECIFIED.,.F.,.F.,.F.,(4,4),(4,4),(-0.00286791014427452,
0.477902879790323),(0.0100271466769346,0.0166015299239864),
 .UNSPECIFIED.);
#3170=B_SPLINE_SURFACE_WITH_KNOTS('',3,3,((#100167,#100168,#100169,#100170),
(#100171,#100172,#100173,#100174),(#100175,#100176,#100177,#100178),(#100179,
#100180,#100181,#100182)),.UNSPECIFIED.,.F.,.F.,.F.,(4,4),(4,4),(0.653230271507165,
1.00206901892629),(0.00656788395381716,0.0131849432430449),
 .UNSPECIFIED.);
#3171=B_SPLINE_SURFACE_WITH_KNOTS('',3,3,((#100190,#100191,#100192,#100193),
(#100194,#100195,#100196,#100197),(#100198,#100199,#100200,#100201),(#100202,
#100203,#100204,#100205)),.UNSPECIFIED.,.F.,.F.,.F.,(4,4),(4,4),(-0.00286780410474001,
0.477902879790114),(0.0200175229646904,0.0265907346180623),
 .UNSPECIFIED.);
#3172=B_SPLINE_SURFACE_WITH_KNOTS('',3,3,((#100207,#100208,#100209,#100210),
(#100211,#100212,#100213,#100214),(#100215,#100216,#100217,#100218),(#100219,
#100220,#100221,#100222)),.UNSPECIFIED.,.F.,.F.,.F.,(4,4),(4,4),(0.522097120209954,
1.00286753160118),(0.0166015299239876,0.0231736788075223),.UNSPECIFIED.);
#3173=B_SPLINE_SURFACE_WITH_KNOTS('',3,3,((#100224,#100225,#100226,#100227),
(#100228,#100229,#100230,#100231),(#100232,#100233,#100234,#100235),(#100236,
#100237,#100238,#100239)),.UNSPECIFIED.,.F.,.F.,.F.,(4,4),(4,4),(0.,1.00600003961382),
(0.0166015299239891,0.0265907346180641),.UNSPECIFIED.);
#3174=B_SPLINE_SURFACE_WITH_KNOTS('',3,3,((#100240,#100241,#100242,#100243),
(#100244,#100245,#100246,#100247),(#100248,#100249,#100250,#100251),(#100252,
#100253,#100254,#100255)),.UNSPECIFIED.,.F.,.F.,.F.,(4,4),(4,4),(-0.0028686220116151,
0.47790287979179),(0.0300094532292791,0.0365944846647015),.UNSPECIFIED.);
#3175=B_SPLINE_SURFACE_WITH_KNOTS('',3,3,((#100257,#100258,#100259,#100260),
(#100261,#100262,#100263,#100264),(#100265,#100266,#100267,#100268),(#100269,
#100270,#100271,#100272)),.UNSPECIFIED.,.F.,.F.,.F.,(4,4),(4,4),(0.522097120209979,
1.00286823669287),(0.0265907346180633,0.0331702036051745),.UNSPECIFIED.);
#3176=B_SPLINE_SURFACE_WITH_KNOTS('',3,3,((#100280,#100281,#100282,#100283),
(#100284,#100285,#100286,#100287),(#100288,#100289,#100290,#100291),(#100292,
#100293,#100294,#100295)),.UNSPECIFIED.,.F.,.F.,.F.,(4,4),(4,4),(-0.00286848453309324,
0.477902879790285),(0.0400218729466604,0.0466073985929427),
 .UNSPECIFIED.);
#3177=B_SPLINE_SURFACE_WITH_KNOTS('',3,3,((#100312,#100313,#100314,#100315),
(#100316,#100317,#100318,#100319),(#100320,#100321,#100322,#100323),(#100324,
#100325,#100326,#100327)),.UNSPECIFIED.,.F.,.F.,.F.,(4,4),(4,4),(0.,1.0060001463973),
(0.0365944846645066,0.0466073985929166),.UNSPECIFIED.);
#3178=B_SPLINE_SURFACE_WITH_KNOTS('',3,3,((#100328,#100329,#100330,#100331),
(#100332,#100333,#100334,#100335),(#100336,#100337,#100338,#100339),(#100340,
#100341,#100342,#100343)),.UNSPECIFIED.,.F.,.F.,.F.,(4,4),(4,4),(-0.00286780122440643,
0.47790287978969),(0.0500263550859002,0.0565997133101408),.UNSPECIFIED.);
#3179=B_SPLINE_SURFACE_WITH_KNOTS('',3,3,((#100345,#100346,#100347,#100348),
(#100349,#100350,#100351,#100352),(#100353,#100354,#100355,#100356),(#100357,
#100358,#100359,#100360)),.UNSPECIFIED.,.F.,.F.,.F.,(4,4),(4,4),(0.522097120210187,
1.00286810177275),(0.0466073985929441,0.0531834933545499),.UNSPECIFIED.);
#3180=B_SPLINE_SURFACE_WITH_KNOTS('',3,3,((#100368,#100369,#100370,#100371),
(#100372,#100373,#100374,#100375),(#100376,#100377,#100378,#100379),(#100380,
#100381,#100382,#100383)),.UNSPECIFIED.,.F.,.F.,.F.,(4,4),(4,4),(-0.0028679259889732,
0.477902879789529),(0.060015686549459,0.0665898698871156),.UNSPECIFIED.);
#3181=B_SPLINE_SURFACE_WITH_KNOTS('',3,3,((#100385,#100386,#100387,#100388),
(#100389,#100390,#100391,#100392),(#100393,#100394,#100395,#100396),(#100397,
#100398,#100399,#100400)),.UNSPECIFIED.,.F.,.F.,.F.,(4,4),(4,4),(0.52209712021033,
1.00286764392038),(0.0565997133101414,0.0631721430887063),.UNSPECIFIED.);
#3182=B_SPLINE_SURFACE_WITH_KNOTS('',3,3,((#100416,#100417,#100418,#100419),
(#100420,#100421,#100422,#100423),(#100424,#100425,#100426,#100427),(#100428,
#100429,#100430,#100431)),.UNSPECIFIED.,.F.,.F.,.F.,(4,4),(4,4),(0.522097120209495,
1.00286833998592),(0.0665898698871184,0.0731716198748455),.UNSPECIFIED.);
#3183=B_SPLINE_SURFACE_WITH_KNOTS('',3,3,((#100432,#100433,#100434,#100435),
(#100436,#100437,#100438,#100439),(#100440,#100441,#100442,#100443),(#100444,
#100445,#100446,#100447)),.UNSPECIFIED.,.F.,.F.,.F.,(4,4),(4,4),(-0.00124731532101882,
0.209045111668745),(0.0700194292965496,0.0749900982976448),
 .UNSPECIFIED.);
#3184=B_SPLINE_SURFACE_WITH_KNOTS('',3,3,((#100454,#100455,#100456,#100457),
(#100458,#100459,#100460,#100461),(#100462,#100463,#100464,#100465),(#100466,
#100467,#100468,#100469)),.UNSPECIFIED.,.F.,.F.,.F.,(4,4),(4,4),(-0.00286791014421451,
0.477902879790404),(0.0100271466769357,0.0166015299239858),
 .UNSPECIFIED.);
#3185=B_SPLINE_SURFACE_WITH_KNOTS('',3,3,((#100471,#100472,#100473,#100474),
(#100475,#100476,#100477,#100478),(#100479,#100480,#100481,#100482),(#100483,
#100484,#100485,#100486)),.UNSPECIFIED.,.F.,.F.,.F.,(4,4),(4,4),(0.653230271507083,
1.0020690189263),(0.0065678839538247,0.0131849432429598),.UNSPECIFIED.);
#3186=B_SPLINE_SURFACE_WITH_KNOTS('',3,3,((#100494,#100495,#100496,#100497),
(#100498,#100499,#100500,#100501),(#100502,#100503,#100504,#100505),(#100506,
#100507,#100508,#100509)),.UNSPECIFIED.,.F.,.F.,.F.,(4,4),(4,4),(-0.00286780410473929,
0.477902879790195),(0.0200175229646904,0.0265907346180615),
 .UNSPECIFIED.);
#3187=B_SPLINE_SURFACE_WITH_KNOTS('',3,3,((#100511,#100512,#100513,#100514),
(#100515,#100516,#100517,#100518),(#100519,#100520,#100521,#100522),(#100523,
#100524,#100525,#100526)),.UNSPECIFIED.,.F.,.F.,.F.,(4,4),(4,4),(0.522097120209717,
1.00286753160124),(0.0166015299239884,0.023173678807522),.UNSPECIFIED.);
#3188=B_SPLINE_SURFACE_WITH_KNOTS('',3,3,((#100528,#100529,#100530,#100531),
(#100532,#100533,#100534,#100535),(#100536,#100537,#100538,#100539),(#100540,
#100541,#100542,#100543)),.UNSPECIFIED.,.F.,.F.,.F.,(4,4),(4,4),(0.,1.00600003961404),
(0.0166015299239892,0.0265907346180639),.UNSPECIFIED.);
#3189=B_SPLINE_SURFACE_WITH_KNOTS('',3,3,((#100544,#100545,#100546,#100547),
(#100548,#100549,#100550,#100551),(#100552,#100553,#100554,#100555),(#100556,
#100557,#100558,#100559)),.UNSPECIFIED.,.F.,.F.,.F.,(4,4),(4,4),(-0.00286862201162821,
0.4779028797919),(0.0300094532292786,0.0365944846647022),.UNSPECIFIED.);
#3190=B_SPLINE_SURFACE_WITH_KNOTS('',3,3,((#100561,#100562,#100563,#100564),
(#100565,#100566,#100567,#100568),(#100569,#100570,#100571,#100572),(#100573,
#100574,#100575,#100576)),.UNSPECIFIED.,.F.,.F.,.F.,(4,4),(4,4),(0.522097120210013,
1.00286823669283),(0.0265907346180632,0.0331702036889939),.UNSPECIFIED.);
#3191=B_SPLINE_SURFACE_WITH_KNOTS('',3,3,((#100584,#100585,#100586,#100587),
(#100588,#100589,#100590,#100591),(#100592,#100593,#100594,#100595),(#100596,
#100597,#100598,#100599)),.UNSPECIFIED.,.F.,.F.,.F.,(4,4),(4,4),(-0.002868484533028,
0.477902879790492),(0.0400218729466594,0.0466073985929433),
 .UNSPECIFIED.);
#3192=B_SPLINE_SURFACE_WITH_KNOTS('',3,3,((#100616,#100617,#100618,#100619),
(#100620,#100621,#100622,#100623),(#100624,#100625,#100626,#100627),(#100628,
#100629,#100630,#100631)),.UNSPECIFIED.,.F.,.F.,.F.,(4,4),(4,4),(0.,1.00600014639751),
(0.0365944846645073,0.0466073985929175),.UNSPECIFIED.);
#3193=B_SPLINE_SURFACE_WITH_KNOTS('',3,3,((#100632,#100633,#100634,#100635),
(#100636,#100637,#100638,#100639),(#100640,#100641,#100642,#100643),(#100644,
#100645,#100646,#100647)),.UNSPECIFIED.,.F.,.F.,.F.,(4,4),(4,4),(-0.00286780122436653,
0.477902879789868),(0.0500263550858999,0.0565997133101414),
 .UNSPECIFIED.);
#3194=B_SPLINE_SURFACE_WITH_KNOTS('',3,3,((#100649,#100650,#100651,#100652),
(#100653,#100654,#100655,#100656),(#100657,#100658,#100659,#100660),(#100661,
#100662,#100663,#100664)),.UNSPECIFIED.,.F.,.F.,.F.,(4,4),(4,4),(0.522097120210068,
1.00286810177241),(0.0466073985929445,0.0531834925888927),.UNSPECIFIED.);
#3195=B_SPLINE_SURFACE_WITH_KNOTS('',3,3,((#100672,#100673,#100674,#100675),
(#100676,#100677,#100678,#100679),(#100680,#100681,#100682,#100683),(#100684,
#100685,#100686,#100687)),.UNSPECIFIED.,.F.,.F.,.F.,(4,4),(4,4),(-0.0028679259889283,
0.477902879789711),(0.0600156865494596,0.0665898698871177),
 .UNSPECIFIED.);
#3196=B_SPLINE_SURFACE_WITH_KNOTS('',3,3,((#100689,#100690,#100691,#100692),
(#100693,#100694,#100695,#100696),(#100697,#100698,#100699,#100700),(#100701,
#100702,#100703,#100704)),.UNSPECIFIED.,.F.,.F.,.F.,(4,4),(4,4),(0.522097120210247,
1.00286764392036),(0.0565997133101416,0.0631721430887064),.UNSPECIFIED.);
#3197=B_SPLINE_SURFACE_WITH_KNOTS('',3,3,((#100720,#100721,#100722,#100723),
(#100724,#100725,#100726,#100727),(#100728,#100729,#100730,#100731),(#100732,
#100733,#100734,#100735)),.UNSPECIFIED.,.F.,.F.,.F.,(4,4),(4,4),(0.522097120209502,
1.00286833998601),(0.0665898698871197,0.0731716198748448),.UNSPECIFIED.);
#3198=B_SPLINE_SURFACE_WITH_KNOTS('',3,3,((#100736,#100737,#100738,#100739),
(#100740,#100741,#100742,#100743),(#100744,#100745,#100746,#100747),(#100748,
#100749,#100750,#100751)),.UNSPECIFIED.,.F.,.F.,.F.,(4,4),(4,4),(-0.00124731532100415,
0.209045111668643),(0.0700194292965383,0.0749900982976484),
 .UNSPECIFIED.);
#3199=B_SPLINE_SURFACE_WITH_KNOTS('',3,3,((#100758,#100759,#100760,#100761),
(#100762,#100763,#100764,#100765),(#100766,#100767,#100768,#100769),(#100770,
#100771,#100772,#100773)),.UNSPECIFIED.,.F.,.F.,.F.,(4,4),(4,4),(-0.00286791014416191,
0.477902879790526),(0.0100271466769333,0.016601529923987),.UNSPECIFIED.);
#3200=B_SPLINE_SURFACE_WITH_KNOTS('',3,3,((#100775,#100776,#100777,#100778),
(#100779,#100780,#100781,#100782),(#100783,#100784,#100785,#100786),(#100787,
#100788,#100789,#100790)),.UNSPECIFIED.,.F.,.F.,.F.,(4,4),(4,4),(0.65323027150715,
1.0020690189263),(0.00656788395383221,0.0131849432429627),.UNSPECIFIED.);
#3201=B_SPLINE_SURFACE_WITH_KNOTS('',3,3,((#100798,#100799,#100800,#100801),
(#100802,#100803,#100804,#100805),(#100806,#100807,#100808,#100809),(#100810,
#100811,#100812,#100813)),.UNSPECIFIED.,.F.,.F.,.F.,(4,4),(4,4),(-0.00286780410472678,
0.47790287979035),(0.0200175229646902,0.0265907346180624),.UNSPECIFIED.);
#3202=B_SPLINE_SURFACE_WITH_KNOTS('',3,3,((#100815,#100816,#100817,#100818),
(#100819,#100820,#100821,#100822),(#100823,#100824,#100825,#100826),(#100827,
#100828,#100829,#100830)),.UNSPECIFIED.,.F.,.F.,.F.,(4,4),(4,4),(0.522097120209711,
1.00286753160107),(0.0166015299239882,0.0231736788075225),.UNSPECIFIED.);
#3203=B_SPLINE_SURFACE_WITH_KNOTS('',3,3,((#100832,#100833,#100834,#100835),
(#100836,#100837,#100838,#100839),(#100840,#100841,#100842,#100843),(#100844,
#100845,#100846,#100847)),.UNSPECIFIED.,.F.,.F.,.F.,(4,4),(4,4),(0.,1.00600003961419),
(0.0166015299239868,0.0265907346180623),.UNSPECIFIED.);
#3204=B_SPLINE_SURFACE_WITH_KNOTS('',3,3,((#100848,#100849,#100850,#100851),
(#100852,#100853,#100854,#100855),(#100856,#100857,#100858,#100859),(#100860,
#100861,#100862,#100863)),.UNSPECIFIED.,.F.,.F.,.F.,(4,4),(4,4),(-0.00286862201159017,
0.477902879792073),(0.0300094532292792,0.036594484664702),.UNSPECIFIED.);
#3205=B_SPLINE_SURFACE_WITH_KNOTS('',3,3,((#100865,#100866,#100867,#100868),
(#100869,#100870,#100871,#100872),(#100873,#100874,#100875,#100876),(#100877,
#100878,#100879,#100880)),.UNSPECIFIED.,.F.,.F.,.F.,(4,4),(4,4),(0.522097120209888,
1.00286823669285),(0.0265907346180635,0.0331702036889926),.UNSPECIFIED.);
#3206=B_SPLINE_SURFACE_WITH_KNOTS('',3,3,((#100888,#100889,#100890,#100891),
(#100892,#100893,#100894,#100895),(#100896,#100897,#100898,#100899),(#100900,
#100901,#100902,#100903)),.UNSPECIFIED.,.F.,.F.,.F.,(4,4),(4,4),(-0.00286848453299057,
0.477902879790606),(0.0400218729466602,0.0466073985929431),
 .UNSPECIFIED.);
#3207=B_SPLINE_SURFACE_WITH_KNOTS('',3,3,((#100920,#100921,#100922,#100923),
(#100924,#100925,#100926,#100927),(#100928,#100929,#100930,#100931),(#100932,
#100933,#100934,#100935)),.UNSPECIFIED.,.F.,.F.,.F.,(4,4),(4,4),(0.,1.00600014639753),
(0.0365944846645068,0.0466073985929167),.UNSPECIFIED.);
#3208=B_SPLINE_SURFACE_WITH_KNOTS('',3,3,((#100936,#100937,#100938,#100939),
(#100940,#100941,#100942,#100943),(#100944,#100945,#100946,#100947),(#100948,
#100949,#100950,#100951)),.UNSPECIFIED.,.F.,.F.,.F.,(4,4),(4,4),(-0.00286780122431204,
0.477902879789971),(0.0500263550858996,0.0565997133101401),
 .UNSPECIFIED.);
#3209=B_SPLINE_SURFACE_WITH_KNOTS('',3,3,((#100953,#100954,#100955,#100956),
(#100957,#100958,#100959,#100960),(#100961,#100962,#100963,#100964),(#100965,
#100966,#100967,#100968)),.UNSPECIFIED.,.F.,.F.,.F.,(4,4),(4,4),(0.522097120209995,
1.00286810177248),(0.0466073985929453,0.0531834925888927),.UNSPECIFIED.);
#3210=B_SPLINE_SURFACE_WITH_KNOTS('',3,3,((#100976,#100977,#100978,#100979),
(#100980,#100981,#100982,#100983),(#100984,#100985,#100986,#100987),(#100988,
#100989,#100990,#100991)),.UNSPECIFIED.,.F.,.F.,.F.,(4,4),(4,4),(-0.00286792598893965,
0.477902879789888),(0.0600156865494596,0.0665898698871179),
 .UNSPECIFIED.);
#3211=B_SPLINE_SURFACE_WITH_KNOTS('',3,3,((#100993,#100994,#100995,#100996),
(#100997,#100998,#100999,#101000),(#101001,#101002,#101003,#101004),(#101005,
#101006,#101007,#101008)),.UNSPECIFIED.,.F.,.F.,.F.,(4,4),(4,4),(0.522097120210143,
1.00286764392032),(0.0565997133101415,0.0631721430887063),.UNSPECIFIED.);
#3212=B_SPLINE_SURFACE_WITH_KNOTS('',3,3,((#101024,#101025,#101026,#101027),
(#101028,#101029,#101030,#101031),(#101032,#101033,#101034,#101035),(#101036,
#101037,#101038,#101039)),.UNSPECIFIED.,.F.,.F.,.F.,(4,4),(4,4),(0.522097120209265,
1.0028683399859),(0.066589869887119,0.0731716198748447),.UNSPECIFIED.);
#3213=B_SPLINE_SURFACE_WITH_KNOTS('',3,3,((#101040,#101041,#101042,#101043),
(#101044,#101045,#101046,#101047),(#101048,#101049,#101050,#101051),(#101052,
#101053,#101054,#101055)),.UNSPECIFIED.,.F.,.F.,.F.,(4,4),(4,4),(-0.00124731532099686,
0.209045111668682),(0.070019429296526,0.0749900982976544),.UNSPECIFIED.);
#3214=B_SPLINE_SURFACE_WITH_KNOTS('',3,3,((#101062,#101063,#101064,#101065),
(#101066,#101067,#101068,#101069),(#101070,#101071,#101072,#101073),(#101074,
#101075,#101076,#101077)),.UNSPECIFIED.,.F.,.F.,.F.,(4,4),(4,4),(-0.00286791014411575,
0.477902879790672),(0.0100271466769346,0.0166015299239877),
 .UNSPECIFIED.);
#3215=B_SPLINE_SURFACE_WITH_KNOTS('',3,3,((#101079,#101080,#101081,#101082),
(#101083,#101084,#101085,#101086),(#101087,#101088,#101089,#101090),(#101091,
#101092,#101093,#101094)),.UNSPECIFIED.,.F.,.F.,.F.,(4,4),(4,4),(0.653230271507093,
1.0020690189263),(0.00656788395384009,0.0131849432430558),.UNSPECIFIED.);
#3216=B_SPLINE_SURFACE_WITH_KNOTS('',3,3,((#101102,#101103,#101104,#101105),
(#101106,#101107,#101108,#101109),(#101110,#101111,#101112,#101113),(#101114,
#101115,#101116,#101117)),.UNSPECIFIED.,.F.,.F.,.F.,(4,4),(4,4),(-0.00286780410468854,
0.477902879790407),(0.0200175229646894,0.0265907346180616),
 .UNSPECIFIED.);
#3217=B_SPLINE_SURFACE_WITH_KNOTS('',3,3,((#101119,#101120,#101121,#101122),
(#101123,#101124,#101125,#101126),(#101127,#101128,#101129,#101130),(#101131,
#101132,#101133,#101134)),.UNSPECIFIED.,.F.,.F.,.F.,(4,4),(4,4),(0.522097120209609,
1.00286753160126),(0.0166015299239883,0.0231736788075222),.UNSPECIFIED.);
#3218=B_SPLINE_SURFACE_WITH_KNOTS('',3,3,((#101136,#101137,#101138,#101139),
(#101140,#101141,#101142,#101143),(#101144,#101145,#101146,#101147),(#101148,
#101149,#101150,#101151)),.UNSPECIFIED.,.F.,.F.,.F.,(4,4),(4,4),(0.,1.00600003961408),
(0.0166015299239858,0.0265907346180616),.UNSPECIFIED.);
#3219=B_SPLINE_SURFACE_WITH_KNOTS('',3,3,((#101152,#101153,#101154,#101155),
(#101156,#101157,#101158,#101159),(#101160,#101161,#101162,#101163),(#101164,
#101165,#101166,#101167)),.UNSPECIFIED.,.F.,.F.,.F.,(4,4),(4,4),(-0.00286862201157823,
0.477902879792094),(0.0300094532292784,0.0365944846647017),
 .UNSPECIFIED.);
#3220=B_SPLINE_SURFACE_WITH_KNOTS('',3,3,((#101169,#101170,#101171,#101172),
(#101173,#101174,#101175,#101176),(#101177,#101178,#101179,#101180),(#101181,
#101182,#101183,#101184)),.UNSPECIFIED.,.F.,.F.,.F.,(4,4),(4,4),(0.522097120209858,
1.00286823669298),(0.0265907346180633,0.033170203688993),.UNSPECIFIED.);
#3221=B_SPLINE_SURFACE_WITH_KNOTS('',3,3,((#101192,#101193,#101194,#101195),
(#101196,#101197,#101198,#101199),(#101200,#101201,#101202,#101203),(#101204,
#101205,#101206,#101207)),.UNSPECIFIED.,.F.,.F.,.F.,(4,4),(4,4),(-0.00286848453291097,
0.47790287979078),(0.0400218729466607,0.0466073985929428),.UNSPECIFIED.);
#3222=B_SPLINE_SURFACE_WITH_KNOTS('',3,3,((#101224,#101225,#101226,#101227),
(#101228,#101229,#101230,#101231),(#101232,#101233,#101234,#101235),(#101236,
#101237,#101238,#101239)),.UNSPECIFIED.,.F.,.F.,.F.,(4,4),(4,4),(0.,1.00600014639742),
(0.0365944846645073,0.0466073985929146),.UNSPECIFIED.);
#3223=B_SPLINE_SURFACE_WITH_KNOTS('',3,3,((#101240,#101241,#101242,#101243),
(#101244,#101245,#101246,#101247),(#101248,#101249,#101250,#101251),(#101252,
#101253,#101254,#101255)),.UNSPECIFIED.,.F.,.F.,.F.,(4,4),(4,4),(-0.00286780122425562,
0.477902879790124),(0.0500263550858987,0.0565997133101411),
 .UNSPECIFIED.);
#3224=B_SPLINE_SURFACE_WITH_KNOTS('',3,3,((#101257,#101258,#101259,#101260),
(#101261,#101262,#101263,#101264),(#101265,#101266,#101267,#101268),(#101269,
#101270,#101271,#101272)),.UNSPECIFIED.,.F.,.F.,.F.,(4,4),(4,4),(0.522097120209903,
1.00286810177251),(0.0466073985929444,0.0531834925888938),.UNSPECIFIED.);
#3225=B_SPLINE_SURFACE_WITH_KNOTS('',3,3,((#101280,#101281,#101282,#101283),
(#101284,#101285,#101286,#101287),(#101288,#101289,#101290,#101291),(#101292,
#101293,#101294,#101295)),.UNSPECIFIED.,.F.,.F.,.F.,(4,4),(4,4),(-0.00286792598893161,
0.477902879789993),(0.0600156865494595,0.0665898698871174),
 .UNSPECIFIED.);
#3226=B_SPLINE_SURFACE_WITH_KNOTS('',3,3,((#101297,#101298,#101299,#101300),
(#101301,#101302,#101303,#101304),(#101305,#101306,#101307,#101308),(#101309,
#101310,#101311,#101312)),.UNSPECIFIED.,.F.,.F.,.F.,(4,4),(4,4),(0.522097120210098,
1.00286764392041),(0.0565997133101421,0.0631721430887063),.UNSPECIFIED.);
#3227=B_SPLINE_SURFACE_WITH_KNOTS('',3,3,((#101328,#101329,#101330,#101331),
(#101332,#101333,#101334,#101335),(#101336,#101337,#101338,#101339),(#101340,
#101341,#101342,#101343)),.UNSPECIFIED.,.F.,.F.,.F.,(4,4),(4,4),(0.522097120209149,
1.00286833998593),(0.0665898698871195,0.0731716198748446),.UNSPECIFIED.);
#3228=B_SPLINE_SURFACE_WITH_KNOTS('',3,3,((#101344,#101345,#101346,#101347),
(#101348,#101349,#101350,#101351),(#101352,#101353,#101354,#101355),(#101356,
#101357,#101358,#101359)),.UNSPECIFIED.,.F.,.F.,.F.,(4,4),(4,4),(-0.0012473153209956,
0.20904511166891),(0.0700194292965164,0.0749900982976622),.UNSPECIFIED.);
#3229=B_SPLINE_SURFACE_WITH_KNOTS('',3,3,((#101366,#101367,#101368,#101369),
(#101370,#101371,#101372,#101373),(#101374,#101375,#101376,#101377),(#101378,
#101379,#101380,#101381)),.UNSPECIFIED.,.F.,.F.,.F.,(4,4),(4,4),(-0.00286791014405807,
0.477902879790714),(0.010027146676934,0.0166015299239858),.UNSPECIFIED.);
#3230=B_SPLINE_SURFACE_WITH_KNOTS('',3,3,((#101383,#101384,#101385,#101386),
(#101387,#101388,#101389,#101390),(#101391,#101392,#101393,#101394),(#101395,
#101396,#101397,#101398)),.UNSPECIFIED.,.F.,.F.,.F.,(4,4),(4,4),(0.653230271507078,
1.00206901892629),(0.00656788395384775,0.0131849432430557),
 .UNSPECIFIED.);
#3231=B_SPLINE_SURFACE_WITH_KNOTS('',3,3,((#101406,#101407,#101408,#101409),
(#101410,#101411,#101412,#101413),(#101414,#101415,#101416,#101417),(#101418,
#101419,#101420,#101421)),.UNSPECIFIED.,.F.,.F.,.F.,(4,4),(4,4),(-0.00286780410470242,
0.477902879790501),(0.0200175229646922,0.0265907346180627),
 .UNSPECIFIED.);
#3232=B_SPLINE_SURFACE_WITH_KNOTS('',3,3,((#101423,#101424,#101425,#101426),
(#101427,#101428,#101429,#101430),(#101431,#101432,#101433,#101434),(#101435,
#101436,#101437,#101438)),.UNSPECIFIED.,.F.,.F.,.F.,(4,4),(4,4),(0.522097120209468,
1.00286753160118),(0.016601529923988,0.0231736788075219),.UNSPECIFIED.);
#3233=B_SPLINE_SURFACE_WITH_KNOTS('',3,3,((#101440,#101441,#101442,#101443),
(#101444,#101445,#101446,#101447),(#101448,#101449,#101450,#101451),(#101452,
#101453,#101454,#101455)),.UNSPECIFIED.,.F.,.F.,.F.,(4,4),(4,4),(0.,1.00600003961353),
(0.0166015299239881,0.0265907346180615),.UNSPECIFIED.);
#3234=B_SPLINE_SURFACE_WITH_KNOTS('',3,3,((#101456,#101457,#101458,#101459),
(#101460,#101461,#101462,#101463),(#101464,#101465,#101466,#101467),(#101468,
#101469,#101470,#101471)),.UNSPECIFIED.,.F.,.F.,.F.,(4,4),(4,4),(-0.00286862201162393,
0.477902879792228),(0.0300094532292793,0.0365944846647173),
 .UNSPECIFIED.);
#3235=B_SPLINE_SURFACE_WITH_KNOTS('',3,3,((#101473,#101474,#101475,#101476),
(#101477,#101478,#101479,#101480),(#101481,#101482,#101483,#101484),(#101485,
#101486,#101487,#101488)),.UNSPECIFIED.,.F.,.F.,.F.,(4,4),(4,4),(0.52209712020978,
1.00286823669302),(0.0265907346180633,0.0331702036889924),.UNSPECIFIED.);
#3236=B_SPLINE_SURFACE_WITH_KNOTS('',3,3,((#101496,#101497,#101498,#101499),
(#101500,#101501,#101502,#101503),(#101504,#101505,#101506,#101507),(#101508,
#101509,#101510,#101511)),.UNSPECIFIED.,.F.,.F.,.F.,(4,4),(4,4),(-0.00286848453286967,
0.477902879790773),(0.0400218729466607,0.0466073985929426),
 .UNSPECIFIED.);
#3237=B_SPLINE_SURFACE_WITH_KNOTS('',3,3,((#101528,#101529,#101530,#101531),
(#101532,#101533,#101534,#101535),(#101536,#101537,#101538,#101539),(#101540,
#101541,#101542,#101543)),.UNSPECIFIED.,.F.,.F.,.F.,(4,4),(4,4),(0.,1.00600014639731),
(0.0365944846645069,0.0466073985929157),.UNSPECIFIED.);
#3238=B_SPLINE_SURFACE_WITH_KNOTS('',3,3,((#101544,#101545,#101546,#101547),
(#101548,#101549,#101550,#101551),(#101552,#101553,#101554,#101555),(#101556,
#101557,#101558,#101559)),.UNSPECIFIED.,.F.,.F.,.F.,(4,4),(4,4),(-0.00286780122421701,
0.477902879790205),(0.0500263550858998,0.0565997133101419),
 .UNSPECIFIED.);
#3239=B_SPLINE_SURFACE_WITH_KNOTS('',3,3,((#101561,#101562,#101563,#101564),
(#101565,#101566,#101567,#101568),(#101569,#101570,#101571,#101572),(#101573,
#101574,#101575,#101576)),.UNSPECIFIED.,.F.,.F.,.F.,(4,4),(4,4),(0.522097120209756,
1.00286810177259),(0.0466073985929451,0.0531834925888926),.UNSPECIFIED.);
#3240=B_SPLINE_SURFACE_WITH_KNOTS('',3,3,((#101584,#101585,#101586,#101587),
(#101588,#101589,#101590,#101591),(#101592,#101593,#101594,#101595),(#101596,
#101597,#101598,#101599)),.UNSPECIFIED.,.F.,.F.,.F.,(4,4),(4,4),(-0.00286792598891565,
0.477902879790097),(0.0600156865494599,0.066589869887118),.UNSPECIFIED.);
#3241=B_SPLINE_SURFACE_WITH_KNOTS('',3,3,((#101601,#101602,#101603,#101604),
(#101605,#101606,#101607,#101608),(#101609,#101610,#101611,#101612),(#101613,
#101614,#101615,#101616)),.UNSPECIFIED.,.F.,.F.,.F.,(4,4),(4,4),(0.52209712020998,
1.00286764392034),(0.0565997133101425,0.0631721430887065),.UNSPECIFIED.);
#3242=B_SPLINE_SURFACE_WITH_KNOTS('',3,3,((#101632,#101633,#101634,#101635),
(#101636,#101637,#101638,#101639),(#101640,#101641,#101642,#101643),(#101644,
#101645,#101646,#101647)),.UNSPECIFIED.,.F.,.F.,.F.,(4,4),(4,4),(0.522097120209037,
1.0028683399859),(0.0665898698871199,0.0731716198748443),.UNSPECIFIED.);
#3243=B_SPLINE_SURFACE_WITH_KNOTS('',3,3,((#101648,#101649,#101650,#101651),
(#101652,#101653,#101654,#101655),(#101656,#101657,#101658,#101659),(#101660,
#101661,#101662,#101663)),.UNSPECIFIED.,.F.,.F.,.F.,(4,4),(4,4),(-0.0012473153210096,
0.209045111670342),(0.0700194292965093,0.0749900982976691),
 .UNSPECIFIED.);
#3244=B_SPLINE_SURFACE_WITH_KNOTS('',3,3,((#101670,#101671,#101672,#101673),
(#101674,#101675,#101676,#101677),(#101678,#101679,#101680,#101681),(#101682,
#101683,#101684,#101685)),.UNSPECIFIED.,.F.,.F.,.F.,(4,4),(4,4),(-0.00286791014400684,
0.477902879790898),(0.0100271466769358,0.0166015299239862),
 .UNSPECIFIED.);
#3245=B_SPLINE_SURFACE_WITH_KNOTS('',3,3,((#101687,#101688,#101689,#101690),
(#101691,#101692,#101693,#101694),(#101695,#101696,#101697,#101698),(#101699,
#101700,#101701,#101702)),.UNSPECIFIED.,.F.,.F.,.F.,(4,4),(4,4),(0.653230271507063,
1.0020690189263),(0.00656788395403927,0.0131849432122613),.UNSPECIFIED.);
#3246=B_SPLINE_SURFACE_WITH_KNOTS('',3,3,((#101710,#101711,#101712,#101713),
(#101714,#101715,#101716,#101717),(#101718,#101719,#101720,#101721),(#101722,
#101723,#101724,#101725)),.UNSPECIFIED.,.F.,.F.,.F.,(4,4),(4,4),(-0.00286780410476689,
0.47790287979065),(0.0200175229646906,0.0265907346180626),.UNSPECIFIED.);
#3247=B_SPLINE_SURFACE_WITH_KNOTS('',3,3,((#101727,#101728,#101729,#101730),
(#101731,#101732,#101733,#101734),(#101735,#101736,#101737,#101738),(#101739,
#101740,#101741,#101742)),.UNSPECIFIED.,.F.,.F.,.F.,(4,4),(4,4),(0.522097120209285,
1.00286753160117),(0.016601529923988,0.0231736788075221),.UNSPECIFIED.);
#3248=B_SPLINE_SURFACE_WITH_KNOTS('',3,3,((#101744,#101745,#101746,#101747),
(#101748,#101749,#101750,#101751),(#101752,#101753,#101754,#101755),(#101756,
#101757,#101758,#101759)),.UNSPECIFIED.,.F.,.F.,.F.,(4,4),(4,4),(0.,1.00600003961394),
(0.0166015299239902,0.0265907346180641),.UNSPECIFIED.);
#3249=B_SPLINE_SURFACE_WITH_KNOTS('',3,3,((#101760,#101761,#101762,#101763),
(#101764,#101765,#101766,#101767),(#101768,#101769,#101770,#101771),(#101772,
#101773,#101774,#101775)),.UNSPECIFIED.,.F.,.F.,.F.,(4,4),(4,4),(-0.00286862201157575,
0.477902879792379),(0.0300094532292789,0.0365944846647167),
 .UNSPECIFIED.);
#3250=B_SPLINE_SURFACE_WITH_KNOTS('',3,3,((#101777,#101778,#101779,#101780),
(#101781,#101782,#101783,#101784),(#101785,#101786,#101787,#101788),(#101789,
#101790,#101791,#101792)),.UNSPECIFIED.,.F.,.F.,.F.,(4,4),(4,4),(0.522097120209556,
1.00286823669293),(0.0265907346180646,0.033170203605174),.UNSPECIFIED.);
#3251=B_SPLINE_SURFACE_WITH_KNOTS('',3,3,((#101800,#101801,#101802,#101803),
(#101804,#101805,#101806,#101807),(#101808,#101809,#101810,#101811),(#101812,
#101813,#101814,#101815)),.UNSPECIFIED.,.F.,.F.,.F.,(4,4),(4,4),(-0.00286848453283359,
0.47790287979088),(0.0400218729466603,0.0466073985929439),.UNSPECIFIED.);
#3252=B_SPLINE_SURFACE_WITH_KNOTS('',3,3,((#101832,#101833,#101834,#101835),
(#101836,#101837,#101838,#101839),(#101840,#101841,#101842,#101843),(#101844,
#101845,#101846,#101847)),.UNSPECIFIED.,.F.,.F.,.F.,(4,4),(4,4),(0.,1.00600014639716),
(0.0365944846645056,0.0466073985929156),.UNSPECIFIED.);
#3253=B_SPLINE_SURFACE_WITH_KNOTS('',3,3,((#101848,#101849,#101850,#101851),
(#101852,#101853,#101854,#101855),(#101856,#101857,#101858,#101859),(#101860,
#101861,#101862,#101863)),.UNSPECIFIED.,.F.,.F.,.F.,(4,4),(4,4),(-0.00286780122415958,
0.477902879790323),(0.0500263550859002,0.0565997133101402),
 .UNSPECIFIED.);
#3254=B_SPLINE_SURFACE_WITH_KNOTS('',3,3,((#101865,#101866,#101867,#101868),
(#101869,#101870,#101871,#101872),(#101873,#101874,#101875,#101876),(#101877,
#101878,#101879,#101880)),.UNSPECIFIED.,.F.,.F.,.F.,(4,4),(4,4),(0.522097120209669,
1.00286810177273),(0.0466073985929445,0.0531834933545507),.UNSPECIFIED.);
#3255=B_SPLINE_SURFACE_WITH_KNOTS('',3,3,((#101888,#101889,#101890,#101891),
(#101892,#101893,#101894,#101895),(#101896,#101897,#101898,#101899),(#101900,
#101901,#101902,#101903)),.UNSPECIFIED.,.F.,.F.,.F.,(4,4),(4,4),(-0.00286792598894784,
0.477902879790276),(0.0600156865494617,0.0665898698871163),
 .UNSPECIFIED.);
#3256=B_SPLINE_SURFACE_WITH_KNOTS('',3,3,((#101905,#101906,#101907,#101908),
(#101909,#101910,#101911,#101912),(#101913,#101914,#101915,#101916),(#101917,
#101918,#101919,#101920)),.UNSPECIFIED.,.F.,.F.,.F.,(4,4),(4,4),(0.522097120209863,
1.00286764392033),(0.0565997133101412,0.0631721430887067),.UNSPECIFIED.);
#3257=B_SPLINE_SURFACE_WITH_KNOTS('',3,3,((#101936,#101937,#101938,#101939),
(#101940,#101941,#101942,#101943),(#101944,#101945,#101946,#101947),(#101948,
#101949,#101950,#101951)),.UNSPECIFIED.,.F.,.F.,.F.,(4,4),(4,4),(0.522097120209008,
1.00286833998591),(0.0665898698871192,0.0731716198748459),.UNSPECIFIED.);
#3258=B_SPLINE_SURFACE_WITH_KNOTS('',3,3,((#101952,#101953,#101954,#101955),
(#101956,#101957,#101958,#101959),(#101960,#101961,#101962,#101963),(#101964,
#101965,#101966,#101967)),.UNSPECIFIED.,.F.,.F.,.F.,(4,4),(4,4),(-0.00124731532103255,
0.209045111672332),(0.0700194292965018,0.0749900982976787),
 .UNSPECIFIED.);
#3259=B_SPLINE_SURFACE_WITH_KNOTS('',3,3,((#101974,#101975,#101976,#101977),
(#101978,#101979,#101980,#101981),(#101982,#101983,#101984,#101985),(#101986,
#101987,#101988,#101989)),.UNSPECIFIED.,.F.,.F.,.F.,(4,4),(4,4),(-0.00286791014398595,
0.477902879790942),(0.0100271466769384,0.0166015299239859),
 .UNSPECIFIED.);
#3260=B_SPLINE_SURFACE_WITH_KNOTS('',3,3,((#101991,#101992,#101993,#101994),
(#101995,#101996,#101997,#101998),(#101999,#102000,#102001,#102002),(#102003,
#102004,#102005,#102006)),.UNSPECIFIED.,.F.,.F.,.F.,(4,4),(4,4),(0.65323027150641,
1.00206901892628),(0.0065678839540488,0.0131849432122596),.UNSPECIFIED.);
#3261=B_SPLINE_SURFACE_WITH_KNOTS('',3,3,((#102014,#102015,#102016,#102017),
(#102018,#102019,#102020,#102021),(#102022,#102023,#102024,#102025),(#102026,
#102027,#102028,#102029)),.UNSPECIFIED.,.F.,.F.,.F.,(4,4),(4,4),(-0.0028678041047262,
0.477902879790764),(0.0200175229646916,0.0265907346180621),
 .UNSPECIFIED.);
#3262=B_SPLINE_SURFACE_WITH_KNOTS('',3,3,((#102031,#102032,#102033,#102034),
(#102035,#102036,#102037,#102038),(#102039,#102040,#102041,#102042),(#102043,
#102044,#102045,#102046)),.UNSPECIFIED.,.F.,.F.,.F.,(4,4),(4,4),(0.522097120209154,
1.00286753160127),(0.0166015299239883,0.0231736788075222),.UNSPECIFIED.);
#3263=B_SPLINE_SURFACE_WITH_KNOTS('',3,3,((#102048,#102049,#102050,#102051),
(#102052,#102053,#102054,#102055),(#102056,#102057,#102058,#102059),(#102060,
#102061,#102062,#102063)),.UNSPECIFIED.,.F.,.F.,.F.,(4,4),(4,4),(0.,1.00600003961365),
(0.016601529923988,0.0265907346180656),.UNSPECIFIED.);
#3264=B_SPLINE_SURFACE_WITH_KNOTS('',3,3,((#102064,#102065,#102066,#102067),
(#102068,#102069,#102070,#102071),(#102072,#102073,#102074,#102075),(#102076,
#102077,#102078,#102079)),.UNSPECIFIED.,.F.,.F.,.F.,(4,4),(4,4),(-0.00286862201160525,
0.477902879792415),(0.0300094532292785,0.0365944846647022),
 .UNSPECIFIED.);
#3265=B_SPLINE_SURFACE_WITH_KNOTS('',3,3,((#102081,#102082,#102083,#102084),
(#102085,#102086,#102087,#102088),(#102089,#102090,#102091,#102092),(#102093,
#102094,#102095,#102096)),.UNSPECIFIED.,.F.,.F.,.F.,(4,4),(4,4),(0.522097120209503,
1.00286823669289),(0.0265907346180636,0.0331702036889927),.UNSPECIFIED.);
#3266=B_SPLINE_SURFACE_WITH_KNOTS('',3,3,((#102104,#102105,#102106,#102107),
(#102108,#102109,#102110,#102111),(#102112,#102113,#102114,#102115),(#102116,
#102117,#102118,#102119)),.UNSPECIFIED.,.F.,.F.,.F.,(4,4),(4,4),(-0.00286848453280808,
0.477902879791013),(0.0400218729466605,0.0466073985929591),
 .UNSPECIFIED.);
#3267=B_SPLINE_SURFACE_WITH_KNOTS('',3,3,((#102136,#102137,#102138,#102139),
(#102140,#102141,#102142,#102143),(#102144,#102145,#102146,#102147),(#102148,
#102149,#102150,#102151)),.UNSPECIFIED.,.F.,.F.,.F.,(4,4),(4,4),(0.,1.00600014639734),
(0.0365944846645064,0.0466073985929166),.UNSPECIFIED.);
#3268=B_SPLINE_SURFACE_WITH_KNOTS('',3,3,((#102152,#102153,#102154,#102155),
(#102156,#102157,#102158,#102159),(#102160,#102161,#102162,#102163),(#102164,
#102165,#102166,#102167)),.UNSPECIFIED.,.F.,.F.,.F.,(4,4),(4,4),(-0.00286780122410264,
0.477902879790367),(0.0500263550859007,0.0565997133101572),
 .UNSPECIFIED.);
#3269=B_SPLINE_SURFACE_WITH_KNOTS('',3,3,((#102169,#102170,#102171,#102172),
(#102173,#102174,#102175,#102176),(#102177,#102178,#102179,#102180),(#102181,
#102182,#102183,#102184)),.UNSPECIFIED.,.F.,.F.,.F.,(4,4),(4,4),(0.522097120209639,
1.00286810177254),(0.0466073985929443,0.0531834925888932),.UNSPECIFIED.);
#3270=B_SPLINE_SURFACE_WITH_KNOTS('',3,3,((#102192,#102193,#102194,#102195),
(#102196,#102197,#102198,#102199),(#102200,#102201,#102202,#102203),(#102204,
#102205,#102206,#102207)),.UNSPECIFIED.,.F.,.F.,.F.,(4,4),(4,4),(-0.00286792598890457,
0.477902879790256),(0.0600156865494609,0.0665898698871165),
 .UNSPECIFIED.);
#3271=B_SPLINE_SURFACE_WITH_KNOTS('',3,3,((#102209,#102210,#102211,#102212),
(#102213,#102214,#102215,#102216),(#102217,#102218,#102219,#102220),(#102221,
#102222,#102223,#102224)),.UNSPECIFIED.,.F.,.F.,.F.,(4,4),(4,4),(0.522097120209762,
1.0028676439204),(0.0565997133101423,0.063172143088706),.UNSPECIFIED.);
#3272=B_SPLINE_SURFACE_WITH_KNOTS('',3,3,((#102240,#102241,#102242,#102243),
(#102244,#102245,#102246,#102247),(#102248,#102249,#102250,#102251),(#102252,
#102253,#102254,#102255)),.UNSPECIFIED.,.F.,.F.,.F.,(4,4),(4,4),(0.522097120208856,
1.00286833998579),(0.0665898698871195,0.0731716198748446),.UNSPECIFIED.);
#3273=B_SPLINE_SURFACE_WITH_KNOTS('',3,3,((#102256,#102257,#102258,#102259),
(#102260,#102261,#102262,#102263),(#102264,#102265,#102266,#102267),(#102268,
#102269,#102270,#102271)),.UNSPECIFIED.,.F.,.F.,.F.,(4,4),(4,4),(-0.00124731532103141,
0.209045111674401),(0.0700194292964963,0.0749900982976873),
 .UNSPECIFIED.);
#3274=B_SPLINE_SURFACE_WITH_KNOTS('',3,3,((#102278,#102279,#102280,#102281),
(#102282,#102283,#102284,#102285),(#102286,#102287,#102288,#102289),(#102290,
#102291,#102292,#102293)),.UNSPECIFIED.,.F.,.F.,.F.,(4,4),(4,4),(-0.00286791014392198,
0.477902879791072),(0.0100271466769366,0.0166015299239864),
 .UNSPECIFIED.);
#3275=B_SPLINE_SURFACE_WITH_KNOTS('',3,3,((#102295,#102296,#102297,#102298),
(#102299,#102300,#102301,#102302),(#102303,#102304,#102305,#102306),(#102307,
#102308,#102309,#102310)),.UNSPECIFIED.,.F.,.F.,.F.,(4,4),(4,4),(0.653230271505284,
1.00206901892634),(0.00656788395387369,0.0131849432430505),
 .UNSPECIFIED.);
#3276=B_SPLINE_SURFACE_WITH_KNOTS('',3,3,((#102318,#102319,#102320,#102321),
(#102322,#102323,#102324,#102325),(#102326,#102327,#102328,#102329),(#102330,
#102331,#102332,#102333)),.UNSPECIFIED.,.F.,.F.,.F.,(4,4),(4,4),(-0.00286780410477936,
0.477902879790937),(0.0200175229646911,0.0265907346180616),
 .UNSPECIFIED.);
#3277=B_SPLINE_SURFACE_WITH_KNOTS('',3,3,((#102335,#102336,#102337,#102338),
(#102339,#102340,#102341,#102342),(#102343,#102344,#102345,#102346),(#102347,
#102348,#102349,#102350)),.UNSPECIFIED.,.F.,.F.,.F.,(4,4),(4,4),(0.522097120209068,
1.00286753160119),(0.0166015299239897,0.0231736788075218),.UNSPECIFIED.);
#3278=B_SPLINE_SURFACE_WITH_KNOTS('',3,3,((#102352,#102353,#102354,#102355),
(#102356,#102357,#102358,#102359),(#102360,#102361,#102362,#102363),(#102364,
#102365,#102366,#102367)),.UNSPECIFIED.,.F.,.F.,.F.,(4,4),(4,4),(0.,1.0060000396133),
(0.016601529923988,0.026590734618064),.UNSPECIFIED.);
#3279=B_SPLINE_SURFACE_WITH_KNOTS('',3,3,((#102368,#102369,#102370,#102371),
(#102372,#102373,#102374,#102375),(#102376,#102377,#102378,#102379),(#102380,
#102381,#102382,#102383)),.UNSPECIFIED.,.F.,.F.,.F.,(4,4),(4,4),(-0.00286862201155799,
0.477902879792543),(0.030009453229278,0.0365944846647016),.UNSPECIFIED.);
#3280=B_SPLINE_SURFACE_WITH_KNOTS('',3,3,((#102385,#102386,#102387,#102388),
(#102389,#102390,#102391,#102392),(#102393,#102394,#102395,#102396),(#102397,
#102398,#102399,#102400)),.UNSPECIFIED.,.F.,.F.,.F.,(4,4),(4,4),(0.522097120209334,
1.0028682366929),(0.0265907346180635,0.0331702036051743),.UNSPECIFIED.);
#3281=B_SPLINE_SURFACE_WITH_KNOTS('',3,3,((#102408,#102409,#102410,#102411),
(#102412,#102413,#102414,#102415),(#102416,#102417,#102418,#102419),(#102420,
#102421,#102422,#102423)),.UNSPECIFIED.,.F.,.F.,.F.,(4,4),(4,4),(-0.00286848453275135,
0.47790287979121),(0.0400218729466611,0.046607398592943),.UNSPECIFIED.);
#3282=B_SPLINE_SURFACE_WITH_KNOTS('',3,3,((#102440,#102441,#102442,#102443),
(#102444,#102445,#102446,#102447),(#102448,#102449,#102450,#102451),(#102452,
#102453,#102454,#102455)),.UNSPECIFIED.,.F.,.F.,.F.,(4,4),(4,4),(0.,1.00600014639758),
(0.0365944846645051,0.0466073985929177),.UNSPECIFIED.);
#3283=B_SPLINE_SURFACE_WITH_KNOTS('',3,3,((#102456,#102457,#102458,#102459),
(#102460,#102461,#102462,#102463),(#102464,#102465,#102466,#102467),(#102468,
#102469,#102470,#102471)),.UNSPECIFIED.,.F.,.F.,.F.,(4,4),(4,4),(-0.0028678012240823,
0.477902879790518),(0.0500263550859009,0.0565997133101415),
 .UNSPECIFIED.);
#3284=B_SPLINE_SURFACE_WITH_KNOTS('',3,3,((#102473,#102474,#102475,#102476),
(#102477,#102478,#102479,#102480),(#102481,#102482,#102483,#102484),(#102485,
#102486,#102487,#102488)),.UNSPECIFIED.,.F.,.F.,.F.,(4,4),(4,4),(0.522097120209443,
1.00286810177263),(0.0466073985929449,0.0531834925888939),.UNSPECIFIED.);
#3285=B_SPLINE_SURFACE_WITH_KNOTS('',3,3,((#102496,#102497,#102498,#102499),
(#102500,#102501,#102502,#102503),(#102504,#102505,#102506,#102507),(#102508,
#102509,#102510,#102511)),.UNSPECIFIED.,.F.,.F.,.F.,(4,4),(4,4),(-0.00286792598893081,
0.477902879790381),(0.0600156865494602,0.0665898698871173),
 .UNSPECIFIED.);
#3286=B_SPLINE_SURFACE_WITH_KNOTS('',3,3,((#102513,#102514,#102515,#102516),
(#102517,#102518,#102519,#102520),(#102521,#102522,#102523,#102524),(#102525,
#102526,#102527,#102528)),.UNSPECIFIED.,.F.,.F.,.F.,(4,4),(4,4),(0.522097120209564,
1.00286764392037),(0.0565997133101422,0.0631721430887063),.UNSPECIFIED.);
#3287=B_SPLINE_SURFACE_WITH_KNOTS('',3,3,((#102544,#102545,#102546,#102547),
(#102548,#102549,#102550,#102551),(#102552,#102553,#102554,#102555),(#102556,
#102557,#102558,#102559)),.UNSPECIFIED.,.F.,.F.,.F.,(4,4),(4,4),(0.522097120208792,
1.0028683399858),(0.0665898698871198,0.0731716198748449),.UNSPECIFIED.);
#3288=B_SPLINE_SURFACE_WITH_KNOTS('',3,3,((#102560,#102561,#102562,#102563),
(#102564,#102565,#102566,#102567),(#102568,#102569,#102570,#102571),(#102572,
#102573,#102574,#102575)),.UNSPECIFIED.,.F.,.F.,.F.,(4,4),(4,4),(-0.00124731532103917,
0.209045111676822),(0.0700194292964934,0.0749900982976999),
 .UNSPECIFIED.);
#3289=B_SPLINE_SURFACE_WITH_KNOTS('',3,3,((#102582,#102583,#102584,#102585),
(#102586,#102587,#102588,#102589),(#102590,#102591,#102592,#102593),(#102594,
#102595,#102596,#102597)),.UNSPECIFIED.,.F.,.F.,.F.,(4,4),(4,4),(-0.00286791014392413,
0.477902879791187),(0.0100271466769363,0.0166015299239868),
 .UNSPECIFIED.);
#3290=B_SPLINE_SURFACE_WITH_KNOTS('',3,3,((#102599,#102600,#102601,#102602),
(#102603,#102604,#102605,#102606),(#102607,#102608,#102609,#102610),(#102611,
#102612,#102613,#102614)),.UNSPECIFIED.,.F.,.F.,.F.,(4,4),(4,4),(0.653230271504036,
1.00206901892632),(0.0065678839538812,0.0131849432430442),.UNSPECIFIED.);
#3291=B_SPLINE_SURFACE_WITH_KNOTS('',3,3,((#102622,#102623,#102624,#102625),
(#102626,#102627,#102628,#102629),(#102630,#102631,#102632,#102633),(#102634,
#102635,#102636,#102637)),.UNSPECIFIED.,.F.,.F.,.F.,(4,4),(4,4),(-0.0028678041048232,
0.477902879791045),(0.0200175229646908,0.0265907346180622),
 .UNSPECIFIED.);
#3292=B_SPLINE_SURFACE_WITH_KNOTS('',3,3,((#102639,#102640,#102641,#102642),
(#102643,#102644,#102645,#102646),(#102647,#102648,#102649,#102650),(#102651,
#102652,#102653,#102654)),.UNSPECIFIED.,.F.,.F.,.F.,(4,4),(4,4),(0.522097120208956,
1.00286753160116),(0.0166015299239884,0.0231736788037111),.UNSPECIFIED.);
#3293=B_SPLINE_SURFACE_WITH_KNOTS('',3,3,((#102656,#102657,#102658,#102659),
(#102660,#102661,#102662,#102663),(#102664,#102665,#102666,#102667),(#102668,
#102669,#102670,#102671)),.UNSPECIFIED.,.F.,.F.,.F.,(4,4),(4,4),(0.,1.00600003961301),
(0.0166015299239882,0.0265907346180623),.UNSPECIFIED.);
#3294=B_SPLINE_SURFACE_WITH_KNOTS('',3,3,((#102672,#102673,#102674,#102675),
(#102676,#102677,#102678,#102679),(#102680,#102681,#102682,#102683),(#102684,
#102685,#102686,#102687)),.UNSPECIFIED.,.F.,.F.,.F.,(4,4),(4,4),(-0.00286862201159097,
0.477902879792634),(0.0300094532292799,0.0365944846647021),
 .UNSPECIFIED.);
#3295=B_SPLINE_SURFACE_WITH_KNOTS('',3,3,((#102689,#102690,#102691,#102692),
(#102693,#102694,#102695,#102696),(#102697,#102698,#102699,#102700),(#102701,
#102702,#102703,#102704)),.UNSPECIFIED.,.F.,.F.,.F.,(4,4),(4,4),(0.522097120209135,
1.00286823669292),(0.026590734618064,0.0331702036622762),.UNSPECIFIED.);
#3296=B_SPLINE_SURFACE_WITH_KNOTS('',3,3,((#102712,#102713,#102714,#102715),
(#102716,#102717,#102718,#102719),(#102720,#102721,#102722,#102723),(#102724,
#102725,#102726,#102727)),.UNSPECIFIED.,.F.,.F.,.F.,(4,4),(4,4),(-0.00286848453271382,
0.477902879791247),(0.0400218729466601,0.0466073985929429),
 .UNSPECIFIED.);
#3297=B_SPLINE_SURFACE_WITH_KNOTS('',3,3,((#102744,#102745,#102746,#102747),
(#102748,#102749,#102750,#102751),(#102752,#102753,#102754,#102755),(#102756,
#102757,#102758,#102759)),.UNSPECIFIED.,.F.,.F.,.F.,(4,4),(4,4),(0.,1.00600014639707),
(0.0365944846645049,0.0466073985929167),.UNSPECIFIED.);
#3298=B_SPLINE_SURFACE_WITH_KNOTS('',3,3,((#102760,#102761,#102762,#102763),
(#102764,#102765,#102766,#102767),(#102768,#102769,#102770,#102771),(#102772,
#102773,#102774,#102775)),.UNSPECIFIED.,.F.,.F.,.F.,(4,4),(4,4),(-0.00286780122400802,
0.477902879790596),(0.0500263550859,0.0565997133101411),.UNSPECIFIED.);
#3299=B_SPLINE_SURFACE_WITH_KNOTS('',3,3,((#102777,#102778,#102779,#102780),
(#102781,#102782,#102783,#102784),(#102785,#102786,#102787,#102788),(#102789,
#102790,#102791,#102792)),.UNSPECIFIED.,.F.,.F.,.F.,(4,4),(4,4),(0.522097120209334,
1.00286810177245),(0.0466073985929444,0.0531834922865668),.UNSPECIFIED.);
#3300=B_SPLINE_SURFACE_WITH_KNOTS('',3,3,((#102800,#102801,#102802,#102803),
(#102804,#102805,#102806,#102807),(#102808,#102809,#102810,#102811),(#102812,
#102813,#102814,#102815)),.UNSPECIFIED.,.F.,.F.,.F.,(4,4),(4,4),(-0.00286792598892004,
0.477902879790578),(0.0600156865494608,0.0665898698871175),
 .UNSPECIFIED.);
#3301=B_SPLINE_SURFACE_WITH_KNOTS('',3,3,((#102817,#102818,#102819,#102820),
(#102821,#102822,#102823,#102824),(#102825,#102826,#102827,#102828),(#102829,
#102830,#102831,#102832)),.UNSPECIFIED.,.F.,.F.,.F.,(4,4),(4,4),(0.522097120209435,
1.00286764392035),(0.0565997133101424,0.0631721430887057),.UNSPECIFIED.);
#3302=B_SPLINE_SURFACE_WITH_KNOTS('',3,3,((#102848,#102849,#102850,#102851),
(#102852,#102853,#102854,#102855),(#102856,#102857,#102858,#102859),(#102860,
#102861,#102862,#102863)),.UNSPECIFIED.,.F.,.F.,.F.,(4,4),(4,4),(0.522097120208655,
1.00286833998586),(0.0665898698871185,0.073171619874845),.UNSPECIFIED.);
#3303=B_SPLINE_SURFACE_WITH_KNOTS('',3,3,((#102864,#102865,#102866,#102867),
(#102868,#102869,#102870,#102871),(#102872,#102873,#102874,#102875),(#102876,
#102877,#102878,#102879)),.UNSPECIFIED.,.F.,.F.,.F.,(4,4),(4,4),(-0.00124731532105724,
0.209045111679254),(0.0700194292964913,0.0749900982977112),
 .UNSPECIFIED.);
#3304=B_SPLINE_SURFACE_WITH_KNOTS('',3,3,((#102886,#102887,#102888,#102889),
(#102890,#102891,#102892,#102893),(#102894,#102895,#102896,#102897),(#102898,
#102899,#102900,#102901)),.UNSPECIFIED.,.F.,.F.,.F.,(4,4),(4,4),(-0.0028679101439003,
0.477902879791482),(0.0100271466769351,0.0166015299239872),
 .UNSPECIFIED.);
#3305=B_SPLINE_SURFACE_WITH_KNOTS('',3,3,((#102903,#102904,#102905,#102906),
(#102907,#102908,#102909,#102910),(#102911,#102912,#102913,#102914),(#102915,
#102916,#102917,#102918)),.UNSPECIFIED.,.F.,.F.,.F.,(4,4),(4,4),(0.653230271502744,
1.00206901892634),(0.00656788395388827,0.0131849432430387),
 .UNSPECIFIED.);
#3306=B_SPLINE_SURFACE_WITH_KNOTS('',3,3,((#102926,#102927,#102928,#102929),
(#102930,#102931,#102932,#102933),(#102934,#102935,#102936,#102937),(#102938,
#102939,#102940,#102941)),.UNSPECIFIED.,.F.,.F.,.F.,(4,4),(4,4),(-0.00286780410472799,
0.477902879791192),(0.0200175229646904,0.0265907346180625),
 .UNSPECIFIED.);
#3307=B_SPLINE_SURFACE_WITH_KNOTS('',3,3,((#102943,#102944,#102945,#102946),
(#102947,#102948,#102949,#102950),(#102951,#102952,#102953,#102954),(#102955,
#102956,#102957,#102958)),.UNSPECIFIED.,.F.,.F.,.F.,(4,4),(4,4),(0.522097120208858,
1.00286753160116),(0.0166015299239879,0.0231736787930316),.UNSPECIFIED.);
#3308=B_SPLINE_SURFACE_WITH_KNOTS('',3,3,((#102960,#102961,#102962,#102963),
(#102964,#102965,#102966,#102967),(#102968,#102969,#102970,#102971),(#102972,
#102973,#102974,#102975)),.UNSPECIFIED.,.F.,.F.,.F.,(4,4),(4,4),(0.,1.00600003961341),
(0.0166015299239869,0.0265907346180636),.UNSPECIFIED.);
#3309=B_SPLINE_SURFACE_WITH_KNOTS('',3,3,((#102976,#102977,#102978,#102979),
(#102980,#102981,#102982,#102983),(#102984,#102985,#102986,#102987),(#102988,
#102989,#102990,#102991)),.UNSPECIFIED.,.F.,.F.,.F.,(4,4),(4,4),(-0.00286862201145934,
0.47790287979285),(0.0300094532292789,0.0365944846647005),.UNSPECIFIED.);
#3310=B_SPLINE_SURFACE_WITH_KNOTS('',3,3,((#102993,#102994,#102995,#102996),
(#102997,#102998,#102999,#103000),(#103001,#103002,#103003,#103004),(#103005,
#103006,#103007,#103008)),.UNSPECIFIED.,.F.,.F.,.F.,(4,4),(4,4),(0.52209712020909,
1.00286823669299),(0.0265907346180636,0.0331702036889924),.UNSPECIFIED.);
#3311=B_SPLINE_SURFACE_WITH_KNOTS('',3,3,((#103016,#103017,#103018,#103019),
(#103020,#103021,#103022,#103023),(#103024,#103025,#103026,#103027),(#103028,
#103029,#103030,#103031)),.UNSPECIFIED.,.F.,.F.,.F.,(4,4),(4,4),(-0.00286848453269722,
0.477902879791497),(0.0400218729466593,0.0466073985929421),
 .UNSPECIFIED.);
#3312=B_SPLINE_SURFACE_WITH_KNOTS('',3,3,((#103048,#103049,#103050,#103051),
(#103052,#103053,#103054,#103055),(#103056,#103057,#103058,#103059),(#103060,
#103061,#103062,#103063)),.UNSPECIFIED.,.F.,.F.,.F.,(4,4),(4,4),(0.,1.00600014639748),
(0.0365944846645053,0.0466073985929157),.UNSPECIFIED.);
#3313=B_SPLINE_SURFACE_WITH_KNOTS('',3,3,((#103064,#103065,#103066,#103067),
(#103068,#103069,#103070,#103071),(#103072,#103073,#103074,#103075),(#103076,
#103077,#103078,#103079)),.UNSPECIFIED.,.F.,.F.,.F.,(4,4),(4,4),(-0.00286780122401915,
0.477902879790796),(0.0500263550858998,0.0565997133101412),
 .UNSPECIFIED.);
#3314=B_SPLINE_SURFACE_WITH_KNOTS('',3,3,((#103081,#103082,#103083,#103084),
(#103085,#103086,#103087,#103088),(#103089,#103090,#103091,#103092),(#103093,
#103094,#103095,#103096)),.UNSPECIFIED.,.F.,.F.,.F.,(4,4),(4,4),(0.522097120209233,
1.0028681017726),(0.0466073985929452,0.0531834925888933),.UNSPECIFIED.);
#3315=B_SPLINE_SURFACE_WITH_KNOTS('',3,3,((#103104,#103105,#103106,#103107),
(#103108,#103109,#103110,#103111),(#103112,#103113,#103114,#103115),(#103116,
#103117,#103118,#103119)),.UNSPECIFIED.,.F.,.F.,.F.,(4,4),(4,4),(-0.0028679259889033,
0.477902879790691),(0.0600156865494593,0.0665898698871172),
 .UNSPECIFIED.);
#3316=B_SPLINE_SURFACE_WITH_KNOTS('',3,3,((#103121,#103122,#103123,#103124),
(#103125,#103126,#103127,#103128),(#103129,#103130,#103131,#103132),(#103133,
#103134,#103135,#103136)),.UNSPECIFIED.,.F.,.F.,.F.,(4,4),(4,4),(0.522097120209315,
1.00286764392042),(0.0565997133101412,0.0631721430887057),.UNSPECIFIED.);
#3317=B_SPLINE_SURFACE_WITH_KNOTS('',3,3,((#103152,#103153,#103154,#103155),
(#103156,#103157,#103158,#103159),(#103160,#103161,#103162,#103163),(#103164,
#103165,#103166,#103167)),.UNSPECIFIED.,.F.,.F.,.F.,(4,4),(4,4),(0.522097120208528,
1.00286833998594),(0.0665898698871192,0.0731716198748449),.UNSPECIFIED.);
#3318=B_SPLINE_SURFACE_WITH_KNOTS('',3,3,((#103168,#103169,#103170,#103171),
(#103172,#103173,#103174,#103175),(#103176,#103177,#103178,#103179),(#103180,
#103181,#103182,#103183)),.UNSPECIFIED.,.F.,.F.,.F.,(4,4),(4,4),(-0.00124731532975596,
0.209045111681729),(0.0700194292964918,0.0749900982977222),
 .UNSPECIFIED.);
#3319=B_SPLINE_SURFACE_WITH_KNOTS('',3,3,((#103190,#103191,#103192,#103193),
(#103194,#103195,#103196,#103197),(#103198,#103199,#103200,#103201),(#103202,
#103203,#103204,#103205)),.UNSPECIFIED.,.F.,.F.,.F.,(4,4),(4,4),(-0.00286791014389224,
0.477902879791565),(0.0100271466769338,0.0166015299239867),
 .UNSPECIFIED.);
#3320=B_SPLINE_SURFACE_WITH_KNOTS('',3,3,((#103207,#103208,#103209,#103210),
(#103211,#103212,#103213,#103214),(#103215,#103216,#103217,#103218),(#103219,
#103220,#103221,#103222)),.UNSPECIFIED.,.F.,.F.,.F.,(4,4),(4,4),(0.653230271501317,
1.00206901893493),(0.00656788395389535,0.0131849432430301),
 .UNSPECIFIED.);
#3321=B_SPLINE_SURFACE_WITH_KNOTS('',3,3,((#103230,#103231,#103232,#103233),
(#103234,#103235,#103236,#103237),(#103238,#103239,#103240,#103241),(#103242,
#103243,#103244,#103245)),.UNSPECIFIED.,.F.,.F.,.F.,(4,4),(4,4),(-0.00286780410465671,
0.477902879791354),(0.0200175229646905,0.0265907346180625),
 .UNSPECIFIED.);
#3322=B_SPLINE_SURFACE_WITH_KNOTS('',3,3,((#103247,#103248,#103249,#103250),
(#103251,#103252,#103253,#103254),(#103255,#103256,#103257,#103258),(#103259,
#103260,#103261,#103262)),.UNSPECIFIED.,.F.,.F.,.F.,(4,4),(4,4),(0.522097120208694,
1.00286753160118),(0.0166015299239879,0.023173678803712),.UNSPECIFIED.);
#3323=B_SPLINE_SURFACE_WITH_KNOTS('',3,3,((#103264,#103265,#103266,#103267),
(#103268,#103269,#103270,#103271),(#103272,#103273,#103274,#103275),(#103276,
#103277,#103278,#103279)),.UNSPECIFIED.,.F.,.F.,.F.,(4,4),(4,4),(0.,1.00600003961334),
(0.0166015299239903,0.0265907346180631),.UNSPECIFIED.);
#3324=B_SPLINE_SURFACE_WITH_KNOTS('',3,3,((#103280,#103281,#103282,#103283),
(#103284,#103285,#103286,#103287),(#103288,#103289,#103290,#103291),(#103292,
#103293,#103294,#103295)),.UNSPECIFIED.,.F.,.F.,.F.,(4,4),(4,4),(-0.00286862201163387,
0.477902879792968),(0.0300094532292794,0.0365944846647019),
 .UNSPECIFIED.);
#3325=B_SPLINE_SURFACE_WITH_KNOTS('',3,3,((#103297,#103298,#103299,#103300),
(#103301,#103302,#103303,#103304),(#103305,#103306,#103307,#103308),(#103309,
#103310,#103311,#103312)),.UNSPECIFIED.,.F.,.F.,.F.,(4,4),(4,4),(0.522097120208964,
1.00286823669293),(0.0265907346180636,0.0331702036889924),.UNSPECIFIED.);
#3326=B_SPLINE_SURFACE_WITH_KNOTS('',3,3,((#103320,#103321,#103322,#103323),
(#103324,#103325,#103326,#103327),(#103328,#103329,#103330,#103331),(#103332,
#103333,#103334,#103335)),.UNSPECIFIED.,.F.,.F.,.F.,(4,4),(4,4),(-0.00286848453307101,
0.477902879860464),(0.0400218729466602,0.0466073985929437),
 .UNSPECIFIED.);
#3327=B_SPLINE_SURFACE_WITH_KNOTS('',3,3,((#103352,#103353,#103354,#103355),
(#103356,#103357,#103358,#103359),(#103360,#103361,#103362,#103363),(#103364,
#103365,#103366,#103367)),.UNSPECIFIED.,.F.,.F.,.F.,(4,4),(4,4),(0.,1.0060001463973),
(0.036594484664504,0.0466073985929155),.UNSPECIFIED.);
#3328=B_SPLINE_SURFACE_WITH_KNOTS('',3,3,((#103368,#103369,#103370,#103371),
(#103372,#103373,#103374,#103375),(#103376,#103377,#103378,#103379),(#103380,
#103381,#103382,#103383)),.UNSPECIFIED.,.F.,.F.,.F.,(4,4),(4,4),(-0.0028678012239562,
0.477902879790876),(0.0500263550859004,0.0565997133101407),
 .UNSPECIFIED.);
#3329=B_SPLINE_SURFACE_WITH_KNOTS('',3,3,((#103385,#103386,#103387,#103388),
(#103389,#103390,#103391,#103392),(#103393,#103394,#103395,#103396),(#103397,
#103398,#103399,#103400)),.UNSPECIFIED.,.F.,.F.,.F.,(4,4),(4,4),(0.522097120209067,
1.00286810177257),(0.0466073985929454,0.0531834925888929),.UNSPECIFIED.);
#3330=B_SPLINE_SURFACE_WITH_KNOTS('',3,3,((#103408,#103409,#103410,#103411),
(#103412,#103413,#103414,#103415),(#103416,#103417,#103418,#103419),(#103420,
#103421,#103422,#103423)),.UNSPECIFIED.,.F.,.F.,.F.,(4,4),(4,4),(-0.00286792598887741,
0.477902879790768),(0.0600156865494596,0.0665898698871164),
 .UNSPECIFIED.);
#3331=B_SPLINE_SURFACE_WITH_KNOTS('',3,3,((#103425,#103426,#103427,#103428),
(#103429,#103430,#103431,#103432),(#103433,#103434,#103435,#103436),(#103437,
#103438,#103439,#103440)),.UNSPECIFIED.,.F.,.F.,.F.,(4,4),(4,4),(0.522097120209252,
1.00286764392032),(0.0565997133101418,0.063172143088706),.UNSPECIFIED.);
#3332=B_SPLINE_SURFACE_WITH_KNOTS('',3,3,((#103456,#103457,#103458,#103459),
(#103460,#103461,#103462,#103463),(#103464,#103465,#103466,#103467),(#103468,
#103469,#103470,#103471)),.UNSPECIFIED.,.F.,.F.,.F.,(4,4),(4,4),(0.522097120208404,
1.00286833998587),(0.0665898698871185,0.0731716198748446),.UNSPECIFIED.);
#3333=B_SPLINE_SURFACE_WITH_KNOTS('',3,3,((#103472,#103473,#103474,#103475),
(#103476,#103477,#103478,#103479),(#103480,#103481,#103482,#103483),(#103484,
#103485,#103486,#103487)),.UNSPECIFIED.,.F.,.F.,.F.,(4,4),(4,4),(-0.00124731532721796,
0.209045111684327),(0.0700194292964934,0.0749900982977344),
 .UNSPECIFIED.);
#3334=B_SPLINE_SURFACE_WITH_KNOTS('',3,3,((#103494,#103495,#103496,#103497),
(#103498,#103499,#103500,#103501),(#103502,#103503,#103504,#103505),(#103506,
#103507,#103508,#103509)),.UNSPECIFIED.,.F.,.F.,.F.,(4,4),(4,4),(-0.00286791014387768,
0.477902879791954),(0.0100271466769349,0.0166015299239877),
 .UNSPECIFIED.);
#3335=B_SPLINE_SURFACE_WITH_KNOTS('',3,3,((#103511,#103512,#103513,#103514),
(#103515,#103516,#103517,#103518),(#103519,#103520,#103521,#103522),(#103523,
#103524,#103525,#103526)),.UNSPECIFIED.,.F.,.F.,.F.,(4,4),(4,4),(0.653230271499819,
1.00206901893299),(0.00656788395390347,0.0131849432430213),
 .UNSPECIFIED.);
#3336=B_SPLINE_SURFACE_WITH_KNOTS('',3,3,((#103534,#103535,#103536,#103537),
(#103538,#103539,#103540,#103541),(#103542,#103543,#103544,#103545),(#103546,
#103547,#103548,#103549)),.UNSPECIFIED.,.F.,.F.,.F.,(4,4),(4,4),(-0.00286780410469178,
0.47790287979141),(0.0200175229646905,0.0265907346180624),.UNSPECIFIED.);
#3337=B_SPLINE_SURFACE_WITH_KNOTS('',3,3,((#103551,#103552,#103553,#103554),
(#103555,#103556,#103557,#103558),(#103559,#103560,#103561,#103562),(#103563,
#103564,#103565,#103566)),.UNSPECIFIED.,.F.,.F.,.F.,(4,4),(4,4),(0.5220971202086,
1.00286753160118),(0.0166015299239897,0.0231736788075225),.UNSPECIFIED.);
#3338=B_SPLINE_SURFACE_WITH_KNOTS('',3,3,((#103568,#103569,#103570,#103571),
(#103572,#103573,#103574,#103575),(#103576,#103577,#103578,#103579),(#103580,
#103581,#103582,#103583)),.UNSPECIFIED.,.F.,.F.,.F.,(4,4),(4,4),(0.,1.00600003961332),
(0.0166015299239879,0.026590734618066),.UNSPECIFIED.);
#3339=B_SPLINE_SURFACE_WITH_KNOTS('',3,3,((#103584,#103585,#103586,#103587),
(#103588,#103589,#103590,#103591),(#103592,#103593,#103594,#103595),(#103596,
#103597,#103598,#103599)),.UNSPECIFIED.,.F.,.F.,.F.,(4,4),(4,4),(-0.0028686220116214,
0.477902879792963),(0.030009453229279,0.036594484664717),.UNSPECIFIED.);
#3340=B_SPLINE_SURFACE_WITH_KNOTS('',3,3,((#103601,#103602,#103603,#103604),
(#103605,#103606,#103607,#103608),(#103609,#103610,#103611,#103612),(#103613,
#103614,#103615,#103616)),.UNSPECIFIED.,.F.,.F.,.F.,(4,4),(4,4),(0.522097120208826,
1.00286823669297),(0.0265907346180652,0.033170203688994),.UNSPECIFIED.);
#3341=B_SPLINE_SURFACE_WITH_KNOTS('',3,3,((#103624,#103625,#103626,#103627),
(#103628,#103629,#103630,#103631),(#103632,#103633,#103634,#103635),(#103636,
#103637,#103638,#103639)),.UNSPECIFIED.,.F.,.F.,.F.,(4,4),(4,4),(-0.00286848453262961,
0.477902879791565),(0.0400218729466602,0.046607398592943),.UNSPECIFIED.);
#3342=B_SPLINE_SURFACE_WITH_KNOTS('',3,3,((#103656,#103657,#103658,#103659),
(#103660,#103661,#103662,#103663),(#103664,#103665,#103666,#103667),(#103668,
#103669,#103670,#103671)),.UNSPECIFIED.,.F.,.F.,.F.,(4,4),(4,4),(0.,1.00600014639743),
(0.0365944846645039,0.0466073985929177),.UNSPECIFIED.);
#3343=B_SPLINE_SURFACE_WITH_KNOTS('',3,3,((#103672,#103673,#103674,#103675),
(#103676,#103677,#103678,#103679),(#103680,#103681,#103682,#103683),(#103684,
#103685,#103686,#103687)),.UNSPECIFIED.,.F.,.F.,.F.,(4,4),(4,4),(-0.00286780122392134,
0.477902879790918),(0.0500263550859004,0.0565997133101405),
 .UNSPECIFIED.);
#3344=B_SPLINE_SURFACE_WITH_KNOTS('',3,3,((#103689,#103690,#103691,#103692),
(#103693,#103694,#103695,#103696),(#103697,#103698,#103699,#103700),(#103701,
#103702,#103703,#103704)),.UNSPECIFIED.,.F.,.F.,.F.,(4,4),(4,4),(0.522097120208999,
1.00286810177259),(0.0466073985929454,0.0531834925888925),.UNSPECIFIED.);
#3345=B_SPLINE_SURFACE_WITH_KNOTS('',3,3,((#103712,#103713,#103714,#103715),
(#103716,#103717,#103718,#103719),(#103720,#103721,#103722,#103723),(#103724,
#103725,#103726,#103727)),.UNSPECIFIED.,.F.,.F.,.F.,(4,4),(4,4),(-0.00286792598891528,
0.477902879790847),(0.0600156865494608,0.0665898698871163),
 .UNSPECIFIED.);
#3346=B_SPLINE_SURFACE_WITH_KNOTS('',3,3,((#103729,#103730,#103731,#103732),
(#103733,#103734,#103735,#103736),(#103737,#103738,#103739,#103740),(#103741,
#103742,#103743,#103744)),.UNSPECIFIED.,.F.,.F.,.F.,(4,4),(4,4),(0.52209712020907,
1.00286764392035),(0.0565997133101428,0.063172143088705),.UNSPECIFIED.);
#3347=B_SPLINE_SURFACE_WITH_KNOTS('',3,3,((#103760,#103761,#103762,#103763),
(#103764,#103765,#103766,#103767),(#103768,#103769,#103770,#103771),(#103772,
#103773,#103774,#103775)),.UNSPECIFIED.,.F.,.F.,.F.,(4,4),(4,4),(0.522097120208342,
1.00286833998585),(0.06658986988712,0.0731716198748447),.UNSPECIFIED.);
#3348=B_SPLINE_SURFACE_WITH_KNOTS('',3,3,((#103776,#103777,#103778,#103779),
(#103780,#103781,#103782,#103783),(#103784,#103785,#103786,#103787),(#103788,
#103789,#103790,#103791)),.UNSPECIFIED.,.F.,.F.,.F.,(4,4),(4,4),(-0.00124731532471121,
0.209045111686916),(0.0700194292964978,0.0749900982977462),
 .UNSPECIFIED.);
#3349=B_SPLINE_SURFACE_WITH_KNOTS('',3,3,((#103798,#103799,#103800,#103801),
(#103802,#103803,#103804,#103805),(#103806,#103807,#103808,#103809),(#103810,
#103811,#103812,#103813)),.UNSPECIFIED.,.F.,.F.,.F.,(4,4),(4,4),(-0.00286791014388252,
0.477902879794285),(0.0100271466769349,0.0166015299239876),
 .UNSPECIFIED.);
#3350=B_SPLINE_SURFACE_WITH_KNOTS('',3,3,((#103815,#103816,#103817,#103818),
(#103819,#103820,#103821,#103822),(#103823,#103824,#103825,#103826),(#103827,
#103828,#103829,#103830)),.UNSPECIFIED.,.F.,.F.,.F.,(4,4),(4,4),(0.653230271498285,
1.0020690189308),(0.00656788395390921,0.013184943243012),.UNSPECIFIED.);
#3351=B_SPLINE_SURFACE_WITH_KNOTS('',3,3,((#103838,#103839,#103840,#103841),
(#103842,#103843,#103844,#103845),(#103846,#103847,#103848,#103849),(#103850,
#103851,#103852,#103853)),.UNSPECIFIED.,.F.,.F.,.F.,(4,4),(4,4),(-0.00286780410476033,
0.477902879793274),(0.0200175229646903,0.0265907346180623),
 .UNSPECIFIED.);
#3352=B_SPLINE_SURFACE_WITH_KNOTS('',3,3,((#103855,#103856,#103857,#103858),
(#103859,#103860,#103861,#103862),(#103863,#103864,#103865,#103866),(#103867,
#103868,#103869,#103870)),.UNSPECIFIED.,.F.,.F.,.F.,(4,4),(4,4),(0.522097120208445,
1.00286753160117),(0.0166015299239883,0.0231736788075214),.UNSPECIFIED.);
#3353=B_SPLINE_SURFACE_WITH_KNOTS('',3,3,((#103872,#103873,#103874,#103875),
(#103876,#103877,#103878,#103879),(#103880,#103881,#103882,#103883),(#103884,
#103885,#103886,#103887)),.UNSPECIFIED.,.F.,.F.,.F.,(4,4),(4,4),(0.,1.00600003961389),
(0.0166015299239904,0.0265907346180634),.UNSPECIFIED.);
#3354=B_SPLINE_SURFACE_WITH_KNOTS('',3,3,((#103888,#103889,#103890,#103891),
(#103892,#103893,#103894,#103895),(#103896,#103897,#103898,#103899),(#103900,
#103901,#103902,#103903)),.UNSPECIFIED.,.F.,.F.,.F.,(4,4),(4,4),(-0.00286862201160333,
0.477902879793387),(0.030009453229279,0.0365944846647018),.UNSPECIFIED.);
#3355=B_SPLINE_SURFACE_WITH_KNOTS('',3,3,((#103905,#103906,#103907,#103908),
(#103909,#103910,#103911,#103912),(#103913,#103914,#103915,#103916),(#103917,
#103918,#103919,#103920)),.UNSPECIFIED.,.F.,.F.,.F.,(4,4),(4,4),(0.522097120208658,
1.00286823669293),(0.0265907346180631,0.0331702036889929),.UNSPECIFIED.);
#3356=B_SPLINE_SURFACE_WITH_KNOTS('',3,3,((#103928,#103929,#103930,#103931),
(#103932,#103933,#103934,#103935),(#103936,#103937,#103938,#103939),(#103940,
#103941,#103942,#103943)),.UNSPECIFIED.,.F.,.F.,.F.,(4,4),(4,4),(-0.00286848453260555,
0.477902879791857),(0.0400218729466597,0.0466073985929431),
 .UNSPECIFIED.);
#3357=B_SPLINE_SURFACE_WITH_KNOTS('',3,3,((#103960,#103961,#103962,#103963),
(#103964,#103965,#103966,#103967),(#103968,#103969,#103970,#103971),(#103972,
#103973,#103974,#103975)),.UNSPECIFIED.,.F.,.F.,.F.,(4,4),(4,4),(0.,1.00600014639731),
(0.0365944846645024,0.0466073985929167),.UNSPECIFIED.);
#3358=B_SPLINE_SURFACE_WITH_KNOTS('',3,3,((#103976,#103977,#103978,#103979),
(#103980,#103981,#103982,#103983),(#103984,#103985,#103986,#103987),(#103988,
#103989,#103990,#103991)),.UNSPECIFIED.,.F.,.F.,.F.,(4,4),(4,4),(-0.00286780122392774,
0.477902879791221),(0.0500263550859004,0.0565997133101403),
 .UNSPECIFIED.);
#3359=B_SPLINE_SURFACE_WITH_KNOTS('',3,3,((#103993,#103994,#103995,#103996),
(#103997,#103998,#103999,#104000),(#104001,#104002,#104003,#104004),(#104005,
#104006,#104007,#104008)),.UNSPECIFIED.,.F.,.F.,.F.,(4,4),(4,4),(0.522097120208844,
1.0028681017726),(0.0466073985929452,0.0531834925888928),.UNSPECIFIED.);
#3360=B_SPLINE_SURFACE_WITH_KNOTS('',3,3,((#104016,#104017,#104018,#104019),
(#104020,#104021,#104022,#104023),(#104024,#104025,#104026,#104027),(#104028,
#104029,#104030,#104031)),.UNSPECIFIED.,.F.,.F.,.F.,(4,4),(4,4),(-0.00286792598900819,
0.47790287979099),(0.0600156865494602,0.0665898698871176),.UNSPECIFIED.);
#3361=B_SPLINE_SURFACE_WITH_KNOTS('',3,3,((#104033,#104034,#104035,#104036),
(#104037,#104038,#104039,#104040),(#104041,#104042,#104043,#104044),(#104045,
#104046,#104047,#104048)),.UNSPECIFIED.,.F.,.F.,.F.,(4,4),(4,4),(0.522097120208971,
1.00286764392034),(0.0565997133101411,0.0631721430887057),.UNSPECIFIED.);
#3362=B_SPLINE_SURFACE_WITH_KNOTS('',3,3,((#104064,#104065,#104066,#104067),
(#104068,#104069,#104070,#104071),(#104072,#104073,#104074,#104075),(#104076,
#104077,#104078,#104079)),.UNSPECIFIED.,.F.,.F.,.F.,(4,4),(4,4),(0.522097120208079,
1.00286833998585),(0.0665898698871197,0.0731716198748446),.UNSPECIFIED.);
#3363=B_SPLINE_SURFACE_WITH_KNOTS('',3,3,((#104080,#104081,#104082,#104083),
(#104084,#104085,#104086,#104087),(#104088,#104089,#104090,#104091),(#104092,
#104093,#104094,#104095)),.UNSPECIFIED.,.F.,.F.,.F.,(4,4),(4,4),(-0.00124731532213843,
0.209045111689404),(0.0700194292965034,0.074990098297759),.UNSPECIFIED.);
#3364=B_SPLINE_SURFACE_WITH_KNOTS('',3,3,((#104096,#104097,#104098,#104099),
(#104100,#104101,#104102,#104103),(#104104,#104105,#104106,#104107),(#104108,
#104109,#104110,#104111)),.UNSPECIFIED.,.F.,.F.,.F.,(4,4),(4,4),(-0.00286791014394406,
0.477902879796325),(0.010027146676379,0.0166015299239868),.UNSPECIFIED.);
#3365=B_SPLINE_SURFACE_WITH_KNOTS('',3,3,((#104113,#104114,#104115,#104116),
(#104117,#104118,#104119,#104120),(#104121,#104122,#104123,#104124),(#104125,
#104126,#104127,#104128)),.UNSPECIFIED.,.F.,.F.,.F.,(4,4),(4,4),(0.653230271496767,
1.0020690189285),(0.00656788395391393,0.0131849432430011),.UNSPECIFIED.);
#3366=B_SPLINE_SURFACE_WITH_KNOTS('',3,3,((#104142,#104143,#104144,#104145),
(#104146,#104147,#104148,#104149),(#104150,#104151,#104152,#104153),(#104154,
#104155,#104156,#104157)),.UNSPECIFIED.,.F.,.F.,.F.,(4,4),(4,4),(-0.0028678041047206,
0.47790287979547),(0.0200175229646906,0.0265907346180621),.UNSPECIFIED.);
#3367=B_SPLINE_SURFACE_WITH_KNOTS('',3,3,((#104159,#104160,#104161,#104162),
(#104163,#104164,#104165,#104166),(#104167,#104168,#104169,#104170),(#104171,
#104172,#104173,#104174)),.UNSPECIFIED.,.F.,.F.,.F.,(4,4),(4,4),(0.522097120208333,
1.00286753160119),(0.0166015299239887,0.0231736788075233),.UNSPECIFIED.);
#3368=B_SPLINE_SURFACE_WITH_KNOTS('',3,3,((#104176,#104177,#104178,#104179),
(#104180,#104181,#104182,#104183),(#104184,#104185,#104186,#104187),(#104188,
#104189,#104190,#104191)),.UNSPECIFIED.,.F.,.F.,.F.,(4,4),(4,4),(0.,1.0060000396136),
(0.016601529923987,0.0265907346180635),.UNSPECIFIED.);
#3369=B_SPLINE_SURFACE_WITH_KNOTS('',3,3,((#104192,#104193,#104194,#104195),
(#104196,#104197,#104198,#104199),(#104200,#104201,#104202,#104203),(#104204,
#104205,#104206,#104207)),.UNSPECIFIED.,.F.,.F.,.F.,(4,4),(4,4),(-0.00286862201162562,
0.477902879794753),(0.0300094532292787,0.0365944846647161),
 .UNSPECIFIED.);
#3370=B_SPLINE_SURFACE_WITH_KNOTS('',3,3,((#104209,#104210,#104211,#104212),
(#104213,#104214,#104215,#104216),(#104217,#104218,#104219,#104220),(#104221,
#104222,#104223,#104224)),.UNSPECIFIED.,.F.,.F.,.F.,(4,4),(4,4),(0.522097120208533,
1.00286823669298),(0.0265907346180623,0.0331702036889942),.UNSPECIFIED.);
#3371=B_SPLINE_SURFACE_WITH_KNOTS('',3,3,((#104232,#104233,#104234,#104235),
(#104236,#104237,#104238,#104239),(#104240,#104241,#104242,#104243),(#104244,
#104245,#104246,#104247)),.UNSPECIFIED.,.F.,.F.,.F.,(4,4),(4,4),(-0.00286848453263586,
0.477902879793197),(0.0400218729466601,0.0466073985929432),
 .UNSPECIFIED.);
#3372=B_SPLINE_SURFACE_WITH_KNOTS('',3,3,((#104264,#104265,#104266,#104267),
(#104268,#104269,#104270,#104271),(#104272,#104273,#104274,#104275),(#104276,
#104277,#104278,#104279)),.UNSPECIFIED.,.F.,.F.,.F.,(4,4),(4,4),(0.,1.0060001463976),
(0.0365944846645023,0.0466073985929169),.UNSPECIFIED.);
#3373=B_SPLINE_SURFACE_WITH_KNOTS('',3,3,((#104280,#104281,#104282,#104283),
(#104284,#104285,#104286,#104287),(#104288,#104289,#104290,#104291),(#104292,
#104293,#104294,#104295)),.UNSPECIFIED.,.F.,.F.,.F.,(4,4),(4,4),(-0.00286780122397318,
0.47790287979194),(0.0500263550859004,0.0565997133101409),.UNSPECIFIED.);
#3374=B_SPLINE_SURFACE_WITH_KNOTS('',3,3,((#104297,#104298,#104299,#104300),
(#104301,#104302,#104303,#104304),(#104305,#104306,#104307,#104308),(#104309,
#104310,#104311,#104312)),.UNSPECIFIED.,.F.,.F.,.F.,(4,4),(4,4),(0.522097120208675,
1.00286810177264),(0.0466073985929447,0.0531834925888942),.UNSPECIFIED.);
#3375=B_SPLINE_SURFACE_WITH_KNOTS('',3,3,((#104320,#104321,#104322,#104323),
(#104324,#104325,#104326,#104327),(#104328,#104329,#104330,#104331),(#104332,
#104333,#104334,#104335)),.UNSPECIFIED.,.F.,.F.,.F.,(4,4),(4,4),(-0.00286792598896076,
0.477902879791154),(0.0600156865494595,0.0665898698871175),
 .UNSPECIFIED.);
#3376=B_SPLINE_SURFACE_WITH_KNOTS('',3,3,((#104337,#104338,#104339,#104340),
(#104341,#104342,#104343,#104344),(#104345,#104346,#104347,#104348),(#104349,
#104350,#104351,#104352)),.UNSPECIFIED.,.F.,.F.,.F.,(4,4),(4,4),(0.522097120208892,
1.00286764392033),(0.056599713310143,0.0631721430887063),.UNSPECIFIED.);
#3377=B_SPLINE_SURFACE_WITH_KNOTS('',3,3,((#104368,#104369,#104370,#104371),
(#104372,#104373,#104374,#104375),(#104376,#104377,#104378,#104379),(#104380,
#104381,#104382,#104383)),.UNSPECIFIED.,.F.,.F.,.F.,(4,4),(4,4),(0.522097120208067,
1.00286833998587),(0.0665898698871201,0.0731716198748447),.UNSPECIFIED.);
#3378=B_SPLINE_SURFACE_WITH_KNOTS('',3,3,((#104384,#104385,#104386,#104387),
(#104388,#104389,#104390,#104391),(#104392,#104393,#104394,#104395),(#104396,
#104397,#104398,#104399)),.UNSPECIFIED.,.F.,.F.,.F.,(4,4),(4,4),(-0.00124731531958877,
0.209045111691966),(0.0700194292965107,0.0749900982977698),
 .UNSPECIFIED.);
#3379=B_SPLINE_SURFACE_WITH_KNOTS('',3,3,((#104406,#104407,#104408,#104409),
(#104410,#104411,#104412,#104413),(#104414,#104415,#104416,#104417),(#104418,
#104419,#104420,#104421)),.UNSPECIFIED.,.F.,.F.,.F.,(4,4),(4,4),(-0.00286791014395316,
0.477902879798327),(0.0100271466769336,0.0166015299239876),
 .UNSPECIFIED.);
#3380=B_SPLINE_SURFACE_WITH_KNOTS('',3,3,((#104423,#104424,#104425,#104426),
(#104427,#104428,#104429,#104430),(#104431,#104432,#104433,#104434),(#104435,
#104436,#104437,#104438)),.UNSPECIFIED.,.F.,.F.,.F.,(4,4),(4,4),(0.653230271495359,
1.00206901892606),(0.00656788395391684,0.0131849432429894),
 .UNSPECIFIED.);
#3381=B_SPLINE_SURFACE_WITH_KNOTS('',3,3,((#104446,#104447,#104448,#104449),
(#104450,#104451,#104452,#104453),(#104454,#104455,#104456,#104457),(#104458,
#104459,#104460,#104461)),.UNSPECIFIED.,.F.,.F.,.F.,(4,4),(4,4),(-0.00286780410466546,
0.477902879797445),(0.0200175229646907,0.0265907346180625),
 .UNSPECIFIED.);
#3382=B_SPLINE_SURFACE_WITH_KNOTS('',3,3,((#104463,#104464,#104465,#104466),
(#104467,#104468,#104469,#104470),(#104471,#104472,#104473,#104474),(#104475,
#104476,#104477,#104478)),.UNSPECIFIED.,.F.,.F.,.F.,(4,4),(4,4),(0.52209712020821,
1.00286753160119),(0.0166015299239882,0.0231736788075225),.UNSPECIFIED.);
#3383=B_SPLINE_SURFACE_WITH_KNOTS('',3,3,((#104480,#104481,#104482,#104483),
(#104484,#104485,#104486,#104487),(#104488,#104489,#104490,#104491),(#104492,
#104493,#104494,#104495)),.UNSPECIFIED.,.F.,.F.,.F.,(4,4),(4,4),(0.,1.00600003961386),
(0.0166015299239892,0.0265907346180634),.UNSPECIFIED.);
#3384=B_SPLINE_SURFACE_WITH_KNOTS('',3,3,((#104496,#104497,#104498,#104499),
(#104500,#104501,#104502,#104503),(#104504,#104505,#104506,#104507),(#104508,
#104509,#104510,#104511)),.UNSPECIFIED.,.F.,.F.,.F.,(4,4),(4,4),(-0.0028686220115229,
0.477902879796868),(0.0300094532292789,0.0365944846647172),
 .UNSPECIFIED.);
#3385=B_SPLINE_SURFACE_WITH_KNOTS('',3,3,((#104513,#104514,#104515,#104516),
(#104517,#104518,#104519,#104520),(#104521,#104522,#104523,#104524),(#104525,
#104526,#104527,#104528)),.UNSPECIFIED.,.F.,.F.,.F.,(4,4),(4,4),(0.522097120208426,
1.00286823669299),(0.0265907346180636,0.0331702036889942),.UNSPECIFIED.);
#3386=B_SPLINE_SURFACE_WITH_KNOTS('',3,3,((#104536,#104537,#104538,#104539),
(#104540,#104541,#104542,#104543),(#104544,#104545,#104546,#104547),(#104548,
#104549,#104550,#104551)),.UNSPECIFIED.,.F.,.F.,.F.,(4,4),(4,4),(-0.00286848453265357,
0.477902879795543),(0.0400218729466598,0.0466073985929427),
 .UNSPECIFIED.);
#3387=B_SPLINE_SURFACE_WITH_KNOTS('',3,3,((#104568,#104569,#104570,#104571),
(#104572,#104573,#104574,#104575),(#104576,#104577,#104578,#104579),(#104580,
#104581,#104582,#104583)),.UNSPECIFIED.,.F.,.F.,.F.,(4,4),(4,4),(0.,1.00600014639755),
(0.0365944846645018,0.0466073985929159),.UNSPECIFIED.);
#3388=B_SPLINE_SURFACE_WITH_KNOTS('',3,3,((#104584,#104585,#104586,#104587),
(#104588,#104589,#104590,#104591),(#104592,#104593,#104594,#104595),(#104596,
#104597,#104598,#104599)),.UNSPECIFIED.,.F.,.F.,.F.,(4,4),(4,4),(-0.00286780122398932,
0.477902879794246),(0.0500263550858991,0.0565997133101411),
 .UNSPECIFIED.);
#3389=B_SPLINE_SURFACE_WITH_KNOTS('',3,3,((#104601,#104602,#104603,#104604),
(#104605,#104606,#104607,#104608),(#104609,#104610,#104611,#104612),(#104613,
#104614,#104615,#104616)),.UNSPECIFIED.,.F.,.F.,.F.,(4,4),(4,4),(0.522097120208498,
1.00286810177262),(0.0466073985929433,0.0531834925888932),.UNSPECIFIED.);
#3390=B_SPLINE_SURFACE_WITH_KNOTS('',3,3,((#104624,#104625,#104626,#104627),
(#104628,#104629,#104630,#104631),(#104632,#104633,#104634,#104635),(#104636,
#104637,#104638,#104639)),.UNSPECIFIED.,.F.,.F.,.F.,(4,4),(4,4),(-0.00286792598894048,
0.477902879792958),(0.0600156865494587,0.0665898698871172),
 .UNSPECIFIED.);
#3391=B_SPLINE_SURFACE_WITH_KNOTS('',3,3,((#104641,#104642,#104643,#104644),
(#104645,#104646,#104647,#104648),(#104649,#104650,#104651,#104652),(#104653,
#104654,#104655,#104656)),.UNSPECIFIED.,.F.,.F.,.F.,(4,4),(4,4),(0.522097120208652,
1.00286764392037),(0.0565997133101409,0.0631721430887067),.UNSPECIFIED.);
#3392=B_SPLINE_SURFACE_WITH_KNOTS('',3,3,((#104672,#104673,#104674,#104675),
(#104676,#104677,#104678,#104679),(#104680,#104681,#104682,#104683),(#104684,
#104685,#104686,#104687)),.UNSPECIFIED.,.F.,.F.,.F.,(4,4),(4,4),(0.522097120207924,
1.00286833998585),(0.0665898698871192,0.0731716198748446),.UNSPECIFIED.);
#3393=B_SPLINE_SURFACE_WITH_KNOTS('',3,3,((#104688,#104689,#104690,#104691),
(#104692,#104693,#104694,#104695),(#104696,#104697,#104698,#104699),(#104700,
#104701,#104702,#104703)),.UNSPECIFIED.,.F.,.F.,.F.,(4,4),(4,4),(-0.00124731531729226,
0.209045111694373),(0.0700194292965185,0.0749900982977811),
 .UNSPECIFIED.);
#3394=B_SPLINE_SURFACE_WITH_KNOTS('',3,3,((#104710,#104711,#104712,#104713),
(#104714,#104715,#104716,#104717),(#104718,#104719,#104720,#104721),(#104722,
#104723,#104724,#104725)),.UNSPECIFIED.,.F.,.F.,.F.,(4,4),(4,4),(-0.00286791014398744,
0.477902879799781),(0.0100271466769349,0.0166015299239874),
 .UNSPECIFIED.);
#3395=B_SPLINE_SURFACE_WITH_KNOTS('',3,3,((#104727,#104728,#104729,#104730),
(#104731,#104732,#104733,#104734),(#104735,#104736,#104737,#104738),(#104739,
#104740,#104741,#104742)),.UNSPECIFIED.,.F.,.F.,.F.,(4,4),(4,4),(0.653230271493824,
1.00206901892362),(0.00656788395392139,0.013184943242896),.UNSPECIFIED.);
#3396=B_SPLINE_SURFACE_WITH_KNOTS('',3,3,((#104750,#104751,#104752,#104753),
(#104754,#104755,#104756,#104757),(#104758,#104759,#104760,#104761),(#104762,
#104763,#104764,#104765)),.UNSPECIFIED.,.F.,.F.,.F.,(4,4),(4,4),(-0.00286780410473367,
0.477902879799223),(0.0200175229646907,0.0265907346180625),
 .UNSPECIFIED.);
#3397=B_SPLINE_SURFACE_WITH_KNOTS('',3,3,((#104767,#104768,#104769,#104770),
(#104771,#104772,#104773,#104774),(#104775,#104776,#104777,#104778),(#104779,
#104780,#104781,#104782)),.UNSPECIFIED.,.F.,.F.,.F.,(4,4),(4,4),(0.522097120208011,
1.0028675316012),(0.0166015299239878,0.0231736788075225),.UNSPECIFIED.);
#3398=B_SPLINE_SURFACE_WITH_KNOTS('',3,3,((#104784,#104785,#104786,#104787),
(#104788,#104789,#104790,#104791),(#104792,#104793,#104794,#104795),(#104796,
#104797,#104798,#104799)),.UNSPECIFIED.,.F.,.F.,.F.,(4,4),(4,4),(0.,1.00600003961381),
(0.016601529923988,0.0265907346180629),.UNSPECIFIED.);
#3399=B_SPLINE_SURFACE_WITH_KNOTS('',3,3,((#104800,#104801,#104802,#104803),
(#104804,#104805,#104806,#104807),(#104808,#104809,#104810,#104811),(#104812,
#104813,#104814,#104815)),.UNSPECIFIED.,.F.,.F.,.F.,(4,4),(4,4),(-0.00286862201153651,
0.477902879798629),(0.0300094532292788,0.0365944846647022),
 .UNSPECIFIED.);
#3400=B_SPLINE_SURFACE_WITH_KNOTS('',3,3,((#104817,#104818,#104819,#104820),
(#104821,#104822,#104823,#104824),(#104825,#104826,#104827,#104828),(#104829,
#104830,#104831,#104832)),.UNSPECIFIED.,.F.,.F.,.F.,(4,4),(4,4),(0.522097120208293,
1.0028682366929),(0.0265907346180642,0.0331702036051743),.UNSPECIFIED.);
#3401=B_SPLINE_SURFACE_WITH_KNOTS('',3,3,((#104840,#104841,#104842,#104843),
(#104844,#104845,#104846,#104847),(#104848,#104849,#104850,#104851),(#104852,
#104853,#104854,#104855)),.UNSPECIFIED.,.F.,.F.,.F.,(4,4),(4,4),(-0.00286848453268432,
0.477902879797276),(0.0400218729466601,0.046607398592943),.UNSPECIFIED.);
#3402=B_SPLINE_SURFACE_WITH_KNOTS('',3,3,((#104872,#104873,#104874,#104875),
(#104876,#104877,#104878,#104879),(#104880,#104881,#104882,#104883),(#104884,
#104885,#104886,#104887)),.UNSPECIFIED.,.F.,.F.,.F.,(4,4),(4,4),(0.,1.00600014639734),
(0.0365944846645009,0.0466073985929168),.UNSPECIFIED.);
#3403=B_SPLINE_SURFACE_WITH_KNOTS('',3,3,((#104888,#104889,#104890,#104891),
(#104892,#104893,#104894,#104895),(#104896,#104897,#104898,#104899),(#104900,
#104901,#104902,#104903)),.UNSPECIFIED.,.F.,.F.,.F.,(4,4),(4,4),(-0.00286780122404455,
0.477902879796201),(0.0500263550858999,0.0565997133101408),
 .UNSPECIFIED.);
#3404=B_SPLINE_SURFACE_WITH_KNOTS('',3,3,((#104905,#104906,#104907,#104908),
(#104909,#104910,#104911,#104912),(#104913,#104914,#104915,#104916),(#104917,
#104918,#104919,#104920)),.UNSPECIFIED.,.F.,.F.,.F.,(4,4),(4,4),(0.522097120208524,
1.00286810177264),(0.0466073985929456,0.0531834925888943),.UNSPECIFIED.);
#3405=B_SPLINE_SURFACE_WITH_KNOTS('',3,3,((#104928,#104929,#104930,#104931),
(#104932,#104933,#104934,#104935),(#104936,#104937,#104938,#104939),(#104940,
#104941,#104942,#104943)),.UNSPECIFIED.,.F.,.F.,.F.,(4,4),(4,4),(-0.0028679259890379,
0.47790287979535),(0.0600156865494599,0.0665898698871175),.UNSPECIFIED.);
#3406=B_SPLINE_SURFACE_WITH_KNOTS('',3,3,((#104945,#104946,#104947,#104948),
(#104949,#104950,#104951,#104952),(#104953,#104954,#104955,#104956),(#104957,
#104958,#104959,#104960)),.UNSPECIFIED.,.F.,.F.,.F.,(4,4),(4,4),(0.522097120208551,
1.00286764392039),(0.0565997133101416,0.0631721430887072),.UNSPECIFIED.);
#3407=B_SPLINE_SURFACE_WITH_KNOTS('',3,3,((#104976,#104977,#104978,#104979),
(#104980,#104981,#104982,#104983),(#104984,#104985,#104986,#104987),(#104988,
#104989,#104990,#104991)),.UNSPECIFIED.,.F.,.F.,.F.,(4,4),(4,4),(0.522097120207716,
1.0028683399859),(0.0665898698871188,0.073171619874846),.UNSPECIFIED.);
#3408=B_SPLINE_SURFACE_WITH_KNOTS('',3,3,((#104992,#104993,#104994,#104995),
(#104996,#104997,#104998,#104999),(#105000,#105001,#105002,#105003),(#105004,
#105005,#105006,#105007)),.UNSPECIFIED.,.F.,.F.,.F.,(4,4),(4,4),(-0.00124731531514357,
0.20904511169649),(0.0700194292965287,0.0749900982977919),.UNSPECIFIED.);
#3409=B_SPLINE_SURFACE_WITH_KNOTS('',3,3,((#105014,#105015,#105016,#105017),
(#105018,#105019,#105020,#105021),(#105022,#105023,#105024,#105025),(#105026,
#105027,#105028,#105029)),.UNSPECIFIED.,.F.,.F.,.F.,(4,4),(4,4),(-0.0028679101440714,
0.477902879801083),(0.0100271466769349,0.0166015299239868),
 .UNSPECIFIED.);
#3410=B_SPLINE_SURFACE_WITH_KNOTS('',3,3,((#105031,#105032,#105033,#105034),
(#105035,#105036,#105037,#105038),(#105039,#105040,#105041,#105042),(#105043,
#105044,#105045,#105046)),.UNSPECIFIED.,.F.,.F.,.F.,(4,4),(4,4),(0.653230271492592,
1.00206901892104),(0.00656788395392352,0.0131849432429891),
 .UNSPECIFIED.);
#3411=B_SPLINE_SURFACE_WITH_KNOTS('',3,3,((#105054,#105055,#105056,#105057),
(#105058,#105059,#105060,#105061),(#105062,#105063,#105064,#105065),(#105066,
#105067,#105068,#105069)),.UNSPECIFIED.,.F.,.F.,.F.,(4,4),(4,4),(-0.00286780410466828,
0.477902879800657),(0.0200175229646911,0.0265907346180624),
 .UNSPECIFIED.);
#3412=B_SPLINE_SURFACE_WITH_KNOTS('',3,3,((#105071,#105072,#105073,#105074),
(#105075,#105076,#105077,#105078),(#105079,#105080,#105081,#105082),(#105083,
#105084,#105085,#105086)),.UNSPECIFIED.,.F.,.F.,.F.,(4,4),(4,4),(0.522097120207656,
1.00286753160124),(0.0166015299239886,0.0231736788075226),.UNSPECIFIED.);
#3413=B_SPLINE_SURFACE_WITH_KNOTS('',3,3,((#105088,#105089,#105090,#105091),
(#105092,#105093,#105094,#105095),(#105096,#105097,#105098,#105099),(#105100,
#105101,#105102,#105103)),.UNSPECIFIED.,.F.,.F.,.F.,(4,4),(4,4),(0.,1.00600003961359),
(0.0166015299239881,0.0265907346180622),.UNSPECIFIED.);
#3414=B_SPLINE_SURFACE_WITH_KNOTS('',3,3,((#105104,#105105,#105106,#105107),
(#105108,#105109,#105110,#105111),(#105112,#105113,#105114,#105115),(#105116,
#105117,#105118,#105119)),.UNSPECIFIED.,.F.,.F.,.F.,(4,4),(4,4),(-0.00286862201158194,
0.477902879799869),(0.030009453229279,0.036594484664716),.UNSPECIFIED.);
#3415=B_SPLINE_SURFACE_WITH_KNOTS('',3,3,((#105121,#105122,#105123,#105124),
(#105125,#105126,#105127,#105128),(#105129,#105130,#105131,#105132),(#105133,
#105134,#105135,#105136)),.UNSPECIFIED.,.F.,.F.,.F.,(4,4),(4,4),(0.522097120208047,
1.00286823669304),(0.0265907346180626,0.0331702036889935),.UNSPECIFIED.);
#3416=B_SPLINE_SURFACE_WITH_KNOTS('',3,3,((#105144,#105145,#105146,#105147),
(#105148,#105149,#105150,#105151),(#105152,#105153,#105154,#105155),(#105156,
#105157,#105158,#105159)),.UNSPECIFIED.,.F.,.F.,.F.,(4,4),(4,4),(-0.0028684845327302,
0.477902879799251),(0.0400218729466597,0.0466073985929431),
 .UNSPECIFIED.);
#3417=B_SPLINE_SURFACE_WITH_KNOTS('',3,3,((#105176,#105177,#105178,#105179),
(#105180,#105181,#105182,#105183),(#105184,#105185,#105186,#105187),(#105188,
#105189,#105190,#105191)),.UNSPECIFIED.,.F.,.F.,.F.,(4,4),(4,4),(0.,1.00600014639743),
(0.0365944846645017,0.0466073985929158),.UNSPECIFIED.);
#3418=B_SPLINE_SURFACE_WITH_KNOTS('',3,3,((#105192,#105193,#105194,#105195),
(#105196,#105197,#105198,#105199),(#105200,#105201,#105202,#105203),(#105204,
#105205,#105206,#105207)),.UNSPECIFIED.,.F.,.F.,.F.,(4,4),(4,4),(-0.00286780122399644,
0.477902879798194),(0.0500263550859006,0.0565997133101405),
 .UNSPECIFIED.);
#3419=B_SPLINE_SURFACE_WITH_KNOTS('',3,3,((#105209,#105210,#105211,#105212),
(#105213,#105214,#105215,#105216),(#105217,#105218,#105219,#105220),(#105221,
#105222,#105223,#105224)),.UNSPECIFIED.,.F.,.F.,.F.,(4,4),(4,4),(0.522097120208366,
1.00286810177262),(0.046607398592945,0.0531834925888933),.UNSPECIFIED.);
#3420=B_SPLINE_SURFACE_WITH_KNOTS('',3,3,((#105232,#105233,#105234,#105235),
(#105236,#105237,#105238,#105239),(#105240,#105241,#105242,#105243),(#105244,
#105245,#105246,#105247)),.UNSPECIFIED.,.F.,.F.,.F.,(4,4),(4,4),(-0.00286792598896392,
0.477902879797277),(0.0600156865494601,0.0665898698871176),
 .UNSPECIFIED.);
#3421=B_SPLINE_SURFACE_WITH_KNOTS('',3,3,((#105249,#105250,#105251,#105252),
(#105253,#105254,#105255,#105256),(#105257,#105258,#105259,#105260),(#105261,
#105262,#105263,#105264)),.UNSPECIFIED.,.F.,.F.,.F.,(4,4),(4,4),(0.522097120208508,
1.0028676439203),(0.0565997133101424,0.0631721430887051),.UNSPECIFIED.);
#3422=B_SPLINE_SURFACE_WITH_KNOTS('',3,3,((#105280,#105281,#105282,#105283),
(#105284,#105285,#105286,#105287),(#105288,#105289,#105290,#105291),(#105292,
#105293,#105294,#105295)),.UNSPECIFIED.,.F.,.F.,.F.,(4,4),(4,4),(0.522097120207604,
1.00286833998584),(0.0665898698871184,0.0731716198748442),.UNSPECIFIED.);
#3423=B_SPLINE_SURFACE_WITH_KNOTS('',3,3,((#105296,#105297,#105298,#105299),
(#105300,#105301,#105302,#105303),(#105304,#105305,#105306,#105307),(#105308,
#105309,#105310,#105311)),.UNSPECIFIED.,.F.,.F.,.F.,(4,4),(4,4),(-0.00124731531299614,
0.209045111698441),(0.0700194292965412,0.074990098297801),.UNSPECIFIED.);
#3424=B_SPLINE_SURFACE_WITH_KNOTS('',3,3,((#105318,#105319,#105320,#105321),
(#105322,#105323,#105324,#105325),(#105326,#105327,#105328,#105329),(#105330,
#105331,#105332,#105333)),.UNSPECIFIED.,.F.,.F.,.F.,(4,4),(4,4),(-0.00286791014406684,
0.477902879802145),(0.0100271466769343,0.0166015299239869),
 .UNSPECIFIED.);
#3425=B_SPLINE_SURFACE_WITH_KNOTS('',3,3,((#105335,#105336,#105337,#105338),
(#105339,#105340,#105341,#105342),(#105343,#105344,#105345,#105346),(#105347,
#105348,#105349,#105350)),.UNSPECIFIED.,.F.,.F.,.F.,(4,4),(4,4),(0.653230271491155,
1.00206901891852),(0.00656788395392543,0.0131849432429894),
 .UNSPECIFIED.);
#3426=B_SPLINE_SURFACE_WITH_KNOTS('',3,3,((#105358,#105359,#105360,#105361),
(#105362,#105363,#105364,#105365),(#105366,#105367,#105368,#105369),(#105370,
#105371,#105372,#105373)),.UNSPECIFIED.,.F.,.F.,.F.,(4,4),(4,4),(-0.00286780410478348,
0.477902879801889),(0.0200175229646909,0.0265907346180623),
 .UNSPECIFIED.);
#3427=B_SPLINE_SURFACE_WITH_KNOTS('',3,3,((#105375,#105376,#105377,#105378),
(#105379,#105380,#105381,#105382),(#105383,#105384,#105385,#105386),(#105387,
#105388,#105389,#105390)),.UNSPECIFIED.,.F.,.F.,.F.,(4,4),(4,4),(0.522097120204887,
1.00286753160122),(0.0166015299239819,0.0231736788075228),.UNSPECIFIED.);
#3428=B_SPLINE_SURFACE_WITH_KNOTS('',3,3,((#105392,#105393,#105394,#105395),
(#105396,#105397,#105398,#105399),(#105400,#105401,#105402,#105403),(#105404,
#105405,#105406,#105407)),.UNSPECIFIED.,.F.,.F.,.F.,(4,4),(4,4),(0.,1.00600003961353),
(0.0166015299239881,0.0265907346180637),.UNSPECIFIED.);
#3429=B_SPLINE_SURFACE_WITH_KNOTS('',3,3,((#105408,#105409,#105410,#105411),
(#105412,#105413,#105414,#105415),(#105416,#105417,#105418,#105419),(#105420,
#105421,#105422,#105423)),.UNSPECIFIED.,.F.,.F.,.F.,(4,4),(4,4),(-0.00286862201163699,
0.47790287980125),(0.0300094532292782,0.036594484664716),.UNSPECIFIED.);
#3430=B_SPLINE_SURFACE_WITH_KNOTS('',3,3,((#105425,#105426,#105427,#105428),
(#105429,#105430,#105431,#105432),(#105433,#105434,#105435,#105436),(#105437,
#105438,#105439,#105440)),.UNSPECIFIED.,.F.,.F.,.F.,(4,4),(4,4),(0.522097120206289,
1.00286823669298),(0.0265907346180629,0.0331702036889933),.UNSPECIFIED.);
#3431=B_SPLINE_SURFACE_WITH_KNOTS('',3,3,((#105448,#105449,#105450,#105451),
(#105452,#105453,#105454,#105455),(#105456,#105457,#105458,#105459),(#105460,
#105461,#105462,#105463)),.UNSPECIFIED.,.F.,.F.,.F.,(4,4),(4,4),(-0.00286848453269418,
0.477902879800586),(0.0400218729466597,0.0466073985929435),
 .UNSPECIFIED.);
#3432=B_SPLINE_SURFACE_WITH_KNOTS('',3,3,((#105480,#105481,#105482,#105483),
(#105484,#105485,#105486,#105487),(#105488,#105489,#105490,#105491),(#105492,
#105493,#105494,#105495)),.UNSPECIFIED.,.F.,.F.,.F.,(4,4),(4,4),(0.,1.00600014639743),
(0.0365944846645011,0.0466073985929158),.UNSPECIFIED.);
#3433=B_SPLINE_SURFACE_WITH_KNOTS('',3,3,((#105496,#105497,#105498,#105499),
(#105500,#105501,#105502,#105503),(#105504,#105505,#105506,#105507),(#105508,
#105509,#105510,#105511)),.UNSPECIFIED.,.F.,.F.,.F.,(4,4),(4,4),(-0.0028678012240359,
0.477902879799762),(0.0500263550858998,0.0565997133101407),
 .UNSPECIFIED.);
#3434=B_SPLINE_SURFACE_WITH_KNOTS('',3,3,((#105513,#105514,#105515,#105516),
(#105517,#105518,#105519,#105520),(#105521,#105522,#105523,#105524),(#105525,
#105526,#105527,#105528)),.UNSPECIFIED.,.F.,.F.,.F.,(4,4),(4,4),(0.522097120208308,
1.00286810177265),(0.0466073985929458,0.0531834925888935),.UNSPECIFIED.);
#3435=B_SPLINE_SURFACE_WITH_KNOTS('',3,3,((#105536,#105537,#105538,#105539),
(#105540,#105541,#105542,#105543),(#105544,#105545,#105546,#105547),(#105548,
#105549,#105550,#105551)),.UNSPECIFIED.,.F.,.F.,.F.,(4,4),(4,4),(-0.00286792598883179,
0.477902879798954),(0.0600156865494597,0.0665898698871172),
 .UNSPECIFIED.);
#3436=B_SPLINE_SURFACE_WITH_KNOTS('',3,3,((#105553,#105554,#105555,#105556),
(#105557,#105558,#105559,#105560),(#105561,#105562,#105563,#105564),(#105565,
#105566,#105567,#105568)),.UNSPECIFIED.,.F.,.F.,.F.,(4,4),(4,4),(0.522097120208306,
1.00286764392041),(0.056599713310142,0.0631721430887071),.UNSPECIFIED.);
#3437=B_SPLINE_SURFACE_WITH_KNOTS('',3,3,((#105584,#105585,#105586,#105587),
(#105588,#105589,#105590,#105591),(#105592,#105593,#105594,#105595),(#105596,
#105597,#105598,#105599)),.UNSPECIFIED.,.F.,.F.,.F.,(4,4),(4,4),(0.522097120207573,
1.00286833998592),(0.0665898698871191,0.0731716198748462),.UNSPECIFIED.);
#3438=B_SPLINE_SURFACE_WITH_KNOTS('',3,3,((#105600,#105601,#105602,#105603),
(#105604,#105605,#105606,#105607),(#105608,#105609,#105610,#105611),(#105612,
#105613,#105614,#105615)),.UNSPECIFIED.,.F.,.F.,.F.,(4,4),(4,4),(-0.00124731531130942,
0.209045111700277),(0.0700194292965537,0.0749900982978096),
 .UNSPECIFIED.);
#3439=B_SPLINE_SURFACE_WITH_KNOTS('',3,3,((#105622,#105623,#105624,#105625),
(#105626,#105627,#105628,#105629),(#105630,#105631,#105632,#105633),(#105634,
#105635,#105636,#105637)),.UNSPECIFIED.,.F.,.F.,.F.,(4,4),(4,4),(-0.0028679101440672,
0.477902879801822),(0.0100271466769372,0.0166015299239861),
 .UNSPECIFIED.);
#3440=B_SPLINE_SURFACE_WITH_KNOTS('',3,3,((#105639,#105640,#105641,#105642),
(#105643,#105644,#105645,#105646),(#105647,#105648,#105649,#105650),(#105651,
#105652,#105653,#105654)),.UNSPECIFIED.,.F.,.F.,.F.,(4,4),(4,4),(0.653230271507192,
1.00206901891588),(0.00656788395410992,0.0131849432121928),
 .UNSPECIFIED.);
#3441=B_SPLINE_SURFACE_WITH_KNOTS('',3,3,((#105662,#105663,#105664,#105665),
(#105666,#105667,#105668,#105669),(#105670,#105671,#105672,#105673),(#105674,
#105675,#105676,#105677)),.UNSPECIFIED.,.F.,.F.,.F.,(4,4),(4,4),(-0.00286780410472287,
0.477902879802779),(0.0200175229646914,0.0265907346180623),
 .UNSPECIFIED.);
#3442=B_SPLINE_SURFACE_WITH_KNOTS('',3,3,((#105679,#105680,#105681,#105682),
(#105683,#105684,#105685,#105686),(#105687,#105688,#105689,#105690),(#105691,
#105692,#105693,#105694)),.UNSPECIFIED.,.F.,.F.,.F.,(4,4),(4,4),(0.522097120202547,
1.00286753160126),(0.0166015299239893,0.0231736788075226),.UNSPECIFIED.);
#3443=B_SPLINE_SURFACE_WITH_KNOTS('',3,3,((#105696,#105697,#105698,#105699),
(#105700,#105701,#105702,#105703),(#105704,#105705,#105706,#105707),(#105708,
#105709,#105710,#105711)),.UNSPECIFIED.,.F.,.F.,.F.,(4,4),(4,4),(0.,1.0060000396138),
(0.0166015299239891,0.0265907346180633),.UNSPECIFIED.);
#3444=B_SPLINE_SURFACE_WITH_KNOTS('',3,3,((#105712,#105713,#105714,#105715),
(#105716,#105717,#105718,#105719),(#105720,#105721,#105722,#105723),(#105724,
#105725,#105726,#105727)),.UNSPECIFIED.,.F.,.F.,.F.,(4,4),(4,4),(-0.00286862201157427,
0.477902879802343),(0.0300094532292775,0.0365944846647152),
 .UNSPECIFIED.);
#3445=B_SPLINE_SURFACE_WITH_KNOTS('',3,3,((#105729,#105730,#105731,#105732),
(#105733,#105734,#105735,#105736),(#105737,#105738,#105739,#105740),(#105741,
#105742,#105743,#105744)),.UNSPECIFIED.,.F.,.F.,.F.,(4,4),(4,4),(0.52209712020368,
1.00286823669299),(0.0265907346180624,0.0331702036889926),.UNSPECIFIED.);
#3446=B_SPLINE_SURFACE_WITH_KNOTS('',3,3,((#105752,#105753,#105754,#105755),
(#105756,#105757,#105758,#105759),(#105760,#105761,#105762,#105763),(#105764,
#105765,#105766,#105767)),.UNSPECIFIED.,.F.,.F.,.F.,(4,4),(4,4),(-0.00286848453279188,
0.477902879802615),(0.040021872946661,0.0466073985929422),.UNSPECIFIED.);
#3447=B_SPLINE_SURFACE_WITH_KNOTS('',3,3,((#105784,#105785,#105786,#105787),
(#105788,#105789,#105790,#105791),(#105792,#105793,#105794,#105795),(#105796,
#105797,#105798,#105799)),.UNSPECIFIED.,.F.,.F.,.F.,(4,4),(4,4),(0.,1.0060001463974),
(0.0365944846645005,0.0466073985929165),.UNSPECIFIED.);
#3448=B_SPLINE_SURFACE_WITH_KNOTS('',3,3,((#105800,#105801,#105802,#105803),
(#105804,#105805,#105806,#105807),(#105808,#105809,#105810,#105811),(#105812,
#105813,#105814,#105815)),.UNSPECIFIED.,.F.,.F.,.F.,(4,4),(4,4),(-0.00286780122402792,
0.47790287980117),(0.0500263550859001,0.0565997133101407),.UNSPECIFIED.);
#3449=B_SPLINE_SURFACE_WITH_KNOTS('',3,3,((#105817,#105818,#105819,#105820),
(#105821,#105822,#105823,#105824),(#105825,#105826,#105827,#105828),(#105829,
#105830,#105831,#105832)),.UNSPECIFIED.,.F.,.F.,.F.,(4,4),(4,4),(0.522097120206262,
1.00286810177263),(0.0466073985929405,0.0531834925888929),.UNSPECIFIED.);
#3450=B_SPLINE_SURFACE_WITH_KNOTS('',3,3,((#105840,#105841,#105842,#105843),
(#105844,#105845,#105846,#105847),(#105848,#105849,#105850,#105851),(#105852,
#105853,#105854,#105855)),.UNSPECIFIED.,.F.,.F.,.F.,(4,4),(4,4),(-0.00286792598904179,
0.477902879800371),(0.060015686549462,0.0665898698871172),.UNSPECIFIED.);
#3451=B_SPLINE_SURFACE_WITH_KNOTS('',3,3,((#105857,#105858,#105859,#105860),
(#105861,#105862,#105863,#105864),(#105865,#105866,#105867,#105868),(#105869,
#105870,#105871,#105872)),.UNSPECIFIED.,.F.,.F.,.F.,(4,4),(4,4),(0.522097120207651,
1.00286764392039),(0.0565997133101423,0.0631721430887065),.UNSPECIFIED.);
#3452=B_SPLINE_SURFACE_WITH_KNOTS('',3,3,((#105888,#105889,#105890,#105891),
(#105892,#105893,#105894,#105895),(#105896,#105897,#105898,#105899),(#105900,
#105901,#105902,#105903)),.UNSPECIFIED.,.F.,.F.,.F.,(4,4),(4,4),(0.522097120207396,
1.0028683399859),(0.0665898698871197,0.0731716198748454),.UNSPECIFIED.);
#3453=B_SPLINE_SURFACE_WITH_KNOTS('',3,3,((#105904,#105905,#105906,#105907),
(#105908,#105909,#105910,#105911),(#105912,#105913,#105914,#105915),(#105916,
#105917,#105918,#105919)),.UNSPECIFIED.,.F.,.F.,.F.,(4,4),(4,4),(-0.0012473153096852,
0.209045111701724),(0.0700194292965668,0.0749900982978162),
 .UNSPECIFIED.);
#3454=B_SPLINE_SURFACE_WITH_KNOTS('',3,3,((#105926,#105927,#105928,#105929),
(#105930,#105931,#105932,#105933),(#105934,#105935,#105936,#105937),(#105938,
#105939,#105940,#105941)),.UNSPECIFIED.,.F.,.F.,.F.,(4,4),(4,4),(-0.00286791014414908,
0.477902879802002),(0.010027146676936,0.0166015299239886),.UNSPECIFIED.);
#3455=B_SPLINE_SURFACE_WITH_KNOTS('',3,3,((#105943,#105944,#105945,#105946),
(#105947,#105948,#105949,#105950),(#105951,#105952,#105953,#105954),(#105955,
#105956,#105957,#105958)),.UNSPECIFIED.,.F.,.F.,.F.,(4,4),(4,4),(0.653230271488838,
1.00206901891347),(0.00656788395410877,0.0131849432121942),
 .UNSPECIFIED.);
#3456=B_SPLINE_SURFACE_WITH_KNOTS('',3,3,((#105966,#105967,#105968,#105969),
(#105970,#105971,#105972,#105973),(#105974,#105975,#105976,#105977),(#105978,
#105979,#105980,#105981)),.UNSPECIFIED.,.F.,.F.,.F.,(4,4),(4,4),(-0.00286780410486259,
0.477902879801869),(0.0200175229646921,0.026590734618063),.UNSPECIFIED.);
#3457=B_SPLINE_SURFACE_WITH_KNOTS('',3,3,((#105983,#105984,#105985,#105986),
(#105987,#105988,#105989,#105990),(#105991,#105992,#105993,#105994),(#105995,
#105996,#105997,#105998)),.UNSPECIFIED.,.F.,.F.,.F.,(4,4),(4,4),(0.522097120201399,
1.00286753160122),(0.0166015299239896,0.023173678807522),.UNSPECIFIED.);
#3458=B_SPLINE_SURFACE_WITH_KNOTS('',3,3,((#106000,#106001,#106002,#106003),
(#106004,#106005,#106006,#106007),(#106008,#106009,#106010,#106011),(#106012,
#106013,#106014,#106015)),.UNSPECIFIED.,.F.,.F.,.F.,(4,4),(4,4),(0.,1.00600003961373),
(0.0166015299239904,0.0265907346180639),.UNSPECIFIED.);
#3459=B_SPLINE_SURFACE_WITH_KNOTS('',3,3,((#106016,#106017,#106018,#106019),
(#106020,#106021,#106022,#106023),(#106024,#106025,#106026,#106027),(#106028,
#106029,#106030,#106031)),.UNSPECIFIED.,.F.,.F.,.F.,(4,4),(4,4),(-0.002868622011642,
0.477902879803106),(0.0300094532292785,0.036594484664702),.UNSPECIFIED.);
#3460=B_SPLINE_SURFACE_WITH_KNOTS('',3,3,((#106033,#106034,#106035,#106036),
(#106037,#106038,#106039,#106040),(#106041,#106042,#106043,#106044),(#106045,
#106046,#106047,#106048)),.UNSPECIFIED.,.F.,.F.,.F.,(4,4),(4,4),(0.522097120201145,
1.00286823669288),(0.0265907346180634,0.0331702036051743),.UNSPECIFIED.);
#3461=B_SPLINE_SURFACE_WITH_KNOTS('',3,3,((#106056,#106057,#106058,#106059),
(#106060,#106061,#106062,#106063),(#106064,#106065,#106066,#106067),(#106068,
#106069,#106070,#106071)),.UNSPECIFIED.,.F.,.F.,.F.,(4,4),(4,4),(-0.00286848453282375,
0.477902879802511),(0.0400218729466607,0.0466073985929425),
 .UNSPECIFIED.);
#3462=B_SPLINE_SURFACE_WITH_KNOTS('',3,3,((#106088,#106089,#106090,#106091),
(#106092,#106093,#106094,#106095),(#106096,#106097,#106098,#106099),(#106100,
#106101,#106102,#106103)),.UNSPECIFIED.,.F.,.F.,.F.,(4,4),(4,4),(0.,1.00600014639744),
(0.0365944846644989,0.0466073985929176),.UNSPECIFIED.);
#3463=B_SPLINE_SURFACE_WITH_KNOTS('',3,3,((#106104,#106105,#106106,#106107),
(#106108,#106109,#106110,#106111),(#106112,#106113,#106114,#106115),(#106116,
#106117,#106118,#106119)),.UNSPECIFIED.,.F.,.F.,.F.,(4,4),(4,4),(-0.0028678012241247,
0.477902879802034),(0.0500263550859004,0.0565997133101407),
 .UNSPECIFIED.);
#3464=B_SPLINE_SURFACE_WITH_KNOTS('',3,3,((#106121,#106122,#106123,#106124),
(#106125,#106126,#106127,#106128),(#106129,#106130,#106131,#106132),(#106133,
#106134,#106135,#106136)),.UNSPECIFIED.,.F.,.F.,.F.,(4,4),(4,4),(0.522097120203794,
1.00286810177261),(0.0466073985929449,0.0531834925888935),.UNSPECIFIED.);
#3465=B_SPLINE_SURFACE_WITH_KNOTS('',3,3,((#106144,#106145,#106146,#106147),
(#106148,#106149,#106150,#106151),(#106152,#106153,#106154,#106155),(#106156,
#106157,#106158,#106159)),.UNSPECIFIED.,.F.,.F.,.F.,(4,4),(4,4),(-0.00286792598902487,
0.477902879801679),(0.0600156865494608,0.0665898698871168),
 .UNSPECIFIED.);
#3466=B_SPLINE_SURFACE_WITH_KNOTS('',3,3,((#106161,#106162,#106163,#106164),
(#106165,#106166,#106167,#106168),(#106169,#106170,#106171,#106172),(#106173,
#106174,#106175,#106176)),.UNSPECIFIED.,.F.,.F.,.F.,(4,4),(4,4),(0.522097120205029,
1.00286764392032),(0.0565997133101419,0.0631721430887061),.UNSPECIFIED.);
#3467=B_SPLINE_SURFACE_WITH_KNOTS('',3,3,((#106192,#106193,#106194,#106195),
(#106196,#106197,#106198,#106199),(#106200,#106201,#106202,#106203),(#106204,
#106205,#106206,#106207)),.UNSPECIFIED.,.F.,.F.,.F.,(4,4),(4,4),(0.522097120206208,
1.00286833998589),(0.0665898698871188,0.0731716198748447),.UNSPECIFIED.);
#3468=B_SPLINE_SURFACE_WITH_KNOTS('',3,3,((#106208,#106209,#106210,#106211),
(#106212,#106213,#106214,#106215),(#106216,#106217,#106218,#106219),(#106220,
#106221,#106222,#106223)),.UNSPECIFIED.,.F.,.F.,.F.,(4,4),(4,4),(-0.00124731530851986,
0.209045111703167),(0.0700194292965804,0.0749900982978226),
 .UNSPECIFIED.);
#3474=SHAPE_REPRESENTATION_RELATIONSHIP('SRR','None',#107952,#3484);
#3484=ADVANCED_BREP_SHAPE_REPRESENTATION('',(#3504),#107905);
#3494=STYLED_ITEM('',(#108010),#3504);
#3504=MANIFOLD_SOLID_BREP('Body1',#45542);
#3513=FACE_BOUND('',#8176,.T.);
#3566=PLANE('',#49124);
#3567=PLANE('',#49125);
#3568=PLANE('',#49126);
#3793=FACE_OUTER_BOUND('',#6721,.T.);
#3794=FACE_OUTER_BOUND('',#6722,.T.);
#3795=FACE_OUTER_BOUND('',#6723,.T.);
#3796=FACE_OUTER_BOUND('',#6724,.T.);
#3797=FACE_OUTER_BOUND('',#6725,.T.);
#3798=FACE_OUTER_BOUND('',#6726,.T.);
#3799=FACE_OUTER_BOUND('',#6727,.T.);
#3800=FACE_OUTER_BOUND('',#6728,.T.);
#3801=FACE_OUTER_BOUND('',#6729,.T.);
#3802=FACE_OUTER_BOUND('',#6730,.T.);
#3803=FACE_OUTER_BOUND('',#6731,.T.);
#3804=FACE_OUTER_BOUND('',#6732,.T.);
#3805=FACE_OUTER_BOUND('',#6733,.T.);
#3806=FACE_OUTER_BOUND('',#6734,.T.);
#3807=FACE_OUTER_BOUND('',#6735,.T.);
#3808=FACE_OUTER_BOUND('',#6736,.T.);
#3809=FACE_OUTER_BOUND('',#6737,.T.);
#3810=FACE_OUTER_BOUND('',#6738,.T.);
#3811=FACE_OUTER_BOUND('',#6739,.T.);
#3812=FACE_OUTER_BOUND('',#6740,.T.);
#3813=FACE_OUTER_BOUND('',#6741,.T.);
#3814=FACE_OUTER_BOUND('',#6742,.T.);
#3815=FACE_OUTER_BOUND('',#6743,.T.);
#3816=FACE_OUTER_BOUND('',#6744,.T.);
#3817=FACE_OUTER_BOUND('',#6745,.T.);
#3818=FACE_OUTER_BOUND('',#6746,.T.);
#3819=FACE_OUTER_BOUND('',#6747,.T.);
#3820=FACE_OUTER_BOUND('',#6748,.T.);
#3821=FACE_OUTER_BOUND('',#6749,.T.);
#3822=FACE_OUTER_BOUND('',#6750,.T.);
#3823=FACE_OUTER_BOUND('',#6751,.T.);
#3824=FACE_OUTER_BOUND('',#6752,.T.);
#3825=FACE_OUTER_BOUND('',#6753,.T.);
#3826=FACE_OUTER_BOUND('',#6754,.T.);
#3827=FACE_OUTER_BOUND('',#6755,.T.);
#3828=FACE_OUTER_BOUND('',#6756,.T.);
#3829=FACE_OUTER_BOUND('',#6757,.T.);
#3830=FACE_OUTER_BOUND('',#6758,.T.);
#3831=FACE_OUTER_BOUND('',#6759,.T.);
#3832=FACE_OUTER_BOUND('',#6760,.T.);
#3833=FACE_OUTER_BOUND('',#6761,.T.);
#3834=FACE_OUTER_BOUND('',#6762,.T.);
#3835=FACE_OUTER_BOUND('',#6763,.T.);
#3836=FACE_OUTER_BOUND('',#6764,.T.);
#3837=FACE_OUTER_BOUND('',#6765,.T.);
#3838=FACE_OUTER_BOUND('',#6766,.T.);
#3839=FACE_OUTER_BOUND('',#6767,.T.);
#3840=FACE_OUTER_BOUND('',#6768,.T.);
#3841=FACE_OUTER_BOUND('',#6769,.T.);
#3842=FACE_OUTER_BOUND('',#6770,.T.);
#3843=FACE_OUTER_BOUND('',#6771,.T.);
#3844=FACE_OUTER_BOUND('',#6772,.T.);
#3845=FACE_OUTER_BOUND('',#6773,.T.);
#3846=FACE_OUTER_BOUND('',#6774,.T.);
#3847=FACE_OUTER_BOUND('',#6775,.T.);
#3848=FACE_OUTER_BOUND('',#6776,.T.);
#3849=FACE_OUTER_BOUND('',#6777,.T.);
#3850=FACE_OUTER_BOUND('',#6778,.T.);
#3851=FACE_OUTER_BOUND('',#6779,.T.);
#3852=FACE_OUTER_BOUND('',#6780,.T.);
#3853=FACE_OUTER_BOUND('',#6781,.T.);
#3854=FACE_OUTER_BOUND('',#6782,.T.);
#3855=FACE_OUTER_BOUND('',#6783,.T.);
#3856=FACE_OUTER_BOUND('',#6784,.T.);
#3857=FACE_OUTER_BOUND('',#6785,.T.);
#3858=FACE_OUTER_BOUND('',#6786,.T.);
#3859=FACE_OUTER_BOUND('',#6787,.T.);
#3860=FACE_OUTER_BOUND('',#6788,.T.);
#3861=FACE_OUTER_BOUND('',#6789,.T.);
#3862=FACE_OUTER_BOUND('',#6790,.T.);
#3863=FACE_OUTER_BOUND('',#6791,.T.);
#3864=FACE_OUTER_BOUND('',#6792,.T.);
#3865=FACE_OUTER_BOUND('',#6793,.T.);
#3866=FACE_OUTER_BOUND('',#6794,.T.);
#3867=FACE_OUTER_BOUND('',#6795,.T.);
#3868=FACE_OUTER_BOUND('',#6796,.T.);
#3869=FACE_OUTER_BOUND('',#6797,.T.);
#3870=FACE_OUTER_BOUND('',#6798,.T.);
#3871=FACE_OUTER_BOUND('',#6799,.T.);
#3872=FACE_OUTER_BOUND('',#6800,.T.);
#3873=FACE_OUTER_BOUND('',#6801,.T.);
#3874=FACE_OUTER_BOUND('',#6802,.T.);
#3875=FACE_OUTER_BOUND('',#6803,.T.);
#3876=FACE_OUTER_BOUND('',#6804,.T.);
#3877=FACE_OUTER_BOUND('',#6805,.T.);
#3878=FACE_OUTER_BOUND('',#6806,.T.);
#3879=FACE_OUTER_BOUND('',#6807,.T.);
#3880=FACE_OUTER_BOUND('',#6808,.T.);
#3881=FACE_OUTER_BOUND('',#6809,.T.);
#3882=FACE_OUTER_BOUND('',#6810,.T.);
#3883=FACE_OUTER_BOUND('',#6811,.T.);
#3884=FACE_OUTER_BOUND('',#6812,.T.);
#3885=FACE_OUTER_BOUND('',#6813,.T.);
#3886=FACE_OUTER_BOUND('',#6814,.T.);
#3887=FACE_OUTER_BOUND('',#6815,.T.);
#3888=FACE_OUTER_BOUND('',#6816,.T.);
#3889=FACE_OUTER_BOUND('',#6817,.T.);
#3890=FACE_OUTER_BOUND('',#6818,.T.);
#3891=FACE_OUTER_BOUND('',#6819,.T.);
#3892=FACE_OUTER_BOUND('',#6820,.T.);
#3893=FACE_OUTER_BOUND('',#6821,.T.);
#3894=FACE_OUTER_BOUND('',#6822,.T.);
#3895=FACE_OUTER_BOUND('',#6823,.T.);
#3896=FACE_OUTER_BOUND('',#6824,.T.);
#3897=FACE_OUTER_BOUND('',#6825,.T.);
#3898=FACE_OUTER_BOUND('',#6826,.T.);
#3899=FACE_OUTER_BOUND('',#6827,.T.);
#3900=FACE_OUTER_BOUND('',#6828,.T.);
#3901=FACE_OUTER_BOUND('',#6829,.T.);
#3902=FACE_OUTER_BOUND('',#6830,.T.);
#3903=FACE_OUTER_BOUND('',#6831,.T.);
#3904=FACE_OUTER_BOUND('',#6832,.T.);
#3905=FACE_OUTER_BOUND('',#6833,.T.);
#3906=FACE_OUTER_BOUND('',#6834,.T.);
#3907=FACE_OUTER_BOUND('',#6835,.T.);
#3908=FACE_OUTER_BOUND('',#6836,.T.);
#3909=FACE_OUTER_BOUND('',#6837,.T.);
#3910=FACE_OUTER_BOUND('',#6838,.T.);
#3911=FACE_OUTER_BOUND('',#6839,.T.);
#3912=FACE_OUTER_BOUND('',#6840,.T.);
#3913=FACE_OUTER_BOUND('',#6841,.T.);
#3914=FACE_OUTER_BOUND('',#6842,.T.);
#3915=FACE_OUTER_BOUND('',#6843,.T.);
#3916=FACE_OUTER_BOUND('',#6844,.T.);
#3917=FACE_OUTER_BOUND('',#6845,.T.);
#3918=FACE_OUTER_BOUND('',#6846,.T.);
#3919=FACE_OUTER_BOUND('',#6847,.T.);
#3920=FACE_OUTER_BOUND('',#6848,.T.);
#3921=FACE_OUTER_BOUND('',#6849,.T.);
#3922=FACE_OUTER_BOUND('',#6850,.T.);
#3923=FACE_OUTER_BOUND('',#6851,.T.);
#3924=FACE_OUTER_BOUND('',#6852,.T.);
#3925=FACE_OUTER_BOUND('',#6853,.T.);
#3926=FACE_OUTER_BOUND('',#6854,.T.);
#3927=FACE_OUTER_BOUND('',#6855,.T.);
#3928=FACE_OUTER_BOUND('',#6856,.T.);
#3929=FACE_OUTER_BOUND('',#6857,.T.);
#3930=FACE_OUTER_BOUND('',#6858,.T.);
#3931=FACE_OUTER_BOUND('',#6859,.T.);
#3932=FACE_OUTER_BOUND('',#6860,.T.);
#3933=FACE_OUTER_BOUND('',#6861,.T.);
#3934=FACE_OUTER_BOUND('',#6862,.T.);
#3935=FACE_OUTER_BOUND('',#6863,.T.);
#3936=FACE_OUTER_BOUND('',#6864,.T.);
#3937=FACE_OUTER_BOUND('',#6865,.T.);
#3938=FACE_OUTER_BOUND('',#6866,.T.);
#3939=FACE_OUTER_BOUND('',#6867,.T.);
#3940=FACE_OUTER_BOUND('',#6868,.T.);
#3941=FACE_OUTER_BOUND('',#6869,.T.);
#3942=FACE_OUTER_BOUND('',#6870,.T.);
#3943=FACE_OUTER_BOUND('',#6871,.T.);
#3944=FACE_OUTER_BOUND('',#6872,.T.);
#3945=FACE_OUTER_BOUND('',#6873,.T.);
#3946=FACE_OUTER_BOUND('',#6874,.T.);
#3947=FACE_OUTER_BOUND('',#6875,.T.);
#3948=FACE_OUTER_BOUND('',#6876,.T.);
#3949=FACE_OUTER_BOUND('',#6877,.T.);
#3950=FACE_OUTER_BOUND('',#6878,.T.);
#3951=FACE_OUTER_BOUND('',#6879,.T.);
#3952=FACE_OUTER_BOUND('',#6880,.T.);
#3953=FACE_OUTER_BOUND('',#6881,.T.);
#3954=FACE_OUTER_BOUND('',#6882,.T.);
#3955=FACE_OUTER_BOUND('',#6883,.T.);
#3956=FACE_OUTER_BOUND('',#6884,.T.);
#3957=FACE_OUTER_BOUND('',#6885,.T.);
#3958=FACE_OUTER_BOUND('',#6886,.T.);
#3959=FACE_OUTER_BOUND('',#6887,.T.);
#3960=FACE_OUTER_BOUND('',#6888,.T.);
#3961=FACE_OUTER_BOUND('',#6889,.T.);
#3962=FACE_OUTER_BOUND('',#6890,.T.);
#3963=FACE_OUTER_BOUND('',#6891,.T.);
#3964=FACE_OUTER_BOUND('',#6892,.T.);
#3965=FACE_OUTER_BOUND('',#6893,.T.);
#3966=FACE_OUTER_BOUND('',#6894,.T.);
#3967=FACE_OUTER_BOUND('',#6895,.T.);
#3968=FACE_OUTER_BOUND('',#6896,.T.);
#3969=FACE_OUTER_BOUND('',#6897,.T.);
#3970=FACE_OUTER_BOUND('',#6898,.T.);
#3971=FACE_OUTER_BOUND('',#6899,.T.);
#3972=FACE_OUTER_BOUND('',#6900,.T.);
#3973=FACE_OUTER_BOUND('',#6901,.T.);
#3974=FACE_OUTER_BOUND('',#6902,.T.);
#3975=FACE_OUTER_BOUND('',#6903,.T.);
#3976=FACE_OUTER_BOUND('',#6904,.T.);
#3977=FACE_OUTER_BOUND('',#6905,.T.);
#3978=FACE_OUTER_BOUND('',#6906,.T.);
#3979=FACE_OUTER_BOUND('',#6907,.T.);
#3980=FACE_OUTER_BOUND('',#6908,.T.);
#3981=FACE_OUTER_BOUND('',#6909,.T.);
#3982=FACE_OUTER_BOUND('',#6910,.T.);
#3983=FACE_OUTER_BOUND('',#6911,.T.);
#3984=FACE_OUTER_BOUND('',#6912,.T.);
#3985=FACE_OUTER_BOUND('',#6913,.T.);
#3986=FACE_OUTER_BOUND('',#6914,.T.);
#3987=FACE_OUTER_BOUND('',#6915,.T.);
#3988=FACE_OUTER_BOUND('',#6916,.T.);
#3989=FACE_OUTER_BOUND('',#6917,.T.);
#3990=FACE_OUTER_BOUND('',#6918,.T.);
#3991=FACE_OUTER_BOUND('',#6919,.T.);
#3992=FACE_OUTER_BOUND('',#6920,.T.);
#3993=FACE_OUTER_BOUND('',#6921,.T.);
#3994=FACE_OUTER_BOUND('',#6922,.T.);
#3995=FACE_OUTER_BOUND('',#6923,.T.);
#3996=FACE_OUTER_BOUND('',#6924,.T.);
#3997=FACE_OUTER_BOUND('',#6925,.T.);
#3998=FACE_OUTER_BOUND('',#6926,.T.);
#3999=FACE_OUTER_BOUND('',#6927,.T.);
#4000=FACE_OUTER_BOUND('',#6928,.T.);
#4001=FACE_OUTER_BOUND('',#6929,.T.);
#4002=FACE_OUTER_BOUND('',#6930,.T.);
#4003=FACE_OUTER_BOUND('',#6931,.T.);
#4004=FACE_OUTER_BOUND('',#6932,.T.);
#4005=FACE_OUTER_BOUND('',#6933,.T.);
#4006=FACE_OUTER_BOUND('',#6934,.T.);
#4007=FACE_OUTER_BOUND('',#6935,.T.);
#4008=FACE_OUTER_BOUND('',#6936,.T.);
#4009=FACE_OUTER_BOUND('',#6937,.T.);
#4010=FACE_OUTER_BOUND('',#6938,.T.);
#4011=FACE_OUTER_BOUND('',#6939,.T.);
#4012=FACE_OUTER_BOUND('',#6940,.T.);
#4013=FACE_OUTER_BOUND('',#6941,.T.);
#4014=FACE_OUTER_BOUND('',#6942,.T.);
#4015=FACE_OUTER_BOUND('',#6943,.T.);
#4016=FACE_OUTER_BOUND('',#6944,.T.);
#4017=FACE_OUTER_BOUND('',#6945,.T.);
#4018=FACE_OUTER_BOUND('',#6946,.T.);
#4019=FACE_OUTER_BOUND('',#6947,.T.);
#4020=FACE_OUTER_BOUND('',#6948,.T.);
#4021=FACE_OUTER_BOUND('',#6949,.T.);
#4022=FACE_OUTER_BOUND('',#6950,.T.);
#4023=FACE_OUTER_BOUND('',#6951,.T.);
#4024=FACE_OUTER_BOUND('',#6952,.T.);
#4025=FACE_OUTER_BOUND('',#6953,.T.);
#4026=FACE_OUTER_BOUND('',#6954,.T.);
#4027=FACE_OUTER_BOUND('',#6955,.T.);
#4028=FACE_OUTER_BOUND('',#6956,.T.);
#4029=FACE_OUTER_BOUND('',#6957,.T.);
#4030=FACE_OUTER_BOUND('',#6958,.T.);
#4031=FACE_OUTER_BOUND('',#6959,.T.);
#4032=FACE_OUTER_BOUND('',#6960,.T.);
#4033=FACE_OUTER_BOUND('',#6961,.T.);
#4034=FACE_OUTER_BOUND('',#6962,.T.);
#4035=FACE_OUTER_BOUND('',#6963,.T.);
#4036=FACE_OUTER_BOUND('',#6964,.T.);
#4037=FACE_OUTER_BOUND('',#6965,.T.);
#4038=FACE_OUTER_BOUND('',#6966,.T.);
#4039=FACE_OUTER_BOUND('',#6967,.T.);
#4040=FACE_OUTER_BOUND('',#6968,.T.);
#4041=FACE_OUTER_BOUND('',#6969,.T.);
#4042=FACE_OUTER_BOUND('',#6970,.T.);
#4043=FACE_OUTER_BOUND('',#6971,.T.);
#4044=FACE_OUTER_BOUND('',#6972,.T.);
#4045=FACE_OUTER_BOUND('',#6973,.T.);
#4046=FACE_OUTER_BOUND('',#6974,.T.);
#4047=FACE_OUTER_BOUND('',#6975,.T.);
#4048=FACE_OUTER_BOUND('',#6976,.T.);
#4049=FACE_OUTER_BOUND('',#6977,.T.);
#4050=FACE_OUTER_BOUND('',#6978,.T.);
#4051=FACE_OUTER_BOUND('',#6979,.T.);
#4052=FACE_OUTER_BOUND('',#6980,.T.);
#4053=FACE_OUTER_BOUND('',#6981,.T.);
#4054=FACE_OUTER_BOUND('',#6982,.T.);
#4055=FACE_OUTER_BOUND('',#6983,.T.);
#4056=FACE_OUTER_BOUND('',#6984,.T.);
#4057=FACE_OUTER_BOUND('',#6985,.T.);
#4058=FACE_OUTER_BOUND('',#6986,.T.);
#4059=FACE_OUTER_BOUND('',#6987,.T.);
#4060=FACE_OUTER_BOUND('',#6988,.T.);
#4061=FACE_OUTER_BOUND('',#6989,.T.);
#4062=FACE_OUTER_BOUND('',#6990,.T.);
#4063=FACE_OUTER_BOUND('',#6991,.T.);
#4064=FACE_OUTER_BOUND('',#6992,.T.);
#4065=FACE_OUTER_BOUND('',#6993,.T.);
#4066=FACE_OUTER_BOUND('',#6994,.T.);
#4067=FACE_OUTER_BOUND('',#6995,.T.);
#4068=FACE_OUTER_BOUND('',#6996,.T.);
#4069=FACE_OUTER_BOUND('',#6997,.T.);
#4070=FACE_OUTER_BOUND('',#6998,.T.);
#4071=FACE_OUTER_BOUND('',#6999,.T.);
#4072=FACE_OUTER_BOUND('',#7000,.T.);
#4073=FACE_OUTER_BOUND('',#7001,.T.);
#4074=FACE_OUTER_BOUND('',#7002,.T.);
#4075=FACE_OUTER_BOUND('',#7003,.T.);
#4076=FACE_OUTER_BOUND('',#7004,.T.);
#4077=FACE_OUTER_BOUND('',#7005,.T.);
#4078=FACE_OUTER_BOUND('',#7006,.T.);
#4079=FACE_OUTER_BOUND('',#7007,.T.);
#4080=FACE_OUTER_BOUND('',#7008,.T.);
#4081=FACE_OUTER_BOUND('',#7009,.T.);
#4082=FACE_OUTER_BOUND('',#7010,.T.);
#4083=FACE_OUTER_BOUND('',#7011,.T.);
#4084=FACE_OUTER_BOUND('',#7012,.T.);
#4085=FACE_OUTER_BOUND('',#7013,.T.);
#4086=FACE_OUTER_BOUND('',#7014,.T.);
#4087=FACE_OUTER_BOUND('',#7015,.T.);
#4088=FACE_OUTER_BOUND('',#7016,.T.);
#4089=FACE_OUTER_BOUND('',#7017,.T.);
#4090=FACE_OUTER_BOUND('',#7018,.T.);
#4091=FACE_OUTER_BOUND('',#7019,.T.);
#4092=FACE_OUTER_BOUND('',#7020,.T.);
#4093=FACE_OUTER_BOUND('',#7021,.T.);
#4094=FACE_OUTER_BOUND('',#7022,.T.);
#4095=FACE_OUTER_BOUND('',#7023,.T.);
#4096=FACE_OUTER_BOUND('',#7024,.T.);
#4097=FACE_OUTER_BOUND('',#7025,.T.);
#4098=FACE_OUTER_BOUND('',#7026,.T.);
#4099=FACE_OUTER_BOUND('',#7027,.T.);
#4100=FACE_OUTER_BOUND('',#7028,.T.);
#4101=FACE_OUTER_BOUND('',#7029,.T.);
#4102=FACE_OUTER_BOUND('',#7030,.T.);
#4103=FACE_OUTER_BOUND('',#7031,.T.);
#4104=FACE_OUTER_BOUND('',#7032,.T.);
#4105=FACE_OUTER_BOUND('',#7033,.T.);
#4106=FACE_OUTER_BOUND('',#7034,.T.);
#4107=FACE_OUTER_BOUND('',#7035,.T.);
#4108=FACE_OUTER_BOUND('',#7036,.T.);
#4109=FACE_OUTER_BOUND('',#7037,.T.);
#4110=FACE_OUTER_BOUND('',#7038,.T.);
#4111=FACE_OUTER_BOUND('',#7039,.T.);
#4112=FACE_OUTER_BOUND('',#7040,.T.);
#4113=FACE_OUTER_BOUND('',#7041,.T.);
#4114=FACE_OUTER_BOUND('',#7042,.T.);
#4115=FACE_OUTER_BOUND('',#7043,.T.);
#4116=FACE_OUTER_BOUND('',#7044,.T.);
#4117=FACE_OUTER_BOUND('',#7045,.T.);
#4118=FACE_OUTER_BOUND('',#7046,.T.);
#4119=FACE_OUTER_BOUND('',#7047,.T.);
#4120=FACE_OUTER_BOUND('',#7048,.T.);
#4121=FACE_OUTER_BOUND('',#7049,.T.);
#4122=FACE_OUTER_BOUND('',#7050,.T.);
#4123=FACE_OUTER_BOUND('',#7051,.T.);
#4124=FACE_OUTER_BOUND('',#7052,.T.);
#4125=FACE_OUTER_BOUND('',#7053,.T.);
#4126=FACE_OUTER_BOUND('',#7054,.T.);
#4127=FACE_OUTER_BOUND('',#7055,.T.);
#4128=FACE_OUTER_BOUND('',#7056,.T.);
#4129=FACE_OUTER_BOUND('',#7057,.T.);
#4130=FACE_OUTER_BOUND('',#7058,.T.);
#4131=FACE_OUTER_BOUND('',#7059,.T.);
#4132=FACE_OUTER_BOUND('',#7060,.T.);
#4133=FACE_OUTER_BOUND('',#7061,.T.);
#4134=FACE_OUTER_BOUND('',#7062,.T.);
#4135=FACE_OUTER_BOUND('',#7063,.T.);
#4136=FACE_OUTER_BOUND('',#7064,.T.);
#4137=FACE_OUTER_BOUND('',#7065,.T.);
#4138=FACE_OUTER_BOUND('',#7066,.T.);
#4139=FACE_OUTER_BOUND('',#7067,.T.);
#4140=FACE_OUTER_BOUND('',#7068,.T.);
#4141=FACE_OUTER_BOUND('',#7069,.T.);
#4142=FACE_OUTER_BOUND('',#7070,.T.);
#4143=FACE_OUTER_BOUND('',#7071,.T.);
#4144=FACE_OUTER_BOUND('',#7072,.T.);
#4145=FACE_OUTER_BOUND('',#7073,.T.);
#4146=FACE_OUTER_BOUND('',#7074,.T.);
#4147=FACE_OUTER_BOUND('',#7075,.T.);
#4148=FACE_OUTER_BOUND('',#7076,.T.);
#4149=FACE_OUTER_BOUND('',#7077,.T.);
#4150=FACE_OUTER_BOUND('',#7078,.T.);
#4151=FACE_OUTER_BOUND('',#7079,.T.);
#4152=FACE_OUTER_BOUND('',#7080,.T.);
#4153=FACE_OUTER_BOUND('',#7081,.T.);
#4154=FACE_OUTER_BOUND('',#7082,.T.);
#4155=FACE_OUTER_BOUND('',#7083,.T.);
#4156=FACE_OUTER_BOUND('',#7084,.T.);
#4157=FACE_OUTER_BOUND('',#7085,.T.);
#4158=FACE_OUTER_BOUND('',#7086,.T.);
#4159=FACE_OUTER_BOUND('',#7087,.T.);
#4160=FACE_OUTER_BOUND('',#7088,.T.);
#4161=FACE_OUTER_BOUND('',#7089,.T.);
#4162=FACE_OUTER_BOUND('',#7090,.T.);
#4163=FACE_OUTER_BOUND('',#7091,.T.);
#4164=FACE_OUTER_BOUND('',#7092,.T.);
#4165=FACE_OUTER_BOUND('',#7093,.T.);
#4166=FACE_OUTER_BOUND('',#7094,.T.);
#4167=FACE_OUTER_BOUND('',#7095,.T.);
#4168=FACE_OUTER_BOUND('',#7096,.T.);
#4169=FACE_OUTER_BOUND('',#7097,.T.);
#4170=FACE_OUTER_BOUND('',#7098,.T.);
#4171=FACE_OUTER_BOUND('',#7099,.T.);
#4172=FACE_OUTER_BOUND('',#7100,.T.);
#4173=FACE_OUTER_BOUND('',#7101,.T.);
#4174=FACE_OUTER_BOUND('',#7102,.T.);
#4175=FACE_OUTER_BOUND('',#7103,.T.);
#4176=FACE_OUTER_BOUND('',#7104,.T.);
#4177=FACE_OUTER_BOUND('',#7105,.T.);
#4178=FACE_OUTER_BOUND('',#7106,.T.);
#4179=FACE_OUTER_BOUND('',#7107,.T.);
#4180=FACE_OUTER_BOUND('',#7108,.T.);
#4181=FACE_OUTER_BOUND('',#7109,.T.);
#4182=FACE_OUTER_BOUND('',#7110,.T.);
#4183=FACE_OUTER_BOUND('',#7111,.T.);
#4184=FACE_OUTER_BOUND('',#7112,.T.);
#4185=FACE_OUTER_BOUND('',#7113,.T.);
#4186=FACE_OUTER_BOUND('',#7114,.T.);
#4187=FACE_OUTER_BOUND('',#7115,.T.);
#4188=FACE_OUTER_BOUND('',#7116,.T.);
#4189=FACE_OUTER_BOUND('',#7117,.T.);
#4190=FACE_OUTER_BOUND('',#7118,.T.);
#4191=FACE_OUTER_BOUND('',#7119,.T.);
#4192=FACE_OUTER_BOUND('',#7120,.T.);
#4193=FACE_OUTER_BOUND('',#7121,.T.);
#4194=FACE_OUTER_BOUND('',#7122,.T.);
#4195=FACE_OUTER_BOUND('',#7123,.T.);
#4196=FACE_OUTER_BOUND('',#7124,.T.);
#4197=FACE_OUTER_BOUND('',#7125,.T.);
#4198=FACE_OUTER_BOUND('',#7126,.T.);
#4199=FACE_OUTER_BOUND('',#7127,.T.);
#4200=FACE_OUTER_BOUND('',#7128,.T.);
#4201=FACE_OUTER_BOUND('',#7129,.T.);
#4202=FACE_OUTER_BOUND('',#7130,.T.);
#4203=FACE_OUTER_BOUND('',#7131,.T.);
#4204=FACE_OUTER_BOUND('',#7132,.T.);
#4205=FACE_OUTER_BOUND('',#7133,.T.);
#4206=FACE_OUTER_BOUND('',#7134,.T.);
#4207=FACE_OUTER_BOUND('',#7135,.T.);
#4208=FACE_OUTER_BOUND('',#7136,.T.);
#4209=FACE_OUTER_BOUND('',#7137,.T.);
#4210=FACE_OUTER_BOUND('',#7138,.T.);
#4211=FACE_OUTER_BOUND('',#7139,.T.);
#4212=FACE_OUTER_BOUND('',#7140,.T.);
#4213=FACE_OUTER_BOUND('',#7141,.T.);
#4214=FACE_OUTER_BOUND('',#7142,.T.);
#4215=FACE_OUTER_BOUND('',#7143,.T.);
#4216=FACE_OUTER_BOUND('',#7144,.T.);
#4217=FACE_OUTER_BOUND('',#7145,.T.);
#4218=FACE_OUTER_BOUND('',#7146,.T.);
#4219=FACE_OUTER_BOUND('',#7147,.T.);
#4220=FACE_OUTER_BOUND('',#7148,.T.);
#4221=FACE_OUTER_BOUND('',#7149,.T.);
#4222=FACE_OUTER_BOUND('',#7150,.T.);
#4223=FACE_OUTER_BOUND('',#7151,.T.);
#4224=FACE_OUTER_BOUND('',#7152,.T.);
#4225=FACE_OUTER_BOUND('',#7153,.T.);
#4226=FACE_OUTER_BOUND('',#7154,.T.);
#4227=FACE_OUTER_BOUND('',#7155,.T.);
#4228=FACE_OUTER_BOUND('',#7156,.T.);
#4229=FACE_OUTER_BOUND('',#7157,.T.);
#4230=FACE_OUTER_BOUND('',#7158,.T.);
#4231=FACE_OUTER_BOUND('',#7159,.T.);
#4232=FACE_OUTER_BOUND('',#7160,.T.);
#4233=FACE_OUTER_BOUND('',#7161,.T.);
#4234=FACE_OUTER_BOUND('',#7162,.T.);
#4235=FACE_OUTER_BOUND('',#7163,.T.);
#4236=FACE_OUTER_BOUND('',#7164,.T.);
#4237=FACE_OUTER_BOUND('',#7165,.T.);
#4238=FACE_OUTER_BOUND('',#7166,.T.);
#4239=FACE_OUTER_BOUND('',#7167,.T.);
#4240=FACE_OUTER_BOUND('',#7168,.T.);
#4241=FACE_OUTER_BOUND('',#7169,.T.);
#4242=FACE_OUTER_BOUND('',#7170,.T.);
#4243=FACE_OUTER_BOUND('',#7171,.T.);
#4244=FACE_OUTER_BOUND('',#7172,.T.);
#4245=FACE_OUTER_BOUND('',#7173,.T.);
#4246=FACE_OUTER_BOUND('',#7174,.T.);
#4247=FACE_OUTER_BOUND('',#7175,.T.);
#4248=FACE_OUTER_BOUND('',#7176,.T.);
#4249=FACE_OUTER_BOUND('',#7177,.T.);
#4250=FACE_OUTER_BOUND('',#7178,.T.);
#4251=FACE_OUTER_BOUND('',#7179,.T.);
#4252=FACE_OUTER_BOUND('',#7180,.T.);
#4253=FACE_OUTER_BOUND('',#7181,.T.);
#4254=FACE_OUTER_BOUND('',#7182,.T.);
#4255=FACE_OUTER_BOUND('',#7183,.T.);
#4256=FACE_OUTER_BOUND('',#7184,.T.);
#4257=FACE_OUTER_BOUND('',#7185,.T.);
#4258=FACE_OUTER_BOUND('',#7186,.T.);
#4259=FACE_OUTER_BOUND('',#7187,.T.);
#4260=FACE_OUTER_BOUND('',#7188,.T.);
#4261=FACE_OUTER_BOUND('',#7189,.T.);
#4262=FACE_OUTER_BOUND('',#7190,.T.);
#4263=FACE_OUTER_BOUND('',#7191,.T.);
#4264=FACE_OUTER_BOUND('',#7192,.T.);
#4265=FACE_OUTER_BOUND('',#7193,.T.);
#4266=FACE_OUTER_BOUND('',#7194,.T.);
#4267=FACE_OUTER_BOUND('',#7195,.T.);
#4268=FACE_OUTER_BOUND('',#7196,.T.);
#4269=FACE_OUTER_BOUND('',#7197,.T.);
#4270=FACE_OUTER_BOUND('',#7198,.T.);
#4271=FACE_OUTER_BOUND('',#7199,.T.);
#4272=FACE_OUTER_BOUND('',#7200,.T.);
#4273=FACE_OUTER_BOUND('',#7201,.T.);
#4274=FACE_OUTER_BOUND('',#7202,.T.);
#4275=FACE_OUTER_BOUND('',#7203,.T.);
#4276=FACE_OUTER_BOUND('',#7204,.T.);
#4277=FACE_OUTER_BOUND('',#7205,.T.);
#4278=FACE_OUTER_BOUND('',#7206,.T.);
#4279=FACE_OUTER_BOUND('',#7207,.T.);
#4280=FACE_OUTER_BOUND('',#7208,.T.);
#4281=FACE_OUTER_BOUND('',#7209,.T.);
#4282=FACE_OUTER_BOUND('',#7210,.T.);
#4283=FACE_OUTER_BOUND('',#7211,.T.);
#4284=FACE_OUTER_BOUND('',#7212,.T.);
#4285=FACE_OUTER_BOUND('',#7213,.T.);
#4286=FACE_OUTER_BOUND('',#7214,.T.);
#4287=FACE_OUTER_BOUND('',#7215,.T.);
#4288=FACE_OUTER_BOUND('',#7216,.T.);
#4289=FACE_OUTER_BOUND('',#7217,.T.);
#4290=FACE_OUTER_BOUND('',#7218,.T.);
#4291=FACE_OUTER_BOUND('',#7219,.T.);
#4292=FACE_OUTER_BOUND('',#7220,.T.);
#4293=FACE_OUTER_BOUND('',#7221,.T.);
#4294=FACE_OUTER_BOUND('',#7222,.T.);
#4295=FACE_OUTER_BOUND('',#7223,.T.);
#4296=FACE_OUTER_BOUND('',#7224,.T.);
#4297=FACE_OUTER_BOUND('',#7225,.T.);
#4298=FACE_OUTER_BOUND('',#7226,.T.);
#4299=FACE_OUTER_BOUND('',#7227,.T.);
#4300=FACE_OUTER_BOUND('',#7228,.T.);
#4301=FACE_OUTER_BOUND('',#7229,.T.);
#4302=FACE_OUTER_BOUND('',#7230,.T.);
#4303=FACE_OUTER_BOUND('',#7231,.T.);
#4304=FACE_OUTER_BOUND('',#7232,.T.);
#4305=FACE_OUTER_BOUND('',#7233,.T.);
#4306=FACE_OUTER_BOUND('',#7234,.T.);
#4307=FACE_OUTER_BOUND('',#7235,.T.);
#4308=FACE_OUTER_BOUND('',#7236,.T.);
#4309=FACE_OUTER_BOUND('',#7237,.T.);
#4310=FACE_OUTER_BOUND('',#7238,.T.);
#4311=FACE_OUTER_BOUND('',#7239,.T.);
#4312=FACE_OUTER_BOUND('',#7240,.T.);
#4313=FACE_OUTER_BOUND('',#7241,.T.);
#4314=FACE_OUTER_BOUND('',#7242,.T.);
#4315=FACE_OUTER_BOUND('',#7243,.T.);
#4316=FACE_OUTER_BOUND('',#7244,.T.);
#4317=FACE_OUTER_BOUND('',#7245,.T.);
#4318=FACE_OUTER_BOUND('',#7246,.T.);
#4319=FACE_OUTER_BOUND('',#7247,.T.);
#4320=FACE_OUTER_BOUND('',#7248,.T.);
#4321=FACE_OUTER_BOUND('',#7249,.T.);
#4322=FACE_OUTER_BOUND('',#7250,.T.);
#4323=FACE_OUTER_BOUND('',#7251,.T.);
#4324=FACE_OUTER_BOUND('',#7252,.T.);
#4325=FACE_OUTER_BOUND('',#7253,.T.);
#4326=FACE_OUTER_BOUND('',#7254,.T.);
#4327=FACE_OUTER_BOUND('',#7255,.T.);
#4328=FACE_OUTER_BOUND('',#7256,.T.);
#4329=FACE_OUTER_BOUND('',#7257,.T.);
#4330=FACE_OUTER_BOUND('',#7258,.T.);
#4331=FACE_OUTER_BOUND('',#7259,.T.);
#4332=FACE_OUTER_BOUND('',#7260,.T.);
#4333=FACE_OUTER_BOUND('',#7261,.T.);
#4334=FACE_OUTER_BOUND('',#7262,.T.);
#4335=FACE_OUTER_BOUND('',#7263,.T.);
#4336=FACE_OUTER_BOUND('',#7264,.T.);
#4337=FACE_OUTER_BOUND('',#7265,.T.);
#4338=FACE_OUTER_BOUND('',#7266,.T.);
#4339=FACE_OUTER_BOUND('',#7267,.T.);
#4340=FACE_OUTER_BOUND('',#7268,.T.);
#4341=FACE_OUTER_BOUND('',#7269,.T.);
#4342=FACE_OUTER_BOUND('',#7270,.T.);
#4343=FACE_OUTER_BOUND('',#7271,.T.);
#4344=FACE_OUTER_BOUND('',#7272,.T.);
#4345=FACE_OUTER_BOUND('',#7273,.T.);
#4346=FACE_OUTER_BOUND('',#7274,.T.);
#4347=FACE_OUTER_BOUND('',#7275,.T.);
#4348=FACE_OUTER_BOUND('',#7276,.T.);
#4349=FACE_OUTER_BOUND('',#7277,.T.);
#4350=FACE_OUTER_BOUND('',#7278,.T.);
#4351=FACE_OUTER_BOUND('',#7279,.T.);
#4352=FACE_OUTER_BOUND('',#7280,.T.);
#4353=FACE_OUTER_BOUND('',#7281,.T.);
#4354=FACE_OUTER_BOUND('',#7282,.T.);
#4355=FACE_OUTER_BOUND('',#7283,.T.);
#4356=FACE_OUTER_BOUND('',#7284,.T.);
#4357=FACE_OUTER_BOUND('',#7285,.T.);
#4358=FACE_OUTER_BOUND('',#7286,.T.);
#4359=FACE_OUTER_BOUND('',#7287,.T.);
#4360=FACE_OUTER_BOUND('',#7288,.T.);
#4361=FACE_OUTER_BOUND('',#7289,.T.);
#4362=FACE_OUTER_BOUND('',#7290,.T.);
#4363=FACE_OUTER_BOUND('',#7291,.T.);
#4364=FACE_OUTER_BOUND('',#7292,.T.);
#4365=FACE_OUTER_BOUND('',#7293,.T.);
#4366=FACE_OUTER_BOUND('',#7294,.T.);
#4367=FACE_OUTER_BOUND('',#7295,.T.);
#4368=FACE_OUTER_BOUND('',#7296,.T.);
#4369=FACE_OUTER_BOUND('',#7297,.T.);
#4370=FACE_OUTER_BOUND('',#7298,.T.);
#4371=FACE_OUTER_BOUND('',#7299,.T.);
#4372=FACE_OUTER_BOUND('',#7300,.T.);
#4373=FACE_OUTER_BOUND('',#7301,.T.);
#4374=FACE_OUTER_BOUND('',#7302,.T.);
#4375=FACE_OUTER_BOUND('',#7303,.T.);
#4376=FACE_OUTER_BOUND('',#7304,.T.);
#4377=FACE_OUTER_BOUND('',#7305,.T.);
#4378=FACE_OUTER_BOUND('',#7306,.T.);
#4379=FACE_OUTER_BOUND('',#7307,.T.);
#4380=FACE_OUTER_BOUND('',#7308,.T.);
#4381=FACE_OUTER_BOUND('',#7309,.T.);
#4382=FACE_OUTER_BOUND('',#7310,.T.);
#4383=FACE_OUTER_BOUND('',#7311,.T.);
#4384=FACE_OUTER_BOUND('',#7312,.T.);
#4385=FACE_OUTER_BOUND('',#7313,.T.);
#4386=FACE_OUTER_BOUND('',#7314,.T.);
#4387=FACE_OUTER_BOUND('',#7315,.T.);
#4388=FACE_OUTER_BOUND('',#7316,.T.);
#4389=FACE_OUTER_BOUND('',#7317,.T.);
#4390=FACE_OUTER_BOUND('',#7318,.T.);
#4391=FACE_OUTER_BOUND('',#7319,.T.);
#4392=FACE_OUTER_BOUND('',#7320,.T.);
#4393=FACE_OUTER_BOUND('',#7321,.T.);
#4394=FACE_OUTER_BOUND('',#7322,.T.);
#4395=FACE_OUTER_BOUND('',#7323,.T.);
#4396=FACE_OUTER_BOUND('',#7324,.T.);
#4397=FACE_OUTER_BOUND('',#7325,.T.);
#4398=FACE_OUTER_BOUND('',#7326,.T.);
#4399=FACE_OUTER_BOUND('',#7327,.T.);
#4400=FACE_OUTER_BOUND('',#7328,.T.);
#4401=FACE_OUTER_BOUND('',#7329,.T.);
#4402=FACE_OUTER_BOUND('',#7330,.T.);
#4403=FACE_OUTER_BOUND('',#7331,.T.);
#4404=FACE_OUTER_BOUND('',#7332,.T.);
#4405=FACE_OUTER_BOUND('',#7333,.T.);
#4406=FACE_OUTER_BOUND('',#7334,.T.);
#4407=FACE_OUTER_BOUND('',#7335,.T.);
#4408=FACE_OUTER_BOUND('',#7336,.T.);
#4409=FACE_OUTER_BOUND('',#7337,.T.);
#4410=FACE_OUTER_BOUND('',#7338,.T.);
#4411=FACE_OUTER_BOUND('',#7339,.T.);
#4412=FACE_OUTER_BOUND('',#7340,.T.);
#4413=FACE_OUTER_BOUND('',#7341,.T.);
#4414=FACE_OUTER_BOUND('',#7342,.T.);
#4415=FACE_OUTER_BOUND('',#7343,.T.);
#4416=FACE_OUTER_BOUND('',#7344,.T.);
#4417=FACE_OUTER_BOUND('',#7345,.T.);
#4418=FACE_OUTER_BOUND('',#7346,.T.);
#4419=FACE_OUTER_BOUND('',#7347,.T.);
#4420=FACE_OUTER_BOUND('',#7348,.T.);
#4421=FACE_OUTER_BOUND('',#7349,.T.);
#4422=FACE_OUTER_BOUND('',#7350,.T.);
#4423=FACE_OUTER_BOUND('',#7351,.T.);
#4424=FACE_OUTER_BOUND('',#7352,.T.);
#4425=FACE_OUTER_BOUND('',#7353,.T.);
#4426=FACE_OUTER_BOUND('',#7354,.T.);
#4427=FACE_OUTER_BOUND('',#7355,.T.);
#4428=FACE_OUTER_BOUND('',#7356,.T.);
#4429=FACE_OUTER_BOUND('',#7357,.T.);
#4430=FACE_OUTER_BOUND('',#7358,.T.);
#4431=FACE_OUTER_BOUND('',#7359,.T.);
#4432=FACE_OUTER_BOUND('',#7360,.T.);
#4433=FACE_OUTER_BOUND('',#7361,.T.);
#4434=FACE_OUTER_BOUND('',#7362,.T.);
#4435=FACE_OUTER_BOUND('',#7363,.T.);
#4436=FACE_OUTER_BOUND('',#7364,.T.);
#4437=FACE_OUTER_BOUND('',#7365,.T.);
#4438=FACE_OUTER_BOUND('',#7366,.T.);
#4439=FACE_OUTER_BOUND('',#7367,.T.);
#4440=FACE_OUTER_BOUND('',#7368,.T.);
#4441=FACE_OUTER_BOUND('',#7369,.T.);
#4442=FACE_OUTER_BOUND('',#7370,.T.);
#4443=FACE_OUTER_BOUND('',#7371,.T.);
#4444=FACE_OUTER_BOUND('',#7372,.T.);
#4445=FACE_OUTER_BOUND('',#7373,.T.);
#4446=FACE_OUTER_BOUND('',#7374,.T.);
#4447=FACE_OUTER_BOUND('',#7375,.T.);
#4448=FACE_OUTER_BOUND('',#7376,.T.);
#4449=FACE_OUTER_BOUND('',#7377,.T.);
#4450=FACE_OUTER_BOUND('',#7378,.T.);
#4451=FACE_OUTER_BOUND('',#7379,.T.);
#4452=FACE_OUTER_BOUND('',#7380,.T.);
#4453=FACE_OUTER_BOUND('',#7381,.T.);
#4454=FACE_OUTER_BOUND('',#7382,.T.);
#4455=FACE_OUTER_BOUND('',#7383,.T.);
#4456=FACE_OUTER_BOUND('',#7384,.T.);
#4457=FACE_OUTER_BOUND('',#7385,.T.);
#4458=FACE_OUTER_BOUND('',#7386,.T.);
#4459=FACE_OUTER_BOUND('',#7387,.T.);
#4460=FACE_OUTER_BOUND('',#7388,.T.);
#4461=FACE_OUTER_BOUND('',#7389,.T.);
#4462=FACE_OUTER_BOUND('',#7390,.T.);
#4463=FACE_OUTER_BOUND('',#7391,.T.);
#4464=FACE_OUTER_BOUND('',#7392,.T.);
#4465=FACE_OUTER_BOUND('',#7393,.T.);
#4466=FACE_OUTER_BOUND('',#7394,.T.);
#4467=FACE_OUTER_BOUND('',#7395,.T.);
#4468=FACE_OUTER_BOUND('',#7396,.T.);
#4469=FACE_OUTER_BOUND('',#7397,.T.);
#4470=FACE_OUTER_BOUND('',#7398,.T.);
#4471=FACE_OUTER_BOUND('',#7399,.T.);
#4472=FACE_OUTER_BOUND('',#7400,.T.);
#4473=FACE_OUTER_BOUND('',#7401,.T.);
#4474=FACE_OUTER_BOUND('',#7402,.T.);
#4475=FACE_OUTER_BOUND('',#7403,.T.);
#4476=FACE_OUTER_BOUND('',#7404,.T.);
#4477=FACE_OUTER_BOUND('',#7405,.T.);
#4478=FACE_OUTER_BOUND('',#7406,.T.);
#4479=FACE_OUTER_BOUND('',#7407,.T.);
#4480=FACE_OUTER_BOUND('',#7408,.T.);
#4481=FACE_OUTER_BOUND('',#7409,.T.);
#4482=FACE_OUTER_BOUND('',#7410,.T.);
#4483=FACE_OUTER_BOUND('',#7411,.T.);
#4484=FACE_OUTER_BOUND('',#7412,.T.);
#4485=FACE_OUTER_BOUND('',#7413,.T.);
#4486=FACE_OUTER_BOUND('',#7414,.T.);
#4487=FACE_OUTER_BOUND('',#7415,.T.);
#4488=FACE_OUTER_BOUND('',#7416,.T.);
#4489=FACE_OUTER_BOUND('',#7417,.T.);
#4490=FACE_OUTER_BOUND('',#7418,.T.);
#4491=FACE_OUTER_BOUND('',#7419,.T.);
#4492=FACE_OUTER_BOUND('',#7420,.T.);
#4493=FACE_OUTER_BOUND('',#7421,.T.);
#4494=FACE_OUTER_BOUND('',#7422,.T.);
#4495=FACE_OUTER_BOUND('',#7423,.T.);
#4496=FACE_OUTER_BOUND('',#7424,.T.);
#4497=FACE_OUTER_BOUND('',#7425,.T.);
#4498=FACE_OUTER_BOUND('',#7426,.T.);
#4499=FACE_OUTER_BOUND('',#7427,.T.);
#4500=FACE_OUTER_BOUND('',#7428,.T.);
#4501=FACE_OUTER_BOUND('',#7429,.T.);
#4502=FACE_OUTER_BOUND('',#7430,.T.);
#4503=FACE_OUTER_BOUND('',#7431,.T.);
#4504=FACE_OUTER_BOUND('',#7432,.T.);
#4505=FACE_OUTER_BOUND('',#7433,.T.);
#4506=FACE_OUTER_BOUND('',#7434,.T.);
#4507=FACE_OUTER_BOUND('',#7435,.T.);
#4508=FACE_OUTER_BOUND('',#7436,.T.);
#4509=FACE_OUTER_BOUND('',#7437,.T.);
#4510=FACE_OUTER_BOUND('',#7438,.T.);
#4511=FACE_OUTER_BOUND('',#7439,.T.);
#4512=FACE_OUTER_BOUND('',#7440,.T.);
#4513=FACE_OUTER_BOUND('',#7441,.T.);
#4514=FACE_OUTER_BOUND('',#7442,.T.);
#4515=FACE_OUTER_BOUND('',#7443,.T.);
#4516=FACE_OUTER_BOUND('',#7444,.T.);
#4517=FACE_OUTER_BOUND('',#7445,.T.);
#4518=FACE_OUTER_BOUND('',#7446,.T.);
#4519=FACE_OUTER_BOUND('',#7447,.T.);
#4520=FACE_OUTER_BOUND('',#7448,.T.);
#4521=FACE_OUTER_BOUND('',#7449,.T.);
#4522=FACE_OUTER_BOUND('',#7450,.T.);
#4523=FACE_OUTER_BOUND('',#7451,.T.);
#4524=FACE_OUTER_BOUND('',#7452,.T.);
#4525=FACE_OUTER_BOUND('',#7453,.T.);
#4526=FACE_OUTER_BOUND('',#7454,.T.);
#4527=FACE_OUTER_BOUND('',#7455,.T.);
#4528=FACE_OUTER_BOUND('',#7456,.T.);
#4529=FACE_OUTER_BOUND('',#7457,.T.);
#4530=FACE_OUTER_BOUND('',#7458,.T.);
#4531=FACE_OUTER_BOUND('',#7459,.T.);
#4532=FACE_OUTER_BOUND('',#7460,.T.);
#4533=FACE_OUTER_BOUND('',#7461,.T.);
#4534=FACE_OUTER_BOUND('',#7462,.T.);
#4535=FACE_OUTER_BOUND('',#7463,.T.);
#4536=FACE_OUTER_BOUND('',#7464,.T.);
#4537=FACE_OUTER_BOUND('',#7465,.T.);
#4538=FACE_OUTER_BOUND('',#7466,.T.);
#4539=FACE_OUTER_BOUND('',#7467,.T.);
#4540=FACE_OUTER_BOUND('',#7468,.T.);
#4541=FACE_OUTER_BOUND('',#7469,.T.);
#4542=FACE_OUTER_BOUND('',#7470,.T.);
#4543=FACE_OUTER_BOUND('',#7471,.T.);
#4544=FACE_OUTER_BOUND('',#7472,.T.);
#4545=FACE_OUTER_BOUND('',#7473,.T.);
#4546=FACE_OUTER_BOUND('',#7474,.T.);
#4547=FACE_OUTER_BOUND('',#7475,.T.);
#4548=FACE_OUTER_BOUND('',#7476,.T.);
#4549=FACE_OUTER_BOUND('',#7477,.T.);
#4550=FACE_OUTER_BOUND('',#7478,.T.);
#4551=FACE_OUTER_BOUND('',#7479,.T.);
#4552=FACE_OUTER_BOUND('',#7480,.T.);
#4553=FACE_OUTER_BOUND('',#7481,.T.);
#4554=FACE_OUTER_BOUND('',#7482,.T.);
#4555=FACE_OUTER_BOUND('',#7483,.T.);
#4556=FACE_OUTER_BOUND('',#7484,.T.);
#4557=FACE_OUTER_BOUND('',#7485,.T.);
#4558=FACE_OUTER_BOUND('',#7486,.T.);
#4559=FACE_OUTER_BOUND('',#7487,.T.);
#4560=FACE_OUTER_BOUND('',#7488,.T.);
#4561=FACE_OUTER_BOUND('',#7489,.T.);
#4562=FACE_OUTER_BOUND('',#7490,.T.);
#4563=FACE_OUTER_BOUND('',#7491,.T.);
#4564=FACE_OUTER_BOUND('',#7492,.T.);
#4565=FACE_OUTER_BOUND('',#7493,.T.);
#4566=FACE_OUTER_BOUND('',#7494,.T.);
#4567=FACE_OUTER_BOUND('',#7495,.T.);
#4568=FACE_OUTER_BOUND('',#7496,.T.);
#4569=FACE_OUTER_BOUND('',#7497,.T.);
#4570=FACE_OUTER_BOUND('',#7498,.T.);
#4571=FACE_OUTER_BOUND('',#7499,.T.);
#4572=FACE_OUTER_BOUND('',#7500,.T.);
#4573=FACE_OUTER_BOUND('',#7501,.T.);
#4574=FACE_OUTER_BOUND('',#7502,.T.);
#4575=FACE_OUTER_BOUND('',#7503,.T.);
#4576=FACE_OUTER_BOUND('',#7504,.T.);
#4577=FACE_OUTER_BOUND('',#7505,.T.);
#4578=FACE_OUTER_BOUND('',#7506,.T.);
#4579=FACE_OUTER_BOUND('',#7507,.T.);
#4580=FACE_OUTER_BOUND('',#7508,.T.);
#4581=FACE_OUTER_BOUND('',#7509,.T.);
#4582=FACE_OUTER_BOUND('',#7510,.T.);
#4583=FACE_OUTER_BOUND('',#7511,.T.);
#4584=FACE_OUTER_BOUND('',#7512,.T.);
#4585=FACE_OUTER_BOUND('',#7513,.T.);
#4586=FACE_OUTER_BOUND('',#7514,.T.);
#4587=FACE_OUTER_BOUND('',#7515,.T.);
#4588=FACE_OUTER_BOUND('',#7516,.T.);
#4589=FACE_OUTER_BOUND('',#7517,.T.);
#4590=FACE_OUTER_BOUND('',#7518,.T.);
#4591=FACE_OUTER_BOUND('',#7519,.T.);
#4592=FACE_OUTER_BOUND('',#7520,.T.);
#4593=FACE_OUTER_BOUND('',#7521,.T.);
#4594=FACE_OUTER_BOUND('',#7522,.T.);
#4595=FACE_OUTER_BOUND('',#7523,.T.);
#4596=FACE_OUTER_BOUND('',#7524,.T.);
#4597=FACE_OUTER_BOUND('',#7525,.T.);
#4598=FACE_OUTER_BOUND('',#7526,.T.);
#4599=FACE_OUTER_BOUND('',#7527,.T.);
#4600=FACE_OUTER_BOUND('',#7528,.T.);
#4601=FACE_OUTER_BOUND('',#7529,.T.);
#4602=FACE_OUTER_BOUND('',#7530,.T.);
#4603=FACE_OUTER_BOUND('',#7531,.T.);
#4604=FACE_OUTER_BOUND('',#7532,.T.);
#4605=FACE_OUTER_BOUND('',#7533,.T.);
#4606=FACE_OUTER_BOUND('',#7534,.T.);
#4607=FACE_OUTER_BOUND('',#7535,.T.);
#4608=FACE_OUTER_BOUND('',#7536,.T.);
#4609=FACE_OUTER_BOUND('',#7537,.T.);
#4610=FACE_OUTER_BOUND('',#7538,.T.);
#4611=FACE_OUTER_BOUND('',#7539,.T.);
#4612=FACE_OUTER_BOUND('',#7540,.T.);
#4613=FACE_OUTER_BOUND('',#7541,.T.);
#4614=FACE_OUTER_BOUND('',#7542,.T.);
#4615=FACE_OUTER_BOUND('',#7543,.T.);
#4616=FACE_OUTER_BOUND('',#7544,.T.);
#4617=FACE_OUTER_BOUND('',#7545,.T.);
#4618=FACE_OUTER_BOUND('',#7546,.T.);
#4619=FACE_OUTER_BOUND('',#7547,.T.);
#4620=FACE_OUTER_BOUND('',#7548,.T.);
#4621=FACE_OUTER_BOUND('',#7549,.T.);
#4622=FACE_OUTER_BOUND('',#7550,.T.);
#4623=FACE_OUTER_BOUND('',#7551,.T.);
#4624=FACE_OUTER_BOUND('',#7552,.T.);
#4625=FACE_OUTER_BOUND('',#7553,.T.);
#4626=FACE_OUTER_BOUND('',#7554,.T.);
#4627=FACE_OUTER_BOUND('',#7555,.T.);
#4628=FACE_OUTER_BOUND('',#7556,.T.);
#4629=FACE_OUTER_BOUND('',#7557,.T.);
#4630=FACE_OUTER_BOUND('',#7558,.T.);
#4631=FACE_OUTER_BOUND('',#7559,.T.);
#4632=FACE_OUTER_BOUND('',#7560,.T.);
#4633=FACE_OUTER_BOUND('',#7561,.T.);
#4634=FACE_OUTER_BOUND('',#7562,.T.);
#4635=FACE_OUTER_BOUND('',#7563,.T.);
#4636=FACE_OUTER_BOUND('',#7564,.T.);
#4637=FACE_OUTER_BOUND('',#7565,.T.);
#4638=FACE_OUTER_BOUND('',#7566,.T.);
#4639=FACE_OUTER_BOUND('',#7567,.T.);
#4640=FACE_OUTER_BOUND('',#7568,.T.);
#4641=FACE_OUTER_BOUND('',#7569,.T.);
#4642=FACE_OUTER_BOUND('',#7570,.T.);
#4643=FACE_OUTER_BOUND('',#7571,.T.);
#4644=FACE_OUTER_BOUND('',#7572,.T.);
#4645=FACE_OUTER_BOUND('',#7573,.T.);
#4646=FACE_OUTER_BOUND('',#7574,.T.);
#4647=FACE_OUTER_BOUND('',#7575,.T.);
#4648=FACE_OUTER_BOUND('',#7576,.T.);
#4649=FACE_OUTER_BOUND('',#7577,.T.);
#4650=FACE_OUTER_BOUND('',#7578,.T.);
#4651=FACE_OUTER_BOUND('',#7579,.T.);
#4652=FACE_OUTER_BOUND('',#7580,.T.);
#4653=FACE_OUTER_BOUND('',#7581,.T.);
#4654=FACE_OUTER_BOUND('',#7582,.T.);
#4655=FACE_OUTER_BOUND('',#7583,.T.);
#4656=FACE_OUTER_BOUND('',#7584,.T.);
#4657=FACE_OUTER_BOUND('',#7585,.T.);
#4658=FACE_OUTER_BOUND('',#7586,.T.);
#4659=FACE_OUTER_BOUND('',#7587,.T.);
#4660=FACE_OUTER_BOUND('',#7588,.T.);
#4661=FACE_OUTER_BOUND('',#7589,.T.);
#4662=FACE_OUTER_BOUND('',#7590,.T.);
#4663=FACE_OUTER_BOUND('',#7591,.T.);
#4664=FACE_OUTER_BOUND('',#7592,.T.);
#4665=FACE_OUTER_BOUND('',#7593,.T.);
#4666=FACE_OUTER_BOUND('',#7594,.T.);
#4667=FACE_OUTER_BOUND('',#7595,.T.);
#4668=FACE_OUTER_BOUND('',#7596,.T.);
#4669=FACE_OUTER_BOUND('',#7597,.T.);
#4670=FACE_OUTER_BOUND('',#7598,.T.);
#4671=FACE_OUTER_BOUND('',#7599,.T.);
#4672=FACE_OUTER_BOUND('',#7600,.T.);
#4673=FACE_OUTER_BOUND('',#7601,.T.);
#4674=FACE_OUTER_BOUND('',#7602,.T.);
#4675=FACE_OUTER_BOUND('',#7603,.T.);
#4676=FACE_OUTER_BOUND('',#7604,.T.);
#4677=FACE_OUTER_BOUND('',#7605,.T.);
#4678=FACE_OUTER_BOUND('',#7606,.T.);
#4679=FACE_OUTER_BOUND('',#7607,.T.);
#4680=FACE_OUTER_BOUND('',#7608,.T.);
#4681=FACE_OUTER_BOUND('',#7609,.T.);
#4682=FACE_OUTER_BOUND('',#7610,.T.);
#4683=FACE_OUTER_BOUND('',#7611,.T.);
#4684=FACE_OUTER_BOUND('',#7612,.T.);
#4685=FACE_OUTER_BOUND('',#7613,.T.);
#4686=FACE_OUTER_BOUND('',#7614,.T.);
#4687=FACE_OUTER_BOUND('',#7615,.T.);
#4688=FACE_OUTER_BOUND('',#7616,.T.);
#4689=FACE_OUTER_BOUND('',#7617,.T.);
#4690=FACE_OUTER_BOUND('',#7618,.T.);
#4691=FACE_OUTER_BOUND('',#7619,.T.);
#4692=FACE_OUTER_BOUND('',#7620,.T.);
#4693=FACE_OUTER_BOUND('',#7621,.T.);
#4694=FACE_OUTER_BOUND('',#7622,.T.);
#4695=FACE_OUTER_BOUND('',#7623,.T.);
#4696=FACE_OUTER_BOUND('',#7624,.T.);
#4697=FACE_OUTER_BOUND('',#7625,.T.);
#4698=FACE_OUTER_BOUND('',#7626,.T.);
#4699=FACE_OUTER_BOUND('',#7627,.T.);
#4700=FACE_OUTER_BOUND('',#7628,.T.);
#4701=FACE_OUTER_BOUND('',#7629,.T.);
#4702=FACE_OUTER_BOUND('',#7630,.T.);
#4703=FACE_OUTER_BOUND('',#7631,.T.);
#4704=FACE_OUTER_BOUND('',#7632,.T.);
#4705=FACE_OUTER_BOUND('',#7633,.T.);
#4706=FACE_OUTER_BOUND('',#7634,.T.);
#4707=FACE_OUTER_BOUND('',#7635,.T.);
#4708=FACE_OUTER_BOUND('',#7636,.T.);
#4709=FACE_OUTER_BOUND('',#7637,.T.);
#4710=FACE_OUTER_BOUND('',#7638,.T.);
#4711=FACE_OUTER_BOUND('',#7639,.T.);
#4712=FACE_OUTER_BOUND('',#7640,.T.);
#4713=FACE_OUTER_BOUND('',#7641,.T.);
#4714=FACE_OUTER_BOUND('',#7642,.T.);
#4715=FACE_OUTER_BOUND('',#7643,.T.);
#4716=FACE_OUTER_BOUND('',#7644,.T.);
#4717=FACE_OUTER_BOUND('',#7645,.T.);
#4718=FACE_OUTER_BOUND('',#7646,.T.);
#4719=FACE_OUTER_BOUND('',#7647,.T.);
#4720=FACE_OUTER_BOUND('',#7648,.T.);
#4721=FACE_OUTER_BOUND('',#7649,.T.);
#4722=FACE_OUTER_BOUND('',#7650,.T.);
#4723=FACE_OUTER_BOUND('',#7651,.T.);
#4724=FACE_OUTER_BOUND('',#7652,.T.);
#4725=FACE_OUTER_BOUND('',#7653,.T.);
#4726=FACE_OUTER_BOUND('',#7654,.T.);
#4727=FACE_OUTER_BOUND('',#7655,.T.);
#4728=FACE_OUTER_BOUND('',#7656,.T.);
#4729=FACE_OUTER_BOUND('',#7657,.T.);
#4730=FACE_OUTER_BOUND('',#7658,.T.);
#4731=FACE_OUTER_BOUND('',#7659,.T.);
#4732=FACE_OUTER_BOUND('',#7660,.T.);
#4733=FACE_OUTER_BOUND('',#7661,.T.);
#4734=FACE_OUTER_BOUND('',#7662,.T.);
#4735=FACE_OUTER_BOUND('',#7663,.T.);
#4736=FACE_OUTER_BOUND('',#7664,.T.);
#4737=FACE_OUTER_BOUND('',#7665,.T.);
#4738=FACE_OUTER_BOUND('',#7666,.T.);
#4739=FACE_OUTER_BOUND('',#7667,.T.);
#4740=FACE_OUTER_BOUND('',#7668,.T.);
#4741=FACE_OUTER_BOUND('',#7669,.T.);
#4742=FACE_OUTER_BOUND('',#7670,.T.);
#4743=FACE_OUTER_BOUND('',#7671,.T.);
#4744=FACE_OUTER_BOUND('',#7672,.T.);
#4745=FACE_OUTER_BOUND('',#7673,.T.);
#4746=FACE_OUTER_BOUND('',#7674,.T.);
#4747=FACE_OUTER_BOUND('',#7675,.T.);
#4748=FACE_OUTER_BOUND('',#7676,.T.);
#4749=FACE_OUTER_BOUND('',#7677,.T.);
#4750=FACE_OUTER_BOUND('',#7678,.T.);
#4751=FACE_OUTER_BOUND('',#7679,.T.);
#4752=FACE_OUTER_BOUND('',#7680,.T.);
#4753=FACE_OUTER_BOUND('',#7681,.T.);
#4754=FACE_OUTER_BOUND('',#7682,.T.);
#4755=FACE_OUTER_BOUND('',#7683,.T.);
#4756=FACE_OUTER_BOUND('',#7684,.T.);
#4757=FACE_OUTER_BOUND('',#7685,.T.);
#4758=FACE_OUTER_BOUND('',#7686,.T.);
#4759=FACE_OUTER_BOUND('',#7687,.T.);
#4760=FACE_OUTER_BOUND('',#7688,.T.);
#4761=FACE_OUTER_BOUND('',#7689,.T.);
#4762=FACE_OUTER_BOUND('',#7690,.T.);
#4763=FACE_OUTER_BOUND('',#7691,.T.);
#4764=FACE_OUTER_BOUND('',#7692,.T.);
#4765=FACE_OUTER_BOUND('',#7693,.T.);
#4766=FACE_OUTER_BOUND('',#7694,.T.);
#4767=FACE_OUTER_BOUND('',#7695,.T.);
#4768=FACE_OUTER_BOUND('',#7696,.T.);
#4769=FACE_OUTER_BOUND('',#7697,.T.);
#4770=FACE_OUTER_BOUND('',#7698,.T.);
#4771=FACE_OUTER_BOUND('',#7699,.T.);
#4772=FACE_OUTER_BOUND('',#7700,.T.);
#4773=FACE_OUTER_BOUND('',#7701,.T.);
#4774=FACE_OUTER_BOUND('',#7702,.T.);
#4775=FACE_OUTER_BOUND('',#7703,.T.);
#4776=FACE_OUTER_BOUND('',#7704,.T.);
#4777=FACE_OUTER_BOUND('',#7705,.T.);
#4778=FACE_OUTER_BOUND('',#7706,.T.);
#4779=FACE_OUTER_BOUND('',#7707,.T.);
#4780=FACE_OUTER_BOUND('',#7708,.T.);
#4781=FACE_OUTER_BOUND('',#7709,.T.);
#4782=FACE_OUTER_BOUND('',#7710,.T.);
#4783=FACE_OUTER_BOUND('',#7711,.T.);
#4784=FACE_OUTER_BOUND('',#7712,.T.);
#4785=FACE_OUTER_BOUND('',#7713,.T.);
#4786=FACE_OUTER_BOUND('',#7714,.T.);
#4787=FACE_OUTER_BOUND('',#7715,.T.);
#4788=FACE_OUTER_BOUND('',#7716,.T.);
#4789=FACE_OUTER_BOUND('',#7717,.T.);
#4790=FACE_OUTER_BOUND('',#7718,.T.);
#4791=FACE_OUTER_BOUND('',#7719,.T.);
#4792=FACE_OUTER_BOUND('',#7720,.T.);
#4793=FACE_OUTER_BOUND('',#7721,.T.);
#4794=FACE_OUTER_BOUND('',#7722,.T.);
#4795=FACE_OUTER_BOUND('',#7723,.T.);
#4796=FACE_OUTER_BOUND('',#7724,.T.);
#4797=FACE_OUTER_BOUND('',#7725,.T.);
#4798=FACE_OUTER_BOUND('',#7726,.T.);
#4799=FACE_OUTER_BOUND('',#7727,.T.);
#4800=FACE_OUTER_BOUND('',#7728,.T.);
#4801=FACE_OUTER_BOUND('',#7729,.T.);
#4802=FACE_OUTER_BOUND('',#7730,.T.);
#4803=FACE_OUTER_BOUND('',#7731,.T.);
#4804=FACE_OUTER_BOUND('',#7732,.T.);
#4805=FACE_OUTER_BOUND('',#7733,.T.);
#4806=FACE_OUTER_BOUND('',#7734,.T.);
#4807=FACE_OUTER_BOUND('',#7735,.T.);
#4808=FACE_OUTER_BOUND('',#7736,.T.);
#4809=FACE_OUTER_BOUND('',#7737,.T.);
#4810=FACE_OUTER_BOUND('',#7738,.T.);
#4811=FACE_OUTER_BOUND('',#7739,.T.);
#4812=FACE_OUTER_BOUND('',#7740,.T.);
#4813=FACE_OUTER_BOUND('',#7741,.T.);
#4814=FACE_OUTER_BOUND('',#7742,.T.);
#4815=FACE_OUTER_BOUND('',#7743,.T.);
#4816=FACE_OUTER_BOUND('',#7744,.T.);
#4817=FACE_OUTER_BOUND('',#7745,.T.);
#4818=FACE_OUTER_BOUND('',#7746,.T.);
#4819=FACE_OUTER_BOUND('',#7747,.T.);
#4820=FACE_OUTER_BOUND('',#7748,.T.);
#4821=FACE_OUTER_BOUND('',#7749,.T.);
#4822=FACE_OUTER_BOUND('',#7750,.T.);
#4823=FACE_OUTER_BOUND('',#7751,.T.);
#4824=FACE_OUTER_BOUND('',#7752,.T.);
#4825=FACE_OUTER_BOUND('',#7753,.T.);
#4826=FACE_OUTER_BOUND('',#7754,.T.);
#4827=FACE_OUTER_BOUND('',#7755,.T.);
#4828=FACE_OUTER_BOUND('',#7756,.T.);
#4829=FACE_OUTER_BOUND('',#7757,.T.);
#4830=FACE_OUTER_BOUND('',#7758,.T.);
#4831=FACE_OUTER_BOUND('',#7759,.T.);
#4832=FACE_OUTER_BOUND('',#7760,.T.);
#4833=FACE_OUTER_BOUND('',#7761,.T.);
#4834=FACE_OUTER_BOUND('',#7762,.T.);
#4835=FACE_OUTER_BOUND('',#7763,.T.);
#4836=FACE_OUTER_BOUND('',#7764,.T.);
#4837=FACE_OUTER_BOUND('',#7765,.T.);
#4838=FACE_OUTER_BOUND('',#7766,.T.);
#4839=FACE_OUTER_BOUND('',#7767,.T.);
#4840=FACE_OUTER_BOUND('',#7768,.T.);
#4841=FACE_OUTER_BOUND('',#7769,.T.);
#4842=FACE_OUTER_BOUND('',#7770,.T.);
#4843=FACE_OUTER_BOUND('',#7771,.T.);
#4844=FACE_OUTER_BOUND('',#7772,.T.);
#4845=FACE_OUTER_BOUND('',#7773,.T.);
#4846=FACE_OUTER_BOUND('',#7774,.T.);
#4847=FACE_OUTER_BOUND('',#7775,.T.);
#4848=FACE_OUTER_BOUND('',#7776,.T.);
#4849=FACE_OUTER_BOUND('',#7777,.T.);
#4850=FACE_OUTER_BOUND('',#7778,.T.);
#4851=FACE_OUTER_BOUND('',#7779,.T.);
#4852=FACE_OUTER_BOUND('',#7780,.T.);
#4853=FACE_OUTER_BOUND('',#7781,.T.);
#4854=FACE_OUTER_BOUND('',#7782,.T.);
#4855=FACE_OUTER_BOUND('',#7783,.T.);
#4856=FACE_OUTER_BOUND('',#7784,.T.);
#4857=FACE_OUTER_BOUND('',#7785,.T.);
#4858=FACE_OUTER_BOUND('',#7786,.T.);
#4859=FACE_OUTER_BOUND('',#7787,.T.);
#4860=FACE_OUTER_BOUND('',#7788,.T.);
#4861=FACE_OUTER_BOUND('',#7789,.T.);
#4862=FACE_OUTER_BOUND('',#7790,.T.);
#4863=FACE_OUTER_BOUND('',#7791,.T.);
#4864=FACE_OUTER_BOUND('',#7792,.T.);
#4865=FACE_OUTER_BOUND('',#7793,.T.);
#4866=FACE_OUTER_BOUND('',#7794,.T.);
#4867=FACE_OUTER_BOUND('',#7795,.T.);
#4868=FACE_OUTER_BOUND('',#7796,.T.);
#4869=FACE_OUTER_BOUND('',#7797,.T.);
#4870=FACE_OUTER_BOUND('',#7798,.T.);
#4871=FACE_OUTER_BOUND('',#7799,.T.);
#4872=FACE_OUTER_BOUND('',#7800,.T.);
#4873=FACE_OUTER_BOUND('',#7801,.T.);
#4874=FACE_OUTER_BOUND('',#7802,.T.);
#4875=FACE_OUTER_BOUND('',#7803,.T.);
#4876=FACE_OUTER_BOUND('',#7804,.T.);
#4877=FACE_OUTER_BOUND('',#7805,.T.);
#4878=FACE_OUTER_BOUND('',#7806,.T.);
#4879=FACE_OUTER_BOUND('',#7807,.T.);
#4880=FACE_OUTER_BOUND('',#7808,.T.);
#4881=FACE_OUTER_BOUND('',#7809,.T.);
#4882=FACE_OUTER_BOUND('',#7810,.T.);
#4883=FACE_OUTER_BOUND('',#7811,.T.);
#4884=FACE_OUTER_BOUND('',#7812,.T.);
#4885=FACE_OUTER_BOUND('',#7813,.T.);
#4886=FACE_OUTER_BOUND('',#7814,.T.);
#4887=FACE_OUTER_BOUND('',#7815,.T.);
#4888=FACE_OUTER_BOUND('',#7816,.T.);
#4889=FACE_OUTER_BOUND('',#7817,.T.);
#4890=FACE_OUTER_BOUND('',#7818,.T.);
#4891=FACE_OUTER_BOUND('',#7819,.T.);
#4892=FACE_OUTER_BOUND('',#7820,.T.);
#4893=FACE_OUTER_BOUND('',#7821,.T.);
#4894=FACE_OUTER_BOUND('',#7822,.T.);
#4895=FACE_OUTER_BOUND('',#7823,.T.);
#4896=FACE_OUTER_BOUND('',#7824,.T.);
#4897=FACE_OUTER_BOUND('',#7825,.T.);
#4898=FACE_OUTER_BOUND('',#7826,.T.);
#4899=FACE_OUTER_BOUND('',#7827,.T.);
#4900=FACE_OUTER_BOUND('',#7828,.T.);
#4901=FACE_OUTER_BOUND('',#7829,.T.);
#4902=FACE_OUTER_BOUND('',#7830,.T.);
#4903=FACE_OUTER_BOUND('',#7831,.T.);
#4904=FACE_OUTER_BOUND('',#7832,.T.);
#4905=FACE_OUTER_BOUND('',#7833,.T.);
#4906=FACE_OUTER_BOUND('',#7834,.T.);
#4907=FACE_OUTER_BOUND('',#7835,.T.);
#4908=FACE_OUTER_BOUND('',#7836,.T.);
#4909=FACE_OUTER_BOUND('',#7837,.T.);
#4910=FACE_OUTER_BOUND('',#7838,.T.);
#4911=FACE_OUTER_BOUND('',#7839,.T.);
#4912=FACE_OUTER_BOUND('',#7840,.T.);
#4913=FACE_OUTER_BOUND('',#7841,.T.);
#4914=FACE_OUTER_BOUND('',#7842,.T.);
#4915=FACE_OUTER_BOUND('',#7843,.T.);
#4916=FACE_OUTER_BOUND('',#7844,.T.);
#4917=FACE_OUTER_BOUND('',#7845,.T.);
#4918=FACE_OUTER_BOUND('',#7846,.T.);
#4919=FACE_OUTER_BOUND('',#7847,.T.);
#4920=FACE_OUTER_BOUND('',#7848,.T.);
#4921=FACE_OUTER_BOUND('',#7849,.T.);
#4922=FACE_OUTER_BOUND('',#7850,.T.);
#4923=FACE_OUTER_BOUND('',#7851,.T.);
#4924=FACE_OUTER_BOUND('',#7852,.T.);
#4925=FACE_OUTER_BOUND('',#7853,.T.);
#4926=FACE_OUTER_BOUND('',#7854,.T.);
#4927=FACE_OUTER_BOUND('',#7855,.T.);
#4928=FACE_OUTER_BOUND('',#7856,.T.);
#4929=FACE_OUTER_BOUND('',#7857,.T.);
#4930=FACE_OUTER_BOUND('',#7858,.T.);
#4931=FACE_OUTER_BOUND('',#7859,.T.);
#4932=FACE_OUTER_BOUND('',#7860,.T.);
#4933=FACE_OUTER_BOUND('',#7861,.T.);
#4934=FACE_OUTER_BOUND('',#7862,.T.);
#4935=FACE_OUTER_BOUND('',#7863,.T.);
#4936=FACE_OUTER_BOUND('',#7864,.T.);
#4937=FACE_OUTER_BOUND('',#7865,.T.);
#4938=FACE_OUTER_BOUND('',#7866,.T.);
#4939=FACE_OUTER_BOUND('',#7867,.T.);
#4940=FACE_OUTER_BOUND('',#7868,.T.);
#4941=FACE_OUTER_BOUND('',#7869,.T.);
#4942=FACE_OUTER_BOUND('',#7870,.T.);
#4943=FACE_OUTER_BOUND('',#7871,.T.);
#4944=FACE_OUTER_BOUND('',#7872,.T.);
#4945=FACE_OUTER_BOUND('',#7873,.T.);
#4946=FACE_OUTER_BOUND('',#7874,.T.);
#4947=FACE_OUTER_BOUND('',#7875,.T.);
#4948=FACE_OUTER_BOUND('',#7876,.T.);
#4949=FACE_OUTER_BOUND('',#7877,.T.);
#4950=FACE_OUTER_BOUND('',#7878,.T.);
#4951=FACE_OUTER_BOUND('',#7879,.T.);
#4952=FACE_OUTER_BOUND('',#7880,.T.);
#4953=FACE_OUTER_BOUND('',#7881,.T.);
#4954=FACE_OUTER_BOUND('',#7882,.T.);
#4955=FACE_OUTER_BOUND('',#7883,.T.);
#4956=FACE_OUTER_BOUND('',#7884,.T.);
#4957=FACE_OUTER_BOUND('',#7885,.T.);
#4958=FACE_OUTER_BOUND('',#7886,.T.);
#4959=FACE_OUTER_BOUND('',#7887,.T.);
#4960=FACE_OUTER_BOUND('',#7888,.T.);
#4961=FACE_OUTER_BOUND('',#7889,.T.);
#4962=FACE_OUTER_BOUND('',#7890,.T.);
#4963=FACE_OUTER_BOUND('',#7891,.T.);
#4964=FACE_OUTER_BOUND('',#7892,.T.);
#4965=FACE_OUTER_BOUND('',#7893,.T.);
#4966=FACE_OUTER_BOUND('',#7894,.T.);
#4967=FACE_OUTER_BOUND('',#7895,.T.);
#4968=FACE_OUTER_BOUND('',#7896,.T.);
#4969=FACE_OUTER_BOUND('',#7897,.T.);
#4970=FACE_OUTER_BOUND('',#7898,.T.);
#4971=FACE_OUTER_BOUND('',#7899,.T.);
#4972=FACE_OUTER_BOUND('',#7900,.T.);
#4973=FACE_OUTER_BOUND('',#7901,.T.);
#4974=FACE_OUTER_BOUND('',#7902,.T.);
#4975=FACE_OUTER_BOUND('',#7903,.T.);
#4976=FACE_OUTER_BOUND('',#7904,.T.);
#4977=FACE_OUTER_BOUND('',#7905,.T.);
#4978=FACE_OUTER_BOUND('',#7906,.T.);
#4979=FACE_OUTER_BOUND('',#7907,.T.);
#4980=FACE_OUTER_BOUND('',#7908,.T.);
#4981=FACE_OUTER_BOUND('',#7909,.T.);
#4982=FACE_OUTER_BOUND('',#7910,.T.);
#4983=FACE_OUTER_BOUND('',#7911,.T.);
#4984=FACE_OUTER_BOUND('',#7912,.T.);
#4985=FACE_OUTER_BOUND('',#7913,.T.);
#4986=FACE_OUTER_BOUND('',#7914,.T.);
#4987=FACE_OUTER_BOUND('',#7915,.T.);
#4988=FACE_OUTER_BOUND('',#7916,.T.);
#4989=FACE_OUTER_BOUND('',#7917,.T.);
#4990=FACE_OUTER_BOUND('',#7918,.T.);
#4991=FACE_OUTER_BOUND('',#7919,.T.);
#4992=FACE_OUTER_BOUND('',#7920,.T.);
#4993=FACE_OUTER_BOUND('',#7921,.T.);
#4994=FACE_OUTER_BOUND('',#7922,.T.);
#4995=FACE_OUTER_BOUND('',#7923,.T.);
#4996=FACE_OUTER_BOUND('',#7924,.T.);
#4997=FACE_OUTER_BOUND('',#7925,.T.);
#4998=FACE_OUTER_BOUND('',#7926,.T.);
#4999=FACE_OUTER_BOUND('',#7927,.T.);
#5000=FACE_OUTER_BOUND('',#7928,.T.);
#5001=FACE_OUTER_BOUND('',#7929,.T.);
#5002=FACE_OUTER_BOUND('',#7930,.T.);
#5003=FACE_OUTER_BOUND('',#7931,.T.);
#5004=FACE_OUTER_BOUND('',#7932,.T.);
#5005=FACE_OUTER_BOUND('',#7933,.T.);
#5006=FACE_OUTER_BOUND('',#7934,.T.);
#5007=FACE_OUTER_BOUND('',#7935,.T.);
#5008=FACE_OUTER_BOUND('',#7936,.T.);
#5009=FACE_OUTER_BOUND('',#7937,.T.);
#5010=FACE_OUTER_BOUND('',#7938,.T.);
#5011=FACE_OUTER_BOUND('',#7939,.T.);
#5012=FACE_OUTER_BOUND('',#7940,.T.);
#5013=FACE_OUTER_BOUND('',#7941,.T.);
#5014=FACE_OUTER_BOUND('',#7942,.T.);
#5015=FACE_OUTER_BOUND('',#7943,.T.);
#5016=FACE_OUTER_BOUND('',#7944,.T.);
#5017=FACE_OUTER_BOUND('',#7945,.T.);
#5018=FACE_OUTER_BOUND('',#7946,.T.);
#5019=FACE_OUTER_BOUND('',#7947,.T.);
#5020=FACE_OUTER_BOUND('',#7948,.T.);
#5021=FACE_OUTER_BOUND('',#7949,.T.);
#5022=FACE_OUTER_BOUND('',#7950,.T.);
#5023=FACE_OUTER_BOUND('',#7951,.T.);
#5024=FACE_OUTER_BOUND('',#7952,.T.);
#5025=FACE_OUTER_BOUND('',#7953,.T.);
#5026=FACE_OUTER_BOUND('',#7954,.T.);
#5027=FACE_OUTER_BOUND('',#7955,.T.);
#5028=FACE_OUTER_BOUND('',#7956,.T.);
#5029=FACE_OUTER_BOUND('',#7957,.T.);
#5030=FACE_OUTER_BOUND('',#7958,.T.);
#5031=FACE_OUTER_BOUND('',#7959,.T.);
#5032=FACE_OUTER_BOUND('',#7960,.T.);
#5033=FACE_OUTER_BOUND('',#7961,.T.);
#5034=FACE_OUTER_BOUND('',#7962,.T.);
#5035=FACE_OUTER_BOUND('',#7963,.T.);
#5036=FACE_OUTER_BOUND('',#7964,.T.);
#5037=FACE_OUTER_BOUND('',#7965,.T.);
#5038=FACE_OUTER_BOUND('',#7966,.T.);
#5039=FACE_OUTER_BOUND('',#7967,.T.);
#5040=FACE_OUTER_BOUND('',#7968,.T.);
#5041=FACE_OUTER_BOUND('',#7969,.T.);
#5042=FACE_OUTER_BOUND('',#7970,.T.);
#5043=FACE_OUTER_BOUND('',#7971,.T.);
#5044=FACE_OUTER_BOUND('',#7972,.T.);
#5045=FACE_OUTER_BOUND('',#7973,.T.);
#5046=FACE_OUTER_BOUND('',#7974,.T.);
#5047=FACE_OUTER_BOUND('',#7975,.T.);
#5048=FACE_OUTER_BOUND('',#7976,.T.);
#5049=FACE_OUTER_BOUND('',#7977,.T.);
#5050=FACE_OUTER_BOUND('',#7978,.T.);
#5051=FACE_OUTER_BOUND('',#7979,.T.);
#5052=FACE_OUTER_BOUND('',#7980,.T.);
#5053=FACE_OUTER_BOUND('',#7981,.T.);
#5054=FACE_OUTER_BOUND('',#7982,.T.);
#5055=FACE_OUTER_BOUND('',#7983,.T.);
#5056=FACE_OUTER_BOUND('',#7984,.T.);
#5057=FACE_OUTER_BOUND('',#7985,.T.);
#5058=FACE_OUTER_BOUND('',#7986,.T.);
#5059=FACE_OUTER_BOUND('',#7987,.T.);
#5060=FACE_OUTER_BOUND('',#7988,.T.);
#5061=FACE_OUTER_BOUND('',#7989,.T.);
#5062=FACE_OUTER_BOUND('',#7990,.T.);
#5063=FACE_OUTER_BOUND('',#7991,.T.);
#5064=FACE_OUTER_BOUND('',#7992,.T.);
#5065=FACE_OUTER_BOUND('',#7993,.T.);
#5066=FACE_OUTER_BOUND('',#7994,.T.);
#5067=FACE_OUTER_BOUND('',#7995,.T.);
#5068=FACE_OUTER_BOUND('',#7996,.T.);
#5069=FACE_OUTER_BOUND('',#7997,.T.);
#5070=FACE_OUTER_BOUND('',#7998,.T.);
#5071=FACE_OUTER_BOUND('',#7999,.T.);
#5072=FACE_OUTER_BOUND('',#8000,.T.);
#5073=FACE_OUTER_BOUND('',#8001,.T.);
#5074=FACE_OUTER_BOUND('',#8002,.T.);
#5075=FACE_OUTER_BOUND('',#8003,.T.);
#5076=FACE_OUTER_BOUND('',#8004,.T.);
#5077=FACE_OUTER_BOUND('',#8005,.T.);
#5078=FACE_OUTER_BOUND('',#8006,.T.);
#5079=FACE_OUTER_BOUND('',#8007,.T.);
#5080=FACE_OUTER_BOUND('',#8008,.T.);
#5081=FACE_OUTER_BOUND('',#8009,.T.);
#5082=FACE_OUTER_BOUND('',#8010,.T.);
#5083=FACE_OUTER_BOUND('',#8011,.T.);
#5084=FACE_OUTER_BOUND('',#8012,.T.);
#5085=FACE_OUTER_BOUND('',#8013,.T.);
#5086=FACE_OUTER_BOUND('',#8014,.T.);
#5087=FACE_OUTER_BOUND('',#8015,.T.);
#5088=FACE_OUTER_BOUND('',#8016,.T.);
#5089=FACE_OUTER_BOUND('',#8017,.T.);
#5090=FACE_OUTER_BOUND('',#8018,.T.);
#5091=FACE_OUTER_BOUND('',#8019,.T.);
#5092=FACE_OUTER_BOUND('',#8020,.T.);
#5093=FACE_OUTER_BOUND('',#8021,.T.);
#5094=FACE_OUTER_BOUND('',#8022,.T.);
#5095=FACE_OUTER_BOUND('',#8023,.T.);
#5096=FACE_OUTER_BOUND('',#8024,.T.);
#5097=FACE_OUTER_BOUND('',#8025,.T.);
#5098=FACE_OUTER_BOUND('',#8026,.T.);
#5099=FACE_OUTER_BOUND('',#8027,.T.);
#5100=FACE_OUTER_BOUND('',#8028,.T.);
#5101=FACE_OUTER_BOUND('',#8029,.T.);
#5102=FACE_OUTER_BOUND('',#8030,.T.);
#5103=FACE_OUTER_BOUND('',#8031,.T.);
#5104=FACE_OUTER_BOUND('',#8032,.T.);
#5105=FACE_OUTER_BOUND('',#8033,.T.);
#5106=FACE_OUTER_BOUND('',#8034,.T.);
#5107=FACE_OUTER_BOUND('',#8035,.T.);
#5108=FACE_OUTER_BOUND('',#8036,.T.);
#5109=FACE_OUTER_BOUND('',#8037,.T.);
#5110=FACE_OUTER_BOUND('',#8038,.T.);
#5111=FACE_OUTER_BOUND('',#8039,.T.);
#5112=FACE_OUTER_BOUND('',#8040,.T.);
#5113=FACE_OUTER_BOUND('',#8041,.T.);
#5114=FACE_OUTER_BOUND('',#8042,.T.);
#5115=FACE_OUTER_BOUND('',#8043,.T.);
#5116=FACE_OUTER_BOUND('',#8044,.T.);
#5117=FACE_OUTER_BOUND('',#8045,.T.);
#5118=FACE_OUTER_BOUND('',#8046,.T.);
#5119=FACE_OUTER_BOUND('',#8047,.T.);
#5120=FACE_OUTER_BOUND('',#8048,.T.);
#5121=FACE_OUTER_BOUND('',#8049,.T.);
#5122=FACE_OUTER_BOUND('',#8050,.T.);
#5123=FACE_OUTER_BOUND('',#8051,.T.);
#5124=FACE_OUTER_BOUND('',#8052,.T.);
#5125=FACE_OUTER_BOUND('',#8053,.T.);
#5126=FACE_OUTER_BOUND('',#8054,.T.);
#5127=FACE_OUTER_BOUND('',#8055,.T.);
#5128=FACE_OUTER_BOUND('',#8056,.T.);
#5129=FACE_OUTER_BOUND('',#8057,.T.);
#5130=FACE_OUTER_BOUND('',#8058,.T.);
#5131=FACE_OUTER_BOUND('',#8059,.T.);
#5132=FACE_OUTER_BOUND('',#8060,.T.);
#5133=FACE_OUTER_BOUND('',#8061,.T.);
#5134=FACE_OUTER_BOUND('',#8062,.T.);
#5135=FACE_OUTER_BOUND('',#8063,.T.);
#5136=FACE_OUTER_BOUND('',#8064,.T.);
#5137=FACE_OUTER_BOUND('',#8065,.T.);
#5138=FACE_OUTER_BOUND('',#8066,.T.);
#5139=FACE_OUTER_BOUND('',#8067,.T.);
#5140=FACE_OUTER_BOUND('',#8068,.T.);
#5141=FACE_OUTER_BOUND('',#8069,.T.);
#5142=FACE_OUTER_BOUND('',#8070,.T.);
#5143=FACE_OUTER_BOUND('',#8071,.T.);
#5144=FACE_OUTER_BOUND('',#8072,.T.);
#5145=FACE_OUTER_BOUND('',#8073,.T.);
#5146=FACE_OUTER_BOUND('',#8074,.T.);
#5147=FACE_OUTER_BOUND('',#8075,.T.);
#5148=FACE_OUTER_BOUND('',#8076,.T.);
#5149=FACE_OUTER_BOUND('',#8077,.T.);
#5150=FACE_OUTER_BOUND('',#8078,.T.);
#5151=FACE_OUTER_BOUND('',#8079,.T.);
#5152=FACE_OUTER_BOUND('',#8080,.T.);
#5153=FACE_OUTER_BOUND('',#8081,.T.);
#5154=FACE_OUTER_BOUND('',#8082,.T.);
#5155=FACE_OUTER_BOUND('',#8083,.T.);
#5156=FACE_OUTER_BOUND('',#8084,.T.);
#5157=FACE_OUTER_BOUND('',#8085,.T.);
#5158=FACE_OUTER_BOUND('',#8086,.T.);
#5159=FACE_OUTER_BOUND('',#8087,.T.);
#5160=FACE_OUTER_BOUND('',#8088,.T.);
#5161=FACE_OUTER_BOUND('',#8089,.T.);
#5162=FACE_OUTER_BOUND('',#8090,.T.);
#5163=FACE_OUTER_BOUND('',#8091,.T.);
#5164=FACE_OUTER_BOUND('',#8092,.T.);
#5165=FACE_OUTER_BOUND('',#8093,.T.);
#5166=FACE_OUTER_BOUND('',#8094,.T.);
#5167=FACE_OUTER_BOUND('',#8095,.T.);
#5168=FACE_OUTER_BOUND('',#8096,.T.);
#5169=FACE_OUTER_BOUND('',#8097,.T.);
#5170=FACE_OUTER_BOUND('',#8098,.T.);
#5171=FACE_OUTER_BOUND('',#8099,.T.);
#5172=FACE_OUTER_BOUND('',#8100,.T.);
#5173=FACE_OUTER_BOUND('',#8101,.T.);
#5174=FACE_OUTER_BOUND('',#8102,.T.);
#5175=FACE_OUTER_BOUND('',#8103,.T.);
#5176=FACE_OUTER_BOUND('',#8104,.T.);
#5177=FACE_OUTER_BOUND('',#8105,.T.);
#5178=FACE_OUTER_BOUND('',#8106,.T.);
#5179=FACE_OUTER_BOUND('',#8107,.T.);
#5180=FACE_OUTER_BOUND('',#8108,.T.);
#5181=FACE_OUTER_BOUND('',#8109,.T.);
#5182=FACE_OUTER_BOUND('',#8110,.T.);
#5183=FACE_OUTER_BOUND('',#8111,.T.);
#5184=FACE_OUTER_BOUND('',#8112,.T.);
#5185=FACE_OUTER_BOUND('',#8113,.T.);
#5186=FACE_OUTER_BOUND('',#8114,.T.);
#5187=FACE_OUTER_BOUND('',#8115,.T.);
#5188=FACE_OUTER_BOUND('',#8116,.T.);
#5189=FACE_OUTER_BOUND('',#8117,.T.);
#5190=FACE_OUTER_BOUND('',#8118,.T.);
#5191=FACE_OUTER_BOUND('',#8119,.T.);
#5192=FACE_OUTER_BOUND('',#8120,.T.);
#5193=FACE_OUTER_BOUND('',#8121,.T.);
#5194=FACE_OUTER_BOUND('',#8122,.T.);
#5195=FACE_OUTER_BOUND('',#8123,.T.);
#5196=FACE_OUTER_BOUND('',#8124,.T.);
#5197=FACE_OUTER_BOUND('',#8125,.T.);
#5198=FACE_OUTER_BOUND('',#8126,.T.);
#5199=FACE_OUTER_BOUND('',#8127,.T.);
#5200=FACE_OUTER_BOUND('',#8128,.T.);
#5201=FACE_OUTER_BOUND('',#8129,.T.);
#5202=FACE_OUTER_BOUND('',#8130,.T.);
#5203=FACE_OUTER_BOUND('',#8131,.T.);
#5204=FACE_OUTER_BOUND('',#8132,.T.);
#5205=FACE_OUTER_BOUND('',#8133,.T.);
#5206=FACE_OUTER_BOUND('',#8134,.T.);
#5207=FACE_OUTER_BOUND('',#8135,.T.);
#5208=FACE_OUTER_BOUND('',#8136,.T.);
#5209=FACE_OUTER_BOUND('',#8137,.T.);
#5210=FACE_OUTER_BOUND('',#8138,.T.);
#5211=FACE_OUTER_BOUND('',#8139,.T.);
#5212=FACE_OUTER_BOUND('',#8140,.T.);
#5213=FACE_OUTER_BOUND('',#8141,.T.);
#5214=FACE_OUTER_BOUND('',#8142,.T.);
#5215=FACE_OUTER_BOUND('',#8143,.T.);
#5216=FACE_OUTER_BOUND('',#8144,.T.);
#5217=FACE_OUTER_BOUND('',#8145,.T.);
#5218=FACE_OUTER_BOUND('',#8146,.T.);
#5219=FACE_OUTER_BOUND('',#8147,.T.);
#5220=FACE_OUTER_BOUND('',#8148,.T.);
#5221=FACE_OUTER_BOUND('',#8149,.T.);
#5222=FACE_OUTER_BOUND('',#8150,.T.);
#5223=FACE_OUTER_BOUND('',#8151,.T.);
#5224=FACE_OUTER_BOUND('',#8152,.T.);
#5225=FACE_OUTER_BOUND('',#8153,.T.);
#5226=FACE_OUTER_BOUND('',#8154,.T.);
#5227=FACE_OUTER_BOUND('',#8155,.T.);
#5228=FACE_OUTER_BOUND('',#8156,.T.);
#5229=FACE_OUTER_BOUND('',#8157,.T.);
#5230=FACE_OUTER_BOUND('',#8158,.T.);
#5231=FACE_OUTER_BOUND('',#8159,.T.);
#5232=FACE_OUTER_BOUND('',#8160,.T.);
#5233=FACE_OUTER_BOUND('',#8161,.T.);
#5234=FACE_OUTER_BOUND('',#8162,.T.);
#5235=FACE_OUTER_BOUND('',#8163,.T.);
#5236=FACE_OUTER_BOUND('',#8164,.T.);
#5237=FACE_OUTER_BOUND('',#8165,.T.);
#5238=FACE_OUTER_BOUND('',#8166,.T.);
#5239=FACE_OUTER_BOUND('',#8167,.T.);
#5240=FACE_OUTER_BOUND('',#8168,.T.);
#5241=FACE_OUTER_BOUND('',#8169,.T.);
#5242=FACE_OUTER_BOUND('',#8170,.T.);
#5243=FACE_OUTER_BOUND('',#8171,.T.);
#5244=FACE_OUTER_BOUND('',#8172,.T.);
#5245=FACE_OUTER_BOUND('',#8173,.T.);
#5246=FACE_OUTER_BOUND('',#8174,.T.);
#5247=FACE_OUTER_BOUND('',#8175,.T.);
#5248=FACE_OUTER_BOUND('',#8177,.T.);
#5249=FACE_OUTER_BOUND('',#8178,.T.);
#5250=FACE_OUTER_BOUND('',#8179,.T.);
#5251=FACE_OUTER_BOUND('',#8180,.T.);
#5252=FACE_OUTER_BOUND('',#8181,.T.);
#5253=FACE_OUTER_BOUND('',#8182,.T.);
#5254=FACE_OUTER_BOUND('',#8183,.T.);
#5255=FACE_OUTER_BOUND('',#8184,.T.);
#5256=FACE_OUTER_BOUND('',#8185,.T.);
#5257=FACE_OUTER_BOUND('',#8186,.T.);
#5258=FACE_OUTER_BOUND('',#8187,.T.);
#5259=FACE_OUTER_BOUND('',#8188,.T.);
#5260=FACE_OUTER_BOUND('',#8189,.T.);
#5261=FACE_OUTER_BOUND('',#8190,.T.);
#5262=FACE_OUTER_BOUND('',#8191,.T.);
#5263=FACE_OUTER_BOUND('',#8192,.T.);
#5264=FACE_OUTER_BOUND('',#8193,.T.);
#5265=FACE_OUTER_BOUND('',#8194,.T.);
#5266=FACE_OUTER_BOUND('',#8195,.T.);
#5267=FACE_OUTER_BOUND('',#8196,.T.);
#5268=FACE_OUTER_BOUND('',#8197,.T.);
#5269=FACE_OUTER_BOUND('',#8198,.T.);
#5270=FACE_OUTER_BOUND('',#8199,.T.);
#5271=FACE_OUTER_BOUND('',#8200,.T.);
#5272=FACE_OUTER_BOUND('',#8201,.T.);
#5273=FACE_OUTER_BOUND('',#8202,.T.);
#5274=FACE_OUTER_BOUND('',#8203,.T.);
#5275=FACE_OUTER_BOUND('',#8204,.T.);
#5276=FACE_OUTER_BOUND('',#8205,.T.);
#5277=FACE_OUTER_BOUND('',#8206,.T.);
#5278=FACE_OUTER_BOUND('',#8207,.T.);
#5279=FACE_OUTER_BOUND('',#8208,.T.);
#5280=FACE_OUTER_BOUND('',#8209,.T.);
#5281=FACE_OUTER_BOUND('',#8210,.T.);
#5282=FACE_OUTER_BOUND('',#8211,.T.);
#5283=FACE_OUTER_BOUND('',#8212,.T.);
#5284=FACE_OUTER_BOUND('',#8213,.T.);
#5285=FACE_OUTER_BOUND('',#8214,.T.);
#5286=FACE_OUTER_BOUND('',#8215,.T.);
#5287=FACE_OUTER_BOUND('',#8216,.T.);
#5288=FACE_OUTER_BOUND('',#8217,.T.);
#5289=FACE_OUTER_BOUND('',#8218,.T.);
#5290=FACE_OUTER_BOUND('',#8219,.T.);
#5291=FACE_OUTER_BOUND('',#8220,.T.);
#5292=FACE_OUTER_BOUND('',#8221,.T.);
#5293=FACE_OUTER_BOUND('',#8222,.T.);
#5294=FACE_OUTER_BOUND('',#8223,.T.);
#5295=FACE_OUTER_BOUND('',#8224,.T.);
#5296=FACE_OUTER_BOUND('',#8225,.T.);
#5297=FACE_OUTER_BOUND('',#8226,.T.);
#5298=FACE_OUTER_BOUND('',#8227,.T.);
#5299=FACE_OUTER_BOUND('',#8228,.T.);
#5300=FACE_OUTER_BOUND('',#8229,.T.);
#5301=FACE_OUTER_BOUND('',#8230,.T.);
#5302=FACE_OUTER_BOUND('',#8231,.T.);
#5303=FACE_OUTER_BOUND('',#8232,.T.);
#5304=FACE_OUTER_BOUND('',#8233,.T.);
#5305=FACE_OUTER_BOUND('',#8234,.T.);
#5306=FACE_OUTER_BOUND('',#8235,.T.);
#5307=FACE_OUTER_BOUND('',#8236,.T.);
#5308=FACE_OUTER_BOUND('',#8237,.T.);
#5309=FACE_OUTER_BOUND('',#8238,.T.);
#5310=FACE_OUTER_BOUND('',#8239,.T.);
#5311=FACE_OUTER_BOUND('',#8240,.T.);
#5312=FACE_OUTER_BOUND('',#8241,.T.);
#5313=FACE_OUTER_BOUND('',#8242,.T.);
#5314=FACE_OUTER_BOUND('',#8243,.T.);
#5315=FACE_OUTER_BOUND('',#8244,.T.);
#5316=FACE_OUTER_BOUND('',#8245,.T.);
#5317=FACE_OUTER_BOUND('',#8246,.T.);
#5318=FACE_OUTER_BOUND('',#8247,.T.);
#5319=FACE_OUTER_BOUND('',#8248,.T.);
#5320=FACE_OUTER_BOUND('',#8249,.T.);
#5321=FACE_OUTER_BOUND('',#8250,.T.);
#5322=FACE_OUTER_BOUND('',#8251,.T.);
#5323=FACE_OUTER_BOUND('',#8252,.T.);
#5324=FACE_OUTER_BOUND('',#8253,.T.);
#5325=FACE_OUTER_BOUND('',#8254,.T.);
#5326=FACE_OUTER_BOUND('',#8255,.T.);
#5327=FACE_OUTER_BOUND('',#8256,.T.);
#5328=FACE_OUTER_BOUND('',#8257,.T.);
#5329=FACE_OUTER_BOUND('',#8258,.T.);
#5330=FACE_OUTER_BOUND('',#8259,.T.);
#5331=FACE_OUTER_BOUND('',#8260,.T.);
#5332=FACE_OUTER_BOUND('',#8261,.T.);
#5333=FACE_OUTER_BOUND('',#8262,.T.);
#5334=FACE_OUTER_BOUND('',#8263,.T.);
#5335=FACE_OUTER_BOUND('',#8264,.T.);
#5336=FACE_OUTER_BOUND('',#8265,.T.);
#5337=FACE_OUTER_BOUND('',#8266,.T.);
#5338=FACE_OUTER_BOUND('',#8267,.T.);
#5339=FACE_OUTER_BOUND('',#8268,.T.);
#5340=FACE_OUTER_BOUND('',#8269,.T.);
#5341=FACE_OUTER_BOUND('',#8270,.T.);
#5342=FACE_OUTER_BOUND('',#8271,.T.);
#5343=FACE_OUTER_BOUND('',#8272,.T.);
#5344=FACE_OUTER_BOUND('',#8273,.T.);
#5345=FACE_OUTER_BOUND('',#8274,.T.);
#5346=FACE_OUTER_BOUND('',#8275,.T.);
#5347=FACE_OUTER_BOUND('',#8276,.T.);
#5348=FACE_OUTER_BOUND('',#8277,.T.);
#5349=FACE_OUTER_BOUND('',#8278,.T.);
#5350=FACE_OUTER_BOUND('',#8279,.T.);
#5351=FACE_OUTER_BOUND('',#8280,.T.);
#5352=FACE_OUTER_BOUND('',#8281,.T.);
#5353=FACE_OUTER_BOUND('',#8282,.T.);
#5354=FACE_OUTER_BOUND('',#8283,.T.);
#5355=FACE_OUTER_BOUND('',#8284,.T.);
#5356=FACE_OUTER_BOUND('',#8285,.T.);
#5357=FACE_OUTER_BOUND('',#8286,.T.);
#5358=FACE_OUTER_BOUND('',#8287,.T.);
#5359=FACE_OUTER_BOUND('',#8288,.T.);
#5360=FACE_OUTER_BOUND('',#8289,.T.);
#5361=FACE_OUTER_BOUND('',#8290,.T.);
#5362=FACE_OUTER_BOUND('',#8291,.T.);
#5363=FACE_OUTER_BOUND('',#8292,.T.);
#5364=FACE_OUTER_BOUND('',#8293,.T.);
#5365=FACE_OUTER_BOUND('',#8294,.T.);
#5366=FACE_OUTER_BOUND('',#8295,.T.);
#5367=FACE_OUTER_BOUND('',#8296,.T.);
#5368=FACE_OUTER_BOUND('',#8297,.T.);
#5369=FACE_OUTER_BOUND('',#8298,.T.);
#5370=FACE_OUTER_BOUND('',#8299,.T.);
#5371=FACE_OUTER_BOUND('',#8300,.T.);
#5372=FACE_OUTER_BOUND('',#8301,.T.);
#5373=FACE_OUTER_BOUND('',#8302,.T.);
#5374=FACE_OUTER_BOUND('',#8303,.T.);
#5375=FACE_OUTER_BOUND('',#8304,.T.);
#5376=FACE_OUTER_BOUND('',#8305,.T.);
#5377=FACE_OUTER_BOUND('',#8306,.T.);
#5378=FACE_OUTER_BOUND('',#8307,.T.);
#5379=FACE_OUTER_BOUND('',#8308,.T.);
#5380=FACE_OUTER_BOUND('',#8309,.T.);
#5381=FACE_OUTER_BOUND('',#8310,.T.);
#5382=FACE_OUTER_BOUND('',#8311,.T.);
#5383=FACE_OUTER_BOUND('',#8312,.T.);
#5384=FACE_OUTER_BOUND('',#8313,.T.);
#5385=FACE_OUTER_BOUND('',#8314,.T.);
#5386=FACE_OUTER_BOUND('',#8315,.T.);
#5387=FACE_OUTER_BOUND('',#8316,.T.);
#5388=FACE_OUTER_BOUND('',#8317,.T.);
#5389=FACE_OUTER_BOUND('',#8318,.T.);
#5390=FACE_OUTER_BOUND('',#8319,.T.);
#5391=FACE_OUTER_BOUND('',#8320,.T.);
#5392=FACE_OUTER_BOUND('',#8321,.T.);
#5393=FACE_OUTER_BOUND('',#8322,.T.);
#5394=FACE_OUTER_BOUND('',#8323,.T.);
#5395=FACE_OUTER_BOUND('',#8324,.T.);
#5396=FACE_OUTER_BOUND('',#8325,.T.);
#5397=FACE_OUTER_BOUND('',#8326,.T.);
#5398=FACE_OUTER_BOUND('',#8327,.T.);
#5399=FACE_OUTER_BOUND('',#8328,.T.);
#5400=FACE_OUTER_BOUND('',#8329,.T.);
#5401=FACE_OUTER_BOUND('',#8330,.T.);
#5402=FACE_OUTER_BOUND('',#8331,.T.);
#5403=FACE_OUTER_BOUND('',#8332,.T.);
#5404=FACE_OUTER_BOUND('',#8333,.T.);
#5405=FACE_OUTER_BOUND('',#8334,.T.);
#5406=FACE_OUTER_BOUND('',#8335,.T.);
#5407=FACE_OUTER_BOUND('',#8336,.T.);
#5408=FACE_OUTER_BOUND('',#8337,.T.);
#5409=FACE_OUTER_BOUND('',#8338,.T.);
#5410=FACE_OUTER_BOUND('',#8339,.T.);
#5411=FACE_OUTER_BOUND('',#8340,.T.);
#5412=FACE_OUTER_BOUND('',#8341,.T.);
#5413=FACE_OUTER_BOUND('',#8342,.T.);
#5414=FACE_OUTER_BOUND('',#8343,.T.);
#5415=FACE_OUTER_BOUND('',#8344,.T.);
#5416=FACE_OUTER_BOUND('',#8345,.T.);
#5417=FACE_OUTER_BOUND('',#8346,.T.);
#5418=FACE_OUTER_BOUND('',#8347,.T.);
#5419=FACE_OUTER_BOUND('',#8348,.T.);
#5420=FACE_OUTER_BOUND('',#8349,.T.);
#5421=FACE_OUTER_BOUND('',#8350,.T.);
#5422=FACE_OUTER_BOUND('',#8351,.T.);
#5423=FACE_OUTER_BOUND('',#8352,.T.);
#5424=FACE_OUTER_BOUND('',#8353,.T.);
#5425=FACE_OUTER_BOUND('',#8354,.T.);
#5426=FACE_OUTER_BOUND('',#8355,.T.);
#5427=FACE_OUTER_BOUND('',#8356,.T.);
#5428=FACE_OUTER_BOUND('',#8357,.T.);
#5429=FACE_OUTER_BOUND('',#8358,.T.);
#5430=FACE_OUTER_BOUND('',#8359,.T.);
#5431=FACE_OUTER_BOUND('',#8360,.T.);
#5432=FACE_OUTER_BOUND('',#8361,.T.);
#5433=FACE_OUTER_BOUND('',#8362,.T.);
#5434=FACE_OUTER_BOUND('',#8363,.T.);
#5435=FACE_OUTER_BOUND('',#8364,.T.);
#5436=FACE_OUTER_BOUND('',#8365,.T.);
#5437=FACE_OUTER_BOUND('',#8366,.T.);
#5438=FACE_OUTER_BOUND('',#8367,.T.);
#5439=FACE_OUTER_BOUND('',#8368,.T.);
#5440=FACE_OUTER_BOUND('',#8369,.T.);
#5441=FACE_OUTER_BOUND('',#8370,.T.);
#5442=FACE_OUTER_BOUND('',#8371,.T.);
#5443=FACE_OUTER_BOUND('',#8372,.T.);
#5444=FACE_OUTER_BOUND('',#8373,.T.);
#5445=FACE_OUTER_BOUND('',#8374,.T.);
#5446=FACE_OUTER_BOUND('',#8375,.T.);
#5447=FACE_OUTER_BOUND('',#8376,.T.);
#5448=FACE_OUTER_BOUND('',#8377,.T.);
#5449=FACE_OUTER_BOUND('',#8378,.T.);
#5450=FACE_OUTER_BOUND('',#8379,.T.);
#5451=FACE_OUTER_BOUND('',#8380,.T.);
#5452=FACE_OUTER_BOUND('',#8381,.T.);
#5453=FACE_OUTER_BOUND('',#8382,.T.);
#5454=FACE_OUTER_BOUND('',#8383,.T.);
#5455=FACE_OUTER_BOUND('',#8384,.T.);
#5456=FACE_OUTER_BOUND('',#8385,.T.);
#5457=FACE_OUTER_BOUND('',#8386,.T.);
#5458=FACE_OUTER_BOUND('',#8387,.T.);
#5459=FACE_OUTER_BOUND('',#8388,.T.);
#5460=FACE_OUTER_BOUND('',#8389,.T.);
#5461=FACE_OUTER_BOUND('',#8390,.T.);
#5462=FACE_OUTER_BOUND('',#8391,.T.);
#5463=FACE_OUTER_BOUND('',#8392,.T.);
#5464=FACE_OUTER_BOUND('',#8393,.T.);
#5465=FACE_OUTER_BOUND('',#8394,.T.);
#5466=FACE_OUTER_BOUND('',#8395,.T.);
#5467=FACE_OUTER_BOUND('',#8396,.T.);
#5468=FACE_OUTER_BOUND('',#8397,.T.);
#5469=FACE_OUTER_BOUND('',#8398,.T.);
#5470=FACE_OUTER_BOUND('',#8399,.T.);
#5471=FACE_OUTER_BOUND('',#8400,.T.);
#5472=FACE_OUTER_BOUND('',#8401,.T.);
#5473=FACE_OUTER_BOUND('',#8402,.T.);
#5474=FACE_OUTER_BOUND('',#8403,.T.);
#5475=FACE_OUTER_BOUND('',#8404,.T.);
#5476=FACE_OUTER_BOUND('',#8405,.T.);
#5477=FACE_OUTER_BOUND('',#8406,.T.);
#5478=FACE_OUTER_BOUND('',#8407,.T.);
#5479=FACE_OUTER_BOUND('',#8408,.T.);
#5480=FACE_OUTER_BOUND('',#8409,.T.);
#5481=FACE_OUTER_BOUND('',#8410,.T.);
#5482=FACE_OUTER_BOUND('',#8411,.T.);
#5483=FACE_OUTER_BOUND('',#8412,.T.);
#5484=FACE_OUTER_BOUND('',#8413,.T.);
#5485=FACE_OUTER_BOUND('',#8414,.T.);
#5486=FACE_OUTER_BOUND('',#8415,.T.);
#5487=FACE_OUTER_BOUND('',#8416,.T.);
#5488=FACE_OUTER_BOUND('',#8417,.T.);
#5489=FACE_OUTER_BOUND('',#8418,.T.);
#5490=FACE_OUTER_BOUND('',#8419,.T.);
#5491=FACE_OUTER_BOUND('',#8420,.T.);
#5492=FACE_OUTER_BOUND('',#8421,.T.);
#5493=FACE_OUTER_BOUND('',#8422,.T.);
#5494=FACE_OUTER_BOUND('',#8423,.T.);
#5495=FACE_OUTER_BOUND('',#8424,.T.);
#5496=FACE_OUTER_BOUND('',#8425,.T.);
#5497=FACE_OUTER_BOUND('',#8426,.T.);
#5498=FACE_OUTER_BOUND('',#8427,.T.);
#5499=FACE_OUTER_BOUND('',#8428,.T.);
#5500=FACE_OUTER_BOUND('',#8429,.T.);
#5501=FACE_OUTER_BOUND('',#8430,.T.);
#5502=FACE_OUTER_BOUND('',#8431,.T.);
#5503=FACE_OUTER_BOUND('',#8432,.T.);
#5504=FACE_OUTER_BOUND('',#8433,.T.);
#5505=FACE_OUTER_BOUND('',#8434,.T.);
#5506=FACE_OUTER_BOUND('',#8435,.T.);
#5507=FACE_OUTER_BOUND('',#8436,.T.);
#5508=FACE_OUTER_BOUND('',#8437,.T.);
#5509=FACE_OUTER_BOUND('',#8438,.T.);
#5510=FACE_OUTER_BOUND('',#8439,.T.);
#5511=FACE_OUTER_BOUND('',#8440,.T.);
#5512=FACE_OUTER_BOUND('',#8441,.T.);
#5513=FACE_OUTER_BOUND('',#8442,.T.);
#5514=FACE_OUTER_BOUND('',#8443,.T.);
#5515=FACE_OUTER_BOUND('',#8444,.T.);
#5516=FACE_OUTER_BOUND('',#8445,.T.);
#5517=FACE_OUTER_BOUND('',#8446,.T.);
#5518=FACE_OUTER_BOUND('',#8447,.T.);
#5519=FACE_OUTER_BOUND('',#8448,.T.);
#5520=FACE_OUTER_BOUND('',#8449,.T.);
#5521=FACE_OUTER_BOUND('',#8450,.T.);
#5522=FACE_OUTER_BOUND('',#8451,.T.);
#5523=FACE_OUTER_BOUND('',#8452,.T.);
#5524=FACE_OUTER_BOUND('',#8453,.T.);
#5525=FACE_OUTER_BOUND('',#8454,.T.);
#5526=FACE_OUTER_BOUND('',#8455,.T.);
#5527=FACE_OUTER_BOUND('',#8456,.T.);
#5528=FACE_OUTER_BOUND('',#8457,.T.);
#5529=FACE_OUTER_BOUND('',#8458,.T.);
#5530=FACE_OUTER_BOUND('',#8459,.T.);
#5531=FACE_OUTER_BOUND('',#8460,.T.);
#5532=FACE_OUTER_BOUND('',#8461,.T.);
#5533=FACE_OUTER_BOUND('',#8462,.T.);
#5534=FACE_OUTER_BOUND('',#8463,.T.);
#5535=FACE_OUTER_BOUND('',#8464,.T.);
#5536=FACE_OUTER_BOUND('',#8465,.T.);
#5537=FACE_OUTER_BOUND('',#8466,.T.);
#5538=FACE_OUTER_BOUND('',#8467,.T.);
#5539=FACE_OUTER_BOUND('',#8468,.T.);
#5540=FACE_OUTER_BOUND('',#8469,.T.);
#5541=FACE_OUTER_BOUND('',#8470,.T.);
#5542=FACE_OUTER_BOUND('',#8471,.T.);
#5543=FACE_OUTER_BOUND('',#8472,.T.);
#5544=FACE_OUTER_BOUND('',#8473,.T.);
#5545=FACE_OUTER_BOUND('',#8474,.T.);
#5546=FACE_OUTER_BOUND('',#8475,.T.);
#5547=FACE_OUTER_BOUND('',#8476,.T.);
#5548=FACE_OUTER_BOUND('',#8477,.T.);
#5549=FACE_OUTER_BOUND('',#8478,.T.);
#5550=FACE_OUTER_BOUND('',#8479,.T.);
#5551=FACE_OUTER_BOUND('',#8480,.T.);
#5552=FACE_OUTER_BOUND('',#8481,.T.);
#5553=FACE_OUTER_BOUND('',#8482,.T.);
#5554=FACE_OUTER_BOUND('',#8483,.T.);
#5555=FACE_OUTER_BOUND('',#8484,.T.);
#5556=FACE_OUTER_BOUND('',#8485,.T.);
#5557=FACE_OUTER_BOUND('',#8486,.T.);
#5558=FACE_OUTER_BOUND('',#8487,.T.);
#5559=FACE_OUTER_BOUND('',#8488,.T.);
#5560=FACE_OUTER_BOUND('',#8489,.T.);
#5561=FACE_OUTER_BOUND('',#8490,.T.);
#5562=FACE_OUTER_BOUND('',#8491,.T.);
#5563=FACE_OUTER_BOUND('',#8492,.T.);
#5564=FACE_OUTER_BOUND('',#8493,.T.);
#5565=FACE_OUTER_BOUND('',#8494,.T.);
#5566=FACE_OUTER_BOUND('',#8495,.T.);
#5567=FACE_OUTER_BOUND('',#8496,.T.);
#5568=FACE_OUTER_BOUND('',#8497,.T.);
#5569=FACE_OUTER_BOUND('',#8498,.T.);
#5570=FACE_OUTER_BOUND('',#8499,.T.);
#5571=FACE_OUTER_BOUND('',#8500,.T.);
#5572=FACE_OUTER_BOUND('',#8501,.T.);
#5573=FACE_OUTER_BOUND('',#8502,.T.);
#5574=FACE_OUTER_BOUND('',#8503,.T.);
#5575=FACE_OUTER_BOUND('',#8504,.T.);
#5576=FACE_OUTER_BOUND('',#8505,.T.);
#5577=FACE_OUTER_BOUND('',#8506,.T.);
#5578=FACE_OUTER_BOUND('',#8507,.T.);
#5579=FACE_OUTER_BOUND('',#8508,.T.);
#5580=FACE_OUTER_BOUND('',#8509,.T.);
#5581=FACE_OUTER_BOUND('',#8510,.T.);
#5582=FACE_OUTER_BOUND('',#8511,.T.);
#5583=FACE_OUTER_BOUND('',#8512,.T.);
#5584=FACE_OUTER_BOUND('',#8513,.T.);
#5585=FACE_OUTER_BOUND('',#8514,.T.);
#5586=FACE_OUTER_BOUND('',#8515,.T.);
#5587=FACE_OUTER_BOUND('',#8516,.T.);
#5588=FACE_OUTER_BOUND('',#8517,.T.);
#5589=FACE_OUTER_BOUND('',#8518,.T.);
#5590=FACE_OUTER_BOUND('',#8519,.T.);
#5591=FACE_OUTER_BOUND('',#8520,.T.);
#5592=FACE_OUTER_BOUND('',#8521,.T.);
#5593=FACE_OUTER_BOUND('',#8522,.T.);
#5594=FACE_OUTER_BOUND('',#8523,.T.);
#5595=FACE_OUTER_BOUND('',#8524,.T.);
#5596=FACE_OUTER_BOUND('',#8525,.T.);
#5597=FACE_OUTER_BOUND('',#8526,.T.);
#5598=FACE_OUTER_BOUND('',#8527,.T.);
#5599=FACE_OUTER_BOUND('',#8528,.T.);
#5600=FACE_OUTER_BOUND('',#8529,.T.);
#5601=FACE_OUTER_BOUND('',#8530,.T.);
#5602=FACE_OUTER_BOUND('',#8531,.T.);
#5603=FACE_OUTER_BOUND('',#8532,.T.);
#5604=FACE_OUTER_BOUND('',#8533,.T.);
#5605=FACE_OUTER_BOUND('',#8534,.T.);
#5606=FACE_OUTER_BOUND('',#8535,.T.);
#5607=FACE_OUTER_BOUND('',#8536,.T.);
#5608=FACE_OUTER_BOUND('',#8537,.T.);
#5609=FACE_OUTER_BOUND('',#8538,.T.);
#5610=FACE_OUTER_BOUND('',#8539,.T.);
#5611=FACE_OUTER_BOUND('',#8540,.T.);
#5612=FACE_OUTER_BOUND('',#8541,.T.);
#5613=FACE_OUTER_BOUND('',#8542,.T.);
#5614=FACE_OUTER_BOUND('',#8543,.T.);
#5615=FACE_OUTER_BOUND('',#8544,.T.);
#5616=FACE_OUTER_BOUND('',#8545,.T.);
#5617=FACE_OUTER_BOUND('',#8546,.T.);
#5618=FACE_OUTER_BOUND('',#8547,.T.);
#5619=FACE_OUTER_BOUND('',#8548,.T.);
#5620=FACE_OUTER_BOUND('',#8549,.T.);
#5621=FACE_OUTER_BOUND('',#8550,.T.);
#5622=FACE_OUTER_BOUND('',#8551,.T.);
#5623=FACE_OUTER_BOUND('',#8552,.T.);
#5624=FACE_OUTER_BOUND('',#8553,.T.);
#5625=FACE_OUTER_BOUND('',#8554,.T.);
#5626=FACE_OUTER_BOUND('',#8555,.T.);
#5627=FACE_OUTER_BOUND('',#8556,.T.);
#5628=FACE_OUTER_BOUND('',#8557,.T.);
#5629=FACE_OUTER_BOUND('',#8558,.T.);
#5630=FACE_OUTER_BOUND('',#8559,.T.);
#5631=FACE_OUTER_BOUND('',#8560,.T.);
#5632=FACE_OUTER_BOUND('',#8561,.T.);
#5633=FACE_OUTER_BOUND('',#8562,.T.);
#5634=FACE_OUTER_BOUND('',#8563,.T.);
#5635=FACE_OUTER_BOUND('',#8564,.T.);
#5636=FACE_OUTER_BOUND('',#8565,.T.);
#5637=FACE_OUTER_BOUND('',#8566,.T.);
#5638=FACE_OUTER_BOUND('',#8567,.T.);
#5639=FACE_OUTER_BOUND('',#8568,.T.);
#5640=FACE_OUTER_BOUND('',#8569,.T.);
#5641=FACE_OUTER_BOUND('',#8570,.T.);
#5642=FACE_OUTER_BOUND('',#8571,.T.);
#5643=FACE_OUTER_BOUND('',#8572,.T.);
#5644=FACE_OUTER_BOUND('',#8573,.T.);
#5645=FACE_OUTER_BOUND('',#8574,.T.);
#5646=FACE_OUTER_BOUND('',#8575,.T.);
#5647=FACE_OUTER_BOUND('',#8576,.T.);
#5648=FACE_OUTER_BOUND('',#8577,.T.);
#5649=FACE_OUTER_BOUND('',#8578,.T.);
#5650=FACE_OUTER_BOUND('',#8579,.T.);
#5651=FACE_OUTER_BOUND('',#8580,.T.);
#5652=FACE_OUTER_BOUND('',#8581,.T.);
#5653=FACE_OUTER_BOUND('',#8582,.T.);
#5654=FACE_OUTER_BOUND('',#8583,.T.);
#5655=FACE_OUTER_BOUND('',#8584,.T.);
#5656=FACE_OUTER_BOUND('',#8585,.T.);
#5657=FACE_OUTER_BOUND('',#8586,.T.);
#5658=FACE_OUTER_BOUND('',#8587,.T.);
#5659=FACE_OUTER_BOUND('',#8588,.T.);
#5660=FACE_OUTER_BOUND('',#8589,.T.);
#5661=FACE_OUTER_BOUND('',#8590,.T.);
#5662=FACE_OUTER_BOUND('',#8591,.T.);
#5663=FACE_OUTER_BOUND('',#8592,.T.);
#5664=FACE_OUTER_BOUND('',#8593,.T.);
#5665=FACE_OUTER_BOUND('',#8594,.T.);
#5666=FACE_OUTER_BOUND('',#8595,.T.);
#5667=FACE_OUTER_BOUND('',#8596,.T.);
#5668=FACE_OUTER_BOUND('',#8597,.T.);
#5669=FACE_OUTER_BOUND('',#8598,.T.);
#5670=FACE_OUTER_BOUND('',#8599,.T.);
#5671=FACE_OUTER_BOUND('',#8600,.T.);
#5672=FACE_OUTER_BOUND('',#8601,.T.);
#5673=FACE_OUTER_BOUND('',#8602,.T.);
#5674=FACE_OUTER_BOUND('',#8603,.T.);
#5675=FACE_OUTER_BOUND('',#8604,.T.);
#5676=FACE_OUTER_BOUND('',#8605,.T.);
#5677=FACE_OUTER_BOUND('',#8606,.T.);
#5678=FACE_OUTER_BOUND('',#8607,.T.);
#5679=FACE_OUTER_BOUND('',#8608,.T.);
#5680=FACE_OUTER_BOUND('',#8609,.T.);
#5681=FACE_OUTER_BOUND('',#8610,.T.);
#5682=FACE_OUTER_BOUND('',#8611,.T.);
#5683=FACE_OUTER_BOUND('',#8612,.T.);
#5684=FACE_OUTER_BOUND('',#8613,.T.);
#5685=FACE_OUTER_BOUND('',#8614,.T.);
#5686=FACE_OUTER_BOUND('',#8615,.T.);
#5687=FACE_OUTER_BOUND('',#8616,.T.);
#5688=FACE_OUTER_BOUND('',#8617,.T.);
#5689=FACE_OUTER_BOUND('',#8618,.T.);
#5690=FACE_OUTER_BOUND('',#8619,.T.);
#5691=FACE_OUTER_BOUND('',#8620,.T.);
#5692=FACE_OUTER_BOUND('',#8621,.T.);
#5693=FACE_OUTER_BOUND('',#8622,.T.);
#5694=FACE_OUTER_BOUND('',#8623,.T.);
#5695=FACE_OUTER_BOUND('',#8624,.T.);
#5696=FACE_OUTER_BOUND('',#8625,.T.);
#5697=FACE_OUTER_BOUND('',#8626,.T.);
#5698=FACE_OUTER_BOUND('',#8627,.T.);
#5699=FACE_OUTER_BOUND('',#8628,.T.);
#5700=FACE_OUTER_BOUND('',#8629,.T.);
#5701=FACE_OUTER_BOUND('',#8630,.T.);
#5702=FACE_OUTER_BOUND('',#8631,.T.);
#5703=FACE_OUTER_BOUND('',#8632,.T.);
#5704=FACE_OUTER_BOUND('',#8633,.T.);
#5705=FACE_OUTER_BOUND('',#8634,.T.);
#5706=FACE_OUTER_BOUND('',#8635,.T.);
#5707=FACE_OUTER_BOUND('',#8636,.T.);
#5708=FACE_OUTER_BOUND('',#8637,.T.);
#5709=FACE_OUTER_BOUND('',#8638,.T.);
#5710=FACE_OUTER_BOUND('',#8639,.T.);
#5711=FACE_OUTER_BOUND('',#8640,.T.);
#5712=FACE_OUTER_BOUND('',#8641,.T.);
#5713=FACE_OUTER_BOUND('',#8642,.T.);
#5714=FACE_OUTER_BOUND('',#8643,.T.);
#5715=FACE_OUTER_BOUND('',#8644,.T.);
#5716=FACE_OUTER_BOUND('',#8645,.T.);
#5717=FACE_OUTER_BOUND('',#8646,.T.);
#5718=FACE_OUTER_BOUND('',#8647,.T.);
#5719=FACE_OUTER_BOUND('',#8648,.T.);
#5720=FACE_OUTER_BOUND('',#8649,.T.);
#5721=FACE_OUTER_BOUND('',#8650,.T.);
#5722=FACE_OUTER_BOUND('',#8651,.T.);
#5723=FACE_OUTER_BOUND('',#8652,.T.);
#5724=FACE_OUTER_BOUND('',#8653,.T.);
#5725=FACE_OUTER_BOUND('',#8654,.T.);
#5726=FACE_OUTER_BOUND('',#8655,.T.);
#5727=FACE_OUTER_BOUND('',#8656,.T.);
#5728=FACE_OUTER_BOUND('',#8657,.T.);
#5729=FACE_OUTER_BOUND('',#8658,.T.);
#5730=FACE_OUTER_BOUND('',#8659,.T.);
#5731=FACE_OUTER_BOUND('',#8660,.T.);
#5732=FACE_OUTER_BOUND('',#8661,.T.);
#5733=FACE_OUTER_BOUND('',#8662,.T.);
#5734=FACE_OUTER_BOUND('',#8663,.T.);
#5735=FACE_OUTER_BOUND('',#8664,.T.);
#5736=FACE_OUTER_BOUND('',#8665,.T.);
#5737=FACE_OUTER_BOUND('',#8666,.T.);
#5738=FACE_OUTER_BOUND('',#8667,.T.);
#5739=FACE_OUTER_BOUND('',#8668,.T.);
#5740=FACE_OUTER_BOUND('',#8669,.T.);
#5741=FACE_OUTER_BOUND('',#8670,.T.);
#5742=FACE_OUTER_BOUND('',#8671,.T.);
#5743=FACE_OUTER_BOUND('',#8672,.T.);
#5744=FACE_OUTER_BOUND('',#8673,.T.);
#5745=FACE_OUTER_BOUND('',#8674,.T.);
#5746=FACE_OUTER_BOUND('',#8675,.T.);
#5747=FACE_OUTER_BOUND('',#8676,.T.);
#5748=FACE_OUTER_BOUND('',#8677,.T.);
#5749=FACE_OUTER_BOUND('',#8678,.T.);
#5750=FACE_OUTER_BOUND('',#8679,.T.);
#5751=FACE_OUTER_BOUND('',#8680,.T.);
#5752=FACE_OUTER_BOUND('',#8681,.T.);
#5753=FACE_OUTER_BOUND('',#8682,.T.);
#5754=FACE_OUTER_BOUND('',#8683,.T.);
#5755=FACE_OUTER_BOUND('',#8684,.T.);
#5756=FACE_OUTER_BOUND('',#8685,.T.);
#5757=FACE_OUTER_BOUND('',#8686,.T.);
#5758=FACE_OUTER_BOUND('',#8687,.T.);
#5759=FACE_OUTER_BOUND('',#8688,.T.);
#5760=FACE_OUTER_BOUND('',#8689,.T.);
#5761=FACE_OUTER_BOUND('',#8690,.T.);
#5762=FACE_OUTER_BOUND('',#8691,.T.);
#5763=FACE_OUTER_BOUND('',#8692,.T.);
#5764=FACE_OUTER_BOUND('',#8693,.T.);
#5765=FACE_OUTER_BOUND('',#8694,.T.);
#5766=FACE_OUTER_BOUND('',#8695,.T.);
#5767=FACE_OUTER_BOUND('',#8696,.T.);
#5768=FACE_OUTER_BOUND('',#8697,.T.);
#5769=FACE_OUTER_BOUND('',#8698,.T.);
#5770=FACE_OUTER_BOUND('',#8699,.T.);
#5771=FACE_OUTER_BOUND('',#8700,.T.);
#5772=FACE_OUTER_BOUND('',#8701,.T.);
#5773=FACE_OUTER_BOUND('',#8702,.T.);
#5774=FACE_OUTER_BOUND('',#8703,.T.);
#5775=FACE_OUTER_BOUND('',#8704,.T.);
#5776=FACE_OUTER_BOUND('',#8705,.T.);
#5777=FACE_OUTER_BOUND('',#8706,.T.);
#5778=FACE_OUTER_BOUND('',#8707,.T.);
#5779=FACE_OUTER_BOUND('',#8708,.T.);
#5780=FACE_OUTER_BOUND('',#8709,.T.);
#5781=FACE_OUTER_BOUND('',#8710,.T.);
#5782=FACE_OUTER_BOUND('',#8711,.T.);
#5783=FACE_OUTER_BOUND('',#8712,.T.);
#5784=FACE_OUTER_BOUND('',#8713,.T.);
#5785=FACE_OUTER_BOUND('',#8714,.T.);
#5786=FACE_OUTER_BOUND('',#8715,.T.);
#5787=FACE_OUTER_BOUND('',#8716,.T.);
#5788=FACE_OUTER_BOUND('',#8717,.T.);
#5789=FACE_OUTER_BOUND('',#8718,.T.);
#5790=FACE_OUTER_BOUND('',#8719,.T.);
#5791=FACE_OUTER_BOUND('',#8720,.T.);
#5792=FACE_OUTER_BOUND('',#8721,.T.);
#5793=FACE_OUTER_BOUND('',#8722,.T.);
#5794=FACE_OUTER_BOUND('',#8723,.T.);
#5795=FACE_OUTER_BOUND('',#8724,.T.);
#5796=FACE_OUTER_BOUND('',#8725,.T.);
#5797=FACE_OUTER_BOUND('',#8726,.T.);
#5798=FACE_OUTER_BOUND('',#8727,.T.);
#5799=FACE_OUTER_BOUND('',#8728,.T.);
#5800=FACE_OUTER_BOUND('',#8729,.T.);
#5801=FACE_OUTER_BOUND('',#8730,.T.);
#5802=FACE_OUTER_BOUND('',#8731,.T.);
#5803=FACE_OUTER_BOUND('',#8732,.T.);
#5804=FACE_OUTER_BOUND('',#8733,.T.);
#5805=FACE_OUTER_BOUND('',#8734,.T.);
#5806=FACE_OUTER_BOUND('',#8735,.T.);
#5807=FACE_OUTER_BOUND('',#8736,.T.);
#5808=FACE_OUTER_BOUND('',#8737,.T.);
#5809=FACE_OUTER_BOUND('',#8738,.T.);
#5810=FACE_OUTER_BOUND('',#8739,.T.);
#5811=FACE_OUTER_BOUND('',#8740,.T.);
#5812=FACE_OUTER_BOUND('',#8741,.T.);
#5813=FACE_OUTER_BOUND('',#8742,.T.);
#5814=FACE_OUTER_BOUND('',#8743,.T.);
#5815=FACE_OUTER_BOUND('',#8744,.T.);
#5816=FACE_OUTER_BOUND('',#8745,.T.);
#5817=FACE_OUTER_BOUND('',#8746,.T.);
#5818=FACE_OUTER_BOUND('',#8747,.T.);
#5819=FACE_OUTER_BOUND('',#8748,.T.);
#5820=FACE_OUTER_BOUND('',#8749,.T.);
#5821=FACE_OUTER_BOUND('',#8750,.T.);
#5822=FACE_OUTER_BOUND('',#8751,.T.);
#5823=FACE_OUTER_BOUND('',#8752,.T.);
#5824=FACE_OUTER_BOUND('',#8753,.T.);
#5825=FACE_OUTER_BOUND('',#8754,.T.);
#5826=FACE_OUTER_BOUND('',#8755,.T.);
#5827=FACE_OUTER_BOUND('',#8756,.T.);
#5828=FACE_OUTER_BOUND('',#8757,.T.);
#5829=FACE_OUTER_BOUND('',#8758,.T.);
#5830=FACE_OUTER_BOUND('',#8759,.T.);
#5831=FACE_OUTER_BOUND('',#8760,.T.);
#5832=FACE_OUTER_BOUND('',#8761,.T.);
#5833=FACE_OUTER_BOUND('',#8762,.T.);
#5834=FACE_OUTER_BOUND('',#8763,.T.);
#5835=FACE_OUTER_BOUND('',#8764,.T.);
#5836=FACE_OUTER_BOUND('',#8765,.T.);
#5837=FACE_OUTER_BOUND('',#8766,.T.);
#5838=FACE_OUTER_BOUND('',#8767,.T.);
#5839=FACE_OUTER_BOUND('',#8768,.T.);
#5840=FACE_OUTER_BOUND('',#8769,.T.);
#5841=FACE_OUTER_BOUND('',#8770,.T.);
#5842=FACE_OUTER_BOUND('',#8771,.T.);
#5843=FACE_OUTER_BOUND('',#8772,.T.);
#5844=FACE_OUTER_BOUND('',#8773,.T.);
#5845=FACE_OUTER_BOUND('',#8774,.T.);
#5846=FACE_OUTER_BOUND('',#8775,.T.);
#5847=FACE_OUTER_BOUND('',#8776,.T.);
#5848=FACE_OUTER_BOUND('',#8777,.T.);
#5849=FACE_OUTER_BOUND('',#8778,.T.);
#5850=FACE_OUTER_BOUND('',#8779,.T.);
#5851=FACE_OUTER_BOUND('',#8780,.T.);
#5852=FACE_OUTER_BOUND('',#8781,.T.);
#5853=FACE_OUTER_BOUND('',#8782,.T.);
#5854=FACE_OUTER_BOUND('',#8783,.T.);
#5855=FACE_OUTER_BOUND('',#8784,.T.);
#5856=FACE_OUTER_BOUND('',#8785,.T.);
#5857=FACE_OUTER_BOUND('',#8786,.T.);
#5858=FACE_OUTER_BOUND('',#8787,.T.);
#5859=FACE_OUTER_BOUND('',#8788,.T.);
#5860=FACE_OUTER_BOUND('',#8789,.T.);
#5861=FACE_OUTER_BOUND('',#8790,.T.);
#5862=FACE_OUTER_BOUND('',#8791,.T.);
#5863=FACE_OUTER_BOUND('',#8792,.T.);
#5864=FACE_OUTER_BOUND('',#8793,.T.);
#5865=FACE_OUTER_BOUND('',#8794,.T.);
#5866=FACE_OUTER_BOUND('',#8795,.T.);
#5867=FACE_OUTER_BOUND('',#8796,.T.);
#5868=FACE_OUTER_BOUND('',#8797,.T.);
#5869=FACE_OUTER_BOUND('',#8798,.T.);
#5870=FACE_OUTER_BOUND('',#8799,.T.);
#5871=FACE_OUTER_BOUND('',#8800,.T.);
#5872=FACE_OUTER_BOUND('',#8801,.T.);
#5873=FACE_OUTER_BOUND('',#8802,.T.);
#5874=FACE_OUTER_BOUND('',#8803,.T.);
#5875=FACE_OUTER_BOUND('',#8804,.T.);
#5876=FACE_OUTER_BOUND('',#8805,.T.);
#5877=FACE_OUTER_BOUND('',#8806,.T.);
#5878=FACE_OUTER_BOUND('',#8807,.T.);
#5879=FACE_OUTER_BOUND('',#8808,.T.);
#5880=FACE_OUTER_BOUND('',#8809,.T.);
#5881=FACE_OUTER_BOUND('',#8810,.T.);
#5882=FACE_OUTER_BOUND('',#8811,.T.);
#5883=FACE_OUTER_BOUND('',#8812,.T.);
#5884=FACE_OUTER_BOUND('',#8813,.T.);
#5885=FACE_OUTER_BOUND('',#8814,.T.);
#5886=FACE_OUTER_BOUND('',#8815,.T.);
#5887=FACE_OUTER_BOUND('',#8816,.T.);
#5888=FACE_OUTER_BOUND('',#8817,.T.);
#5889=FACE_OUTER_BOUND('',#8818,.T.);
#5890=FACE_OUTER_BOUND('',#8819,.T.);
#5891=FACE_OUTER_BOUND('',#8820,.T.);
#5892=FACE_OUTER_BOUND('',#8821,.T.);
#5893=FACE_OUTER_BOUND('',#8822,.T.);
#5894=FACE_OUTER_BOUND('',#8823,.T.);
#5895=FACE_OUTER_BOUND('',#8824,.T.);
#5896=FACE_OUTER_BOUND('',#8825,.T.);
#5897=FACE_OUTER_BOUND('',#8826,.T.);
#5898=FACE_OUTER_BOUND('',#8827,.T.);
#5899=FACE_OUTER_BOUND('',#8828,.T.);
#5900=FACE_OUTER_BOUND('',#8829,.T.);
#5901=FACE_OUTER_BOUND('',#8830,.T.);
#5902=FACE_OUTER_BOUND('',#8831,.T.);
#5903=FACE_OUTER_BOUND('',#8832,.T.);
#5904=FACE_OUTER_BOUND('',#8833,.T.);
#5905=FACE_OUTER_BOUND('',#8834,.T.);
#5906=FACE_OUTER_BOUND('',#8835,.T.);
#5907=FACE_OUTER_BOUND('',#8836,.T.);
#5908=FACE_OUTER_BOUND('',#8837,.T.);
#5909=FACE_OUTER_BOUND('',#8838,.T.);
#5910=FACE_OUTER_BOUND('',#8839,.T.);
#5911=FACE_OUTER_BOUND('',#8840,.T.);
#5912=FACE_OUTER_BOUND('',#8841,.T.);
#5913=FACE_OUTER_BOUND('',#8842,.T.);
#5914=FACE_OUTER_BOUND('',#8843,.T.);
#5915=FACE_OUTER_BOUND('',#8844,.T.);
#5916=FACE_OUTER_BOUND('',#8845,.T.);
#5917=FACE_OUTER_BOUND('',#8846,.T.);
#5918=FACE_OUTER_BOUND('',#8847,.T.);
#5919=FACE_OUTER_BOUND('',#8848,.T.);
#5920=FACE_OUTER_BOUND('',#8849,.T.);
#5921=FACE_OUTER_BOUND('',#8850,.T.);
#5922=FACE_OUTER_BOUND('',#8851,.T.);
#5923=FACE_OUTER_BOUND('',#8852,.T.);
#5924=FACE_OUTER_BOUND('',#8853,.T.);
#5925=FACE_OUTER_BOUND('',#8854,.T.);
#5926=FACE_OUTER_BOUND('',#8855,.T.);
#5927=FACE_OUTER_BOUND('',#8856,.T.);
#5928=FACE_OUTER_BOUND('',#8857,.T.);
#5929=FACE_OUTER_BOUND('',#8858,.T.);
#5930=FACE_OUTER_BOUND('',#8859,.T.);
#5931=FACE_OUTER_BOUND('',#8860,.T.);
#5932=FACE_OUTER_BOUND('',#8861,.T.);
#5933=FACE_OUTER_BOUND('',#8862,.T.);
#5934=FACE_OUTER_BOUND('',#8863,.T.);
#5935=FACE_OUTER_BOUND('',#8864,.T.);
#5936=FACE_OUTER_BOUND('',#8865,.T.);
#5937=FACE_OUTER_BOUND('',#8866,.T.);
#5938=FACE_OUTER_BOUND('',#8867,.T.);
#5939=FACE_OUTER_BOUND('',#8868,.T.);
#5940=FACE_OUTER_BOUND('',#8869,.T.);
#5941=FACE_OUTER_BOUND('',#8870,.T.);
#5942=FACE_OUTER_BOUND('',#8871,.T.);
#5943=FACE_OUTER_BOUND('',#8872,.T.);
#5944=FACE_OUTER_BOUND('',#8873,.T.);
#5945=FACE_OUTER_BOUND('',#8874,.T.);
#5946=FACE_OUTER_BOUND('',#8875,.T.);
#5947=FACE_OUTER_BOUND('',#8876,.T.);
#5948=FACE_OUTER_BOUND('',#8877,.T.);
#5949=FACE_OUTER_BOUND('',#8878,.T.);
#5950=FACE_OUTER_BOUND('',#8879,.T.);
#5951=FACE_OUTER_BOUND('',#8880,.T.);
#5952=FACE_OUTER_BOUND('',#8881,.T.);
#5953=FACE_OUTER_BOUND('',#8882,.T.);
#5954=FACE_OUTER_BOUND('',#8883,.T.);
#5955=FACE_OUTER_BOUND('',#8884,.T.);
#5956=FACE_OUTER_BOUND('',#8885,.T.);
#5957=FACE_OUTER_BOUND('',#8886,.T.);
#5958=FACE_OUTER_BOUND('',#8887,.T.);
#5959=FACE_OUTER_BOUND('',#8888,.T.);
#5960=FACE_OUTER_BOUND('',#8889,.T.);
#5961=FACE_OUTER_BOUND('',#8890,.T.);
#5962=FACE_OUTER_BOUND('',#8891,.T.);
#5963=FACE_OUTER_BOUND('',#8892,.T.);
#5964=FACE_OUTER_BOUND('',#8893,.T.);
#5965=FACE_OUTER_BOUND('',#8894,.T.);
#5966=FACE_OUTER_BOUND('',#8895,.T.);
#5967=FACE_OUTER_BOUND('',#8896,.T.);
#5968=FACE_OUTER_BOUND('',#8897,.T.);
#5969=FACE_OUTER_BOUND('',#8898,.T.);
#5970=FACE_OUTER_BOUND('',#8899,.T.);
#5971=FACE_OUTER_BOUND('',#8900,.T.);
#5972=FACE_OUTER_BOUND('',#8901,.T.);
#5973=FACE_OUTER_BOUND('',#8902,.T.);
#5974=FACE_OUTER_BOUND('',#8903,.T.);
#5975=FACE_OUTER_BOUND('',#8904,.T.);
#5976=FACE_OUTER_BOUND('',#8905,.T.);
#5977=FACE_OUTER_BOUND('',#8906,.T.);
#5978=FACE_OUTER_BOUND('',#8907,.T.);
#5979=FACE_OUTER_BOUND('',#8908,.T.);
#5980=FACE_OUTER_BOUND('',#8909,.T.);
#5981=FACE_OUTER_BOUND('',#8910,.T.);
#5982=FACE_OUTER_BOUND('',#8911,.T.);
#5983=FACE_OUTER_BOUND('',#8912,.T.);
#5984=FACE_OUTER_BOUND('',#8913,.T.);
#5985=FACE_OUTER_BOUND('',#8914,.T.);
#5986=FACE_OUTER_BOUND('',#8915,.T.);
#5987=FACE_OUTER_BOUND('',#8916,.T.);
#5988=FACE_OUTER_BOUND('',#8917,.T.);
#5989=FACE_OUTER_BOUND('',#8918,.T.);
#5990=FACE_OUTER_BOUND('',#8919,.T.);
#5991=FACE_OUTER_BOUND('',#8920,.T.);
#5992=FACE_OUTER_BOUND('',#8921,.T.);
#5993=FACE_OUTER_BOUND('',#8922,.T.);
#5994=FACE_OUTER_BOUND('',#8923,.T.);
#5995=FACE_OUTER_BOUND('',#8924,.T.);
#5996=FACE_OUTER_BOUND('',#8925,.T.);
#5997=FACE_OUTER_BOUND('',#8926,.T.);
#5998=FACE_OUTER_BOUND('',#8927,.T.);
#5999=FACE_OUTER_BOUND('',#8928,.T.);
#6000=FACE_OUTER_BOUND('',#8929,.T.);
#6001=FACE_OUTER_BOUND('',#8930,.T.);
#6002=FACE_OUTER_BOUND('',#8931,.T.);
#6003=FACE_OUTER_BOUND('',#8932,.T.);
#6004=FACE_OUTER_BOUND('',#8933,.T.);
#6005=FACE_OUTER_BOUND('',#8934,.T.);
#6006=FACE_OUTER_BOUND('',#8935,.T.);
#6007=FACE_OUTER_BOUND('',#8936,.T.);
#6008=FACE_OUTER_BOUND('',#8937,.T.);
#6009=FACE_OUTER_BOUND('',#8938,.T.);
#6010=FACE_OUTER_BOUND('',#8939,.T.);
#6011=FACE_OUTER_BOUND('',#8940,.T.);
#6012=FACE_OUTER_BOUND('',#8941,.T.);
#6013=FACE_OUTER_BOUND('',#8942,.T.);
#6014=FACE_OUTER_BOUND('',#8943,.T.);
#6015=FACE_OUTER_BOUND('',#8944,.T.);
#6016=FACE_OUTER_BOUND('',#8945,.T.);
#6017=FACE_OUTER_BOUND('',#8946,.T.);
#6018=FACE_OUTER_BOUND('',#8947,.T.);
#6019=FACE_OUTER_BOUND('',#8948,.T.);
#6020=FACE_OUTER_BOUND('',#8949,.T.);
#6021=FACE_OUTER_BOUND('',#8950,.T.);
#6022=FACE_OUTER_BOUND('',#8951,.T.);
#6023=FACE_OUTER_BOUND('',#8952,.T.);
#6024=FACE_OUTER_BOUND('',#8953,.T.);
#6025=FACE_OUTER_BOUND('',#8954,.T.);
#6026=FACE_OUTER_BOUND('',#8955,.T.);
#6027=FACE_OUTER_BOUND('',#8956,.T.);
#6028=FACE_OUTER_BOUND('',#8957,.T.);
#6029=FACE_OUTER_BOUND('',#8958,.T.);
#6030=FACE_OUTER_BOUND('',#8959,.T.);
#6031=FACE_OUTER_BOUND('',#8960,.T.);
#6032=FACE_OUTER_BOUND('',#8961,.T.);
#6033=FACE_OUTER_BOUND('',#8962,.T.);
#6034=FACE_OUTER_BOUND('',#8963,.T.);
#6035=FACE_OUTER_BOUND('',#8964,.T.);
#6036=FACE_OUTER_BOUND('',#8965,.T.);
#6037=FACE_OUTER_BOUND('',#8966,.T.);
#6038=FACE_OUTER_BOUND('',#8967,.T.);
#6039=FACE_OUTER_BOUND('',#8968,.T.);
#6040=FACE_OUTER_BOUND('',#8969,.T.);
#6041=FACE_OUTER_BOUND('',#8970,.T.);
#6042=FACE_OUTER_BOUND('',#8971,.T.);
#6043=FACE_OUTER_BOUND('',#8972,.T.);
#6044=FACE_OUTER_BOUND('',#8973,.T.);
#6045=FACE_OUTER_BOUND('',#8974,.T.);
#6046=FACE_OUTER_BOUND('',#8975,.T.);
#6047=FACE_OUTER_BOUND('',#8976,.T.);
#6048=FACE_OUTER_BOUND('',#8977,.T.);
#6049=FACE_OUTER_BOUND('',#8978,.T.);
#6050=FACE_OUTER_BOUND('',#8979,.T.);
#6051=FACE_OUTER_BOUND('',#8980,.T.);
#6052=FACE_OUTER_BOUND('',#8981,.T.);
#6053=FACE_OUTER_BOUND('',#8982,.T.);
#6054=FACE_OUTER_BOUND('',#8983,.T.);
#6055=FACE_OUTER_BOUND('',#8984,.T.);
#6056=FACE_OUTER_BOUND('',#8985,.T.);
#6057=FACE_OUTER_BOUND('',#8986,.T.);
#6058=FACE_OUTER_BOUND('',#8987,.T.);
#6059=FACE_OUTER_BOUND('',#8988,.T.);
#6060=FACE_OUTER_BOUND('',#8989,.T.);
#6061=FACE_OUTER_BOUND('',#8990,.T.);
#6062=FACE_OUTER_BOUND('',#8991,.T.);
#6063=FACE_OUTER_BOUND('',#8992,.T.);
#6064=FACE_OUTER_BOUND('',#8993,.T.);
#6065=FACE_OUTER_BOUND('',#8994,.T.);
#6066=FACE_OUTER_BOUND('',#8995,.T.);
#6067=FACE_OUTER_BOUND('',#8996,.T.);
#6068=FACE_OUTER_BOUND('',#8997,.T.);
#6069=FACE_OUTER_BOUND('',#8998,.T.);
#6070=FACE_OUTER_BOUND('',#8999,.T.);
#6071=FACE_OUTER_BOUND('',#9000,.T.);
#6072=FACE_OUTER_BOUND('',#9001,.T.);
#6073=FACE_OUTER_BOUND('',#9002,.T.);
#6074=FACE_OUTER_BOUND('',#9003,.T.);
#6075=FACE_OUTER_BOUND('',#9004,.T.);
#6076=FACE_OUTER_BOUND('',#9005,.T.);
#6077=FACE_OUTER_BOUND('',#9006,.T.);
#6078=FACE_OUTER_BOUND('',#9007,.T.);
#6079=FACE_OUTER_BOUND('',#9008,.T.);
#6080=FACE_OUTER_BOUND('',#9009,.T.);
#6081=FACE_OUTER_BOUND('',#9010,.T.);
#6082=FACE_OUTER_BOUND('',#9011,.T.);
#6083=FACE_OUTER_BOUND('',#9012,.T.);
#6084=FACE_OUTER_BOUND('',#9013,.T.);
#6085=FACE_OUTER_BOUND('',#9014,.T.);
#6086=FACE_OUTER_BOUND('',#9015,.T.);
#6087=FACE_OUTER_BOUND('',#9016,.T.);
#6088=FACE_OUTER_BOUND('',#9017,.T.);
#6089=FACE_OUTER_BOUND('',#9018,.T.);
#6090=FACE_OUTER_BOUND('',#9019,.T.);
#6091=FACE_OUTER_BOUND('',#9020,.T.);
#6092=FACE_OUTER_BOUND('',#9021,.T.);
#6093=FACE_OUTER_BOUND('',#9022,.T.);
#6094=FACE_OUTER_BOUND('',#9023,.T.);
#6095=FACE_OUTER_BOUND('',#9024,.T.);
#6096=FACE_OUTER_BOUND('',#9025,.T.);
#6097=FACE_OUTER_BOUND('',#9026,.T.);
#6098=FACE_OUTER_BOUND('',#9027,.T.);
#6099=FACE_OUTER_BOUND('',#9028,.T.);
#6100=FACE_OUTER_BOUND('',#9029,.T.);
#6101=FACE_OUTER_BOUND('',#9030,.T.);
#6102=FACE_OUTER_BOUND('',#9031,.T.);
#6103=FACE_OUTER_BOUND('',#9032,.T.);
#6104=FACE_OUTER_BOUND('',#9033,.T.);
#6105=FACE_OUTER_BOUND('',#9034,.T.);
#6106=FACE_OUTER_BOUND('',#9035,.T.);
#6107=FACE_OUTER_BOUND('',#9036,.T.);
#6108=FACE_OUTER_BOUND('',#9037,.T.);
#6109=FACE_OUTER_BOUND('',#9038,.T.);
#6110=FACE_OUTER_BOUND('',#9039,.T.);
#6111=FACE_OUTER_BOUND('',#9040,.T.);
#6112=FACE_OUTER_BOUND('',#9041,.T.);
#6113=FACE_OUTER_BOUND('',#9042,.T.);
#6114=FACE_OUTER_BOUND('',#9043,.T.);
#6115=FACE_OUTER_BOUND('',#9044,.T.);
#6116=FACE_OUTER_BOUND('',#9045,.T.);
#6117=FACE_OUTER_BOUND('',#9046,.T.);
#6118=FACE_OUTER_BOUND('',#9047,.T.);
#6119=FACE_OUTER_BOUND('',#9048,.T.);
#6120=FACE_OUTER_BOUND('',#9049,.T.);
#6121=FACE_OUTER_BOUND('',#9050,.T.);
#6122=FACE_OUTER_BOUND('',#9051,.T.);
#6123=FACE_OUTER_BOUND('',#9052,.T.);
#6124=FACE_OUTER_BOUND('',#9053,.T.);
#6125=FACE_OUTER_BOUND('',#9054,.T.);
#6126=FACE_OUTER_BOUND('',#9055,.T.);
#6127=FACE_OUTER_BOUND('',#9056,.T.);
#6128=FACE_OUTER_BOUND('',#9057,.T.);
#6129=FACE_OUTER_BOUND('',#9058,.T.);
#6130=FACE_OUTER_BOUND('',#9059,.T.);
#6131=FACE_OUTER_BOUND('',#9060,.T.);
#6132=FACE_OUTER_BOUND('',#9061,.T.);
#6133=FACE_OUTER_BOUND('',#9062,.T.);
#6134=FACE_OUTER_BOUND('',#9063,.T.);
#6135=FACE_OUTER_BOUND('',#9064,.T.);
#6136=FACE_OUTER_BOUND('',#9065,.T.);
#6137=FACE_OUTER_BOUND('',#9066,.T.);
#6138=FACE_OUTER_BOUND('',#9067,.T.);
#6139=FACE_OUTER_BOUND('',#9068,.T.);
#6140=FACE_OUTER_BOUND('',#9069,.T.);
#6141=FACE_OUTER_BOUND('',#9070,.T.);
#6142=FACE_OUTER_BOUND('',#9071,.T.);
#6143=FACE_OUTER_BOUND('',#9072,.T.);
#6144=FACE_OUTER_BOUND('',#9073,.T.);
#6145=FACE_OUTER_BOUND('',#9074,.T.);
#6146=FACE_OUTER_BOUND('',#9075,.T.);
#6147=FACE_OUTER_BOUND('',#9076,.T.);
#6148=FACE_OUTER_BOUND('',#9077,.T.);
#6149=FACE_OUTER_BOUND('',#9078,.T.);
#6150=FACE_OUTER_BOUND('',#9079,.T.);
#6151=FACE_OUTER_BOUND('',#9080,.T.);
#6152=FACE_OUTER_BOUND('',#9081,.T.);
#6153=FACE_OUTER_BOUND('',#9082,.T.);
#6154=FACE_OUTER_BOUND('',#9083,.T.);
#6155=FACE_OUTER_BOUND('',#9084,.T.);
#6156=FACE_OUTER_BOUND('',#9085,.T.);
#6157=FACE_OUTER_BOUND('',#9086,.T.);
#6158=FACE_OUTER_BOUND('',#9087,.T.);
#6159=FACE_OUTER_BOUND('',#9088,.T.);
#6160=FACE_OUTER_BOUND('',#9089,.T.);
#6161=FACE_OUTER_BOUND('',#9090,.T.);
#6162=FACE_OUTER_BOUND('',#9091,.T.);
#6163=FACE_OUTER_BOUND('',#9092,.T.);
#6164=FACE_OUTER_BOUND('',#9093,.T.);
#6165=FACE_OUTER_BOUND('',#9094,.T.);
#6166=FACE_OUTER_BOUND('',#9095,.T.);
#6167=FACE_OUTER_BOUND('',#9096,.T.);
#6168=FACE_OUTER_BOUND('',#9097,.T.);
#6169=FACE_OUTER_BOUND('',#9098,.T.);
#6170=FACE_OUTER_BOUND('',#9099,.T.);
#6171=FACE_OUTER_BOUND('',#9100,.T.);
#6172=FACE_OUTER_BOUND('',#9101,.T.);
#6173=FACE_OUTER_BOUND('',#9102,.T.);
#6174=FACE_OUTER_BOUND('',#9103,.T.);
#6175=FACE_OUTER_BOUND('',#9104,.T.);
#6176=FACE_OUTER_BOUND('',#9105,.T.);
#6177=FACE_OUTER_BOUND('',#9106,.T.);
#6178=FACE_OUTER_BOUND('',#9107,.T.);
#6179=FACE_OUTER_BOUND('',#9108,.T.);
#6180=FACE_OUTER_BOUND('',#9109,.T.);
#6181=FACE_OUTER_BOUND('',#9110,.T.);
#6182=FACE_OUTER_BOUND('',#9111,.T.);
#6183=FACE_OUTER_BOUND('',#9112,.T.);
#6184=FACE_OUTER_BOUND('',#9113,.T.);
#6185=FACE_OUTER_BOUND('',#9114,.T.);
#6186=FACE_OUTER_BOUND('',#9115,.T.);
#6187=FACE_OUTER_BOUND('',#9116,.T.);
#6188=FACE_OUTER_BOUND('',#9117,.T.);
#6189=FACE_OUTER_BOUND('',#9118,.T.);
#6190=FACE_OUTER_BOUND('',#9119,.T.);
#6191=FACE_OUTER_BOUND('',#9120,.T.);
#6192=FACE_OUTER_BOUND('',#9121,.T.);
#6193=FACE_OUTER_BOUND('',#9122,.T.);
#6194=FACE_OUTER_BOUND('',#9123,.T.);
#6195=FACE_OUTER_BOUND('',#9124,.T.);
#6196=FACE_OUTER_BOUND('',#9125,.T.);
#6197=FACE_OUTER_BOUND('',#9126,.T.);
#6198=FACE_OUTER_BOUND('',#9127,.T.);
#6199=FACE_OUTER_BOUND('',#9128,.T.);
#6200=FACE_OUTER_BOUND('',#9129,.T.);
#6201=FACE_OUTER_BOUND('',#9130,.T.);
#6202=FACE_OUTER_BOUND('',#9131,.T.);
#6203=FACE_OUTER_BOUND('',#9132,.T.);
#6204=FACE_OUTER_BOUND('',#9133,.T.);
#6205=FACE_OUTER_BOUND('',#9134,.T.);
#6206=FACE_OUTER_BOUND('',#9135,.T.);
#6207=FACE_OUTER_BOUND('',#9136,.T.);
#6208=FACE_OUTER_BOUND('',#9137,.T.);
#6209=FACE_OUTER_BOUND('',#9138,.T.);
#6210=FACE_OUTER_BOUND('',#9139,.T.);
#6211=FACE_OUTER_BOUND('',#9140,.T.);
#6212=FACE_OUTER_BOUND('',#9141,.T.);
#6213=FACE_OUTER_BOUND('',#9142,.T.);
#6214=FACE_OUTER_BOUND('',#9143,.T.);
#6215=FACE_OUTER_BOUND('',#9144,.T.);
#6216=FACE_OUTER_BOUND('',#9145,.T.);
#6217=FACE_OUTER_BOUND('',#9146,.T.);
#6218=FACE_OUTER_BOUND('',#9147,.T.);
#6219=FACE_OUTER_BOUND('',#9148,.T.);
#6220=FACE_OUTER_BOUND('',#9149,.T.);
#6221=FACE_OUTER_BOUND('',#9150,.T.);
#6222=FACE_OUTER_BOUND('',#9151,.T.);
#6223=FACE_OUTER_BOUND('',#9152,.T.);
#6224=FACE_OUTER_BOUND('',#9153,.T.);
#6225=FACE_OUTER_BOUND('',#9154,.T.);
#6226=FACE_OUTER_BOUND('',#9155,.T.);
#6227=FACE_OUTER_BOUND('',#9156,.T.);
#6228=FACE_OUTER_BOUND('',#9157,.T.);
#6229=FACE_OUTER_BOUND('',#9158,.T.);
#6230=FACE_OUTER_BOUND('',#9159,.T.);
#6231=FACE_OUTER_BOUND('',#9160,.T.);
#6232=FACE_OUTER_BOUND('',#9161,.T.);
#6233=FACE_OUTER_BOUND('',#9162,.T.);
#6234=FACE_OUTER_BOUND('',#9163,.T.);
#6235=FACE_OUTER_BOUND('',#9164,.T.);
#6236=FACE_OUTER_BOUND('',#9165,.T.);
#6237=FACE_OUTER_BOUND('',#9166,.T.);
#6238=FACE_OUTER_BOUND('',#9167,.T.);
#6239=FACE_OUTER_BOUND('',#9168,.T.);
#6240=FACE_OUTER_BOUND('',#9169,.T.);
#6241=FACE_OUTER_BOUND('',#9170,.T.);
#6242=FACE_OUTER_BOUND('',#9171,.T.);
#6243=FACE_OUTER_BOUND('',#9172,.T.);
#6244=FACE_OUTER_BOUND('',#9173,.T.);
#6245=FACE_OUTER_BOUND('',#9174,.T.);
#6246=FACE_OUTER_BOUND('',#9175,.T.);
#6247=FACE_OUTER_BOUND('',#9176,.T.);
#6248=FACE_OUTER_BOUND('',#9177,.T.);
#6249=FACE_OUTER_BOUND('',#9178,.T.);
#6250=FACE_OUTER_BOUND('',#9179,.T.);
#6251=FACE_OUTER_BOUND('',#9180,.T.);
#6252=FACE_OUTER_BOUND('',#9181,.T.);
#6253=FACE_OUTER_BOUND('',#9182,.T.);
#6254=FACE_OUTER_BOUND('',#9183,.T.);
#6255=FACE_OUTER_BOUND('',#9184,.T.);
#6256=FACE_OUTER_BOUND('',#9185,.T.);
#6257=FACE_OUTER_BOUND('',#9186,.T.);
#6258=FACE_OUTER_BOUND('',#9187,.T.);
#6259=FACE_OUTER_BOUND('',#9188,.T.);
#6260=FACE_OUTER_BOUND('',#9189,.T.);
#6261=FACE_OUTER_BOUND('',#9190,.T.);
#6262=FACE_OUTER_BOUND('',#9191,.T.);
#6263=FACE_OUTER_BOUND('',#9192,.T.);
#6264=FACE_OUTER_BOUND('',#9193,.T.);
#6265=FACE_OUTER_BOUND('',#9194,.T.);
#6266=FACE_OUTER_BOUND('',#9195,.T.);
#6267=FACE_OUTER_BOUND('',#9196,.T.);
#6268=FACE_OUTER_BOUND('',#9197,.T.);
#6269=FACE_OUTER_BOUND('',#9198,.T.);
#6270=FACE_OUTER_BOUND('',#9199,.T.);
#6271=FACE_OUTER_BOUND('',#9200,.T.);
#6272=FACE_OUTER_BOUND('',#9201,.T.);
#6273=FACE_OUTER_BOUND('',#9202,.T.);
#6274=FACE_OUTER_BOUND('',#9203,.T.);
#6275=FACE_OUTER_BOUND('',#9204,.T.);
#6276=FACE_OUTER_BOUND('',#9205,.T.);
#6277=FACE_OUTER_BOUND('',#9206,.T.);
#6278=FACE_OUTER_BOUND('',#9207,.T.);
#6279=FACE_OUTER_BOUND('',#9208,.T.);
#6280=FACE_OUTER_BOUND('',#9209,.T.);
#6281=FACE_OUTER_BOUND('',#9210,.T.);
#6282=FACE_OUTER_BOUND('',#9211,.T.);
#6283=FACE_OUTER_BOUND('',#9212,.T.);
#6284=FACE_OUTER_BOUND('',#9213,.T.);
#6285=FACE_OUTER_BOUND('',#9214,.T.);
#6286=FACE_OUTER_BOUND('',#9215,.T.);
#6287=FACE_OUTER_BOUND('',#9216,.T.);
#6288=FACE_OUTER_BOUND('',#9217,.T.);
#6289=FACE_OUTER_BOUND('',#9218,.T.);
#6290=FACE_OUTER_BOUND('',#9219,.T.);
#6291=FACE_OUTER_BOUND('',#9220,.T.);
#6292=FACE_OUTER_BOUND('',#9221,.T.);
#6293=FACE_OUTER_BOUND('',#9222,.T.);
#6294=FACE_OUTER_BOUND('',#9223,.T.);
#6295=FACE_OUTER_BOUND('',#9224,.T.);
#6296=FACE_OUTER_BOUND('',#9225,.T.);
#6297=FACE_OUTER_BOUND('',#9226,.T.);
#6298=FACE_OUTER_BOUND('',#9227,.T.);
#6299=FACE_OUTER_BOUND('',#9228,.T.);
#6300=FACE_OUTER_BOUND('',#9229,.T.);
#6301=FACE_OUTER_BOUND('',#9230,.T.);
#6302=FACE_OUTER_BOUND('',#9231,.T.);
#6303=FACE_OUTER_BOUND('',#9232,.T.);
#6304=FACE_OUTER_BOUND('',#9233,.T.);
#6305=FACE_OUTER_BOUND('',#9234,.T.);
#6306=FACE_OUTER_BOUND('',#9235,.T.);
#6307=FACE_OUTER_BOUND('',#9236,.T.);
#6308=FACE_OUTER_BOUND('',#9237,.T.);
#6309=FACE_OUTER_BOUND('',#9238,.T.);
#6310=FACE_OUTER_BOUND('',#9239,.T.);
#6311=FACE_OUTER_BOUND('',#9240,.T.);
#6312=FACE_OUTER_BOUND('',#9241,.T.);
#6313=FACE_OUTER_BOUND('',#9242,.T.);
#6314=FACE_OUTER_BOUND('',#9243,.T.);
#6315=FACE_OUTER_BOUND('',#9244,.T.);
#6316=FACE_OUTER_BOUND('',#9245,.T.);
#6317=FACE_OUTER_BOUND('',#9246,.T.);
#6318=FACE_OUTER_BOUND('',#9247,.T.);
#6319=FACE_OUTER_BOUND('',#9248,.T.);
#6320=FACE_OUTER_BOUND('',#9249,.T.);
#6321=FACE_OUTER_BOUND('',#9250,.T.);
#6322=FACE_OUTER_BOUND('',#9251,.T.);
#6323=FACE_OUTER_BOUND('',#9252,.T.);
#6324=FACE_OUTER_BOUND('',#9253,.T.);
#6325=FACE_OUTER_BOUND('',#9254,.T.);
#6326=FACE_OUTER_BOUND('',#9255,.T.);
#6327=FACE_OUTER_BOUND('',#9256,.T.);
#6328=FACE_OUTER_BOUND('',#9257,.T.);
#6329=FACE_OUTER_BOUND('',#9258,.T.);
#6330=FACE_OUTER_BOUND('',#9259,.T.);
#6331=FACE_OUTER_BOUND('',#9260,.T.);
#6332=FACE_OUTER_BOUND('',#9261,.T.);
#6333=FACE_OUTER_BOUND('',#9262,.T.);
#6334=FACE_OUTER_BOUND('',#9263,.T.);
#6335=FACE_OUTER_BOUND('',#9264,.T.);
#6336=FACE_OUTER_BOUND('',#9265,.T.);
#6337=FACE_OUTER_BOUND('',#9266,.T.);
#6338=FACE_OUTER_BOUND('',#9267,.T.);
#6339=FACE_OUTER_BOUND('',#9268,.T.);
#6340=FACE_OUTER_BOUND('',#9269,.T.);
#6341=FACE_OUTER_BOUND('',#9270,.T.);
#6342=FACE_OUTER_BOUND('',#9271,.T.);
#6343=FACE_OUTER_BOUND('',#9272,.T.);
#6344=FACE_OUTER_BOUND('',#9273,.T.);
#6345=FACE_OUTER_BOUND('',#9274,.T.);
#6346=FACE_OUTER_BOUND('',#9275,.T.);
#6347=FACE_OUTER_BOUND('',#9276,.T.);
#6348=FACE_OUTER_BOUND('',#9277,.T.);
#6349=FACE_OUTER_BOUND('',#9278,.T.);
#6350=FACE_OUTER_BOUND('',#9279,.T.);
#6351=FACE_OUTER_BOUND('',#9280,.T.);
#6352=FACE_OUTER_BOUND('',#9281,.T.);
#6353=FACE_OUTER_BOUND('',#9282,.T.);
#6354=FACE_OUTER_BOUND('',#9283,.T.);
#6355=FACE_OUTER_BOUND('',#9284,.T.);
#6356=FACE_OUTER_BOUND('',#9285,.T.);
#6357=FACE_OUTER_BOUND('',#9286,.T.);
#6358=FACE_OUTER_BOUND('',#9287,.T.);
#6359=FACE_OUTER_BOUND('',#9288,.T.);
#6360=FACE_OUTER_BOUND('',#9289,.T.);
#6361=FACE_OUTER_BOUND('',#9290,.T.);
#6362=FACE_OUTER_BOUND('',#9291,.T.);
#6363=FACE_OUTER_BOUND('',#9292,.T.);
#6364=FACE_OUTER_BOUND('',#9293,.T.);
#6365=FACE_OUTER_BOUND('',#9294,.T.);
#6366=FACE_OUTER_BOUND('',#9295,.T.);
#6367=FACE_OUTER_BOUND('',#9296,.T.);
#6368=FACE_OUTER_BOUND('',#9297,.T.);
#6369=FACE_OUTER_BOUND('',#9298,.T.);
#6370=FACE_OUTER_BOUND('',#9299,.T.);
#6371=FACE_OUTER_BOUND('',#9300,.T.);
#6372=FACE_OUTER_BOUND('',#9301,.T.);
#6373=FACE_OUTER_BOUND('',#9302,.T.);
#6374=FACE_OUTER_BOUND('',#9303,.T.);
#6375=FACE_OUTER_BOUND('',#9304,.T.);
#6376=FACE_OUTER_BOUND('',#9305,.T.);
#6377=FACE_OUTER_BOUND('',#9306,.T.);
#6378=FACE_OUTER_BOUND('',#9307,.T.);
#6379=FACE_OUTER_BOUND('',#9308,.T.);
#6380=FACE_OUTER_BOUND('',#9309,.T.);
#6381=FACE_OUTER_BOUND('',#9310,.T.);
#6382=FACE_OUTER_BOUND('',#9311,.T.);
#6383=FACE_OUTER_BOUND('',#9312,.T.);
#6384=FACE_OUTER_BOUND('',#9313,.T.);
#6385=FACE_OUTER_BOUND('',#9314,.T.);
#6386=FACE_OUTER_BOUND('',#9315,.T.);
#6387=FACE_OUTER_BOUND('',#9316,.T.);
#6388=FACE_OUTER_BOUND('',#9317,.T.);
#6389=FACE_OUTER_BOUND('',#9318,.T.);
#6390=FACE_OUTER_BOUND('',#9319,.T.);
#6391=FACE_OUTER_BOUND('',#9320,.T.);
#6392=FACE_OUTER_BOUND('',#9321,.T.);
#6393=FACE_OUTER_BOUND('',#9322,.T.);
#6394=FACE_OUTER_BOUND('',#9323,.T.);
#6395=FACE_OUTER_BOUND('',#9324,.T.);
#6396=FACE_OUTER_BOUND('',#9325,.T.);
#6397=FACE_OUTER_BOUND('',#9326,.T.);
#6398=FACE_OUTER_BOUND('',#9327,.T.);
#6721=EDGE_LOOP('',(#28264,#28265,#28266,#28267));
#6722=EDGE_LOOP('',(#28268,#28269,#28270,#28271,#28272,#28273,#28274,#28275,
#28276,#28277,#28278,#28279,#28280,#28281,#28282,#28283,#28284,#28285,#28286,
#28287,#28288,#28289,#28290,#28291,#28292,#28293,#28294,#28295,#28296,#28297,
#28298,#28299,#28300,#28301,#28302,#28303,#28304,#28305,#28306,#28307,#28308,
#28309,#28310,#28311,#28312,#28313,#28314,#28315,#28316,#28317,#28318,#28319,
#28320,#28321,#28322,#28323,#28324,#28325,#28326,#28327,#28328,#28329,#28330,
#28331,#28332,#28333,#28334,#28335,#28336,#28337,#28338,#28339,#28340,#28341,
#28342,#28343,#28344,#28345,#28346,#28347,#28348,#28349,#28350,#28351,#28352,
#28353,#28354,#28355,#28356,#28357,#28358,#28359,#28360,#28361,#28362,#28363,
#28364,#28365,#28366,#28367,#28368,#28369,#28370,#28371,#28372,#28373,#28374,
#28375,#28376,#28377,#28378,#28379,#28380,#28381,#28382,#28383,#28384,#28385,
#28386,#28387,#28388,#28389,#28390,#28391,#28392,#28393,#28394,#28395,#28396,
#28397,#28398,#28399,#28400,#28401,#28402,#28403,#28404,#28405,#28406,#28407,
#28408,#28409,#28410,#28411,#28412,#28413,#28414,#28415,#28416,#28417,#28418,
#28419,#28420,#28421,#28422,#28423,#28424,#28425,#28426,#28427,#28428,#28429,
#28430,#28431,#28432,#28433,#28434,#28435,#28436,#28437,#28438,#28439,#28440,
#28441,#28442,#28443,#28444,#28445,#28446,#28447,#28448,#28449,#28450,#28451,
#28452,#28453,#28454,#28455,#28456,#28457,#28458,#28459,#28460,#28461,#28462,
#28463,#28464,#28465,#28466,#28467,#28468,#28469,#28470,#28471));
#6723=EDGE_LOOP('',(#28472,#28473,#28474,#28475,#28476,#28477,#28478,#28479,
#28480,#28481,#28482,#28483,#28484,#28485,#28486,#28487,#28488,#28489,#28490,
#28491,#28492,#28493,#28494,#28495,#28496,#28497,#28498,#28499,#28500,#28501,
#28502,#28503,#28504,#28505,#28506,#28507,#28508,#28509,#28510,#28511,#28512,
#28513,#28514,#28515,#28516,#28517,#28518,#28519,#28520,#28521,#28522,#28523,
#28524,#28525,#28526,#28527,#28528,#28529,#28530,#28531,#28532,#28533,#28534,
#28535,#28536,#28537,#28538,#28539,#28540,#28541,#28542,#28543,#28544,#28545,
#28546,#28547,#28548,#28549,#28550,#28551,#28552,#28553,#28554,#28555,#28556,
#28557,#28558,#28559,#28560,#28561,#28562,#28563,#28564,#28565,#28566,#28567,
#28568,#28569,#28570,#28571,#28572,#28573,#28574,#28575,#28576,#28577,#28578,
#28579,#28580,#28581,#28582,#28583,#28584,#28585,#28586,#28587,#28588,#28589,
#28590,#28591,#28592,#28593,#28594,#28595,#28596,#28597,#28598,#28599,#28600,
#28601,#28602,#28603,#28604,#28605,#28606,#28607,#28608,#28609,#28610,#28611,
#28612,#28613,#28614,#28615,#28616,#28617,#28618,#28619,#28620,#28621,#28622,
#28623,#28624,#28625,#28626,#28627,#28628,#28629,#28630,#28631,#28632,#28633,
#28634,#28635,#28636,#28637,#28638,#28639,#28640,#28641,#28642,#28643,#28644,
#28645,#28646,#28647,#28648,#28649,#28650,#28651,#28652,#28653,#28654,#28655,
#28656,#28657,#28658,#28659,#28660,#28661,#28662,#28663,#28664,#28665,#28666,
#28667,#28668,#28669,#28670,#28671,#28672,#28673,#28674,#28675,#28676,#28677,
#28678,#28679,#28680,#28681,#28682,#28683,#28684,#28685,#28686,#28687,#28688,
#28689,#28690,#28691,#28692,#28693,#28694,#28695,#28696,#28697,#28698,#28699,
#28700,#28701,#28702,#28703,#28704,#28705,#28706,#28707,#28708,#28709,#28710,
#28711,#28712,#28713,#28714,#28715,#28716,#28717,#28718,#28719,#28720,#28721,
#28722,#28723,#28724,#28725,#28726,#28727,#28728,#28729,#28730,#28731,#28732,
#28733,#28734,#28735,#28736,#28737,#28738,#28739,#28740,#28741,#28742,#28743,
#28744,#28745,#28746,#28747,#28748,#28749,#28750,#28751,#28752,#28753,#28754,
#28755,#28756,#28757,#28758,#28759,#28760,#28761,#28762,#28763,#28764,#28765,
#28766,#28767,#28768,#28769,#28770,#28771,#28772,#28773,#28774,#28775));
#6724=EDGE_LOOP('',(#28776,#28777,#28778,#28779,#28780,#28781));
#6725=EDGE_LOOP('',(#28782,#28783,#28784,#28785));
#6726=EDGE_LOOP('',(#28786,#28787,#28788,#28789,#28790,#28791));
#6727=EDGE_LOOP('',(#28792,#28793,#28794,#28795,#28796,#28797));
#6728=EDGE_LOOP('',(#28798,#28799,#28800,#28801));
#6729=EDGE_LOOP('',(#28802,#28803,#28804,#28805));
#6730=EDGE_LOOP('',(#28806,#28807,#28808,#28809));
#6731=EDGE_LOOP('',(#28810,#28811,#28812,#28813));
#6732=EDGE_LOOP('',(#28814,#28815,#28816));
#6733=EDGE_LOOP('',(#28817,#28818,#28819,#28820));
#6734=EDGE_LOOP('',(#28821,#28822,#28823,#28824));
#6735=EDGE_LOOP('',(#28825,#28826,#28827,#28828,#28829,#28830));
#6736=EDGE_LOOP('',(#28831,#28832,#28833,#28834,#28835,#28836));
#6737=EDGE_LOOP('',(#28837,#28838,#28839,#28840));
#6738=EDGE_LOOP('',(#28841,#28842,#28843,#28844));
#6739=EDGE_LOOP('',(#28845,#28846,#28847,#28848));
#6740=EDGE_LOOP('',(#28849,#28850,#28851,#28852));
#6741=EDGE_LOOP('',(#28853,#28854,#28855,#28856));
#6742=EDGE_LOOP('',(#28857,#28858,#28859,#28860));
#6743=EDGE_LOOP('',(#28861,#28862,#28863,#28864,#28865,#28866));
#6744=EDGE_LOOP('',(#28867,#28868,#28869,#28870,#28871,#28872));
#6745=EDGE_LOOP('',(#28873,#28874,#28875,#28876));
#6746=EDGE_LOOP('',(#28877,#28878,#28879,#28880));
#6747=EDGE_LOOP('',(#28881,#28882,#28883,#28884));
#6748=EDGE_LOOP('',(#28885,#28886,#28887,#28888));
#6749=EDGE_LOOP('',(#28889,#28890,#28891,#28892));
#6750=EDGE_LOOP('',(#28893,#28894,#28895,#28896));
#6751=EDGE_LOOP('',(#28897,#28898,#28899,#28900,#28901,#28902));
#6752=EDGE_LOOP('',(#28903,#28904,#28905,#28906,#28907,#28908));
#6753=EDGE_LOOP('',(#28909,#28910,#28911,#28912));
#6754=EDGE_LOOP('',(#28913,#28914,#28915,#28916));
#6755=EDGE_LOOP('',(#28917,#28918,#28919,#28920));
#6756=EDGE_LOOP('',(#28921,#28922,#28923,#28924));
#6757=EDGE_LOOP('',(#28925,#28926,#28927,#28928));
#6758=EDGE_LOOP('',(#28929,#28930,#28931,#28932));
#6759=EDGE_LOOP('',(#28933,#28934,#28935,#28936,#28937,#28938));
#6760=EDGE_LOOP('',(#28939,#28940,#28941,#28942,#28943,#28944));
#6761=EDGE_LOOP('',(#28945,#28946,#28947,#28948));
#6762=EDGE_LOOP('',(#28949,#28950,#28951,#28952));
#6763=EDGE_LOOP('',(#28953,#28954,#28955,#28956));
#6764=EDGE_LOOP('',(#28957,#28958,#28959,#28960));
#6765=EDGE_LOOP('',(#28961,#28962,#28963,#28964));
#6766=EDGE_LOOP('',(#28965,#28966,#28967,#28968));
#6767=EDGE_LOOP('',(#28969,#28970,#28971,#28972,#28973,#28974));
#6768=EDGE_LOOP('',(#28975,#28976,#28977,#28978,#28979,#28980));
#6769=EDGE_LOOP('',(#28981,#28982,#28983,#28984));
#6770=EDGE_LOOP('',(#28985,#28986,#28987,#28988));
#6771=EDGE_LOOP('',(#28989,#28990,#28991,#28992));
#6772=EDGE_LOOP('',(#28993,#28994,#28995,#28996));
#6773=EDGE_LOOP('',(#28997,#28998,#28999,#29000));
#6774=EDGE_LOOP('',(#29001,#29002,#29003,#29004));
#6775=EDGE_LOOP('',(#29005,#29006,#29007,#29008,#29009,#29010));
#6776=EDGE_LOOP('',(#29011,#29012,#29013));
#6777=EDGE_LOOP('',(#29014,#29015,#29016,#29017));
#6778=EDGE_LOOP('',(#29018,#29019,#29020,#29021));
#6779=EDGE_LOOP('',(#29022,#29023,#29024,#29025,#29026,#29027));
#6780=EDGE_LOOP('',(#29028,#29029,#29030,#29031));
#6781=EDGE_LOOP('',(#29032,#29033,#29034,#29035));
#6782=EDGE_LOOP('',(#29036,#29037,#29038,#29039,#29040,#29041));
#6783=EDGE_LOOP('',(#29042,#29043,#29044,#29045));
#6784=EDGE_LOOP('',(#29046,#29047,#29048));
#6785=EDGE_LOOP('',(#29049,#29050,#29051,#29052));
#6786=EDGE_LOOP('',(#29053,#29054,#29055,#29056,#29057,#29058));
#6787=EDGE_LOOP('',(#29059,#29060,#29061,#29062));
#6788=EDGE_LOOP('',(#29063,#29064,#29065,#29066));
#6789=EDGE_LOOP('',(#29067,#29068,#29069,#29070));
#6790=EDGE_LOOP('',(#29071,#29072,#29073,#29074));
#6791=EDGE_LOOP('',(#29075,#29076,#29077,#29078,#29079,#29080));
#6792=EDGE_LOOP('',(#29081,#29082,#29083,#29084));
#6793=EDGE_LOOP('',(#29085,#29086,#29087,#29088));
#6794=EDGE_LOOP('',(#29089,#29090,#29091,#29092));
#6795=EDGE_LOOP('',(#29093,#29094,#29095,#29096,#29097,#29098));
#6796=EDGE_LOOP('',(#29099,#29100,#29101,#29102));
#6797=EDGE_LOOP('',(#29103,#29104,#29105,#29106));
#6798=EDGE_LOOP('',(#29107,#29108,#29109,#29110));
#6799=EDGE_LOOP('',(#29111,#29112,#29113,#29114,#29115,#29116));
#6800=EDGE_LOOP('',(#29117,#29118,#29119,#29120));
#6801=EDGE_LOOP('',(#29121,#29122,#29123,#29124));
#6802=EDGE_LOOP('',(#29125,#29126,#29127,#29128));
#6803=EDGE_LOOP('',(#29129,#29130,#29131,#29132,#29133,#29134));
#6804=EDGE_LOOP('',(#29135,#29136,#29137,#29138));
#6805=EDGE_LOOP('',(#29139,#29140,#29141,#29142));
#6806=EDGE_LOOP('',(#29143,#29144,#29145,#29146));
#6807=EDGE_LOOP('',(#29147,#29148,#29149));
#6808=EDGE_LOOP('',(#29150,#29151,#29152,#29153,#29154,#29155));
#6809=EDGE_LOOP('',(#29156,#29157,#29158,#29159));
#6810=EDGE_LOOP('',(#29160,#29161,#29162,#29163));
#6811=EDGE_LOOP('',(#29164,#29165,#29166,#29167,#29168,#29169));
#6812=EDGE_LOOP('',(#29170,#29171,#29172,#29173));
#6813=EDGE_LOOP('',(#29174,#29175,#29176));
#6814=EDGE_LOOP('',(#29177,#29178,#29179,#29180));
#6815=EDGE_LOOP('',(#29181,#29182,#29183,#29184));
#6816=EDGE_LOOP('',(#29185,#29186,#29187,#29188,#29189,#29190));
#6817=EDGE_LOOP('',(#29191,#29192,#29193,#29194));
#6818=EDGE_LOOP('',(#29195,#29196,#29197,#29198));
#6819=EDGE_LOOP('',(#29199,#29200,#29201,#29202,#29203,#29204));
#6820=EDGE_LOOP('',(#29205,#29206,#29207,#29208));
#6821=EDGE_LOOP('',(#29209,#29210,#29211,#29212));
#6822=EDGE_LOOP('',(#29213,#29214,#29215,#29216));
#6823=EDGE_LOOP('',(#29217,#29218,#29219,#29220));
#6824=EDGE_LOOP('',(#29221,#29222,#29223,#29224,#29225,#29226));
#6825=EDGE_LOOP('',(#29227,#29228,#29229,#29230));
#6826=EDGE_LOOP('',(#29231,#29232,#29233,#29234));
#6827=EDGE_LOOP('',(#29235,#29236,#29237,#29238));
#6828=EDGE_LOOP('',(#29239,#29240,#29241,#29242,#29243,#29244));
#6829=EDGE_LOOP('',(#29245,#29246,#29247,#29248));
#6830=EDGE_LOOP('',(#29249,#29250,#29251,#29252));
#6831=EDGE_LOOP('',(#29253,#29254,#29255,#29256));
#6832=EDGE_LOOP('',(#29257,#29258,#29259,#29260,#29261,#29262));
#6833=EDGE_LOOP('',(#29263,#29264,#29265,#29266));
#6834=EDGE_LOOP('',(#29267,#29268,#29269,#29270));
#6835=EDGE_LOOP('',(#29271,#29272,#29273,#29274));
#6836=EDGE_LOOP('',(#29275,#29276,#29277));
#6837=EDGE_LOOP('',(#29278,#29279,#29280,#29281,#29282,#29283));
#6838=EDGE_LOOP('',(#29284,#29285,#29286,#29287));
#6839=EDGE_LOOP('',(#29288,#29289,#29290,#29291));
#6840=EDGE_LOOP('',(#29292,#29293,#29294,#29295,#29296,#29297));
#6841=EDGE_LOOP('',(#29298,#29299,#29300,#29301));
#6842=EDGE_LOOP('',(#29302,#29303,#29304));
#6843=EDGE_LOOP('',(#29305,#29306,#29307,#29308));
#6844=EDGE_LOOP('',(#29309,#29310,#29311,#29312));
#6845=EDGE_LOOP('',(#29313,#29314,#29315,#29316,#29317,#29318));
#6846=EDGE_LOOP('',(#29319,#29320,#29321,#29322));
#6847=EDGE_LOOP('',(#29323,#29324,#29325,#29326));
#6848=EDGE_LOOP('',(#29327,#29328,#29329,#29330));
#6849=EDGE_LOOP('',(#29331,#29332,#29333,#29334,#29335,#29336));
#6850=EDGE_LOOP('',(#29337,#29338,#29339,#29340));
#6851=EDGE_LOOP('',(#29341,#29342,#29343,#29344));
#6852=EDGE_LOOP('',(#29345,#29346,#29347,#29348,#29349,#29350));
#6853=EDGE_LOOP('',(#29351,#29352,#29353,#29354));
#6854=EDGE_LOOP('',(#29355,#29356,#29357,#29358));
#6855=EDGE_LOOP('',(#29359,#29360,#29361,#29362));
#6856=EDGE_LOOP('',(#29363,#29364,#29365,#29366));
#6857=EDGE_LOOP('',(#29367,#29368,#29369,#29370,#29371,#29372));
#6858=EDGE_LOOP('',(#29373,#29374,#29375,#29376));
#6859=EDGE_LOOP('',(#29377,#29378,#29379,#29380));
#6860=EDGE_LOOP('',(#29381,#29382,#29383,#29384));
#6861=EDGE_LOOP('',(#29385,#29386,#29387,#29388,#29389,#29390));
#6862=EDGE_LOOP('',(#29391,#29392,#29393,#29394));
#6863=EDGE_LOOP('',(#29395,#29396,#29397,#29398));
#6864=EDGE_LOOP('',(#29399,#29400,#29401,#29402));
#6865=EDGE_LOOP('',(#29403,#29404,#29405));
#6866=EDGE_LOOP('',(#29406,#29407,#29408,#29409,#29410,#29411));
#6867=EDGE_LOOP('',(#29412,#29413,#29414,#29415));
#6868=EDGE_LOOP('',(#29416,#29417,#29418,#29419));
#6869=EDGE_LOOP('',(#29420,#29421,#29422,#29423,#29424,#29425));
#6870=EDGE_LOOP('',(#29426,#29427,#29428,#29429));
#6871=EDGE_LOOP('',(#29430,#29431,#29432));
#6872=EDGE_LOOP('',(#29433,#29434,#29435,#29436));
#6873=EDGE_LOOP('',(#29437,#29438,#29439,#29440));
#6874=EDGE_LOOP('',(#29441,#29442,#29443,#29444,#29445,#29446));
#6875=EDGE_LOOP('',(#29447,#29448,#29449,#29450));
#6876=EDGE_LOOP('',(#29451,#29452,#29453,#29454));
#6877=EDGE_LOOP('',(#29455,#29456,#29457,#29458));
#6878=EDGE_LOOP('',(#29459,#29460,#29461,#29462,#29463,#29464));
#6879=EDGE_LOOP('',(#29465,#29466,#29467,#29468));
#6880=EDGE_LOOP('',(#29469,#29470,#29471,#29472));
#6881=EDGE_LOOP('',(#29473,#29474,#29475,#29476));
#6882=EDGE_LOOP('',(#29477,#29478,#29479,#29480,#29481,#29482));
#6883=EDGE_LOOP('',(#29483,#29484,#29485,#29486));
#6884=EDGE_LOOP('',(#29487,#29488,#29489,#29490));
#6885=EDGE_LOOP('',(#29491,#29492,#29493,#29494,#29495,#29496));
#6886=EDGE_LOOP('',(#29497,#29498,#29499,#29500));
#6887=EDGE_LOOP('',(#29501,#29502,#29503,#29504));
#6888=EDGE_LOOP('',(#29505,#29506,#29507,#29508));
#6889=EDGE_LOOP('',(#29509,#29510,#29511,#29512));
#6890=EDGE_LOOP('',(#29513,#29514,#29515,#29516,#29517,#29518));
#6891=EDGE_LOOP('',(#29519,#29520,#29521,#29522));
#6892=EDGE_LOOP('',(#29523,#29524,#29525,#29526));
#6893=EDGE_LOOP('',(#29527,#29528,#29529,#29530));
#6894=EDGE_LOOP('',(#29531,#29532,#29533));
#6895=EDGE_LOOP('',(#29534,#29535,#29536,#29537,#29538,#29539));
#6896=EDGE_LOOP('',(#29540,#29541,#29542,#29543));
#6897=EDGE_LOOP('',(#29544,#29545,#29546,#29547));
#6898=EDGE_LOOP('',(#29548,#29549,#29550,#29551,#29552,#29553));
#6899=EDGE_LOOP('',(#29554,#29555,#29556,#29557));
#6900=EDGE_LOOP('',(#29558,#29559,#29560));
#6901=EDGE_LOOP('',(#29561,#29562,#29563,#29564));
#6902=EDGE_LOOP('',(#29565,#29566,#29567,#29568));
#6903=EDGE_LOOP('',(#29569,#29570,#29571,#29572,#29573,#29574));
#6904=EDGE_LOOP('',(#29575,#29576,#29577,#29578));
#6905=EDGE_LOOP('',(#29579,#29580,#29581,#29582));
#6906=EDGE_LOOP('',(#29583,#29584,#29585,#29586));
#6907=EDGE_LOOP('',(#29587,#29588,#29589,#29590,#29591,#29592));
#6908=EDGE_LOOP('',(#29593,#29594,#29595,#29596));
#6909=EDGE_LOOP('',(#29597,#29598,#29599,#29600));
#6910=EDGE_LOOP('',(#29601,#29602,#29603,#29604));
#6911=EDGE_LOOP('',(#29605,#29606,#29607,#29608,#29609,#29610));
#6912=EDGE_LOOP('',(#29611,#29612,#29613,#29614));
#6913=EDGE_LOOP('',(#29615,#29616,#29617,#29618));
#6914=EDGE_LOOP('',(#29619,#29620,#29621,#29622));
#6915=EDGE_LOOP('',(#29623,#29624,#29625,#29626,#29627,#29628));
#6916=EDGE_LOOP('',(#29629,#29630,#29631,#29632));
#6917=EDGE_LOOP('',(#29633,#29634,#29635,#29636));
#6918=EDGE_LOOP('',(#29637,#29638,#29639,#29640,#29641,#29642));
#6919=EDGE_LOOP('',(#29643,#29644,#29645,#29646));
#6920=EDGE_LOOP('',(#29647,#29648,#29649,#29650));
#6921=EDGE_LOOP('',(#29651,#29652,#29653,#29654));
#6922=EDGE_LOOP('',(#29655,#29656,#29657,#29658));
#6923=EDGE_LOOP('',(#29659,#29660,#29661));
#6924=EDGE_LOOP('',(#29662,#29663,#29664,#29665,#29666,#29667));
#6925=EDGE_LOOP('',(#29668,#29669,#29670,#29671));
#6926=EDGE_LOOP('',(#29672,#29673,#29674,#29675));
#6927=EDGE_LOOP('',(#29676,#29677,#29678,#29679,#29680,#29681));
#6928=EDGE_LOOP('',(#29682,#29683,#29684,#29685));
#6929=EDGE_LOOP('',(#29686,#29687,#29688));
#6930=EDGE_LOOP('',(#29689,#29690,#29691,#29692));
#6931=EDGE_LOOP('',(#29693,#29694,#29695,#29696));
#6932=EDGE_LOOP('',(#29697,#29698,#29699,#29700,#29701,#29702));
#6933=EDGE_LOOP('',(#29703,#29704,#29705,#29706));
#6934=EDGE_LOOP('',(#29707,#29708,#29709,#29710));
#6935=EDGE_LOOP('',(#29711,#29712,#29713,#29714));
#6936=EDGE_LOOP('',(#29715,#29716,#29717,#29718,#29719,#29720));
#6937=EDGE_LOOP('',(#29721,#29722,#29723,#29724));
#6938=EDGE_LOOP('',(#29725,#29726,#29727,#29728));
#6939=EDGE_LOOP('',(#29729,#29730,#29731,#29732));
#6940=EDGE_LOOP('',(#29733,#29734,#29735,#29736,#29737,#29738));
#6941=EDGE_LOOP('',(#29739,#29740,#29741,#29742));
#6942=EDGE_LOOP('',(#29743,#29744,#29745,#29746));
#6943=EDGE_LOOP('',(#29747,#29748,#29749,#29750));
#6944=EDGE_LOOP('',(#29751,#29752,#29753,#29754,#29755,#29756));
#6945=EDGE_LOOP('',(#29757,#29758,#29759,#29760));
#6946=EDGE_LOOP('',(#29761,#29762,#29763,#29764));
#6947=EDGE_LOOP('',(#29765,#29766,#29767,#29768));
#6948=EDGE_LOOP('',(#29769,#29770,#29771,#29772,#29773,#29774));
#6949=EDGE_LOOP('',(#29775,#29776,#29777,#29778));
#6950=EDGE_LOOP('',(#29779,#29780,#29781,#29782));
#6951=EDGE_LOOP('',(#29783,#29784,#29785,#29786));
#6952=EDGE_LOOP('',(#29787,#29788,#29789));
#6953=EDGE_LOOP('',(#29790,#29791,#29792,#29793,#29794,#29795));
#6954=EDGE_LOOP('',(#29796,#29797,#29798,#29799));
#6955=EDGE_LOOP('',(#29800,#29801,#29802,#29803));
#6956=EDGE_LOOP('',(#29804,#29805,#29806,#29807,#29808,#29809));
#6957=EDGE_LOOP('',(#29810,#29811,#29812,#29813));
#6958=EDGE_LOOP('',(#29814,#29815,#29816));
#6959=EDGE_LOOP('',(#29817,#29818,#29819,#29820));
#6960=EDGE_LOOP('',(#29821,#29822,#29823,#29824));
#6961=EDGE_LOOP('',(#29825,#29826,#29827,#29828,#29829,#29830));
#6962=EDGE_LOOP('',(#29831,#29832,#29833,#29834));
#6963=EDGE_LOOP('',(#29835,#29836,#29837,#29838));
#6964=EDGE_LOOP('',(#29839,#29840,#29841,#29842));
#6965=EDGE_LOOP('',(#29843,#29844,#29845,#29846,#29847,#29848));
#6966=EDGE_LOOP('',(#29849,#29850,#29851,#29852));
#6967=EDGE_LOOP('',(#29853,#29854,#29855,#29856));
#6968=EDGE_LOOP('',(#29857,#29858,#29859,#29860));
#6969=EDGE_LOOP('',(#29861,#29862,#29863,#29864,#29865,#29866));
#6970=EDGE_LOOP('',(#29867,#29868,#29869,#29870));
#6971=EDGE_LOOP('',(#29871,#29872,#29873,#29874));
#6972=EDGE_LOOP('',(#29875,#29876,#29877,#29878));
#6973=EDGE_LOOP('',(#29879,#29880,#29881,#29882,#29883,#29884));
#6974=EDGE_LOOP('',(#29885,#29886,#29887,#29888));
#6975=EDGE_LOOP('',(#29889,#29890,#29891,#29892));
#6976=EDGE_LOOP('',(#29893,#29894,#29895,#29896));
#6977=EDGE_LOOP('',(#29897,#29898,#29899,#29900,#29901,#29902));
#6978=EDGE_LOOP('',(#29903,#29904,#29905,#29906));
#6979=EDGE_LOOP('',(#29907,#29908,#29909,#29910));
#6980=EDGE_LOOP('',(#29911,#29912,#29913,#29914));
#6981=EDGE_LOOP('',(#29915,#29916,#29917));
#6982=EDGE_LOOP('',(#29918,#29919,#29920,#29921,#29922,#29923));
#6983=EDGE_LOOP('',(#29924,#29925,#29926,#29927));
#6984=EDGE_LOOP('',(#29928,#29929,#29930,#29931));
#6985=EDGE_LOOP('',(#29932,#29933,#29934,#29935,#29936,#29937));
#6986=EDGE_LOOP('',(#29938,#29939,#29940,#29941));
#6987=EDGE_LOOP('',(#29942,#29943,#29944));
#6988=EDGE_LOOP('',(#29945,#29946,#29947,#29948));
#6989=EDGE_LOOP('',(#29949,#29950,#29951,#29952));
#6990=EDGE_LOOP('',(#29953,#29954,#29955,#29956,#29957,#29958));
#6991=EDGE_LOOP('',(#29959,#29960,#29961,#29962));
#6992=EDGE_LOOP('',(#29963,#29964,#29965,#29966));
#6993=EDGE_LOOP('',(#29967,#29968,#29969,#29970));
#6994=EDGE_LOOP('',(#29971,#29972,#29973,#29974,#29975,#29976));
#6995=EDGE_LOOP('',(#29977,#29978,#29979,#29980));
#6996=EDGE_LOOP('',(#29981,#29982,#29983,#29984));
#6997=EDGE_LOOP('',(#29985,#29986,#29987,#29988));
#6998=EDGE_LOOP('',(#29989,#29990,#29991,#29992,#29993,#29994));
#6999=EDGE_LOOP('',(#29995,#29996,#29997,#29998));
#7000=EDGE_LOOP('',(#29999,#30000,#30001,#30002));
#7001=EDGE_LOOP('',(#30003,#30004,#30005,#30006));
#7002=EDGE_LOOP('',(#30007,#30008,#30009,#30010,#30011,#30012));
#7003=EDGE_LOOP('',(#30013,#30014,#30015,#30016));
#7004=EDGE_LOOP('',(#30017,#30018,#30019,#30020));
#7005=EDGE_LOOP('',(#30021,#30022,#30023,#30024));
#7006=EDGE_LOOP('',(#30025,#30026,#30027,#30028,#30029,#30030));
#7007=EDGE_LOOP('',(#30031,#30032,#30033,#30034));
#7008=EDGE_LOOP('',(#30035,#30036,#30037,#30038));
#7009=EDGE_LOOP('',(#30039,#30040,#30041,#30042));
#7010=EDGE_LOOP('',(#30043,#30044,#30045));
#7011=EDGE_LOOP('',(#30046,#30047,#30048,#30049,#30050,#30051));
#7012=EDGE_LOOP('',(#30052,#30053,#30054,#30055));
#7013=EDGE_LOOP('',(#30056,#30057,#30058,#30059));
#7014=EDGE_LOOP('',(#30060,#30061,#30062,#30063,#30064,#30065));
#7015=EDGE_LOOP('',(#30066,#30067,#30068,#30069));
#7016=EDGE_LOOP('',(#30070,#30071,#30072));
#7017=EDGE_LOOP('',(#30073,#30074,#30075,#30076));
#7018=EDGE_LOOP('',(#30077,#30078,#30079,#30080));
#7019=EDGE_LOOP('',(#30081,#30082,#30083,#30084,#30085,#30086));
#7020=EDGE_LOOP('',(#30087,#30088,#30089,#30090));
#7021=EDGE_LOOP('',(#30091,#30092,#30093,#30094));
#7022=EDGE_LOOP('',(#30095,#30096,#30097,#30098));
#7023=EDGE_LOOP('',(#30099,#30100,#30101,#30102,#30103,#30104));
#7024=EDGE_LOOP('',(#30105,#30106,#30107,#30108));
#7025=EDGE_LOOP('',(#30109,#30110,#30111,#30112));
#7026=EDGE_LOOP('',(#30113,#30114,#30115,#30116));
#7027=EDGE_LOOP('',(#30117,#30118,#30119,#30120,#30121,#30122));
#7028=EDGE_LOOP('',(#30123,#30124,#30125,#30126));
#7029=EDGE_LOOP('',(#30127,#30128,#30129,#30130));
#7030=EDGE_LOOP('',(#30131,#30132,#30133,#30134));
#7031=EDGE_LOOP('',(#30135,#30136,#30137,#30138,#30139,#30140));
#7032=EDGE_LOOP('',(#30141,#30142,#30143,#30144));
#7033=EDGE_LOOP('',(#30145,#30146,#30147,#30148));
#7034=EDGE_LOOP('',(#30149,#30150,#30151,#30152));
#7035=EDGE_LOOP('',(#30153,#30154,#30155,#30156,#30157,#30158));
#7036=EDGE_LOOP('',(#30159,#30160,#30161,#30162));
#7037=EDGE_LOOP('',(#30163,#30164,#30165,#30166));
#7038=EDGE_LOOP('',(#30167,#30168,#30169,#30170));
#7039=EDGE_LOOP('',(#30171,#30172,#30173));
#7040=EDGE_LOOP('',(#30174,#30175,#30176,#30177,#30178,#30179));
#7041=EDGE_LOOP('',(#30180,#30181,#30182,#30183));
#7042=EDGE_LOOP('',(#30184,#30185,#30186,#30187));
#7043=EDGE_LOOP('',(#30188,#30189,#30190,#30191,#30192,#30193));
#7044=EDGE_LOOP('',(#30194,#30195,#30196,#30197));
#7045=EDGE_LOOP('',(#30198,#30199,#30200));
#7046=EDGE_LOOP('',(#30201,#30202,#30203,#30204));
#7047=EDGE_LOOP('',(#30205,#30206,#30207,#30208));
#7048=EDGE_LOOP('',(#30209,#30210,#30211,#30212,#30213,#30214));
#7049=EDGE_LOOP('',(#30215,#30216,#30217,#30218));
#7050=EDGE_LOOP('',(#30219,#30220,#30221,#30222));
#7051=EDGE_LOOP('',(#30223,#30224,#30225,#30226));
#7052=EDGE_LOOP('',(#30227,#30228,#30229,#30230,#30231,#30232));
#7053=EDGE_LOOP('',(#30233,#30234,#30235,#30236));
#7054=EDGE_LOOP('',(#30237,#30238,#30239,#30240));
#7055=EDGE_LOOP('',(#30241,#30242,#30243,#30244));
#7056=EDGE_LOOP('',(#30245,#30246,#30247,#30248,#30249,#30250));
#7057=EDGE_LOOP('',(#30251,#30252,#30253,#30254));
#7058=EDGE_LOOP('',(#30255,#30256,#30257,#30258));
#7059=EDGE_LOOP('',(#30259,#30260,#30261,#30262));
#7060=EDGE_LOOP('',(#30263,#30264,#30265,#30266,#30267,#30268));
#7061=EDGE_LOOP('',(#30269,#30270,#30271,#30272));
#7062=EDGE_LOOP('',(#30273,#30274,#30275,#30276));
#7063=EDGE_LOOP('',(#30277,#30278,#30279,#30280));
#7064=EDGE_LOOP('',(#30281,#30282,#30283,#30284,#30285,#30286));
#7065=EDGE_LOOP('',(#30287,#30288,#30289,#30290));
#7066=EDGE_LOOP('',(#30291,#30292,#30293,#30294));
#7067=EDGE_LOOP('',(#30295,#30296,#30297,#30298));
#7068=EDGE_LOOP('',(#30299,#30300,#30301));
#7069=EDGE_LOOP('',(#30302,#30303,#30304,#30305,#30306,#30307));
#7070=EDGE_LOOP('',(#30308,#30309,#30310,#30311));
#7071=EDGE_LOOP('',(#30312,#30313,#30314,#30315));
#7072=EDGE_LOOP('',(#30316,#30317,#30318,#30319,#30320,#30321));
#7073=EDGE_LOOP('',(#30322,#30323,#30324,#30325));
#7074=EDGE_LOOP('',(#30326,#30327,#30328));
#7075=EDGE_LOOP('',(#30329,#30330,#30331,#30332));
#7076=EDGE_LOOP('',(#30333,#30334,#30335,#30336));
#7077=EDGE_LOOP('',(#30337,#30338,#30339,#30340,#30341,#30342));
#7078=EDGE_LOOP('',(#30343,#30344,#30345,#30346));
#7079=EDGE_LOOP('',(#30347,#30348,#30349,#30350));
#7080=EDGE_LOOP('',(#30351,#30352,#30353,#30354));
#7081=EDGE_LOOP('',(#30355,#30356,#30357,#30358,#30359,#30360));
#7082=EDGE_LOOP('',(#30361,#30362,#30363,#30364));
#7083=EDGE_LOOP('',(#30365,#30366,#30367,#30368));
#7084=EDGE_LOOP('',(#30369,#30370,#30371,#30372));
#7085=EDGE_LOOP('',(#30373,#30374,#30375,#30376,#30377,#30378));
#7086=EDGE_LOOP('',(#30379,#30380,#30381,#30382));
#7087=EDGE_LOOP('',(#30383,#30384,#30385,#30386));
#7088=EDGE_LOOP('',(#30387,#30388,#30389,#30390));
#7089=EDGE_LOOP('',(#30391,#30392,#30393,#30394,#30395,#30396));
#7090=EDGE_LOOP('',(#30397,#30398,#30399,#30400));
#7091=EDGE_LOOP('',(#30401,#30402,#30403,#30404));
#7092=EDGE_LOOP('',(#30405,#30406,#30407,#30408));
#7093=EDGE_LOOP('',(#30409,#30410,#30411,#30412,#30413,#30414));
#7094=EDGE_LOOP('',(#30415,#30416,#30417,#30418));
#7095=EDGE_LOOP('',(#30419,#30420,#30421,#30422));
#7096=EDGE_LOOP('',(#30423,#30424,#30425,#30426));
#7097=EDGE_LOOP('',(#30427,#30428,#30429));
#7098=EDGE_LOOP('',(#30430,#30431,#30432,#30433,#30434,#30435));
#7099=EDGE_LOOP('',(#30436,#30437,#30438,#30439));
#7100=EDGE_LOOP('',(#30440,#30441,#30442,#30443));
#7101=EDGE_LOOP('',(#30444,#30445,#30446,#30447,#30448,#30449));
#7102=EDGE_LOOP('',(#30450,#30451,#30452,#30453));
#7103=EDGE_LOOP('',(#30454,#30455,#30456));
#7104=EDGE_LOOP('',(#30457,#30458,#30459,#30460));
#7105=EDGE_LOOP('',(#30461,#30462,#30463,#30464));
#7106=EDGE_LOOP('',(#30465,#30466,#30467,#30468,#30469,#30470));
#7107=EDGE_LOOP('',(#30471,#30472,#30473,#30474));
#7108=EDGE_LOOP('',(#30475,#30476,#30477,#30478));
#7109=EDGE_LOOP('',(#30479,#30480,#30481,#30482));
#7110=EDGE_LOOP('',(#30483,#30484,#30485,#30486,#30487,#30488));
#7111=EDGE_LOOP('',(#30489,#30490,#30491,#30492));
#7112=EDGE_LOOP('',(#30493,#30494,#30495,#30496));
#7113=EDGE_LOOP('',(#30497,#30498,#30499,#30500));
#7114=EDGE_LOOP('',(#30501,#30502,#30503,#30504,#30505,#30506));
#7115=EDGE_LOOP('',(#30507,#30508,#30509,#30510));
#7116=EDGE_LOOP('',(#30511,#30512,#30513,#30514));
#7117=EDGE_LOOP('',(#30515,#30516,#30517,#30518));
#7118=EDGE_LOOP('',(#30519,#30520,#30521,#30522,#30523,#30524));
#7119=EDGE_LOOP('',(#30525,#30526,#30527,#30528));
#7120=EDGE_LOOP('',(#30529,#30530,#30531,#30532));
#7121=EDGE_LOOP('',(#30533,#30534,#30535,#30536));
#7122=EDGE_LOOP('',(#30537,#30538,#30539,#30540,#30541,#30542));
#7123=EDGE_LOOP('',(#30543,#30544,#30545,#30546));
#7124=EDGE_LOOP('',(#30547,#30548,#30549,#30550));
#7125=EDGE_LOOP('',(#30551,#30552,#30553,#30554));
#7126=EDGE_LOOP('',(#30555,#30556,#30557));
#7127=EDGE_LOOP('',(#30558,#30559,#30560,#30561,#30562,#30563));
#7128=EDGE_LOOP('',(#30564,#30565,#30566,#30567));
#7129=EDGE_LOOP('',(#30568,#30569,#30570,#30571));
#7130=EDGE_LOOP('',(#30572,#30573,#30574,#30575,#30576,#30577));
#7131=EDGE_LOOP('',(#30578,#30579,#30580,#30581));
#7132=EDGE_LOOP('',(#30582,#30583,#30584));
#7133=EDGE_LOOP('',(#30585,#30586,#30587,#30588));
#7134=EDGE_LOOP('',(#30589,#30590,#30591,#30592));
#7135=EDGE_LOOP('',(#30593,#30594,#30595,#30596,#30597,#30598));
#7136=EDGE_LOOP('',(#30599,#30600,#30601,#30602));
#7137=EDGE_LOOP('',(#30603,#30604,#30605,#30606));
#7138=EDGE_LOOP('',(#30607,#30608,#30609,#30610));
#7139=EDGE_LOOP('',(#30611,#30612,#30613,#30614,#30615,#30616));
#7140=EDGE_LOOP('',(#30617,#30618,#30619,#30620));
#7141=EDGE_LOOP('',(#30621,#30622,#30623,#30624));
#7142=EDGE_LOOP('',(#30625,#30626,#30627,#30628));
#7143=EDGE_LOOP('',(#30629,#30630,#30631,#30632,#30633,#30634));
#7144=EDGE_LOOP('',(#30635,#30636,#30637,#30638));
#7145=EDGE_LOOP('',(#30639,#30640,#30641,#30642));
#7146=EDGE_LOOP('',(#30643,#30644,#30645,#30646));
#7147=EDGE_LOOP('',(#30647,#30648,#30649,#30650,#30651,#30652));
#7148=EDGE_LOOP('',(#30653,#30654,#30655,#30656));
#7149=EDGE_LOOP('',(#30657,#30658,#30659,#30660));
#7150=EDGE_LOOP('',(#30661,#30662,#30663,#30664));
#7151=EDGE_LOOP('',(#30665,#30666,#30667,#30668,#30669,#30670));
#7152=EDGE_LOOP('',(#30671,#30672,#30673,#30674));
#7153=EDGE_LOOP('',(#30675,#30676,#30677,#30678));
#7154=EDGE_LOOP('',(#30679,#30680,#30681,#30682));
#7155=EDGE_LOOP('',(#30683,#30684,#30685));
#7156=EDGE_LOOP('',(#30686,#30687,#30688,#30689,#30690,#30691));
#7157=EDGE_LOOP('',(#30692,#30693,#30694,#30695));
#7158=EDGE_LOOP('',(#30696,#30697,#30698,#30699));
#7159=EDGE_LOOP('',(#30700,#30701,#30702,#30703,#30704,#30705));
#7160=EDGE_LOOP('',(#30706,#30707,#30708,#30709));
#7161=EDGE_LOOP('',(#30710,#30711,#30712));
#7162=EDGE_LOOP('',(#30713,#30714,#30715,#30716));
#7163=EDGE_LOOP('',(#30717,#30718,#30719,#30720));
#7164=EDGE_LOOP('',(#30721,#30722,#30723,#30724,#30725,#30726));
#7165=EDGE_LOOP('',(#30727,#30728,#30729,#30730));
#7166=EDGE_LOOP('',(#30731,#30732,#30733,#30734));
#7167=EDGE_LOOP('',(#30735,#30736,#30737,#30738));
#7168=EDGE_LOOP('',(#30739,#30740,#30741,#30742,#30743,#30744));
#7169=EDGE_LOOP('',(#30745,#30746,#30747,#30748));
#7170=EDGE_LOOP('',(#30749,#30750,#30751,#30752));
#7171=EDGE_LOOP('',(#30753,#30754,#30755,#30756));
#7172=EDGE_LOOP('',(#30757,#30758,#30759,#30760,#30761,#30762));
#7173=EDGE_LOOP('',(#30763,#30764,#30765,#30766));
#7174=EDGE_LOOP('',(#30767,#30768,#30769,#30770));
#7175=EDGE_LOOP('',(#30771,#30772,#30773,#30774));
#7176=EDGE_LOOP('',(#30775,#30776,#30777,#30778,#30779,#30780));
#7177=EDGE_LOOP('',(#30781,#30782,#30783,#30784));
#7178=EDGE_LOOP('',(#30785,#30786,#30787,#30788));
#7179=EDGE_LOOP('',(#30789,#30790,#30791,#30792));
#7180=EDGE_LOOP('',(#30793,#30794,#30795,#30796,#30797,#30798));
#7181=EDGE_LOOP('',(#30799,#30800,#30801,#30802));
#7182=EDGE_LOOP('',(#30803,#30804,#30805,#30806));
#7183=EDGE_LOOP('',(#30807,#30808,#30809,#30810));
#7184=EDGE_LOOP('',(#30811,#30812,#30813));
#7185=EDGE_LOOP('',(#30814,#30815,#30816,#30817,#30818,#30819));
#7186=EDGE_LOOP('',(#30820,#30821,#30822,#30823));
#7187=EDGE_LOOP('',(#30824,#30825,#30826,#30827));
#7188=EDGE_LOOP('',(#30828,#30829,#30830,#30831,#30832,#30833));
#7189=EDGE_LOOP('',(#30834,#30835,#30836,#30837));
#7190=EDGE_LOOP('',(#30838,#30839,#30840));
#7191=EDGE_LOOP('',(#30841,#30842,#30843,#30844));
#7192=EDGE_LOOP('',(#30845,#30846,#30847,#30848));
#7193=EDGE_LOOP('',(#30849,#30850,#30851,#30852,#30853,#30854));
#7194=EDGE_LOOP('',(#30855,#30856,#30857,#30858));
#7195=EDGE_LOOP('',(#30859,#30860,#30861,#30862));
#7196=EDGE_LOOP('',(#30863,#30864,#30865,#30866));
#7197=EDGE_LOOP('',(#30867,#30868,#30869,#30870,#30871,#30872));
#7198=EDGE_LOOP('',(#30873,#30874,#30875,#30876));
#7199=EDGE_LOOP('',(#30877,#30878,#30879,#30880));
#7200=EDGE_LOOP('',(#30881,#30882,#30883,#30884));
#7201=EDGE_LOOP('',(#30885,#30886,#30887,#30888,#30889,#30890));
#7202=EDGE_LOOP('',(#30891,#30892,#30893,#30894));
#7203=EDGE_LOOP('',(#30895,#30896,#30897,#30898));
#7204=EDGE_LOOP('',(#30899,#30900,#30901,#30902));
#7205=EDGE_LOOP('',(#30903,#30904,#30905,#30906,#30907,#30908));
#7206=EDGE_LOOP('',(#30909,#30910,#30911,#30912));
#7207=EDGE_LOOP('',(#30913,#30914,#30915,#30916));
#7208=EDGE_LOOP('',(#30917,#30918,#30919,#30920));
#7209=EDGE_LOOP('',(#30921,#30922,#30923,#30924,#30925,#30926));
#7210=EDGE_LOOP('',(#30927,#30928,#30929,#30930));
#7211=EDGE_LOOP('',(#30931,#30932,#30933,#30934));
#7212=EDGE_LOOP('',(#30935,#30936,#30937,#30938));
#7213=EDGE_LOOP('',(#30939,#30940,#30941));
#7214=EDGE_LOOP('',(#30942,#30943,#30944,#30945,#30946,#30947));
#7215=EDGE_LOOP('',(#30948,#30949,#30950,#30951));
#7216=EDGE_LOOP('',(#30952,#30953,#30954,#30955));
#7217=EDGE_LOOP('',(#30956,#30957,#30958,#30959,#30960,#30961));
#7218=EDGE_LOOP('',(#30962,#30963,#30964,#30965));
#7219=EDGE_LOOP('',(#30966,#30967,#30968));
#7220=EDGE_LOOP('',(#30969,#30970,#30971,#30972));
#7221=EDGE_LOOP('',(#30973,#30974,#30975,#30976));
#7222=EDGE_LOOP('',(#30977,#30978,#30979,#30980,#30981,#30982));
#7223=EDGE_LOOP('',(#30983,#30984,#30985,#30986));
#7224=EDGE_LOOP('',(#30987,#30988,#30989,#30990));
#7225=EDGE_LOOP('',(#30991,#30992,#30993,#30994));
#7226=EDGE_LOOP('',(#30995,#30996,#30997,#30998,#30999,#31000));
#7227=EDGE_LOOP('',(#31001,#31002,#31003,#31004));
#7228=EDGE_LOOP('',(#31005,#31006,#31007,#31008));
#7229=EDGE_LOOP('',(#31009,#31010,#31011,#31012));
#7230=EDGE_LOOP('',(#31013,#31014,#31015,#31016,#31017,#31018));
#7231=EDGE_LOOP('',(#31019,#31020,#31021,#31022));
#7232=EDGE_LOOP('',(#31023,#31024,#31025,#31026));
#7233=EDGE_LOOP('',(#31027,#31028,#31029,#31030));
#7234=EDGE_LOOP('',(#31031,#31032,#31033,#31034,#31035,#31036));
#7235=EDGE_LOOP('',(#31037,#31038,#31039,#31040));
#7236=EDGE_LOOP('',(#31041,#31042,#31043,#31044));
#7237=EDGE_LOOP('',(#31045,#31046,#31047,#31048));
#7238=EDGE_LOOP('',(#31049,#31050,#31051,#31052,#31053,#31054));
#7239=EDGE_LOOP('',(#31055,#31056,#31057,#31058));
#7240=EDGE_LOOP('',(#31059,#31060,#31061,#31062));
#7241=EDGE_LOOP('',(#31063,#31064,#31065,#31066));
#7242=EDGE_LOOP('',(#31067,#31068,#31069));
#7243=EDGE_LOOP('',(#31070,#31071,#31072,#31073,#31074,#31075));
#7244=EDGE_LOOP('',(#31076,#31077,#31078,#31079));
#7245=EDGE_LOOP('',(#31080,#31081,#31082,#31083));
#7246=EDGE_LOOP('',(#31084,#31085,#31086,#31087,#31088,#31089));
#7247=EDGE_LOOP('',(#31090,#31091,#31092,#31093));
#7248=EDGE_LOOP('',(#31094,#31095,#31096));
#7249=EDGE_LOOP('',(#31097,#31098,#31099,#31100));
#7250=EDGE_LOOP('',(#31101,#31102,#31103,#31104));
#7251=EDGE_LOOP('',(#31105,#31106,#31107,#31108,#31109,#31110));
#7252=EDGE_LOOP('',(#31111,#31112,#31113,#31114));
#7253=EDGE_LOOP('',(#31115,#31116,#31117,#31118));
#7254=EDGE_LOOP('',(#31119,#31120,#31121,#31122));
#7255=EDGE_LOOP('',(#31123,#31124,#31125,#31126,#31127,#31128));
#7256=EDGE_LOOP('',(#31129,#31130,#31131,#31132));
#7257=EDGE_LOOP('',(#31133,#31134,#31135,#31136));
#7258=EDGE_LOOP('',(#31137,#31138,#31139,#31140));
#7259=EDGE_LOOP('',(#31141,#31142,#31143,#31144,#31145,#31146));
#7260=EDGE_LOOP('',(#31147,#31148,#31149,#31150));
#7261=EDGE_LOOP('',(#31151,#31152,#31153,#31154));
#7262=EDGE_LOOP('',(#31155,#31156,#31157,#31158));
#7263=EDGE_LOOP('',(#31159,#31160,#31161,#31162,#31163,#31164));
#7264=EDGE_LOOP('',(#31165,#31166,#31167,#31168));
#7265=EDGE_LOOP('',(#31169,#31170,#31171,#31172));
#7266=EDGE_LOOP('',(#31173,#31174,#31175,#31176));
#7267=EDGE_LOOP('',(#31177,#31178,#31179,#31180,#31181,#31182));
#7268=EDGE_LOOP('',(#31183,#31184,#31185,#31186));
#7269=EDGE_LOOP('',(#31187,#31188,#31189,#31190));
#7270=EDGE_LOOP('',(#31191,#31192,#31193,#31194));
#7271=EDGE_LOOP('',(#31195,#31196,#31197));
#7272=EDGE_LOOP('',(#31198,#31199,#31200,#31201,#31202,#31203));
#7273=EDGE_LOOP('',(#31204,#31205,#31206,#31207));
#7274=EDGE_LOOP('',(#31208,#31209,#31210,#31211));
#7275=EDGE_LOOP('',(#31212,#31213,#31214,#31215,#31216,#31217));
#7276=EDGE_LOOP('',(#31218,#31219,#31220,#31221));
#7277=EDGE_LOOP('',(#31222,#31223,#31224));
#7278=EDGE_LOOP('',(#31225,#31226,#31227,#31228));
#7279=EDGE_LOOP('',(#31229,#31230,#31231,#31232));
#7280=EDGE_LOOP('',(#31233,#31234,#31235,#31236,#31237,#31238));
#7281=EDGE_LOOP('',(#31239,#31240,#31241,#31242));
#7282=EDGE_LOOP('',(#31243,#31244,#31245,#31246));
#7283=EDGE_LOOP('',(#31247,#31248,#31249,#31250));
#7284=EDGE_LOOP('',(#31251,#31252,#31253,#31254,#31255,#31256));
#7285=EDGE_LOOP('',(#31257,#31258,#31259,#31260));
#7286=EDGE_LOOP('',(#31261,#31262,#31263,#31264));
#7287=EDGE_LOOP('',(#31265,#31266,#31267,#31268));
#7288=EDGE_LOOP('',(#31269,#31270,#31271,#31272,#31273,#31274));
#7289=EDGE_LOOP('',(#31275,#31276,#31277,#31278));
#7290=EDGE_LOOP('',(#31279,#31280,#31281,#31282));
#7291=EDGE_LOOP('',(#31283,#31284,#31285,#31286));
#7292=EDGE_LOOP('',(#31287,#31288,#31289,#31290,#31291,#31292));
#7293=EDGE_LOOP('',(#31293,#31294,#31295,#31296));
#7294=EDGE_LOOP('',(#31297,#31298,#31299,#31300));
#7295=EDGE_LOOP('',(#31301,#31302,#31303,#31304));
#7296=EDGE_LOOP('',(#31305,#31306,#31307,#31308,#31309,#31310));
#7297=EDGE_LOOP('',(#31311,#31312,#31313,#31314));
#7298=EDGE_LOOP('',(#31315,#31316,#31317,#31318));
#7299=EDGE_LOOP('',(#31319,#31320,#31321,#31322));
#7300=EDGE_LOOP('',(#31323,#31324,#31325));
#7301=EDGE_LOOP('',(#31326,#31327,#31328,#31329,#31330,#31331));
#7302=EDGE_LOOP('',(#31332,#31333,#31334,#31335));
#7303=EDGE_LOOP('',(#31336,#31337,#31338,#31339));
#7304=EDGE_LOOP('',(#31340,#31341,#31342,#31343,#31344,#31345));
#7305=EDGE_LOOP('',(#31346,#31347,#31348,#31349));
#7306=EDGE_LOOP('',(#31350,#31351,#31352));
#7307=EDGE_LOOP('',(#31353,#31354,#31355,#31356));
#7308=EDGE_LOOP('',(#31357,#31358,#31359,#31360));
#7309=EDGE_LOOP('',(#31361,#31362,#31363,#31364,#31365,#31366));
#7310=EDGE_LOOP('',(#31367,#31368,#31369,#31370));
#7311=EDGE_LOOP('',(#31371,#31372,#31373,#31374));
#7312=EDGE_LOOP('',(#31375,#31376,#31377,#31378));
#7313=EDGE_LOOP('',(#31379,#31380,#31381,#31382,#31383,#31384));
#7314=EDGE_LOOP('',(#31385,#31386,#31387,#31388));
#7315=EDGE_LOOP('',(#31389,#31390,#31391,#31392));
#7316=EDGE_LOOP('',(#31393,#31394,#31395,#31396));
#7317=EDGE_LOOP('',(#31397,#31398,#31399,#31400,#31401,#31402));
#7318=EDGE_LOOP('',(#31403,#31404,#31405,#31406));
#7319=EDGE_LOOP('',(#31407,#31408,#31409,#31410));
#7320=EDGE_LOOP('',(#31411,#31412,#31413,#31414));
#7321=EDGE_LOOP('',(#31415,#31416,#31417,#31418,#31419,#31420));
#7322=EDGE_LOOP('',(#31421,#31422,#31423,#31424));
#7323=EDGE_LOOP('',(#31425,#31426,#31427,#31428));
#7324=EDGE_LOOP('',(#31429,#31430,#31431,#31432));
#7325=EDGE_LOOP('',(#31433,#31434,#31435,#31436,#31437,#31438));
#7326=EDGE_LOOP('',(#31439,#31440,#31441,#31442));
#7327=EDGE_LOOP('',(#31443,#31444,#31445,#31446));
#7328=EDGE_LOOP('',(#31447,#31448,#31449,#31450));
#7329=EDGE_LOOP('',(#31451,#31452,#31453));
#7330=EDGE_LOOP('',(#31454,#31455,#31456,#31457,#31458,#31459));
#7331=EDGE_LOOP('',(#31460,#31461,#31462,#31463));
#7332=EDGE_LOOP('',(#31464,#31465,#31466,#31467));
#7333=EDGE_LOOP('',(#31468,#31469,#31470,#31471,#31472,#31473));
#7334=EDGE_LOOP('',(#31474,#31475,#31476,#31477));
#7335=EDGE_LOOP('',(#31478,#31479,#31480));
#7336=EDGE_LOOP('',(#31481,#31482,#31483,#31484));
#7337=EDGE_LOOP('',(#31485,#31486,#31487,#31488));
#7338=EDGE_LOOP('',(#31489,#31490,#31491,#31492,#31493,#31494));
#7339=EDGE_LOOP('',(#31495,#31496,#31497,#31498));
#7340=EDGE_LOOP('',(#31499,#31500,#31501,#31502));
#7341=EDGE_LOOP('',(#31503,#31504,#31505,#31506));
#7342=EDGE_LOOP('',(#31507,#31508,#31509,#31510,#31511,#31512));
#7343=EDGE_LOOP('',(#31513,#31514,#31515,#31516));
#7344=EDGE_LOOP('',(#31517,#31518,#31519,#31520));
#7345=EDGE_LOOP('',(#31521,#31522,#31523,#31524));
#7346=EDGE_LOOP('',(#31525,#31526,#31527,#31528,#31529,#31530));
#7347=EDGE_LOOP('',(#31531,#31532,#31533,#31534));
#7348=EDGE_LOOP('',(#31535,#31536,#31537,#31538));
#7349=EDGE_LOOP('',(#31539,#31540,#31541,#31542));
#7350=EDGE_LOOP('',(#31543,#31544,#31545,#31546,#31547,#31548));
#7351=EDGE_LOOP('',(#31549,#31550,#31551,#31552));
#7352=EDGE_LOOP('',(#31553,#31554,#31555,#31556));
#7353=EDGE_LOOP('',(#31557,#31558,#31559,#31560));
#7354=EDGE_LOOP('',(#31561,#31562,#31563,#31564,#31565,#31566));
#7355=EDGE_LOOP('',(#31567,#31568,#31569,#31570));
#7356=EDGE_LOOP('',(#31571,#31572,#31573,#31574));
#7357=EDGE_LOOP('',(#31575,#31576,#31577,#31578));
#7358=EDGE_LOOP('',(#31579,#31580,#31581));
#7359=EDGE_LOOP('',(#31582,#31583,#31584,#31585,#31586,#31587));
#7360=EDGE_LOOP('',(#31588,#31589,#31590,#31591));
#7361=EDGE_LOOP('',(#31592,#31593,#31594,#31595));
#7362=EDGE_LOOP('',(#31596,#31597,#31598,#31599,#31600,#31601));
#7363=EDGE_LOOP('',(#31602,#31603,#31604,#31605));
#7364=EDGE_LOOP('',(#31606,#31607,#31608));
#7365=EDGE_LOOP('',(#31609,#31610,#31611,#31612));
#7366=EDGE_LOOP('',(#31613,#31614,#31615,#31616));
#7367=EDGE_LOOP('',(#31617,#31618,#31619,#31620,#31621,#31622));
#7368=EDGE_LOOP('',(#31623,#31624,#31625,#31626));
#7369=EDGE_LOOP('',(#31627,#31628,#31629,#31630));
#7370=EDGE_LOOP('',(#31631,#31632,#31633,#31634));
#7371=EDGE_LOOP('',(#31635,#31636,#31637,#31638,#31639,#31640));
#7372=EDGE_LOOP('',(#31641,#31642,#31643,#31644));
#7373=EDGE_LOOP('',(#31645,#31646,#31647,#31648));
#7374=EDGE_LOOP('',(#31649,#31650,#31651,#31652));
#7375=EDGE_LOOP('',(#31653,#31654,#31655,#31656,#31657,#31658));
#7376=EDGE_LOOP('',(#31659,#31660,#31661,#31662));
#7377=EDGE_LOOP('',(#31663,#31664,#31665,#31666));
#7378=EDGE_LOOP('',(#31667,#31668,#31669,#31670));
#7379=EDGE_LOOP('',(#31671,#31672,#31673,#31674,#31675,#31676));
#7380=EDGE_LOOP('',(#31677,#31678,#31679,#31680));
#7381=EDGE_LOOP('',(#31681,#31682,#31683,#31684));
#7382=EDGE_LOOP('',(#31685,#31686,#31687,#31688));
#7383=EDGE_LOOP('',(#31689,#31690,#31691,#31692,#31693,#31694));
#7384=EDGE_LOOP('',(#31695,#31696,#31697,#31698));
#7385=EDGE_LOOP('',(#31699,#31700,#31701,#31702));
#7386=EDGE_LOOP('',(#31703,#31704,#31705,#31706));
#7387=EDGE_LOOP('',(#31707,#31708,#31709));
#7388=EDGE_LOOP('',(#31710,#31711,#31712,#31713,#31714,#31715));
#7389=EDGE_LOOP('',(#31716,#31717,#31718,#31719));
#7390=EDGE_LOOP('',(#31720,#31721,#31722,#31723));
#7391=EDGE_LOOP('',(#31724,#31725,#31726,#31727,#31728,#31729));
#7392=EDGE_LOOP('',(#31730,#31731,#31732,#31733));
#7393=EDGE_LOOP('',(#31734,#31735,#31736));
#7394=EDGE_LOOP('',(#31737,#31738,#31739,#31740));
#7395=EDGE_LOOP('',(#31741,#31742,#31743,#31744));
#7396=EDGE_LOOP('',(#31745,#31746,#31747,#31748,#31749,#31750));
#7397=EDGE_LOOP('',(#31751,#31752,#31753,#31754));
#7398=EDGE_LOOP('',(#31755,#31756,#31757,#31758));
#7399=EDGE_LOOP('',(#31759,#31760,#31761,#31762));
#7400=EDGE_LOOP('',(#31763,#31764,#31765,#31766,#31767,#31768));
#7401=EDGE_LOOP('',(#31769,#31770,#31771,#31772));
#7402=EDGE_LOOP('',(#31773,#31774,#31775,#31776));
#7403=EDGE_LOOP('',(#31777,#31778,#31779,#31780));
#7404=EDGE_LOOP('',(#31781,#31782,#31783,#31784,#31785,#31786));
#7405=EDGE_LOOP('',(#31787,#31788,#31789,#31790));
#7406=EDGE_LOOP('',(#31791,#31792,#31793,#31794));
#7407=EDGE_LOOP('',(#31795,#31796,#31797,#31798));
#7408=EDGE_LOOP('',(#31799,#31800,#31801,#31802,#31803,#31804));
#7409=EDGE_LOOP('',(#31805,#31806,#31807,#31808));
#7410=EDGE_LOOP('',(#31809,#31810,#31811,#31812));
#7411=EDGE_LOOP('',(#31813,#31814,#31815,#31816));
#7412=EDGE_LOOP('',(#31817,#31818,#31819,#31820,#31821,#31822));
#7413=EDGE_LOOP('',(#31823,#31824,#31825,#31826));
#7414=EDGE_LOOP('',(#31827,#31828,#31829,#31830));
#7415=EDGE_LOOP('',(#31831,#31832,#31833,#31834));
#7416=EDGE_LOOP('',(#31835,#31836,#31837));
#7417=EDGE_LOOP('',(#31838,#31839,#31840,#31841,#31842,#31843));
#7418=EDGE_LOOP('',(#31844,#31845,#31846,#31847));
#7419=EDGE_LOOP('',(#31848,#31849,#31850,#31851));
#7420=EDGE_LOOP('',(#31852,#31853,#31854,#31855,#31856,#31857));
#7421=EDGE_LOOP('',(#31858,#31859,#31860,#31861));
#7422=EDGE_LOOP('',(#31862,#31863,#31864));
#7423=EDGE_LOOP('',(#31865,#31866,#31867,#31868));
#7424=EDGE_LOOP('',(#31869,#31870,#31871,#31872));
#7425=EDGE_LOOP('',(#31873,#31874,#31875,#31876,#31877,#31878));
#7426=EDGE_LOOP('',(#31879,#31880,#31881,#31882));
#7427=EDGE_LOOP('',(#31883,#31884,#31885,#31886));
#7428=EDGE_LOOP('',(#31887,#31888,#31889,#31890));
#7429=EDGE_LOOP('',(#31891,#31892,#31893,#31894,#31895,#31896));
#7430=EDGE_LOOP('',(#31897,#31898,#31899,#31900));
#7431=EDGE_LOOP('',(#31901,#31902,#31903,#31904));
#7432=EDGE_LOOP('',(#31905,#31906,#31907,#31908));
#7433=EDGE_LOOP('',(#31909,#31910,#31911,#31912,#31913,#31914));
#7434=EDGE_LOOP('',(#31915,#31916,#31917,#31918));
#7435=EDGE_LOOP('',(#31919,#31920,#31921,#31922));
#7436=EDGE_LOOP('',(#31923,#31924,#31925,#31926));
#7437=EDGE_LOOP('',(#31927,#31928,#31929,#31930,#31931,#31932));
#7438=EDGE_LOOP('',(#31933,#31934,#31935,#31936));
#7439=EDGE_LOOP('',(#31937,#31938,#31939,#31940));
#7440=EDGE_LOOP('',(#31941,#31942,#31943,#31944));
#7441=EDGE_LOOP('',(#31945,#31946,#31947,#31948,#31949,#31950));
#7442=EDGE_LOOP('',(#31951,#31952,#31953,#31954));
#7443=EDGE_LOOP('',(#31955,#31956,#31957,#31958));
#7444=EDGE_LOOP('',(#31959,#31960,#31961,#31962));
#7445=EDGE_LOOP('',(#31963,#31964,#31965));
#7446=EDGE_LOOP('',(#31966,#31967,#31968,#31969,#31970,#31971));
#7447=EDGE_LOOP('',(#31972,#31973,#31974,#31975));
#7448=EDGE_LOOP('',(#31976,#31977,#31978,#31979));
#7449=EDGE_LOOP('',(#31980,#31981,#31982,#31983,#31984,#31985));
#7450=EDGE_LOOP('',(#31986,#31987,#31988,#31989));
#7451=EDGE_LOOP('',(#31990,#31991,#31992));
#7452=EDGE_LOOP('',(#31993,#31994,#31995,#31996));
#7453=EDGE_LOOP('',(#31997,#31998,#31999,#32000));
#7454=EDGE_LOOP('',(#32001,#32002,#32003,#32004,#32005,#32006));
#7455=EDGE_LOOP('',(#32007,#32008,#32009,#32010));
#7456=EDGE_LOOP('',(#32011,#32012,#32013,#32014));
#7457=EDGE_LOOP('',(#32015,#32016,#32017,#32018));
#7458=EDGE_LOOP('',(#32019,#32020,#32021,#32022,#32023,#32024));
#7459=EDGE_LOOP('',(#32025,#32026,#32027,#32028));
#7460=EDGE_LOOP('',(#32029,#32030,#32031,#32032));
#7461=EDGE_LOOP('',(#32033,#32034,#32035,#32036));
#7462=EDGE_LOOP('',(#32037,#32038,#32039,#32040,#32041,#32042));
#7463=EDGE_LOOP('',(#32043,#32044,#32045,#32046));
#7464=EDGE_LOOP('',(#32047,#32048,#32049,#32050));
#7465=EDGE_LOOP('',(#32051,#32052,#32053,#32054));
#7466=EDGE_LOOP('',(#32055,#32056,#32057,#32058,#32059,#32060));
#7467=EDGE_LOOP('',(#32061,#32062,#32063,#32064));
#7468=EDGE_LOOP('',(#32065,#32066,#32067,#32068));
#7469=EDGE_LOOP('',(#32069,#32070,#32071,#32072));
#7470=EDGE_LOOP('',(#32073,#32074,#32075,#32076,#32077,#32078));
#7471=EDGE_LOOP('',(#32079,#32080,#32081,#32082));
#7472=EDGE_LOOP('',(#32083,#32084,#32085,#32086));
#7473=EDGE_LOOP('',(#32087,#32088,#32089,#32090));
#7474=EDGE_LOOP('',(#32091,#32092,#32093));
#7475=EDGE_LOOP('',(#32094,#32095,#32096,#32097,#32098,#32099));
#7476=EDGE_LOOP('',(#32100,#32101,#32102,#32103));
#7477=EDGE_LOOP('',(#32104,#32105,#32106,#32107));
#7478=EDGE_LOOP('',(#32108,#32109,#32110,#32111,#32112,#32113));
#7479=EDGE_LOOP('',(#32114,#32115,#32116,#32117));
#7480=EDGE_LOOP('',(#32118,#32119,#32120));
#7481=EDGE_LOOP('',(#32121,#32122,#32123,#32124));
#7482=EDGE_LOOP('',(#32125,#32126,#32127,#32128));
#7483=EDGE_LOOP('',(#32129,#32130,#32131,#32132,#32133,#32134));
#7484=EDGE_LOOP('',(#32135,#32136,#32137,#32138));
#7485=EDGE_LOOP('',(#32139,#32140,#32141,#32142));
#7486=EDGE_LOOP('',(#32143,#32144,#32145,#32146));
#7487=EDGE_LOOP('',(#32147,#32148,#32149,#32150,#32151,#32152));
#7488=EDGE_LOOP('',(#32153,#32154,#32155,#32156));
#7489=EDGE_LOOP('',(#32157,#32158,#32159,#32160));
#7490=EDGE_LOOP('',(#32161,#32162,#32163,#32164));
#7491=EDGE_LOOP('',(#32165,#32166,#32167,#32168,#32169,#32170));
#7492=EDGE_LOOP('',(#32171,#32172,#32173,#32174));
#7493=EDGE_LOOP('',(#32175,#32176,#32177,#32178));
#7494=EDGE_LOOP('',(#32179,#32180,#32181,#32182));
#7495=EDGE_LOOP('',(#32183,#32184,#32185,#32186,#32187,#32188));
#7496=EDGE_LOOP('',(#32189,#32190,#32191,#32192));
#7497=EDGE_LOOP('',(#32193,#32194,#32195,#32196));
#7498=EDGE_LOOP('',(#32197,#32198,#32199,#32200));
#7499=EDGE_LOOP('',(#32201,#32202,#32203,#32204,#32205,#32206));
#7500=EDGE_LOOP('',(#32207,#32208,#32209,#32210));
#7501=EDGE_LOOP('',(#32211,#32212,#32213,#32214));
#7502=EDGE_LOOP('',(#32215,#32216,#32217,#32218));
#7503=EDGE_LOOP('',(#32219,#32220,#32221));
#7504=EDGE_LOOP('',(#32222,#32223,#32224,#32225,#32226,#32227));
#7505=EDGE_LOOP('',(#32228,#32229,#32230,#32231));
#7506=EDGE_LOOP('',(#32232,#32233,#32234,#32235));
#7507=EDGE_LOOP('',(#32236,#32237,#32238,#32239,#32240,#32241));
#7508=EDGE_LOOP('',(#32242,#32243,#32244,#32245));
#7509=EDGE_LOOP('',(#32246,#32247,#32248));
#7510=EDGE_LOOP('',(#32249,#32250,#32251,#32252));
#7511=EDGE_LOOP('',(#32253,#32254,#32255,#32256));
#7512=EDGE_LOOP('',(#32257,#32258,#32259,#32260,#32261,#32262));
#7513=EDGE_LOOP('',(#32263,#32264,#32265,#32266));
#7514=EDGE_LOOP('',(#32267,#32268,#32269,#32270));
#7515=EDGE_LOOP('',(#32271,#32272,#32273,#32274));
#7516=EDGE_LOOP('',(#32275,#32276,#32277,#32278,#32279,#32280));
#7517=EDGE_LOOP('',(#32281,#32282,#32283,#32284));
#7518=EDGE_LOOP('',(#32285,#32286,#32287,#32288));
#7519=EDGE_LOOP('',(#32289,#32290,#32291,#32292));
#7520=EDGE_LOOP('',(#32293,#32294,#32295,#32296,#32297,#32298));
#7521=EDGE_LOOP('',(#32299,#32300,#32301,#32302));
#7522=EDGE_LOOP('',(#32303,#32304,#32305,#32306));
#7523=EDGE_LOOP('',(#32307,#32308,#32309,#32310));
#7524=EDGE_LOOP('',(#32311,#32312,#32313,#32314,#32315,#32316));
#7525=EDGE_LOOP('',(#32317,#32318,#32319,#32320));
#7526=EDGE_LOOP('',(#32321,#32322,#32323,#32324));
#7527=EDGE_LOOP('',(#32325,#32326,#32327,#32328));
#7528=EDGE_LOOP('',(#32329,#32330,#32331,#32332,#32333,#32334));
#7529=EDGE_LOOP('',(#32335,#32336,#32337,#32338));
#7530=EDGE_LOOP('',(#32339,#32340,#32341,#32342));
#7531=EDGE_LOOP('',(#32343,#32344,#32345,#32346));
#7532=EDGE_LOOP('',(#32347,#32348,#32349));
#7533=EDGE_LOOP('',(#32350,#32351,#32352,#32353,#32354,#32355));
#7534=EDGE_LOOP('',(#32356,#32357,#32358,#32359));
#7535=EDGE_LOOP('',(#32360,#32361,#32362,#32363));
#7536=EDGE_LOOP('',(#32364,#32365,#32366,#32367,#32368,#32369));
#7537=EDGE_LOOP('',(#32370,#32371,#32372,#32373));
#7538=EDGE_LOOP('',(#32374,#32375,#32376));
#7539=EDGE_LOOP('',(#32377,#32378,#32379,#32380));
#7540=EDGE_LOOP('',(#32381,#32382,#32383,#32384));
#7541=EDGE_LOOP('',(#32385,#32386,#32387,#32388,#32389,#32390));
#7542=EDGE_LOOP('',(#32391,#32392,#32393,#32394));
#7543=EDGE_LOOP('',(#32395,#32396,#32397,#32398));
#7544=EDGE_LOOP('',(#32399,#32400,#32401,#32402));
#7545=EDGE_LOOP('',(#32403,#32404,#32405,#32406,#32407,#32408));
#7546=EDGE_LOOP('',(#32409,#32410,#32411,#32412));
#7547=EDGE_LOOP('',(#32413,#32414,#32415,#32416));
#7548=EDGE_LOOP('',(#32417,#32418,#32419,#32420));
#7549=EDGE_LOOP('',(#32421,#32422,#32423,#32424,#32425,#32426));
#7550=EDGE_LOOP('',(#32427,#32428,#32429,#32430));
#7551=EDGE_LOOP('',(#32431,#32432,#32433,#32434));
#7552=EDGE_LOOP('',(#32435,#32436,#32437,#32438));
#7553=EDGE_LOOP('',(#32439,#32440,#32441,#32442,#32443,#32444));
#7554=EDGE_LOOP('',(#32445,#32446,#32447,#32448));
#7555=EDGE_LOOP('',(#32449,#32450,#32451,#32452));
#7556=EDGE_LOOP('',(#32453,#32454,#32455,#32456));
#7557=EDGE_LOOP('',(#32457,#32458,#32459,#32460,#32461,#32462));
#7558=EDGE_LOOP('',(#32463,#32464,#32465,#32466));
#7559=EDGE_LOOP('',(#32467,#32468,#32469,#32470));
#7560=EDGE_LOOP('',(#32471,#32472,#32473,#32474));
#7561=EDGE_LOOP('',(#32475,#32476,#32477));
#7562=EDGE_LOOP('',(#32478,#32479,#32480,#32481,#32482,#32483));
#7563=EDGE_LOOP('',(#32484,#32485,#32486,#32487));
#7564=EDGE_LOOP('',(#32488,#32489,#32490,#32491));
#7565=EDGE_LOOP('',(#32492,#32493,#32494,#32495,#32496,#32497));
#7566=EDGE_LOOP('',(#32498,#32499,#32500,#32501));
#7567=EDGE_LOOP('',(#32502,#32503,#32504));
#7568=EDGE_LOOP('',(#32505,#32506,#32507,#32508));
#7569=EDGE_LOOP('',(#32509,#32510,#32511,#32512));
#7570=EDGE_LOOP('',(#32513,#32514,#32515,#32516,#32517,#32518));
#7571=EDGE_LOOP('',(#32519,#32520,#32521,#32522));
#7572=EDGE_LOOP('',(#32523,#32524,#32525,#32526));
#7573=EDGE_LOOP('',(#32527,#32528,#32529,#32530));
#7574=EDGE_LOOP('',(#32531,#32532,#32533,#32534,#32535,#32536));
#7575=EDGE_LOOP('',(#32537,#32538,#32539,#32540));
#7576=EDGE_LOOP('',(#32541,#32542,#32543,#32544));
#7577=EDGE_LOOP('',(#32545,#32546,#32547,#32548));
#7578=EDGE_LOOP('',(#32549,#32550,#32551,#32552,#32553,#32554));
#7579=EDGE_LOOP('',(#32555,#32556,#32557,#32558));
#7580=EDGE_LOOP('',(#32559,#32560,#32561,#32562));
#7581=EDGE_LOOP('',(#32563,#32564,#32565,#32566));
#7582=EDGE_LOOP('',(#32567,#32568,#32569,#32570,#32571,#32572));
#7583=EDGE_LOOP('',(#32573,#32574,#32575,#32576));
#7584=EDGE_LOOP('',(#32577,#32578,#32579,#32580));
#7585=EDGE_LOOP('',(#32581,#32582,#32583,#32584));
#7586=EDGE_LOOP('',(#32585,#32586,#32587,#32588,#32589,#32590));
#7587=EDGE_LOOP('',(#32591,#32592,#32593,#32594));
#7588=EDGE_LOOP('',(#32595,#32596,#32597,#32598));
#7589=EDGE_LOOP('',(#32599,#32600,#32601,#32602));
#7590=EDGE_LOOP('',(#32603,#32604,#32605));
#7591=EDGE_LOOP('',(#32606,#32607,#32608,#32609,#32610,#32611));
#7592=EDGE_LOOP('',(#32612,#32613,#32614,#32615));
#7593=EDGE_LOOP('',(#32616,#32617,#32618,#32619));
#7594=EDGE_LOOP('',(#32620,#32621,#32622,#32623,#32624,#32625));
#7595=EDGE_LOOP('',(#32626,#32627,#32628,#32629));
#7596=EDGE_LOOP('',(#32630,#32631,#32632));
#7597=EDGE_LOOP('',(#32633,#32634,#32635,#32636));
#7598=EDGE_LOOP('',(#32637,#32638,#32639,#32640));
#7599=EDGE_LOOP('',(#32641,#32642,#32643,#32644,#32645,#32646));
#7600=EDGE_LOOP('',(#32647,#32648,#32649,#32650));
#7601=EDGE_LOOP('',(#32651,#32652,#32653,#32654));
#7602=EDGE_LOOP('',(#32655,#32656,#32657,#32658));
#7603=EDGE_LOOP('',(#32659,#32660,#32661,#32662,#32663,#32664));
#7604=EDGE_LOOP('',(#32665,#32666,#32667,#32668));
#7605=EDGE_LOOP('',(#32669,#32670,#32671,#32672));
#7606=EDGE_LOOP('',(#32673,#32674,#32675,#32676));
#7607=EDGE_LOOP('',(#32677,#32678,#32679,#32680,#32681,#32682));
#7608=EDGE_LOOP('',(#32683,#32684,#32685,#32686));
#7609=EDGE_LOOP('',(#32687,#32688,#32689,#32690));
#7610=EDGE_LOOP('',(#32691,#32692,#32693,#32694));
#7611=EDGE_LOOP('',(#32695,#32696,#32697,#32698,#32699,#32700));
#7612=EDGE_LOOP('',(#32701,#32702,#32703,#32704));
#7613=EDGE_LOOP('',(#32705,#32706,#32707,#32708));
#7614=EDGE_LOOP('',(#32709,#32710,#32711,#32712));
#7615=EDGE_LOOP('',(#32713,#32714,#32715,#32716,#32717,#32718));
#7616=EDGE_LOOP('',(#32719,#32720,#32721,#32722));
#7617=EDGE_LOOP('',(#32723,#32724,#32725,#32726));
#7618=EDGE_LOOP('',(#32727,#32728,#32729,#32730));
#7619=EDGE_LOOP('',(#32731,#32732,#32733));
#7620=EDGE_LOOP('',(#32734,#32735,#32736,#32737,#32738,#32739));
#7621=EDGE_LOOP('',(#32740,#32741,#32742,#32743));
#7622=EDGE_LOOP('',(#32744,#32745,#32746,#32747));
#7623=EDGE_LOOP('',(#32748,#32749,#32750,#32751,#32752,#32753));
#7624=EDGE_LOOP('',(#32754,#32755,#32756,#32757));
#7625=EDGE_LOOP('',(#32758,#32759,#32760));
#7626=EDGE_LOOP('',(#32761,#32762,#32763,#32764));
#7627=EDGE_LOOP('',(#32765,#32766,#32767,#32768));
#7628=EDGE_LOOP('',(#32769,#32770,#32771,#32772,#32773,#32774));
#7629=EDGE_LOOP('',(#32775,#32776,#32777,#32778));
#7630=EDGE_LOOP('',(#32779,#32780,#32781,#32782));
#7631=EDGE_LOOP('',(#32783,#32784,#32785,#32786));
#7632=EDGE_LOOP('',(#32787,#32788,#32789,#32790,#32791,#32792));
#7633=EDGE_LOOP('',(#32793,#32794,#32795,#32796));
#7634=EDGE_LOOP('',(#32797,#32798,#32799,#32800));
#7635=EDGE_LOOP('',(#32801,#32802,#32803,#32804));
#7636=EDGE_LOOP('',(#32805,#32806,#32807,#32808,#32809,#32810));
#7637=EDGE_LOOP('',(#32811,#32812,#32813,#32814));
#7638=EDGE_LOOP('',(#32815,#32816,#32817,#32818));
#7639=EDGE_LOOP('',(#32819,#32820,#32821,#32822));
#7640=EDGE_LOOP('',(#32823,#32824,#32825,#32826,#32827,#32828));
#7641=EDGE_LOOP('',(#32829,#32830,#32831,#32832));
#7642=EDGE_LOOP('',(#32833,#32834,#32835,#32836));
#7643=EDGE_LOOP('',(#32837,#32838,#32839,#32840));
#7644=EDGE_LOOP('',(#32841,#32842,#32843,#32844,#32845,#32846));
#7645=EDGE_LOOP('',(#32847,#32848,#32849,#32850));
#7646=EDGE_LOOP('',(#32851,#32852,#32853,#32854));
#7647=EDGE_LOOP('',(#32855,#32856,#32857,#32858));
#7648=EDGE_LOOP('',(#32859,#32860,#32861));
#7649=EDGE_LOOP('',(#32862,#32863,#32864,#32865,#32866,#32867));
#7650=EDGE_LOOP('',(#32868,#32869,#32870,#32871));
#7651=EDGE_LOOP('',(#32872,#32873,#32874,#32875));
#7652=EDGE_LOOP('',(#32876,#32877,#32878,#32879,#32880,#32881));
#7653=EDGE_LOOP('',(#32882,#32883,#32884,#32885));
#7654=EDGE_LOOP('',(#32886,#32887,#32888));
#7655=EDGE_LOOP('',(#32889,#32890,#32891,#32892));
#7656=EDGE_LOOP('',(#32893,#32894,#32895,#32896));
#7657=EDGE_LOOP('',(#32897,#32898,#32899,#32900,#32901,#32902));
#7658=EDGE_LOOP('',(#32903,#32904,#32905,#32906));
#7659=EDGE_LOOP('',(#32907,#32908,#32909,#32910));
#7660=EDGE_LOOP('',(#32911,#32912,#32913,#32914));
#7661=EDGE_LOOP('',(#32915,#32916,#32917,#32918,#32919,#32920));
#7662=EDGE_LOOP('',(#32921,#32922,#32923,#32924));
#7663=EDGE_LOOP('',(#32925,#32926,#32927,#32928));
#7664=EDGE_LOOP('',(#32929,#32930,#32931,#32932));
#7665=EDGE_LOOP('',(#32933,#32934,#32935,#32936,#32937,#32938));
#7666=EDGE_LOOP('',(#32939,#32940,#32941,#32942));
#7667=EDGE_LOOP('',(#32943,#32944,#32945,#32946));
#7668=EDGE_LOOP('',(#32947,#32948,#32949,#32950));
#7669=EDGE_LOOP('',(#32951,#32952,#32953,#32954,#32955,#32956));
#7670=EDGE_LOOP('',(#32957,#32958,#32959,#32960));
#7671=EDGE_LOOP('',(#32961,#32962,#32963,#32964));
#7672=EDGE_LOOP('',(#32965,#32966,#32967,#32968));
#7673=EDGE_LOOP('',(#32969,#32970,#32971,#32972,#32973,#32974));
#7674=EDGE_LOOP('',(#32975,#32976,#32977,#32978));
#7675=EDGE_LOOP('',(#32979,#32980,#32981,#32982));
#7676=EDGE_LOOP('',(#32983,#32984,#32985,#32986));
#7677=EDGE_LOOP('',(#32987,#32988,#32989));
#7678=EDGE_LOOP('',(#32990,#32991,#32992,#32993,#32994,#32995));
#7679=EDGE_LOOP('',(#32996,#32997,#32998,#32999));
#7680=EDGE_LOOP('',(#33000,#33001,#33002,#33003));
#7681=EDGE_LOOP('',(#33004,#33005,#33006,#33007,#33008,#33009));
#7682=EDGE_LOOP('',(#33010,#33011,#33012,#33013));
#7683=EDGE_LOOP('',(#33014,#33015,#33016));
#7684=EDGE_LOOP('',(#33017,#33018,#33019,#33020));
#7685=EDGE_LOOP('',(#33021,#33022,#33023,#33024));
#7686=EDGE_LOOP('',(#33025,#33026,#33027,#33028,#33029,#33030));
#7687=EDGE_LOOP('',(#33031,#33032,#33033,#33034));
#7688=EDGE_LOOP('',(#33035,#33036,#33037,#33038));
#7689=EDGE_LOOP('',(#33039,#33040,#33041,#33042));
#7690=EDGE_LOOP('',(#33043,#33044,#33045,#33046,#33047,#33048));
#7691=EDGE_LOOP('',(#33049,#33050,#33051,#33052));
#7692=EDGE_LOOP('',(#33053,#33054,#33055,#33056));
#7693=EDGE_LOOP('',(#33057,#33058,#33059,#33060));
#7694=EDGE_LOOP('',(#33061,#33062,#33063,#33064,#33065,#33066));
#7695=EDGE_LOOP('',(#33067,#33068,#33069,#33070));
#7696=EDGE_LOOP('',(#33071,#33072,#33073,#33074));
#7697=EDGE_LOOP('',(#33075,#33076,#33077,#33078));
#7698=EDGE_LOOP('',(#33079,#33080,#33081,#33082,#33083,#33084));
#7699=EDGE_LOOP('',(#33085,#33086,#33087,#33088));
#7700=EDGE_LOOP('',(#33089,#33090,#33091,#33092));
#7701=EDGE_LOOP('',(#33093,#33094,#33095,#33096));
#7702=EDGE_LOOP('',(#33097,#33098,#33099,#33100,#33101,#33102));
#7703=EDGE_LOOP('',(#33103,#33104,#33105,#33106));
#7704=EDGE_LOOP('',(#33107,#33108,#33109,#33110));
#7705=EDGE_LOOP('',(#33111,#33112,#33113,#33114));
#7706=EDGE_LOOP('',(#33115,#33116,#33117));
#7707=EDGE_LOOP('',(#33118,#33119,#33120,#33121,#33122,#33123));
#7708=EDGE_LOOP('',(#33124,#33125,#33126,#33127));
#7709=EDGE_LOOP('',(#33128,#33129,#33130,#33131));
#7710=EDGE_LOOP('',(#33132,#33133,#33134,#33135,#33136,#33137));
#7711=EDGE_LOOP('',(#33138,#33139,#33140,#33141));
#7712=EDGE_LOOP('',(#33142,#33143,#33144));
#7713=EDGE_LOOP('',(#33145,#33146,#33147,#33148));
#7714=EDGE_LOOP('',(#33149,#33150,#33151,#33152));
#7715=EDGE_LOOP('',(#33153,#33154,#33155,#33156,#33157,#33158));
#7716=EDGE_LOOP('',(#33159,#33160,#33161,#33162));
#7717=EDGE_LOOP('',(#33163,#33164,#33165,#33166));
#7718=EDGE_LOOP('',(#33167,#33168,#33169,#33170));
#7719=EDGE_LOOP('',(#33171,#33172,#33173,#33174,#33175,#33176));
#7720=EDGE_LOOP('',(#33177,#33178,#33179,#33180));
#7721=EDGE_LOOP('',(#33181,#33182,#33183,#33184));
#7722=EDGE_LOOP('',(#33185,#33186,#33187,#33188));
#7723=EDGE_LOOP('',(#33189,#33190,#33191,#33192,#33193,#33194));
#7724=EDGE_LOOP('',(#33195,#33196,#33197,#33198));
#7725=EDGE_LOOP('',(#33199,#33200,#33201,#33202));
#7726=EDGE_LOOP('',(#33203,#33204,#33205,#33206));
#7727=EDGE_LOOP('',(#33207,#33208,#33209,#33210,#33211,#33212));
#7728=EDGE_LOOP('',(#33213,#33214,#33215,#33216));
#7729=EDGE_LOOP('',(#33217,#33218,#33219,#33220));
#7730=EDGE_LOOP('',(#33221,#33222,#33223,#33224));
#7731=EDGE_LOOP('',(#33225,#33226,#33227,#33228,#33229,#33230));
#7732=EDGE_LOOP('',(#33231,#33232,#33233,#33234));
#7733=EDGE_LOOP('',(#33235,#33236,#33237,#33238));
#7734=EDGE_LOOP('',(#33239,#33240,#33241,#33242));
#7735=EDGE_LOOP('',(#33243,#33244,#33245));
#7736=EDGE_LOOP('',(#33246,#33247,#33248,#33249,#33250,#33251));
#7737=EDGE_LOOP('',(#33252,#33253,#33254,#33255));
#7738=EDGE_LOOP('',(#33256,#33257,#33258,#33259));
#7739=EDGE_LOOP('',(#33260,#33261,#33262,#33263,#33264,#33265));
#7740=EDGE_LOOP('',(#33266,#33267,#33268,#33269));
#7741=EDGE_LOOP('',(#33270,#33271,#33272));
#7742=EDGE_LOOP('',(#33273,#33274,#33275,#33276));
#7743=EDGE_LOOP('',(#33277,#33278,#33279,#33280));
#7744=EDGE_LOOP('',(#33281,#33282,#33283,#33284,#33285,#33286));
#7745=EDGE_LOOP('',(#33287,#33288,#33289,#33290));
#7746=EDGE_LOOP('',(#33291,#33292,#33293,#33294));
#7747=EDGE_LOOP('',(#33295,#33296,#33297,#33298));
#7748=EDGE_LOOP('',(#33299,#33300,#33301,#33302,#33303,#33304));
#7749=EDGE_LOOP('',(#33305,#33306,#33307,#33308));
#7750=EDGE_LOOP('',(#33309,#33310,#33311,#33312));
#7751=EDGE_LOOP('',(#33313,#33314,#33315,#33316));
#7752=EDGE_LOOP('',(#33317,#33318,#33319,#33320,#33321,#33322));
#7753=EDGE_LOOP('',(#33323,#33324,#33325,#33326));
#7754=EDGE_LOOP('',(#33327,#33328,#33329,#33330));
#7755=EDGE_LOOP('',(#33331,#33332,#33333,#33334));
#7756=EDGE_LOOP('',(#33335,#33336,#33337,#33338,#33339,#33340));
#7757=EDGE_LOOP('',(#33341,#33342,#33343,#33344));
#7758=EDGE_LOOP('',(#33345,#33346,#33347,#33348));
#7759=EDGE_LOOP('',(#33349,#33350,#33351,#33352));
#7760=EDGE_LOOP('',(#33353,#33354,#33355,#33356,#33357,#33358));
#7761=EDGE_LOOP('',(#33359,#33360,#33361,#33362));
#7762=EDGE_LOOP('',(#33363,#33364,#33365,#33366));
#7763=EDGE_LOOP('',(#33367,#33368,#33369,#33370));
#7764=EDGE_LOOP('',(#33371,#33372,#33373));
#7765=EDGE_LOOP('',(#33374,#33375,#33376,#33377,#33378,#33379));
#7766=EDGE_LOOP('',(#33380,#33381,#33382,#33383));
#7767=EDGE_LOOP('',(#33384,#33385,#33386,#33387));
#7768=EDGE_LOOP('',(#33388,#33389,#33390,#33391,#33392,#33393));
#7769=EDGE_LOOP('',(#33394,#33395,#33396,#33397));
#7770=EDGE_LOOP('',(#33398,#33399,#33400));
#7771=EDGE_LOOP('',(#33401,#33402,#33403,#33404));
#7772=EDGE_LOOP('',(#33405,#33406,#33407,#33408));
#7773=EDGE_LOOP('',(#33409,#33410,#33411,#33412,#33413,#33414));
#7774=EDGE_LOOP('',(#33415,#33416,#33417,#33418));
#7775=EDGE_LOOP('',(#33419,#33420,#33421,#33422));
#7776=EDGE_LOOP('',(#33423,#33424,#33425,#33426));
#7777=EDGE_LOOP('',(#33427,#33428,#33429,#33430,#33431,#33432));
#7778=EDGE_LOOP('',(#33433,#33434,#33435,#33436));
#7779=EDGE_LOOP('',(#33437,#33438,#33439,#33440));
#7780=EDGE_LOOP('',(#33441,#33442,#33443,#33444));
#7781=EDGE_LOOP('',(#33445,#33446,#33447,#33448,#33449,#33450));
#7782=EDGE_LOOP('',(#33451,#33452,#33453,#33454));
#7783=EDGE_LOOP('',(#33455,#33456,#33457,#33458));
#7784=EDGE_LOOP('',(#33459,#33460,#33461,#33462));
#7785=EDGE_LOOP('',(#33463,#33464,#33465,#33466,#33467,#33468));
#7786=EDGE_LOOP('',(#33469,#33470,#33471,#33472));
#7787=EDGE_LOOP('',(#33473,#33474,#33475,#33476));
#7788=EDGE_LOOP('',(#33477,#33478,#33479,#33480));
#7789=EDGE_LOOP('',(#33481,#33482,#33483,#33484,#33485,#33486));
#7790=EDGE_LOOP('',(#33487,#33488,#33489,#33490));
#7791=EDGE_LOOP('',(#33491,#33492,#33493,#33494));
#7792=EDGE_LOOP('',(#33495,#33496,#33497,#33498));
#7793=EDGE_LOOP('',(#33499,#33500,#33501));
#7794=EDGE_LOOP('',(#33502,#33503,#33504,#33505,#33506,#33507));
#7795=EDGE_LOOP('',(#33508,#33509,#33510,#33511));
#7796=EDGE_LOOP('',(#33512,#33513,#33514,#33515));
#7797=EDGE_LOOP('',(#33516,#33517,#33518,#33519,#33520,#33521));
#7798=EDGE_LOOP('',(#33522,#33523,#33524,#33525));
#7799=EDGE_LOOP('',(#33526,#33527,#33528));
#7800=EDGE_LOOP('',(#33529,#33530,#33531,#33532));
#7801=EDGE_LOOP('',(#33533,#33534,#33535,#33536));
#7802=EDGE_LOOP('',(#33537,#33538,#33539,#33540,#33541,#33542));
#7803=EDGE_LOOP('',(#33543,#33544,#33545,#33546));
#7804=EDGE_LOOP('',(#33547,#33548,#33549,#33550));
#7805=EDGE_LOOP('',(#33551,#33552,#33553,#33554));
#7806=EDGE_LOOP('',(#33555,#33556,#33557,#33558,#33559,#33560));
#7807=EDGE_LOOP('',(#33561,#33562,#33563,#33564));
#7808=EDGE_LOOP('',(#33565,#33566,#33567,#33568));
#7809=EDGE_LOOP('',(#33569,#33570,#33571,#33572));
#7810=EDGE_LOOP('',(#33573,#33574,#33575,#33576,#33577,#33578));
#7811=EDGE_LOOP('',(#33579,#33580,#33581,#33582));
#7812=EDGE_LOOP('',(#33583,#33584,#33585,#33586));
#7813=EDGE_LOOP('',(#33587,#33588,#33589,#33590));
#7814=EDGE_LOOP('',(#33591,#33592,#33593,#33594,#33595,#33596));
#7815=EDGE_LOOP('',(#33597,#33598,#33599,#33600));
#7816=EDGE_LOOP('',(#33601,#33602,#33603,#33604));
#7817=EDGE_LOOP('',(#33605,#33606,#33607,#33608));
#7818=EDGE_LOOP('',(#33609,#33610,#33611,#33612,#33613,#33614));
#7819=EDGE_LOOP('',(#33615,#33616,#33617,#33618));
#7820=EDGE_LOOP('',(#33619,#33620,#33621,#33622));
#7821=EDGE_LOOP('',(#33623,#33624,#33625,#33626));
#7822=EDGE_LOOP('',(#33627,#33628,#33629));
#7823=EDGE_LOOP('',(#33630,#33631,#33632,#33633,#33634,#33635));
#7824=EDGE_LOOP('',(#33636,#33637,#33638,#33639));
#7825=EDGE_LOOP('',(#33640,#33641,#33642,#33643));
#7826=EDGE_LOOP('',(#33644,#33645,#33646,#33647,#33648,#33649));
#7827=EDGE_LOOP('',(#33650,#33651,#33652,#33653));
#7828=EDGE_LOOP('',(#33654,#33655,#33656));
#7829=EDGE_LOOP('',(#33657,#33658,#33659,#33660));
#7830=EDGE_LOOP('',(#33661,#33662,#33663,#33664));
#7831=EDGE_LOOP('',(#33665,#33666,#33667,#33668,#33669,#33670));
#7832=EDGE_LOOP('',(#33671,#33672,#33673,#33674));
#7833=EDGE_LOOP('',(#33675,#33676,#33677,#33678));
#7834=EDGE_LOOP('',(#33679,#33680,#33681,#33682));
#7835=EDGE_LOOP('',(#33683,#33684,#33685,#33686,#33687,#33688));
#7836=EDGE_LOOP('',(#33689,#33690,#33691,#33692));
#7837=EDGE_LOOP('',(#33693,#33694,#33695,#33696));
#7838=EDGE_LOOP('',(#33697,#33698,#33699,#33700));
#7839=EDGE_LOOP('',(#33701,#33702,#33703,#33704,#33705,#33706));
#7840=EDGE_LOOP('',(#33707,#33708,#33709,#33710));
#7841=EDGE_LOOP('',(#33711,#33712,#33713,#33714));
#7842=EDGE_LOOP('',(#33715,#33716,#33717,#33718));
#7843=EDGE_LOOP('',(#33719,#33720,#33721,#33722,#33723,#33724));
#7844=EDGE_LOOP('',(#33725,#33726,#33727,#33728));
#7845=EDGE_LOOP('',(#33729,#33730,#33731,#33732));
#7846=EDGE_LOOP('',(#33733,#33734,#33735,#33736));
#7847=EDGE_LOOP('',(#33737,#33738,#33739,#33740,#33741,#33742));
#7848=EDGE_LOOP('',(#33743,#33744,#33745,#33746));
#7849=EDGE_LOOP('',(#33747,#33748,#33749,#33750));
#7850=EDGE_LOOP('',(#33751,#33752,#33753,#33754));
#7851=EDGE_LOOP('',(#33755,#33756,#33757));
#7852=EDGE_LOOP('',(#33758,#33759,#33760,#33761,#33762,#33763));
#7853=EDGE_LOOP('',(#33764,#33765,#33766,#33767));
#7854=EDGE_LOOP('',(#33768,#33769,#33770,#33771));
#7855=EDGE_LOOP('',(#33772,#33773,#33774,#33775,#33776,#33777));
#7856=EDGE_LOOP('',(#33778,#33779,#33780,#33781));
#7857=EDGE_LOOP('',(#33782,#33783,#33784));
#7858=EDGE_LOOP('',(#33785,#33786,#33787,#33788));
#7859=EDGE_LOOP('',(#33789,#33790,#33791,#33792));
#7860=EDGE_LOOP('',(#33793,#33794,#33795,#33796,#33797,#33798));
#7861=EDGE_LOOP('',(#33799,#33800,#33801,#33802));
#7862=EDGE_LOOP('',(#33803,#33804,#33805,#33806));
#7863=EDGE_LOOP('',(#33807,#33808,#33809,#33810));
#7864=EDGE_LOOP('',(#33811,#33812,#33813,#33814,#33815,#33816));
#7865=EDGE_LOOP('',(#33817,#33818,#33819,#33820));
#7866=EDGE_LOOP('',(#33821,#33822,#33823,#33824));
#7867=EDGE_LOOP('',(#33825,#33826,#33827,#33828));
#7868=EDGE_LOOP('',(#33829,#33830,#33831,#33832,#33833,#33834));
#7869=EDGE_LOOP('',(#33835,#33836,#33837,#33838));
#7870=EDGE_LOOP('',(#33839,#33840,#33841,#33842));
#7871=EDGE_LOOP('',(#33843,#33844,#33845,#33846));
#7872=EDGE_LOOP('',(#33847,#33848,#33849,#33850,#33851,#33852));
#7873=EDGE_LOOP('',(#33853,#33854,#33855,#33856));
#7874=EDGE_LOOP('',(#33857,#33858,#33859,#33860));
#7875=EDGE_LOOP('',(#33861,#33862,#33863,#33864));
#7876=EDGE_LOOP('',(#33865,#33866,#33867,#33868,#33869,#33870));
#7877=EDGE_LOOP('',(#33871,#33872,#33873,#33874));
#7878=EDGE_LOOP('',(#33875,#33876,#33877,#33878));
#7879=EDGE_LOOP('',(#33879,#33880,#33881,#33882));
#7880=EDGE_LOOP('',(#33883,#33884,#33885));
#7881=EDGE_LOOP('',(#33886,#33887,#33888,#33889,#33890,#33891));
#7882=EDGE_LOOP('',(#33892,#33893,#33894,#33895));
#7883=EDGE_LOOP('',(#33896,#33897,#33898,#33899));
#7884=EDGE_LOOP('',(#33900,#33901,#33902,#33903,#33904,#33905));
#7885=EDGE_LOOP('',(#33906,#33907,#33908,#33909));
#7886=EDGE_LOOP('',(#33910,#33911,#33912));
#7887=EDGE_LOOP('',(#33913,#33914,#33915,#33916));
#7888=EDGE_LOOP('',(#33917,#33918,#33919,#33920));
#7889=EDGE_LOOP('',(#33921,#33922,#33923,#33924,#33925,#33926));
#7890=EDGE_LOOP('',(#33927,#33928,#33929,#33930));
#7891=EDGE_LOOP('',(#33931,#33932,#33933,#33934));
#7892=EDGE_LOOP('',(#33935,#33936,#33937,#33938));
#7893=EDGE_LOOP('',(#33939,#33940,#33941,#33942,#33943,#33944));
#7894=EDGE_LOOP('',(#33945,#33946,#33947,#33948));
#7895=EDGE_LOOP('',(#33949,#33950,#33951,#33952));
#7896=EDGE_LOOP('',(#33953,#33954,#33955,#33956));
#7897=EDGE_LOOP('',(#33957,#33958,#33959,#33960,#33961,#33962));
#7898=EDGE_LOOP('',(#33963,#33964,#33965,#33966));
#7899=EDGE_LOOP('',(#33967,#33968,#33969,#33970));
#7900=EDGE_LOOP('',(#33971,#33972,#33973,#33974));
#7901=EDGE_LOOP('',(#33975,#33976,#33977,#33978,#33979,#33980));
#7902=EDGE_LOOP('',(#33981,#33982,#33983,#33984));
#7903=EDGE_LOOP('',(#33985,#33986,#33987,#33988));
#7904=EDGE_LOOP('',(#33989,#33990,#33991,#33992));
#7905=EDGE_LOOP('',(#33993,#33994,#33995,#33996,#33997,#33998));
#7906=EDGE_LOOP('',(#33999,#34000,#34001,#34002));
#7907=EDGE_LOOP('',(#34003,#34004,#34005,#34006));
#7908=EDGE_LOOP('',(#34007,#34008,#34009,#34010));
#7909=EDGE_LOOP('',(#34011,#34012,#34013));
#7910=EDGE_LOOP('',(#34014,#34015,#34016,#34017,#34018,#34019));
#7911=EDGE_LOOP('',(#34020,#34021,#34022,#34023));
#7912=EDGE_LOOP('',(#34024,#34025,#34026,#34027));
#7913=EDGE_LOOP('',(#34028,#34029,#34030,#34031,#34032,#34033));
#7914=EDGE_LOOP('',(#34034,#34035,#34036,#34037));
#7915=EDGE_LOOP('',(#34038,#34039,#34040));
#7916=EDGE_LOOP('',(#34041,#34042,#34043,#34044));
#7917=EDGE_LOOP('',(#34045,#34046,#34047,#34048));
#7918=EDGE_LOOP('',(#34049,#34050,#34051,#34052,#34053,#34054));
#7919=EDGE_LOOP('',(#34055,#34056,#34057,#34058));
#7920=EDGE_LOOP('',(#34059,#34060,#34061,#34062));
#7921=EDGE_LOOP('',(#34063,#34064,#34065,#34066));
#7922=EDGE_LOOP('',(#34067,#34068,#34069,#34070,#34071,#34072));
#7923=EDGE_LOOP('',(#34073,#34074,#34075,#34076));
#7924=EDGE_LOOP('',(#34077,#34078,#34079,#34080));
#7925=EDGE_LOOP('',(#34081,#34082,#34083,#34084));
#7926=EDGE_LOOP('',(#34085,#34086,#34087,#34088,#34089,#34090));
#7927=EDGE_LOOP('',(#34091,#34092,#34093,#34094));
#7928=EDGE_LOOP('',(#34095,#34096,#34097,#34098));
#7929=EDGE_LOOP('',(#34099,#34100,#34101,#34102));
#7930=EDGE_LOOP('',(#34103,#34104,#34105,#34106,#34107,#34108));
#7931=EDGE_LOOP('',(#34109,#34110,#34111,#34112));
#7932=EDGE_LOOP('',(#34113,#34114,#34115,#34116));
#7933=EDGE_LOOP('',(#34117,#34118,#34119,#34120));
#7934=EDGE_LOOP('',(#34121,#34122,#34123,#34124,#34125,#34126));
#7935=EDGE_LOOP('',(#34127,#34128,#34129,#34130));
#7936=EDGE_LOOP('',(#34131,#34132,#34133,#34134));
#7937=EDGE_LOOP('',(#34135,#34136,#34137,#34138));
#7938=EDGE_LOOP('',(#34139,#34140,#34141));
#7939=EDGE_LOOP('',(#34142,#34143,#34144,#34145,#34146,#34147));
#7940=EDGE_LOOP('',(#34148,#34149,#34150,#34151));
#7941=EDGE_LOOP('',(#34152,#34153,#34154,#34155));
#7942=EDGE_LOOP('',(#34156,#34157,#34158,#34159,#34160,#34161));
#7943=EDGE_LOOP('',(#34162,#34163,#34164,#34165));
#7944=EDGE_LOOP('',(#34166,#34167,#34168));
#7945=EDGE_LOOP('',(#34169,#34170,#34171,#34172));
#7946=EDGE_LOOP('',(#34173,#34174,#34175,#34176));
#7947=EDGE_LOOP('',(#34177,#34178,#34179,#34180,#34181,#34182));
#7948=EDGE_LOOP('',(#34183,#34184,#34185,#34186));
#7949=EDGE_LOOP('',(#34187,#34188,#34189,#34190));
#7950=EDGE_LOOP('',(#34191,#34192,#34193,#34194));
#7951=EDGE_LOOP('',(#34195,#34196,#34197,#34198,#34199,#34200));
#7952=EDGE_LOOP('',(#34201,#34202,#34203,#34204));
#7953=EDGE_LOOP('',(#34205,#34206,#34207,#34208));
#7954=EDGE_LOOP('',(#34209,#34210,#34211,#34212));
#7955=EDGE_LOOP('',(#34213,#34214,#34215,#34216,#34217,#34218));
#7956=EDGE_LOOP('',(#34219,#34220,#34221,#34222));
#7957=EDGE_LOOP('',(#34223,#34224,#34225,#34226));
#7958=EDGE_LOOP('',(#34227,#34228,#34229,#34230));
#7959=EDGE_LOOP('',(#34231,#34232,#34233,#34234,#34235,#34236));
#7960=EDGE_LOOP('',(#34237,#34238,#34239,#34240));
#7961=EDGE_LOOP('',(#34241,#34242,#34243,#34244));
#7962=EDGE_LOOP('',(#34245,#34246,#34247,#34248));
#7963=EDGE_LOOP('',(#34249,#34250,#34251,#34252,#34253,#34254));
#7964=EDGE_LOOP('',(#34255,#34256,#34257,#34258));
#7965=EDGE_LOOP('',(#34259,#34260,#34261,#34262));
#7966=EDGE_LOOP('',(#34263,#34264,#34265,#34266));
#7967=EDGE_LOOP('',(#34267,#34268,#34269));
#7968=EDGE_LOOP('',(#34270,#34271,#34272,#34273,#34274,#34275));
#7969=EDGE_LOOP('',(#34276,#34277,#34278,#34279));
#7970=EDGE_LOOP('',(#34280,#34281,#34282,#34283));
#7971=EDGE_LOOP('',(#34284,#34285,#34286,#34287,#34288,#34289));
#7972=EDGE_LOOP('',(#34290,#34291,#34292,#34293));
#7973=EDGE_LOOP('',(#34294,#34295,#34296));
#7974=EDGE_LOOP('',(#34297,#34298,#34299,#34300));
#7975=EDGE_LOOP('',(#34301,#34302,#34303,#34304));
#7976=EDGE_LOOP('',(#34305,#34306,#34307,#34308,#34309,#34310));
#7977=EDGE_LOOP('',(#34311,#34312,#34313,#34314));
#7978=EDGE_LOOP('',(#34315,#34316,#34317,#34318));
#7979=EDGE_LOOP('',(#34319,#34320,#34321,#34322));
#7980=EDGE_LOOP('',(#34323,#34324,#34325,#34326,#34327,#34328));
#7981=EDGE_LOOP('',(#34329,#34330,#34331,#34332));
#7982=EDGE_LOOP('',(#34333,#34334,#34335,#34336));
#7983=EDGE_LOOP('',(#34337,#34338,#34339,#34340));
#7984=EDGE_LOOP('',(#34341,#34342,#34343,#34344,#34345,#34346));
#7985=EDGE_LOOP('',(#34347,#34348,#34349,#34350));
#7986=EDGE_LOOP('',(#34351,#34352,#34353,#34354));
#7987=EDGE_LOOP('',(#34355,#34356,#34357,#34358));
#7988=EDGE_LOOP('',(#34359,#34360,#34361,#34362,#34363,#34364));
#7989=EDGE_LOOP('',(#34365,#34366,#34367,#34368));
#7990=EDGE_LOOP('',(#34369,#34370,#34371,#34372));
#7991=EDGE_LOOP('',(#34373,#34374,#34375,#34376));
#7992=EDGE_LOOP('',(#34377,#34378,#34379,#34380,#34381,#34382));
#7993=EDGE_LOOP('',(#34383,#34384,#34385,#34386));
#7994=EDGE_LOOP('',(#34387,#34388,#34389,#34390));
#7995=EDGE_LOOP('',(#34391,#34392,#34393,#34394));
#7996=EDGE_LOOP('',(#34395,#34396,#34397));
#7997=EDGE_LOOP('',(#34398,#34399,#34400,#34401));
#7998=EDGE_LOOP('',(#34402,#34403,#34404,#34405,#34406,#34407));
#7999=EDGE_LOOP('',(#34408,#34409,#34410,#34411));
#8000=EDGE_LOOP('',(#34412,#34413,#34414,#34415,#34416,#34417));
#8001=EDGE_LOOP('',(#34418,#34419,#34420,#34421));
#8002=EDGE_LOOP('',(#34422,#34423,#34424));
#8003=EDGE_LOOP('',(#34425,#34426,#34427,#34428));
#8004=EDGE_LOOP('',(#34429,#34430,#34431,#34432));
#8005=EDGE_LOOP('',(#34433,#34434,#34435,#34436,#34437,#34438));
#8006=EDGE_LOOP('',(#34439,#34440,#34441,#34442));
#8007=EDGE_LOOP('',(#34443,#34444,#34445,#34446));
#8008=EDGE_LOOP('',(#34447,#34448,#34449,#34450));
#8009=EDGE_LOOP('',(#34451,#34452,#34453,#34454,#34455,#34456));
#8010=EDGE_LOOP('',(#34457,#34458,#34459,#34460));
#8011=EDGE_LOOP('',(#34461,#34462,#34463,#34464));
#8012=EDGE_LOOP('',(#34465,#34466,#34467,#34468));
#8013=EDGE_LOOP('',(#34469,#34470,#34471,#34472,#34473,#34474));
#8014=EDGE_LOOP('',(#34475,#34476,#34477,#34478));
#8015=EDGE_LOOP('',(#34479,#34480,#34481,#34482));
#8016=EDGE_LOOP('',(#34483,#34484,#34485,#34486));
#8017=EDGE_LOOP('',(#34487,#34488,#34489,#34490,#34491,#34492));
#8018=EDGE_LOOP('',(#34493,#34494,#34495,#34496));
#8019=EDGE_LOOP('',(#34497,#34498,#34499,#34500));
#8020=EDGE_LOOP('',(#34501,#34502,#34503,#34504));
#8021=EDGE_LOOP('',(#34505,#34506,#34507,#34508,#34509,#34510));
#8022=EDGE_LOOP('',(#34511,#34512,#34513,#34514));
#8023=EDGE_LOOP('',(#34515,#34516,#34517,#34518));
#8024=EDGE_LOOP('',(#34519,#34520,#34521,#34522));
#8025=EDGE_LOOP('',(#34523,#34524,#34525));
#8026=EDGE_LOOP('',(#34526,#34527,#34528,#34529));
#8027=EDGE_LOOP('',(#34530,#34531,#34532,#34533));
#8028=EDGE_LOOP('',(#34534,#34535,#34536,#34537,#34538,#34539));
#8029=EDGE_LOOP('',(#34540,#34541,#34542,#34543));
#8030=EDGE_LOOP('',(#34544,#34545,#34546,#34547,#34548,#34549));
#8031=EDGE_LOOP('',(#34550,#34551,#34552,#34553));
#8032=EDGE_LOOP('',(#34554,#34555,#34556));
#8033=EDGE_LOOP('',(#34557,#34558,#34559,#34560));
#8034=EDGE_LOOP('',(#34561,#34562,#34563,#34564,#34565,#34566));
#8035=EDGE_LOOP('',(#34567,#34568,#34569,#34570));
#8036=EDGE_LOOP('',(#34571,#34572,#34573,#34574));
#8037=EDGE_LOOP('',(#34575,#34576,#34577,#34578));
#8038=EDGE_LOOP('',(#34579,#34580,#34581,#34582,#34583,#34584));
#8039=EDGE_LOOP('',(#34585,#34586,#34587,#34588));
#8040=EDGE_LOOP('',(#34589,#34590,#34591,#34592));
#8041=EDGE_LOOP('',(#34593,#34594,#34595,#34596));
#8042=EDGE_LOOP('',(#34597,#34598,#34599,#34600,#34601,#34602));
#8043=EDGE_LOOP('',(#34603,#34604,#34605,#34606));
#8044=EDGE_LOOP('',(#34607,#34608,#34609,#34610));
#8045=EDGE_LOOP('',(#34611,#34612,#34613,#34614));
#8046=EDGE_LOOP('',(#34615,#34616,#34617,#34618,#34619,#34620));
#8047=EDGE_LOOP('',(#34621,#34622,#34623,#34624));
#8048=EDGE_LOOP('',(#34625,#34626,#34627,#34628));
#8049=EDGE_LOOP('',(#34629,#34630,#34631,#34632));
#8050=EDGE_LOOP('',(#34633,#34634,#34635,#34636,#34637,#34638));
#8051=EDGE_LOOP('',(#34639,#34640,#34641,#34642));
#8052=EDGE_LOOP('',(#34643,#34644,#34645,#34646));
#8053=EDGE_LOOP('',(#34647,#34648,#34649,#34650));
#8054=EDGE_LOOP('',(#34651,#34652,#34653));
#8055=EDGE_LOOP('',(#34654,#34655,#34656,#34657));
#8056=EDGE_LOOP('',(#34658,#34659,#34660,#34661));
#8057=EDGE_LOOP('',(#34662,#34663,#34664,#34665));
#8058=EDGE_LOOP('',(#34666,#34667,#34668,#34669,#34670,#34671));
#8059=EDGE_LOOP('',(#34672,#34673,#34674,#34675));
#8060=EDGE_LOOP('',(#34676,#34677,#34678));
#8061=EDGE_LOOP('',(#34679,#34680,#34681,#34682));
#8062=EDGE_LOOP('',(#34683,#34684,#34685,#34686,#34687,#34688));
#8063=EDGE_LOOP('',(#34689,#34690,#34691,#34692));
#8064=EDGE_LOOP('',(#34693,#34694,#34695,#34696));
#8065=EDGE_LOOP('',(#34697,#34698,#34699,#34700,#34701,#34702));
#8066=EDGE_LOOP('',(#34703,#34704,#34705,#34706));
#8067=EDGE_LOOP('',(#34707,#34708,#34709,#34710));
#8068=EDGE_LOOP('',(#34711,#34712,#34713,#34714,#34715,#34716));
#8069=EDGE_LOOP('',(#34717,#34718,#34719,#34720));
#8070=EDGE_LOOP('',(#34721,#34722,#34723,#34724));
#8071=EDGE_LOOP('',(#34725,#34726,#34727,#34728,#34729,#34730));
#8072=EDGE_LOOP('',(#34731,#34732,#34733,#34734));
#8073=EDGE_LOOP('',(#34735,#34736,#34737,#34738));
#8074=EDGE_LOOP('',(#34739,#34740,#34741,#34742));
#8075=EDGE_LOOP('',(#34743,#34744,#34745,#34746,#34747,#34748));
#8076=EDGE_LOOP('',(#34749,#34750,#34751,#34752));
#8077=EDGE_LOOP('',(#34753,#34754,#34755,#34756));
#8078=EDGE_LOOP('',(#34757,#34758,#34759,#34760));
#8079=EDGE_LOOP('',(#34761,#34762,#34763,#34764,#34765,#34766));
#8080=EDGE_LOOP('',(#34767,#34768,#34769,#34770));
#8081=EDGE_LOOP('',(#34771,#34772,#34773,#34774));
#8082=EDGE_LOOP('',(#34775,#34776,#34777,#34778));
#8083=EDGE_LOOP('',(#34779,#34780,#34781));
#8084=EDGE_LOOP('',(#34782,#34783,#34784,#34785));
#8085=EDGE_LOOP('',(#34786,#34787,#34788,#34789));
#8086=EDGE_LOOP('',(#34790,#34791,#34792,#34793));
#8087=EDGE_LOOP('',(#34794,#34795,#34796,#34797));
#8088=EDGE_LOOP('',(#34798,#34799,#34800,#34801,#34802,#34803));
#8089=EDGE_LOOP('',(#34804,#34805,#34806,#34807));
#8090=EDGE_LOOP('',(#34808,#34809,#34810,#34811));
#8091=EDGE_LOOP('',(#34812,#34813,#34814,#34815,#34816,#34817));
#8092=EDGE_LOOP('',(#34818,#34819,#34820,#34821));
#8093=EDGE_LOOP('',(#34822,#34823,#34824,#34825));
#8094=EDGE_LOOP('',(#34826,#34827,#34828,#34829,#34830,#34831));
#8095=EDGE_LOOP('',(#34832,#34833,#34834,#34835));
#8096=EDGE_LOOP('',(#34836,#34837,#34838,#34839));
#8097=EDGE_LOOP('',(#34840,#34841,#34842,#34843,#34844,#34845));
#8098=EDGE_LOOP('',(#34846,#34847,#34848,#34849));
#8099=EDGE_LOOP('',(#34850,#34851,#34852,#34853,#34854,#34855));
#8100=EDGE_LOOP('',(#34856,#34857,#34858,#34859));
#8101=EDGE_LOOP('',(#34860,#34861,#34862));
#8102=EDGE_LOOP('',(#34863,#34864,#34865,#34866));
#8103=EDGE_LOOP('',(#34867,#34868,#34869,#34870));
#8104=EDGE_LOOP('',(#34871,#34872,#34873,#34874,#34875,#34876));
#8105=EDGE_LOOP('',(#34877,#34878,#34879,#34880));
#8106=EDGE_LOOP('',(#34881,#34882,#34883,#34884));
#8107=EDGE_LOOP('',(#34885,#34886,#34887,#34888));
#8108=EDGE_LOOP('',(#34889,#34890,#34891,#34892,#34893,#34894));
#8109=EDGE_LOOP('',(#34895,#34896,#34897,#34898));
#8110=EDGE_LOOP('',(#34899,#34900,#34901,#34902));
#8111=EDGE_LOOP('',(#34903,#34904,#34905,#34906));
#8112=EDGE_LOOP('',(#34907,#34908,#34909));
#8113=EDGE_LOOP('',(#34910,#34911,#34912,#34913));
#8114=EDGE_LOOP('',(#34914,#34915,#34916,#34917));
#8115=EDGE_LOOP('',(#34918,#34919,#34920,#34921));
#8116=EDGE_LOOP('',(#34922,#34923,#34924,#34925));
#8117=EDGE_LOOP('',(#34926,#34927,#34928,#34929));
#8118=EDGE_LOOP('',(#34930,#34931,#34932,#34933,#34934,#34935));
#8119=EDGE_LOOP('',(#34936,#34937,#34938,#34939));
#8120=EDGE_LOOP('',(#34940,#34941,#34942,#34943));
#8121=EDGE_LOOP('',(#34944,#34945,#34946,#34947,#34948,#34949));
#8122=EDGE_LOOP('',(#34950,#34951,#34952,#34953));
#8123=EDGE_LOOP('',(#34954,#34955,#34956,#34957));
#8124=EDGE_LOOP('',(#34958,#34959,#34960,#34961,#34962,#34963));
#8125=EDGE_LOOP('',(#34964,#34965,#34966,#34967));
#8126=EDGE_LOOP('',(#34968,#34969,#34970,#34971));
#8127=EDGE_LOOP('',(#34972,#34973,#34974,#34975,#34976,#34977));
#8128=EDGE_LOOP('',(#34978,#34979,#34980,#34981));
#8129=EDGE_LOOP('',(#34982,#34983,#34984,#34985,#34986,#34987));
#8130=EDGE_LOOP('',(#34988,#34989,#34990,#34991));
#8131=EDGE_LOOP('',(#34992,#34993,#34994));
#8132=EDGE_LOOP('',(#34995,#34996,#34997,#34998));
#8133=EDGE_LOOP('',(#34999,#35000,#35001,#35002,#35003,#35004));
#8134=EDGE_LOOP('',(#35005,#35006,#35007,#35008));
#8135=EDGE_LOOP('',(#35009,#35010,#35011,#35012));
#8136=EDGE_LOOP('',(#35013,#35014,#35015,#35016));
#8137=EDGE_LOOP('',(#35017,#35018,#35019,#35020,#35021,#35022));
#8138=EDGE_LOOP('',(#35023,#35024,#35025,#35026));
#8139=EDGE_LOOP('',(#35027,#35028,#35029,#35030));
#8140=EDGE_LOOP('',(#35031,#35032,#35033,#35034));
#8141=EDGE_LOOP('',(#35035,#35036,#35037));
#8142=EDGE_LOOP('',(#35038,#35039,#35040,#35041));
#8143=EDGE_LOOP('',(#35042,#35043,#35044,#35045));
#8144=EDGE_LOOP('',(#35046,#35047,#35048,#35049));
#8145=EDGE_LOOP('',(#35050,#35051,#35052,#35053));
#8146=EDGE_LOOP('',(#35054,#35055,#35056,#35057));
#8147=EDGE_LOOP('',(#35058,#35059,#35060,#35061));
#8148=EDGE_LOOP('',(#35062,#35063,#35064,#35065,#35066,#35067));
#8149=EDGE_LOOP('',(#35068,#35069,#35070,#35071));
#8150=EDGE_LOOP('',(#35072,#35073,#35074,#35075));
#8151=EDGE_LOOP('',(#35076,#35077,#35078,#35079,#35080,#35081));
#8152=EDGE_LOOP('',(#35082,#35083,#35084,#35085));
#8153=EDGE_LOOP('',(#35086,#35087,#35088,#35089));
#8154=EDGE_LOOP('',(#35090,#35091,#35092,#35093,#35094,#35095));
#8155=EDGE_LOOP('',(#35096,#35097,#35098,#35099));
#8156=EDGE_LOOP('',(#35100,#35101,#35102,#35103));
#8157=EDGE_LOOP('',(#35104,#35105,#35106,#35107,#35108,#35109));
#8158=EDGE_LOOP('',(#35110,#35111,#35112,#35113));
#8159=EDGE_LOOP('',(#35114,#35115,#35116,#35117,#35118,#35119));
#8160=EDGE_LOOP('',(#35120,#35121,#35122,#35123));
#8161=EDGE_LOOP('',(#35124,#35125,#35126));
#8162=EDGE_LOOP('',(#35127,#35128,#35129,#35130));
#8163=EDGE_LOOP('',(#35131,#35132,#35133,#35134,#35135,#35136));
#8164=EDGE_LOOP('',(#35137,#35138,#35139,#35140));
#8165=EDGE_LOOP('',(#35141,#35142,#35143,#35144));
#8166=EDGE_LOOP('',(#35145,#35146,#35147,#35148,#35149,#35150));
#8167=EDGE_LOOP('',(#35151,#35152,#35153,#35154));
#8168=EDGE_LOOP('',(#35155,#35156,#35157,#35158));
#8169=EDGE_LOOP('',(#35159,#35160,#35161,#35162));
#8170=EDGE_LOOP('',(#35163,#35164,#35165));
#8171=EDGE_LOOP('',(#35166,#35167,#35168,#35169));
#8172=EDGE_LOOP('',(#35170,#35171,#35172));
#8173=EDGE_LOOP('',(#35173,#35174,#35175));
#8174=EDGE_LOOP('',(#35176));
#8175=EDGE_LOOP('',(#35177));
#8176=EDGE_LOOP('',(#35178));
#8177=EDGE_LOOP('',(#35179));
#8178=EDGE_LOOP('',(#35180,#35181,#35182,#35183));
#8179=EDGE_LOOP('',(#35184,#35185,#35186,#35187));
#8180=EDGE_LOOP('',(#35188,#35189,#35190,#35191,#35192,#35193));
#8181=EDGE_LOOP('',(#35194,#35195,#35196,#35197));
#8182=EDGE_LOOP('',(#35198,#35199,#35200,#35201));
#8183=EDGE_LOOP('',(#35202,#35203,#35204,#35205,#35206,#35207));
#8184=EDGE_LOOP('',(#35208,#35209,#35210,#35211));
#8185=EDGE_LOOP('',(#35212,#35213,#35214,#35215));
#8186=EDGE_LOOP('',(#35216,#35217,#35218,#35219,#35220,#35221));
#8187=EDGE_LOOP('',(#35222,#35223,#35224,#35225));
#8188=EDGE_LOOP('',(#35226,#35227,#35228,#35229));
#8189=EDGE_LOOP('',(#35230,#35231,#35232,#35233,#35234,#35235));
#8190=EDGE_LOOP('',(#35236,#35237,#35238,#35239));
#8191=EDGE_LOOP('',(#35240,#35241,#35242));
#8192=EDGE_LOOP('',(#35243,#35244,#35245,#35246,#35247,#35248));
#8193=EDGE_LOOP('',(#35249,#35250,#35251));
#8194=EDGE_LOOP('',(#35252,#35253,#35254,#35255));
#8195=EDGE_LOOP('',(#35256,#35257,#35258,#35259));
#8196=EDGE_LOOP('',(#35260,#35261,#35262,#35263));
#8197=EDGE_LOOP('',(#35264,#35265,#35266,#35267,#35268,#35269));
#8198=EDGE_LOOP('',(#35270,#35271,#35272,#35273,#35274,#35275));
#8199=EDGE_LOOP('',(#35276,#35277,#35278,#35279));
#8200=EDGE_LOOP('',(#35280,#35281,#35282,#35283));
#8201=EDGE_LOOP('',(#35284,#35285,#35286));
#8202=EDGE_LOOP('',(#35287,#35288,#35289,#35290));
#8203=EDGE_LOOP('',(#35291,#35292,#35293,#35294));
#8204=EDGE_LOOP('',(#35295,#35296,#35297,#35298));
#8205=EDGE_LOOP('',(#35299,#35300,#35301,#35302,#35303,#35304));
#8206=EDGE_LOOP('',(#35305,#35306,#35307,#35308));
#8207=EDGE_LOOP('',(#35309,#35310,#35311,#35312));
#8208=EDGE_LOOP('',(#35313,#35314,#35315,#35316,#35317,#35318));
#8209=EDGE_LOOP('',(#35319,#35320,#35321,#35322));
#8210=EDGE_LOOP('',(#35323,#35324,#35325,#35326));
#8211=EDGE_LOOP('',(#35327,#35328,#35329,#35330,#35331,#35332));
#8212=EDGE_LOOP('',(#35333,#35334,#35335,#35336));
#8213=EDGE_LOOP('',(#35337,#35338,#35339,#35340));
#8214=EDGE_LOOP('',(#35341,#35342,#35343,#35344,#35345,#35346));
#8215=EDGE_LOOP('',(#35347,#35348,#35349,#35350));
#8216=EDGE_LOOP('',(#35351,#35352,#35353));
#8217=EDGE_LOOP('',(#35354,#35355,#35356,#35357,#35358,#35359,#35360));
#8218=EDGE_LOOP('',(#35361,#35362,#35363,#35364));
#8219=EDGE_LOOP('',(#35365,#35366,#35367,#35368));
#8220=EDGE_LOOP('',(#35369,#35370,#35371,#35372,#35373,#35374));
#8221=EDGE_LOOP('',(#35375,#35376,#35377,#35378,#35379,#35380));
#8222=EDGE_LOOP('',(#35381,#35382,#35383,#35384));
#8223=EDGE_LOOP('',(#35385,#35386,#35387,#35388));
#8224=EDGE_LOOP('',(#35389,#35390,#35391));
#8225=EDGE_LOOP('',(#35392,#35393,#35394,#35395));
#8226=EDGE_LOOP('',(#35396,#35397,#35398,#35399));
#8227=EDGE_LOOP('',(#35400,#35401,#35402,#35403));
#8228=EDGE_LOOP('',(#35404,#35405,#35406,#35407,#35408,#35409));
#8229=EDGE_LOOP('',(#35410,#35411,#35412,#35413));
#8230=EDGE_LOOP('',(#35414,#35415,#35416,#35417));
#8231=EDGE_LOOP('',(#35418,#35419,#35420,#35421,#35422,#35423));
#8232=EDGE_LOOP('',(#35424,#35425,#35426,#35427));
#8233=EDGE_LOOP('',(#35428,#35429,#35430,#35431));
#8234=EDGE_LOOP('',(#35432,#35433,#35434,#35435,#35436,#35437));
#8235=EDGE_LOOP('',(#35438,#35439,#35440,#35441));
#8236=EDGE_LOOP('',(#35442,#35443,#35444,#35445));
#8237=EDGE_LOOP('',(#35446,#35447,#35448,#35449,#35450,#35451));
#8238=EDGE_LOOP('',(#35452,#35453,#35454,#35455));
#8239=EDGE_LOOP('',(#35456,#35457,#35458));
#8240=EDGE_LOOP('',(#35459,#35460,#35461,#35462,#35463,#35464));
#8241=EDGE_LOOP('',(#35465,#35466,#35467,#35468));
#8242=EDGE_LOOP('',(#35469,#35470,#35471,#35472));
#8243=EDGE_LOOP('',(#35473,#35474,#35475,#35476,#35477,#35478));
#8244=EDGE_LOOP('',(#35479,#35480,#35481,#35482,#35483,#35484));
#8245=EDGE_LOOP('',(#35485,#35486,#35487,#35488));
#8246=EDGE_LOOP('',(#35489,#35490,#35491,#35492));
#8247=EDGE_LOOP('',(#35493,#35494,#35495));
#8248=EDGE_LOOP('',(#35496,#35497,#35498,#35499));
#8249=EDGE_LOOP('',(#35500,#35501,#35502,#35503));
#8250=EDGE_LOOP('',(#35504,#35505,#35506,#35507));
#8251=EDGE_LOOP('',(#35508,#35509,#35510,#35511,#35512,#35513));
#8252=EDGE_LOOP('',(#35514,#35515,#35516,#35517));
#8253=EDGE_LOOP('',(#35518,#35519,#35520,#35521));
#8254=EDGE_LOOP('',(#35522,#35523,#35524,#35525,#35526,#35527));
#8255=EDGE_LOOP('',(#35528,#35529,#35530,#35531));
#8256=EDGE_LOOP('',(#35532,#35533,#35534,#35535));
#8257=EDGE_LOOP('',(#35536,#35537,#35538,#35539,#35540,#35541));
#8258=EDGE_LOOP('',(#35542,#35543,#35544,#35545));
#8259=EDGE_LOOP('',(#35546,#35547,#35548,#35549));
#8260=EDGE_LOOP('',(#35550,#35551,#35552,#35553,#35554,#35555));
#8261=EDGE_LOOP('',(#35556,#35557,#35558,#35559));
#8262=EDGE_LOOP('',(#35560,#35561,#35562));
#8263=EDGE_LOOP('',(#35563,#35564,#35565,#35566,#35567,#35568));
#8264=EDGE_LOOP('',(#35569,#35570,#35571,#35572));
#8265=EDGE_LOOP('',(#35573,#35574,#35575,#35576));
#8266=EDGE_LOOP('',(#35577,#35578,#35579,#35580,#35581,#35582));
#8267=EDGE_LOOP('',(#35583,#35584,#35585,#35586,#35587,#35588));
#8268=EDGE_LOOP('',(#35589,#35590,#35591,#35592));
#8269=EDGE_LOOP('',(#35593,#35594,#35595,#35596));
#8270=EDGE_LOOP('',(#35597,#35598,#35599));
#8271=EDGE_LOOP('',(#35600,#35601,#35602,#35603));
#8272=EDGE_LOOP('',(#35604,#35605,#35606,#35607));
#8273=EDGE_LOOP('',(#35608,#35609,#35610,#35611));
#8274=EDGE_LOOP('',(#35612,#35613,#35614,#35615,#35616,#35617));
#8275=EDGE_LOOP('',(#35618,#35619,#35620,#35621));
#8276=EDGE_LOOP('',(#35622,#35623,#35624,#35625));
#8277=EDGE_LOOP('',(#35626,#35627,#35628,#35629,#35630,#35631));
#8278=EDGE_LOOP('',(#35632,#35633,#35634,#35635));
#8279=EDGE_LOOP('',(#35636,#35637,#35638,#35639));
#8280=EDGE_LOOP('',(#35640,#35641,#35642,#35643,#35644,#35645));
#8281=EDGE_LOOP('',(#35646,#35647,#35648,#35649));
#8282=EDGE_LOOP('',(#35650,#35651,#35652,#35653));
#8283=EDGE_LOOP('',(#35654,#35655,#35656,#35657,#35658,#35659));
#8284=EDGE_LOOP('',(#35660,#35661,#35662,#35663));
#8285=EDGE_LOOP('',(#35664,#35665,#35666,#35667,#35668,#35669));
#8286=EDGE_LOOP('',(#35670,#35671,#35672));
#8287=EDGE_LOOP('',(#35673,#35674,#35675,#35676));
#8288=EDGE_LOOP('',(#35677,#35678,#35679,#35680));
#8289=EDGE_LOOP('',(#35681,#35682,#35683,#35684,#35685,#35686));
#8290=EDGE_LOOP('',(#35687,#35688,#35689,#35690,#35691,#35692));
#8291=EDGE_LOOP('',(#35693,#35694,#35695,#35696));
#8292=EDGE_LOOP('',(#35697,#35698,#35699,#35700));
#8293=EDGE_LOOP('',(#35701,#35702,#35703));
#8294=EDGE_LOOP('',(#35704,#35705,#35706,#35707));
#8295=EDGE_LOOP('',(#35708,#35709,#35710,#35711));
#8296=EDGE_LOOP('',(#35712,#35713,#35714,#35715));
#8297=EDGE_LOOP('',(#35716,#35717,#35718,#35719,#35720,#35721));
#8298=EDGE_LOOP('',(#35722,#35723,#35724,#35725));
#8299=EDGE_LOOP('',(#35726,#35727,#35728,#35729));
#8300=EDGE_LOOP('',(#35730,#35731,#35732,#35733,#35734,#35735));
#8301=EDGE_LOOP('',(#35736,#35737,#35738,#35739));
#8302=EDGE_LOOP('',(#35740,#35741,#35742,#35743));
#8303=EDGE_LOOP('',(#35744,#35745,#35746,#35747,#35748,#35749));
#8304=EDGE_LOOP('',(#35750,#35751,#35752,#35753));
#8305=EDGE_LOOP('',(#35754,#35755,#35756,#35757));
#8306=EDGE_LOOP('',(#35758,#35759,#35760,#35761,#35762,#35763));
#8307=EDGE_LOOP('',(#35764,#35765,#35766,#35767));
#8308=EDGE_LOOP('',(#35768,#35769,#35770,#35771));
#8309=EDGE_LOOP('',(#35772,#35773,#35774,#35775,#35776,#35777));
#8310=EDGE_LOOP('',(#35778,#35779,#35780,#35781));
#8311=EDGE_LOOP('',(#35782,#35783,#35784,#35785));
#8312=EDGE_LOOP('',(#35786,#35787,#35788,#35789,#35790,#35791));
#8313=EDGE_LOOP('',(#35792,#35793,#35794,#35795,#35796,#35797));
#8314=EDGE_LOOP('',(#35798,#35799,#35800,#35801));
#8315=EDGE_LOOP('',(#35802,#35803,#35804));
#8316=EDGE_LOOP('',(#35805,#35806,#35807));
#8317=EDGE_LOOP('',(#35808,#35809,#35810,#35811));
#8318=EDGE_LOOP('',(#35812,#35813,#35814,#35815));
#8319=EDGE_LOOP('',(#35816,#35817,#35818,#35819));
#8320=EDGE_LOOP('',(#35820,#35821,#35822,#35823,#35824,#35825));
#8321=EDGE_LOOP('',(#35826,#35827,#35828,#35829));
#8322=EDGE_LOOP('',(#35830,#35831,#35832,#35833));
#8323=EDGE_LOOP('',(#35834,#35835,#35836,#35837,#35838,#35839));
#8324=EDGE_LOOP('',(#35840,#35841,#35842,#35843));
#8325=EDGE_LOOP('',(#35844,#35845,#35846,#35847));
#8326=EDGE_LOOP('',(#35848,#35849,#35850,#35851,#35852,#35853));
#8327=EDGE_LOOP('',(#35854,#35855,#35856,#35857));
#8328=EDGE_LOOP('',(#35858,#35859,#35860,#35861));
#8329=EDGE_LOOP('',(#35862,#35863,#35864,#35865,#35866,#35867));
#8330=EDGE_LOOP('',(#35868,#35869,#35870,#35871));
#8331=EDGE_LOOP('',(#35872,#35873,#35874,#35875));
#8332=EDGE_LOOP('',(#35876,#35877,#35878,#35879,#35880,#35881));
#8333=EDGE_LOOP('',(#35882,#35883,#35884,#35885));
#8334=EDGE_LOOP('',(#35886,#35887,#35888,#35889));
#8335=EDGE_LOOP('',(#35890,#35891,#35892,#35893,#35894,#35895));
#8336=EDGE_LOOP('',(#35896,#35897,#35898,#35899,#35900,#35901));
#8337=EDGE_LOOP('',(#35902,#35903,#35904,#35905));
#8338=EDGE_LOOP('',(#35906,#35907,#35908));
#8339=EDGE_LOOP('',(#35909,#35910,#35911));
#8340=EDGE_LOOP('',(#35912,#35913,#35914,#35915));
#8341=EDGE_LOOP('',(#35916,#35917,#35918,#35919));
#8342=EDGE_LOOP('',(#35920,#35921,#35922,#35923));
#8343=EDGE_LOOP('',(#35924,#35925,#35926,#35927,#35928,#35929));
#8344=EDGE_LOOP('',(#35930,#35931,#35932,#35933));
#8345=EDGE_LOOP('',(#35934,#35935,#35936,#35937));
#8346=EDGE_LOOP('',(#35938,#35939,#35940,#35941,#35942,#35943));
#8347=EDGE_LOOP('',(#35944,#35945,#35946,#35947));
#8348=EDGE_LOOP('',(#35948,#35949,#35950,#35951));
#8349=EDGE_LOOP('',(#35952,#35953,#35954,#35955,#35956,#35957));
#8350=EDGE_LOOP('',(#35958,#35959,#35960,#35961));
#8351=EDGE_LOOP('',(#35962,#35963,#35964,#35965));
#8352=EDGE_LOOP('',(#35966,#35967,#35968,#35969,#35970,#35971));
#8353=EDGE_LOOP('',(#35972,#35973,#35974,#35975));
#8354=EDGE_LOOP('',(#35976,#35977,#35978,#35979));
#8355=EDGE_LOOP('',(#35980,#35981,#35982,#35983,#35984,#35985));
#8356=EDGE_LOOP('',(#35986,#35987,#35988,#35989));
#8357=EDGE_LOOP('',(#35990,#35991,#35992,#35993));
#8358=EDGE_LOOP('',(#35994,#35995,#35996,#35997,#35998,#35999));
#8359=EDGE_LOOP('',(#36000,#36001,#36002,#36003,#36004,#36005));
#8360=EDGE_LOOP('',(#36006,#36007,#36008,#36009));
#8361=EDGE_LOOP('',(#36010,#36011,#36012));
#8362=EDGE_LOOP('',(#36013,#36014,#36015));
#8363=EDGE_LOOP('',(#36016,#36017,#36018,#36019));
#8364=EDGE_LOOP('',(#36020,#36021,#36022,#36023));
#8365=EDGE_LOOP('',(#36024,#36025,#36026,#36027));
#8366=EDGE_LOOP('',(#36028,#36029,#36030,#36031,#36032,#36033));
#8367=EDGE_LOOP('',(#36034,#36035,#36036,#36037));
#8368=EDGE_LOOP('',(#36038,#36039,#36040,#36041));
#8369=EDGE_LOOP('',(#36042,#36043,#36044,#36045,#36046,#36047));
#8370=EDGE_LOOP('',(#36048,#36049,#36050,#36051));
#8371=EDGE_LOOP('',(#36052,#36053,#36054,#36055));
#8372=EDGE_LOOP('',(#36056,#36057,#36058,#36059,#36060,#36061));
#8373=EDGE_LOOP('',(#36062,#36063,#36064,#36065));
#8374=EDGE_LOOP('',(#36066,#36067,#36068,#36069));
#8375=EDGE_LOOP('',(#36070,#36071,#36072,#36073,#36074,#36075));
#8376=EDGE_LOOP('',(#36076,#36077,#36078,#36079));
#8377=EDGE_LOOP('',(#36080,#36081,#36082,#36083));
#8378=EDGE_LOOP('',(#36084,#36085,#36086,#36087,#36088,#36089));
#8379=EDGE_LOOP('',(#36090,#36091,#36092,#36093));
#8380=EDGE_LOOP('',(#36094,#36095,#36096,#36097));
#8381=EDGE_LOOP('',(#36098,#36099,#36100,#36101,#36102,#36103));
#8382=EDGE_LOOP('',(#36104,#36105,#36106,#36107,#36108,#36109));
#8383=EDGE_LOOP('',(#36110,#36111,#36112,#36113));
#8384=EDGE_LOOP('',(#36114,#36115,#36116));
#8385=EDGE_LOOP('',(#36117,#36118,#36119));
#8386=EDGE_LOOP('',(#36120,#36121,#36122,#36123));
#8387=EDGE_LOOP('',(#36124,#36125,#36126,#36127));
#8388=EDGE_LOOP('',(#36128,#36129,#36130,#36131));
#8389=EDGE_LOOP('',(#36132,#36133,#36134,#36135,#36136,#36137));
#8390=EDGE_LOOP('',(#36138,#36139,#36140,#36141));
#8391=EDGE_LOOP('',(#36142,#36143,#36144,#36145));
#8392=EDGE_LOOP('',(#36146,#36147,#36148,#36149,#36150,#36151));
#8393=EDGE_LOOP('',(#36152,#36153,#36154,#36155));
#8394=EDGE_LOOP('',(#36156,#36157,#36158,#36159));
#8395=EDGE_LOOP('',(#36160,#36161,#36162,#36163,#36164,#36165));
#8396=EDGE_LOOP('',(#36166,#36167,#36168,#36169));
#8397=EDGE_LOOP('',(#36170,#36171,#36172,#36173));
#8398=EDGE_LOOP('',(#36174,#36175,#36176,#36177,#36178,#36179));
#8399=EDGE_LOOP('',(#36180,#36181,#36182,#36183));
#8400=EDGE_LOOP('',(#36184,#36185,#36186,#36187));
#8401=EDGE_LOOP('',(#36188,#36189,#36190,#36191,#36192,#36193));
#8402=EDGE_LOOP('',(#36194,#36195,#36196,#36197));
#8403=EDGE_LOOP('',(#36198,#36199,#36200,#36201));
#8404=EDGE_LOOP('',(#36202,#36203,#36204,#36205,#36206,#36207));
#8405=EDGE_LOOP('',(#36208,#36209,#36210,#36211,#36212,#36213));
#8406=EDGE_LOOP('',(#36214,#36215,#36216,#36217));
#8407=EDGE_LOOP('',(#36218,#36219,#36220));
#8408=EDGE_LOOP('',(#36221,#36222,#36223));
#8409=EDGE_LOOP('',(#36224,#36225,#36226,#36227));
#8410=EDGE_LOOP('',(#36228,#36229,#36230,#36231));
#8411=EDGE_LOOP('',(#36232,#36233,#36234,#36235));
#8412=EDGE_LOOP('',(#36236,#36237,#36238,#36239,#36240,#36241));
#8413=EDGE_LOOP('',(#36242,#36243,#36244,#36245));
#8414=EDGE_LOOP('',(#36246,#36247,#36248,#36249));
#8415=EDGE_LOOP('',(#36250,#36251,#36252,#36253,#36254,#36255));
#8416=EDGE_LOOP('',(#36256,#36257,#36258,#36259));
#8417=EDGE_LOOP('',(#36260,#36261,#36262,#36263));
#8418=EDGE_LOOP('',(#36264,#36265,#36266,#36267,#36268,#36269));
#8419=EDGE_LOOP('',(#36270,#36271,#36272,#36273));
#8420=EDGE_LOOP('',(#36274,#36275,#36276,#36277));
#8421=EDGE_LOOP('',(#36278,#36279,#36280,#36281,#36282,#36283));
#8422=EDGE_LOOP('',(#36284,#36285,#36286,#36287));
#8423=EDGE_LOOP('',(#36288,#36289,#36290,#36291));
#8424=EDGE_LOOP('',(#36292,#36293,#36294,#36295,#36296,#36297));
#8425=EDGE_LOOP('',(#36298,#36299,#36300,#36301));
#8426=EDGE_LOOP('',(#36302,#36303,#36304,#36305));
#8427=EDGE_LOOP('',(#36306,#36307,#36308,#36309,#36310,#36311));
#8428=EDGE_LOOP('',(#36312,#36313,#36314,#36315,#36316,#36317));
#8429=EDGE_LOOP('',(#36318,#36319,#36320,#36321));
#8430=EDGE_LOOP('',(#36322,#36323,#36324));
#8431=EDGE_LOOP('',(#36325,#36326,#36327));
#8432=EDGE_LOOP('',(#36328,#36329,#36330,#36331));
#8433=EDGE_LOOP('',(#36332,#36333,#36334,#36335));
#8434=EDGE_LOOP('',(#36336,#36337,#36338,#36339));
#8435=EDGE_LOOP('',(#36340,#36341,#36342,#36343,#36344,#36345));
#8436=EDGE_LOOP('',(#36346,#36347,#36348,#36349));
#8437=EDGE_LOOP('',(#36350,#36351,#36352,#36353));
#8438=EDGE_LOOP('',(#36354,#36355,#36356,#36357,#36358,#36359));
#8439=EDGE_LOOP('',(#36360,#36361,#36362,#36363));
#8440=EDGE_LOOP('',(#36364,#36365,#36366,#36367));
#8441=EDGE_LOOP('',(#36368,#36369,#36370,#36371,#36372,#36373));
#8442=EDGE_LOOP('',(#36374,#36375,#36376,#36377));
#8443=EDGE_LOOP('',(#36378,#36379,#36380,#36381));
#8444=EDGE_LOOP('',(#36382,#36383,#36384,#36385,#36386,#36387));
#8445=EDGE_LOOP('',(#36388,#36389,#36390,#36391));
#8446=EDGE_LOOP('',(#36392,#36393,#36394,#36395));
#8447=EDGE_LOOP('',(#36396,#36397,#36398,#36399,#36400,#36401));
#8448=EDGE_LOOP('',(#36402,#36403,#36404,#36405));
#8449=EDGE_LOOP('',(#36406,#36407,#36408,#36409));
#8450=EDGE_LOOP('',(#36410,#36411,#36412,#36413,#36414,#36415));
#8451=EDGE_LOOP('',(#36416,#36417,#36418,#36419,#36420,#36421));
#8452=EDGE_LOOP('',(#36422,#36423,#36424,#36425));
#8453=EDGE_LOOP('',(#36426,#36427,#36428));
#8454=EDGE_LOOP('',(#36429,#36430,#36431));
#8455=EDGE_LOOP('',(#36432,#36433,#36434,#36435));
#8456=EDGE_LOOP('',(#36436,#36437,#36438,#36439));
#8457=EDGE_LOOP('',(#36440,#36441,#36442,#36443));
#8458=EDGE_LOOP('',(#36444,#36445,#36446,#36447,#36448,#36449));
#8459=EDGE_LOOP('',(#36450,#36451,#36452,#36453));
#8460=EDGE_LOOP('',(#36454,#36455,#36456,#36457));
#8461=EDGE_LOOP('',(#36458,#36459,#36460,#36461,#36462,#36463));
#8462=EDGE_LOOP('',(#36464,#36465,#36466,#36467));
#8463=EDGE_LOOP('',(#36468,#36469,#36470,#36471));
#8464=EDGE_LOOP('',(#36472,#36473,#36474,#36475,#36476,#36477));
#8465=EDGE_LOOP('',(#36478,#36479,#36480,#36481));
#8466=EDGE_LOOP('',(#36482,#36483,#36484,#36485));
#8467=EDGE_LOOP('',(#36486,#36487,#36488,#36489,#36490,#36491));
#8468=EDGE_LOOP('',(#36492,#36493,#36494,#36495));
#8469=EDGE_LOOP('',(#36496,#36497,#36498,#36499));
#8470=EDGE_LOOP('',(#36500,#36501,#36502,#36503,#36504,#36505));
#8471=EDGE_LOOP('',(#36506,#36507,#36508,#36509));
#8472=EDGE_LOOP('',(#36510,#36511,#36512,#36513));
#8473=EDGE_LOOP('',(#36514,#36515,#36516,#36517,#36518,#36519));
#8474=EDGE_LOOP('',(#36520,#36521,#36522,#36523,#36524,#36525));
#8475=EDGE_LOOP('',(#36526,#36527,#36528,#36529));
#8476=EDGE_LOOP('',(#36530,#36531,#36532));
#8477=EDGE_LOOP('',(#36533,#36534,#36535));
#8478=EDGE_LOOP('',(#36536,#36537,#36538,#36539));
#8479=EDGE_LOOP('',(#36540,#36541,#36542,#36543));
#8480=EDGE_LOOP('',(#36544,#36545,#36546,#36547));
#8481=EDGE_LOOP('',(#36548,#36549,#36550,#36551,#36552,#36553));
#8482=EDGE_LOOP('',(#36554,#36555,#36556,#36557));
#8483=EDGE_LOOP('',(#36558,#36559,#36560,#36561));
#8484=EDGE_LOOP('',(#36562,#36563,#36564,#36565,#36566,#36567));
#8485=EDGE_LOOP('',(#36568,#36569,#36570,#36571));
#8486=EDGE_LOOP('',(#36572,#36573,#36574,#36575));
#8487=EDGE_LOOP('',(#36576,#36577,#36578,#36579,#36580,#36581));
#8488=EDGE_LOOP('',(#36582,#36583,#36584,#36585));
#8489=EDGE_LOOP('',(#36586,#36587,#36588,#36589));
#8490=EDGE_LOOP('',(#36590,#36591,#36592,#36593,#36594,#36595));
#8491=EDGE_LOOP('',(#36596,#36597,#36598,#36599));
#8492=EDGE_LOOP('',(#36600,#36601,#36602,#36603));
#8493=EDGE_LOOP('',(#36604,#36605,#36606,#36607,#36608,#36609));
#8494=EDGE_LOOP('',(#36610,#36611,#36612,#36613));
#8495=EDGE_LOOP('',(#36614,#36615,#36616,#36617));
#8496=EDGE_LOOP('',(#36618,#36619,#36620,#36621,#36622,#36623));
#8497=EDGE_LOOP('',(#36624,#36625,#36626,#36627,#36628,#36629));
#8498=EDGE_LOOP('',(#36630,#36631,#36632,#36633));
#8499=EDGE_LOOP('',(#36634,#36635,#36636));
#8500=EDGE_LOOP('',(#36637,#36638,#36639));
#8501=EDGE_LOOP('',(#36640,#36641,#36642,#36643));
#8502=EDGE_LOOP('',(#36644,#36645,#36646,#36647));
#8503=EDGE_LOOP('',(#36648,#36649,#36650,#36651));
#8504=EDGE_LOOP('',(#36652,#36653,#36654,#36655,#36656,#36657));
#8505=EDGE_LOOP('',(#36658,#36659,#36660,#36661));
#8506=EDGE_LOOP('',(#36662,#36663,#36664,#36665));
#8507=EDGE_LOOP('',(#36666,#36667,#36668,#36669,#36670,#36671));
#8508=EDGE_LOOP('',(#36672,#36673,#36674,#36675));
#8509=EDGE_LOOP('',(#36676,#36677,#36678,#36679));
#8510=EDGE_LOOP('',(#36680,#36681,#36682,#36683,#36684,#36685));
#8511=EDGE_LOOP('',(#36686,#36687,#36688,#36689));
#8512=EDGE_LOOP('',(#36690,#36691,#36692,#36693));
#8513=EDGE_LOOP('',(#36694,#36695,#36696,#36697,#36698,#36699));
#8514=EDGE_LOOP('',(#36700,#36701,#36702,#36703));
#8515=EDGE_LOOP('',(#36704,#36705,#36706,#36707));
#8516=EDGE_LOOP('',(#36708,#36709,#36710,#36711,#36712,#36713));
#8517=EDGE_LOOP('',(#36714,#36715,#36716,#36717));
#8518=EDGE_LOOP('',(#36718,#36719,#36720,#36721));
#8519=EDGE_LOOP('',(#36722,#36723,#36724,#36725,#36726,#36727));
#8520=EDGE_LOOP('',(#36728,#36729,#36730,#36731,#36732,#36733));
#8521=EDGE_LOOP('',(#36734,#36735,#36736,#36737));
#8522=EDGE_LOOP('',(#36738,#36739,#36740));
#8523=EDGE_LOOP('',(#36741,#36742,#36743));
#8524=EDGE_LOOP('',(#36744,#36745,#36746,#36747));
#8525=EDGE_LOOP('',(#36748,#36749,#36750,#36751));
#8526=EDGE_LOOP('',(#36752,#36753,#36754,#36755));
#8527=EDGE_LOOP('',(#36756,#36757,#36758,#36759,#36760,#36761));
#8528=EDGE_LOOP('',(#36762,#36763,#36764,#36765));
#8529=EDGE_LOOP('',(#36766,#36767,#36768,#36769));
#8530=EDGE_LOOP('',(#36770,#36771,#36772,#36773,#36774,#36775));
#8531=EDGE_LOOP('',(#36776,#36777,#36778,#36779));
#8532=EDGE_LOOP('',(#36780,#36781,#36782,#36783));
#8533=EDGE_LOOP('',(#36784,#36785,#36786,#36787,#36788,#36789));
#8534=EDGE_LOOP('',(#36790,#36791,#36792,#36793));
#8535=EDGE_LOOP('',(#36794,#36795,#36796,#36797));
#8536=EDGE_LOOP('',(#36798,#36799,#36800,#36801,#36802,#36803));
#8537=EDGE_LOOP('',(#36804,#36805,#36806,#36807));
#8538=EDGE_LOOP('',(#36808,#36809,#36810,#36811));
#8539=EDGE_LOOP('',(#36812,#36813,#36814,#36815,#36816,#36817));
#8540=EDGE_LOOP('',(#36818,#36819,#36820,#36821));
#8541=EDGE_LOOP('',(#36822,#36823,#36824,#36825));
#8542=EDGE_LOOP('',(#36826,#36827,#36828,#36829,#36830,#36831));
#8543=EDGE_LOOP('',(#36832,#36833,#36834,#36835,#36836,#36837));
#8544=EDGE_LOOP('',(#36838,#36839,#36840,#36841));
#8545=EDGE_LOOP('',(#36842,#36843,#36844));
#8546=EDGE_LOOP('',(#36845,#36846,#36847));
#8547=EDGE_LOOP('',(#36848,#36849,#36850,#36851));
#8548=EDGE_LOOP('',(#36852,#36853,#36854,#36855));
#8549=EDGE_LOOP('',(#36856,#36857,#36858,#36859));
#8550=EDGE_LOOP('',(#36860,#36861,#36862,#36863,#36864,#36865));
#8551=EDGE_LOOP('',(#36866,#36867,#36868,#36869));
#8552=EDGE_LOOP('',(#36870,#36871,#36872,#36873));
#8553=EDGE_LOOP('',(#36874,#36875,#36876,#36877,#36878,#36879));
#8554=EDGE_LOOP('',(#36880,#36881,#36882,#36883));
#8555=EDGE_LOOP('',(#36884,#36885,#36886,#36887));
#8556=EDGE_LOOP('',(#36888,#36889,#36890,#36891,#36892,#36893));
#8557=EDGE_LOOP('',(#36894,#36895,#36896,#36897));
#8558=EDGE_LOOP('',(#36898,#36899,#36900,#36901));
#8559=EDGE_LOOP('',(#36902,#36903,#36904,#36905,#36906,#36907));
#8560=EDGE_LOOP('',(#36908,#36909,#36910,#36911));
#8561=EDGE_LOOP('',(#36912,#36913,#36914,#36915));
#8562=EDGE_LOOP('',(#36916,#36917,#36918,#36919,#36920,#36921));
#8563=EDGE_LOOP('',(#36922,#36923,#36924,#36925));
#8564=EDGE_LOOP('',(#36926,#36927,#36928,#36929));
#8565=EDGE_LOOP('',(#36930,#36931,#36932,#36933,#36934,#36935));
#8566=EDGE_LOOP('',(#36936,#36937,#36938,#36939,#36940,#36941));
#8567=EDGE_LOOP('',(#36942,#36943,#36944,#36945));
#8568=EDGE_LOOP('',(#36946,#36947,#36948));
#8569=EDGE_LOOP('',(#36949,#36950,#36951));
#8570=EDGE_LOOP('',(#36952,#36953,#36954,#36955));
#8571=EDGE_LOOP('',(#36956,#36957,#36958,#36959));
#8572=EDGE_LOOP('',(#36960,#36961,#36962,#36963));
#8573=EDGE_LOOP('',(#36964,#36965,#36966,#36967,#36968,#36969));
#8574=EDGE_LOOP('',(#36970,#36971,#36972,#36973));
#8575=EDGE_LOOP('',(#36974,#36975,#36976,#36977));
#8576=EDGE_LOOP('',(#36978,#36979,#36980,#36981,#36982,#36983));
#8577=EDGE_LOOP('',(#36984,#36985,#36986,#36987));
#8578=EDGE_LOOP('',(#36988,#36989,#36990,#36991));
#8579=EDGE_LOOP('',(#36992,#36993,#36994,#36995,#36996,#36997));
#8580=EDGE_LOOP('',(#36998,#36999,#37000,#37001));
#8581=EDGE_LOOP('',(#37002,#37003,#37004,#37005));
#8582=EDGE_LOOP('',(#37006,#37007,#37008,#37009,#37010,#37011));
#8583=EDGE_LOOP('',(#37012,#37013,#37014,#37015));
#8584=EDGE_LOOP('',(#37016,#37017,#37018,#37019));
#8585=EDGE_LOOP('',(#37020,#37021,#37022,#37023,#37024,#37025));
#8586=EDGE_LOOP('',(#37026,#37027,#37028,#37029));
#8587=EDGE_LOOP('',(#37030,#37031,#37032,#37033));
#8588=EDGE_LOOP('',(#37034,#37035,#37036,#37037,#37038,#37039));
#8589=EDGE_LOOP('',(#37040,#37041,#37042,#37043,#37044,#37045));
#8590=EDGE_LOOP('',(#37046,#37047,#37048,#37049));
#8591=EDGE_LOOP('',(#37050,#37051,#37052));
#8592=EDGE_LOOP('',(#37053,#37054,#37055));
#8593=EDGE_LOOP('',(#37056,#37057,#37058,#37059));
#8594=EDGE_LOOP('',(#37060,#37061,#37062,#37063));
#8595=EDGE_LOOP('',(#37064,#37065,#37066,#37067));
#8596=EDGE_LOOP('',(#37068,#37069,#37070,#37071,#37072,#37073));
#8597=EDGE_LOOP('',(#37074,#37075,#37076,#37077));
#8598=EDGE_LOOP('',(#37078,#37079,#37080,#37081));
#8599=EDGE_LOOP('',(#37082,#37083,#37084,#37085,#37086,#37087));
#8600=EDGE_LOOP('',(#37088,#37089,#37090,#37091));
#8601=EDGE_LOOP('',(#37092,#37093,#37094,#37095));
#8602=EDGE_LOOP('',(#37096,#37097,#37098,#37099,#37100,#37101));
#8603=EDGE_LOOP('',(#37102,#37103,#37104,#37105));
#8604=EDGE_LOOP('',(#37106,#37107,#37108,#37109));
#8605=EDGE_LOOP('',(#37110,#37111,#37112,#37113,#37114,#37115));
#8606=EDGE_LOOP('',(#37116,#37117,#37118,#37119));
#8607=EDGE_LOOP('',(#37120,#37121,#37122,#37123));
#8608=EDGE_LOOP('',(#37124,#37125,#37126,#37127,#37128,#37129));
#8609=EDGE_LOOP('',(#37130,#37131,#37132,#37133));
#8610=EDGE_LOOP('',(#37134,#37135,#37136,#37137));
#8611=EDGE_LOOP('',(#37138,#37139,#37140,#37141,#37142,#37143));
#8612=EDGE_LOOP('',(#37144,#37145,#37146,#37147,#37148,#37149));
#8613=EDGE_LOOP('',(#37150,#37151,#37152,#37153));
#8614=EDGE_LOOP('',(#37154,#37155,#37156));
#8615=EDGE_LOOP('',(#37157,#37158,#37159));
#8616=EDGE_LOOP('',(#37160,#37161,#37162,#37163));
#8617=EDGE_LOOP('',(#37164,#37165,#37166,#37167));
#8618=EDGE_LOOP('',(#37168,#37169,#37170,#37171));
#8619=EDGE_LOOP('',(#37172,#37173,#37174,#37175,#37176,#37177));
#8620=EDGE_LOOP('',(#37178,#37179,#37180,#37181));
#8621=EDGE_LOOP('',(#37182,#37183,#37184,#37185));
#8622=EDGE_LOOP('',(#37186,#37187,#37188,#37189,#37190,#37191));
#8623=EDGE_LOOP('',(#37192,#37193,#37194,#37195));
#8624=EDGE_LOOP('',(#37196,#37197,#37198,#37199));
#8625=EDGE_LOOP('',(#37200,#37201,#37202,#37203,#37204,#37205));
#8626=EDGE_LOOP('',(#37206,#37207,#37208,#37209));
#8627=EDGE_LOOP('',(#37210,#37211,#37212,#37213));
#8628=EDGE_LOOP('',(#37214,#37215,#37216,#37217,#37218,#37219));
#8629=EDGE_LOOP('',(#37220,#37221,#37222,#37223));
#8630=EDGE_LOOP('',(#37224,#37225,#37226,#37227));
#8631=EDGE_LOOP('',(#37228,#37229,#37230,#37231,#37232,#37233));
#8632=EDGE_LOOP('',(#37234,#37235,#37236,#37237));
#8633=EDGE_LOOP('',(#37238,#37239,#37240,#37241));
#8634=EDGE_LOOP('',(#37242,#37243,#37244,#37245,#37246,#37247));
#8635=EDGE_LOOP('',(#37248,#37249,#37250,#37251,#37252,#37253));
#8636=EDGE_LOOP('',(#37254,#37255,#37256,#37257));
#8637=EDGE_LOOP('',(#37258,#37259,#37260));
#8638=EDGE_LOOP('',(#37261,#37262,#37263));
#8639=EDGE_LOOP('',(#37264,#37265,#37266,#37267));
#8640=EDGE_LOOP('',(#37268,#37269,#37270,#37271));
#8641=EDGE_LOOP('',(#37272,#37273,#37274,#37275));
#8642=EDGE_LOOP('',(#37276,#37277,#37278,#37279,#37280,#37281));
#8643=EDGE_LOOP('',(#37282,#37283,#37284,#37285));
#8644=EDGE_LOOP('',(#37286,#37287,#37288,#37289));
#8645=EDGE_LOOP('',(#37290,#37291,#37292,#37293,#37294,#37295));
#8646=EDGE_LOOP('',(#37296,#37297,#37298,#37299));
#8647=EDGE_LOOP('',(#37300,#37301,#37302,#37303));
#8648=EDGE_LOOP('',(#37304,#37305,#37306,#37307,#37308,#37309));
#8649=EDGE_LOOP('',(#37310,#37311,#37312,#37313));
#8650=EDGE_LOOP('',(#37314,#37315,#37316,#37317));
#8651=EDGE_LOOP('',(#37318,#37319,#37320,#37321,#37322,#37323));
#8652=EDGE_LOOP('',(#37324,#37325,#37326,#37327));
#8653=EDGE_LOOP('',(#37328,#37329,#37330,#37331));
#8654=EDGE_LOOP('',(#37332,#37333,#37334,#37335,#37336,#37337));
#8655=EDGE_LOOP('',(#37338,#37339,#37340,#37341));
#8656=EDGE_LOOP('',(#37342,#37343,#37344,#37345));
#8657=EDGE_LOOP('',(#37346,#37347,#37348,#37349,#37350,#37351));
#8658=EDGE_LOOP('',(#37352,#37353,#37354,#37355,#37356,#37357));
#8659=EDGE_LOOP('',(#37358,#37359,#37360,#37361));
#8660=EDGE_LOOP('',(#37362,#37363,#37364));
#8661=EDGE_LOOP('',(#37365,#37366,#37367));
#8662=EDGE_LOOP('',(#37368,#37369,#37370,#37371));
#8663=EDGE_LOOP('',(#37372,#37373,#37374,#37375));
#8664=EDGE_LOOP('',(#37376,#37377,#37378,#37379));
#8665=EDGE_LOOP('',(#37380,#37381,#37382,#37383,#37384,#37385));
#8666=EDGE_LOOP('',(#37386,#37387,#37388,#37389));
#8667=EDGE_LOOP('',(#37390,#37391,#37392,#37393));
#8668=EDGE_LOOP('',(#37394,#37395,#37396,#37397,#37398,#37399));
#8669=EDGE_LOOP('',(#37400,#37401,#37402,#37403));
#8670=EDGE_LOOP('',(#37404,#37405,#37406,#37407));
#8671=EDGE_LOOP('',(#37408,#37409,#37410,#37411,#37412,#37413));
#8672=EDGE_LOOP('',(#37414,#37415,#37416,#37417));
#8673=EDGE_LOOP('',(#37418,#37419,#37420,#37421));
#8674=EDGE_LOOP('',(#37422,#37423,#37424,#37425,#37426,#37427));
#8675=EDGE_LOOP('',(#37428,#37429,#37430,#37431));
#8676=EDGE_LOOP('',(#37432,#37433,#37434,#37435));
#8677=EDGE_LOOP('',(#37436,#37437,#37438,#37439,#37440,#37441));
#8678=EDGE_LOOP('',(#37442,#37443,#37444,#37445));
#8679=EDGE_LOOP('',(#37446,#37447,#37448,#37449));
#8680=EDGE_LOOP('',(#37450,#37451,#37452,#37453,#37454,#37455));
#8681=EDGE_LOOP('',(#37456,#37457,#37458,#37459,#37460,#37461));
#8682=EDGE_LOOP('',(#37462,#37463,#37464,#37465));
#8683=EDGE_LOOP('',(#37466,#37467,#37468));
#8684=EDGE_LOOP('',(#37469,#37470,#37471));
#8685=EDGE_LOOP('',(#37472,#37473,#37474,#37475));
#8686=EDGE_LOOP('',(#37476,#37477,#37478,#37479));
#8687=EDGE_LOOP('',(#37480,#37481,#37482,#37483));
#8688=EDGE_LOOP('',(#37484,#37485,#37486,#37487,#37488,#37489));
#8689=EDGE_LOOP('',(#37490,#37491,#37492,#37493));
#8690=EDGE_LOOP('',(#37494,#37495,#37496,#37497));
#8691=EDGE_LOOP('',(#37498,#37499,#37500,#37501,#37502,#37503));
#8692=EDGE_LOOP('',(#37504,#37505,#37506,#37507));
#8693=EDGE_LOOP('',(#37508,#37509,#37510,#37511));
#8694=EDGE_LOOP('',(#37512,#37513,#37514,#37515,#37516,#37517));
#8695=EDGE_LOOP('',(#37518,#37519,#37520,#37521));
#8696=EDGE_LOOP('',(#37522,#37523,#37524,#37525));
#8697=EDGE_LOOP('',(#37526,#37527,#37528,#37529,#37530,#37531));
#8698=EDGE_LOOP('',(#37532,#37533,#37534,#37535));
#8699=EDGE_LOOP('',(#37536,#37537,#37538,#37539));
#8700=EDGE_LOOP('',(#37540,#37541,#37542,#37543,#37544,#37545));
#8701=EDGE_LOOP('',(#37546,#37547,#37548,#37549));
#8702=EDGE_LOOP('',(#37550,#37551,#37552,#37553));
#8703=EDGE_LOOP('',(#37554,#37555,#37556,#37557,#37558,#37559));
#8704=EDGE_LOOP('',(#37560,#37561,#37562,#37563,#37564,#37565));
#8705=EDGE_LOOP('',(#37566,#37567,#37568,#37569));
#8706=EDGE_LOOP('',(#37570,#37571,#37572));
#8707=EDGE_LOOP('',(#37573,#37574,#37575));
#8708=EDGE_LOOP('',(#37576,#37577,#37578,#37579));
#8709=EDGE_LOOP('',(#37580,#37581,#37582,#37583));
#8710=EDGE_LOOP('',(#37584,#37585,#37586,#37587,#37588));
#8711=EDGE_LOOP('',(#37589,#37590,#37591,#37592,#37593,#37594));
#8712=EDGE_LOOP('',(#37595,#37596,#37597,#37598));
#8713=EDGE_LOOP('',(#37599,#37600,#37601,#37602));
#8714=EDGE_LOOP('',(#37603,#37604,#37605,#37606,#37607,#37608));
#8715=EDGE_LOOP('',(#37609,#37610,#37611,#37612));
#8716=EDGE_LOOP('',(#37613,#37614,#37615,#37616));
#8717=EDGE_LOOP('',(#37617,#37618,#37619,#37620,#37621,#37622));
#8718=EDGE_LOOP('',(#37623,#37624,#37625,#37626));
#8719=EDGE_LOOP('',(#37627,#37628,#37629,#37630));
#8720=EDGE_LOOP('',(#37631,#37632,#37633,#37634,#37635,#37636));
#8721=EDGE_LOOP('',(#37637,#37638,#37639,#37640));
#8722=EDGE_LOOP('',(#37641,#37642,#37643,#37644));
#8723=EDGE_LOOP('',(#37645,#37646,#37647,#37648,#37649,#37650));
#8724=EDGE_LOOP('',(#37651,#37652,#37653,#37654));
#8725=EDGE_LOOP('',(#37655,#37656,#37657,#37658));
#8726=EDGE_LOOP('',(#37659,#37660,#37661,#37662,#37663,#37664));
#8727=EDGE_LOOP('',(#37665,#37666,#37667,#37668,#37669,#37670));
#8728=EDGE_LOOP('',(#37671,#37672,#37673,#37674));
#8729=EDGE_LOOP('',(#37675,#37676,#37677));
#8730=EDGE_LOOP('',(#37678,#37679,#37680));
#8731=EDGE_LOOP('',(#37681,#37682,#37683,#37684));
#8732=EDGE_LOOP('',(#37685,#37686,#37687,#37688));
#8733=EDGE_LOOP('',(#37689,#37690,#37691,#37692));
#8734=EDGE_LOOP('',(#37693,#37694,#37695,#37696,#37697,#37698));
#8735=EDGE_LOOP('',(#37699,#37700,#37701,#37702));
#8736=EDGE_LOOP('',(#37703,#37704,#37705,#37706));
#8737=EDGE_LOOP('',(#37707,#37708,#37709,#37710,#37711,#37712));
#8738=EDGE_LOOP('',(#37713,#37714,#37715,#37716));
#8739=EDGE_LOOP('',(#37717,#37718,#37719,#37720));
#8740=EDGE_LOOP('',(#37721,#37722,#37723,#37724,#37725,#37726));
#8741=EDGE_LOOP('',(#37727,#37728,#37729,#37730));
#8742=EDGE_LOOP('',(#37731,#37732,#37733,#37734));
#8743=EDGE_LOOP('',(#37735,#37736,#37737,#37738,#37739,#37740));
#8744=EDGE_LOOP('',(#37741,#37742,#37743,#37744));
#8745=EDGE_LOOP('',(#37745,#37746,#37747,#37748));
#8746=EDGE_LOOP('',(#37749,#37750,#37751,#37752,#37753,#37754));
#8747=EDGE_LOOP('',(#37755,#37756,#37757,#37758));
#8748=EDGE_LOOP('',(#37759,#37760,#37761,#37762));
#8749=EDGE_LOOP('',(#37763,#37764,#37765,#37766,#37767,#37768));
#8750=EDGE_LOOP('',(#37769,#37770,#37771,#37772,#37773,#37774));
#8751=EDGE_LOOP('',(#37775,#37776,#37777,#37778));
#8752=EDGE_LOOP('',(#37779,#37780,#37781));
#8753=EDGE_LOOP('',(#37782,#37783,#37784));
#8754=EDGE_LOOP('',(#37785,#37786,#37787,#37788));
#8755=EDGE_LOOP('',(#37789,#37790,#37791,#37792));
#8756=EDGE_LOOP('',(#37793,#37794,#37795,#37796));
#8757=EDGE_LOOP('',(#37797,#37798,#37799,#37800,#37801,#37802));
#8758=EDGE_LOOP('',(#37803,#37804,#37805,#37806));
#8759=EDGE_LOOP('',(#37807,#37808,#37809,#37810));
#8760=EDGE_LOOP('',(#37811,#37812,#37813,#37814,#37815,#37816));
#8761=EDGE_LOOP('',(#37817,#37818,#37819,#37820));
#8762=EDGE_LOOP('',(#37821,#37822,#37823,#37824));
#8763=EDGE_LOOP('',(#37825,#37826,#37827,#37828,#37829,#37830));
#8764=EDGE_LOOP('',(#37831,#37832,#37833,#37834));
#8765=EDGE_LOOP('',(#37835,#37836,#37837,#37838));
#8766=EDGE_LOOP('',(#37839,#37840,#37841,#37842,#37843,#37844));
#8767=EDGE_LOOP('',(#37845,#37846,#37847,#37848));
#8768=EDGE_LOOP('',(#37849,#37850,#37851,#37852));
#8769=EDGE_LOOP('',(#37853,#37854,#37855,#37856,#37857,#37858));
#8770=EDGE_LOOP('',(#37859,#37860,#37861,#37862));
#8771=EDGE_LOOP('',(#37863,#37864,#37865,#37866));
#8772=EDGE_LOOP('',(#37867,#37868,#37869,#37870,#37871,#37872));
#8773=EDGE_LOOP('',(#37873,#37874,#37875,#37876,#37877,#37878));
#8774=EDGE_LOOP('',(#37879,#37880,#37881,#37882));
#8775=EDGE_LOOP('',(#37883,#37884,#37885));
#8776=EDGE_LOOP('',(#37886,#37887,#37888));
#8777=EDGE_LOOP('',(#37889,#37890,#37891,#37892));
#8778=EDGE_LOOP('',(#37893,#37894,#37895,#37896));
#8779=EDGE_LOOP('',(#37897,#37898,#37899,#37900));
#8780=EDGE_LOOP('',(#37901,#37902,#37903,#37904,#37905,#37906));
#8781=EDGE_LOOP('',(#37907,#37908,#37909,#37910));
#8782=EDGE_LOOP('',(#37911,#37912,#37913,#37914));
#8783=EDGE_LOOP('',(#37915,#37916,#37917,#37918,#37919,#37920));
#8784=EDGE_LOOP('',(#37921,#37922,#37923,#37924));
#8785=EDGE_LOOP('',(#37925,#37926,#37927,#37928));
#8786=EDGE_LOOP('',(#37929,#37930,#37931,#37932,#37933,#37934));
#8787=EDGE_LOOP('',(#37935,#37936,#37937,#37938));
#8788=EDGE_LOOP('',(#37939,#37940,#37941,#37942));
#8789=EDGE_LOOP('',(#37943,#37944,#37945,#37946,#37947,#37948));
#8790=EDGE_LOOP('',(#37949,#37950,#37951,#37952));
#8791=EDGE_LOOP('',(#37953,#37954,#37955,#37956));
#8792=EDGE_LOOP('',(#37957,#37958,#37959,#37960,#37961,#37962));
#8793=EDGE_LOOP('',(#37963,#37964,#37965,#37966));
#8794=EDGE_LOOP('',(#37967,#37968,#37969,#37970));
#8795=EDGE_LOOP('',(#37971,#37972,#37973,#37974,#37975,#37976));
#8796=EDGE_LOOP('',(#37977,#37978,#37979,#37980,#37981,#37982));
#8797=EDGE_LOOP('',(#37983,#37984,#37985,#37986));
#8798=EDGE_LOOP('',(#37987,#37988,#37989));
#8799=EDGE_LOOP('',(#37990,#37991,#37992));
#8800=EDGE_LOOP('',(#37993,#37994,#37995,#37996));
#8801=EDGE_LOOP('',(#37997,#37998,#37999,#38000));
#8802=EDGE_LOOP('',(#38001,#38002,#38003,#38004));
#8803=EDGE_LOOP('',(#38005,#38006,#38007,#38008,#38009,#38010));
#8804=EDGE_LOOP('',(#38011,#38012,#38013,#38014));
#8805=EDGE_LOOP('',(#38015,#38016,#38017,#38018));
#8806=EDGE_LOOP('',(#38019,#38020,#38021,#38022,#38023,#38024));
#8807=EDGE_LOOP('',(#38025,#38026,#38027,#38028));
#8808=EDGE_LOOP('',(#38029,#38030,#38031,#38032));
#8809=EDGE_LOOP('',(#38033,#38034,#38035,#38036,#38037,#38038));
#8810=EDGE_LOOP('',(#38039,#38040,#38041,#38042));
#8811=EDGE_LOOP('',(#38043,#38044,#38045,#38046));
#8812=EDGE_LOOP('',(#38047,#38048,#38049,#38050,#38051,#38052));
#8813=EDGE_LOOP('',(#38053,#38054,#38055,#38056));
#8814=EDGE_LOOP('',(#38057,#38058,#38059,#38060));
#8815=EDGE_LOOP('',(#38061,#38062,#38063,#38064,#38065,#38066));
#8816=EDGE_LOOP('',(#38067,#38068,#38069,#38070));
#8817=EDGE_LOOP('',(#38071,#38072,#38073,#38074));
#8818=EDGE_LOOP('',(#38075,#38076,#38077,#38078,#38079,#38080));
#8819=EDGE_LOOP('',(#38081,#38082,#38083,#38084,#38085,#38086));
#8820=EDGE_LOOP('',(#38087,#38088,#38089,#38090));
#8821=EDGE_LOOP('',(#38091,#38092,#38093));
#8822=EDGE_LOOP('',(#38094,#38095,#38096));
#8823=EDGE_LOOP('',(#38097,#38098,#38099,#38100));
#8824=EDGE_LOOP('',(#38101,#38102,#38103,#38104));
#8825=EDGE_LOOP('',(#38105,#38106,#38107,#38108));
#8826=EDGE_LOOP('',(#38109,#38110,#38111,#38112,#38113,#38114));
#8827=EDGE_LOOP('',(#38115,#38116,#38117,#38118));
#8828=EDGE_LOOP('',(#38119,#38120,#38121,#38122));
#8829=EDGE_LOOP('',(#38123,#38124,#38125,#38126,#38127,#38128));
#8830=EDGE_LOOP('',(#38129,#38130,#38131,#38132));
#8831=EDGE_LOOP('',(#38133,#38134,#38135,#38136));
#8832=EDGE_LOOP('',(#38137,#38138,#38139,#38140,#38141,#38142));
#8833=EDGE_LOOP('',(#38143,#38144,#38145,#38146));
#8834=EDGE_LOOP('',(#38147,#38148,#38149,#38150));
#8835=EDGE_LOOP('',(#38151,#38152,#38153,#38154,#38155,#38156));
#8836=EDGE_LOOP('',(#38157,#38158,#38159,#38160));
#8837=EDGE_LOOP('',(#38161,#38162,#38163,#38164));
#8838=EDGE_LOOP('',(#38165,#38166,#38167,#38168,#38169,#38170));
#8839=EDGE_LOOP('',(#38171,#38172,#38173,#38174));
#8840=EDGE_LOOP('',(#38175,#38176,#38177,#38178));
#8841=EDGE_LOOP('',(#38179,#38180,#38181,#38182,#38183,#38184));
#8842=EDGE_LOOP('',(#38185,#38186,#38187,#38188,#38189,#38190));
#8843=EDGE_LOOP('',(#38191,#38192,#38193,#38194));
#8844=EDGE_LOOP('',(#38195,#38196,#38197));
#8845=EDGE_LOOP('',(#38198,#38199,#38200));
#8846=EDGE_LOOP('',(#38201,#38202,#38203,#38204));
#8847=EDGE_LOOP('',(#38205,#38206,#38207,#38208));
#8848=EDGE_LOOP('',(#38209,#38210,#38211,#38212));
#8849=EDGE_LOOP('',(#38213,#38214,#38215,#38216,#38217,#38218));
#8850=EDGE_LOOP('',(#38219,#38220,#38221,#38222));
#8851=EDGE_LOOP('',(#38223,#38224,#38225,#38226));
#8852=EDGE_LOOP('',(#38227,#38228,#38229,#38230,#38231,#38232));
#8853=EDGE_LOOP('',(#38233,#38234,#38235,#38236));
#8854=EDGE_LOOP('',(#38237,#38238,#38239,#38240));
#8855=EDGE_LOOP('',(#38241,#38242,#38243,#38244,#38245,#38246));
#8856=EDGE_LOOP('',(#38247,#38248,#38249,#38250));
#8857=EDGE_LOOP('',(#38251,#38252,#38253,#38254));
#8858=EDGE_LOOP('',(#38255,#38256,#38257,#38258,#38259,#38260));
#8859=EDGE_LOOP('',(#38261,#38262,#38263,#38264));
#8860=EDGE_LOOP('',(#38265,#38266,#38267,#38268));
#8861=EDGE_LOOP('',(#38269,#38270,#38271,#38272,#38273,#38274));
#8862=EDGE_LOOP('',(#38275,#38276,#38277,#38278));
#8863=EDGE_LOOP('',(#38279,#38280,#38281,#38282));
#8864=EDGE_LOOP('',(#38283,#38284,#38285,#38286,#38287,#38288));
#8865=EDGE_LOOP('',(#38289,#38290,#38291,#38292,#38293,#38294));
#8866=EDGE_LOOP('',(#38295,#38296,#38297,#38298));
#8867=EDGE_LOOP('',(#38299,#38300,#38301));
#8868=EDGE_LOOP('',(#38302,#38303,#38304));
#8869=EDGE_LOOP('',(#38305,#38306,#38307,#38308));
#8870=EDGE_LOOP('',(#38309,#38310,#38311,#38312));
#8871=EDGE_LOOP('',(#38313,#38314,#38315,#38316));
#8872=EDGE_LOOP('',(#38317,#38318,#38319,#38320,#38321,#38322));
#8873=EDGE_LOOP('',(#38323,#38324,#38325,#38326));
#8874=EDGE_LOOP('',(#38327,#38328,#38329,#38330));
#8875=EDGE_LOOP('',(#38331,#38332,#38333,#38334,#38335,#38336));
#8876=EDGE_LOOP('',(#38337,#38338,#38339,#38340));
#8877=EDGE_LOOP('',(#38341,#38342,#38343,#38344));
#8878=EDGE_LOOP('',(#38345,#38346,#38347,#38348,#38349,#38350));
#8879=EDGE_LOOP('',(#38351,#38352,#38353,#38354));
#8880=EDGE_LOOP('',(#38355,#38356,#38357,#38358));
#8881=EDGE_LOOP('',(#38359,#38360,#38361,#38362,#38363,#38364));
#8882=EDGE_LOOP('',(#38365,#38366,#38367,#38368));
#8883=EDGE_LOOP('',(#38369,#38370,#38371,#38372));
#8884=EDGE_LOOP('',(#38373,#38374,#38375,#38376,#38377,#38378));
#8885=EDGE_LOOP('',(#38379,#38380,#38381,#38382));
#8886=EDGE_LOOP('',(#38383,#38384,#38385,#38386));
#8887=EDGE_LOOP('',(#38387,#38388,#38389,#38390,#38391,#38392));
#8888=EDGE_LOOP('',(#38393,#38394,#38395,#38396,#38397,#38398));
#8889=EDGE_LOOP('',(#38399,#38400,#38401,#38402));
#8890=EDGE_LOOP('',(#38403,#38404,#38405));
#8891=EDGE_LOOP('',(#38406,#38407,#38408));
#8892=EDGE_LOOP('',(#38409,#38410,#38411,#38412));
#8893=EDGE_LOOP('',(#38413,#38414,#38415,#38416));
#8894=EDGE_LOOP('',(#38417,#38418,#38419,#38420));
#8895=EDGE_LOOP('',(#38421,#38422,#38423,#38424,#38425,#38426));
#8896=EDGE_LOOP('',(#38427,#38428,#38429,#38430));
#8897=EDGE_LOOP('',(#38431,#38432,#38433,#38434));
#8898=EDGE_LOOP('',(#38435,#38436,#38437,#38438,#38439,#38440));
#8899=EDGE_LOOP('',(#38441,#38442,#38443,#38444));
#8900=EDGE_LOOP('',(#38445,#38446,#38447,#38448));
#8901=EDGE_LOOP('',(#38449,#38450,#38451,#38452,#38453,#38454));
#8902=EDGE_LOOP('',(#38455,#38456,#38457,#38458));
#8903=EDGE_LOOP('',(#38459,#38460,#38461,#38462));
#8904=EDGE_LOOP('',(#38463,#38464,#38465,#38466,#38467,#38468));
#8905=EDGE_LOOP('',(#38469,#38470,#38471,#38472));
#8906=EDGE_LOOP('',(#38473,#38474,#38475,#38476));
#8907=EDGE_LOOP('',(#38477,#38478,#38479,#38480,#38481,#38482));
#8908=EDGE_LOOP('',(#38483,#38484,#38485,#38486));
#8909=EDGE_LOOP('',(#38487,#38488,#38489,#38490));
#8910=EDGE_LOOP('',(#38491,#38492,#38493,#38494,#38495,#38496));
#8911=EDGE_LOOP('',(#38497,#38498,#38499,#38500,#38501,#38502));
#8912=EDGE_LOOP('',(#38503,#38504,#38505,#38506));
#8913=EDGE_LOOP('',(#38507,#38508,#38509));
#8914=EDGE_LOOP('',(#38510,#38511,#38512));
#8915=EDGE_LOOP('',(#38513,#38514,#38515,#38516));
#8916=EDGE_LOOP('',(#38517,#38518,#38519,#38520));
#8917=EDGE_LOOP('',(#38521,#38522,#38523,#38524));
#8918=EDGE_LOOP('',(#38525,#38526,#38527,#38528,#38529,#38530));
#8919=EDGE_LOOP('',(#38531,#38532,#38533,#38534));
#8920=EDGE_LOOP('',(#38535,#38536,#38537,#38538));
#8921=EDGE_LOOP('',(#38539,#38540,#38541,#38542,#38543,#38544));
#8922=EDGE_LOOP('',(#38545,#38546,#38547,#38548));
#8923=EDGE_LOOP('',(#38549,#38550,#38551,#38552));
#8924=EDGE_LOOP('',(#38553,#38554,#38555,#38556,#38557,#38558));
#8925=EDGE_LOOP('',(#38559,#38560,#38561,#38562));
#8926=EDGE_LOOP('',(#38563,#38564,#38565,#38566));
#8927=EDGE_LOOP('',(#38567,#38568,#38569,#38570,#38571,#38572));
#8928=EDGE_LOOP('',(#38573,#38574,#38575,#38576));
#8929=EDGE_LOOP('',(#38577,#38578,#38579,#38580));
#8930=EDGE_LOOP('',(#38581,#38582,#38583,#38584,#38585,#38586));
#8931=EDGE_LOOP('',(#38587,#38588,#38589,#38590));
#8932=EDGE_LOOP('',(#38591,#38592,#38593,#38594));
#8933=EDGE_LOOP('',(#38595,#38596,#38597,#38598,#38599,#38600));
#8934=EDGE_LOOP('',(#38601,#38602,#38603,#38604,#38605,#38606));
#8935=EDGE_LOOP('',(#38607,#38608,#38609,#38610));
#8936=EDGE_LOOP('',(#38611,#38612,#38613));
#8937=EDGE_LOOP('',(#38614,#38615,#38616));
#8938=EDGE_LOOP('',(#38617,#38618,#38619,#38620));
#8939=EDGE_LOOP('',(#38621,#38622,#38623,#38624));
#8940=EDGE_LOOP('',(#38625,#38626,#38627,#38628));
#8941=EDGE_LOOP('',(#38629,#38630,#38631,#38632,#38633,#38634));
#8942=EDGE_LOOP('',(#38635,#38636,#38637,#38638));
#8943=EDGE_LOOP('',(#38639,#38640,#38641,#38642));
#8944=EDGE_LOOP('',(#38643,#38644,#38645,#38646,#38647,#38648));
#8945=EDGE_LOOP('',(#38649,#38650,#38651,#38652));
#8946=EDGE_LOOP('',(#38653,#38654,#38655,#38656));
#8947=EDGE_LOOP('',(#38657,#38658,#38659,#38660,#38661,#38662));
#8948=EDGE_LOOP('',(#38663,#38664,#38665,#38666));
#8949=EDGE_LOOP('',(#38667,#38668,#38669,#38670));
#8950=EDGE_LOOP('',(#38671,#38672,#38673,#38674,#38675,#38676));
#8951=EDGE_LOOP('',(#38677,#38678,#38679,#38680));
#8952=EDGE_LOOP('',(#38681,#38682,#38683,#38684));
#8953=EDGE_LOOP('',(#38685,#38686,#38687,#38688,#38689,#38690));
#8954=EDGE_LOOP('',(#38691,#38692,#38693,#38694));
#8955=EDGE_LOOP('',(#38695,#38696,#38697,#38698));
#8956=EDGE_LOOP('',(#38699,#38700,#38701,#38702,#38703,#38704));
#8957=EDGE_LOOP('',(#38705,#38706,#38707,#38708,#38709,#38710));
#8958=EDGE_LOOP('',(#38711,#38712,#38713,#38714));
#8959=EDGE_LOOP('',(#38715,#38716,#38717));
#8960=EDGE_LOOP('',(#38718,#38719,#38720));
#8961=EDGE_LOOP('',(#38721,#38722,#38723,#38724));
#8962=EDGE_LOOP('',(#38725,#38726,#38727,#38728));
#8963=EDGE_LOOP('',(#38729,#38730,#38731,#38732));
#8964=EDGE_LOOP('',(#38733,#38734,#38735,#38736,#38737,#38738));
#8965=EDGE_LOOP('',(#38739,#38740,#38741,#38742));
#8966=EDGE_LOOP('',(#38743,#38744,#38745,#38746));
#8967=EDGE_LOOP('',(#38747,#38748,#38749,#38750,#38751,#38752));
#8968=EDGE_LOOP('',(#38753,#38754,#38755,#38756));
#8969=EDGE_LOOP('',(#38757,#38758,#38759,#38760));
#8970=EDGE_LOOP('',(#38761,#38762,#38763,#38764,#38765,#38766));
#8971=EDGE_LOOP('',(#38767,#38768,#38769,#38770));
#8972=EDGE_LOOP('',(#38771,#38772,#38773,#38774));
#8973=EDGE_LOOP('',(#38775,#38776,#38777,#38778,#38779,#38780));
#8974=EDGE_LOOP('',(#38781,#38782,#38783,#38784));
#8975=EDGE_LOOP('',(#38785,#38786,#38787,#38788));
#8976=EDGE_LOOP('',(#38789,#38790,#38791,#38792,#38793,#38794));
#8977=EDGE_LOOP('',(#38795,#38796,#38797,#38798));
#8978=EDGE_LOOP('',(#38799,#38800,#38801,#38802));
#8979=EDGE_LOOP('',(#38803,#38804,#38805,#38806,#38807,#38808));
#8980=EDGE_LOOP('',(#38809,#38810,#38811,#38812,#38813,#38814));
#8981=EDGE_LOOP('',(#38815,#38816,#38817,#38818));
#8982=EDGE_LOOP('',(#38819,#38820,#38821));
#8983=EDGE_LOOP('',(#38822,#38823,#38824));
#8984=EDGE_LOOP('',(#38825,#38826,#38827,#38828));
#8985=EDGE_LOOP('',(#38829,#38830,#38831,#38832));
#8986=EDGE_LOOP('',(#38833,#38834,#38835,#38836));
#8987=EDGE_LOOP('',(#38837,#38838,#38839,#38840,#38841,#38842));
#8988=EDGE_LOOP('',(#38843,#38844,#38845,#38846));
#8989=EDGE_LOOP('',(#38847,#38848,#38849,#38850));
#8990=EDGE_LOOP('',(#38851,#38852,#38853,#38854,#38855,#38856));
#8991=EDGE_LOOP('',(#38857,#38858,#38859,#38860));
#8992=EDGE_LOOP('',(#38861,#38862,#38863,#38864));
#8993=EDGE_LOOP('',(#38865,#38866,#38867,#38868,#38869,#38870));
#8994=EDGE_LOOP('',(#38871,#38872,#38873,#38874));
#8995=EDGE_LOOP('',(#38875,#38876,#38877,#38878));
#8996=EDGE_LOOP('',(#38879,#38880,#38881,#38882,#38883,#38884));
#8997=EDGE_LOOP('',(#38885,#38886,#38887,#38888));
#8998=EDGE_LOOP('',(#38889,#38890,#38891,#38892));
#8999=EDGE_LOOP('',(#38893,#38894,#38895,#38896,#38897,#38898));
#9000=EDGE_LOOP('',(#38899,#38900,#38901,#38902));
#9001=EDGE_LOOP('',(#38903,#38904,#38905,#38906));
#9002=EDGE_LOOP('',(#38907,#38908,#38909,#38910,#38911,#38912));
#9003=EDGE_LOOP('',(#38913,#38914,#38915,#38916,#38917,#38918));
#9004=EDGE_LOOP('',(#38919,#38920,#38921,#38922));
#9005=EDGE_LOOP('',(#38923,#38924,#38925));
#9006=EDGE_LOOP('',(#38926,#38927,#38928));
#9007=EDGE_LOOP('',(#38929,#38930,#38931,#38932));
#9008=EDGE_LOOP('',(#38933,#38934,#38935,#38936));
#9009=EDGE_LOOP('',(#38937,#38938,#38939,#38940));
#9010=EDGE_LOOP('',(#38941,#38942,#38943,#38944,#38945,#38946));
#9011=EDGE_LOOP('',(#38947,#38948,#38949,#38950));
#9012=EDGE_LOOP('',(#38951,#38952,#38953,#38954));
#9013=EDGE_LOOP('',(#38955,#38956,#38957,#38958,#38959,#38960));
#9014=EDGE_LOOP('',(#38961,#38962,#38963,#38964));
#9015=EDGE_LOOP('',(#38965,#38966,#38967,#38968));
#9016=EDGE_LOOP('',(#38969,#38970,#38971,#38972,#38973,#38974));
#9017=EDGE_LOOP('',(#38975,#38976,#38977,#38978));
#9018=EDGE_LOOP('',(#38979,#38980,#38981,#38982));
#9019=EDGE_LOOP('',(#38983,#38984,#38985,#38986,#38987,#38988));
#9020=EDGE_LOOP('',(#38989,#38990,#38991,#38992));
#9021=EDGE_LOOP('',(#38993,#38994,#38995,#38996));
#9022=EDGE_LOOP('',(#38997,#38998,#38999,#39000,#39001,#39002));
#9023=EDGE_LOOP('',(#39003,#39004,#39005,#39006));
#9024=EDGE_LOOP('',(#39007,#39008,#39009,#39010));
#9025=EDGE_LOOP('',(#39011,#39012,#39013,#39014,#39015,#39016));
#9026=EDGE_LOOP('',(#39017,#39018,#39019,#39020,#39021,#39022));
#9027=EDGE_LOOP('',(#39023,#39024,#39025,#39026));
#9028=EDGE_LOOP('',(#39027,#39028,#39029));
#9029=EDGE_LOOP('',(#39030,#39031,#39032));
#9030=EDGE_LOOP('',(#39033,#39034,#39035,#39036));
#9031=EDGE_LOOP('',(#39037,#39038,#39039,#39040));
#9032=EDGE_LOOP('',(#39041,#39042,#39043,#39044));
#9033=EDGE_LOOP('',(#39045,#39046,#39047,#39048,#39049,#39050));
#9034=EDGE_LOOP('',(#39051,#39052,#39053,#39054));
#9035=EDGE_LOOP('',(#39055,#39056,#39057,#39058));
#9036=EDGE_LOOP('',(#39059,#39060,#39061,#39062,#39063,#39064));
#9037=EDGE_LOOP('',(#39065,#39066,#39067,#39068));
#9038=EDGE_LOOP('',(#39069,#39070,#39071,#39072));
#9039=EDGE_LOOP('',(#39073,#39074,#39075,#39076,#39077,#39078));
#9040=EDGE_LOOP('',(#39079,#39080,#39081,#39082));
#9041=EDGE_LOOP('',(#39083,#39084,#39085,#39086));
#9042=EDGE_LOOP('',(#39087,#39088,#39089,#39090,#39091,#39092));
#9043=EDGE_LOOP('',(#39093,#39094,#39095,#39096));
#9044=EDGE_LOOP('',(#39097,#39098,#39099,#39100));
#9045=EDGE_LOOP('',(#39101,#39102,#39103,#39104,#39105,#39106));
#9046=EDGE_LOOP('',(#39107,#39108,#39109,#39110));
#9047=EDGE_LOOP('',(#39111,#39112,#39113,#39114));
#9048=EDGE_LOOP('',(#39115,#39116,#39117,#39118,#39119,#39120));
#9049=EDGE_LOOP('',(#39121,#39122,#39123,#39124,#39125,#39126));
#9050=EDGE_LOOP('',(#39127,#39128,#39129,#39130));
#9051=EDGE_LOOP('',(#39131,#39132,#39133));
#9052=EDGE_LOOP('',(#39134,#39135,#39136));
#9053=EDGE_LOOP('',(#39137,#39138,#39139,#39140));
#9054=EDGE_LOOP('',(#39141,#39142,#39143,#39144));
#9055=EDGE_LOOP('',(#39145,#39146,#39147,#39148));
#9056=EDGE_LOOP('',(#39149,#39150,#39151,#39152,#39153,#39154));
#9057=EDGE_LOOP('',(#39155,#39156,#39157,#39158));
#9058=EDGE_LOOP('',(#39159,#39160,#39161,#39162));
#9059=EDGE_LOOP('',(#39163,#39164,#39165,#39166,#39167,#39168));
#9060=EDGE_LOOP('',(#39169,#39170,#39171,#39172));
#9061=EDGE_LOOP('',(#39173,#39174,#39175,#39176));
#9062=EDGE_LOOP('',(#39177,#39178,#39179,#39180,#39181,#39182));
#9063=EDGE_LOOP('',(#39183,#39184,#39185,#39186));
#9064=EDGE_LOOP('',(#39187,#39188,#39189,#39190));
#9065=EDGE_LOOP('',(#39191,#39192,#39193,#39194,#39195,#39196));
#9066=EDGE_LOOP('',(#39197,#39198,#39199,#39200));
#9067=EDGE_LOOP('',(#39201,#39202,#39203,#39204));
#9068=EDGE_LOOP('',(#39205,#39206,#39207,#39208,#39209,#39210));
#9069=EDGE_LOOP('',(#39211,#39212,#39213,#39214));
#9070=EDGE_LOOP('',(#39215,#39216,#39217,#39218));
#9071=EDGE_LOOP('',(#39219,#39220,#39221,#39222,#39223,#39224));
#9072=EDGE_LOOP('',(#39225,#39226,#39227,#39228,#39229,#39230));
#9073=EDGE_LOOP('',(#39231,#39232,#39233,#39234));
#9074=EDGE_LOOP('',(#39235,#39236,#39237));
#9075=EDGE_LOOP('',(#39238,#39239,#39240));
#9076=EDGE_LOOP('',(#39241,#39242,#39243,#39244));
#9077=EDGE_LOOP('',(#39245,#39246,#39247,#39248));
#9078=EDGE_LOOP('',(#39249,#39250,#39251,#39252));
#9079=EDGE_LOOP('',(#39253,#39254,#39255,#39256,#39257,#39258));
#9080=EDGE_LOOP('',(#39259,#39260,#39261,#39262));
#9081=EDGE_LOOP('',(#39263,#39264,#39265,#39266));
#9082=EDGE_LOOP('',(#39267,#39268,#39269,#39270,#39271,#39272));
#9083=EDGE_LOOP('',(#39273,#39274,#39275,#39276));
#9084=EDGE_LOOP('',(#39277,#39278,#39279,#39280));
#9085=EDGE_LOOP('',(#39281,#39282,#39283,#39284,#39285,#39286));
#9086=EDGE_LOOP('',(#39287,#39288,#39289,#39290));
#9087=EDGE_LOOP('',(#39291,#39292,#39293,#39294));
#9088=EDGE_LOOP('',(#39295,#39296,#39297,#39298,#39299,#39300));
#9089=EDGE_LOOP('',(#39301,#39302,#39303,#39304));
#9090=EDGE_LOOP('',(#39305,#39306,#39307,#39308));
#9091=EDGE_LOOP('',(#39309,#39310,#39311,#39312,#39313,#39314));
#9092=EDGE_LOOP('',(#39315,#39316,#39317,#39318));
#9093=EDGE_LOOP('',(#39319,#39320,#39321,#39322));
#9094=EDGE_LOOP('',(#39323,#39324,#39325,#39326,#39327,#39328));
#9095=EDGE_LOOP('',(#39329,#39330,#39331,#39332,#39333,#39334));
#9096=EDGE_LOOP('',(#39335,#39336,#39337,#39338));
#9097=EDGE_LOOP('',(#39339,#39340,#39341));
#9098=EDGE_LOOP('',(#39342,#39343,#39344));
#9099=EDGE_LOOP('',(#39345,#39346,#39347,#39348));
#9100=EDGE_LOOP('',(#39349,#39350,#39351,#39352));
#9101=EDGE_LOOP('',(#39353,#39354,#39355,#39356));
#9102=EDGE_LOOP('',(#39357,#39358,#39359,#39360,#39361,#39362));
#9103=EDGE_LOOP('',(#39363,#39364,#39365,#39366));
#9104=EDGE_LOOP('',(#39367,#39368,#39369,#39370));
#9105=EDGE_LOOP('',(#39371,#39372,#39373,#39374,#39375,#39376));
#9106=EDGE_LOOP('',(#39377,#39378,#39379,#39380));
#9107=EDGE_LOOP('',(#39381,#39382,#39383,#39384));
#9108=EDGE_LOOP('',(#39385,#39386,#39387,#39388,#39389,#39390));
#9109=EDGE_LOOP('',(#39391,#39392,#39393,#39394));
#9110=EDGE_LOOP('',(#39395,#39396,#39397,#39398));
#9111=EDGE_LOOP('',(#39399,#39400,#39401,#39402,#39403,#39404));
#9112=EDGE_LOOP('',(#39405,#39406,#39407,#39408));
#9113=EDGE_LOOP('',(#39409,#39410,#39411,#39412));
#9114=EDGE_LOOP('',(#39413,#39414,#39415,#39416,#39417,#39418));
#9115=EDGE_LOOP('',(#39419,#39420,#39421,#39422));
#9116=EDGE_LOOP('',(#39423,#39424,#39425,#39426));
#9117=EDGE_LOOP('',(#39427,#39428,#39429,#39430,#39431,#39432));
#9118=EDGE_LOOP('',(#39433,#39434,#39435,#39436,#39437,#39438));
#9119=EDGE_LOOP('',(#39439,#39440,#39441,#39442));
#9120=EDGE_LOOP('',(#39443,#39444,#39445));
#9121=EDGE_LOOP('',(#39446,#39447,#39448));
#9122=EDGE_LOOP('',(#39449,#39450,#39451,#39452));
#9123=EDGE_LOOP('',(#39453,#39454,#39455,#39456));
#9124=EDGE_LOOP('',(#39457,#39458,#39459,#39460));
#9125=EDGE_LOOP('',(#39461,#39462,#39463,#39464,#39465,#39466));
#9126=EDGE_LOOP('',(#39467,#39468,#39469,#39470));
#9127=EDGE_LOOP('',(#39471,#39472,#39473,#39474));
#9128=EDGE_LOOP('',(#39475,#39476,#39477,#39478,#39479,#39480));
#9129=EDGE_LOOP('',(#39481,#39482,#39483,#39484));
#9130=EDGE_LOOP('',(#39485,#39486,#39487,#39488));
#9131=EDGE_LOOP('',(#39489,#39490,#39491,#39492,#39493,#39494));
#9132=EDGE_LOOP('',(#39495,#39496,#39497,#39498));
#9133=EDGE_LOOP('',(#39499,#39500,#39501,#39502));
#9134=EDGE_LOOP('',(#39503,#39504,#39505,#39506,#39507,#39508));
#9135=EDGE_LOOP('',(#39509,#39510,#39511,#39512));
#9136=EDGE_LOOP('',(#39513,#39514,#39515,#39516));
#9137=EDGE_LOOP('',(#39517,#39518,#39519,#39520,#39521,#39522));
#9138=EDGE_LOOP('',(#39523,#39524,#39525,#39526));
#9139=EDGE_LOOP('',(#39527,#39528,#39529,#39530));
#9140=EDGE_LOOP('',(#39531,#39532,#39533,#39534,#39535,#39536));
#9141=EDGE_LOOP('',(#39537,#39538,#39539,#39540,#39541,#39542));
#9142=EDGE_LOOP('',(#39543,#39544,#39545,#39546));
#9143=EDGE_LOOP('',(#39547,#39548,#39549));
#9144=EDGE_LOOP('',(#39550,#39551,#39552));
#9145=EDGE_LOOP('',(#39553,#39554,#39555,#39556));
#9146=EDGE_LOOP('',(#39557,#39558,#39559,#39560));
#9147=EDGE_LOOP('',(#39561,#39562,#39563,#39564));
#9148=EDGE_LOOP('',(#39565,#39566,#39567,#39568,#39569,#39570));
#9149=EDGE_LOOP('',(#39571,#39572,#39573,#39574));
#9150=EDGE_LOOP('',(#39575,#39576,#39577,#39578));
#9151=EDGE_LOOP('',(#39579,#39580,#39581,#39582,#39583,#39584));
#9152=EDGE_LOOP('',(#39585,#39586,#39587,#39588));
#9153=EDGE_LOOP('',(#39589,#39590,#39591,#39592));
#9154=EDGE_LOOP('',(#39593,#39594,#39595,#39596,#39597,#39598));
#9155=EDGE_LOOP('',(#39599,#39600,#39601,#39602));
#9156=EDGE_LOOP('',(#39603,#39604,#39605,#39606));
#9157=EDGE_LOOP('',(#39607,#39608,#39609,#39610,#39611,#39612));
#9158=EDGE_LOOP('',(#39613,#39614,#39615,#39616));
#9159=EDGE_LOOP('',(#39617,#39618,#39619,#39620));
#9160=EDGE_LOOP('',(#39621,#39622,#39623,#39624,#39625,#39626));
#9161=EDGE_LOOP('',(#39627,#39628,#39629,#39630));
#9162=EDGE_LOOP('',(#39631,#39632,#39633,#39634));
#9163=EDGE_LOOP('',(#39635,#39636,#39637,#39638,#39639,#39640));
#9164=EDGE_LOOP('',(#39641,#39642,#39643,#39644,#39645,#39646));
#9165=EDGE_LOOP('',(#39647,#39648,#39649,#39650));
#9166=EDGE_LOOP('',(#39651,#39652,#39653));
#9167=EDGE_LOOP('',(#39654,#39655,#39656,#39657));
#9168=EDGE_LOOP('',(#39658,#39659,#39660,#39661));
#9169=EDGE_LOOP('',(#39662,#39663,#39664,#39665,#39666,#39667));
#9170=EDGE_LOOP('',(#39668,#39669,#39670));
#9171=EDGE_LOOP('',(#39671,#39672,#39673,#39674));
#9172=EDGE_LOOP('',(#39675,#39676,#39677,#39678));
#9173=EDGE_LOOP('',(#39679,#39680,#39681,#39682));
#9174=EDGE_LOOP('',(#39683,#39684,#39685,#39686,#39687,#39688));
#9175=EDGE_LOOP('',(#39689,#39690,#39691,#39692));
#9176=EDGE_LOOP('',(#39693,#39694,#39695,#39696));
#9177=EDGE_LOOP('',(#39697,#39698,#39699,#39700,#39701,#39702));
#9178=EDGE_LOOP('',(#39703,#39704,#39705,#39706));
#9179=EDGE_LOOP('',(#39707,#39708,#39709,#39710));
#9180=EDGE_LOOP('',(#39711,#39712,#39713,#39714,#39715,#39716));
#9181=EDGE_LOOP('',(#39717,#39718,#39719,#39720));
#9182=EDGE_LOOP('',(#39721,#39722,#39723,#39724));
#9183=EDGE_LOOP('',(#39725,#39726,#39727,#39728,#39729,#39730));
#9184=EDGE_LOOP('',(#39731,#39732,#39733,#39734));
#9185=EDGE_LOOP('',(#39735,#39736,#39737,#39738));
#9186=EDGE_LOOP('',(#39739,#39740,#39741,#39742,#39743,#39744));
#9187=EDGE_LOOP('',(#39745,#39746,#39747,#39748,#39749,#39750));
#9188=EDGE_LOOP('',(#39751,#39752,#39753,#39754));
#9189=EDGE_LOOP('',(#39755,#39756,#39757));
#9190=EDGE_LOOP('',(#39758,#39759,#39760));
#9191=EDGE_LOOP('',(#39761,#39762,#39763,#39764));
#9192=EDGE_LOOP('',(#39765,#39766,#39767,#39768));
#9193=EDGE_LOOP('',(#39769,#39770,#39771,#39772));
#9194=EDGE_LOOP('',(#39773,#39774,#39775,#39776,#39777,#39778));
#9195=EDGE_LOOP('',(#39779,#39780,#39781,#39782));
#9196=EDGE_LOOP('',(#39783,#39784,#39785,#39786));
#9197=EDGE_LOOP('',(#39787,#39788,#39789,#39790,#39791,#39792));
#9198=EDGE_LOOP('',(#39793,#39794,#39795,#39796));
#9199=EDGE_LOOP('',(#39797,#39798,#39799,#39800));
#9200=EDGE_LOOP('',(#39801,#39802,#39803,#39804,#39805,#39806));
#9201=EDGE_LOOP('',(#39807,#39808,#39809,#39810));
#9202=EDGE_LOOP('',(#39811,#39812,#39813,#39814));
#9203=EDGE_LOOP('',(#39815,#39816,#39817,#39818,#39819,#39820));
#9204=EDGE_LOOP('',(#39821,#39822,#39823,#39824));
#9205=EDGE_LOOP('',(#39825,#39826,#39827,#39828));
#9206=EDGE_LOOP('',(#39829,#39830,#39831,#39832,#39833,#39834));
#9207=EDGE_LOOP('',(#39835,#39836,#39837,#39838));
#9208=EDGE_LOOP('',(#39839,#39840,#39841,#39842));
#9209=EDGE_LOOP('',(#39843,#39844,#39845,#39846,#39847,#39848));
#9210=EDGE_LOOP('',(#39849,#39850,#39851,#39852,#39853,#39854));
#9211=EDGE_LOOP('',(#39855,#39856,#39857,#39858));
#9212=EDGE_LOOP('',(#39859,#39860,#39861));
#9213=EDGE_LOOP('',(#39862,#39863,#39864));
#9214=EDGE_LOOP('',(#39865,#39866,#39867,#39868));
#9215=EDGE_LOOP('',(#39869,#39870,#39871,#39872));
#9216=EDGE_LOOP('',(#39873,#39874,#39875,#39876));
#9217=EDGE_LOOP('',(#39877,#39878,#39879,#39880,#39881,#39882));
#9218=EDGE_LOOP('',(#39883,#39884,#39885,#39886));
#9219=EDGE_LOOP('',(#39887,#39888,#39889,#39890));
#9220=EDGE_LOOP('',(#39891,#39892,#39893,#39894,#39895,#39896));
#9221=EDGE_LOOP('',(#39897,#39898,#39899,#39900));
#9222=EDGE_LOOP('',(#39901,#39902,#39903,#39904));
#9223=EDGE_LOOP('',(#39905,#39906,#39907,#39908,#39909,#39910));
#9224=EDGE_LOOP('',(#39911,#39912,#39913,#39914));
#9225=EDGE_LOOP('',(#39915,#39916,#39917,#39918));
#9226=EDGE_LOOP('',(#39919,#39920,#39921,#39922,#39923,#39924));
#9227=EDGE_LOOP('',(#39925,#39926,#39927,#39928));
#9228=EDGE_LOOP('',(#39929,#39930,#39931,#39932));
#9229=EDGE_LOOP('',(#39933,#39934,#39935,#39936,#39937,#39938));
#9230=EDGE_LOOP('',(#39939,#39940,#39941,#39942));
#9231=EDGE_LOOP('',(#39943,#39944,#39945,#39946));
#9232=EDGE_LOOP('',(#39947,#39948,#39949,#39950,#39951,#39952));
#9233=EDGE_LOOP('',(#39953,#39954,#39955,#39956,#39957,#39958));
#9234=EDGE_LOOP('',(#39959,#39960,#39961,#39962));
#9235=EDGE_LOOP('',(#39963,#39964,#39965));
#9236=EDGE_LOOP('',(#39966,#39967,#39968));
#9237=EDGE_LOOP('',(#39969,#39970,#39971,#39972));
#9238=EDGE_LOOP('',(#39973,#39974,#39975,#39976));
#9239=EDGE_LOOP('',(#39977,#39978,#39979,#39980));
#9240=EDGE_LOOP('',(#39981,#39982,#39983,#39984,#39985,#39986));
#9241=EDGE_LOOP('',(#39987,#39988,#39989,#39990));
#9242=EDGE_LOOP('',(#39991,#39992,#39993,#39994));
#9243=EDGE_LOOP('',(#39995,#39996,#39997,#39998,#39999,#40000));
#9244=EDGE_LOOP('',(#40001,#40002,#40003,#40004));
#9245=EDGE_LOOP('',(#40005,#40006,#40007,#40008));
#9246=EDGE_LOOP('',(#40009,#40010,#40011,#40012,#40013,#40014));
#9247=EDGE_LOOP('',(#40015,#40016,#40017,#40018));
#9248=EDGE_LOOP('',(#40019,#40020,#40021,#40022));
#9249=EDGE_LOOP('',(#40023,#40024,#40025,#40026,#40027,#40028));
#9250=EDGE_LOOP('',(#40029,#40030,#40031,#40032));
#9251=EDGE_LOOP('',(#40033,#40034,#40035,#40036));
#9252=EDGE_LOOP('',(#40037,#40038,#40039,#40040,#40041,#40042));
#9253=EDGE_LOOP('',(#40043,#40044,#40045,#40046));
#9254=EDGE_LOOP('',(#40047,#40048,#40049,#40050));
#9255=EDGE_LOOP('',(#40051,#40052,#40053,#40054,#40055,#40056));
#9256=EDGE_LOOP('',(#40057,#40058,#40059,#40060,#40061,#40062));
#9257=EDGE_LOOP('',(#40063,#40064,#40065,#40066));
#9258=EDGE_LOOP('',(#40067,#40068,#40069));
#9259=EDGE_LOOP('',(#40070,#40071,#40072));
#9260=EDGE_LOOP('',(#40073,#40074,#40075,#40076));
#9261=EDGE_LOOP('',(#40077,#40078,#40079,#40080));
#9262=EDGE_LOOP('',(#40081,#40082,#40083,#40084));
#9263=EDGE_LOOP('',(#40085,#40086,#40087,#40088,#40089,#40090));
#9264=EDGE_LOOP('',(#40091,#40092,#40093,#40094));
#9265=EDGE_LOOP('',(#40095,#40096,#40097,#40098));
#9266=EDGE_LOOP('',(#40099,#40100,#40101,#40102,#40103,#40104));
#9267=EDGE_LOOP('',(#40105,#40106,#40107,#40108));
#9268=EDGE_LOOP('',(#40109,#40110,#40111,#40112));
#9269=EDGE_LOOP('',(#40113,#40114,#40115,#40116,#40117,#40118));
#9270=EDGE_LOOP('',(#40119,#40120,#40121,#40122));
#9271=EDGE_LOOP('',(#40123,#40124,#40125,#40126));
#9272=EDGE_LOOP('',(#40127,#40128,#40129,#40130,#40131,#40132));
#9273=EDGE_LOOP('',(#40133,#40134,#40135,#40136));
#9274=EDGE_LOOP('',(#40137,#40138,#40139,#40140));
#9275=EDGE_LOOP('',(#40141,#40142,#40143,#40144,#40145,#40146));
#9276=EDGE_LOOP('',(#40147,#40148,#40149,#40150));
#9277=EDGE_LOOP('',(#40151,#40152,#40153,#40154));
#9278=EDGE_LOOP('',(#40155,#40156,#40157,#40158,#40159,#40160));
#9279=EDGE_LOOP('',(#40161,#40162,#40163,#40164,#40165,#40166));
#9280=EDGE_LOOP('',(#40167,#40168,#40169,#40170));
#9281=EDGE_LOOP('',(#40171,#40172,#40173));
#9282=EDGE_LOOP('',(#40174,#40175,#40176));
#9283=EDGE_LOOP('',(#40177,#40178,#40179,#40180));
#9284=EDGE_LOOP('',(#40181,#40182,#40183,#40184));
#9285=EDGE_LOOP('',(#40185,#40186,#40187,#40188));
#9286=EDGE_LOOP('',(#40189,#40190,#40191,#40192,#40193,#40194));
#9287=EDGE_LOOP('',(#40195,#40196,#40197,#40198));
#9288=EDGE_LOOP('',(#40199,#40200,#40201,#40202));
#9289=EDGE_LOOP('',(#40203,#40204,#40205,#40206,#40207,#40208));
#9290=EDGE_LOOP('',(#40209,#40210,#40211,#40212));
#9291=EDGE_LOOP('',(#40213,#40214,#40215,#40216));
#9292=EDGE_LOOP('',(#40217,#40218,#40219,#40220,#40221,#40222));
#9293=EDGE_LOOP('',(#40223,#40224,#40225,#40226));
#9294=EDGE_LOOP('',(#40227,#40228,#40229,#40230));
#9295=EDGE_LOOP('',(#40231,#40232,#40233,#40234,#40235,#40236));
#9296=EDGE_LOOP('',(#40237,#40238,#40239,#40240));
#9297=EDGE_LOOP('',(#40241,#40242,#40243,#40244));
#9298=EDGE_LOOP('',(#40245,#40246,#40247,#40248,#40249,#40250));
#9299=EDGE_LOOP('',(#40251,#40252,#40253,#40254));
#9300=EDGE_LOOP('',(#40255,#40256,#40257,#40258));
#9301=EDGE_LOOP('',(#40259,#40260,#40261,#40262,#40263,#40264));
#9302=EDGE_LOOP('',(#40265,#40266,#40267,#40268,#40269,#40270));
#9303=EDGE_LOOP('',(#40271,#40272,#40273,#40274));
#9304=EDGE_LOOP('',(#40275,#40276,#40277));
#9305=EDGE_LOOP('',(#40278,#40279,#40280));
#9306=EDGE_LOOP('',(#40281,#40282,#40283,#40284));
#9307=EDGE_LOOP('',(#40285,#40286,#40287,#40288));
#9308=EDGE_LOOP('',(#40289,#40290,#40291,#40292));
#9309=EDGE_LOOP('',(#40293,#40294,#40295,#40296,#40297,#40298));
#9310=EDGE_LOOP('',(#40299,#40300,#40301,#40302));
#9311=EDGE_LOOP('',(#40303,#40304,#40305,#40306));
#9312=EDGE_LOOP('',(#40307,#40308,#40309,#40310,#40311,#40312));
#9313=EDGE_LOOP('',(#40313,#40314,#40315,#40316));
#9314=EDGE_LOOP('',(#40317,#40318,#40319,#40320));
#9315=EDGE_LOOP('',(#40321,#40322,#40323,#40324,#40325,#40326));
#9316=EDGE_LOOP('',(#40327,#40328,#40329,#40330));
#9317=EDGE_LOOP('',(#40331,#40332,#40333,#40334));
#9318=EDGE_LOOP('',(#40335,#40336,#40337,#40338,#40339,#40340));
#9319=EDGE_LOOP('',(#40341,#40342,#40343,#40344));
#9320=EDGE_LOOP('',(#40345,#40346,#40347,#40348));
#9321=EDGE_LOOP('',(#40349,#40350,#40351,#40352,#40353,#40354));
#9322=EDGE_LOOP('',(#40355,#40356,#40357,#40358));
#9323=EDGE_LOOP('',(#40359,#40360,#40361,#40362));
#9324=EDGE_LOOP('',(#40363,#40364,#40365,#40366,#40367,#40368));
#9325=EDGE_LOOP('',(#40369,#40370,#40371,#40372,#40373,#40374));
#9326=EDGE_LOOP('',(#40375,#40376,#40377,#40378));
#9327=EDGE_LOOP('',(#40379,#40380,#40381));
#9686=LINE('',#63527,#11670);
#9687=LINE('',#63539,#11671);
#9688=LINE('',#64446,#11672);
#9689=LINE('',#65232,#11673);
#9690=LINE('',#65258,#11674);
#9691=LINE('',#65271,#11675);
#9692=LINE('',#65276,#11676);
#9693=LINE('',#65296,#11677);
#9694=LINE('',#65325,#11678);
#9695=LINE('',#65343,#11679);
#9696=LINE('',#65374,#11680);
#9697=LINE('',#65410,#11681);
#9698=LINE('',#65415,#11682);
#9699=LINE('',#65430,#11683);
#9700=LINE('',#65435,#11684);
#9701=LINE('',#65452,#11685);
#9702=LINE('',#65481,#11686);
#9703=LINE('',#65500,#11687);
#9704=LINE('',#65511,#11688);
#9705=LINE('',#65566,#11689);
#9706=LINE('',#65571,#11690);
#9707=LINE('',#65583,#11691);
#9708=LINE('',#65588,#11692);
#9709=LINE('',#65605,#11693);
#9710=LINE('',#65634,#11694);
#9711=LINE('',#65664,#11695);
#9712=LINE('',#65675,#11696);
#9713=LINE('',#65713,#11697);
#9714=LINE('',#65718,#11698);
#9715=LINE('',#65739,#11699);
#9716=LINE('',#65757,#11700);
#9717=LINE('',#65774,#11701);
#9718=LINE('',#65803,#11702);
#9719=LINE('',#65829,#11703);
#9720=LINE('',#65841,#11704);
#9721=LINE('',#65894,#11705);
#9722=LINE('',#65899,#11706);
#9723=LINE('',#65914,#11707);
#9724=LINE('',#65919,#11708);
#9725=LINE('',#65936,#11709);
#9726=LINE('',#65965,#11710);
#9727=LINE('',#65991,#11711);
#9728=LINE('',#66009,#11712);
#9729=LINE('',#66045,#11713);
#9730=LINE('',#66050,#11714);
#9731=LINE('',#66072,#11715);
#9732=LINE('',#66077,#11716);
#9733=LINE('',#66094,#11717);
#9734=LINE('',#66123,#11718);
#9735=LINE('',#66141,#11719);
#9736=LINE('',#66159,#11720);
#9737=LINE('',#66178,#11721);
#9738=LINE('',#66194,#11722);
#9739=LINE('',#66199,#11723);
#9740=LINE('',#66224,#11724);
#9741=LINE('',#66241,#11725);
#9742=LINE('',#66273,#11726);
#9743=LINE('',#66299,#11727);
#9744=LINE('',#66317,#11728);
#9745=LINE('',#66322,#11729);
#9746=LINE('',#66339,#11730);
#9747=LINE('',#66373,#11731);
#9748=LINE('',#66388,#11732);
#9749=LINE('',#66393,#11733);
#9750=LINE('',#66412,#11734);
#9751=LINE('',#66435,#11735);
#9752=LINE('',#66481,#11736);
#9753=LINE('',#66486,#11737);
#9754=LINE('',#66503,#11738);
#9755=LINE('',#66539,#11739);
#9756=LINE('',#66562,#11740);
#9757=LINE('',#66567,#11741);
#9758=LINE('',#66584,#11742);
#9759=LINE('',#66609,#11743);
#9760=LINE('',#66637,#11744);
#9761=LINE('',#66642,#11745);
#9762=LINE('',#66659,#11746);
#9763=LINE('',#66691,#11747);
#9764=LINE('',#66715,#11748);
#9765=LINE('',#66720,#11749);
#9766=LINE('',#66737,#11750);
#9767=LINE('',#66761,#11751);
#9768=LINE('',#66765,#11752);
#9769=LINE('',#66799,#11753);
#9770=LINE('',#66825,#11754);
#9771=LINE('',#66843,#11755);
#9772=LINE('',#66848,#11756);
#9773=LINE('',#66865,#11757);
#9774=LINE('',#66899,#11758);
#9775=LINE('',#66920,#11759);
#9776=LINE('',#66925,#11760);
#9777=LINE('',#66942,#11761);
#9778=LINE('',#66967,#11762);
#9779=LINE('',#67001,#11763);
#9780=LINE('',#67006,#11764);
#9781=LINE('',#67036,#11765);
#9782=LINE('',#67059,#11766);
#9783=LINE('',#67091,#11767);
#9784=LINE('',#67096,#11768);
#9785=LINE('',#67113,#11769);
#9786=LINE('',#67138,#11770);
#9787=LINE('',#67166,#11771);
#9788=LINE('',#67171,#11772);
#9789=LINE('',#67188,#11773);
#9790=LINE('',#67213,#11774);
#9791=LINE('',#67237,#11775);
#9792=LINE('',#67242,#11776);
#9793=LINE('',#67259,#11777);
#9794=LINE('',#67283,#11778);
#9795=LINE('',#67287,#11779);
#9796=LINE('',#67321,#11780);
#9797=LINE('',#67347,#11781);
#9798=LINE('',#67365,#11782);
#9799=LINE('',#67370,#11783);
#9800=LINE('',#67387,#11784);
#9801=LINE('',#67421,#11785);
#9802=LINE('',#67442,#11786);
#9803=LINE('',#67447,#11787);
#9804=LINE('',#67464,#11788);
#9805=LINE('',#67489,#11789);
#9806=LINE('',#67529,#11790);
#9807=LINE('',#67534,#11791);
#9808=LINE('',#67551,#11792);
#9809=LINE('',#67587,#11793);
#9810=LINE('',#67602,#11794);
#9811=LINE('',#67607,#11795);
#9812=LINE('',#67626,#11796);
#9813=LINE('',#67654,#11797);
#9814=LINE('',#67688,#11798);
#9815=LINE('',#67693,#11799);
#9816=LINE('',#67710,#11800);
#9817=LINE('',#67735,#11801);
#9818=LINE('',#67756,#11802);
#9819=LINE('',#67761,#11803);
#9820=LINE('',#67778,#11804);
#9821=LINE('',#67795,#11805);
#9822=LINE('',#67799,#11806);
#9823=LINE('',#67833,#11807);
#9824=LINE('',#67859,#11808);
#9825=LINE('',#67877,#11809);
#9826=LINE('',#67882,#11810);
#9827=LINE('',#67899,#11811);
#9828=LINE('',#67933,#11812);
#9829=LINE('',#67954,#11813);
#9830=LINE('',#67959,#11814);
#9831=LINE('',#67976,#11815);
#9832=LINE('',#68001,#11816);
#9833=LINE('',#68041,#11817);
#9834=LINE('',#68046,#11818);
#9835=LINE('',#68063,#11819);
#9836=LINE('',#68099,#11820);
#9837=LINE('',#68125,#11821);
#9838=LINE('',#68130,#11822);
#9839=LINE('',#68147,#11823);
#9840=LINE('',#68172,#11824);
#9841=LINE('',#68194,#11825);
#9842=LINE('',#68199,#11826);
#9843=LINE('',#68218,#11827);
#9844=LINE('',#68241,#11828);
#9845=LINE('',#68268,#11829);
#9846=LINE('',#68273,#11830);
#9847=LINE('',#68290,#11831);
#9848=LINE('',#68307,#11832);
#9849=LINE('',#68311,#11833);
#9850=LINE('',#68345,#11834);
#9851=LINE('',#68371,#11835);
#9852=LINE('',#68389,#11836);
#9853=LINE('',#68394,#11837);
#9854=LINE('',#68411,#11838);
#9855=LINE('',#68445,#11839);
#9856=LINE('',#68466,#11840);
#9857=LINE('',#68471,#11841);
#9858=LINE('',#68488,#11842);
#9859=LINE('',#68513,#11843);
#9860=LINE('',#68553,#11844);
#9861=LINE('',#68558,#11845);
#9862=LINE('',#68575,#11846);
#9863=LINE('',#68611,#11847);
#9864=LINE('',#68637,#11848);
#9865=LINE('',#68642,#11849);
#9866=LINE('',#68659,#11850);
#9867=LINE('',#68684,#11851);
#9868=LINE('',#68712,#11852);
#9869=LINE('',#68717,#11853);
#9870=LINE('',#68734,#11854);
#9871=LINE('',#68759,#11855);
#9872=LINE('',#68777,#11856);
#9873=LINE('',#68782,#11857);
#9874=LINE('',#68793,#11858);
#9875=LINE('',#68816,#11859);
#9876=LINE('',#68826,#11860);
#9877=LINE('',#68860,#11861);
#9878=LINE('',#68886,#11862);
#9879=LINE('',#68904,#11863);
#9880=LINE('',#68909,#11864);
#9881=LINE('',#68926,#11865);
#9882=LINE('',#68960,#11866);
#9883=LINE('',#68981,#11867);
#9884=LINE('',#68986,#11868);
#9885=LINE('',#69003,#11869);
#9886=LINE('',#69028,#11870);
#9887=LINE('',#69068,#11871);
#9888=LINE('',#69073,#11872);
#9889=LINE('',#69090,#11873);
#9890=LINE('',#69126,#11874);
#9891=LINE('',#69152,#11875);
#9892=LINE('',#69157,#11876);
#9893=LINE('',#69174,#11877);
#9894=LINE('',#69199,#11878);
#9895=LINE('',#69227,#11879);
#9896=LINE('',#69232,#11880);
#9897=LINE('',#69249,#11881);
#9898=LINE('',#69274,#11882);
#9899=LINE('',#69298,#11883);
#9900=LINE('',#69303,#11884);
#9901=LINE('',#69320,#11885);
#9902=LINE('',#69337,#11886);
#9903=LINE('',#69341,#11887);
#9904=LINE('',#69375,#11888);
#9905=LINE('',#69401,#11889);
#9906=LINE('',#69419,#11890);
#9907=LINE('',#69424,#11891);
#9908=LINE('',#69441,#11892);
#9909=LINE('',#69475,#11893);
#9910=LINE('',#69496,#11894);
#9911=LINE('',#69501,#11895);
#9912=LINE('',#69518,#11896);
#9913=LINE('',#69543,#11897);
#9914=LINE('',#69583,#11898);
#9915=LINE('',#69588,#11899);
#9916=LINE('',#69605,#11900);
#9917=LINE('',#69641,#11901);
#9918=LINE('',#69667,#11902);
#9919=LINE('',#69672,#11903);
#9920=LINE('',#69689,#11904);
#9921=LINE('',#69714,#11905);
#9922=LINE('',#69742,#11906);
#9923=LINE('',#69747,#11907);
#9924=LINE('',#69764,#11908);
#9925=LINE('',#69789,#11909);
#9926=LINE('',#69813,#11910);
#9927=LINE('',#69818,#11911);
#9928=LINE('',#69835,#11912);
#9929=LINE('',#69852,#11913);
#9930=LINE('',#69856,#11914);
#9931=LINE('',#69890,#11915);
#9932=LINE('',#69916,#11916);
#9933=LINE('',#69934,#11917);
#9934=LINE('',#69939,#11918);
#9935=LINE('',#69956,#11919);
#9936=LINE('',#69990,#11920);
#9937=LINE('',#70011,#11921);
#9938=LINE('',#70016,#11922);
#9939=LINE('',#70033,#11923);
#9940=LINE('',#70058,#11924);
#9941=LINE('',#70098,#11925);
#9942=LINE('',#70103,#11926);
#9943=LINE('',#70120,#11927);
#9944=LINE('',#70156,#11928);
#9945=LINE('',#70182,#11929);
#9946=LINE('',#70187,#11930);
#9947=LINE('',#70204,#11931);
#9948=LINE('',#70229,#11932);
#9949=LINE('',#70257,#11933);
#9950=LINE('',#70262,#11934);
#9951=LINE('',#70279,#11935);
#9952=LINE('',#70304,#11936);
#9953=LINE('',#70328,#11937);
#9954=LINE('',#70333,#11938);
#9955=LINE('',#70350,#11939);
#9956=LINE('',#70367,#11940);
#9957=LINE('',#70371,#11941);
#9958=LINE('',#70405,#11942);
#9959=LINE('',#70431,#11943);
#9960=LINE('',#70449,#11944);
#9961=LINE('',#70454,#11945);
#9962=LINE('',#70471,#11946);
#9963=LINE('',#70505,#11947);
#9964=LINE('',#70526,#11948);
#9965=LINE('',#70531,#11949);
#9966=LINE('',#70548,#11950);
#9967=LINE('',#70573,#11951);
#9968=LINE('',#70613,#11952);
#9969=LINE('',#70618,#11953);
#9970=LINE('',#70635,#11954);
#9971=LINE('',#70671,#11955);
#9972=LINE('',#70697,#11956);
#9973=LINE('',#70702,#11957);
#9974=LINE('',#70719,#11958);
#9975=LINE('',#70744,#11959);
#9976=LINE('',#70772,#11960);
#9977=LINE('',#70777,#11961);
#9978=LINE('',#70794,#11962);
#9979=LINE('',#70819,#11963);
#9980=LINE('',#70843,#11964);
#9981=LINE('',#70848,#11965);
#9982=LINE('',#70865,#11966);
#9983=LINE('',#70882,#11967);
#9984=LINE('',#70886,#11968);
#9985=LINE('',#70920,#11969);
#9986=LINE('',#70946,#11970);
#9987=LINE('',#70964,#11971);
#9988=LINE('',#70969,#11972);
#9989=LINE('',#70986,#11973);
#9990=LINE('',#71020,#11974);
#9991=LINE('',#71041,#11975);
#9992=LINE('',#71046,#11976);
#9993=LINE('',#71063,#11977);
#9994=LINE('',#71088,#11978);
#9995=LINE('',#71128,#11979);
#9996=LINE('',#71133,#11980);
#9997=LINE('',#71150,#11981);
#9998=LINE('',#71186,#11982);
#9999=LINE('',#71212,#11983);
#10000=LINE('',#71217,#11984);
#10001=LINE('',#71234,#11985);
#10002=LINE('',#71259,#11986);
#10003=LINE('',#71287,#11987);
#10004=LINE('',#71292,#11988);
#10005=LINE('',#71309,#11989);
#10006=LINE('',#71334,#11990);
#10007=LINE('',#71358,#11991);
#10008=LINE('',#71363,#11992);
#10009=LINE('',#71380,#11993);
#10010=LINE('',#71397,#11994);
#10011=LINE('',#71401,#11995);
#10012=LINE('',#71435,#11996);
#10013=LINE('',#71461,#11997);
#10014=LINE('',#71479,#11998);
#10015=LINE('',#71484,#11999);
#10016=LINE('',#71501,#12000);
#10017=LINE('',#71535,#12001);
#10018=LINE('',#71556,#12002);
#10019=LINE('',#71561,#12003);
#10020=LINE('',#71578,#12004);
#10021=LINE('',#71603,#12005);
#10022=LINE('',#71643,#12006);
#10023=LINE('',#71648,#12007);
#10024=LINE('',#71665,#12008);
#10025=LINE('',#71701,#12009);
#10026=LINE('',#71727,#12010);
#10027=LINE('',#71732,#12011);
#10028=LINE('',#71749,#12012);
#10029=LINE('',#71774,#12013);
#10030=LINE('',#71802,#12014);
#10031=LINE('',#71807,#12015);
#10032=LINE('',#71824,#12016);
#10033=LINE('',#71849,#12017);
#10034=LINE('',#71873,#12018);
#10035=LINE('',#71878,#12019);
#10036=LINE('',#71895,#12020);
#10037=LINE('',#71912,#12021);
#10038=LINE('',#71916,#12022);
#10039=LINE('',#71950,#12023);
#10040=LINE('',#71976,#12024);
#10041=LINE('',#71994,#12025);
#10042=LINE('',#71999,#12026);
#10043=LINE('',#72016,#12027);
#10044=LINE('',#72050,#12028);
#10045=LINE('',#72071,#12029);
#10046=LINE('',#72076,#12030);
#10047=LINE('',#72093,#12031);
#10048=LINE('',#72118,#12032);
#10049=LINE('',#72158,#12033);
#10050=LINE('',#72163,#12034);
#10051=LINE('',#72180,#12035);
#10052=LINE('',#72216,#12036);
#10053=LINE('',#72242,#12037);
#10054=LINE('',#72247,#12038);
#10055=LINE('',#72264,#12039);
#10056=LINE('',#72289,#12040);
#10057=LINE('',#72317,#12041);
#10058=LINE('',#72322,#12042);
#10059=LINE('',#72339,#12043);
#10060=LINE('',#72364,#12044);
#10061=LINE('',#72388,#12045);
#10062=LINE('',#72393,#12046);
#10063=LINE('',#72410,#12047);
#10064=LINE('',#72427,#12048);
#10065=LINE('',#72431,#12049);
#10066=LINE('',#72465,#12050);
#10067=LINE('',#72491,#12051);
#10068=LINE('',#72509,#12052);
#10069=LINE('',#72514,#12053);
#10070=LINE('',#72531,#12054);
#10071=LINE('',#72565,#12055);
#10072=LINE('',#72586,#12056);
#10073=LINE('',#72591,#12057);
#10074=LINE('',#72608,#12058);
#10075=LINE('',#72633,#12059);
#10076=LINE('',#72673,#12060);
#10077=LINE('',#72678,#12061);
#10078=LINE('',#72695,#12062);
#10079=LINE('',#72731,#12063);
#10080=LINE('',#72757,#12064);
#10081=LINE('',#72762,#12065);
#10082=LINE('',#72779,#12066);
#10083=LINE('',#72804,#12067);
#10084=LINE('',#72832,#12068);
#10085=LINE('',#72837,#12069);
#10086=LINE('',#72854,#12070);
#10087=LINE('',#72879,#12071);
#10088=LINE('',#72903,#12072);
#10089=LINE('',#72908,#12073);
#10090=LINE('',#72925,#12074);
#10091=LINE('',#72942,#12075);
#10092=LINE('',#72946,#12076);
#10093=LINE('',#72980,#12077);
#10094=LINE('',#73006,#12078);
#10095=LINE('',#73024,#12079);
#10096=LINE('',#73029,#12080);
#10097=LINE('',#73046,#12081);
#10098=LINE('',#73080,#12082);
#10099=LINE('',#73098,#12083);
#10100=LINE('',#73103,#12084);
#10101=LINE('',#73120,#12085);
#10102=LINE('',#73152,#12086);
#10103=LINE('',#73192,#12087);
#10104=LINE('',#73197,#12088);
#10105=LINE('',#73214,#12089);
#10106=LINE('',#73250,#12090);
#10107=LINE('',#73276,#12091);
#10108=LINE('',#73281,#12092);
#10109=LINE('',#73298,#12093);
#10110=LINE('',#73323,#12094);
#10111=LINE('',#73351,#12095);
#10112=LINE('',#73356,#12096);
#10113=LINE('',#73373,#12097);
#10114=LINE('',#73398,#12098);
#10115=LINE('',#73422,#12099);
#10116=LINE('',#73427,#12100);
#10117=LINE('',#73444,#12101);
#10118=LINE('',#73461,#12102);
#10119=LINE('',#73465,#12103);
#10120=LINE('',#73499,#12104);
#10121=LINE('',#73525,#12105);
#10122=LINE('',#73543,#12106);
#10123=LINE('',#73548,#12107);
#10124=LINE('',#73565,#12108);
#10125=LINE('',#73599,#12109);
#10126=LINE('',#73620,#12110);
#10127=LINE('',#73625,#12111);
#10128=LINE('',#73642,#12112);
#10129=LINE('',#73667,#12113);
#10130=LINE('',#73707,#12114);
#10131=LINE('',#73712,#12115);
#10132=LINE('',#73729,#12116);
#10133=LINE('',#73765,#12117);
#10134=LINE('',#73791,#12118);
#10135=LINE('',#73796,#12119);
#10136=LINE('',#73813,#12120);
#10137=LINE('',#73838,#12121);
#10138=LINE('',#73866,#12122);
#10139=LINE('',#73871,#12123);
#10140=LINE('',#73888,#12124);
#10141=LINE('',#73913,#12125);
#10142=LINE('',#73937,#12126);
#10143=LINE('',#73942,#12127);
#10144=LINE('',#73959,#12128);
#10145=LINE('',#73976,#12129);
#10146=LINE('',#73980,#12130);
#10147=LINE('',#74014,#12131);
#10148=LINE('',#74040,#12132);
#10149=LINE('',#74058,#12133);
#10150=LINE('',#74063,#12134);
#10151=LINE('',#74080,#12135);
#10152=LINE('',#74114,#12136);
#10153=LINE('',#74135,#12137);
#10154=LINE('',#74140,#12138);
#10155=LINE('',#74157,#12139);
#10156=LINE('',#74182,#12140);
#10157=LINE('',#74222,#12141);
#10158=LINE('',#74227,#12142);
#10159=LINE('',#74244,#12143);
#10160=LINE('',#74280,#12144);
#10161=LINE('',#74306,#12145);
#10162=LINE('',#74311,#12146);
#10163=LINE('',#74328,#12147);
#10164=LINE('',#74353,#12148);
#10165=LINE('',#74381,#12149);
#10166=LINE('',#74386,#12150);
#10167=LINE('',#74403,#12151);
#10168=LINE('',#74428,#12152);
#10169=LINE('',#74452,#12153);
#10170=LINE('',#74457,#12154);
#10171=LINE('',#74474,#12155);
#10172=LINE('',#74491,#12156);
#10173=LINE('',#74495,#12157);
#10174=LINE('',#74529,#12158);
#10175=LINE('',#74555,#12159);
#10176=LINE('',#74573,#12160);
#10177=LINE('',#74578,#12161);
#10178=LINE('',#74595,#12162);
#10179=LINE('',#74629,#12163);
#10180=LINE('',#74650,#12164);
#10181=LINE('',#74655,#12165);
#10182=LINE('',#74672,#12166);
#10183=LINE('',#74697,#12167);
#10184=LINE('',#74737,#12168);
#10185=LINE('',#74742,#12169);
#10186=LINE('',#74759,#12170);
#10187=LINE('',#74795,#12171);
#10188=LINE('',#74821,#12172);
#10189=LINE('',#74826,#12173);
#10190=LINE('',#74843,#12174);
#10191=LINE('',#74868,#12175);
#10192=LINE('',#74896,#12176);
#10193=LINE('',#74901,#12177);
#10194=LINE('',#74918,#12178);
#10195=LINE('',#74943,#12179);
#10196=LINE('',#74967,#12180);
#10197=LINE('',#74972,#12181);
#10198=LINE('',#74989,#12182);
#10199=LINE('',#75006,#12183);
#10200=LINE('',#75010,#12184);
#10201=LINE('',#75044,#12185);
#10202=LINE('',#75070,#12186);
#10203=LINE('',#75088,#12187);
#10204=LINE('',#75093,#12188);
#10205=LINE('',#75110,#12189);
#10206=LINE('',#75144,#12190);
#10207=LINE('',#75165,#12191);
#10208=LINE('',#75170,#12192);
#10209=LINE('',#75187,#12193);
#10210=LINE('',#75212,#12194);
#10211=LINE('',#75252,#12195);
#10212=LINE('',#75257,#12196);
#10213=LINE('',#75274,#12197);
#10214=LINE('',#75310,#12198);
#10215=LINE('',#75336,#12199);
#10216=LINE('',#75341,#12200);
#10217=LINE('',#75358,#12201);
#10218=LINE('',#75383,#12202);
#10219=LINE('',#75411,#12203);
#10220=LINE('',#75416,#12204);
#10221=LINE('',#75433,#12205);
#10222=LINE('',#75458,#12206);
#10223=LINE('',#75482,#12207);
#10224=LINE('',#75487,#12208);
#10225=LINE('',#75504,#12209);
#10226=LINE('',#75521,#12210);
#10227=LINE('',#75525,#12211);
#10228=LINE('',#75559,#12212);
#10229=LINE('',#75585,#12213);
#10230=LINE('',#75603,#12214);
#10231=LINE('',#75608,#12215);
#10232=LINE('',#75625,#12216);
#10233=LINE('',#75659,#12217);
#10234=LINE('',#75677,#12218);
#10235=LINE('',#75682,#12219);
#10236=LINE('',#75699,#12220);
#10237=LINE('',#75731,#12221);
#10238=LINE('',#75771,#12222);
#10239=LINE('',#75776,#12223);
#10240=LINE('',#75793,#12224);
#10241=LINE('',#75829,#12225);
#10242=LINE('',#75855,#12226);
#10243=LINE('',#75860,#12227);
#10244=LINE('',#75877,#12228);
#10245=LINE('',#75902,#12229);
#10246=LINE('',#75930,#12230);
#10247=LINE('',#75935,#12231);
#10248=LINE('',#75952,#12232);
#10249=LINE('',#75977,#12233);
#10250=LINE('',#76001,#12234);
#10251=LINE('',#76006,#12235);
#10252=LINE('',#76023,#12236);
#10253=LINE('',#76040,#12237);
#10254=LINE('',#76044,#12238);
#10255=LINE('',#76078,#12239);
#10256=LINE('',#76104,#12240);
#10257=LINE('',#76122,#12241);
#10258=LINE('',#76127,#12242);
#10259=LINE('',#76144,#12243);
#10260=LINE('',#76178,#12244);
#10261=LINE('',#76199,#12245);
#10262=LINE('',#76204,#12246);
#10263=LINE('',#76221,#12247);
#10264=LINE('',#76246,#12248);
#10265=LINE('',#76285,#12249);
#10266=LINE('',#76290,#12250);
#10267=LINE('',#76307,#12251);
#10268=LINE('',#76338,#12252);
#10269=LINE('',#76364,#12253);
#10270=LINE('',#76369,#12254);
#10271=LINE('',#76386,#12255);
#10272=LINE('',#76411,#12256);
#10273=LINE('',#76439,#12257);
#10274=LINE('',#76444,#12258);
#10275=LINE('',#76461,#12259);
#10276=LINE('',#76486,#12260);
#10277=LINE('',#76510,#12261);
#10278=LINE('',#76515,#12262);
#10279=LINE('',#76532,#12263);
#10280=LINE('',#76549,#12264);
#10281=LINE('',#76553,#12265);
#10282=LINE('',#76587,#12266);
#10283=LINE('',#76613,#12267);
#10284=LINE('',#76631,#12268);
#10285=LINE('',#76636,#12269);
#10286=LINE('',#76653,#12270);
#10287=LINE('',#76687,#12271);
#10288=LINE('',#76705,#12272);
#10289=LINE('',#76710,#12273);
#10290=LINE('',#76727,#12274);
#10291=LINE('',#76759,#12275);
#10292=LINE('',#76799,#12276);
#10293=LINE('',#76804,#12277);
#10294=LINE('',#76821,#12278);
#10295=LINE('',#76857,#12279);
#10296=LINE('',#76880,#12280);
#10297=LINE('',#76885,#12281);
#10298=LINE('',#76902,#12282);
#10299=LINE('',#76934,#12283);
#10300=LINE('',#76962,#12284);
#10301=LINE('',#76967,#12285);
#10302=LINE('',#76984,#12286);
#10303=LINE('',#77009,#12287);
#10304=LINE('',#77033,#12288);
#10305=LINE('',#77038,#12289);
#10306=LINE('',#77055,#12290);
#10307=LINE('',#77072,#12291);
#10308=LINE('',#77076,#12292);
#10309=LINE('',#77110,#12293);
#10310=LINE('',#77136,#12294);
#10311=LINE('',#77154,#12295);
#10312=LINE('',#77159,#12296);
#10313=LINE('',#77176,#12297);
#10314=LINE('',#77210,#12298);
#10315=LINE('',#77231,#12299);
#10316=LINE('',#77236,#12300);
#10317=LINE('',#77253,#12301);
#10318=LINE('',#77278,#12302);
#10319=LINE('',#77318,#12303);
#10320=LINE('',#77323,#12304);
#10321=LINE('',#77340,#12305);
#10322=LINE('',#77376,#12306);
#10323=LINE('',#77402,#12307);
#10324=LINE('',#77407,#12308);
#10325=LINE('',#77424,#12309);
#10326=LINE('',#77449,#12310);
#10327=LINE('',#77477,#12311);
#10328=LINE('',#77482,#12312);
#10329=LINE('',#77499,#12313);
#10330=LINE('',#77531,#12314);
#10331=LINE('',#77555,#12315);
#10332=LINE('',#77560,#12316);
#10333=LINE('',#77577,#12317);
#10334=LINE('',#77594,#12318);
#10335=LINE('',#77598,#12319);
#10336=LINE('',#77632,#12320);
#10337=LINE('',#77658,#12321);
#10338=LINE('',#77676,#12322);
#10339=LINE('',#77681,#12323);
#10340=LINE('',#77698,#12324);
#10341=LINE('',#77732,#12325);
#10342=LINE('',#77753,#12326);
#10343=LINE('',#77758,#12327);
#10344=LINE('',#77775,#12328);
#10345=LINE('',#77800,#12329);
#10346=LINE('',#77840,#12330);
#10347=LINE('',#77845,#12331);
#10348=LINE('',#77862,#12332);
#10349=LINE('',#77898,#12333);
#10350=LINE('',#77924,#12334);
#10351=LINE('',#77929,#12335);
#10352=LINE('',#77946,#12336);
#10353=LINE('',#77971,#12337);
#10354=LINE('',#77999,#12338);
#10355=LINE('',#78004,#12339);
#10356=LINE('',#78021,#12340);
#10357=LINE('',#78046,#12341);
#10358=LINE('',#78067,#12342);
#10359=LINE('',#78072,#12343);
#10360=LINE('',#78089,#12344);
#10361=LINE('',#78113,#12345);
#10362=LINE('',#78117,#12346);
#10363=LINE('',#78151,#12347);
#10364=LINE('',#78177,#12348);
#10365=LINE('',#78195,#12349);
#10366=LINE('',#78200,#12350);
#10367=LINE('',#78217,#12351);
#10368=LINE('',#78251,#12352);
#10369=LINE('',#78272,#12353);
#10370=LINE('',#78277,#12354);
#10371=LINE('',#78294,#12355);
#10372=LINE('',#78319,#12356);
#10373=LINE('',#78359,#12357);
#10374=LINE('',#78364,#12358);
#10375=LINE('',#78381,#12359);
#10376=LINE('',#78417,#12360);
#10377=LINE('',#78443,#12361);
#10378=LINE('',#78448,#12362);
#10379=LINE('',#78465,#12363);
#10380=LINE('',#78490,#12364);
#10381=LINE('',#78518,#12365);
#10382=LINE('',#78523,#12366);
#10383=LINE('',#78540,#12367);
#10384=LINE('',#78565,#12368);
#10385=LINE('',#78589,#12369);
#10386=LINE('',#78594,#12370);
#10387=LINE('',#78611,#12371);
#10388=LINE('',#78628,#12372);
#10389=LINE('',#78632,#12373);
#10390=LINE('',#78666,#12374);
#10391=LINE('',#78692,#12375);
#10392=LINE('',#78710,#12376);
#10393=LINE('',#78715,#12377);
#10394=LINE('',#78732,#12378);
#10395=LINE('',#78766,#12379);
#10396=LINE('',#78787,#12380);
#10397=LINE('',#78792,#12381);
#10398=LINE('',#78809,#12382);
#10399=LINE('',#78834,#12383);
#10400=LINE('',#78874,#12384);
#10401=LINE('',#78879,#12385);
#10402=LINE('',#78896,#12386);
#10403=LINE('',#78932,#12387);
#10404=LINE('',#78958,#12388);
#10405=LINE('',#78963,#12389);
#10406=LINE('',#78980,#12390);
#10407=LINE('',#79005,#12391);
#10408=LINE('',#79033,#12392);
#10409=LINE('',#79038,#12393);
#10410=LINE('',#79055,#12394);
#10411=LINE('',#79080,#12395);
#10412=LINE('',#79104,#12396);
#10413=LINE('',#79109,#12397);
#10414=LINE('',#79126,#12398);
#10415=LINE('',#79143,#12399);
#10416=LINE('',#79147,#12400);
#10417=LINE('',#79181,#12401);
#10418=LINE('',#79207,#12402);
#10419=LINE('',#79225,#12403);
#10420=LINE('',#79230,#12404);
#10421=LINE('',#79247,#12405);
#10422=LINE('',#79281,#12406);
#10423=LINE('',#79302,#12407);
#10424=LINE('',#79307,#12408);
#10425=LINE('',#79324,#12409);
#10426=LINE('',#79349,#12410);
#10427=LINE('',#79389,#12411);
#10428=LINE('',#79394,#12412);
#10429=LINE('',#79411,#12413);
#10430=LINE('',#79447,#12414);
#10431=LINE('',#79473,#12415);
#10432=LINE('',#79478,#12416);
#10433=LINE('',#79495,#12417);
#10434=LINE('',#79520,#12418);
#10435=LINE('',#79548,#12419);
#10436=LINE('',#79553,#12420);
#10437=LINE('',#79570,#12421);
#10438=LINE('',#79595,#12422);
#10439=LINE('',#79619,#12423);
#10440=LINE('',#79624,#12424);
#10441=LINE('',#79641,#12425);
#10442=LINE('',#79658,#12426);
#10443=LINE('',#79662,#12427);
#10444=LINE('',#79696,#12428);
#10445=LINE('',#79722,#12429);
#10446=LINE('',#79740,#12430);
#10447=LINE('',#79745,#12431);
#10448=LINE('',#79762,#12432);
#10449=LINE('',#79796,#12433);
#10450=LINE('',#79817,#12434);
#10451=LINE('',#79822,#12435);
#10452=LINE('',#79839,#12436);
#10453=LINE('',#79864,#12437);
#10454=LINE('',#79904,#12438);
#10455=LINE('',#79909,#12439);
#10456=LINE('',#79926,#12440);
#10457=LINE('',#79962,#12441);
#10458=LINE('',#79988,#12442);
#10459=LINE('',#79993,#12443);
#10460=LINE('',#80010,#12444);
#10461=LINE('',#80035,#12445);
#10462=LINE('',#80063,#12446);
#10463=LINE('',#80068,#12447);
#10464=LINE('',#80085,#12448);
#10465=LINE('',#80110,#12449);
#10466=LINE('',#80134,#12450);
#10467=LINE('',#80139,#12451);
#10468=LINE('',#80156,#12452);
#10469=LINE('',#80173,#12453);
#10470=LINE('',#80177,#12454);
#10471=LINE('',#80211,#12455);
#10472=LINE('',#80237,#12456);
#10473=LINE('',#80255,#12457);
#10474=LINE('',#80260,#12458);
#10475=LINE('',#80277,#12459);
#10476=LINE('',#80311,#12460);
#10477=LINE('',#80332,#12461);
#10478=LINE('',#80337,#12462);
#10479=LINE('',#80354,#12463);
#10480=LINE('',#80379,#12464);
#10481=LINE('',#80419,#12465);
#10482=LINE('',#80424,#12466);
#10483=LINE('',#80441,#12467);
#10484=LINE('',#80477,#12468);
#10485=LINE('',#80503,#12469);
#10486=LINE('',#80508,#12470);
#10487=LINE('',#80525,#12471);
#10488=LINE('',#80550,#12472);
#10489=LINE('',#80578,#12473);
#10490=LINE('',#80583,#12474);
#10491=LINE('',#80600,#12475);
#10492=LINE('',#80625,#12476);
#10493=LINE('',#80649,#12477);
#10494=LINE('',#80654,#12478);
#10495=LINE('',#80671,#12479);
#10496=LINE('',#80688,#12480);
#10497=LINE('',#80692,#12481);
#10498=LINE('',#80726,#12482);
#10499=LINE('',#80752,#12483);
#10500=LINE('',#80770,#12484);
#10501=LINE('',#80775,#12485);
#10502=LINE('',#80792,#12486);
#10503=LINE('',#80826,#12487);
#10504=LINE('',#80847,#12488);
#10505=LINE('',#80852,#12489);
#10506=LINE('',#80869,#12490);
#10507=LINE('',#80894,#12491);
#10508=LINE('',#80934,#12492);
#10509=LINE('',#80939,#12493);
#10510=LINE('',#80956,#12494);
#10511=LINE('',#80992,#12495);
#10512=LINE('',#81018,#12496);
#10513=LINE('',#81023,#12497);
#10514=LINE('',#81040,#12498);
#10515=LINE('',#81065,#12499);
#10516=LINE('',#81093,#12500);
#10517=LINE('',#81098,#12501);
#10518=LINE('',#81115,#12502);
#10519=LINE('',#81140,#12503);
#10520=LINE('',#81164,#12504);
#10521=LINE('',#81169,#12505);
#10522=LINE('',#81186,#12506);
#10523=LINE('',#81203,#12507);
#10524=LINE('',#81207,#12508);
#10525=LINE('',#81241,#12509);
#10526=LINE('',#81267,#12510);
#10527=LINE('',#81285,#12511);
#10528=LINE('',#81290,#12512);
#10529=LINE('',#81307,#12513);
#10530=LINE('',#81341,#12514);
#10531=LINE('',#81359,#12515);
#10532=LINE('',#81364,#12516);
#10533=LINE('',#81381,#12517);
#10534=LINE('',#81413,#12518);
#10535=LINE('',#81453,#12519);
#10536=LINE('',#81458,#12520);
#10537=LINE('',#81475,#12521);
#10538=LINE('',#81511,#12522);
#10539=LINE('',#81537,#12523);
#10540=LINE('',#81542,#12524);
#10541=LINE('',#81559,#12525);
#10542=LINE('',#81584,#12526);
#10543=LINE('',#81612,#12527);
#10544=LINE('',#81617,#12528);
#10545=LINE('',#81634,#12529);
#10546=LINE('',#81659,#12530);
#10547=LINE('',#81683,#12531);
#10548=LINE('',#81688,#12532);
#10549=LINE('',#81705,#12533);
#10550=LINE('',#81722,#12534);
#10551=LINE('',#81726,#12535);
#10552=LINE('',#81760,#12536);
#10553=LINE('',#81786,#12537);
#10554=LINE('',#81804,#12538);
#10555=LINE('',#81809,#12539);
#10556=LINE('',#81826,#12540);
#10557=LINE('',#81860,#12541);
#10558=LINE('',#81881,#12542);
#10559=LINE('',#81886,#12543);
#10560=LINE('',#81903,#12544);
#10561=LINE('',#81928,#12545);
#10562=LINE('',#81967,#12546);
#10563=LINE('',#81972,#12547);
#10564=LINE('',#81989,#12548);
#10565=LINE('',#82020,#12549);
#10566=LINE('',#82046,#12550);
#10567=LINE('',#82051,#12551);
#10568=LINE('',#82068,#12552);
#10569=LINE('',#82093,#12553);
#10570=LINE('',#82121,#12554);
#10571=LINE('',#82126,#12555);
#10572=LINE('',#82143,#12556);
#10573=LINE('',#82168,#12557);
#10574=LINE('',#82192,#12558);
#10575=LINE('',#82197,#12559);
#10576=LINE('',#82214,#12560);
#10577=LINE('',#82231,#12561);
#10578=LINE('',#82235,#12562);
#10579=LINE('',#82269,#12563);
#10580=LINE('',#82295,#12564);
#10581=LINE('',#82313,#12565);
#10582=LINE('',#82318,#12566);
#10583=LINE('',#82335,#12567);
#10584=LINE('',#82369,#12568);
#10585=LINE('',#82390,#12569);
#10586=LINE('',#82395,#12570);
#10587=LINE('',#82412,#12571);
#10588=LINE('',#82437,#12572);
#10589=LINE('',#82477,#12573);
#10590=LINE('',#82482,#12574);
#10591=LINE('',#82499,#12575);
#10592=LINE('',#82535,#12576);
#10593=LINE('',#82558,#12577);
#10594=LINE('',#82563,#12578);
#10595=LINE('',#82580,#12579);
#10596=LINE('',#82612,#12580);
#10597=LINE('',#82640,#12581);
#10598=LINE('',#82645,#12582);
#10599=LINE('',#82662,#12583);
#10600=LINE('',#82687,#12584);
#10601=LINE('',#82711,#12585);
#10602=LINE('',#82716,#12586);
#10603=LINE('',#82733,#12587);
#10604=LINE('',#82750,#12588);
#10605=LINE('',#82754,#12589);
#10606=LINE('',#82788,#12590);
#10607=LINE('',#82814,#12591);
#10608=LINE('',#82832,#12592);
#10609=LINE('',#82837,#12593);
#10610=LINE('',#82854,#12594);
#10611=LINE('',#82888,#12595);
#10612=LINE('',#82909,#12596);
#10613=LINE('',#82914,#12597);
#10614=LINE('',#82931,#12598);
#10615=LINE('',#82956,#12599);
#10616=LINE('',#82996,#12600);
#10617=LINE('',#83001,#12601);
#10618=LINE('',#83018,#12602);
#10619=LINE('',#83054,#12603);
#10620=LINE('',#83080,#12604);
#10621=LINE('',#83085,#12605);
#10622=LINE('',#83102,#12606);
#10623=LINE('',#83127,#12607);
#10624=LINE('',#83155,#12608);
#10625=LINE('',#83160,#12609);
#10626=LINE('',#83177,#12610);
#10627=LINE('',#83209,#12611);
#10628=LINE('',#83233,#12612);
#10629=LINE('',#83238,#12613);
#10630=LINE('',#83255,#12614);
#10631=LINE('',#83272,#12615);
#10632=LINE('',#83276,#12616);
#10633=LINE('',#83310,#12617);
#10634=LINE('',#83336,#12618);
#10635=LINE('',#83354,#12619);
#10636=LINE('',#83359,#12620);
#10637=LINE('',#83376,#12621);
#10638=LINE('',#83410,#12622);
#10639=LINE('',#83431,#12623);
#10640=LINE('',#83436,#12624);
#10641=LINE('',#83453,#12625);
#10642=LINE('',#83478,#12626);
#10643=LINE('',#83518,#12627);
#10644=LINE('',#83523,#12628);
#10645=LINE('',#83540,#12629);
#10646=LINE('',#83576,#12630);
#10647=LINE('',#83602,#12631);
#10648=LINE('',#83607,#12632);
#10649=LINE('',#83624,#12633);
#10650=LINE('',#83649,#12634);
#10651=LINE('',#83677,#12635);
#10652=LINE('',#83682,#12636);
#10653=LINE('',#83699,#12637);
#10654=LINE('',#83724,#12638);
#10655=LINE('',#83745,#12639);
#10656=LINE('',#83750,#12640);
#10657=LINE('',#83767,#12641);
#10658=LINE('',#83791,#12642);
#10659=LINE('',#83795,#12643);
#10660=LINE('',#83829,#12644);
#10661=LINE('',#83855,#12645);
#10662=LINE('',#83873,#12646);
#10663=LINE('',#83878,#12647);
#10664=LINE('',#83895,#12648);
#10665=LINE('',#83929,#12649);
#10666=LINE('',#83950,#12650);
#10667=LINE('',#83955,#12651);
#10668=LINE('',#83972,#12652);
#10669=LINE('',#83997,#12653);
#10670=LINE('',#84037,#12654);
#10671=LINE('',#84042,#12655);
#10672=LINE('',#84059,#12656);
#10673=LINE('',#84095,#12657);
#10674=LINE('',#84121,#12658);
#10675=LINE('',#84126,#12659);
#10676=LINE('',#84143,#12660);
#10677=LINE('',#84168,#12661);
#10678=LINE('',#84196,#12662);
#10679=LINE('',#84201,#12663);
#10680=LINE('',#84218,#12664);
#10681=LINE('',#84243,#12665);
#10682=LINE('',#84267,#12666);
#10683=LINE('',#84272,#12667);
#10684=LINE('',#84289,#12668);
#10685=LINE('',#84306,#12669);
#10686=LINE('',#84310,#12670);
#10687=LINE('',#84344,#12671);
#10688=LINE('',#84370,#12672);
#10689=LINE('',#84388,#12673);
#10690=LINE('',#84393,#12674);
#10691=LINE('',#84410,#12675);
#10692=LINE('',#84444,#12676);
#10693=LINE('',#84465,#12677);
#10694=LINE('',#84470,#12678);
#10695=LINE('',#84487,#12679);
#10696=LINE('',#84512,#12680);
#10697=LINE('',#84552,#12681);
#10698=LINE('',#84557,#12682);
#10699=LINE('',#84574,#12683);
#10700=LINE('',#84610,#12684);
#10701=LINE('',#84636,#12685);
#10702=LINE('',#84641,#12686);
#10703=LINE('',#84658,#12687);
#10704=LINE('',#84683,#12688);
#10705=LINE('',#84711,#12689);
#10706=LINE('',#84716,#12690);
#10707=LINE('',#84733,#12691);
#10708=LINE('',#84758,#12692);
#10709=LINE('',#84782,#12693);
#10710=LINE('',#84787,#12694);
#10711=LINE('',#84804,#12695);
#10712=LINE('',#84821,#12696);
#10713=LINE('',#84825,#12697);
#10714=LINE('',#84859,#12698);
#10715=LINE('',#84885,#12699);
#10716=LINE('',#84903,#12700);
#10717=LINE('',#84908,#12701);
#10718=LINE('',#84925,#12702);
#10719=LINE('',#84959,#12703);
#10720=LINE('',#84980,#12704);
#10721=LINE('',#84985,#12705);
#10722=LINE('',#85002,#12706);
#10723=LINE('',#85027,#12707);
#10724=LINE('',#85067,#12708);
#10725=LINE('',#85072,#12709);
#10726=LINE('',#85089,#12710);
#10727=LINE('',#85125,#12711);
#10728=LINE('',#85151,#12712);
#10729=LINE('',#85156,#12713);
#10730=LINE('',#85173,#12714);
#10731=LINE('',#85198,#12715);
#10732=LINE('',#85226,#12716);
#10733=LINE('',#85231,#12717);
#10734=LINE('',#85248,#12718);
#10735=LINE('',#85273,#12719);
#10736=LINE('',#85297,#12720);
#10737=LINE('',#85302,#12721);
#10738=LINE('',#85319,#12722);
#10739=LINE('',#85336,#12723);
#10740=LINE('',#85340,#12724);
#10741=LINE('',#85374,#12725);
#10742=LINE('',#85400,#12726);
#10743=LINE('',#85418,#12727);
#10744=LINE('',#85423,#12728);
#10745=LINE('',#85440,#12729);
#10746=LINE('',#85474,#12730);
#10747=LINE('',#85495,#12731);
#10748=LINE('',#85500,#12732);
#10749=LINE('',#85517,#12733);
#10750=LINE('',#85542,#12734);
#10751=LINE('',#85582,#12735);
#10752=LINE('',#85587,#12736);
#10753=LINE('',#85604,#12737);
#10754=LINE('',#85640,#12738);
#10755=LINE('',#85666,#12739);
#10756=LINE('',#85671,#12740);
#10757=LINE('',#85688,#12741);
#10758=LINE('',#85713,#12742);
#10759=LINE('',#85741,#12743);
#10760=LINE('',#85746,#12744);
#10761=LINE('',#85763,#12745);
#10762=LINE('',#85788,#12746);
#10763=LINE('',#85812,#12747);
#10764=LINE('',#85817,#12748);
#10765=LINE('',#85834,#12749);
#10766=LINE('',#85851,#12750);
#10767=LINE('',#85855,#12751);
#10768=LINE('',#85889,#12752);
#10769=LINE('',#85915,#12753);
#10770=LINE('',#85933,#12754);
#10771=LINE('',#85938,#12755);
#10772=LINE('',#85955,#12756);
#10773=LINE('',#85989,#12757);
#10774=LINE('',#86010,#12758);
#10775=LINE('',#86015,#12759);
#10776=LINE('',#86032,#12760);
#10777=LINE('',#86057,#12761);
#10778=LINE('',#86097,#12762);
#10779=LINE('',#86102,#12763);
#10780=LINE('',#86119,#12764);
#10781=LINE('',#86155,#12765);
#10782=LINE('',#86181,#12766);
#10783=LINE('',#86186,#12767);
#10784=LINE('',#86203,#12768);
#10785=LINE('',#86228,#12769);
#10786=LINE('',#86256,#12770);
#10787=LINE('',#86261,#12771);
#10788=LINE('',#86278,#12772);
#10789=LINE('',#86303,#12773);
#10790=LINE('',#86327,#12774);
#10791=LINE('',#86332,#12775);
#10792=LINE('',#86349,#12776);
#10793=LINE('',#86366,#12777);
#10794=LINE('',#86370,#12778);
#10795=LINE('',#86404,#12779);
#10796=LINE('',#86430,#12780);
#10797=LINE('',#86448,#12781);
#10798=LINE('',#86453,#12782);
#10799=LINE('',#86470,#12783);
#10800=LINE('',#86504,#12784);
#10801=LINE('',#86525,#12785);
#10802=LINE('',#86530,#12786);
#10803=LINE('',#86547,#12787);
#10804=LINE('',#86572,#12788);
#10805=LINE('',#86612,#12789);
#10806=LINE('',#86617,#12790);
#10807=LINE('',#86634,#12791);
#10808=LINE('',#86670,#12792);
#10809=LINE('',#86696,#12793);
#10810=LINE('',#86701,#12794);
#10811=LINE('',#86718,#12795);
#10812=LINE('',#86743,#12796);
#10813=LINE('',#86771,#12797);
#10814=LINE('',#86776,#12798);
#10815=LINE('',#86793,#12799);
#10816=LINE('',#86818,#12800);
#10817=LINE('',#86842,#12801);
#10818=LINE('',#86847,#12802);
#10819=LINE('',#86864,#12803);
#10820=LINE('',#86881,#12804);
#10821=LINE('',#86885,#12805);
#10822=LINE('',#86919,#12806);
#10823=LINE('',#86945,#12807);
#10824=LINE('',#86963,#12808);
#10825=LINE('',#86968,#12809);
#10826=LINE('',#86985,#12810);
#10827=LINE('',#87019,#12811);
#10828=LINE('',#87040,#12812);
#10829=LINE('',#87045,#12813);
#10830=LINE('',#87062,#12814);
#10831=LINE('',#87087,#12815);
#10832=LINE('',#87127,#12816);
#10833=LINE('',#87132,#12817);
#10834=LINE('',#87149,#12818);
#10835=LINE('',#87185,#12819);
#10836=LINE('',#87211,#12820);
#10837=LINE('',#87216,#12821);
#10838=LINE('',#87233,#12822);
#10839=LINE('',#87258,#12823);
#10840=LINE('',#87286,#12824);
#10841=LINE('',#87291,#12825);
#10842=LINE('',#87308,#12826);
#10843=LINE('',#87333,#12827);
#10844=LINE('',#87357,#12828);
#10845=LINE('',#87362,#12829);
#10846=LINE('',#87379,#12830);
#10847=LINE('',#87396,#12831);
#10848=LINE('',#87400,#12832);
#10849=LINE('',#87434,#12833);
#10850=LINE('',#87460,#12834);
#10851=LINE('',#87478,#12835);
#10852=LINE('',#87483,#12836);
#10853=LINE('',#87500,#12837);
#10854=LINE('',#87534,#12838);
#10855=LINE('',#87555,#12839);
#10856=LINE('',#87560,#12840);
#10857=LINE('',#87577,#12841);
#10858=LINE('',#87602,#12842);
#10859=LINE('',#87642,#12843);
#10860=LINE('',#87647,#12844);
#10861=LINE('',#87664,#12845);
#10862=LINE('',#87700,#12846);
#10863=LINE('',#87726,#12847);
#10864=LINE('',#87731,#12848);
#10865=LINE('',#87748,#12849);
#10866=LINE('',#87773,#12850);
#10867=LINE('',#87801,#12851);
#10868=LINE('',#87806,#12852);
#10869=LINE('',#87823,#12853);
#10870=LINE('',#87848,#12854);
#10871=LINE('',#87872,#12855);
#10872=LINE('',#87877,#12856);
#10873=LINE('',#87894,#12857);
#10874=LINE('',#87911,#12858);
#10875=LINE('',#87915,#12859);
#10876=LINE('',#87958,#12860);
#10877=LINE('',#87981,#12861);
#10878=LINE('',#87993,#12862);
#10879=LINE('',#87998,#12863);
#10880=LINE('',#88015,#12864);
#10881=LINE('',#88049,#12865);
#10882=LINE('',#88070,#12866);
#10883=LINE('',#88075,#12867);
#10884=LINE('',#88092,#12868);
#10885=LINE('',#88117,#12869);
#10886=LINE('',#88157,#12870);
#10887=LINE('',#88162,#12871);
#10888=LINE('',#88179,#12872);
#10889=LINE('',#88215,#12873);
#10890=LINE('',#88241,#12874);
#10891=LINE('',#88246,#12875);
#10892=LINE('',#88263,#12876);
#10893=LINE('',#88288,#12877);
#10894=LINE('',#88316,#12878);
#10895=LINE('',#88321,#12879);
#10896=LINE('',#88338,#12880);
#10897=LINE('',#88363,#12881);
#10898=LINE('',#88387,#12882);
#10899=LINE('',#88392,#12883);
#10900=LINE('',#88409,#12884);
#10901=LINE('',#88426,#12885);
#10902=LINE('',#88430,#12886);
#10903=LINE('',#88482,#12887);
#10904=LINE('',#88505,#12888);
#10905=LINE('',#88520,#12889);
#10906=LINE('',#88525,#12890);
#10907=LINE('',#88542,#12891);
#10908=LINE('',#88573,#12892);
#10909=LINE('',#88585,#12893);
#10910=LINE('',#88590,#12894);
#10911=LINE('',#88607,#12895);
#10912=LINE('',#88639,#12896);
#10913=LINE('',#88679,#12897);
#10914=LINE('',#88684,#12898);
#10915=LINE('',#88701,#12899);
#10916=LINE('',#88737,#12900);
#10917=LINE('',#88763,#12901);
#10918=LINE('',#88768,#12902);
#10919=LINE('',#88785,#12903);
#10920=LINE('',#88810,#12904);
#10921=LINE('',#88838,#12905);
#10922=LINE('',#88843,#12906);
#10923=LINE('',#88860,#12907);
#10924=LINE('',#88885,#12908);
#10925=LINE('',#88909,#12909);
#10926=LINE('',#88914,#12910);
#10927=LINE('',#88931,#12911);
#10928=LINE('',#88948,#12912);
#10929=LINE('',#88952,#12913);
#10930=LINE('',#88994,#12914);
#10931=LINE('',#88999,#12915);
#10932=LINE('',#89016,#12916);
#10933=LINE('',#89047,#12917);
#10934=LINE('',#89065,#12918);
#10935=LINE('',#89070,#12919);
#10936=LINE('',#89087,#12920);
#10937=LINE('',#89109,#12921);
#10938=LINE('',#89142,#12922);
#10939=LINE('',#89147,#12923);
#10940=LINE('',#89164,#12924);
#10941=LINE('',#89195,#12925);
#10942=LINE('',#89219,#12926);
#10943=LINE('',#89242,#12927);
#10944=LINE('',#89268,#12928);
#10945=LINE('',#89273,#12929);
#10946=LINE('',#89290,#12930);
#10947=LINE('',#89315,#12931);
#10948=LINE('',#89343,#12932);
#10949=LINE('',#89348,#12933);
#10950=LINE('',#89365,#12934);
#10951=LINE('',#89390,#12935);
#10952=LINE('',#89414,#12936);
#10953=LINE('',#89419,#12937);
#10954=LINE('',#89436,#12938);
#10955=LINE('',#89453,#12939);
#10956=LINE('',#89457,#12940);
#10957=LINE('',#89518,#12941);
#10958=LINE('',#89523,#12942);
#10959=LINE('',#89540,#12943);
#10960=LINE('',#89569,#12944);
#10961=LINE('',#89608,#12945);
#10962=LINE('',#89613,#12946);
#10963=LINE('',#89630,#12947);
#10964=LINE('',#89658,#12948);
#10965=LINE('',#89670,#12949);
#10966=LINE('',#89675,#12950);
#10967=LINE('',#89692,#12951);
#10968=LINE('',#89724,#12952);
#10969=LINE('',#89748,#12953);
#10970=LINE('',#89771,#12954);
#10971=LINE('',#89789,#12955);
#10972=LINE('',#89794,#12956);
#10973=LINE('',#89811,#12957);
#10974=LINE('',#89842,#12958);
#10975=LINE('',#89870,#12959);
#10976=LINE('',#89875,#12960);
#10977=LINE('',#89892,#12961);
#10978=LINE('',#89917,#12962);
#10979=LINE('',#89941,#12963);
#10980=LINE('',#89946,#12964);
#10981=LINE('',#89963,#12965);
#10982=LINE('',#89980,#12966);
#10983=LINE('',#89984,#12967);
#10984=LINE('',#90075,#12968);
#10985=LINE('',#90080,#12969);
#10986=LINE('',#90097,#12970);
#10987=LINE('',#90120,#12971);
#10988=LINE('',#90138,#12972);
#10989=LINE('',#90143,#12973);
#10990=LINE('',#90160,#12974);
#10991=LINE('',#90182,#12975);
#10992=LINE('',#90204,#12976);
#10993=LINE('',#90209,#12977);
#10994=LINE('',#90226,#12978);
#10995=LINE('',#90258,#12979);
#10996=LINE('',#90289,#12980);
#10997=LINE('',#90305,#12981);
#10998=LINE('',#90323,#12982);
#10999=LINE('',#90328,#12983);
#11000=LINE('',#90345,#12984);
#11001=LINE('',#90376,#12985);
#11002=LINE('',#90394,#12986);
#11003=LINE('',#90399,#12987);
#11004=LINE('',#90416,#12988);
#11005=LINE('',#90438,#12989);
#11006=LINE('',#90462,#12990);
#11007=LINE('',#90467,#12991);
#11008=LINE('',#90484,#12992);
#11009=LINE('',#90501,#12993);
#11010=LINE('',#90505,#12994);
#11011=LINE('',#90584,#12995);
#11012=LINE('',#90588,#12996);
#11013=LINE('',#90605,#12997);
#11014=LINE('',#90634,#12998);
#11015=LINE('',#90652,#12999);
#11016=LINE('',#90656,#13000);
#11017=LINE('',#90673,#13001);
#11018=LINE('',#90695,#13002);
#11019=LINE('',#90710,#13003);
#11020=LINE('',#90715,#13004);
#11021=LINE('',#90732,#13005);
#11022=LINE('',#90756,#13006);
#11023=LINE('',#90779,#13007);
#11024=LINE('',#90795,#13008);
#11025=LINE('',#90810,#13009);
#11026=LINE('',#90814,#13010);
#11027=LINE('',#90831,#13011);
#11028=LINE('',#90855,#13012);
#11029=LINE('',#90873,#13013);
#11030=LINE('',#90877,#13014);
#11031=LINE('',#90894,#13015);
#11032=LINE('',#90916,#13016);
#11033=LINE('',#90955,#13017);
#11034=LINE('',#90959,#13018);
#11035=LINE('',#90976,#13019);
#11036=LINE('',#91004,#13020);
#11037=LINE('',#91008,#13021);
#11038=LINE('',#91015,#13022);
#11670=VECTOR('',#50547,0.0015);
#11671=VECTOR('',#50552,0.006);
#11672=VECTOR('',#50757,0.0055);
#11673=VECTOR('',#51264,1.);
#11674=VECTOR('',#51267,1.);
#11675=VECTOR('',#51272,0.999999999999999);
#11676=VECTOR('',#51277,1.);
#11677=VECTOR('',#51280,1.);
#11678=VECTOR('',#51287,1.);
#11679=VECTOR('',#51288,1.);
#11680=VECTOR('',#51299,1.);
#11681=VECTOR('',#51324,1.);
#11682=VECTOR('',#51329,1.);
#11683=VECTOR('',#51334,1.);
#11684=VECTOR('',#51339,1.);
#11685=VECTOR('',#51340,1.);
#11686=VECTOR('',#51341,0.999999999999999);
#11687=VECTOR('',#51344,1.);
#11688=VECTOR('',#51345,1.);
#11689=VECTOR('',#51364,1.);
#11690=VECTOR('',#51369,1.);
#11691=VECTOR('',#51374,1.);
#11692=VECTOR('',#51379,1.);
#11693=VECTOR('',#51380,0.999999999999999);
#11694=VECTOR('',#51381,1.);
#11695=VECTOR('',#51382,1.);
#11696=VECTOR('',#51383,1.);
#11697=VECTOR('',#51404,1.);
#11698=VECTOR('',#51409,1.);
#11699=VECTOR('',#51414,1.);
#11700=VECTOR('',#51415,1.);
#11701=VECTOR('',#51416,1.);
#11702=VECTOR('',#51417,1.);
#11703=VECTOR('',#51420,1.);
#11704=VECTOR('',#51421,1.);
#11705=VECTOR('',#51440,1.);
#11706=VECTOR('',#51445,1.);
#11707=VECTOR('',#51450,1.);
#11708=VECTOR('',#51455,1.);
#11709=VECTOR('',#51456,1.);
#11710=VECTOR('',#51457,1.);
#11711=VECTOR('',#51460,1.);
#11712=VECTOR('',#51461,1.);
#11713=VECTOR('',#51484,1.);
#11714=VECTOR('',#51489,0.01);
#11715=VECTOR('',#51494,1.);
#11716=VECTOR('',#51499,1.);
#11717=VECTOR('',#51500,1.);
#11718=VECTOR('',#51501,1.);
#11719=VECTOR('',#51504,0.01);
#11720=VECTOR('',#51505,1.);
#11721=VECTOR('',#51520,0.01);
#11722=VECTOR('',#51527,0.01);
#11723=VECTOR('',#51532,1.);
#11724=VECTOR('',#51537,1.);
#11725=VECTOR('',#51538,0.01);
#11726=VECTOR('',#51547,1.);
#11727=VECTOR('',#51550,1.);
#11728=VECTOR('',#51563,1.);
#11729=VECTOR('',#51568,1.);
#11730=VECTOR('',#51569,1.);
#11731=VECTOR('',#51576,1.);
#11732=VECTOR('',#51581,1.);
#11733=VECTOR('',#51586,1.);
#11734=VECTOR('',#51589,1.);
#11735=VECTOR('',#51598,1.);
#11736=VECTOR('',#51607,1.);
#11737=VECTOR('',#51612,1.);
#11738=VECTOR('',#51613,1.);
#11739=VECTOR('',#51614,1.);
#11740=VECTOR('',#51625,1.);
#11741=VECTOR('',#51630,1.);
#11742=VECTOR('',#51631,1.);
#11743=VECTOR('',#51634,1.);
#11744=VECTOR('',#51647,1.);
#11745=VECTOR('',#51652,1.);
#11746=VECTOR('',#51653,1.);
#11747=VECTOR('',#51656,1.);
#11748=VECTOR('',#51669,1.);
#11749=VECTOR('',#51674,0.01);
#11750=VECTOR('',#51675,1.);
#11751=VECTOR('',#51678,0.01);
#11752=VECTOR('',#51683,0.01);
#11753=VECTOR('',#51696,1.);
#11754=VECTOR('',#51699,1.);
#11755=VECTOR('',#51712,1.);
#11756=VECTOR('',#51717,1.);
#11757=VECTOR('',#51718,1.);
#11758=VECTOR('',#51725,1.);
#11759=VECTOR('',#51738,0.999999999999999);
#11760=VECTOR('',#51743,1.);
#11761=VECTOR('',#51744,1.);
#11762=VECTOR('',#51747,1.);
#11763=VECTOR('',#51748,1.);
#11764=VECTOR('',#51753,1.);
#11765=VECTOR('',#51754,1.);
#11766=VECTOR('',#51763,1.);
#11767=VECTOR('',#51774,1.);
#11768=VECTOR('',#51779,1.);
#11769=VECTOR('',#51780,1.);
#11770=VECTOR('',#51783,1.);
#11771=VECTOR('',#51796,1.);
#11772=VECTOR('',#51801,1.);
#11773=VECTOR('',#51802,1.);
#11774=VECTOR('',#51805,1.);
#11775=VECTOR('',#51818,1.);
#11776=VECTOR('',#51823,0.01);
#11777=VECTOR('',#51824,1.);
#11778=VECTOR('',#51827,0.01);
#11779=VECTOR('',#51832,0.01);
#11780=VECTOR('',#51845,1.);
#11781=VECTOR('',#51848,1.);
#11782=VECTOR('',#51861,1.);
#11783=VECTOR('',#51866,1.);
#11784=VECTOR('',#51867,1.);
#11785=VECTOR('',#51874,1.);
#11786=VECTOR('',#51887,1.);
#11787=VECTOR('',#51892,1.);
#11788=VECTOR('',#51893,1.);
#11789=VECTOR('',#51896,1.);
#11790=VECTOR('',#51905,1.);
#11791=VECTOR('',#51910,1.);
#11792=VECTOR('',#51911,1.);
#11793=VECTOR('',#51912,1.);
#11794=VECTOR('',#51917,1.);
#11795=VECTOR('',#51922,1.);
#11796=VECTOR('',#51925,1.);
#11797=VECTOR('',#51932,1.);
#11798=VECTOR('',#51945,1.);
#11799=VECTOR('',#51950,1.);
#11800=VECTOR('',#51951,1.);
#11801=VECTOR('',#51954,1.);
#11802=VECTOR('',#51967,1.);
#11803=VECTOR('',#51972,0.01);
#11804=VECTOR('',#51973,1.);
#11805=VECTOR('',#51976,0.01);
#11806=VECTOR('',#51981,0.01);
#11807=VECTOR('',#51994,1.);
#11808=VECTOR('',#51997,1.);
#11809=VECTOR('',#52010,1.);
#11810=VECTOR('',#52015,1.);
#11811=VECTOR('',#52016,1.);
#11812=VECTOR('',#52023,1.);
#11813=VECTOR('',#52036,1.);
#11814=VECTOR('',#52041,1.);
#11815=VECTOR('',#52042,1.);
#11816=VECTOR('',#52045,1.);
#11817=VECTOR('',#52054,1.);
#11818=VECTOR('',#52059,1.);
#11819=VECTOR('',#52060,1.);
#11820=VECTOR('',#52061,1.);
#11821=VECTOR('',#52072,1.);
#11822=VECTOR('',#52077,1.);
#11823=VECTOR('',#52078,1.);
#11824=VECTOR('',#52081,1.);
#11825=VECTOR('',#52086,1.);
#11826=VECTOR('',#52091,1.);
#11827=VECTOR('',#52094,1.);
#11828=VECTOR('',#52103,1.);
#11829=VECTOR('',#52116,0.999999999999999);
#11830=VECTOR('',#52121,0.01);
#11831=VECTOR('',#52122,1.);
#11832=VECTOR('',#52125,0.01);
#11833=VECTOR('',#52130,0.01);
#11834=VECTOR('',#52143,1.);
#11835=VECTOR('',#52146,1.);
#11836=VECTOR('',#52159,1.);
#11837=VECTOR('',#52164,1.);
#11838=VECTOR('',#52165,1.);
#11839=VECTOR('',#52172,1.);
#11840=VECTOR('',#52185,1.);
#11841=VECTOR('',#52190,1.);
#11842=VECTOR('',#52191,1.);
#11843=VECTOR('',#52194,1.);
#11844=VECTOR('',#52203,1.);
#11845=VECTOR('',#52208,1.);
#11846=VECTOR('',#52209,1.);
#11847=VECTOR('',#52210,1.);
#11848=VECTOR('',#52221,1.);
#11849=VECTOR('',#52226,1.);
#11850=VECTOR('',#52227,1.);
#11851=VECTOR('',#52230,1.);
#11852=VECTOR('',#52243,1.);
#11853=VECTOR('',#52248,1.);
#11854=VECTOR('',#52249,1.);
#11855=VECTOR('',#52252,1.);
#11856=VECTOR('',#52257,1.);
#11857=VECTOR('',#52262,0.01);
#11858=VECTOR('',#52265,0.01);
#11859=VECTOR('',#52274,1.);
#11860=VECTOR('',#52279,0.01);
#11861=VECTOR('',#52292,1.);
#11862=VECTOR('',#52295,1.);
#11863=VECTOR('',#52308,1.);
#11864=VECTOR('',#52313,1.);
#11865=VECTOR('',#52314,1.);
#11866=VECTOR('',#52321,1.);
#11867=VECTOR('',#52334,1.);
#11868=VECTOR('',#52339,1.);
#11869=VECTOR('',#52340,1.);
#11870=VECTOR('',#52343,1.);
#11871=VECTOR('',#52352,1.);
#11872=VECTOR('',#52357,1.);
#11873=VECTOR('',#52358,1.);
#11874=VECTOR('',#52359,1.);
#11875=VECTOR('',#52370,1.);
#11876=VECTOR('',#52375,1.);
#11877=VECTOR('',#52376,1.);
#11878=VECTOR('',#52379,1.);
#11879=VECTOR('',#52392,0.999999999999998);
#11880=VECTOR('',#52397,1.);
#11881=VECTOR('',#52398,1.);
#11882=VECTOR('',#52401,1.);
#11883=VECTOR('',#52414,1.);
#11884=VECTOR('',#52419,0.01);
#11885=VECTOR('',#52420,1.);
#11886=VECTOR('',#52423,0.01);
#11887=VECTOR('',#52428,0.01);
#11888=VECTOR('',#52441,1.);
#11889=VECTOR('',#52444,1.);
#11890=VECTOR('',#52457,1.);
#11891=VECTOR('',#52462,1.);
#11892=VECTOR('',#52463,1.);
#11893=VECTOR('',#52470,1.);
#11894=VECTOR('',#52483,1.);
#11895=VECTOR('',#52488,1.);
#11896=VECTOR('',#52489,1.);
#11897=VECTOR('',#52492,1.);
#11898=VECTOR('',#52501,1.);
#11899=VECTOR('',#52506,1.);
#11900=VECTOR('',#52507,1.);
#11901=VECTOR('',#52508,1.);
#11902=VECTOR('',#52519,1.);
#11903=VECTOR('',#52524,1.);
#11904=VECTOR('',#52525,1.);
#11905=VECTOR('',#52528,1.);
#11906=VECTOR('',#52541,1.);
#11907=VECTOR('',#52546,1.);
#11908=VECTOR('',#52547,1.);
#11909=VECTOR('',#52550,1.);
#11910=VECTOR('',#52563,1.);
#11911=VECTOR('',#52568,0.01);
#11912=VECTOR('',#52569,1.);
#11913=VECTOR('',#52572,0.01);
#11914=VECTOR('',#52577,0.01);
#11915=VECTOR('',#52590,1.);
#11916=VECTOR('',#52593,1.);
#11917=VECTOR('',#52606,1.);
#11918=VECTOR('',#52611,1.);
#11919=VECTOR('',#52612,1.);
#11920=VECTOR('',#52619,1.);
#11921=VECTOR('',#52632,1.);
#11922=VECTOR('',#52637,1.);
#11923=VECTOR('',#52638,1.);
#11924=VECTOR('',#52641,1.);
#11925=VECTOR('',#52650,1.);
#11926=VECTOR('',#52655,1.);
#11927=VECTOR('',#52656,1.);
#11928=VECTOR('',#52657,1.);
#11929=VECTOR('',#52668,1.);
#11930=VECTOR('',#52673,1.);
#11931=VECTOR('',#52674,1.);
#11932=VECTOR('',#52677,1.);
#11933=VECTOR('',#52690,1.);
#11934=VECTOR('',#52695,1.);
#11935=VECTOR('',#52696,1.);
#11936=VECTOR('',#52699,1.);
#11937=VECTOR('',#52712,1.);
#11938=VECTOR('',#52717,0.01);
#11939=VECTOR('',#52718,1.);
#11940=VECTOR('',#52721,0.01);
#11941=VECTOR('',#52726,0.01);
#11942=VECTOR('',#52739,1.);
#11943=VECTOR('',#52742,1.);
#11944=VECTOR('',#52755,1.);
#11945=VECTOR('',#52760,1.);
#11946=VECTOR('',#52761,1.);
#11947=VECTOR('',#52768,1.);
#11948=VECTOR('',#52781,1.);
#11949=VECTOR('',#52786,1.);
#11950=VECTOR('',#52787,1.);
#11951=VECTOR('',#52790,1.);
#11952=VECTOR('',#52799,1.);
#11953=VECTOR('',#52804,1.);
#11954=VECTOR('',#52805,1.);
#11955=VECTOR('',#52806,1.);
#11956=VECTOR('',#52817,1.);
#11957=VECTOR('',#52822,0.999999999999999);
#11958=VECTOR('',#52823,1.);
#11959=VECTOR('',#52826,1.);
#11960=VECTOR('',#52839,1.);
#11961=VECTOR('',#52844,1.);
#11962=VECTOR('',#52845,1.);
#11963=VECTOR('',#52848,1.);
#11964=VECTOR('',#52861,1.);
#11965=VECTOR('',#52866,0.01);
#11966=VECTOR('',#52867,1.);
#11967=VECTOR('',#52870,0.01);
#11968=VECTOR('',#52875,0.01);
#11969=VECTOR('',#52888,1.);
#11970=VECTOR('',#52891,1.);
#11971=VECTOR('',#52904,1.);
#11972=VECTOR('',#52909,1.);
#11973=VECTOR('',#52910,1.);
#11974=VECTOR('',#52917,1.);
#11975=VECTOR('',#52930,1.);
#11976=VECTOR('',#52935,1.);
#11977=VECTOR('',#52936,1.);
#11978=VECTOR('',#52939,1.);
#11979=VECTOR('',#52948,1.);
#11980=VECTOR('',#52953,1.);
#11981=VECTOR('',#52954,1.);
#11982=VECTOR('',#52955,1.);
#11983=VECTOR('',#52966,1.);
#11984=VECTOR('',#52971,1.);
#11985=VECTOR('',#52972,1.);
#11986=VECTOR('',#52975,1.);
#11987=VECTOR('',#52988,1.);
#11988=VECTOR('',#52993,1.);
#11989=VECTOR('',#52994,1.);
#11990=VECTOR('',#52997,1.);
#11991=VECTOR('',#53010,0.999999999999999);
#11992=VECTOR('',#53015,0.01);
#11993=VECTOR('',#53016,1.);
#11994=VECTOR('',#53019,0.01);
#11995=VECTOR('',#53024,0.01);
#11996=VECTOR('',#53037,1.);
#11997=VECTOR('',#53040,1.);
#11998=VECTOR('',#53053,1.);
#11999=VECTOR('',#53058,1.);
#12000=VECTOR('',#53059,1.);
#12001=VECTOR('',#53066,1.);
#12002=VECTOR('',#53079,1.);
#12003=VECTOR('',#53084,0.999999999999999);
#12004=VECTOR('',#53085,1.);
#12005=VECTOR('',#53088,1.);
#12006=VECTOR('',#53097,1.);
#12007=VECTOR('',#53102,1.);
#12008=VECTOR('',#53103,1.);
#12009=VECTOR('',#53104,1.);
#12010=VECTOR('',#53115,1.);
#12011=VECTOR('',#53120,1.);
#12012=VECTOR('',#53121,1.);
#12013=VECTOR('',#53124,1.);
#12014=VECTOR('',#53137,1.);
#12015=VECTOR('',#53142,1.);
#12016=VECTOR('',#53143,1.);
#12017=VECTOR('',#53146,1.);
#12018=VECTOR('',#53159,1.);
#12019=VECTOR('',#53164,0.01);
#12020=VECTOR('',#53165,1.);
#12021=VECTOR('',#53168,0.01);
#12022=VECTOR('',#53173,0.01);
#12023=VECTOR('',#53186,1.);
#12024=VECTOR('',#53189,1.);
#12025=VECTOR('',#53202,1.);
#12026=VECTOR('',#53207,1.);
#12027=VECTOR('',#53208,1.);
#12028=VECTOR('',#53215,1.);
#12029=VECTOR('',#53228,1.);
#12030=VECTOR('',#53233,1.);
#12031=VECTOR('',#53234,1.);
#12032=VECTOR('',#53237,1.);
#12033=VECTOR('',#53246,1.);
#12034=VECTOR('',#53251,1.);
#12035=VECTOR('',#53252,1.);
#12036=VECTOR('',#53253,1.);
#12037=VECTOR('',#53264,1.);
#12038=VECTOR('',#53269,0.999999999999999);
#12039=VECTOR('',#53270,1.);
#12040=VECTOR('',#53273,1.);
#12041=VECTOR('',#53286,1.);
#12042=VECTOR('',#53291,1.);
#12043=VECTOR('',#53292,1.);
#12044=VECTOR('',#53295,1.);
#12045=VECTOR('',#53308,1.);
#12046=VECTOR('',#53313,0.01);
#12047=VECTOR('',#53314,1.);
#12048=VECTOR('',#53317,0.01);
#12049=VECTOR('',#53322,0.01);
#12050=VECTOR('',#53335,1.);
#12051=VECTOR('',#53338,1.);
#12052=VECTOR('',#53351,1.);
#12053=VECTOR('',#53356,1.);
#12054=VECTOR('',#53357,1.);
#12055=VECTOR('',#53364,1.);
#12056=VECTOR('',#53377,1.);
#12057=VECTOR('',#53382,1.);
#12058=VECTOR('',#53383,1.);
#12059=VECTOR('',#53386,1.);
#12060=VECTOR('',#53395,1.);
#12061=VECTOR('',#53400,1.);
#12062=VECTOR('',#53401,1.);
#12063=VECTOR('',#53402,1.);
#12064=VECTOR('',#53413,1.);
#12065=VECTOR('',#53418,1.);
#12066=VECTOR('',#53419,1.);
#12067=VECTOR('',#53422,1.);
#12068=VECTOR('',#53435,1.);
#12069=VECTOR('',#53440,1.);
#12070=VECTOR('',#53441,1.);
#12071=VECTOR('',#53444,1.);
#12072=VECTOR('',#53457,1.);
#12073=VECTOR('',#53462,0.01);
#12074=VECTOR('',#53463,1.);
#12075=VECTOR('',#53466,0.01);
#12076=VECTOR('',#53471,0.01);
#12077=VECTOR('',#53484,1.);
#12078=VECTOR('',#53487,1.);
#12079=VECTOR('',#53500,1.);
#12080=VECTOR('',#53505,1.);
#12081=VECTOR('',#53506,1.);
#12082=VECTOR('',#53513,1.);
#12083=VECTOR('',#53526,1.);
#12084=VECTOR('',#53531,1.);
#12085=VECTOR('',#53532,1.);
#12086=VECTOR('',#53535,1.);
#12087=VECTOR('',#53544,1.);
#12088=VECTOR('',#53549,1.);
#12089=VECTOR('',#53550,1.);
#12090=VECTOR('',#53551,0.999999999999999);
#12091=VECTOR('',#53562,1.);
#12092=VECTOR('',#53567,1.);
#12093=VECTOR('',#53568,1.);
#12094=VECTOR('',#53571,1.);
#12095=VECTOR('',#53584,1.);
#12096=VECTOR('',#53589,1.);
#12097=VECTOR('',#53590,1.);
#12098=VECTOR('',#53593,1.);
#12099=VECTOR('',#53606,1.);
#12100=VECTOR('',#53611,0.01);
#12101=VECTOR('',#53612,1.);
#12102=VECTOR('',#53615,0.01);
#12103=VECTOR('',#53620,0.01);
#12104=VECTOR('',#53633,1.);
#12105=VECTOR('',#53636,1.);
#12106=VECTOR('',#53649,1.);
#12107=VECTOR('',#53654,1.);
#12108=VECTOR('',#53655,1.);
#12109=VECTOR('',#53662,1.);
#12110=VECTOR('',#53675,1.);
#12111=VECTOR('',#53680,1.);
#12112=VECTOR('',#53681,1.);
#12113=VECTOR('',#53684,1.);
#12114=VECTOR('',#53693,1.);
#12115=VECTOR('',#53698,1.);
#12116=VECTOR('',#53699,1.);
#12117=VECTOR('',#53700,1.);
#12118=VECTOR('',#53711,1.);
#12119=VECTOR('',#53716,1.);
#12120=VECTOR('',#53717,1.);
#12121=VECTOR('',#53720,1.);
#12122=VECTOR('',#53733,1.);
#12123=VECTOR('',#53738,1.);
#12124=VECTOR('',#53739,1.);
#12125=VECTOR('',#53742,1.);
#12126=VECTOR('',#53755,1.);
#12127=VECTOR('',#53760,0.01);
#12128=VECTOR('',#53761,1.);
#12129=VECTOR('',#53764,0.01);
#12130=VECTOR('',#53769,0.01);
#12131=VECTOR('',#53782,1.);
#12132=VECTOR('',#53785,1.);
#12133=VECTOR('',#53798,1.);
#12134=VECTOR('',#53803,1.);
#12135=VECTOR('',#53804,1.);
#12136=VECTOR('',#53811,1.);
#12137=VECTOR('',#53824,1.);
#12138=VECTOR('',#53829,1.);
#12139=VECTOR('',#53830,1.);
#12140=VECTOR('',#53833,1.);
#12141=VECTOR('',#53842,1.);
#12142=VECTOR('',#53847,1.);
#12143=VECTOR('',#53848,1.);
#12144=VECTOR('',#53849,1.);
#12145=VECTOR('',#53860,1.);
#12146=VECTOR('',#53865,1.);
#12147=VECTOR('',#53866,1.);
#12148=VECTOR('',#53869,1.);
#12149=VECTOR('',#53882,1.);
#12150=VECTOR('',#53887,1.);
#12151=VECTOR('',#53888,1.);
#12152=VECTOR('',#53891,1.);
#12153=VECTOR('',#53904,1.);
#12154=VECTOR('',#53909,0.01);
#12155=VECTOR('',#53910,1.);
#12156=VECTOR('',#53913,0.01);
#12157=VECTOR('',#53918,0.01);
#12158=VECTOR('',#53931,1.);
#12159=VECTOR('',#53934,1.);
#12160=VECTOR('',#53947,1.);
#12161=VECTOR('',#53952,1.);
#12162=VECTOR('',#53953,1.);
#12163=VECTOR('',#53960,1.);
#12164=VECTOR('',#53973,1.);
#12165=VECTOR('',#53978,1.);
#12166=VECTOR('',#53979,0.999999999999999);
#12167=VECTOR('',#53982,1.);
#12168=VECTOR('',#53991,1.);
#12169=VECTOR('',#53996,1.);
#12170=VECTOR('',#53997,1.);
#12171=VECTOR('',#53998,1.);
#12172=VECTOR('',#54009,1.);
#12173=VECTOR('',#54014,1.);
#12174=VECTOR('',#54015,1.);
#12175=VECTOR('',#54018,1.);
#12176=VECTOR('',#54031,1.);
#12177=VECTOR('',#54036,1.);
#12178=VECTOR('',#54037,1.);
#12179=VECTOR('',#54040,1.);
#12180=VECTOR('',#54053,0.999999999999999);
#12181=VECTOR('',#54058,0.01);
#12182=VECTOR('',#54059,1.);
#12183=VECTOR('',#54062,0.01);
#12184=VECTOR('',#54067,0.01);
#12185=VECTOR('',#54080,1.);
#12186=VECTOR('',#54083,1.);
#12187=VECTOR('',#54096,1.);
#12188=VECTOR('',#54101,1.);
#12189=VECTOR('',#54102,0.999999999999999);
#12190=VECTOR('',#54109,1.);
#12191=VECTOR('',#54122,1.);
#12192=VECTOR('',#54127,1.);
#12193=VECTOR('',#54128,1.);
#12194=VECTOR('',#54131,1.);
#12195=VECTOR('',#54140,1.);
#12196=VECTOR('',#54145,1.);
#12197=VECTOR('',#54146,1.);
#12198=VECTOR('',#54147,1.);
#12199=VECTOR('',#54158,1.);
#12200=VECTOR('',#54163,1.);
#12201=VECTOR('',#54164,1.);
#12202=VECTOR('',#54167,1.);
#12203=VECTOR('',#54180,0.999999999999999);
#12204=VECTOR('',#54185,0.999999999999998);
#12205=VECTOR('',#54186,1.);
#12206=VECTOR('',#54189,1.);
#12207=VECTOR('',#54202,1.);
#12208=VECTOR('',#54207,0.01);
#12209=VECTOR('',#54208,1.);
#12210=VECTOR('',#54211,0.01);
#12211=VECTOR('',#54216,0.01);
#12212=VECTOR('',#54229,1.);
#12213=VECTOR('',#54232,1.);
#12214=VECTOR('',#54245,1.);
#12215=VECTOR('',#54250,1.);
#12216=VECTOR('',#54251,1.);
#12217=VECTOR('',#54258,1.);
#12218=VECTOR('',#54271,1.);
#12219=VECTOR('',#54276,0.999999999999998);
#12220=VECTOR('',#54277,1.);
#12221=VECTOR('',#54280,1.);
#12222=VECTOR('',#54289,1.);
#12223=VECTOR('',#54294,1.);
#12224=VECTOR('',#54295,1.);
#12225=VECTOR('',#54296,1.);
#12226=VECTOR('',#54307,1.);
#12227=VECTOR('',#54312,1.);
#12228=VECTOR('',#54313,1.);
#12229=VECTOR('',#54316,1.);
#12230=VECTOR('',#54329,1.);
#12231=VECTOR('',#54334,1.);
#12232=VECTOR('',#54335,1.);
#12233=VECTOR('',#54338,1.);
#12234=VECTOR('',#54351,1.);
#12235=VECTOR('',#54356,0.00999999999999998);
#12236=VECTOR('',#54357,1.);
#12237=VECTOR('',#54360,0.01);
#12238=VECTOR('',#54365,0.01);
#12239=VECTOR('',#54378,1.);
#12240=VECTOR('',#54381,1.);
#12241=VECTOR('',#54394,1.);
#12242=VECTOR('',#54399,1.);
#12243=VECTOR('',#54400,1.);
#12244=VECTOR('',#54407,0.999999999999999);
#12245=VECTOR('',#54420,1.);
#12246=VECTOR('',#54425,1.);
#12247=VECTOR('',#54426,1.);
#12248=VECTOR('',#54429,1.);
#12249=VECTOR('',#54438,1.);
#12250=VECTOR('',#54443,1.);
#12251=VECTOR('',#54444,1.);
#12252=VECTOR('',#54445,1.);
#12253=VECTOR('',#54456,1.);
#12254=VECTOR('',#54461,1.);
#12255=VECTOR('',#54462,1.);
#12256=VECTOR('',#54465,1.);
#12257=VECTOR('',#54478,1.);
#12258=VECTOR('',#54483,1.);
#12259=VECTOR('',#54484,1.);
#12260=VECTOR('',#54487,1.);
#12261=VECTOR('',#54500,1.);
#12262=VECTOR('',#54505,0.01);
#12263=VECTOR('',#54506,1.);
#12264=VECTOR('',#54509,0.01);
#12265=VECTOR('',#54514,0.01);
#12266=VECTOR('',#54527,1.);
#12267=VECTOR('',#54530,1.);
#12268=VECTOR('',#54543,1.);
#12269=VECTOR('',#54548,1.);
#12270=VECTOR('',#54549,1.);
#12271=VECTOR('',#54556,1.);
#12272=VECTOR('',#54569,1.);
#12273=VECTOR('',#54574,1.);
#12274=VECTOR('',#54575,1.);
#12275=VECTOR('',#54578,1.);
#12276=VECTOR('',#54587,1.);
#12277=VECTOR('',#54592,1.);
#12278=VECTOR('',#54593,1.);
#12279=VECTOR('',#54594,1.);
#12280=VECTOR('',#54605,1.);
#12281=VECTOR('',#54610,1.);
#12282=VECTOR('',#54611,1.);
#12283=VECTOR('',#54614,1.);
#12284=VECTOR('',#54627,1.);
#12285=VECTOR('',#54632,0.999999999999999);
#12286=VECTOR('',#54633,1.);
#12287=VECTOR('',#54636,1.);
#12288=VECTOR('',#54649,1.);
#12289=VECTOR('',#54654,0.01);
#12290=VECTOR('',#54655,1.);
#12291=VECTOR('',#54658,0.01);
#12292=VECTOR('',#54663,0.01);
#12293=VECTOR('',#54676,1.);
#12294=VECTOR('',#54679,1.);
#12295=VECTOR('',#54692,1.);
#12296=VECTOR('',#54697,1.);
#12297=VECTOR('',#54698,1.);
#12298=VECTOR('',#54705,1.);
#12299=VECTOR('',#54718,1.);
#12300=VECTOR('',#54723,1.);
#12301=VECTOR('',#54724,1.);
#12302=VECTOR('',#54727,1.);
#12303=VECTOR('',#54736,1.);
#12304=VECTOR('',#54741,1.);
#12305=VECTOR('',#54742,1.);
#12306=VECTOR('',#54743,1.);
#12307=VECTOR('',#54754,1.);
#12308=VECTOR('',#54759,1.);
#12309=VECTOR('',#54760,0.999999999999999);
#12310=VECTOR('',#54763,1.);
#12311=VECTOR('',#54776,1.);
#12312=VECTOR('',#54781,1.);
#12313=VECTOR('',#54782,1.);
#12314=VECTOR('',#54785,1.);
#12315=VECTOR('',#54798,1.);
#12316=VECTOR('',#54803,0.01);
#12317=VECTOR('',#54804,1.);
#12318=VECTOR('',#54807,0.01);
#12319=VECTOR('',#54812,0.01);
#12320=VECTOR('',#54825,1.);
#12321=VECTOR('',#54828,1.);
#12322=VECTOR('',#54841,1.);
#12323=VECTOR('',#54846,1.);
#12324=VECTOR('',#54847,1.);
#12325=VECTOR('',#54854,1.);
#12326=VECTOR('',#54867,1.);
#12327=VECTOR('',#54872,1.);
#12328=VECTOR('',#54873,1.);
#12329=VECTOR('',#54876,1.);
#12330=VECTOR('',#54885,1.);
#12331=VECTOR('',#54890,1.);
#12332=VECTOR('',#54891,1.);
#12333=VECTOR('',#54892,1.);
#12334=VECTOR('',#54903,1.);
#12335=VECTOR('',#54908,1.);
#12336=VECTOR('',#54909,1.);
#12337=VECTOR('',#54912,1.);
#12338=VECTOR('',#54925,1.);
#12339=VECTOR('',#54930,1.);
#12340=VECTOR('',#54931,1.);
#12341=VECTOR('',#54934,1.);
#12342=VECTOR('',#54947,1.);
#12343=VECTOR('',#54952,0.01);
#12344=VECTOR('',#54953,1.);
#12345=VECTOR('',#54956,0.01);
#12346=VECTOR('',#54961,0.01);
#12347=VECTOR('',#54974,1.);
#12348=VECTOR('',#54977,1.);
#12349=VECTOR('',#54990,1.);
#12350=VECTOR('',#54995,1.);
#12351=VECTOR('',#54996,1.);
#12352=VECTOR('',#55003,1.);
#12353=VECTOR('',#55016,1.);
#12354=VECTOR('',#55021,1.);
#12355=VECTOR('',#55022,1.);
#12356=VECTOR('',#55025,1.);
#12357=VECTOR('',#55034,1.);
#12358=VECTOR('',#55039,1.);
#12359=VECTOR('',#55040,1.);
#12360=VECTOR('',#55041,1.);
#12361=VECTOR('',#55052,1.);
#12362=VECTOR('',#55057,1.);
#12363=VECTOR('',#55058,1.);
#12364=VECTOR('',#55061,1.);
#12365=VECTOR('',#55074,1.);
#12366=VECTOR('',#55079,1.);
#12367=VECTOR('',#55080,1.);
#12368=VECTOR('',#55083,1.);
#12369=VECTOR('',#55096,1.);
#12370=VECTOR('',#55101,0.01);
#12371=VECTOR('',#55102,1.);
#12372=VECTOR('',#55105,0.01);
#12373=VECTOR('',#55110,0.01);
#12374=VECTOR('',#55123,1.);
#12375=VECTOR('',#55126,1.);
#12376=VECTOR('',#55139,1.);
#12377=VECTOR('',#55144,1.);
#12378=VECTOR('',#55145,1.);
#12379=VECTOR('',#55152,1.);
#12380=VECTOR('',#55165,1.);
#12381=VECTOR('',#55170,1.);
#12382=VECTOR('',#55171,1.);
#12383=VECTOR('',#55174,1.);
#12384=VECTOR('',#55183,1.);
#12385=VECTOR('',#55188,1.);
#12386=VECTOR('',#55189,1.);
#12387=VECTOR('',#55190,1.);
#12388=VECTOR('',#55201,1.);
#12389=VECTOR('',#55206,1.);
#12390=VECTOR('',#55207,1.);
#12391=VECTOR('',#55210,1.);
#12392=VECTOR('',#55223,1.);
#12393=VECTOR('',#55228,1.);
#12394=VECTOR('',#55229,1.);
#12395=VECTOR('',#55232,1.);
#12396=VECTOR('',#55245,1.);
#12397=VECTOR('',#55250,0.01);
#12398=VECTOR('',#55251,1.);
#12399=VECTOR('',#55254,0.01);
#12400=VECTOR('',#55259,0.01);
#12401=VECTOR('',#55272,1.);
#12402=VECTOR('',#55275,1.);
#12403=VECTOR('',#55288,1.);
#12404=VECTOR('',#55293,1.);
#12405=VECTOR('',#55294,1.);
#12406=VECTOR('',#55301,1.);
#12407=VECTOR('',#55314,1.);
#12408=VECTOR('',#55319,1.);
#12409=VECTOR('',#55320,1.);
#12410=VECTOR('',#55323,1.);
#12411=VECTOR('',#55332,1.);
#12412=VECTOR('',#55337,1.);
#12413=VECTOR('',#55338,1.);
#12414=VECTOR('',#55339,1.);
#12415=VECTOR('',#55350,1.);
#12416=VECTOR('',#55355,1.);
#12417=VECTOR('',#55356,1.);
#12418=VECTOR('',#55359,1.);
#12419=VECTOR('',#55372,1.);
#12420=VECTOR('',#55377,1.);
#12421=VECTOR('',#55378,1.);
#12422=VECTOR('',#55381,1.);
#12423=VECTOR('',#55394,1.);
#12424=VECTOR('',#55399,0.01);
#12425=VECTOR('',#55400,1.);
#12426=VECTOR('',#55403,0.01);
#12427=VECTOR('',#55408,0.01);
#12428=VECTOR('',#55421,1.);
#12429=VECTOR('',#55424,1.);
#12430=VECTOR('',#55437,1.);
#12431=VECTOR('',#55442,1.);
#12432=VECTOR('',#55443,1.);
#12433=VECTOR('',#55450,1.);
#12434=VECTOR('',#55463,1.);
#12435=VECTOR('',#55468,1.);
#12436=VECTOR('',#55469,1.);
#12437=VECTOR('',#55472,1.);
#12438=VECTOR('',#55481,1.);
#12439=VECTOR('',#55486,0.999999999999999);
#12440=VECTOR('',#55487,1.);
#12441=VECTOR('',#55488,1.);
#12442=VECTOR('',#55499,1.);
#12443=VECTOR('',#55504,1.);
#12444=VECTOR('',#55505,1.);
#12445=VECTOR('',#55508,1.);
#12446=VECTOR('',#55521,1.);
#12447=VECTOR('',#55526,1.);
#12448=VECTOR('',#55527,1.);
#12449=VECTOR('',#55530,1.);
#12450=VECTOR('',#55543,0.999999999999998);
#12451=VECTOR('',#55548,0.01);
#12452=VECTOR('',#55549,1.);
#12453=VECTOR('',#55552,0.01);
#12454=VECTOR('',#55557,0.01);
#12455=VECTOR('',#55570,1.);
#12456=VECTOR('',#55573,1.);
#12457=VECTOR('',#55586,1.);
#12458=VECTOR('',#55591,1.);
#12459=VECTOR('',#55592,1.);
#12460=VECTOR('',#55599,1.);
#12461=VECTOR('',#55612,1.);
#12462=VECTOR('',#55617,1.);
#12463=VECTOR('',#55618,1.);
#12464=VECTOR('',#55621,1.);
#12465=VECTOR('',#55630,1.);
#12466=VECTOR('',#55635,1.);
#12467=VECTOR('',#55636,1.);
#12468=VECTOR('',#55637,1.);
#12469=VECTOR('',#55648,1.);
#12470=VECTOR('',#55653,1.);
#12471=VECTOR('',#55654,1.);
#12472=VECTOR('',#55657,1.);
#12473=VECTOR('',#55670,1.);
#12474=VECTOR('',#55675,0.999999999999999);
#12475=VECTOR('',#55676,1.);
#12476=VECTOR('',#55679,1.);
#12477=VECTOR('',#55692,1.);
#12478=VECTOR('',#55697,0.01);
#12479=VECTOR('',#55698,1.);
#12480=VECTOR('',#55701,0.01);
#12481=VECTOR('',#55706,0.01);
#12482=VECTOR('',#55719,1.);
#12483=VECTOR('',#55722,1.);
#12484=VECTOR('',#55735,0.999999999999998);
#12485=VECTOR('',#55740,1.);
#12486=VECTOR('',#55741,1.);
#12487=VECTOR('',#55748,1.);
#12488=VECTOR('',#55761,1.);
#12489=VECTOR('',#55766,1.);
#12490=VECTOR('',#55767,1.);
#12491=VECTOR('',#55770,1.);
#12492=VECTOR('',#55779,1.);
#12493=VECTOR('',#55784,1.);
#12494=VECTOR('',#55785,1.);
#12495=VECTOR('',#55786,1.);
#12496=VECTOR('',#55797,1.);
#12497=VECTOR('',#55802,1.);
#12498=VECTOR('',#55803,1.);
#12499=VECTOR('',#55806,1.);
#12500=VECTOR('',#55819,1.);
#12501=VECTOR('',#55824,1.);
#12502=VECTOR('',#55825,1.);
#12503=VECTOR('',#55828,1.);
#12504=VECTOR('',#55841,1.);
#12505=VECTOR('',#55846,0.01);
#12506=VECTOR('',#55847,1.);
#12507=VECTOR('',#55850,0.01);
#12508=VECTOR('',#55855,0.01);
#12509=VECTOR('',#55868,1.);
#12510=VECTOR('',#55871,1.);
#12511=VECTOR('',#55884,1.);
#12512=VECTOR('',#55889,1.);
#12513=VECTOR('',#55890,1.);
#12514=VECTOR('',#55897,1.);
#12515=VECTOR('',#55910,1.);
#12516=VECTOR('',#55915,1.);
#12517=VECTOR('',#55916,1.);
#12518=VECTOR('',#55919,1.);
#12519=VECTOR('',#55928,1.);
#12520=VECTOR('',#55933,1.);
#12521=VECTOR('',#55934,1.);
#12522=VECTOR('',#55935,1.);
#12523=VECTOR('',#55946,1.);
#12524=VECTOR('',#55951,1.);
#12525=VECTOR('',#55952,1.);
#12526=VECTOR('',#55955,1.);
#12527=VECTOR('',#55968,1.);
#12528=VECTOR('',#55973,1.);
#12529=VECTOR('',#55974,1.);
#12530=VECTOR('',#55977,1.);
#12531=VECTOR('',#55990,1.);
#12532=VECTOR('',#55995,0.01);
#12533=VECTOR('',#55996,1.);
#12534=VECTOR('',#55999,0.01);
#12535=VECTOR('',#56004,0.01);
#12536=VECTOR('',#56017,1.);
#12537=VECTOR('',#56020,1.);
#12538=VECTOR('',#56033,1.);
#12539=VECTOR('',#56038,1.);
#12540=VECTOR('',#56039,1.);
#12541=VECTOR('',#56046,1.);
#12542=VECTOR('',#56059,1.);
#12543=VECTOR('',#56064,1.);
#12544=VECTOR('',#56065,1.);
#12545=VECTOR('',#56068,1.);
#12546=VECTOR('',#56077,1.);
#12547=VECTOR('',#56082,1.);
#12548=VECTOR('',#56083,1.);
#12549=VECTOR('',#56084,1.);
#12550=VECTOR('',#56095,1.);
#12551=VECTOR('',#56100,1.);
#12552=VECTOR('',#56101,1.);
#12553=VECTOR('',#56104,1.);
#12554=VECTOR('',#56117,0.999999999999998);
#12555=VECTOR('',#56122,1.);
#12556=VECTOR('',#56123,1.);
#12557=VECTOR('',#56126,1.);
#12558=VECTOR('',#56139,1.);
#12559=VECTOR('',#56144,0.01);
#12560=VECTOR('',#56145,1.);
#12561=VECTOR('',#56148,0.01);
#12562=VECTOR('',#56153,0.01);
#12563=VECTOR('',#56166,1.);
#12564=VECTOR('',#56169,1.);
#12565=VECTOR('',#56182,1.);
#12566=VECTOR('',#56187,1.);
#12567=VECTOR('',#56188,1.);
#12568=VECTOR('',#56195,1.);
#12569=VECTOR('',#56208,1.);
#12570=VECTOR('',#56213,1.);
#12571=VECTOR('',#56214,1.);
#12572=VECTOR('',#56217,1.);
#12573=VECTOR('',#56226,1.);
#12574=VECTOR('',#56231,1.);
#12575=VECTOR('',#56232,0.999999999999999);
#12576=VECTOR('',#56233,1.);
#12577=VECTOR('',#56244,1.);
#12578=VECTOR('',#56249,1.);
#12579=VECTOR('',#56250,1.);
#12580=VECTOR('',#56253,1.);
#12581=VECTOR('',#56266,1.);
#12582=VECTOR('',#56271,1.);
#12583=VECTOR('',#56272,1.);
#12584=VECTOR('',#56275,1.);
#12585=VECTOR('',#56288,1.);
#12586=VECTOR('',#56293,0.01);
#12587=VECTOR('',#56294,1.);
#12588=VECTOR('',#56297,0.01);
#12589=VECTOR('',#56302,0.01);
#12590=VECTOR('',#56315,1.);
#12591=VECTOR('',#56318,1.);
#12592=VECTOR('',#56331,1.);
#12593=VECTOR('',#56336,0.999999999999999);
#12594=VECTOR('',#56337,1.);
#12595=VECTOR('',#56344,1.);
#12596=VECTOR('',#56357,1.);
#12597=VECTOR('',#56362,1.);
#12598=VECTOR('',#56363,1.);
#12599=VECTOR('',#56366,1.);
#12600=VECTOR('',#56375,1.);
#12601=VECTOR('',#56380,1.);
#12602=VECTOR('',#56381,1.);
#12603=VECTOR('',#56382,1.);
#12604=VECTOR('',#56393,1.);
#12605=VECTOR('',#56398,1.);
#12606=VECTOR('',#56399,1.);
#12607=VECTOR('',#56402,1.);
#12608=VECTOR('',#56415,1.);
#12609=VECTOR('',#56420,0.999999999999998);
#12610=VECTOR('',#56421,1.);
#12611=VECTOR('',#56424,1.);
#12612=VECTOR('',#56437,1.);
#12613=VECTOR('',#56442,0.01);
#12614=VECTOR('',#56443,1.);
#12615=VECTOR('',#56446,0.01);
#12616=VECTOR('',#56451,0.01);
#12617=VECTOR('',#56464,1.);
#12618=VECTOR('',#56467,1.);
#12619=VECTOR('',#56480,1.);
#12620=VECTOR('',#56485,1.);
#12621=VECTOR('',#56486,1.);
#12622=VECTOR('',#56493,1.);
#12623=VECTOR('',#56506,1.);
#12624=VECTOR('',#56511,1.);
#12625=VECTOR('',#56512,1.);
#12626=VECTOR('',#56515,1.);
#12627=VECTOR('',#56524,1.);
#12628=VECTOR('',#56529,1.);
#12629=VECTOR('',#56530,1.);
#12630=VECTOR('',#56531,1.);
#12631=VECTOR('',#56542,1.);
#12632=VECTOR('',#56547,1.);
#12633=VECTOR('',#56548,1.);
#12634=VECTOR('',#56551,1.);
#12635=VECTOR('',#56564,1.);
#12636=VECTOR('',#56569,1.);
#12637=VECTOR('',#56570,1.);
#12638=VECTOR('',#56573,1.);
#12639=VECTOR('',#56586,1.);
#12640=VECTOR('',#56591,0.01);
#12641=VECTOR('',#56592,1.);
#12642=VECTOR('',#56595,0.01);
#12643=VECTOR('',#56600,0.01);
#12644=VECTOR('',#56613,1.);
#12645=VECTOR('',#56616,1.);
#12646=VECTOR('',#56629,1.);
#12647=VECTOR('',#56634,1.);
#12648=VECTOR('',#56635,1.);
#12649=VECTOR('',#56642,1.);
#12650=VECTOR('',#56655,1.);
#12651=VECTOR('',#56660,1.);
#12652=VECTOR('',#56661,1.);
#12653=VECTOR('',#56664,1.);
#12654=VECTOR('',#56673,1.);
#12655=VECTOR('',#56678,1.);
#12656=VECTOR('',#56679,1.);
#12657=VECTOR('',#56680,1.);
#12658=VECTOR('',#56691,1.);
#12659=VECTOR('',#56696,1.);
#12660=VECTOR('',#56697,1.);
#12661=VECTOR('',#56700,1.);
#12662=VECTOR('',#56713,1.);
#12663=VECTOR('',#56718,1.);
#12664=VECTOR('',#56719,1.);
#12665=VECTOR('',#56722,1.);
#12666=VECTOR('',#56735,1.);
#12667=VECTOR('',#56740,0.01);
#12668=VECTOR('',#56741,1.);
#12669=VECTOR('',#56744,0.01);
#12670=VECTOR('',#56749,0.01);
#12671=VECTOR('',#56762,1.);
#12672=VECTOR('',#56765,1.);
#12673=VECTOR('',#56778,1.);
#12674=VECTOR('',#56783,1.);
#12675=VECTOR('',#56784,1.);
#12676=VECTOR('',#56791,1.);
#12677=VECTOR('',#56804,1.);
#12678=VECTOR('',#56809,1.);
#12679=VECTOR('',#56810,1.);
#12680=VECTOR('',#56813,1.);
#12681=VECTOR('',#56822,1.);
#12682=VECTOR('',#56827,1.);
#12683=VECTOR('',#56828,1.);
#12684=VECTOR('',#56829,1.);
#12685=VECTOR('',#56840,1.);
#12686=VECTOR('',#56845,1.);
#12687=VECTOR('',#56846,1.);
#12688=VECTOR('',#56849,1.);
#12689=VECTOR('',#56862,1.);
#12690=VECTOR('',#56867,1.);
#12691=VECTOR('',#56868,1.);
#12692=VECTOR('',#56871,1.);
#12693=VECTOR('',#56884,1.);
#12694=VECTOR('',#56889,0.01);
#12695=VECTOR('',#56890,1.);
#12696=VECTOR('',#56893,0.01);
#12697=VECTOR('',#56898,0.01);
#12698=VECTOR('',#56911,1.);
#12699=VECTOR('',#56914,1.);
#12700=VECTOR('',#56927,1.);
#12701=VECTOR('',#56932,1.);
#12702=VECTOR('',#56933,1.);
#12703=VECTOR('',#56940,1.);
#12704=VECTOR('',#56953,1.);
#12705=VECTOR('',#56958,1.);
#12706=VECTOR('',#56959,1.);
#12707=VECTOR('',#56962,1.);
#12708=VECTOR('',#56971,1.);
#12709=VECTOR('',#56976,1.);
#12710=VECTOR('',#56977,1.);
#12711=VECTOR('',#56978,1.);
#12712=VECTOR('',#56989,1.);
#12713=VECTOR('',#56994,1.);
#12714=VECTOR('',#56995,1.);
#12715=VECTOR('',#56998,1.);
#12716=VECTOR('',#57011,1.);
#12717=VECTOR('',#57016,1.);
#12718=VECTOR('',#57017,1.);
#12719=VECTOR('',#57020,1.);
#12720=VECTOR('',#57033,1.);
#12721=VECTOR('',#57038,0.01);
#12722=VECTOR('',#57039,1.);
#12723=VECTOR('',#57042,0.01);
#12724=VECTOR('',#57047,0.01);
#12725=VECTOR('',#57060,1.);
#12726=VECTOR('',#57063,1.);
#12727=VECTOR('',#57076,1.);
#12728=VECTOR('',#57081,1.);
#12729=VECTOR('',#57082,1.);
#12730=VECTOR('',#57089,1.);
#12731=VECTOR('',#57102,1.);
#12732=VECTOR('',#57107,0.999999999999999);
#12733=VECTOR('',#57108,1.);
#12734=VECTOR('',#57111,1.);
#12735=VECTOR('',#57120,1.);
#12736=VECTOR('',#57125,1.);
#12737=VECTOR('',#57126,1.);
#12738=VECTOR('',#57127,1.);
#12739=VECTOR('',#57138,1.);
#12740=VECTOR('',#57143,1.);
#12741=VECTOR('',#57144,1.);
#12742=VECTOR('',#57147,1.);
#12743=VECTOR('',#57160,1.);
#12744=VECTOR('',#57165,1.);
#12745=VECTOR('',#57166,1.);
#12746=VECTOR('',#57169,1.);
#12747=VECTOR('',#57182,1.);
#12748=VECTOR('',#57187,0.01);
#12749=VECTOR('',#57188,1.);
#12750=VECTOR('',#57191,0.01);
#12751=VECTOR('',#57196,0.01);
#12752=VECTOR('',#57209,1.);
#12753=VECTOR('',#57212,1.);
#12754=VECTOR('',#57225,1.);
#12755=VECTOR('',#57230,1.);
#12756=VECTOR('',#57231,1.);
#12757=VECTOR('',#57238,1.);
#12758=VECTOR('',#57251,1.);
#12759=VECTOR('',#57256,1.);
#12760=VECTOR('',#57257,1.);
#12761=VECTOR('',#57260,1.);
#12762=VECTOR('',#57269,1.);
#12763=VECTOR('',#57274,1.);
#12764=VECTOR('',#57275,1.);
#12765=VECTOR('',#57276,1.);
#12766=VECTOR('',#57287,1.);
#12767=VECTOR('',#57292,1.);
#12768=VECTOR('',#57293,1.);
#12769=VECTOR('',#57296,1.);
#12770=VECTOR('',#57309,1.);
#12771=VECTOR('',#57314,1.);
#12772=VECTOR('',#57315,1.);
#12773=VECTOR('',#57318,1.);
#12774=VECTOR('',#57331,1.);
#12775=VECTOR('',#57336,0.01);
#12776=VECTOR('',#57337,1.);
#12777=VECTOR('',#57340,0.01);
#12778=VECTOR('',#57345,0.01);
#12779=VECTOR('',#57358,1.);
#12780=VECTOR('',#57361,1.);
#12781=VECTOR('',#57374,0.999999999999998);
#12782=VECTOR('',#57379,1.);
#12783=VECTOR('',#57380,1.);
#12784=VECTOR('',#57387,1.);
#12785=VECTOR('',#57400,1.);
#12786=VECTOR('',#57405,1.);
#12787=VECTOR('',#57406,1.);
#12788=VECTOR('',#57409,1.);
#12789=VECTOR('',#57418,1.);
#12790=VECTOR('',#57423,1.);
#12791=VECTOR('',#57424,1.);
#12792=VECTOR('',#57425,1.);
#12793=VECTOR('',#57436,1.);
#12794=VECTOR('',#57441,1.);
#12795=VECTOR('',#57442,0.999999999999999);
#12796=VECTOR('',#57445,1.);
#12797=VECTOR('',#57458,1.);
#12798=VECTOR('',#57463,1.);
#12799=VECTOR('',#57464,1.);
#12800=VECTOR('',#57467,1.);
#12801=VECTOR('',#57480,1.);
#12802=VECTOR('',#57485,0.01);
#12803=VECTOR('',#57486,1.);
#12804=VECTOR('',#57489,0.01);
#12805=VECTOR('',#57494,0.01);
#12806=VECTOR('',#57507,1.);
#12807=VECTOR('',#57510,1.);
#12808=VECTOR('',#57523,1.);
#12809=VECTOR('',#57528,1.);
#12810=VECTOR('',#57529,1.);
#12811=VECTOR('',#57536,1.);
#12812=VECTOR('',#57549,1.);
#12813=VECTOR('',#57554,1.);
#12814=VECTOR('',#57555,1.);
#12815=VECTOR('',#57558,1.);
#12816=VECTOR('',#57567,1.);
#12817=VECTOR('',#57572,1.);
#12818=VECTOR('',#57573,1.);
#12819=VECTOR('',#57574,1.);
#12820=VECTOR('',#57585,1.);
#12821=VECTOR('',#57590,1.);
#12822=VECTOR('',#57591,1.);
#12823=VECTOR('',#57594,1.);
#12824=VECTOR('',#57607,1.);
#12825=VECTOR('',#57612,1.);
#12826=VECTOR('',#57613,1.);
#12827=VECTOR('',#57616,1.);
#12828=VECTOR('',#57629,1.);
#12829=VECTOR('',#57634,0.01);
#12830=VECTOR('',#57635,1.);
#12831=VECTOR('',#57638,0.01);
#12832=VECTOR('',#57643,0.01);
#12833=VECTOR('',#57656,1.);
#12834=VECTOR('',#57659,1.);
#12835=VECTOR('',#57672,1.);
#12836=VECTOR('',#57677,1.);
#12837=VECTOR('',#57678,1.);
#12838=VECTOR('',#57685,1.);
#12839=VECTOR('',#57698,1.);
#12840=VECTOR('',#57703,1.);
#12841=VECTOR('',#57704,1.);
#12842=VECTOR('',#57707,1.);
#12843=VECTOR('',#57716,0.999999999999999);
#12844=VECTOR('',#57721,1.);
#12845=VECTOR('',#57722,1.);
#12846=VECTOR('',#57723,1.);
#12847=VECTOR('',#57734,1.);
#12848=VECTOR('',#57739,1.);
#12849=VECTOR('',#57740,1.);
#12850=VECTOR('',#57743,1.);
#12851=VECTOR('',#57756,1.);
#12852=VECTOR('',#57761,1.);
#12853=VECTOR('',#57762,1.);
#12854=VECTOR('',#57765,1.);
#12855=VECTOR('',#57778,1.);
#12856=VECTOR('',#57783,0.01);
#12857=VECTOR('',#57784,1.);
#12858=VECTOR('',#57787,0.01);
#12859=VECTOR('',#57792,0.01);
#12860=VECTOR('',#57815,1.);
#12861=VECTOR('',#57816,1.);
#12862=VECTOR('',#57821,1.);
#12863=VECTOR('',#57826,0.999999999999998);
#12864=VECTOR('',#57827,1.);
#12865=VECTOR('',#57834,1.);
#12866=VECTOR('',#57847,1.);
#12867=VECTOR('',#57852,1.);
#12868=VECTOR('',#57853,1.);
#12869=VECTOR('',#57856,1.);
#12870=VECTOR('',#57865,1.);
#12871=VECTOR('',#57870,1.);
#12872=VECTOR('',#57871,1.);
#12873=VECTOR('',#57872,1.);
#12874=VECTOR('',#57883,1.);
#12875=VECTOR('',#57888,1.);
#12876=VECTOR('',#57889,1.);
#12877=VECTOR('',#57892,1.);
#12878=VECTOR('',#57905,1.);
#12879=VECTOR('',#57910,1.);
#12880=VECTOR('',#57911,1.);
#12881=VECTOR('',#57914,1.);
#12882=VECTOR('',#57927,1.);
#12883=VECTOR('',#57932,0.01);
#12884=VECTOR('',#57933,1.);
#12885=VECTOR('',#57936,0.01);
#12886=VECTOR('',#57941,0.01);
#12887=VECTOR('',#57974,1.);
#12888=VECTOR('',#57975,1.);
#12889=VECTOR('',#57980,1.);
#12890=VECTOR('',#57985,1.);
#12891=VECTOR('',#57986,1.);
#12892=VECTOR('',#57991,1.);
#12893=VECTOR('',#57996,1.);
#12894=VECTOR('',#58001,1.);
#12895=VECTOR('',#58002,1.);
#12896=VECTOR('',#58005,1.);
#12897=VECTOR('',#58014,1.);
#12898=VECTOR('',#58019,1.);
#12899=VECTOR('',#58020,1.);
#12900=VECTOR('',#58021,1.);
#12901=VECTOR('',#58032,1.);
#12902=VECTOR('',#58037,1.);
#12903=VECTOR('',#58038,1.);
#12904=VECTOR('',#58041,1.);
#12905=VECTOR('',#58054,1.);
#12906=VECTOR('',#58059,1.);
#12907=VECTOR('',#58060,1.);
#12908=VECTOR('',#58063,1.);
#12909=VECTOR('',#58076,1.);
#12910=VECTOR('',#58081,0.01);
#12911=VECTOR('',#58082,1.);
#12912=VECTOR('',#58085,0.01);
#12913=VECTOR('',#58090,0.01);
#12914=VECTOR('',#58131,1.);
#12915=VECTOR('',#58136,1.);
#12916=VECTOR('',#58137,1.);
#12917=VECTOR('',#58142,1.);
#12918=VECTOR('',#58147,1.);
#12919=VECTOR('',#58152,1.);
#12920=VECTOR('',#58153,1.);
#12921=VECTOR('',#58154,1.);
#12922=VECTOR('',#58155,1.);
#12923=VECTOR('',#58160,1.);
#12924=VECTOR('',#58161,1.);
#12925=VECTOR('',#58162,1.);
#12926=VECTOR('',#58169,1.);
#12927=VECTOR('',#58170,1.);
#12928=VECTOR('',#58181,1.);
#12929=VECTOR('',#58186,1.);
#12930=VECTOR('',#58187,1.);
#12931=VECTOR('',#58190,1.);
#12932=VECTOR('',#58203,1.);
#12933=VECTOR('',#58208,1.);
#12934=VECTOR('',#58209,1.);
#12935=VECTOR('',#58212,1.);
#12936=VECTOR('',#58225,1.);
#12937=VECTOR('',#58230,0.01);
#12938=VECTOR('',#58231,1.);
#12939=VECTOR('',#58234,0.01);
#12940=VECTOR('',#58239,0.01);
#12941=VECTOR('',#58286,1.);
#12942=VECTOR('',#58291,1.);
#12943=VECTOR('',#58292,1.);
#12944=VECTOR('',#58293,1.);
#12945=VECTOR('',#58294,0.999999999999999);
#12946=VECTOR('',#58299,1.);
#12947=VECTOR('',#58300,1.);
#12948=VECTOR('',#58301,1.);
#12949=VECTOR('',#58306,1.);
#12950=VECTOR('',#58311,0.999999999999999);
#12951=VECTOR('',#58312,1.);
#12952=VECTOR('',#58315,1.);
#12953=VECTOR('',#58322,0.999999999999999);
#12954=VECTOR('',#58323,1.);
#12955=VECTOR('',#58328,1.);
#12956=VECTOR('',#58333,1.);
#12957=VECTOR('',#58334,1.);
#12958=VECTOR('',#58339,1.);
#12959=VECTOR('',#58352,1.);
#12960=VECTOR('',#58357,1.);
#12961=VECTOR('',#58358,1.);
#12962=VECTOR('',#58361,1.);
#12963=VECTOR('',#58374,1.);
#12964=VECTOR('',#58379,0.01);
#12965=VECTOR('',#58380,1.);
#12966=VECTOR('',#58383,0.01);
#12967=VECTOR('',#58388,0.01);
#12968=VECTOR('',#58441,1.);
#12969=VECTOR('',#58446,1.);
#12970=VECTOR('',#58447,1.);
#12971=VECTOR('',#58448,1.);
#12972=VECTOR('',#58453,1.);
#12973=VECTOR('',#58458,0.999999999999999);
#12974=VECTOR('',#58459,1.);
#12975=VECTOR('',#58460,1.);
#12976=VECTOR('',#58465,1.);
#12977=VECTOR('',#58470,1.);
#12978=VECTOR('',#58471,1.);
#12979=VECTOR('',#58474,1.);
#12980=VECTOR('',#58481,1.);
#12981=VECTOR('',#58482,1.);
#12982=VECTOR('',#58487,1.);
#12983=VECTOR('',#58492,1.);
#12984=VECTOR('',#58493,1.);
#12985=VECTOR('',#58498,1.);
#12986=VECTOR('',#58503,1.);
#12987=VECTOR('',#58508,1.);
#12988=VECTOR('',#58509,1.);
#12989=VECTOR('',#58510,1.);
#12990=VECTOR('',#58523,1.);
#12991=VECTOR('',#58528,0.01);
#12992=VECTOR('',#58529,1.);
#12993=VECTOR('',#58532,0.01);
#12994=VECTOR('',#58537,0.01);
#12995=VECTOR('',#58604,1.);
#12996=VECTOR('',#58609,1.);
#12997=VECTOR('',#58610,1.);
#12998=VECTOR('',#58611,1.);
#12999=VECTOR('',#58616,1.);
#13000=VECTOR('',#58621,1.);
#13001=VECTOR('',#58622,1.);
#13002=VECTOR('',#58623,1.);
#13003=VECTOR('',#58628,1.);
#13004=VECTOR('',#58633,0.01);
#13005=VECTOR('',#58634,1.);
#13006=VECTOR('',#58637,0.01);
#13007=VECTOR('',#58644,1.);
#13008=VECTOR('',#58645,1.);
#13009=VECTOR('',#58650,1.);
#13010=VECTOR('',#58655,1.);
#13011=VECTOR('',#58656,1.);
#13012=VECTOR('',#58661,1.);
#13013=VECTOR('',#58666,1.);
#13014=VECTOR('',#58671,1.);
#13015=VECTOR('',#58672,1.);
#13016=VECTOR('',#58673,1.);
#13017=VECTOR('',#58674,1.);
#13018=VECTOR('',#58679,1.);
#13019=VECTOR('',#58680,1.);
#13020=VECTOR('',#58681,1.);
#13021=VECTOR('',#58686,0.01);
#13022=VECTOR('',#58697,0.01);
#13624=CIRCLE('',#45719,0.00150000000001001);
#13625=CIRCLE('',#45720,0.00150000000001001);
#13626=CIRCLE('',#45722,0.00550000000001001);
#13627=CIRCLE('',#45723,0.0101999634198228);
#13628=CIRCLE('',#45724,0.00961011190536243);
#13629=CIRCLE('',#45725,0.010199963424716);
#13630=CIRCLE('',#45726,0.00961011190549176);
#13631=CIRCLE('',#45727,0.010199963406456);
#13632=CIRCLE('',#45728,0.0096101119054614);
#13633=CIRCLE('',#45729,0.0101999634077649);
#13634=CIRCLE('',#45730,0.00961011190527579);
#13635=CIRCLE('',#45731,0.0101999634686637);
#13636=CIRCLE('',#45732,0.00961011190568892);
#13637=CIRCLE('',#45733,0.010199963468495);
#13638=CIRCLE('',#45734,0.0096101119055966);
#13639=CIRCLE('',#45735,0.0101999634692665);
#13640=CIRCLE('',#45736,0.0096101119055853);
#13641=CIRCLE('',#45737,0.010199963406071);
#13642=CIRCLE('',#45738,0.00961011190544941);
#13643=CIRCLE('',#45739,0.0101999634685094);
#13644=CIRCLE('',#45740,0.00961011190559131);
#13645=CIRCLE('',#45741,0.0101999634061418);
#13646=CIRCLE('',#45742,0.00961011190556026);
#13647=CIRCLE('',#45743,0.0101999634122045);
#13648=CIRCLE('',#45744,0.00961011190565787);
#13649=CIRCLE('',#45745,0.0101999634683188);
#13650=CIRCLE('',#45746,0.00961011190573388);
#13651=CIRCLE('',#45747,0.010199963468478);
#13652=CIRCLE('',#45748,0.00961011190561557);
#13653=CIRCLE('',#45749,0.010199963468907);
#13654=CIRCLE('',#45750,0.00961011190548147);
#13655=CIRCLE('',#45751,0.0101999634060557);
#13656=CIRCLE('',#45752,0.00961011190541856);
#13657=CIRCLE('',#45753,0.0101999634064124);
#13658=CIRCLE('',#45754,0.00961011190591087);
#13659=CIRCLE('',#45755,0.0101999634061439);
#13660=CIRCLE('',#45756,0.00961011190542911);
#13661=CIRCLE('',#45757,0.0101999634689394);
#13662=CIRCLE('',#45758,0.00961011190529722);
#13663=CIRCLE('',#45759,0.0101999634686951);
#13664=CIRCLE('',#45760,0.00961011190550351);
#13665=CIRCLE('',#45761,0.0101999634689749);
#13666=CIRCLE('',#45762,0.0096101119053556);
#13667=CIRCLE('',#45763,0.0101999634535387);
#13668=CIRCLE('',#45764,0.00961011190563452);
#13669=CIRCLE('',#45765,0.010199963468864);
#13670=CIRCLE('',#45766,0.00961011190551607);
#13671=CIRCLE('',#45767,0.0101999634130628);
#13672=CIRCLE('',#45768,0.00961011190524368);
#13673=CIRCLE('',#45769,0.0101999634342632);
#13674=CIRCLE('',#45770,0.00961011190543232);
#13675=CIRCLE('',#45771,0.0101999634059357);
#13676=CIRCLE('',#45772,0.00961011190551928);
#13677=CIRCLE('',#45773,0.0101999634691664);
#13678=CIRCLE('',#45774,0.00961011257877421);
#13679=CIRCLE('',#45775,0.0101999634074436);
#13680=CIRCLE('',#45776,0.00961011257877713);
#13681=CIRCLE('',#45777,0.0101999634064149);
#13682=CIRCLE('',#45778,0.00961011190539081);
#13683=CIRCLE('',#45779,0.0101999634680358);
#13684=CIRCLE('',#45780,0.00961011190545386);
#13685=CIRCLE('',#45781,0.0101999634383056);
#13686=CIRCLE('',#45782,0.00961011190542872);
#13687=CIRCLE('',#45783,0.0101999634686043);
#13688=CIRCLE('',#45784,0.00961011190523193);
#13689=CIRCLE('',#45785,0.0101999634688037);
#13690=CIRCLE('',#45786,0.00961011190527582);
#13691=CIRCLE('',#45787,0.0101999634682683);
#13692=CIRCLE('',#45788,0.00961011190538962);
#13693=CIRCLE('',#45789,0.010199963406837);
#13694=CIRCLE('',#45790,0.00961011190522354);
#13695=CIRCLE('',#45791,0.0101999634066951);
#13696=CIRCLE('',#45792,0.00961011190518779);
#13697=CIRCLE('',#45793,0.0101999634687797);
#13698=CIRCLE('',#45794,0.0096101119054408);
#13699=CIRCLE('',#45795,0.0101999634124819);
#13700=CIRCLE('',#45796,0.00961011190539864);
#13701=CIRCLE('',#45797,0.0101999634688732);
#13702=CIRCLE('',#45798,0.00961011190543064);
#13703=CIRCLE('',#45799,0.0101999634686598);
#13704=CIRCLE('',#45800,0.00961011190546885);
#13705=CIRCLE('',#45801,0.0101999634685102);
#13706=CIRCLE('',#45802,0.00961011190533588);
#13707=CIRCLE('',#45803,0.0101999634689061);
#13708=CIRCLE('',#45804,0.00961011190537567);
#13709=CIRCLE('',#45805,0.010199963468622);
#13710=CIRCLE('',#45806,0.00961011190512478);
#13711=CIRCLE('',#45807,0.0101999634685834);
#13712=CIRCLE('',#45808,0.00961011190557325);
#13713=CIRCLE('',#45809,0.0101999634135171);
#13714=CIRCLE('',#45810,0.00961011190532499);
#13715=CIRCLE('',#45811,0.0101999634144479);
#13716=CIRCLE('',#45812,0.00961011190541419);
#13717=CIRCLE('',#45813,0.0101999634682382);
#13718=CIRCLE('',#45814,0.00961011190539613);
#13719=CIRCLE('',#45815,0.010199963468837);
#13720=CIRCLE('',#45816,0.0096101119055694);
#13721=CIRCLE('',#45817,0.0101999634070027);
#13722=CIRCLE('',#45818,0.00961011257882628);
#13723=CIRCLE('',#45819,0.0101999634068588);
#13724=CIRCLE('',#45820,0.00961011190535638);
#13725=CIRCLE('',#45821,0.0101999634058789);
#13726=CIRCLE('',#45822,0.00961011190522167);
#13727=CIRCLE('',#45824,0.00550000000000999);
#13728=CIRCLE('',#45825,0.0102493166482249);
#13729=CIRCLE('',#45826,0.0053246973266101);
#13730=CIRCLE('',#45827,0.00475546947659179);
#13731=CIRCLE('',#45828,0.00648603628634445);
#13732=CIRCLE('',#45829,0.0102493166718611);
#13733=CIRCLE('',#45830,0.0102493166487836);
#13734=CIRCLE('',#45831,0.00532469732665603);
#13735=CIRCLE('',#45832,0.00475546947669687);
#13736=CIRCLE('',#45833,0.00648603628675515);
#13737=CIRCLE('',#45834,0.0102493166715216);
#13738=CIRCLE('',#45835,0.0102493166104809);
#13739=CIRCLE('',#45836,0.00532469732652641);
#13740=CIRCLE('',#45837,0.00475546947650176);
#13741=CIRCLE('',#45838,0.00648603628632398);
#13742=CIRCLE('',#45839,0.0102493166719252);
#13743=CIRCLE('',#45840,0.0102493166009724);
#13744=CIRCLE('',#45841,0.00532469721575116);
#13745=CIRCLE('',#45842,0.00475546947660697);
#13746=CIRCLE('',#45843,0.00648603622544307);
#13747=CIRCLE('',#45844,0.0102493166717213);
#13748=CIRCLE('',#45845,0.010249316648423);
#13749=CIRCLE('',#45846,0.00532469732666842);
#13750=CIRCLE('',#45847,0.00475546947669352);
#13751=CIRCLE('',#45848,0.00648603628637552);
#13752=CIRCLE('',#45849,0.0102493166245638);
#13753=CIRCLE('',#45850,0.0102493166005703);
#13754=CIRCLE('',#45851,0.0053246973264583);
#13755=CIRCLE('',#45852,0.00475546947661744);
#13756=CIRCLE('',#45853,0.00648603622472093);
#13757=CIRCLE('',#45854,0.0102493166718273);
#13758=CIRCLE('',#45855,0.0102493166425282);
#13759=CIRCLE('',#45856,0.0053246973263111);
#13760=CIRCLE('',#45857,0.00475546947674408);
#13761=CIRCLE('',#45858,0.00648603628642182);
#13762=CIRCLE('',#45859,0.0102493166722208);
#13763=CIRCLE('',#45860,0.0102493166480392);
#13764=CIRCLE('',#45861,0.00532469732662197);
#13765=CIRCLE('',#45862,0.00475546947672397);
#13766=CIRCLE('',#45863,0.00648603622510153);
#13767=CIRCLE('',#45864,0.0102493166712224);
#13768=CIRCLE('',#45865,0.0102493166012379);
#13769=CIRCLE('',#45866,0.00532469732691152);
#13770=CIRCLE('',#45867,0.00475546947675362);
#13771=CIRCLE('',#45868,0.00648603628632466);
#13772=CIRCLE('',#45869,0.0102493166716241);
#13773=CIRCLE('',#45870,0.0102493166479186);
#13774=CIRCLE('',#45871,0.00532469732665895);
#13775=CIRCLE('',#45872,0.00475546947660793);
#13776=CIRCLE('',#45873,0.00648603628636125);
#13777=CIRCLE('',#45874,0.0102493166710006);
#13778=CIRCLE('',#45875,0.0102493166008836);
#13779=CIRCLE('',#45876,0.00532469732698949);
#13780=CIRCLE('',#45877,0.004755469476696);
#13781=CIRCLE('',#45878,0.00648603628639426);
#13782=CIRCLE('',#45879,0.0102493166718501);
#13783=CIRCLE('',#45880,0.0102493166025515);
#13784=CIRCLE('',#45881,0.00532469732649169);
#13785=CIRCLE('',#45882,0.00475546947661964);
#13786=CIRCLE('',#45883,0.00648603628593725);
#13787=CIRCLE('',#45884,0.0102493166238904);
#13788=CIRCLE('',#45885,0.0102493166011681);
#13789=CIRCLE('',#45886,0.00532469732651491);
#13790=CIRCLE('',#45887,0.00475546947656947);
#13791=CIRCLE('',#45888,0.00648603628638922);
#13792=CIRCLE('',#45889,0.0102493166717296);
#13793=CIRCLE('',#45890,0.0102493166477823);
#13794=CIRCLE('',#45891,0.00532469732669679);
#13795=CIRCLE('',#45892,0.0047554694767808);
#13796=CIRCLE('',#45893,0.0064860362863431);
#13797=CIRCLE('',#45894,0.0102493166250233);
#13798=CIRCLE('',#45895,0.0102493166054584);
#13799=CIRCLE('',#45896,0.00532469714696864);
#13800=CIRCLE('',#45897,0.00475546947657628);
#13801=CIRCLE('',#45898,0.00648603628645712);
#13802=CIRCLE('',#45899,0.0102493166243565);
#13803=CIRCLE('',#45900,0.0102493166004352);
#13804=CIRCLE('',#45901,0.00532469719186945);
#13805=CIRCLE('',#45902,0.00475546947659521);
#13806=CIRCLE('',#45903,0.00648603622541537);
#13807=CIRCLE('',#45904,0.0102493166714882);
#13808=CIRCLE('',#45905,0.0102493166051678);
#13809=CIRCLE('',#45906,0.00532469732704207);
#13810=CIRCLE('',#45907,0.00475546947651806);
#13811=CIRCLE('',#45908,0.00648603628635028);
#13812=CIRCLE('',#45909,0.0102493166241683);
#13813=CIRCLE('',#45910,0.0102493166050561);
#13814=CIRCLE('',#45911,0.00532469732762967);
#13815=CIRCLE('',#45912,0.00475546947641074);
#13816=CIRCLE('',#45913,0.00648603628667914);
#13817=CIRCLE('',#45914,0.0102493166242875);
#13818=CIRCLE('',#45915,0.0102493166003182);
#13819=CIRCLE('',#45916,0.00532469732627292);
#13820=CIRCLE('',#45917,0.00475546947642505);
#13821=CIRCLE('',#45918,0.00648603628637591);
#13822=CIRCLE('',#45919,0.01024931662477);
#13823=CIRCLE('',#45920,0.0102493166012571);
#13824=CIRCLE('',#45921,0.00532469732746319);
#13825=CIRCLE('',#45922,0.00475546947649367);
#13826=CIRCLE('',#45923,0.00648603628630755);
#13827=CIRCLE('',#45924,0.0102493166718604);
#13828=CIRCLE('',#45925,0.0102493166484345);
#13829=CIRCLE('',#45926,0.00532469732665917);
#13830=CIRCLE('',#45927,0.00475546947633255);
#13831=CIRCLE('',#45928,0.0064860362254672);
#13832=CIRCLE('',#45929,0.0102493166247972);
#13833=CIRCLE('',#45930,0.0102493166483869);
#13834=CIRCLE('',#45931,0.00532469732679201);
#13835=CIRCLE('',#45932,0.00475546947631373);
#13836=CIRCLE('',#45933,0.0064860362863926);
#13837=CIRCLE('',#45934,0.0102493166720589);
#13838=CIRCLE('',#45935,0.0102493166714337);
#13839=CIRCLE('',#45936,0.00532469722681492);
#13840=CIRCLE('',#45937,0.0047554694764722);
#13841=CIRCLE('',#45938,0.0064860362862893);
#13842=CIRCLE('',#45939,0.0102493166242712);
#13843=CIRCLE('',#45940,0.0102493166052055);
#13844=CIRCLE('',#45941,0.00532469736046863);
#13845=CIRCLE('',#45942,0.00475546947651302);
#13846=CIRCLE('',#45943,0.00648603629473408);
#13847=CIRCLE('',#45944,0.0102493166288082);
#13848=CIRCLE('',#45945,0.0102493166484294);
#13849=CIRCLE('',#45946,0.00532469732671263);
#13850=CIRCLE('',#45947,0.00475546947665501);
#13851=CIRCLE('',#45948,0.0064860362944419);
#13852=CIRCLE('',#45949,0.0102496495656366);
#13853=CIRCLE('',#45950,0.0102493166480359);
#13854=CIRCLE('',#45951,0.00532469732665437);
#13855=CIRCLE('',#45952,0.00475546947623826);
#13856=CIRCLE('',#45953,0.00648603628674945);
#13857=CIRCLE('',#45954,0.0102493166717214);
#13858=CIRCLE('',#45955,0.0102493166485119);
#13859=CIRCLE('',#45956,0.00532469732678191);
#13860=CIRCLE('',#45957,0.00475546947640079);
#13861=CIRCLE('',#45958,0.00648603628633778);
#13862=CIRCLE('',#45959,0.0102493166239895);
#13863=CIRCLE('',#45960,0.0102493166330884);
#13864=CIRCLE('',#45961,0.00532469732685707);
#13865=CIRCLE('',#45962,0.00475546947639237);
#13866=CIRCLE('',#45963,0.00648603628599675);
#13867=CIRCLE('',#45964,0.0102493166297343);
#13868=CIRCLE('',#45965,0.0102493166013718);
#13869=CIRCLE('',#45966,0.00532469732648639);
#13870=CIRCLE('',#45967,0.00475546947668858);
#13871=CIRCLE('',#45968,0.00648603623363353);
#13872=CIRCLE('',#45969,0.0102493166243019);
#13873=CIRCLE('',#45970,0.0102493166717791);
#13874=CIRCLE('',#45971,0.00532469733008092);
#13875=CIRCLE('',#45972,0.00475546947645808);
#13876=CIRCLE('',#45973,0.00648603628640931);
#13877=CIRCLE('',#45974,0.0102493166719781);
#13878=CIRCLE('',#45975,0.010249316648395);
#13879=CIRCLE('',#45976,0.005324697326878);
#13880=CIRCLE('',#45977,0.00475546947653182);
#13881=CIRCLE('',#45978,0.00648603628598081);
#13882=CIRCLE('',#45979,0.0102493166237232);
#13883=CIRCLE('',#45980,0.0102493166023052);
#13884=CIRCLE('',#45981,0.0053246973266947);
#13885=CIRCLE('',#45982,0.00475546947629264);
#13886=CIRCLE('',#45983,0.00648603628636186);
#13887=CIRCLE('',#45984,0.0102493166717635);
#13888=CIRCLE('',#45985,0.0102493166479927);
#13889=CIRCLE('',#45986,0.00532469732661717);
#13890=CIRCLE('',#45987,0.0047554694764501);
#13891=CIRCLE('',#45988,0.00648603628640458);
#13892=CIRCLE('',#45989,0.0102493166719148);
#13893=CIRCLE('',#45990,0.0102493166007194);
#13894=CIRCLE('',#45991,0.00532469732664688);
#13895=CIRCLE('',#45992,0.00475546947636627);
#13896=CIRCLE('',#45993,0.00648603622475047);
#13897=CIRCLE('',#45994,0.0102493166241635);
#13898=CIRCLE('',#45995,0.0102493166052413);
#13899=CIRCLE('',#45996,0.00532469732675286);
#13900=CIRCLE('',#45997,0.00475546947649013);
#13901=CIRCLE('',#45998,0.00648603628639659);
#13902=CIRCLE('',#45999,0.0102493166716537);
#13903=CIRCLE('',#46000,0.0102493166482303);
#13904=CIRCLE('',#46001,0.0053246973262865);
#13905=CIRCLE('',#46002,0.00475546947630579);
#13906=CIRCLE('',#46003,0.00648603622505416);
#13907=CIRCLE('',#46004,0.0102493166239091);
#13908=CIRCLE('',#46005,0.0102493166478681);
#13909=CIRCLE('',#46006,0.00532469732668171);
#13910=CIRCLE('',#46007,0.00475546947629698);
#13911=CIRCLE('',#46008,0.00648603622531174);
#13912=CIRCLE('',#46009,0.0102493166240524);
#13913=CIRCLE('',#46010,0.0102493166479907);
#13914=CIRCLE('',#46011,0.0053246973267911);
#13915=CIRCLE('',#46012,0.00475546947628155);
#13916=CIRCLE('',#46013,0.00648603628643135);
#13917=CIRCLE('',#46014,0.0102493166717961);
#13918=CIRCLE('',#46015,0.0102493166481149);
#13919=CIRCLE('',#46016,0.00532469732675658);
#13920=CIRCLE('',#46017,0.00475546947656979);
#13921=CIRCLE('',#46018,0.00648603628637084);
#13922=CIRCLE('',#46019,0.0102493166494609);
#13923=CIRCLE('',#46020,0.0102493166022047);
#13924=CIRCLE('',#46021,0.00532469732677744);
#13925=CIRCLE('',#46022,0.00475546947636188);
#13926=CIRCLE('',#46023,0.00648603628633145);
#13927=CIRCLE('',#46024,0.0102493166241846);
#13928=CIRCLE('',#46025,0.0102493166181535);
#13929=CIRCLE('',#46026,0.0053246971466303);
#13930=CIRCLE('',#46027,0.00475546947635082);
#13931=CIRCLE('',#46028,0.00648603628599);
#13932=CIRCLE('',#46029,0.0102493166246586);
#13933=CIRCLE('',#46030,0.0102493166006857);
#13934=CIRCLE('',#46031,0.00532469732601802);
#13935=CIRCLE('',#46032,0.00475546947642643);
#13936=CIRCLE('',#46033,0.00648603628591527);
#13937=CIRCLE('',#46034,0.0102493166716824);
#13938=CIRCLE('',#46035,0.0102493166441937);
#13939=CIRCLE('',#46036,0.00532469732637081);
#13940=CIRCLE('',#46037,0.0047554694765186);
#13941=CIRCLE('',#46038,0.00648603628632817);
#13942=CIRCLE('',#46039,0.0102493166241877);
#13943=CIRCLE('',#46040,0.0102493166338346);
#13944=CIRCLE('',#46041,0.00532469732662526);
#13945=CIRCLE('',#46042,0.00475546947642523);
#13946=CIRCLE('',#46043,0.00648603628644076);
#13947=CIRCLE('',#46044,0.0102493166242875);
#13948=CIRCLE('',#46045,0.0102493166008074);
#13949=CIRCLE('',#46046,0.00532469732655984);
#13950=CIRCLE('',#46047,0.00475546947646747);
#13951=CIRCLE('',#46048,0.00648603628642339);
#13952=CIRCLE('',#46049,0.0102493166386258);
#13953=CIRCLE('',#46050,0.0102493166015152);
#13954=CIRCLE('',#46051,0.00532469732729442);
#13955=CIRCLE('',#46052,0.0047554694765978);
#13956=CIRCLE('',#46053,0.00648603628666572);
#13957=CIRCLE('',#46054,0.0102493166713575);
#13958=CIRCLE('',#46055,0.0102493166001166);
#13959=CIRCLE('',#46056,0.00532469732654698);
#13960=CIRCLE('',#46057,0.00475546947657245);
#13961=CIRCLE('',#46058,0.00648603628626377);
#13962=CIRCLE('',#46059,0.0102493166244758);
#13963=CIRCLE('',#46060,0.0102493166486952);
#13964=CIRCLE('',#46061,0.00532469732693619);
#13965=CIRCLE('',#46062,0.00475546947644521);
#13966=CIRCLE('',#46063,0.00648603628674011);
#13967=CIRCLE('',#46064,0.010249316671993);
#13968=CIRCLE('',#46065,0.0102493166001336);
#13969=CIRCLE('',#46066,0.00532469732673807);
#13970=CIRCLE('',#46067,0.00475546947659657);
#13971=CIRCLE('',#46068,0.00648603628634253);
#13972=CIRCLE('',#46069,0.0102493166245827);
#13973=CIRCLE('',#46070,0.0102493166485861);
#13974=CIRCLE('',#46071,0.00532469732688642);
#13975=CIRCLE('',#46072,0.00475546947650669);
#13976=CIRCLE('',#46073,0.00648603628629632);
#13977=CIRCLE('',#46074,0.0167157066785444);
#13978=CIRCLE('',#46075,0.0109625450112925);
#13979=CIRCLE('',#46077,0.0165541458345315);
#13980=CIRCLE('',#46078,0.0168110399842234);
#13981=CIRCLE('',#46079,0.0110459668039187);
#13982=CIRCLE('',#46080,0.0167928000137521);
#13983=CIRCLE('',#46081,0.0110624552741157);
#13984=CIRCLE('',#46083,0.0167157066790098);
#13985=CIRCLE('',#46084,0.010962545020111);
#13986=CIRCLE('',#46085,0.0166052621069394);
#13987=CIRCLE('',#46086,0.016554145912157);
#13988=CIRCLE('',#46088,0.016557944649642);
#13989=CIRCLE('',#46089,0.0165541496597369);
#13990=CIRCLE('',#46090,0.0165579409211877);
#13991=CIRCLE('',#46094,0.0166048023975909);
#13992=CIRCLE('',#46095,0.0166052658421244);
#13993=CIRCLE('',#46096,0.0166047988011243);
#13994=CIRCLE('',#46098,0.0165579409681659);
#13995=CIRCLE('',#46099,0.016557944360907);
#13996=CIRCLE('',#46100,0.0165541492774108);
#13997=CIRCLE('',#46101,0.0167731971567229);
#13998=CIRCLE('',#46102,0.0110573244852915);
#13999=CIRCLE('',#46103,0.0168013216994734);
#14000=CIRCLE('',#46104,0.0110316530748901);
#14001=CIRCLE('',#46105,0.0167928000125642);
#14002=CIRCLE('',#46106,0.0110624552748644);
#14003=CIRCLE('',#46107,0.0168110399833315);
#14004=CIRCLE('',#46108,0.011045966807248);
#14005=CIRCLE('',#46109,0.0165310254138195);
#14006=CIRCLE('',#46110,0.016605262361828);
#14007=CIRCLE('',#46112,0.0165263187395066);
#14008=CIRCLE('',#46113,0.016531029156974);
#14009=CIRCLE('',#46114,0.0165263151375714);
#14010=CIRCLE('',#46116,0.0166047989403509);
#14011=CIRCLE('',#46117,0.0166048024058239);
#14012=CIRCLE('',#46118,0.0166052659708717);
#14013=CIRCLE('',#46119,0.0166775856851178);
#14014=CIRCLE('',#46120,0.0109205691229868);
#14015=CIRCLE('',#46121,0.0168013216990798);
#14016=CIRCLE('',#46122,0.0110316530724368);
#14017=CIRCLE('',#46123,0.0167731941324261);
#14018=CIRCLE('',#46124,0.0110573150837526);
#14019=CIRCLE('',#46125,0.0165310252579689);
#14020=CIRCLE('',#46127,0.0164211205749457);
#14021=CIRCLE('',#46128,0.0164211166382376);
#14022=CIRCLE('',#46130,0.0165263140892247);
#14023=CIRCLE('',#46131,0.016526317515756);
#14024=CIRCLE('',#46132,0.0165310292173529);
#14025=CIRCLE('',#46133,0.0167388235410816);
#14026=CIRCLE('',#46134,0.0109676133194785);
#14027=CIRCLE('',#46135,0.0166825658002112);
#14028=CIRCLE('',#46136,0.011019447276401);
#14029=CIRCLE('',#46137,0.0166775856847206);
#14030=CIRCLE('',#46138,0.0109205691226522);
#14031=CIRCLE('',#46139,0.0165701550626842);
#14032=CIRCLE('',#46141,0.0165733022770367);
#14033=CIRCLE('',#46142,0.0165701587329592);
#14034=CIRCLE('',#46143,0.0165732980302487);
#14035=CIRCLE('',#46145,0.0164211167233465);
#14036=CIRCLE('',#46146,0.016421120810035);
#14037=CIRCLE('',#46147,0.0168141206455738);
#14038=CIRCLE('',#46148,0.0110535372551865);
#14039=CIRCLE('',#46149,0.0168028432283268);
#14040=CIRCLE('',#46150,0.0110635670224663);
#14041=CIRCLE('',#46151,0.0166825658000333);
#14042=CIRCLE('',#46152,0.0110194472775248);
#14043=CIRCLE('',#46153,0.0167388244010463);
#14044=CIRCLE('',#46154,0.0109676127118324);
#14045=CIRCLE('',#46155,0.016601990891616);
#14046=CIRCLE('',#46156,0.0165701584781876);
#14047=CIRCLE('',#46158,0.0166008671691556);
#14048=CIRCLE('',#46159,0.016601990770559);
#14049=CIRCLE('',#46160,0.016600866394852);
#14050=CIRCLE('',#46162,0.0165732944442546);
#14051=CIRCLE('',#46163,0.0165732946042444);
#14052=CIRCLE('',#46164,0.0165701587076333);
#14053=CIRCLE('',#46165,0.0167577810051783);
#14054=CIRCLE('',#46166,0.01105120005134);
#14055=CIRCLE('',#46167,0.0167907391087188);
#14056=CIRCLE('',#46168,0.0110190981868938);
#14057=CIRCLE('',#46169,0.0168028429615406);
#14058=CIRCLE('',#46170,0.0110635670194223);
#14059=CIRCLE('',#46171,0.0168141206274235);
#14060=CIRCLE('',#46172,0.0110535372956647);
#14061=CIRCLE('',#46173,0.00665874948993467);
#14062=CIRCLE('',#46174,0.0166019908649283);
#14063=CIRCLE('',#46176,0.0166008673107098);
#14064=CIRCLE('',#46177,0.016600867411406);
#14065=CIRCLE('',#46178,0.0166019908993219);
#14066=CIRCLE('',#46182,0.0167907391088827);
#14067=CIRCLE('',#46183,0.0110190981864188);
#14068=CIRCLE('',#46184,0.0167577810055165);
#14069=CIRCLE('',#46185,0.0110511996786626);
#14070=CIRCLE('',#46188,0.00665874807859034);
#14071=CIRCLE('',#46189,0.0167157066782481);
#14072=CIRCLE('',#46190,0.0109625450129288);
#14073=CIRCLE('',#46192,0.0165541458650858);
#14074=CIRCLE('',#46194,0.0165579447496526);
#14075=CIRCLE('',#46195,0.0165541495550316);
#14076=CIRCLE('',#46196,0.0165579407230662);
#14077=CIRCLE('',#46197,0.0168110399843813);
#14078=CIRCLE('',#46198,0.0110459668052798);
#14079=CIRCLE('',#46199,0.0167928000139607);
#14080=CIRCLE('',#46200,0.011062455274128);
#14081=CIRCLE('',#46203,0.0166052623896179);
#14082=CIRCLE('',#46204,0.0167731971566023);
#14083=CIRCLE('',#46205,0.0110573244863002);
#14084=CIRCLE('',#46206,0.0168013216994758);
#14085=CIRCLE('',#46207,0.0110316530728458);
#14086=CIRCLE('',#46208,0.0165310255530965);
#14087=CIRCLE('',#46210,0.0166048020948578);
#14088=CIRCLE('',#46211,0.0166052658282088);
#14089=CIRCLE('',#46212,0.0166047987187429);
#14090=CIRCLE('',#46214,0.0165263176787315);
#14091=CIRCLE('',#46215,0.0165310292102148);
#14092=CIRCLE('',#46216,0.0165263141083913);
#14093=CIRCLE('',#46217,0.0166775856847837);
#14094=CIRCLE('',#46218,0.01092056912188);
#14095=CIRCLE('',#46220,0.0164211204563653);
#14096=CIRCLE('',#46221,0.0164211165490995);
#14097=CIRCLE('',#46222,0.0167388248040795);
#14098=CIRCLE('',#46223,0.0109676124292381);
#14099=CIRCLE('',#46224,0.0166825658003758);
#14100=CIRCLE('',#46225,0.0110194472778358);
#14101=CIRCLE('',#46226,0.0165701550024346);
#14102=CIRCLE('',#46228,0.0165733020496899);
#14103=CIRCLE('',#46229,0.0165701586099358);
#14104=CIRCLE('',#46230,0.0165732979706372);
#14105=CIRCLE('',#46231,0.0168141206457996);
#14106=CIRCLE('',#46232,0.0110535372520998);
#14107=CIRCLE('',#46233,0.0168028429612458);
#14108=CIRCLE('',#46234,0.0110635670226642);
#14109=CIRCLE('',#46235,0.0166019908703622);
#14110=CIRCLE('',#46237,0.0166008745056209);
#14111=CIRCLE('',#46238,0.0166019945478856);
#14112=CIRCLE('',#46239,0.0166008708537231);
#14113=CIRCLE('',#46240,0.0167570839933584);
#14114=CIRCLE('',#46241,0.0110512000528469);
#14115=CIRCLE('',#46242,0.0167907391092656);
#14116=CIRCLE('',#46243,0.0110190981844322);
#14117=CIRCLE('',#46244,0.00665874948996591);
#14118=CIRCLE('',#46250,0.0167157066788449);
#14119=CIRCLE('',#46251,0.0109625450157349);
#14120=CIRCLE('',#46253,0.0165541456612475);
#14121=CIRCLE('',#46255,0.016557944529206);
#14122=CIRCLE('',#46256,0.0165541495662002);
#14123=CIRCLE('',#46257,0.0165579404686478);
#14124=CIRCLE('',#46258,0.0168110399833158);
#14125=CIRCLE('',#46259,0.0110459668058598);
#14126=CIRCLE('',#46260,0.0167928000133157);
#14127=CIRCLE('',#46261,0.0110624552757788);
#14128=CIRCLE('',#46264,0.0166052622563343);
#14129=CIRCLE('',#46266,0.0166048019880859);
#14130=CIRCLE('',#46267,0.016605265693657);
#14131=CIRCLE('',#46268,0.0166047985415224);
#14132=CIRCLE('',#46269,0.016773197157004);
#14133=CIRCLE('',#46270,0.0110573244844948);
#14134=CIRCLE('',#46271,0.0168013217003487);
#14135=CIRCLE('',#46272,0.0110316530741932);
#14136=CIRCLE('',#46273,0.016531025536569);
#14137=CIRCLE('',#46274,0.016677585684276);
#14138=CIRCLE('',#46275,0.010920569120958);
#14139=CIRCLE('',#46277,0.0165263177240885);
#14140=CIRCLE('',#46278,0.0165310290137369);
#14141=CIRCLE('',#46279,0.0165263140293687);
#14142=CIRCLE('',#46281,0.0164211203137004);
#14143=CIRCLE('',#46282,0.0164211163601858);
#14144=CIRCLE('',#46283,0.0167388248040086);
#14145=CIRCLE('',#46284,0.0109676124278852);
#14146=CIRCLE('',#46285,0.0166825658000735);
#14147=CIRCLE('',#46286,0.0110194472744378);
#14148=CIRCLE('',#46287,0.01657015489151);
#14149=CIRCLE('',#46289,0.0165733019052232);
#14150=CIRCLE('',#46290,0.0165701584063188);
#14151=CIRCLE('',#46291,0.0165732978847224);
#14152=CIRCLE('',#46292,0.0168141206460675);
#14153=CIRCLE('',#46293,0.0110535372543768);
#14154=CIRCLE('',#46294,0.0168028429612253);
#14155=CIRCLE('',#46295,0.0110635670207699);
#14156=CIRCLE('',#46296,0.0166019908452381);
#14157=CIRCLE('',#46298,0.0166008745510226);
#14158=CIRCLE('',#46299,0.0166019945379808);
#14159=CIRCLE('',#46300,0.0166008707896187);
#14160=CIRCLE('',#46301,0.0167570839934763);
#14161=CIRCLE('',#46302,0.0110511996765818);
#14162=CIRCLE('',#46303,0.0167907391089836);
#14163=CIRCLE('',#46304,0.011019098183272);
#14164=CIRCLE('',#46305,0.00665874807858906);
#14165=CIRCLE('',#46311,0.0167157066783153);
#14166=CIRCLE('',#46312,0.0109625450148706);
#14167=CIRCLE('',#46314,0.0165541457136845);
#14168=CIRCLE('',#46316,0.0165579445181912);
#14169=CIRCLE('',#46317,0.0165541494994364);
#14170=CIRCLE('',#46318,0.0165579404832497);
#14171=CIRCLE('',#46319,0.0168110399843214);
#14172=CIRCLE('',#46320,0.0110459668049122);
#14173=CIRCLE('',#46321,0.0167928000136182);
#14174=CIRCLE('',#46322,0.0110624552755236);
#14175=CIRCLE('',#46325,0.0166052620429394);
#14176=CIRCLE('',#46327,0.0166048019728615);
#14177=CIRCLE('',#46328,0.0166052654892367);
#14178=CIRCLE('',#46329,0.016604798338537);
#14179=CIRCLE('',#46330,0.0167731971568726);
#14180=CIRCLE('',#46331,0.0110573244857002);
#14181=CIRCLE('',#46332,0.0168013216997007);
#14182=CIRCLE('',#46333,0.0110316530729538);
#14183=CIRCLE('',#46334,0.0165310253681436);
#14184=CIRCLE('',#46336,0.016526317656267);
#14185=CIRCLE('',#46337,0.0165310290197966);
#14186=CIRCLE('',#46338,0.016526313977243);
#14187=CIRCLE('',#46339,0.0166775856850731);
#14188=CIRCLE('',#46340,0.0109205691226483);
#14189=CIRCLE('',#46341,0.0167388248041618);
#14190=CIRCLE('',#46342,0.0109676124265561);
#14191=CIRCLE('',#46343,0.0166825658007631);
#14192=CIRCLE('',#46344,0.0110194472758072);
#14193=CIRCLE('',#46345,0.0165701549483552);
#14194=CIRCLE('',#46347,0.016421120963718);
#14195=CIRCLE('',#46348,0.0164211172523543);
#14196=CIRCLE('',#46350,0.0165733019619278);
#14197=CIRCLE('',#46351,0.0165701584484713);
#14198=CIRCLE('',#46352,0.0165732979233713);
#14199=CIRCLE('',#46353,0.0168141206459143);
#14200=CIRCLE('',#46354,0.0110535372553736);
#14201=CIRCLE('',#46355,0.0168028429611379);
#14202=CIRCLE('',#46356,0.0110635670204192);
#14203=CIRCLE('',#46357,0.01660199084655);
#14204=CIRCLE('',#46359,0.0166008740135834);
#14205=CIRCLE('',#46360,0.0166019943862027);
#14206=CIRCLE('',#46361,0.0166008706679157);
#14207=CIRCLE('',#46362,0.0167571840016751);
#14208=CIRCLE('',#46363,0.0110511996779237);
#14209=CIRCLE('',#46364,0.0167907391086096);
#14210=CIRCLE('',#46365,0.0110190981845606);
#14211=CIRCLE('',#46366,0.00665874807872191);
#14212=CIRCLE('',#46372,0.0167157066787399);
#14213=CIRCLE('',#46373,0.0109625450172281);
#14214=CIRCLE('',#46375,0.016554145863149);
#14215=CIRCLE('',#46377,0.0165579443223679);
#14216=CIRCLE('',#46378,0.0165541494393283);
#14217=CIRCLE('',#46379,0.0165579404080053);
#14218=CIRCLE('',#46380,0.0168110399831297);
#14219=CIRCLE('',#46381,0.0110459668041232);
#14220=CIRCLE('',#46382,0.0167928000133307);
#14221=CIRCLE('',#46383,0.0110624552729397);
#14222=CIRCLE('',#46386,0.0166052621959235);
#14223=CIRCLE('',#46388,0.0166048017987275);
#14224=CIRCLE('',#46389,0.0166052655757444);
#14225=CIRCLE('',#46390,0.0166047982632794);
#14226=CIRCLE('',#46391,0.0167731971567896);
#14227=CIRCLE('',#46392,0.0110573244857354);
#14228=CIRCLE('',#46393,0.0168013216998883);
#14229=CIRCLE('',#46394,0.0110316530750987);
#14230=CIRCLE('',#46395,0.0165310254000604);
#14231=CIRCLE('',#46397,0.0165263173244825);
#14232=CIRCLE('',#46398,0.016531029121176);
#14233=CIRCLE('',#46399,0.016526313649102);
#14234=CIRCLE('',#46400,0.0166775856846902);
#14235=CIRCLE('',#46401,0.0109205691217964);
#14236=CIRCLE('',#46403,0.0164211208389438);
#14237=CIRCLE('',#46404,0.0164211169206929);
#14238=CIRCLE('',#46405,0.0167388235414725);
#14239=CIRCLE('',#46406,0.0109676133176049);
#14240=CIRCLE('',#46407,0.0166825658009187);
#14241=CIRCLE('',#46408,0.0110194472773788);
#14242=CIRCLE('',#46409,0.01657015512772);
#14243=CIRCLE('',#46410,0.0168141206463138);
#14244=CIRCLE('',#46411,0.0110535372541819);
#14245=CIRCLE('',#46412,0.0168028429613);
#14246=CIRCLE('',#46413,0.0110635670202627);
#14247=CIRCLE('',#46414,0.0166019908518525);
#14248=CIRCLE('',#46416,0.0165733014219288);
#14249=CIRCLE('',#46417,0.0165701585380017);
#14250=CIRCLE('',#46418,0.0165732976051541);
#14251=CIRCLE('',#46420,0.0166008740668358);
#14252=CIRCLE('',#46421,0.016601994282197);
#14253=CIRCLE('',#46422,0.0166008706697224);
#14254=CIRCLE('',#46423,0.0167571840017961);
#14255=CIRCLE('',#46424,0.0110511996801296);
#14256=CIRCLE('',#46425,0.0167907401351506);
#14257=CIRCLE('',#46426,0.0110190981852389);
#14258=CIRCLE('',#46427,0.00665874808269402);
#14259=CIRCLE('',#46433,0.0167157066787735);
#14260=CIRCLE('',#46434,0.0109625450086395);
#14261=CIRCLE('',#46436,0.0165541457433777);
#14262=CIRCLE('',#46438,0.0165579439802928);
#14263=CIRCLE('',#46439,0.016554149180976);
#14264=CIRCLE('',#46440,0.0165579403754774);
#14265=CIRCLE('',#46441,0.0168110399834262);
#14266=CIRCLE('',#46442,0.0110459668053105);
#14267=CIRCLE('',#46443,0.0167928000135676);
#14268=CIRCLE('',#46444,0.0110624552748488);
#14269=CIRCLE('',#46447,0.0166052621504435);
#14270=CIRCLE('',#46449,0.0166048016472146);
#14271=CIRCLE('',#46450,0.0166052654283215);
#14272=CIRCLE('',#46451,0.0166047981204781);
#14273=CIRCLE('',#46452,0.0167731971565139);
#14274=CIRCLE('',#46453,0.0110573244859286);
#14275=CIRCLE('',#46454,0.0168013216996024);
#14276=CIRCLE('',#46455,0.0110316530737568);
#14277=CIRCLE('',#46456,0.0165310253926076);
#14278=CIRCLE('',#46458,0.0165263173436374);
#14279=CIRCLE('',#46459,0.0165310288225687);
#14280=CIRCLE('',#46460,0.0165263139459922);
#14281=CIRCLE('',#46461,0.0166775856845203);
#14282=CIRCLE('',#46462,0.0109205691218795);
#14283=CIRCLE('',#46464,0.016421120591577);
#14284=CIRCLE('',#46465,0.0164211170893945);
#14285=CIRCLE('',#46466,0.0167388248044872);
#14286=CIRCLE('',#46467,0.0109676124278148);
#14287=CIRCLE('',#46468,0.0166825658003588);
#14288=CIRCLE('',#46469,0.0110194472751782);
#14289=CIRCLE('',#46470,0.0165701550372275);
#14290=CIRCLE('',#46472,0.016573301534994);
#14291=CIRCLE('',#46473,0.0165701582749609);
#14292=CIRCLE('',#46474,0.0165732975210063);
#14293=CIRCLE('',#46475,0.0168141206462113);
#14294=CIRCLE('',#46476,0.011053537257143);
#14295=CIRCLE('',#46477,0.016802842961573);
#14296=CIRCLE('',#46478,0.0110635670197482);
#14297=CIRCLE('',#46479,0.0166019907560126);
#14298=CIRCLE('',#46480,0.0167571840018051);
#14299=CIRCLE('',#46481,0.0110511996746033);
#14300=CIRCLE('',#46482,0.0167907391147266);
#14301=CIRCLE('',#46483,0.0110190981801841);
#14302=CIRCLE('',#46484,0.00665874807845964);
#14303=CIRCLE('',#46486,0.0166008736798517);
#14304=CIRCLE('',#46487,0.0166019943376052);
#14305=CIRCLE('',#46488,0.0166008704639832);
#14306=CIRCLE('',#46494,0.0167157066787271);
#14307=CIRCLE('',#46495,0.0109625450155126);
#14308=CIRCLE('',#46497,0.0165541457593406);
#14309=CIRCLE('',#46499,0.0165579439133504);
#14310=CIRCLE('',#46500,0.016554149284651);
#14311=CIRCLE('',#46501,0.0165579402711089);
#14312=CIRCLE('',#46502,0.0168110399834225);
#14313=CIRCLE('',#46503,0.0110459668054873);
#14314=CIRCLE('',#46504,0.0167928000134005);
#14315=CIRCLE('',#46505,0.0110624552730069);
#14316=CIRCLE('',#46508,0.0166052623894506);
#14317=CIRCLE('',#46510,0.0166048012956226);
#14318=CIRCLE('',#46511,0.0166052652614101);
#14319=CIRCLE('',#46512,0.0166047979814454);
#14320=CIRCLE('',#46513,0.016773197156408);
#14321=CIRCLE('',#46514,0.011057324485339);
#14322=CIRCLE('',#46515,0.0168013216999789);
#14323=CIRCLE('',#46516,0.0110316530746973);
#14324=CIRCLE('',#46517,0.0165310254083766);
#14325=CIRCLE('',#46519,0.0165263171113626);
#14326=CIRCLE('',#46520,0.0165310288164899);
#14327=CIRCLE('',#46521,0.016526313804532);
#14328=CIRCLE('',#46522,0.0166775856843033);
#14329=CIRCLE('',#46523,0.0109205691207937);
#14330=CIRCLE('',#46525,0.0164211206244058);
#14331=CIRCLE('',#46526,0.0164211168117424);
#14332=CIRCLE('',#46527,0.0167388248044568);
#14333=CIRCLE('',#46528,0.0109676124300459);
#14334=CIRCLE('',#46529,0.0166825658003417);
#14335=CIRCLE('',#46530,0.0110194472761544);
#14336=CIRCLE('',#46531,0.0165701550713745);
#14337=CIRCLE('',#46533,0.0165733013649083);
#14338=CIRCLE('',#46534,0.0165701582459345);
#14339=CIRCLE('',#46535,0.0165732975853571);
#14340=CIRCLE('',#46536,0.0168141206461695);
#14341=CIRCLE('',#46537,0.0110535372551713);
#14342=CIRCLE('',#46538,0.0168028429611972);
#14343=CIRCLE('',#46539,0.0110635670196212);
#14344=CIRCLE('',#46540,0.0166019906622895);
#14345=CIRCLE('',#46542,0.0166008736566399);
#14346=CIRCLE('',#46543,0.0166019942352781);
#14347=CIRCLE('',#46544,0.0166008704873754);
#14348=CIRCLE('',#46545,0.0167571840019032);
#14349=CIRCLE('',#46546,0.0110511996781316);
#14350=CIRCLE('',#46547,0.0167907391094546);
#14351=CIRCLE('',#46548,0.0110190981863504);
#14352=CIRCLE('',#46549,0.00665874807845054);
#14353=CIRCLE('',#46555,0.0167157066788714);
#14354=CIRCLE('',#46556,0.0109625450156485);
#14355=CIRCLE('',#46558,0.0165541458403176);
#14356=CIRCLE('',#46560,0.0165579438000108);
#14357=CIRCLE('',#46561,0.0165541491923771);
#14358=CIRCLE('',#46562,0.0165579401565676);
#14359=CIRCLE('',#46563,0.0168110399837841);
#14360=CIRCLE('',#46564,0.01104596680535);
#14361=CIRCLE('',#46565,0.0167928000135096);
#14362=CIRCLE('',#46566,0.0110624552742451);
#14363=CIRCLE('',#46569,0.0166052623307736);
#14364=CIRCLE('',#46571,0.0166048011321904);
#14365=CIRCLE('',#46572,0.0166052652850872);
#14366=CIRCLE('',#46573,0.0166047979680738);
#14367=CIRCLE('',#46574,0.0167731971565765);
#14368=CIRCLE('',#46575,0.0110573244859317);
#14369=CIRCLE('',#46576,0.0168013216998573);
#14370=CIRCLE('',#46577,0.0110316530736586);
#14371=CIRCLE('',#46578,0.0165310254666878);
#14372=CIRCLE('',#46580,0.0165263168519717);
#14373=CIRCLE('',#46581,0.0165310286498186);
#14374=CIRCLE('',#46582,0.0165263136882871);
#14375=CIRCLE('',#46583,0.0166775856847044);
#14376=CIRCLE('',#46584,0.0109205691215522);
#14377=CIRCLE('',#46586,0.0164211204165485);
#14378=CIRCLE('',#46587,0.01642111702004);
#14379=CIRCLE('',#46588,0.0167388248040759);
#14380=CIRCLE('',#46589,0.010967612429176);
#14381=CIRCLE('',#46590,0.0166825658002452);
#14382=CIRCLE('',#46591,0.0110194472759032);
#14383=CIRCLE('',#46592,0.0165701549294572);
#14384=CIRCLE('',#46594,0.0165733010869347);
#14385=CIRCLE('',#46595,0.0165701581404128);
#14386=CIRCLE('',#46596,0.0165732974129815);
#14387=CIRCLE('',#46597,0.0168141206456206);
#14388=CIRCLE('',#46598,0.0110535372554596);
#14389=CIRCLE('',#46599,0.016802842961168);
#14390=CIRCLE('',#46600,0.0110635670198317);
#14391=CIRCLE('',#46601,0.0166019909206233);
#14392=CIRCLE('',#46603,0.0166008736960907);
#14393=CIRCLE('',#46604,0.0166019942659323);
#14394=CIRCLE('',#46605,0.0166008703795521);
#14395=CIRCLE('',#46606,0.0167571840017354);
#14396=CIRCLE('',#46607,0.0110511996746513);
#14397=CIRCLE('',#46608,0.016790739109306);
#14398=CIRCLE('',#46609,0.0110190981849237);
#14399=CIRCLE('',#46610,0.00665874807849537);
#14400=CIRCLE('',#46616,0.0167157066788494);
#14401=CIRCLE('',#46617,0.0109625450144348);
#14402=CIRCLE('',#46619,0.0165541457392142);
#14403=CIRCLE('',#46621,0.0165579435275741);
#14404=CIRCLE('',#46622,0.0165541490391494);
#14405=CIRCLE('',#46623,0.01655794009905);
#14406=CIRCLE('',#46624,0.0168110399836772);
#14407=CIRCLE('',#46625,0.0110459668047881);
#14408=CIRCLE('',#46626,0.0167928000132441);
#14409=CIRCLE('',#46627,0.011062455274256);
#14410=CIRCLE('',#46630,0.0166052622859872);
#14411=CIRCLE('',#46632,0.0166048011030158);
#14412=CIRCLE('',#46633,0.016605265295473);
#14413=CIRCLE('',#46634,0.0166047979887019);
#14414=CIRCLE('',#46635,0.0167731971568965);
#14415=CIRCLE('',#46636,0.0110573244855055);
#14416=CIRCLE('',#46637,0.0168013216999169);
#14417=CIRCLE('',#46638,0.0110316530742442);
#14418=CIRCLE('',#46639,0.0165310254614906);
#14419=CIRCLE('',#46641,0.0165263165791028);
#14420=CIRCLE('',#46642,0.0165310285681001);
#14421=CIRCLE('',#46643,0.01652631359464);
#14422=CIRCLE('',#46644,0.0166775856846869);
#14423=CIRCLE('',#46645,0.0109205691221241);
#14424=CIRCLE('',#46647,0.0164211201277747);
#14425=CIRCLE('',#46648,0.0164211167583284);
#14426=CIRCLE('',#46649,0.0167388248042462);
#14427=CIRCLE('',#46650,0.010967612427505);
#14428=CIRCLE('',#46651,0.0166825658003648);
#14429=CIRCLE('',#46652,0.0110194472768145);
#14430=CIRCLE('',#46653,0.0165701550156401);
#14431=CIRCLE('',#46655,0.016573300951402);
#14432=CIRCLE('',#46656,0.0165701580778124);
#14433=CIRCLE('',#46657,0.0165732974503698);
#14434=CIRCLE('',#46658,0.0168141206459052);
#14435=CIRCLE('',#46659,0.0110535372556727);
#14436=CIRCLE('',#46660,0.0168028429610878);
#14437=CIRCLE('',#46661,0.0110635670209691);
#14438=CIRCLE('',#46662,0.0166019907928354);
#14439=CIRCLE('',#46664,0.0166008734712458);
#14440=CIRCLE('',#46665,0.0166019940729384);
#14441=CIRCLE('',#46666,0.0166008703331209);
#14442=CIRCLE('',#46667,0.0167571840018693);
#14443=CIRCLE('',#46668,0.0110511996747374);
#14444=CIRCLE('',#46669,0.0167907391089814);
#14445=CIRCLE('',#46670,0.0110190981862152);
#14446=CIRCLE('',#46671,0.0066587480786164);
#14447=CIRCLE('',#46677,0.0167157066788542);
#14448=CIRCLE('',#46678,0.010962545014382);
#14449=CIRCLE('',#46680,0.0165541458107732);
#14450=CIRCLE('',#46682,0.01655794340933);
#14451=CIRCLE('',#46683,0.0165541490562889);
#14452=CIRCLE('',#46684,0.0165579399946687);
#14453=CIRCLE('',#46685,0.0168110399835196);
#14454=CIRCLE('',#46686,0.0110459668056131);
#14455=CIRCLE('',#46687,0.0167928000130259);
#14456=CIRCLE('',#46688,0.0110624552743332);
#14457=CIRCLE('',#46691,0.0166052623067422);
#14458=CIRCLE('',#46693,0.0166048008214679);
#14459=CIRCLE('',#46694,0.0166052651212716);
#14460=CIRCLE('',#46695,0.0166047978286768);
#14461=CIRCLE('',#46696,0.0167731971563245);
#14462=CIRCLE('',#46697,0.0110573244853286);
#14463=CIRCLE('',#46698,0.0168013216997433);
#14464=CIRCLE('',#46699,0.0110316530741568);
#14465=CIRCLE('',#46700,0.0165310254486529);
#14466=CIRCLE('',#46702,0.0165263165711203);
#14467=CIRCLE('',#46703,0.0165310285556837);
#14468=CIRCLE('',#46704,0.0165263135008287);
#14469=CIRCLE('',#46705,0.016677585684674);
#14470=CIRCLE('',#46706,0.0109205691216249);
#14471=CIRCLE('',#46708,0.016421119933082);
#14472=CIRCLE('',#46709,0.0164211167102725);
#14473=CIRCLE('',#46710,0.0167388248042328);
#14474=CIRCLE('',#46711,0.0109676124278834);
#14475=CIRCLE('',#46712,0.016682565800226);
#14476=CIRCLE('',#46713,0.0110194472759658);
#14477=CIRCLE('',#46714,0.0165701548739711);
#14478=CIRCLE('',#46716,0.0165733007123841);
#14479=CIRCLE('',#46717,0.0165701579072542);
#14480=CIRCLE('',#46718,0.0165732973056387);
#14481=CIRCLE('',#46719,0.0168141206272229);
#14482=CIRCLE('',#46720,0.0110535372947043);
#14483=CIRCLE('',#46721,0.0168028429611657);
#14484=CIRCLE('',#46722,0.0110635670203127);
#14485=CIRCLE('',#46723,0.0166019907732245);
#14486=CIRCLE('',#46725,0.0166008734031971);
#14487=CIRCLE('',#46726,0.0166019940334412);
#14488=CIRCLE('',#46727,0.0166008701570932);
#14489=CIRCLE('',#46728,0.0167571840017254);
#14490=CIRCLE('',#46729,0.0110511996794246);
#14491=CIRCLE('',#46730,0.0167907391086331);
#14492=CIRCLE('',#46731,0.0110190981843864);
#14493=CIRCLE('',#46732,0.00665874807867345);
#14494=CIRCLE('',#46738,0.0167157066786842);
#14495=CIRCLE('',#46739,0.0109625450142564);
#14496=CIRCLE('',#46741,0.016554145839149);
#14497=CIRCLE('',#46743,0.0165579433023043);
#14498=CIRCLE('',#46744,0.016554148987948);
#14499=CIRCLE('',#46745,0.0165579399145523);
#14500=CIRCLE('',#46746,0.0168110399836963);
#14501=CIRCLE('',#46747,0.0110459668052039);
#14502=CIRCLE('',#46748,0.0167928000132366);
#14503=CIRCLE('',#46749,0.011062455274358);
#14504=CIRCLE('',#46752,0.016605262351716);
#14505=CIRCLE('',#46754,0.0166048007004478);
#14506=CIRCLE('',#46755,0.0166052650989619);
#14507=CIRCLE('',#46756,0.0166047977419434);
#14508=CIRCLE('',#46757,0.0167731971563632);
#14509=CIRCLE('',#46758,0.011057324485821);
#14510=CIRCLE('',#46759,0.0168013216996036);
#14511=CIRCLE('',#46760,0.01103165307418);
#14512=CIRCLE('',#46761,0.01653102540833);
#14513=CIRCLE('',#46763,0.0165263163781144);
#14514=CIRCLE('',#46764,0.0165310283781746);
#14515=CIRCLE('',#46765,0.0165263134035609);
#14516=CIRCLE('',#46766,0.0166775856847597);
#14517=CIRCLE('',#46767,0.0109205691216858);
#14518=CIRCLE('',#46769,0.0164211197695146);
#14519=CIRCLE('',#46770,0.0164211166578231);
#14520=CIRCLE('',#46771,0.0167388248042642);
#14521=CIRCLE('',#46772,0.0109676124290397);
#14522=CIRCLE('',#46773,0.0166825658005341);
#14523=CIRCLE('',#46774,0.0110194472766462);
#14524=CIRCLE('',#46775,0.0165701549958441);
#14525=CIRCLE('',#46777,0.0165733005409841);
#14526=CIRCLE('',#46778,0.0165701578815627);
#14527=CIRCLE('',#46779,0.016573297179401);
#14528=CIRCLE('',#46780,0.0168141205746601);
#14529=CIRCLE('',#46781,0.0110535374113562);
#14530=CIRCLE('',#46782,0.0168028429611159);
#14531=CIRCLE('',#46783,0.0110635670203989);
#14532=CIRCLE('',#46784,0.0166019907645692);
#14533=CIRCLE('',#46786,0.0166008731501757);
#14534=CIRCLE('',#46787,0.0166019938578661);
#14535=CIRCLE('',#46788,0.0166008700795619);
#14536=CIRCLE('',#46789,0.0167571840018104);
#14537=CIRCLE('',#46790,0.0110511996752243);
#14538=CIRCLE('',#46791,0.0167907391089732);
#14539=CIRCLE('',#46792,0.0110190981849284);
#14540=CIRCLE('',#46793,0.00665874807864357);
#14541=CIRCLE('',#46799,0.016715706679058);
#14542=CIRCLE('',#46800,0.0109625450134028);
#14543=CIRCLE('',#46802,0.0165541457916914);
#14544=CIRCLE('',#46804,0.0165579430656142);
#14545=CIRCLE('',#46805,0.0165541488951878);
#14546=CIRCLE('',#46806,0.016557939800831);
#14547=CIRCLE('',#46807,0.0168110399835283);
#14548=CIRCLE('',#46808,0.0110459668053988);
#14549=CIRCLE('',#46809,0.0167928000128959);
#14550=CIRCLE('',#46810,0.0110624552746248);
#14551=CIRCLE('',#46813,0.0166052621808357);
#14552=CIRCLE('',#46815,0.0166048005591929);
#14553=CIRCLE('',#46816,0.0166052650439038);
#14554=CIRCLE('',#46817,0.0166047976643043);
#14555=CIRCLE('',#46818,0.0167731983501938);
#14556=CIRCLE('',#46819,0.011057328194232);
#14557=CIRCLE('',#46820,0.0168013216996613);
#14558=CIRCLE('',#46821,0.0110316530736681);
#14559=CIRCLE('',#46822,0.0165310254746411);
#14560=CIRCLE('',#46824,0.0165263162138977);
#14561=CIRCLE('',#46825,0.0165310283187957);
#14562=CIRCLE('',#46826,0.016526313348087);
#14563=CIRCLE('',#46827,0.0166775856844355);
#14564=CIRCLE('',#46828,0.0109205691220054);
#14565=CIRCLE('',#46830,0.0164211195586707);
#14566=CIRCLE('',#46831,0.0164211165641859);
#14567=CIRCLE('',#46832,0.0167388244016766);
#14568=CIRCLE('',#46833,0.0109676127118461);
#14569=CIRCLE('',#46834,0.0166825658004541);
#14570=CIRCLE('',#46835,0.0110194472760805);
#14571=CIRCLE('',#46836,0.0165701549651593);
#14572=CIRCLE('',#46838,0.0165733004050165);
#14573=CIRCLE('',#46839,0.0165701577605721);
#14574=CIRCLE('',#46840,0.0165732971634873);
#14575=CIRCLE('',#46841,0.0168141206270518);
#14576=CIRCLE('',#46842,0.0110535372968108);
#14577=CIRCLE('',#46843,0.016802842961495);
#14578=CIRCLE('',#46844,0.0110635670201626);
#14579=CIRCLE('',#46845,0.0166019908199673);
#14580=CIRCLE('',#46847,0.0166008730003544);
#14581=CIRCLE('',#46848,0.0166019937860896);
#14582=CIRCLE('',#46849,0.0166008699897132);
#14583=CIRCLE('',#46850,0.0167571840016942);
#14584=CIRCLE('',#46851,0.0110511996751948);
#14585=CIRCLE('',#46852,0.0167907391086622);
#14586=CIRCLE('',#46853,0.0110190981851049);
#14587=CIRCLE('',#46854,0.00665874807858149);
#14588=CIRCLE('',#46860,0.0167157066789418);
#14589=CIRCLE('',#46861,0.0109625450120428);
#14590=CIRCLE('',#46863,0.0165541458124077);
#14591=CIRCLE('',#46865,0.0165579429181672);
#14592=CIRCLE('',#46866,0.0165541488045164);
#14593=CIRCLE('',#46867,0.0165579397757552);
#14594=CIRCLE('',#46868,0.016811039983842);
#14595=CIRCLE('',#46869,0.0110459668054937);
#14596=CIRCLE('',#46870,0.0167928000132036);
#14597=CIRCLE('',#46871,0.0110624552742704);
#14598=CIRCLE('',#46874,0.016605262184445);
#14599=CIRCLE('',#46876,0.0166048003609683);
#14600=CIRCLE('',#46877,0.0166052649419975);
#14601=CIRCLE('',#46878,0.0166047976138641);
#14602=CIRCLE('',#46879,0.0167731971563786);
#14603=CIRCLE('',#46880,0.0110573244859619);
#14604=CIRCLE('',#46881,0.0168013216995128);
#14605=CIRCLE('',#46882,0.0110316530734511);
#14606=CIRCLE('',#46883,0.0165310254124807);
#14607=CIRCLE('',#46885,0.0165263161039668);
#14608=CIRCLE('',#46886,0.0165310282256654);
#14609=CIRCLE('',#46887,0.0165263132667817);
#14610=CIRCLE('',#46888,0.0166775856848087);
#14611=CIRCLE('',#46889,0.0109205691216089);
#14612=CIRCLE('',#46891,0.0164211194140629);
#14613=CIRCLE('',#46892,0.0164211164742805);
#14614=CIRCLE('',#46893,0.0167388235415256);
#14615=CIRCLE('',#46894,0.0109676133181102);
#14616=CIRCLE('',#46895,0.0166825658003835);
#14617=CIRCLE('',#46896,0.0110194472759929);
#14618=CIRCLE('',#46897,0.0165701550060228);
#14619=CIRCLE('',#46899,0.0165733002568834);
#14620=CIRCLE('',#46900,0.0165701577318853);
#14621=CIRCLE('',#46901,0.0165732970574261);
#14622=CIRCLE('',#46902,0.0168141206458311);
#14623=CIRCLE('',#46903,0.0110535372534871);
#14624=CIRCLE('',#46904,0.0168028429615044);
#14625=CIRCLE('',#46905,0.0110635670200074);
#14626=CIRCLE('',#46906,0.0166019907981289);
#14627=CIRCLE('',#46908,0.0166008728515721);
#14628=CIRCLE('',#46909,0.016601993743918);
#14629=CIRCLE('',#46910,0.01660086994767);
#14630=CIRCLE('',#46911,0.0167571840017539);
#14631=CIRCLE('',#46912,0.0110511996747717);
#14632=CIRCLE('',#46913,0.016790739109151);
#14633=CIRCLE('',#46914,0.011019098184771);
#14634=CIRCLE('',#46915,0.00665874807852504);
#14635=CIRCLE('',#46921,0.016715706679042);
#14636=CIRCLE('',#46922,0.0109625450121176);
#14637=CIRCLE('',#46924,0.0165541458179537);
#14638=CIRCLE('',#46926,0.0165579428661948);
#14639=CIRCLE('',#46927,0.0165541488386055);
#14640=CIRCLE('',#46928,0.0165579396627073);
#14641=CIRCLE('',#46929,0.0168110399837985);
#14642=CIRCLE('',#46930,0.0110459668053948);
#14643=CIRCLE('',#46931,0.016792800013335);
#14644=CIRCLE('',#46932,0.0110624552740833);
#14645=CIRCLE('',#46935,0.016605262299189);
#14646=CIRCLE('',#46937,0.016604800193468);
#14647=CIRCLE('',#46938,0.0166052648195743);
#14648=CIRCLE('',#46939,0.0166047975317367);
#14649=CIRCLE('',#46940,0.0167731971566556);
#14650=CIRCLE('',#46941,0.0110573244856772);
#14651=CIRCLE('',#46942,0.0168013216995712);
#14652=CIRCLE('',#46943,0.0110316530743037);
#14653=CIRCLE('',#46944,0.0165310254920278);
#14654=CIRCLE('',#46946,0.016526315910392);
#14655=CIRCLE('',#46947,0.016531028181923);
#14656=CIRCLE('',#46948,0.0165263132269298);
#14657=CIRCLE('',#46949,0.0166775856844546);
#14658=CIRCLE('',#46950,0.0109205691225738);
#14659=CIRCLE('',#46952,0.0164211193103871);
#14660=CIRCLE('',#46953,0.0164211163289822);
#14661=CIRCLE('',#46954,0.016738824804311);
#14662=CIRCLE('',#46955,0.0109676124277876);
#14663=CIRCLE('',#46956,0.0166825658006998);
#14664=CIRCLE('',#46957,0.0110194472765826);
#14665=CIRCLE('',#46958,0.0165701550441626);
#14666=CIRCLE('',#46960,0.016573300064543);
#14667=CIRCLE('',#46961,0.0165701576417903);
#14668=CIRCLE('',#46962,0.0165732970357012);
#14669=CIRCLE('',#46963,0.0168141206457594);
#14670=CIRCLE('',#46964,0.0110535372561457);
#14671=CIRCLE('',#46965,0.0168028429613552);
#14672=CIRCLE('',#46966,0.0110635670203864);
#14673=CIRCLE('',#46967,0.0166019907852403);
#14674=CIRCLE('',#46969,0.0166008726533189);
#14675=CIRCLE('',#46970,0.0166019936781065);
#14676=CIRCLE('',#46971,0.0166008698380475);
#14677=CIRCLE('',#46972,0.0167571840015755);
#14678=CIRCLE('',#46973,0.0110512000527843);
#14679=CIRCLE('',#46974,0.0167907391090083);
#14680=CIRCLE('',#46975,0.0110190981853154);
#14681=CIRCLE('',#46976,0.00665874948998041);
#14682=CIRCLE('',#46982,0.0167157066789768);
#14683=CIRCLE('',#46983,0.0109625450124528);
#14684=CIRCLE('',#46985,0.0165541458153592);
#14685=CIRCLE('',#46987,0.0165579426819535);
#14686=CIRCLE('',#46988,0.0165541486417264);
#14687=CIRCLE('',#46989,0.0165579395870733);
#14688=CIRCLE('',#46990,0.0168110399838875);
#14689=CIRCLE('',#46991,0.0110459668057296);
#14690=CIRCLE('',#46992,0.0167928000131379);
#14691=CIRCLE('',#46993,0.0110624552743193);
#14692=CIRCLE('',#46996,0.016605262379085);
#14693=CIRCLE('',#46998,0.0166048001267036);
#14694=CIRCLE('',#46999,0.0166052648636375);
#14695=CIRCLE('',#47000,0.0166047974056641);
#14696=CIRCLE('',#47001,0.0167731941322786);
#14697=CIRCLE('',#47002,0.011057315084616);
#14698=CIRCLE('',#47003,0.0168013216997332);
#14699=CIRCLE('',#47004,0.0110316530734077);
#14700=CIRCLE('',#47005,0.0165310255275055);
#14701=CIRCLE('',#47007,0.0165263158442697);
#14702=CIRCLE('',#47008,0.0165310280287164);
#14703=CIRCLE('',#47009,0.0165263130706467);
#14704=CIRCLE('',#47010,0.0166775856847185);
#14705=CIRCLE('',#47011,0.0109205691218712);
#14706=CIRCLE('',#47013,0.0164211191001963);
#14707=CIRCLE('',#47014,0.0164211163212165);
#14708=CIRCLE('',#47015,0.0167388235414893);
#14709=CIRCLE('',#47016,0.0109676133206887);
#14710=CIRCLE('',#47017,0.0166825658000383);
#14711=CIRCLE('',#47018,0.0110194472761275);
#14712=CIRCLE('',#47019,0.0165701550641018);
#14713=CIRCLE('',#47021,0.016573299955908);
#14714=CIRCLE('',#47022,0.0165701575707523);
#14715=CIRCLE('',#47023,0.0165732969049596);
#14716=CIRCLE('',#47024,0.0168141206460598);
#14717=CIRCLE('',#47025,0.0110535372557423);
#14718=CIRCLE('',#47026,0.0168028429616789);
#14719=CIRCLE('',#47027,0.0110635670200694);
#14720=CIRCLE('',#47028,0.0166019907372786);
#14721=CIRCLE('',#47030,0.0166008724580541);
#14722=CIRCLE('',#47031,0.0166019935357958);
#14723=CIRCLE('',#47032,0.0166008697383443);
#14724=CIRCLE('',#47033,0.0167571840016023);
#14725=CIRCLE('',#47034,0.0110512000530287);
#14726=CIRCLE('',#47035,0.0167907391088295);
#14727=CIRCLE('',#47036,0.0110190981855165);
#14728=CIRCLE('',#47037,0.00665874948993921);
#14729=CIRCLE('',#47043,0.0167157066789882);
#14730=CIRCLE('',#47044,0.0109625450150047);
#14731=CIRCLE('',#47046,0.0165541458574325);
#14732=CIRCLE('',#47048,0.016557942526337);
#14733=CIRCLE('',#47049,0.0165541486090743);
#14734=CIRCLE('',#47050,0.0165579394753156);
#14735=CIRCLE('',#47051,0.0168110399838102);
#14736=CIRCLE('',#47052,0.0110459668051484);
#14737=CIRCLE('',#47053,0.0167928000130372);
#14738=CIRCLE('',#47054,0.0110624552742874);
#14739=CIRCLE('',#47057,0.0166052623608482);
#14740=CIRCLE('',#47059,0.0166047998884685);
#14741=CIRCLE('',#47060,0.0166052647263381);
#14742=CIRCLE('',#47061,0.0166047973426093);
#14743=CIRCLE('',#47062,0.0167731971565137);
#14744=CIRCLE('',#47063,0.011057324485952);
#14745=CIRCLE('',#47064,0.0168013216994156);
#14746=CIRCLE('',#47065,0.011031653073398);
#14747=CIRCLE('',#47066,0.0165310255032138);
#14748=CIRCLE('',#47068,0.0165263157542874);
#14749=CIRCLE('',#47069,0.016531027963222);
#14750=CIRCLE('',#47070,0.0165263130548289);
#14751=CIRCLE('',#47071,0.0166775856847766);
#14752=CIRCLE('',#47072,0.0109205691221087);
#14753=CIRCLE('',#47074,0.0164211189896864);
#14754=CIRCLE('',#47075,0.0164211161722232);
#14755=CIRCLE('',#47076,0.0167388248043622);
#14756=CIRCLE('',#47077,0.0109676124277629);
#14757=CIRCLE('',#47078,0.0166825658002222);
#14758=CIRCLE('',#47079,0.0110194472759779);
#14759=CIRCLE('',#47080,0.0165701550303073);
#14760=CIRCLE('',#47082,0.0165732997875192);
#14761=CIRCLE('',#47083,0.0165701574824665);
#14762=CIRCLE('',#47084,0.0165732968390795);
#14763=CIRCLE('',#47085,0.0168141206456921);
#14764=CIRCLE('',#47086,0.011053537253665);
#14765=CIRCLE('',#47087,0.0168028429613703);
#14766=CIRCLE('',#47088,0.0110635670200615);
#14767=CIRCLE('',#47089,0.0166019907613543);
#14768=CIRCLE('',#47091,0.0166008723040521);
#14769=CIRCLE('',#47092,0.0166019935105866);
#14770=CIRCLE('',#47093,0.0166008696361459);
#14771=CIRCLE('',#47094,0.016757184001689);
#14772=CIRCLE('',#47095,0.011051199674271);
#14773=CIRCLE('',#47096,0.0167907391089668);
#14774=CIRCLE('',#47097,0.0110190981851912);
#14775=CIRCLE('',#47098,0.00665874807851366);
#14776=CIRCLE('',#47104,0.0167157066787324);
#14777=CIRCLE('',#47105,0.0109625450149831);
#14778=CIRCLE('',#47107,0.0165541458174054);
#14779=CIRCLE('',#47109,0.0165579423489387);
#14780=CIRCLE('',#47110,0.0165541485712035);
#14781=CIRCLE('',#47111,0.0165579393901184);
#14782=CIRCLE('',#47112,0.0168110399833972);
#14783=CIRCLE('',#47113,0.0110459668042894);
#14784=CIRCLE('',#47114,0.0167928000130159);
#14785=CIRCLE('',#47115,0.0110624552742632);
#14786=CIRCLE('',#47118,0.0166052622705376);
#14787=CIRCLE('',#47120,0.0166047997474789);
#14788=CIRCLE('',#47121,0.0166052646439818);
#14789=CIRCLE('',#47122,0.0166047971632048);
#14790=CIRCLE('',#47123,0.0167731971566282);
#14791=CIRCLE('',#47124,0.0110573244865126);
#14792=CIRCLE('',#47125,0.0168013216993064);
#14793=CIRCLE('',#47126,0.0110316530755126);
#14794=CIRCLE('',#47127,0.0165310255575995);
#14795=CIRCLE('',#47129,0.0165263155511315);
#14796=CIRCLE('',#47130,0.0165310280119525);
#14797=CIRCLE('',#47131,0.0165263129783182);
#14798=CIRCLE('',#47132,0.0166775856846212);
#14799=CIRCLE('',#47133,0.0109205691222008);
#14800=CIRCLE('',#47135,0.0164211188655515);
#14801=CIRCLE('',#47136,0.0164211160635202);
#14802=CIRCLE('',#47137,0.0167388248043554);
#14803=CIRCLE('',#47138,0.0109676124277361);
#14804=CIRCLE('',#47139,0.0166825658003021);
#14805=CIRCLE('',#47140,0.011019447276877);
#14806=CIRCLE('',#47141,0.0165701549917329);
#14807=CIRCLE('',#47143,0.0165732995310219);
#14808=CIRCLE('',#47144,0.0165701573426138);
#14809=CIRCLE('',#47145,0.0165732967230516);
#14810=CIRCLE('',#47146,0.0168141206453851);
#14811=CIRCLE('',#47147,0.011053537253855);
#14812=CIRCLE('',#47148,0.0168028429613918);
#14813=CIRCLE('',#47149,0.0110635670201788);
#14814=CIRCLE('',#47150,0.016601990699506);
#14815=CIRCLE('',#47152,0.0166008721089114);
#14816=CIRCLE('',#47153,0.0166019934077686);
#14817=CIRCLE('',#47154,0.0166008695465524);
#14818=CIRCLE('',#47155,0.0167571840016732);
#14819=CIRCLE('',#47156,0.011051199674904);
#14820=CIRCLE('',#47157,0.0167907391085881);
#14821=CIRCLE('',#47158,0.0110190981861391);
#14822=CIRCLE('',#47159,0.00665874807863435);
#14823=CIRCLE('',#47165,0.0167157066789665);
#14824=CIRCLE('',#47166,0.0109625450168683);
#14825=CIRCLE('',#47168,0.0165541458960314);
#14826=CIRCLE('',#47170,0.0165579424243726);
#14827=CIRCLE('',#47171,0.0165541486047321);
#14828=CIRCLE('',#47172,0.0165579395243273);
#14829=CIRCLE('',#47173,0.0168110399840367);
#14830=CIRCLE('',#47174,0.0110459668047921);
#14831=CIRCLE('',#47175,0.0167928000131094);
#14832=CIRCLE('',#47176,0.0110624552733874);
#14833=CIRCLE('',#47179,0.0166052624151451);
#14834=CIRCLE('',#47181,0.0166047997039492);
#14835=CIRCLE('',#47182,0.0166052646301021);
#14836=CIRCLE('',#47183,0.0166047971334831);
#14837=CIRCLE('',#47184,0.0167731971565164);
#14838=CIRCLE('',#47185,0.0110573244858054);
#14839=CIRCLE('',#47186,0.0168013216993822);
#14840=CIRCLE('',#47187,0.0110316530729965);
#14841=CIRCLE('',#47188,0.01653102537938);
#14842=CIRCLE('',#47190,0.0165263154516607);
#14843=CIRCLE('',#47191,0.0165310277099439);
#14844=CIRCLE('',#47192,0.0165263127670499);
#14845=CIRCLE('',#47193,0.016677585684748);
#14846=CIRCLE('',#47194,0.0109205691220697);
#14847=CIRCLE('',#47196,0.01642111861694);
#14848=CIRCLE('',#47197,0.0164211160383969);
#14849=CIRCLE('',#47198,0.0167388248040173);
#14850=CIRCLE('',#47199,0.0109676124293361);
#14851=CIRCLE('',#47200,0.0166825658006657);
#14852=CIRCLE('',#47201,0.0110194472766751);
#14853=CIRCLE('',#47202,0.016570155060932);
#14854=CIRCLE('',#47204,0.0165732995806975);
#14855=CIRCLE('',#47205,0.0165701573868749);
#14856=CIRCLE('',#47206,0.0165732966694879);
#14857=CIRCLE('',#47207,0.0168141206458845);
#14858=CIRCLE('',#47208,0.0110535372544796);
#14859=CIRCLE('',#47209,0.0168028429614423);
#14860=CIRCLE('',#47210,0.0110635670200312);
#14861=CIRCLE('',#47211,0.0166019907852894);
#14862=CIRCLE('',#47213,0.0166008721177798);
#14863=CIRCLE('',#47214,0.016601993410395);
#14864=CIRCLE('',#47215,0.0166008694719737);
#14865=CIRCLE('',#47216,0.0167571840017142);
#14866=CIRCLE('',#47217,0.0110511996802703);
#14867=CIRCLE('',#47218,0.0167907391087389);
#14868=CIRCLE('',#47219,0.0110190981851166);
#14869=CIRCLE('',#47220,0.00665874808274784);
#14870=CIRCLE('',#47226,0.016715706679209);
#14871=CIRCLE('',#47227,0.0109625450128583);
#14872=CIRCLE('',#47229,0.0165541458902804);
#14873=CIRCLE('',#47231,0.0165579419073244);
#14874=CIRCLE('',#47232,0.0165541485288617);
#14875=CIRCLE('',#47233,0.0165579392048);
#14876=CIRCLE('',#47234,0.0168110399835751);
#14877=CIRCLE('',#47235,0.0110459668060784);
#14878=CIRCLE('',#47236,0.016792800012697);
#14879=CIRCLE('',#47237,0.0110624552745184);
#14880=CIRCLE('',#47240,0.0166052624316687);
#14881=CIRCLE('',#47242,0.0166047995343761);
#14882=CIRCLE('',#47243,0.0166052644243831);
#14883=CIRCLE('',#47244,0.0166047970554349);
#14884=CIRCLE('',#47245,0.0167731971566083);
#14885=CIRCLE('',#47246,0.0110573244837942);
#14886=CIRCLE('',#47247,0.0168013216994279);
#14887=CIRCLE('',#47248,0.0110316530744061);
#14888=CIRCLE('',#47249,0.0165310256090931);
#14889=CIRCLE('',#47251,0.0165263151740798);
#14890=CIRCLE('',#47252,0.0165310277948519);
#14891=CIRCLE('',#47253,0.0165263129250178);
#14892=CIRCLE('',#47254,0.0166775856848588);
#14893=CIRCLE('',#47255,0.0109205691212204);
#14894=CIRCLE('',#47257,0.0164211185950565);
#14895=CIRCLE('',#47258,0.0164211159847808);
#14896=CIRCLE('',#47259,0.0167388248045614);
#14897=CIRCLE('',#47260,0.0109676124270857);
#14898=CIRCLE('',#47261,0.0166825658002627);
#14899=CIRCLE('',#47262,0.0110194472759807);
#14900=CIRCLE('',#47263,0.016570155040469);
#14901=CIRCLE('',#47265,0.0165732993554859);
#14902=CIRCLE('',#47266,0.0165701572968777);
#14903=CIRCLE('',#47267,0.0165732965929683);
#14904=CIRCLE('',#47268,0.0168141206459158);
#14905=CIRCLE('',#47269,0.0110535372569532);
#14906=CIRCLE('',#47270,0.016802842961278);
#14907=CIRCLE('',#47271,0.011063567019422);
#14908=CIRCLE('',#47272,0.0166019907597247);
#14909=CIRCLE('',#47274,0.01660087193563);
#14910=CIRCLE('',#47275,0.0166019931914076);
#14911=CIRCLE('',#47276,0.0166008694194318);
#14912=CIRCLE('',#47277,0.0167571840016429);
#14913=CIRCLE('',#47278,0.0110511996751358);
#14914=CIRCLE('',#47279,0.0167907391090019);
#14915=CIRCLE('',#47280,0.0110190981850566);
#14916=CIRCLE('',#47281,0.00665874808271733);
#14917=CIRCLE('',#47287,0.0167157066786898);
#14918=CIRCLE('',#47288,0.0109625450140703);
#14919=CIRCLE('',#47290,0.0165541457088435);
#14920=CIRCLE('',#47292,0.0165579419209612);
#14921=CIRCLE('',#47293,0.0165541485096187);
#14922=CIRCLE('',#47294,0.0165579394649361);
#14923=CIRCLE('',#47295,0.0168110399840163);
#14924=CIRCLE('',#47296,0.0110459668046887);
#14925=CIRCLE('',#47297,0.0167928000131629);
#14926=CIRCLE('',#47298,0.0110624552738361);
#14927=CIRCLE('',#47301,0.0166052623317775);
#14928=CIRCLE('',#47303,0.0166047993749498);
#14929=CIRCLE('',#47304,0.0166052644755989);
#14930=CIRCLE('',#47305,0.0166047969454479);
#14931=CIRCLE('',#47306,0.0167731941325696);
#14932=CIRCLE('',#47307,0.0110573150844451);
#14933=CIRCLE('',#47308,0.0168013216993458);
#14934=CIRCLE('',#47309,0.011031653074156);
#14935=CIRCLE('',#47310,0.0165310256288537);
#14936=CIRCLE('',#47312,0.0165263150151698);
#14937=CIRCLE('',#47313,0.0165310275145087);
#14938=CIRCLE('',#47314,0.016526312778801);
#14939=CIRCLE('',#47315,0.0166775856842448);
#14940=CIRCLE('',#47316,0.0109205691234822);
#14941=CIRCLE('',#47318,0.0164211183560543);
#14942=CIRCLE('',#47319,0.0164211160009157);
#14943=CIRCLE('',#47320,0.0167388235414568);
#14944=CIRCLE('',#47321,0.0109676133201212);
#14945=CIRCLE('',#47322,0.016682565800537);
#14946=CIRCLE('',#47323,0.0110194472762134);
#14947=CIRCLE('',#47324,0.0165701548825087);
#14948=CIRCLE('',#47326,0.0165732991360922);
#14949=CIRCLE('',#47327,0.0165701570900863);
#14950=CIRCLE('',#47328,0.0165732967225825);
#14951=CIRCLE('',#47329,0.016814120645603);
#14952=CIRCLE('',#47330,0.01105353725617);
#14953=CIRCLE('',#47331,0.0168028429620497);
#14954=CIRCLE('',#47332,0.0110635670191861);
#14955=CIRCLE('',#47333,0.0166019907656715);
#14956=CIRCLE('',#47335,0.0166008718074278);
#14957=CIRCLE('',#47336,0.0166019931546632);
#14958=CIRCLE('',#47337,0.0166008693989611);
#14959=CIRCLE('',#47338,0.016757184001536);
#14960=CIRCLE('',#47339,0.011051199674654);
#14961=CIRCLE('',#47340,0.0167907391090067);
#14962=CIRCLE('',#47341,0.0110190981853047);
#14963=CIRCLE('',#47342,0.00665874807851997);
#14964=CIRCLE('',#47348,0.016715706679377);
#14965=CIRCLE('',#47349,0.0109625450099256);
#14966=CIRCLE('',#47351,0.0165541456677397);
#14967=CIRCLE('',#47353,0.0165579417570842);
#14968=CIRCLE('',#47354,0.0165541482253256);
#14969=CIRCLE('',#47355,0.0165579391842505);
#14970=CIRCLE('',#47356,0.0168110399838653);
#14971=CIRCLE('',#47357,0.011045966806135);
#14972=CIRCLE('',#47358,0.0167928000128381);
#14973=CIRCLE('',#47359,0.0110624552737996);
#14974=CIRCLE('',#47362,0.0166052622330066);
#14975=CIRCLE('',#47364,0.0166047990110056);
#14976=CIRCLE('',#47365,0.016605264397152);
#14977=CIRCLE('',#47366,0.0166047967671889);
#14978=CIRCLE('',#47367,0.0167731971567163);
#14979=CIRCLE('',#47368,0.0110573244864769);
#14980=CIRCLE('',#47369,0.0168013216997017);
#14981=CIRCLE('',#47370,0.0110316530730052);
#14982=CIRCLE('',#47371,0.0165310253924406);
#14983=CIRCLE('',#47373,0.0165263148442778);
#14984=CIRCLE('',#47374,0.0165310274387597);
#14985=CIRCLE('',#47375,0.0165263127470437);
#14986=CIRCLE('',#47376,0.016677585684615);
#14987=CIRCLE('',#47377,0.0109205691231124);
#14988=CIRCLE('',#47379,0.0164211182503939);
#14989=CIRCLE('',#47380,0.01642111586262);
#14990=CIRCLE('',#47381,0.0167388235416579);
#14991=CIRCLE('',#47382,0.0109676133205617);
#14992=CIRCLE('',#47383,0.0166825658001667);
#14993=CIRCLE('',#47384,0.0110194472749627);
#14994=CIRCLE('',#47385,0.016570155031964);
#14995=CIRCLE('',#47387,0.0165732988903193);
#14996=CIRCLE('',#47388,0.0165701570326878);
#14997=CIRCLE('',#47389,0.0165732964484296);
#14998=CIRCLE('',#47390,0.0168141206453718);
#14999=CIRCLE('',#47391,0.0110535372569656);
#15000=CIRCLE('',#47392,0.0168028429610742);
#15001=CIRCLE('',#47393,0.0110635670206168);
#15002=CIRCLE('',#47394,0.0166019908598596);
#15003=CIRCLE('',#47396,0.0166008716102798);
#15004=CIRCLE('',#47397,0.0166019931695136);
#15005=CIRCLE('',#47398,0.0166008692496937);
#15006=CIRCLE('',#47399,0.0167571840016719);
#15007=CIRCLE('',#47400,0.011051199674668);
#15008=CIRCLE('',#47401,0.0167907391088039);
#15009=CIRCLE('',#47402,0.0110190981857932);
#15010=CIRCLE('',#47403,0.00665874807867338);
#15011=CIRCLE('',#47409,0.0167157066790264);
#15012=CIRCLE('',#47410,0.0109625450122563);
#15013=CIRCLE('',#47412,0.0165541459279617);
#15014=CIRCLE('',#47414,0.0165579415750164);
#15015=CIRCLE('',#47415,0.0165541483771701);
#15016=CIRCLE('',#47416,0.0165579391484975);
#15017=CIRCLE('',#47417,0.0168110399833571);
#15018=CIRCLE('',#47418,0.0110459668047138);
#15019=CIRCLE('',#47419,0.0167928000136081);
#15020=CIRCLE('',#47420,0.0110624552749001);
#15021=CIRCLE('',#47423,0.0166052623945908);
#15022=CIRCLE('',#47425,0.0166047990219055);
#15023=CIRCLE('',#47426,0.0166052642669552);
#15024=CIRCLE('',#47427,0.0166047967670206);
#15025=CIRCLE('',#47428,0.0167731941320866);
#15026=CIRCLE('',#47429,0.0110573150842326);
#15027=CIRCLE('',#47430,0.0168013216996376);
#15028=CIRCLE('',#47431,0.0110316530743853);
#15029=CIRCLE('',#47432,0.0165310255787377);
#15030=CIRCLE('',#47434,0.0165263146387248);
#15031=CIRCLE('',#47435,0.0165310275016277);
#15032=CIRCLE('',#47436,0.0165263127901589);
#15033=CIRCLE('',#47437,0.0166775856845433);
#15034=CIRCLE('',#47438,0.0109205691215517);
#15035=CIRCLE('',#47440,0.0164211177556893);
#15036=CIRCLE('',#47441,0.0164211158516326);
#15037=CIRCLE('',#47442,0.0167388235420917);
#15038=CIRCLE('',#47443,0.0109676133174696);
#15039=CIRCLE('',#47444,0.0166825658003095);
#15040=CIRCLE('',#47445,0.0110194472756285);
#15041=CIRCLE('',#47446,0.0165701551070582);
#15042=CIRCLE('',#47448,0.0165732988655155);
#15043=CIRCLE('',#47449,0.0165701569487744);
#15044=CIRCLE('',#47450,0.0165732963152157);
#15045=CIRCLE('',#47451,0.016814120627371);
#15046=CIRCLE('',#47452,0.011053537295479);
#15047=CIRCLE('',#47453,0.0168028429613983);
#15048=CIRCLE('',#47454,0.0110635670202091);
#15049=CIRCLE('',#47455,0.0166019907132379);
#15050=CIRCLE('',#47457,0.0166008713632373);
#15051=CIRCLE('',#47458,0.0166019930618939);
#15052=CIRCLE('',#47459,0.0166008693209907);
#15053=CIRCLE('',#47460,0.0167571840018115);
#15054=CIRCLE('',#47461,0.0110511996753908);
#15055=CIRCLE('',#47462,0.0167907391084152);
#15056=CIRCLE('',#47463,0.0110190981848113);
#15057=CIRCLE('',#47464,0.00665874807856962);
#15058=CIRCLE('',#47470,0.0167157066795252);
#15059=CIRCLE('',#47471,0.0109625450105399);
#15060=CIRCLE('',#47473,0.0165541458488985);
#15061=CIRCLE('',#47475,0.0165579414961178);
#15062=CIRCLE('',#47476,0.016554148203893);
#15063=CIRCLE('',#47477,0.0165579390888471);
#15064=CIRCLE('',#47478,0.016811039983394);
#15065=CIRCLE('',#47479,0.0110459668054207);
#15066=CIRCLE('',#47480,0.0167928000126915);
#15067=CIRCLE('',#47481,0.0110624552731583);
#15068=CIRCLE('',#47484,0.0166052623744163);
#15069=CIRCLE('',#47486,0.0166047989081871);
#15070=CIRCLE('',#47487,0.0166052641204778);
#15071=CIRCLE('',#47488,0.0166047967765761);
#15072=CIRCLE('',#47489,0.0167731971564122);
#15073=CIRCLE('',#47490,0.0110573244848604);
#15074=CIRCLE('',#47491,0.0168013216996565);
#15075=CIRCLE('',#47492,0.0110316530728958);
#15076=CIRCLE('',#47493,0.016531025437288);
#15077=CIRCLE('',#47495,0.0165263146554168);
#15078=CIRCLE('',#47496,0.0165310275404691);
#15079=CIRCLE('',#47497,0.0165263124377282);
#15080=CIRCLE('',#47498,0.0166775856846072);
#15081=CIRCLE('',#47499,0.0109205691214054);
#15082=CIRCLE('',#47501,0.0164211179394138);
#15083=CIRCLE('',#47502,0.0164211156339015);
#15084=CIRCLE('',#47503,0.0167388248040325);
#15085=CIRCLE('',#47504,0.0109676124287069);
#15086=CIRCLE('',#47505,0.0166825658000452);
#15087=CIRCLE('',#47506,0.0110194472757815);
#15088=CIRCLE('',#47507,0.0165701549775579);
#15089=CIRCLE('',#47509,0.0165732987883178);
#15090=CIRCLE('',#47510,0.0165701570277774);
#15091=CIRCLE('',#47511,0.0165732961623271);
#15092=CIRCLE('',#47512,0.016814120626826);
#15093=CIRCLE('',#47513,0.0110535372950808);
#15094=CIRCLE('',#47514,0.0168028429613692);
#15095=CIRCLE('',#47515,0.0110635670209873);
#15096=CIRCLE('',#47516,0.0166019907930465);
#15097=CIRCLE('',#47518,0.0166008712589892);
#15098=CIRCLE('',#47519,0.0166019928145345);
#15099=CIRCLE('',#47520,0.0166008692132377);
#15100=CIRCLE('',#47521,0.0167571840016013);
#15101=CIRCLE('',#47522,0.0110511996738178);
#15102=CIRCLE('',#47523,0.01679073910861);
#15103=CIRCLE('',#47524,0.0110190981842078);
#15104=CIRCLE('',#47525,0.00665874807848039);
#15105=CIRCLE('',#47531,0.0167157066795619);
#15106=CIRCLE('',#47532,0.0109625450129655);
#15107=CIRCLE('',#47534,0.0165541457243246);
#15108=CIRCLE('',#47536,0.0165579412106767);
#15109=CIRCLE('',#47537,0.0165541482558227);
#15110=CIRCLE('',#47538,0.0165579386921517);
#15111=CIRCLE('',#47539,0.0168110399838667);
#15112=CIRCLE('',#47540,0.0110459668055425);
#15113=CIRCLE('',#47541,0.0167928000128198);
#15114=CIRCLE('',#47542,0.0110624552748793);
#15115=CIRCLE('',#47545,0.0166052622059834);
#15116=CIRCLE('',#47547,0.016604798651343);
#15117=CIRCLE('',#47548,0.0166052642067028);
#15118=CIRCLE('',#47549,0.0166047966805386);
#15119=CIRCLE('',#47550,0.0167731971562434);
#15120=CIRCLE('',#47551,0.0110573244854881);
#15121=CIRCLE('',#47552,0.0168013216999379);
#15122=CIRCLE('',#47553,0.0110316530754383);
#15123=CIRCLE('',#47554,0.0165310255164065);
#15124=CIRCLE('',#47556,0.0165263144958598);
#15125=CIRCLE('',#47557,0.0165310272807434);
#15126=CIRCLE('',#47558,0.0165263123171155);
#15127=CIRCLE('',#47559,0.0166775856848886);
#15128=CIRCLE('',#47560,0.0109205691224704);
#15129=CIRCLE('',#47562,0.0164211176536645);
#15130=CIRCLE('',#47563,0.0164211156591293);
#15131=CIRCLE('',#47564,0.0167388244022555);
#15132=CIRCLE('',#47565,0.0109676127120857);
#15133=CIRCLE('',#47566,0.0166825658003426);
#15134=CIRCLE('',#47567,0.0110194472767055);
#15135=CIRCLE('',#47568,0.0165701550072313);
#15136=CIRCLE('',#47570,0.0165732986276967);
#15137=CIRCLE('',#47571,0.0165701568562288);
#15138=CIRCLE('',#47572,0.0165732962912302);
#15139=CIRCLE('',#47573,0.0168141206268075);
#15140=CIRCLE('',#47574,0.0110535372934106);
#15141=CIRCLE('',#47575,0.0168028429615418);
#15142=CIRCLE('',#47576,0.0110635670205629);
#15143=CIRCLE('',#47577,0.0166019906012785);
#15144=CIRCLE('',#47579,0.0166008713097932);
#15145=CIRCLE('',#47580,0.0166019929578284);
#15146=CIRCLE('',#47581,0.0166008690696432);
#15147=CIRCLE('',#47582,0.016757781005222);
#15148=CIRCLE('',#47583,0.0110511996751157);
#15149=CIRCLE('',#47584,0.0167907391087404);
#15150=CIRCLE('',#47585,0.0110190981859409);
#15151=CIRCLE('',#47586,0.00665874807854453);
#15152=CIRCLE('',#47592,0.0167157066788644);
#15153=CIRCLE('',#47593,0.0109625450154754);
#15154=CIRCLE('',#47595,0.016554146073238);
#15155=CIRCLE('',#47597,0.0165579411825587);
#15156=CIRCLE('',#47598,0.0165541481365723);
#15157=CIRCLE('',#47599,0.0165579388524576);
#15158=CIRCLE('',#47600,0.0168110399839204);
#15159=CIRCLE('',#47601,0.0110459668037209);
#15160=CIRCLE('',#47602,0.0167928000128627);
#15161=CIRCLE('',#47603,0.0110624552745945);
#15162=CIRCLE('',#47606,0.0166052623891851);
#15163=CIRCLE('',#47608,0.0166047984747976);
#15164=CIRCLE('',#47609,0.0166052639005878);
#15165=CIRCLE('',#47610,0.0166047965284398);
#15166=CIRCLE('',#47611,0.0167731983504133);
#15167=CIRCLE('',#47612,0.0110573281940185);
#15168=CIRCLE('',#47613,0.0168013216993258);
#15169=CIRCLE('',#47614,0.0110316530733178);
#15170=CIRCLE('',#47615,0.0165310256300649);
#15171=CIRCLE('',#47617,0.0165263143157291);
#15172=CIRCLE('',#47618,0.0165310273691108);
#15173=CIRCLE('',#47619,0.0165263125268229);
#15174=CIRCLE('',#47620,0.0166775856847163);
#15175=CIRCLE('',#47621,0.0109205691211382);
#15176=CIRCLE('',#47623,0.0164211175690923);
#15177=CIRCLE('',#47624,0.0164211156634918);
#15178=CIRCLE('',#47625,0.016738824402298);
#15179=CIRCLE('',#47626,0.0109676127131101);
#15180=CIRCLE('',#47627,0.0166825658003235);
#15181=CIRCLE('',#47628,0.0110194472769563);
#15182=CIRCLE('',#47629,0.0165701551403399);
#15183=CIRCLE('',#47631,0.0165732983967805);
#15184=CIRCLE('',#47632,0.0165701565626166);
#15185=CIRCLE('',#47633,0.0165732960775949);
#15186=CIRCLE('',#47634,0.0168141206266248);
#15187=CIRCLE('',#47635,0.0110535372955402);
#15188=CIRCLE('',#47636,0.0168028429610133);
#15189=CIRCLE('',#47637,0.0110635670199097);
#15190=CIRCLE('',#47638,0.0166019906551576);
#15191=CIRCLE('',#47640,0.0166008708466768);
#15192=CIRCLE('',#47641,0.0166019927018465);
#15193=CIRCLE('',#47642,0.0166008689412734);
#15194=CIRCLE('',#47643,0.016757184001705);
#15195=CIRCLE('',#47644,0.0110511996761176);
#15196=CIRCLE('',#47645,0.016790739109215);
#15197=CIRCLE('',#47646,0.011019098184434);
#15198=CIRCLE('',#47647,0.0066587480828286);
#15199=CIRCLE('',#47653,0.0167157066790089);
#15200=CIRCLE('',#47654,0.0109625450117604);
#15201=CIRCLE('',#47656,0.0165541457909729);
#15202=CIRCLE('',#47658,0.016557940910524);
#15203=CIRCLE('',#47659,0.0165541480837066);
#15204=CIRCLE('',#47660,0.0165579387559605);
#15205=CIRCLE('',#47661,0.0168110399839677);
#15206=CIRCLE('',#47662,0.0110459668065405);
#15207=CIRCLE('',#47663,0.0167928000131899);
#15208=CIRCLE('',#47664,0.0110624552729814);
#15209=CIRCLE('',#47667,0.0166052623997871);
#15210=CIRCLE('',#47669,0.0166047984590974);
#15211=CIRCLE('',#47670,0.0166052638884078);
#15212=CIRCLE('',#47671,0.0166047966615301);
#15213=CIRCLE('',#47672,0.0167731971561139);
#15214=CIRCLE('',#47673,0.0110573244858449);
#15215=CIRCLE('',#47674,0.0168013216993788);
#15216=CIRCLE('',#47675,0.0110316530767841);
#15217=CIRCLE('',#47676,0.0165310255307904);
#15218=CIRCLE('',#47678,0.0165263141351347);
#15219=CIRCLE('',#47679,0.0165310269859533);
#15220=CIRCLE('',#47680,0.0165263124289528);
#15221=CIRCLE('',#47681,0.0166775856839762);
#15222=CIRCLE('',#47682,0.0109205691225622);
#15223=CIRCLE('',#47684,0.0164211174216821);
#15224=CIRCLE('',#47685,0.0164211152287567);
#15225=CIRCLE('',#47686,0.0167388248049001);
#15226=CIRCLE('',#47687,0.0109676124289856);
#15227=CIRCLE('',#47688,0.0166825658005866);
#15228=CIRCLE('',#47689,0.0110194472755798);
#15229=CIRCLE('',#47690,0.0165701552119444);
#15230=CIRCLE('',#47692,0.0165732982632728);
#15231=CIRCLE('',#47693,0.016570156637561);
#15232=CIRCLE('',#47694,0.0165732960426156);
#15233=CIRCLE('',#47695,0.0168141205742218);
#15234=CIRCLE('',#47696,0.011053537412211);
#15235=CIRCLE('',#47697,0.0168028429618933);
#15236=CIRCLE('',#47698,0.0110635670201166);
#15237=CIRCLE('',#47699,0.0166019906886142);
#15238=CIRCLE('',#47701,0.0166008709183064);
#15239=CIRCLE('',#47702,0.0166019926437347);
#15240=CIRCLE('',#47703,0.0166008689366435);
#15241=CIRCLE('',#47704,0.0167571840014403);
#15242=CIRCLE('',#47705,0.0110512000530764);
#15243=CIRCLE('',#47706,0.0167907391089602);
#15244=CIRCLE('',#47707,0.0110190981855417);
#15245=CIRCLE('',#47708,0.00665874948987581);
#15246=CIRCLE('',#47714,0.0167157066787763);
#15247=CIRCLE('',#47715,0.0109625450161231);
#15248=CIRCLE('',#47717,0.0165541458013739);
#15249=CIRCLE('',#47719,0.0165579408335849);
#15250=CIRCLE('',#47720,0.0165541479190511);
#15251=CIRCLE('',#47721,0.0165579387335229);
#15252=CIRCLE('',#47722,0.0168110399839455);
#15253=CIRCLE('',#47723,0.0110459668054762);
#15254=CIRCLE('',#47724,0.0167928000127178);
#15255=CIRCLE('',#47725,0.0110624552735594);
#15256=CIRCLE('',#47728,0.0166052624219195);
#15257=CIRCLE('',#47730,0.0166047982868483);
#15258=CIRCLE('',#47731,0.0166052639548341);
#15259=CIRCLE('',#47732,0.0166047965522661);
#15260=CIRCLE('',#47733,0.0167731971567446);
#15261=CIRCLE('',#47734,0.0110573244853783);
#15262=CIRCLE('',#47735,0.0168013216992766);
#15263=CIRCLE('',#47736,0.0110316530731178);
#15264=CIRCLE('',#47737,0.0165310254682502);
#15265=CIRCLE('',#47739,0.0165263139662139);
#15266=CIRCLE('',#47740,0.0165310273029044);
#15267=CIRCLE('',#47741,0.0165263122502954);
#15268=CIRCLE('',#47742,0.0166775856841097);
#15269=CIRCLE('',#47743,0.0109205691214897);
#15270=CIRCLE('',#47745,0.0164211170610155);
#15271=CIRCLE('',#47746,0.0164211153185495);
#15272=CIRCLE('',#47747,0.0167388248045554);
#15273=CIRCLE('',#47748,0.0109676124278452);
#15274=CIRCLE('',#47749,0.0166825658004723);
#15275=CIRCLE('',#47750,0.0110194472759086);
#15276=CIRCLE('',#47751,0.0165701549486484);
#15277=CIRCLE('',#47753,0.0165732980341184);
#15278=CIRCLE('',#47754,0.0165701566511404);
#15279=CIRCLE('',#47755,0.0165732959899662);
#15280=CIRCLE('',#47756,0.0168141206453934);
#15281=CIRCLE('',#47757,0.0110535372533032);
#15282=CIRCLE('',#47758,0.0168028429606526);
#15283=CIRCLE('',#47759,0.0110635670195936);
#15284=CIRCLE('',#47760,0.0166019908025361);
#15285=CIRCLE('',#47762,0.0166008705740594);
#15286=CIRCLE('',#47763,0.0166019925677242);
#15287=CIRCLE('',#47764,0.0166008688871382);
#15288=CIRCLE('',#47765,0.0167571840018058);
#15289=CIRCLE('',#47766,0.0110512000569864);
#15290=CIRCLE('',#47767,0.0167907391092407);
#15291=CIRCLE('',#47768,0.0110190981863241);
#15292=CIRCLE('',#47769,0.00665874948993972);
#15293=CIRCLE('',#47775,0.0167157066786719);
#15294=CIRCLE('',#47776,0.0109625450160374);
#15295=CIRCLE('',#47778,0.0165541458229972);
#15296=CIRCLE('',#47780,0.0165579405587508);
#15297=CIRCLE('',#47781,0.0165541479749883);
#15298=CIRCLE('',#47782,0.0165579385078735);
#15299=CIRCLE('',#47783,0.0168110399838372);
#15300=CIRCLE('',#47784,0.0110459668048916);
#15301=CIRCLE('',#47785,0.0167928000129713);
#15302=CIRCLE('',#47786,0.0110624552756187);
#15303=CIRCLE('',#47789,0.0166052622979043);
#15304=CIRCLE('',#47791,0.0166047980078517);
#15305=CIRCLE('',#47792,0.0166052637458812);
#15306=CIRCLE('',#47793,0.016604796546177);
#15307=CIRCLE('',#47794,0.0167731971562877);
#15308=CIRCLE('',#47795,0.0110573244849338);
#15309=CIRCLE('',#47796,0.0168013216991658);
#15310=CIRCLE('',#47797,0.011031653076038);
#15311=CIRCLE('',#47798,0.0165310254980791);
#15312=CIRCLE('',#47800,0.016526313867048);
#15313=CIRCLE('',#47801,0.0165310270047356);
#15314=CIRCLE('',#47802,0.0165263124988837);
#15315=CIRCLE('',#47803,0.0166775856851045);
#15316=CIRCLE('',#47804,0.01092056912089);
#15317=CIRCLE('',#47806,0.0164211169494706);
#15318=CIRCLE('',#47807,0.0164211152668151);
#15319=CIRCLE('',#47808,0.0167388248044777);
#15320=CIRCLE('',#47809,0.0109676124279146);
#15321=CIRCLE('',#47810,0.016682565800564);
#15322=CIRCLE('',#47811,0.0110194472766535);
#15323=CIRCLE('',#47812,0.0165701548917864);
#15324=CIRCLE('',#47814,0.0165732978045151);
#15325=CIRCLE('',#47815,0.0165701564472872);
#15326=CIRCLE('',#47816,0.0165732957486762);
#15327=CIRCLE('',#47817,0.0168141206453714);
#15328=CIRCLE('',#47818,0.0110535372567067);
#15329=CIRCLE('',#47819,0.0168028429617165);
#15330=CIRCLE('',#47820,0.0110635670195438);
#15331=CIRCLE('',#47821,0.0166019906461126);
#15332=CIRCLE('',#47823,0.0166008704437203);
#15333=CIRCLE('',#47824,0.0166019927691166);
#15334=CIRCLE('',#47825,0.016600868870716);
#15335=CIRCLE('',#47826,0.0167571840013951);
#15336=CIRCLE('',#47827,0.0110511996790365);
#15337=CIRCLE('',#47828,0.016790739108159);
#15338=CIRCLE('',#47829,0.0110190981859346);
#15339=CIRCLE('',#47830,0.00665874807865914);
#15340=CIRCLE('',#47836,0.0167157066790517);
#15341=CIRCLE('',#47837,0.0109625450109347);
#15342=CIRCLE('',#47839,0.0165541458621187);
#15343=CIRCLE('',#47841,0.0165579404282209);
#15344=CIRCLE('',#47842,0.0165541478979011);
#15345=CIRCLE('',#47843,0.016557938488688);
#15346=CIRCLE('',#47844,0.01681103998369);
#15347=CIRCLE('',#47845,0.0110459668054687);
#15348=CIRCLE('',#47846,0.0167928000124603);
#15349=CIRCLE('',#47847,0.0110624552742697);
#15350=CIRCLE('',#47850,0.0166052623411055);
#15351=CIRCLE('',#47852,0.0166047979258038);
#15352=CIRCLE('',#47853,0.0166052638195381);
#15353=CIRCLE('',#47854,0.016604796415447);
#15354=CIRCLE('',#47855,0.016773197156601);
#15355=CIRCLE('',#47856,0.0110573244864894);
#15356=CIRCLE('',#47857,0.0168013216997676);
#15357=CIRCLE('',#47858,0.0110316530752986);
#15358=CIRCLE('',#47859,0.0165310253501258);
#15359=CIRCLE('',#47861,0.0165263137831181);
#15360=CIRCLE('',#47862,0.0165310270138886);
#15361=CIRCLE('',#47863,0.0165263123403775);
#15362=CIRCLE('',#47864,0.0166775856843488);
#15363=CIRCLE('',#47865,0.0109205691222831);
#15364=CIRCLE('',#47867,0.0164211168538974);
#15365=CIRCLE('',#47868,0.0164211151504863);
#15366=CIRCLE('',#47869,0.0167388235417016);
#15367=CIRCLE('',#47870,0.0109676133178113);
#15368=CIRCLE('',#47871,0.0166825658009599);
#15369=CIRCLE('',#47872,0.0110194472770996);
#15370=CIRCLE('',#47873,0.0165701548115593);
#15371=CIRCLE('',#47875,0.01657329760585);
#15372=CIRCLE('',#47876,0.016570156674166);
#15373=CIRCLE('',#47877,0.0165732958903677);
#15374=CIRCLE('',#47878,0.0168141206461625);
#15375=CIRCLE('',#47879,0.0110535372541906);
#15376=CIRCLE('',#47880,0.0168028429615073);
#15377=CIRCLE('',#47881,0.0110635670195637);
#15378=CIRCLE('',#47882,0.0166019906026257);
#15379=CIRCLE('',#47884,0.0166008702318525);
#15380=CIRCLE('',#47885,0.0166019925762392);
#15381=CIRCLE('',#47886,0.0166008685776365);
#15382=CIRCLE('',#47887,0.0167571840015236);
#15383=CIRCLE('',#47888,0.0110511996751507);
#15384=CIRCLE('',#47889,0.0167907391088176);
#15385=CIRCLE('',#47890,0.0110190981854031);
#15386=CIRCLE('',#47891,0.00665874807872873);
#15387=CIRCLE('',#47897,0.0167157066787157);
#15388=CIRCLE('',#47898,0.0109625450142858);
#15389=CIRCLE('',#47900,0.0165541457909352);
#15390=CIRCLE('',#47902,0.0165579402781184);
#15391=CIRCLE('',#47903,0.0165541477545415);
#15392=CIRCLE('',#47904,0.016557938424068);
#15393=CIRCLE('',#47905,0.0168110399836047);
#15394=CIRCLE('',#47906,0.0110459668051156);
#15395=CIRCLE('',#47907,0.0167928000128988);
#15396=CIRCLE('',#47908,0.0110624552738703);
#15397=CIRCLE('',#47911,0.0166052624109867);
#15398=CIRCLE('',#47913,0.0166047977841876);
#15399=CIRCLE('',#47914,0.0166052636354893);
#15400=CIRCLE('',#47915,0.0166047962325927);
#15401=CIRCLE('',#47916,0.0167731971560594);
#15402=CIRCLE('',#47917,0.0110573244858153);
#15403=CIRCLE('',#47918,0.0168013216994829);
#15404=CIRCLE('',#47919,0.0110316530742135);
#15405=CIRCLE('',#47920,0.0165310254867642);
#15406=CIRCLE('',#47922,0.0165263134594726);
#15407=CIRCLE('',#47923,0.0165310267542607);
#15408=CIRCLE('',#47924,0.0165263119891698);
#15409=CIRCLE('',#47925,0.0166775856848237);
#15410=CIRCLE('',#47926,0.0109205691213332);
#15411=CIRCLE('',#47928,0.0164211167562658);
#15412=CIRCLE('',#47929,0.0164211150069546);
#15413=CIRCLE('',#47930,0.0167388248040529);
#15414=CIRCLE('',#47931,0.0109676124294812);
#15415=CIRCLE('',#47932,0.0166825658009133);
#15416=CIRCLE('',#47933,0.0110194472761536);
#15417=CIRCLE('',#47934,0.0165701548909676);
#15418=CIRCLE('',#47936,0.0165732976153206);
#15419=CIRCLE('',#47937,0.0165701563546957);
#15420=CIRCLE('',#47938,0.0165732959810528);
#15421=CIRCLE('',#47939,0.0168141206457686);
#15422=CIRCLE('',#47940,0.0110535372541688);
#15423=CIRCLE('',#47941,0.0168028429613712);
#15424=CIRCLE('',#47942,0.011063567020347);
#15425=CIRCLE('',#47943,0.0166019905963711);
#15426=CIRCLE('',#47945,0.0166008702286165);
#15427=CIRCLE('',#47946,0.016601992541578);
#15428=CIRCLE('',#47947,0.0166008686459998);
#15429=CIRCLE('',#47948,0.016757184001533);
#15430=CIRCLE('',#47949,0.0110511996795091);
#15431=CIRCLE('',#47950,0.016790739108611);
#15432=CIRCLE('',#47951,0.0110190981835215);
#15433=CIRCLE('',#47952,0.00665874807857607);
#15434=CIRCLE('',#47958,0.0167157066788821);
#15435=CIRCLE('',#47959,0.0109625450166771);
#15436=CIRCLE('',#47961,0.0165541458400344);
#15437=CIRCLE('',#47963,0.0165579399865424);
#15438=CIRCLE('',#47964,0.0165541474848087);
#15439=CIRCLE('',#47965,0.0165579382754252);
#15440=CIRCLE('',#47966,0.0168110399835032);
#15441=CIRCLE('',#47967,0.0110459668042796);
#15442=CIRCLE('',#47968,0.0167928000129298);
#15443=CIRCLE('',#47969,0.0110624552747411);
#15444=CIRCLE('',#47972,0.0166052624204165);
#15445=CIRCLE('',#47974,0.0166047975298572);
#15446=CIRCLE('',#47975,0.0166052635696027);
#15447=CIRCLE('',#47976,0.0166047961541093);
#15448=CIRCLE('',#47977,0.0167731941320965);
#15449=CIRCLE('',#47978,0.0110573150844861);
#15450=CIRCLE('',#47979,0.0168013216988545);
#15451=CIRCLE('',#47980,0.0110316530737055);
#15452=CIRCLE('',#47981,0.01653102561324);
#15453=CIRCLE('',#47983,0.0165263134535438);
#15454=CIRCLE('',#47984,0.0165310266894553);
#15455=CIRCLE('',#47985,0.0165263119606172);
#15456=CIRCLE('',#47986,0.016677585684666);
#15457=CIRCLE('',#47987,0.0109205691211641);
#15458=CIRCLE('',#47989,0.0164211164846049);
#15459=CIRCLE('',#47990,0.0164211149742223);
#15460=CIRCLE('',#47991,0.0167388248041252);
#15461=CIRCLE('',#47992,0.0109676124298911);
#15462=CIRCLE('',#47993,0.0166825658006233);
#15463=CIRCLE('',#47994,0.0110194472786196);
#15464=CIRCLE('',#47995,0.016570155027543);
#15465=CIRCLE('',#47997,0.0165732973038302);
#15466=CIRCLE('',#47998,0.0165701565528539);
#15467=CIRCLE('',#47999,0.0165732957936516);
#15468=CIRCLE('',#48000,0.0168141205743096);
#15469=CIRCLE('',#48001,0.0110535374095543);
#15470=CIRCLE('',#48002,0.0168028429616262);
#15471=CIRCLE('',#48003,0.0110635670192313);
#15472=CIRCLE('',#48004,0.0166019907953388);
#15473=CIRCLE('',#48006,0.0166008699165455);
#15474=CIRCLE('',#48007,0.0166019924266547);
#15475=CIRCLE('',#48008,0.0166008685549454);
#15476=CIRCLE('',#48009,0.0167571840015528);
#15477=CIRCLE('',#48010,0.0110511996804726);
#15478=CIRCLE('',#48011,0.0167907391088268);
#15479=CIRCLE('',#48012,0.0110190981846686);
#15480=CIRCLE('',#48013,0.00665874807857608);
#15481=CIRCLE('',#48019,0.0167157066791692);
#15482=CIRCLE('',#48020,0.0109625450124005);
#15483=CIRCLE('',#48022,0.0165541458563792);
#15484=CIRCLE('',#48024,0.0165579398708296);
#15485=CIRCLE('',#48025,0.016554147259951);
#15486=CIRCLE('',#48026,0.0165579381717781);
#15487=CIRCLE('',#48027,0.0168110399835602);
#15488=CIRCLE('',#48028,0.0110459668058413);
#15489=CIRCLE('',#48029,0.0167928000130561);
#15490=CIRCLE('',#48030,0.0110624552745106);
#15491=CIRCLE('',#48033,0.0166052621606994);
#15492=CIRCLE('',#48035,0.0166047975523418);
#15493=CIRCLE('',#48036,0.0166052634410576);
#15494=CIRCLE('',#48037,0.0166047961237714);
#15495=CIRCLE('',#48038,0.0167731971564195);
#15496=CIRCLE('',#48039,0.0110573244853963);
#15497=CIRCLE('',#48040,0.0168013216996777);
#15498=CIRCLE('',#48041,0.0110316530737103);
#15499=CIRCLE('',#48042,0.0165310255839058);
#15500=CIRCLE('',#48044,0.0165263131899507);
#15501=CIRCLE('',#48045,0.0165310267138344);
#15502=CIRCLE('',#48046,0.0165263117828695);
#15503=CIRCLE('',#48047,0.0166775856839844);
#15504=CIRCLE('',#48048,0.010920569122766);
#15505=CIRCLE('',#48050,0.0164211163471286);
#15506=CIRCLE('',#48051,0.0164211148702252);
#15507=CIRCLE('',#48052,0.0167388248043213);
#15508=CIRCLE('',#48053,0.010967612427291);
#15509=CIRCLE('',#48054,0.0166825658003235);
#15510=CIRCLE('',#48055,0.0110194472750709);
#15511=CIRCLE('',#48056,0.0165701549840473);
#15512=CIRCLE('',#48058,0.0165732971979771);
#15513=CIRCLE('',#48059,0.0165701563441456);
#15514=CIRCLE('',#48060,0.016573295686663);
#15515=CIRCLE('',#48061,0.0168141206459555);
#15516=CIRCLE('',#48062,0.01105353725616);
#15517=CIRCLE('',#48063,0.0168028429614426);
#15518=CIRCLE('',#48064,0.0110635670200517);
#15519=CIRCLE('',#48065,0.0166019908585466);
#15520=CIRCLE('',#48067,0.0166008697863184);
#15521=CIRCLE('',#48068,0.0166019923320812);
#15522=CIRCLE('',#48069,0.0166008684816235);
#15523=CIRCLE('',#48070,0.0167571840014785);
#15524=CIRCLE('',#48071,0.0110511996761483);
#15525=CIRCLE('',#48072,0.0167907391088928);
#15526=CIRCLE('',#48073,0.0110190981840285);
#15527=CIRCLE('',#48074,0.00665874807855417);
#15528=CIRCLE('',#48080,0.0167157066790624);
#15529=CIRCLE('',#48081,0.0109625450150895);
#15530=CIRCLE('',#48083,0.0165541458221566);
#15531=CIRCLE('',#48085,0.0165579397651312);
#15532=CIRCLE('',#48086,0.0165541473401467);
#15533=CIRCLE('',#48087,0.0165579381811266);
#15534=CIRCLE('',#48088,0.016811039983551);
#15535=CIRCLE('',#48089,0.0110459668053132);
#15536=CIRCLE('',#48090,0.0167928000130745);
#15537=CIRCLE('',#48091,0.0110624552748131);
#15538=CIRCLE('',#48094,0.016605262299557);
#15539=CIRCLE('',#48096,0.0166047972767696);
#15540=CIRCLE('',#48097,0.016605263291903);
#15541=CIRCLE('',#48098,0.01660479606158);
#15542=CIRCLE('',#48099,0.0167731971567289);
#15543=CIRCLE('',#48100,0.0110573244852766);
#15544=CIRCLE('',#48101,0.0168013216995077);
#15545=CIRCLE('',#48102,0.0110316530736745);
#15546=CIRCLE('',#48103,0.0165310253844543);
#15547=CIRCLE('',#48105,0.0165263132517026);
#15548=CIRCLE('',#48106,0.0165310266599294);
#15549=CIRCLE('',#48107,0.01652631182441);
#15550=CIRCLE('',#48108,0.0166775856846773);
#15551=CIRCLE('',#48109,0.0109205691231875);
#15552=CIRCLE('',#48111,0.0164211161921942);
#15553=CIRCLE('',#48112,0.0164211148656089);
#15554=CIRCLE('',#48113,0.0167388248043935);
#15555=CIRCLE('',#48114,0.0109676124288808);
#15556=CIRCLE('',#48115,0.016682565800743);
#15557=CIRCLE('',#48116,0.0110194472768691);
#15558=CIRCLE('',#48117,0.0165701549825662);
#15559=CIRCLE('',#48119,0.0165732970168302);
#15560=CIRCLE('',#48120,0.016570156277062);
#15561=CIRCLE('',#48121,0.0165732954740135);
#15562=CIRCLE('',#48122,0.0168141205745554);
#15563=CIRCLE('',#48123,0.0110535374087421);
#15564=CIRCLE('',#48124,0.0168028429610667);
#15565=CIRCLE('',#48125,0.0110635670195058);
#15566=CIRCLE('',#48126,0.0166019907129225);
#15567=CIRCLE('',#48128,0.0166008698804845);
#15568=CIRCLE('',#48129,0.016601992082684);
#15569=CIRCLE('',#48130,0.0166008685783328);
#15570=CIRCLE('',#48131,0.0167571840014611);
#15571=CIRCLE('',#48132,0.0110511996805999);
#15572=CIRCLE('',#48133,0.0167907391091645);
#15573=CIRCLE('',#48134,0.0110190981845518);
#15574=CIRCLE('',#48135,0.00665874808267189);
#15575=CIRCLE('',#48141,0.016715706678982);
#15576=CIRCLE('',#48142,0.0109625450123671);
#15577=CIRCLE('',#48144,0.0165541458429362);
#15578=CIRCLE('',#48146,0.0165579396121371);
#15579=CIRCLE('',#48147,0.0165541473073873);
#15580=CIRCLE('',#48148,0.0165579381287537);
#15581=CIRCLE('',#48149,0.0168110399837888);
#15582=CIRCLE('',#48150,0.0110459668050407);
#15583=CIRCLE('',#48151,0.0167928000131913);
#15584=CIRCLE('',#48152,0.0110624552739991);
#15585=CIRCLE('',#48155,0.0166052623178069);
#15586=CIRCLE('',#48157,0.0166047971419355);
#15587=CIRCLE('',#48158,0.0166052632661251);
#15588=CIRCLE('',#48159,0.0166047959270355);
#15589=CIRCLE('',#48160,0.0167731971565613);
#15590=CIRCLE('',#48161,0.0110573244865064);
#15591=CIRCLE('',#48162,0.0168013216995224);
#15592=CIRCLE('',#48163,0.0110316530744794);
#15593=CIRCLE('',#48164,0.0165310255747975);
#15594=CIRCLE('',#48166,0.0165263129036402);
#15595=CIRCLE('',#48167,0.0165310265276423);
#15596=CIRCLE('',#48168,0.0165263117199402);
#15597=CIRCLE('',#48169,0.0166775856847219);
#15598=CIRCLE('',#48170,0.010920569121723);
#15599=CIRCLE('',#48172,0.016421116098934);
#15600=CIRCLE('',#48173,0.0164211148099697);
#15601=CIRCLE('',#48174,0.0167388248042058);
#15602=CIRCLE('',#48175,0.0109676124285651);
#15603=CIRCLE('',#48176,0.0166825658005706);
#15604=CIRCLE('',#48177,0.0110194472756133);
#15605=CIRCLE('',#48178,0.0165701550852875);
#15606=CIRCLE('',#48180,0.0165732968920231);
#15607=CIRCLE('',#48181,0.0165701561472083);
#15608=CIRCLE('',#48182,0.0165732954569517);
#15609=CIRCLE('',#48183,0.0168141206459413);
#15610=CIRCLE('',#48184,0.0110535372534566);
#15611=CIRCLE('',#48185,0.0168028429612771);
#15612=CIRCLE('',#48186,0.0110635670198656);
#15613=CIRCLE('',#48187,0.0166019908312719);
#15614=CIRCLE('',#48189,0.0166008696419111);
#15615=CIRCLE('',#48190,0.0166019921364906);
#15616=CIRCLE('',#48191,0.0166008683378502);
#15617=CIRCLE('',#48192,0.0167571840016696);
#15618=CIRCLE('',#48193,0.0110511996786392);
#15619=CIRCLE('',#48194,0.0167907391087163);
#15620=CIRCLE('',#48195,0.0110190981851326);
#15621=CIRCLE('',#48196,0.00665874807863192);
#15622=CIRCLE('',#48202,0.0167157066786652);
#15623=CIRCLE('',#48203,0.01096254501372);
#15624=CIRCLE('',#48205,0.0165541458428756);
#15625=CIRCLE('',#48207,0.0165579395212262);
#15626=CIRCLE('',#48208,0.0165541472262184);
#15627=CIRCLE('',#48209,0.0165579380173231);
#15628=CIRCLE('',#48210,0.0168110399836305);
#15629=CIRCLE('',#48211,0.0110459668053802);
#15630=CIRCLE('',#48212,0.0167928000132902);
#15631=CIRCLE('',#48213,0.0110624552750508);
#15632=CIRCLE('',#48216,0.0166052622985171);
#15633=CIRCLE('',#48218,0.0166047969953593);
#15634=CIRCLE('',#48219,0.0166052632596361);
#15635=CIRCLE('',#48220,0.0166047958844994);
#15636=CIRCLE('',#48221,0.0167731971564568);
#15637=CIRCLE('',#48222,0.0110573244851529);
#15638=CIRCLE('',#48223,0.0168013216996);
#15639=CIRCLE('',#48224,0.0110316530734903);
#15640=CIRCLE('',#48225,0.016531025524901);
#15641=CIRCLE('',#48227,0.0165263128517349);
#15642=CIRCLE('',#48228,0.0165310265016073);
#15643=CIRCLE('',#48229,0.0165263115872939);
#15644=CIRCLE('',#48230,0.0166775856845724);
#15645=CIRCLE('',#48231,0.0109205691219406);
#15646=CIRCLE('',#48233,0.0164211159073852);
#15647=CIRCLE('',#48234,0.0164211147625774);
#15648=CIRCLE('',#48235,0.0167388235417366);
#15649=CIRCLE('',#48236,0.0109676133178607);
#15650=CIRCLE('',#48237,0.0166825658004808);
#15651=CIRCLE('',#48238,0.0110194472764579);
#15652=CIRCLE('',#48239,0.0165701550086192);
#15653=CIRCLE('',#48241,0.0165732968106716);
#15654=CIRCLE('',#48242,0.0165701560854755);
#15655=CIRCLE('',#48243,0.0165732953410207);
#15656=CIRCLE('',#48244,0.0168141206272819);
#15657=CIRCLE('',#48245,0.0110535372938326);
#15658=CIRCLE('',#48246,0.0168028429616766);
#15659=CIRCLE('',#48247,0.0110635670196207);
#15660=CIRCLE('',#48248,0.0166019908311988);
#15661=CIRCLE('',#48250,0.016600869402183);
#15662=CIRCLE('',#48251,0.0166019920672427);
#15663=CIRCLE('',#48252,0.0166008681241324);
#15664=CIRCLE('',#48253,0.0167577810054763);
#15665=CIRCLE('',#48254,0.011051199676122);
#15666=CIRCLE('',#48255,0.0167907391087387);
#15667=CIRCLE('',#48256,0.0110190981854095);
#15668=CIRCLE('',#48257,0.00665874808266081);
#15669=CIRCLE('',#48263,0.0167157066785781);
#15670=CIRCLE('',#48264,0.0109625450129892);
#15671=CIRCLE('',#48266,0.0165541458625202);
#15672=CIRCLE('',#48268,0.0165579392760386);
#15673=CIRCLE('',#48269,0.0165541470496618);
#15674=CIRCLE('',#48270,0.0165579379144359);
#15675=CIRCLE('',#48271,0.0168110399834894);
#15676=CIRCLE('',#48272,0.0110459668055838);
#15677=CIRCLE('',#48273,0.0167928000130272);
#15678=CIRCLE('',#48274,0.0110624552745341);
#15679=CIRCLE('',#48277,0.0166052622900365);
#15680=CIRCLE('',#48279,0.016604796869262);
#15681=CIRCLE('',#48280,0.0166052631782005);
#15682=CIRCLE('',#48281,0.0166047958522747);
#15683=CIRCLE('',#48282,0.0167731971564835);
#15684=CIRCLE('',#48283,0.011057324485878);
#15685=CIRCLE('',#48284,0.0168013216995648);
#15686=CIRCLE('',#48285,0.0110316530741046);
#15687=CIRCLE('',#48286,0.0165310254682413);
#15688=CIRCLE('',#48288,0.0165263126814153);
#15689=CIRCLE('',#48289,0.0165310264424974);
#15690=CIRCLE('',#48290,0.0165263115926201);
#15691=CIRCLE('',#48291,0.0166775856846586);
#15692=CIRCLE('',#48292,0.0109205691217816);
#15693=CIRCLE('',#48294,0.0164211156962373);
#15694=CIRCLE('',#48295,0.0164211145902099);
#15695=CIRCLE('',#48296,0.0167388248044593);
#15696=CIRCLE('',#48297,0.0109676124272191);
#15697=CIRCLE('',#48298,0.0166825658002918);
#15698=CIRCLE('',#48299,0.0110194472756495);
#15699=CIRCLE('',#48300,0.0165701549805964);
#15700=CIRCLE('',#48302,0.0165732964757245);
#15701=CIRCLE('',#48303,0.016570155993251);
#15702=CIRCLE('',#48304,0.0165732952076342);
#15703=CIRCLE('',#48305,0.0168141206270738);
#15704=CIRCLE('',#48306,0.0110535372948799);
#15705=CIRCLE('',#48307,0.0168028429613149);
#15706=CIRCLE('',#48308,0.0110635670197968);
#15707=CIRCLE('',#48309,0.0166019907856206);
#15708=CIRCLE('',#48311,0.016600869281246);
#15709=CIRCLE('',#48312,0.0166019919750651);
#15710=CIRCLE('',#48313,0.0166008681437444);
#15711=CIRCLE('',#48314,0.0167571840016302);
#15712=CIRCLE('',#48315,0.0110511996784197);
#15713=CIRCLE('',#48316,0.0167907391087342);
#15714=CIRCLE('',#48317,0.0110190981852672);
#15715=CIRCLE('',#48318,0.00665874807857735);
#15716=CIRCLE('',#48324,0.0167157066788082);
#15717=CIRCLE('',#48325,0.0109625450139715);
#15718=CIRCLE('',#48327,0.0165541457528717);
#15719=CIRCLE('',#48329,0.0165579391310576);
#15720=CIRCLE('',#48330,0.0165541470455079);
#15721=CIRCLE('',#48331,0.0165579378864428);
#15722=CIRCLE('',#48332,0.0168110399835194);
#15723=CIRCLE('',#48333,0.0110459668048852);
#15724=CIRCLE('',#48334,0.0167928000131374);
#15725=CIRCLE('',#48335,0.0110624552741263);
#15726=CIRCLE('',#48338,0.0166052623235493);
#15727=CIRCLE('',#48340,0.0166047966343837);
#15728=CIRCLE('',#48341,0.0166052630637473);
#15729=CIRCLE('',#48342,0.0166047956728293);
#15730=CIRCLE('',#48343,0.016773198350099);
#15731=CIRCLE('',#48344,0.0110573281946764);
#15732=CIRCLE('',#48345,0.0168013216995328);
#15733=CIRCLE('',#48346,0.0110316530739007);
#15734=CIRCLE('',#48347,0.0165310254915807);
#15735=CIRCLE('',#48349,0.0165263125359947);
#15736=CIRCLE('',#48350,0.0165310263328488);
#15737=CIRCLE('',#48351,0.0165263115654509);
#15738=CIRCLE('',#48352,0.0166775856846347);
#15739=CIRCLE('',#48353,0.0109205691218874);
#15740=CIRCLE('',#48355,0.0164211155053557);
#15741=CIRCLE('',#48356,0.0164211145217507);
#15742=CIRCLE('',#48357,0.0167388244017953);
#15743=CIRCLE('',#48358,0.0109676127120334);
#15744=CIRCLE('',#48359,0.0166825658004791);
#15745=CIRCLE('',#48360,0.0110194472762198);
#15746=CIRCLE('',#48361,0.0165701550928783);
#15747=CIRCLE('',#48363,0.0165732963879411);
#15748=CIRCLE('',#48364,0.0165701559310954);
#15749=CIRCLE('',#48365,0.016573295223886);
#15750=CIRCLE('',#48366,0.0168141206271986);
#15751=CIRCLE('',#48367,0.0110535372945764);
#15752=CIRCLE('',#48368,0.0168028429614001);
#15753=CIRCLE('',#48369,0.0110635670197259);
#15754=CIRCLE('',#48370,0.0166019908106737);
#15755=CIRCLE('',#48372,0.016600869078043);
#15756=CIRCLE('',#48373,0.0166019918428707);
#15757=CIRCLE('',#48374,0.016600868010713);
#15758=CIRCLE('',#48375,0.0167571840015784);
#15759=CIRCLE('',#48376,0.0110511996800335);
#15760=CIRCLE('',#48377,0.016790739109042);
#15761=CIRCLE('',#48378,0.0110190981854062);
#15762=CIRCLE('',#48379,0.00665874808278241);
#15763=CIRCLE('',#48385,0.0167157066788378);
#15764=CIRCLE('',#48386,0.0109625450137759);
#15765=CIRCLE('',#48388,0.016554145781167);
#15766=CIRCLE('',#48390,0.0165579390814041);
#15767=CIRCLE('',#48391,0.016554146981822);
#15768=CIRCLE('',#48392,0.0165579378221229);
#15769=CIRCLE('',#48393,0.016811039983634);
#15770=CIRCLE('',#48394,0.0110459668055729);
#15771=CIRCLE('',#48395,0.0167928000132035);
#15772=CIRCLE('',#48396,0.0110624552743364);
#15773=CIRCLE('',#48399,0.0166052621326915);
#15774=CIRCLE('',#48401,0.0166047965546541);
#15775=CIRCLE('',#48402,0.0166052629654533);
#15776=CIRCLE('',#48403,0.0166047956448385);
#15777=CIRCLE('',#48404,0.0167731971564053);
#15778=CIRCLE('',#48405,0.0110573244857942);
#15779=CIRCLE('',#48406,0.0168013216995398);
#15780=CIRCLE('',#48407,0.0110316530743371);
#15781=CIRCLE('',#48408,0.0165310254751661);
#15782=CIRCLE('',#48410,0.016526312332431);
#15783=CIRCLE('',#48411,0.0165310263076625);
#15784=CIRCLE('',#48412,0.016526311446041);
#15785=CIRCLE('',#48413,0.0166775856843973);
#15786=CIRCLE('',#48414,0.0109205691218644);
#15787=CIRCLE('',#48416,0.0164211154121946);
#15788=CIRCLE('',#48417,0.016421114517602);
#15789=CIRCLE('',#48418,0.0167388248043828);
#15790=CIRCLE('',#48419,0.0109676124297309);
#15791=CIRCLE('',#48420,0.0166825658004906);
#15792=CIRCLE('',#48421,0.0110194472759386);
#15793=CIRCLE('',#48422,0.0165701549459977);
#15794=CIRCLE('',#48424,0.0165732962478553);
#15795=CIRCLE('',#48425,0.0165701557827074);
#15796=CIRCLE('',#48426,0.0165732950593365);
#15797=CIRCLE('',#48427,0.0168141206459375);
#15798=CIRCLE('',#48428,0.0110535372538286);
#15799=CIRCLE('',#48429,0.0168028429614107);
#15800=CIRCLE('',#48430,0.0110635670204726);
#15801=CIRCLE('',#48431,0.0166019907581878);
#15802=CIRCLE('',#48433,0.0166008689277773);
#15803=CIRCLE('',#48434,0.0166019917505441);
#15804=CIRCLE('',#48435,0.0166008679730606);
#15805=CIRCLE('',#48436,0.0167571840016015);
#15806=CIRCLE('',#48437,0.0110511996782994);
#15807=CIRCLE('',#48438,0.0167907391087864);
#15808=CIRCLE('',#48439,0.0110190981847917);
#15809=CIRCLE('',#48440,0.00665874807856375);
#15810=CIRCLE('',#48446,0.0167157066788102);
#15811=CIRCLE('',#48447,0.0109625450123883);
#15812=CIRCLE('',#48449,0.0165541457930371);
#15813=CIRCLE('',#48451,0.0165579390065225);
#15814=CIRCLE('',#48452,0.0165541470235924);
#15815=CIRCLE('',#48453,0.0165579377120552);
#15816=CIRCLE('',#48454,0.0168110399836019);
#15817=CIRCLE('',#48455,0.0110459668046012);
#15818=CIRCLE('',#48456,0.0167928000133165);
#15819=CIRCLE('',#48457,0.0110624552745342);
#15820=CIRCLE('',#48460,0.0166052623962907);
#15821=CIRCLE('',#48462,0.0166047964871083);
#15822=CIRCLE('',#48463,0.0166052630584548);
#15823=CIRCLE('',#48464,0.0166047955723545);
#15824=CIRCLE('',#48465,0.0167731971564806);
#15825=CIRCLE('',#48466,0.011057324486099);
#15826=CIRCLE('',#48467,0.0168013216996322);
#15827=CIRCLE('',#48468,0.0110316530750212);
#15828=CIRCLE('',#48469,0.0165310254445976);
#15829=CIRCLE('',#48471,0.0165263122162804);
#15830=CIRCLE('',#48472,0.0165310261855289);
#15831=CIRCLE('',#48473,0.0165263113676245);
#15832=CIRCLE('',#48474,0.0166775856844551);
#15833=CIRCLE('',#48475,0.0109205691223334);
#15834=CIRCLE('',#48477,0.0164211151716581);
#15835=CIRCLE('',#48478,0.0164211143291737);
#15836=CIRCLE('',#48479,0.0167388248041972);
#15837=CIRCLE('',#48480,0.0109676124278026);
#15838=CIRCLE('',#48481,0.0166825658002287);
#15839=CIRCLE('',#48482,0.0110194472760281);
#15840=CIRCLE('',#48483,0.0165701549962637);
#15841=CIRCLE('',#48485,0.0165732961308722);
#15842=CIRCLE('',#48486,0.0165701557733917);
#15843=CIRCLE('',#48487,0.016573294988113);
#15844=CIRCLE('',#48488,0.0168141206457764);
#15845=CIRCLE('',#48489,0.0110535372558345);
#15846=CIRCLE('',#48490,0.0168028429614474);
#15847=CIRCLE('',#48491,0.0110635670202249);
#15848=CIRCLE('',#48492,0.0166019907868911);
#15849=CIRCLE('',#48494,0.0166008687725664);
#15850=CIRCLE('',#48495,0.0166019916684501);
#15851=CIRCLE('',#48496,0.0166008679137632);
#15852=CIRCLE('',#48497,0.016757184001683);
#15853=CIRCLE('',#48498,0.0110512000569263);
#15854=CIRCLE('',#48499,0.016790739108977);
#15855=CIRCLE('',#48500,0.0110190981844742);
#15856=CIRCLE('',#48501,0.00665874948999836);
#15857=CIRCLE('',#48507,0.0167157066788402);
#15858=CIRCLE('',#48508,0.0109625450147756);
#15859=CIRCLE('',#48510,0.016554145772189);
#15860=CIRCLE('',#48512,0.0165579387522727);
#15861=CIRCLE('',#48513,0.016554146838596);
#15862=CIRCLE('',#48514,0.0165579376418337);
#15863=CIRCLE('',#48515,0.016811039983612);
#15864=CIRCLE('',#48516,0.0110459668047955);
#15865=CIRCLE('',#48517,0.0167928000134311);
#15866=CIRCLE('',#48518,0.0110624552743749);
#15867=CIRCLE('',#48521,0.0166052623598551);
#15868=CIRCLE('',#48523,0.0166047964320598);
#15869=CIRCLE('',#48524,0.0166052629385756);
#15870=CIRCLE('',#48525,0.0166047955511812);
#15871=CIRCLE('',#48526,0.0167731971563387);
#15872=CIRCLE('',#48527,0.011057324484739);
#15873=CIRCLE('',#48528,0.0168013216997687);
#15874=CIRCLE('',#48529,0.0110316530744769);
#15875=CIRCLE('',#48530,0.0165310254871738);
#15876=CIRCLE('',#48532,0.0165263120948897);
#15877=CIRCLE('',#48533,0.0165310260521502);
#15878=CIRCLE('',#48534,0.016526311314141);
#15879=CIRCLE('',#48535,0.0166775856846251);
#15880=CIRCLE('',#48536,0.0109205691213651);
#15881=CIRCLE('',#48538,0.0164211151214994);
#15882=CIRCLE('',#48539,0.0164211142044887);
#15883=CIRCLE('',#48540,0.0167388248042407);
#15884=CIRCLE('',#48541,0.0109676124279531);
#15885=CIRCLE('',#48542,0.0166825658003064);
#15886=CIRCLE('',#48543,0.0110194472762773);
#15887=CIRCLE('',#48544,0.0165701549300338);
#15888=CIRCLE('',#48546,0.01657329596834);
#15889=CIRCLE('',#48547,0.0165701556722587);
#15890=CIRCLE('',#48548,0.0165732949097595);
#15891=CIRCLE('',#48549,0.0168141206458614);
#15892=CIRCLE('',#48550,0.0110535372562175);
#15893=CIRCLE('',#48551,0.0168028429609649);
#15894=CIRCLE('',#48552,0.0110635670204018);
#15895=CIRCLE('',#48553,0.0166019907899111);
#15896=CIRCLE('',#48555,0.0166008687324912);
#15897=CIRCLE('',#48556,0.0166019915912748);
#15898=CIRCLE('',#48557,0.0166008678302651);
#15899=CIRCLE('',#48558,0.0167571840016815);
#15900=CIRCLE('',#48559,0.0110511996755867);
#15901=CIRCLE('',#48560,0.0167907391091693);
#15902=CIRCLE('',#48561,0.0110190981847612);
#15903=CIRCLE('',#48562,0.00665874808285124);
#15904=CIRCLE('',#48568,0.0167157066788687);
#15905=CIRCLE('',#48569,0.0109625450105235);
#15906=CIRCLE('',#48571,0.0165541458689486);
#15907=CIRCLE('',#48573,0.0165579387376058);
#15908=CIRCLE('',#48574,0.016554146790368);
#15909=CIRCLE('',#48575,0.0165579377385169);
#15910=CIRCLE('',#48576,0.0168110399836123);
#15911=CIRCLE('',#48577,0.0110459668052381);
#15912=CIRCLE('',#48578,0.0167928000134394);
#15913=CIRCLE('',#48579,0.0110624552747778);
#15914=CIRCLE('',#48582,0.0166052622177305);
#15915=CIRCLE('',#48584,0.0166047963821227);
#15916=CIRCLE('',#48585,0.0166052627674726);
#15917=CIRCLE('',#48586,0.0166047954504736);
#15918=CIRCLE('',#48587,0.0167731971567311);
#15919=CIRCLE('',#48588,0.0110573244852228);
#15920=CIRCLE('',#48589,0.0168013217001361);
#15921=CIRCLE('',#48590,0.0110316530738364);
#15922=CIRCLE('',#48591,0.0165310254896641);
#15923=CIRCLE('',#48593,0.0165263120151855);
#15924=CIRCLE('',#48594,0.016531026053535);
#15925=CIRCLE('',#48595,0.0165263111919852);
#15926=CIRCLE('',#48596,0.0166775856847841);
#15927=CIRCLE('',#48597,0.0109205691208038);
#15928=CIRCLE('',#48599,0.0164211150348133);
#15929=CIRCLE('',#48600,0.0164211142243237);
#15930=CIRCLE('',#48601,0.0167388248044049);
#15931=CIRCLE('',#48602,0.010967612429207);
#15932=CIRCLE('',#48603,0.0166825658005772);
#15933=CIRCLE('',#48604,0.011019447276484);
#15934=CIRCLE('',#48605,0.0165701548872828);
#15935=CIRCLE('',#48607,0.0165732958098313);
#15936=CIRCLE('',#48608,0.0165701556355031);
#15937=CIRCLE('',#48609,0.0165732948914799);
#15938=CIRCLE('',#48610,0.016814120646272);
#15939=CIRCLE('',#48611,0.011053537253304);
#15940=CIRCLE('',#48612,0.0168028429611533);
#15941=CIRCLE('',#48613,0.0110635670201188);
#15942=CIRCLE('',#48614,0.0166019907902361);
#15943=CIRCLE('',#48616,0.0166008685032828);
#15944=CIRCLE('',#48617,0.0166019914916695);
#15945=CIRCLE('',#48618,0.016600867649731);
#15946=CIRCLE('',#48619,0.0167571840015815);
#15947=CIRCLE('',#48620,0.011051199679);
#15948=CIRCLE('',#48621,0.0167907391088403);
#15949=CIRCLE('',#48622,0.0110190981841265);
#15950=CIRCLE('',#48623,0.00665874807866852);
#15951=CIRCLE('',#48629,0.0167157066790663);
#15952=CIRCLE('',#48630,0.0109625450116274);
#15953=CIRCLE('',#48632,0.0165541457744851);
#15954=CIRCLE('',#48634,0.0165579387507397);
#15955=CIRCLE('',#48635,0.016554146743131);
#15956=CIRCLE('',#48636,0.0165579377034758);
#15957=CIRCLE('',#48637,0.0168110399838886);
#15958=CIRCLE('',#48638,0.0110459668054311);
#15959=CIRCLE('',#48639,0.0167928000134423);
#15960=CIRCLE('',#48640,0.0110624552738554);
#15961=CIRCLE('',#48643,0.0166052623210084);
#15962=CIRCLE('',#48645,0.0166047962621703);
#15963=CIRCLE('',#48646,0.0166052628393574);
#15964=CIRCLE('',#48647,0.0166047955580633);
#15965=CIRCLE('',#48648,0.0167731971565687);
#15966=CIRCLE('',#48649,0.0110573244856284);
#15967=CIRCLE('',#48650,0.0168013217000599);
#15968=CIRCLE('',#48651,0.0110316530737674);
#15969=CIRCLE('',#48652,0.016531025343733);
#15970=CIRCLE('',#48654,0.0165263119423416);
#15971=CIRCLE('',#48655,0.0165310259885897);
#15972=CIRCLE('',#48656,0.0165263111618812);
#15973=CIRCLE('',#48657,0.0166775856845741);
#15974=CIRCLE('',#48658,0.0109205691218698);
#15975=CIRCLE('',#48660,0.0164211148044813);
#15976=CIRCLE('',#48661,0.0164211140991842);
#15977=CIRCLE('',#48662,0.0167388248044534);
#15978=CIRCLE('',#48663,0.0109676124283774);
#15979=CIRCLE('',#48664,0.0166825658003316);
#15980=CIRCLE('',#48665,0.011019447275932);
#15981=CIRCLE('',#48666,0.0165701549382436);
#15982=CIRCLE('',#48668,0.0165732957156712);
#15983=CIRCLE('',#48669,0.0165701555936647);
#15984=CIRCLE('',#48670,0.0165732948439745);
#15985=CIRCLE('',#48671,0.0168141205747683);
#15986=CIRCLE('',#48672,0.011053537408688);
#15987=CIRCLE('',#48673,0.0168028429614129);
#15988=CIRCLE('',#48674,0.0110635670205279);
#15989=CIRCLE('',#48675,0.0166019907724184);
#15990=CIRCLE('',#48677,0.0166008684458131);
#15991=CIRCLE('',#48678,0.0166019915037999);
#15992=CIRCLE('',#48679,0.0166008675674056);
#15993=CIRCLE('',#48680,0.0167571840019693);
#15994=CIRCLE('',#48681,0.0110511996785788);
#15995=CIRCLE('',#48682,0.0167907391089601);
#15996=CIRCLE('',#48683,0.0110190981854491);
#15997=CIRCLE('',#48684,0.00665874807856069);
#15998=CIRCLE('',#48690,0.016715706678537);
#15999=CIRCLE('',#48691,0.0109625450197299);
#16000=CIRCLE('',#48693,0.016554145832691);
#16001=CIRCLE('',#48695,0.0165579388535833);
#16002=CIRCLE('',#48696,0.0165541468078329);
#16003=CIRCLE('',#48697,0.0165579376714078);
#16004=CIRCLE('',#48698,0.0168110399839155);
#16005=CIRCLE('',#48699,0.0110459668052241);
#16006=CIRCLE('',#48700,0.0167928000135522);
#16007=CIRCLE('',#48701,0.0110624552747427);
#16008=CIRCLE('',#48704,0.0166052622016704);
#16009=CIRCLE('',#48706,0.016604796182051);
#16010=CIRCLE('',#48707,0.0166052627553303);
#16011=CIRCLE('',#48708,0.0166047954861773);
#16012=CIRCLE('',#48709,0.016773197156293);
#16013=CIRCLE('',#48710,0.0110573244845348);
#16014=CIRCLE('',#48711,0.0168013216996969);
#16015=CIRCLE('',#48712,0.0110316530734857);
#16016=CIRCLE('',#48713,0.0165310253971778);
#16017=CIRCLE('',#48715,0.0165263117090146);
#16018=CIRCLE('',#48716,0.0165310260091766);
#16019=CIRCLE('',#48717,0.0165263111336701);
#16020=CIRCLE('',#48718,0.0166775856849231);
#16021=CIRCLE('',#48719,0.0109205691220921);
#16022=CIRCLE('',#48721,0.0164211147379008);
#16023=CIRCLE('',#48722,0.0164211140186072);
#16024=CIRCLE('',#48723,0.0167388248039756);
#16025=CIRCLE('',#48724,0.0109676124295965);
#16026=CIRCLE('',#48725,0.0166825658000704);
#16027=CIRCLE('',#48726,0.0110194472757774);
#16028=CIRCLE('',#48727,0.0165701550589786);
#16029=CIRCLE('',#48729,0.0165732955439304);
#16030=CIRCLE('',#48730,0.0165701554623967);
#16031=CIRCLE('',#48731,0.0165732947607562);
#16032=CIRCLE('',#48732,0.0168141206460369);
#16033=CIRCLE('',#48733,0.0110535372552296);
#16034=CIRCLE('',#48734,0.016802842961279);
#16035=CIRCLE('',#48735,0.0110635670194712);
#16036=CIRCLE('',#48736,0.016601990558003);
#16037=CIRCLE('',#48738,0.0166008682641072);
#16038=CIRCLE('',#48739,0.0166019914886659);
#16039=CIRCLE('',#48740,0.0166008676115602);
#16040=CIRCLE('',#48741,0.0167571840015966);
#16041=CIRCLE('',#48742,0.0110511996789531);
#16042=CIRCLE('',#48743,0.0167907391091812);
#16043=CIRCLE('',#48744,0.0110190981859215);
#16044=CIRCLE('',#48745,0.0066587480786017);
#16045=CIRCLE('',#48752,0.016557938393399);
#16046=CIRCLE('',#48753,0.0165541465800056);
#16047=CIRCLE('',#48754,0.0165541457005333);
#16048=CIRCLE('',#48755,0.0165579375969566);
#16049=CIRCLE('',#48756,0.0167157066784803);
#16050=CIRCLE('',#48757,0.0109625450132406);
#16051=CIRCLE('',#48759,0.0168110399838593);
#16052=CIRCLE('',#48760,0.0110459668052074);
#16053=CIRCLE('',#48761,0.0167928000132456);
#16054=CIRCLE('',#48762,0.0110624552747817);
#16055=CIRCLE('',#48765,0.0166052620204301);
#16056=CIRCLE('',#48767,0.0166047961639415);
#16057=CIRCLE('',#48768,0.0166052628105858);
#16058=CIRCLE('',#48769,0.0166047955823238);
#16059=CIRCLE('',#48770,0.0167731971571948);
#16060=CIRCLE('',#48771,0.0110573244863);
#16061=CIRCLE('',#48772,0.0168013216971416);
#16062=CIRCLE('',#48773,0.0110316530737572);
#16063=CIRCLE('',#48774,0.0165310253747238);
#16064=CIRCLE('',#48776,0.016526312005147);
#16065=CIRCLE('',#48777,0.0165310260705086);
#16066=CIRCLE('',#48778,0.0165263109804035);
#16067=CIRCLE('',#48779,0.0166775856847484);
#16068=CIRCLE('',#48780,0.0109205691222534);
#16069=CIRCLE('',#48782,0.0164211146382283);
#16070=CIRCLE('',#48783,0.0164211139468424);
#16071=CIRCLE('',#48784,0.016738824804484);
#16072=CIRCLE('',#48785,0.0109676124291467);
#16073=CIRCLE('',#48786,0.0166825658004142);
#16074=CIRCLE('',#48787,0.0110194472756397);
#16075=CIRCLE('',#48788,0.016570155142403);
#16076=CIRCLE('',#48790,0.0165732953358236);
#16077=CIRCLE('',#48791,0.0165701555271706);
#16078=CIRCLE('',#48792,0.0165732944523174);
#16079=CIRCLE('',#48793,0.0168141205740459);
#16080=CIRCLE('',#48794,0.011053537408101);
#16081=CIRCLE('',#48795,0.0168028429610983);
#16082=CIRCLE('',#48796,0.0110635670202757);
#16083=CIRCLE('',#48797,0.016601990873592);
#16084=CIRCLE('',#48799,0.0166008681138699);
#16085=CIRCLE('',#48800,0.0166019914981724);
#16086=CIRCLE('',#48801,0.016600867635325);
#16087=CIRCLE('',#48802,0.0167571840016304);
#16088=CIRCLE('',#48803,0.0110511996746034);
#16089=CIRCLE('',#48804,0.0167907391096125);
#16090=CIRCLE('',#48805,0.0110190981856332);
#16091=CIRCLE('',#48806,0.00665874807864147);
#16092=CIRCLE('',#48813,0.0166047962151536);
#16093=CIRCLE('',#48814,0.0166052626736676);
#16094=CIRCLE('',#48815,0.0166052623558693);
#16095=CIRCLE('',#48816,0.0166047953839558);
#16096=CIRCLE('',#48818,0.0165579386710114);
#16097=CIRCLE('',#48819,0.0165541467375174);
#16098=CIRCLE('',#48820,0.0165541458003313);
#16099=CIRCLE('',#48821,0.0165579376502966);
#16100=CIRCLE('',#48822,0.0167157066782624);
#16101=CIRCLE('',#48823,0.0109625450121743);
#16102=CIRCLE('',#48825,0.0168110399837832);
#16103=CIRCLE('',#48826,0.0110459668064786);
#16104=CIRCLE('',#48827,0.0167928000131371);
#16105=CIRCLE('',#48828,0.0110624552742206);
#16106=CIRCLE('',#48831,0.0167731941318447);
#16107=CIRCLE('',#48832,0.0110573150854568);
#16108=CIRCLE('',#48833,0.016801321700207);
#16109=CIRCLE('',#48834,0.0110316530747847);
#16110=CIRCLE('',#48835,0.0165310253466521);
#16111=CIRCLE('',#48837,0.0165263118016029);
#16112=CIRCLE('',#48838,0.0165310260720093);
#16113=CIRCLE('',#48839,0.0165263109786302);
#16114=CIRCLE('',#48840,0.0166775856849412);
#16115=CIRCLE('',#48841,0.0109205691228325);
#16116=CIRCLE('',#48843,0.0164211146258441);
#16117=CIRCLE('',#48844,0.0164211141132704);
#16118=CIRCLE('',#48845,0.0167388248046037);
#16119=CIRCLE('',#48846,0.010967612428738);
#16120=CIRCLE('',#48847,0.0166825658000916);
#16121=CIRCLE('',#48848,0.0110194472760106);
#16122=CIRCLE('',#48849,0.0165701550493577);
#16123=CIRCLE('',#48851,0.0165732951167833);
#16124=CIRCLE('',#48852,0.0165701554481991);
#16125=CIRCLE('',#48853,0.0165732947079051);
#16126=CIRCLE('',#48854,0.0168141206459652);
#16127=CIRCLE('',#48855,0.0110535372533542);
#16128=CIRCLE('',#48856,0.0168028429612053);
#16129=CIRCLE('',#48857,0.011063567020668);
#16130=CIRCLE('',#48858,0.016601990796754);
#16131=CIRCLE('',#48860,0.0166008681495549);
#16132=CIRCLE('',#48861,0.016601991287057);
#16133=CIRCLE('',#48862,0.0166008676670592);
#16134=CIRCLE('',#48863,0.0167571840015897);
#16135=CIRCLE('',#48864,0.0110511996792007);
#16136=CIRCLE('',#48865,0.0167907391090489);
#16137=CIRCLE('',#48866,0.011019098184922);
#16138=CIRCLE('',#48867,0.00665874807852574);
#16139=CIRCLE('',#48874,0.016557937242374);
#16140=CIRCLE('',#48875,0.0165541493793539);
#16141=CIRCLE('',#48876,0.0165541529820997);
#16142=CIRCLE('',#48877,0.0165579410864609);
#16143=CIRCLE('',#48879,0.0165263116215834);
#16144=CIRCLE('',#48880,0.0165310258878028);
#16145=CIRCLE('',#48881,0.0165310253924632);
#16146=CIRCLE('',#48882,0.0165263111348691);
#16147=CIRCLE('',#48884,0.0166047959564872);
#16148=CIRCLE('',#48885,0.0166052625710691);
#16149=CIRCLE('',#48886,0.016605262158595);
#16150=CIRCLE('',#48887,0.0166047955076839);
#16151=CIRCLE('',#48888,0.0168110399834951);
#16152=CIRCLE('',#48889,0.0110459668057758);
#16153=CIRCLE('',#48890,0.0167928000131421);
#16154=CIRCLE('',#48891,0.0110624552741314);
#16155=CIRCLE('',#48894,0.0167731971562018);
#16156=CIRCLE('',#48895,0.011057324484393);
#16157=CIRCLE('',#48896,0.0168013216998445);
#16158=CIRCLE('',#48897,0.0110316530740487);
#16159=CIRCLE('',#48898,0.016677585684157);
#16160=CIRCLE('',#48899,0.0109205691204241);
#16161=CIRCLE('',#48900,0.0167157066790715);
#16162=CIRCLE('',#48901,0.0109625450147775);
#16163=CIRCLE('',#48904,0.0164211142969033);
#16164=CIRCLE('',#48905,0.0164211138522741);
#16165=CIRCLE('',#48906,0.0167388248042754);
#16166=CIRCLE('',#48907,0.0109676124296621);
#16167=CIRCLE('',#48908,0.0166825658001335);
#16168=CIRCLE('',#48909,0.0110194472755734);
#16169=CIRCLE('',#48910,0.016570154969177);
#16170=CIRCLE('',#48912,0.0165732952369211);
#16171=CIRCLE('',#48913,0.0165701552418422);
#16172=CIRCLE('',#48914,0.0165732945809266);
#16173=CIRCLE('',#48915,0.0168141205748277);
#16174=CIRCLE('',#48916,0.0110535374108902);
#16175=CIRCLE('',#48917,0.0168028429609699);
#16176=CIRCLE('',#48918,0.0110635670205065);
#16177=CIRCLE('',#48919,0.0166019908221658);
#16178=CIRCLE('',#48921,0.0166008677448166);
#16179=CIRCLE('',#48922,0.0166019910949407);
#16180=CIRCLE('',#48923,0.0166008676018247);
#16181=CIRCLE('',#48924,0.0167571840016316);
#16182=CIRCLE('',#48925,0.0110511996795116);
#16183=CIRCLE('',#48926,0.0167907391092683);
#16184=CIRCLE('',#48927,0.0110190981847272);
#16185=CIRCLE('',#48928,0.00665874807855451);
#16186=CIRCLE('',#48935,0.0165579455857381);
#16187=CIRCLE('',#48936,0.0165541498437811);
#16188=CIRCLE('',#48937,0.0165541457456698);
#16189=CIRCLE('',#48938,0.0165579408786856);
#16190=CIRCLE('',#48940,0.016604795239985);
#16191=CIRCLE('',#48941,0.0166052660684846);
#16192=CIRCLE('',#48942,0.0166052697732378);
#16193=CIRCLE('',#48943,0.0166047985728746);
#16194=CIRCLE('',#48945,0.016421114122627);
#16195=CIRCLE('',#48946,0.0164211138454056);
#16196=CIRCLE('',#48948,0.0165263119725143);
#16197=CIRCLE('',#48949,0.0165310259092296);
#16198=CIRCLE('',#48950,0.0165310254281581);
#16199=CIRCLE('',#48951,0.0165263110945175);
#16200=CIRCLE('',#48952,0.0167731941324389);
#16201=CIRCLE('',#48953,0.0110573150841859);
#16202=CIRCLE('',#48954,0.0168013216994028);
#16203=CIRCLE('',#48955,0.0110316530738022);
#16204=CIRCLE('',#48956,0.0166775856846015);
#16205=CIRCLE('',#48957,0.0109205691205302);
#16206=CIRCLE('',#48958,0.0167388248039332);
#16207=CIRCLE('',#48959,0.0109676124292315);
#16208=CIRCLE('',#48960,0.0166825658001939);
#16209=CIRCLE('',#48961,0.0110194472762046);
#16210=CIRCLE('',#48962,0.0165701550429815);
#16211=CIRCLE('',#48963,0.0167157066790929);
#16212=CIRCLE('',#48964,0.0109625450184708);
#16213=CIRCLE('',#48966,0.0168110399829948);
#16214=CIRCLE('',#48967,0.0110459668038541);
#16215=CIRCLE('',#48968,0.0167928000131439);
#16216=CIRCLE('',#48969,0.0110624552739188);
#16217=CIRCLE('',#48973,0.0165732949494959);
#16218=CIRCLE('',#48974,0.0165701553102014);
#16219=CIRCLE('',#48975,0.016573294404056);
#16220=CIRCLE('',#48976,0.0168141206275132);
#16221=CIRCLE('',#48977,0.0110535372967461);
#16222=CIRCLE('',#48978,0.0168028429610256);
#16223=CIRCLE('',#48979,0.0110635670189512);
#16224=CIRCLE('',#48980,0.016601990634965);
#16225=CIRCLE('',#48982,0.0166008677966898);
#16226=CIRCLE('',#48983,0.0166019912748291);
#16227=CIRCLE('',#48984,0.0166008673365702);
#16228=CIRCLE('',#48985,0.0167571840017735);
#16229=CIRCLE('',#48986,0.0110511996760864);
#16230=CIRCLE('',#48987,0.016790739108973);
#16231=CIRCLE('',#48988,0.0110190981836151);
#16232=CIRCLE('',#48989,0.006658748078702);
#16233=CIRCLE('',#48996,0.0166048028270532);
#16234=CIRCLE('',#48997,0.0166052661745815);
#16235=CIRCLE('',#48998,0.0166052620760957);
#16236=CIRCLE('',#48999,0.0166047986766637);
#16237=CIRCLE('',#49001,0.0165263107944059);
#16238=CIRCLE('',#49002,0.0165310291800569);
#16239=CIRCLE('',#49003,0.016531033258646);
#16240=CIRCLE('',#49004,0.0165263139561476);
#16241=CIRCLE('',#49006,0.0165579452785632);
#16242=CIRCLE('',#49007,0.0165541498850607);
#16243=CIRCLE('',#49008,0.0165541458961846);
#16244=CIRCLE('',#49009,0.0165579408553482);
#16245=CIRCLE('',#49011,0.0165732946997177);
#16246=CIRCLE('',#49012,0.0165701553210565);
#16247=CIRCLE('',#49013,0.0165701549414162);
#16248=CIRCLE('',#49014,0.0165732941125412);
#16249=CIRCLE('',#49016,0.0164211139334697);
#16250=CIRCLE('',#49017,0.0164211136739296);
#16251=CIRCLE('',#49018,0.0166775856845022);
#16252=CIRCLE('',#49019,0.0109205691229004);
#16253=CIRCLE('',#49020,0.0167388248043908);
#16254=CIRCLE('',#49021,0.0109676124286852);
#16255=CIRCLE('',#49022,0.0166825658001782);
#16256=CIRCLE('',#49023,0.0110194472770084);
#16257=CIRCLE('',#49024,0.0168141206268823);
#16258=CIRCLE('',#49025,0.0110535372941716);
#16259=CIRCLE('',#49026,0.0168028429606942);
#16260=CIRCLE('',#49027,0.0110635670207016);
#16261=CIRCLE('',#49028,0.0166019907542044);
#16262=CIRCLE('',#49029,0.0167157066784153);
#16263=CIRCLE('',#49030,0.0109625450155666);
#16264=CIRCLE('',#49032,0.0168110399837356);
#16265=CIRCLE('',#49033,0.0110459668043168);
#16266=CIRCLE('',#49034,0.0167928000125649);
#16267=CIRCLE('',#49035,0.0110624552757974);
#16268=CIRCLE('',#49038,0.0167731971566166);
#16269=CIRCLE('',#49039,0.0110573244865956);
#16270=CIRCLE('',#49040,0.0168013216996847);
#16271=CIRCLE('',#49041,0.0110316530734883);
#16272=CIRCLE('',#49043,0.016600867675102);
#16273=CIRCLE('',#49044,0.0166019908963819);
#16274=CIRCLE('',#49045,0.0166008673124711);
#16275=CIRCLE('',#49046,0.0167571840015828);
#16276=CIRCLE('',#49047,0.0110511996731572);
#16277=CIRCLE('',#49048,0.0167907391094298);
#16278=CIRCLE('',#49049,0.0110190981840155);
#16279=CIRCLE('',#49050,0.00665874807849252);
#16280=CIRCLE('',#49057,0.0165263179950152);
#16281=CIRCLE('',#49058,0.0165310293667509);
#16282=CIRCLE('',#49059,0.0165310254750887);
#16283=CIRCLE('',#49060,0.0165263142576533);
#16284=CIRCLE('',#49062,0.016421112801567);
#16285=CIRCLE('',#49063,0.0164211129684179);
#16286=CIRCLE('',#49065,0.0166048025454181);
#16287=CIRCLE('',#49066,0.0166052658521807);
#16288=CIRCLE('',#49067,0.0166052623722192);
#16289=CIRCLE('',#49068,0.016604799156512);
#16290=CIRCLE('',#49070,0.0165579450668964);
#16291=CIRCLE('',#49071,0.0165541497704911);
#16292=CIRCLE('',#49072,0.0165541458562401);
#16293=CIRCLE('',#49073,0.0165579409363684);
#16294=CIRCLE('',#49075,0.0166008675583637);
#16295=CIRCLE('',#49076,0.0166019911921346);
#16296=CIRCLE('',#49077,0.0166019909806196);
#16297=CIRCLE('',#49078,0.0166008674180751);
#16298=CIRCLE('',#49080,0.0165732948516365);
#16299=CIRCLE('',#49081,0.0165701549539817);
#16300=CIRCLE('',#49082,0.0165701548215611);
#16301=CIRCLE('',#49083,0.0165732946310353);
#16302=CIRCLE('',#49084,0.0167388235414638);
#16303=CIRCLE('',#49085,0.0109676133208622);
#16304=CIRCLE('',#49086,0.0166825658004335);
#16305=CIRCLE('',#49087,0.0110194472763306);
#16306=CIRCLE('',#49088,0.0168141206269654);
#16307=CIRCLE('',#49089,0.0110535372941354);
#16308=CIRCLE('',#49090,0.0168028429606016);
#16309=CIRCLE('',#49091,0.0110635670210023);
#16310=CIRCLE('',#49092,0.0167577810042491);
#16311=CIRCLE('',#49093,0.0110511996741528);
#16312=CIRCLE('',#49094,0.0167907391083702);
#16313=CIRCLE('',#49095,0.0110190981849621);
#16314=CIRCLE('',#49096,0.00665874807860464);
#16315=CIRCLE('',#49097,0.016715706678561);
#16316=CIRCLE('',#49098,0.0109625450139336);
#16317=CIRCLE('',#49100,0.01681103998381);
#16318=CIRCLE('',#49101,0.0110459668040065);
#16319=CIRCLE('',#49102,0.0167928000129461);
#16320=CIRCLE('',#49103,0.011062455275826);
#16321=CIRCLE('',#49106,0.0167731971564552);
#16322=CIRCLE('',#49107,0.0110573244867307);
#16323=CIRCLE('',#49108,0.0168013217000393);
#16324=CIRCLE('',#49109,0.0110316530743163);
#16325=CIRCLE('',#49110,0.0166775856850414);
#16326=CIRCLE('',#49111,0.0109205691219998);
#16327=CIRCLE('',#49127,0.0167388260783937);
#16328=CIRCLE('',#49128,0.0166825657982655);
#16329=CIRCLE('',#49129,0.016677585688039);
#16330=CIRCLE('',#49130,0.0168013216997719);
#16331=CIRCLE('',#49131,0.0167731941307207);
#16332=CIRCLE('',#49132,0.0167927979163913);
#16333=CIRCLE('',#49133,0.0168110399834981);
#16334=CIRCLE('',#49134,0.0167157066894911);
#16335=CIRCLE('',#49135,0.016669993461729);
#16336=CIRCLE('',#49138,0.016790740140474);
#16337=CIRCLE('',#49139,0.0167556795651006);
#16338=CIRCLE('',#49140,0.0168141206870994);
#16339=CIRCLE('',#49141,0.0168028429614352);
#16340=CIRCLE('',#49144,0.0167907401409518);
#16341=CIRCLE('',#49145,0.0167556795649506);
#16342=CIRCLE('',#49146,0.0166775856879641);
#16343=CIRCLE('',#49147,0.0168013216996554);
#16344=CIRCLE('',#49148,0.0167731941280413);
#16345=CIRCLE('',#49149,0.0167927979156723);
#16346=CIRCLE('',#49150,0.0168110399832801);
#16347=CIRCLE('',#49151,0.0167157066891269);
#16348=CIRCLE('',#49152,0.0166699934626322);
#16349=CIRCLE('',#49153,0.0168028429612061);
#16350=CIRCLE('',#49154,0.0168141206870611);
#16351=CIRCLE('',#49155,0.0167388260793371);
#16352=CIRCLE('',#49156,0.016682565798012);
#16353=CIRCLE('',#49159,0.0167907401408078);
#16354=CIRCLE('',#49160,0.0167556795652516);
#16355=CIRCLE('',#49161,0.0168028429610846);
#16356=CIRCLE('',#49162,0.0168141206870671);
#16357=CIRCLE('',#49163,0.0167731941284153);
#16358=CIRCLE('',#49164,0.0168013216997419);
#16359=CIRCLE('',#49165,0.016792797915505);
#16360=CIRCLE('',#49166,0.0168110399837014);
#16361=CIRCLE('',#49167,0.0167157066890383);
#16362=CIRCLE('',#49168,0.0166699934636628);
#16363=CIRCLE('',#49169,0.0166825657979271);
#16364=CIRCLE('',#49170,0.0167388260780698);
#16365=CIRCLE('',#49171,0.0166775856878139);
#16366=CIRCLE('',#49174,0.0167907401403366);
#16367=CIRCLE('',#49175,0.0167556795651758);
#16368=CIRCLE('',#49176,0.0168028429612437);
#16369=CIRCLE('',#49177,0.016814120686832);
#16370=CIRCLE('',#49178,0.0166825657979198);
#16371=CIRCLE('',#49179,0.0167388260787839);
#16372=CIRCLE('',#49180,0.0168110399833388);
#16373=CIRCLE('',#49181,0.0167927979159865);
#16374=CIRCLE('',#49182,0.0167157066893643);
#16375=CIRCLE('',#49183,0.0166699934636401);
#16376=CIRCLE('',#49184,0.0166775856879577);
#16377=CIRCLE('',#49185,0.0167731941306356);
#16378=CIRCLE('',#49186,0.0168013217000056);
#16379=CIRCLE('',#49189,0.016790740140676);
#16380=CIRCLE('',#49190,0.0167556795647294);
#16381=CIRCLE('',#49191,0.0168028429607678);
#16382=CIRCLE('',#49192,0.016814120686581);
#16383=CIRCLE('',#49193,0.016682565798137);
#16384=CIRCLE('',#49194,0.0167388260784122);
#16385=CIRCLE('',#49195,0.0166775856881153);
#16386=CIRCLE('',#49196,0.0167157066889213);
#16387=CIRCLE('',#49197,0.0166699934634911);
#16388=CIRCLE('',#49198,0.0168013217001458);
#16389=CIRCLE('',#49199,0.0167731941276694);
#16390=CIRCLE('',#49200,0.0168110399835617);
#16391=CIRCLE('',#49201,0.0167927979161373);
#16392=CIRCLE('',#49204,0.0167907401403663);
#16393=CIRCLE('',#49205,0.0167556795645121);
#16394=CIRCLE('',#49206,0.0168028429610977);
#16395=CIRCLE('',#49207,0.0168141206872044);
#16396=CIRCLE('',#49208,0.0166825657978588);
#16397=CIRCLE('',#49209,0.0167388260786764);
#16398=CIRCLE('',#49210,0.0166775856875181);
#16399=CIRCLE('',#49211,0.0168013216997636);
#16400=CIRCLE('',#49212,0.0167731941312831);
#16401=CIRCLE('',#49213,0.0167927979156146);
#16402=CIRCLE('',#49214,0.0168110399829328);
#16403=CIRCLE('',#49215,0.0167157066892931);
#16404=CIRCLE('',#49216,0.0166699934628592);
#16405=CIRCLE('',#49219,0.0167907401406868);
#16406=CIRCLE('',#49220,0.016755679564891);
#16407=CIRCLE('',#49221,0.0168028429609253);
#16408=CIRCLE('',#49222,0.016814120687073);
#16409=CIRCLE('',#49223,0.0166825657976404);
#16410=CIRCLE('',#49224,0.0167388260782794);
#16411=CIRCLE('',#49225,0.0166775856880801);
#16412=CIRCLE('',#49226,0.0168013217001565);
#16413=CIRCLE('',#49227,0.0167731941275393);
#16414=CIRCLE('',#49228,0.0167927979158512);
#16415=CIRCLE('',#49229,0.0168110399828972);
#16416=CIRCLE('',#49230,0.016715706690013);
#16417=CIRCLE('',#49231,0.0166699934626573);
#16418=CIRCLE('',#49234,0.0167907401409215);
#16419=CIRCLE('',#49235,0.0167556795649318);
#16420=CIRCLE('',#49236,0.0168028429612012);
#16421=CIRCLE('',#49237,0.0168141206870639);
#16422=CIRCLE('',#49238,0.0166825657980482);
#16423=CIRCLE('',#49239,0.0167388260785539);
#16424=CIRCLE('',#49240,0.0166775856881294);
#16425=CIRCLE('',#49241,0.0168013217002588);
#16426=CIRCLE('',#49242,0.0167731941275873);
#16427=CIRCLE('',#49243,0.0167927979163074);
#16428=CIRCLE('',#49244,0.0168110399834913);
#16429=CIRCLE('',#49245,0.01671570669022);
#16430=CIRCLE('',#49246,0.0166699934637729);
#16431=CIRCLE('',#49249,0.0167907401408375);
#16432=CIRCLE('',#49250,0.0167556795644563);
#16433=CIRCLE('',#49251,0.0168028429614237);
#16434=CIRCLE('',#49252,0.0168141206867054);
#16435=CIRCLE('',#49253,0.0166825657978822);
#16436=CIRCLE('',#49254,0.0167388260784786);
#16437=CIRCLE('',#49255,0.0166775856882109);
#16438=CIRCLE('',#49256,0.0168013217001937);
#16439=CIRCLE('',#49257,0.0167731941272391);
#16440=CIRCLE('',#49258,0.0167927979160117);
#16441=CIRCLE('',#49259,0.0168110399832238);
#16442=CIRCLE('',#49260,0.0167157066898009);
#16443=CIRCLE('',#49261,0.0166699934627845);
#16444=CIRCLE('',#49264,0.0167907401407062);
#16445=CIRCLE('',#49265,0.0167556795646256);
#16446=CIRCLE('',#49266,0.0168028429611231);
#16447=CIRCLE('',#49267,0.0168141206869206);
#16448=CIRCLE('',#49268,0.0166825657980672);
#16449=CIRCLE('',#49269,0.0167388260784666);
#16450=CIRCLE('',#49270,0.0166775856878968);
#16451=CIRCLE('',#49271,0.0168013217000833);
#16452=CIRCLE('',#49272,0.0167731941274843);
#16453=CIRCLE('',#49273,0.0167927979160231);
#16454=CIRCLE('',#49274,0.0168110399832967);
#16455=CIRCLE('',#49275,0.0167157066900166);
#16456=CIRCLE('',#49276,0.0166699934635313);
#16457=CIRCLE('',#49279,0.0167907401405469);
#16458=CIRCLE('',#49280,0.0167556795646356);
#16459=CIRCLE('',#49281,0.0168028429610838);
#16460=CIRCLE('',#49282,0.0168141206869845);
#16461=CIRCLE('',#49283,0.0166825657980557);
#16462=CIRCLE('',#49284,0.0167388260783001);
#16463=CIRCLE('',#49285,0.0166775856879415);
#16464=CIRCLE('',#49286,0.0168013216996465);
#16465=CIRCLE('',#49287,0.0167731941273415);
#16466=CIRCLE('',#49288,0.0167927979157984);
#16467=CIRCLE('',#49289,0.0168110399832164);
#16468=CIRCLE('',#49290,0.0167157066897016);
#16469=CIRCLE('',#49291,0.0166699934628616);
#16470=CIRCLE('',#49294,0.0167907401405266);
#16471=CIRCLE('',#49295,0.0167556795645506);
#16472=CIRCLE('',#49296,0.0168028429611932);
#16473=CIRCLE('',#49297,0.0168141206868017);
#16474=CIRCLE('',#49298,0.016682565798159);
#16475=CIRCLE('',#49299,0.0167388260783459);
#16476=CIRCLE('',#49300,0.0166775856879777);
#16477=CIRCLE('',#49301,0.0168013216996097);
#16478=CIRCLE('',#49302,0.0167731941274576);
#16479=CIRCLE('',#49303,0.0167927979157949);
#16480=CIRCLE('',#49304,0.0168110399830942);
#16481=CIRCLE('',#49305,0.0167157066896616);
#16482=CIRCLE('',#49306,0.0166699934630128);
#16483=CIRCLE('',#49309,0.0167907401404702);
#16484=CIRCLE('',#49310,0.0167556795647818);
#16485=CIRCLE('',#49311,0.0168028429611256);
#16486=CIRCLE('',#49312,0.0168141206869255);
#16487=CIRCLE('',#49313,0.0166825657979659);
#16488=CIRCLE('',#49314,0.0167388260782657);
#16489=CIRCLE('',#49315,0.0166775856881158);
#16490=CIRCLE('',#49316,0.0168013216998003);
#16491=CIRCLE('',#49317,0.0167731941278287);
#16492=CIRCLE('',#49318,0.0167927979158031);
#16493=CIRCLE('',#49319,0.0168110399831387);
#16494=CIRCLE('',#49320,0.0167157066897092);
#16495=CIRCLE('',#49321,0.0166699934632686);
#16496=CIRCLE('',#49324,0.0167907401404887);
#16497=CIRCLE('',#49325,0.0167556795649006);
#16498=CIRCLE('',#49326,0.0168028429610311);
#16499=CIRCLE('',#49327,0.0168141206867439);
#16500=CIRCLE('',#49328,0.0166825657981543);
#16501=CIRCLE('',#49329,0.0167388260782707);
#16502=CIRCLE('',#49330,0.0166775856879633);
#16503=CIRCLE('',#49331,0.0168013216997165);
#16504=CIRCLE('',#49332,0.0167731941261392);
#16505=CIRCLE('',#49333,0.0167927979157724);
#16506=CIRCLE('',#49334,0.0168110399830984);
#16507=CIRCLE('',#49335,0.0167157066895802);
#16508=CIRCLE('',#49336,0.0166699934630215);
#16509=CIRCLE('',#49339,0.0167907401405266);
#16510=CIRCLE('',#49340,0.0167556795647706);
#16511=CIRCLE('',#49341,0.0168028429610707);
#16512=CIRCLE('',#49342,0.0168141206869169);
#16513=CIRCLE('',#49343,0.0166825657981712);
#16514=CIRCLE('',#49344,0.0167388260781345);
#16515=CIRCLE('',#49345,0.0166775856880515);
#16516=CIRCLE('',#49346,0.0168013216996411);
#16517=CIRCLE('',#49347,0.0167731941277484);
#16518=CIRCLE('',#49348,0.0167927979158021);
#16519=CIRCLE('',#49349,0.0168110399831109);
#16520=CIRCLE('',#49350,0.0167157066894836);
#16521=CIRCLE('',#49351,0.01666999346303);
#16522=CIRCLE('',#49354,0.0167907401402849);
#16523=CIRCLE('',#49355,0.0167556795649538);
#16524=CIRCLE('',#49356,0.0168028429613468);
#16525=CIRCLE('',#49357,0.0168141206865413);
#16526=CIRCLE('',#49358,0.0166825657981593);
#16527=CIRCLE('',#49359,0.0167388260788683);
#16528=CIRCLE('',#49360,0.0166775856882428);
#16529=CIRCLE('',#49361,0.0168013216994228);
#16530=CIRCLE('',#49362,0.016773194127514);
#16531=CIRCLE('',#49363,0.0167927979156933);
#16532=CIRCLE('',#49364,0.0168110399830131);
#16533=CIRCLE('',#49365,0.0167157066897977);
#16534=CIRCLE('',#49366,0.0166699934631597);
#16535=CIRCLE('',#49369,0.0167907401403453);
#16536=CIRCLE('',#49370,0.0167556795646501);
#16537=CIRCLE('',#49371,0.0168028429612447);
#16538=CIRCLE('',#49372,0.0168141206866647);
#16539=CIRCLE('',#49373,0.0166825657980678);
#16540=CIRCLE('',#49374,0.016738826078584);
#16541=CIRCLE('',#49375,0.0166775856878689);
#16542=CIRCLE('',#49376,0.0168013216998913);
#16543=CIRCLE('',#49377,0.0167731941274802);
#16544=CIRCLE('',#49378,0.0167927979155802);
#16545=CIRCLE('',#49379,0.0168110399832431);
#16546=CIRCLE('',#49380,0.0167157066894647);
#16547=CIRCLE('',#49381,0.0166699934627573);
#16548=CIRCLE('',#49384,0.0167907401399346);
#16549=CIRCLE('',#49385,0.016755679564844);
#16550=CIRCLE('',#49386,0.0168028429610995);
#16551=CIRCLE('',#49387,0.0168141206868666);
#16552=CIRCLE('',#49388,0.0166825657982027);
#16553=CIRCLE('',#49389,0.0167388260782498);
#16554=CIRCLE('',#49390,0.0166775856882351);
#16555=CIRCLE('',#49391,0.0168013216997972);
#16556=CIRCLE('',#49392,0.0167731941278249);
#16557=CIRCLE('',#49393,0.0167927979153362);
#16558=CIRCLE('',#49394,0.0168110399829424);
#16559=CIRCLE('',#49395,0.016715706689545);
#16560=CIRCLE('',#49396,0.0166699934633333);
#16561=CIRCLE('',#49399,0.0167907401404065);
#16562=CIRCLE('',#49400,0.0167556795645056);
#16563=CIRCLE('',#49401,0.0168028429610298);
#16564=CIRCLE('',#49402,0.0168141206869512);
#16565=CIRCLE('',#49403,0.0166825657981821);
#16566=CIRCLE('',#49404,0.0167388260779847);
#16567=CIRCLE('',#49405,0.0166775856883076);
#16568=CIRCLE('',#49406,0.0168013217000258);
#16569=CIRCLE('',#49407,0.016773194127048);
#16570=CIRCLE('',#49408,0.0167927979160005);
#16571=CIRCLE('',#49409,0.0168110399829486);
#16572=CIRCLE('',#49410,0.016715706689756);
#16573=CIRCLE('',#49411,0.0166699934628589);
#16574=CIRCLE('',#49414,0.0167907401403316);
#16575=CIRCLE('',#49415,0.0167556795644366);
#16576=CIRCLE('',#49416,0.0168028429610019);
#16577=CIRCLE('',#49417,0.016814120687397);
#16578=CIRCLE('',#49418,0.0166825657985891);
#16579=CIRCLE('',#49419,0.0167388260779154);
#16580=CIRCLE('',#49420,0.0166775856881447);
#16581=CIRCLE('',#49421,0.0168013216997569);
#16582=CIRCLE('',#49422,0.0167731941313463);
#16583=CIRCLE('',#49423,0.0167927979160407);
#16584=CIRCLE('',#49424,0.0168110399828166);
#16585=CIRCLE('',#49425,0.016715706689698);
#16586=CIRCLE('',#49426,0.0166699934624352);
#16587=CIRCLE('',#49429,0.0167907401401542);
#16588=CIRCLE('',#49430,0.0167556795645292);
#16589=CIRCLE('',#49431,0.016802842961176);
#16590=CIRCLE('',#49432,0.016814120686921);
#16591=CIRCLE('',#49433,0.0166825657981214);
#16592=CIRCLE('',#49434,0.0167388260781204);
#16593=CIRCLE('',#49435,0.0166775856878453);
#16594=CIRCLE('',#49436,0.0168013217000734);
#16595=CIRCLE('',#49437,0.0167731941274432);
#16596=CIRCLE('',#49438,0.0167927979156718);
#16597=CIRCLE('',#49439,0.0168110399831377);
#16598=CIRCLE('',#49440,0.0167157066896371);
#16599=CIRCLE('',#49441,0.0166699934621213);
#16600=CIRCLE('',#49444,0.0167907401408063);
#16601=CIRCLE('',#49445,0.0167556795650037);
#16602=CIRCLE('',#49446,0.0168028429611068);
#16603=CIRCLE('',#49447,0.0168141206864774);
#16604=CIRCLE('',#49448,0.0166825657986373);
#16605=CIRCLE('',#49449,0.0167388260793153);
#16606=CIRCLE('',#49450,0.0166775856881973);
#16607=CIRCLE('',#49451,0.0168013216999736);
#16608=CIRCLE('',#49452,0.0167731941279987);
#16609=CIRCLE('',#49453,0.0167927979157798);
#16610=CIRCLE('',#49454,0.0168110399829498);
#16611=CIRCLE('',#49455,0.0167157066894906);
#16612=CIRCLE('',#49456,0.0166699934635282);
#16613=CIRCLE('',#49459,0.0167907401399869);
#16614=CIRCLE('',#49460,0.0167556795645096);
#16615=CIRCLE('',#49461,0.0168028429608607);
#16616=CIRCLE('',#49462,0.0168141206866532);
#16617=CIRCLE('',#49463,0.0166825657986826);
#16618=CIRCLE('',#49464,0.0167388260779909);
#16619=CIRCLE('',#49465,0.0166775856878773);
#16620=CIRCLE('',#49466,0.0168013216998194);
#16621=CIRCLE('',#49467,0.0167731941269337);
#16622=CIRCLE('',#49468,0.0167927979154591);
#16623=CIRCLE('',#49469,0.0168110399830451);
#16624=CIRCLE('',#49470,0.016715706689462);
#16625=CIRCLE('',#49471,0.0166699934625152);
#16626=CIRCLE('',#49474,0.0167907401401331);
#16627=CIRCLE('',#49475,0.0167556795646395);
#16628=CIRCLE('',#49476,0.0168028429616909);
#16629=CIRCLE('',#49477,0.0168141206867984);
#16630=CIRCLE('',#49478,0.0166825657987859);
#16631=CIRCLE('',#49479,0.0167388260782469);
#16632=CIRCLE('',#49480,0.0166775856879888);
#16633=CIRCLE('',#49481,0.0168013216991336);
#16634=CIRCLE('',#49482,0.0167731941268989);
#16635=CIRCLE('',#49483,0.0167927979157023);
#16636=CIRCLE('',#49484,0.0168110399830373);
#16637=CIRCLE('',#49485,0.0167157066891133);
#16638=CIRCLE('',#49486,0.0166699934636415);
#16639=CIRCLE('',#49489,0.0167907401399268);
#16640=CIRCLE('',#49490,0.016755679564799);
#16641=CIRCLE('',#49491,0.0168028429610272);
#16642=CIRCLE('',#49492,0.0168141206865376);
#16643=CIRCLE('',#49493,0.0166825657977261);
#16644=CIRCLE('',#49494,0.0167388260780295);
#16645=CIRCLE('',#49495,0.0166775856882616);
#16646=CIRCLE('',#49496,0.0168013216989463);
#16647=CIRCLE('',#49497,0.016773194127227);
#16648=CIRCLE('',#49498,0.0167927979160616);
#16649=CIRCLE('',#49499,0.0168110399825236);
#16650=CIRCLE('',#49500,0.0167157066891566);
#16651=CIRCLE('',#49501,0.0166699934635826);
#16652=CIRCLE('',#49504,0.0167907401403848);
#16653=CIRCLE('',#49505,0.0167556795649154);
#16654=CIRCLE('',#49506,0.0168028429616512);
#16655=CIRCLE('',#49507,0.0168141206873185);
#16656=CIRCLE('',#49508,0.0166825657986855);
#16657=CIRCLE('',#49509,0.0167388260784559);
#16658=CIRCLE('',#49510,0.0166775856884377);
#16659=CIRCLE('',#49511,0.016801321699798);
#16660=CIRCLE('',#49512,0.0167731941264143);
#16661=CIRCLE('',#49513,0.0167927979155266);
#16662=CIRCLE('',#49514,0.0168110399834553);
#16663=CIRCLE('',#49515,0.0167157066896358);
#16664=CIRCLE('',#49516,0.0166699934627382);
#16665=CIRCLE('',#49519,0.0167907401403515);
#16666=CIRCLE('',#49520,0.0167556795649599);
#16667=CIRCLE('',#49521,0.0168028429606613);
#16668=CIRCLE('',#49522,0.0168141206865821);
#16669=CIRCLE('',#49523,0.016682565798408);
#16670=CIRCLE('',#49524,0.0167388260783537);
#16671=CIRCLE('',#49525,0.0166775856878138);
#16672=CIRCLE('',#49526,0.016801321699649);
#16673=CIRCLE('',#49527,0.0167731941281915);
#16674=CIRCLE('',#49528,0.0167927979157696);
#16675=CIRCLE('',#49529,0.016811039982445);
#16676=CIRCLE('',#49530,0.0167157066896602);
#16677=CIRCLE('',#49531,0.0166699934624107);
#16678=CIRCLE('',#49534,0.0167907401405091);
#16679=CIRCLE('',#49535,0.0167556795648695);
#16680=CIRCLE('',#49536,0.0168028429605574);
#16681=CIRCLE('',#49537,0.0168141206868357);
#16682=CIRCLE('',#49538,0.0166825657984589);
#16683=CIRCLE('',#49539,0.0167388260780524);
#16684=CIRCLE('',#49540,0.0166775856881515);
#16685=CIRCLE('',#49541,0.0168013216994995);
#16686=CIRCLE('',#49542,0.0167731941274536);
#16687=CIRCLE('',#49543,0.016792797915285);
#16688=CIRCLE('',#49544,0.016811039983189);
#16689=CIRCLE('',#49545,0.0167157066899231);
#16690=CIRCLE('',#49546,0.0166699934630661);
#16691=CIRCLE('',#49549,0.016790740140516);
#16692=CIRCLE('',#49550,0.0167556795648152);
#16693=CIRCLE('',#49551,0.0168028429611241);
#16694=CIRCLE('',#49552,0.0168141206865178);
#16695=CIRCLE('',#49553,0.0166825657986247);
#16696=CIRCLE('',#49554,0.0167388260789807);
#16697=CIRCLE('',#49555,0.0166775856883438);
#16698=CIRCLE('',#49556,0.0168013216988337);
#16699=CIRCLE('',#49557,0.0167731941308824);
#16700=CIRCLE('',#49558,0.0167927979151636);
#16701=CIRCLE('',#49559,0.0168110399829744);
#16702=CIRCLE('',#49560,0.0167157066897106);
#16703=CIRCLE('',#49561,0.0166699934627811);
#16704=CIRCLE('',#49564,0.0167907401403223);
#16705=CIRCLE('',#49565,0.0167556795648479);
#16706=CIRCLE('',#49566,0.0168028429613066);
#16707=CIRCLE('',#49567,0.0168141206867935);
#16708=CIRCLE('',#49568,0.016682565798211);
#16709=CIRCLE('',#49569,0.0167388260791185);
#16710=CIRCLE('',#49570,0.0166775856879496);
#16711=CIRCLE('',#49571,0.0168013216997423);
#16712=CIRCLE('',#49572,0.0167731941268201);
#16713=CIRCLE('',#49573,0.0167927979157175);
#16714=CIRCLE('',#49574,0.0168110399830299);
#16715=CIRCLE('',#49575,0.0167157066894611);
#16716=CIRCLE('',#49576,0.0166699934627715);
#16717=CIRCLE('',#49579,0.0167907401406675);
#16718=CIRCLE('',#49580,0.0167556795651135);
#16719=CIRCLE('',#49581,0.0168028429611185);
#16720=CIRCLE('',#49582,0.0168141206868113);
#16721=CIRCLE('',#49583,0.0166825657981354);
#16722=CIRCLE('',#49584,0.016738826078842);
#16723=CIRCLE('',#49585,0.0166775856879909);
#16724=CIRCLE('',#49586,0.0168013216996849);
#16725=CIRCLE('',#49587,0.0167731941309764);
#16726=CIRCLE('',#49588,0.0167927979155125);
#16727=CIRCLE('',#49589,0.0168110399827123);
#16728=CIRCLE('',#49590,0.0167157066899265);
#16729=CIRCLE('',#49591,0.0166699934632962);
#16730=CIRCLE('',#49594,0.0167907401400898);
#16731=CIRCLE('',#49595,0.0167556795648269);
#16732=CIRCLE('',#49596,0.0168028429611803);
#16733=CIRCLE('',#49597,0.0168141206869151);
#16734=CIRCLE('',#49598,0.0166825657981214);
#16735=CIRCLE('',#49599,0.0167388260780384);
#16736=CIRCLE('',#49600,0.0166775856876485);
#16737=CIRCLE('',#49601,0.0168013216999341);
#16738=CIRCLE('',#49602,0.0167731941273188);
#16739=CIRCLE('',#49603,0.0167927979155007);
#16740=CIRCLE('',#49604,0.0168110399830011);
#16741=CIRCLE('',#49605,0.0167157066896642);
#16742=CIRCLE('',#49606,0.0166699934625497);
#16743=CIRCLE('',#49609,0.0167907401400955);
#16744=CIRCLE('',#49610,0.016755679564979);
#16745=CIRCLE('',#49611,0.016802842961219);
#16746=CIRCLE('',#49612,0.0168141206866368);
#16747=CIRCLE('',#49613,0.0166825657982672);
#16748=CIRCLE('',#49614,0.0167388260779614);
#16749=CIRCLE('',#49615,0.0166775856879899);
#16750=CIRCLE('',#49616,0.0168013216996006);
#16751=CIRCLE('',#49617,0.0167731941275982);
#16752=CIRCLE('',#49618,0.0167927979154729);
#16753=CIRCLE('',#49619,0.0168110399826746);
#16754=CIRCLE('',#49620,0.016715706689989);
#16755=CIRCLE('',#49621,0.0166699934626932);
#16756=CIRCLE('',#49624,0.0167907401402084);
#16757=CIRCLE('',#49625,0.0167556795648738);
#16758=CIRCLE('',#49626,0.0168028429612814);
#16759=CIRCLE('',#49627,0.0168141206866302);
#16760=CIRCLE('',#49628,0.016682565798374);
#16761=CIRCLE('',#49629,0.016738826078286);
#16762=CIRCLE('',#49630,0.0166775856882792);
#16763=CIRCLE('',#49631,0.0168013216997163);
#16764=CIRCLE('',#49632,0.0167731941269379);
#16765=CIRCLE('',#49633,0.0167927979155145);
#16766=CIRCLE('',#49634,0.0168110399830661);
#16767=CIRCLE('',#49635,0.0167157066895842);
#16768=CIRCLE('',#49636,0.016669993462965);
#16769=CIRCLE('',#49639,0.0167907401403724);
#16770=CIRCLE('',#49640,0.0167556795647631);
#16771=CIRCLE('',#49641,0.0168028429611403);
#16772=CIRCLE('',#49642,0.0168141206867779);
#16773=CIRCLE('',#49643,0.0166825657980329);
#16774=CIRCLE('',#49644,0.0167388260781292);
#16775=CIRCLE('',#49645,0.0166775856880859);
#16776=CIRCLE('',#49646,0.0168013216996242);
#16777=CIRCLE('',#49647,0.0167731941274905);
#16778=CIRCLE('',#49648,0.0167927979153934);
#16779=CIRCLE('',#49649,0.0168110399830263);
#16780=CIRCLE('',#49650,0.0167157066893938);
#16781=CIRCLE('',#49651,0.016669993463144);
#16782=CIRCLE('',#49654,0.0167907401403581);
#16783=CIRCLE('',#49655,0.0167556795646162);
#16784=CIRCLE('',#49656,0.0168028429611157);
#16785=CIRCLE('',#49657,0.0168141206868219);
#16786=CIRCLE('',#49658,0.0166825657980236);
#16787=CIRCLE('',#49659,0.0167388260788799);
#16788=CIRCLE('',#49660,0.0166775856879766);
#16789=CIRCLE('',#49661,0.0168013216995879);
#16790=CIRCLE('',#49662,0.016773194130988);
#16791=CIRCLE('',#49663,0.016792797915703);
#16792=CIRCLE('',#49664,0.0168110399831045);
#16793=CIRCLE('',#49665,0.0167157066894689);
#16794=CIRCLE('',#49666,0.0166699934630159);
#16795=CIRCLE('',#49669,0.0167907401404635);
#16796=CIRCLE('',#49670,0.0167556795646378);
#16797=CIRCLE('',#49671,0.0168028429611376);
#16798=CIRCLE('',#49672,0.0168141206868429);
#16799=CIRCLE('',#49673,0.0166825657981163);
#16800=CIRCLE('',#49674,0.0167388260782811);
#16801=CIRCLE('',#49675,0.0166775856879326);
#16802=CIRCLE('',#49676,0.0168013216998213);
#16803=CIRCLE('',#49677,0.0167731941273884);
#16804=CIRCLE('',#49678,0.0167927979156772);
#16805=CIRCLE('',#49679,0.0168110399831208);
#16806=CIRCLE('',#49680,0.0167157066895047);
#16807=CIRCLE('',#49681,0.0166699934629633);
#16808=CIRCLE('',#49684,0.0167907401403066);
#16809=CIRCLE('',#49685,0.0167556795646854);
#16810=CIRCLE('',#49686,0.0168028429612024);
#16811=CIRCLE('',#49687,0.0168141206868642);
#16812=CIRCLE('',#49688,0.0166825657981071);
#16813=CIRCLE('',#49689,0.0167388260788764);
#16814=CIRCLE('',#49690,0.0166775856879837);
#16815=CIRCLE('',#49691,0.0168013216997269);
#16816=CIRCLE('',#49692,0.0167731941275909);
#16817=CIRCLE('',#49693,0.01679279791573);
#16818=CIRCLE('',#49694,0.0168110399830354);
#16819=CIRCLE('',#49695,0.0167157066893839);
#16820=CIRCLE('',#49696,0.0166699934630788);
#16821=CIRCLE('',#49699,0.0167907401404595);
#16822=CIRCLE('',#49700,0.0167556795646726);
#16823=CIRCLE('',#49701,0.01680284296134);
#16824=CIRCLE('',#49702,0.0168141206869116);
#16825=CIRCLE('',#49703,0.0166825657980472);
#16826=CIRCLE('',#49704,0.0167388260786423);
#16827=CIRCLE('',#49705,0.0166775856880389);
#16828=CIRCLE('',#49706,0.016801321699758);
#16829=CIRCLE('',#49707,0.0167731941261841);
#16830=CIRCLE('',#49708,0.0167927979157453);
#16831=CIRCLE('',#49709,0.0168110399831073);
#16832=CIRCLE('',#49710,0.0167157066895967);
#16833=CIRCLE('',#49711,0.0166699934629367);
#16834=CIRCLE('',#49714,0.01679074014056);
#16835=CIRCLE('',#49715,0.0167556795644209);
#16836=CIRCLE('',#49716,0.016802842961138);
#16837=CIRCLE('',#49717,0.0168141206869105);
#16838=CIRCLE('',#49718,0.0166825657980409);
#16839=CIRCLE('',#49719,0.0167388260784289);
#16840=CIRCLE('',#49720,0.0166775856880623);
#16841=CIRCLE('',#49721,0.0168013216998352);
#16842=CIRCLE('',#49722,0.0167731941275654);
#16843=CIRCLE('',#49723,0.0167927979156913);
#16844=CIRCLE('',#49724,0.0168110399832004);
#16845=CIRCLE('',#49725,0.0167157066896417);
#16846=CIRCLE('',#49726,0.0166699934631642);
#16847=CIRCLE('',#49729,0.0167907401404596);
#16848=CIRCLE('',#49730,0.0167556795643878);
#16849=CIRCLE('',#49731,0.0168028429611488);
#16850=CIRCLE('',#49732,0.0168141206869211);
#16851=CIRCLE('',#49733,0.0166825657981752);
#16852=CIRCLE('',#49734,0.0167388260781587);
#16853=CIRCLE('',#49735,0.0166775856880192);
#16854=CIRCLE('',#49736,0.0168013216997431);
#16855=CIRCLE('',#49737,0.016773194127811);
#16856=CIRCLE('',#49738,0.0167927979156636);
#16857=CIRCLE('',#49739,0.0168110399832791);
#16858=CIRCLE('',#49740,0.0167157066895083);
#16859=CIRCLE('',#49741,0.0166699934633002);
#16860=CIRCLE('',#49744,0.0167907401407301);
#16861=CIRCLE('',#49745,0.0167556795646886);
#16862=CIRCLE('',#49746,0.0168028429607967);
#16863=CIRCLE('',#49747,0.0168141206869222);
#16864=CIRCLE('',#49748,0.0166825657982171);
#16865=CIRCLE('',#49749,0.0167388260786759);
#16866=CIRCLE('',#49750,0.0166775856879533);
#16867=CIRCLE('',#49751,0.0168013216996623);
#16868=CIRCLE('',#49752,0.0167731941276768);
#16869=CIRCLE('',#49753,0.0167927979160612);
#16870=CIRCLE('',#49754,0.0168110399831404);
#16871=CIRCLE('',#49755,0.0167157066895039);
#16872=CIRCLE('',#49756,0.0166699934630218);
#16873=CIRCLE('',#49759,0.0167907401403511);
#16874=CIRCLE('',#49760,0.016755679564925);
#16875=CIRCLE('',#49761,0.0168028429611863);
#16876=CIRCLE('',#49762,0.0168141206870156);
#16877=CIRCLE('',#49763,0.0166825657983043);
#16878=CIRCLE('',#49764,0.0167388260785622);
#16879=CIRCLE('',#49765,0.0166775856880007);
#16880=CIRCLE('',#49766,0.0168013216997968);
#16881=CIRCLE('',#49767,0.0167731941278823);
#16882=CIRCLE('',#49768,0.0167927979159493);
#16883=CIRCLE('',#49769,0.0168110399835583);
#16884=CIRCLE('',#49770,0.016715706689841);
#16885=CIRCLE('',#49771,0.0166699934630285);
#16886=CIRCLE('',#49772,0.0167907401418377);
#16887=CIRCLE('',#49773,0.0167556795640797);
#16888=CIRCLE('',#49776,0.0168028429612844);
#16889=CIRCLE('',#49777,0.0168141206872066);
#16890=CIRCLE('',#49778,0.0166825657981722);
#16891=CIRCLE('',#49779,0.0167388260782425);
#16892=CIRCLE('',#49780,0.0166775856877683);
#16893=CIRCLE('',#49781,0.0168013216998571);
#16894=CIRCLE('',#49782,0.016773194127473);
#16895=CIRCLE('',#49783,0.016792797915847);
#16896=CIRCLE('',#49784,0.0168110399827025);
#16897=CIRCLE('',#49785,0.0167157066896251);
#16898=CIRCLE('',#49786,0.0166699934631566);
#16899=CIRCLE('',#49789,0.0167907401405);
#16900=CIRCLE('',#49790,0.0167556795643959);
#16901=CIRCLE('',#49791,0.0168028429608355);
#16902=CIRCLE('',#49792,0.0168141206870379);
#16903=CIRCLE('',#49793,0.0166825657980907);
#16904=CIRCLE('',#49794,0.0167388260782623);
#16905=CIRCLE('',#49795,0.0166775856876276);
#16906=CIRCLE('',#49796,0.0168013216998691);
#16907=CIRCLE('',#49797,0.0167731941274095);
#16908=CIRCLE('',#49798,0.0167927979157214);
#16909=CIRCLE('',#49799,0.0168110399835694);
#16910=CIRCLE('',#49800,0.0167157066893231);
#16911=CIRCLE('',#49801,0.0166699934625659);
#16912=CIRCLE('',#49804,0.0167907401407283);
#16913=CIRCLE('',#49805,0.0167556795645328);
#16914=CIRCLE('',#49806,0.0168028429606754);
#16915=CIRCLE('',#49807,0.0168141206867869);
#16916=CIRCLE('',#49808,0.016682565797981);
#16917=CIRCLE('',#49809,0.0167388260789757);
#16918=CIRCLE('',#49810,0.0166775856879619);
#16919=CIRCLE('',#49811,0.0168013217004705);
#16920=CIRCLE('',#49812,0.0167731941274059);
#16921=CIRCLE('',#49813,0.0167927979162409);
#16922=CIRCLE('',#49814,0.0168110399829851);
#16923=CIRCLE('',#49815,0.0167157066898108);
#16924=CIRCLE('',#49816,0.0166699934630458);
#16925=CIRCLE('',#49819,0.0167907401412662);
#16926=CIRCLE('',#49820,0.0167556795648169);
#16927=CIRCLE('',#49821,0.0168028429607998);
#16928=CIRCLE('',#49822,0.0168141206873158);
#16929=CIRCLE('',#49823,0.0166825657978841);
#16930=CIRCLE('',#49824,0.0167388260784621);
#16931=CIRCLE('',#49825,0.0166775856881556);
#16932=CIRCLE('',#49826,0.0168013217001323);
#16933=CIRCLE('',#49827,0.0167731941280479);
#16934=CIRCLE('',#49828,0.0167927979162208);
#16935=CIRCLE('',#49829,0.016811039983661);
#16936=CIRCLE('',#49830,0.0167157066894465);
#16937=CIRCLE('',#49831,0.016669993463765);
#16938=CIRCLE('',#49834,0.0167907401410194);
#16939=CIRCLE('',#49835,0.0167556795644157);
#16940=CIRCLE('',#49836,0.0168028429605724);
#16941=CIRCLE('',#49837,0.0168141206871603);
#16942=CIRCLE('',#49838,0.016682565797517);
#16943=CIRCLE('',#49839,0.0167388260786104);
#16944=CIRCLE('',#49840,0.0166775856879752);
#16945=CIRCLE('',#49841,0.0168013216999819);
#16946=CIRCLE('',#49842,0.0167731941273484);
#16947=CIRCLE('',#49843,0.0167927979161244);
#16948=CIRCLE('',#49844,0.0168110399832073);
#16949=CIRCLE('',#49845,0.0167157066895601);
#16950=CIRCLE('',#49846,0.0166699934631375);
#16951=CIRCLE('',#49849,0.0167907401403971);
#16952=CIRCLE('',#49850,0.016755679564564);
#16953=CIRCLE('',#49851,0.0168028429616715);
#16954=CIRCLE('',#49852,0.0168141206866833);
#16955=CIRCLE('',#49853,0.0166825657981775);
#16956=CIRCLE('',#49854,0.0167388260789031);
#16957=CIRCLE('',#49855,0.0166775856879953);
#16958=CIRCLE('',#49856,0.016801321700032);
#16959=CIRCLE('',#49857,0.0167731941275527);
#16960=CIRCLE('',#49858,0.0167927979159458);
#16961=CIRCLE('',#49859,0.0168110399835324);
#16962=CIRCLE('',#49860,0.016715706689142);
#16963=CIRCLE('',#49861,0.0166699934637507);
#16964=CIRCLE('',#49864,0.0167907401408317);
#16965=CIRCLE('',#49865,0.0167556795649818);
#16966=CIRCLE('',#49866,0.0168028429617713);
#16967=CIRCLE('',#49867,0.0168141206868476);
#16968=CIRCLE('',#49868,0.0166825657982996);
#16969=CIRCLE('',#49869,0.0167388260788473);
#16970=CIRCLE('',#49870,0.0166775856876856);
#16971=CIRCLE('',#49871,0.0168013217002675);
#16972=CIRCLE('',#49872,0.0167731941280441);
#16973=CIRCLE('',#49873,0.0167927979160106);
#16974=CIRCLE('',#49874,0.0168110399831407);
#16975=CIRCLE('',#49875,0.0167157066898652);
#16976=CIRCLE('',#49876,0.0166699934632956);
#17225=VERTEX_POINT('',#63524);
#17226=VERTEX_POINT('',#63526);
#17227=VERTEX_POINT('',#63530);
#17228=VERTEX_POINT('',#63531);
#17229=VERTEX_POINT('',#63538);
#17230=VERTEX_POINT('',#63541);
#17231=VERTEX_POINT('',#63546);
#17232=VERTEX_POINT('',#63548);
#17233=VERTEX_POINT('',#63550);
#17234=VERTEX_POINT('',#63557);
#17235=VERTEX_POINT('',#63564);
#17236=VERTEX_POINT('',#63566);
#17237=VERTEX_POINT('',#63568);
#17238=VERTEX_POINT('',#63575);
#17239=VERTEX_POINT('',#63582);
#17240=VERTEX_POINT('',#63584);
#17241=VERTEX_POINT('',#63586);
#17242=VERTEX_POINT('',#63593);
#17243=VERTEX_POINT('',#63600);
#17244=VERTEX_POINT('',#63602);
#17245=VERTEX_POINT('',#63604);
#17246=VERTEX_POINT('',#63611);
#17247=VERTEX_POINT('',#63618);
#17248=VERTEX_POINT('',#63620);
#17249=VERTEX_POINT('',#63622);
#17250=VERTEX_POINT('',#63629);
#17251=VERTEX_POINT('',#63636);
#17252=VERTEX_POINT('',#63638);
#17253=VERTEX_POINT('',#63640);
#17254=VERTEX_POINT('',#63647);
#17255=VERTEX_POINT('',#63654);
#17256=VERTEX_POINT('',#63656);
#17257=VERTEX_POINT('',#63658);
#17258=VERTEX_POINT('',#63665);
#17259=VERTEX_POINT('',#63672);
#17260=VERTEX_POINT('',#63674);
#17261=VERTEX_POINT('',#63676);
#17262=VERTEX_POINT('',#63683);
#17263=VERTEX_POINT('',#63690);
#17264=VERTEX_POINT('',#63692);
#17265=VERTEX_POINT('',#63694);
#17266=VERTEX_POINT('',#63701);
#17267=VERTEX_POINT('',#63708);
#17268=VERTEX_POINT('',#63710);
#17269=VERTEX_POINT('',#63712);
#17270=VERTEX_POINT('',#63719);
#17271=VERTEX_POINT('',#63726);
#17272=VERTEX_POINT('',#63728);
#17273=VERTEX_POINT('',#63730);
#17274=VERTEX_POINT('',#63737);
#17275=VERTEX_POINT('',#63744);
#17276=VERTEX_POINT('',#63746);
#17277=VERTEX_POINT('',#63748);
#17278=VERTEX_POINT('',#63755);
#17279=VERTEX_POINT('',#63762);
#17280=VERTEX_POINT('',#63764);
#17281=VERTEX_POINT('',#63766);
#17282=VERTEX_POINT('',#63773);
#17283=VERTEX_POINT('',#63780);
#17284=VERTEX_POINT('',#63782);
#17285=VERTEX_POINT('',#63784);
#17286=VERTEX_POINT('',#63791);
#17287=VERTEX_POINT('',#63798);
#17288=VERTEX_POINT('',#63800);
#17289=VERTEX_POINT('',#63802);
#17290=VERTEX_POINT('',#63809);
#17291=VERTEX_POINT('',#63816);
#17292=VERTEX_POINT('',#63818);
#17293=VERTEX_POINT('',#63820);
#17294=VERTEX_POINT('',#63827);
#17295=VERTEX_POINT('',#63834);
#17296=VERTEX_POINT('',#63836);
#17297=VERTEX_POINT('',#63838);
#17298=VERTEX_POINT('',#63845);
#17299=VERTEX_POINT('',#63852);
#17300=VERTEX_POINT('',#63854);
#17301=VERTEX_POINT('',#63856);
#17302=VERTEX_POINT('',#63863);
#17303=VERTEX_POINT('',#63870);
#17304=VERTEX_POINT('',#63872);
#17305=VERTEX_POINT('',#63874);
#17306=VERTEX_POINT('',#63881);
#17307=VERTEX_POINT('',#63888);
#17308=VERTEX_POINT('',#63890);
#17309=VERTEX_POINT('',#63892);
#17310=VERTEX_POINT('',#63899);
#17311=VERTEX_POINT('',#63906);
#17312=VERTEX_POINT('',#63908);
#17313=VERTEX_POINT('',#63910);
#17314=VERTEX_POINT('',#63917);
#17315=VERTEX_POINT('',#63924);
#17316=VERTEX_POINT('',#63926);
#17317=VERTEX_POINT('',#63928);
#17318=VERTEX_POINT('',#63935);
#17319=VERTEX_POINT('',#63942);
#17320=VERTEX_POINT('',#63944);
#17321=VERTEX_POINT('',#63946);
#17322=VERTEX_POINT('',#63953);
#17323=VERTEX_POINT('',#63960);
#17324=VERTEX_POINT('',#63962);
#17325=VERTEX_POINT('',#63964);
#17326=VERTEX_POINT('',#63971);
#17327=VERTEX_POINT('',#63978);
#17328=VERTEX_POINT('',#63980);
#17329=VERTEX_POINT('',#63982);
#17330=VERTEX_POINT('',#63989);
#17331=VERTEX_POINT('',#63996);
#17332=VERTEX_POINT('',#63998);
#17333=VERTEX_POINT('',#64000);
#17334=VERTEX_POINT('',#64007);
#17335=VERTEX_POINT('',#64014);
#17336=VERTEX_POINT('',#64016);
#17337=VERTEX_POINT('',#64018);
#17338=VERTEX_POINT('',#64025);
#17339=VERTEX_POINT('',#64032);
#17340=VERTEX_POINT('',#64034);
#17341=VERTEX_POINT('',#64036);
#17342=VERTEX_POINT('',#64043);
#17343=VERTEX_POINT('',#64050);
#17344=VERTEX_POINT('',#64052);
#17345=VERTEX_POINT('',#64054);
#17346=VERTEX_POINT('',#64061);
#17347=VERTEX_POINT('',#64068);
#17348=VERTEX_POINT('',#64070);
#17349=VERTEX_POINT('',#64072);
#17350=VERTEX_POINT('',#64079);
#17351=VERTEX_POINT('',#64086);
#17352=VERTEX_POINT('',#64088);
#17353=VERTEX_POINT('',#64090);
#17354=VERTEX_POINT('',#64097);
#17355=VERTEX_POINT('',#64104);
#17356=VERTEX_POINT('',#64106);
#17357=VERTEX_POINT('',#64108);
#17358=VERTEX_POINT('',#64115);
#17359=VERTEX_POINT('',#64122);
#17360=VERTEX_POINT('',#64124);
#17361=VERTEX_POINT('',#64126);
#17362=VERTEX_POINT('',#64133);
#17363=VERTEX_POINT('',#64140);
#17364=VERTEX_POINT('',#64142);
#17365=VERTEX_POINT('',#64144);
#17366=VERTEX_POINT('',#64151);
#17367=VERTEX_POINT('',#64158);
#17368=VERTEX_POINT('',#64160);
#17369=VERTEX_POINT('',#64162);
#17370=VERTEX_POINT('',#64169);
#17371=VERTEX_POINT('',#64176);
#17372=VERTEX_POINT('',#64178);
#17373=VERTEX_POINT('',#64180);
#17374=VERTEX_POINT('',#64187);
#17375=VERTEX_POINT('',#64194);
#17376=VERTEX_POINT('',#64196);
#17377=VERTEX_POINT('',#64198);
#17378=VERTEX_POINT('',#64205);
#17379=VERTEX_POINT('',#64212);
#17380=VERTEX_POINT('',#64214);
#17381=VERTEX_POINT('',#64216);
#17382=VERTEX_POINT('',#64223);
#17383=VERTEX_POINT('',#64230);
#17384=VERTEX_POINT('',#64232);
#17385=VERTEX_POINT('',#64234);
#17386=VERTEX_POINT('',#64241);
#17387=VERTEX_POINT('',#64248);
#17388=VERTEX_POINT('',#64250);
#17389=VERTEX_POINT('',#64252);
#17390=VERTEX_POINT('',#64259);
#17391=VERTEX_POINT('',#64266);
#17392=VERTEX_POINT('',#64268);
#17393=VERTEX_POINT('',#64270);
#17394=VERTEX_POINT('',#64277);
#17395=VERTEX_POINT('',#64284);
#17396=VERTEX_POINT('',#64286);
#17397=VERTEX_POINT('',#64288);
#17398=VERTEX_POINT('',#64295);
#17399=VERTEX_POINT('',#64302);
#17400=VERTEX_POINT('',#64304);
#17401=VERTEX_POINT('',#64306);
#17402=VERTEX_POINT('',#64313);
#17403=VERTEX_POINT('',#64320);
#17404=VERTEX_POINT('',#64322);
#17405=VERTEX_POINT('',#64324);
#17406=VERTEX_POINT('',#64331);
#17407=VERTEX_POINT('',#64338);
#17408=VERTEX_POINT('',#64340);
#17409=VERTEX_POINT('',#64342);
#17410=VERTEX_POINT('',#64349);
#17411=VERTEX_POINT('',#64356);
#17412=VERTEX_POINT('',#64358);
#17413=VERTEX_POINT('',#64360);
#17414=VERTEX_POINT('',#64367);
#17415=VERTEX_POINT('',#64374);
#17416=VERTEX_POINT('',#64376);
#17417=VERTEX_POINT('',#64378);
#17418=VERTEX_POINT('',#64385);
#17419=VERTEX_POINT('',#64392);
#17420=VERTEX_POINT('',#64394);
#17421=VERTEX_POINT('',#64396);
#17422=VERTEX_POINT('',#64403);
#17423=VERTEX_POINT('',#64410);
#17424=VERTEX_POINT('',#64412);
#17425=VERTEX_POINT('',#64414);
#17426=VERTEX_POINT('',#64421);
#17427=VERTEX_POINT('',#64428);
#17428=VERTEX_POINT('',#64430);
#17429=VERTEX_POINT('',#64439);
#17430=VERTEX_POINT('',#64440);
#17431=VERTEX_POINT('',#64445);
#17432=VERTEX_POINT('',#64448);
#17433=VERTEX_POINT('',#64455);
#17434=VERTEX_POINT('',#64457);
#17435=VERTEX_POINT('',#64459);
#17436=VERTEX_POINT('',#64461);
#17437=VERTEX_POINT('',#64463);
#17438=VERTEX_POINT('',#64468);
#17439=VERTEX_POINT('',#64470);
#17440=VERTEX_POINT('',#64472);
#17441=VERTEX_POINT('',#64474);
#17442=VERTEX_POINT('',#64476);
#17443=VERTEX_POINT('',#64478);
#17444=VERTEX_POINT('',#64483);
#17445=VERTEX_POINT('',#64485);
#17446=VERTEX_POINT('',#64487);
#17447=VERTEX_POINT('',#64489);
#17448=VERTEX_POINT('',#64491);
#17449=VERTEX_POINT('',#64493);
#17450=VERTEX_POINT('',#64498);
#17451=VERTEX_POINT('',#64500);
#17452=VERTEX_POINT('',#64502);
#17453=VERTEX_POINT('',#64504);
#17454=VERTEX_POINT('',#64506);
#17455=VERTEX_POINT('',#64508);
#17456=VERTEX_POINT('',#64513);
#17457=VERTEX_POINT('',#64515);
#17458=VERTEX_POINT('',#64517);
#17459=VERTEX_POINT('',#64519);
#17460=VERTEX_POINT('',#64521);
#17461=VERTEX_POINT('',#64523);
#17462=VERTEX_POINT('',#64528);
#17463=VERTEX_POINT('',#64530);
#17464=VERTEX_POINT('',#64532);
#17465=VERTEX_POINT('',#64534);
#17466=VERTEX_POINT('',#64536);
#17467=VERTEX_POINT('',#64538);
#17468=VERTEX_POINT('',#64543);
#17469=VERTEX_POINT('',#64545);
#17470=VERTEX_POINT('',#64547);
#17471=VERTEX_POINT('',#64549);
#17472=VERTEX_POINT('',#64551);
#17473=VERTEX_POINT('',#64553);
#17474=VERTEX_POINT('',#64558);
#17475=VERTEX_POINT('',#64560);
#17476=VERTEX_POINT('',#64562);
#17477=VERTEX_POINT('',#64564);
#17478=VERTEX_POINT('',#64566);
#17479=VERTEX_POINT('',#64568);
#17480=VERTEX_POINT('',#64573);
#17481=VERTEX_POINT('',#64575);
#17482=VERTEX_POINT('',#64577);
#17483=VERTEX_POINT('',#64579);
#17484=VERTEX_POINT('',#64581);
#17485=VERTEX_POINT('',#64583);
#17486=VERTEX_POINT('',#64588);
#17487=VERTEX_POINT('',#64590);
#17488=VERTEX_POINT('',#64592);
#17489=VERTEX_POINT('',#64594);
#17490=VERTEX_POINT('',#64596);
#17491=VERTEX_POINT('',#64598);
#17492=VERTEX_POINT('',#64603);
#17493=VERTEX_POINT('',#64605);
#17494=VERTEX_POINT('',#64607);
#17495=VERTEX_POINT('',#64609);
#17496=VERTEX_POINT('',#64611);
#17497=VERTEX_POINT('',#64613);
#17498=VERTEX_POINT('',#64618);
#17499=VERTEX_POINT('',#64620);
#17500=VERTEX_POINT('',#64622);
#17501=VERTEX_POINT('',#64624);
#17502=VERTEX_POINT('',#64626);
#17503=VERTEX_POINT('',#64628);
#17504=VERTEX_POINT('',#64633);
#17505=VERTEX_POINT('',#64635);
#17506=VERTEX_POINT('',#64637);
#17507=VERTEX_POINT('',#64639);
#17508=VERTEX_POINT('',#64641);
#17509=VERTEX_POINT('',#64643);
#17510=VERTEX_POINT('',#64648);
#17511=VERTEX_POINT('',#64650);
#17512=VERTEX_POINT('',#64652);
#17513=VERTEX_POINT('',#64654);
#17514=VERTEX_POINT('',#64656);
#17515=VERTEX_POINT('',#64658);
#17516=VERTEX_POINT('',#64663);
#17517=VERTEX_POINT('',#64665);
#17518=VERTEX_POINT('',#64667);
#17519=VERTEX_POINT('',#64669);
#17520=VERTEX_POINT('',#64671);
#17521=VERTEX_POINT('',#64673);
#17522=VERTEX_POINT('',#64678);
#17523=VERTEX_POINT('',#64680);
#17524=VERTEX_POINT('',#64682);
#17525=VERTEX_POINT('',#64684);
#17526=VERTEX_POINT('',#64686);
#17527=VERTEX_POINT('',#64688);
#17528=VERTEX_POINT('',#64693);
#17529=VERTEX_POINT('',#64695);
#17530=VERTEX_POINT('',#64697);
#17531=VERTEX_POINT('',#64699);
#17532=VERTEX_POINT('',#64701);
#17533=VERTEX_POINT('',#64703);
#17534=VERTEX_POINT('',#64708);
#17535=VERTEX_POINT('',#64710);
#17536=VERTEX_POINT('',#64712);
#17537=VERTEX_POINT('',#64714);
#17538=VERTEX_POINT('',#64716);
#17539=VERTEX_POINT('',#64718);
#17540=VERTEX_POINT('',#64723);
#17541=VERTEX_POINT('',#64725);
#17542=VERTEX_POINT('',#64727);
#17543=VERTEX_POINT('',#64729);
#17544=VERTEX_POINT('',#64731);
#17545=VERTEX_POINT('',#64733);
#17546=VERTEX_POINT('',#64738);
#17547=VERTEX_POINT('',#64740);
#17548=VERTEX_POINT('',#64742);
#17549=VERTEX_POINT('',#64744);
#17550=VERTEX_POINT('',#64746);
#17551=VERTEX_POINT('',#64748);
#17552=VERTEX_POINT('',#64753);
#17553=VERTEX_POINT('',#64755);
#17554=VERTEX_POINT('',#64757);
#17555=VERTEX_POINT('',#64759);
#17556=VERTEX_POINT('',#64761);
#17557=VERTEX_POINT('',#64763);
#17558=VERTEX_POINT('',#64768);
#17559=VERTEX_POINT('',#64770);
#17560=VERTEX_POINT('',#64772);
#17561=VERTEX_POINT('',#64774);
#17562=VERTEX_POINT('',#64776);
#17563=VERTEX_POINT('',#64778);
#17564=VERTEX_POINT('',#64783);
#17565=VERTEX_POINT('',#64785);
#17566=VERTEX_POINT('',#64787);
#17567=VERTEX_POINT('',#64789);
#17568=VERTEX_POINT('',#64791);
#17569=VERTEX_POINT('',#64793);
#17570=VERTEX_POINT('',#64798);
#17571=VERTEX_POINT('',#64800);
#17572=VERTEX_POINT('',#64802);
#17573=VERTEX_POINT('',#64804);
#17574=VERTEX_POINT('',#64806);
#17575=VERTEX_POINT('',#64808);
#17576=VERTEX_POINT('',#64813);
#17577=VERTEX_POINT('',#64815);
#17578=VERTEX_POINT('',#64817);
#17579=VERTEX_POINT('',#64819);
#17580=VERTEX_POINT('',#64821);
#17581=VERTEX_POINT('',#64823);
#17582=VERTEX_POINT('',#64828);
#17583=VERTEX_POINT('',#64830);
#17584=VERTEX_POINT('',#64832);
#17585=VERTEX_POINT('',#64834);
#17586=VERTEX_POINT('',#64836);
#17587=VERTEX_POINT('',#64838);
#17588=VERTEX_POINT('',#64843);
#17589=VERTEX_POINT('',#64845);
#17590=VERTEX_POINT('',#64847);
#17591=VERTEX_POINT('',#64849);
#17592=VERTEX_POINT('',#64851);
#17593=VERTEX_POINT('',#64853);
#17594=VERTEX_POINT('',#64858);
#17595=VERTEX_POINT('',#64860);
#17596=VERTEX_POINT('',#64862);
#17597=VERTEX_POINT('',#64864);
#17598=VERTEX_POINT('',#64866);
#17599=VERTEX_POINT('',#64868);
#17600=VERTEX_POINT('',#64873);
#17601=VERTEX_POINT('',#64875);
#17602=VERTEX_POINT('',#64877);
#17603=VERTEX_POINT('',#64879);
#17604=VERTEX_POINT('',#64881);
#17605=VERTEX_POINT('',#64883);
#17606=VERTEX_POINT('',#64888);
#17607=VERTEX_POINT('',#64890);
#17608=VERTEX_POINT('',#64892);
#17609=VERTEX_POINT('',#64894);
#17610=VERTEX_POINT('',#64896);
#17611=VERTEX_POINT('',#64898);
#17612=VERTEX_POINT('',#64903);
#17613=VERTEX_POINT('',#64905);
#17614=VERTEX_POINT('',#64907);
#17615=VERTEX_POINT('',#64909);
#17616=VERTEX_POINT('',#64911);
#17617=VERTEX_POINT('',#64913);
#17618=VERTEX_POINT('',#64918);
#17619=VERTEX_POINT('',#64920);
#17620=VERTEX_POINT('',#64922);
#17621=VERTEX_POINT('',#64924);
#17622=VERTEX_POINT('',#64926);
#17623=VERTEX_POINT('',#64928);
#17624=VERTEX_POINT('',#64933);
#17625=VERTEX_POINT('',#64935);
#17626=VERTEX_POINT('',#64937);
#17627=VERTEX_POINT('',#64939);
#17628=VERTEX_POINT('',#64941);
#17629=VERTEX_POINT('',#64943);
#17630=VERTEX_POINT('',#64948);
#17631=VERTEX_POINT('',#64950);
#17632=VERTEX_POINT('',#64952);
#17633=VERTEX_POINT('',#64954);
#17634=VERTEX_POINT('',#64956);
#17635=VERTEX_POINT('',#64958);
#17636=VERTEX_POINT('',#64963);
#17637=VERTEX_POINT('',#64965);
#17638=VERTEX_POINT('',#64967);
#17639=VERTEX_POINT('',#64969);
#17640=VERTEX_POINT('',#64971);
#17641=VERTEX_POINT('',#64973);
#17642=VERTEX_POINT('',#64978);
#17643=VERTEX_POINT('',#64980);
#17644=VERTEX_POINT('',#64982);
#17645=VERTEX_POINT('',#64984);
#17646=VERTEX_POINT('',#64986);
#17647=VERTEX_POINT('',#64988);
#17648=VERTEX_POINT('',#64993);
#17649=VERTEX_POINT('',#64995);
#17650=VERTEX_POINT('',#64997);
#17651=VERTEX_POINT('',#64999);
#17652=VERTEX_POINT('',#65001);
#17653=VERTEX_POINT('',#65003);
#17654=VERTEX_POINT('',#65008);
#17655=VERTEX_POINT('',#65010);
#17656=VERTEX_POINT('',#65012);
#17657=VERTEX_POINT('',#65014);
#17658=VERTEX_POINT('',#65016);
#17659=VERTEX_POINT('',#65018);
#17660=VERTEX_POINT('',#65023);
#17661=VERTEX_POINT('',#65025);
#17662=VERTEX_POINT('',#65027);
#17663=VERTEX_POINT('',#65029);
#17664=VERTEX_POINT('',#65031);
#17665=VERTEX_POINT('',#65033);
#17666=VERTEX_POINT('',#65038);
#17667=VERTEX_POINT('',#65040);
#17668=VERTEX_POINT('',#65042);
#17669=VERTEX_POINT('',#65044);
#17670=VERTEX_POINT('',#65046);
#17671=VERTEX_POINT('',#65048);
#17672=VERTEX_POINT('',#65053);
#17673=VERTEX_POINT('',#65055);
#17674=VERTEX_POINT('',#65057);
#17675=VERTEX_POINT('',#65059);
#17676=VERTEX_POINT('',#65061);
#17677=VERTEX_POINT('',#65063);
#17678=VERTEX_POINT('',#65068);
#17679=VERTEX_POINT('',#65070);
#17680=VERTEX_POINT('',#65072);
#17681=VERTEX_POINT('',#65074);
#17682=VERTEX_POINT('',#65076);
#17683=VERTEX_POINT('',#65078);
#17684=VERTEX_POINT('',#65083);
#17685=VERTEX_POINT('',#65085);
#17686=VERTEX_POINT('',#65087);
#17687=VERTEX_POINT('',#65089);
#17688=VERTEX_POINT('',#65091);
#17689=VERTEX_POINT('',#65093);
#17690=VERTEX_POINT('',#65098);
#17691=VERTEX_POINT('',#65100);
#17692=VERTEX_POINT('',#65102);
#17693=VERTEX_POINT('',#65104);
#17694=VERTEX_POINT('',#65106);
#17695=VERTEX_POINT('',#65108);
#17696=VERTEX_POINT('',#65113);
#17697=VERTEX_POINT('',#65115);
#17698=VERTEX_POINT('',#65117);
#17699=VERTEX_POINT('',#65119);
#17700=VERTEX_POINT('',#65121);
#17701=VERTEX_POINT('',#65123);
#17702=VERTEX_POINT('',#65128);
#17703=VERTEX_POINT('',#65130);
#17704=VERTEX_POINT('',#65132);
#17705=VERTEX_POINT('',#65134);
#17706=VERTEX_POINT('',#65136);
#17707=VERTEX_POINT('',#65138);
#17708=VERTEX_POINT('',#65143);
#17709=VERTEX_POINT('',#65145);
#17710=VERTEX_POINT('',#65147);
#17711=VERTEX_POINT('',#65149);
#17712=VERTEX_POINT('',#65151);
#17713=VERTEX_POINT('',#65153);
#17714=VERTEX_POINT('',#65158);
#17715=VERTEX_POINT('',#65160);
#17716=VERTEX_POINT('',#65162);
#17717=VERTEX_POINT('',#65164);
#17718=VERTEX_POINT('',#65166);
#17719=VERTEX_POINT('',#65168);
#17720=VERTEX_POINT('',#65173);
#17721=VERTEX_POINT('',#65175);
#17722=VERTEX_POINT('',#65177);
#17723=VERTEX_POINT('',#65179);
#17724=VERTEX_POINT('',#65181);
#17725=VERTEX_POINT('',#65183);
#17726=VERTEX_POINT('',#65188);
#17727=VERTEX_POINT('',#65190);
#17728=VERTEX_POINT('',#65192);
#17729=VERTEX_POINT('',#65194);
#17730=VERTEX_POINT('',#65196);
#17731=VERTEX_POINT('',#65218);
#17732=VERTEX_POINT('',#65219);
#17733=VERTEX_POINT('',#65222);
#17734=VERTEX_POINT('',#65230);
#17735=VERTEX_POINT('',#65249);
#17736=VERTEX_POINT('',#65250);
#17737=VERTEX_POINT('',#65265);
#17738=VERTEX_POINT('',#65266);
#17739=VERTEX_POINT('',#65268);
#17740=VERTEX_POINT('',#65270);
#17741=VERTEX_POINT('',#65272);
#17742=VERTEX_POINT('',#65274);
#17743=VERTEX_POINT('',#65286);
#17744=VERTEX_POINT('',#65295);
#17745=VERTEX_POINT('',#65297);
#17746=VERTEX_POINT('',#65316);
#17747=VERTEX_POINT('',#65317);
#17748=VERTEX_POINT('',#65342);
#17749=VERTEX_POINT('',#65344);
#17750=VERTEX_POINT('',#65353);
#17751=VERTEX_POINT('',#65354);
#17752=VERTEX_POINT('',#65384);
#17753=VERTEX_POINT('',#65385);
#17754=VERTEX_POINT('',#65390);
#17755=VERTEX_POINT('',#65392);
#17756=VERTEX_POINT('',#65404);
#17757=VERTEX_POINT('',#65405);
#17758=VERTEX_POINT('',#65407);
#17759=VERTEX_POINT('',#65409);
#17760=VERTEX_POINT('',#65411);
#17761=VERTEX_POINT('',#65413);
#17762=VERTEX_POINT('',#65425);
#17763=VERTEX_POINT('',#65426);
#17764=VERTEX_POINT('',#65429);
#17765=VERTEX_POINT('',#65431);
#17766=VERTEX_POINT('',#65433);
#17767=VERTEX_POINT('',#65491);
#17768=VERTEX_POINT('',#65492);
#17769=VERTEX_POINT('',#65510);
#17770=VERTEX_POINT('',#65512);
#17771=VERTEX_POINT('',#65521);
#17772=VERTEX_POINT('',#65522);
#17773=VERTEX_POINT('',#65527);
#17774=VERTEX_POINT('',#65529);
#17775=VERTEX_POINT('',#65547);
#17776=VERTEX_POINT('',#65548);
#17777=VERTEX_POINT('',#65556);
#17778=VERTEX_POINT('',#65565);
#17779=VERTEX_POINT('',#65567);
#17780=VERTEX_POINT('',#65569);
#17781=VERTEX_POINT('',#65578);
#17782=VERTEX_POINT('',#65579);
#17783=VERTEX_POINT('',#65582);
#17784=VERTEX_POINT('',#65584);
#17785=VERTEX_POINT('',#65586);
#17786=VERTEX_POINT('',#65650);
#17787=VERTEX_POINT('',#65651);
#17788=VERTEX_POINT('',#65674);
#17789=VERTEX_POINT('',#65676);
#17790=VERTEX_POINT('',#65685);
#17791=VERTEX_POINT('',#65686);
#17792=VERTEX_POINT('',#65696);
#17793=VERTEX_POINT('',#65698);
#17794=VERTEX_POINT('',#65707);
#17795=VERTEX_POINT('',#65708);
#17796=VERTEX_POINT('',#65710);
#17797=VERTEX_POINT('',#65712);
#17798=VERTEX_POINT('',#65714);
#17799=VERTEX_POINT('',#65716);
#17800=VERTEX_POINT('',#65734);
#17801=VERTEX_POINT('',#65735);
#17802=VERTEX_POINT('',#65738);
#17803=VERTEX_POINT('',#65740);
#17804=VERTEX_POINT('',#65748);
#17805=VERTEX_POINT('',#65820);
#17806=VERTEX_POINT('',#65821);
#17807=VERTEX_POINT('',#65840);
#17808=VERTEX_POINT('',#65842);
#17809=VERTEX_POINT('',#65856);
#17810=VERTEX_POINT('',#65857);
#17811=VERTEX_POINT('',#65862);
#17812=VERTEX_POINT('',#65864);
#17813=VERTEX_POINT('',#65888);
#17814=VERTEX_POINT('',#65889);
#17815=VERTEX_POINT('',#65891);
#17816=VERTEX_POINT('',#65893);
#17817=VERTEX_POINT('',#65895);
#17818=VERTEX_POINT('',#65897);
#17819=VERTEX_POINT('',#65909);
#17820=VERTEX_POINT('',#65910);
#17821=VERTEX_POINT('',#65913);
#17822=VERTEX_POINT('',#65915);
#17823=VERTEX_POINT('',#65917);
#17824=VERTEX_POINT('',#65982);
#17825=VERTEX_POINT('',#65983);
#17826=VERTEX_POINT('',#66008);
#17827=VERTEX_POINT('',#66010);
#17828=VERTEX_POINT('',#66019);
#17829=VERTEX_POINT('',#66020);
#17830=VERTEX_POINT('',#66025);
#17831=VERTEX_POINT('',#66027);
#17832=VERTEX_POINT('',#66039);
#17833=VERTEX_POINT('',#66040);
#17834=VERTEX_POINT('',#66042);
#17835=VERTEX_POINT('',#66044);
#17836=VERTEX_POINT('',#66046);
#17837=VERTEX_POINT('',#66048);
#17838=VERTEX_POINT('',#66067);
#17839=VERTEX_POINT('',#66068);
#17840=VERTEX_POINT('',#66071);
#17841=VERTEX_POINT('',#66073);
#17842=VERTEX_POINT('',#66075);
#17843=VERTEX_POINT('',#66158);
#17844=VERTEX_POINT('',#66160);
#17845=VERTEX_POINT('',#66169);
#17846=VERTEX_POINT('',#66171);
#17847=VERTEX_POINT('',#66175);
#17848=VERTEX_POINT('',#66177);
#17849=VERTEX_POINT('',#66189);
#17850=VERTEX_POINT('',#66190);
#17851=VERTEX_POINT('',#66193);
#17852=VERTEX_POINT('',#66195);
#17853=VERTEX_POINT('',#66197);
#17854=VERTEX_POINT('',#66259);
#17855=VERTEX_POINT('',#66260);
#17856=VERTEX_POINT('',#66263);
#17857=VERTEX_POINT('',#66271);
#17858=VERTEX_POINT('',#66290);
#17859=VERTEX_POINT('',#66291);
#17860=VERTEX_POINT('',#66301);
#17861=VERTEX_POINT('',#66302);
#17862=VERTEX_POINT('',#66312);
#17863=VERTEX_POINT('',#66313);
#17864=VERTEX_POINT('',#66316);
#17865=VERTEX_POINT('',#66318);
#17866=VERTEX_POINT('',#66320);
#17867=VERTEX_POINT('',#66364);
#17868=VERTEX_POINT('',#66365);
#17869=VERTEX_POINT('',#66383);
#17870=VERTEX_POINT('',#66384);
#17871=VERTEX_POINT('',#66387);
#17872=VERTEX_POINT('',#66389);
#17873=VERTEX_POINT('',#66391);
#17874=VERTEX_POINT('',#66403);
#17875=VERTEX_POINT('',#66404);
#17876=VERTEX_POINT('',#66414);
#17877=VERTEX_POINT('',#66415);
#17878=VERTEX_POINT('',#66443);
#17879=VERTEX_POINT('',#66444);
#17880=VERTEX_POINT('',#66463);
#17881=VERTEX_POINT('',#66464);
#17882=VERTEX_POINT('',#66480);
#17883=VERTEX_POINT('',#66482);
#17884=VERTEX_POINT('',#66484);
#17885=VERTEX_POINT('',#66525);
#17886=VERTEX_POINT('',#66526);
#17887=VERTEX_POINT('',#66541);
#17888=VERTEX_POINT('',#66542);
#17889=VERTEX_POINT('',#66557);
#17890=VERTEX_POINT('',#66558);
#17891=VERTEX_POINT('',#66561);
#17892=VERTEX_POINT('',#66563);
#17893=VERTEX_POINT('',#66565);
#17894=VERTEX_POINT('',#66600);
#17895=VERTEX_POINT('',#66601);
#17896=VERTEX_POINT('',#66611);
#17897=VERTEX_POINT('',#66612);
#17898=VERTEX_POINT('',#66632);
#17899=VERTEX_POINT('',#66633);
#17900=VERTEX_POINT('',#66636);
#17901=VERTEX_POINT('',#66638);
#17902=VERTEX_POINT('',#66640);
#17903=VERTEX_POINT('',#66682);
#17904=VERTEX_POINT('',#66683);
#17905=VERTEX_POINT('',#66693);
#17906=VERTEX_POINT('',#66694);
#17907=VERTEX_POINT('',#66710);
#17908=VERTEX_POINT('',#66711);
#17909=VERTEX_POINT('',#66714);
#17910=VERTEX_POINT('',#66716);
#17911=VERTEX_POINT('',#66718);
#17912=VERTEX_POINT('',#66764);
#17913=VERTEX_POINT('',#66785);
#17914=VERTEX_POINT('',#66786);
#17915=VERTEX_POINT('',#66789);
#17916=VERTEX_POINT('',#66797);
#17917=VERTEX_POINT('',#66816);
#17918=VERTEX_POINT('',#66817);
#17919=VERTEX_POINT('',#66827);
#17920=VERTEX_POINT('',#66828);
#17921=VERTEX_POINT('',#66838);
#17922=VERTEX_POINT('',#66839);
#17923=VERTEX_POINT('',#66842);
#17924=VERTEX_POINT('',#66844);
#17925=VERTEX_POINT('',#66846);
#17926=VERTEX_POINT('',#66890);
#17927=VERTEX_POINT('',#66891);
#17928=VERTEX_POINT('',#66901);
#17929=VERTEX_POINT('',#66902);
#17930=VERTEX_POINT('',#66915);
#17931=VERTEX_POINT('',#66916);
#17932=VERTEX_POINT('',#66919);
#17933=VERTEX_POINT('',#66921);
#17934=VERTEX_POINT('',#66923);
#17935=VERTEX_POINT('',#66958);
#17936=VERTEX_POINT('',#66959);
#17937=VERTEX_POINT('',#66983);
#17938=VERTEX_POINT('',#66984);
#17939=VERTEX_POINT('',#67000);
#17940=VERTEX_POINT('',#67002);
#17941=VERTEX_POINT('',#67004);
#17942=VERTEX_POINT('',#67022);
#17943=VERTEX_POINT('',#67023);
#17944=VERTEX_POINT('',#67038);
#17945=VERTEX_POINT('',#67039);
#17946=VERTEX_POINT('',#67067);
#17947=VERTEX_POINT('',#67068);
#17948=VERTEX_POINT('',#67086);
#17949=VERTEX_POINT('',#67087);
#17950=VERTEX_POINT('',#67090);
#17951=VERTEX_POINT('',#67092);
#17952=VERTEX_POINT('',#67094);
#17953=VERTEX_POINT('',#67129);
#17954=VERTEX_POINT('',#67130);
#17955=VERTEX_POINT('',#67140);
#17956=VERTEX_POINT('',#67141);
#17957=VERTEX_POINT('',#67161);
#17958=VERTEX_POINT('',#67162);
#17959=VERTEX_POINT('',#67165);
#17960=VERTEX_POINT('',#67167);
#17961=VERTEX_POINT('',#67169);
#17962=VERTEX_POINT('',#67204);
#17963=VERTEX_POINT('',#67205);
#17964=VERTEX_POINT('',#67215);
#17965=VERTEX_POINT('',#67216);
#17966=VERTEX_POINT('',#67232);
#17967=VERTEX_POINT('',#67233);
#17968=VERTEX_POINT('',#67236);
#17969=VERTEX_POINT('',#67238);
#17970=VERTEX_POINT('',#67240);
#17971=VERTEX_POINT('',#67286);
#17972=VERTEX_POINT('',#67307);
#17973=VERTEX_POINT('',#67308);
#17974=VERTEX_POINT('',#67311);
#17975=VERTEX_POINT('',#67319);
#17976=VERTEX_POINT('',#67338);
#17977=VERTEX_POINT('',#67339);
#17978=VERTEX_POINT('',#67349);
#17979=VERTEX_POINT('',#67350);
#17980=VERTEX_POINT('',#67360);
#17981=VERTEX_POINT('',#67361);
#17982=VERTEX_POINT('',#67364);
#17983=VERTEX_POINT('',#67366);
#17984=VERTEX_POINT('',#67368);
#17985=VERTEX_POINT('',#67412);
#17986=VERTEX_POINT('',#67413);
#17987=VERTEX_POINT('',#67423);
#17988=VERTEX_POINT('',#67424);
#17989=VERTEX_POINT('',#67437);
#17990=VERTEX_POINT('',#67438);
#17991=VERTEX_POINT('',#67441);
#17992=VERTEX_POINT('',#67443);
#17993=VERTEX_POINT('',#67445);
#17994=VERTEX_POINT('',#67480);
#17995=VERTEX_POINT('',#67481);
#17996=VERTEX_POINT('',#67491);
#17997=VERTEX_POINT('',#67492);
#17998=VERTEX_POINT('',#67511);
#17999=VERTEX_POINT('',#67512);
#18000=VERTEX_POINT('',#67528);
#18001=VERTEX_POINT('',#67530);
#18002=VERTEX_POINT('',#67532);
#18003=VERTEX_POINT('',#67573);
#18004=VERTEX_POINT('',#67574);
#18005=VERTEX_POINT('',#67597);
#18006=VERTEX_POINT('',#67598);
#18007=VERTEX_POINT('',#67601);
#18008=VERTEX_POINT('',#67603);
#18009=VERTEX_POINT('',#67605);
#18010=VERTEX_POINT('',#67617);
#18011=VERTEX_POINT('',#67618);
#18012=VERTEX_POINT('',#67628);
#18013=VERTEX_POINT('',#67629);
#18014=VERTEX_POINT('',#67662);
#18015=VERTEX_POINT('',#67663);
#18016=VERTEX_POINT('',#67683);
#18017=VERTEX_POINT('',#67684);
#18018=VERTEX_POINT('',#67687);
#18019=VERTEX_POINT('',#67689);
#18020=VERTEX_POINT('',#67691);
#18021=VERTEX_POINT('',#67726);
#18022=VERTEX_POINT('',#67727);
#18023=VERTEX_POINT('',#67737);
#18024=VERTEX_POINT('',#67738);
#18025=VERTEX_POINT('',#67751);
#18026=VERTEX_POINT('',#67752);
#18027=VERTEX_POINT('',#67755);
#18028=VERTEX_POINT('',#67757);
#18029=VERTEX_POINT('',#67759);
#18030=VERTEX_POINT('',#67798);
#18031=VERTEX_POINT('',#67819);
#18032=VERTEX_POINT('',#67820);
#18033=VERTEX_POINT('',#67823);
#18034=VERTEX_POINT('',#67831);
#18035=VERTEX_POINT('',#67850);
#18036=VERTEX_POINT('',#67851);
#18037=VERTEX_POINT('',#67861);
#18038=VERTEX_POINT('',#67862);
#18039=VERTEX_POINT('',#67872);
#18040=VERTEX_POINT('',#67873);
#18041=VERTEX_POINT('',#67876);
#18042=VERTEX_POINT('',#67878);
#18043=VERTEX_POINT('',#67880);
#18044=VERTEX_POINT('',#67924);
#18045=VERTEX_POINT('',#67925);
#18046=VERTEX_POINT('',#67935);
#18047=VERTEX_POINT('',#67936);
#18048=VERTEX_POINT('',#67949);
#18049=VERTEX_POINT('',#67950);
#18050=VERTEX_POINT('',#67953);
#18051=VERTEX_POINT('',#67955);
#18052=VERTEX_POINT('',#67957);
#18053=VERTEX_POINT('',#67992);
#18054=VERTEX_POINT('',#67993);
#18055=VERTEX_POINT('',#68003);
#18056=VERTEX_POINT('',#68004);
#18057=VERTEX_POINT('',#68023);
#18058=VERTEX_POINT('',#68024);
#18059=VERTEX_POINT('',#68040);
#18060=VERTEX_POINT('',#68042);
#18061=VERTEX_POINT('',#68044);
#18062=VERTEX_POINT('',#68085);
#18063=VERTEX_POINT('',#68086);
#18064=VERTEX_POINT('',#68101);
#18065=VERTEX_POINT('',#68102);
#18066=VERTEX_POINT('',#68120);
#18067=VERTEX_POINT('',#68121);
#18068=VERTEX_POINT('',#68124);
#18069=VERTEX_POINT('',#68126);
#18070=VERTEX_POINT('',#68128);
#18071=VERTEX_POINT('',#68163);
#18072=VERTEX_POINT('',#68164);
#18073=VERTEX_POINT('',#68189);
#18074=VERTEX_POINT('',#68190);
#18075=VERTEX_POINT('',#68193);
#18076=VERTEX_POINT('',#68195);
#18077=VERTEX_POINT('',#68197);
#18078=VERTEX_POINT('',#68209);
#18079=VERTEX_POINT('',#68210);
#18080=VERTEX_POINT('',#68220);
#18081=VERTEX_POINT('',#68221);
#18082=VERTEX_POINT('',#68249);
#18083=VERTEX_POINT('',#68250);
#18084=VERTEX_POINT('',#68263);
#18085=VERTEX_POINT('',#68264);
#18086=VERTEX_POINT('',#68267);
#18087=VERTEX_POINT('',#68269);
#18088=VERTEX_POINT('',#68271);
#18089=VERTEX_POINT('',#68310);
#18090=VERTEX_POINT('',#68331);
#18091=VERTEX_POINT('',#68332);
#18092=VERTEX_POINT('',#68335);
#18093=VERTEX_POINT('',#68343);
#18094=VERTEX_POINT('',#68362);
#18095=VERTEX_POINT('',#68363);
#18096=VERTEX_POINT('',#68373);
#18097=VERTEX_POINT('',#68374);
#18098=VERTEX_POINT('',#68384);
#18099=VERTEX_POINT('',#68385);
#18100=VERTEX_POINT('',#68388);
#18101=VERTEX_POINT('',#68390);
#18102=VERTEX_POINT('',#68392);
#18103=VERTEX_POINT('',#68436);
#18104=VERTEX_POINT('',#68437);
#18105=VERTEX_POINT('',#68447);
#18106=VERTEX_POINT('',#68448);
#18107=VERTEX_POINT('',#68461);
#18108=VERTEX_POINT('',#68462);
#18109=VERTEX_POINT('',#68465);
#18110=VERTEX_POINT('',#68467);
#18111=VERTEX_POINT('',#68469);
#18112=VERTEX_POINT('',#68504);
#18113=VERTEX_POINT('',#68505);
#18114=VERTEX_POINT('',#68515);
#18115=VERTEX_POINT('',#68516);
#18116=VERTEX_POINT('',#68535);
#18117=VERTEX_POINT('',#68536);
#18118=VERTEX_POINT('',#68552);
#18119=VERTEX_POINT('',#68554);
#18120=VERTEX_POINT('',#68556);
#18121=VERTEX_POINT('',#68597);
#18122=VERTEX_POINT('',#68598);
#18123=VERTEX_POINT('',#68613);
#18124=VERTEX_POINT('',#68614);
#18125=VERTEX_POINT('',#68632);
#18126=VERTEX_POINT('',#68633);
#18127=VERTEX_POINT('',#68636);
#18128=VERTEX_POINT('',#68638);
#18129=VERTEX_POINT('',#68640);
#18130=VERTEX_POINT('',#68675);
#18131=VERTEX_POINT('',#68676);
#18132=VERTEX_POINT('',#68686);
#18133=VERTEX_POINT('',#68687);
#18134=VERTEX_POINT('',#68707);
#18135=VERTEX_POINT('',#68708);
#18136=VERTEX_POINT('',#68711);
#18137=VERTEX_POINT('',#68713);
#18138=VERTEX_POINT('',#68715);
#18139=VERTEX_POINT('',#68750);
#18140=VERTEX_POINT('',#68751);
#18141=VERTEX_POINT('',#68772);
#18142=VERTEX_POINT('',#68773);
#18143=VERTEX_POINT('',#68776);
#18144=VERTEX_POINT('',#68778);
#18145=VERTEX_POINT('',#68780);
#18146=VERTEX_POINT('',#68795);
#18147=VERTEX_POINT('',#68796);
#18148=VERTEX_POINT('',#68825);
#18149=VERTEX_POINT('',#68846);
#18150=VERTEX_POINT('',#68847);
#18151=VERTEX_POINT('',#68850);
#18152=VERTEX_POINT('',#68858);
#18153=VERTEX_POINT('',#68877);
#18154=VERTEX_POINT('',#68878);
#18155=VERTEX_POINT('',#68888);
#18156=VERTEX_POINT('',#68889);
#18157=VERTEX_POINT('',#68899);
#18158=VERTEX_POINT('',#68900);
#18159=VERTEX_POINT('',#68903);
#18160=VERTEX_POINT('',#68905);
#18161=VERTEX_POINT('',#68907);
#18162=VERTEX_POINT('',#68951);
#18163=VERTEX_POINT('',#68952);
#18164=VERTEX_POINT('',#68962);
#18165=VERTEX_POINT('',#68963);
#18166=VERTEX_POINT('',#68976);
#18167=VERTEX_POINT('',#68977);
#18168=VERTEX_POINT('',#68980);
#18169=VERTEX_POINT('',#68982);
#18170=VERTEX_POINT('',#68984);
#18171=VERTEX_POINT('',#69019);
#18172=VERTEX_POINT('',#69020);
#18173=VERTEX_POINT('',#69030);
#18174=VERTEX_POINT('',#69031);
#18175=VERTEX_POINT('',#69050);
#18176=VERTEX_POINT('',#69051);
#18177=VERTEX_POINT('',#69067);
#18178=VERTEX_POINT('',#69069);
#18179=VERTEX_POINT('',#69071);
#18180=VERTEX_POINT('',#69112);
#18181=VERTEX_POINT('',#69113);
#18182=VERTEX_POINT('',#69128);
#18183=VERTEX_POINT('',#69129);
#18184=VERTEX_POINT('',#69147);
#18185=VERTEX_POINT('',#69148);
#18186=VERTEX_POINT('',#69151);
#18187=VERTEX_POINT('',#69153);
#18188=VERTEX_POINT('',#69155);
#18189=VERTEX_POINT('',#69190);
#18190=VERTEX_POINT('',#69191);
#18191=VERTEX_POINT('',#69201);
#18192=VERTEX_POINT('',#69202);
#18193=VERTEX_POINT('',#69222);
#18194=VERTEX_POINT('',#69223);
#18195=VERTEX_POINT('',#69226);
#18196=VERTEX_POINT('',#69228);
#18197=VERTEX_POINT('',#69230);
#18198=VERTEX_POINT('',#69265);
#18199=VERTEX_POINT('',#69266);
#18200=VERTEX_POINT('',#69276);
#18201=VERTEX_POINT('',#69277);
#18202=VERTEX_POINT('',#69293);
#18203=VERTEX_POINT('',#69294);
#18204=VERTEX_POINT('',#69297);
#18205=VERTEX_POINT('',#69299);
#18206=VERTEX_POINT('',#69301);
#18207=VERTEX_POINT('',#69340);
#18208=VERTEX_POINT('',#69361);
#18209=VERTEX_POINT('',#69362);
#18210=VERTEX_POINT('',#69365);
#18211=VERTEX_POINT('',#69373);
#18212=VERTEX_POINT('',#69392);
#18213=VERTEX_POINT('',#69393);
#18214=VERTEX_POINT('',#69403);
#18215=VERTEX_POINT('',#69404);
#18216=VERTEX_POINT('',#69414);
#18217=VERTEX_POINT('',#69415);
#18218=VERTEX_POINT('',#69418);
#18219=VERTEX_POINT('',#69420);
#18220=VERTEX_POINT('',#69422);
#18221=VERTEX_POINT('',#69466);
#18222=VERTEX_POINT('',#69467);
#18223=VERTEX_POINT('',#69477);
#18224=VERTEX_POINT('',#69478);
#18225=VERTEX_POINT('',#69491);
#18226=VERTEX_POINT('',#69492);
#18227=VERTEX_POINT('',#69495);
#18228=VERTEX_POINT('',#69497);
#18229=VERTEX_POINT('',#69499);
#18230=VERTEX_POINT('',#69534);
#18231=VERTEX_POINT('',#69535);
#18232=VERTEX_POINT('',#69545);
#18233=VERTEX_POINT('',#69546);
#18234=VERTEX_POINT('',#69565);
#18235=VERTEX_POINT('',#69566);
#18236=VERTEX_POINT('',#69582);
#18237=VERTEX_POINT('',#69584);
#18238=VERTEX_POINT('',#69586);
#18239=VERTEX_POINT('',#69627);
#18240=VERTEX_POINT('',#69628);
#18241=VERTEX_POINT('',#69643);
#18242=VERTEX_POINT('',#69644);
#18243=VERTEX_POINT('',#69662);
#18244=VERTEX_POINT('',#69663);
#18245=VERTEX_POINT('',#69666);
#18246=VERTEX_POINT('',#69668);
#18247=VERTEX_POINT('',#69670);
#18248=VERTEX_POINT('',#69705);
#18249=VERTEX_POINT('',#69706);
#18250=VERTEX_POINT('',#69716);
#18251=VERTEX_POINT('',#69717);
#18252=VERTEX_POINT('',#69737);
#18253=VERTEX_POINT('',#69738);
#18254=VERTEX_POINT('',#69741);
#18255=VERTEX_POINT('',#69743);
#18256=VERTEX_POINT('',#69745);
#18257=VERTEX_POINT('',#69780);
#18258=VERTEX_POINT('',#69781);
#18259=VERTEX_POINT('',#69791);
#18260=VERTEX_POINT('',#69792);
#18261=VERTEX_POINT('',#69808);
#18262=VERTEX_POINT('',#69809);
#18263=VERTEX_POINT('',#69812);
#18264=VERTEX_POINT('',#69814);
#18265=VERTEX_POINT('',#69816);
#18266=VERTEX_POINT('',#69855);
#18267=VERTEX_POINT('',#69876);
#18268=VERTEX_POINT('',#69877);
#18269=VERTEX_POINT('',#69880);
#18270=VERTEX_POINT('',#69888);
#18271=VERTEX_POINT('',#69907);
#18272=VERTEX_POINT('',#69908);
#18273=VERTEX_POINT('',#69918);
#18274=VERTEX_POINT('',#69919);
#18275=VERTEX_POINT('',#69929);
#18276=VERTEX_POINT('',#69930);
#18277=VERTEX_POINT('',#69933);
#18278=VERTEX_POINT('',#69935);
#18279=VERTEX_POINT('',#69937);
#18280=VERTEX_POINT('',#69981);
#18281=VERTEX_POINT('',#69982);
#18282=VERTEX_POINT('',#69992);
#18283=VERTEX_POINT('',#69993);
#18284=VERTEX_POINT('',#70006);
#18285=VERTEX_POINT('',#70007);
#18286=VERTEX_POINT('',#70010);
#18287=VERTEX_POINT('',#70012);
#18288=VERTEX_POINT('',#70014);
#18289=VERTEX_POINT('',#70049);
#18290=VERTEX_POINT('',#70050);
#18291=VERTEX_POINT('',#70060);
#18292=VERTEX_POINT('',#70061);
#18293=VERTEX_POINT('',#70080);
#18294=VERTEX_POINT('',#70081);
#18295=VERTEX_POINT('',#70097);
#18296=VERTEX_POINT('',#70099);
#18297=VERTEX_POINT('',#70101);
#18298=VERTEX_POINT('',#70142);
#18299=VERTEX_POINT('',#70143);
#18300=VERTEX_POINT('',#70158);
#18301=VERTEX_POINT('',#70159);
#18302=VERTEX_POINT('',#70177);
#18303=VERTEX_POINT('',#70178);
#18304=VERTEX_POINT('',#70181);
#18305=VERTEX_POINT('',#70183);
#18306=VERTEX_POINT('',#70185);
#18307=VERTEX_POINT('',#70220);
#18308=VERTEX_POINT('',#70221);
#18309=VERTEX_POINT('',#70231);
#18310=VERTEX_POINT('',#70232);
#18311=VERTEX_POINT('',#70252);
#18312=VERTEX_POINT('',#70253);
#18313=VERTEX_POINT('',#70256);
#18314=VERTEX_POINT('',#70258);
#18315=VERTEX_POINT('',#70260);
#18316=VERTEX_POINT('',#70295);
#18317=VERTEX_POINT('',#70296);
#18318=VERTEX_POINT('',#70306);
#18319=VERTEX_POINT('',#70307);
#18320=VERTEX_POINT('',#70323);
#18321=VERTEX_POINT('',#70324);
#18322=VERTEX_POINT('',#70327);
#18323=VERTEX_POINT('',#70329);
#18324=VERTEX_POINT('',#70331);
#18325=VERTEX_POINT('',#70370);
#18326=VERTEX_POINT('',#70391);
#18327=VERTEX_POINT('',#70392);
#18328=VERTEX_POINT('',#70395);
#18329=VERTEX_POINT('',#70403);
#18330=VERTEX_POINT('',#70422);
#18331=VERTEX_POINT('',#70423);
#18332=VERTEX_POINT('',#70433);
#18333=VERTEX_POINT('',#70434);
#18334=VERTEX_POINT('',#70444);
#18335=VERTEX_POINT('',#70445);
#18336=VERTEX_POINT('',#70448);
#18337=VERTEX_POINT('',#70450);
#18338=VERTEX_POINT('',#70452);
#18339=VERTEX_POINT('',#70496);
#18340=VERTEX_POINT('',#70497);
#18341=VERTEX_POINT('',#70507);
#18342=VERTEX_POINT('',#70508);
#18343=VERTEX_POINT('',#70521);
#18344=VERTEX_POINT('',#70522);
#18345=VERTEX_POINT('',#70525);
#18346=VERTEX_POINT('',#70527);
#18347=VERTEX_POINT('',#70529);
#18348=VERTEX_POINT('',#70564);
#18349=VERTEX_POINT('',#70565);
#18350=VERTEX_POINT('',#70575);
#18351=VERTEX_POINT('',#70576);
#18352=VERTEX_POINT('',#70595);
#18353=VERTEX_POINT('',#70596);
#18354=VERTEX_POINT('',#70612);
#18355=VERTEX_POINT('',#70614);
#18356=VERTEX_POINT('',#70616);
#18357=VERTEX_POINT('',#70657);
#18358=VERTEX_POINT('',#70658);
#18359=VERTEX_POINT('',#70673);
#18360=VERTEX_POINT('',#70674);
#18361=VERTEX_POINT('',#70692);
#18362=VERTEX_POINT('',#70693);
#18363=VERTEX_POINT('',#70696);
#18364=VERTEX_POINT('',#70698);
#18365=VERTEX_POINT('',#70700);
#18366=VERTEX_POINT('',#70735);
#18367=VERTEX_POINT('',#70736);
#18368=VERTEX_POINT('',#70746);
#18369=VERTEX_POINT('',#70747);
#18370=VERTEX_POINT('',#70767);
#18371=VERTEX_POINT('',#70768);
#18372=VERTEX_POINT('',#70771);
#18373=VERTEX_POINT('',#70773);
#18374=VERTEX_POINT('',#70775);
#18375=VERTEX_POINT('',#70810);
#18376=VERTEX_POINT('',#70811);
#18377=VERTEX_POINT('',#70821);
#18378=VERTEX_POINT('',#70822);
#18379=VERTEX_POINT('',#70838);
#18380=VERTEX_POINT('',#70839);
#18381=VERTEX_POINT('',#70842);
#18382=VERTEX_POINT('',#70844);
#18383=VERTEX_POINT('',#70846);
#18384=VERTEX_POINT('',#70885);
#18385=VERTEX_POINT('',#70906);
#18386=VERTEX_POINT('',#70907);
#18387=VERTEX_POINT('',#70910);
#18388=VERTEX_POINT('',#70918);
#18389=VERTEX_POINT('',#70937);
#18390=VERTEX_POINT('',#70938);
#18391=VERTEX_POINT('',#70948);
#18392=VERTEX_POINT('',#70949);
#18393=VERTEX_POINT('',#70959);
#18394=VERTEX_POINT('',#70960);
#18395=VERTEX_POINT('',#70963);
#18396=VERTEX_POINT('',#70965);
#18397=VERTEX_POINT('',#70967);
#18398=VERTEX_POINT('',#71011);
#18399=VERTEX_POINT('',#71012);
#18400=VERTEX_POINT('',#71022);
#18401=VERTEX_POINT('',#71023);
#18402=VERTEX_POINT('',#71036);
#18403=VERTEX_POINT('',#71037);
#18404=VERTEX_POINT('',#71040);
#18405=VERTEX_POINT('',#71042);
#18406=VERTEX_POINT('',#71044);
#18407=VERTEX_POINT('',#71079);
#18408=VERTEX_POINT('',#71080);
#18409=VERTEX_POINT('',#71090);
#18410=VERTEX_POINT('',#71091);
#18411=VERTEX_POINT('',#71110);
#18412=VERTEX_POINT('',#71111);
#18413=VERTEX_POINT('',#71127);
#18414=VERTEX_POINT('',#71129);
#18415=VERTEX_POINT('',#71131);
#18416=VERTEX_POINT('',#71172);
#18417=VERTEX_POINT('',#71173);
#18418=VERTEX_POINT('',#71188);
#18419=VERTEX_POINT('',#71189);
#18420=VERTEX_POINT('',#71207);
#18421=VERTEX_POINT('',#71208);
#18422=VERTEX_POINT('',#71211);
#18423=VERTEX_POINT('',#71213);
#18424=VERTEX_POINT('',#71215);
#18425=VERTEX_POINT('',#71250);
#18426=VERTEX_POINT('',#71251);
#18427=VERTEX_POINT('',#71261);
#18428=VERTEX_POINT('',#71262);
#18429=VERTEX_POINT('',#71282);
#18430=VERTEX_POINT('',#71283);
#18431=VERTEX_POINT('',#71286);
#18432=VERTEX_POINT('',#71288);
#18433=VERTEX_POINT('',#71290);
#18434=VERTEX_POINT('',#71325);
#18435=VERTEX_POINT('',#71326);
#18436=VERTEX_POINT('',#71336);
#18437=VERTEX_POINT('',#71337);
#18438=VERTEX_POINT('',#71353);
#18439=VERTEX_POINT('',#71354);
#18440=VERTEX_POINT('',#71357);
#18441=VERTEX_POINT('',#71359);
#18442=VERTEX_POINT('',#71361);
#18443=VERTEX_POINT('',#71400);
#18444=VERTEX_POINT('',#71421);
#18445=VERTEX_POINT('',#71422);
#18446=VERTEX_POINT('',#71425);
#18447=VERTEX_POINT('',#71433);
#18448=VERTEX_POINT('',#71452);
#18449=VERTEX_POINT('',#71453);
#18450=VERTEX_POINT('',#71463);
#18451=VERTEX_POINT('',#71464);
#18452=VERTEX_POINT('',#71474);
#18453=VERTEX_POINT('',#71475);
#18454=VERTEX_POINT('',#71478);
#18455=VERTEX_POINT('',#71480);
#18456=VERTEX_POINT('',#71482);
#18457=VERTEX_POINT('',#71526);
#18458=VERTEX_POINT('',#71527);
#18459=VERTEX_POINT('',#71537);
#18460=VERTEX_POINT('',#71538);
#18461=VERTEX_POINT('',#71551);
#18462=VERTEX_POINT('',#71552);
#18463=VERTEX_POINT('',#71555);
#18464=VERTEX_POINT('',#71557);
#18465=VERTEX_POINT('',#71559);
#18466=VERTEX_POINT('',#71594);
#18467=VERTEX_POINT('',#71595);
#18468=VERTEX_POINT('',#71605);
#18469=VERTEX_POINT('',#71606);
#18470=VERTEX_POINT('',#71625);
#18471=VERTEX_POINT('',#71626);
#18472=VERTEX_POINT('',#71642);
#18473=VERTEX_POINT('',#71644);
#18474=VERTEX_POINT('',#71646);
#18475=VERTEX_POINT('',#71687);
#18476=VERTEX_POINT('',#71688);
#18477=VERTEX_POINT('',#71703);
#18478=VERTEX_POINT('',#71704);
#18479=VERTEX_POINT('',#71722);
#18480=VERTEX_POINT('',#71723);
#18481=VERTEX_POINT('',#71726);
#18482=VERTEX_POINT('',#71728);
#18483=VERTEX_POINT('',#71730);
#18484=VERTEX_POINT('',#71765);
#18485=VERTEX_POINT('',#71766);
#18486=VERTEX_POINT('',#71776);
#18487=VERTEX_POINT('',#71777);
#18488=VERTEX_POINT('',#71797);
#18489=VERTEX_POINT('',#71798);
#18490=VERTEX_POINT('',#71801);
#18491=VERTEX_POINT('',#71803);
#18492=VERTEX_POINT('',#71805);
#18493=VERTEX_POINT('',#71840);
#18494=VERTEX_POINT('',#71841);
#18495=VERTEX_POINT('',#71851);
#18496=VERTEX_POINT('',#71852);
#18497=VERTEX_POINT('',#71868);
#18498=VERTEX_POINT('',#71869);
#18499=VERTEX_POINT('',#71872);
#18500=VERTEX_POINT('',#71874);
#18501=VERTEX_POINT('',#71876);
#18502=VERTEX_POINT('',#71915);
#18503=VERTEX_POINT('',#71936);
#18504=VERTEX_POINT('',#71937);
#18505=VERTEX_POINT('',#71940);
#18506=VERTEX_POINT('',#71948);
#18507=VERTEX_POINT('',#71967);
#18508=VERTEX_POINT('',#71968);
#18509=VERTEX_POINT('',#71978);
#18510=VERTEX_POINT('',#71979);
#18511=VERTEX_POINT('',#71989);
#18512=VERTEX_POINT('',#71990);
#18513=VERTEX_POINT('',#71993);
#18514=VERTEX_POINT('',#71995);
#18515=VERTEX_POINT('',#71997);
#18516=VERTEX_POINT('',#72041);
#18517=VERTEX_POINT('',#72042);
#18518=VERTEX_POINT('',#72052);
#18519=VERTEX_POINT('',#72053);
#18520=VERTEX_POINT('',#72066);
#18521=VERTEX_POINT('',#72067);
#18522=VERTEX_POINT('',#72070);
#18523=VERTEX_POINT('',#72072);
#18524=VERTEX_POINT('',#72074);
#18525=VERTEX_POINT('',#72109);
#18526=VERTEX_POINT('',#72110);
#18527=VERTEX_POINT('',#72120);
#18528=VERTEX_POINT('',#72121);
#18529=VERTEX_POINT('',#72140);
#18530=VERTEX_POINT('',#72141);
#18531=VERTEX_POINT('',#72157);
#18532=VERTEX_POINT('',#72159);
#18533=VERTEX_POINT('',#72161);
#18534=VERTEX_POINT('',#72202);
#18535=VERTEX_POINT('',#72203);
#18536=VERTEX_POINT('',#72218);
#18537=VERTEX_POINT('',#72219);
#18538=VERTEX_POINT('',#72237);
#18539=VERTEX_POINT('',#72238);
#18540=VERTEX_POINT('',#72241);
#18541=VERTEX_POINT('',#72243);
#18542=VERTEX_POINT('',#72245);
#18543=VERTEX_POINT('',#72280);
#18544=VERTEX_POINT('',#72281);
#18545=VERTEX_POINT('',#72291);
#18546=VERTEX_POINT('',#72292);
#18547=VERTEX_POINT('',#72312);
#18548=VERTEX_POINT('',#72313);
#18549=VERTEX_POINT('',#72316);
#18550=VERTEX_POINT('',#72318);
#18551=VERTEX_POINT('',#72320);
#18552=VERTEX_POINT('',#72355);
#18553=VERTEX_POINT('',#72356);
#18554=VERTEX_POINT('',#72366);
#18555=VERTEX_POINT('',#72367);
#18556=VERTEX_POINT('',#72383);
#18557=VERTEX_POINT('',#72384);
#18558=VERTEX_POINT('',#72387);
#18559=VERTEX_POINT('',#72389);
#18560=VERTEX_POINT('',#72391);
#18561=VERTEX_POINT('',#72430);
#18562=VERTEX_POINT('',#72451);
#18563=VERTEX_POINT('',#72452);
#18564=VERTEX_POINT('',#72455);
#18565=VERTEX_POINT('',#72463);
#18566=VERTEX_POINT('',#72482);
#18567=VERTEX_POINT('',#72483);
#18568=VERTEX_POINT('',#72493);
#18569=VERTEX_POINT('',#72494);
#18570=VERTEX_POINT('',#72504);
#18571=VERTEX_POINT('',#72505);
#18572=VERTEX_POINT('',#72508);
#18573=VERTEX_POINT('',#72510);
#18574=VERTEX_POINT('',#72512);
#18575=VERTEX_POINT('',#72556);
#18576=VERTEX_POINT('',#72557);
#18577=VERTEX_POINT('',#72567);
#18578=VERTEX_POINT('',#72568);
#18579=VERTEX_POINT('',#72581);
#18580=VERTEX_POINT('',#72582);
#18581=VERTEX_POINT('',#72585);
#18582=VERTEX_POINT('',#72587);
#18583=VERTEX_POINT('',#72589);
#18584=VERTEX_POINT('',#72624);
#18585=VERTEX_POINT('',#72625);
#18586=VERTEX_POINT('',#72635);
#18587=VERTEX_POINT('',#72636);
#18588=VERTEX_POINT('',#72655);
#18589=VERTEX_POINT('',#72656);
#18590=VERTEX_POINT('',#72672);
#18591=VERTEX_POINT('',#72674);
#18592=VERTEX_POINT('',#72676);
#18593=VERTEX_POINT('',#72717);
#18594=VERTEX_POINT('',#72718);
#18595=VERTEX_POINT('',#72733);
#18596=VERTEX_POINT('',#72734);
#18597=VERTEX_POINT('',#72752);
#18598=VERTEX_POINT('',#72753);
#18599=VERTEX_POINT('',#72756);
#18600=VERTEX_POINT('',#72758);
#18601=VERTEX_POINT('',#72760);
#18602=VERTEX_POINT('',#72795);
#18603=VERTEX_POINT('',#72796);
#18604=VERTEX_POINT('',#72806);
#18605=VERTEX_POINT('',#72807);
#18606=VERTEX_POINT('',#72827);
#18607=VERTEX_POINT('',#72828);
#18608=VERTEX_POINT('',#72831);
#18609=VERTEX_POINT('',#72833);
#18610=VERTEX_POINT('',#72835);
#18611=VERTEX_POINT('',#72870);
#18612=VERTEX_POINT('',#72871);
#18613=VERTEX_POINT('',#72881);
#18614=VERTEX_POINT('',#72882);
#18615=VERTEX_POINT('',#72898);
#18616=VERTEX_POINT('',#72899);
#18617=VERTEX_POINT('',#72902);
#18618=VERTEX_POINT('',#72904);
#18619=VERTEX_POINT('',#72906);
#18620=VERTEX_POINT('',#72945);
#18621=VERTEX_POINT('',#72966);
#18622=VERTEX_POINT('',#72967);
#18623=VERTEX_POINT('',#72970);
#18624=VERTEX_POINT('',#72978);
#18625=VERTEX_POINT('',#72997);
#18626=VERTEX_POINT('',#72998);
#18627=VERTEX_POINT('',#73008);
#18628=VERTEX_POINT('',#73009);
#18629=VERTEX_POINT('',#73019);
#18630=VERTEX_POINT('',#73020);
#18631=VERTEX_POINT('',#73023);
#18632=VERTEX_POINT('',#73025);
#18633=VERTEX_POINT('',#73027);
#18634=VERTEX_POINT('',#73071);
#18635=VERTEX_POINT('',#73072);
#18636=VERTEX_POINT('',#73082);
#18637=VERTEX_POINT('',#73083);
#18638=VERTEX_POINT('',#73093);
#18639=VERTEX_POINT('',#73094);
#18640=VERTEX_POINT('',#73097);
#18641=VERTEX_POINT('',#73099);
#18642=VERTEX_POINT('',#73101);
#18643=VERTEX_POINT('',#73143);
#18644=VERTEX_POINT('',#73144);
#18645=VERTEX_POINT('',#73154);
#18646=VERTEX_POINT('',#73155);
#18647=VERTEX_POINT('',#73174);
#18648=VERTEX_POINT('',#73175);
#18649=VERTEX_POINT('',#73191);
#18650=VERTEX_POINT('',#73193);
#18651=VERTEX_POINT('',#73195);
#18652=VERTEX_POINT('',#73236);
#18653=VERTEX_POINT('',#73237);
#18654=VERTEX_POINT('',#73252);
#18655=VERTEX_POINT('',#73253);
#18656=VERTEX_POINT('',#73271);
#18657=VERTEX_POINT('',#73272);
#18658=VERTEX_POINT('',#73275);
#18659=VERTEX_POINT('',#73277);
#18660=VERTEX_POINT('',#73279);
#18661=VERTEX_POINT('',#73314);
#18662=VERTEX_POINT('',#73315);
#18663=VERTEX_POINT('',#73325);
#18664=VERTEX_POINT('',#73326);
#18665=VERTEX_POINT('',#73346);
#18666=VERTEX_POINT('',#73347);
#18667=VERTEX_POINT('',#73350);
#18668=VERTEX_POINT('',#73352);
#18669=VERTEX_POINT('',#73354);
#18670=VERTEX_POINT('',#73389);
#18671=VERTEX_POINT('',#73390);
#18672=VERTEX_POINT('',#73400);
#18673=VERTEX_POINT('',#73401);
#18674=VERTEX_POINT('',#73417);
#18675=VERTEX_POINT('',#73418);
#18676=VERTEX_POINT('',#73421);
#18677=VERTEX_POINT('',#73423);
#18678=VERTEX_POINT('',#73425);
#18679=VERTEX_POINT('',#73464);
#18680=VERTEX_POINT('',#73485);
#18681=VERTEX_POINT('',#73486);
#18682=VERTEX_POINT('',#73489);
#18683=VERTEX_POINT('',#73497);
#18684=VERTEX_POINT('',#73516);
#18685=VERTEX_POINT('',#73517);
#18686=VERTEX_POINT('',#73527);
#18687=VERTEX_POINT('',#73528);
#18688=VERTEX_POINT('',#73538);
#18689=VERTEX_POINT('',#73539);
#18690=VERTEX_POINT('',#73542);
#18691=VERTEX_POINT('',#73544);
#18692=VERTEX_POINT('',#73546);
#18693=VERTEX_POINT('',#73590);
#18694=VERTEX_POINT('',#73591);
#18695=VERTEX_POINT('',#73601);
#18696=VERTEX_POINT('',#73602);
#18697=VERTEX_POINT('',#73615);
#18698=VERTEX_POINT('',#73616);
#18699=VERTEX_POINT('',#73619);
#18700=VERTEX_POINT('',#73621);
#18701=VERTEX_POINT('',#73623);
#18702=VERTEX_POINT('',#73658);
#18703=VERTEX_POINT('',#73659);
#18704=VERTEX_POINT('',#73669);
#18705=VERTEX_POINT('',#73670);
#18706=VERTEX_POINT('',#73689);
#18707=VERTEX_POINT('',#73690);
#18708=VERTEX_POINT('',#73706);
#18709=VERTEX_POINT('',#73708);
#18710=VERTEX_POINT('',#73710);
#18711=VERTEX_POINT('',#73751);
#18712=VERTEX_POINT('',#73752);
#18713=VERTEX_POINT('',#73767);
#18714=VERTEX_POINT('',#73768);
#18715=VERTEX_POINT('',#73786);
#18716=VERTEX_POINT('',#73787);
#18717=VERTEX_POINT('',#73790);
#18718=VERTEX_POINT('',#73792);
#18719=VERTEX_POINT('',#73794);
#18720=VERTEX_POINT('',#73829);
#18721=VERTEX_POINT('',#73830);
#18722=VERTEX_POINT('',#73840);
#18723=VERTEX_POINT('',#73841);
#18724=VERTEX_POINT('',#73861);
#18725=VERTEX_POINT('',#73862);
#18726=VERTEX_POINT('',#73865);
#18727=VERTEX_POINT('',#73867);
#18728=VERTEX_POINT('',#73869);
#18729=VERTEX_POINT('',#73904);
#18730=VERTEX_POINT('',#73905);
#18731=VERTEX_POINT('',#73915);
#18732=VERTEX_POINT('',#73916);
#18733=VERTEX_POINT('',#73932);
#18734=VERTEX_POINT('',#73933);
#18735=VERTEX_POINT('',#73936);
#18736=VERTEX_POINT('',#73938);
#18737=VERTEX_POINT('',#73940);
#18738=VERTEX_POINT('',#73979);
#18739=VERTEX_POINT('',#74000);
#18740=VERTEX_POINT('',#74001);
#18741=VERTEX_POINT('',#74004);
#18742=VERTEX_POINT('',#74012);
#18743=VERTEX_POINT('',#74031);
#18744=VERTEX_POINT('',#74032);
#18745=VERTEX_POINT('',#74042);
#18746=VERTEX_POINT('',#74043);
#18747=VERTEX_POINT('',#74053);
#18748=VERTEX_POINT('',#74054);
#18749=VERTEX_POINT('',#74057);
#18750=VERTEX_POINT('',#74059);
#18751=VERTEX_POINT('',#74061);
#18752=VERTEX_POINT('',#74105);
#18753=VERTEX_POINT('',#74106);
#18754=VERTEX_POINT('',#74116);
#18755=VERTEX_POINT('',#74117);
#18756=VERTEX_POINT('',#74130);
#18757=VERTEX_POINT('',#74131);
#18758=VERTEX_POINT('',#74134);
#18759=VERTEX_POINT('',#74136);
#18760=VERTEX_POINT('',#74138);
#18761=VERTEX_POINT('',#74173);
#18762=VERTEX_POINT('',#74174);
#18763=VERTEX_POINT('',#74184);
#18764=VERTEX_POINT('',#74185);
#18765=VERTEX_POINT('',#74204);
#18766=VERTEX_POINT('',#74205);
#18767=VERTEX_POINT('',#74221);
#18768=VERTEX_POINT('',#74223);
#18769=VERTEX_POINT('',#74225);
#18770=VERTEX_POINT('',#74266);
#18771=VERTEX_POINT('',#74267);
#18772=VERTEX_POINT('',#74282);
#18773=VERTEX_POINT('',#74283);
#18774=VERTEX_POINT('',#74301);
#18775=VERTEX_POINT('',#74302);
#18776=VERTEX_POINT('',#74305);
#18777=VERTEX_POINT('',#74307);
#18778=VERTEX_POINT('',#74309);
#18779=VERTEX_POINT('',#74344);
#18780=VERTEX_POINT('',#74345);
#18781=VERTEX_POINT('',#74355);
#18782=VERTEX_POINT('',#74356);
#18783=VERTEX_POINT('',#74376);
#18784=VERTEX_POINT('',#74377);
#18785=VERTEX_POINT('',#74380);
#18786=VERTEX_POINT('',#74382);
#18787=VERTEX_POINT('',#74384);
#18788=VERTEX_POINT('',#74419);
#18789=VERTEX_POINT('',#74420);
#18790=VERTEX_POINT('',#74430);
#18791=VERTEX_POINT('',#74431);
#18792=VERTEX_POINT('',#74447);
#18793=VERTEX_POINT('',#74448);
#18794=VERTEX_POINT('',#74451);
#18795=VERTEX_POINT('',#74453);
#18796=VERTEX_POINT('',#74455);
#18797=VERTEX_POINT('',#74494);
#18798=VERTEX_POINT('',#74515);
#18799=VERTEX_POINT('',#74516);
#18800=VERTEX_POINT('',#74519);
#18801=VERTEX_POINT('',#74527);
#18802=VERTEX_POINT('',#74546);
#18803=VERTEX_POINT('',#74547);
#18804=VERTEX_POINT('',#74557);
#18805=VERTEX_POINT('',#74558);
#18806=VERTEX_POINT('',#74568);
#18807=VERTEX_POINT('',#74569);
#18808=VERTEX_POINT('',#74572);
#18809=VERTEX_POINT('',#74574);
#18810=VERTEX_POINT('',#74576);
#18811=VERTEX_POINT('',#74620);
#18812=VERTEX_POINT('',#74621);
#18813=VERTEX_POINT('',#74631);
#18814=VERTEX_POINT('',#74632);
#18815=VERTEX_POINT('',#74645);
#18816=VERTEX_POINT('',#74646);
#18817=VERTEX_POINT('',#74649);
#18818=VERTEX_POINT('',#74651);
#18819=VERTEX_POINT('',#74653);
#18820=VERTEX_POINT('',#74688);
#18821=VERTEX_POINT('',#74689);
#18822=VERTEX_POINT('',#74699);
#18823=VERTEX_POINT('',#74700);
#18824=VERTEX_POINT('',#74719);
#18825=VERTEX_POINT('',#74720);
#18826=VERTEX_POINT('',#74736);
#18827=VERTEX_POINT('',#74738);
#18828=VERTEX_POINT('',#74740);
#18829=VERTEX_POINT('',#74781);
#18830=VERTEX_POINT('',#74782);
#18831=VERTEX_POINT('',#74797);
#18832=VERTEX_POINT('',#74798);
#18833=VERTEX_POINT('',#74816);
#18834=VERTEX_POINT('',#74817);
#18835=VERTEX_POINT('',#74820);
#18836=VERTEX_POINT('',#74822);
#18837=VERTEX_POINT('',#74824);
#18838=VERTEX_POINT('',#74859);
#18839=VERTEX_POINT('',#74860);
#18840=VERTEX_POINT('',#74870);
#18841=VERTEX_POINT('',#74871);
#18842=VERTEX_POINT('',#74891);
#18843=VERTEX_POINT('',#74892);
#18844=VERTEX_POINT('',#74895);
#18845=VERTEX_POINT('',#74897);
#18846=VERTEX_POINT('',#74899);
#18847=VERTEX_POINT('',#74934);
#18848=VERTEX_POINT('',#74935);
#18849=VERTEX_POINT('',#74945);
#18850=VERTEX_POINT('',#74946);
#18851=VERTEX_POINT('',#74962);
#18852=VERTEX_POINT('',#74963);
#18853=VERTEX_POINT('',#74966);
#18854=VERTEX_POINT('',#74968);
#18855=VERTEX_POINT('',#74970);
#18856=VERTEX_POINT('',#75009);
#18857=VERTEX_POINT('',#75030);
#18858=VERTEX_POINT('',#75031);
#18859=VERTEX_POINT('',#75034);
#18860=VERTEX_POINT('',#75042);
#18861=VERTEX_POINT('',#75061);
#18862=VERTEX_POINT('',#75062);
#18863=VERTEX_POINT('',#75072);
#18864=VERTEX_POINT('',#75073);
#18865=VERTEX_POINT('',#75083);
#18866=VERTEX_POINT('',#75084);
#18867=VERTEX_POINT('',#75087);
#18868=VERTEX_POINT('',#75089);
#18869=VERTEX_POINT('',#75091);
#18870=VERTEX_POINT('',#75135);
#18871=VERTEX_POINT('',#75136);
#18872=VERTEX_POINT('',#75146);
#18873=VERTEX_POINT('',#75147);
#18874=VERTEX_POINT('',#75160);
#18875=VERTEX_POINT('',#75161);
#18876=VERTEX_POINT('',#75164);
#18877=VERTEX_POINT('',#75166);
#18878=VERTEX_POINT('',#75168);
#18879=VERTEX_POINT('',#75203);
#18880=VERTEX_POINT('',#75204);
#18881=VERTEX_POINT('',#75214);
#18882=VERTEX_POINT('',#75215);
#18883=VERTEX_POINT('',#75234);
#18884=VERTEX_POINT('',#75235);
#18885=VERTEX_POINT('',#75251);
#18886=VERTEX_POINT('',#75253);
#18887=VERTEX_POINT('',#75255);
#18888=VERTEX_POINT('',#75296);
#18889=VERTEX_POINT('',#75297);
#18890=VERTEX_POINT('',#75312);
#18891=VERTEX_POINT('',#75313);
#18892=VERTEX_POINT('',#75331);
#18893=VERTEX_POINT('',#75332);
#18894=VERTEX_POINT('',#75335);
#18895=VERTEX_POINT('',#75337);
#18896=VERTEX_POINT('',#75339);
#18897=VERTEX_POINT('',#75374);
#18898=VERTEX_POINT('',#75375);
#18899=VERTEX_POINT('',#75385);
#18900=VERTEX_POINT('',#75386);
#18901=VERTEX_POINT('',#75406);
#18902=VERTEX_POINT('',#75407);
#18903=VERTEX_POINT('',#75410);
#18904=VERTEX_POINT('',#75412);
#18905=VERTEX_POINT('',#75414);
#18906=VERTEX_POINT('',#75449);
#18907=VERTEX_POINT('',#75450);
#18908=VERTEX_POINT('',#75460);
#18909=VERTEX_POINT('',#75461);
#18910=VERTEX_POINT('',#75477);
#18911=VERTEX_POINT('',#75478);
#18912=VERTEX_POINT('',#75481);
#18913=VERTEX_POINT('',#75483);
#18914=VERTEX_POINT('',#75485);
#18915=VERTEX_POINT('',#75524);
#18916=VERTEX_POINT('',#75545);
#18917=VERTEX_POINT('',#75546);
#18918=VERTEX_POINT('',#75549);
#18919=VERTEX_POINT('',#75557);
#18920=VERTEX_POINT('',#75576);
#18921=VERTEX_POINT('',#75577);
#18922=VERTEX_POINT('',#75587);
#18923=VERTEX_POINT('',#75588);
#18924=VERTEX_POINT('',#75598);
#18925=VERTEX_POINT('',#75599);
#18926=VERTEX_POINT('',#75602);
#18927=VERTEX_POINT('',#75604);
#18928=VERTEX_POINT('',#75606);
#18929=VERTEX_POINT('',#75650);
#18930=VERTEX_POINT('',#75651);
#18931=VERTEX_POINT('',#75661);
#18932=VERTEX_POINT('',#75662);
#18933=VERTEX_POINT('',#75672);
#18934=VERTEX_POINT('',#75673);
#18935=VERTEX_POINT('',#75676);
#18936=VERTEX_POINT('',#75678);
#18937=VERTEX_POINT('',#75680);
#18938=VERTEX_POINT('',#75722);
#18939=VERTEX_POINT('',#75723);
#18940=VERTEX_POINT('',#75733);
#18941=VERTEX_POINT('',#75734);
#18942=VERTEX_POINT('',#75753);
#18943=VERTEX_POINT('',#75754);
#18944=VERTEX_POINT('',#75770);
#18945=VERTEX_POINT('',#75772);
#18946=VERTEX_POINT('',#75774);
#18947=VERTEX_POINT('',#75815);
#18948=VERTEX_POINT('',#75816);
#18949=VERTEX_POINT('',#75831);
#18950=VERTEX_POINT('',#75832);
#18951=VERTEX_POINT('',#75850);
#18952=VERTEX_POINT('',#75851);
#18953=VERTEX_POINT('',#75854);
#18954=VERTEX_POINT('',#75856);
#18955=VERTEX_POINT('',#75858);
#18956=VERTEX_POINT('',#75893);
#18957=VERTEX_POINT('',#75894);
#18958=VERTEX_POINT('',#75904);
#18959=VERTEX_POINT('',#75905);
#18960=VERTEX_POINT('',#75925);
#18961=VERTEX_POINT('',#75926);
#18962=VERTEX_POINT('',#75929);
#18963=VERTEX_POINT('',#75931);
#18964=VERTEX_POINT('',#75933);
#18965=VERTEX_POINT('',#75968);
#18966=VERTEX_POINT('',#75969);
#18967=VERTEX_POINT('',#75979);
#18968=VERTEX_POINT('',#75980);
#18969=VERTEX_POINT('',#75996);
#18970=VERTEX_POINT('',#75997);
#18971=VERTEX_POINT('',#76000);
#18972=VERTEX_POINT('',#76002);
#18973=VERTEX_POINT('',#76004);
#18974=VERTEX_POINT('',#76043);
#18975=VERTEX_POINT('',#76064);
#18976=VERTEX_POINT('',#76065);
#18977=VERTEX_POINT('',#76068);
#18978=VERTEX_POINT('',#76076);
#18979=VERTEX_POINT('',#76095);
#18980=VERTEX_POINT('',#76096);
#18981=VERTEX_POINT('',#76106);
#18982=VERTEX_POINT('',#76107);
#18983=VERTEX_POINT('',#76117);
#18984=VERTEX_POINT('',#76118);
#18985=VERTEX_POINT('',#76121);
#18986=VERTEX_POINT('',#76123);
#18987=VERTEX_POINT('',#76125);
#18988=VERTEX_POINT('',#76169);
#18989=VERTEX_POINT('',#76170);
#18990=VERTEX_POINT('',#76180);
#18991=VERTEX_POINT('',#76181);
#18992=VERTEX_POINT('',#76194);
#18993=VERTEX_POINT('',#76195);
#18994=VERTEX_POINT('',#76198);
#18995=VERTEX_POINT('',#76200);
#18996=VERTEX_POINT('',#76202);
#18997=VERTEX_POINT('',#76237);
#18998=VERTEX_POINT('',#76238);
#18999=VERTEX_POINT('',#76248);
#19000=VERTEX_POINT('',#76249);
#19001=VERTEX_POINT('',#76269);
#19002=VERTEX_POINT('',#76270);
#19003=VERTEX_POINT('',#76284);
#19004=VERTEX_POINT('',#76286);
#19005=VERTEX_POINT('',#76288);
#19006=VERTEX_POINT('',#76324);
#19007=VERTEX_POINT('',#76325);
#19008=VERTEX_POINT('',#76340);
#19009=VERTEX_POINT('',#76341);
#19010=VERTEX_POINT('',#76359);
#19011=VERTEX_POINT('',#76360);
#19012=VERTEX_POINT('',#76363);
#19013=VERTEX_POINT('',#76365);
#19014=VERTEX_POINT('',#76367);
#19015=VERTEX_POINT('',#76402);
#19016=VERTEX_POINT('',#76403);
#19017=VERTEX_POINT('',#76413);
#19018=VERTEX_POINT('',#76414);
#19019=VERTEX_POINT('',#76434);
#19020=VERTEX_POINT('',#76435);
#19021=VERTEX_POINT('',#76438);
#19022=VERTEX_POINT('',#76440);
#19023=VERTEX_POINT('',#76442);
#19024=VERTEX_POINT('',#76477);
#19025=VERTEX_POINT('',#76478);
#19026=VERTEX_POINT('',#76488);
#19027=VERTEX_POINT('',#76489);
#19028=VERTEX_POINT('',#76505);
#19029=VERTEX_POINT('',#76506);
#19030=VERTEX_POINT('',#76509);
#19031=VERTEX_POINT('',#76511);
#19032=VERTEX_POINT('',#76513);
#19033=VERTEX_POINT('',#76552);
#19034=VERTEX_POINT('',#76573);
#19035=VERTEX_POINT('',#76574);
#19036=VERTEX_POINT('',#76577);
#19037=VERTEX_POINT('',#76585);
#19038=VERTEX_POINT('',#76604);
#19039=VERTEX_POINT('',#76605);
#19040=VERTEX_POINT('',#76615);
#19041=VERTEX_POINT('',#76616);
#19042=VERTEX_POINT('',#76626);
#19043=VERTEX_POINT('',#76627);
#19044=VERTEX_POINT('',#76630);
#19045=VERTEX_POINT('',#76632);
#19046=VERTEX_POINT('',#76634);
#19047=VERTEX_POINT('',#76678);
#19048=VERTEX_POINT('',#76679);
#19049=VERTEX_POINT('',#76689);
#19050=VERTEX_POINT('',#76690);
#19051=VERTEX_POINT('',#76700);
#19052=VERTEX_POINT('',#76701);
#19053=VERTEX_POINT('',#76704);
#19054=VERTEX_POINT('',#76706);
#19055=VERTEX_POINT('',#76708);
#19056=VERTEX_POINT('',#76750);
#19057=VERTEX_POINT('',#76751);
#19058=VERTEX_POINT('',#76761);
#19059=VERTEX_POINT('',#76762);
#19060=VERTEX_POINT('',#76781);
#19061=VERTEX_POINT('',#76782);
#19062=VERTEX_POINT('',#76798);
#19063=VERTEX_POINT('',#76800);
#19064=VERTEX_POINT('',#76802);
#19065=VERTEX_POINT('',#76843);
#19066=VERTEX_POINT('',#76844);
#19067=VERTEX_POINT('',#76859);
#19068=VERTEX_POINT('',#76860);
#19069=VERTEX_POINT('',#76875);
#19070=VERTEX_POINT('',#76876);
#19071=VERTEX_POINT('',#76879);
#19072=VERTEX_POINT('',#76881);
#19073=VERTEX_POINT('',#76883);
#19074=VERTEX_POINT('',#76925);
#19075=VERTEX_POINT('',#76926);
#19076=VERTEX_POINT('',#76936);
#19077=VERTEX_POINT('',#76937);
#19078=VERTEX_POINT('',#76957);
#19079=VERTEX_POINT('',#76958);
#19080=VERTEX_POINT('',#76961);
#19081=VERTEX_POINT('',#76963);
#19082=VERTEX_POINT('',#76965);
#19083=VERTEX_POINT('',#77000);
#19084=VERTEX_POINT('',#77001);
#19085=VERTEX_POINT('',#77011);
#19086=VERTEX_POINT('',#77012);
#19087=VERTEX_POINT('',#77028);
#19088=VERTEX_POINT('',#77029);
#19089=VERTEX_POINT('',#77032);
#19090=VERTEX_POINT('',#77034);
#19091=VERTEX_POINT('',#77036);
#19092=VERTEX_POINT('',#77075);
#19093=VERTEX_POINT('',#77096);
#19094=VERTEX_POINT('',#77097);
#19095=VERTEX_POINT('',#77100);
#19096=VERTEX_POINT('',#77108);
#19097=VERTEX_POINT('',#77127);
#19098=VERTEX_POINT('',#77128);
#19099=VERTEX_POINT('',#77138);
#19100=VERTEX_POINT('',#77139);
#19101=VERTEX_POINT('',#77149);
#19102=VERTEX_POINT('',#77150);
#19103=VERTEX_POINT('',#77153);
#19104=VERTEX_POINT('',#77155);
#19105=VERTEX_POINT('',#77157);
#19106=VERTEX_POINT('',#77201);
#19107=VERTEX_POINT('',#77202);
#19108=VERTEX_POINT('',#77212);
#19109=VERTEX_POINT('',#77213);
#19110=VERTEX_POINT('',#77226);
#19111=VERTEX_POINT('',#77227);
#19112=VERTEX_POINT('',#77230);
#19113=VERTEX_POINT('',#77232);
#19114=VERTEX_POINT('',#77234);
#19115=VERTEX_POINT('',#77269);
#19116=VERTEX_POINT('',#77270);
#19117=VERTEX_POINT('',#77280);
#19118=VERTEX_POINT('',#77281);
#19119=VERTEX_POINT('',#77300);
#19120=VERTEX_POINT('',#77301);
#19121=VERTEX_POINT('',#77317);
#19122=VERTEX_POINT('',#77319);
#19123=VERTEX_POINT('',#77321);
#19124=VERTEX_POINT('',#77362);
#19125=VERTEX_POINT('',#77363);
#19126=VERTEX_POINT('',#77378);
#19127=VERTEX_POINT('',#77379);
#19128=VERTEX_POINT('',#77397);
#19129=VERTEX_POINT('',#77398);
#19130=VERTEX_POINT('',#77401);
#19131=VERTEX_POINT('',#77403);
#19132=VERTEX_POINT('',#77405);
#19133=VERTEX_POINT('',#77440);
#19134=VERTEX_POINT('',#77441);
#19135=VERTEX_POINT('',#77451);
#19136=VERTEX_POINT('',#77452);
#19137=VERTEX_POINT('',#77472);
#19138=VERTEX_POINT('',#77473);
#19139=VERTEX_POINT('',#77476);
#19140=VERTEX_POINT('',#77478);
#19141=VERTEX_POINT('',#77480);
#19142=VERTEX_POINT('',#77522);
#19143=VERTEX_POINT('',#77523);
#19144=VERTEX_POINT('',#77533);
#19145=VERTEX_POINT('',#77534);
#19146=VERTEX_POINT('',#77550);
#19147=VERTEX_POINT('',#77551);
#19148=VERTEX_POINT('',#77554);
#19149=VERTEX_POINT('',#77556);
#19150=VERTEX_POINT('',#77558);
#19151=VERTEX_POINT('',#77597);
#19152=VERTEX_POINT('',#77618);
#19153=VERTEX_POINT('',#77619);
#19154=VERTEX_POINT('',#77622);
#19155=VERTEX_POINT('',#77630);
#19156=VERTEX_POINT('',#77649);
#19157=VERTEX_POINT('',#77650);
#19158=VERTEX_POINT('',#77660);
#19159=VERTEX_POINT('',#77661);
#19160=VERTEX_POINT('',#77671);
#19161=VERTEX_POINT('',#77672);
#19162=VERTEX_POINT('',#77675);
#19163=VERTEX_POINT('',#77677);
#19164=VERTEX_POINT('',#77679);
#19165=VERTEX_POINT('',#77723);
#19166=VERTEX_POINT('',#77724);
#19167=VERTEX_POINT('',#77734);
#19168=VERTEX_POINT('',#77735);
#19169=VERTEX_POINT('',#77748);
#19170=VERTEX_POINT('',#77749);
#19171=VERTEX_POINT('',#77752);
#19172=VERTEX_POINT('',#77754);
#19173=VERTEX_POINT('',#77756);
#19174=VERTEX_POINT('',#77791);
#19175=VERTEX_POINT('',#77792);
#19176=VERTEX_POINT('',#77802);
#19177=VERTEX_POINT('',#77803);
#19178=VERTEX_POINT('',#77822);
#19179=VERTEX_POINT('',#77823);
#19180=VERTEX_POINT('',#77839);
#19181=VERTEX_POINT('',#77841);
#19182=VERTEX_POINT('',#77843);
#19183=VERTEX_POINT('',#77884);
#19184=VERTEX_POINT('',#77885);
#19185=VERTEX_POINT('',#77900);
#19186=VERTEX_POINT('',#77901);
#19187=VERTEX_POINT('',#77919);
#19188=VERTEX_POINT('',#77920);
#19189=VERTEX_POINT('',#77923);
#19190=VERTEX_POINT('',#77925);
#19191=VERTEX_POINT('',#77927);
#19192=VERTEX_POINT('',#77962);
#19193=VERTEX_POINT('',#77963);
#19194=VERTEX_POINT('',#77973);
#19195=VERTEX_POINT('',#77974);
#19196=VERTEX_POINT('',#77994);
#19197=VERTEX_POINT('',#77995);
#19198=VERTEX_POINT('',#77998);
#19199=VERTEX_POINT('',#78000);
#19200=VERTEX_POINT('',#78002);
#19201=VERTEX_POINT('',#78037);
#19202=VERTEX_POINT('',#78038);
#19203=VERTEX_POINT('',#78048);
#19204=VERTEX_POINT('',#78049);
#19205=VERTEX_POINT('',#78062);
#19206=VERTEX_POINT('',#78063);
#19207=VERTEX_POINT('',#78066);
#19208=VERTEX_POINT('',#78068);
#19209=VERTEX_POINT('',#78070);
#19210=VERTEX_POINT('',#78116);
#19211=VERTEX_POINT('',#78137);
#19212=VERTEX_POINT('',#78138);
#19213=VERTEX_POINT('',#78141);
#19214=VERTEX_POINT('',#78149);
#19215=VERTEX_POINT('',#78168);
#19216=VERTEX_POINT('',#78169);
#19217=VERTEX_POINT('',#78179);
#19218=VERTEX_POINT('',#78180);
#19219=VERTEX_POINT('',#78190);
#19220=VERTEX_POINT('',#78191);
#19221=VERTEX_POINT('',#78194);
#19222=VERTEX_POINT('',#78196);
#19223=VERTEX_POINT('',#78198);
#19224=VERTEX_POINT('',#78242);
#19225=VERTEX_POINT('',#78243);
#19226=VERTEX_POINT('',#78253);
#19227=VERTEX_POINT('',#78254);
#19228=VERTEX_POINT('',#78267);
#19229=VERTEX_POINT('',#78268);
#19230=VERTEX_POINT('',#78271);
#19231=VERTEX_POINT('',#78273);
#19232=VERTEX_POINT('',#78275);
#19233=VERTEX_POINT('',#78310);
#19234=VERTEX_POINT('',#78311);
#19235=VERTEX_POINT('',#78321);
#19236=VERTEX_POINT('',#78322);
#19237=VERTEX_POINT('',#78341);
#19238=VERTEX_POINT('',#78342);
#19239=VERTEX_POINT('',#78358);
#19240=VERTEX_POINT('',#78360);
#19241=VERTEX_POINT('',#78362);
#19242=VERTEX_POINT('',#78403);
#19243=VERTEX_POINT('',#78404);
#19244=VERTEX_POINT('',#78419);
#19245=VERTEX_POINT('',#78420);
#19246=VERTEX_POINT('',#78438);
#19247=VERTEX_POINT('',#78439);
#19248=VERTEX_POINT('',#78442);
#19249=VERTEX_POINT('',#78444);
#19250=VERTEX_POINT('',#78446);
#19251=VERTEX_POINT('',#78481);
#19252=VERTEX_POINT('',#78482);
#19253=VERTEX_POINT('',#78492);
#19254=VERTEX_POINT('',#78493);
#19255=VERTEX_POINT('',#78513);
#19256=VERTEX_POINT('',#78514);
#19257=VERTEX_POINT('',#78517);
#19258=VERTEX_POINT('',#78519);
#19259=VERTEX_POINT('',#78521);
#19260=VERTEX_POINT('',#78556);
#19261=VERTEX_POINT('',#78557);
#19262=VERTEX_POINT('',#78567);
#19263=VERTEX_POINT('',#78568);
#19264=VERTEX_POINT('',#78584);
#19265=VERTEX_POINT('',#78585);
#19266=VERTEX_POINT('',#78588);
#19267=VERTEX_POINT('',#78590);
#19268=VERTEX_POINT('',#78592);
#19269=VERTEX_POINT('',#78631);
#19270=VERTEX_POINT('',#78652);
#19271=VERTEX_POINT('',#78653);
#19272=VERTEX_POINT('',#78656);
#19273=VERTEX_POINT('',#78664);
#19274=VERTEX_POINT('',#78683);
#19275=VERTEX_POINT('',#78684);
#19276=VERTEX_POINT('',#78694);
#19277=VERTEX_POINT('',#78695);
#19278=VERTEX_POINT('',#78705);
#19279=VERTEX_POINT('',#78706);
#19280=VERTEX_POINT('',#78709);
#19281=VERTEX_POINT('',#78711);
#19282=VERTEX_POINT('',#78713);
#19283=VERTEX_POINT('',#78757);
#19284=VERTEX_POINT('',#78758);
#19285=VERTEX_POINT('',#78768);
#19286=VERTEX_POINT('',#78769);
#19287=VERTEX_POINT('',#78782);
#19288=VERTEX_POINT('',#78783);
#19289=VERTEX_POINT('',#78786);
#19290=VERTEX_POINT('',#78788);
#19291=VERTEX_POINT('',#78790);
#19292=VERTEX_POINT('',#78825);
#19293=VERTEX_POINT('',#78826);
#19294=VERTEX_POINT('',#78836);
#19295=VERTEX_POINT('',#78837);
#19296=VERTEX_POINT('',#78856);
#19297=VERTEX_POINT('',#78857);
#19298=VERTEX_POINT('',#78873);
#19299=VERTEX_POINT('',#78875);
#19300=VERTEX_POINT('',#78877);
#19301=VERTEX_POINT('',#78918);
#19302=VERTEX_POINT('',#78919);
#19303=VERTEX_POINT('',#78934);
#19304=VERTEX_POINT('',#78935);
#19305=VERTEX_POINT('',#78953);
#19306=VERTEX_POINT('',#78954);
#19307=VERTEX_POINT('',#78957);
#19308=VERTEX_POINT('',#78959);
#19309=VERTEX_POINT('',#78961);
#19310=VERTEX_POINT('',#78996);
#19311=VERTEX_POINT('',#78997);
#19312=VERTEX_POINT('',#79007);
#19313=VERTEX_POINT('',#79008);
#19314=VERTEX_POINT('',#79028);
#19315=VERTEX_POINT('',#79029);
#19316=VERTEX_POINT('',#79032);
#19317=VERTEX_POINT('',#79034);
#19318=VERTEX_POINT('',#79036);
#19319=VERTEX_POINT('',#79071);
#19320=VERTEX_POINT('',#79072);
#19321=VERTEX_POINT('',#79082);
#19322=VERTEX_POINT('',#79083);
#19323=VERTEX_POINT('',#79099);
#19324=VERTEX_POINT('',#79100);
#19325=VERTEX_POINT('',#79103);
#19326=VERTEX_POINT('',#79105);
#19327=VERTEX_POINT('',#79107);
#19328=VERTEX_POINT('',#79146);
#19329=VERTEX_POINT('',#79167);
#19330=VERTEX_POINT('',#79168);
#19331=VERTEX_POINT('',#79171);
#19332=VERTEX_POINT('',#79179);
#19333=VERTEX_POINT('',#79198);
#19334=VERTEX_POINT('',#79199);
#19335=VERTEX_POINT('',#79209);
#19336=VERTEX_POINT('',#79210);
#19337=VERTEX_POINT('',#79220);
#19338=VERTEX_POINT('',#79221);
#19339=VERTEX_POINT('',#79224);
#19340=VERTEX_POINT('',#79226);
#19341=VERTEX_POINT('',#79228);
#19342=VERTEX_POINT('',#79272);
#19343=VERTEX_POINT('',#79273);
#19344=VERTEX_POINT('',#79283);
#19345=VERTEX_POINT('',#79284);
#19346=VERTEX_POINT('',#79297);
#19347=VERTEX_POINT('',#79298);
#19348=VERTEX_POINT('',#79301);
#19349=VERTEX_POINT('',#79303);
#19350=VERTEX_POINT('',#79305);
#19351=VERTEX_POINT('',#79340);
#19352=VERTEX_POINT('',#79341);
#19353=VERTEX_POINT('',#79351);
#19354=VERTEX_POINT('',#79352);
#19355=VERTEX_POINT('',#79371);
#19356=VERTEX_POINT('',#79372);
#19357=VERTEX_POINT('',#79388);
#19358=VERTEX_POINT('',#79390);
#19359=VERTEX_POINT('',#79392);
#19360=VERTEX_POINT('',#79433);
#19361=VERTEX_POINT('',#79434);
#19362=VERTEX_POINT('',#79449);
#19363=VERTEX_POINT('',#79450);
#19364=VERTEX_POINT('',#79468);
#19365=VERTEX_POINT('',#79469);
#19366=VERTEX_POINT('',#79472);
#19367=VERTEX_POINT('',#79474);
#19368=VERTEX_POINT('',#79476);
#19369=VERTEX_POINT('',#79511);
#19370=VERTEX_POINT('',#79512);
#19371=VERTEX_POINT('',#79522);
#19372=VERTEX_POINT('',#79523);
#19373=VERTEX_POINT('',#79543);
#19374=VERTEX_POINT('',#79544);
#19375=VERTEX_POINT('',#79547);
#19376=VERTEX_POINT('',#79549);
#19377=VERTEX_POINT('',#79551);
#19378=VERTEX_POINT('',#79586);
#19379=VERTEX_POINT('',#79587);
#19380=VERTEX_POINT('',#79597);
#19381=VERTEX_POINT('',#79598);
#19382=VERTEX_POINT('',#79614);
#19383=VERTEX_POINT('',#79615);
#19384=VERTEX_POINT('',#79618);
#19385=VERTEX_POINT('',#79620);
#19386=VERTEX_POINT('',#79622);
#19387=VERTEX_POINT('',#79661);
#19388=VERTEX_POINT('',#79682);
#19389=VERTEX_POINT('',#79683);
#19390=VERTEX_POINT('',#79686);
#19391=VERTEX_POINT('',#79694);
#19392=VERTEX_POINT('',#79713);
#19393=VERTEX_POINT('',#79714);
#19394=VERTEX_POINT('',#79724);
#19395=VERTEX_POINT('',#79725);
#19396=VERTEX_POINT('',#79735);
#19397=VERTEX_POINT('',#79736);
#19398=VERTEX_POINT('',#79739);
#19399=VERTEX_POINT('',#79741);
#19400=VERTEX_POINT('',#79743);
#19401=VERTEX_POINT('',#79787);
#19402=VERTEX_POINT('',#79788);
#19403=VERTEX_POINT('',#79798);
#19404=VERTEX_POINT('',#79799);
#19405=VERTEX_POINT('',#79812);
#19406=VERTEX_POINT('',#79813);
#19407=VERTEX_POINT('',#79816);
#19408=VERTEX_POINT('',#79818);
#19409=VERTEX_POINT('',#79820);
#19410=VERTEX_POINT('',#79855);
#19411=VERTEX_POINT('',#79856);
#19412=VERTEX_POINT('',#79866);
#19413=VERTEX_POINT('',#79867);
#19414=VERTEX_POINT('',#79886);
#19415=VERTEX_POINT('',#79887);
#19416=VERTEX_POINT('',#79903);
#19417=VERTEX_POINT('',#79905);
#19418=VERTEX_POINT('',#79907);
#19419=VERTEX_POINT('',#79948);
#19420=VERTEX_POINT('',#79949);
#19421=VERTEX_POINT('',#79964);
#19422=VERTEX_POINT('',#79965);
#19423=VERTEX_POINT('',#79983);
#19424=VERTEX_POINT('',#79984);
#19425=VERTEX_POINT('',#79987);
#19426=VERTEX_POINT('',#79989);
#19427=VERTEX_POINT('',#79991);
#19428=VERTEX_POINT('',#80026);
#19429=VERTEX_POINT('',#80027);
#19430=VERTEX_POINT('',#80037);
#19431=VERTEX_POINT('',#80038);
#19432=VERTEX_POINT('',#80058);
#19433=VERTEX_POINT('',#80059);
#19434=VERTEX_POINT('',#80062);
#19435=VERTEX_POINT('',#80064);
#19436=VERTEX_POINT('',#80066);
#19437=VERTEX_POINT('',#80101);
#19438=VERTEX_POINT('',#80102);
#19439=VERTEX_POINT('',#80112);
#19440=VERTEX_POINT('',#80113);
#19441=VERTEX_POINT('',#80129);
#19442=VERTEX_POINT('',#80130);
#19443=VERTEX_POINT('',#80133);
#19444=VERTEX_POINT('',#80135);
#19445=VERTEX_POINT('',#80137);
#19446=VERTEX_POINT('',#80176);
#19447=VERTEX_POINT('',#80197);
#19448=VERTEX_POINT('',#80198);
#19449=VERTEX_POINT('',#80201);
#19450=VERTEX_POINT('',#80209);
#19451=VERTEX_POINT('',#80228);
#19452=VERTEX_POINT('',#80229);
#19453=VERTEX_POINT('',#80239);
#19454=VERTEX_POINT('',#80240);
#19455=VERTEX_POINT('',#80250);
#19456=VERTEX_POINT('',#80251);
#19457=VERTEX_POINT('',#80254);
#19458=VERTEX_POINT('',#80256);
#19459=VERTEX_POINT('',#80258);
#19460=VERTEX_POINT('',#80302);
#19461=VERTEX_POINT('',#80303);
#19462=VERTEX_POINT('',#80313);
#19463=VERTEX_POINT('',#80314);
#19464=VERTEX_POINT('',#80327);
#19465=VERTEX_POINT('',#80328);
#19466=VERTEX_POINT('',#80331);
#19467=VERTEX_POINT('',#80333);
#19468=VERTEX_POINT('',#80335);
#19469=VERTEX_POINT('',#80370);
#19470=VERTEX_POINT('',#80371);
#19471=VERTEX_POINT('',#80381);
#19472=VERTEX_POINT('',#80382);
#19473=VERTEX_POINT('',#80401);
#19474=VERTEX_POINT('',#80402);
#19475=VERTEX_POINT('',#80418);
#19476=VERTEX_POINT('',#80420);
#19477=VERTEX_POINT('',#80422);
#19478=VERTEX_POINT('',#80463);
#19479=VERTEX_POINT('',#80464);
#19480=VERTEX_POINT('',#80479);
#19481=VERTEX_POINT('',#80480);
#19482=VERTEX_POINT('',#80498);
#19483=VERTEX_POINT('',#80499);
#19484=VERTEX_POINT('',#80502);
#19485=VERTEX_POINT('',#80504);
#19486=VERTEX_POINT('',#80506);
#19487=VERTEX_POINT('',#80541);
#19488=VERTEX_POINT('',#80542);
#19489=VERTEX_POINT('',#80552);
#19490=VERTEX_POINT('',#80553);
#19491=VERTEX_POINT('',#80573);
#19492=VERTEX_POINT('',#80574);
#19493=VERTEX_POINT('',#80577);
#19494=VERTEX_POINT('',#80579);
#19495=VERTEX_POINT('',#80581);
#19496=VERTEX_POINT('',#80616);
#19497=VERTEX_POINT('',#80617);
#19498=VERTEX_POINT('',#80627);
#19499=VERTEX_POINT('',#80628);
#19500=VERTEX_POINT('',#80644);
#19501=VERTEX_POINT('',#80645);
#19502=VERTEX_POINT('',#80648);
#19503=VERTEX_POINT('',#80650);
#19504=VERTEX_POINT('',#80652);
#19505=VERTEX_POINT('',#80691);
#19506=VERTEX_POINT('',#80712);
#19507=VERTEX_POINT('',#80713);
#19508=VERTEX_POINT('',#80716);
#19509=VERTEX_POINT('',#80724);
#19510=VERTEX_POINT('',#80743);
#19511=VERTEX_POINT('',#80744);
#19512=VERTEX_POINT('',#80754);
#19513=VERTEX_POINT('',#80755);
#19514=VERTEX_POINT('',#80765);
#19515=VERTEX_POINT('',#80766);
#19516=VERTEX_POINT('',#80769);
#19517=VERTEX_POINT('',#80771);
#19518=VERTEX_POINT('',#80773);
#19519=VERTEX_POINT('',#80817);
#19520=VERTEX_POINT('',#80818);
#19521=VERTEX_POINT('',#80828);
#19522=VERTEX_POINT('',#80829);
#19523=VERTEX_POINT('',#80842);
#19524=VERTEX_POINT('',#80843);
#19525=VERTEX_POINT('',#80846);
#19526=VERTEX_POINT('',#80848);
#19527=VERTEX_POINT('',#80850);
#19528=VERTEX_POINT('',#80885);
#19529=VERTEX_POINT('',#80886);
#19530=VERTEX_POINT('',#80896);
#19531=VERTEX_POINT('',#80897);
#19532=VERTEX_POINT('',#80916);
#19533=VERTEX_POINT('',#80917);
#19534=VERTEX_POINT('',#80933);
#19535=VERTEX_POINT('',#80935);
#19536=VERTEX_POINT('',#80937);
#19537=VERTEX_POINT('',#80978);
#19538=VERTEX_POINT('',#80979);
#19539=VERTEX_POINT('',#80994);
#19540=VERTEX_POINT('',#80995);
#19541=VERTEX_POINT('',#81013);
#19542=VERTEX_POINT('',#81014);
#19543=VERTEX_POINT('',#81017);
#19544=VERTEX_POINT('',#81019);
#19545=VERTEX_POINT('',#81021);
#19546=VERTEX_POINT('',#81056);
#19547=VERTEX_POINT('',#81057);
#19548=VERTEX_POINT('',#81067);
#19549=VERTEX_POINT('',#81068);
#19550=VERTEX_POINT('',#81088);
#19551=VERTEX_POINT('',#81089);
#19552=VERTEX_POINT('',#81092);
#19553=VERTEX_POINT('',#81094);
#19554=VERTEX_POINT('',#81096);
#19555=VERTEX_POINT('',#81131);
#19556=VERTEX_POINT('',#81132);
#19557=VERTEX_POINT('',#81142);
#19558=VERTEX_POINT('',#81143);
#19559=VERTEX_POINT('',#81159);
#19560=VERTEX_POINT('',#81160);
#19561=VERTEX_POINT('',#81163);
#19562=VERTEX_POINT('',#81165);
#19563=VERTEX_POINT('',#81167);
#19564=VERTEX_POINT('',#81206);
#19565=VERTEX_POINT('',#81227);
#19566=VERTEX_POINT('',#81228);
#19567=VERTEX_POINT('',#81231);
#19568=VERTEX_POINT('',#81239);
#19569=VERTEX_POINT('',#81258);
#19570=VERTEX_POINT('',#81259);
#19571=VERTEX_POINT('',#81269);
#19572=VERTEX_POINT('',#81270);
#19573=VERTEX_POINT('',#81280);
#19574=VERTEX_POINT('',#81281);
#19575=VERTEX_POINT('',#81284);
#19576=VERTEX_POINT('',#81286);
#19577=VERTEX_POINT('',#81288);
#19578=VERTEX_POINT('',#81332);
#19579=VERTEX_POINT('',#81333);
#19580=VERTEX_POINT('',#81343);
#19581=VERTEX_POINT('',#81344);
#19582=VERTEX_POINT('',#81354);
#19583=VERTEX_POINT('',#81355);
#19584=VERTEX_POINT('',#81358);
#19585=VERTEX_POINT('',#81360);
#19586=VERTEX_POINT('',#81362);
#19587=VERTEX_POINT('',#81404);
#19588=VERTEX_POINT('',#81405);
#19589=VERTEX_POINT('',#81415);
#19590=VERTEX_POINT('',#81416);
#19591=VERTEX_POINT('',#81435);
#19592=VERTEX_POINT('',#81436);
#19593=VERTEX_POINT('',#81452);
#19594=VERTEX_POINT('',#81454);
#19595=VERTEX_POINT('',#81456);
#19596=VERTEX_POINT('',#81497);
#19597=VERTEX_POINT('',#81498);
#19598=VERTEX_POINT('',#81513);
#19599=VERTEX_POINT('',#81514);
#19600=VERTEX_POINT('',#81532);
#19601=VERTEX_POINT('',#81533);
#19602=VERTEX_POINT('',#81536);
#19603=VERTEX_POINT('',#81538);
#19604=VERTEX_POINT('',#81540);
#19605=VERTEX_POINT('',#81575);
#19606=VERTEX_POINT('',#81576);
#19607=VERTEX_POINT('',#81586);
#19608=VERTEX_POINT('',#81587);
#19609=VERTEX_POINT('',#81607);
#19610=VERTEX_POINT('',#81608);
#19611=VERTEX_POINT('',#81611);
#19612=VERTEX_POINT('',#81613);
#19613=VERTEX_POINT('',#81615);
#19614=VERTEX_POINT('',#81650);
#19615=VERTEX_POINT('',#81651);
#19616=VERTEX_POINT('',#81661);
#19617=VERTEX_POINT('',#81662);
#19618=VERTEX_POINT('',#81678);
#19619=VERTEX_POINT('',#81679);
#19620=VERTEX_POINT('',#81682);
#19621=VERTEX_POINT('',#81684);
#19622=VERTEX_POINT('',#81686);
#19623=VERTEX_POINT('',#81725);
#19624=VERTEX_POINT('',#81746);
#19625=VERTEX_POINT('',#81747);
#19626=VERTEX_POINT('',#81750);
#19627=VERTEX_POINT('',#81758);
#19628=VERTEX_POINT('',#81777);
#19629=VERTEX_POINT('',#81778);
#19630=VERTEX_POINT('',#81788);
#19631=VERTEX_POINT('',#81789);
#19632=VERTEX_POINT('',#81799);
#19633=VERTEX_POINT('',#81800);
#19634=VERTEX_POINT('',#81803);
#19635=VERTEX_POINT('',#81805);
#19636=VERTEX_POINT('',#81807);
#19637=VERTEX_POINT('',#81851);
#19638=VERTEX_POINT('',#81852);
#19639=VERTEX_POINT('',#81862);
#19640=VERTEX_POINT('',#81863);
#19641=VERTEX_POINT('',#81876);
#19642=VERTEX_POINT('',#81877);
#19643=VERTEX_POINT('',#81880);
#19644=VERTEX_POINT('',#81882);
#19645=VERTEX_POINT('',#81884);
#19646=VERTEX_POINT('',#81919);
#19647=VERTEX_POINT('',#81920);
#19648=VERTEX_POINT('',#81930);
#19649=VERTEX_POINT('',#81931);
#19650=VERTEX_POINT('',#81951);
#19651=VERTEX_POINT('',#81952);
#19652=VERTEX_POINT('',#81966);
#19653=VERTEX_POINT('',#81968);
#19654=VERTEX_POINT('',#81970);
#19655=VERTEX_POINT('',#82006);
#19656=VERTEX_POINT('',#82007);
#19657=VERTEX_POINT('',#82022);
#19658=VERTEX_POINT('',#82023);
#19659=VERTEX_POINT('',#82041);
#19660=VERTEX_POINT('',#82042);
#19661=VERTEX_POINT('',#82045);
#19662=VERTEX_POINT('',#82047);
#19663=VERTEX_POINT('',#82049);
#19664=VERTEX_POINT('',#82084);
#19665=VERTEX_POINT('',#82085);
#19666=VERTEX_POINT('',#82095);
#19667=VERTEX_POINT('',#82096);
#19668=VERTEX_POINT('',#82116);
#19669=VERTEX_POINT('',#82117);
#19670=VERTEX_POINT('',#82120);
#19671=VERTEX_POINT('',#82122);
#19672=VERTEX_POINT('',#82124);
#19673=VERTEX_POINT('',#82159);
#19674=VERTEX_POINT('',#82160);
#19675=VERTEX_POINT('',#82170);
#19676=VERTEX_POINT('',#82171);
#19677=VERTEX_POINT('',#82187);
#19678=VERTEX_POINT('',#82188);
#19679=VERTEX_POINT('',#82191);
#19680=VERTEX_POINT('',#82193);
#19681=VERTEX_POINT('',#82195);
#19682=VERTEX_POINT('',#82234);
#19683=VERTEX_POINT('',#82255);
#19684=VERTEX_POINT('',#82256);
#19685=VERTEX_POINT('',#82259);
#19686=VERTEX_POINT('',#82267);
#19687=VERTEX_POINT('',#82286);
#19688=VERTEX_POINT('',#82287);
#19689=VERTEX_POINT('',#82297);
#19690=VERTEX_POINT('',#82298);
#19691=VERTEX_POINT('',#82308);
#19692=VERTEX_POINT('',#82309);
#19693=VERTEX_POINT('',#82312);
#19694=VERTEX_POINT('',#82314);
#19695=VERTEX_POINT('',#82316);
#19696=VERTEX_POINT('',#82360);
#19697=VERTEX_POINT('',#82361);
#19698=VERTEX_POINT('',#82371);
#19699=VERTEX_POINT('',#82372);
#19700=VERTEX_POINT('',#82385);
#19701=VERTEX_POINT('',#82386);
#19702=VERTEX_POINT('',#82389);
#19703=VERTEX_POINT('',#82391);
#19704=VERTEX_POINT('',#82393);
#19705=VERTEX_POINT('',#82428);
#19706=VERTEX_POINT('',#82429);
#19707=VERTEX_POINT('',#82439);
#19708=VERTEX_POINT('',#82440);
#19709=VERTEX_POINT('',#82459);
#19710=VERTEX_POINT('',#82460);
#19711=VERTEX_POINT('',#82476);
#19712=VERTEX_POINT('',#82478);
#19713=VERTEX_POINT('',#82480);
#19714=VERTEX_POINT('',#82521);
#19715=VERTEX_POINT('',#82522);
#19716=VERTEX_POINT('',#82537);
#19717=VERTEX_POINT('',#82538);
#19718=VERTEX_POINT('',#82553);
#19719=VERTEX_POINT('',#82554);
#19720=VERTEX_POINT('',#82557);
#19721=VERTEX_POINT('',#82559);
#19722=VERTEX_POINT('',#82561);
#19723=VERTEX_POINT('',#82603);
#19724=VERTEX_POINT('',#82604);
#19725=VERTEX_POINT('',#82614);
#19726=VERTEX_POINT('',#82615);
#19727=VERTEX_POINT('',#82635);
#19728=VERTEX_POINT('',#82636);
#19729=VERTEX_POINT('',#82639);
#19730=VERTEX_POINT('',#82641);
#19731=VERTEX_POINT('',#82643);
#19732=VERTEX_POINT('',#82678);
#19733=VERTEX_POINT('',#82679);
#19734=VERTEX_POINT('',#82689);
#19735=VERTEX_POINT('',#82690);
#19736=VERTEX_POINT('',#82706);
#19737=VERTEX_POINT('',#82707);
#19738=VERTEX_POINT('',#82710);
#19739=VERTEX_POINT('',#82712);
#19740=VERTEX_POINT('',#82714);
#19741=VERTEX_POINT('',#82753);
#19742=VERTEX_POINT('',#82774);
#19743=VERTEX_POINT('',#82775);
#19744=VERTEX_POINT('',#82778);
#19745=VERTEX_POINT('',#82786);
#19746=VERTEX_POINT('',#82805);
#19747=VERTEX_POINT('',#82806);
#19748=VERTEX_POINT('',#82816);
#19749=VERTEX_POINT('',#82817);
#19750=VERTEX_POINT('',#82827);
#19751=VERTEX_POINT('',#82828);
#19752=VERTEX_POINT('',#82831);
#19753=VERTEX_POINT('',#82833);
#19754=VERTEX_POINT('',#82835);
#19755=VERTEX_POINT('',#82879);
#19756=VERTEX_POINT('',#82880);
#19757=VERTEX_POINT('',#82890);
#19758=VERTEX_POINT('',#82891);
#19759=VERTEX_POINT('',#82904);
#19760=VERTEX_POINT('',#82905);
#19761=VERTEX_POINT('',#82908);
#19762=VERTEX_POINT('',#82910);
#19763=VERTEX_POINT('',#82912);
#19764=VERTEX_POINT('',#82947);
#19765=VERTEX_POINT('',#82948);
#19766=VERTEX_POINT('',#82958);
#19767=VERTEX_POINT('',#82959);
#19768=VERTEX_POINT('',#82978);
#19769=VERTEX_POINT('',#82979);
#19770=VERTEX_POINT('',#82995);
#19771=VERTEX_POINT('',#82997);
#19772=VERTEX_POINT('',#82999);
#19773=VERTEX_POINT('',#83040);
#19774=VERTEX_POINT('',#83041);
#19775=VERTEX_POINT('',#83056);
#19776=VERTEX_POINT('',#83057);
#19777=VERTEX_POINT('',#83075);
#19778=VERTEX_POINT('',#83076);
#19779=VERTEX_POINT('',#83079);
#19780=VERTEX_POINT('',#83081);
#19781=VERTEX_POINT('',#83083);
#19782=VERTEX_POINT('',#83118);
#19783=VERTEX_POINT('',#83119);
#19784=VERTEX_POINT('',#83129);
#19785=VERTEX_POINT('',#83130);
#19786=VERTEX_POINT('',#83150);
#19787=VERTEX_POINT('',#83151);
#19788=VERTEX_POINT('',#83154);
#19789=VERTEX_POINT('',#83156);
#19790=VERTEX_POINT('',#83158);
#19791=VERTEX_POINT('',#83200);
#19792=VERTEX_POINT('',#83201);
#19793=VERTEX_POINT('',#83211);
#19794=VERTEX_POINT('',#83212);
#19795=VERTEX_POINT('',#83228);
#19796=VERTEX_POINT('',#83229);
#19797=VERTEX_POINT('',#83232);
#19798=VERTEX_POINT('',#83234);
#19799=VERTEX_POINT('',#83236);
#19800=VERTEX_POINT('',#83275);
#19801=VERTEX_POINT('',#83296);
#19802=VERTEX_POINT('',#83297);
#19803=VERTEX_POINT('',#83300);
#19804=VERTEX_POINT('',#83308);
#19805=VERTEX_POINT('',#83327);
#19806=VERTEX_POINT('',#83328);
#19807=VERTEX_POINT('',#83338);
#19808=VERTEX_POINT('',#83339);
#19809=VERTEX_POINT('',#83349);
#19810=VERTEX_POINT('',#83350);
#19811=VERTEX_POINT('',#83353);
#19812=VERTEX_POINT('',#83355);
#19813=VERTEX_POINT('',#83357);
#19814=VERTEX_POINT('',#83401);
#19815=VERTEX_POINT('',#83402);
#19816=VERTEX_POINT('',#83412);
#19817=VERTEX_POINT('',#83413);
#19818=VERTEX_POINT('',#83426);
#19819=VERTEX_POINT('',#83427);
#19820=VERTEX_POINT('',#83430);
#19821=VERTEX_POINT('',#83432);
#19822=VERTEX_POINT('',#83434);
#19823=VERTEX_POINT('',#83469);
#19824=VERTEX_POINT('',#83470);
#19825=VERTEX_POINT('',#83480);
#19826=VERTEX_POINT('',#83481);
#19827=VERTEX_POINT('',#83500);
#19828=VERTEX_POINT('',#83501);
#19829=VERTEX_POINT('',#83517);
#19830=VERTEX_POINT('',#83519);
#19831=VERTEX_POINT('',#83521);
#19832=VERTEX_POINT('',#83562);
#19833=VERTEX_POINT('',#83563);
#19834=VERTEX_POINT('',#83578);
#19835=VERTEX_POINT('',#83579);
#19836=VERTEX_POINT('',#83597);
#19837=VERTEX_POINT('',#83598);
#19838=VERTEX_POINT('',#83601);
#19839=VERTEX_POINT('',#83603);
#19840=VERTEX_POINT('',#83605);
#19841=VERTEX_POINT('',#83640);
#19842=VERTEX_POINT('',#83641);
#19843=VERTEX_POINT('',#83651);
#19844=VERTEX_POINT('',#83652);
#19845=VERTEX_POINT('',#83672);
#19846=VERTEX_POINT('',#83673);
#19847=VERTEX_POINT('',#83676);
#19848=VERTEX_POINT('',#83678);
#19849=VERTEX_POINT('',#83680);
#19850=VERTEX_POINT('',#83715);
#19851=VERTEX_POINT('',#83716);
#19852=VERTEX_POINT('',#83726);
#19853=VERTEX_POINT('',#83727);
#19854=VERTEX_POINT('',#83740);
#19855=VERTEX_POINT('',#83741);
#19856=VERTEX_POINT('',#83744);
#19857=VERTEX_POINT('',#83746);
#19858=VERTEX_POINT('',#83748);
#19859=VERTEX_POINT('',#83794);
#19860=VERTEX_POINT('',#83815);
#19861=VERTEX_POINT('',#83816);
#19862=VERTEX_POINT('',#83819);
#19863=VERTEX_POINT('',#83827);
#19864=VERTEX_POINT('',#83846);
#19865=VERTEX_POINT('',#83847);
#19866=VERTEX_POINT('',#83857);
#19867=VERTEX_POINT('',#83858);
#19868=VERTEX_POINT('',#83868);
#19869=VERTEX_POINT('',#83869);
#19870=VERTEX_POINT('',#83872);
#19871=VERTEX_POINT('',#83874);
#19872=VERTEX_POINT('',#83876);
#19873=VERTEX_POINT('',#83920);
#19874=VERTEX_POINT('',#83921);
#19875=VERTEX_POINT('',#83931);
#19876=VERTEX_POINT('',#83932);
#19877=VERTEX_POINT('',#83945);
#19878=VERTEX_POINT('',#83946);
#19879=VERTEX_POINT('',#83949);
#19880=VERTEX_POINT('',#83951);
#19881=VERTEX_POINT('',#83953);
#19882=VERTEX_POINT('',#83988);
#19883=VERTEX_POINT('',#83989);
#19884=VERTEX_POINT('',#83999);
#19885=VERTEX_POINT('',#84000);
#19886=VERTEX_POINT('',#84019);
#19887=VERTEX_POINT('',#84020);
#19888=VERTEX_POINT('',#84036);
#19889=VERTEX_POINT('',#84038);
#19890=VERTEX_POINT('',#84040);
#19891=VERTEX_POINT('',#84081);
#19892=VERTEX_POINT('',#84082);
#19893=VERTEX_POINT('',#84097);
#19894=VERTEX_POINT('',#84098);
#19895=VERTEX_POINT('',#84116);
#19896=VERTEX_POINT('',#84117);
#19897=VERTEX_POINT('',#84120);
#19898=VERTEX_POINT('',#84122);
#19899=VERTEX_POINT('',#84124);
#19900=VERTEX_POINT('',#84159);
#19901=VERTEX_POINT('',#84160);
#19902=VERTEX_POINT('',#84170);
#19903=VERTEX_POINT('',#84171);
#19904=VERTEX_POINT('',#84191);
#19905=VERTEX_POINT('',#84192);
#19906=VERTEX_POINT('',#84195);
#19907=VERTEX_POINT('',#84197);
#19908=VERTEX_POINT('',#84199);
#19909=VERTEX_POINT('',#84234);
#19910=VERTEX_POINT('',#84235);
#19911=VERTEX_POINT('',#84245);
#19912=VERTEX_POINT('',#84246);
#19913=VERTEX_POINT('',#84262);
#19914=VERTEX_POINT('',#84263);
#19915=VERTEX_POINT('',#84266);
#19916=VERTEX_POINT('',#84268);
#19917=VERTEX_POINT('',#84270);
#19918=VERTEX_POINT('',#84309);
#19919=VERTEX_POINT('',#84330);
#19920=VERTEX_POINT('',#84331);
#19921=VERTEX_POINT('',#84334);
#19922=VERTEX_POINT('',#84342);
#19923=VERTEX_POINT('',#84361);
#19924=VERTEX_POINT('',#84362);
#19925=VERTEX_POINT('',#84372);
#19926=VERTEX_POINT('',#84373);
#19927=VERTEX_POINT('',#84383);
#19928=VERTEX_POINT('',#84384);
#19929=VERTEX_POINT('',#84387);
#19930=VERTEX_POINT('',#84389);
#19931=VERTEX_POINT('',#84391);
#19932=VERTEX_POINT('',#84435);
#19933=VERTEX_POINT('',#84436);
#19934=VERTEX_POINT('',#84446);
#19935=VERTEX_POINT('',#84447);
#19936=VERTEX_POINT('',#84460);
#19937=VERTEX_POINT('',#84461);
#19938=VERTEX_POINT('',#84464);
#19939=VERTEX_POINT('',#84466);
#19940=VERTEX_POINT('',#84468);
#19941=VERTEX_POINT('',#84503);
#19942=VERTEX_POINT('',#84504);
#19943=VERTEX_POINT('',#84514);
#19944=VERTEX_POINT('',#84515);
#19945=VERTEX_POINT('',#84534);
#19946=VERTEX_POINT('',#84535);
#19947=VERTEX_POINT('',#84551);
#19948=VERTEX_POINT('',#84553);
#19949=VERTEX_POINT('',#84555);
#19950=VERTEX_POINT('',#84596);
#19951=VERTEX_POINT('',#84597);
#19952=VERTEX_POINT('',#84612);
#19953=VERTEX_POINT('',#84613);
#19954=VERTEX_POINT('',#84631);
#19955=VERTEX_POINT('',#84632);
#19956=VERTEX_POINT('',#84635);
#19957=VERTEX_POINT('',#84637);
#19958=VERTEX_POINT('',#84639);
#19959=VERTEX_POINT('',#84674);
#19960=VERTEX_POINT('',#84675);
#19961=VERTEX_POINT('',#84685);
#19962=VERTEX_POINT('',#84686);
#19963=VERTEX_POINT('',#84706);
#19964=VERTEX_POINT('',#84707);
#19965=VERTEX_POINT('',#84710);
#19966=VERTEX_POINT('',#84712);
#19967=VERTEX_POINT('',#84714);
#19968=VERTEX_POINT('',#84749);
#19969=VERTEX_POINT('',#84750);
#19970=VERTEX_POINT('',#84760);
#19971=VERTEX_POINT('',#84761);
#19972=VERTEX_POINT('',#84777);
#19973=VERTEX_POINT('',#84778);
#19974=VERTEX_POINT('',#84781);
#19975=VERTEX_POINT('',#84783);
#19976=VERTEX_POINT('',#84785);
#19977=VERTEX_POINT('',#84824);
#19978=VERTEX_POINT('',#84845);
#19979=VERTEX_POINT('',#84846);
#19980=VERTEX_POINT('',#84849);
#19981=VERTEX_POINT('',#84857);
#19982=VERTEX_POINT('',#84876);
#19983=VERTEX_POINT('',#84877);
#19984=VERTEX_POINT('',#84887);
#19985=VERTEX_POINT('',#84888);
#19986=VERTEX_POINT('',#84898);
#19987=VERTEX_POINT('',#84899);
#19988=VERTEX_POINT('',#84902);
#19989=VERTEX_POINT('',#84904);
#19990=VERTEX_POINT('',#84906);
#19991=VERTEX_POINT('',#84950);
#19992=VERTEX_POINT('',#84951);
#19993=VERTEX_POINT('',#84961);
#19994=VERTEX_POINT('',#84962);
#19995=VERTEX_POINT('',#84975);
#19996=VERTEX_POINT('',#84976);
#19997=VERTEX_POINT('',#84979);
#19998=VERTEX_POINT('',#84981);
#19999=VERTEX_POINT('',#84983);
#20000=VERTEX_POINT('',#85018);
#20001=VERTEX_POINT('',#85019);
#20002=VERTEX_POINT('',#85029);
#20003=VERTEX_POINT('',#85030);
#20004=VERTEX_POINT('',#85049);
#20005=VERTEX_POINT('',#85050);
#20006=VERTEX_POINT('',#85066);
#20007=VERTEX_POINT('',#85068);
#20008=VERTEX_POINT('',#85070);
#20009=VERTEX_POINT('',#85111);
#20010=VERTEX_POINT('',#85112);
#20011=VERTEX_POINT('',#85127);
#20012=VERTEX_POINT('',#85128);
#20013=VERTEX_POINT('',#85146);
#20014=VERTEX_POINT('',#85147);
#20015=VERTEX_POINT('',#85150);
#20016=VERTEX_POINT('',#85152);
#20017=VERTEX_POINT('',#85154);
#20018=VERTEX_POINT('',#85189);
#20019=VERTEX_POINT('',#85190);
#20020=VERTEX_POINT('',#85200);
#20021=VERTEX_POINT('',#85201);
#20022=VERTEX_POINT('',#85221);
#20023=VERTEX_POINT('',#85222);
#20024=VERTEX_POINT('',#85225);
#20025=VERTEX_POINT('',#85227);
#20026=VERTEX_POINT('',#85229);
#20027=VERTEX_POINT('',#85264);
#20028=VERTEX_POINT('',#85265);
#20029=VERTEX_POINT('',#85275);
#20030=VERTEX_POINT('',#85276);
#20031=VERTEX_POINT('',#85292);
#20032=VERTEX_POINT('',#85293);
#20033=VERTEX_POINT('',#85296);
#20034=VERTEX_POINT('',#85298);
#20035=VERTEX_POINT('',#85300);
#20036=VERTEX_POINT('',#85339);
#20037=VERTEX_POINT('',#85360);
#20038=VERTEX_POINT('',#85361);
#20039=VERTEX_POINT('',#85364);
#20040=VERTEX_POINT('',#85372);
#20041=VERTEX_POINT('',#85391);
#20042=VERTEX_POINT('',#85392);
#20043=VERTEX_POINT('',#85402);
#20044=VERTEX_POINT('',#85403);
#20045=VERTEX_POINT('',#85413);
#20046=VERTEX_POINT('',#85414);
#20047=VERTEX_POINT('',#85417);
#20048=VERTEX_POINT('',#85419);
#20049=VERTEX_POINT('',#85421);
#20050=VERTEX_POINT('',#85465);
#20051=VERTEX_POINT('',#85466);
#20052=VERTEX_POINT('',#85476);
#20053=VERTEX_POINT('',#85477);
#20054=VERTEX_POINT('',#85490);
#20055=VERTEX_POINT('',#85491);
#20056=VERTEX_POINT('',#85494);
#20057=VERTEX_POINT('',#85496);
#20058=VERTEX_POINT('',#85498);
#20059=VERTEX_POINT('',#85533);
#20060=VERTEX_POINT('',#85534);
#20061=VERTEX_POINT('',#85544);
#20062=VERTEX_POINT('',#85545);
#20063=VERTEX_POINT('',#85564);
#20064=VERTEX_POINT('',#85565);
#20065=VERTEX_POINT('',#85581);
#20066=VERTEX_POINT('',#85583);
#20067=VERTEX_POINT('',#85585);
#20068=VERTEX_POINT('',#85626);
#20069=VERTEX_POINT('',#85627);
#20070=VERTEX_POINT('',#85642);
#20071=VERTEX_POINT('',#85643);
#20072=VERTEX_POINT('',#85661);
#20073=VERTEX_POINT('',#85662);
#20074=VERTEX_POINT('',#85665);
#20075=VERTEX_POINT('',#85667);
#20076=VERTEX_POINT('',#85669);
#20077=VERTEX_POINT('',#85704);
#20078=VERTEX_POINT('',#85705);
#20079=VERTEX_POINT('',#85715);
#20080=VERTEX_POINT('',#85716);
#20081=VERTEX_POINT('',#85736);
#20082=VERTEX_POINT('',#85737);
#20083=VERTEX_POINT('',#85740);
#20084=VERTEX_POINT('',#85742);
#20085=VERTEX_POINT('',#85744);
#20086=VERTEX_POINT('',#85779);
#20087=VERTEX_POINT('',#85780);
#20088=VERTEX_POINT('',#85790);
#20089=VERTEX_POINT('',#85791);
#20090=VERTEX_POINT('',#85807);
#20091=VERTEX_POINT('',#85808);
#20092=VERTEX_POINT('',#85811);
#20093=VERTEX_POINT('',#85813);
#20094=VERTEX_POINT('',#85815);
#20095=VERTEX_POINT('',#85854);
#20096=VERTEX_POINT('',#85875);
#20097=VERTEX_POINT('',#85876);
#20098=VERTEX_POINT('',#85879);
#20099=VERTEX_POINT('',#85887);
#20100=VERTEX_POINT('',#85906);
#20101=VERTEX_POINT('',#85907);
#20102=VERTEX_POINT('',#85917);
#20103=VERTEX_POINT('',#85918);
#20104=VERTEX_POINT('',#85928);
#20105=VERTEX_POINT('',#85929);
#20106=VERTEX_POINT('',#85932);
#20107=VERTEX_POINT('',#85934);
#20108=VERTEX_POINT('',#85936);
#20109=VERTEX_POINT('',#85980);
#20110=VERTEX_POINT('',#85981);
#20111=VERTEX_POINT('',#85991);
#20112=VERTEX_POINT('',#85992);
#20113=VERTEX_POINT('',#86005);
#20114=VERTEX_POINT('',#86006);
#20115=VERTEX_POINT('',#86009);
#20116=VERTEX_POINT('',#86011);
#20117=VERTEX_POINT('',#86013);
#20118=VERTEX_POINT('',#86048);
#20119=VERTEX_POINT('',#86049);
#20120=VERTEX_POINT('',#86059);
#20121=VERTEX_POINT('',#86060);
#20122=VERTEX_POINT('',#86079);
#20123=VERTEX_POINT('',#86080);
#20124=VERTEX_POINT('',#86096);
#20125=VERTEX_POINT('',#86098);
#20126=VERTEX_POINT('',#86100);
#20127=VERTEX_POINT('',#86141);
#20128=VERTEX_POINT('',#86142);
#20129=VERTEX_POINT('',#86157);
#20130=VERTEX_POINT('',#86158);
#20131=VERTEX_POINT('',#86176);
#20132=VERTEX_POINT('',#86177);
#20133=VERTEX_POINT('',#86180);
#20134=VERTEX_POINT('',#86182);
#20135=VERTEX_POINT('',#86184);
#20136=VERTEX_POINT('',#86219);
#20137=VERTEX_POINT('',#86220);
#20138=VERTEX_POINT('',#86230);
#20139=VERTEX_POINT('',#86231);
#20140=VERTEX_POINT('',#86251);
#20141=VERTEX_POINT('',#86252);
#20142=VERTEX_POINT('',#86255);
#20143=VERTEX_POINT('',#86257);
#20144=VERTEX_POINT('',#86259);
#20145=VERTEX_POINT('',#86294);
#20146=VERTEX_POINT('',#86295);
#20147=VERTEX_POINT('',#86305);
#20148=VERTEX_POINT('',#86306);
#20149=VERTEX_POINT('',#86322);
#20150=VERTEX_POINT('',#86323);
#20151=VERTEX_POINT('',#86326);
#20152=VERTEX_POINT('',#86328);
#20153=VERTEX_POINT('',#86330);
#20154=VERTEX_POINT('',#86369);
#20155=VERTEX_POINT('',#86390);
#20156=VERTEX_POINT('',#86391);
#20157=VERTEX_POINT('',#86394);
#20158=VERTEX_POINT('',#86402);
#20159=VERTEX_POINT('',#86421);
#20160=VERTEX_POINT('',#86422);
#20161=VERTEX_POINT('',#86432);
#20162=VERTEX_POINT('',#86433);
#20163=VERTEX_POINT('',#86443);
#20164=VERTEX_POINT('',#86444);
#20165=VERTEX_POINT('',#86447);
#20166=VERTEX_POINT('',#86449);
#20167=VERTEX_POINT('',#86451);
#20168=VERTEX_POINT('',#86495);
#20169=VERTEX_POINT('',#86496);
#20170=VERTEX_POINT('',#86506);
#20171=VERTEX_POINT('',#86507);
#20172=VERTEX_POINT('',#86520);
#20173=VERTEX_POINT('',#86521);
#20174=VERTEX_POINT('',#86524);
#20175=VERTEX_POINT('',#86526);
#20176=VERTEX_POINT('',#86528);
#20177=VERTEX_POINT('',#86563);
#20178=VERTEX_POINT('',#86564);
#20179=VERTEX_POINT('',#86574);
#20180=VERTEX_POINT('',#86575);
#20181=VERTEX_POINT('',#86594);
#20182=VERTEX_POINT('',#86595);
#20183=VERTEX_POINT('',#86611);
#20184=VERTEX_POINT('',#86613);
#20185=VERTEX_POINT('',#86615);
#20186=VERTEX_POINT('',#86656);
#20187=VERTEX_POINT('',#86657);
#20188=VERTEX_POINT('',#86672);
#20189=VERTEX_POINT('',#86673);
#20190=VERTEX_POINT('',#86691);
#20191=VERTEX_POINT('',#86692);
#20192=VERTEX_POINT('',#86695);
#20193=VERTEX_POINT('',#86697);
#20194=VERTEX_POINT('',#86699);
#20195=VERTEX_POINT('',#86734);
#20196=VERTEX_POINT('',#86735);
#20197=VERTEX_POINT('',#86745);
#20198=VERTEX_POINT('',#86746);
#20199=VERTEX_POINT('',#86766);
#20200=VERTEX_POINT('',#86767);
#20201=VERTEX_POINT('',#86770);
#20202=VERTEX_POINT('',#86772);
#20203=VERTEX_POINT('',#86774);
#20204=VERTEX_POINT('',#86809);
#20205=VERTEX_POINT('',#86810);
#20206=VERTEX_POINT('',#86820);
#20207=VERTEX_POINT('',#86821);
#20208=VERTEX_POINT('',#86837);
#20209=VERTEX_POINT('',#86838);
#20210=VERTEX_POINT('',#86841);
#20211=VERTEX_POINT('',#86843);
#20212=VERTEX_POINT('',#86845);
#20213=VERTEX_POINT('',#86884);
#20214=VERTEX_POINT('',#86905);
#20215=VERTEX_POINT('',#86906);
#20216=VERTEX_POINT('',#86909);
#20217=VERTEX_POINT('',#86917);
#20218=VERTEX_POINT('',#86936);
#20219=VERTEX_POINT('',#86937);
#20220=VERTEX_POINT('',#86947);
#20221=VERTEX_POINT('',#86948);
#20222=VERTEX_POINT('',#86958);
#20223=VERTEX_POINT('',#86959);
#20224=VERTEX_POINT('',#86962);
#20225=VERTEX_POINT('',#86964);
#20226=VERTEX_POINT('',#86966);
#20227=VERTEX_POINT('',#87010);
#20228=VERTEX_POINT('',#87011);
#20229=VERTEX_POINT('',#87021);
#20230=VERTEX_POINT('',#87022);
#20231=VERTEX_POINT('',#87035);
#20232=VERTEX_POINT('',#87036);
#20233=VERTEX_POINT('',#87039);
#20234=VERTEX_POINT('',#87041);
#20235=VERTEX_POINT('',#87043);
#20236=VERTEX_POINT('',#87078);
#20237=VERTEX_POINT('',#87079);
#20238=VERTEX_POINT('',#87089);
#20239=VERTEX_POINT('',#87090);
#20240=VERTEX_POINT('',#87109);
#20241=VERTEX_POINT('',#87110);
#20242=VERTEX_POINT('',#87126);
#20243=VERTEX_POINT('',#87128);
#20244=VERTEX_POINT('',#87130);
#20245=VERTEX_POINT('',#87171);
#20246=VERTEX_POINT('',#87172);
#20247=VERTEX_POINT('',#87187);
#20248=VERTEX_POINT('',#87188);
#20249=VERTEX_POINT('',#87206);
#20250=VERTEX_POINT('',#87207);
#20251=VERTEX_POINT('',#87210);
#20252=VERTEX_POINT('',#87212);
#20253=VERTEX_POINT('',#87214);
#20254=VERTEX_POINT('',#87249);
#20255=VERTEX_POINT('',#87250);
#20256=VERTEX_POINT('',#87260);
#20257=VERTEX_POINT('',#87261);
#20258=VERTEX_POINT('',#87281);
#20259=VERTEX_POINT('',#87282);
#20260=VERTEX_POINT('',#87285);
#20261=VERTEX_POINT('',#87287);
#20262=VERTEX_POINT('',#87289);
#20263=VERTEX_POINT('',#87324);
#20264=VERTEX_POINT('',#87325);
#20265=VERTEX_POINT('',#87335);
#20266=VERTEX_POINT('',#87336);
#20267=VERTEX_POINT('',#87352);
#20268=VERTEX_POINT('',#87353);
#20269=VERTEX_POINT('',#87356);
#20270=VERTEX_POINT('',#87358);
#20271=VERTEX_POINT('',#87360);
#20272=VERTEX_POINT('',#87399);
#20273=VERTEX_POINT('',#87420);
#20274=VERTEX_POINT('',#87421);
#20275=VERTEX_POINT('',#87424);
#20276=VERTEX_POINT('',#87432);
#20277=VERTEX_POINT('',#87451);
#20278=VERTEX_POINT('',#87452);
#20279=VERTEX_POINT('',#87462);
#20280=VERTEX_POINT('',#87463);
#20281=VERTEX_POINT('',#87473);
#20282=VERTEX_POINT('',#87474);
#20283=VERTEX_POINT('',#87477);
#20284=VERTEX_POINT('',#87479);
#20285=VERTEX_POINT('',#87481);
#20286=VERTEX_POINT('',#87525);
#20287=VERTEX_POINT('',#87526);
#20288=VERTEX_POINT('',#87536);
#20289=VERTEX_POINT('',#87537);
#20290=VERTEX_POINT('',#87550);
#20291=VERTEX_POINT('',#87551);
#20292=VERTEX_POINT('',#87554);
#20293=VERTEX_POINT('',#87556);
#20294=VERTEX_POINT('',#87558);
#20295=VERTEX_POINT('',#87593);
#20296=VERTEX_POINT('',#87594);
#20297=VERTEX_POINT('',#87604);
#20298=VERTEX_POINT('',#87605);
#20299=VERTEX_POINT('',#87624);
#20300=VERTEX_POINT('',#87625);
#20301=VERTEX_POINT('',#87641);
#20302=VERTEX_POINT('',#87643);
#20303=VERTEX_POINT('',#87645);
#20304=VERTEX_POINT('',#87686);
#20305=VERTEX_POINT('',#87687);
#20306=VERTEX_POINT('',#87702);
#20307=VERTEX_POINT('',#87703);
#20308=VERTEX_POINT('',#87721);
#20309=VERTEX_POINT('',#87722);
#20310=VERTEX_POINT('',#87725);
#20311=VERTEX_POINT('',#87727);
#20312=VERTEX_POINT('',#87729);
#20313=VERTEX_POINT('',#87764);
#20314=VERTEX_POINT('',#87765);
#20315=VERTEX_POINT('',#87775);
#20316=VERTEX_POINT('',#87776);
#20317=VERTEX_POINT('',#87796);
#20318=VERTEX_POINT('',#87797);
#20319=VERTEX_POINT('',#87800);
#20320=VERTEX_POINT('',#87802);
#20321=VERTEX_POINT('',#87804);
#20322=VERTEX_POINT('',#87839);
#20323=VERTEX_POINT('',#87840);
#20324=VERTEX_POINT('',#87850);
#20325=VERTEX_POINT('',#87851);
#20326=VERTEX_POINT('',#87867);
#20327=VERTEX_POINT('',#87868);
#20328=VERTEX_POINT('',#87871);
#20329=VERTEX_POINT('',#87873);
#20330=VERTEX_POINT('',#87875);
#20331=VERTEX_POINT('',#87914);
#20332=VERTEX_POINT('',#87920);
#20333=VERTEX_POINT('',#87921);
#20334=VERTEX_POINT('',#87923);
#20335=VERTEX_POINT('',#87925);
#20336=VERTEX_POINT('',#87944);
#20337=VERTEX_POINT('',#87945);
#20338=VERTEX_POINT('',#87948);
#20339=VERTEX_POINT('',#87956);
#20340=VERTEX_POINT('',#87988);
#20341=VERTEX_POINT('',#87989);
#20342=VERTEX_POINT('',#87992);
#20343=VERTEX_POINT('',#87994);
#20344=VERTEX_POINT('',#87996);
#20345=VERTEX_POINT('',#88040);
#20346=VERTEX_POINT('',#88041);
#20347=VERTEX_POINT('',#88051);
#20348=VERTEX_POINT('',#88052);
#20349=VERTEX_POINT('',#88065);
#20350=VERTEX_POINT('',#88066);
#20351=VERTEX_POINT('',#88069);
#20352=VERTEX_POINT('',#88071);
#20353=VERTEX_POINT('',#88073);
#20354=VERTEX_POINT('',#88108);
#20355=VERTEX_POINT('',#88109);
#20356=VERTEX_POINT('',#88119);
#20357=VERTEX_POINT('',#88120);
#20358=VERTEX_POINT('',#88139);
#20359=VERTEX_POINT('',#88140);
#20360=VERTEX_POINT('',#88156);
#20361=VERTEX_POINT('',#88158);
#20362=VERTEX_POINT('',#88160);
#20363=VERTEX_POINT('',#88201);
#20364=VERTEX_POINT('',#88202);
#20365=VERTEX_POINT('',#88217);
#20366=VERTEX_POINT('',#88218);
#20367=VERTEX_POINT('',#88236);
#20368=VERTEX_POINT('',#88237);
#20369=VERTEX_POINT('',#88240);
#20370=VERTEX_POINT('',#88242);
#20371=VERTEX_POINT('',#88244);
#20372=VERTEX_POINT('',#88279);
#20373=VERTEX_POINT('',#88280);
#20374=VERTEX_POINT('',#88290);
#20375=VERTEX_POINT('',#88291);
#20376=VERTEX_POINT('',#88311);
#20377=VERTEX_POINT('',#88312);
#20378=VERTEX_POINT('',#88315);
#20379=VERTEX_POINT('',#88317);
#20380=VERTEX_POINT('',#88319);
#20381=VERTEX_POINT('',#88354);
#20382=VERTEX_POINT('',#88355);
#20383=VERTEX_POINT('',#88365);
#20384=VERTEX_POINT('',#88366);
#20385=VERTEX_POINT('',#88382);
#20386=VERTEX_POINT('',#88383);
#20387=VERTEX_POINT('',#88386);
#20388=VERTEX_POINT('',#88388);
#20389=VERTEX_POINT('',#88390);
#20390=VERTEX_POINT('',#88429);
#20391=VERTEX_POINT('',#88435);
#20392=VERTEX_POINT('',#88436);
#20393=VERTEX_POINT('',#88438);
#20394=VERTEX_POINT('',#88440);
#20395=VERTEX_POINT('',#88444);
#20396=VERTEX_POINT('',#88445);
#20397=VERTEX_POINT('',#88447);
#20398=VERTEX_POINT('',#88449);
#20399=VERTEX_POINT('',#88468);
#20400=VERTEX_POINT('',#88469);
#20401=VERTEX_POINT('',#88472);
#20402=VERTEX_POINT('',#88480);
#20403=VERTEX_POINT('',#88515);
#20404=VERTEX_POINT('',#88516);
#20405=VERTEX_POINT('',#88519);
#20406=VERTEX_POINT('',#88521);
#20407=VERTEX_POINT('',#88523);
#20408=VERTEX_POINT('',#88580);
#20409=VERTEX_POINT('',#88581);
#20410=VERTEX_POINT('',#88584);
#20411=VERTEX_POINT('',#88586);
#20412=VERTEX_POINT('',#88588);
#20413=VERTEX_POINT('',#88630);
#20414=VERTEX_POINT('',#88631);
#20415=VERTEX_POINT('',#88641);
#20416=VERTEX_POINT('',#88642);
#20417=VERTEX_POINT('',#88661);
#20418=VERTEX_POINT('',#88662);
#20419=VERTEX_POINT('',#88678);
#20420=VERTEX_POINT('',#88680);
#20421=VERTEX_POINT('',#88682);
#20422=VERTEX_POINT('',#88723);
#20423=VERTEX_POINT('',#88724);
#20424=VERTEX_POINT('',#88739);
#20425=VERTEX_POINT('',#88740);
#20426=VERTEX_POINT('',#88758);
#20427=VERTEX_POINT('',#88759);
#20428=VERTEX_POINT('',#88762);
#20429=VERTEX_POINT('',#88764);
#20430=VERTEX_POINT('',#88766);
#20431=VERTEX_POINT('',#88801);
#20432=VERTEX_POINT('',#88802);
#20433=VERTEX_POINT('',#88812);
#20434=VERTEX_POINT('',#88813);
#20435=VERTEX_POINT('',#88833);
#20436=VERTEX_POINT('',#88834);
#20437=VERTEX_POINT('',#88837);
#20438=VERTEX_POINT('',#88839);
#20439=VERTEX_POINT('',#88841);
#20440=VERTEX_POINT('',#88876);
#20441=VERTEX_POINT('',#88877);
#20442=VERTEX_POINT('',#88887);
#20443=VERTEX_POINT('',#88888);
#20444=VERTEX_POINT('',#88904);
#20445=VERTEX_POINT('',#88905);
#20446=VERTEX_POINT('',#88908);
#20447=VERTEX_POINT('',#88910);
#20448=VERTEX_POINT('',#88912);
#20449=VERTEX_POINT('',#88951);
#20450=VERTEX_POINT('',#88957);
#20451=VERTEX_POINT('',#88958);
#20452=VERTEX_POINT('',#88960);
#20453=VERTEX_POINT('',#88962);
#20454=VERTEX_POINT('',#88966);
#20455=VERTEX_POINT('',#88967);
#20456=VERTEX_POINT('',#88969);
#20457=VERTEX_POINT('',#88971);
#20458=VERTEX_POINT('',#88975);
#20459=VERTEX_POINT('',#88976);
#20460=VERTEX_POINT('',#88978);
#20461=VERTEX_POINT('',#88980);
#20462=VERTEX_POINT('',#88989);
#20463=VERTEX_POINT('',#88990);
#20464=VERTEX_POINT('',#88993);
#20465=VERTEX_POINT('',#88995);
#20466=VERTEX_POINT('',#88997);
#20467=VERTEX_POINT('',#89060);
#20468=VERTEX_POINT('',#89061);
#20469=VERTEX_POINT('',#89064);
#20470=VERTEX_POINT('',#89066);
#20471=VERTEX_POINT('',#89068);
#20472=VERTEX_POINT('',#89126);
#20473=VERTEX_POINT('',#89127);
#20474=VERTEX_POINT('',#89141);
#20475=VERTEX_POINT('',#89143);
#20476=VERTEX_POINT('',#89145);
#20477=VERTEX_POINT('',#89181);
#20478=VERTEX_POINT('',#89182);
#20479=VERTEX_POINT('',#89205);
#20480=VERTEX_POINT('',#89206);
#20481=VERTEX_POINT('',#89209);
#20482=VERTEX_POINT('',#89217);
#20483=VERTEX_POINT('',#89244);
#20484=VERTEX_POINT('',#89245);
#20485=VERTEX_POINT('',#89263);
#20486=VERTEX_POINT('',#89264);
#20487=VERTEX_POINT('',#89267);
#20488=VERTEX_POINT('',#89269);
#20489=VERTEX_POINT('',#89271);
#20490=VERTEX_POINT('',#89306);
#20491=VERTEX_POINT('',#89307);
#20492=VERTEX_POINT('',#89317);
#20493=VERTEX_POINT('',#89318);
#20494=VERTEX_POINT('',#89338);
#20495=VERTEX_POINT('',#89339);
#20496=VERTEX_POINT('',#89342);
#20497=VERTEX_POINT('',#89344);
#20498=VERTEX_POINT('',#89346);
#20499=VERTEX_POINT('',#89381);
#20500=VERTEX_POINT('',#89382);
#20501=VERTEX_POINT('',#89392);
#20502=VERTEX_POINT('',#89393);
#20503=VERTEX_POINT('',#89409);
#20504=VERTEX_POINT('',#89410);
#20505=VERTEX_POINT('',#89413);
#20506=VERTEX_POINT('',#89415);
#20507=VERTEX_POINT('',#89417);
#20508=VERTEX_POINT('',#89456);
#20509=VERTEX_POINT('',#89462);
#20510=VERTEX_POINT('',#89463);
#20511=VERTEX_POINT('',#89465);
#20512=VERTEX_POINT('',#89467);
#20513=VERTEX_POINT('',#89471);
#20514=VERTEX_POINT('',#89472);
#20515=VERTEX_POINT('',#89474);
#20516=VERTEX_POINT('',#89476);
#20517=VERTEX_POINT('',#89480);
#20518=VERTEX_POINT('',#89481);
#20519=VERTEX_POINT('',#89483);
#20520=VERTEX_POINT('',#89490);
#20521=VERTEX_POINT('',#89499);
#20522=VERTEX_POINT('',#89500);
#20523=VERTEX_POINT('',#89502);
#20524=VERTEX_POINT('',#89504);
#20525=VERTEX_POINT('',#89513);
#20526=VERTEX_POINT('',#89514);
#20527=VERTEX_POINT('',#89517);
#20528=VERTEX_POINT('',#89519);
#20529=VERTEX_POINT('',#89521);
#20530=VERTEX_POINT('',#89590);
#20531=VERTEX_POINT('',#89591);
#20532=VERTEX_POINT('',#89607);
#20533=VERTEX_POINT('',#89609);
#20534=VERTEX_POINT('',#89611);
#20535=VERTEX_POINT('',#89665);
#20536=VERTEX_POINT('',#89666);
#20537=VERTEX_POINT('',#89669);
#20538=VERTEX_POINT('',#89671);
#20539=VERTEX_POINT('',#89673);
#20540=VERTEX_POINT('',#89715);
#20541=VERTEX_POINT('',#89716);
#20542=VERTEX_POINT('',#89734);
#20543=VERTEX_POINT('',#89735);
#20544=VERTEX_POINT('',#89738);
#20545=VERTEX_POINT('',#89746);
#20546=VERTEX_POINT('',#89784);
#20547=VERTEX_POINT('',#89785);
#20548=VERTEX_POINT('',#89788);
#20549=VERTEX_POINT('',#89790);
#20550=VERTEX_POINT('',#89792);
#20551=VERTEX_POINT('',#89844);
#20552=VERTEX_POINT('',#89845);
#20553=VERTEX_POINT('',#89865);
#20554=VERTEX_POINT('',#89866);
#20555=VERTEX_POINT('',#89869);
#20556=VERTEX_POINT('',#89871);
#20557=VERTEX_POINT('',#89873);
#20558=VERTEX_POINT('',#89908);
#20559=VERTEX_POINT('',#89909);
#20560=VERTEX_POINT('',#89919);
#20561=VERTEX_POINT('',#89920);
#20562=VERTEX_POINT('',#89936);
#20563=VERTEX_POINT('',#89937);
#20564=VERTEX_POINT('',#89940);
#20565=VERTEX_POINT('',#89942);
#20566=VERTEX_POINT('',#89944);
#20567=VERTEX_POINT('',#89983);
#20568=VERTEX_POINT('',#89989);
#20569=VERTEX_POINT('',#89990);
#20570=VERTEX_POINT('',#89992);
#20571=VERTEX_POINT('',#89994);
#20572=VERTEX_POINT('',#89998);
#20573=VERTEX_POINT('',#89999);
#20574=VERTEX_POINT('',#90001);
#20575=VERTEX_POINT('',#90003);
#20576=VERTEX_POINT('',#90007);
#20577=VERTEX_POINT('',#90008);
#20578=VERTEX_POINT('',#90010);
#20579=VERTEX_POINT('',#90012);
#20580=VERTEX_POINT('',#90016);
#20581=VERTEX_POINT('',#90017);
#20582=VERTEX_POINT('',#90019);
#20583=VERTEX_POINT('',#90021);
#20584=VERTEX_POINT('',#90025);
#20585=VERTEX_POINT('',#90026);
#20586=VERTEX_POINT('',#90028);
#20587=VERTEX_POINT('',#90035);
#20588=VERTEX_POINT('',#90059);
#20589=VERTEX_POINT('',#90060);
#20590=VERTEX_POINT('',#90074);
#20591=VERTEX_POINT('',#90076);
#20592=VERTEX_POINT('',#90078);
#20593=VERTEX_POINT('',#90133);
#20594=VERTEX_POINT('',#90134);
#20595=VERTEX_POINT('',#90137);
#20596=VERTEX_POINT('',#90139);
#20597=VERTEX_POINT('',#90141);
#20598=VERTEX_POINT('',#90199);
#20599=VERTEX_POINT('',#90200);
#20600=VERTEX_POINT('',#90203);
#20601=VERTEX_POINT('',#90205);
#20602=VERTEX_POINT('',#90207);
#20603=VERTEX_POINT('',#90249);
#20604=VERTEX_POINT('',#90250);
#20605=VERTEX_POINT('',#90275);
#20606=VERTEX_POINT('',#90276);
#20607=VERTEX_POINT('',#90279);
#20608=VERTEX_POINT('',#90287);
#20609=VERTEX_POINT('',#90318);
#20610=VERTEX_POINT('',#90319);
#20611=VERTEX_POINT('',#90322);
#20612=VERTEX_POINT('',#90324);
#20613=VERTEX_POINT('',#90326);
#20614=VERTEX_POINT('',#90389);
#20615=VERTEX_POINT('',#90390);
#20616=VERTEX_POINT('',#90393);
#20617=VERTEX_POINT('',#90395);
#20618=VERTEX_POINT('',#90397);
#20619=VERTEX_POINT('',#90440);
#20620=VERTEX_POINT('',#90441);
#20621=VERTEX_POINT('',#90457);
#20622=VERTEX_POINT('',#90458);
#20623=VERTEX_POINT('',#90461);
#20624=VERTEX_POINT('',#90463);
#20625=VERTEX_POINT('',#90465);
#20626=VERTEX_POINT('',#90504);
#20627=VERTEX_POINT('',#90510);
#20628=VERTEX_POINT('',#90511);
#20629=VERTEX_POINT('',#90513);
#20630=VERTEX_POINT('',#90515);
#20631=VERTEX_POINT('',#90519);
#20632=VERTEX_POINT('',#90520);
#20633=VERTEX_POINT('',#90522);
#20634=VERTEX_POINT('',#90529);
#20635=VERTEX_POINT('',#90538);
#20636=VERTEX_POINT('',#90539);
#20637=VERTEX_POINT('',#90541);
#20638=VERTEX_POINT('',#90543);
#20639=VERTEX_POINT('',#90547);
#20640=VERTEX_POINT('',#90548);
#20641=VERTEX_POINT('',#90550);
#20642=VERTEX_POINT('',#90552);
#20643=VERTEX_POINT('',#90556);
#20644=VERTEX_POINT('',#90557);
#20645=VERTEX_POINT('',#90559);
#20646=VERTEX_POINT('',#90561);
#20647=VERTEX_POINT('',#90565);
#20648=VERTEX_POINT('',#90566);
#20649=VERTEX_POINT('',#90568);
#20650=VERTEX_POINT('',#90570);
#20651=VERTEX_POINT('',#90579);
#20652=VERTEX_POINT('',#90580);
#20653=VERTEX_POINT('',#90583);
#20654=VERTEX_POINT('',#90585);
#20655=VERTEX_POINT('',#90647);
#20656=VERTEX_POINT('',#90648);
#20657=VERTEX_POINT('',#90651);
#20658=VERTEX_POINT('',#90653);
#20659=VERTEX_POINT('',#90705);
#20660=VERTEX_POINT('',#90706);
#20661=VERTEX_POINT('',#90709);
#20662=VERTEX_POINT('',#90711);
#20663=VERTEX_POINT('',#90713);
#20664=VERTEX_POINT('',#90766);
#20665=VERTEX_POINT('',#90767);
#20666=VERTEX_POINT('',#90770);
#20667=VERTEX_POINT('',#90805);
#20668=VERTEX_POINT('',#90806);
#20669=VERTEX_POINT('',#90809);
#20670=VERTEX_POINT('',#90811);
#20671=VERTEX_POINT('',#90868);
#20672=VERTEX_POINT('',#90869);
#20673=VERTEX_POINT('',#90872);
#20674=VERTEX_POINT('',#90874);
#20675=VERTEX_POINT('',#90937);
#20676=VERTEX_POINT('',#90938);
#20677=VERTEX_POINT('',#90954);
#20678=VERTEX_POINT('',#90956);
#20679=VERTEX_POINT('',#91007);
#20680=VERTEX_POINT('',#91014);
#21274=EDGE_CURVE('',#17225,#17225,#13624,.T.);
#21275=EDGE_CURVE('',#17225,#17226,#9686,.T.);
#21276=EDGE_CURVE('',#17226,#17226,#13625,.T.);
#21277=EDGE_CURVE('',#17227,#17228,#1142,.F.);
#21278=EDGE_CURVE('',#17228,#17229,#9687,.T.);
#21279=EDGE_CURVE('',#17229,#17229,#13626,.T.);
#21280=EDGE_CURVE('',#17228,#17230,#1143,.F.);
#21281=EDGE_CURVE('',#17230,#17231,#13627,.T.);
#21282=EDGE_CURVE('',#17231,#17232,#13628,.T.);
#21283=EDGE_CURVE('',#17232,#17233,#1144,.T.);
#21284=EDGE_CURVE('',#17233,#17234,#1145,.T.);
#21285=EDGE_CURVE('',#17234,#17235,#13629,.T.);
#21286=EDGE_CURVE('',#17235,#17236,#13630,.T.);
#21287=EDGE_CURVE('',#17236,#17237,#1146,.T.);
#21288=EDGE_CURVE('',#17237,#17238,#1147,.T.);
#21289=EDGE_CURVE('',#17238,#17239,#13631,.T.);
#21290=EDGE_CURVE('',#17239,#17240,#13632,.T.);
#21291=EDGE_CURVE('',#17240,#17241,#1148,.T.);
#21292=EDGE_CURVE('',#17241,#17242,#1149,.T.);
#21293=EDGE_CURVE('',#17242,#17243,#13633,.T.);
#21294=EDGE_CURVE('',#17243,#17244,#13634,.T.);
#21295=EDGE_CURVE('',#17244,#17245,#1150,.T.);
#21296=EDGE_CURVE('',#17245,#17246,#1151,.T.);
#21297=EDGE_CURVE('',#17246,#17247,#13635,.T.);
#21298=EDGE_CURVE('',#17247,#17248,#13636,.T.);
#21299=EDGE_CURVE('',#17248,#17249,#1152,.T.);
#21300=EDGE_CURVE('',#17249,#17250,#1153,.T.);
#21301=EDGE_CURVE('',#17250,#17251,#13637,.T.);
#21302=EDGE_CURVE('',#17251,#17252,#13638,.T.);
#21303=EDGE_CURVE('',#17252,#17253,#1154,.T.);
#21304=EDGE_CURVE('',#17253,#17254,#1155,.T.);
#21305=EDGE_CURVE('',#17254,#17255,#13639,.T.);
#21306=EDGE_CURVE('',#17255,#17256,#13640,.T.);
#21307=EDGE_CURVE('',#17256,#17257,#1156,.T.);
#21308=EDGE_CURVE('',#17257,#17258,#1157,.T.);
#21309=EDGE_CURVE('',#17258,#17259,#13641,.T.);
#21310=EDGE_CURVE('',#17259,#17260,#13642,.T.);
#21311=EDGE_CURVE('',#17260,#17261,#1158,.T.);
#21312=EDGE_CURVE('',#17261,#17262,#1159,.T.);
#21313=EDGE_CURVE('',#17262,#17263,#13643,.T.);
#21314=EDGE_CURVE('',#17263,#17264,#13644,.T.);
#21315=EDGE_CURVE('',#17264,#17265,#1160,.T.);
#21316=EDGE_CURVE('',#17265,#17266,#1161,.T.);
#21317=EDGE_CURVE('',#17266,#17267,#13645,.T.);
#21318=EDGE_CURVE('',#17267,#17268,#13646,.T.);
#21319=EDGE_CURVE('',#17268,#17269,#1162,.T.);
#21320=EDGE_CURVE('',#17269,#17270,#1163,.T.);
#21321=EDGE_CURVE('',#17270,#17271,#13647,.T.);
#21322=EDGE_CURVE('',#17271,#17272,#13648,.T.);
#21323=EDGE_CURVE('',#17272,#17273,#1164,.T.);
#21324=EDGE_CURVE('',#17273,#17274,#1165,.T.);
#21325=EDGE_CURVE('',#17274,#17275,#13649,.T.);
#21326=EDGE_CURVE('',#17275,#17276,#13650,.T.);
#21327=EDGE_CURVE('',#17276,#17277,#1166,.T.);
#21328=EDGE_CURVE('',#17277,#17278,#1167,.T.);
#21329=EDGE_CURVE('',#17278,#17279,#13651,.T.);
#21330=EDGE_CURVE('',#17279,#17280,#13652,.T.);
#21331=EDGE_CURVE('',#17280,#17281,#1168,.T.);
#21332=EDGE_CURVE('',#17281,#17282,#1169,.T.);
#21333=EDGE_CURVE('',#17282,#17283,#13653,.T.);
#21334=EDGE_CURVE('',#17283,#17284,#13654,.T.);
#21335=EDGE_CURVE('',#17284,#17285,#1170,.T.);
#21336=EDGE_CURVE('',#17285,#17286,#1171,.T.);
#21337=EDGE_CURVE('',#17286,#17287,#13655,.T.);
#21338=EDGE_CURVE('',#17287,#17288,#13656,.T.);
#21339=EDGE_CURVE('',#17288,#17289,#1172,.T.);
#21340=EDGE_CURVE('',#17289,#17290,#1173,.T.);
#21341=EDGE_CURVE('',#17290,#17291,#13657,.T.);
#21342=EDGE_CURVE('',#17291,#17292,#13658,.T.);
#21343=EDGE_CURVE('',#17292,#17293,#1174,.T.);
#21344=EDGE_CURVE('',#17293,#17294,#1175,.T.);
#21345=EDGE_CURVE('',#17294,#17295,#13659,.T.);
#21346=EDGE_CURVE('',#17295,#17296,#13660,.T.);
#21347=EDGE_CURVE('',#17296,#17297,#1176,.T.);
#21348=EDGE_CURVE('',#17297,#17298,#1177,.T.);
#21349=EDGE_CURVE('',#17298,#17299,#13661,.T.);
#21350=EDGE_CURVE('',#17299,#17300,#13662,.T.);
#21351=EDGE_CURVE('',#17300,#17301,#1178,.T.);
#21352=EDGE_CURVE('',#17301,#17302,#1179,.T.);
#21353=EDGE_CURVE('',#17302,#17303,#13663,.T.);
#21354=EDGE_CURVE('',#17303,#17304,#13664,.T.);
#21355=EDGE_CURVE('',#17304,#17305,#1180,.T.);
#21356=EDGE_CURVE('',#17305,#17306,#1181,.T.);
#21357=EDGE_CURVE('',#17306,#17307,#13665,.T.);
#21358=EDGE_CURVE('',#17307,#17308,#13666,.T.);
#21359=EDGE_CURVE('',#17308,#17309,#1182,.T.);
#21360=EDGE_CURVE('',#17309,#17310,#1183,.T.);
#21361=EDGE_CURVE('',#17310,#17311,#13667,.T.);
#21362=EDGE_CURVE('',#17311,#17312,#13668,.T.);
#21363=EDGE_CURVE('',#17312,#17313,#1184,.T.);
#21364=EDGE_CURVE('',#17313,#17314,#1185,.T.);
#21365=EDGE_CURVE('',#17314,#17315,#13669,.T.);
#21366=EDGE_CURVE('',#17315,#17316,#13670,.T.);
#21367=EDGE_CURVE('',#17316,#17317,#1186,.T.);
#21368=EDGE_CURVE('',#17317,#17318,#1187,.T.);
#21369=EDGE_CURVE('',#17318,#17319,#13671,.T.);
#21370=EDGE_CURVE('',#17319,#17320,#13672,.T.);
#21371=EDGE_CURVE('',#17320,#17321,#1188,.T.);
#21372=EDGE_CURVE('',#17321,#17322,#1189,.T.);
#21373=EDGE_CURVE('',#17322,#17323,#13673,.T.);
#21374=EDGE_CURVE('',#17323,#17324,#13674,.T.);
#21375=EDGE_CURVE('',#17324,#17325,#1190,.T.);
#21376=EDGE_CURVE('',#17325,#17326,#1191,.T.);
#21377=EDGE_CURVE('',#17326,#17327,#13675,.T.);
#21378=EDGE_CURVE('',#17327,#17328,#13676,.T.);
#21379=EDGE_CURVE('',#17328,#17329,#1192,.T.);
#21380=EDGE_CURVE('',#17329,#17330,#1193,.T.);
#21381=EDGE_CURVE('',#17330,#17331,#13677,.T.);
#21382=EDGE_CURVE('',#17331,#17332,#13678,.T.);
#21383=EDGE_CURVE('',#17332,#17333,#1194,.T.);
#21384=EDGE_CURVE('',#17333,#17334,#1195,.T.);
#21385=EDGE_CURVE('',#17334,#17335,#13679,.T.);
#21386=EDGE_CURVE('',#17335,#17336,#13680,.T.);
#21387=EDGE_CURVE('',#17336,#17337,#1196,.T.);
#21388=EDGE_CURVE('',#17337,#17338,#1197,.T.);
#21389=EDGE_CURVE('',#17338,#17339,#13681,.T.);
#21390=EDGE_CURVE('',#17339,#17340,#13682,.T.);
#21391=EDGE_CURVE('',#17340,#17341,#1198,.T.);
#21392=EDGE_CURVE('',#17341,#17342,#1199,.T.);
#21393=EDGE_CURVE('',#17342,#17343,#13683,.T.);
#21394=EDGE_CURVE('',#17343,#17344,#13684,.T.);
#21395=EDGE_CURVE('',#17344,#17345,#1200,.T.);
#21396=EDGE_CURVE('',#17345,#17346,#1201,.T.);
#21397=EDGE_CURVE('',#17346,#17347,#13685,.T.);
#21398=EDGE_CURVE('',#17347,#17348,#13686,.T.);
#21399=EDGE_CURVE('',#17348,#17349,#1202,.T.);
#21400=EDGE_CURVE('',#17349,#17350,#1203,.T.);
#21401=EDGE_CURVE('',#17350,#17351,#13687,.T.);
#21402=EDGE_CURVE('',#17351,#17352,#13688,.T.);
#21403=EDGE_CURVE('',#17352,#17353,#1204,.T.);
#21404=EDGE_CURVE('',#17353,#17354,#1205,.T.);
#21405=EDGE_CURVE('',#17354,#17355,#13689,.T.);
#21406=EDGE_CURVE('',#17355,#17356,#13690,.T.);
#21407=EDGE_CURVE('',#17356,#17357,#1206,.T.);
#21408=EDGE_CURVE('',#17357,#17358,#1207,.T.);
#21409=EDGE_CURVE('',#17358,#17359,#13691,.T.);
#21410=EDGE_CURVE('',#17359,#17360,#13692,.T.);
#21411=EDGE_CURVE('',#17360,#17361,#1208,.T.);
#21412=EDGE_CURVE('',#17361,#17362,#1209,.T.);
#21413=EDGE_CURVE('',#17362,#17363,#13693,.T.);
#21414=EDGE_CURVE('',#17363,#17364,#13694,.T.);
#21415=EDGE_CURVE('',#17364,#17365,#1210,.T.);
#21416=EDGE_CURVE('',#17365,#17366,#1211,.T.);
#21417=EDGE_CURVE('',#17366,#17367,#13695,.T.);
#21418=EDGE_CURVE('',#17367,#17368,#13696,.T.);
#21419=EDGE_CURVE('',#17368,#17369,#1212,.T.);
#21420=EDGE_CURVE('',#17369,#17370,#1213,.T.);
#21421=EDGE_CURVE('',#17370,#17371,#13697,.T.);
#21422=EDGE_CURVE('',#17371,#17372,#13698,.T.);
#21423=EDGE_CURVE('',#17372,#17373,#1214,.T.);
#21424=EDGE_CURVE('',#17373,#17374,#1215,.T.);
#21425=EDGE_CURVE('',#17374,#17375,#13699,.T.);
#21426=EDGE_CURVE('',#17375,#17376,#13700,.T.);
#21427=EDGE_CURVE('',#17376,#17377,#1216,.T.);
#21428=EDGE_CURVE('',#17377,#17378,#1217,.T.);
#21429=EDGE_CURVE('',#17378,#17379,#13701,.T.);
#21430=EDGE_CURVE('',#17379,#17380,#13702,.T.);
#21431=EDGE_CURVE('',#17380,#17381,#1218,.T.);
#21432=EDGE_CURVE('',#17381,#17382,#1219,.T.);
#21433=EDGE_CURVE('',#17382,#17383,#13703,.T.);
#21434=EDGE_CURVE('',#17383,#17384,#13704,.T.);
#21435=EDGE_CURVE('',#17384,#17385,#1220,.T.);
#21436=EDGE_CURVE('',#17385,#17386,#1221,.T.);
#21437=EDGE_CURVE('',#17386,#17387,#13705,.T.);
#21438=EDGE_CURVE('',#17387,#17388,#13706,.T.);
#21439=EDGE_CURVE('',#17388,#17389,#1222,.T.);
#21440=EDGE_CURVE('',#17389,#17390,#1223,.T.);
#21441=EDGE_CURVE('',#17390,#17391,#13707,.T.);
#21442=EDGE_CURVE('',#17391,#17392,#13708,.T.);
#21443=EDGE_CURVE('',#17392,#17393,#1224,.T.);
#21444=EDGE_CURVE('',#17393,#17394,#1225,.T.);
#21445=EDGE_CURVE('',#17394,#17395,#13709,.T.);
#21446=EDGE_CURVE('',#17395,#17396,#13710,.T.);
#21447=EDGE_CURVE('',#17396,#17397,#1226,.T.);
#21448=EDGE_CURVE('',#17397,#17398,#1227,.T.);
#21449=EDGE_CURVE('',#17398,#17399,#13711,.T.);
#21450=EDGE_CURVE('',#17399,#17400,#13712,.T.);
#21451=EDGE_CURVE('',#17400,#17401,#1228,.T.);
#21452=EDGE_CURVE('',#17401,#17402,#1229,.T.);
#21453=EDGE_CURVE('',#17402,#17403,#13713,.T.);
#21454=EDGE_CURVE('',#17403,#17404,#13714,.T.);
#21455=EDGE_CURVE('',#17404,#17405,#1230,.T.);
#21456=EDGE_CURVE('',#17405,#17406,#1231,.T.);
#21457=EDGE_CURVE('',#17406,#17407,#13715,.T.);
#21458=EDGE_CURVE('',#17407,#17408,#13716,.T.);
#21459=EDGE_CURVE('',#17408,#17409,#1232,.T.);
#21460=EDGE_CURVE('',#17409,#17410,#1233,.T.);
#21461=EDGE_CURVE('',#17410,#17411,#13717,.T.);
#21462=EDGE_CURVE('',#17411,#17412,#13718,.T.);
#21463=EDGE_CURVE('',#17412,#17413,#1234,.T.);
#21464=EDGE_CURVE('',#17413,#17414,#1235,.T.);
#21465=EDGE_CURVE('',#17414,#17415,#13719,.T.);
#21466=EDGE_CURVE('',#17415,#17416,#13720,.T.);
#21467=EDGE_CURVE('',#17416,#17417,#1236,.T.);
#21468=EDGE_CURVE('',#17417,#17418,#1237,.T.);
#21469=EDGE_CURVE('',#17418,#17419,#13721,.T.);
#21470=EDGE_CURVE('',#17419,#17420,#13722,.T.);
#21471=EDGE_CURVE('',#17420,#17421,#1238,.T.);
#21472=EDGE_CURVE('',#17421,#17422,#1239,.T.);
#21473=EDGE_CURVE('',#17422,#17423,#13723,.T.);
#21474=EDGE_CURVE('',#17423,#17424,#13724,.T.);
#21475=EDGE_CURVE('',#17424,#17425,#1240,.T.);
#21476=EDGE_CURVE('',#17425,#17426,#1241,.T.);
#21477=EDGE_CURVE('',#17426,#17427,#13725,.T.);
#21478=EDGE_CURVE('',#17427,#17428,#13726,.T.);
#21479=EDGE_CURVE('',#17428,#17227,#1242,.T.);
#21480=EDGE_CURVE('',#17429,#17430,#1243,.F.);
#21481=EDGE_CURVE('',#17430,#17431,#9688,.T.);
#21482=EDGE_CURVE('',#17431,#17431,#13727,.T.);
#21483=EDGE_CURVE('',#17430,#17432,#1244,.F.);
#21484=EDGE_CURVE('',#17432,#17433,#13728,.T.);
#21485=EDGE_CURVE('',#17433,#17434,#13729,.T.);
#21486=EDGE_CURVE('',#17434,#17435,#13730,.T.);
#21487=EDGE_CURVE('',#17435,#17436,#13731,.T.);
#21488=EDGE_CURVE('',#17436,#17437,#1245,.T.);
#21489=EDGE_CURVE('',#17437,#17438,#13732,.T.);
#21490=EDGE_CURVE('',#17438,#17439,#13733,.T.);
#21491=EDGE_CURVE('',#17439,#17440,#13734,.T.);
#21492=EDGE_CURVE('',#17440,#17441,#13735,.T.);
#21493=EDGE_CURVE('',#17441,#17442,#13736,.T.);
#21494=EDGE_CURVE('',#17442,#17443,#1246,.T.);
#21495=EDGE_CURVE('',#17443,#17444,#13737,.T.);
#21496=EDGE_CURVE('',#17444,#17445,#13738,.T.);
#21497=EDGE_CURVE('',#17445,#17446,#13739,.T.);
#21498=EDGE_CURVE('',#17446,#17447,#13740,.T.);
#21499=EDGE_CURVE('',#17447,#17448,#13741,.T.);
#21500=EDGE_CURVE('',#17448,#17449,#1247,.T.);
#21501=EDGE_CURVE('',#17449,#17450,#13742,.T.);
#21502=EDGE_CURVE('',#17450,#17451,#13743,.T.);
#21503=EDGE_CURVE('',#17451,#17452,#13744,.T.);
#21504=EDGE_CURVE('',#17452,#17453,#13745,.T.);
#21505=EDGE_CURVE('',#17453,#17454,#13746,.T.);
#21506=EDGE_CURVE('',#17454,#17455,#1248,.T.);
#21507=EDGE_CURVE('',#17455,#17456,#13747,.T.);
#21508=EDGE_CURVE('',#17456,#17457,#13748,.T.);
#21509=EDGE_CURVE('',#17457,#17458,#13749,.T.);
#21510=EDGE_CURVE('',#17458,#17459,#13750,.T.);
#21511=EDGE_CURVE('',#17459,#17460,#13751,.T.);
#21512=EDGE_CURVE('',#17460,#17461,#1249,.T.);
#21513=EDGE_CURVE('',#17461,#17462,#13752,.T.);
#21514=EDGE_CURVE('',#17462,#17463,#13753,.T.);
#21515=EDGE_CURVE('',#17463,#17464,#13754,.T.);
#21516=EDGE_CURVE('',#17464,#17465,#13755,.T.);
#21517=EDGE_CURVE('',#17465,#17466,#13756,.T.);
#21518=EDGE_CURVE('',#17466,#17467,#1250,.T.);
#21519=EDGE_CURVE('',#17467,#17468,#13757,.T.);
#21520=EDGE_CURVE('',#17468,#17469,#13758,.T.);
#21521=EDGE_CURVE('',#17469,#17470,#13759,.T.);
#21522=EDGE_CURVE('',#17470,#17471,#13760,.T.);
#21523=EDGE_CURVE('',#17471,#17472,#13761,.T.);
#21524=EDGE_CURVE('',#17472,#17473,#1251,.T.);
#21525=EDGE_CURVE('',#17473,#17474,#13762,.T.);
#21526=EDGE_CURVE('',#17474,#17475,#13763,.T.);
#21527=EDGE_CURVE('',#17475,#17476,#13764,.T.);
#21528=EDGE_CURVE('',#17476,#17477,#13765,.T.);
#21529=EDGE_CURVE('',#17477,#17478,#13766,.T.);
#21530=EDGE_CURVE('',#17478,#17479,#1252,.T.);
#21531=EDGE_CURVE('',#17479,#17480,#13767,.T.);
#21532=EDGE_CURVE('',#17480,#17481,#13768,.T.);
#21533=EDGE_CURVE('',#17481,#17482,#13769,.T.);
#21534=EDGE_CURVE('',#17482,#17483,#13770,.T.);
#21535=EDGE_CURVE('',#17483,#17484,#13771,.T.);
#21536=EDGE_CURVE('',#17484,#17485,#1253,.T.);
#21537=EDGE_CURVE('',#17485,#17486,#13772,.T.);
#21538=EDGE_CURVE('',#17486,#17487,#13773,.T.);
#21539=EDGE_CURVE('',#17487,#17488,#13774,.T.);
#21540=EDGE_CURVE('',#17488,#17489,#13775,.T.);
#21541=EDGE_CURVE('',#17489,#17490,#13776,.T.);
#21542=EDGE_CURVE('',#17490,#17491,#1254,.T.);
#21543=EDGE_CURVE('',#17491,#17492,#13777,.T.);
#21544=EDGE_CURVE('',#17492,#17493,#13778,.T.);
#21545=EDGE_CURVE('',#17493,#17494,#13779,.T.);
#21546=EDGE_CURVE('',#17494,#17495,#13780,.T.);
#21547=EDGE_CURVE('',#17495,#17496,#13781,.T.);
#21548=EDGE_CURVE('',#17496,#17497,#1255,.T.);
#21549=EDGE_CURVE('',#17497,#17498,#13782,.T.);
#21550=EDGE_CURVE('',#17498,#17499,#13783,.T.);
#21551=EDGE_CURVE('',#17499,#17500,#13784,.T.);
#21552=EDGE_CURVE('',#17500,#17501,#13785,.T.);
#21553=EDGE_CURVE('',#17501,#17502,#13786,.T.);
#21554=EDGE_CURVE('',#17502,#17503,#1256,.T.);
#21555=EDGE_CURVE('',#17503,#17504,#13787,.T.);
#21556=EDGE_CURVE('',#17504,#17505,#13788,.T.);
#21557=EDGE_CURVE('',#17505,#17506,#13789,.T.);
#21558=EDGE_CURVE('',#17506,#17507,#13790,.T.);
#21559=EDGE_CURVE('',#17507,#17508,#13791,.T.);
#21560=EDGE_CURVE('',#17508,#17509,#1257,.T.);
#21561=EDGE_CURVE('',#17509,#17510,#13792,.T.);
#21562=EDGE_CURVE('',#17510,#17511,#13793,.T.);
#21563=EDGE_CURVE('',#17511,#17512,#13794,.T.);
#21564=EDGE_CURVE('',#17512,#17513,#13795,.T.);
#21565=EDGE_CURVE('',#17513,#17514,#13796,.T.);
#21566=EDGE_CURVE('',#17514,#17515,#1258,.T.);
#21567=EDGE_CURVE('',#17515,#17516,#13797,.T.);
#21568=EDGE_CURVE('',#17516,#17517,#13798,.T.);
#21569=EDGE_CURVE('',#17517,#17518,#13799,.T.);
#21570=EDGE_CURVE('',#17518,#17519,#13800,.T.);
#21571=EDGE_CURVE('',#17519,#17520,#13801,.T.);
#21572=EDGE_CURVE('',#17520,#17521,#1259,.T.);
#21573=EDGE_CURVE('',#17521,#17522,#13802,.T.);
#21574=EDGE_CURVE('',#17522,#17523,#13803,.T.);
#21575=EDGE_CURVE('',#17523,#17524,#13804,.T.);
#21576=EDGE_CURVE('',#17524,#17525,#13805,.T.);
#21577=EDGE_CURVE('',#17525,#17526,#13806,.T.);
#21578=EDGE_CURVE('',#17526,#17527,#1260,.T.);
#21579=EDGE_CURVE('',#17527,#17528,#13807,.T.);
#21580=EDGE_CURVE('',#17528,#17529,#13808,.T.);
#21581=EDGE_CURVE('',#17529,#17530,#13809,.T.);
#21582=EDGE_CURVE('',#17530,#17531,#13810,.T.);
#21583=EDGE_CURVE('',#17531,#17532,#13811,.T.);
#21584=EDGE_CURVE('',#17532,#17533,#1261,.T.);
#21585=EDGE_CURVE('',#17533,#17534,#13812,.T.);
#21586=EDGE_CURVE('',#17534,#17535,#13813,.T.);
#21587=EDGE_CURVE('',#17535,#17536,#13814,.T.);
#21588=EDGE_CURVE('',#17536,#17537,#13815,.T.);
#21589=EDGE_CURVE('',#17537,#17538,#13816,.T.);
#21590=EDGE_CURVE('',#17538,#17539,#1262,.T.);
#21591=EDGE_CURVE('',#17539,#17540,#13817,.T.);
#21592=EDGE_CURVE('',#17540,#17541,#13818,.T.);
#21593=EDGE_CURVE('',#17541,#17542,#13819,.T.);
#21594=EDGE_CURVE('',#17542,#17543,#13820,.T.);
#21595=EDGE_CURVE('',#17543,#17544,#13821,.T.);
#21596=EDGE_CURVE('',#17544,#17545,#1263,.T.);
#21597=EDGE_CURVE('',#17545,#17546,#13822,.T.);
#21598=EDGE_CURVE('',#17546,#17547,#13823,.T.);
#21599=EDGE_CURVE('',#17547,#17548,#13824,.T.);
#21600=EDGE_CURVE('',#17548,#17549,#13825,.T.);
#21601=EDGE_CURVE('',#17549,#17550,#13826,.T.);
#21602=EDGE_CURVE('',#17550,#17551,#1264,.T.);
#21603=EDGE_CURVE('',#17551,#17552,#13827,.T.);
#21604=EDGE_CURVE('',#17552,#17553,#13828,.T.);
#21605=EDGE_CURVE('',#17553,#17554,#13829,.T.);
#21606=EDGE_CURVE('',#17554,#17555,#13830,.T.);
#21607=EDGE_CURVE('',#17555,#17556,#13831,.T.);
#21608=EDGE_CURVE('',#17556,#17557,#1265,.T.);
#21609=EDGE_CURVE('',#17557,#17558,#13832,.T.);
#21610=EDGE_CURVE('',#17558,#17559,#13833,.T.);
#21611=EDGE_CURVE('',#17559,#17560,#13834,.T.);
#21612=EDGE_CURVE('',#17560,#17561,#13835,.T.);
#21613=EDGE_CURVE('',#17561,#17562,#13836,.T.);
#21614=EDGE_CURVE('',#17562,#17563,#1266,.T.);
#21615=EDGE_CURVE('',#17563,#17564,#13837,.T.);
#21616=EDGE_CURVE('',#17564,#17565,#13838,.T.);
#21617=EDGE_CURVE('',#17565,#17566,#13839,.T.);
#21618=EDGE_CURVE('',#17566,#17567,#13840,.T.);
#21619=EDGE_CURVE('',#17567,#17568,#13841,.T.);
#21620=EDGE_CURVE('',#17568,#17569,#1267,.T.);
#21621=EDGE_CURVE('',#17569,#17570,#13842,.T.);
#21622=EDGE_CURVE('',#17570,#17571,#13843,.T.);
#21623=EDGE_CURVE('',#17571,#17572,#13844,.T.);
#21624=EDGE_CURVE('',#17572,#17573,#13845,.T.);
#21625=EDGE_CURVE('',#17573,#17574,#13846,.T.);
#21626=EDGE_CURVE('',#17574,#17575,#1268,.T.);
#21627=EDGE_CURVE('',#17575,#17576,#13847,.T.);
#21628=EDGE_CURVE('',#17576,#17577,#13848,.T.);
#21629=EDGE_CURVE('',#17577,#17578,#13849,.T.);
#21630=EDGE_CURVE('',#17578,#17579,#13850,.T.);
#21631=EDGE_CURVE('',#17579,#17580,#13851,.T.);
#21632=EDGE_CURVE('',#17580,#17581,#1269,.T.);
#21633=EDGE_CURVE('',#17581,#17582,#13852,.T.);
#21634=EDGE_CURVE('',#17582,#17583,#13853,.T.);
#21635=EDGE_CURVE('',#17583,#17584,#13854,.T.);
#21636=EDGE_CURVE('',#17584,#17585,#13855,.T.);
#21637=EDGE_CURVE('',#17585,#17586,#13856,.T.);
#21638=EDGE_CURVE('',#17586,#17587,#1270,.T.);
#21639=EDGE_CURVE('',#17587,#17588,#13857,.T.);
#21640=EDGE_CURVE('',#17588,#17589,#13858,.T.);
#21641=EDGE_CURVE('',#17589,#17590,#13859,.T.);
#21642=EDGE_CURVE('',#17590,#17591,#13860,.T.);
#21643=EDGE_CURVE('',#17591,#17592,#13861,.T.);
#21644=EDGE_CURVE('',#17592,#17593,#1271,.T.);
#21645=EDGE_CURVE('',#17593,#17594,#13862,.T.);
#21646=EDGE_CURVE('',#17594,#17595,#13863,.T.);
#21647=EDGE_CURVE('',#17595,#17596,#13864,.T.);
#21648=EDGE_CURVE('',#17596,#17597,#13865,.T.);
#21649=EDGE_CURVE('',#17597,#17598,#13866,.T.);
#21650=EDGE_CURVE('',#17598,#17599,#1272,.T.);
#21651=EDGE_CURVE('',#17599,#17600,#13867,.T.);
#21652=EDGE_CURVE('',#17600,#17601,#13868,.T.);
#21653=EDGE_CURVE('',#17601,#17602,#13869,.T.);
#21654=EDGE_CURVE('',#17602,#17603,#13870,.T.);
#21655=EDGE_CURVE('',#17603,#17604,#13871,.T.);
#21656=EDGE_CURVE('',#17604,#17605,#1273,.T.);
#21657=EDGE_CURVE('',#17605,#17606,#13872,.T.);
#21658=EDGE_CURVE('',#17606,#17607,#13873,.T.);
#21659=EDGE_CURVE('',#17607,#17608,#13874,.T.);
#21660=EDGE_CURVE('',#17608,#17609,#13875,.T.);
#21661=EDGE_CURVE('',#17609,#17610,#13876,.T.);
#21662=EDGE_CURVE('',#17610,#17611,#1274,.T.);
#21663=EDGE_CURVE('',#17611,#17612,#13877,.T.);
#21664=EDGE_CURVE('',#17612,#17613,#13878,.T.);
#21665=EDGE_CURVE('',#17613,#17614,#13879,.T.);
#21666=EDGE_CURVE('',#17614,#17615,#13880,.T.);
#21667=EDGE_CURVE('',#17615,#17616,#13881,.T.);
#21668=EDGE_CURVE('',#17616,#17617,#1275,.T.);
#21669=EDGE_CURVE('',#17617,#17618,#13882,.T.);
#21670=EDGE_CURVE('',#17618,#17619,#13883,.T.);
#21671=EDGE_CURVE('',#17619,#17620,#13884,.T.);
#21672=EDGE_CURVE('',#17620,#17621,#13885,.T.);
#21673=EDGE_CURVE('',#17621,#17622,#13886,.T.);
#21674=EDGE_CURVE('',#17622,#17623,#1276,.T.);
#21675=EDGE_CURVE('',#17623,#17624,#13887,.T.);
#21676=EDGE_CURVE('',#17624,#17625,#13888,.T.);
#21677=EDGE_CURVE('',#17625,#17626,#13889,.T.);
#21678=EDGE_CURVE('',#17626,#17627,#13890,.T.);
#21679=EDGE_CURVE('',#17627,#17628,#13891,.T.);
#21680=EDGE_CURVE('',#17628,#17629,#1277,.T.);
#21681=EDGE_CURVE('',#17629,#17630,#13892,.T.);
#21682=EDGE_CURVE('',#17630,#17631,#13893,.T.);
#21683=EDGE_CURVE('',#17631,#17632,#13894,.T.);
#21684=EDGE_CURVE('',#17632,#17633,#13895,.T.);
#21685=EDGE_CURVE('',#17633,#17634,#13896,.T.);
#21686=EDGE_CURVE('',#17634,#17635,#1278,.T.);
#21687=EDGE_CURVE('',#17635,#17636,#13897,.T.);
#21688=EDGE_CURVE('',#17636,#17637,#13898,.T.);
#21689=EDGE_CURVE('',#17637,#17638,#13899,.T.);
#21690=EDGE_CURVE('',#17638,#17639,#13900,.T.);
#21691=EDGE_CURVE('',#17639,#17640,#13901,.T.);
#21692=EDGE_CURVE('',#17640,#17641,#1279,.T.);
#21693=EDGE_CURVE('',#17641,#17642,#13902,.T.);
#21694=EDGE_CURVE('',#17642,#17643,#13903,.T.);
#21695=EDGE_CURVE('',#17643,#17644,#13904,.T.);
#21696=EDGE_CURVE('',#17644,#17645,#13905,.T.);
#21697=EDGE_CURVE('',#17645,#17646,#13906,.T.);
#21698=EDGE_CURVE('',#17646,#17647,#1280,.T.);
#21699=EDGE_CURVE('',#17647,#17648,#13907,.T.);
#21700=EDGE_CURVE('',#17648,#17649,#13908,.T.);
#21701=EDGE_CURVE('',#17649,#17650,#13909,.T.);
#21702=EDGE_CURVE('',#17650,#17651,#13910,.T.);
#21703=EDGE_CURVE('',#17651,#17652,#13911,.T.);
#21704=EDGE_CURVE('',#17652,#17653,#1281,.T.);
#21705=EDGE_CURVE('',#17653,#17654,#13912,.T.);
#21706=EDGE_CURVE('',#17654,#17655,#13913,.T.);
#21707=EDGE_CURVE('',#17655,#17656,#13914,.T.);
#21708=EDGE_CURVE('',#17656,#17657,#13915,.T.);
#21709=EDGE_CURVE('',#17657,#17658,#13916,.T.);
#21710=EDGE_CURVE('',#17658,#17659,#1282,.T.);
#21711=EDGE_CURVE('',#17659,#17660,#13917,.T.);
#21712=EDGE_CURVE('',#17660,#17661,#13918,.T.);
#21713=EDGE_CURVE('',#17661,#17662,#13919,.T.);
#21714=EDGE_CURVE('',#17662,#17663,#13920,.T.);
#21715=EDGE_CURVE('',#17663,#17664,#13921,.T.);
#21716=EDGE_CURVE('',#17664,#17665,#1283,.T.);
#21717=EDGE_CURVE('',#17665,#17666,#13922,.T.);
#21718=EDGE_CURVE('',#17666,#17667,#13923,.T.);
#21719=EDGE_CURVE('',#17667,#17668,#13924,.T.);
#21720=EDGE_CURVE('',#17668,#17669,#13925,.T.);
#21721=EDGE_CURVE('',#17669,#17670,#13926,.T.);
#21722=EDGE_CURVE('',#17670,#17671,#1284,.T.);
#21723=EDGE_CURVE('',#17671,#17672,#13927,.T.);
#21724=EDGE_CURVE('',#17672,#17673,#13928,.T.);
#21725=EDGE_CURVE('',#17673,#17674,#13929,.T.);
#21726=EDGE_CURVE('',#17674,#17675,#13930,.T.);
#21727=EDGE_CURVE('',#17675,#17676,#13931,.T.);
#21728=EDGE_CURVE('',#17676,#17677,#1285,.T.);
#21729=EDGE_CURVE('',#17677,#17678,#13932,.T.);
#21730=EDGE_CURVE('',#17678,#17679,#13933,.T.);
#21731=EDGE_CURVE('',#17679,#17680,#13934,.T.);
#21732=EDGE_CURVE('',#17680,#17681,#13935,.T.);
#21733=EDGE_CURVE('',#17681,#17682,#13936,.T.);
#21734=EDGE_CURVE('',#17682,#17683,#1286,.T.);
#21735=EDGE_CURVE('',#17683,#17684,#13937,.T.);
#21736=EDGE_CURVE('',#17684,#17685,#13938,.T.);
#21737=EDGE_CURVE('',#17685,#17686,#13939,.T.);
#21738=EDGE_CURVE('',#17686,#17687,#13940,.T.);
#21739=EDGE_CURVE('',#17687,#17688,#13941,.T.);
#21740=EDGE_CURVE('',#17688,#17689,#1287,.T.);
#21741=EDGE_CURVE('',#17689,#17690,#13942,.T.);
#21742=EDGE_CURVE('',#17690,#17691,#13943,.T.);
#21743=EDGE_CURVE('',#17691,#17692,#13944,.T.);
#21744=EDGE_CURVE('',#17692,#17693,#13945,.T.);
#21745=EDGE_CURVE('',#17693,#17694,#13946,.T.);
#21746=EDGE_CURVE('',#17694,#17695,#1288,.T.);
#21747=EDGE_CURVE('',#17695,#17696,#13947,.T.);
#21748=EDGE_CURVE('',#17696,#17697,#13948,.T.);
#21749=EDGE_CURVE('',#17697,#17698,#13949,.T.);
#21750=EDGE_CURVE('',#17698,#17699,#13950,.T.);
#21751=EDGE_CURVE('',#17699,#17700,#13951,.T.);
#21752=EDGE_CURVE('',#17700,#17701,#1289,.T.);
#21753=EDGE_CURVE('',#17701,#17702,#13952,.T.);
#21754=EDGE_CURVE('',#17702,#17703,#13953,.T.);
#21755=EDGE_CURVE('',#17703,#17704,#13954,.T.);
#21756=EDGE_CURVE('',#17704,#17705,#13955,.T.);
#21757=EDGE_CURVE('',#17705,#17706,#13956,.T.);
#21758=EDGE_CURVE('',#17706,#17707,#1290,.T.);
#21759=EDGE_CURVE('',#17707,#17708,#13957,.T.);
#21760=EDGE_CURVE('',#17708,#17709,#13958,.T.);
#21761=EDGE_CURVE('',#17709,#17710,#13959,.T.);
#21762=EDGE_CURVE('',#17710,#17711,#13960,.T.);
#21763=EDGE_CURVE('',#17711,#17712,#13961,.T.);
#21764=EDGE_CURVE('',#17712,#17713,#1291,.T.);
#21765=EDGE_CURVE('',#17713,#17714,#13962,.T.);
#21766=EDGE_CURVE('',#17714,#17715,#13963,.T.);
#21767=EDGE_CURVE('',#17715,#17716,#13964,.T.);
#21768=EDGE_CURVE('',#17716,#17717,#13965,.T.);
#21769=EDGE_CURVE('',#17717,#17718,#13966,.T.);
#21770=EDGE_CURVE('',#17718,#17719,#1292,.T.);
#21771=EDGE_CURVE('',#17719,#17720,#13967,.T.);
#21772=EDGE_CURVE('',#17720,#17721,#13968,.T.);
#21773=EDGE_CURVE('',#17721,#17722,#13969,.T.);
#21774=EDGE_CURVE('',#17722,#17723,#13970,.T.);
#21775=EDGE_CURVE('',#17723,#17724,#13971,.T.);
#21776=EDGE_CURVE('',#17724,#17725,#1293,.T.);
#21777=EDGE_CURVE('',#17725,#17726,#13972,.T.);
#21778=EDGE_CURVE('',#17726,#17727,#13973,.T.);
#21779=EDGE_CURVE('',#17727,#17728,#13974,.T.);
#21780=EDGE_CURVE('',#17728,#17729,#13975,.T.);
#21781=EDGE_CURVE('',#17729,#17730,#13976,.T.);
#21782=EDGE_CURVE('',#17730,#17429,#1294,.T.);
#21783=EDGE_CURVE('',#17731,#17732,#13977,.T.);
#21784=EDGE_CURVE('',#17732,#17421,#13978,.T.);
#21785=EDGE_CURVE('',#17733,#17420,#1295,.T.);
#21786=EDGE_CURVE('',#17733,#17734,#886,.T.);
#21787=EDGE_CURVE('',#17734,#17731,#9689,.T.);
#21788=EDGE_CURVE('',#17735,#17736,#13979,.T.);
#21789=EDGE_CURVE('',#17735,#17732,#1296,.T.);
#21790=EDGE_CURVE('',#17731,#17736,#9690,.T.);
#21791=EDGE_CURVE('',#17737,#17738,#13980,.T.);
#21792=EDGE_CURVE('',#17738,#17739,#13981,.T.);
#21793=EDGE_CURVE('',#17739,#17740,#9691,.T.);
#21794=EDGE_CURVE('',#17741,#17740,#13982,.T.);
#21795=EDGE_CURVE('',#17741,#17742,#13983,.T.);
#21796=EDGE_CURVE('',#17742,#17737,#9692,.T.);
#21797=EDGE_CURVE('',#17743,#17424,#1297,.T.);
#21798=EDGE_CURVE('',#17743,#17739,#887,.T.);
#21799=EDGE_CURVE('',#17739,#17744,#9693,.T.);
#21800=EDGE_CURVE('',#17744,#17745,#13984,.T.);
#21801=EDGE_CURVE('',#17745,#17425,#13985,.T.);
#21802=EDGE_CURVE('',#17746,#17747,#13986,.T.);
#21803=EDGE_CURVE('',#17746,#17738,#1298,.T.);
#21804=EDGE_CURVE('',#17737,#17747,#9694,.T.);
#21805=EDGE_CURVE('',#17744,#17748,#9695,.T.);
#21806=EDGE_CURVE('',#17749,#17748,#13987,.T.);
#21807=EDGE_CURVE('',#17749,#17745,#1299,.T.);
#21808=EDGE_CURVE('',#17750,#17751,#13988,.T.);
#21809=EDGE_CURVE('',#17751,#17735,#13989,.T.);
#21810=EDGE_CURVE('',#17736,#17750,#13990,.T.);
#21811=EDGE_CURVE('',#17740,#17751,#9696,.T.);
#21812=EDGE_CURVE('',#17750,#17741,#1300,.T.);
#21813=EDGE_CURVE('',#17423,#17743,#888,.T.);
#21814=EDGE_CURVE('',#17752,#17753,#13991,.T.);
#21815=EDGE_CURVE('',#17753,#17746,#13992,.T.);
#21816=EDGE_CURVE('',#17747,#17752,#13993,.T.);
#21817=EDGE_CURVE('',#17748,#17754,#13994,.T.);
#21818=EDGE_CURVE('',#17754,#17755,#13995,.T.);
#21819=EDGE_CURVE('',#17755,#17749,#13996,.T.);
#21820=EDGE_CURVE('',#17756,#17757,#13997,.T.);
#21821=EDGE_CURVE('',#17757,#17758,#13998,.T.);
#21822=EDGE_CURVE('',#17758,#17759,#9697,.T.);
#21823=EDGE_CURVE('',#17760,#17759,#13999,.T.);
#21824=EDGE_CURVE('',#17760,#17761,#14000,.T.);
#21825=EDGE_CURVE('',#17761,#17756,#9698,.T.);
#21826=EDGE_CURVE('',#17762,#17763,#14001,.T.);
#21827=EDGE_CURVE('',#17762,#17758,#14002,.T.);
#21828=EDGE_CURVE('',#17758,#17764,#9699,.T.);
#21829=EDGE_CURVE('',#17764,#17765,#14003,.T.);
#21830=EDGE_CURVE('',#17765,#17766,#14004,.T.);
#21831=EDGE_CURVE('',#17766,#17763,#9700,.T.);
#21832=EDGE_CURVE('',#17759,#17753,#9701,.T.);
#21833=EDGE_CURVE('',#17752,#17760,#1301,.T.);
#21834=EDGE_CURVE('',#17754,#17762,#1302,.T.);
#21835=EDGE_CURVE('',#17763,#17755,#9702,.T.);
#21836=EDGE_CURVE('',#17767,#17768,#14005,.T.);
#21837=EDGE_CURVE('',#17767,#17757,#1303,.T.);
#21838=EDGE_CURVE('',#17756,#17768,#9703,.T.);
#21839=EDGE_CURVE('',#17764,#17769,#9704,.T.);
#21840=EDGE_CURVE('',#17770,#17769,#14006,.T.);
#21841=EDGE_CURVE('',#17770,#17765,#1304,.T.);
#21842=EDGE_CURVE('',#17771,#17772,#14007,.T.);
#21843=EDGE_CURVE('',#17772,#17767,#14008,.T.);
#21844=EDGE_CURVE('',#17768,#17771,#14009,.T.);
#21845=EDGE_CURVE('',#17769,#17773,#14010,.T.);
#21846=EDGE_CURVE('',#17773,#17774,#14011,.T.);
#21847=EDGE_CURVE('',#17774,#17770,#14012,.T.);
#21848=EDGE_CURVE('',#17775,#17776,#1305,.T.);
#21849=EDGE_CURVE('',#17776,#17777,#1306,.T.);
#21850=EDGE_CURVE('',#17777,#17778,#9705,.T.);
#21851=EDGE_CURVE('',#17779,#17778,#14013,.T.);
#21852=EDGE_CURVE('',#17779,#17780,#14014,.T.);
#21853=EDGE_CURVE('',#17780,#17775,#9706,.T.);
#21854=EDGE_CURVE('',#17781,#17782,#14015,.T.);
#21855=EDGE_CURVE('',#17781,#17777,#14016,.T.);
#21856=EDGE_CURVE('',#17777,#17783,#9707,.T.);
#21857=EDGE_CURVE('',#17783,#17784,#14017,.T.);
#21858=EDGE_CURVE('',#17784,#17785,#14018,.T.);
#21859=EDGE_CURVE('',#17785,#17782,#9708,.T.);
#21860=EDGE_CURVE('',#17778,#17772,#9709,.T.);
#21861=EDGE_CURVE('',#17771,#17779,#1307,.T.);
#21862=EDGE_CURVE('',#17773,#17781,#1308,.T.);
#21863=EDGE_CURVE('',#17782,#17774,#9710,.T.);
#21864=EDGE_CURVE('',#17786,#17787,#1309,.T.);
#21865=EDGE_CURVE('',#17786,#17776,#1310,.T.);
#21866=EDGE_CURVE('',#17775,#17787,#9711,.T.);
#21867=EDGE_CURVE('',#17783,#17788,#9712,.T.);
#21868=EDGE_CURVE('',#17789,#17788,#14019,.T.);
#21869=EDGE_CURVE('',#17789,#17784,#1311,.T.);
#21870=EDGE_CURVE('',#17790,#17791,#14020,.T.);
#21871=EDGE_CURVE('',#17791,#17786,#1312,.T.);
#21872=EDGE_CURVE('',#17787,#17790,#14021,.T.);
#21873=EDGE_CURVE('',#17788,#17792,#14022,.T.);
#21874=EDGE_CURVE('',#17792,#17793,#14023,.T.);
#21875=EDGE_CURVE('',#17793,#17789,#14024,.T.);
#21876=EDGE_CURVE('',#17794,#17795,#14025,.T.);
#21877=EDGE_CURVE('',#17795,#17796,#14026,.T.);
#21878=EDGE_CURVE('',#17796,#17797,#9713,.T.);
#21879=EDGE_CURVE('',#17798,#17797,#14027,.T.);
#21880=EDGE_CURVE('',#17798,#17799,#14028,.T.);
#21881=EDGE_CURVE('',#17799,#17794,#9714,.T.);
#21882=EDGE_CURVE('',#17800,#17801,#14029,.T.);
#21883=EDGE_CURVE('',#17800,#17796,#14030,.T.);
#21884=EDGE_CURVE('',#17796,#17802,#9715,.T.);
#21885=EDGE_CURVE('',#17802,#17803,#1313,.T.);
#21886=EDGE_CURVE('',#17803,#17804,#1314,.T.);
#21887=EDGE_CURVE('',#17804,#17801,#9716,.T.);
#21888=EDGE_CURVE('',#17797,#17791,#9717,.T.);
#21889=EDGE_CURVE('',#17790,#17798,#1315,.T.);
#21890=EDGE_CURVE('',#17792,#17800,#1316,.T.);
#21891=EDGE_CURVE('',#17801,#17793,#9718,.T.);
#21892=EDGE_CURVE('',#17805,#17806,#14031,.T.);
#21893=EDGE_CURVE('',#17805,#17795,#1317,.T.);
#21894=EDGE_CURVE('',#17794,#17806,#9719,.T.);
#21895=EDGE_CURVE('',#17802,#17807,#9720,.T.);
#21896=EDGE_CURVE('',#17808,#17807,#1318,.T.);
#21897=EDGE_CURVE('',#17808,#17803,#1319,.T.);
#21898=EDGE_CURVE('',#17809,#17810,#14032,.T.);
#21899=EDGE_CURVE('',#17810,#17805,#14033,.T.);
#21900=EDGE_CURVE('',#17806,#17809,#14034,.T.);
#21901=EDGE_CURVE('',#17807,#17811,#14035,.T.);
#21902=EDGE_CURVE('',#17811,#17812,#14036,.T.);
#21903=EDGE_CURVE('',#17812,#17808,#1320,.T.);
#21904=EDGE_CURVE('',#17813,#17814,#14037,.T.);
#21905=EDGE_CURVE('',#17814,#17815,#14038,.T.);
#21906=EDGE_CURVE('',#17815,#17816,#9721,.T.);
#21907=EDGE_CURVE('',#17817,#17816,#14039,.T.);
#21908=EDGE_CURVE('',#17817,#17818,#14040,.T.);
#21909=EDGE_CURVE('',#17818,#17813,#9722,.T.);
#21910=EDGE_CURVE('',#17819,#17820,#14041,.T.);
#21911=EDGE_CURVE('',#17819,#17815,#14042,.T.);
#21912=EDGE_CURVE('',#17815,#17821,#9723,.T.);
#21913=EDGE_CURVE('',#17821,#17822,#14043,.T.);
#21914=EDGE_CURVE('',#17822,#17823,#14044,.T.);
#21915=EDGE_CURVE('',#17823,#17820,#9724,.T.);
#21916=EDGE_CURVE('',#17816,#17810,#9725,.T.);
#21917=EDGE_CURVE('',#17809,#17817,#1321,.T.);
#21918=EDGE_CURVE('',#17811,#17819,#1322,.T.);
#21919=EDGE_CURVE('',#17820,#17812,#9726,.T.);
#21920=EDGE_CURVE('',#17824,#17825,#14045,.T.);
#21921=EDGE_CURVE('',#17824,#17814,#1323,.T.);
#21922=EDGE_CURVE('',#17813,#17825,#9727,.T.);
#21923=EDGE_CURVE('',#17821,#17826,#9728,.T.);
#21924=EDGE_CURVE('',#17827,#17826,#14046,.T.);
#21925=EDGE_CURVE('',#17827,#17822,#1324,.T.);
#21926=EDGE_CURVE('',#17828,#17829,#14047,.T.);
#21927=EDGE_CURVE('',#17829,#17824,#14048,.T.);
#21928=EDGE_CURVE('',#17825,#17828,#14049,.T.);
#21929=EDGE_CURVE('',#17826,#17830,#14050,.T.);
#21930=EDGE_CURVE('',#17830,#17831,#14051,.T.);
#21931=EDGE_CURVE('',#17831,#17827,#14052,.T.);
#21932=EDGE_CURVE('',#17832,#17833,#14053,.T.);
#21933=EDGE_CURVE('',#17833,#17834,#14054,.T.);
#21934=EDGE_CURVE('',#17834,#17835,#9729,.T.);
#21935=EDGE_CURVE('',#17836,#17835,#14055,.T.);
#21936=EDGE_CURVE('',#17836,#17837,#14056,.T.);
#21937=EDGE_CURVE('',#17837,#17832,#9730,.F.);
#21938=EDGE_CURVE('',#17838,#17839,#14057,.T.);
#21939=EDGE_CURVE('',#17838,#17834,#14058,.T.);
#21940=EDGE_CURVE('',#17834,#17840,#9731,.T.);
#21941=EDGE_CURVE('',#17840,#17841,#14059,.T.);
#21942=EDGE_CURVE('',#17841,#17842,#14060,.T.);
#21943=EDGE_CURVE('',#17842,#17839,#9732,.T.);
#21944=EDGE_CURVE('',#17835,#17829,#9733,.T.);
#21945=EDGE_CURVE('',#17828,#17836,#1325,.T.);
#21946=EDGE_CURVE('',#17830,#17838,#1326,.T.);
#21947=EDGE_CURVE('',#17839,#17831,#9734,.T.);
#21948=EDGE_CURVE('',#17576,#17833,#14061,.T.);
#21949=EDGE_CURVE('',#17832,#17577,#9735,.F.);
#21950=EDGE_CURVE('',#17840,#17843,#9736,.T.);
#21951=EDGE_CURVE('',#17844,#17843,#14062,.T.);
#21952=EDGE_CURVE('',#17844,#17841,#1327,.T.);
#21953=EDGE_CURVE('',#17843,#17845,#14063,.T.);
#21954=EDGE_CURVE('',#17845,#17846,#14064,.T.);
#21955=EDGE_CURVE('',#17846,#17844,#14065,.T.);
#21956=EDGE_CURVE('',#17573,#17847,#889,.T.);
#21957=EDGE_CURVE('',#17847,#17848,#9737,.T.);
#21958=EDGE_CURVE('',#17574,#17848,#890,.T.);
#21959=EDGE_CURVE('',#17849,#17850,#14066,.T.);
#21960=EDGE_CURVE('',#17849,#17847,#14067,.T.);
#21961=EDGE_CURVE('',#17847,#17851,#9738,.F.);
#21962=EDGE_CURVE('',#17851,#17852,#14068,.T.);
#21963=EDGE_CURVE('',#17852,#17853,#14069,.T.);
#21964=EDGE_CURVE('',#17853,#17850,#9739,.T.);
#21965=EDGE_CURVE('',#17848,#17575,#891,.T.);
#21966=EDGE_CURVE('',#17845,#17849,#1328,.T.);
#21967=EDGE_CURVE('',#17850,#17846,#9740,.T.);
#21968=EDGE_CURVE('',#17851,#17571,#9741,.F.);
#21969=EDGE_CURVE('',#17570,#17852,#14070,.T.);
#21970=EDGE_CURVE('',#17854,#17855,#14071,.T.);
#21971=EDGE_CURVE('',#17855,#17417,#14072,.T.);
#21972=EDGE_CURVE('',#17856,#17416,#1329,.T.);
#21973=EDGE_CURVE('',#17856,#17857,#892,.T.);
#21974=EDGE_CURVE('',#17857,#17854,#9742,.T.);
#21975=EDGE_CURVE('',#17858,#17859,#14073,.T.);
#21976=EDGE_CURVE('',#17858,#17855,#1330,.T.);
#21977=EDGE_CURVE('',#17854,#17859,#9743,.T.);
#21978=EDGE_CURVE('',#17860,#17861,#14074,.T.);
#21979=EDGE_CURVE('',#17861,#17858,#14075,.T.);
#21980=EDGE_CURVE('',#17859,#17860,#14076,.T.);
#21981=EDGE_CURVE('',#17862,#17863,#14077,.T.);
#21982=EDGE_CURVE('',#17863,#17734,#14078,.T.);
#21983=EDGE_CURVE('',#17734,#17864,#9744,.T.);
#21984=EDGE_CURVE('',#17865,#17864,#14079,.T.);
#21985=EDGE_CURVE('',#17865,#17866,#14080,.T.);
#21986=EDGE_CURVE('',#17866,#17862,#9745,.T.);
#21987=EDGE_CURVE('',#17864,#17861,#9746,.T.);
#21988=EDGE_CURVE('',#17860,#17865,#1331,.T.);
#21989=EDGE_CURVE('',#17419,#17733,#893,.T.);
#21990=EDGE_CURVE('',#17867,#17868,#14081,.T.);
#21991=EDGE_CURVE('',#17867,#17863,#1332,.T.);
#21992=EDGE_CURVE('',#17862,#17868,#9747,.T.);
#21993=EDGE_CURVE('',#17869,#17870,#14082,.T.);
#21994=EDGE_CURVE('',#17870,#17742,#14083,.T.);
#21995=EDGE_CURVE('',#17742,#17871,#9748,.T.);
#21996=EDGE_CURVE('',#17872,#17871,#14084,.T.);
#21997=EDGE_CURVE('',#17872,#17873,#14085,.T.);
#21998=EDGE_CURVE('',#17873,#17869,#9749,.T.);
#21999=EDGE_CURVE('',#17874,#17875,#14086,.T.);
#22000=EDGE_CURVE('',#17874,#17870,#1333,.T.);
#22001=EDGE_CURVE('',#17869,#17875,#9750,.T.);
#22002=EDGE_CURVE('',#17876,#17877,#14087,.T.);
#22003=EDGE_CURVE('',#17877,#17867,#14088,.T.);
#22004=EDGE_CURVE('',#17868,#17876,#14089,.T.);
#22005=EDGE_CURVE('',#17871,#17877,#9751,.T.);
#22006=EDGE_CURVE('',#17876,#17872,#1334,.T.);
#22007=EDGE_CURVE('',#17878,#17879,#14090,.T.);
#22008=EDGE_CURVE('',#17879,#17874,#14091,.T.);
#22009=EDGE_CURVE('',#17875,#17878,#14092,.T.);
#22010=EDGE_CURVE('',#17880,#17881,#1335,.T.);
#22011=EDGE_CURVE('',#17881,#17761,#1336,.T.);
#22012=EDGE_CURVE('',#17761,#17882,#9752,.T.);
#22013=EDGE_CURVE('',#17883,#17882,#14093,.T.);
#22014=EDGE_CURVE('',#17883,#17884,#14094,.T.);
#22015=EDGE_CURVE('',#17884,#17880,#9753,.T.);
#22016=EDGE_CURVE('',#17882,#17879,#9754,.T.);
#22017=EDGE_CURVE('',#17878,#17883,#1337,.T.);
#22018=EDGE_CURVE('',#17885,#17886,#1338,.T.);
#22019=EDGE_CURVE('',#17885,#17881,#1339,.T.);
#22020=EDGE_CURVE('',#17880,#17886,#9755,.T.);
#22021=EDGE_CURVE('',#17887,#17888,#14095,.T.);
#22022=EDGE_CURVE('',#17888,#17885,#1340,.T.);
#22023=EDGE_CURVE('',#17886,#17887,#14096,.T.);
#22024=EDGE_CURVE('',#17889,#17890,#14097,.T.);
#22025=EDGE_CURVE('',#17890,#17780,#14098,.T.);
#22026=EDGE_CURVE('',#17780,#17891,#9756,.T.);
#22027=EDGE_CURVE('',#17892,#17891,#14099,.T.);
#22028=EDGE_CURVE('',#17892,#17893,#14100,.T.);
#22029=EDGE_CURVE('',#17893,#17889,#9757,.T.);
#22030=EDGE_CURVE('',#17891,#17888,#9758,.T.);
#22031=EDGE_CURVE('',#17887,#17892,#1341,.T.);
#22032=EDGE_CURVE('',#17894,#17895,#14101,.T.);
#22033=EDGE_CURVE('',#17894,#17890,#1342,.T.);
#22034=EDGE_CURVE('',#17889,#17895,#9759,.T.);
#22035=EDGE_CURVE('',#17896,#17897,#14102,.T.);
#22036=EDGE_CURVE('',#17897,#17894,#14103,.T.);
#22037=EDGE_CURVE('',#17895,#17896,#14104,.T.);
#22038=EDGE_CURVE('',#17898,#17899,#14105,.T.);
#22039=EDGE_CURVE('',#17899,#17799,#14106,.T.);
#22040=EDGE_CURVE('',#17799,#17900,#9760,.T.);
#22041=EDGE_CURVE('',#17901,#17900,#14107,.T.);
#22042=EDGE_CURVE('',#17901,#17902,#14108,.T.);
#22043=EDGE_CURVE('',#17902,#17898,#9761,.T.);
#22044=EDGE_CURVE('',#17900,#17897,#9762,.T.);
#22045=EDGE_CURVE('',#17896,#17901,#1343,.T.);
#22046=EDGE_CURVE('',#17903,#17904,#14109,.T.);
#22047=EDGE_CURVE('',#17903,#17899,#1344,.T.);
#22048=EDGE_CURVE('',#17898,#17904,#9763,.T.);
#22049=EDGE_CURVE('',#17905,#17906,#14110,.T.);
#22050=EDGE_CURVE('',#17906,#17903,#14111,.T.);
#22051=EDGE_CURVE('',#17904,#17905,#14112,.T.);
#22052=EDGE_CURVE('',#17907,#17908,#14113,.T.);
#22053=EDGE_CURVE('',#17908,#17818,#14114,.T.);
#22054=EDGE_CURVE('',#17818,#17909,#9764,.T.);
#22055=EDGE_CURVE('',#17910,#17909,#14115,.T.);
#22056=EDGE_CURVE('',#17910,#17911,#14116,.T.);
#22057=EDGE_CURVE('',#17911,#17907,#9765,.F.);
#22058=EDGE_CURVE('',#17909,#17906,#9766,.T.);
#22059=EDGE_CURVE('',#17905,#17910,#1345,.T.);
#22060=EDGE_CURVE('',#17582,#17908,#14117,.T.);
#22061=EDGE_CURVE('',#17907,#17583,#9767,.F.);
#22062=EDGE_CURVE('',#17579,#17837,#894,.T.);
#22063=EDGE_CURVE('',#17837,#17912,#9768,.T.);
#22064=EDGE_CURVE('',#17580,#17912,#895,.T.);
#22065=EDGE_CURVE('',#17912,#17581,#896,.T.);
#22066=EDGE_CURVE('',#17913,#17914,#14118,.T.);
#22067=EDGE_CURVE('',#17914,#17413,#14119,.T.);
#22068=EDGE_CURVE('',#17915,#17412,#1346,.T.);
#22069=EDGE_CURVE('',#17915,#17916,#897,.T.);
#22070=EDGE_CURVE('',#17916,#17913,#9769,.T.);
#22071=EDGE_CURVE('',#17917,#17918,#14120,.T.);
#22072=EDGE_CURVE('',#17917,#17914,#1347,.T.);
#22073=EDGE_CURVE('',#17913,#17918,#9770,.T.);
#22074=EDGE_CURVE('',#17919,#17920,#14121,.T.);
#22075=EDGE_CURVE('',#17920,#17917,#14122,.T.);
#22076=EDGE_CURVE('',#17918,#17919,#14123,.T.);
#22077=EDGE_CURVE('',#17921,#17922,#14124,.T.);
#22078=EDGE_CURVE('',#17922,#17857,#14125,.T.);
#22079=EDGE_CURVE('',#17857,#17923,#9771,.T.);
#22080=EDGE_CURVE('',#17924,#17923,#14126,.T.);
#22081=EDGE_CURVE('',#17924,#17925,#14127,.T.);
#22082=EDGE_CURVE('',#17925,#17921,#9772,.T.);
#22083=EDGE_CURVE('',#17923,#17920,#9773,.T.);
#22084=EDGE_CURVE('',#17919,#17924,#1348,.T.);
#22085=EDGE_CURVE('',#17415,#17856,#898,.T.);
#22086=EDGE_CURVE('',#17926,#17927,#14128,.T.);
#22087=EDGE_CURVE('',#17926,#17922,#1349,.T.);
#22088=EDGE_CURVE('',#17921,#17927,#9774,.T.);
#22089=EDGE_CURVE('',#17928,#17929,#14129,.T.);
#22090=EDGE_CURVE('',#17929,#17926,#14130,.T.);
#22091=EDGE_CURVE('',#17927,#17928,#14131,.T.);
#22092=EDGE_CURVE('',#17930,#17931,#14132,.T.);
#22093=EDGE_CURVE('',#17931,#17866,#14133,.T.);
#22094=EDGE_CURVE('',#17866,#17932,#9775,.T.);
#22095=EDGE_CURVE('',#17933,#17932,#14134,.T.);
#22096=EDGE_CURVE('',#17933,#17934,#14135,.T.);
#22097=EDGE_CURVE('',#17934,#17930,#9776,.T.);
#22098=EDGE_CURVE('',#17932,#17929,#9777,.T.);
#22099=EDGE_CURVE('',#17928,#17933,#1350,.T.);
#22100=EDGE_CURVE('',#17935,#17936,#14136,.T.);
#22101=EDGE_CURVE('',#17935,#17931,#1351,.T.);
#22102=EDGE_CURVE('',#17930,#17936,#9778,.T.);
#22103=EDGE_CURVE('',#17937,#17938,#1352,.T.);
#22104=EDGE_CURVE('',#17938,#17873,#1353,.T.);
#22105=EDGE_CURVE('',#17873,#17939,#9779,.T.);
#22106=EDGE_CURVE('',#17940,#17939,#14137,.T.);
#22107=EDGE_CURVE('',#17940,#17941,#14138,.T.);
#22108=EDGE_CURVE('',#17941,#17937,#9780,.T.);
#22109=EDGE_CURVE('',#17942,#17943,#1354,.T.);
#22110=EDGE_CURVE('',#17942,#17938,#1355,.T.);
#22111=EDGE_CURVE('',#17937,#17943,#9781,.T.);
#22112=EDGE_CURVE('',#17944,#17945,#14139,.T.);
#22113=EDGE_CURVE('',#17945,#17935,#14140,.T.);
#22114=EDGE_CURVE('',#17936,#17944,#14141,.T.);
#22115=EDGE_CURVE('',#17939,#17945,#9782,.T.);
#22116=EDGE_CURVE('',#17944,#17940,#1356,.T.);
#22117=EDGE_CURVE('',#17946,#17947,#14142,.T.);
#22118=EDGE_CURVE('',#17947,#17942,#1357,.T.);
#22119=EDGE_CURVE('',#17943,#17946,#14143,.T.);
#22120=EDGE_CURVE('',#17948,#17949,#14144,.T.);
#22121=EDGE_CURVE('',#17949,#17884,#14145,.T.);
#22122=EDGE_CURVE('',#17884,#17950,#9783,.T.);
#22123=EDGE_CURVE('',#17951,#17950,#14146,.T.);
#22124=EDGE_CURVE('',#17951,#17952,#14147,.T.);
#22125=EDGE_CURVE('',#17952,#17948,#9784,.T.);
#22126=EDGE_CURVE('',#17950,#17947,#9785,.T.);
#22127=EDGE_CURVE('',#17946,#17951,#1358,.T.);
#22128=EDGE_CURVE('',#17953,#17954,#14148,.T.);
#22129=EDGE_CURVE('',#17953,#17949,#1359,.T.);
#22130=EDGE_CURVE('',#17948,#17954,#9786,.T.);
#22131=EDGE_CURVE('',#17955,#17956,#14149,.T.);
#22132=EDGE_CURVE('',#17956,#17953,#14150,.T.);
#22133=EDGE_CURVE('',#17954,#17955,#14151,.T.);
#22134=EDGE_CURVE('',#17957,#17958,#14152,.T.);
#22135=EDGE_CURVE('',#17958,#17893,#14153,.T.);
#22136=EDGE_CURVE('',#17893,#17959,#9787,.T.);
#22137=EDGE_CURVE('',#17960,#17959,#14154,.T.);
#22138=EDGE_CURVE('',#17960,#17961,#14155,.T.);
#22139=EDGE_CURVE('',#17961,#17957,#9788,.T.);
#22140=EDGE_CURVE('',#17959,#17956,#9789,.T.);
#22141=EDGE_CURVE('',#17955,#17960,#1360,.T.);
#22142=EDGE_CURVE('',#17962,#17963,#14156,.T.);
#22143=EDGE_CURVE('',#17962,#17958,#1361,.T.);
#22144=EDGE_CURVE('',#17957,#17963,#9790,.T.);
#22145=EDGE_CURVE('',#17964,#17965,#14157,.T.);
#22146=EDGE_CURVE('',#17965,#17962,#14158,.T.);
#22147=EDGE_CURVE('',#17963,#17964,#14159,.T.);
#22148=EDGE_CURVE('',#17966,#17967,#14160,.T.);
#22149=EDGE_CURVE('',#17967,#17902,#14161,.T.);
#22150=EDGE_CURVE('',#17902,#17968,#9791,.T.);
#22151=EDGE_CURVE('',#17969,#17968,#14162,.T.);
#22152=EDGE_CURVE('',#17969,#17970,#14163,.T.);
#22153=EDGE_CURVE('',#17970,#17966,#9792,.F.);
#22154=EDGE_CURVE('',#17968,#17965,#9793,.T.);
#22155=EDGE_CURVE('',#17964,#17969,#1362,.T.);
#22156=EDGE_CURVE('',#17588,#17967,#14164,.T.);
#22157=EDGE_CURVE('',#17966,#17589,#9794,.F.);
#22158=EDGE_CURVE('',#17585,#17911,#899,.T.);
#22159=EDGE_CURVE('',#17911,#17971,#9795,.T.);
#22160=EDGE_CURVE('',#17586,#17971,#900,.T.);
#22161=EDGE_CURVE('',#17971,#17587,#901,.T.);
#22162=EDGE_CURVE('',#17972,#17973,#14165,.T.);
#22163=EDGE_CURVE('',#17973,#17409,#14166,.T.);
#22164=EDGE_CURVE('',#17974,#17408,#1363,.T.);
#22165=EDGE_CURVE('',#17974,#17975,#902,.T.);
#22166=EDGE_CURVE('',#17975,#17972,#9796,.T.);
#22167=EDGE_CURVE('',#17976,#17977,#14167,.T.);
#22168=EDGE_CURVE('',#17976,#17973,#1364,.T.);
#22169=EDGE_CURVE('',#17972,#17977,#9797,.T.);
#22170=EDGE_CURVE('',#17978,#17979,#14168,.T.);
#22171=EDGE_CURVE('',#17979,#17976,#14169,.T.);
#22172=EDGE_CURVE('',#17977,#17978,#14170,.T.);
#22173=EDGE_CURVE('',#17980,#17981,#14171,.T.);
#22174=EDGE_CURVE('',#17981,#17916,#14172,.T.);
#22175=EDGE_CURVE('',#17916,#17982,#9798,.T.);
#22176=EDGE_CURVE('',#17983,#17982,#14173,.T.);
#22177=EDGE_CURVE('',#17983,#17984,#14174,.T.);
#22178=EDGE_CURVE('',#17984,#17980,#9799,.T.);
#22179=EDGE_CURVE('',#17982,#17979,#9800,.T.);
#22180=EDGE_CURVE('',#17978,#17983,#1365,.T.);
#22181=EDGE_CURVE('',#17411,#17915,#903,.T.);
#22182=EDGE_CURVE('',#17985,#17986,#14175,.T.);
#22183=EDGE_CURVE('',#17985,#17981,#1366,.T.);
#22184=EDGE_CURVE('',#17980,#17986,#9801,.T.);
#22185=EDGE_CURVE('',#17987,#17988,#14176,.T.);
#22186=EDGE_CURVE('',#17988,#17985,#14177,.T.);
#22187=EDGE_CURVE('',#17986,#17987,#14178,.T.);
#22188=EDGE_CURVE('',#17989,#17990,#14179,.T.);
#22189=EDGE_CURVE('',#17990,#17925,#14180,.T.);
#22190=EDGE_CURVE('',#17925,#17991,#9802,.T.);
#22191=EDGE_CURVE('',#17992,#17991,#14181,.T.);
#22192=EDGE_CURVE('',#17992,#17993,#14182,.T.);
#22193=EDGE_CURVE('',#17993,#17989,#9803,.T.);
#22194=EDGE_CURVE('',#17991,#17988,#9804,.T.);
#22195=EDGE_CURVE('',#17987,#17992,#1367,.T.);
#22196=EDGE_CURVE('',#17994,#17995,#14183,.T.);
#22197=EDGE_CURVE('',#17994,#17990,#1368,.T.);
#22198=EDGE_CURVE('',#17989,#17995,#9805,.T.);
#22199=EDGE_CURVE('',#17996,#17997,#14184,.T.);
#22200=EDGE_CURVE('',#17997,#17994,#14185,.T.);
#22201=EDGE_CURVE('',#17995,#17996,#14186,.T.);
#22202=EDGE_CURVE('',#17998,#17999,#1369,.T.);
#22203=EDGE_CURVE('',#17999,#17934,#1370,.T.);
#22204=EDGE_CURVE('',#17934,#18000,#9806,.T.);
#22205=EDGE_CURVE('',#18001,#18000,#14187,.T.);
#22206=EDGE_CURVE('',#18001,#18002,#14188,.T.);
#22207=EDGE_CURVE('',#18002,#17998,#9807,.T.);
#22208=EDGE_CURVE('',#18000,#17997,#9808,.T.);
#22209=EDGE_CURVE('',#17996,#18001,#1371,.T.);
#22210=EDGE_CURVE('',#18003,#18004,#1372,.T.);
#22211=EDGE_CURVE('',#18003,#17999,#1373,.T.);
#22212=EDGE_CURVE('',#17998,#18004,#9809,.T.);
#22213=EDGE_CURVE('',#18005,#18006,#14189,.T.);
#22214=EDGE_CURVE('',#18006,#17941,#14190,.T.);
#22215=EDGE_CURVE('',#17941,#18007,#9810,.T.);
#22216=EDGE_CURVE('',#18008,#18007,#14191,.T.);
#22217=EDGE_CURVE('',#18008,#18009,#14192,.T.);
#22218=EDGE_CURVE('',#18009,#18005,#9811,.T.);
#22219=EDGE_CURVE('',#18010,#18011,#14193,.T.);
#22220=EDGE_CURVE('',#18010,#18006,#1374,.T.);
#22221=EDGE_CURVE('',#18005,#18011,#9812,.T.);
#22222=EDGE_CURVE('',#18012,#18013,#14194,.T.);
#22223=EDGE_CURVE('',#18013,#18003,#1375,.T.);
#22224=EDGE_CURVE('',#18004,#18012,#14195,.T.);
#22225=EDGE_CURVE('',#18007,#18013,#9813,.T.);
#22226=EDGE_CURVE('',#18012,#18008,#1376,.T.);
#22227=EDGE_CURVE('',#18014,#18015,#14196,.T.);
#22228=EDGE_CURVE('',#18015,#18010,#14197,.T.);
#22229=EDGE_CURVE('',#18011,#18014,#14198,.T.);
#22230=EDGE_CURVE('',#18016,#18017,#14199,.T.);
#22231=EDGE_CURVE('',#18017,#17952,#14200,.T.);
#22232=EDGE_CURVE('',#17952,#18018,#9814,.T.);
#22233=EDGE_CURVE('',#18019,#18018,#14201,.T.);
#22234=EDGE_CURVE('',#18019,#18020,#14202,.T.);
#22235=EDGE_CURVE('',#18020,#18016,#9815,.T.);
#22236=EDGE_CURVE('',#18018,#18015,#9816,.T.);
#22237=EDGE_CURVE('',#18014,#18019,#1377,.T.);
#22238=EDGE_CURVE('',#18021,#18022,#14203,.T.);
#22239=EDGE_CURVE('',#18021,#18017,#1378,.T.);
#22240=EDGE_CURVE('',#18016,#18022,#9817,.T.);
#22241=EDGE_CURVE('',#18023,#18024,#14204,.T.);
#22242=EDGE_CURVE('',#18024,#18021,#14205,.T.);
#22243=EDGE_CURVE('',#18022,#18023,#14206,.T.);
#22244=EDGE_CURVE('',#18025,#18026,#14207,.T.);
#22245=EDGE_CURVE('',#18026,#17961,#14208,.T.);
#22246=EDGE_CURVE('',#17961,#18027,#9818,.T.);
#22247=EDGE_CURVE('',#18028,#18027,#14209,.T.);
#22248=EDGE_CURVE('',#18028,#18029,#14210,.T.);
#22249=EDGE_CURVE('',#18029,#18025,#9819,.F.);
#22250=EDGE_CURVE('',#18027,#18024,#9820,.T.);
#22251=EDGE_CURVE('',#18023,#18028,#1379,.T.);
#22252=EDGE_CURVE('',#17594,#18026,#14211,.T.);
#22253=EDGE_CURVE('',#18025,#17595,#9821,.F.);
#22254=EDGE_CURVE('',#17591,#17970,#904,.T.);
#22255=EDGE_CURVE('',#17970,#18030,#9822,.T.);
#22256=EDGE_CURVE('',#17592,#18030,#905,.T.);
#22257=EDGE_CURVE('',#18030,#17593,#906,.T.);
#22258=EDGE_CURVE('',#18031,#18032,#14212,.T.);
#22259=EDGE_CURVE('',#18032,#17405,#14213,.T.);
#22260=EDGE_CURVE('',#18033,#17404,#1380,.T.);
#22261=EDGE_CURVE('',#18033,#18034,#907,.T.);
#22262=EDGE_CURVE('',#18034,#18031,#9823,.T.);
#22263=EDGE_CURVE('',#18035,#18036,#14214,.T.);
#22264=EDGE_CURVE('',#18035,#18032,#1381,.T.);
#22265=EDGE_CURVE('',#18031,#18036,#9824,.T.);
#22266=EDGE_CURVE('',#18037,#18038,#14215,.T.);
#22267=EDGE_CURVE('',#18038,#18035,#14216,.T.);
#22268=EDGE_CURVE('',#18036,#18037,#14217,.T.);
#22269=EDGE_CURVE('',#18039,#18040,#14218,.T.);
#22270=EDGE_CURVE('',#18040,#17975,#14219,.T.);
#22271=EDGE_CURVE('',#17975,#18041,#9825,.T.);
#22272=EDGE_CURVE('',#18042,#18041,#14220,.T.);
#22273=EDGE_CURVE('',#18042,#18043,#14221,.T.);
#22274=EDGE_CURVE('',#18043,#18039,#9826,.T.);
#22275=EDGE_CURVE('',#18041,#18038,#9827,.T.);
#22276=EDGE_CURVE('',#18037,#18042,#1382,.T.);
#22277=EDGE_CURVE('',#17407,#17974,#908,.T.);
#22278=EDGE_CURVE('',#18044,#18045,#14222,.T.);
#22279=EDGE_CURVE('',#18044,#18040,#1383,.T.);
#22280=EDGE_CURVE('',#18039,#18045,#9828,.T.);
#22281=EDGE_CURVE('',#18046,#18047,#14223,.T.);
#22282=EDGE_CURVE('',#18047,#18044,#14224,.T.);
#22283=EDGE_CURVE('',#18045,#18046,#14225,.T.);
#22284=EDGE_CURVE('',#18048,#18049,#14226,.T.);
#22285=EDGE_CURVE('',#18049,#17984,#14227,.T.);
#22286=EDGE_CURVE('',#17984,#18050,#9829,.T.);
#22287=EDGE_CURVE('',#18051,#18050,#14228,.T.);
#22288=EDGE_CURVE('',#18051,#18052,#14229,.T.);
#22289=EDGE_CURVE('',#18052,#18048,#9830,.T.);
#22290=EDGE_CURVE('',#18050,#18047,#9831,.T.);
#22291=EDGE_CURVE('',#18046,#18051,#1384,.T.);
#22292=EDGE_CURVE('',#18053,#18054,#14230,.T.);
#22293=EDGE_CURVE('',#18053,#18049,#1385,.T.);
#22294=EDGE_CURVE('',#18048,#18054,#9832,.T.);
#22295=EDGE_CURVE('',#18055,#18056,#14231,.T.);
#22296=EDGE_CURVE('',#18056,#18053,#14232,.T.);
#22297=EDGE_CURVE('',#18054,#18055,#14233,.T.);
#22298=EDGE_CURVE('',#18057,#18058,#1386,.T.);
#22299=EDGE_CURVE('',#18058,#17993,#1387,.T.);
#22300=EDGE_CURVE('',#17993,#18059,#9833,.T.);
#22301=EDGE_CURVE('',#18060,#18059,#14234,.T.);
#22302=EDGE_CURVE('',#18060,#18061,#14235,.T.);
#22303=EDGE_CURVE('',#18061,#18057,#9834,.T.);
#22304=EDGE_CURVE('',#18059,#18056,#9835,.T.);
#22305=EDGE_CURVE('',#18055,#18060,#1388,.T.);
#22306=EDGE_CURVE('',#18062,#18063,#1389,.T.);
#22307=EDGE_CURVE('',#18062,#18058,#1390,.T.);
#22308=EDGE_CURVE('',#18057,#18063,#9836,.T.);
#22309=EDGE_CURVE('',#18064,#18065,#14236,.T.);
#22310=EDGE_CURVE('',#18065,#18062,#1391,.T.);
#22311=EDGE_CURVE('',#18063,#18064,#14237,.T.);
#22312=EDGE_CURVE('',#18066,#18067,#14238,.T.);
#22313=EDGE_CURVE('',#18067,#18002,#14239,.T.);
#22314=EDGE_CURVE('',#18002,#18068,#9837,.T.);
#22315=EDGE_CURVE('',#18069,#18068,#14240,.T.);
#22316=EDGE_CURVE('',#18069,#18070,#14241,.T.);
#22317=EDGE_CURVE('',#18070,#18066,#9838,.T.);
#22318=EDGE_CURVE('',#18068,#18065,#9839,.T.);
#22319=EDGE_CURVE('',#18064,#18069,#1392,.T.);
#22320=EDGE_CURVE('',#18071,#18072,#14242,.T.);
#22321=EDGE_CURVE('',#18071,#18067,#1393,.T.);
#22322=EDGE_CURVE('',#18066,#18072,#9840,.T.);
#22323=EDGE_CURVE('',#18073,#18074,#14243,.T.);
#22324=EDGE_CURVE('',#18074,#18009,#14244,.T.);
#22325=EDGE_CURVE('',#18009,#18075,#9841,.T.);
#22326=EDGE_CURVE('',#18076,#18075,#14245,.T.);
#22327=EDGE_CURVE('',#18076,#18077,#14246,.T.);
#22328=EDGE_CURVE('',#18077,#18073,#9842,.T.);
#22329=EDGE_CURVE('',#18078,#18079,#14247,.T.);
#22330=EDGE_CURVE('',#18078,#18074,#1394,.T.);
#22331=EDGE_CURVE('',#18073,#18079,#9843,.T.);
#22332=EDGE_CURVE('',#18080,#18081,#14248,.T.);
#22333=EDGE_CURVE('',#18081,#18071,#14249,.T.);
#22334=EDGE_CURVE('',#18072,#18080,#14250,.T.);
#22335=EDGE_CURVE('',#18075,#18081,#9844,.T.);
#22336=EDGE_CURVE('',#18080,#18076,#1395,.T.);
#22337=EDGE_CURVE('',#18082,#18083,#14251,.T.);
#22338=EDGE_CURVE('',#18083,#18078,#14252,.T.);
#22339=EDGE_CURVE('',#18079,#18082,#14253,.T.);
#22340=EDGE_CURVE('',#18084,#18085,#14254,.T.);
#22341=EDGE_CURVE('',#18085,#18020,#14255,.T.);
#22342=EDGE_CURVE('',#18020,#18086,#9845,.T.);
#22343=EDGE_CURVE('',#18087,#18086,#14256,.T.);
#22344=EDGE_CURVE('',#18087,#18088,#14257,.T.);
#22345=EDGE_CURVE('',#18088,#18084,#9846,.F.);
#22346=EDGE_CURVE('',#18086,#18083,#9847,.T.);
#22347=EDGE_CURVE('',#18082,#18087,#1396,.T.);
#22348=EDGE_CURVE('',#17600,#18085,#14258,.T.);
#22349=EDGE_CURVE('',#18084,#17601,#9848,.F.);
#22350=EDGE_CURVE('',#17597,#18029,#909,.T.);
#22351=EDGE_CURVE('',#18029,#18089,#9849,.T.);
#22352=EDGE_CURVE('',#17598,#18089,#910,.T.);
#22353=EDGE_CURVE('',#18089,#17599,#911,.T.);
#22354=EDGE_CURVE('',#18090,#18091,#14259,.T.);
#22355=EDGE_CURVE('',#18091,#17401,#14260,.T.);
#22356=EDGE_CURVE('',#18092,#17400,#1397,.T.);
#22357=EDGE_CURVE('',#18092,#18093,#912,.T.);
#22358=EDGE_CURVE('',#18093,#18090,#9850,.T.);
#22359=EDGE_CURVE('',#18094,#18095,#14261,.T.);
#22360=EDGE_CURVE('',#18094,#18091,#1398,.T.);
#22361=EDGE_CURVE('',#18090,#18095,#9851,.T.);
#22362=EDGE_CURVE('',#18096,#18097,#14262,.T.);
#22363=EDGE_CURVE('',#18097,#18094,#14263,.T.);
#22364=EDGE_CURVE('',#18095,#18096,#14264,.T.);
#22365=EDGE_CURVE('',#18098,#18099,#14265,.T.);
#22366=EDGE_CURVE('',#18099,#18034,#14266,.T.);
#22367=EDGE_CURVE('',#18034,#18100,#9852,.T.);
#22368=EDGE_CURVE('',#18101,#18100,#14267,.T.);
#22369=EDGE_CURVE('',#18101,#18102,#14268,.T.);
#22370=EDGE_CURVE('',#18102,#18098,#9853,.T.);
#22371=EDGE_CURVE('',#18100,#18097,#9854,.T.);
#22372=EDGE_CURVE('',#18096,#18101,#1399,.T.);
#22373=EDGE_CURVE('',#17403,#18033,#913,.T.);
#22374=EDGE_CURVE('',#18103,#18104,#14269,.T.);
#22375=EDGE_CURVE('',#18103,#18099,#1400,.T.);
#22376=EDGE_CURVE('',#18098,#18104,#9855,.T.);
#22377=EDGE_CURVE('',#18105,#18106,#14270,.T.);
#22378=EDGE_CURVE('',#18106,#18103,#14271,.T.);
#22379=EDGE_CURVE('',#18104,#18105,#14272,.T.);
#22380=EDGE_CURVE('',#18107,#18108,#14273,.T.);
#22381=EDGE_CURVE('',#18108,#18043,#14274,.T.);
#22382=EDGE_CURVE('',#18043,#18109,#9856,.T.);
#22383=EDGE_CURVE('',#18110,#18109,#14275,.T.);
#22384=EDGE_CURVE('',#18110,#18111,#14276,.T.);
#22385=EDGE_CURVE('',#18111,#18107,#9857,.T.);
#22386=EDGE_CURVE('',#18109,#18106,#9858,.T.);
#22387=EDGE_CURVE('',#18105,#18110,#1401,.T.);
#22388=EDGE_CURVE('',#18112,#18113,#14277,.T.);
#22389=EDGE_CURVE('',#18112,#18108,#1402,.T.);
#22390=EDGE_CURVE('',#18107,#18113,#9859,.T.);
#22391=EDGE_CURVE('',#18114,#18115,#14278,.T.);
#22392=EDGE_CURVE('',#18115,#18112,#14279,.T.);
#22393=EDGE_CURVE('',#18113,#18114,#14280,.T.);
#22394=EDGE_CURVE('',#18116,#18117,#1403,.T.);
#22395=EDGE_CURVE('',#18117,#18052,#1404,.T.);
#22396=EDGE_CURVE('',#18052,#18118,#9860,.T.);
#22397=EDGE_CURVE('',#18119,#18118,#14281,.T.);
#22398=EDGE_CURVE('',#18119,#18120,#14282,.T.);
#22399=EDGE_CURVE('',#18120,#18116,#9861,.T.);
#22400=EDGE_CURVE('',#18118,#18115,#9862,.T.);
#22401=EDGE_CURVE('',#18114,#18119,#1405,.T.);
#22402=EDGE_CURVE('',#18121,#18122,#1406,.T.);
#22403=EDGE_CURVE('',#18121,#18117,#1407,.T.);
#22404=EDGE_CURVE('',#18116,#18122,#9863,.T.);
#22405=EDGE_CURVE('',#18123,#18124,#14283,.T.);
#22406=EDGE_CURVE('',#18124,#18121,#1408,.T.);
#22407=EDGE_CURVE('',#18122,#18123,#14284,.T.);
#22408=EDGE_CURVE('',#18125,#18126,#14285,.T.);
#22409=EDGE_CURVE('',#18126,#18061,#14286,.T.);
#22410=EDGE_CURVE('',#18061,#18127,#9864,.T.);
#22411=EDGE_CURVE('',#18128,#18127,#14287,.T.);
#22412=EDGE_CURVE('',#18128,#18129,#14288,.T.);
#22413=EDGE_CURVE('',#18129,#18125,#9865,.T.);
#22414=EDGE_CURVE('',#18127,#18124,#9866,.T.);
#22415=EDGE_CURVE('',#18123,#18128,#1409,.T.);
#22416=EDGE_CURVE('',#18130,#18131,#14289,.T.);
#22417=EDGE_CURVE('',#18130,#18126,#1410,.T.);
#22418=EDGE_CURVE('',#18125,#18131,#9867,.T.);
#22419=EDGE_CURVE('',#18132,#18133,#14290,.T.);
#22420=EDGE_CURVE('',#18133,#18130,#14291,.T.);
#22421=EDGE_CURVE('',#18131,#18132,#14292,.T.);
#22422=EDGE_CURVE('',#18134,#18135,#14293,.T.);
#22423=EDGE_CURVE('',#18135,#18070,#14294,.T.);
#22424=EDGE_CURVE('',#18070,#18136,#9868,.T.);
#22425=EDGE_CURVE('',#18137,#18136,#14295,.T.);
#22426=EDGE_CURVE('',#18137,#18138,#14296,.T.);
#22427=EDGE_CURVE('',#18138,#18134,#9869,.T.);
#22428=EDGE_CURVE('',#18136,#18133,#9870,.T.);
#22429=EDGE_CURVE('',#18132,#18137,#1411,.T.);
#22430=EDGE_CURVE('',#18139,#18140,#14297,.T.);
#22431=EDGE_CURVE('',#18139,#18135,#1412,.T.);
#22432=EDGE_CURVE('',#18134,#18140,#9871,.T.);
#22433=EDGE_CURVE('',#18141,#18142,#14298,.T.);
#22434=EDGE_CURVE('',#18142,#18077,#14299,.T.);
#22435=EDGE_CURVE('',#18077,#18143,#9872,.T.);
#22436=EDGE_CURVE('',#18144,#18143,#14300,.T.);
#22437=EDGE_CURVE('',#18144,#18145,#14301,.T.);
#22438=EDGE_CURVE('',#18145,#18141,#9873,.F.);
#22439=EDGE_CURVE('',#17606,#18142,#14302,.T.);
#22440=EDGE_CURVE('',#18141,#17607,#9874,.F.);
#22441=EDGE_CURVE('',#18146,#18147,#14303,.T.);
#22442=EDGE_CURVE('',#18147,#18139,#14304,.T.);
#22443=EDGE_CURVE('',#18140,#18146,#14305,.T.);
#22444=EDGE_CURVE('',#18143,#18147,#9875,.T.);
#22445=EDGE_CURVE('',#18146,#18144,#1413,.T.);
#22446=EDGE_CURVE('',#17603,#18088,#914,.T.);
#22447=EDGE_CURVE('',#18088,#18148,#9876,.T.);
#22448=EDGE_CURVE('',#17604,#18148,#915,.T.);
#22449=EDGE_CURVE('',#18148,#17605,#916,.T.);
#22450=EDGE_CURVE('',#18149,#18150,#14306,.T.);
#22451=EDGE_CURVE('',#18150,#17397,#14307,.T.);
#22452=EDGE_CURVE('',#18151,#17396,#1414,.T.);
#22453=EDGE_CURVE('',#18151,#18152,#917,.T.);
#22454=EDGE_CURVE('',#18152,#18149,#9877,.T.);
#22455=EDGE_CURVE('',#18153,#18154,#14308,.T.);
#22456=EDGE_CURVE('',#18153,#18150,#1415,.T.);
#22457=EDGE_CURVE('',#18149,#18154,#9878,.T.);
#22458=EDGE_CURVE('',#18155,#18156,#14309,.T.);
#22459=EDGE_CURVE('',#18156,#18153,#14310,.T.);
#22460=EDGE_CURVE('',#18154,#18155,#14311,.T.);
#22461=EDGE_CURVE('',#18157,#18158,#14312,.T.);
#22462=EDGE_CURVE('',#18158,#18093,#14313,.T.);
#22463=EDGE_CURVE('',#18093,#18159,#9879,.T.);
#22464=EDGE_CURVE('',#18160,#18159,#14314,.T.);
#22465=EDGE_CURVE('',#18160,#18161,#14315,.T.);
#22466=EDGE_CURVE('',#18161,#18157,#9880,.T.);
#22467=EDGE_CURVE('',#18159,#18156,#9881,.T.);
#22468=EDGE_CURVE('',#18155,#18160,#1416,.T.);
#22469=EDGE_CURVE('',#17399,#18092,#918,.T.);
#22470=EDGE_CURVE('',#18162,#18163,#14316,.T.);
#22471=EDGE_CURVE('',#18162,#18158,#1417,.T.);
#22472=EDGE_CURVE('',#18157,#18163,#9882,.T.);
#22473=EDGE_CURVE('',#18164,#18165,#14317,.T.);
#22474=EDGE_CURVE('',#18165,#18162,#14318,.T.);
#22475=EDGE_CURVE('',#18163,#18164,#14319,.T.);
#22476=EDGE_CURVE('',#18166,#18167,#14320,.T.);
#22477=EDGE_CURVE('',#18167,#18102,#14321,.T.);
#22478=EDGE_CURVE('',#18102,#18168,#9883,.T.);
#22479=EDGE_CURVE('',#18169,#18168,#14322,.T.);
#22480=EDGE_CURVE('',#18169,#18170,#14323,.T.);
#22481=EDGE_CURVE('',#18170,#18166,#9884,.T.);
#22482=EDGE_CURVE('',#18168,#18165,#9885,.T.);
#22483=EDGE_CURVE('',#18164,#18169,#1418,.T.);
#22484=EDGE_CURVE('',#18171,#18172,#14324,.T.);
#22485=EDGE_CURVE('',#18171,#18167,#1419,.T.);
#22486=EDGE_CURVE('',#18166,#18172,#9886,.T.);
#22487=EDGE_CURVE('',#18173,#18174,#14325,.T.);
#22488=EDGE_CURVE('',#18174,#18171,#14326,.T.);
#22489=EDGE_CURVE('',#18172,#18173,#14327,.T.);
#22490=EDGE_CURVE('',#18175,#18176,#1420,.T.);
#22491=EDGE_CURVE('',#18176,#18111,#1421,.T.);
#22492=EDGE_CURVE('',#18111,#18177,#9887,.T.);
#22493=EDGE_CURVE('',#18178,#18177,#14328,.T.);
#22494=EDGE_CURVE('',#18178,#18179,#14329,.T.);
#22495=EDGE_CURVE('',#18179,#18175,#9888,.T.);
#22496=EDGE_CURVE('',#18177,#18174,#9889,.T.);
#22497=EDGE_CURVE('',#18173,#18178,#1422,.T.);
#22498=EDGE_CURVE('',#18180,#18181,#1423,.T.);
#22499=EDGE_CURVE('',#18180,#18176,#1424,.T.);
#22500=EDGE_CURVE('',#18175,#18181,#9890,.T.);
#22501=EDGE_CURVE('',#18182,#18183,#14330,.T.);
#22502=EDGE_CURVE('',#18183,#18180,#1425,.T.);
#22503=EDGE_CURVE('',#18181,#18182,#14331,.T.);
#22504=EDGE_CURVE('',#18184,#18185,#14332,.T.);
#22505=EDGE_CURVE('',#18185,#18120,#14333,.T.);
#22506=EDGE_CURVE('',#18120,#18186,#9891,.T.);
#22507=EDGE_CURVE('',#18187,#18186,#14334,.T.);
#22508=EDGE_CURVE('',#18187,#18188,#14335,.T.);
#22509=EDGE_CURVE('',#18188,#18184,#9892,.T.);
#22510=EDGE_CURVE('',#18186,#18183,#9893,.T.);
#22511=EDGE_CURVE('',#18182,#18187,#1426,.T.);
#22512=EDGE_CURVE('',#18189,#18190,#14336,.T.);
#22513=EDGE_CURVE('',#18189,#18185,#1427,.T.);
#22514=EDGE_CURVE('',#18184,#18190,#9894,.T.);
#22515=EDGE_CURVE('',#18191,#18192,#14337,.T.);
#22516=EDGE_CURVE('',#18192,#18189,#14338,.T.);
#22517=EDGE_CURVE('',#18190,#18191,#14339,.T.);
#22518=EDGE_CURVE('',#18193,#18194,#14340,.T.);
#22519=EDGE_CURVE('',#18194,#18129,#14341,.T.);
#22520=EDGE_CURVE('',#18129,#18195,#9895,.T.);
#22521=EDGE_CURVE('',#18196,#18195,#14342,.T.);
#22522=EDGE_CURVE('',#18196,#18197,#14343,.T.);
#22523=EDGE_CURVE('',#18197,#18193,#9896,.T.);
#22524=EDGE_CURVE('',#18195,#18192,#9897,.T.);
#22525=EDGE_CURVE('',#18191,#18196,#1428,.T.);
#22526=EDGE_CURVE('',#18198,#18199,#14344,.T.);
#22527=EDGE_CURVE('',#18198,#18194,#1429,.T.);
#22528=EDGE_CURVE('',#18193,#18199,#9898,.T.);
#22529=EDGE_CURVE('',#18200,#18201,#14345,.T.);
#22530=EDGE_CURVE('',#18201,#18198,#14346,.T.);
#22531=EDGE_CURVE('',#18199,#18200,#14347,.T.);
#22532=EDGE_CURVE('',#18202,#18203,#14348,.T.);
#22533=EDGE_CURVE('',#18203,#18138,#14349,.T.);
#22534=EDGE_CURVE('',#18138,#18204,#9899,.T.);
#22535=EDGE_CURVE('',#18205,#18204,#14350,.T.);
#22536=EDGE_CURVE('',#18205,#18206,#14351,.T.);
#22537=EDGE_CURVE('',#18206,#18202,#9900,.F.);
#22538=EDGE_CURVE('',#18204,#18201,#9901,.T.);
#22539=EDGE_CURVE('',#18200,#18205,#1430,.T.);
#22540=EDGE_CURVE('',#17612,#18203,#14352,.T.);
#22541=EDGE_CURVE('',#18202,#17613,#9902,.F.);
#22542=EDGE_CURVE('',#17609,#18145,#919,.T.);
#22543=EDGE_CURVE('',#18145,#18207,#9903,.T.);
#22544=EDGE_CURVE('',#17610,#18207,#920,.T.);
#22545=EDGE_CURVE('',#18207,#17611,#921,.T.);
#22546=EDGE_CURVE('',#18208,#18209,#14353,.T.);
#22547=EDGE_CURVE('',#18209,#17393,#14354,.T.);
#22548=EDGE_CURVE('',#18210,#17392,#1431,.T.);
#22549=EDGE_CURVE('',#18210,#18211,#922,.T.);
#22550=EDGE_CURVE('',#18211,#18208,#9904,.T.);
#22551=EDGE_CURVE('',#18212,#18213,#14355,.T.);
#22552=EDGE_CURVE('',#18212,#18209,#1432,.T.);
#22553=EDGE_CURVE('',#18208,#18213,#9905,.T.);
#22554=EDGE_CURVE('',#18214,#18215,#14356,.T.);
#22555=EDGE_CURVE('',#18215,#18212,#14357,.T.);
#22556=EDGE_CURVE('',#18213,#18214,#14358,.T.);
#22557=EDGE_CURVE('',#18216,#18217,#14359,.T.);
#22558=EDGE_CURVE('',#18217,#18152,#14360,.T.);
#22559=EDGE_CURVE('',#18152,#18218,#9906,.T.);
#22560=EDGE_CURVE('',#18219,#18218,#14361,.T.);
#22561=EDGE_CURVE('',#18219,#18220,#14362,.T.);
#22562=EDGE_CURVE('',#18220,#18216,#9907,.T.);
#22563=EDGE_CURVE('',#18218,#18215,#9908,.T.);
#22564=EDGE_CURVE('',#18214,#18219,#1433,.T.);
#22565=EDGE_CURVE('',#17395,#18151,#923,.T.);
#22566=EDGE_CURVE('',#18221,#18222,#14363,.T.);
#22567=EDGE_CURVE('',#18221,#18217,#1434,.T.);
#22568=EDGE_CURVE('',#18216,#18222,#9909,.T.);
#22569=EDGE_CURVE('',#18223,#18224,#14364,.T.);
#22570=EDGE_CURVE('',#18224,#18221,#14365,.T.);
#22571=EDGE_CURVE('',#18222,#18223,#14366,.T.);
#22572=EDGE_CURVE('',#18225,#18226,#14367,.T.);
#22573=EDGE_CURVE('',#18226,#18161,#14368,.T.);
#22574=EDGE_CURVE('',#18161,#18227,#9910,.T.);
#22575=EDGE_CURVE('',#18228,#18227,#14369,.T.);
#22576=EDGE_CURVE('',#18228,#18229,#14370,.T.);
#22577=EDGE_CURVE('',#18229,#18225,#9911,.T.);
#22578=EDGE_CURVE('',#18227,#18224,#9912,.T.);
#22579=EDGE_CURVE('',#18223,#18228,#1435,.T.);
#22580=EDGE_CURVE('',#18230,#18231,#14371,.T.);
#22581=EDGE_CURVE('',#18230,#18226,#1436,.T.);
#22582=EDGE_CURVE('',#18225,#18231,#9913,.T.);
#22583=EDGE_CURVE('',#18232,#18233,#14372,.T.);
#22584=EDGE_CURVE('',#18233,#18230,#14373,.T.);
#22585=EDGE_CURVE('',#18231,#18232,#14374,.T.);
#22586=EDGE_CURVE('',#18234,#18235,#1437,.T.);
#22587=EDGE_CURVE('',#18235,#18170,#1438,.T.);
#22588=EDGE_CURVE('',#18170,#18236,#9914,.T.);
#22589=EDGE_CURVE('',#18237,#18236,#14375,.T.);
#22590=EDGE_CURVE('',#18237,#18238,#14376,.T.);
#22591=EDGE_CURVE('',#18238,#18234,#9915,.T.);
#22592=EDGE_CURVE('',#18236,#18233,#9916,.T.);
#22593=EDGE_CURVE('',#18232,#18237,#1439,.T.);
#22594=EDGE_CURVE('',#18239,#18240,#1440,.T.);
#22595=EDGE_CURVE('',#18239,#18235,#1441,.T.);
#22596=EDGE_CURVE('',#18234,#18240,#9917,.T.);
#22597=EDGE_CURVE('',#18241,#18242,#14377,.T.);
#22598=EDGE_CURVE('',#18242,#18239,#1442,.T.);
#22599=EDGE_CURVE('',#18240,#18241,#14378,.T.);
#22600=EDGE_CURVE('',#18243,#18244,#14379,.T.);
#22601=EDGE_CURVE('',#18244,#18179,#14380,.T.);
#22602=EDGE_CURVE('',#18179,#18245,#9918,.T.);
#22603=EDGE_CURVE('',#18246,#18245,#14381,.T.);
#22604=EDGE_CURVE('',#18246,#18247,#14382,.T.);
#22605=EDGE_CURVE('',#18247,#18243,#9919,.T.);
#22606=EDGE_CURVE('',#18245,#18242,#9920,.T.);
#22607=EDGE_CURVE('',#18241,#18246,#1443,.T.);
#22608=EDGE_CURVE('',#18248,#18249,#14383,.T.);
#22609=EDGE_CURVE('',#18248,#18244,#1444,.T.);
#22610=EDGE_CURVE('',#18243,#18249,#9921,.T.);
#22611=EDGE_CURVE('',#18250,#18251,#14384,.T.);
#22612=EDGE_CURVE('',#18251,#18248,#14385,.T.);
#22613=EDGE_CURVE('',#18249,#18250,#14386,.T.);
#22614=EDGE_CURVE('',#18252,#18253,#14387,.T.);
#22615=EDGE_CURVE('',#18253,#18188,#14388,.T.);
#22616=EDGE_CURVE('',#18188,#18254,#9922,.T.);
#22617=EDGE_CURVE('',#18255,#18254,#14389,.T.);
#22618=EDGE_CURVE('',#18255,#18256,#14390,.T.);
#22619=EDGE_CURVE('',#18256,#18252,#9923,.T.);
#22620=EDGE_CURVE('',#18254,#18251,#9924,.T.);
#22621=EDGE_CURVE('',#18250,#18255,#1445,.T.);
#22622=EDGE_CURVE('',#18257,#18258,#14391,.T.);
#22623=EDGE_CURVE('',#18257,#18253,#1446,.T.);
#22624=EDGE_CURVE('',#18252,#18258,#9925,.T.);
#22625=EDGE_CURVE('',#18259,#18260,#14392,.T.);
#22626=EDGE_CURVE('',#18260,#18257,#14393,.T.);
#22627=EDGE_CURVE('',#18258,#18259,#14394,.T.);
#22628=EDGE_CURVE('',#18261,#18262,#14395,.T.);
#22629=EDGE_CURVE('',#18262,#18197,#14396,.T.);
#22630=EDGE_CURVE('',#18197,#18263,#9926,.T.);
#22631=EDGE_CURVE('',#18264,#18263,#14397,.T.);
#22632=EDGE_CURVE('',#18264,#18265,#14398,.T.);
#22633=EDGE_CURVE('',#18265,#18261,#9927,.F.);
#22634=EDGE_CURVE('',#18263,#18260,#9928,.T.);
#22635=EDGE_CURVE('',#18259,#18264,#1447,.T.);
#22636=EDGE_CURVE('',#17618,#18262,#14399,.T.);
#22637=EDGE_CURVE('',#18261,#17619,#9929,.F.);
#22638=EDGE_CURVE('',#17615,#18206,#924,.T.);
#22639=EDGE_CURVE('',#18206,#18266,#9930,.T.);
#22640=EDGE_CURVE('',#17616,#18266,#925,.T.);
#22641=EDGE_CURVE('',#18266,#17617,#926,.T.);
#22642=EDGE_CURVE('',#18267,#18268,#14400,.T.);
#22643=EDGE_CURVE('',#18268,#17389,#14401,.T.);
#22644=EDGE_CURVE('',#18269,#17388,#1448,.T.);
#22645=EDGE_CURVE('',#18269,#18270,#927,.T.);
#22646=EDGE_CURVE('',#18270,#18267,#9931,.T.);
#22647=EDGE_CURVE('',#18271,#18272,#14402,.T.);
#22648=EDGE_CURVE('',#18271,#18268,#1449,.T.);
#22649=EDGE_CURVE('',#18267,#18272,#9932,.T.);
#22650=EDGE_CURVE('',#18273,#18274,#14403,.T.);
#22651=EDGE_CURVE('',#18274,#18271,#14404,.T.);
#22652=EDGE_CURVE('',#18272,#18273,#14405,.T.);
#22653=EDGE_CURVE('',#18275,#18276,#14406,.T.);
#22654=EDGE_CURVE('',#18276,#18211,#14407,.T.);
#22655=EDGE_CURVE('',#18211,#18277,#9933,.T.);
#22656=EDGE_CURVE('',#18278,#18277,#14408,.T.);
#22657=EDGE_CURVE('',#18278,#18279,#14409,.T.);
#22658=EDGE_CURVE('',#18279,#18275,#9934,.T.);
#22659=EDGE_CURVE('',#18277,#18274,#9935,.T.);
#22660=EDGE_CURVE('',#18273,#18278,#1450,.T.);
#22661=EDGE_CURVE('',#17391,#18210,#928,.T.);
#22662=EDGE_CURVE('',#18280,#18281,#14410,.T.);
#22663=EDGE_CURVE('',#18280,#18276,#1451,.T.);
#22664=EDGE_CURVE('',#18275,#18281,#9936,.T.);
#22665=EDGE_CURVE('',#18282,#18283,#14411,.T.);
#22666=EDGE_CURVE('',#18283,#18280,#14412,.T.);
#22667=EDGE_CURVE('',#18281,#18282,#14413,.T.);
#22668=EDGE_CURVE('',#18284,#18285,#14414,.T.);
#22669=EDGE_CURVE('',#18285,#18220,#14415,.T.);
#22670=EDGE_CURVE('',#18220,#18286,#9937,.T.);
#22671=EDGE_CURVE('',#18287,#18286,#14416,.T.);
#22672=EDGE_CURVE('',#18287,#18288,#14417,.T.);
#22673=EDGE_CURVE('',#18288,#18284,#9938,.T.);
#22674=EDGE_CURVE('',#18286,#18283,#9939,.T.);
#22675=EDGE_CURVE('',#18282,#18287,#1452,.T.);
#22676=EDGE_CURVE('',#18289,#18290,#14418,.T.);
#22677=EDGE_CURVE('',#18289,#18285,#1453,.T.);
#22678=EDGE_CURVE('',#18284,#18290,#9940,.T.);
#22679=EDGE_CURVE('',#18291,#18292,#14419,.T.);
#22680=EDGE_CURVE('',#18292,#18289,#14420,.T.);
#22681=EDGE_CURVE('',#18290,#18291,#14421,.T.);
#22682=EDGE_CURVE('',#18293,#18294,#1454,.T.);
#22683=EDGE_CURVE('',#18294,#18229,#1455,.T.);
#22684=EDGE_CURVE('',#18229,#18295,#9941,.T.);
#22685=EDGE_CURVE('',#18296,#18295,#14422,.T.);
#22686=EDGE_CURVE('',#18296,#18297,#14423,.T.);
#22687=EDGE_CURVE('',#18297,#18293,#9942,.T.);
#22688=EDGE_CURVE('',#18295,#18292,#9943,.T.);
#22689=EDGE_CURVE('',#18291,#18296,#1456,.T.);
#22690=EDGE_CURVE('',#18298,#18299,#1457,.T.);
#22691=EDGE_CURVE('',#18298,#18294,#1458,.T.);
#22692=EDGE_CURVE('',#18293,#18299,#9944,.T.);
#22693=EDGE_CURVE('',#18300,#18301,#14424,.T.);
#22694=EDGE_CURVE('',#18301,#18298,#1459,.T.);
#22695=EDGE_CURVE('',#18299,#18300,#14425,.T.);
#22696=EDGE_CURVE('',#18302,#18303,#14426,.T.);
#22697=EDGE_CURVE('',#18303,#18238,#14427,.T.);
#22698=EDGE_CURVE('',#18238,#18304,#9945,.T.);
#22699=EDGE_CURVE('',#18305,#18304,#14428,.T.);
#22700=EDGE_CURVE('',#18305,#18306,#14429,.T.);
#22701=EDGE_CURVE('',#18306,#18302,#9946,.T.);
#22702=EDGE_CURVE('',#18304,#18301,#9947,.T.);
#22703=EDGE_CURVE('',#18300,#18305,#1460,.T.);
#22704=EDGE_CURVE('',#18307,#18308,#14430,.T.);
#22705=EDGE_CURVE('',#18307,#18303,#1461,.T.);
#22706=EDGE_CURVE('',#18302,#18308,#9948,.T.);
#22707=EDGE_CURVE('',#18309,#18310,#14431,.T.);
#22708=EDGE_CURVE('',#18310,#18307,#14432,.T.);
#22709=EDGE_CURVE('',#18308,#18309,#14433,.T.);
#22710=EDGE_CURVE('',#18311,#18312,#14434,.T.);
#22711=EDGE_CURVE('',#18312,#18247,#14435,.T.);
#22712=EDGE_CURVE('',#18247,#18313,#9949,.T.);
#22713=EDGE_CURVE('',#18314,#18313,#14436,.T.);
#22714=EDGE_CURVE('',#18314,#18315,#14437,.T.);
#22715=EDGE_CURVE('',#18315,#18311,#9950,.T.);
#22716=EDGE_CURVE('',#18313,#18310,#9951,.T.);
#22717=EDGE_CURVE('',#18309,#18314,#1462,.T.);
#22718=EDGE_CURVE('',#18316,#18317,#14438,.T.);
#22719=EDGE_CURVE('',#18316,#18312,#1463,.T.);
#22720=EDGE_CURVE('',#18311,#18317,#9952,.T.);
#22721=EDGE_CURVE('',#18318,#18319,#14439,.T.);
#22722=EDGE_CURVE('',#18319,#18316,#14440,.T.);
#22723=EDGE_CURVE('',#18317,#18318,#14441,.T.);
#22724=EDGE_CURVE('',#18320,#18321,#14442,.T.);
#22725=EDGE_CURVE('',#18321,#18256,#14443,.T.);
#22726=EDGE_CURVE('',#18256,#18322,#9953,.T.);
#22727=EDGE_CURVE('',#18323,#18322,#14444,.T.);
#22728=EDGE_CURVE('',#18323,#18324,#14445,.T.);
#22729=EDGE_CURVE('',#18324,#18320,#9954,.F.);
#22730=EDGE_CURVE('',#18322,#18319,#9955,.T.);
#22731=EDGE_CURVE('',#18318,#18323,#1464,.T.);
#22732=EDGE_CURVE('',#17624,#18321,#14446,.T.);
#22733=EDGE_CURVE('',#18320,#17625,#9956,.F.);
#22734=EDGE_CURVE('',#17621,#18265,#929,.T.);
#22735=EDGE_CURVE('',#18265,#18325,#9957,.T.);
#22736=EDGE_CURVE('',#17622,#18325,#930,.T.);
#22737=EDGE_CURVE('',#18325,#17623,#931,.T.);
#22738=EDGE_CURVE('',#18326,#18327,#14447,.T.);
#22739=EDGE_CURVE('',#18327,#17385,#14448,.T.);
#22740=EDGE_CURVE('',#18328,#17384,#1465,.T.);
#22741=EDGE_CURVE('',#18328,#18329,#932,.T.);
#22742=EDGE_CURVE('',#18329,#18326,#9958,.T.);
#22743=EDGE_CURVE('',#18330,#18331,#14449,.T.);
#22744=EDGE_CURVE('',#18330,#18327,#1466,.T.);
#22745=EDGE_CURVE('',#18326,#18331,#9959,.T.);
#22746=EDGE_CURVE('',#18332,#18333,#14450,.T.);
#22747=EDGE_CURVE('',#18333,#18330,#14451,.T.);
#22748=EDGE_CURVE('',#18331,#18332,#14452,.T.);
#22749=EDGE_CURVE('',#18334,#18335,#14453,.T.);
#22750=EDGE_CURVE('',#18335,#18270,#14454,.T.);
#22751=EDGE_CURVE('',#18270,#18336,#9960,.T.);
#22752=EDGE_CURVE('',#18337,#18336,#14455,.T.);
#22753=EDGE_CURVE('',#18337,#18338,#14456,.T.);
#22754=EDGE_CURVE('',#18338,#18334,#9961,.T.);
#22755=EDGE_CURVE('',#18336,#18333,#9962,.T.);
#22756=EDGE_CURVE('',#18332,#18337,#1467,.T.);
#22757=EDGE_CURVE('',#17387,#18269,#933,.T.);
#22758=EDGE_CURVE('',#18339,#18340,#14457,.T.);
#22759=EDGE_CURVE('',#18339,#18335,#1468,.T.);
#22760=EDGE_CURVE('',#18334,#18340,#9963,.T.);
#22761=EDGE_CURVE('',#18341,#18342,#14458,.T.);
#22762=EDGE_CURVE('',#18342,#18339,#14459,.T.);
#22763=EDGE_CURVE('',#18340,#18341,#14460,.T.);
#22764=EDGE_CURVE('',#18343,#18344,#14461,.T.);
#22765=EDGE_CURVE('',#18344,#18279,#14462,.T.);
#22766=EDGE_CURVE('',#18279,#18345,#9964,.T.);
#22767=EDGE_CURVE('',#18346,#18345,#14463,.T.);
#22768=EDGE_CURVE('',#18346,#18347,#14464,.T.);
#22769=EDGE_CURVE('',#18347,#18343,#9965,.T.);
#22770=EDGE_CURVE('',#18345,#18342,#9966,.T.);
#22771=EDGE_CURVE('',#18341,#18346,#1469,.T.);
#22772=EDGE_CURVE('',#18348,#18349,#14465,.T.);
#22773=EDGE_CURVE('',#18348,#18344,#1470,.T.);
#22774=EDGE_CURVE('',#18343,#18349,#9967,.T.);
#22775=EDGE_CURVE('',#18350,#18351,#14466,.T.);
#22776=EDGE_CURVE('',#18351,#18348,#14467,.T.);
#22777=EDGE_CURVE('',#18349,#18350,#14468,.T.);
#22778=EDGE_CURVE('',#18352,#18353,#1471,.T.);
#22779=EDGE_CURVE('',#18353,#18288,#1472,.T.);
#22780=EDGE_CURVE('',#18288,#18354,#9968,.T.);
#22781=EDGE_CURVE('',#18355,#18354,#14469,.T.);
#22782=EDGE_CURVE('',#18355,#18356,#14470,.T.);
#22783=EDGE_CURVE('',#18356,#18352,#9969,.T.);
#22784=EDGE_CURVE('',#18354,#18351,#9970,.T.);
#22785=EDGE_CURVE('',#18350,#18355,#1473,.T.);
#22786=EDGE_CURVE('',#18357,#18358,#1474,.T.);
#22787=EDGE_CURVE('',#18357,#18353,#1475,.T.);
#22788=EDGE_CURVE('',#18352,#18358,#9971,.T.);
#22789=EDGE_CURVE('',#18359,#18360,#14471,.T.);
#22790=EDGE_CURVE('',#18360,#18357,#1476,.T.);
#22791=EDGE_CURVE('',#18358,#18359,#14472,.T.);
#22792=EDGE_CURVE('',#18361,#18362,#14473,.T.);
#22793=EDGE_CURVE('',#18362,#18297,#14474,.T.);
#22794=EDGE_CURVE('',#18297,#18363,#9972,.T.);
#22795=EDGE_CURVE('',#18364,#18363,#14475,.T.);
#22796=EDGE_CURVE('',#18364,#18365,#14476,.T.);
#22797=EDGE_CURVE('',#18365,#18361,#9973,.T.);
#22798=EDGE_CURVE('',#18363,#18360,#9974,.T.);
#22799=EDGE_CURVE('',#18359,#18364,#1477,.T.);
#22800=EDGE_CURVE('',#18366,#18367,#14477,.T.);
#22801=EDGE_CURVE('',#18366,#18362,#1478,.T.);
#22802=EDGE_CURVE('',#18361,#18367,#9975,.T.);
#22803=EDGE_CURVE('',#18368,#18369,#14478,.T.);
#22804=EDGE_CURVE('',#18369,#18366,#14479,.T.);
#22805=EDGE_CURVE('',#18367,#18368,#14480,.T.);
#22806=EDGE_CURVE('',#18370,#18371,#14481,.T.);
#22807=EDGE_CURVE('',#18371,#18306,#14482,.T.);
#22808=EDGE_CURVE('',#18306,#18372,#9976,.T.);
#22809=EDGE_CURVE('',#18373,#18372,#14483,.T.);
#22810=EDGE_CURVE('',#18373,#18374,#14484,.T.);
#22811=EDGE_CURVE('',#18374,#18370,#9977,.T.);
#22812=EDGE_CURVE('',#18372,#18369,#9978,.T.);
#22813=EDGE_CURVE('',#18368,#18373,#1479,.T.);
#22814=EDGE_CURVE('',#18375,#18376,#14485,.T.);
#22815=EDGE_CURVE('',#18375,#18371,#1480,.T.);
#22816=EDGE_CURVE('',#18370,#18376,#9979,.T.);
#22817=EDGE_CURVE('',#18377,#18378,#14486,.T.);
#22818=EDGE_CURVE('',#18378,#18375,#14487,.T.);
#22819=EDGE_CURVE('',#18376,#18377,#14488,.T.);
#22820=EDGE_CURVE('',#18379,#18380,#14489,.T.);
#22821=EDGE_CURVE('',#18380,#18315,#14490,.T.);
#22822=EDGE_CURVE('',#18315,#18381,#9980,.T.);
#22823=EDGE_CURVE('',#18382,#18381,#14491,.T.);
#22824=EDGE_CURVE('',#18382,#18383,#14492,.T.);
#22825=EDGE_CURVE('',#18383,#18379,#9981,.F.);
#22826=EDGE_CURVE('',#18381,#18378,#9982,.T.);
#22827=EDGE_CURVE('',#18377,#18382,#1481,.T.);
#22828=EDGE_CURVE('',#17630,#18380,#14493,.T.);
#22829=EDGE_CURVE('',#18379,#17631,#9983,.F.);
#22830=EDGE_CURVE('',#17627,#18324,#934,.T.);
#22831=EDGE_CURVE('',#18324,#18384,#9984,.T.);
#22832=EDGE_CURVE('',#17628,#18384,#935,.T.);
#22833=EDGE_CURVE('',#18384,#17629,#936,.T.);
#22834=EDGE_CURVE('',#18385,#18386,#14494,.T.);
#22835=EDGE_CURVE('',#18386,#17381,#14495,.T.);
#22836=EDGE_CURVE('',#18387,#17380,#1482,.T.);
#22837=EDGE_CURVE('',#18387,#18388,#937,.T.);
#22838=EDGE_CURVE('',#18388,#18385,#9985,.T.);
#22839=EDGE_CURVE('',#18389,#18390,#14496,.T.);
#22840=EDGE_CURVE('',#18389,#18386,#1483,.T.);
#22841=EDGE_CURVE('',#18385,#18390,#9986,.T.);
#22842=EDGE_CURVE('',#18391,#18392,#14497,.T.);
#22843=EDGE_CURVE('',#18392,#18389,#14498,.T.);
#22844=EDGE_CURVE('',#18390,#18391,#14499,.T.);
#22845=EDGE_CURVE('',#18393,#18394,#14500,.T.);
#22846=EDGE_CURVE('',#18394,#18329,#14501,.T.);
#22847=EDGE_CURVE('',#18329,#18395,#9987,.T.);
#22848=EDGE_CURVE('',#18396,#18395,#14502,.T.);
#22849=EDGE_CURVE('',#18396,#18397,#14503,.T.);
#22850=EDGE_CURVE('',#18397,#18393,#9988,.T.);
#22851=EDGE_CURVE('',#18395,#18392,#9989,.T.);
#22852=EDGE_CURVE('',#18391,#18396,#1484,.T.);
#22853=EDGE_CURVE('',#17383,#18328,#938,.T.);
#22854=EDGE_CURVE('',#18398,#18399,#14504,.T.);
#22855=EDGE_CURVE('',#18398,#18394,#1485,.T.);
#22856=EDGE_CURVE('',#18393,#18399,#9990,.T.);
#22857=EDGE_CURVE('',#18400,#18401,#14505,.T.);
#22858=EDGE_CURVE('',#18401,#18398,#14506,.T.);
#22859=EDGE_CURVE('',#18399,#18400,#14507,.T.);
#22860=EDGE_CURVE('',#18402,#18403,#14508,.T.);
#22861=EDGE_CURVE('',#18403,#18338,#14509,.T.);
#22862=EDGE_CURVE('',#18338,#18404,#9991,.T.);
#22863=EDGE_CURVE('',#18405,#18404,#14510,.T.);
#22864=EDGE_CURVE('',#18405,#18406,#14511,.T.);
#22865=EDGE_CURVE('',#18406,#18402,#9992,.T.);
#22866=EDGE_CURVE('',#18404,#18401,#9993,.T.);
#22867=EDGE_CURVE('',#18400,#18405,#1486,.T.);
#22868=EDGE_CURVE('',#18407,#18408,#14512,.T.);
#22869=EDGE_CURVE('',#18407,#18403,#1487,.T.);
#22870=EDGE_CURVE('',#18402,#18408,#9994,.T.);
#22871=EDGE_CURVE('',#18409,#18410,#14513,.T.);
#22872=EDGE_CURVE('',#18410,#18407,#14514,.T.);
#22873=EDGE_CURVE('',#18408,#18409,#14515,.T.);
#22874=EDGE_CURVE('',#18411,#18412,#1488,.T.);
#22875=EDGE_CURVE('',#18412,#18347,#1489,.T.);
#22876=EDGE_CURVE('',#18347,#18413,#9995,.T.);
#22877=EDGE_CURVE('',#18414,#18413,#14516,.T.);
#22878=EDGE_CURVE('',#18414,#18415,#14517,.T.);
#22879=EDGE_CURVE('',#18415,#18411,#9996,.T.);
#22880=EDGE_CURVE('',#18413,#18410,#9997,.T.);
#22881=EDGE_CURVE('',#18409,#18414,#1490,.T.);
#22882=EDGE_CURVE('',#18416,#18417,#1491,.T.);
#22883=EDGE_CURVE('',#18416,#18412,#1492,.T.);
#22884=EDGE_CURVE('',#18411,#18417,#9998,.T.);
#22885=EDGE_CURVE('',#18418,#18419,#14518,.T.);
#22886=EDGE_CURVE('',#18419,#18416,#1493,.T.);
#22887=EDGE_CURVE('',#18417,#18418,#14519,.T.);
#22888=EDGE_CURVE('',#18420,#18421,#14520,.T.);
#22889=EDGE_CURVE('',#18421,#18356,#14521,.T.);
#22890=EDGE_CURVE('',#18356,#18422,#9999,.T.);
#22891=EDGE_CURVE('',#18423,#18422,#14522,.T.);
#22892=EDGE_CURVE('',#18423,#18424,#14523,.T.);
#22893=EDGE_CURVE('',#18424,#18420,#10000,.T.);
#22894=EDGE_CURVE('',#18422,#18419,#10001,.T.);
#22895=EDGE_CURVE('',#18418,#18423,#1494,.T.);
#22896=EDGE_CURVE('',#18425,#18426,#14524,.T.);
#22897=EDGE_CURVE('',#18425,#18421,#1495,.T.);
#22898=EDGE_CURVE('',#18420,#18426,#10002,.T.);
#22899=EDGE_CURVE('',#18427,#18428,#14525,.T.);
#22900=EDGE_CURVE('',#18428,#18425,#14526,.T.);
#22901=EDGE_CURVE('',#18426,#18427,#14527,.T.);
#22902=EDGE_CURVE('',#18429,#18430,#14528,.T.);
#22903=EDGE_CURVE('',#18430,#18365,#14529,.T.);
#22904=EDGE_CURVE('',#18365,#18431,#10003,.T.);
#22905=EDGE_CURVE('',#18432,#18431,#14530,.T.);
#22906=EDGE_CURVE('',#18432,#18433,#14531,.T.);
#22907=EDGE_CURVE('',#18433,#18429,#10004,.T.);
#22908=EDGE_CURVE('',#18431,#18428,#10005,.T.);
#22909=EDGE_CURVE('',#18427,#18432,#1496,.T.);
#22910=EDGE_CURVE('',#18434,#18435,#14532,.T.);
#22911=EDGE_CURVE('',#18434,#18430,#1497,.T.);
#22912=EDGE_CURVE('',#18429,#18435,#10006,.T.);
#22913=EDGE_CURVE('',#18436,#18437,#14533,.T.);
#22914=EDGE_CURVE('',#18437,#18434,#14534,.T.);
#22915=EDGE_CURVE('',#18435,#18436,#14535,.T.);
#22916=EDGE_CURVE('',#18438,#18439,#14536,.T.);
#22917=EDGE_CURVE('',#18439,#18374,#14537,.T.);
#22918=EDGE_CURVE('',#18374,#18440,#10007,.T.);
#22919=EDGE_CURVE('',#18441,#18440,#14538,.T.);
#22920=EDGE_CURVE('',#18441,#18442,#14539,.T.);
#22921=EDGE_CURVE('',#18442,#18438,#10008,.F.);
#22922=EDGE_CURVE('',#18440,#18437,#10009,.T.);
#22923=EDGE_CURVE('',#18436,#18441,#1498,.T.);
#22924=EDGE_CURVE('',#17636,#18439,#14540,.T.);
#22925=EDGE_CURVE('',#18438,#17637,#10010,.F.);
#22926=EDGE_CURVE('',#17633,#18383,#939,.T.);
#22927=EDGE_CURVE('',#18383,#18443,#10011,.T.);
#22928=EDGE_CURVE('',#17634,#18443,#940,.T.);
#22929=EDGE_CURVE('',#18443,#17635,#941,.T.);
#22930=EDGE_CURVE('',#18444,#18445,#14541,.T.);
#22931=EDGE_CURVE('',#18445,#17377,#14542,.T.);
#22932=EDGE_CURVE('',#18446,#17376,#1499,.T.);
#22933=EDGE_CURVE('',#18446,#18447,#942,.T.);
#22934=EDGE_CURVE('',#18447,#18444,#10012,.T.);
#22935=EDGE_CURVE('',#18448,#18449,#14543,.T.);
#22936=EDGE_CURVE('',#18448,#18445,#1500,.T.);
#22937=EDGE_CURVE('',#18444,#18449,#10013,.T.);
#22938=EDGE_CURVE('',#18450,#18451,#14544,.T.);
#22939=EDGE_CURVE('',#18451,#18448,#14545,.T.);
#22940=EDGE_CURVE('',#18449,#18450,#14546,.T.);
#22941=EDGE_CURVE('',#18452,#18453,#14547,.T.);
#22942=EDGE_CURVE('',#18453,#18388,#14548,.T.);
#22943=EDGE_CURVE('',#18388,#18454,#10014,.T.);
#22944=EDGE_CURVE('',#18455,#18454,#14549,.T.);
#22945=EDGE_CURVE('',#18455,#18456,#14550,.T.);
#22946=EDGE_CURVE('',#18456,#18452,#10015,.T.);
#22947=EDGE_CURVE('',#18454,#18451,#10016,.T.);
#22948=EDGE_CURVE('',#18450,#18455,#1501,.T.);
#22949=EDGE_CURVE('',#17379,#18387,#943,.T.);
#22950=EDGE_CURVE('',#18457,#18458,#14551,.T.);
#22951=EDGE_CURVE('',#18457,#18453,#1502,.T.);
#22952=EDGE_CURVE('',#18452,#18458,#10017,.T.);
#22953=EDGE_CURVE('',#18459,#18460,#14552,.T.);
#22954=EDGE_CURVE('',#18460,#18457,#14553,.T.);
#22955=EDGE_CURVE('',#18458,#18459,#14554,.T.);
#22956=EDGE_CURVE('',#18461,#18462,#14555,.T.);
#22957=EDGE_CURVE('',#18462,#18397,#14556,.T.);
#22958=EDGE_CURVE('',#18397,#18463,#10018,.T.);
#22959=EDGE_CURVE('',#18464,#18463,#14557,.T.);
#22960=EDGE_CURVE('',#18464,#18465,#14558,.T.);
#22961=EDGE_CURVE('',#18465,#18461,#10019,.T.);
#22962=EDGE_CURVE('',#18463,#18460,#10020,.T.);
#22963=EDGE_CURVE('',#18459,#18464,#1503,.T.);
#22964=EDGE_CURVE('',#18466,#18467,#14559,.T.);
#22965=EDGE_CURVE('',#18466,#18462,#1504,.T.);
#22966=EDGE_CURVE('',#18461,#18467,#10021,.T.);
#22967=EDGE_CURVE('',#18468,#18469,#14560,.T.);
#22968=EDGE_CURVE('',#18469,#18466,#14561,.T.);
#22969=EDGE_CURVE('',#18467,#18468,#14562,.T.);
#22970=EDGE_CURVE('',#18470,#18471,#1505,.T.);
#22971=EDGE_CURVE('',#18471,#18406,#1506,.T.);
#22972=EDGE_CURVE('',#18406,#18472,#10022,.T.);
#22973=EDGE_CURVE('',#18473,#18472,#14563,.T.);
#22974=EDGE_CURVE('',#18473,#18474,#14564,.T.);
#22975=EDGE_CURVE('',#18474,#18470,#10023,.T.);
#22976=EDGE_CURVE('',#18472,#18469,#10024,.T.);
#22977=EDGE_CURVE('',#18468,#18473,#1507,.T.);
#22978=EDGE_CURVE('',#18475,#18476,#1508,.T.);
#22979=EDGE_CURVE('',#18475,#18471,#1509,.T.);
#22980=EDGE_CURVE('',#18470,#18476,#10025,.T.);
#22981=EDGE_CURVE('',#18477,#18478,#14565,.T.);
#22982=EDGE_CURVE('',#18478,#18475,#1510,.T.);
#22983=EDGE_CURVE('',#18476,#18477,#14566,.T.);
#22984=EDGE_CURVE('',#18479,#18480,#14567,.T.);
#22985=EDGE_CURVE('',#18480,#18415,#14568,.T.);
#22986=EDGE_CURVE('',#18415,#18481,#10026,.T.);
#22987=EDGE_CURVE('',#18482,#18481,#14569,.T.);
#22988=EDGE_CURVE('',#18482,#18483,#14570,.T.);
#22989=EDGE_CURVE('',#18483,#18479,#10027,.T.);
#22990=EDGE_CURVE('',#18481,#18478,#10028,.T.);
#22991=EDGE_CURVE('',#18477,#18482,#1511,.T.);
#22992=EDGE_CURVE('',#18484,#18485,#14571,.T.);
#22993=EDGE_CURVE('',#18484,#18480,#1512,.T.);
#22994=EDGE_CURVE('',#18479,#18485,#10029,.T.);
#22995=EDGE_CURVE('',#18486,#18487,#14572,.T.);
#22996=EDGE_CURVE('',#18487,#18484,#14573,.T.);
#22997=EDGE_CURVE('',#18485,#18486,#14574,.T.);
#22998=EDGE_CURVE('',#18488,#18489,#14575,.T.);
#22999=EDGE_CURVE('',#18489,#18424,#14576,.T.);
#23000=EDGE_CURVE('',#18424,#18490,#10030,.T.);
#23001=EDGE_CURVE('',#18491,#18490,#14577,.T.);
#23002=EDGE_CURVE('',#18491,#18492,#14578,.T.);
#23003=EDGE_CURVE('',#18492,#18488,#10031,.T.);
#23004=EDGE_CURVE('',#18490,#18487,#10032,.T.);
#23005=EDGE_CURVE('',#18486,#18491,#1513,.T.);
#23006=EDGE_CURVE('',#18493,#18494,#14579,.T.);
#23007=EDGE_CURVE('',#18493,#18489,#1514,.T.);
#23008=EDGE_CURVE('',#18488,#18494,#10033,.T.);
#23009=EDGE_CURVE('',#18495,#18496,#14580,.T.);
#23010=EDGE_CURVE('',#18496,#18493,#14581,.T.);
#23011=EDGE_CURVE('',#18494,#18495,#14582,.T.);
#23012=EDGE_CURVE('',#18497,#18498,#14583,.T.);
#23013=EDGE_CURVE('',#18498,#18433,#14584,.T.);
#23014=EDGE_CURVE('',#18433,#18499,#10034,.T.);
#23015=EDGE_CURVE('',#18500,#18499,#14585,.T.);
#23016=EDGE_CURVE('',#18500,#18501,#14586,.T.);
#23017=EDGE_CURVE('',#18501,#18497,#10035,.F.);
#23018=EDGE_CURVE('',#18499,#18496,#10036,.T.);
#23019=EDGE_CURVE('',#18495,#18500,#1515,.T.);
#23020=EDGE_CURVE('',#17642,#18498,#14587,.T.);
#23021=EDGE_CURVE('',#18497,#17643,#10037,.F.);
#23022=EDGE_CURVE('',#17639,#18442,#944,.T.);
#23023=EDGE_CURVE('',#18442,#18502,#10038,.T.);
#23024=EDGE_CURVE('',#17640,#18502,#945,.T.);
#23025=EDGE_CURVE('',#18502,#17641,#946,.T.);
#23026=EDGE_CURVE('',#18503,#18504,#14588,.T.);
#23027=EDGE_CURVE('',#18504,#17373,#14589,.T.);
#23028=EDGE_CURVE('',#18505,#17372,#1516,.T.);
#23029=EDGE_CURVE('',#18505,#18506,#947,.T.);
#23030=EDGE_CURVE('',#18506,#18503,#10039,.T.);
#23031=EDGE_CURVE('',#18507,#18508,#14590,.T.);
#23032=EDGE_CURVE('',#18507,#18504,#1517,.T.);
#23033=EDGE_CURVE('',#18503,#18508,#10040,.T.);
#23034=EDGE_CURVE('',#18509,#18510,#14591,.T.);
#23035=EDGE_CURVE('',#18510,#18507,#14592,.T.);
#23036=EDGE_CURVE('',#18508,#18509,#14593,.T.);
#23037=EDGE_CURVE('',#18511,#18512,#14594,.T.);
#23038=EDGE_CURVE('',#18512,#18447,#14595,.T.);
#23039=EDGE_CURVE('',#18447,#18513,#10041,.T.);
#23040=EDGE_CURVE('',#18514,#18513,#14596,.T.);
#23041=EDGE_CURVE('',#18514,#18515,#14597,.T.);
#23042=EDGE_CURVE('',#18515,#18511,#10042,.T.);
#23043=EDGE_CURVE('',#18513,#18510,#10043,.T.);
#23044=EDGE_CURVE('',#18509,#18514,#1518,.T.);
#23045=EDGE_CURVE('',#17375,#18446,#948,.T.);
#23046=EDGE_CURVE('',#18516,#18517,#14598,.T.);
#23047=EDGE_CURVE('',#18516,#18512,#1519,.T.);
#23048=EDGE_CURVE('',#18511,#18517,#10044,.T.);
#23049=EDGE_CURVE('',#18518,#18519,#14599,.T.);
#23050=EDGE_CURVE('',#18519,#18516,#14600,.T.);
#23051=EDGE_CURVE('',#18517,#18518,#14601,.T.);
#23052=EDGE_CURVE('',#18520,#18521,#14602,.T.);
#23053=EDGE_CURVE('',#18521,#18456,#14603,.T.);
#23054=EDGE_CURVE('',#18456,#18522,#10045,.T.);
#23055=EDGE_CURVE('',#18523,#18522,#14604,.T.);
#23056=EDGE_CURVE('',#18523,#18524,#14605,.T.);
#23057=EDGE_CURVE('',#18524,#18520,#10046,.T.);
#23058=EDGE_CURVE('',#18522,#18519,#10047,.T.);
#23059=EDGE_CURVE('',#18518,#18523,#1520,.T.);
#23060=EDGE_CURVE('',#18525,#18526,#14606,.T.);
#23061=EDGE_CURVE('',#18525,#18521,#1521,.T.);
#23062=EDGE_CURVE('',#18520,#18526,#10048,.T.);
#23063=EDGE_CURVE('',#18527,#18528,#14607,.T.);
#23064=EDGE_CURVE('',#18528,#18525,#14608,.T.);
#23065=EDGE_CURVE('',#18526,#18527,#14609,.T.);
#23066=EDGE_CURVE('',#18529,#18530,#1522,.T.);
#23067=EDGE_CURVE('',#18530,#18465,#1523,.T.);
#23068=EDGE_CURVE('',#18465,#18531,#10049,.T.);
#23069=EDGE_CURVE('',#18532,#18531,#14610,.T.);
#23070=EDGE_CURVE('',#18532,#18533,#14611,.T.);
#23071=EDGE_CURVE('',#18533,#18529,#10050,.T.);
#23072=EDGE_CURVE('',#18531,#18528,#10051,.T.);
#23073=EDGE_CURVE('',#18527,#18532,#1524,.T.);
#23074=EDGE_CURVE('',#18534,#18535,#1525,.T.);
#23075=EDGE_CURVE('',#18534,#18530,#1526,.T.);
#23076=EDGE_CURVE('',#18529,#18535,#10052,.T.);
#23077=EDGE_CURVE('',#18536,#18537,#14612,.T.);
#23078=EDGE_CURVE('',#18537,#18534,#1527,.T.);
#23079=EDGE_CURVE('',#18535,#18536,#14613,.T.);
#23080=EDGE_CURVE('',#18538,#18539,#14614,.T.);
#23081=EDGE_CURVE('',#18539,#18474,#14615,.T.);
#23082=EDGE_CURVE('',#18474,#18540,#10053,.T.);
#23083=EDGE_CURVE('',#18541,#18540,#14616,.T.);
#23084=EDGE_CURVE('',#18541,#18542,#14617,.T.);
#23085=EDGE_CURVE('',#18542,#18538,#10054,.T.);
#23086=EDGE_CURVE('',#18540,#18537,#10055,.T.);
#23087=EDGE_CURVE('',#18536,#18541,#1528,.T.);
#23088=EDGE_CURVE('',#18543,#18544,#14618,.T.);
#23089=EDGE_CURVE('',#18543,#18539,#1529,.T.);
#23090=EDGE_CURVE('',#18538,#18544,#10056,.T.);
#23091=EDGE_CURVE('',#18545,#18546,#14619,.T.);
#23092=EDGE_CURVE('',#18546,#18543,#14620,.T.);
#23093=EDGE_CURVE('',#18544,#18545,#14621,.T.);
#23094=EDGE_CURVE('',#18547,#18548,#14622,.T.);
#23095=EDGE_CURVE('',#18548,#18483,#14623,.T.);
#23096=EDGE_CURVE('',#18483,#18549,#10057,.T.);
#23097=EDGE_CURVE('',#18550,#18549,#14624,.T.);
#23098=EDGE_CURVE('',#18550,#18551,#14625,.T.);
#23099=EDGE_CURVE('',#18551,#18547,#10058,.T.);
#23100=EDGE_CURVE('',#18549,#18546,#10059,.T.);
#23101=EDGE_CURVE('',#18545,#18550,#1530,.T.);
#23102=EDGE_CURVE('',#18552,#18553,#14626,.T.);
#23103=EDGE_CURVE('',#18552,#18548,#1531,.T.);
#23104=EDGE_CURVE('',#18547,#18553,#10060,.T.);
#23105=EDGE_CURVE('',#18554,#18555,#14627,.T.);
#23106=EDGE_CURVE('',#18555,#18552,#14628,.T.);
#23107=EDGE_CURVE('',#18553,#18554,#14629,.T.);
#23108=EDGE_CURVE('',#18556,#18557,#14630,.T.);
#23109=EDGE_CURVE('',#18557,#18492,#14631,.T.);
#23110=EDGE_CURVE('',#18492,#18558,#10061,.T.);
#23111=EDGE_CURVE('',#18559,#18558,#14632,.T.);
#23112=EDGE_CURVE('',#18559,#18560,#14633,.T.);
#23113=EDGE_CURVE('',#18560,#18556,#10062,.F.);
#23114=EDGE_CURVE('',#18558,#18555,#10063,.T.);
#23115=EDGE_CURVE('',#18554,#18559,#1532,.T.);
#23116=EDGE_CURVE('',#17648,#18557,#14634,.T.);
#23117=EDGE_CURVE('',#18556,#17649,#10064,.F.);
#23118=EDGE_CURVE('',#17645,#18501,#949,.T.);
#23119=EDGE_CURVE('',#18501,#18561,#10065,.T.);
#23120=EDGE_CURVE('',#17646,#18561,#950,.T.);
#23121=EDGE_CURVE('',#18561,#17647,#951,.T.);
#23122=EDGE_CURVE('',#18562,#18563,#14635,.T.);
#23123=EDGE_CURVE('',#18563,#17369,#14636,.T.);
#23124=EDGE_CURVE('',#18564,#17368,#1533,.T.);
#23125=EDGE_CURVE('',#18564,#18565,#952,.T.);
#23126=EDGE_CURVE('',#18565,#18562,#10066,.T.);
#23127=EDGE_CURVE('',#18566,#18567,#14637,.T.);
#23128=EDGE_CURVE('',#18566,#18563,#1534,.T.);
#23129=EDGE_CURVE('',#18562,#18567,#10067,.T.);
#23130=EDGE_CURVE('',#18568,#18569,#14638,.T.);
#23131=EDGE_CURVE('',#18569,#18566,#14639,.T.);
#23132=EDGE_CURVE('',#18567,#18568,#14640,.T.);
#23133=EDGE_CURVE('',#18570,#18571,#14641,.T.);
#23134=EDGE_CURVE('',#18571,#18506,#14642,.T.);
#23135=EDGE_CURVE('',#18506,#18572,#10068,.T.);
#23136=EDGE_CURVE('',#18573,#18572,#14643,.T.);
#23137=EDGE_CURVE('',#18573,#18574,#14644,.T.);
#23138=EDGE_CURVE('',#18574,#18570,#10069,.T.);
#23139=EDGE_CURVE('',#18572,#18569,#10070,.T.);
#23140=EDGE_CURVE('',#18568,#18573,#1535,.T.);
#23141=EDGE_CURVE('',#17371,#18505,#953,.T.);
#23142=EDGE_CURVE('',#18575,#18576,#14645,.T.);
#23143=EDGE_CURVE('',#18575,#18571,#1536,.T.);
#23144=EDGE_CURVE('',#18570,#18576,#10071,.T.);
#23145=EDGE_CURVE('',#18577,#18578,#14646,.T.);
#23146=EDGE_CURVE('',#18578,#18575,#14647,.T.);
#23147=EDGE_CURVE('',#18576,#18577,#14648,.T.);
#23148=EDGE_CURVE('',#18579,#18580,#14649,.T.);
#23149=EDGE_CURVE('',#18580,#18515,#14650,.T.);
#23150=EDGE_CURVE('',#18515,#18581,#10072,.T.);
#23151=EDGE_CURVE('',#18582,#18581,#14651,.T.);
#23152=EDGE_CURVE('',#18582,#18583,#14652,.T.);
#23153=EDGE_CURVE('',#18583,#18579,#10073,.T.);
#23154=EDGE_CURVE('',#18581,#18578,#10074,.T.);
#23155=EDGE_CURVE('',#18577,#18582,#1537,.T.);
#23156=EDGE_CURVE('',#18584,#18585,#14653,.T.);
#23157=EDGE_CURVE('',#18584,#18580,#1538,.T.);
#23158=EDGE_CURVE('',#18579,#18585,#10075,.T.);
#23159=EDGE_CURVE('',#18586,#18587,#14654,.T.);
#23160=EDGE_CURVE('',#18587,#18584,#14655,.T.);
#23161=EDGE_CURVE('',#18585,#18586,#14656,.T.);
#23162=EDGE_CURVE('',#18588,#18589,#1539,.T.);
#23163=EDGE_CURVE('',#18589,#18524,#1540,.T.);
#23164=EDGE_CURVE('',#18524,#18590,#10076,.T.);
#23165=EDGE_CURVE('',#18591,#18590,#14657,.T.);
#23166=EDGE_CURVE('',#18591,#18592,#14658,.T.);
#23167=EDGE_CURVE('',#18592,#18588,#10077,.T.);
#23168=EDGE_CURVE('',#18590,#18587,#10078,.T.);
#23169=EDGE_CURVE('',#18586,#18591,#1541,.T.);
#23170=EDGE_CURVE('',#18593,#18594,#1542,.T.);
#23171=EDGE_CURVE('',#18593,#18589,#1543,.T.);
#23172=EDGE_CURVE('',#18588,#18594,#10079,.T.);
#23173=EDGE_CURVE('',#18595,#18596,#14659,.T.);
#23174=EDGE_CURVE('',#18596,#18593,#1544,.T.);
#23175=EDGE_CURVE('',#18594,#18595,#14660,.T.);
#23176=EDGE_CURVE('',#18597,#18598,#14661,.T.);
#23177=EDGE_CURVE('',#18598,#18533,#14662,.T.);
#23178=EDGE_CURVE('',#18533,#18599,#10080,.T.);
#23179=EDGE_CURVE('',#18600,#18599,#14663,.T.);
#23180=EDGE_CURVE('',#18600,#18601,#14664,.T.);
#23181=EDGE_CURVE('',#18601,#18597,#10081,.T.);
#23182=EDGE_CURVE('',#18599,#18596,#10082,.T.);
#23183=EDGE_CURVE('',#18595,#18600,#1545,.T.);
#23184=EDGE_CURVE('',#18602,#18603,#14665,.T.);
#23185=EDGE_CURVE('',#18602,#18598,#1546,.T.);
#23186=EDGE_CURVE('',#18597,#18603,#10083,.T.);
#23187=EDGE_CURVE('',#18604,#18605,#14666,.T.);
#23188=EDGE_CURVE('',#18605,#18602,#14667,.T.);
#23189=EDGE_CURVE('',#18603,#18604,#14668,.T.);
#23190=EDGE_CURVE('',#18606,#18607,#14669,.T.);
#23191=EDGE_CURVE('',#18607,#18542,#14670,.T.);
#23192=EDGE_CURVE('',#18542,#18608,#10084,.T.);
#23193=EDGE_CURVE('',#18609,#18608,#14671,.T.);
#23194=EDGE_CURVE('',#18609,#18610,#14672,.T.);
#23195=EDGE_CURVE('',#18610,#18606,#10085,.T.);
#23196=EDGE_CURVE('',#18608,#18605,#10086,.T.);
#23197=EDGE_CURVE('',#18604,#18609,#1547,.T.);
#23198=EDGE_CURVE('',#18611,#18612,#14673,.T.);
#23199=EDGE_CURVE('',#18611,#18607,#1548,.T.);
#23200=EDGE_CURVE('',#18606,#18612,#10087,.T.);
#23201=EDGE_CURVE('',#18613,#18614,#14674,.T.);
#23202=EDGE_CURVE('',#18614,#18611,#14675,.T.);
#23203=EDGE_CURVE('',#18612,#18613,#14676,.T.);
#23204=EDGE_CURVE('',#18615,#18616,#14677,.T.);
#23205=EDGE_CURVE('',#18616,#18551,#14678,.T.);
#23206=EDGE_CURVE('',#18551,#18617,#10088,.T.);
#23207=EDGE_CURVE('',#18618,#18617,#14679,.T.);
#23208=EDGE_CURVE('',#18618,#18619,#14680,.T.);
#23209=EDGE_CURVE('',#18619,#18615,#10089,.F.);
#23210=EDGE_CURVE('',#18617,#18614,#10090,.T.);
#23211=EDGE_CURVE('',#18613,#18618,#1549,.T.);
#23212=EDGE_CURVE('',#17654,#18616,#14681,.T.);
#23213=EDGE_CURVE('',#18615,#17655,#10091,.F.);
#23214=EDGE_CURVE('',#17651,#18560,#954,.T.);
#23215=EDGE_CURVE('',#18560,#18620,#10092,.T.);
#23216=EDGE_CURVE('',#17652,#18620,#955,.T.);
#23217=EDGE_CURVE('',#18620,#17653,#956,.T.);
#23218=EDGE_CURVE('',#18621,#18622,#14682,.T.);
#23219=EDGE_CURVE('',#18622,#17365,#14683,.T.);
#23220=EDGE_CURVE('',#18623,#17364,#1550,.T.);
#23221=EDGE_CURVE('',#18623,#18624,#957,.T.);
#23222=EDGE_CURVE('',#18624,#18621,#10093,.T.);
#23223=EDGE_CURVE('',#18625,#18626,#14684,.T.);
#23224=EDGE_CURVE('',#18625,#18622,#1551,.T.);
#23225=EDGE_CURVE('',#18621,#18626,#10094,.T.);
#23226=EDGE_CURVE('',#18627,#18628,#14685,.T.);
#23227=EDGE_CURVE('',#18628,#18625,#14686,.T.);
#23228=EDGE_CURVE('',#18626,#18627,#14687,.T.);
#23229=EDGE_CURVE('',#18629,#18630,#14688,.T.);
#23230=EDGE_CURVE('',#18630,#18565,#14689,.T.);
#23231=EDGE_CURVE('',#18565,#18631,#10095,.T.);
#23232=EDGE_CURVE('',#18632,#18631,#14690,.T.);
#23233=EDGE_CURVE('',#18632,#18633,#14691,.T.);
#23234=EDGE_CURVE('',#18633,#18629,#10096,.T.);
#23235=EDGE_CURVE('',#18631,#18628,#10097,.T.);
#23236=EDGE_CURVE('',#18627,#18632,#1552,.T.);
#23237=EDGE_CURVE('',#17367,#18564,#958,.T.);
#23238=EDGE_CURVE('',#18634,#18635,#14692,.T.);
#23239=EDGE_CURVE('',#18634,#18630,#1553,.T.);
#23240=EDGE_CURVE('',#18629,#18635,#10098,.T.);
#23241=EDGE_CURVE('',#18636,#18637,#14693,.T.);
#23242=EDGE_CURVE('',#18637,#18634,#14694,.T.);
#23243=EDGE_CURVE('',#18635,#18636,#14695,.T.);
#23244=EDGE_CURVE('',#18638,#18639,#14696,.T.);
#23245=EDGE_CURVE('',#18639,#18574,#14697,.T.);
#23246=EDGE_CURVE('',#18574,#18640,#10099,.T.);
#23247=EDGE_CURVE('',#18641,#18640,#14698,.T.);
#23248=EDGE_CURVE('',#18641,#18642,#14699,.T.);
#23249=EDGE_CURVE('',#18642,#18638,#10100,.T.);
#23250=EDGE_CURVE('',#18640,#18637,#10101,.T.);
#23251=EDGE_CURVE('',#18636,#18641,#1554,.T.);
#23252=EDGE_CURVE('',#18643,#18644,#14700,.T.);
#23253=EDGE_CURVE('',#18643,#18639,#1555,.T.);
#23254=EDGE_CURVE('',#18638,#18644,#10102,.T.);
#23255=EDGE_CURVE('',#18645,#18646,#14701,.T.);
#23256=EDGE_CURVE('',#18646,#18643,#14702,.T.);
#23257=EDGE_CURVE('',#18644,#18645,#14703,.T.);
#23258=EDGE_CURVE('',#18647,#18648,#1556,.T.);
#23259=EDGE_CURVE('',#18648,#18583,#1557,.T.);
#23260=EDGE_CURVE('',#18583,#18649,#10103,.T.);
#23261=EDGE_CURVE('',#18650,#18649,#14704,.T.);
#23262=EDGE_CURVE('',#18650,#18651,#14705,.T.);
#23263=EDGE_CURVE('',#18651,#18647,#10104,.T.);
#23264=EDGE_CURVE('',#18649,#18646,#10105,.T.);
#23265=EDGE_CURVE('',#18645,#18650,#1558,.T.);
#23266=EDGE_CURVE('',#18652,#18653,#1559,.T.);
#23267=EDGE_CURVE('',#18652,#18648,#1560,.T.);
#23268=EDGE_CURVE('',#18647,#18653,#10106,.T.);
#23269=EDGE_CURVE('',#18654,#18655,#14706,.T.);
#23270=EDGE_CURVE('',#18655,#18652,#1561,.T.);
#23271=EDGE_CURVE('',#18653,#18654,#14707,.T.);
#23272=EDGE_CURVE('',#18656,#18657,#14708,.T.);
#23273=EDGE_CURVE('',#18657,#18592,#14709,.T.);
#23274=EDGE_CURVE('',#18592,#18658,#10107,.T.);
#23275=EDGE_CURVE('',#18659,#18658,#14710,.T.);
#23276=EDGE_CURVE('',#18659,#18660,#14711,.T.);
#23277=EDGE_CURVE('',#18660,#18656,#10108,.T.);
#23278=EDGE_CURVE('',#18658,#18655,#10109,.T.);
#23279=EDGE_CURVE('',#18654,#18659,#1562,.T.);
#23280=EDGE_CURVE('',#18661,#18662,#14712,.T.);
#23281=EDGE_CURVE('',#18661,#18657,#1563,.T.);
#23282=EDGE_CURVE('',#18656,#18662,#10110,.T.);
#23283=EDGE_CURVE('',#18663,#18664,#14713,.T.);
#23284=EDGE_CURVE('',#18664,#18661,#14714,.T.);
#23285=EDGE_CURVE('',#18662,#18663,#14715,.T.);
#23286=EDGE_CURVE('',#18665,#18666,#14716,.T.);
#23287=EDGE_CURVE('',#18666,#18601,#14717,.T.);
#23288=EDGE_CURVE('',#18601,#18667,#10111,.T.);
#23289=EDGE_CURVE('',#18668,#18667,#14718,.T.);
#23290=EDGE_CURVE('',#18668,#18669,#14719,.T.);
#23291=EDGE_CURVE('',#18669,#18665,#10112,.T.);
#23292=EDGE_CURVE('',#18667,#18664,#10113,.T.);
#23293=EDGE_CURVE('',#18663,#18668,#1564,.T.);
#23294=EDGE_CURVE('',#18670,#18671,#14720,.T.);
#23295=EDGE_CURVE('',#18670,#18666,#1565,.T.);
#23296=EDGE_CURVE('',#18665,#18671,#10114,.T.);
#23297=EDGE_CURVE('',#18672,#18673,#14721,.T.);
#23298=EDGE_CURVE('',#18673,#18670,#14722,.T.);
#23299=EDGE_CURVE('',#18671,#18672,#14723,.T.);
#23300=EDGE_CURVE('',#18674,#18675,#14724,.T.);
#23301=EDGE_CURVE('',#18675,#18610,#14725,.T.);
#23302=EDGE_CURVE('',#18610,#18676,#10115,.T.);
#23303=EDGE_CURVE('',#18677,#18676,#14726,.T.);
#23304=EDGE_CURVE('',#18677,#18678,#14727,.T.);
#23305=EDGE_CURVE('',#18678,#18674,#10116,.F.);
#23306=EDGE_CURVE('',#18676,#18673,#10117,.T.);
#23307=EDGE_CURVE('',#18672,#18677,#1566,.T.);
#23308=EDGE_CURVE('',#17660,#18675,#14728,.T.);
#23309=EDGE_CURVE('',#18674,#17661,#10118,.F.);
#23310=EDGE_CURVE('',#17657,#18619,#959,.T.);
#23311=EDGE_CURVE('',#18619,#18679,#10119,.T.);
#23312=EDGE_CURVE('',#17658,#18679,#960,.T.);
#23313=EDGE_CURVE('',#18679,#17659,#961,.T.);
#23314=EDGE_CURVE('',#18680,#18681,#14729,.T.);
#23315=EDGE_CURVE('',#18681,#17361,#14730,.T.);
#23316=EDGE_CURVE('',#18682,#17360,#1567,.T.);
#23317=EDGE_CURVE('',#18682,#18683,#962,.T.);
#23318=EDGE_CURVE('',#18683,#18680,#10120,.T.);
#23319=EDGE_CURVE('',#18684,#18685,#14731,.T.);
#23320=EDGE_CURVE('',#18684,#18681,#1568,.T.);
#23321=EDGE_CURVE('',#18680,#18685,#10121,.T.);
#23322=EDGE_CURVE('',#18686,#18687,#14732,.T.);
#23323=EDGE_CURVE('',#18687,#18684,#14733,.T.);
#23324=EDGE_CURVE('',#18685,#18686,#14734,.T.);
#23325=EDGE_CURVE('',#18688,#18689,#14735,.T.);
#23326=EDGE_CURVE('',#18689,#18624,#14736,.T.);
#23327=EDGE_CURVE('',#18624,#18690,#10122,.T.);
#23328=EDGE_CURVE('',#18691,#18690,#14737,.T.);
#23329=EDGE_CURVE('',#18691,#18692,#14738,.T.);
#23330=EDGE_CURVE('',#18692,#18688,#10123,.T.);
#23331=EDGE_CURVE('',#18690,#18687,#10124,.T.);
#23332=EDGE_CURVE('',#18686,#18691,#1569,.T.);
#23333=EDGE_CURVE('',#17363,#18623,#963,.T.);
#23334=EDGE_CURVE('',#18693,#18694,#14739,.T.);
#23335=EDGE_CURVE('',#18693,#18689,#1570,.T.);
#23336=EDGE_CURVE('',#18688,#18694,#10125,.T.);
#23337=EDGE_CURVE('',#18695,#18696,#14740,.T.);
#23338=EDGE_CURVE('',#18696,#18693,#14741,.T.);
#23339=EDGE_CURVE('',#18694,#18695,#14742,.T.);
#23340=EDGE_CURVE('',#18697,#18698,#14743,.T.);
#23341=EDGE_CURVE('',#18698,#18633,#14744,.T.);
#23342=EDGE_CURVE('',#18633,#18699,#10126,.T.);
#23343=EDGE_CURVE('',#18700,#18699,#14745,.T.);
#23344=EDGE_CURVE('',#18700,#18701,#14746,.T.);
#23345=EDGE_CURVE('',#18701,#18697,#10127,.T.);
#23346=EDGE_CURVE('',#18699,#18696,#10128,.T.);
#23347=EDGE_CURVE('',#18695,#18700,#1571,.T.);
#23348=EDGE_CURVE('',#18702,#18703,#14747,.T.);
#23349=EDGE_CURVE('',#18702,#18698,#1572,.T.);
#23350=EDGE_CURVE('',#18697,#18703,#10129,.T.);
#23351=EDGE_CURVE('',#18704,#18705,#14748,.T.);
#23352=EDGE_CURVE('',#18705,#18702,#14749,.T.);
#23353=EDGE_CURVE('',#18703,#18704,#14750,.T.);
#23354=EDGE_CURVE('',#18706,#18707,#1573,.T.);
#23355=EDGE_CURVE('',#18707,#18642,#1574,.T.);
#23356=EDGE_CURVE('',#18642,#18708,#10130,.T.);
#23357=EDGE_CURVE('',#18709,#18708,#14751,.T.);
#23358=EDGE_CURVE('',#18709,#18710,#14752,.T.);
#23359=EDGE_CURVE('',#18710,#18706,#10131,.T.);
#23360=EDGE_CURVE('',#18708,#18705,#10132,.T.);
#23361=EDGE_CURVE('',#18704,#18709,#1575,.T.);
#23362=EDGE_CURVE('',#18711,#18712,#1576,.T.);
#23363=EDGE_CURVE('',#18711,#18707,#1577,.T.);
#23364=EDGE_CURVE('',#18706,#18712,#10133,.T.);
#23365=EDGE_CURVE('',#18713,#18714,#14753,.T.);
#23366=EDGE_CURVE('',#18714,#18711,#1578,.T.);
#23367=EDGE_CURVE('',#18712,#18713,#14754,.T.);
#23368=EDGE_CURVE('',#18715,#18716,#14755,.T.);
#23369=EDGE_CURVE('',#18716,#18651,#14756,.T.);
#23370=EDGE_CURVE('',#18651,#18717,#10134,.T.);
#23371=EDGE_CURVE('',#18718,#18717,#14757,.T.);
#23372=EDGE_CURVE('',#18718,#18719,#14758,.T.);
#23373=EDGE_CURVE('',#18719,#18715,#10135,.T.);
#23374=EDGE_CURVE('',#18717,#18714,#10136,.T.);
#23375=EDGE_CURVE('',#18713,#18718,#1579,.T.);
#23376=EDGE_CURVE('',#18720,#18721,#14759,.T.);
#23377=EDGE_CURVE('',#18720,#18716,#1580,.T.);
#23378=EDGE_CURVE('',#18715,#18721,#10137,.T.);
#23379=EDGE_CURVE('',#18722,#18723,#14760,.T.);
#23380=EDGE_CURVE('',#18723,#18720,#14761,.T.);
#23381=EDGE_CURVE('',#18721,#18722,#14762,.T.);
#23382=EDGE_CURVE('',#18724,#18725,#14763,.T.);
#23383=EDGE_CURVE('',#18725,#18660,#14764,.T.);
#23384=EDGE_CURVE('',#18660,#18726,#10138,.T.);
#23385=EDGE_CURVE('',#18727,#18726,#14765,.T.);
#23386=EDGE_CURVE('',#18727,#18728,#14766,.T.);
#23387=EDGE_CURVE('',#18728,#18724,#10139,.T.);
#23388=EDGE_CURVE('',#18726,#18723,#10140,.T.);
#23389=EDGE_CURVE('',#18722,#18727,#1581,.T.);
#23390=EDGE_CURVE('',#18729,#18730,#14767,.T.);
#23391=EDGE_CURVE('',#18729,#18725,#1582,.T.);
#23392=EDGE_CURVE('',#18724,#18730,#10141,.T.);
#23393=EDGE_CURVE('',#18731,#18732,#14768,.T.);
#23394=EDGE_CURVE('',#18732,#18729,#14769,.T.);
#23395=EDGE_CURVE('',#18730,#18731,#14770,.T.);
#23396=EDGE_CURVE('',#18733,#18734,#14771,.T.);
#23397=EDGE_CURVE('',#18734,#18669,#14772,.T.);
#23398=EDGE_CURVE('',#18669,#18735,#10142,.T.);
#23399=EDGE_CURVE('',#18736,#18735,#14773,.T.);
#23400=EDGE_CURVE('',#18736,#18737,#14774,.T.);
#23401=EDGE_CURVE('',#18737,#18733,#10143,.F.);
#23402=EDGE_CURVE('',#18735,#18732,#10144,.T.);
#23403=EDGE_CURVE('',#18731,#18736,#1583,.T.);
#23404=EDGE_CURVE('',#17666,#18734,#14775,.T.);
#23405=EDGE_CURVE('',#18733,#17667,#10145,.F.);
#23406=EDGE_CURVE('',#17663,#18678,#964,.T.);
#23407=EDGE_CURVE('',#18678,#18738,#10146,.T.);
#23408=EDGE_CURVE('',#17664,#18738,#965,.T.);
#23409=EDGE_CURVE('',#18738,#17665,#966,.T.);
#23410=EDGE_CURVE('',#18739,#18740,#14776,.T.);
#23411=EDGE_CURVE('',#18740,#17357,#14777,.T.);
#23412=EDGE_CURVE('',#18741,#17356,#1584,.T.);
#23413=EDGE_CURVE('',#18741,#18742,#967,.T.);
#23414=EDGE_CURVE('',#18742,#18739,#10147,.T.);
#23415=EDGE_CURVE('',#18743,#18744,#14778,.T.);
#23416=EDGE_CURVE('',#18743,#18740,#1585,.T.);
#23417=EDGE_CURVE('',#18739,#18744,#10148,.T.);
#23418=EDGE_CURVE('',#18745,#18746,#14779,.T.);
#23419=EDGE_CURVE('',#18746,#18743,#14780,.T.);
#23420=EDGE_CURVE('',#18744,#18745,#14781,.T.);
#23421=EDGE_CURVE('',#18747,#18748,#14782,.T.);
#23422=EDGE_CURVE('',#18748,#18683,#14783,.T.);
#23423=EDGE_CURVE('',#18683,#18749,#10149,.T.);
#23424=EDGE_CURVE('',#18750,#18749,#14784,.T.);
#23425=EDGE_CURVE('',#18750,#18751,#14785,.T.);
#23426=EDGE_CURVE('',#18751,#18747,#10150,.T.);
#23427=EDGE_CURVE('',#18749,#18746,#10151,.T.);
#23428=EDGE_CURVE('',#18745,#18750,#1586,.T.);
#23429=EDGE_CURVE('',#17359,#18682,#968,.T.);
#23430=EDGE_CURVE('',#18752,#18753,#14786,.T.);
#23431=EDGE_CURVE('',#18752,#18748,#1587,.T.);
#23432=EDGE_CURVE('',#18747,#18753,#10152,.T.);
#23433=EDGE_CURVE('',#18754,#18755,#14787,.T.);
#23434=EDGE_CURVE('',#18755,#18752,#14788,.T.);
#23435=EDGE_CURVE('',#18753,#18754,#14789,.T.);
#23436=EDGE_CURVE('',#18756,#18757,#14790,.T.);
#23437=EDGE_CURVE('',#18757,#18692,#14791,.T.);
#23438=EDGE_CURVE('',#18692,#18758,#10153,.T.);
#23439=EDGE_CURVE('',#18759,#18758,#14792,.T.);
#23440=EDGE_CURVE('',#18759,#18760,#14793,.T.);
#23441=EDGE_CURVE('',#18760,#18756,#10154,.T.);
#23442=EDGE_CURVE('',#18758,#18755,#10155,.T.);
#23443=EDGE_CURVE('',#18754,#18759,#1588,.T.);
#23444=EDGE_CURVE('',#18761,#18762,#14794,.T.);
#23445=EDGE_CURVE('',#18761,#18757,#1589,.T.);
#23446=EDGE_CURVE('',#18756,#18762,#10156,.T.);
#23447=EDGE_CURVE('',#18763,#18764,#14795,.T.);
#23448=EDGE_CURVE('',#18764,#18761,#14796,.T.);
#23449=EDGE_CURVE('',#18762,#18763,#14797,.T.);
#23450=EDGE_CURVE('',#18765,#18766,#1590,.T.);
#23451=EDGE_CURVE('',#18766,#18701,#1591,.T.);
#23452=EDGE_CURVE('',#18701,#18767,#10157,.T.);
#23453=EDGE_CURVE('',#18768,#18767,#14798,.T.);
#23454=EDGE_CURVE('',#18768,#18769,#14799,.T.);
#23455=EDGE_CURVE('',#18769,#18765,#10158,.T.);
#23456=EDGE_CURVE('',#18767,#18764,#10159,.T.);
#23457=EDGE_CURVE('',#18763,#18768,#1592,.T.);
#23458=EDGE_CURVE('',#18770,#18771,#1593,.T.);
#23459=EDGE_CURVE('',#18770,#18766,#1594,.T.);
#23460=EDGE_CURVE('',#18765,#18771,#10160,.T.);
#23461=EDGE_CURVE('',#18772,#18773,#14800,.T.);
#23462=EDGE_CURVE('',#18773,#18770,#1595,.T.);
#23463=EDGE_CURVE('',#18771,#18772,#14801,.T.);
#23464=EDGE_CURVE('',#18774,#18775,#14802,.T.);
#23465=EDGE_CURVE('',#18775,#18710,#14803,.T.);
#23466=EDGE_CURVE('',#18710,#18776,#10161,.T.);
#23467=EDGE_CURVE('',#18777,#18776,#14804,.T.);
#23468=EDGE_CURVE('',#18777,#18778,#14805,.T.);
#23469=EDGE_CURVE('',#18778,#18774,#10162,.T.);
#23470=EDGE_CURVE('',#18776,#18773,#10163,.T.);
#23471=EDGE_CURVE('',#18772,#18777,#1596,.T.);
#23472=EDGE_CURVE('',#18779,#18780,#14806,.T.);
#23473=EDGE_CURVE('',#18779,#18775,#1597,.T.);
#23474=EDGE_CURVE('',#18774,#18780,#10164,.T.);
#23475=EDGE_CURVE('',#18781,#18782,#14807,.T.);
#23476=EDGE_CURVE('',#18782,#18779,#14808,.T.);
#23477=EDGE_CURVE('',#18780,#18781,#14809,.T.);
#23478=EDGE_CURVE('',#18783,#18784,#14810,.T.);
#23479=EDGE_CURVE('',#18784,#18719,#14811,.T.);
#23480=EDGE_CURVE('',#18719,#18785,#10165,.T.);
#23481=EDGE_CURVE('',#18786,#18785,#14812,.T.);
#23482=EDGE_CURVE('',#18786,#18787,#14813,.T.);
#23483=EDGE_CURVE('',#18787,#18783,#10166,.T.);
#23484=EDGE_CURVE('',#18785,#18782,#10167,.T.);
#23485=EDGE_CURVE('',#18781,#18786,#1598,.T.);
#23486=EDGE_CURVE('',#18788,#18789,#14814,.T.);
#23487=EDGE_CURVE('',#18788,#18784,#1599,.T.);
#23488=EDGE_CURVE('',#18783,#18789,#10168,.T.);
#23489=EDGE_CURVE('',#18790,#18791,#14815,.T.);
#23490=EDGE_CURVE('',#18791,#18788,#14816,.T.);
#23491=EDGE_CURVE('',#18789,#18790,#14817,.T.);
#23492=EDGE_CURVE('',#18792,#18793,#14818,.T.);
#23493=EDGE_CURVE('',#18793,#18728,#14819,.T.);
#23494=EDGE_CURVE('',#18728,#18794,#10169,.T.);
#23495=EDGE_CURVE('',#18795,#18794,#14820,.T.);
#23496=EDGE_CURVE('',#18795,#18796,#14821,.T.);
#23497=EDGE_CURVE('',#18796,#18792,#10170,.F.);
#23498=EDGE_CURVE('',#18794,#18791,#10171,.T.);
#23499=EDGE_CURVE('',#18790,#18795,#1600,.T.);
#23500=EDGE_CURVE('',#17672,#18793,#14822,.T.);
#23501=EDGE_CURVE('',#18792,#17673,#10172,.F.);
#23502=EDGE_CURVE('',#17669,#18737,#969,.T.);
#23503=EDGE_CURVE('',#18737,#18797,#10173,.T.);
#23504=EDGE_CURVE('',#17670,#18797,#970,.T.);
#23505=EDGE_CURVE('',#18797,#17671,#971,.T.);
#23506=EDGE_CURVE('',#18798,#18799,#14823,.T.);
#23507=EDGE_CURVE('',#18799,#17353,#14824,.T.);
#23508=EDGE_CURVE('',#18800,#17352,#1601,.T.);
#23509=EDGE_CURVE('',#18800,#18801,#972,.T.);
#23510=EDGE_CURVE('',#18801,#18798,#10174,.T.);
#23511=EDGE_CURVE('',#18802,#18803,#14825,.T.);
#23512=EDGE_CURVE('',#18802,#18799,#1602,.T.);
#23513=EDGE_CURVE('',#18798,#18803,#10175,.T.);
#23514=EDGE_CURVE('',#18804,#18805,#14826,.T.);
#23515=EDGE_CURVE('',#18805,#18802,#14827,.T.);
#23516=EDGE_CURVE('',#18803,#18804,#14828,.T.);
#23517=EDGE_CURVE('',#18806,#18807,#14829,.T.);
#23518=EDGE_CURVE('',#18807,#18742,#14830,.T.);
#23519=EDGE_CURVE('',#18742,#18808,#10176,.T.);
#23520=EDGE_CURVE('',#18809,#18808,#14831,.T.);
#23521=EDGE_CURVE('',#18809,#18810,#14832,.T.);
#23522=EDGE_CURVE('',#18810,#18806,#10177,.T.);
#23523=EDGE_CURVE('',#18808,#18805,#10178,.T.);
#23524=EDGE_CURVE('',#18804,#18809,#1603,.T.);
#23525=EDGE_CURVE('',#17355,#18741,#973,.T.);
#23526=EDGE_CURVE('',#18811,#18812,#14833,.T.);
#23527=EDGE_CURVE('',#18811,#18807,#1604,.T.);
#23528=EDGE_CURVE('',#18806,#18812,#10179,.T.);
#23529=EDGE_CURVE('',#18813,#18814,#14834,.T.);
#23530=EDGE_CURVE('',#18814,#18811,#14835,.T.);
#23531=EDGE_CURVE('',#18812,#18813,#14836,.T.);
#23532=EDGE_CURVE('',#18815,#18816,#14837,.T.);
#23533=EDGE_CURVE('',#18816,#18751,#14838,.T.);
#23534=EDGE_CURVE('',#18751,#18817,#10180,.T.);
#23535=EDGE_CURVE('',#18818,#18817,#14839,.T.);
#23536=EDGE_CURVE('',#18818,#18819,#14840,.T.);
#23537=EDGE_CURVE('',#18819,#18815,#10181,.T.);
#23538=EDGE_CURVE('',#18817,#18814,#10182,.T.);
#23539=EDGE_CURVE('',#18813,#18818,#1605,.T.);
#23540=EDGE_CURVE('',#18820,#18821,#14841,.T.);
#23541=EDGE_CURVE('',#18820,#18816,#1606,.T.);
#23542=EDGE_CURVE('',#18815,#18821,#10183,.T.);
#23543=EDGE_CURVE('',#18822,#18823,#14842,.T.);
#23544=EDGE_CURVE('',#18823,#18820,#14843,.T.);
#23545=EDGE_CURVE('',#18821,#18822,#14844,.T.);
#23546=EDGE_CURVE('',#18824,#18825,#1607,.T.);
#23547=EDGE_CURVE('',#18825,#18760,#1608,.T.);
#23548=EDGE_CURVE('',#18760,#18826,#10184,.T.);
#23549=EDGE_CURVE('',#18827,#18826,#14845,.T.);
#23550=EDGE_CURVE('',#18827,#18828,#14846,.T.);
#23551=EDGE_CURVE('',#18828,#18824,#10185,.T.);
#23552=EDGE_CURVE('',#18826,#18823,#10186,.T.);
#23553=EDGE_CURVE('',#18822,#18827,#1609,.T.);
#23554=EDGE_CURVE('',#18829,#18830,#1610,.T.);
#23555=EDGE_CURVE('',#18829,#18825,#1611,.T.);
#23556=EDGE_CURVE('',#18824,#18830,#10187,.T.);
#23557=EDGE_CURVE('',#18831,#18832,#14847,.T.);
#23558=EDGE_CURVE('',#18832,#18829,#1612,.T.);
#23559=EDGE_CURVE('',#18830,#18831,#14848,.T.);
#23560=EDGE_CURVE('',#18833,#18834,#14849,.T.);
#23561=EDGE_CURVE('',#18834,#18769,#14850,.T.);
#23562=EDGE_CURVE('',#18769,#18835,#10188,.T.);
#23563=EDGE_CURVE('',#18836,#18835,#14851,.T.);
#23564=EDGE_CURVE('',#18836,#18837,#14852,.T.);
#23565=EDGE_CURVE('',#18837,#18833,#10189,.T.);
#23566=EDGE_CURVE('',#18835,#18832,#10190,.T.);
#23567=EDGE_CURVE('',#18831,#18836,#1613,.T.);
#23568=EDGE_CURVE('',#18838,#18839,#14853,.T.);
#23569=EDGE_CURVE('',#18838,#18834,#1614,.T.);
#23570=EDGE_CURVE('',#18833,#18839,#10191,.T.);
#23571=EDGE_CURVE('',#18840,#18841,#14854,.T.);
#23572=EDGE_CURVE('',#18841,#18838,#14855,.T.);
#23573=EDGE_CURVE('',#18839,#18840,#14856,.T.);
#23574=EDGE_CURVE('',#18842,#18843,#14857,.T.);
#23575=EDGE_CURVE('',#18843,#18778,#14858,.T.);
#23576=EDGE_CURVE('',#18778,#18844,#10192,.T.);
#23577=EDGE_CURVE('',#18845,#18844,#14859,.T.);
#23578=EDGE_CURVE('',#18845,#18846,#14860,.T.);
#23579=EDGE_CURVE('',#18846,#18842,#10193,.T.);
#23580=EDGE_CURVE('',#18844,#18841,#10194,.T.);
#23581=EDGE_CURVE('',#18840,#18845,#1615,.T.);
#23582=EDGE_CURVE('',#18847,#18848,#14861,.T.);
#23583=EDGE_CURVE('',#18847,#18843,#1616,.T.);
#23584=EDGE_CURVE('',#18842,#18848,#10195,.T.);
#23585=EDGE_CURVE('',#18849,#18850,#14862,.T.);
#23586=EDGE_CURVE('',#18850,#18847,#14863,.T.);
#23587=EDGE_CURVE('',#18848,#18849,#14864,.T.);
#23588=EDGE_CURVE('',#18851,#18852,#14865,.T.);
#23589=EDGE_CURVE('',#18852,#18787,#14866,.T.);
#23590=EDGE_CURVE('',#18787,#18853,#10196,.T.);
#23591=EDGE_CURVE('',#18854,#18853,#14867,.T.);
#23592=EDGE_CURVE('',#18854,#18855,#14868,.T.);
#23593=EDGE_CURVE('',#18855,#18851,#10197,.F.);
#23594=EDGE_CURVE('',#18853,#18850,#10198,.T.);
#23595=EDGE_CURVE('',#18849,#18854,#1617,.T.);
#23596=EDGE_CURVE('',#17678,#18852,#14869,.T.);
#23597=EDGE_CURVE('',#18851,#17679,#10199,.F.);
#23598=EDGE_CURVE('',#17675,#18796,#974,.T.);
#23599=EDGE_CURVE('',#18796,#18856,#10200,.T.);
#23600=EDGE_CURVE('',#17676,#18856,#975,.T.);
#23601=EDGE_CURVE('',#18856,#17677,#976,.T.);
#23602=EDGE_CURVE('',#18857,#18858,#14870,.T.);
#23603=EDGE_CURVE('',#18858,#17349,#14871,.T.);
#23604=EDGE_CURVE('',#18859,#17348,#1618,.T.);
#23605=EDGE_CURVE('',#18859,#18860,#977,.T.);
#23606=EDGE_CURVE('',#18860,#18857,#10201,.T.);
#23607=EDGE_CURVE('',#18861,#18862,#14872,.T.);
#23608=EDGE_CURVE('',#18861,#18858,#1619,.T.);
#23609=EDGE_CURVE('',#18857,#18862,#10202,.T.);
#23610=EDGE_CURVE('',#18863,#18864,#14873,.T.);
#23611=EDGE_CURVE('',#18864,#18861,#14874,.T.);
#23612=EDGE_CURVE('',#18862,#18863,#14875,.T.);
#23613=EDGE_CURVE('',#18865,#18866,#14876,.T.);
#23614=EDGE_CURVE('',#18866,#18801,#14877,.T.);
#23615=EDGE_CURVE('',#18801,#18867,#10203,.T.);
#23616=EDGE_CURVE('',#18868,#18867,#14878,.T.);
#23617=EDGE_CURVE('',#18868,#18869,#14879,.T.);
#23618=EDGE_CURVE('',#18869,#18865,#10204,.T.);
#23619=EDGE_CURVE('',#18867,#18864,#10205,.T.);
#23620=EDGE_CURVE('',#18863,#18868,#1620,.T.);
#23621=EDGE_CURVE('',#17351,#18800,#978,.T.);
#23622=EDGE_CURVE('',#18870,#18871,#14880,.T.);
#23623=EDGE_CURVE('',#18870,#18866,#1621,.T.);
#23624=EDGE_CURVE('',#18865,#18871,#10206,.T.);
#23625=EDGE_CURVE('',#18872,#18873,#14881,.T.);
#23626=EDGE_CURVE('',#18873,#18870,#14882,.T.);
#23627=EDGE_CURVE('',#18871,#18872,#14883,.T.);
#23628=EDGE_CURVE('',#18874,#18875,#14884,.T.);
#23629=EDGE_CURVE('',#18875,#18810,#14885,.T.);
#23630=EDGE_CURVE('',#18810,#18876,#10207,.T.);
#23631=EDGE_CURVE('',#18877,#18876,#14886,.T.);
#23632=EDGE_CURVE('',#18877,#18878,#14887,.T.);
#23633=EDGE_CURVE('',#18878,#18874,#10208,.T.);
#23634=EDGE_CURVE('',#18876,#18873,#10209,.T.);
#23635=EDGE_CURVE('',#18872,#18877,#1622,.T.);
#23636=EDGE_CURVE('',#18879,#18880,#14888,.T.);
#23637=EDGE_CURVE('',#18879,#18875,#1623,.T.);
#23638=EDGE_CURVE('',#18874,#18880,#10210,.T.);
#23639=EDGE_CURVE('',#18881,#18882,#14889,.T.);
#23640=EDGE_CURVE('',#18882,#18879,#14890,.T.);
#23641=EDGE_CURVE('',#18880,#18881,#14891,.T.);
#23642=EDGE_CURVE('',#18883,#18884,#1624,.T.);
#23643=EDGE_CURVE('',#18884,#18819,#1625,.T.);
#23644=EDGE_CURVE('',#18819,#18885,#10211,.T.);
#23645=EDGE_CURVE('',#18886,#18885,#14892,.T.);
#23646=EDGE_CURVE('',#18886,#18887,#14893,.T.);
#23647=EDGE_CURVE('',#18887,#18883,#10212,.T.);
#23648=EDGE_CURVE('',#18885,#18882,#10213,.T.);
#23649=EDGE_CURVE('',#18881,#18886,#1626,.T.);
#23650=EDGE_CURVE('',#18888,#18889,#1627,.T.);
#23651=EDGE_CURVE('',#18888,#18884,#1628,.T.);
#23652=EDGE_CURVE('',#18883,#18889,#10214,.T.);
#23653=EDGE_CURVE('',#18890,#18891,#14894,.T.);
#23654=EDGE_CURVE('',#18891,#18888,#1629,.T.);
#23655=EDGE_CURVE('',#18889,#18890,#14895,.T.);
#23656=EDGE_CURVE('',#18892,#18893,#14896,.T.);
#23657=EDGE_CURVE('',#18893,#18828,#14897,.T.);
#23658=EDGE_CURVE('',#18828,#18894,#10215,.T.);
#23659=EDGE_CURVE('',#18895,#18894,#14898,.T.);
#23660=EDGE_CURVE('',#18895,#18896,#14899,.T.);
#23661=EDGE_CURVE('',#18896,#18892,#10216,.T.);
#23662=EDGE_CURVE('',#18894,#18891,#10217,.T.);
#23663=EDGE_CURVE('',#18890,#18895,#1630,.T.);
#23664=EDGE_CURVE('',#18897,#18898,#14900,.T.);
#23665=EDGE_CURVE('',#18897,#18893,#1631,.T.);
#23666=EDGE_CURVE('',#18892,#18898,#10218,.T.);
#23667=EDGE_CURVE('',#18899,#18900,#14901,.T.);
#23668=EDGE_CURVE('',#18900,#18897,#14902,.T.);
#23669=EDGE_CURVE('',#18898,#18899,#14903,.T.);
#23670=EDGE_CURVE('',#18901,#18902,#14904,.T.);
#23671=EDGE_CURVE('',#18902,#18837,#14905,.T.);
#23672=EDGE_CURVE('',#18837,#18903,#10219,.T.);
#23673=EDGE_CURVE('',#18904,#18903,#14906,.T.);
#23674=EDGE_CURVE('',#18904,#18905,#14907,.T.);
#23675=EDGE_CURVE('',#18905,#18901,#10220,.T.);
#23676=EDGE_CURVE('',#18903,#18900,#10221,.T.);
#23677=EDGE_CURVE('',#18899,#18904,#1632,.T.);
#23678=EDGE_CURVE('',#18906,#18907,#14908,.T.);
#23679=EDGE_CURVE('',#18906,#18902,#1633,.T.);
#23680=EDGE_CURVE('',#18901,#18907,#10222,.T.);
#23681=EDGE_CURVE('',#18908,#18909,#14909,.T.);
#23682=EDGE_CURVE('',#18909,#18906,#14910,.T.);
#23683=EDGE_CURVE('',#18907,#18908,#14911,.T.);
#23684=EDGE_CURVE('',#18910,#18911,#14912,.T.);
#23685=EDGE_CURVE('',#18911,#18846,#14913,.T.);
#23686=EDGE_CURVE('',#18846,#18912,#10223,.T.);
#23687=EDGE_CURVE('',#18913,#18912,#14914,.T.);
#23688=EDGE_CURVE('',#18913,#18914,#14915,.T.);
#23689=EDGE_CURVE('',#18914,#18910,#10224,.F.);
#23690=EDGE_CURVE('',#18912,#18909,#10225,.T.);
#23691=EDGE_CURVE('',#18908,#18913,#1634,.T.);
#23692=EDGE_CURVE('',#17684,#18911,#14916,.T.);
#23693=EDGE_CURVE('',#18910,#17685,#10226,.F.);
#23694=EDGE_CURVE('',#17681,#18855,#979,.T.);
#23695=EDGE_CURVE('',#18855,#18915,#10227,.T.);
#23696=EDGE_CURVE('',#17682,#18915,#980,.T.);
#23697=EDGE_CURVE('',#18915,#17683,#981,.T.);
#23698=EDGE_CURVE('',#18916,#18917,#14917,.T.);
#23699=EDGE_CURVE('',#18917,#17345,#14918,.T.);
#23700=EDGE_CURVE('',#18918,#17344,#1635,.T.);
#23701=EDGE_CURVE('',#18918,#18919,#982,.T.);
#23702=EDGE_CURVE('',#18919,#18916,#10228,.T.);
#23703=EDGE_CURVE('',#18920,#18921,#14919,.T.);
#23704=EDGE_CURVE('',#18920,#18917,#1636,.T.);
#23705=EDGE_CURVE('',#18916,#18921,#10229,.T.);
#23706=EDGE_CURVE('',#18922,#18923,#14920,.T.);
#23707=EDGE_CURVE('',#18923,#18920,#14921,.T.);
#23708=EDGE_CURVE('',#18921,#18922,#14922,.T.);
#23709=EDGE_CURVE('',#18924,#18925,#14923,.T.);
#23710=EDGE_CURVE('',#18925,#18860,#14924,.T.);
#23711=EDGE_CURVE('',#18860,#18926,#10230,.T.);
#23712=EDGE_CURVE('',#18927,#18926,#14925,.T.);
#23713=EDGE_CURVE('',#18927,#18928,#14926,.T.);
#23714=EDGE_CURVE('',#18928,#18924,#10231,.T.);
#23715=EDGE_CURVE('',#18926,#18923,#10232,.T.);
#23716=EDGE_CURVE('',#18922,#18927,#1637,.T.);
#23717=EDGE_CURVE('',#17347,#18859,#983,.T.);
#23718=EDGE_CURVE('',#18929,#18930,#14927,.T.);
#23719=EDGE_CURVE('',#18929,#18925,#1638,.T.);
#23720=EDGE_CURVE('',#18924,#18930,#10233,.T.);
#23721=EDGE_CURVE('',#18931,#18932,#14928,.T.);
#23722=EDGE_CURVE('',#18932,#18929,#14929,.T.);
#23723=EDGE_CURVE('',#18930,#18931,#14930,.T.);
#23724=EDGE_CURVE('',#18933,#18934,#14931,.T.);
#23725=EDGE_CURVE('',#18934,#18869,#14932,.T.);
#23726=EDGE_CURVE('',#18869,#18935,#10234,.T.);
#23727=EDGE_CURVE('',#18936,#18935,#14933,.T.);
#23728=EDGE_CURVE('',#18936,#18937,#14934,.T.);
#23729=EDGE_CURVE('',#18937,#18933,#10235,.T.);
#23730=EDGE_CURVE('',#18935,#18932,#10236,.T.);
#23731=EDGE_CURVE('',#18931,#18936,#1639,.T.);
#23732=EDGE_CURVE('',#18938,#18939,#14935,.T.);
#23733=EDGE_CURVE('',#18938,#18934,#1640,.T.);
#23734=EDGE_CURVE('',#18933,#18939,#10237,.T.);
#23735=EDGE_CURVE('',#18940,#18941,#14936,.T.);
#23736=EDGE_CURVE('',#18941,#18938,#14937,.T.);
#23737=EDGE_CURVE('',#18939,#18940,#14938,.T.);
#23738=EDGE_CURVE('',#18942,#18943,#1641,.T.);
#23739=EDGE_CURVE('',#18943,#18878,#1642,.T.);
#23740=EDGE_CURVE('',#18878,#18944,#10238,.T.);
#23741=EDGE_CURVE('',#18945,#18944,#14939,.T.);
#23742=EDGE_CURVE('',#18945,#18946,#14940,.T.);
#23743=EDGE_CURVE('',#18946,#18942,#10239,.T.);
#23744=EDGE_CURVE('',#18944,#18941,#10240,.T.);
#23745=EDGE_CURVE('',#18940,#18945,#1643,.T.);
#23746=EDGE_CURVE('',#18947,#18948,#1644,.T.);
#23747=EDGE_CURVE('',#18947,#18943,#1645,.T.);
#23748=EDGE_CURVE('',#18942,#18948,#10241,.T.);
#23749=EDGE_CURVE('',#18949,#18950,#14941,.T.);
#23750=EDGE_CURVE('',#18950,#18947,#1646,.T.);
#23751=EDGE_CURVE('',#18948,#18949,#14942,.T.);
#23752=EDGE_CURVE('',#18951,#18952,#14943,.T.);
#23753=EDGE_CURVE('',#18952,#18887,#14944,.T.);
#23754=EDGE_CURVE('',#18887,#18953,#10242,.T.);
#23755=EDGE_CURVE('',#18954,#18953,#14945,.T.);
#23756=EDGE_CURVE('',#18954,#18955,#14946,.T.);
#23757=EDGE_CURVE('',#18955,#18951,#10243,.T.);
#23758=EDGE_CURVE('',#18953,#18950,#10244,.T.);
#23759=EDGE_CURVE('',#18949,#18954,#1647,.T.);
#23760=EDGE_CURVE('',#18956,#18957,#14947,.T.);
#23761=EDGE_CURVE('',#18956,#18952,#1648,.T.);
#23762=EDGE_CURVE('',#18951,#18957,#10245,.T.);
#23763=EDGE_CURVE('',#18958,#18959,#14948,.T.);
#23764=EDGE_CURVE('',#18959,#18956,#14949,.T.);
#23765=EDGE_CURVE('',#18957,#18958,#14950,.T.);
#23766=EDGE_CURVE('',#18960,#18961,#14951,.T.);
#23767=EDGE_CURVE('',#18961,#18896,#14952,.T.);
#23768=EDGE_CURVE('',#18896,#18962,#10246,.T.);
#23769=EDGE_CURVE('',#18963,#18962,#14953,.T.);
#23770=EDGE_CURVE('',#18963,#18964,#14954,.T.);
#23771=EDGE_CURVE('',#18964,#18960,#10247,.T.);
#23772=EDGE_CURVE('',#18962,#18959,#10248,.T.);
#23773=EDGE_CURVE('',#18958,#18963,#1649,.T.);
#23774=EDGE_CURVE('',#18965,#18966,#14955,.T.);
#23775=EDGE_CURVE('',#18965,#18961,#1650,.T.);
#23776=EDGE_CURVE('',#18960,#18966,#10249,.T.);
#23777=EDGE_CURVE('',#18967,#18968,#14956,.T.);
#23778=EDGE_CURVE('',#18968,#18965,#14957,.T.);
#23779=EDGE_CURVE('',#18966,#18967,#14958,.T.);
#23780=EDGE_CURVE('',#18969,#18970,#14959,.T.);
#23781=EDGE_CURVE('',#18970,#18905,#14960,.T.);
#23782=EDGE_CURVE('',#18905,#18971,#10250,.T.);
#23783=EDGE_CURVE('',#18972,#18971,#14961,.T.);
#23784=EDGE_CURVE('',#18972,#18973,#14962,.T.);
#23785=EDGE_CURVE('',#18973,#18969,#10251,.F.);
#23786=EDGE_CURVE('',#18971,#18968,#10252,.T.);
#23787=EDGE_CURVE('',#18967,#18972,#1651,.T.);
#23788=EDGE_CURVE('',#17690,#18970,#14963,.T.);
#23789=EDGE_CURVE('',#18969,#17691,#10253,.F.);
#23790=EDGE_CURVE('',#17687,#18914,#984,.T.);
#23791=EDGE_CURVE('',#18914,#18974,#10254,.T.);
#23792=EDGE_CURVE('',#17688,#18974,#985,.T.);
#23793=EDGE_CURVE('',#18974,#17689,#986,.T.);
#23794=EDGE_CURVE('',#18975,#18976,#14964,.T.);
#23795=EDGE_CURVE('',#18976,#17341,#14965,.T.);
#23796=EDGE_CURVE('',#18977,#17340,#1652,.T.);
#23797=EDGE_CURVE('',#18977,#18978,#987,.T.);
#23798=EDGE_CURVE('',#18978,#18975,#10255,.T.);
#23799=EDGE_CURVE('',#18979,#18980,#14966,.T.);
#23800=EDGE_CURVE('',#18979,#18976,#1653,.T.);
#23801=EDGE_CURVE('',#18975,#18980,#10256,.T.);
#23802=EDGE_CURVE('',#18981,#18982,#14967,.T.);
#23803=EDGE_CURVE('',#18982,#18979,#14968,.T.);
#23804=EDGE_CURVE('',#18980,#18981,#14969,.T.);
#23805=EDGE_CURVE('',#18983,#18984,#14970,.T.);
#23806=EDGE_CURVE('',#18984,#18919,#14971,.T.);
#23807=EDGE_CURVE('',#18919,#18985,#10257,.T.);
#23808=EDGE_CURVE('',#18986,#18985,#14972,.T.);
#23809=EDGE_CURVE('',#18986,#18987,#14973,.T.);
#23810=EDGE_CURVE('',#18987,#18983,#10258,.T.);
#23811=EDGE_CURVE('',#18985,#18982,#10259,.T.);
#23812=EDGE_CURVE('',#18981,#18986,#1654,.T.);
#23813=EDGE_CURVE('',#17343,#18918,#988,.T.);
#23814=EDGE_CURVE('',#18988,#18989,#14974,.T.);
#23815=EDGE_CURVE('',#18988,#18984,#1655,.T.);
#23816=EDGE_CURVE('',#18983,#18989,#10260,.T.);
#23817=EDGE_CURVE('',#18990,#18991,#14975,.T.);
#23818=EDGE_CURVE('',#18991,#18988,#14976,.T.);
#23819=EDGE_CURVE('',#18989,#18990,#14977,.T.);
#23820=EDGE_CURVE('',#18992,#18993,#14978,.T.);
#23821=EDGE_CURVE('',#18993,#18928,#14979,.T.);
#23822=EDGE_CURVE('',#18928,#18994,#10261,.T.);
#23823=EDGE_CURVE('',#18995,#18994,#14980,.T.);
#23824=EDGE_CURVE('',#18995,#18996,#14981,.T.);
#23825=EDGE_CURVE('',#18996,#18992,#10262,.T.);
#23826=EDGE_CURVE('',#18994,#18991,#10263,.T.);
#23827=EDGE_CURVE('',#18990,#18995,#1656,.T.);
#23828=EDGE_CURVE('',#18997,#18998,#14982,.T.);
#23829=EDGE_CURVE('',#18997,#18993,#1657,.T.);
#23830=EDGE_CURVE('',#18992,#18998,#10264,.T.);
#23831=EDGE_CURVE('',#18999,#19000,#14983,.T.);
#23832=EDGE_CURVE('',#19000,#18997,#14984,.T.);
#23833=EDGE_CURVE('',#18998,#18999,#14985,.T.);
#23834=EDGE_CURVE('',#19001,#19002,#1658,.T.);
#23835=EDGE_CURVE('',#19002,#18937,#1659,.T.);
#23836=EDGE_CURVE('',#18937,#19003,#10265,.T.);
#23837=EDGE_CURVE('',#19004,#19003,#14986,.T.);
#23838=EDGE_CURVE('',#19004,#19005,#14987,.T.);
#23839=EDGE_CURVE('',#19005,#19001,#10266,.T.);
#23840=EDGE_CURVE('',#19003,#19000,#10267,.T.);
#23841=EDGE_CURVE('',#18999,#19004,#1660,.T.);
#23842=EDGE_CURVE('',#19006,#19007,#1661,.T.);
#23843=EDGE_CURVE('',#19006,#19002,#1662,.T.);
#23844=EDGE_CURVE('',#19001,#19007,#10268,.T.);
#23845=EDGE_CURVE('',#19008,#19009,#14988,.T.);
#23846=EDGE_CURVE('',#19009,#19006,#1663,.T.);
#23847=EDGE_CURVE('',#19007,#19008,#14989,.T.);
#23848=EDGE_CURVE('',#19010,#19011,#14990,.T.);
#23849=EDGE_CURVE('',#19011,#18946,#14991,.T.);
#23850=EDGE_CURVE('',#18946,#19012,#10269,.T.);
#23851=EDGE_CURVE('',#19013,#19012,#14992,.T.);
#23852=EDGE_CURVE('',#19013,#19014,#14993,.T.);
#23853=EDGE_CURVE('',#19014,#19010,#10270,.T.);
#23854=EDGE_CURVE('',#19012,#19009,#10271,.T.);
#23855=EDGE_CURVE('',#19008,#19013,#1664,.T.);
#23856=EDGE_CURVE('',#19015,#19016,#14994,.T.);
#23857=EDGE_CURVE('',#19015,#19011,#1665,.T.);
#23858=EDGE_CURVE('',#19010,#19016,#10272,.T.);
#23859=EDGE_CURVE('',#19017,#19018,#14995,.T.);
#23860=EDGE_CURVE('',#19018,#19015,#14996,.T.);
#23861=EDGE_CURVE('',#19016,#19017,#14997,.T.);
#23862=EDGE_CURVE('',#19019,#19020,#14998,.T.);
#23863=EDGE_CURVE('',#19020,#18955,#14999,.T.);
#23864=EDGE_CURVE('',#18955,#19021,#10273,.T.);
#23865=EDGE_CURVE('',#19022,#19021,#15000,.T.);
#23866=EDGE_CURVE('',#19022,#19023,#15001,.T.);
#23867=EDGE_CURVE('',#19023,#19019,#10274,.T.);
#23868=EDGE_CURVE('',#19021,#19018,#10275,.T.);
#23869=EDGE_CURVE('',#19017,#19022,#1666,.T.);
#23870=EDGE_CURVE('',#19024,#19025,#15002,.T.);
#23871=EDGE_CURVE('',#19024,#19020,#1667,.T.);
#23872=EDGE_CURVE('',#19019,#19025,#10276,.T.);
#23873=EDGE_CURVE('',#19026,#19027,#15003,.T.);
#23874=EDGE_CURVE('',#19027,#19024,#15004,.T.);
#23875=EDGE_CURVE('',#19025,#19026,#15005,.T.);
#23876=EDGE_CURVE('',#19028,#19029,#15006,.T.);
#23877=EDGE_CURVE('',#19029,#18964,#15007,.T.);
#23878=EDGE_CURVE('',#18964,#19030,#10277,.T.);
#23879=EDGE_CURVE('',#19031,#19030,#15008,.T.);
#23880=EDGE_CURVE('',#19031,#19032,#15009,.T.);
#23881=EDGE_CURVE('',#19032,#19028,#10278,.F.);
#23882=EDGE_CURVE('',#19030,#19027,#10279,.T.);
#23883=EDGE_CURVE('',#19026,#19031,#1668,.T.);
#23884=EDGE_CURVE('',#17696,#19029,#15010,.T.);
#23885=EDGE_CURVE('',#19028,#17697,#10280,.F.);
#23886=EDGE_CURVE('',#17693,#18973,#989,.T.);
#23887=EDGE_CURVE('',#18973,#19033,#10281,.T.);
#23888=EDGE_CURVE('',#17694,#19033,#990,.T.);
#23889=EDGE_CURVE('',#19033,#17695,#991,.T.);
#23890=EDGE_CURVE('',#19034,#19035,#15011,.T.);
#23891=EDGE_CURVE('',#19035,#17337,#15012,.T.);
#23892=EDGE_CURVE('',#19036,#17336,#1669,.T.);
#23893=EDGE_CURVE('',#19036,#19037,#992,.T.);
#23894=EDGE_CURVE('',#19037,#19034,#10282,.T.);
#23895=EDGE_CURVE('',#19038,#19039,#15013,.T.);
#23896=EDGE_CURVE('',#19038,#19035,#1670,.T.);
#23897=EDGE_CURVE('',#19034,#19039,#10283,.T.);
#23898=EDGE_CURVE('',#19040,#19041,#15014,.T.);
#23899=EDGE_CURVE('',#19041,#19038,#15015,.T.);
#23900=EDGE_CURVE('',#19039,#19040,#15016,.T.);
#23901=EDGE_CURVE('',#19042,#19043,#15017,.T.);
#23902=EDGE_CURVE('',#19043,#18978,#15018,.T.);
#23903=EDGE_CURVE('',#18978,#19044,#10284,.T.);
#23904=EDGE_CURVE('',#19045,#19044,#15019,.T.);
#23905=EDGE_CURVE('',#19045,#19046,#15020,.T.);
#23906=EDGE_CURVE('',#19046,#19042,#10285,.T.);
#23907=EDGE_CURVE('',#19044,#19041,#10286,.T.);
#23908=EDGE_CURVE('',#19040,#19045,#1671,.T.);
#23909=EDGE_CURVE('',#17339,#18977,#993,.T.);
#23910=EDGE_CURVE('',#19047,#19048,#15021,.T.);
#23911=EDGE_CURVE('',#19047,#19043,#1672,.T.);
#23912=EDGE_CURVE('',#19042,#19048,#10287,.T.);
#23913=EDGE_CURVE('',#19049,#19050,#15022,.T.);
#23914=EDGE_CURVE('',#19050,#19047,#15023,.T.);
#23915=EDGE_CURVE('',#19048,#19049,#15024,.T.);
#23916=EDGE_CURVE('',#19051,#19052,#15025,.T.);
#23917=EDGE_CURVE('',#19052,#18987,#15026,.T.);
#23918=EDGE_CURVE('',#18987,#19053,#10288,.T.);
#23919=EDGE_CURVE('',#19054,#19053,#15027,.T.);
#23920=EDGE_CURVE('',#19054,#19055,#15028,.T.);
#23921=EDGE_CURVE('',#19055,#19051,#10289,.T.);
#23922=EDGE_CURVE('',#19053,#19050,#10290,.T.);
#23923=EDGE_CURVE('',#19049,#19054,#1673,.T.);
#23924=EDGE_CURVE('',#19056,#19057,#15029,.T.);
#23925=EDGE_CURVE('',#19056,#19052,#1674,.T.);
#23926=EDGE_CURVE('',#19051,#19057,#10291,.T.);
#23927=EDGE_CURVE('',#19058,#19059,#15030,.T.);
#23928=EDGE_CURVE('',#19059,#19056,#15031,.T.);
#23929=EDGE_CURVE('',#19057,#19058,#15032,.T.);
#23930=EDGE_CURVE('',#19060,#19061,#1675,.T.);
#23931=EDGE_CURVE('',#19061,#18996,#1676,.T.);
#23932=EDGE_CURVE('',#18996,#19062,#10292,.T.);
#23933=EDGE_CURVE('',#19063,#19062,#15033,.T.);
#23934=EDGE_CURVE('',#19063,#19064,#15034,.T.);
#23935=EDGE_CURVE('',#19064,#19060,#10293,.T.);
#23936=EDGE_CURVE('',#19062,#19059,#10294,.T.);
#23937=EDGE_CURVE('',#19058,#19063,#1677,.T.);
#23938=EDGE_CURVE('',#19065,#19066,#1678,.T.);
#23939=EDGE_CURVE('',#19065,#19061,#1679,.T.);
#23940=EDGE_CURVE('',#19060,#19066,#10295,.T.);
#23941=EDGE_CURVE('',#19067,#19068,#15035,.T.);
#23942=EDGE_CURVE('',#19068,#19065,#1680,.T.);
#23943=EDGE_CURVE('',#19066,#19067,#15036,.T.);
#23944=EDGE_CURVE('',#19069,#19070,#15037,.T.);
#23945=EDGE_CURVE('',#19070,#19005,#15038,.T.);
#23946=EDGE_CURVE('',#19005,#19071,#10296,.T.);
#23947=EDGE_CURVE('',#19072,#19071,#15039,.T.);
#23948=EDGE_CURVE('',#19072,#19073,#15040,.T.);
#23949=EDGE_CURVE('',#19073,#19069,#10297,.T.);
#23950=EDGE_CURVE('',#19071,#19068,#10298,.T.);
#23951=EDGE_CURVE('',#19067,#19072,#1681,.T.);
#23952=EDGE_CURVE('',#19074,#19075,#15041,.T.);
#23953=EDGE_CURVE('',#19074,#19070,#1682,.T.);
#23954=EDGE_CURVE('',#19069,#19075,#10299,.T.);
#23955=EDGE_CURVE('',#19076,#19077,#15042,.T.);
#23956=EDGE_CURVE('',#19077,#19074,#15043,.T.);
#23957=EDGE_CURVE('',#19075,#19076,#15044,.T.);
#23958=EDGE_CURVE('',#19078,#19079,#15045,.T.);
#23959=EDGE_CURVE('',#19079,#19014,#15046,.T.);
#23960=EDGE_CURVE('',#19014,#19080,#10300,.T.);
#23961=EDGE_CURVE('',#19081,#19080,#15047,.T.);
#23962=EDGE_CURVE('',#19081,#19082,#15048,.T.);
#23963=EDGE_CURVE('',#19082,#19078,#10301,.T.);
#23964=EDGE_CURVE('',#19080,#19077,#10302,.T.);
#23965=EDGE_CURVE('',#19076,#19081,#1683,.T.);
#23966=EDGE_CURVE('',#19083,#19084,#15049,.T.);
#23967=EDGE_CURVE('',#19083,#19079,#1684,.T.);
#23968=EDGE_CURVE('',#19078,#19084,#10303,.T.);
#23969=EDGE_CURVE('',#19085,#19086,#15050,.T.);
#23970=EDGE_CURVE('',#19086,#19083,#15051,.T.);
#23971=EDGE_CURVE('',#19084,#19085,#15052,.T.);
#23972=EDGE_CURVE('',#19087,#19088,#15053,.T.);
#23973=EDGE_CURVE('',#19088,#19023,#15054,.T.);
#23974=EDGE_CURVE('',#19023,#19089,#10304,.T.);
#23975=EDGE_CURVE('',#19090,#19089,#15055,.T.);
#23976=EDGE_CURVE('',#19090,#19091,#15056,.T.);
#23977=EDGE_CURVE('',#19091,#19087,#10305,.F.);
#23978=EDGE_CURVE('',#19089,#19086,#10306,.T.);
#23979=EDGE_CURVE('',#19085,#19090,#1685,.T.);
#23980=EDGE_CURVE('',#17702,#19088,#15057,.T.);
#23981=EDGE_CURVE('',#19087,#17703,#10307,.F.);
#23982=EDGE_CURVE('',#17699,#19032,#994,.T.);
#23983=EDGE_CURVE('',#19032,#19092,#10308,.T.);
#23984=EDGE_CURVE('',#17700,#19092,#995,.T.);
#23985=EDGE_CURVE('',#19092,#17701,#996,.T.);
#23986=EDGE_CURVE('',#19093,#19094,#15058,.T.);
#23987=EDGE_CURVE('',#19094,#17333,#15059,.T.);
#23988=EDGE_CURVE('',#19095,#17332,#1686,.T.);
#23989=EDGE_CURVE('',#19095,#19096,#997,.T.);
#23990=EDGE_CURVE('',#19096,#19093,#10309,.T.);
#23991=EDGE_CURVE('',#19097,#19098,#15060,.T.);
#23992=EDGE_CURVE('',#19097,#19094,#1687,.T.);
#23993=EDGE_CURVE('',#19093,#19098,#10310,.T.);
#23994=EDGE_CURVE('',#19099,#19100,#15061,.T.);
#23995=EDGE_CURVE('',#19100,#19097,#15062,.T.);
#23996=EDGE_CURVE('',#19098,#19099,#15063,.T.);
#23997=EDGE_CURVE('',#19101,#19102,#15064,.T.);
#23998=EDGE_CURVE('',#19102,#19037,#15065,.T.);
#23999=EDGE_CURVE('',#19037,#19103,#10311,.T.);
#24000=EDGE_CURVE('',#19104,#19103,#15066,.T.);
#24001=EDGE_CURVE('',#19104,#19105,#15067,.T.);
#24002=EDGE_CURVE('',#19105,#19101,#10312,.T.);
#24003=EDGE_CURVE('',#19103,#19100,#10313,.T.);
#24004=EDGE_CURVE('',#19099,#19104,#1688,.T.);
#24005=EDGE_CURVE('',#17335,#19036,#998,.T.);
#24006=EDGE_CURVE('',#19106,#19107,#15068,.T.);
#24007=EDGE_CURVE('',#19106,#19102,#1689,.T.);
#24008=EDGE_CURVE('',#19101,#19107,#10314,.T.);
#24009=EDGE_CURVE('',#19108,#19109,#15069,.T.);
#24010=EDGE_CURVE('',#19109,#19106,#15070,.T.);
#24011=EDGE_CURVE('',#19107,#19108,#15071,.T.);
#24012=EDGE_CURVE('',#19110,#19111,#15072,.T.);
#24013=EDGE_CURVE('',#19111,#19046,#15073,.T.);
#24014=EDGE_CURVE('',#19046,#19112,#10315,.T.);
#24015=EDGE_CURVE('',#19113,#19112,#15074,.T.);
#24016=EDGE_CURVE('',#19113,#19114,#15075,.T.);
#24017=EDGE_CURVE('',#19114,#19110,#10316,.T.);
#24018=EDGE_CURVE('',#19112,#19109,#10317,.T.);
#24019=EDGE_CURVE('',#19108,#19113,#1690,.T.);
#24020=EDGE_CURVE('',#19115,#19116,#15076,.T.);
#24021=EDGE_CURVE('',#19115,#19111,#1691,.T.);
#24022=EDGE_CURVE('',#19110,#19116,#10318,.T.);
#24023=EDGE_CURVE('',#19117,#19118,#15077,.T.);
#24024=EDGE_CURVE('',#19118,#19115,#15078,.T.);
#24025=EDGE_CURVE('',#19116,#19117,#15079,.T.);
#24026=EDGE_CURVE('',#19119,#19120,#1692,.T.);
#24027=EDGE_CURVE('',#19120,#19055,#1693,.T.);
#24028=EDGE_CURVE('',#19055,#19121,#10319,.T.);
#24029=EDGE_CURVE('',#19122,#19121,#15080,.T.);
#24030=EDGE_CURVE('',#19122,#19123,#15081,.T.);
#24031=EDGE_CURVE('',#19123,#19119,#10320,.T.);
#24032=EDGE_CURVE('',#19121,#19118,#10321,.T.);
#24033=EDGE_CURVE('',#19117,#19122,#1694,.T.);
#24034=EDGE_CURVE('',#19124,#19125,#1695,.T.);
#24035=EDGE_CURVE('',#19124,#19120,#1696,.T.);
#24036=EDGE_CURVE('',#19119,#19125,#10322,.T.);
#24037=EDGE_CURVE('',#19126,#19127,#15082,.T.);
#24038=EDGE_CURVE('',#19127,#19124,#1697,.T.);
#24039=EDGE_CURVE('',#19125,#19126,#15083,.T.);
#24040=EDGE_CURVE('',#19128,#19129,#15084,.T.);
#24041=EDGE_CURVE('',#19129,#19064,#15085,.T.);
#24042=EDGE_CURVE('',#19064,#19130,#10323,.T.);
#24043=EDGE_CURVE('',#19131,#19130,#15086,.T.);
#24044=EDGE_CURVE('',#19131,#19132,#15087,.T.);
#24045=EDGE_CURVE('',#19132,#19128,#10324,.T.);
#24046=EDGE_CURVE('',#19130,#19127,#10325,.T.);
#24047=EDGE_CURVE('',#19126,#19131,#1698,.T.);
#24048=EDGE_CURVE('',#19133,#19134,#15088,.T.);
#24049=EDGE_CURVE('',#19133,#19129,#1699,.T.);
#24050=EDGE_CURVE('',#19128,#19134,#10326,.T.);
#24051=EDGE_CURVE('',#19135,#19136,#15089,.T.);
#24052=EDGE_CURVE('',#19136,#19133,#15090,.T.);
#24053=EDGE_CURVE('',#19134,#19135,#15091,.T.);
#24054=EDGE_CURVE('',#19137,#19138,#15092,.T.);
#24055=EDGE_CURVE('',#19138,#19073,#15093,.T.);
#24056=EDGE_CURVE('',#19073,#19139,#10327,.T.);
#24057=EDGE_CURVE('',#19140,#19139,#15094,.T.);
#24058=EDGE_CURVE('',#19140,#19141,#15095,.T.);
#24059=EDGE_CURVE('',#19141,#19137,#10328,.T.);
#24060=EDGE_CURVE('',#19139,#19136,#10329,.T.);
#24061=EDGE_CURVE('',#19135,#19140,#1700,.T.);
#24062=EDGE_CURVE('',#19142,#19143,#15096,.T.);
#24063=EDGE_CURVE('',#19142,#19138,#1701,.T.);
#24064=EDGE_CURVE('',#19137,#19143,#10330,.T.);
#24065=EDGE_CURVE('',#19144,#19145,#15097,.T.);
#24066=EDGE_CURVE('',#19145,#19142,#15098,.T.);
#24067=EDGE_CURVE('',#19143,#19144,#15099,.T.);
#24068=EDGE_CURVE('',#19146,#19147,#15100,.T.);
#24069=EDGE_CURVE('',#19147,#19082,#15101,.T.);
#24070=EDGE_CURVE('',#19082,#19148,#10331,.T.);
#24071=EDGE_CURVE('',#19149,#19148,#15102,.T.);
#24072=EDGE_CURVE('',#19149,#19150,#15103,.T.);
#24073=EDGE_CURVE('',#19150,#19146,#10332,.F.);
#24074=EDGE_CURVE('',#19148,#19145,#10333,.T.);
#24075=EDGE_CURVE('',#19144,#19149,#1702,.T.);
#24076=EDGE_CURVE('',#17708,#19147,#15104,.T.);
#24077=EDGE_CURVE('',#19146,#17709,#10334,.F.);
#24078=EDGE_CURVE('',#17705,#19091,#999,.T.);
#24079=EDGE_CURVE('',#19091,#19151,#10335,.T.);
#24080=EDGE_CURVE('',#17706,#19151,#1000,.T.);
#24081=EDGE_CURVE('',#19151,#17707,#1001,.T.);
#24082=EDGE_CURVE('',#19152,#19153,#15105,.T.);
#24083=EDGE_CURVE('',#19153,#17329,#15106,.T.);
#24084=EDGE_CURVE('',#19154,#17328,#1703,.T.);
#24085=EDGE_CURVE('',#19154,#19155,#1002,.T.);
#24086=EDGE_CURVE('',#19155,#19152,#10336,.T.);
#24087=EDGE_CURVE('',#19156,#19157,#15107,.T.);
#24088=EDGE_CURVE('',#19156,#19153,#1704,.T.);
#24089=EDGE_CURVE('',#19152,#19157,#10337,.T.);
#24090=EDGE_CURVE('',#19158,#19159,#15108,.T.);
#24091=EDGE_CURVE('',#19159,#19156,#15109,.T.);
#24092=EDGE_CURVE('',#19157,#19158,#15110,.T.);
#24093=EDGE_CURVE('',#19160,#19161,#15111,.T.);
#24094=EDGE_CURVE('',#19161,#19096,#15112,.T.);
#24095=EDGE_CURVE('',#19096,#19162,#10338,.T.);
#24096=EDGE_CURVE('',#19163,#19162,#15113,.T.);
#24097=EDGE_CURVE('',#19163,#19164,#15114,.T.);
#24098=EDGE_CURVE('',#19164,#19160,#10339,.T.);
#24099=EDGE_CURVE('',#19162,#19159,#10340,.T.);
#24100=EDGE_CURVE('',#19158,#19163,#1705,.T.);
#24101=EDGE_CURVE('',#17331,#19095,#1003,.T.);
#24102=EDGE_CURVE('',#19165,#19166,#15115,.T.);
#24103=EDGE_CURVE('',#19165,#19161,#1706,.T.);
#24104=EDGE_CURVE('',#19160,#19166,#10341,.T.);
#24105=EDGE_CURVE('',#19167,#19168,#15116,.T.);
#24106=EDGE_CURVE('',#19168,#19165,#15117,.T.);
#24107=EDGE_CURVE('',#19166,#19167,#15118,.T.);
#24108=EDGE_CURVE('',#19169,#19170,#15119,.T.);
#24109=EDGE_CURVE('',#19170,#19105,#15120,.T.);
#24110=EDGE_CURVE('',#19105,#19171,#10342,.T.);
#24111=EDGE_CURVE('',#19172,#19171,#15121,.T.);
#24112=EDGE_CURVE('',#19172,#19173,#15122,.T.);
#24113=EDGE_CURVE('',#19173,#19169,#10343,.T.);
#24114=EDGE_CURVE('',#19171,#19168,#10344,.T.);
#24115=EDGE_CURVE('',#19167,#19172,#1707,.T.);
#24116=EDGE_CURVE('',#19174,#19175,#15123,.T.);
#24117=EDGE_CURVE('',#19174,#19170,#1708,.T.);
#24118=EDGE_CURVE('',#19169,#19175,#10345,.T.);
#24119=EDGE_CURVE('',#19176,#19177,#15124,.T.);
#24120=EDGE_CURVE('',#19177,#19174,#15125,.T.);
#24121=EDGE_CURVE('',#19175,#19176,#15126,.T.);
#24122=EDGE_CURVE('',#19178,#19179,#1709,.T.);
#24123=EDGE_CURVE('',#19179,#19114,#1710,.T.);
#24124=EDGE_CURVE('',#19114,#19180,#10346,.T.);
#24125=EDGE_CURVE('',#19181,#19180,#15127,.T.);
#24126=EDGE_CURVE('',#19181,#19182,#15128,.T.);
#24127=EDGE_CURVE('',#19182,#19178,#10347,.T.);
#24128=EDGE_CURVE('',#19180,#19177,#10348,.T.);
#24129=EDGE_CURVE('',#19176,#19181,#1711,.T.);
#24130=EDGE_CURVE('',#19183,#19184,#1712,.T.);
#24131=EDGE_CURVE('',#19183,#19179,#1713,.T.);
#24132=EDGE_CURVE('',#19178,#19184,#10349,.T.);
#24133=EDGE_CURVE('',#19185,#19186,#15129,.T.);
#24134=EDGE_CURVE('',#19186,#19183,#1714,.T.);
#24135=EDGE_CURVE('',#19184,#19185,#15130,.T.);
#24136=EDGE_CURVE('',#19187,#19188,#15131,.T.);
#24137=EDGE_CURVE('',#19188,#19123,#15132,.T.);
#24138=EDGE_CURVE('',#19123,#19189,#10350,.T.);
#24139=EDGE_CURVE('',#19190,#19189,#15133,.T.);
#24140=EDGE_CURVE('',#19190,#19191,#15134,.T.);
#24141=EDGE_CURVE('',#19191,#19187,#10351,.T.);
#24142=EDGE_CURVE('',#19189,#19186,#10352,.T.);
#24143=EDGE_CURVE('',#19185,#19190,#1715,.T.);
#24144=EDGE_CURVE('',#19192,#19193,#15135,.T.);
#24145=EDGE_CURVE('',#19192,#19188,#1716,.T.);
#24146=EDGE_CURVE('',#19187,#19193,#10353,.T.);
#24147=EDGE_CURVE('',#19194,#19195,#15136,.T.);
#24148=EDGE_CURVE('',#19195,#19192,#15137,.T.);
#24149=EDGE_CURVE('',#19193,#19194,#15138,.T.);
#24150=EDGE_CURVE('',#19196,#19197,#15139,.T.);
#24151=EDGE_CURVE('',#19197,#19132,#15140,.T.);
#24152=EDGE_CURVE('',#19132,#19198,#10354,.T.);
#24153=EDGE_CURVE('',#19199,#19198,#15141,.T.);
#24154=EDGE_CURVE('',#19199,#19200,#15142,.T.);
#24155=EDGE_CURVE('',#19200,#19196,#10355,.T.);
#24156=EDGE_CURVE('',#19198,#19195,#10356,.T.);
#24157=EDGE_CURVE('',#19194,#19199,#1717,.T.);
#24158=EDGE_CURVE('',#19201,#19202,#15143,.T.);
#24159=EDGE_CURVE('',#19201,#19197,#1718,.T.);
#24160=EDGE_CURVE('',#19196,#19202,#10357,.T.);
#24161=EDGE_CURVE('',#19203,#19204,#15144,.T.);
#24162=EDGE_CURVE('',#19204,#19201,#15145,.T.);
#24163=EDGE_CURVE('',#19202,#19203,#15146,.T.);
#24164=EDGE_CURVE('',#19205,#19206,#15147,.T.);
#24165=EDGE_CURVE('',#19206,#19141,#15148,.T.);
#24166=EDGE_CURVE('',#19141,#19207,#10358,.T.);
#24167=EDGE_CURVE('',#19208,#19207,#15149,.T.);
#24168=EDGE_CURVE('',#19208,#19209,#15150,.T.);
#24169=EDGE_CURVE('',#19209,#19205,#10359,.F.);
#24170=EDGE_CURVE('',#19207,#19204,#10360,.T.);
#24171=EDGE_CURVE('',#19203,#19208,#1719,.T.);
#24172=EDGE_CURVE('',#17714,#19206,#15151,.T.);
#24173=EDGE_CURVE('',#19205,#17715,#10361,.F.);
#24174=EDGE_CURVE('',#17711,#19150,#1004,.T.);
#24175=EDGE_CURVE('',#19150,#19210,#10362,.T.);
#24176=EDGE_CURVE('',#17712,#19210,#1005,.T.);
#24177=EDGE_CURVE('',#19210,#17713,#1006,.T.);
#24178=EDGE_CURVE('',#19211,#19212,#15152,.T.);
#24179=EDGE_CURVE('',#19212,#17325,#15153,.T.);
#24180=EDGE_CURVE('',#19213,#17324,#1720,.T.);
#24181=EDGE_CURVE('',#19213,#19214,#1007,.T.);
#24182=EDGE_CURVE('',#19214,#19211,#10363,.T.);
#24183=EDGE_CURVE('',#19215,#19216,#15154,.T.);
#24184=EDGE_CURVE('',#19215,#19212,#1721,.T.);
#24185=EDGE_CURVE('',#19211,#19216,#10364,.T.);
#24186=EDGE_CURVE('',#19217,#19218,#15155,.T.);
#24187=EDGE_CURVE('',#19218,#19215,#15156,.T.);
#24188=EDGE_CURVE('',#19216,#19217,#15157,.T.);
#24189=EDGE_CURVE('',#19219,#19220,#15158,.T.);
#24190=EDGE_CURVE('',#19220,#19155,#15159,.T.);
#24191=EDGE_CURVE('',#19155,#19221,#10365,.T.);
#24192=EDGE_CURVE('',#19222,#19221,#15160,.T.);
#24193=EDGE_CURVE('',#19222,#19223,#15161,.T.);
#24194=EDGE_CURVE('',#19223,#19219,#10366,.T.);
#24195=EDGE_CURVE('',#19221,#19218,#10367,.T.);
#24196=EDGE_CURVE('',#19217,#19222,#1722,.T.);
#24197=EDGE_CURVE('',#17327,#19154,#1008,.T.);
#24198=EDGE_CURVE('',#19224,#19225,#15162,.T.);
#24199=EDGE_CURVE('',#19224,#19220,#1723,.T.);
#24200=EDGE_CURVE('',#19219,#19225,#10368,.T.);
#24201=EDGE_CURVE('',#19226,#19227,#15163,.T.);
#24202=EDGE_CURVE('',#19227,#19224,#15164,.T.);
#24203=EDGE_CURVE('',#19225,#19226,#15165,.T.);
#24204=EDGE_CURVE('',#19228,#19229,#15166,.T.);
#24205=EDGE_CURVE('',#19229,#19164,#15167,.T.);
#24206=EDGE_CURVE('',#19164,#19230,#10369,.T.);
#24207=EDGE_CURVE('',#19231,#19230,#15168,.T.);
#24208=EDGE_CURVE('',#19231,#19232,#15169,.T.);
#24209=EDGE_CURVE('',#19232,#19228,#10370,.T.);
#24210=EDGE_CURVE('',#19230,#19227,#10371,.T.);
#24211=EDGE_CURVE('',#19226,#19231,#1724,.T.);
#24212=EDGE_CURVE('',#19233,#19234,#15170,.T.);
#24213=EDGE_CURVE('',#19233,#19229,#1725,.T.);
#24214=EDGE_CURVE('',#19228,#19234,#10372,.T.);
#24215=EDGE_CURVE('',#19235,#19236,#15171,.T.);
#24216=EDGE_CURVE('',#19236,#19233,#15172,.T.);
#24217=EDGE_CURVE('',#19234,#19235,#15173,.T.);
#24218=EDGE_CURVE('',#19237,#19238,#1726,.T.);
#24219=EDGE_CURVE('',#19238,#19173,#1727,.T.);
#24220=EDGE_CURVE('',#19173,#19239,#10373,.T.);
#24221=EDGE_CURVE('',#19240,#19239,#15174,.T.);
#24222=EDGE_CURVE('',#19240,#19241,#15175,.T.);
#24223=EDGE_CURVE('',#19241,#19237,#10374,.T.);
#24224=EDGE_CURVE('',#19239,#19236,#10375,.T.);
#24225=EDGE_CURVE('',#19235,#19240,#1728,.T.);
#24226=EDGE_CURVE('',#19242,#19243,#1729,.T.);
#24227=EDGE_CURVE('',#19242,#19238,#1730,.T.);
#24228=EDGE_CURVE('',#19237,#19243,#10376,.T.);
#24229=EDGE_CURVE('',#19244,#19245,#15176,.T.);
#24230=EDGE_CURVE('',#19245,#19242,#1731,.T.);
#24231=EDGE_CURVE('',#19243,#19244,#15177,.T.);
#24232=EDGE_CURVE('',#19246,#19247,#15178,.T.);
#24233=EDGE_CURVE('',#19247,#19182,#15179,.T.);
#24234=EDGE_CURVE('',#19182,#19248,#10377,.T.);
#24235=EDGE_CURVE('',#19249,#19248,#15180,.T.);
#24236=EDGE_CURVE('',#19249,#19250,#15181,.T.);
#24237=EDGE_CURVE('',#19250,#19246,#10378,.T.);
#24238=EDGE_CURVE('',#19248,#19245,#10379,.T.);
#24239=EDGE_CURVE('',#19244,#19249,#1732,.T.);
#24240=EDGE_CURVE('',#19251,#19252,#15182,.T.);
#24241=EDGE_CURVE('',#19251,#19247,#1733,.T.);
#24242=EDGE_CURVE('',#19246,#19252,#10380,.T.);
#24243=EDGE_CURVE('',#19253,#19254,#15183,.T.);
#24244=EDGE_CURVE('',#19254,#19251,#15184,.T.);
#24245=EDGE_CURVE('',#19252,#19253,#15185,.T.);
#24246=EDGE_CURVE('',#19255,#19256,#15186,.T.);
#24247=EDGE_CURVE('',#19256,#19191,#15187,.T.);
#24248=EDGE_CURVE('',#19191,#19257,#10381,.T.);
#24249=EDGE_CURVE('',#19258,#19257,#15188,.T.);
#24250=EDGE_CURVE('',#19258,#19259,#15189,.T.);
#24251=EDGE_CURVE('',#19259,#19255,#10382,.T.);
#24252=EDGE_CURVE('',#19257,#19254,#10383,.T.);
#24253=EDGE_CURVE('',#19253,#19258,#1734,.T.);
#24254=EDGE_CURVE('',#19260,#19261,#15190,.T.);
#24255=EDGE_CURVE('',#19260,#19256,#1735,.T.);
#24256=EDGE_CURVE('',#19255,#19261,#10384,.T.);
#24257=EDGE_CURVE('',#19262,#19263,#15191,.T.);
#24258=EDGE_CURVE('',#19263,#19260,#15192,.T.);
#24259=EDGE_CURVE('',#19261,#19262,#15193,.T.);
#24260=EDGE_CURVE('',#19264,#19265,#15194,.T.);
#24261=EDGE_CURVE('',#19265,#19200,#15195,.T.);
#24262=EDGE_CURVE('',#19200,#19266,#10385,.T.);
#24263=EDGE_CURVE('',#19267,#19266,#15196,.T.);
#24264=EDGE_CURVE('',#19267,#19268,#15197,.T.);
#24265=EDGE_CURVE('',#19268,#19264,#10386,.F.);
#24266=EDGE_CURVE('',#19266,#19263,#10387,.T.);
#24267=EDGE_CURVE('',#19262,#19267,#1736,.T.);
#24268=EDGE_CURVE('',#17720,#19265,#15198,.T.);
#24269=EDGE_CURVE('',#19264,#17721,#10388,.F.);
#24270=EDGE_CURVE('',#17717,#19209,#1009,.T.);
#24271=EDGE_CURVE('',#19209,#19269,#10389,.T.);
#24272=EDGE_CURVE('',#17718,#19269,#1010,.T.);
#24273=EDGE_CURVE('',#19269,#17719,#1011,.T.);
#24274=EDGE_CURVE('',#19270,#19271,#15199,.T.);
#24275=EDGE_CURVE('',#19271,#17321,#15200,.T.);
#24276=EDGE_CURVE('',#19272,#17320,#1737,.T.);
#24277=EDGE_CURVE('',#19272,#19273,#1012,.T.);
#24278=EDGE_CURVE('',#19273,#19270,#10390,.T.);
#24279=EDGE_CURVE('',#19274,#19275,#15201,.T.);
#24280=EDGE_CURVE('',#19274,#19271,#1738,.T.);
#24281=EDGE_CURVE('',#19270,#19275,#10391,.T.);
#24282=EDGE_CURVE('',#19276,#19277,#15202,.T.);
#24283=EDGE_CURVE('',#19277,#19274,#15203,.T.);
#24284=EDGE_CURVE('',#19275,#19276,#15204,.T.);
#24285=EDGE_CURVE('',#19278,#19279,#15205,.T.);
#24286=EDGE_CURVE('',#19279,#19214,#15206,.T.);
#24287=EDGE_CURVE('',#19214,#19280,#10392,.T.);
#24288=EDGE_CURVE('',#19281,#19280,#15207,.T.);
#24289=EDGE_CURVE('',#19281,#19282,#15208,.T.);
#24290=EDGE_CURVE('',#19282,#19278,#10393,.T.);
#24291=EDGE_CURVE('',#19280,#19277,#10394,.T.);
#24292=EDGE_CURVE('',#19276,#19281,#1739,.T.);
#24293=EDGE_CURVE('',#17323,#19213,#1013,.T.);
#24294=EDGE_CURVE('',#19283,#19284,#15209,.T.);
#24295=EDGE_CURVE('',#19283,#19279,#1740,.T.);
#24296=EDGE_CURVE('',#19278,#19284,#10395,.T.);
#24297=EDGE_CURVE('',#19285,#19286,#15210,.T.);
#24298=EDGE_CURVE('',#19286,#19283,#15211,.T.);
#24299=EDGE_CURVE('',#19284,#19285,#15212,.T.);
#24300=EDGE_CURVE('',#19287,#19288,#15213,.T.);
#24301=EDGE_CURVE('',#19288,#19223,#15214,.T.);
#24302=EDGE_CURVE('',#19223,#19289,#10396,.T.);
#24303=EDGE_CURVE('',#19290,#19289,#15215,.T.);
#24304=EDGE_CURVE('',#19290,#19291,#15216,.T.);
#24305=EDGE_CURVE('',#19291,#19287,#10397,.T.);
#24306=EDGE_CURVE('',#19289,#19286,#10398,.T.);
#24307=EDGE_CURVE('',#19285,#19290,#1741,.T.);
#24308=EDGE_CURVE('',#19292,#19293,#15217,.T.);
#24309=EDGE_CURVE('',#19292,#19288,#1742,.T.);
#24310=EDGE_CURVE('',#19287,#19293,#10399,.T.);
#24311=EDGE_CURVE('',#19294,#19295,#15218,.T.);
#24312=EDGE_CURVE('',#19295,#19292,#15219,.T.);
#24313=EDGE_CURVE('',#19293,#19294,#15220,.T.);
#24314=EDGE_CURVE('',#19296,#19297,#1743,.T.);
#24315=EDGE_CURVE('',#19297,#19232,#1744,.T.);
#24316=EDGE_CURVE('',#19232,#19298,#10400,.T.);
#24317=EDGE_CURVE('',#19299,#19298,#15221,.T.);
#24318=EDGE_CURVE('',#19299,#19300,#15222,.T.);
#24319=EDGE_CURVE('',#19300,#19296,#10401,.T.);
#24320=EDGE_CURVE('',#19298,#19295,#10402,.T.);
#24321=EDGE_CURVE('',#19294,#19299,#1745,.T.);
#24322=EDGE_CURVE('',#19301,#19302,#1746,.T.);
#24323=EDGE_CURVE('',#19301,#19297,#1747,.T.);
#24324=EDGE_CURVE('',#19296,#19302,#10403,.T.);
#24325=EDGE_CURVE('',#19303,#19304,#15223,.T.);
#24326=EDGE_CURVE('',#19304,#19301,#1748,.T.);
#24327=EDGE_CURVE('',#19302,#19303,#15224,.T.);
#24328=EDGE_CURVE('',#19305,#19306,#15225,.T.);
#24329=EDGE_CURVE('',#19306,#19241,#15226,.T.);
#24330=EDGE_CURVE('',#19241,#19307,#10404,.T.);
#24331=EDGE_CURVE('',#19308,#19307,#15227,.T.);
#24332=EDGE_CURVE('',#19308,#19309,#15228,.T.);
#24333=EDGE_CURVE('',#19309,#19305,#10405,.T.);
#24334=EDGE_CURVE('',#19307,#19304,#10406,.T.);
#24335=EDGE_CURVE('',#19303,#19308,#1749,.T.);
#24336=EDGE_CURVE('',#19310,#19311,#15229,.T.);
#24337=EDGE_CURVE('',#19310,#19306,#1750,.T.);
#24338=EDGE_CURVE('',#19305,#19311,#10407,.T.);
#24339=EDGE_CURVE('',#19312,#19313,#15230,.T.);
#24340=EDGE_CURVE('',#19313,#19310,#15231,.T.);
#24341=EDGE_CURVE('',#19311,#19312,#15232,.T.);
#24342=EDGE_CURVE('',#19314,#19315,#15233,.T.);
#24343=EDGE_CURVE('',#19315,#19250,#15234,.T.);
#24344=EDGE_CURVE('',#19250,#19316,#10408,.T.);
#24345=EDGE_CURVE('',#19317,#19316,#15235,.T.);
#24346=EDGE_CURVE('',#19317,#19318,#15236,.T.);
#24347=EDGE_CURVE('',#19318,#19314,#10409,.T.);
#24348=EDGE_CURVE('',#19316,#19313,#10410,.T.);
#24349=EDGE_CURVE('',#19312,#19317,#1751,.T.);
#24350=EDGE_CURVE('',#19319,#19320,#15237,.T.);
#24351=EDGE_CURVE('',#19319,#19315,#1752,.T.);
#24352=EDGE_CURVE('',#19314,#19320,#10411,.T.);
#24353=EDGE_CURVE('',#19321,#19322,#15238,.T.);
#24354=EDGE_CURVE('',#19322,#19319,#15239,.T.);
#24355=EDGE_CURVE('',#19320,#19321,#15240,.T.);
#24356=EDGE_CURVE('',#19323,#19324,#15241,.T.);
#24357=EDGE_CURVE('',#19324,#19259,#15242,.T.);
#24358=EDGE_CURVE('',#19259,#19325,#10412,.T.);
#24359=EDGE_CURVE('',#19326,#19325,#15243,.T.);
#24360=EDGE_CURVE('',#19326,#19327,#15244,.T.);
#24361=EDGE_CURVE('',#19327,#19323,#10413,.F.);
#24362=EDGE_CURVE('',#19325,#19322,#10414,.T.);
#24363=EDGE_CURVE('',#19321,#19326,#1753,.T.);
#24364=EDGE_CURVE('',#17726,#19324,#15245,.T.);
#24365=EDGE_CURVE('',#19323,#17727,#10415,.F.);
#24366=EDGE_CURVE('',#17723,#19268,#1014,.T.);
#24367=EDGE_CURVE('',#19268,#19328,#10416,.T.);
#24368=EDGE_CURVE('',#17724,#19328,#1015,.T.);
#24369=EDGE_CURVE('',#19328,#17725,#1016,.T.);
#24370=EDGE_CURVE('',#19329,#19330,#15246,.T.);
#24371=EDGE_CURVE('',#19330,#17317,#15247,.T.);
#24372=EDGE_CURVE('',#19331,#17316,#1754,.T.);
#24373=EDGE_CURVE('',#19331,#19332,#1017,.T.);
#24374=EDGE_CURVE('',#19332,#19329,#10417,.T.);
#24375=EDGE_CURVE('',#19333,#19334,#15248,.T.);
#24376=EDGE_CURVE('',#19333,#19330,#1755,.T.);
#24377=EDGE_CURVE('',#19329,#19334,#10418,.T.);
#24378=EDGE_CURVE('',#19335,#19336,#15249,.T.);
#24379=EDGE_CURVE('',#19336,#19333,#15250,.T.);
#24380=EDGE_CURVE('',#19334,#19335,#15251,.T.);
#24381=EDGE_CURVE('',#19337,#19338,#15252,.T.);
#24382=EDGE_CURVE('',#19338,#19273,#15253,.T.);
#24383=EDGE_CURVE('',#19273,#19339,#10419,.T.);
#24384=EDGE_CURVE('',#19340,#19339,#15254,.T.);
#24385=EDGE_CURVE('',#19340,#19341,#15255,.T.);
#24386=EDGE_CURVE('',#19341,#19337,#10420,.T.);
#24387=EDGE_CURVE('',#19339,#19336,#10421,.T.);
#24388=EDGE_CURVE('',#19335,#19340,#1756,.T.);
#24389=EDGE_CURVE('',#17319,#19272,#1018,.T.);
#24390=EDGE_CURVE('',#19342,#19343,#15256,.T.);
#24391=EDGE_CURVE('',#19342,#19338,#1757,.T.);
#24392=EDGE_CURVE('',#19337,#19343,#10422,.T.);
#24393=EDGE_CURVE('',#19344,#19345,#15257,.T.);
#24394=EDGE_CURVE('',#19345,#19342,#15258,.T.);
#24395=EDGE_CURVE('',#19343,#19344,#15259,.T.);
#24396=EDGE_CURVE('',#19346,#19347,#15260,.T.);
#24397=EDGE_CURVE('',#19347,#19282,#15261,.T.);
#24398=EDGE_CURVE('',#19282,#19348,#10423,.T.);
#24399=EDGE_CURVE('',#19349,#19348,#15262,.T.);
#24400=EDGE_CURVE('',#19349,#19350,#15263,.T.);
#24401=EDGE_CURVE('',#19350,#19346,#10424,.T.);
#24402=EDGE_CURVE('',#19348,#19345,#10425,.T.);
#24403=EDGE_CURVE('',#19344,#19349,#1758,.T.);
#24404=EDGE_CURVE('',#19351,#19352,#15264,.T.);
#24405=EDGE_CURVE('',#19351,#19347,#1759,.T.);
#24406=EDGE_CURVE('',#19346,#19352,#10426,.T.);
#24407=EDGE_CURVE('',#19353,#19354,#15265,.T.);
#24408=EDGE_CURVE('',#19354,#19351,#15266,.T.);
#24409=EDGE_CURVE('',#19352,#19353,#15267,.T.);
#24410=EDGE_CURVE('',#19355,#19356,#1760,.T.);
#24411=EDGE_CURVE('',#19356,#19291,#1761,.T.);
#24412=EDGE_CURVE('',#19291,#19357,#10427,.T.);
#24413=EDGE_CURVE('',#19358,#19357,#15268,.T.);
#24414=EDGE_CURVE('',#19358,#19359,#15269,.T.);
#24415=EDGE_CURVE('',#19359,#19355,#10428,.T.);
#24416=EDGE_CURVE('',#19357,#19354,#10429,.T.);
#24417=EDGE_CURVE('',#19353,#19358,#1762,.T.);
#24418=EDGE_CURVE('',#19360,#19361,#1763,.T.);
#24419=EDGE_CURVE('',#19360,#19356,#1764,.T.);
#24420=EDGE_CURVE('',#19355,#19361,#10430,.T.);
#24421=EDGE_CURVE('',#19362,#19363,#15270,.T.);
#24422=EDGE_CURVE('',#19363,#19360,#1765,.T.);
#24423=EDGE_CURVE('',#19361,#19362,#15271,.T.);
#24424=EDGE_CURVE('',#19364,#19365,#15272,.T.);
#24425=EDGE_CURVE('',#19365,#19300,#15273,.T.);
#24426=EDGE_CURVE('',#19300,#19366,#10431,.T.);
#24427=EDGE_CURVE('',#19367,#19366,#15274,.T.);
#24428=EDGE_CURVE('',#19367,#19368,#15275,.T.);
#24429=EDGE_CURVE('',#19368,#19364,#10432,.T.);
#24430=EDGE_CURVE('',#19366,#19363,#10433,.T.);
#24431=EDGE_CURVE('',#19362,#19367,#1766,.T.);
#24432=EDGE_CURVE('',#19369,#19370,#15276,.T.);
#24433=EDGE_CURVE('',#19369,#19365,#1767,.T.);
#24434=EDGE_CURVE('',#19364,#19370,#10434,.T.);
#24435=EDGE_CURVE('',#19371,#19372,#15277,.T.);
#24436=EDGE_CURVE('',#19372,#19369,#15278,.T.);
#24437=EDGE_CURVE('',#19370,#19371,#15279,.T.);
#24438=EDGE_CURVE('',#19373,#19374,#15280,.T.);
#24439=EDGE_CURVE('',#19374,#19309,#15281,.T.);
#24440=EDGE_CURVE('',#19309,#19375,#10435,.T.);
#24441=EDGE_CURVE('',#19376,#19375,#15282,.T.);
#24442=EDGE_CURVE('',#19376,#19377,#15283,.T.);
#24443=EDGE_CURVE('',#19377,#19373,#10436,.T.);
#24444=EDGE_CURVE('',#19375,#19372,#10437,.T.);
#24445=EDGE_CURVE('',#19371,#19376,#1768,.T.);
#24446=EDGE_CURVE('',#19378,#19379,#15284,.T.);
#24447=EDGE_CURVE('',#19378,#19374,#1769,.T.);
#24448=EDGE_CURVE('',#19373,#19379,#10438,.T.);
#24449=EDGE_CURVE('',#19380,#19381,#15285,.T.);
#24450=EDGE_CURVE('',#19381,#19378,#15286,.T.);
#24451=EDGE_CURVE('',#19379,#19380,#15287,.T.);
#24452=EDGE_CURVE('',#19382,#19383,#15288,.T.);
#24453=EDGE_CURVE('',#19383,#19318,#15289,.T.);
#24454=EDGE_CURVE('',#19318,#19384,#10439,.T.);
#24455=EDGE_CURVE('',#19385,#19384,#15290,.T.);
#24456=EDGE_CURVE('',#19385,#19386,#15291,.T.);
#24457=EDGE_CURVE('',#19386,#19382,#10440,.F.);
#24458=EDGE_CURVE('',#19384,#19381,#10441,.T.);
#24459=EDGE_CURVE('',#19380,#19385,#1770,.T.);
#24460=EDGE_CURVE('',#17432,#19383,#15292,.T.);
#24461=EDGE_CURVE('',#19382,#17433,#10442,.F.);
#24462=EDGE_CURVE('',#17729,#19327,#1019,.T.);
#24463=EDGE_CURVE('',#19327,#19387,#10443,.T.);
#24464=EDGE_CURVE('',#17730,#19387,#1020,.T.);
#24465=EDGE_CURVE('',#19387,#17429,#1021,.T.);
#24466=EDGE_CURVE('',#19388,#19389,#15293,.T.);
#24467=EDGE_CURVE('',#19389,#17313,#15294,.T.);
#24468=EDGE_CURVE('',#19390,#17312,#1771,.T.);
#24469=EDGE_CURVE('',#19390,#19391,#1022,.T.);
#24470=EDGE_CURVE('',#19391,#19388,#10444,.T.);
#24471=EDGE_CURVE('',#19392,#19393,#15295,.T.);
#24472=EDGE_CURVE('',#19392,#19389,#1772,.T.);
#24473=EDGE_CURVE('',#19388,#19393,#10445,.T.);
#24474=EDGE_CURVE('',#19394,#19395,#15296,.T.);
#24475=EDGE_CURVE('',#19395,#19392,#15297,.T.);
#24476=EDGE_CURVE('',#19393,#19394,#15298,.T.);
#24477=EDGE_CURVE('',#19396,#19397,#15299,.T.);
#24478=EDGE_CURVE('',#19397,#19332,#15300,.T.);
#24479=EDGE_CURVE('',#19332,#19398,#10446,.T.);
#24480=EDGE_CURVE('',#19399,#19398,#15301,.T.);
#24481=EDGE_CURVE('',#19399,#19400,#15302,.T.);
#24482=EDGE_CURVE('',#19400,#19396,#10447,.T.);
#24483=EDGE_CURVE('',#19398,#19395,#10448,.T.);
#24484=EDGE_CURVE('',#19394,#19399,#1773,.T.);
#24485=EDGE_CURVE('',#17315,#19331,#1023,.T.);
#24486=EDGE_CURVE('',#19401,#19402,#15303,.T.);
#24487=EDGE_CURVE('',#19401,#19397,#1774,.T.);
#24488=EDGE_CURVE('',#19396,#19402,#10449,.T.);
#24489=EDGE_CURVE('',#19403,#19404,#15304,.T.);
#24490=EDGE_CURVE('',#19404,#19401,#15305,.T.);
#24491=EDGE_CURVE('',#19402,#19403,#15306,.T.);
#24492=EDGE_CURVE('',#19405,#19406,#15307,.T.);
#24493=EDGE_CURVE('',#19406,#19341,#15308,.T.);
#24494=EDGE_CURVE('',#19341,#19407,#10450,.T.);
#24495=EDGE_CURVE('',#19408,#19407,#15309,.T.);
#24496=EDGE_CURVE('',#19408,#19409,#15310,.T.);
#24497=EDGE_CURVE('',#19409,#19405,#10451,.T.);
#24498=EDGE_CURVE('',#19407,#19404,#10452,.T.);
#24499=EDGE_CURVE('',#19403,#19408,#1775,.T.);
#24500=EDGE_CURVE('',#19410,#19411,#15311,.T.);
#24501=EDGE_CURVE('',#19410,#19406,#1776,.T.);
#24502=EDGE_CURVE('',#19405,#19411,#10453,.T.);
#24503=EDGE_CURVE('',#19412,#19413,#15312,.T.);
#24504=EDGE_CURVE('',#19413,#19410,#15313,.T.);
#24505=EDGE_CURVE('',#19411,#19412,#15314,.T.);
#24506=EDGE_CURVE('',#19414,#19415,#1777,.T.);
#24507=EDGE_CURVE('',#19415,#19350,#1778,.T.);
#24508=EDGE_CURVE('',#19350,#19416,#10454,.T.);
#24509=EDGE_CURVE('',#19417,#19416,#15315,.T.);
#24510=EDGE_CURVE('',#19417,#19418,#15316,.T.);
#24511=EDGE_CURVE('',#19418,#19414,#10455,.T.);
#24512=EDGE_CURVE('',#19416,#19413,#10456,.T.);
#24513=EDGE_CURVE('',#19412,#19417,#1779,.T.);
#24514=EDGE_CURVE('',#19419,#19420,#1780,.T.);
#24515=EDGE_CURVE('',#19419,#19415,#1781,.T.);
#24516=EDGE_CURVE('',#19414,#19420,#10457,.T.);
#24517=EDGE_CURVE('',#19421,#19422,#15317,.T.);
#24518=EDGE_CURVE('',#19422,#19419,#1782,.T.);
#24519=EDGE_CURVE('',#19420,#19421,#15318,.T.);
#24520=EDGE_CURVE('',#19423,#19424,#15319,.T.);
#24521=EDGE_CURVE('',#19424,#19359,#15320,.T.);
#24522=EDGE_CURVE('',#19359,#19425,#10458,.T.);
#24523=EDGE_CURVE('',#19426,#19425,#15321,.T.);
#24524=EDGE_CURVE('',#19426,#19427,#15322,.T.);
#24525=EDGE_CURVE('',#19427,#19423,#10459,.T.);
#24526=EDGE_CURVE('',#19425,#19422,#10460,.T.);
#24527=EDGE_CURVE('',#19421,#19426,#1783,.T.);
#24528=EDGE_CURVE('',#19428,#19429,#15323,.T.);
#24529=EDGE_CURVE('',#19428,#19424,#1784,.T.);
#24530=EDGE_CURVE('',#19423,#19429,#10461,.T.);
#24531=EDGE_CURVE('',#19430,#19431,#15324,.T.);
#24532=EDGE_CURVE('',#19431,#19428,#15325,.T.);
#24533=EDGE_CURVE('',#19429,#19430,#15326,.T.);
#24534=EDGE_CURVE('',#19432,#19433,#15327,.T.);
#24535=EDGE_CURVE('',#19433,#19368,#15328,.T.);
#24536=EDGE_CURVE('',#19368,#19434,#10462,.T.);
#24537=EDGE_CURVE('',#19435,#19434,#15329,.T.);
#24538=EDGE_CURVE('',#19435,#19436,#15330,.T.);
#24539=EDGE_CURVE('',#19436,#19432,#10463,.T.);
#24540=EDGE_CURVE('',#19434,#19431,#10464,.T.);
#24541=EDGE_CURVE('',#19430,#19435,#1785,.T.);
#24542=EDGE_CURVE('',#19437,#19438,#15331,.T.);
#24543=EDGE_CURVE('',#19437,#19433,#1786,.T.);
#24544=EDGE_CURVE('',#19432,#19438,#10465,.T.);
#24545=EDGE_CURVE('',#19439,#19440,#15332,.T.);
#24546=EDGE_CURVE('',#19440,#19437,#15333,.T.);
#24547=EDGE_CURVE('',#19438,#19439,#15334,.T.);
#24548=EDGE_CURVE('',#19441,#19442,#15335,.T.);
#24549=EDGE_CURVE('',#19442,#19377,#15336,.T.);
#24550=EDGE_CURVE('',#19377,#19443,#10466,.T.);
#24551=EDGE_CURVE('',#19444,#19443,#15337,.T.);
#24552=EDGE_CURVE('',#19444,#19445,#15338,.T.);
#24553=EDGE_CURVE('',#19445,#19441,#10467,.F.);
#24554=EDGE_CURVE('',#19443,#19440,#10468,.T.);
#24555=EDGE_CURVE('',#19439,#19444,#1787,.T.);
#24556=EDGE_CURVE('',#17438,#19442,#15339,.T.);
#24557=EDGE_CURVE('',#19441,#17439,#10469,.F.);
#24558=EDGE_CURVE('',#17435,#19386,#1024,.T.);
#24559=EDGE_CURVE('',#19386,#19446,#10470,.T.);
#24560=EDGE_CURVE('',#17436,#19446,#1025,.T.);
#24561=EDGE_CURVE('',#19446,#17437,#1026,.T.);
#24562=EDGE_CURVE('',#19447,#19448,#15340,.T.);
#24563=EDGE_CURVE('',#19448,#17309,#15341,.T.);
#24564=EDGE_CURVE('',#19449,#17308,#1788,.T.);
#24565=EDGE_CURVE('',#19449,#19450,#1027,.T.);
#24566=EDGE_CURVE('',#19450,#19447,#10471,.T.);
#24567=EDGE_CURVE('',#19451,#19452,#15342,.T.);
#24568=EDGE_CURVE('',#19451,#19448,#1789,.T.);
#24569=EDGE_CURVE('',#19447,#19452,#10472,.T.);
#24570=EDGE_CURVE('',#19453,#19454,#15343,.T.);
#24571=EDGE_CURVE('',#19454,#19451,#15344,.T.);
#24572=EDGE_CURVE('',#19452,#19453,#15345,.T.);
#24573=EDGE_CURVE('',#19455,#19456,#15346,.T.);
#24574=EDGE_CURVE('',#19456,#19391,#15347,.T.);
#24575=EDGE_CURVE('',#19391,#19457,#10473,.T.);
#24576=EDGE_CURVE('',#19458,#19457,#15348,.T.);
#24577=EDGE_CURVE('',#19458,#19459,#15349,.T.);
#24578=EDGE_CURVE('',#19459,#19455,#10474,.T.);
#24579=EDGE_CURVE('',#19457,#19454,#10475,.T.);
#24580=EDGE_CURVE('',#19453,#19458,#1790,.T.);
#24581=EDGE_CURVE('',#17311,#19390,#1028,.T.);
#24582=EDGE_CURVE('',#19460,#19461,#15350,.T.);
#24583=EDGE_CURVE('',#19460,#19456,#1791,.T.);
#24584=EDGE_CURVE('',#19455,#19461,#10476,.T.);
#24585=EDGE_CURVE('',#19462,#19463,#15351,.T.);
#24586=EDGE_CURVE('',#19463,#19460,#15352,.T.);
#24587=EDGE_CURVE('',#19461,#19462,#15353,.T.);
#24588=EDGE_CURVE('',#19464,#19465,#15354,.T.);
#24589=EDGE_CURVE('',#19465,#19400,#15355,.T.);
#24590=EDGE_CURVE('',#19400,#19466,#10477,.T.);
#24591=EDGE_CURVE('',#19467,#19466,#15356,.T.);
#24592=EDGE_CURVE('',#19467,#19468,#15357,.T.);
#24593=EDGE_CURVE('',#19468,#19464,#10478,.T.);
#24594=EDGE_CURVE('',#19466,#19463,#10479,.T.);
#24595=EDGE_CURVE('',#19462,#19467,#1792,.T.);
#24596=EDGE_CURVE('',#19469,#19470,#15358,.T.);
#24597=EDGE_CURVE('',#19469,#19465,#1793,.T.);
#24598=EDGE_CURVE('',#19464,#19470,#10480,.T.);
#24599=EDGE_CURVE('',#19471,#19472,#15359,.T.);
#24600=EDGE_CURVE('',#19472,#19469,#15360,.T.);
#24601=EDGE_CURVE('',#19470,#19471,#15361,.T.);
#24602=EDGE_CURVE('',#19473,#19474,#1794,.T.);
#24603=EDGE_CURVE('',#19474,#19409,#1795,.T.);
#24604=EDGE_CURVE('',#19409,#19475,#10481,.T.);
#24605=EDGE_CURVE('',#19476,#19475,#15362,.T.);
#24606=EDGE_CURVE('',#19476,#19477,#15363,.T.);
#24607=EDGE_CURVE('',#19477,#19473,#10482,.T.);
#24608=EDGE_CURVE('',#19475,#19472,#10483,.T.);
#24609=EDGE_CURVE('',#19471,#19476,#1796,.T.);
#24610=EDGE_CURVE('',#19478,#19479,#1797,.T.);
#24611=EDGE_CURVE('',#19478,#19474,#1798,.T.);
#24612=EDGE_CURVE('',#19473,#19479,#10484,.T.);
#24613=EDGE_CURVE('',#19480,#19481,#15364,.T.);
#24614=EDGE_CURVE('',#19481,#19478,#1799,.T.);
#24615=EDGE_CURVE('',#19479,#19480,#15365,.T.);
#24616=EDGE_CURVE('',#19482,#19483,#15366,.T.);
#24617=EDGE_CURVE('',#19483,#19418,#15367,.T.);
#24618=EDGE_CURVE('',#19418,#19484,#10485,.T.);
#24619=EDGE_CURVE('',#19485,#19484,#15368,.T.);
#24620=EDGE_CURVE('',#19485,#19486,#15369,.T.);
#24621=EDGE_CURVE('',#19486,#19482,#10486,.T.);
#24622=EDGE_CURVE('',#19484,#19481,#10487,.T.);
#24623=EDGE_CURVE('',#19480,#19485,#1800,.T.);
#24624=EDGE_CURVE('',#19487,#19488,#15370,.T.);
#24625=EDGE_CURVE('',#19487,#19483,#1801,.T.);
#24626=EDGE_CURVE('',#19482,#19488,#10488,.T.);
#24627=EDGE_CURVE('',#19489,#19490,#15371,.T.);
#24628=EDGE_CURVE('',#19490,#19487,#15372,.T.);
#24629=EDGE_CURVE('',#19488,#19489,#15373,.T.);
#24630=EDGE_CURVE('',#19491,#19492,#15374,.T.);
#24631=EDGE_CURVE('',#19492,#19427,#15375,.T.);
#24632=EDGE_CURVE('',#19427,#19493,#10489,.T.);
#24633=EDGE_CURVE('',#19494,#19493,#15376,.T.);
#24634=EDGE_CURVE('',#19494,#19495,#15377,.T.);
#24635=EDGE_CURVE('',#19495,#19491,#10490,.T.);
#24636=EDGE_CURVE('',#19493,#19490,#10491,.T.);
#24637=EDGE_CURVE('',#19489,#19494,#1802,.T.);
#24638=EDGE_CURVE('',#19496,#19497,#15378,.T.);
#24639=EDGE_CURVE('',#19496,#19492,#1803,.T.);
#24640=EDGE_CURVE('',#19491,#19497,#10492,.T.);
#24641=EDGE_CURVE('',#19498,#19499,#15379,.T.);
#24642=EDGE_CURVE('',#19499,#19496,#15380,.T.);
#24643=EDGE_CURVE('',#19497,#19498,#15381,.T.);
#24644=EDGE_CURVE('',#19500,#19501,#15382,.T.);
#24645=EDGE_CURVE('',#19501,#19436,#15383,.T.);
#24646=EDGE_CURVE('',#19436,#19502,#10493,.T.);
#24647=EDGE_CURVE('',#19503,#19502,#15384,.T.);
#24648=EDGE_CURVE('',#19503,#19504,#15385,.T.);
#24649=EDGE_CURVE('',#19504,#19500,#10494,.F.);
#24650=EDGE_CURVE('',#19502,#19499,#10495,.T.);
#24651=EDGE_CURVE('',#19498,#19503,#1804,.T.);
#24652=EDGE_CURVE('',#17444,#19501,#15386,.T.);
#24653=EDGE_CURVE('',#19500,#17445,#10496,.F.);
#24654=EDGE_CURVE('',#17441,#19445,#1029,.T.);
#24655=EDGE_CURVE('',#19445,#19505,#10497,.T.);
#24656=EDGE_CURVE('',#17442,#19505,#1030,.T.);
#24657=EDGE_CURVE('',#19505,#17443,#1031,.T.);
#24658=EDGE_CURVE('',#19506,#19507,#15387,.T.);
#24659=EDGE_CURVE('',#19507,#17305,#15388,.T.);
#24660=EDGE_CURVE('',#19508,#17304,#1805,.T.);
#24661=EDGE_CURVE('',#19508,#19509,#1032,.T.);
#24662=EDGE_CURVE('',#19509,#19506,#10498,.T.);
#24663=EDGE_CURVE('',#19510,#19511,#15389,.T.);
#24664=EDGE_CURVE('',#19510,#19507,#1806,.T.);
#24665=EDGE_CURVE('',#19506,#19511,#10499,.T.);
#24666=EDGE_CURVE('',#19512,#19513,#15390,.T.);
#24667=EDGE_CURVE('',#19513,#19510,#15391,.T.);
#24668=EDGE_CURVE('',#19511,#19512,#15392,.T.);
#24669=EDGE_CURVE('',#19514,#19515,#15393,.T.);
#24670=EDGE_CURVE('',#19515,#19450,#15394,.T.);
#24671=EDGE_CURVE('',#19450,#19516,#10500,.T.);
#24672=EDGE_CURVE('',#19517,#19516,#15395,.T.);
#24673=EDGE_CURVE('',#19517,#19518,#15396,.T.);
#24674=EDGE_CURVE('',#19518,#19514,#10501,.T.);
#24675=EDGE_CURVE('',#19516,#19513,#10502,.T.);
#24676=EDGE_CURVE('',#19512,#19517,#1807,.T.);
#24677=EDGE_CURVE('',#17307,#19449,#1033,.T.);
#24678=EDGE_CURVE('',#19519,#19520,#15397,.T.);
#24679=EDGE_CURVE('',#19519,#19515,#1808,.T.);
#24680=EDGE_CURVE('',#19514,#19520,#10503,.T.);
#24681=EDGE_CURVE('',#19521,#19522,#15398,.T.);
#24682=EDGE_CURVE('',#19522,#19519,#15399,.T.);
#24683=EDGE_CURVE('',#19520,#19521,#15400,.T.);
#24684=EDGE_CURVE('',#19523,#19524,#15401,.T.);
#24685=EDGE_CURVE('',#19524,#19459,#15402,.T.);
#24686=EDGE_CURVE('',#19459,#19525,#10504,.T.);
#24687=EDGE_CURVE('',#19526,#19525,#15403,.T.);
#24688=EDGE_CURVE('',#19526,#19527,#15404,.T.);
#24689=EDGE_CURVE('',#19527,#19523,#10505,.T.);
#24690=EDGE_CURVE('',#19525,#19522,#10506,.T.);
#24691=EDGE_CURVE('',#19521,#19526,#1809,.T.);
#24692=EDGE_CURVE('',#19528,#19529,#15405,.T.);
#24693=EDGE_CURVE('',#19528,#19524,#1810,.T.);
#24694=EDGE_CURVE('',#19523,#19529,#10507,.T.);
#24695=EDGE_CURVE('',#19530,#19531,#15406,.T.);
#24696=EDGE_CURVE('',#19531,#19528,#15407,.T.);
#24697=EDGE_CURVE('',#19529,#19530,#15408,.T.);
#24698=EDGE_CURVE('',#19532,#19533,#1811,.T.);
#24699=EDGE_CURVE('',#19533,#19468,#1812,.T.);
#24700=EDGE_CURVE('',#19468,#19534,#10508,.T.);
#24701=EDGE_CURVE('',#19535,#19534,#15409,.T.);
#24702=EDGE_CURVE('',#19535,#19536,#15410,.T.);
#24703=EDGE_CURVE('',#19536,#19532,#10509,.T.);
#24704=EDGE_CURVE('',#19534,#19531,#10510,.T.);
#24705=EDGE_CURVE('',#19530,#19535,#1813,.T.);
#24706=EDGE_CURVE('',#19537,#19538,#1814,.T.);
#24707=EDGE_CURVE('',#19537,#19533,#1815,.T.);
#24708=EDGE_CURVE('',#19532,#19538,#10511,.T.);
#24709=EDGE_CURVE('',#19539,#19540,#15411,.T.);
#24710=EDGE_CURVE('',#19540,#19537,#1816,.T.);
#24711=EDGE_CURVE('',#19538,#19539,#15412,.T.);
#24712=EDGE_CURVE('',#19541,#19542,#15413,.T.);
#24713=EDGE_CURVE('',#19542,#19477,#15414,.T.);
#24714=EDGE_CURVE('',#19477,#19543,#10512,.T.);
#24715=EDGE_CURVE('',#19544,#19543,#15415,.T.);
#24716=EDGE_CURVE('',#19544,#19545,#15416,.T.);
#24717=EDGE_CURVE('',#19545,#19541,#10513,.T.);
#24718=EDGE_CURVE('',#19543,#19540,#10514,.T.);
#24719=EDGE_CURVE('',#19539,#19544,#1817,.T.);
#24720=EDGE_CURVE('',#19546,#19547,#15417,.T.);
#24721=EDGE_CURVE('',#19546,#19542,#1818,.T.);
#24722=EDGE_CURVE('',#19541,#19547,#10515,.T.);
#24723=EDGE_CURVE('',#19548,#19549,#15418,.T.);
#24724=EDGE_CURVE('',#19549,#19546,#15419,.T.);
#24725=EDGE_CURVE('',#19547,#19548,#15420,.T.);
#24726=EDGE_CURVE('',#19550,#19551,#15421,.T.);
#24727=EDGE_CURVE('',#19551,#19486,#15422,.T.);
#24728=EDGE_CURVE('',#19486,#19552,#10516,.T.);
#24729=EDGE_CURVE('',#19553,#19552,#15423,.T.);
#24730=EDGE_CURVE('',#19553,#19554,#15424,.T.);
#24731=EDGE_CURVE('',#19554,#19550,#10517,.T.);
#24732=EDGE_CURVE('',#19552,#19549,#10518,.T.);
#24733=EDGE_CURVE('',#19548,#19553,#1819,.T.);
#24734=EDGE_CURVE('',#19555,#19556,#15425,.T.);
#24735=EDGE_CURVE('',#19555,#19551,#1820,.T.);
#24736=EDGE_CURVE('',#19550,#19556,#10519,.T.);
#24737=EDGE_CURVE('',#19557,#19558,#15426,.T.);
#24738=EDGE_CURVE('',#19558,#19555,#15427,.T.);
#24739=EDGE_CURVE('',#19556,#19557,#15428,.T.);
#24740=EDGE_CURVE('',#19559,#19560,#15429,.T.);
#24741=EDGE_CURVE('',#19560,#19495,#15430,.T.);
#24742=EDGE_CURVE('',#19495,#19561,#10520,.T.);
#24743=EDGE_CURVE('',#19562,#19561,#15431,.T.);
#24744=EDGE_CURVE('',#19562,#19563,#15432,.T.);
#24745=EDGE_CURVE('',#19563,#19559,#10521,.F.);
#24746=EDGE_CURVE('',#19561,#19558,#10522,.T.);
#24747=EDGE_CURVE('',#19557,#19562,#1821,.T.);
#24748=EDGE_CURVE('',#17450,#19560,#15433,.T.);
#24749=EDGE_CURVE('',#19559,#17451,#10523,.F.);
#24750=EDGE_CURVE('',#17447,#19504,#1034,.T.);
#24751=EDGE_CURVE('',#19504,#19564,#10524,.T.);
#24752=EDGE_CURVE('',#17448,#19564,#1035,.T.);
#24753=EDGE_CURVE('',#19564,#17449,#1036,.T.);
#24754=EDGE_CURVE('',#19565,#19566,#15434,.T.);
#24755=EDGE_CURVE('',#19566,#17301,#15435,.T.);
#24756=EDGE_CURVE('',#19567,#17300,#1822,.T.);
#24757=EDGE_CURVE('',#19567,#19568,#1037,.T.);
#24758=EDGE_CURVE('',#19568,#19565,#10525,.T.);
#24759=EDGE_CURVE('',#19569,#19570,#15436,.T.);
#24760=EDGE_CURVE('',#19569,#19566,#1823,.T.);
#24761=EDGE_CURVE('',#19565,#19570,#10526,.T.);
#24762=EDGE_CURVE('',#19571,#19572,#15437,.T.);
#24763=EDGE_CURVE('',#19572,#19569,#15438,.T.);
#24764=EDGE_CURVE('',#19570,#19571,#15439,.T.);
#24765=EDGE_CURVE('',#19573,#19574,#15440,.T.);
#24766=EDGE_CURVE('',#19574,#19509,#15441,.T.);
#24767=EDGE_CURVE('',#19509,#19575,#10527,.T.);
#24768=EDGE_CURVE('',#19576,#19575,#15442,.T.);
#24769=EDGE_CURVE('',#19576,#19577,#15443,.T.);
#24770=EDGE_CURVE('',#19577,#19573,#10528,.T.);
#24771=EDGE_CURVE('',#19575,#19572,#10529,.T.);
#24772=EDGE_CURVE('',#19571,#19576,#1824,.T.);
#24773=EDGE_CURVE('',#17303,#19508,#1038,.T.);
#24774=EDGE_CURVE('',#19578,#19579,#15444,.T.);
#24775=EDGE_CURVE('',#19578,#19574,#1825,.T.);
#24776=EDGE_CURVE('',#19573,#19579,#10530,.T.);
#24777=EDGE_CURVE('',#19580,#19581,#15445,.T.);
#24778=EDGE_CURVE('',#19581,#19578,#15446,.T.);
#24779=EDGE_CURVE('',#19579,#19580,#15447,.T.);
#24780=EDGE_CURVE('',#19582,#19583,#15448,.T.);
#24781=EDGE_CURVE('',#19583,#19518,#15449,.T.);
#24782=EDGE_CURVE('',#19518,#19584,#10531,.T.);
#24783=EDGE_CURVE('',#19585,#19584,#15450,.T.);
#24784=EDGE_CURVE('',#19585,#19586,#15451,.T.);
#24785=EDGE_CURVE('',#19586,#19582,#10532,.T.);
#24786=EDGE_CURVE('',#19584,#19581,#10533,.T.);
#24787=EDGE_CURVE('',#19580,#19585,#1826,.T.);
#24788=EDGE_CURVE('',#19587,#19588,#15452,.T.);
#24789=EDGE_CURVE('',#19587,#19583,#1827,.T.);
#24790=EDGE_CURVE('',#19582,#19588,#10534,.T.);
#24791=EDGE_CURVE('',#19589,#19590,#15453,.T.);
#24792=EDGE_CURVE('',#19590,#19587,#15454,.T.);
#24793=EDGE_CURVE('',#19588,#19589,#15455,.T.);
#24794=EDGE_CURVE('',#19591,#19592,#1828,.T.);
#24795=EDGE_CURVE('',#19592,#19527,#1829,.T.);
#24796=EDGE_CURVE('',#19527,#19593,#10535,.T.);
#24797=EDGE_CURVE('',#19594,#19593,#15456,.T.);
#24798=EDGE_CURVE('',#19594,#19595,#15457,.T.);
#24799=EDGE_CURVE('',#19595,#19591,#10536,.T.);
#24800=EDGE_CURVE('',#19593,#19590,#10537,.T.);
#24801=EDGE_CURVE('',#19589,#19594,#1830,.T.);
#24802=EDGE_CURVE('',#19596,#19597,#1831,.T.);
#24803=EDGE_CURVE('',#19596,#19592,#1832,.T.);
#24804=EDGE_CURVE('',#19591,#19597,#10538,.T.);
#24805=EDGE_CURVE('',#19598,#19599,#15458,.T.);
#24806=EDGE_CURVE('',#19599,#19596,#1833,.T.);
#24807=EDGE_CURVE('',#19597,#19598,#15459,.T.);
#24808=EDGE_CURVE('',#19600,#19601,#15460,.T.);
#24809=EDGE_CURVE('',#19601,#19536,#15461,.T.);
#24810=EDGE_CURVE('',#19536,#19602,#10539,.T.);
#24811=EDGE_CURVE('',#19603,#19602,#15462,.T.);
#24812=EDGE_CURVE('',#19603,#19604,#15463,.T.);
#24813=EDGE_CURVE('',#19604,#19600,#10540,.T.);
#24814=EDGE_CURVE('',#19602,#19599,#10541,.T.);
#24815=EDGE_CURVE('',#19598,#19603,#1834,.T.);
#24816=EDGE_CURVE('',#19605,#19606,#15464,.T.);
#24817=EDGE_CURVE('',#19605,#19601,#1835,.T.);
#24818=EDGE_CURVE('',#19600,#19606,#10542,.T.);
#24819=EDGE_CURVE('',#19607,#19608,#15465,.T.);
#24820=EDGE_CURVE('',#19608,#19605,#15466,.T.);
#24821=EDGE_CURVE('',#19606,#19607,#15467,.T.);
#24822=EDGE_CURVE('',#19609,#19610,#15468,.T.);
#24823=EDGE_CURVE('',#19610,#19545,#15469,.T.);
#24824=EDGE_CURVE('',#19545,#19611,#10543,.T.);
#24825=EDGE_CURVE('',#19612,#19611,#15470,.T.);
#24826=EDGE_CURVE('',#19612,#19613,#15471,.T.);
#24827=EDGE_CURVE('',#19613,#19609,#10544,.T.);
#24828=EDGE_CURVE('',#19611,#19608,#10545,.T.);
#24829=EDGE_CURVE('',#19607,#19612,#1836,.T.);
#24830=EDGE_CURVE('',#19614,#19615,#15472,.T.);
#24831=EDGE_CURVE('',#19614,#19610,#1837,.T.);
#24832=EDGE_CURVE('',#19609,#19615,#10546,.T.);
#24833=EDGE_CURVE('',#19616,#19617,#15473,.T.);
#24834=EDGE_CURVE('',#19617,#19614,#15474,.T.);
#24835=EDGE_CURVE('',#19615,#19616,#15475,.T.);
#24836=EDGE_CURVE('',#19618,#19619,#15476,.T.);
#24837=EDGE_CURVE('',#19619,#19554,#15477,.T.);
#24838=EDGE_CURVE('',#19554,#19620,#10547,.T.);
#24839=EDGE_CURVE('',#19621,#19620,#15478,.T.);
#24840=EDGE_CURVE('',#19621,#19622,#15479,.T.);
#24841=EDGE_CURVE('',#19622,#19618,#10548,.F.);
#24842=EDGE_CURVE('',#19620,#19617,#10549,.T.);
#24843=EDGE_CURVE('',#19616,#19621,#1838,.T.);
#24844=EDGE_CURVE('',#17456,#19619,#15480,.T.);
#24845=EDGE_CURVE('',#19618,#17457,#10550,.F.);
#24846=EDGE_CURVE('',#17453,#19563,#1039,.T.);
#24847=EDGE_CURVE('',#19563,#19623,#10551,.T.);
#24848=EDGE_CURVE('',#17454,#19623,#1040,.T.);
#24849=EDGE_CURVE('',#19623,#17455,#1041,.T.);
#24850=EDGE_CURVE('',#19624,#19625,#15481,.T.);
#24851=EDGE_CURVE('',#19625,#17297,#15482,.T.);
#24852=EDGE_CURVE('',#19626,#17296,#1839,.T.);
#24853=EDGE_CURVE('',#19626,#19627,#1042,.T.);
#24854=EDGE_CURVE('',#19627,#19624,#10552,.T.);
#24855=EDGE_CURVE('',#19628,#19629,#15483,.T.);
#24856=EDGE_CURVE('',#19628,#19625,#1840,.T.);
#24857=EDGE_CURVE('',#19624,#19629,#10553,.T.);
#24858=EDGE_CURVE('',#19630,#19631,#15484,.T.);
#24859=EDGE_CURVE('',#19631,#19628,#15485,.T.);
#24860=EDGE_CURVE('',#19629,#19630,#15486,.T.);
#24861=EDGE_CURVE('',#19632,#19633,#15487,.T.);
#24862=EDGE_CURVE('',#19633,#19568,#15488,.T.);
#24863=EDGE_CURVE('',#19568,#19634,#10554,.T.);
#24864=EDGE_CURVE('',#19635,#19634,#15489,.T.);
#24865=EDGE_CURVE('',#19635,#19636,#15490,.T.);
#24866=EDGE_CURVE('',#19636,#19632,#10555,.T.);
#24867=EDGE_CURVE('',#19634,#19631,#10556,.T.);
#24868=EDGE_CURVE('',#19630,#19635,#1841,.T.);
#24869=EDGE_CURVE('',#17299,#19567,#1043,.T.);
#24870=EDGE_CURVE('',#19637,#19638,#15491,.T.);
#24871=EDGE_CURVE('',#19637,#19633,#1842,.T.);
#24872=EDGE_CURVE('',#19632,#19638,#10557,.T.);
#24873=EDGE_CURVE('',#19639,#19640,#15492,.T.);
#24874=EDGE_CURVE('',#19640,#19637,#15493,.T.);
#24875=EDGE_CURVE('',#19638,#19639,#15494,.T.);
#24876=EDGE_CURVE('',#19641,#19642,#15495,.T.);
#24877=EDGE_CURVE('',#19642,#19577,#15496,.T.);
#24878=EDGE_CURVE('',#19577,#19643,#10558,.T.);
#24879=EDGE_CURVE('',#19644,#19643,#15497,.T.);
#24880=EDGE_CURVE('',#19644,#19645,#15498,.T.);
#24881=EDGE_CURVE('',#19645,#19641,#10559,.T.);
#24882=EDGE_CURVE('',#19643,#19640,#10560,.T.);
#24883=EDGE_CURVE('',#19639,#19644,#1843,.T.);
#24884=EDGE_CURVE('',#19646,#19647,#15499,.T.);
#24885=EDGE_CURVE('',#19646,#19642,#1844,.T.);
#24886=EDGE_CURVE('',#19641,#19647,#10561,.T.);
#24887=EDGE_CURVE('',#19648,#19649,#15500,.T.);
#24888=EDGE_CURVE('',#19649,#19646,#15501,.T.);
#24889=EDGE_CURVE('',#19647,#19648,#15502,.T.);
#24890=EDGE_CURVE('',#19650,#19651,#1845,.T.);
#24891=EDGE_CURVE('',#19651,#19586,#1846,.T.);
#24892=EDGE_CURVE('',#19586,#19652,#10562,.T.);
#24893=EDGE_CURVE('',#19653,#19652,#15503,.T.);
#24894=EDGE_CURVE('',#19653,#19654,#15504,.T.);
#24895=EDGE_CURVE('',#19654,#19650,#10563,.T.);
#24896=EDGE_CURVE('',#19652,#19649,#10564,.T.);
#24897=EDGE_CURVE('',#19648,#19653,#1847,.T.);
#24898=EDGE_CURVE('',#19655,#19656,#1848,.T.);
#24899=EDGE_CURVE('',#19655,#19651,#1849,.T.);
#24900=EDGE_CURVE('',#19650,#19656,#10565,.T.);
#24901=EDGE_CURVE('',#19657,#19658,#15505,.T.);
#24902=EDGE_CURVE('',#19658,#19655,#1850,.T.);
#24903=EDGE_CURVE('',#19656,#19657,#15506,.T.);
#24904=EDGE_CURVE('',#19659,#19660,#15507,.T.);
#24905=EDGE_CURVE('',#19660,#19595,#15508,.T.);
#24906=EDGE_CURVE('',#19595,#19661,#10566,.T.);
#24907=EDGE_CURVE('',#19662,#19661,#15509,.T.);
#24908=EDGE_CURVE('',#19662,#19663,#15510,.T.);
#24909=EDGE_CURVE('',#19663,#19659,#10567,.T.);
#24910=EDGE_CURVE('',#19661,#19658,#10568,.T.);
#24911=EDGE_CURVE('',#19657,#19662,#1851,.T.);
#24912=EDGE_CURVE('',#19664,#19665,#15511,.T.);
#24913=EDGE_CURVE('',#19664,#19660,#1852,.T.);
#24914=EDGE_CURVE('',#19659,#19665,#10569,.T.);
#24915=EDGE_CURVE('',#19666,#19667,#15512,.T.);
#24916=EDGE_CURVE('',#19667,#19664,#15513,.T.);
#24917=EDGE_CURVE('',#19665,#19666,#15514,.T.);
#24918=EDGE_CURVE('',#19668,#19669,#15515,.T.);
#24919=EDGE_CURVE('',#19669,#19604,#15516,.T.);
#24920=EDGE_CURVE('',#19604,#19670,#10570,.T.);
#24921=EDGE_CURVE('',#19671,#19670,#15517,.T.);
#24922=EDGE_CURVE('',#19671,#19672,#15518,.T.);
#24923=EDGE_CURVE('',#19672,#19668,#10571,.T.);
#24924=EDGE_CURVE('',#19670,#19667,#10572,.T.);
#24925=EDGE_CURVE('',#19666,#19671,#1853,.T.);
#24926=EDGE_CURVE('',#19673,#19674,#15519,.T.);
#24927=EDGE_CURVE('',#19673,#19669,#1854,.T.);
#24928=EDGE_CURVE('',#19668,#19674,#10573,.T.);
#24929=EDGE_CURVE('',#19675,#19676,#15520,.T.);
#24930=EDGE_CURVE('',#19676,#19673,#15521,.T.);
#24931=EDGE_CURVE('',#19674,#19675,#15522,.T.);
#24932=EDGE_CURVE('',#19677,#19678,#15523,.T.);
#24933=EDGE_CURVE('',#19678,#19613,#15524,.T.);
#24934=EDGE_CURVE('',#19613,#19679,#10574,.T.);
#24935=EDGE_CURVE('',#19680,#19679,#15525,.T.);
#24936=EDGE_CURVE('',#19680,#19681,#15526,.T.);
#24937=EDGE_CURVE('',#19681,#19677,#10575,.F.);
#24938=EDGE_CURVE('',#19679,#19676,#10576,.T.);
#24939=EDGE_CURVE('',#19675,#19680,#1855,.T.);
#24940=EDGE_CURVE('',#17462,#19678,#15527,.T.);
#24941=EDGE_CURVE('',#19677,#17463,#10577,.F.);
#24942=EDGE_CURVE('',#17459,#19622,#1044,.T.);
#24943=EDGE_CURVE('',#19622,#19682,#10578,.T.);
#24944=EDGE_CURVE('',#17460,#19682,#1045,.T.);
#24945=EDGE_CURVE('',#19682,#17461,#1046,.T.);
#24946=EDGE_CURVE('',#19683,#19684,#15528,.T.);
#24947=EDGE_CURVE('',#19684,#17293,#15529,.T.);
#24948=EDGE_CURVE('',#19685,#17292,#1856,.T.);
#24949=EDGE_CURVE('',#19685,#19686,#1047,.T.);
#24950=EDGE_CURVE('',#19686,#19683,#10579,.T.);
#24951=EDGE_CURVE('',#19687,#19688,#15530,.T.);
#24952=EDGE_CURVE('',#19687,#19684,#1857,.T.);
#24953=EDGE_CURVE('',#19683,#19688,#10580,.T.);
#24954=EDGE_CURVE('',#19689,#19690,#15531,.T.);
#24955=EDGE_CURVE('',#19690,#19687,#15532,.T.);
#24956=EDGE_CURVE('',#19688,#19689,#15533,.T.);
#24957=EDGE_CURVE('',#19691,#19692,#15534,.T.);
#24958=EDGE_CURVE('',#19692,#19627,#15535,.T.);
#24959=EDGE_CURVE('',#19627,#19693,#10581,.T.);
#24960=EDGE_CURVE('',#19694,#19693,#15536,.T.);
#24961=EDGE_CURVE('',#19694,#19695,#15537,.T.);
#24962=EDGE_CURVE('',#19695,#19691,#10582,.T.);
#24963=EDGE_CURVE('',#19693,#19690,#10583,.T.);
#24964=EDGE_CURVE('',#19689,#19694,#1858,.T.);
#24965=EDGE_CURVE('',#17295,#19626,#1048,.T.);
#24966=EDGE_CURVE('',#19696,#19697,#15538,.T.);
#24967=EDGE_CURVE('',#19696,#19692,#1859,.T.);
#24968=EDGE_CURVE('',#19691,#19697,#10584,.T.);
#24969=EDGE_CURVE('',#19698,#19699,#15539,.T.);
#24970=EDGE_CURVE('',#19699,#19696,#15540,.T.);
#24971=EDGE_CURVE('',#19697,#19698,#15541,.T.);
#24972=EDGE_CURVE('',#19700,#19701,#15542,.T.);
#24973=EDGE_CURVE('',#19701,#19636,#15543,.T.);
#24974=EDGE_CURVE('',#19636,#19702,#10585,.T.);
#24975=EDGE_CURVE('',#19703,#19702,#15544,.T.);
#24976=EDGE_CURVE('',#19703,#19704,#15545,.T.);
#24977=EDGE_CURVE('',#19704,#19700,#10586,.T.);
#24978=EDGE_CURVE('',#19702,#19699,#10587,.T.);
#24979=EDGE_CURVE('',#19698,#19703,#1860,.T.);
#24980=EDGE_CURVE('',#19705,#19706,#15546,.T.);
#24981=EDGE_CURVE('',#19705,#19701,#1861,.T.);
#24982=EDGE_CURVE('',#19700,#19706,#10588,.T.);
#24983=EDGE_CURVE('',#19707,#19708,#15547,.T.);
#24984=EDGE_CURVE('',#19708,#19705,#15548,.T.);
#24985=EDGE_CURVE('',#19706,#19707,#15549,.T.);
#24986=EDGE_CURVE('',#19709,#19710,#1862,.T.);
#24987=EDGE_CURVE('',#19710,#19645,#1863,.T.);
#24988=EDGE_CURVE('',#19645,#19711,#10589,.T.);
#24989=EDGE_CURVE('',#19712,#19711,#15550,.T.);
#24990=EDGE_CURVE('',#19712,#19713,#15551,.T.);
#24991=EDGE_CURVE('',#19713,#19709,#10590,.T.);
#24992=EDGE_CURVE('',#19711,#19708,#10591,.T.);
#24993=EDGE_CURVE('',#19707,#19712,#1864,.T.);
#24994=EDGE_CURVE('',#19714,#19715,#1865,.T.);
#24995=EDGE_CURVE('',#19714,#19710,#1866,.T.);
#24996=EDGE_CURVE('',#19709,#19715,#10592,.T.);
#24997=EDGE_CURVE('',#19716,#19717,#15552,.T.);
#24998=EDGE_CURVE('',#19717,#19714,#1867,.T.);
#24999=EDGE_CURVE('',#19715,#19716,#15553,.T.);
#25000=EDGE_CURVE('',#19718,#19719,#15554,.T.);
#25001=EDGE_CURVE('',#19719,#19654,#15555,.T.);
#25002=EDGE_CURVE('',#19654,#19720,#10593,.T.);
#25003=EDGE_CURVE('',#19721,#19720,#15556,.T.);
#25004=EDGE_CURVE('',#19721,#19722,#15557,.T.);
#25005=EDGE_CURVE('',#19722,#19718,#10594,.T.);
#25006=EDGE_CURVE('',#19720,#19717,#10595,.T.);
#25007=EDGE_CURVE('',#19716,#19721,#1868,.T.);
#25008=EDGE_CURVE('',#19723,#19724,#15558,.T.);
#25009=EDGE_CURVE('',#19723,#19719,#1869,.T.);
#25010=EDGE_CURVE('',#19718,#19724,#10596,.T.);
#25011=EDGE_CURVE('',#19725,#19726,#15559,.T.);
#25012=EDGE_CURVE('',#19726,#19723,#15560,.T.);
#25013=EDGE_CURVE('',#19724,#19725,#15561,.T.);
#25014=EDGE_CURVE('',#19727,#19728,#15562,.T.);
#25015=EDGE_CURVE('',#19728,#19663,#15563,.T.);
#25016=EDGE_CURVE('',#19663,#19729,#10597,.T.);
#25017=EDGE_CURVE('',#19730,#19729,#15564,.T.);
#25018=EDGE_CURVE('',#19730,#19731,#15565,.T.);
#25019=EDGE_CURVE('',#19731,#19727,#10598,.T.);
#25020=EDGE_CURVE('',#19729,#19726,#10599,.T.);
#25021=EDGE_CURVE('',#19725,#19730,#1870,.T.);
#25022=EDGE_CURVE('',#19732,#19733,#15566,.T.);
#25023=EDGE_CURVE('',#19732,#19728,#1871,.T.);
#25024=EDGE_CURVE('',#19727,#19733,#10600,.T.);
#25025=EDGE_CURVE('',#19734,#19735,#15567,.T.);
#25026=EDGE_CURVE('',#19735,#19732,#15568,.T.);
#25027=EDGE_CURVE('',#19733,#19734,#15569,.T.);
#25028=EDGE_CURVE('',#19736,#19737,#15570,.T.);
#25029=EDGE_CURVE('',#19737,#19672,#15571,.T.);
#25030=EDGE_CURVE('',#19672,#19738,#10601,.T.);
#25031=EDGE_CURVE('',#19739,#19738,#15572,.T.);
#25032=EDGE_CURVE('',#19739,#19740,#15573,.T.);
#25033=EDGE_CURVE('',#19740,#19736,#10602,.F.);
#25034=EDGE_CURVE('',#19738,#19735,#10603,.T.);
#25035=EDGE_CURVE('',#19734,#19739,#1872,.T.);
#25036=EDGE_CURVE('',#17468,#19737,#15574,.T.);
#25037=EDGE_CURVE('',#19736,#17469,#10604,.F.);
#25038=EDGE_CURVE('',#17465,#19681,#1049,.T.);
#25039=EDGE_CURVE('',#19681,#19741,#10605,.T.);
#25040=EDGE_CURVE('',#17466,#19741,#1050,.T.);
#25041=EDGE_CURVE('',#19741,#17467,#1051,.T.);
#25042=EDGE_CURVE('',#19742,#19743,#15575,.T.);
#25043=EDGE_CURVE('',#19743,#17289,#15576,.T.);
#25044=EDGE_CURVE('',#19744,#17288,#1873,.T.);
#25045=EDGE_CURVE('',#19744,#19745,#1052,.T.);
#25046=EDGE_CURVE('',#19745,#19742,#10606,.T.);
#25047=EDGE_CURVE('',#19746,#19747,#15577,.T.);
#25048=EDGE_CURVE('',#19746,#19743,#1874,.T.);
#25049=EDGE_CURVE('',#19742,#19747,#10607,.T.);
#25050=EDGE_CURVE('',#19748,#19749,#15578,.T.);
#25051=EDGE_CURVE('',#19749,#19746,#15579,.T.);
#25052=EDGE_CURVE('',#19747,#19748,#15580,.T.);
#25053=EDGE_CURVE('',#19750,#19751,#15581,.T.);
#25054=EDGE_CURVE('',#19751,#19686,#15582,.T.);
#25055=EDGE_CURVE('',#19686,#19752,#10608,.T.);
#25056=EDGE_CURVE('',#19753,#19752,#15583,.T.);
#25057=EDGE_CURVE('',#19753,#19754,#15584,.T.);
#25058=EDGE_CURVE('',#19754,#19750,#10609,.T.);
#25059=EDGE_CURVE('',#19752,#19749,#10610,.T.);
#25060=EDGE_CURVE('',#19748,#19753,#1875,.T.);
#25061=EDGE_CURVE('',#17291,#19685,#1053,.T.);
#25062=EDGE_CURVE('',#19755,#19756,#15585,.T.);
#25063=EDGE_CURVE('',#19755,#19751,#1876,.T.);
#25064=EDGE_CURVE('',#19750,#19756,#10611,.T.);
#25065=EDGE_CURVE('',#19757,#19758,#15586,.T.);
#25066=EDGE_CURVE('',#19758,#19755,#15587,.T.);
#25067=EDGE_CURVE('',#19756,#19757,#15588,.T.);
#25068=EDGE_CURVE('',#19759,#19760,#15589,.T.);
#25069=EDGE_CURVE('',#19760,#19695,#15590,.T.);
#25070=EDGE_CURVE('',#19695,#19761,#10612,.T.);
#25071=EDGE_CURVE('',#19762,#19761,#15591,.T.);
#25072=EDGE_CURVE('',#19762,#19763,#15592,.T.);
#25073=EDGE_CURVE('',#19763,#19759,#10613,.T.);
#25074=EDGE_CURVE('',#19761,#19758,#10614,.T.);
#25075=EDGE_CURVE('',#19757,#19762,#1877,.T.);
#25076=EDGE_CURVE('',#19764,#19765,#15593,.T.);
#25077=EDGE_CURVE('',#19764,#19760,#1878,.T.);
#25078=EDGE_CURVE('',#19759,#19765,#10615,.T.);
#25079=EDGE_CURVE('',#19766,#19767,#15594,.T.);
#25080=EDGE_CURVE('',#19767,#19764,#15595,.T.);
#25081=EDGE_CURVE('',#19765,#19766,#15596,.T.);
#25082=EDGE_CURVE('',#19768,#19769,#1879,.T.);
#25083=EDGE_CURVE('',#19769,#19704,#1880,.T.);
#25084=EDGE_CURVE('',#19704,#19770,#10616,.T.);
#25085=EDGE_CURVE('',#19771,#19770,#15597,.T.);
#25086=EDGE_CURVE('',#19771,#19772,#15598,.T.);
#25087=EDGE_CURVE('',#19772,#19768,#10617,.T.);
#25088=EDGE_CURVE('',#19770,#19767,#10618,.T.);
#25089=EDGE_CURVE('',#19766,#19771,#1881,.T.);
#25090=EDGE_CURVE('',#19773,#19774,#1882,.T.);
#25091=EDGE_CURVE('',#19773,#19769,#1883,.T.);
#25092=EDGE_CURVE('',#19768,#19774,#10619,.T.);
#25093=EDGE_CURVE('',#19775,#19776,#15599,.T.);
#25094=EDGE_CURVE('',#19776,#19773,#1884,.T.);
#25095=EDGE_CURVE('',#19774,#19775,#15600,.T.);
#25096=EDGE_CURVE('',#19777,#19778,#15601,.T.);
#25097=EDGE_CURVE('',#19778,#19713,#15602,.T.);
#25098=EDGE_CURVE('',#19713,#19779,#10620,.T.);
#25099=EDGE_CURVE('',#19780,#19779,#15603,.T.);
#25100=EDGE_CURVE('',#19780,#19781,#15604,.T.);
#25101=EDGE_CURVE('',#19781,#19777,#10621,.T.);
#25102=EDGE_CURVE('',#19779,#19776,#10622,.T.);
#25103=EDGE_CURVE('',#19775,#19780,#1885,.T.);
#25104=EDGE_CURVE('',#19782,#19783,#15605,.T.);
#25105=EDGE_CURVE('',#19782,#19778,#1886,.T.);
#25106=EDGE_CURVE('',#19777,#19783,#10623,.T.);
#25107=EDGE_CURVE('',#19784,#19785,#15606,.T.);
#25108=EDGE_CURVE('',#19785,#19782,#15607,.T.);
#25109=EDGE_CURVE('',#19783,#19784,#15608,.T.);
#25110=EDGE_CURVE('',#19786,#19787,#15609,.T.);
#25111=EDGE_CURVE('',#19787,#19722,#15610,.T.);
#25112=EDGE_CURVE('',#19722,#19788,#10624,.T.);
#25113=EDGE_CURVE('',#19789,#19788,#15611,.T.);
#25114=EDGE_CURVE('',#19789,#19790,#15612,.T.);
#25115=EDGE_CURVE('',#19790,#19786,#10625,.T.);
#25116=EDGE_CURVE('',#19788,#19785,#10626,.T.);
#25117=EDGE_CURVE('',#19784,#19789,#1887,.T.);
#25118=EDGE_CURVE('',#19791,#19792,#15613,.T.);
#25119=EDGE_CURVE('',#19791,#19787,#1888,.T.);
#25120=EDGE_CURVE('',#19786,#19792,#10627,.T.);
#25121=EDGE_CURVE('',#19793,#19794,#15614,.T.);
#25122=EDGE_CURVE('',#19794,#19791,#15615,.T.);
#25123=EDGE_CURVE('',#19792,#19793,#15616,.T.);
#25124=EDGE_CURVE('',#19795,#19796,#15617,.T.);
#25125=EDGE_CURVE('',#19796,#19731,#15618,.T.);
#25126=EDGE_CURVE('',#19731,#19797,#10628,.T.);
#25127=EDGE_CURVE('',#19798,#19797,#15619,.T.);
#25128=EDGE_CURVE('',#19798,#19799,#15620,.T.);
#25129=EDGE_CURVE('',#19799,#19795,#10629,.F.);
#25130=EDGE_CURVE('',#19797,#19794,#10630,.T.);
#25131=EDGE_CURVE('',#19793,#19798,#1889,.T.);
#25132=EDGE_CURVE('',#17474,#19796,#15621,.T.);
#25133=EDGE_CURVE('',#19795,#17475,#10631,.F.);
#25134=EDGE_CURVE('',#17471,#19740,#1054,.T.);
#25135=EDGE_CURVE('',#19740,#19800,#10632,.T.);
#25136=EDGE_CURVE('',#17472,#19800,#1055,.T.);
#25137=EDGE_CURVE('',#19800,#17473,#1056,.T.);
#25138=EDGE_CURVE('',#19801,#19802,#15622,.T.);
#25139=EDGE_CURVE('',#19802,#17285,#15623,.T.);
#25140=EDGE_CURVE('',#19803,#17284,#1890,.T.);
#25141=EDGE_CURVE('',#19803,#19804,#1057,.T.);
#25142=EDGE_CURVE('',#19804,#19801,#10633,.T.);
#25143=EDGE_CURVE('',#19805,#19806,#15624,.T.);
#25144=EDGE_CURVE('',#19805,#19802,#1891,.T.);
#25145=EDGE_CURVE('',#19801,#19806,#10634,.T.);
#25146=EDGE_CURVE('',#19807,#19808,#15625,.T.);
#25147=EDGE_CURVE('',#19808,#19805,#15626,.T.);
#25148=EDGE_CURVE('',#19806,#19807,#15627,.T.);
#25149=EDGE_CURVE('',#19809,#19810,#15628,.T.);
#25150=EDGE_CURVE('',#19810,#19745,#15629,.T.);
#25151=EDGE_CURVE('',#19745,#19811,#10635,.T.);
#25152=EDGE_CURVE('',#19812,#19811,#15630,.T.);
#25153=EDGE_CURVE('',#19812,#19813,#15631,.T.);
#25154=EDGE_CURVE('',#19813,#19809,#10636,.T.);
#25155=EDGE_CURVE('',#19811,#19808,#10637,.T.);
#25156=EDGE_CURVE('',#19807,#19812,#1892,.T.);
#25157=EDGE_CURVE('',#17287,#19744,#1058,.T.);
#25158=EDGE_CURVE('',#19814,#19815,#15632,.T.);
#25159=EDGE_CURVE('',#19814,#19810,#1893,.T.);
#25160=EDGE_CURVE('',#19809,#19815,#10638,.T.);
#25161=EDGE_CURVE('',#19816,#19817,#15633,.T.);
#25162=EDGE_CURVE('',#19817,#19814,#15634,.T.);
#25163=EDGE_CURVE('',#19815,#19816,#15635,.T.);
#25164=EDGE_CURVE('',#19818,#19819,#15636,.T.);
#25165=EDGE_CURVE('',#19819,#19754,#15637,.T.);
#25166=EDGE_CURVE('',#19754,#19820,#10639,.T.);
#25167=EDGE_CURVE('',#19821,#19820,#15638,.T.);
#25168=EDGE_CURVE('',#19821,#19822,#15639,.T.);
#25169=EDGE_CURVE('',#19822,#19818,#10640,.T.);
#25170=EDGE_CURVE('',#19820,#19817,#10641,.T.);
#25171=EDGE_CURVE('',#19816,#19821,#1894,.T.);
#25172=EDGE_CURVE('',#19823,#19824,#15640,.T.);
#25173=EDGE_CURVE('',#19823,#19819,#1895,.T.);
#25174=EDGE_CURVE('',#19818,#19824,#10642,.T.);
#25175=EDGE_CURVE('',#19825,#19826,#15641,.T.);
#25176=EDGE_CURVE('',#19826,#19823,#15642,.T.);
#25177=EDGE_CURVE('',#19824,#19825,#15643,.T.);
#25178=EDGE_CURVE('',#19827,#19828,#1896,.T.);
#25179=EDGE_CURVE('',#19828,#19763,#1897,.T.);
#25180=EDGE_CURVE('',#19763,#19829,#10643,.T.);
#25181=EDGE_CURVE('',#19830,#19829,#15644,.T.);
#25182=EDGE_CURVE('',#19830,#19831,#15645,.T.);
#25183=EDGE_CURVE('',#19831,#19827,#10644,.T.);
#25184=EDGE_CURVE('',#19829,#19826,#10645,.T.);
#25185=EDGE_CURVE('',#19825,#19830,#1898,.T.);
#25186=EDGE_CURVE('',#19832,#19833,#1899,.T.);
#25187=EDGE_CURVE('',#19832,#19828,#1900,.T.);
#25188=EDGE_CURVE('',#19827,#19833,#10646,.T.);
#25189=EDGE_CURVE('',#19834,#19835,#15646,.T.);
#25190=EDGE_CURVE('',#19835,#19832,#1901,.T.);
#25191=EDGE_CURVE('',#19833,#19834,#15647,.T.);
#25192=EDGE_CURVE('',#19836,#19837,#15648,.T.);
#25193=EDGE_CURVE('',#19837,#19772,#15649,.T.);
#25194=EDGE_CURVE('',#19772,#19838,#10647,.T.);
#25195=EDGE_CURVE('',#19839,#19838,#15650,.T.);
#25196=EDGE_CURVE('',#19839,#19840,#15651,.T.);
#25197=EDGE_CURVE('',#19840,#19836,#10648,.T.);
#25198=EDGE_CURVE('',#19838,#19835,#10649,.T.);
#25199=EDGE_CURVE('',#19834,#19839,#1902,.T.);
#25200=EDGE_CURVE('',#19841,#19842,#15652,.T.);
#25201=EDGE_CURVE('',#19841,#19837,#1903,.T.);
#25202=EDGE_CURVE('',#19836,#19842,#10650,.T.);
#25203=EDGE_CURVE('',#19843,#19844,#15653,.T.);
#25204=EDGE_CURVE('',#19844,#19841,#15654,.T.);
#25205=EDGE_CURVE('',#19842,#19843,#15655,.T.);
#25206=EDGE_CURVE('',#19845,#19846,#15656,.T.);
#25207=EDGE_CURVE('',#19846,#19781,#15657,.T.);
#25208=EDGE_CURVE('',#19781,#19847,#10651,.T.);
#25209=EDGE_CURVE('',#19848,#19847,#15658,.T.);
#25210=EDGE_CURVE('',#19848,#19849,#15659,.T.);
#25211=EDGE_CURVE('',#19849,#19845,#10652,.T.);
#25212=EDGE_CURVE('',#19847,#19844,#10653,.T.);
#25213=EDGE_CURVE('',#19843,#19848,#1904,.T.);
#25214=EDGE_CURVE('',#19850,#19851,#15660,.T.);
#25215=EDGE_CURVE('',#19850,#19846,#1905,.T.);
#25216=EDGE_CURVE('',#19845,#19851,#10654,.T.);
#25217=EDGE_CURVE('',#19852,#19853,#15661,.T.);
#25218=EDGE_CURVE('',#19853,#19850,#15662,.T.);
#25219=EDGE_CURVE('',#19851,#19852,#15663,.T.);
#25220=EDGE_CURVE('',#19854,#19855,#15664,.T.);
#25221=EDGE_CURVE('',#19855,#19790,#15665,.T.);
#25222=EDGE_CURVE('',#19790,#19856,#10655,.T.);
#25223=EDGE_CURVE('',#19857,#19856,#15666,.T.);
#25224=EDGE_CURVE('',#19857,#19858,#15667,.T.);
#25225=EDGE_CURVE('',#19858,#19854,#10656,.F.);
#25226=EDGE_CURVE('',#19856,#19853,#10657,.T.);
#25227=EDGE_CURVE('',#19852,#19857,#1906,.T.);
#25228=EDGE_CURVE('',#17480,#19855,#15668,.T.);
#25229=EDGE_CURVE('',#19854,#17481,#10658,.F.);
#25230=EDGE_CURVE('',#17477,#19799,#1059,.T.);
#25231=EDGE_CURVE('',#19799,#19859,#10659,.T.);
#25232=EDGE_CURVE('',#17478,#19859,#1060,.T.);
#25233=EDGE_CURVE('',#19859,#17479,#1061,.T.);
#25234=EDGE_CURVE('',#19860,#19861,#15669,.T.);
#25235=EDGE_CURVE('',#19861,#17281,#15670,.T.);
#25236=EDGE_CURVE('',#19862,#17280,#1907,.T.);
#25237=EDGE_CURVE('',#19862,#19863,#1062,.T.);
#25238=EDGE_CURVE('',#19863,#19860,#10660,.T.);
#25239=EDGE_CURVE('',#19864,#19865,#15671,.T.);
#25240=EDGE_CURVE('',#19864,#19861,#1908,.T.);
#25241=EDGE_CURVE('',#19860,#19865,#10661,.T.);
#25242=EDGE_CURVE('',#19866,#19867,#15672,.T.);
#25243=EDGE_CURVE('',#19867,#19864,#15673,.T.);
#25244=EDGE_CURVE('',#19865,#19866,#15674,.T.);
#25245=EDGE_CURVE('',#19868,#19869,#15675,.T.);
#25246=EDGE_CURVE('',#19869,#19804,#15676,.T.);
#25247=EDGE_CURVE('',#19804,#19870,#10662,.T.);
#25248=EDGE_CURVE('',#19871,#19870,#15677,.T.);
#25249=EDGE_CURVE('',#19871,#19872,#15678,.T.);
#25250=EDGE_CURVE('',#19872,#19868,#10663,.T.);
#25251=EDGE_CURVE('',#19870,#19867,#10664,.T.);
#25252=EDGE_CURVE('',#19866,#19871,#1909,.T.);
#25253=EDGE_CURVE('',#17283,#19803,#1063,.T.);
#25254=EDGE_CURVE('',#19873,#19874,#15679,.T.);
#25255=EDGE_CURVE('',#19873,#19869,#1910,.T.);
#25256=EDGE_CURVE('',#19868,#19874,#10665,.T.);
#25257=EDGE_CURVE('',#19875,#19876,#15680,.T.);
#25258=EDGE_CURVE('',#19876,#19873,#15681,.T.);
#25259=EDGE_CURVE('',#19874,#19875,#15682,.T.);
#25260=EDGE_CURVE('',#19877,#19878,#15683,.T.);
#25261=EDGE_CURVE('',#19878,#19813,#15684,.T.);
#25262=EDGE_CURVE('',#19813,#19879,#10666,.T.);
#25263=EDGE_CURVE('',#19880,#19879,#15685,.T.);
#25264=EDGE_CURVE('',#19880,#19881,#15686,.T.);
#25265=EDGE_CURVE('',#19881,#19877,#10667,.T.);
#25266=EDGE_CURVE('',#19879,#19876,#10668,.T.);
#25267=EDGE_CURVE('',#19875,#19880,#1911,.T.);
#25268=EDGE_CURVE('',#19882,#19883,#15687,.T.);
#25269=EDGE_CURVE('',#19882,#19878,#1912,.T.);
#25270=EDGE_CURVE('',#19877,#19883,#10669,.T.);
#25271=EDGE_CURVE('',#19884,#19885,#15688,.T.);
#25272=EDGE_CURVE('',#19885,#19882,#15689,.T.);
#25273=EDGE_CURVE('',#19883,#19884,#15690,.T.);
#25274=EDGE_CURVE('',#19886,#19887,#1913,.T.);
#25275=EDGE_CURVE('',#19887,#19822,#1914,.T.);
#25276=EDGE_CURVE('',#19822,#19888,#10670,.T.);
#25277=EDGE_CURVE('',#19889,#19888,#15691,.T.);
#25278=EDGE_CURVE('',#19889,#19890,#15692,.T.);
#25279=EDGE_CURVE('',#19890,#19886,#10671,.T.);
#25280=EDGE_CURVE('',#19888,#19885,#10672,.T.);
#25281=EDGE_CURVE('',#19884,#19889,#1915,.T.);
#25282=EDGE_CURVE('',#19891,#19892,#1916,.T.);
#25283=EDGE_CURVE('',#19891,#19887,#1917,.T.);
#25284=EDGE_CURVE('',#19886,#19892,#10673,.T.);
#25285=EDGE_CURVE('',#19893,#19894,#15693,.T.);
#25286=EDGE_CURVE('',#19894,#19891,#1918,.T.);
#25287=EDGE_CURVE('',#19892,#19893,#15694,.T.);
#25288=EDGE_CURVE('',#19895,#19896,#15695,.T.);
#25289=EDGE_CURVE('',#19896,#19831,#15696,.T.);
#25290=EDGE_CURVE('',#19831,#19897,#10674,.T.);
#25291=EDGE_CURVE('',#19898,#19897,#15697,.T.);
#25292=EDGE_CURVE('',#19898,#19899,#15698,.T.);
#25293=EDGE_CURVE('',#19899,#19895,#10675,.T.);
#25294=EDGE_CURVE('',#19897,#19894,#10676,.T.);
#25295=EDGE_CURVE('',#19893,#19898,#1919,.T.);
#25296=EDGE_CURVE('',#19900,#19901,#15699,.T.);
#25297=EDGE_CURVE('',#19900,#19896,#1920,.T.);
#25298=EDGE_CURVE('',#19895,#19901,#10677,.T.);
#25299=EDGE_CURVE('',#19902,#19903,#15700,.T.);
#25300=EDGE_CURVE('',#19903,#19900,#15701,.T.);
#25301=EDGE_CURVE('',#19901,#19902,#15702,.T.);
#25302=EDGE_CURVE('',#19904,#19905,#15703,.T.);
#25303=EDGE_CURVE('',#19905,#19840,#15704,.T.);
#25304=EDGE_CURVE('',#19840,#19906,#10678,.T.);
#25305=EDGE_CURVE('',#19907,#19906,#15705,.T.);
#25306=EDGE_CURVE('',#19907,#19908,#15706,.T.);
#25307=EDGE_CURVE('',#19908,#19904,#10679,.T.);
#25308=EDGE_CURVE('',#19906,#19903,#10680,.T.);
#25309=EDGE_CURVE('',#19902,#19907,#1921,.T.);
#25310=EDGE_CURVE('',#19909,#19910,#15707,.T.);
#25311=EDGE_CURVE('',#19909,#19905,#1922,.T.);
#25312=EDGE_CURVE('',#19904,#19910,#10681,.T.);
#25313=EDGE_CURVE('',#19911,#19912,#15708,.T.);
#25314=EDGE_CURVE('',#19912,#19909,#15709,.T.);
#25315=EDGE_CURVE('',#19910,#19911,#15710,.T.);
#25316=EDGE_CURVE('',#19913,#19914,#15711,.T.);
#25317=EDGE_CURVE('',#19914,#19849,#15712,.T.);
#25318=EDGE_CURVE('',#19849,#19915,#10682,.T.);
#25319=EDGE_CURVE('',#19916,#19915,#15713,.T.);
#25320=EDGE_CURVE('',#19916,#19917,#15714,.T.);
#25321=EDGE_CURVE('',#19917,#19913,#10683,.F.);
#25322=EDGE_CURVE('',#19915,#19912,#10684,.T.);
#25323=EDGE_CURVE('',#19911,#19916,#1923,.T.);
#25324=EDGE_CURVE('',#17486,#19914,#15715,.T.);
#25325=EDGE_CURVE('',#19913,#17487,#10685,.F.);
#25326=EDGE_CURVE('',#17483,#19858,#1064,.T.);
#25327=EDGE_CURVE('',#19858,#19918,#10686,.T.);
#25328=EDGE_CURVE('',#17484,#19918,#1065,.T.);
#25329=EDGE_CURVE('',#19918,#17485,#1066,.T.);
#25330=EDGE_CURVE('',#19919,#19920,#15716,.T.);
#25331=EDGE_CURVE('',#19920,#17277,#15717,.T.);
#25332=EDGE_CURVE('',#19921,#17276,#1924,.T.);
#25333=EDGE_CURVE('',#19921,#19922,#1067,.T.);
#25334=EDGE_CURVE('',#19922,#19919,#10687,.T.);
#25335=EDGE_CURVE('',#19923,#19924,#15718,.T.);
#25336=EDGE_CURVE('',#19923,#19920,#1925,.T.);
#25337=EDGE_CURVE('',#19919,#19924,#10688,.T.);
#25338=EDGE_CURVE('',#19925,#19926,#15719,.T.);
#25339=EDGE_CURVE('',#19926,#19923,#15720,.T.);
#25340=EDGE_CURVE('',#19924,#19925,#15721,.T.);
#25341=EDGE_CURVE('',#19927,#19928,#15722,.T.);
#25342=EDGE_CURVE('',#19928,#19863,#15723,.T.);
#25343=EDGE_CURVE('',#19863,#19929,#10689,.T.);
#25344=EDGE_CURVE('',#19930,#19929,#15724,.T.);
#25345=EDGE_CURVE('',#19930,#19931,#15725,.T.);
#25346=EDGE_CURVE('',#19931,#19927,#10690,.T.);
#25347=EDGE_CURVE('',#19929,#19926,#10691,.T.);
#25348=EDGE_CURVE('',#19925,#19930,#1926,.T.);
#25349=EDGE_CURVE('',#17279,#19862,#1068,.T.);
#25350=EDGE_CURVE('',#19932,#19933,#15726,.T.);
#25351=EDGE_CURVE('',#19932,#19928,#1927,.T.);
#25352=EDGE_CURVE('',#19927,#19933,#10692,.T.);
#25353=EDGE_CURVE('',#19934,#19935,#15727,.T.);
#25354=EDGE_CURVE('',#19935,#19932,#15728,.T.);
#25355=EDGE_CURVE('',#19933,#19934,#15729,.T.);
#25356=EDGE_CURVE('',#19936,#19937,#15730,.T.);
#25357=EDGE_CURVE('',#19937,#19872,#15731,.T.);
#25358=EDGE_CURVE('',#19872,#19938,#10693,.T.);
#25359=EDGE_CURVE('',#19939,#19938,#15732,.T.);
#25360=EDGE_CURVE('',#19939,#19940,#15733,.T.);
#25361=EDGE_CURVE('',#19940,#19936,#10694,.T.);
#25362=EDGE_CURVE('',#19938,#19935,#10695,.T.);
#25363=EDGE_CURVE('',#19934,#19939,#1928,.T.);
#25364=EDGE_CURVE('',#19941,#19942,#15734,.T.);
#25365=EDGE_CURVE('',#19941,#19937,#1929,.T.);
#25366=EDGE_CURVE('',#19936,#19942,#10696,.T.);
#25367=EDGE_CURVE('',#19943,#19944,#15735,.T.);
#25368=EDGE_CURVE('',#19944,#19941,#15736,.T.);
#25369=EDGE_CURVE('',#19942,#19943,#15737,.T.);
#25370=EDGE_CURVE('',#19945,#19946,#1930,.T.);
#25371=EDGE_CURVE('',#19946,#19881,#1931,.T.);
#25372=EDGE_CURVE('',#19881,#19947,#10697,.T.);
#25373=EDGE_CURVE('',#19948,#19947,#15738,.T.);
#25374=EDGE_CURVE('',#19948,#19949,#15739,.T.);
#25375=EDGE_CURVE('',#19949,#19945,#10698,.T.);
#25376=EDGE_CURVE('',#19947,#19944,#10699,.T.);
#25377=EDGE_CURVE('',#19943,#19948,#1932,.T.);
#25378=EDGE_CURVE('',#19950,#19951,#1933,.T.);
#25379=EDGE_CURVE('',#19950,#19946,#1934,.T.);
#25380=EDGE_CURVE('',#19945,#19951,#10700,.T.);
#25381=EDGE_CURVE('',#19952,#19953,#15740,.T.);
#25382=EDGE_CURVE('',#19953,#19950,#1935,.T.);
#25383=EDGE_CURVE('',#19951,#19952,#15741,.T.);
#25384=EDGE_CURVE('',#19954,#19955,#15742,.T.);
#25385=EDGE_CURVE('',#19955,#19890,#15743,.T.);
#25386=EDGE_CURVE('',#19890,#19956,#10701,.T.);
#25387=EDGE_CURVE('',#19957,#19956,#15744,.T.);
#25388=EDGE_CURVE('',#19957,#19958,#15745,.T.);
#25389=EDGE_CURVE('',#19958,#19954,#10702,.T.);
#25390=EDGE_CURVE('',#19956,#19953,#10703,.T.);
#25391=EDGE_CURVE('',#19952,#19957,#1936,.T.);
#25392=EDGE_CURVE('',#19959,#19960,#15746,.T.);
#25393=EDGE_CURVE('',#19959,#19955,#1937,.T.);
#25394=EDGE_CURVE('',#19954,#19960,#10704,.T.);
#25395=EDGE_CURVE('',#19961,#19962,#15747,.T.);
#25396=EDGE_CURVE('',#19962,#19959,#15748,.T.);
#25397=EDGE_CURVE('',#19960,#19961,#15749,.T.);
#25398=EDGE_CURVE('',#19963,#19964,#15750,.T.);
#25399=EDGE_CURVE('',#19964,#19899,#15751,.T.);
#25400=EDGE_CURVE('',#19899,#19965,#10705,.T.);
#25401=EDGE_CURVE('',#19966,#19965,#15752,.T.);
#25402=EDGE_CURVE('',#19966,#19967,#15753,.T.);
#25403=EDGE_CURVE('',#19967,#19963,#10706,.T.);
#25404=EDGE_CURVE('',#19965,#19962,#10707,.T.);
#25405=EDGE_CURVE('',#19961,#19966,#1938,.T.);
#25406=EDGE_CURVE('',#19968,#19969,#15754,.T.);
#25407=EDGE_CURVE('',#19968,#19964,#1939,.T.);
#25408=EDGE_CURVE('',#19963,#19969,#10708,.T.);
#25409=EDGE_CURVE('',#19970,#19971,#15755,.T.);
#25410=EDGE_CURVE('',#19971,#19968,#15756,.T.);
#25411=EDGE_CURVE('',#19969,#19970,#15757,.T.);
#25412=EDGE_CURVE('',#19972,#19973,#15758,.T.);
#25413=EDGE_CURVE('',#19973,#19908,#15759,.T.);
#25414=EDGE_CURVE('',#19908,#19974,#10709,.T.);
#25415=EDGE_CURVE('',#19975,#19974,#15760,.T.);
#25416=EDGE_CURVE('',#19975,#19976,#15761,.T.);
#25417=EDGE_CURVE('',#19976,#19972,#10710,.F.);
#25418=EDGE_CURVE('',#19974,#19971,#10711,.T.);
#25419=EDGE_CURVE('',#19970,#19975,#1940,.T.);
#25420=EDGE_CURVE('',#17492,#19973,#15762,.T.);
#25421=EDGE_CURVE('',#19972,#17493,#10712,.F.);
#25422=EDGE_CURVE('',#17489,#19917,#1069,.T.);
#25423=EDGE_CURVE('',#19917,#19977,#10713,.T.);
#25424=EDGE_CURVE('',#17490,#19977,#1070,.T.);
#25425=EDGE_CURVE('',#19977,#17491,#1071,.T.);
#25426=EDGE_CURVE('',#19978,#19979,#15763,.T.);
#25427=EDGE_CURVE('',#19979,#17273,#15764,.T.);
#25428=EDGE_CURVE('',#19980,#17272,#1941,.T.);
#25429=EDGE_CURVE('',#19980,#19981,#1072,.T.);
#25430=EDGE_CURVE('',#19981,#19978,#10714,.T.);
#25431=EDGE_CURVE('',#19982,#19983,#15765,.T.);
#25432=EDGE_CURVE('',#19982,#19979,#1942,.T.);
#25433=EDGE_CURVE('',#19978,#19983,#10715,.T.);
#25434=EDGE_CURVE('',#19984,#19985,#15766,.T.);
#25435=EDGE_CURVE('',#19985,#19982,#15767,.T.);
#25436=EDGE_CURVE('',#19983,#19984,#15768,.T.);
#25437=EDGE_CURVE('',#19986,#19987,#15769,.T.);
#25438=EDGE_CURVE('',#19987,#19922,#15770,.T.);
#25439=EDGE_CURVE('',#19922,#19988,#10716,.T.);
#25440=EDGE_CURVE('',#19989,#19988,#15771,.T.);
#25441=EDGE_CURVE('',#19989,#19990,#15772,.T.);
#25442=EDGE_CURVE('',#19990,#19986,#10717,.T.);
#25443=EDGE_CURVE('',#19988,#19985,#10718,.T.);
#25444=EDGE_CURVE('',#19984,#19989,#1943,.T.);
#25445=EDGE_CURVE('',#17275,#19921,#1073,.T.);
#25446=EDGE_CURVE('',#19991,#19992,#15773,.T.);
#25447=EDGE_CURVE('',#19991,#19987,#1944,.T.);
#25448=EDGE_CURVE('',#19986,#19992,#10719,.T.);
#25449=EDGE_CURVE('',#19993,#19994,#15774,.T.);
#25450=EDGE_CURVE('',#19994,#19991,#15775,.T.);
#25451=EDGE_CURVE('',#19992,#19993,#15776,.T.);
#25452=EDGE_CURVE('',#19995,#19996,#15777,.T.);
#25453=EDGE_CURVE('',#19996,#19931,#15778,.T.);
#25454=EDGE_CURVE('',#19931,#19997,#10720,.T.);
#25455=EDGE_CURVE('',#19998,#19997,#15779,.T.);
#25456=EDGE_CURVE('',#19998,#19999,#15780,.T.);
#25457=EDGE_CURVE('',#19999,#19995,#10721,.T.);
#25458=EDGE_CURVE('',#19997,#19994,#10722,.T.);
#25459=EDGE_CURVE('',#19993,#19998,#1945,.T.);
#25460=EDGE_CURVE('',#20000,#20001,#15781,.T.);
#25461=EDGE_CURVE('',#20000,#19996,#1946,.T.);
#25462=EDGE_CURVE('',#19995,#20001,#10723,.T.);
#25463=EDGE_CURVE('',#20002,#20003,#15782,.T.);
#25464=EDGE_CURVE('',#20003,#20000,#15783,.T.);
#25465=EDGE_CURVE('',#20001,#20002,#15784,.T.);
#25466=EDGE_CURVE('',#20004,#20005,#1947,.T.);
#25467=EDGE_CURVE('',#20005,#19940,#1948,.T.);
#25468=EDGE_CURVE('',#19940,#20006,#10724,.T.);
#25469=EDGE_CURVE('',#20007,#20006,#15785,.T.);
#25470=EDGE_CURVE('',#20007,#20008,#15786,.T.);
#25471=EDGE_CURVE('',#20008,#20004,#10725,.T.);
#25472=EDGE_CURVE('',#20006,#20003,#10726,.T.);
#25473=EDGE_CURVE('',#20002,#20007,#1949,.T.);
#25474=EDGE_CURVE('',#20009,#20010,#1950,.T.);
#25475=EDGE_CURVE('',#20009,#20005,#1951,.T.);
#25476=EDGE_CURVE('',#20004,#20010,#10727,.T.);
#25477=EDGE_CURVE('',#20011,#20012,#15787,.T.);
#25478=EDGE_CURVE('',#20012,#20009,#1952,.T.);
#25479=EDGE_CURVE('',#20010,#20011,#15788,.T.);
#25480=EDGE_CURVE('',#20013,#20014,#15789,.T.);
#25481=EDGE_CURVE('',#20014,#19949,#15790,.T.);
#25482=EDGE_CURVE('',#19949,#20015,#10728,.T.);
#25483=EDGE_CURVE('',#20016,#20015,#15791,.T.);
#25484=EDGE_CURVE('',#20016,#20017,#15792,.T.);
#25485=EDGE_CURVE('',#20017,#20013,#10729,.T.);
#25486=EDGE_CURVE('',#20015,#20012,#10730,.T.);
#25487=EDGE_CURVE('',#20011,#20016,#1953,.T.);
#25488=EDGE_CURVE('',#20018,#20019,#15793,.T.);
#25489=EDGE_CURVE('',#20018,#20014,#1954,.T.);
#25490=EDGE_CURVE('',#20013,#20019,#10731,.T.);
#25491=EDGE_CURVE('',#20020,#20021,#15794,.T.);
#25492=EDGE_CURVE('',#20021,#20018,#15795,.T.);
#25493=EDGE_CURVE('',#20019,#20020,#15796,.T.);
#25494=EDGE_CURVE('',#20022,#20023,#15797,.T.);
#25495=EDGE_CURVE('',#20023,#19958,#15798,.T.);
#25496=EDGE_CURVE('',#19958,#20024,#10732,.T.);
#25497=EDGE_CURVE('',#20025,#20024,#15799,.T.);
#25498=EDGE_CURVE('',#20025,#20026,#15800,.T.);
#25499=EDGE_CURVE('',#20026,#20022,#10733,.T.);
#25500=EDGE_CURVE('',#20024,#20021,#10734,.T.);
#25501=EDGE_CURVE('',#20020,#20025,#1955,.T.);
#25502=EDGE_CURVE('',#20027,#20028,#15801,.T.);
#25503=EDGE_CURVE('',#20027,#20023,#1956,.T.);
#25504=EDGE_CURVE('',#20022,#20028,#10735,.T.);
#25505=EDGE_CURVE('',#20029,#20030,#15802,.T.);
#25506=EDGE_CURVE('',#20030,#20027,#15803,.T.);
#25507=EDGE_CURVE('',#20028,#20029,#15804,.T.);
#25508=EDGE_CURVE('',#20031,#20032,#15805,.T.);
#25509=EDGE_CURVE('',#20032,#19967,#15806,.T.);
#25510=EDGE_CURVE('',#19967,#20033,#10736,.T.);
#25511=EDGE_CURVE('',#20034,#20033,#15807,.T.);
#25512=EDGE_CURVE('',#20034,#20035,#15808,.T.);
#25513=EDGE_CURVE('',#20035,#20031,#10737,.F.);
#25514=EDGE_CURVE('',#20033,#20030,#10738,.T.);
#25515=EDGE_CURVE('',#20029,#20034,#1957,.T.);
#25516=EDGE_CURVE('',#17498,#20032,#15809,.T.);
#25517=EDGE_CURVE('',#20031,#17499,#10739,.F.);
#25518=EDGE_CURVE('',#17495,#19976,#1074,.T.);
#25519=EDGE_CURVE('',#19976,#20036,#10740,.T.);
#25520=EDGE_CURVE('',#17496,#20036,#1075,.T.);
#25521=EDGE_CURVE('',#20036,#17497,#1076,.T.);
#25522=EDGE_CURVE('',#20037,#20038,#15810,.T.);
#25523=EDGE_CURVE('',#20038,#17269,#15811,.T.);
#25524=EDGE_CURVE('',#20039,#17268,#1958,.T.);
#25525=EDGE_CURVE('',#20039,#20040,#1077,.T.);
#25526=EDGE_CURVE('',#20040,#20037,#10741,.T.);
#25527=EDGE_CURVE('',#20041,#20042,#15812,.T.);
#25528=EDGE_CURVE('',#20041,#20038,#1959,.T.);
#25529=EDGE_CURVE('',#20037,#20042,#10742,.T.);
#25530=EDGE_CURVE('',#20043,#20044,#15813,.T.);
#25531=EDGE_CURVE('',#20044,#20041,#15814,.T.);
#25532=EDGE_CURVE('',#20042,#20043,#15815,.T.);
#25533=EDGE_CURVE('',#20045,#20046,#15816,.T.);
#25534=EDGE_CURVE('',#20046,#19981,#15817,.T.);
#25535=EDGE_CURVE('',#19981,#20047,#10743,.T.);
#25536=EDGE_CURVE('',#20048,#20047,#15818,.T.);
#25537=EDGE_CURVE('',#20048,#20049,#15819,.T.);
#25538=EDGE_CURVE('',#20049,#20045,#10744,.T.);
#25539=EDGE_CURVE('',#20047,#20044,#10745,.T.);
#25540=EDGE_CURVE('',#20043,#20048,#1960,.T.);
#25541=EDGE_CURVE('',#17271,#19980,#1078,.T.);
#25542=EDGE_CURVE('',#20050,#20051,#15820,.T.);
#25543=EDGE_CURVE('',#20050,#20046,#1961,.T.);
#25544=EDGE_CURVE('',#20045,#20051,#10746,.T.);
#25545=EDGE_CURVE('',#20052,#20053,#15821,.T.);
#25546=EDGE_CURVE('',#20053,#20050,#15822,.T.);
#25547=EDGE_CURVE('',#20051,#20052,#15823,.T.);
#25548=EDGE_CURVE('',#20054,#20055,#15824,.T.);
#25549=EDGE_CURVE('',#20055,#19990,#15825,.T.);
#25550=EDGE_CURVE('',#19990,#20056,#10747,.T.);
#25551=EDGE_CURVE('',#20057,#20056,#15826,.T.);
#25552=EDGE_CURVE('',#20057,#20058,#15827,.T.);
#25553=EDGE_CURVE('',#20058,#20054,#10748,.T.);
#25554=EDGE_CURVE('',#20056,#20053,#10749,.T.);
#25555=EDGE_CURVE('',#20052,#20057,#1962,.T.);
#25556=EDGE_CURVE('',#20059,#20060,#15828,.T.);
#25557=EDGE_CURVE('',#20059,#20055,#1963,.T.);
#25558=EDGE_CURVE('',#20054,#20060,#10750,.T.);
#25559=EDGE_CURVE('',#20061,#20062,#15829,.T.);
#25560=EDGE_CURVE('',#20062,#20059,#15830,.T.);
#25561=EDGE_CURVE('',#20060,#20061,#15831,.T.);
#25562=EDGE_CURVE('',#20063,#20064,#1964,.T.);
#25563=EDGE_CURVE('',#20064,#19999,#1965,.T.);
#25564=EDGE_CURVE('',#19999,#20065,#10751,.T.);
#25565=EDGE_CURVE('',#20066,#20065,#15832,.T.);
#25566=EDGE_CURVE('',#20066,#20067,#15833,.T.);
#25567=EDGE_CURVE('',#20067,#20063,#10752,.T.);
#25568=EDGE_CURVE('',#20065,#20062,#10753,.T.);
#25569=EDGE_CURVE('',#20061,#20066,#1966,.T.);
#25570=EDGE_CURVE('',#20068,#20069,#1967,.T.);
#25571=EDGE_CURVE('',#20068,#20064,#1968,.T.);
#25572=EDGE_CURVE('',#20063,#20069,#10754,.T.);
#25573=EDGE_CURVE('',#20070,#20071,#15834,.T.);
#25574=EDGE_CURVE('',#20071,#20068,#1969,.T.);
#25575=EDGE_CURVE('',#20069,#20070,#15835,.T.);
#25576=EDGE_CURVE('',#20072,#20073,#15836,.T.);
#25577=EDGE_CURVE('',#20073,#20008,#15837,.T.);
#25578=EDGE_CURVE('',#20008,#20074,#10755,.T.);
#25579=EDGE_CURVE('',#20075,#20074,#15838,.T.);
#25580=EDGE_CURVE('',#20075,#20076,#15839,.T.);
#25581=EDGE_CURVE('',#20076,#20072,#10756,.T.);
#25582=EDGE_CURVE('',#20074,#20071,#10757,.T.);
#25583=EDGE_CURVE('',#20070,#20075,#1970,.T.);
#25584=EDGE_CURVE('',#20077,#20078,#15840,.T.);
#25585=EDGE_CURVE('',#20077,#20073,#1971,.T.);
#25586=EDGE_CURVE('',#20072,#20078,#10758,.T.);
#25587=EDGE_CURVE('',#20079,#20080,#15841,.T.);
#25588=EDGE_CURVE('',#20080,#20077,#15842,.T.);
#25589=EDGE_CURVE('',#20078,#20079,#15843,.T.);
#25590=EDGE_CURVE('',#20081,#20082,#15844,.T.);
#25591=EDGE_CURVE('',#20082,#20017,#15845,.T.);
#25592=EDGE_CURVE('',#20017,#20083,#10759,.T.);
#25593=EDGE_CURVE('',#20084,#20083,#15846,.T.);
#25594=EDGE_CURVE('',#20084,#20085,#15847,.T.);
#25595=EDGE_CURVE('',#20085,#20081,#10760,.T.);
#25596=EDGE_CURVE('',#20083,#20080,#10761,.T.);
#25597=EDGE_CURVE('',#20079,#20084,#1972,.T.);
#25598=EDGE_CURVE('',#20086,#20087,#15848,.T.);
#25599=EDGE_CURVE('',#20086,#20082,#1973,.T.);
#25600=EDGE_CURVE('',#20081,#20087,#10762,.T.);
#25601=EDGE_CURVE('',#20088,#20089,#15849,.T.);
#25602=EDGE_CURVE('',#20089,#20086,#15850,.T.);
#25603=EDGE_CURVE('',#20087,#20088,#15851,.T.);
#25604=EDGE_CURVE('',#20090,#20091,#15852,.T.);
#25605=EDGE_CURVE('',#20091,#20026,#15853,.T.);
#25606=EDGE_CURVE('',#20026,#20092,#10763,.T.);
#25607=EDGE_CURVE('',#20093,#20092,#15854,.T.);
#25608=EDGE_CURVE('',#20093,#20094,#15855,.T.);
#25609=EDGE_CURVE('',#20094,#20090,#10764,.F.);
#25610=EDGE_CURVE('',#20092,#20089,#10765,.T.);
#25611=EDGE_CURVE('',#20088,#20093,#1974,.T.);
#25612=EDGE_CURVE('',#17504,#20091,#15856,.T.);
#25613=EDGE_CURVE('',#20090,#17505,#10766,.F.);
#25614=EDGE_CURVE('',#17501,#20035,#1079,.T.);
#25615=EDGE_CURVE('',#20035,#20095,#10767,.T.);
#25616=EDGE_CURVE('',#17502,#20095,#1080,.T.);
#25617=EDGE_CURVE('',#20095,#17503,#1081,.T.);
#25618=EDGE_CURVE('',#20096,#20097,#15857,.T.);
#25619=EDGE_CURVE('',#20097,#17265,#15858,.T.);
#25620=EDGE_CURVE('',#20098,#17264,#1975,.T.);
#25621=EDGE_CURVE('',#20098,#20099,#1082,.T.);
#25622=EDGE_CURVE('',#20099,#20096,#10768,.T.);
#25623=EDGE_CURVE('',#20100,#20101,#15859,.T.);
#25624=EDGE_CURVE('',#20100,#20097,#1976,.T.);
#25625=EDGE_CURVE('',#20096,#20101,#10769,.T.);
#25626=EDGE_CURVE('',#20102,#20103,#15860,.T.);
#25627=EDGE_CURVE('',#20103,#20100,#15861,.T.);
#25628=EDGE_CURVE('',#20101,#20102,#15862,.T.);
#25629=EDGE_CURVE('',#20104,#20105,#15863,.T.);
#25630=EDGE_CURVE('',#20105,#20040,#15864,.T.);
#25631=EDGE_CURVE('',#20040,#20106,#10770,.T.);
#25632=EDGE_CURVE('',#20107,#20106,#15865,.T.);
#25633=EDGE_CURVE('',#20107,#20108,#15866,.T.);
#25634=EDGE_CURVE('',#20108,#20104,#10771,.T.);
#25635=EDGE_CURVE('',#20106,#20103,#10772,.T.);
#25636=EDGE_CURVE('',#20102,#20107,#1977,.T.);
#25637=EDGE_CURVE('',#17267,#20039,#1083,.T.);
#25638=EDGE_CURVE('',#20109,#20110,#15867,.T.);
#25639=EDGE_CURVE('',#20109,#20105,#1978,.T.);
#25640=EDGE_CURVE('',#20104,#20110,#10773,.T.);
#25641=EDGE_CURVE('',#20111,#20112,#15868,.T.);
#25642=EDGE_CURVE('',#20112,#20109,#15869,.T.);
#25643=EDGE_CURVE('',#20110,#20111,#15870,.T.);
#25644=EDGE_CURVE('',#20113,#20114,#15871,.T.);
#25645=EDGE_CURVE('',#20114,#20049,#15872,.T.);
#25646=EDGE_CURVE('',#20049,#20115,#10774,.T.);
#25647=EDGE_CURVE('',#20116,#20115,#15873,.T.);
#25648=EDGE_CURVE('',#20116,#20117,#15874,.T.);
#25649=EDGE_CURVE('',#20117,#20113,#10775,.T.);
#25650=EDGE_CURVE('',#20115,#20112,#10776,.T.);
#25651=EDGE_CURVE('',#20111,#20116,#1979,.T.);
#25652=EDGE_CURVE('',#20118,#20119,#15875,.T.);
#25653=EDGE_CURVE('',#20118,#20114,#1980,.T.);
#25654=EDGE_CURVE('',#20113,#20119,#10777,.T.);
#25655=EDGE_CURVE('',#20120,#20121,#15876,.T.);
#25656=EDGE_CURVE('',#20121,#20118,#15877,.T.);
#25657=EDGE_CURVE('',#20119,#20120,#15878,.T.);
#25658=EDGE_CURVE('',#20122,#20123,#1981,.T.);
#25659=EDGE_CURVE('',#20123,#20058,#1982,.T.);
#25660=EDGE_CURVE('',#20058,#20124,#10778,.T.);
#25661=EDGE_CURVE('',#20125,#20124,#15879,.T.);
#25662=EDGE_CURVE('',#20125,#20126,#15880,.T.);
#25663=EDGE_CURVE('',#20126,#20122,#10779,.T.);
#25664=EDGE_CURVE('',#20124,#20121,#10780,.T.);
#25665=EDGE_CURVE('',#20120,#20125,#1983,.T.);
#25666=EDGE_CURVE('',#20127,#20128,#1984,.T.);
#25667=EDGE_CURVE('',#20127,#20123,#1985,.T.);
#25668=EDGE_CURVE('',#20122,#20128,#10781,.T.);
#25669=EDGE_CURVE('',#20129,#20130,#15881,.T.);
#25670=EDGE_CURVE('',#20130,#20127,#1986,.T.);
#25671=EDGE_CURVE('',#20128,#20129,#15882,.T.);
#25672=EDGE_CURVE('',#20131,#20132,#15883,.T.);
#25673=EDGE_CURVE('',#20132,#20067,#15884,.T.);
#25674=EDGE_CURVE('',#20067,#20133,#10782,.T.);
#25675=EDGE_CURVE('',#20134,#20133,#15885,.T.);
#25676=EDGE_CURVE('',#20134,#20135,#15886,.T.);
#25677=EDGE_CURVE('',#20135,#20131,#10783,.T.);
#25678=EDGE_CURVE('',#20133,#20130,#10784,.T.);
#25679=EDGE_CURVE('',#20129,#20134,#1987,.T.);
#25680=EDGE_CURVE('',#20136,#20137,#15887,.T.);
#25681=EDGE_CURVE('',#20136,#20132,#1988,.T.);
#25682=EDGE_CURVE('',#20131,#20137,#10785,.T.);
#25683=EDGE_CURVE('',#20138,#20139,#15888,.T.);
#25684=EDGE_CURVE('',#20139,#20136,#15889,.T.);
#25685=EDGE_CURVE('',#20137,#20138,#15890,.T.);
#25686=EDGE_CURVE('',#20140,#20141,#15891,.T.);
#25687=EDGE_CURVE('',#20141,#20076,#15892,.T.);
#25688=EDGE_CURVE('',#20076,#20142,#10786,.T.);
#25689=EDGE_CURVE('',#20143,#20142,#15893,.T.);
#25690=EDGE_CURVE('',#20143,#20144,#15894,.T.);
#25691=EDGE_CURVE('',#20144,#20140,#10787,.T.);
#25692=EDGE_CURVE('',#20142,#20139,#10788,.T.);
#25693=EDGE_CURVE('',#20138,#20143,#1989,.T.);
#25694=EDGE_CURVE('',#20145,#20146,#15895,.T.);
#25695=EDGE_CURVE('',#20145,#20141,#1990,.T.);
#25696=EDGE_CURVE('',#20140,#20146,#10789,.T.);
#25697=EDGE_CURVE('',#20147,#20148,#15896,.T.);
#25698=EDGE_CURVE('',#20148,#20145,#15897,.T.);
#25699=EDGE_CURVE('',#20146,#20147,#15898,.T.);
#25700=EDGE_CURVE('',#20149,#20150,#15899,.T.);
#25701=EDGE_CURVE('',#20150,#20085,#15900,.T.);
#25702=EDGE_CURVE('',#20085,#20151,#10790,.T.);
#25703=EDGE_CURVE('',#20152,#20151,#15901,.T.);
#25704=EDGE_CURVE('',#20152,#20153,#15902,.T.);
#25705=EDGE_CURVE('',#20153,#20149,#10791,.F.);
#25706=EDGE_CURVE('',#20151,#20148,#10792,.T.);
#25707=EDGE_CURVE('',#20147,#20152,#1991,.T.);
#25708=EDGE_CURVE('',#17510,#20150,#15903,.T.);
#25709=EDGE_CURVE('',#20149,#17511,#10793,.F.);
#25710=EDGE_CURVE('',#17507,#20094,#1084,.T.);
#25711=EDGE_CURVE('',#20094,#20154,#10794,.T.);
#25712=EDGE_CURVE('',#17508,#20154,#1085,.T.);
#25713=EDGE_CURVE('',#20154,#17509,#1086,.T.);
#25714=EDGE_CURVE('',#20155,#20156,#15904,.T.);
#25715=EDGE_CURVE('',#20156,#17261,#15905,.T.);
#25716=EDGE_CURVE('',#20157,#17260,#1992,.T.);
#25717=EDGE_CURVE('',#20157,#20158,#1087,.T.);
#25718=EDGE_CURVE('',#20158,#20155,#10795,.T.);
#25719=EDGE_CURVE('',#20159,#20160,#15906,.T.);
#25720=EDGE_CURVE('',#20159,#20156,#1993,.T.);
#25721=EDGE_CURVE('',#20155,#20160,#10796,.T.);
#25722=EDGE_CURVE('',#20161,#20162,#15907,.T.);
#25723=EDGE_CURVE('',#20162,#20159,#15908,.T.);
#25724=EDGE_CURVE('',#20160,#20161,#15909,.T.);
#25725=EDGE_CURVE('',#20163,#20164,#15910,.T.);
#25726=EDGE_CURVE('',#20164,#20099,#15911,.T.);
#25727=EDGE_CURVE('',#20099,#20165,#10797,.T.);
#25728=EDGE_CURVE('',#20166,#20165,#15912,.T.);
#25729=EDGE_CURVE('',#20166,#20167,#15913,.T.);
#25730=EDGE_CURVE('',#20167,#20163,#10798,.T.);
#25731=EDGE_CURVE('',#20165,#20162,#10799,.T.);
#25732=EDGE_CURVE('',#20161,#20166,#1994,.T.);
#25733=EDGE_CURVE('',#17263,#20098,#1088,.T.);
#25734=EDGE_CURVE('',#20168,#20169,#15914,.T.);
#25735=EDGE_CURVE('',#20168,#20164,#1995,.T.);
#25736=EDGE_CURVE('',#20163,#20169,#10800,.T.);
#25737=EDGE_CURVE('',#20170,#20171,#15915,.T.);
#25738=EDGE_CURVE('',#20171,#20168,#15916,.T.);
#25739=EDGE_CURVE('',#20169,#20170,#15917,.T.);
#25740=EDGE_CURVE('',#20172,#20173,#15918,.T.);
#25741=EDGE_CURVE('',#20173,#20108,#15919,.T.);
#25742=EDGE_CURVE('',#20108,#20174,#10801,.T.);
#25743=EDGE_CURVE('',#20175,#20174,#15920,.T.);
#25744=EDGE_CURVE('',#20175,#20176,#15921,.T.);
#25745=EDGE_CURVE('',#20176,#20172,#10802,.T.);
#25746=EDGE_CURVE('',#20174,#20171,#10803,.T.);
#25747=EDGE_CURVE('',#20170,#20175,#1996,.T.);
#25748=EDGE_CURVE('',#20177,#20178,#15922,.T.);
#25749=EDGE_CURVE('',#20177,#20173,#1997,.T.);
#25750=EDGE_CURVE('',#20172,#20178,#10804,.T.);
#25751=EDGE_CURVE('',#20179,#20180,#15923,.T.);
#25752=EDGE_CURVE('',#20180,#20177,#15924,.T.);
#25753=EDGE_CURVE('',#20178,#20179,#15925,.T.);
#25754=EDGE_CURVE('',#20181,#20182,#1998,.T.);
#25755=EDGE_CURVE('',#20182,#20117,#1999,.T.);
#25756=EDGE_CURVE('',#20117,#20183,#10805,.T.);
#25757=EDGE_CURVE('',#20184,#20183,#15926,.T.);
#25758=EDGE_CURVE('',#20184,#20185,#15927,.T.);
#25759=EDGE_CURVE('',#20185,#20181,#10806,.T.);
#25760=EDGE_CURVE('',#20183,#20180,#10807,.T.);
#25761=EDGE_CURVE('',#20179,#20184,#2000,.T.);
#25762=EDGE_CURVE('',#20186,#20187,#2001,.T.);
#25763=EDGE_CURVE('',#20186,#20182,#2002,.T.);
#25764=EDGE_CURVE('',#20181,#20187,#10808,.T.);
#25765=EDGE_CURVE('',#20188,#20189,#15928,.T.);
#25766=EDGE_CURVE('',#20189,#20186,#2003,.T.);
#25767=EDGE_CURVE('',#20187,#20188,#15929,.T.);
#25768=EDGE_CURVE('',#20190,#20191,#15930,.T.);
#25769=EDGE_CURVE('',#20191,#20126,#15931,.T.);
#25770=EDGE_CURVE('',#20126,#20192,#10809,.T.);
#25771=EDGE_CURVE('',#20193,#20192,#15932,.T.);
#25772=EDGE_CURVE('',#20193,#20194,#15933,.T.);
#25773=EDGE_CURVE('',#20194,#20190,#10810,.T.);
#25774=EDGE_CURVE('',#20192,#20189,#10811,.T.);
#25775=EDGE_CURVE('',#20188,#20193,#2004,.T.);
#25776=EDGE_CURVE('',#20195,#20196,#15934,.T.);
#25777=EDGE_CURVE('',#20195,#20191,#2005,.T.);
#25778=EDGE_CURVE('',#20190,#20196,#10812,.T.);
#25779=EDGE_CURVE('',#20197,#20198,#15935,.T.);
#25780=EDGE_CURVE('',#20198,#20195,#15936,.T.);
#25781=EDGE_CURVE('',#20196,#20197,#15937,.T.);
#25782=EDGE_CURVE('',#20199,#20200,#15938,.T.);
#25783=EDGE_CURVE('',#20200,#20135,#15939,.T.);
#25784=EDGE_CURVE('',#20135,#20201,#10813,.T.);
#25785=EDGE_CURVE('',#20202,#20201,#15940,.T.);
#25786=EDGE_CURVE('',#20202,#20203,#15941,.T.);
#25787=EDGE_CURVE('',#20203,#20199,#10814,.T.);
#25788=EDGE_CURVE('',#20201,#20198,#10815,.T.);
#25789=EDGE_CURVE('',#20197,#20202,#2006,.T.);
#25790=EDGE_CURVE('',#20204,#20205,#15942,.T.);
#25791=EDGE_CURVE('',#20204,#20200,#2007,.T.);
#25792=EDGE_CURVE('',#20199,#20205,#10816,.T.);
#25793=EDGE_CURVE('',#20206,#20207,#15943,.T.);
#25794=EDGE_CURVE('',#20207,#20204,#15944,.T.);
#25795=EDGE_CURVE('',#20205,#20206,#15945,.T.);
#25796=EDGE_CURVE('',#20208,#20209,#15946,.T.);
#25797=EDGE_CURVE('',#20209,#20144,#15947,.T.);
#25798=EDGE_CURVE('',#20144,#20210,#10817,.T.);
#25799=EDGE_CURVE('',#20211,#20210,#15948,.T.);
#25800=EDGE_CURVE('',#20211,#20212,#15949,.T.);
#25801=EDGE_CURVE('',#20212,#20208,#10818,.F.);
#25802=EDGE_CURVE('',#20210,#20207,#10819,.T.);
#25803=EDGE_CURVE('',#20206,#20211,#2008,.T.);
#25804=EDGE_CURVE('',#17516,#20209,#15950,.T.);
#25805=EDGE_CURVE('',#20208,#17517,#10820,.F.);
#25806=EDGE_CURVE('',#17513,#20153,#1089,.T.);
#25807=EDGE_CURVE('',#20153,#20213,#10821,.T.);
#25808=EDGE_CURVE('',#17514,#20213,#1090,.T.);
#25809=EDGE_CURVE('',#20213,#17515,#1091,.T.);
#25810=EDGE_CURVE('',#20214,#20215,#15951,.T.);
#25811=EDGE_CURVE('',#20215,#17257,#15952,.T.);
#25812=EDGE_CURVE('',#20216,#17256,#2009,.T.);
#25813=EDGE_CURVE('',#20216,#20217,#1092,.T.);
#25814=EDGE_CURVE('',#20217,#20214,#10822,.T.);
#25815=EDGE_CURVE('',#20218,#20219,#15953,.T.);
#25816=EDGE_CURVE('',#20218,#20215,#2010,.T.);
#25817=EDGE_CURVE('',#20214,#20219,#10823,.T.);
#25818=EDGE_CURVE('',#20220,#20221,#15954,.T.);
#25819=EDGE_CURVE('',#20221,#20218,#15955,.T.);
#25820=EDGE_CURVE('',#20219,#20220,#15956,.T.);
#25821=EDGE_CURVE('',#20222,#20223,#15957,.T.);
#25822=EDGE_CURVE('',#20223,#20158,#15958,.T.);
#25823=EDGE_CURVE('',#20158,#20224,#10824,.T.);
#25824=EDGE_CURVE('',#20225,#20224,#15959,.T.);
#25825=EDGE_CURVE('',#20225,#20226,#15960,.T.);
#25826=EDGE_CURVE('',#20226,#20222,#10825,.T.);
#25827=EDGE_CURVE('',#20224,#20221,#10826,.T.);
#25828=EDGE_CURVE('',#20220,#20225,#2011,.T.);
#25829=EDGE_CURVE('',#17259,#20157,#1093,.T.);
#25830=EDGE_CURVE('',#20227,#20228,#15961,.T.);
#25831=EDGE_CURVE('',#20227,#20223,#2012,.T.);
#25832=EDGE_CURVE('',#20222,#20228,#10827,.T.);
#25833=EDGE_CURVE('',#20229,#20230,#15962,.T.);
#25834=EDGE_CURVE('',#20230,#20227,#15963,.T.);
#25835=EDGE_CURVE('',#20228,#20229,#15964,.T.);
#25836=EDGE_CURVE('',#20231,#20232,#15965,.T.);
#25837=EDGE_CURVE('',#20232,#20167,#15966,.T.);
#25838=EDGE_CURVE('',#20167,#20233,#10828,.T.);
#25839=EDGE_CURVE('',#20234,#20233,#15967,.T.);
#25840=EDGE_CURVE('',#20234,#20235,#15968,.T.);
#25841=EDGE_CURVE('',#20235,#20231,#10829,.T.);
#25842=EDGE_CURVE('',#20233,#20230,#10830,.T.);
#25843=EDGE_CURVE('',#20229,#20234,#2013,.T.);
#25844=EDGE_CURVE('',#20236,#20237,#15969,.T.);
#25845=EDGE_CURVE('',#20236,#20232,#2014,.T.);
#25846=EDGE_CURVE('',#20231,#20237,#10831,.T.);
#25847=EDGE_CURVE('',#20238,#20239,#15970,.T.);
#25848=EDGE_CURVE('',#20239,#20236,#15971,.T.);
#25849=EDGE_CURVE('',#20237,#20238,#15972,.T.);
#25850=EDGE_CURVE('',#20240,#20241,#2015,.T.);
#25851=EDGE_CURVE('',#20241,#20176,#2016,.T.);
#25852=EDGE_CURVE('',#20176,#20242,#10832,.T.);
#25853=EDGE_CURVE('',#20243,#20242,#15973,.T.);
#25854=EDGE_CURVE('',#20243,#20244,#15974,.T.);
#25855=EDGE_CURVE('',#20244,#20240,#10833,.T.);
#25856=EDGE_CURVE('',#20242,#20239,#10834,.T.);
#25857=EDGE_CURVE('',#20238,#20243,#2017,.T.);
#25858=EDGE_CURVE('',#20245,#20246,#2018,.T.);
#25859=EDGE_CURVE('',#20245,#20241,#2019,.T.);
#25860=EDGE_CURVE('',#20240,#20246,#10835,.T.);
#25861=EDGE_CURVE('',#20247,#20248,#15975,.T.);
#25862=EDGE_CURVE('',#20248,#20245,#2020,.T.);
#25863=EDGE_CURVE('',#20246,#20247,#15976,.T.);
#25864=EDGE_CURVE('',#20249,#20250,#15977,.T.);
#25865=EDGE_CURVE('',#20250,#20185,#15978,.T.);
#25866=EDGE_CURVE('',#20185,#20251,#10836,.T.);
#25867=EDGE_CURVE('',#20252,#20251,#15979,.T.);
#25868=EDGE_CURVE('',#20252,#20253,#15980,.T.);
#25869=EDGE_CURVE('',#20253,#20249,#10837,.T.);
#25870=EDGE_CURVE('',#20251,#20248,#10838,.T.);
#25871=EDGE_CURVE('',#20247,#20252,#2021,.T.);
#25872=EDGE_CURVE('',#20254,#20255,#15981,.T.);
#25873=EDGE_CURVE('',#20254,#20250,#2022,.T.);
#25874=EDGE_CURVE('',#20249,#20255,#10839,.T.);
#25875=EDGE_CURVE('',#20256,#20257,#15982,.T.);
#25876=EDGE_CURVE('',#20257,#20254,#15983,.T.);
#25877=EDGE_CURVE('',#20255,#20256,#15984,.T.);
#25878=EDGE_CURVE('',#20258,#20259,#15985,.T.);
#25879=EDGE_CURVE('',#20259,#20194,#15986,.T.);
#25880=EDGE_CURVE('',#20194,#20260,#10840,.T.);
#25881=EDGE_CURVE('',#20261,#20260,#15987,.T.);
#25882=EDGE_CURVE('',#20261,#20262,#15988,.T.);
#25883=EDGE_CURVE('',#20262,#20258,#10841,.T.);
#25884=EDGE_CURVE('',#20260,#20257,#10842,.T.);
#25885=EDGE_CURVE('',#20256,#20261,#2023,.T.);
#25886=EDGE_CURVE('',#20263,#20264,#15989,.T.);
#25887=EDGE_CURVE('',#20263,#20259,#2024,.T.);
#25888=EDGE_CURVE('',#20258,#20264,#10843,.T.);
#25889=EDGE_CURVE('',#20265,#20266,#15990,.T.);
#25890=EDGE_CURVE('',#20266,#20263,#15991,.T.);
#25891=EDGE_CURVE('',#20264,#20265,#15992,.T.);
#25892=EDGE_CURVE('',#20267,#20268,#15993,.T.);
#25893=EDGE_CURVE('',#20268,#20203,#15994,.T.);
#25894=EDGE_CURVE('',#20203,#20269,#10844,.T.);
#25895=EDGE_CURVE('',#20270,#20269,#15995,.T.);
#25896=EDGE_CURVE('',#20270,#20271,#15996,.T.);
#25897=EDGE_CURVE('',#20271,#20267,#10845,.F.);
#25898=EDGE_CURVE('',#20269,#20266,#10846,.T.);
#25899=EDGE_CURVE('',#20265,#20270,#2025,.T.);
#25900=EDGE_CURVE('',#17522,#20268,#15997,.T.);
#25901=EDGE_CURVE('',#20267,#17523,#10847,.F.);
#25902=EDGE_CURVE('',#17519,#20212,#1094,.T.);
#25903=EDGE_CURVE('',#20212,#20272,#10848,.T.);
#25904=EDGE_CURVE('',#17520,#20272,#1095,.T.);
#25905=EDGE_CURVE('',#20272,#17521,#1096,.T.);
#25906=EDGE_CURVE('',#20273,#20274,#15998,.T.);
#25907=EDGE_CURVE('',#20274,#17253,#15999,.T.);
#25908=EDGE_CURVE('',#20275,#17252,#2026,.T.);
#25909=EDGE_CURVE('',#20275,#20276,#1097,.T.);
#25910=EDGE_CURVE('',#20276,#20273,#10849,.T.);
#25911=EDGE_CURVE('',#20277,#20278,#16000,.T.);
#25912=EDGE_CURVE('',#20277,#20274,#2027,.T.);
#25913=EDGE_CURVE('',#20273,#20278,#10850,.T.);
#25914=EDGE_CURVE('',#20279,#20280,#16001,.T.);
#25915=EDGE_CURVE('',#20280,#20277,#16002,.T.);
#25916=EDGE_CURVE('',#20278,#20279,#16003,.T.);
#25917=EDGE_CURVE('',#20281,#20282,#16004,.T.);
#25918=EDGE_CURVE('',#20282,#20217,#16005,.T.);
#25919=EDGE_CURVE('',#20217,#20283,#10851,.T.);
#25920=EDGE_CURVE('',#20284,#20283,#16006,.T.);
#25921=EDGE_CURVE('',#20284,#20285,#16007,.T.);
#25922=EDGE_CURVE('',#20285,#20281,#10852,.T.);
#25923=EDGE_CURVE('',#20283,#20280,#10853,.T.);
#25924=EDGE_CURVE('',#20279,#20284,#2028,.T.);
#25925=EDGE_CURVE('',#17255,#20216,#1098,.T.);
#25926=EDGE_CURVE('',#20286,#20287,#16008,.T.);
#25927=EDGE_CURVE('',#20286,#20282,#2029,.T.);
#25928=EDGE_CURVE('',#20281,#20287,#10854,.T.);
#25929=EDGE_CURVE('',#20288,#20289,#16009,.T.);
#25930=EDGE_CURVE('',#20289,#20286,#16010,.T.);
#25931=EDGE_CURVE('',#20287,#20288,#16011,.T.);
#25932=EDGE_CURVE('',#20290,#20291,#16012,.T.);
#25933=EDGE_CURVE('',#20291,#20226,#16013,.T.);
#25934=EDGE_CURVE('',#20226,#20292,#10855,.T.);
#25935=EDGE_CURVE('',#20293,#20292,#16014,.T.);
#25936=EDGE_CURVE('',#20293,#20294,#16015,.T.);
#25937=EDGE_CURVE('',#20294,#20290,#10856,.T.);
#25938=EDGE_CURVE('',#20292,#20289,#10857,.T.);
#25939=EDGE_CURVE('',#20288,#20293,#2030,.T.);
#25940=EDGE_CURVE('',#20295,#20296,#16016,.T.);
#25941=EDGE_CURVE('',#20295,#20291,#2031,.T.);
#25942=EDGE_CURVE('',#20290,#20296,#10858,.T.);
#25943=EDGE_CURVE('',#20297,#20298,#16017,.T.);
#25944=EDGE_CURVE('',#20298,#20295,#16018,.T.);
#25945=EDGE_CURVE('',#20296,#20297,#16019,.T.);
#25946=EDGE_CURVE('',#20299,#20300,#2032,.T.);
#25947=EDGE_CURVE('',#20300,#20235,#2033,.T.);
#25948=EDGE_CURVE('',#20235,#20301,#10859,.T.);
#25949=EDGE_CURVE('',#20302,#20301,#16020,.T.);
#25950=EDGE_CURVE('',#20302,#20303,#16021,.T.);
#25951=EDGE_CURVE('',#20303,#20299,#10860,.T.);
#25952=EDGE_CURVE('',#20301,#20298,#10861,.T.);
#25953=EDGE_CURVE('',#20297,#20302,#2034,.T.);
#25954=EDGE_CURVE('',#20304,#20305,#2035,.T.);
#25955=EDGE_CURVE('',#20304,#20300,#2036,.T.);
#25956=EDGE_CURVE('',#20299,#20305,#10862,.T.);
#25957=EDGE_CURVE('',#20306,#20307,#16022,.T.);
#25958=EDGE_CURVE('',#20307,#20304,#2037,.T.);
#25959=EDGE_CURVE('',#20305,#20306,#16023,.T.);
#25960=EDGE_CURVE('',#20308,#20309,#16024,.T.);
#25961=EDGE_CURVE('',#20309,#20244,#16025,.T.);
#25962=EDGE_CURVE('',#20244,#20310,#10863,.T.);
#25963=EDGE_CURVE('',#20311,#20310,#16026,.T.);
#25964=EDGE_CURVE('',#20311,#20312,#16027,.T.);
#25965=EDGE_CURVE('',#20312,#20308,#10864,.T.);
#25966=EDGE_CURVE('',#20310,#20307,#10865,.T.);
#25967=EDGE_CURVE('',#20306,#20311,#2038,.T.);
#25968=EDGE_CURVE('',#20313,#20314,#16028,.T.);
#25969=EDGE_CURVE('',#20313,#20309,#2039,.T.);
#25970=EDGE_CURVE('',#20308,#20314,#10866,.T.);
#25971=EDGE_CURVE('',#20315,#20316,#16029,.T.);
#25972=EDGE_CURVE('',#20316,#20313,#16030,.T.);
#25973=EDGE_CURVE('',#20314,#20315,#16031,.T.);
#25974=EDGE_CURVE('',#20317,#20318,#16032,.T.);
#25975=EDGE_CURVE('',#20318,#20253,#16033,.T.);
#25976=EDGE_CURVE('',#20253,#20319,#10867,.T.);
#25977=EDGE_CURVE('',#20320,#20319,#16034,.T.);
#25978=EDGE_CURVE('',#20320,#20321,#16035,.T.);
#25979=EDGE_CURVE('',#20321,#20317,#10868,.T.);
#25980=EDGE_CURVE('',#20319,#20316,#10869,.T.);
#25981=EDGE_CURVE('',#20315,#20320,#2040,.T.);
#25982=EDGE_CURVE('',#20322,#20323,#16036,.T.);
#25983=EDGE_CURVE('',#20322,#20318,#2041,.T.);
#25984=EDGE_CURVE('',#20317,#20323,#10870,.T.);
#25985=EDGE_CURVE('',#20324,#20325,#16037,.T.);
#25986=EDGE_CURVE('',#20325,#20322,#16038,.T.);
#25987=EDGE_CURVE('',#20323,#20324,#16039,.T.);
#25988=EDGE_CURVE('',#20326,#20327,#16040,.T.);
#25989=EDGE_CURVE('',#20327,#20262,#16041,.T.);
#25990=EDGE_CURVE('',#20262,#20328,#10871,.T.);
#25991=EDGE_CURVE('',#20329,#20328,#16042,.T.);
#25992=EDGE_CURVE('',#20329,#20330,#16043,.T.);
#25993=EDGE_CURVE('',#20330,#20326,#10872,.F.);
#25994=EDGE_CURVE('',#20328,#20325,#10873,.T.);
#25995=EDGE_CURVE('',#20324,#20329,#2042,.T.);
#25996=EDGE_CURVE('',#17528,#20327,#16044,.T.);
#25997=EDGE_CURVE('',#20326,#17529,#10874,.F.);
#25998=EDGE_CURVE('',#17525,#20271,#1099,.T.);
#25999=EDGE_CURVE('',#20271,#20331,#10875,.T.);
#26000=EDGE_CURVE('',#17526,#20331,#1100,.T.);
#26001=EDGE_CURVE('',#20331,#17527,#1101,.T.);
#26002=EDGE_CURVE('',#20332,#20333,#16045,.T.);
#26003=EDGE_CURVE('',#20333,#20334,#16046,.T.);
#26004=EDGE_CURVE('',#20334,#20335,#16047,.T.);
#26005=EDGE_CURVE('',#20335,#20332,#16048,.T.);
#26006=EDGE_CURVE('',#20336,#20337,#16049,.T.);
#26007=EDGE_CURVE('',#20337,#17249,#16050,.T.);
#26008=EDGE_CURVE('',#20338,#17248,#2043,.T.);
#26009=EDGE_CURVE('',#20338,#20339,#1102,.T.);
#26010=EDGE_CURVE('',#20339,#20336,#10876,.T.);
#26011=EDGE_CURVE('',#20334,#20337,#2044,.T.);
#26012=EDGE_CURVE('',#20336,#20335,#10877,.T.);
#26013=EDGE_CURVE('',#20340,#20341,#16051,.T.);
#26014=EDGE_CURVE('',#20341,#20276,#16052,.T.);
#26015=EDGE_CURVE('',#20276,#20342,#10878,.T.);
#26016=EDGE_CURVE('',#20343,#20342,#16053,.T.);
#26017=EDGE_CURVE('',#20343,#20344,#16054,.T.);
#26018=EDGE_CURVE('',#20344,#20340,#10879,.T.);
#26019=EDGE_CURVE('',#20342,#20333,#10880,.T.);
#26020=EDGE_CURVE('',#20332,#20343,#2045,.T.);
#26021=EDGE_CURVE('',#17251,#20275,#1103,.T.);
#26022=EDGE_CURVE('',#20345,#20346,#16055,.T.);
#26023=EDGE_CURVE('',#20345,#20341,#2046,.T.);
#26024=EDGE_CURVE('',#20340,#20346,#10881,.T.);
#26025=EDGE_CURVE('',#20347,#20348,#16056,.T.);
#26026=EDGE_CURVE('',#20348,#20345,#16057,.T.);
#26027=EDGE_CURVE('',#20346,#20347,#16058,.T.);
#26028=EDGE_CURVE('',#20349,#20350,#16059,.T.);
#26029=EDGE_CURVE('',#20350,#20285,#16060,.T.);
#26030=EDGE_CURVE('',#20285,#20351,#10882,.T.);
#26031=EDGE_CURVE('',#20352,#20351,#16061,.T.);
#26032=EDGE_CURVE('',#20352,#20353,#16062,.T.);
#26033=EDGE_CURVE('',#20353,#20349,#10883,.T.);
#26034=EDGE_CURVE('',#20351,#20348,#10884,.T.);
#26035=EDGE_CURVE('',#20347,#20352,#2047,.T.);
#26036=EDGE_CURVE('',#20354,#20355,#16063,.T.);
#26037=EDGE_CURVE('',#20354,#20350,#2048,.T.);
#26038=EDGE_CURVE('',#20349,#20355,#10885,.T.);
#26039=EDGE_CURVE('',#20356,#20357,#16064,.T.);
#26040=EDGE_CURVE('',#20357,#20354,#16065,.T.);
#26041=EDGE_CURVE('',#20355,#20356,#16066,.T.);
#26042=EDGE_CURVE('',#20358,#20359,#2049,.T.);
#26043=EDGE_CURVE('',#20359,#20294,#2050,.T.);
#26044=EDGE_CURVE('',#20294,#20360,#10886,.T.);
#26045=EDGE_CURVE('',#20361,#20360,#16067,.T.);
#26046=EDGE_CURVE('',#20361,#20362,#16068,.T.);
#26047=EDGE_CURVE('',#20362,#20358,#10887,.T.);
#26048=EDGE_CURVE('',#20360,#20357,#10888,.T.);
#26049=EDGE_CURVE('',#20356,#20361,#2051,.T.);
#26050=EDGE_CURVE('',#20363,#20364,#2052,.T.);
#26051=EDGE_CURVE('',#20363,#20359,#2053,.T.);
#26052=EDGE_CURVE('',#20358,#20364,#10889,.T.);
#26053=EDGE_CURVE('',#20365,#20366,#16069,.T.);
#26054=EDGE_CURVE('',#20366,#20363,#2054,.T.);
#26055=EDGE_CURVE('',#20364,#20365,#16070,.T.);
#26056=EDGE_CURVE('',#20367,#20368,#16071,.T.);
#26057=EDGE_CURVE('',#20368,#20303,#16072,.T.);
#26058=EDGE_CURVE('',#20303,#20369,#10890,.T.);
#26059=EDGE_CURVE('',#20370,#20369,#16073,.T.);
#26060=EDGE_CURVE('',#20370,#20371,#16074,.T.);
#26061=EDGE_CURVE('',#20371,#20367,#10891,.T.);
#26062=EDGE_CURVE('',#20369,#20366,#10892,.T.);
#26063=EDGE_CURVE('',#20365,#20370,#2055,.T.);
#26064=EDGE_CURVE('',#20372,#20373,#16075,.T.);
#26065=EDGE_CURVE('',#20372,#20368,#2056,.T.);
#26066=EDGE_CURVE('',#20367,#20373,#10893,.T.);
#26067=EDGE_CURVE('',#20374,#20375,#16076,.T.);
#26068=EDGE_CURVE('',#20375,#20372,#16077,.T.);
#26069=EDGE_CURVE('',#20373,#20374,#16078,.T.);
#26070=EDGE_CURVE('',#20376,#20377,#16079,.T.);
#26071=EDGE_CURVE('',#20377,#20312,#16080,.T.);
#26072=EDGE_CURVE('',#20312,#20378,#10894,.T.);
#26073=EDGE_CURVE('',#20379,#20378,#16081,.T.);
#26074=EDGE_CURVE('',#20379,#20380,#16082,.T.);
#26075=EDGE_CURVE('',#20380,#20376,#10895,.T.);
#26076=EDGE_CURVE('',#20378,#20375,#10896,.T.);
#26077=EDGE_CURVE('',#20374,#20379,#2057,.T.);
#26078=EDGE_CURVE('',#20381,#20382,#16083,.T.);
#26079=EDGE_CURVE('',#20381,#20377,#2058,.T.);
#26080=EDGE_CURVE('',#20376,#20382,#10897,.T.);
#26081=EDGE_CURVE('',#20383,#20384,#16084,.T.);
#26082=EDGE_CURVE('',#20384,#20381,#16085,.T.);
#26083=EDGE_CURVE('',#20382,#20383,#16086,.T.);
#26084=EDGE_CURVE('',#20385,#20386,#16087,.T.);
#26085=EDGE_CURVE('',#20386,#20321,#16088,.T.);
#26086=EDGE_CURVE('',#20321,#20387,#10898,.T.);
#26087=EDGE_CURVE('',#20388,#20387,#16089,.T.);
#26088=EDGE_CURVE('',#20388,#20389,#16090,.T.);
#26089=EDGE_CURVE('',#20389,#20385,#10899,.F.);
#26090=EDGE_CURVE('',#20387,#20384,#10900,.T.);
#26091=EDGE_CURVE('',#20383,#20388,#2059,.T.);
#26092=EDGE_CURVE('',#17534,#20386,#16091,.T.);
#26093=EDGE_CURVE('',#20385,#17535,#10901,.F.);
#26094=EDGE_CURVE('',#17531,#20330,#1104,.T.);
#26095=EDGE_CURVE('',#20330,#20390,#10902,.T.);
#26096=EDGE_CURVE('',#17532,#20390,#1105,.T.);
#26097=EDGE_CURVE('',#20390,#17533,#1106,.T.);
#26098=EDGE_CURVE('',#20391,#20392,#16092,.T.);
#26099=EDGE_CURVE('',#20392,#20393,#16093,.T.);
#26100=EDGE_CURVE('',#20393,#20394,#16094,.T.);
#26101=EDGE_CURVE('',#20394,#20391,#16095,.T.);
#26102=EDGE_CURVE('',#20395,#20396,#16096,.T.);
#26103=EDGE_CURVE('',#20396,#20397,#16097,.T.);
#26104=EDGE_CURVE('',#20397,#20398,#16098,.T.);
#26105=EDGE_CURVE('',#20398,#20395,#16099,.T.);
#26106=EDGE_CURVE('',#20399,#20400,#16100,.T.);
#26107=EDGE_CURVE('',#20400,#17245,#16101,.T.);
#26108=EDGE_CURVE('',#20401,#17244,#2060,.T.);
#26109=EDGE_CURVE('',#20401,#20402,#1107,.T.);
#26110=EDGE_CURVE('',#20402,#20399,#10903,.T.);
#26111=EDGE_CURVE('',#20397,#20400,#2061,.T.);
#26112=EDGE_CURVE('',#20399,#20398,#10904,.T.);
#26113=EDGE_CURVE('',#20403,#20404,#16102,.T.);
#26114=EDGE_CURVE('',#20404,#20339,#16103,.T.);
#26115=EDGE_CURVE('',#20339,#20405,#10905,.T.);
#26116=EDGE_CURVE('',#20406,#20405,#16104,.T.);
#26117=EDGE_CURVE('',#20406,#20407,#16105,.T.);
#26118=EDGE_CURVE('',#20407,#20403,#10906,.T.);
#26119=EDGE_CURVE('',#20405,#20396,#10907,.T.);
#26120=EDGE_CURVE('',#20395,#20406,#2062,.T.);
#26121=EDGE_CURVE('',#17247,#20338,#1108,.T.);
#26122=EDGE_CURVE('',#20393,#20404,#2063,.T.);
#26123=EDGE_CURVE('',#20403,#20394,#10908,.T.);
#26124=EDGE_CURVE('',#20408,#20409,#16106,.T.);
#26125=EDGE_CURVE('',#20409,#20344,#16107,.T.);
#26126=EDGE_CURVE('',#20344,#20410,#10909,.T.);
#26127=EDGE_CURVE('',#20411,#20410,#16108,.T.);
#26128=EDGE_CURVE('',#20411,#20412,#16109,.T.);
#26129=EDGE_CURVE('',#20412,#20408,#10910,.T.);
#26130=EDGE_CURVE('',#20410,#20392,#10911,.T.);
#26131=EDGE_CURVE('',#20391,#20411,#2064,.T.);
#26132=EDGE_CURVE('',#20413,#20414,#16110,.T.);
#26133=EDGE_CURVE('',#20413,#20409,#2065,.T.);
#26134=EDGE_CURVE('',#20408,#20414,#10912,.T.);
#26135=EDGE_CURVE('',#20415,#20416,#16111,.T.);
#26136=EDGE_CURVE('',#20416,#20413,#16112,.T.);
#26137=EDGE_CURVE('',#20414,#20415,#16113,.T.);
#26138=EDGE_CURVE('',#20417,#20418,#2066,.T.);
#26139=EDGE_CURVE('',#20418,#20353,#2067,.T.);
#26140=EDGE_CURVE('',#20353,#20419,#10913,.T.);
#26141=EDGE_CURVE('',#20420,#20419,#16114,.T.);
#26142=EDGE_CURVE('',#20420,#20421,#16115,.T.);
#26143=EDGE_CURVE('',#20421,#20417,#10914,.T.);
#26144=EDGE_CURVE('',#20419,#20416,#10915,.T.);
#26145=EDGE_CURVE('',#20415,#20420,#2068,.T.);
#26146=EDGE_CURVE('',#20422,#20423,#2069,.T.);
#26147=EDGE_CURVE('',#20422,#20418,#2070,.T.);
#26148=EDGE_CURVE('',#20417,#20423,#10916,.T.);
#26149=EDGE_CURVE('',#20424,#20425,#16116,.T.);
#26150=EDGE_CURVE('',#20425,#20422,#2071,.T.);
#26151=EDGE_CURVE('',#20423,#20424,#16117,.T.);
#26152=EDGE_CURVE('',#20426,#20427,#16118,.T.);
#26153=EDGE_CURVE('',#20427,#20362,#16119,.T.);
#26154=EDGE_CURVE('',#20362,#20428,#10917,.T.);
#26155=EDGE_CURVE('',#20429,#20428,#16120,.T.);
#26156=EDGE_CURVE('',#20429,#20430,#16121,.T.);
#26157=EDGE_CURVE('',#20430,#20426,#10918,.T.);
#26158=EDGE_CURVE('',#20428,#20425,#10919,.T.);
#26159=EDGE_CURVE('',#20424,#20429,#2072,.T.);
#26160=EDGE_CURVE('',#20431,#20432,#16122,.T.);
#26161=EDGE_CURVE('',#20431,#20427,#2073,.T.);
#26162=EDGE_CURVE('',#20426,#20432,#10920,.T.);
#26163=EDGE_CURVE('',#20433,#20434,#16123,.T.);
#26164=EDGE_CURVE('',#20434,#20431,#16124,.T.);
#26165=EDGE_CURVE('',#20432,#20433,#16125,.T.);
#26166=EDGE_CURVE('',#20435,#20436,#16126,.T.);
#26167=EDGE_CURVE('',#20436,#20371,#16127,.T.);
#26168=EDGE_CURVE('',#20371,#20437,#10921,.T.);
#26169=EDGE_CURVE('',#20438,#20437,#16128,.T.);
#26170=EDGE_CURVE('',#20438,#20439,#16129,.T.);
#26171=EDGE_CURVE('',#20439,#20435,#10922,.T.);
#26172=EDGE_CURVE('',#20437,#20434,#10923,.T.);
#26173=EDGE_CURVE('',#20433,#20438,#2074,.T.);
#26174=EDGE_CURVE('',#20440,#20441,#16130,.T.);
#26175=EDGE_CURVE('',#20440,#20436,#2075,.T.);
#26176=EDGE_CURVE('',#20435,#20441,#10924,.T.);
#26177=EDGE_CURVE('',#20442,#20443,#16131,.T.);
#26178=EDGE_CURVE('',#20443,#20440,#16132,.T.);
#26179=EDGE_CURVE('',#20441,#20442,#16133,.T.);
#26180=EDGE_CURVE('',#20444,#20445,#16134,.T.);
#26181=EDGE_CURVE('',#20445,#20380,#16135,.T.);
#26182=EDGE_CURVE('',#20380,#20446,#10925,.T.);
#26183=EDGE_CURVE('',#20447,#20446,#16136,.T.);
#26184=EDGE_CURVE('',#20447,#20448,#16137,.T.);
#26185=EDGE_CURVE('',#20448,#20444,#10926,.F.);
#26186=EDGE_CURVE('',#20446,#20443,#10927,.T.);
#26187=EDGE_CURVE('',#20442,#20447,#2076,.T.);
#26188=EDGE_CURVE('',#17540,#20445,#16138,.T.);
#26189=EDGE_CURVE('',#20444,#17541,#10928,.F.);
#26190=EDGE_CURVE('',#17537,#20389,#1109,.T.);
#26191=EDGE_CURVE('',#20389,#20449,#10929,.T.);
#26192=EDGE_CURVE('',#17538,#20449,#1110,.T.);
#26193=EDGE_CURVE('',#20449,#17539,#1111,.T.);
#26194=EDGE_CURVE('',#20450,#20451,#16139,.T.);
#26195=EDGE_CURVE('',#20451,#20452,#16140,.T.);
#26196=EDGE_CURVE('',#20452,#20453,#16141,.T.);
#26197=EDGE_CURVE('',#20453,#20450,#16142,.T.);
#26198=EDGE_CURVE('',#20454,#20455,#16143,.T.);
#26199=EDGE_CURVE('',#20455,#20456,#16144,.T.);
#26200=EDGE_CURVE('',#20456,#20457,#16145,.T.);
#26201=EDGE_CURVE('',#20457,#20454,#16146,.T.);
#26202=EDGE_CURVE('',#20458,#20459,#16147,.T.);
#26203=EDGE_CURVE('',#20459,#20460,#16148,.T.);
#26204=EDGE_CURVE('',#20460,#20461,#16149,.T.);
#26205=EDGE_CURVE('',#20461,#20458,#16150,.T.);
#26206=EDGE_CURVE('',#20462,#20463,#16151,.T.);
#26207=EDGE_CURVE('',#20463,#20402,#16152,.T.);
#26208=EDGE_CURVE('',#20402,#20464,#10930,.T.);
#26209=EDGE_CURVE('',#20465,#20464,#16153,.T.);
#26210=EDGE_CURVE('',#20465,#20466,#16154,.T.);
#26211=EDGE_CURVE('',#20466,#20462,#10931,.T.);
#26212=EDGE_CURVE('',#20464,#20451,#10932,.T.);
#26213=EDGE_CURVE('',#20450,#20465,#2077,.T.);
#26214=EDGE_CURVE('',#17243,#20401,#1112,.T.);
#26215=EDGE_CURVE('',#20460,#20463,#2078,.T.);
#26216=EDGE_CURVE('',#20462,#20461,#10933,.T.);
#26217=EDGE_CURVE('',#20467,#20468,#16155,.T.);
#26218=EDGE_CURVE('',#20468,#20407,#16156,.T.);
#26219=EDGE_CURVE('',#20407,#20469,#10934,.T.);
#26220=EDGE_CURVE('',#20470,#20469,#16157,.T.);
#26221=EDGE_CURVE('',#20470,#20471,#16158,.T.);
#26222=EDGE_CURVE('',#20471,#20467,#10935,.T.);
#26223=EDGE_CURVE('',#20469,#20459,#10936,.T.);
#26224=EDGE_CURVE('',#20458,#20470,#2079,.T.);
#26225=EDGE_CURVE('',#20456,#20468,#2080,.T.);
#26226=EDGE_CURVE('',#20467,#20457,#10937,.T.);
#26227=EDGE_CURVE('',#20472,#20473,#2081,.T.);
#26228=EDGE_CURVE('',#20473,#20412,#2082,.T.);
#26229=EDGE_CURVE('',#20412,#20474,#10938,.T.);
#26230=EDGE_CURVE('',#20475,#20474,#16159,.T.);
#26231=EDGE_CURVE('',#20475,#20476,#16160,.T.);
#26232=EDGE_CURVE('',#20476,#20472,#10939,.T.);
#26233=EDGE_CURVE('',#20474,#20455,#10940,.T.);
#26234=EDGE_CURVE('',#20454,#20475,#2083,.T.);
#26235=EDGE_CURVE('',#20477,#20478,#2084,.T.);
#26236=EDGE_CURVE('',#20477,#20473,#2085,.T.);
#26237=EDGE_CURVE('',#20472,#20478,#10941,.T.);
#26238=EDGE_CURVE('',#20479,#20480,#16161,.T.);
#26239=EDGE_CURVE('',#20480,#17241,#16162,.T.);
#26240=EDGE_CURVE('',#20481,#17240,#2086,.T.);
#26241=EDGE_CURVE('',#20481,#20482,#1113,.T.);
#26242=EDGE_CURVE('',#20482,#20479,#10942,.T.);
#26243=EDGE_CURVE('',#20452,#20480,#2087,.T.);
#26244=EDGE_CURVE('',#20479,#20453,#10943,.T.);
#26245=EDGE_CURVE('',#20483,#20484,#16163,.T.);
#26246=EDGE_CURVE('',#20484,#20477,#2088,.T.);
#26247=EDGE_CURVE('',#20478,#20483,#16164,.T.);
#26248=EDGE_CURVE('',#20485,#20486,#16165,.T.);
#26249=EDGE_CURVE('',#20486,#20421,#16166,.T.);
#26250=EDGE_CURVE('',#20421,#20487,#10944,.T.);
#26251=EDGE_CURVE('',#20488,#20487,#16167,.T.);
#26252=EDGE_CURVE('',#20488,#20489,#16168,.T.);
#26253=EDGE_CURVE('',#20489,#20485,#10945,.T.);
#26254=EDGE_CURVE('',#20487,#20484,#10946,.T.);
#26255=EDGE_CURVE('',#20483,#20488,#2089,.T.);
#26256=EDGE_CURVE('',#20490,#20491,#16169,.T.);
#26257=EDGE_CURVE('',#20490,#20486,#2090,.T.);
#26258=EDGE_CURVE('',#20485,#20491,#10947,.T.);
#26259=EDGE_CURVE('',#20492,#20493,#16170,.T.);
#26260=EDGE_CURVE('',#20493,#20490,#16171,.T.);
#26261=EDGE_CURVE('',#20491,#20492,#16172,.T.);
#26262=EDGE_CURVE('',#20494,#20495,#16173,.T.);
#26263=EDGE_CURVE('',#20495,#20430,#16174,.T.);
#26264=EDGE_CURVE('',#20430,#20496,#10948,.T.);
#26265=EDGE_CURVE('',#20497,#20496,#16175,.T.);
#26266=EDGE_CURVE('',#20497,#20498,#16176,.T.);
#26267=EDGE_CURVE('',#20498,#20494,#10949,.T.);
#26268=EDGE_CURVE('',#20496,#20493,#10950,.T.);
#26269=EDGE_CURVE('',#20492,#20497,#2091,.T.);
#26270=EDGE_CURVE('',#20499,#20500,#16177,.T.);
#26271=EDGE_CURVE('',#20499,#20495,#2092,.T.);
#26272=EDGE_CURVE('',#20494,#20500,#10951,.T.);
#26273=EDGE_CURVE('',#20501,#20502,#16178,.T.);
#26274=EDGE_CURVE('',#20502,#20499,#16179,.T.);
#26275=EDGE_CURVE('',#20500,#20501,#16180,.T.);
#26276=EDGE_CURVE('',#20503,#20504,#16181,.T.);
#26277=EDGE_CURVE('',#20504,#20439,#16182,.T.);
#26278=EDGE_CURVE('',#20439,#20505,#10952,.T.);
#26279=EDGE_CURVE('',#20506,#20505,#16183,.T.);
#26280=EDGE_CURVE('',#20506,#20507,#16184,.T.);
#26281=EDGE_CURVE('',#20507,#20503,#10953,.F.);
#26282=EDGE_CURVE('',#20505,#20502,#10954,.T.);
#26283=EDGE_CURVE('',#20501,#20506,#2093,.T.);
#26284=EDGE_CURVE('',#17546,#20504,#16185,.T.);
#26285=EDGE_CURVE('',#20503,#17547,#10955,.F.);
#26286=EDGE_CURVE('',#17543,#20448,#1114,.T.);
#26287=EDGE_CURVE('',#20448,#20508,#10956,.T.);
#26288=EDGE_CURVE('',#17544,#20508,#1115,.T.);
#26289=EDGE_CURVE('',#20508,#17545,#1116,.T.);
#26290=EDGE_CURVE('',#20509,#20510,#16186,.T.);
#26291=EDGE_CURVE('',#20510,#20511,#16187,.T.);
#26292=EDGE_CURVE('',#20511,#20512,#16188,.T.);
#26293=EDGE_CURVE('',#20512,#20509,#16189,.T.);
#26294=EDGE_CURVE('',#20513,#20514,#16190,.T.);
#26295=EDGE_CURVE('',#20514,#20515,#16191,.T.);
#26296=EDGE_CURVE('',#20515,#20516,#16192,.T.);
#26297=EDGE_CURVE('',#20516,#20513,#16193,.T.);
#26298=EDGE_CURVE('',#20517,#20518,#16194,.T.);
#26299=EDGE_CURVE('',#20518,#20519,#2094,.T.);
#26300=EDGE_CURVE('',#20519,#20520,#2095,.T.);
#26301=EDGE_CURVE('',#20520,#20517,#16195,.T.);
#26302=EDGE_CURVE('',#20521,#20522,#16196,.T.);
#26303=EDGE_CURVE('',#20522,#20523,#16197,.T.);
#26304=EDGE_CURVE('',#20523,#20524,#16198,.T.);
#26305=EDGE_CURVE('',#20524,#20521,#16199,.T.);
#26306=EDGE_CURVE('',#20525,#20526,#16200,.T.);
#26307=EDGE_CURVE('',#20526,#20466,#16201,.T.);
#26308=EDGE_CURVE('',#20466,#20527,#10957,.T.);
#26309=EDGE_CURVE('',#20528,#20527,#16202,.T.);
#26310=EDGE_CURVE('',#20528,#20529,#16203,.T.);
#26311=EDGE_CURVE('',#20529,#20525,#10958,.T.);
#26312=EDGE_CURVE('',#20527,#20514,#10959,.T.);
#26313=EDGE_CURVE('',#20513,#20528,#2096,.T.);
#26314=EDGE_CURVE('',#20523,#20526,#2097,.T.);
#26315=EDGE_CURVE('',#20525,#20524,#10960,.T.);
#26316=EDGE_CURVE('',#20530,#20531,#2098,.T.);
#26317=EDGE_CURVE('',#20531,#20471,#2099,.T.);
#26318=EDGE_CURVE('',#20471,#20532,#10961,.T.);
#26319=EDGE_CURVE('',#20533,#20532,#16204,.T.);
#26320=EDGE_CURVE('',#20533,#20534,#16205,.T.);
#26321=EDGE_CURVE('',#20534,#20530,#10962,.T.);
#26322=EDGE_CURVE('',#20532,#20522,#10963,.T.);
#26323=EDGE_CURVE('',#20521,#20533,#2100,.T.);
#26324=EDGE_CURVE('',#20519,#20531,#2101,.T.);
#26325=EDGE_CURVE('',#20530,#20520,#10964,.T.);
#26326=EDGE_CURVE('',#20535,#20536,#16206,.T.);
#26327=EDGE_CURVE('',#20536,#20476,#16207,.T.);
#26328=EDGE_CURVE('',#20476,#20537,#10965,.T.);
#26329=EDGE_CURVE('',#20538,#20537,#16208,.T.);
#26330=EDGE_CURVE('',#20538,#20539,#16209,.T.);
#26331=EDGE_CURVE('',#20539,#20535,#10966,.T.);
#26332=EDGE_CURVE('',#20537,#20518,#10967,.T.);
#26333=EDGE_CURVE('',#20517,#20538,#2102,.T.);
#26334=EDGE_CURVE('',#20540,#20541,#16210,.T.);
#26335=EDGE_CURVE('',#20540,#20536,#2103,.T.);
#26336=EDGE_CURVE('',#20535,#20541,#10968,.T.);
#26337=EDGE_CURVE('',#20542,#20543,#16211,.T.);
#26338=EDGE_CURVE('',#20543,#17237,#16212,.T.);
#26339=EDGE_CURVE('',#20544,#17236,#2104,.T.);
#26340=EDGE_CURVE('',#20544,#20545,#1117,.T.);
#26341=EDGE_CURVE('',#20545,#20542,#10969,.T.);
#26342=EDGE_CURVE('',#20511,#20543,#2105,.T.);
#26343=EDGE_CURVE('',#20542,#20512,#10970,.T.);
#26344=EDGE_CURVE('',#20546,#20547,#16213,.T.);
#26345=EDGE_CURVE('',#20547,#20482,#16214,.T.);
#26346=EDGE_CURVE('',#20482,#20548,#10971,.T.);
#26347=EDGE_CURVE('',#20549,#20548,#16215,.T.);
#26348=EDGE_CURVE('',#20549,#20550,#16216,.T.);
#26349=EDGE_CURVE('',#20550,#20546,#10972,.T.);
#26350=EDGE_CURVE('',#20548,#20510,#10973,.T.);
#26351=EDGE_CURVE('',#20509,#20549,#2106,.T.);
#26352=EDGE_CURVE('',#17239,#20481,#1118,.T.);
#26353=EDGE_CURVE('',#20515,#20547,#2107,.T.);
#26354=EDGE_CURVE('',#20546,#20516,#10974,.T.);
#26355=EDGE_CURVE('',#20551,#20552,#16217,.T.);
#26356=EDGE_CURVE('',#20552,#20540,#16218,.T.);
#26357=EDGE_CURVE('',#20541,#20551,#16219,.T.);
#26358=EDGE_CURVE('',#20553,#20554,#16220,.T.);
#26359=EDGE_CURVE('',#20554,#20489,#16221,.T.);
#26360=EDGE_CURVE('',#20489,#20555,#10975,.T.);
#26361=EDGE_CURVE('',#20556,#20555,#16222,.T.);
#26362=EDGE_CURVE('',#20556,#20557,#16223,.T.);
#26363=EDGE_CURVE('',#20557,#20553,#10976,.T.);
#26364=EDGE_CURVE('',#20555,#20552,#10977,.T.);
#26365=EDGE_CURVE('',#20551,#20556,#2108,.T.);
#26366=EDGE_CURVE('',#20558,#20559,#16224,.T.);
#26367=EDGE_CURVE('',#20558,#20554,#2109,.T.);
#26368=EDGE_CURVE('',#20553,#20559,#10978,.T.);
#26369=EDGE_CURVE('',#20560,#20561,#16225,.T.);
#26370=EDGE_CURVE('',#20561,#20558,#16226,.T.);
#26371=EDGE_CURVE('',#20559,#20560,#16227,.T.);
#26372=EDGE_CURVE('',#20562,#20563,#16228,.T.);
#26373=EDGE_CURVE('',#20563,#20498,#16229,.T.);
#26374=EDGE_CURVE('',#20498,#20564,#10979,.T.);
#26375=EDGE_CURVE('',#20565,#20564,#16230,.T.);
#26376=EDGE_CURVE('',#20565,#20566,#16231,.T.);
#26377=EDGE_CURVE('',#20566,#20562,#10980,.F.);
#26378=EDGE_CURVE('',#20564,#20561,#10981,.T.);
#26379=EDGE_CURVE('',#20560,#20565,#2110,.T.);
#26380=EDGE_CURVE('',#17552,#20563,#16232,.T.);
#26381=EDGE_CURVE('',#20562,#17553,#10982,.F.);
#26382=EDGE_CURVE('',#17549,#20507,#1119,.T.);
#26383=EDGE_CURVE('',#20507,#20567,#10983,.T.);
#26384=EDGE_CURVE('',#17550,#20567,#1120,.T.);
#26385=EDGE_CURVE('',#20567,#17551,#1121,.T.);
#26386=EDGE_CURVE('',#20568,#20569,#16233,.T.);
#26387=EDGE_CURVE('',#20569,#20570,#16234,.T.);
#26388=EDGE_CURVE('',#20570,#20571,#16235,.T.);
#26389=EDGE_CURVE('',#20571,#20568,#16236,.T.);
#26390=EDGE_CURVE('',#20572,#20573,#16237,.T.);
#26391=EDGE_CURVE('',#20573,#20574,#16238,.T.);
#26392=EDGE_CURVE('',#20574,#20575,#16239,.T.);
#26393=EDGE_CURVE('',#20575,#20572,#16240,.T.);
#26394=EDGE_CURVE('',#20576,#20577,#16241,.T.);
#26395=EDGE_CURVE('',#20577,#20578,#16242,.T.);
#26396=EDGE_CURVE('',#20578,#20579,#16243,.T.);
#26397=EDGE_CURVE('',#20579,#20576,#16244,.T.);
#26398=EDGE_CURVE('',#20580,#20581,#16245,.T.);
#26399=EDGE_CURVE('',#20581,#20582,#16246,.T.);
#26400=EDGE_CURVE('',#20582,#20583,#16247,.T.);
#26401=EDGE_CURVE('',#20583,#20580,#16248,.T.);
#26402=EDGE_CURVE('',#20584,#20585,#16249,.T.);
#26403=EDGE_CURVE('',#20585,#20586,#2111,.T.);
#26404=EDGE_CURVE('',#20586,#20587,#2112,.T.);
#26405=EDGE_CURVE('',#20587,#20584,#16250,.T.);
#26406=EDGE_CURVE('',#20588,#20589,#2113,.T.);
#26407=EDGE_CURVE('',#20589,#20529,#2114,.T.);
#26408=EDGE_CURVE('',#20529,#20590,#10984,.T.);
#26409=EDGE_CURVE('',#20591,#20590,#16251,.T.);
#26410=EDGE_CURVE('',#20591,#20592,#16252,.T.);
#26411=EDGE_CURVE('',#20592,#20588,#10985,.T.);
#26412=EDGE_CURVE('',#20590,#20573,#10986,.T.);
#26413=EDGE_CURVE('',#20572,#20591,#2115,.T.);
#26414=EDGE_CURVE('',#20586,#20589,#2116,.T.);
#26415=EDGE_CURVE('',#20588,#20587,#10987,.T.);
#26416=EDGE_CURVE('',#20593,#20594,#16253,.T.);
#26417=EDGE_CURVE('',#20594,#20534,#16254,.T.);
#26418=EDGE_CURVE('',#20534,#20595,#10988,.T.);
#26419=EDGE_CURVE('',#20596,#20595,#16255,.T.);
#26420=EDGE_CURVE('',#20596,#20597,#16256,.T.);
#26421=EDGE_CURVE('',#20597,#20593,#10989,.T.);
#26422=EDGE_CURVE('',#20595,#20585,#10990,.T.);
#26423=EDGE_CURVE('',#20584,#20596,#2117,.T.);
#26424=EDGE_CURVE('',#20582,#20594,#2118,.T.);
#26425=EDGE_CURVE('',#20593,#20583,#10991,.T.);
#26426=EDGE_CURVE('',#20598,#20599,#16257,.T.);
#26427=EDGE_CURVE('',#20599,#20539,#16258,.T.);
#26428=EDGE_CURVE('',#20539,#20600,#10992,.T.);
#26429=EDGE_CURVE('',#20601,#20600,#16259,.T.);
#26430=EDGE_CURVE('',#20601,#20602,#16260,.T.);
#26431=EDGE_CURVE('',#20602,#20598,#10993,.T.);
#26432=EDGE_CURVE('',#20600,#20581,#10994,.T.);
#26433=EDGE_CURVE('',#20580,#20601,#2119,.T.);
#26434=EDGE_CURVE('',#20603,#20604,#16261,.T.);
#26435=EDGE_CURVE('',#20603,#20599,#2120,.T.);
#26436=EDGE_CURVE('',#20598,#20604,#10995,.T.);
#26437=EDGE_CURVE('',#20605,#20606,#16262,.T.);
#26438=EDGE_CURVE('',#20606,#17233,#16263,.T.);
#26439=EDGE_CURVE('',#20607,#17232,#2121,.T.);
#26440=EDGE_CURVE('',#20607,#20608,#1122,.T.);
#26441=EDGE_CURVE('',#20608,#20605,#10996,.T.);
#26442=EDGE_CURVE('',#20578,#20606,#2122,.T.);
#26443=EDGE_CURVE('',#20605,#20579,#10997,.T.);
#26444=EDGE_CURVE('',#20609,#20610,#16264,.T.);
#26445=EDGE_CURVE('',#20610,#20545,#16265,.T.);
#26446=EDGE_CURVE('',#20545,#20611,#10998,.T.);
#26447=EDGE_CURVE('',#20612,#20611,#16266,.T.);
#26448=EDGE_CURVE('',#20612,#20613,#16267,.T.);
#26449=EDGE_CURVE('',#20613,#20609,#10999,.T.);
#26450=EDGE_CURVE('',#20611,#20577,#11000,.T.);
#26451=EDGE_CURVE('',#20576,#20612,#2123,.T.);
#26452=EDGE_CURVE('',#17235,#20544,#1123,.T.);
#26453=EDGE_CURVE('',#20570,#20610,#2124,.T.);
#26454=EDGE_CURVE('',#20609,#20571,#11001,.T.);
#26455=EDGE_CURVE('',#20614,#20615,#16268,.T.);
#26456=EDGE_CURVE('',#20615,#20550,#16269,.T.);
#26457=EDGE_CURVE('',#20550,#20616,#11002,.T.);
#26458=EDGE_CURVE('',#20617,#20616,#16270,.T.);
#26459=EDGE_CURVE('',#20617,#20618,#16271,.T.);
#26460=EDGE_CURVE('',#20618,#20614,#11003,.T.);
#26461=EDGE_CURVE('',#20616,#20569,#11004,.T.);
#26462=EDGE_CURVE('',#20568,#20617,#2125,.T.);
#26463=EDGE_CURVE('',#20574,#20615,#2126,.T.);
#26464=EDGE_CURVE('',#20614,#20575,#11005,.T.);
#26465=EDGE_CURVE('',#20619,#20620,#16272,.T.);
#26466=EDGE_CURVE('',#20620,#20603,#16273,.T.);
#26467=EDGE_CURVE('',#20604,#20619,#16274,.T.);
#26468=EDGE_CURVE('',#20621,#20622,#16275,.T.);
#26469=EDGE_CURVE('',#20622,#20557,#16276,.T.);
#26470=EDGE_CURVE('',#20557,#20623,#11006,.T.);
#26471=EDGE_CURVE('',#20624,#20623,#16277,.T.);
#26472=EDGE_CURVE('',#20624,#20625,#16278,.T.);
#26473=EDGE_CURVE('',#20625,#20621,#11007,.F.);
#26474=EDGE_CURVE('',#20623,#20620,#11008,.T.);
#26475=EDGE_CURVE('',#20619,#20624,#2127,.T.);
#26476=EDGE_CURVE('',#17558,#20622,#16279,.T.);
#26477=EDGE_CURVE('',#20621,#17559,#11009,.F.);
#26478=EDGE_CURVE('',#17555,#20566,#1124,.T.);
#26479=EDGE_CURVE('',#20566,#20626,#11010,.T.);
#26480=EDGE_CURVE('',#17556,#20626,#1125,.T.);
#26481=EDGE_CURVE('',#20626,#17557,#1126,.T.);
#26482=EDGE_CURVE('',#20627,#20628,#16280,.T.);
#26483=EDGE_CURVE('',#20628,#20629,#16281,.T.);
#26484=EDGE_CURVE('',#20629,#20630,#16282,.T.);
#26485=EDGE_CURVE('',#20630,#20627,#16283,.T.);
#26486=EDGE_CURVE('',#20631,#20632,#16284,.T.);
#26487=EDGE_CURVE('',#20632,#20633,#2128,.T.);
#26488=EDGE_CURVE('',#20633,#20634,#2129,.T.);
#26489=EDGE_CURVE('',#20634,#20631,#16285,.T.);
#26490=EDGE_CURVE('',#20635,#20636,#16286,.T.);
#26491=EDGE_CURVE('',#20636,#20637,#16287,.T.);
#26492=EDGE_CURVE('',#20637,#20638,#16288,.T.);
#26493=EDGE_CURVE('',#20638,#20635,#16289,.T.);
#26494=EDGE_CURVE('',#20639,#20640,#16290,.T.);
#26495=EDGE_CURVE('',#20640,#20641,#16291,.T.);
#26496=EDGE_CURVE('',#20641,#20642,#16292,.T.);
#26497=EDGE_CURVE('',#20642,#20639,#16293,.T.);
#26498=EDGE_CURVE('',#20643,#20644,#16294,.T.);
#26499=EDGE_CURVE('',#20644,#20645,#16295,.T.);
#26500=EDGE_CURVE('',#20645,#20646,#16296,.T.);
#26501=EDGE_CURVE('',#20646,#20643,#16297,.T.);
#26502=EDGE_CURVE('',#20647,#20648,#16298,.T.);
#26503=EDGE_CURVE('',#20648,#20649,#16299,.T.);
#26504=EDGE_CURVE('',#20649,#20650,#16300,.T.);
#26505=EDGE_CURVE('',#20650,#20647,#16301,.T.);
#26506=EDGE_CURVE('',#20651,#20652,#16302,.T.);
#26507=EDGE_CURVE('',#20652,#20592,#16303,.T.);
#26508=EDGE_CURVE('',#20592,#20653,#11011,.T.);
#26509=EDGE_CURVE('',#20654,#20653,#16304,.T.);
#26510=EDGE_CURVE('',#20654,#17842,#16305,.T.);
#26511=EDGE_CURVE('',#17842,#20651,#11012,.T.);
#26512=EDGE_CURVE('',#20653,#20632,#11013,.T.);
#26513=EDGE_CURVE('',#20631,#20654,#2130,.T.);
#26514=EDGE_CURVE('',#20649,#20652,#2131,.T.);
#26515=EDGE_CURVE('',#20651,#20650,#11014,.T.);
#26516=EDGE_CURVE('',#20655,#20656,#16306,.T.);
#26517=EDGE_CURVE('',#20656,#20597,#16307,.T.);
#26518=EDGE_CURVE('',#20597,#20657,#11015,.T.);
#26519=EDGE_CURVE('',#20658,#20657,#16308,.T.);
#26520=EDGE_CURVE('',#20658,#17853,#16309,.T.);
#26521=EDGE_CURVE('',#17853,#20655,#11016,.T.);
#26522=EDGE_CURVE('',#20657,#20648,#11017,.T.);
#26523=EDGE_CURVE('',#20647,#20658,#2132,.T.);
#26524=EDGE_CURVE('',#20645,#20656,#2133,.T.);
#26525=EDGE_CURVE('',#20655,#20646,#11018,.T.);
#26526=EDGE_CURVE('',#20659,#20660,#16310,.T.);
#26527=EDGE_CURVE('',#20660,#20602,#16311,.T.);
#26528=EDGE_CURVE('',#20602,#20661,#11019,.T.);
#26529=EDGE_CURVE('',#20662,#20661,#16312,.T.);
#26530=EDGE_CURVE('',#20662,#20663,#16313,.T.);
#26531=EDGE_CURVE('',#20663,#20659,#11020,.F.);
#26532=EDGE_CURVE('',#20661,#20644,#11021,.T.);
#26533=EDGE_CURVE('',#20643,#20662,#2134,.T.);
#26534=EDGE_CURVE('',#17564,#20660,#16314,.T.);
#26535=EDGE_CURVE('',#20659,#17565,#11022,.F.);
#26536=EDGE_CURVE('',#20664,#20665,#16315,.T.);
#26537=EDGE_CURVE('',#20665,#17227,#16316,.T.);
#26538=EDGE_CURVE('',#20666,#17428,#2135,.T.);
#26539=EDGE_CURVE('',#20666,#17766,#1127,.T.);
#26540=EDGE_CURVE('',#17766,#20664,#11023,.T.);
#26541=EDGE_CURVE('',#20641,#20665,#2136,.T.);
#26542=EDGE_CURVE('',#20664,#20642,#11024,.T.);
#26543=EDGE_CURVE('',#20667,#20668,#16317,.T.);
#26544=EDGE_CURVE('',#20668,#20608,#16318,.T.);
#26545=EDGE_CURVE('',#20608,#20669,#11025,.T.);
#26546=EDGE_CURVE('',#20670,#20669,#16319,.T.);
#26547=EDGE_CURVE('',#20670,#17785,#16320,.T.);
#26548=EDGE_CURVE('',#17785,#20667,#11026,.T.);
#26549=EDGE_CURVE('',#20669,#20640,#11027,.T.);
#26550=EDGE_CURVE('',#20639,#20670,#2137,.T.);
#26551=EDGE_CURVE('',#17231,#20607,#1128,.T.);
#26552=EDGE_CURVE('',#20637,#20668,#2138,.T.);
#26553=EDGE_CURVE('',#20667,#20638,#11028,.T.);
#26554=EDGE_CURVE('',#20671,#20672,#16321,.T.);
#26555=EDGE_CURVE('',#20672,#20613,#16322,.T.);
#26556=EDGE_CURVE('',#20613,#20673,#11029,.T.);
#26557=EDGE_CURVE('',#20674,#20673,#16323,.T.);
#26558=EDGE_CURVE('',#20674,#17804,#16324,.T.);
#26559=EDGE_CURVE('',#17804,#20671,#11030,.T.);
#26560=EDGE_CURVE('',#20673,#20636,#11031,.T.);
#26561=EDGE_CURVE('',#20635,#20674,#2139,.T.);
#26562=EDGE_CURVE('',#20629,#20672,#2140,.T.);
#26563=EDGE_CURVE('',#20671,#20630,#11032,.T.);
#26564=EDGE_CURVE('',#20675,#20676,#2141,.T.);
#26565=EDGE_CURVE('',#20676,#20618,#2142,.T.);
#26566=EDGE_CURVE('',#20618,#20677,#11033,.T.);
#26567=EDGE_CURVE('',#20678,#20677,#16325,.T.);
#26568=EDGE_CURVE('',#20678,#17823,#16326,.T.);
#26569=EDGE_CURVE('',#17823,#20675,#11034,.T.);
#26570=EDGE_CURVE('',#20677,#20628,#11035,.T.);
#26571=EDGE_CURVE('',#20627,#20678,#2143,.T.);
#26572=EDGE_CURVE('',#20633,#20676,#2144,.T.);
#26573=EDGE_CURVE('',#20675,#20634,#11036,.T.);
#26574=EDGE_CURVE('',#17561,#20625,#1129,.T.);
#26575=EDGE_CURVE('',#20625,#20679,#11037,.T.);
#26576=EDGE_CURVE('',#17562,#20679,#1130,.T.);
#26577=EDGE_CURVE('',#20679,#17563,#1131,.T.);
#26578=EDGE_CURVE('',#17567,#20663,#1132,.T.);
#26579=EDGE_CURVE('',#20663,#20680,#11038,.T.);
#26580=EDGE_CURVE('',#17568,#20680,#1133,.T.);
#26581=EDGE_CURVE('',#20680,#17569,#1134,.T.);
#26582=EDGE_CURVE('',#17427,#20666,#1135,.T.);
#26583=EDGE_CURVE('',#17839,#17822,#16327,.T.);
#26584=EDGE_CURVE('',#20654,#20675,#16328,.T.);
#26585=EDGE_CURVE('',#20678,#20671,#16329,.T.);
#26586=EDGE_CURVE('',#17820,#17803,#51,.T.);
#26587=EDGE_CURVE('',#20674,#20667,#16330,.T.);
#26588=EDGE_CURVE('',#17801,#17784,#16331,.T.);
#26589=EDGE_CURVE('',#20670,#20664,#16332,.T.);
#26590=EDGE_CURVE('',#17782,#17765,#16333,.T.);
#26591=EDGE_CURVE('',#17763,#17745,#16334,.T.);
#26592=EDGE_CURVE('',#20666,#17426,#16335,.T.);
#26593=EDGE_CURVE('',#17566,#20659,#2145,.T.);
#26594=EDGE_CURVE('',#20662,#20655,#16336,.T.);
#26595=EDGE_CURVE('',#20680,#17852,#16337,.T.);
#26596=EDGE_CURVE('',#17850,#17841,#16338,.T.);
#26597=EDGE_CURVE('',#20658,#20651,#16339,.T.);
#26598=EDGE_CURVE('',#17560,#20621,#2146,.T.);
#26599=EDGE_CURVE('',#20624,#20598,#16340,.T.);
#26600=EDGE_CURVE('',#20679,#20660,#16341,.T.);
#26601=EDGE_CURVE('',#20653,#20676,#52,.T.);
#26602=EDGE_CURVE('',#20591,#20614,#16342,.T.);
#26603=EDGE_CURVE('',#20617,#20609,#16343,.T.);
#26604=EDGE_CURVE('',#20677,#20672,#16344,.T.);
#26605=EDGE_CURVE('',#20612,#20605,#16345,.T.);
#26606=EDGE_CURVE('',#20673,#20668,#16346,.T.);
#26607=EDGE_CURVE('',#20669,#20665,#16347,.T.);
#26608=EDGE_CURVE('',#20607,#17230,#16348,.T.);
#26609=EDGE_CURVE('',#20601,#20593,#16349,.T.);
#26610=EDGE_CURVE('',#20661,#20656,#16350,.T.);
#26611=EDGE_CURVE('',#20657,#20652,#16351,.T.);
#26612=EDGE_CURVE('',#20596,#20588,#16352,.T.);
#26613=EDGE_CURVE('',#17554,#20562,#2147,.T.);
#26614=EDGE_CURVE('',#20565,#20553,#16353,.T.);
#26615=EDGE_CURVE('',#20626,#20622,#16354,.T.);
#26616=EDGE_CURVE('',#20556,#20535,#16355,.T.);
#26617=EDGE_CURVE('',#20623,#20599,#16356,.T.);
#26618=EDGE_CURVE('',#20590,#20615,#16357,.T.);
#26619=EDGE_CURVE('',#20528,#20546,#16358,.T.);
#26620=EDGE_CURVE('',#20549,#20542,#16359,.T.);
#26621=EDGE_CURVE('',#20616,#20610,#16360,.T.);
#26622=EDGE_CURVE('',#20611,#20606,#16361,.T.);
#26623=EDGE_CURVE('',#20544,#17234,#16362,.T.);
#26624=EDGE_CURVE('',#20538,#20530,#16363,.T.);
#26625=EDGE_CURVE('',#20600,#20594,#16364,.T.);
#26626=EDGE_CURVE('',#20595,#20589,#53,.T.);
#26627=EDGE_CURVE('',#20533,#20525,#16365,.T.);
#26628=EDGE_CURVE('',#17548,#20503,#2148,.T.);
#26629=EDGE_CURVE('',#20506,#20494,#16366,.T.);
#26630=EDGE_CURVE('',#20567,#20563,#16367,.T.);
#26631=EDGE_CURVE('',#20497,#20485,#16368,.T.);
#26632=EDGE_CURVE('',#20564,#20554,#16369,.T.);
#26633=EDGE_CURVE('',#20488,#20472,#16370,.T.);
#26634=EDGE_CURVE('',#20555,#20536,#16371,.T.);
#26635=EDGE_CURVE('',#20527,#20547,#16372,.T.);
#26636=EDGE_CURVE('',#20465,#20479,#16373,.T.);
#26637=EDGE_CURVE('',#20548,#20543,#16374,.T.);
#26638=EDGE_CURVE('',#20481,#17238,#16375,.T.);
#26639=EDGE_CURVE('',#20475,#20467,#16376,.T.);
#26640=EDGE_CURVE('',#20537,#20531,#54,.T.);
#26641=EDGE_CURVE('',#20532,#20526,#16377,.T.);
#26642=EDGE_CURVE('',#20470,#20462,#16378,.T.);
#26643=EDGE_CURVE('',#17542,#20444,#2149,.T.);
#26644=EDGE_CURVE('',#20447,#20435,#16379,.T.);
#26645=EDGE_CURVE('',#20508,#20504,#16380,.T.);
#26646=EDGE_CURVE('',#20438,#20426,#16381,.T.);
#26647=EDGE_CURVE('',#20505,#20495,#16382,.T.);
#26648=EDGE_CURVE('',#20429,#20417,#16383,.T.);
#26649=EDGE_CURVE('',#20496,#20486,#16384,.T.);
#26650=EDGE_CURVE('',#20420,#20408,#16385,.T.);
#26651=EDGE_CURVE('',#20487,#20473,#55,.T.);
#26652=EDGE_CURVE('',#20464,#20480,#16386,.T.);
#26653=EDGE_CURVE('',#20401,#17242,#16387,.T.);
#26654=EDGE_CURVE('',#20411,#20403,#16388,.T.);
#26655=EDGE_CURVE('',#20474,#20468,#16389,.T.);
#26656=EDGE_CURVE('',#20469,#20463,#16390,.T.);
#26657=EDGE_CURVE('',#20406,#20399,#16391,.T.);
#26658=EDGE_CURVE('',#17536,#20385,#2150,.T.);
#26659=EDGE_CURVE('',#20388,#20376,#16392,.T.);
#26660=EDGE_CURVE('',#20449,#20445,#16393,.T.);
#26661=EDGE_CURVE('',#20379,#20367,#16394,.T.);
#26662=EDGE_CURVE('',#20446,#20436,#16395,.T.);
#26663=EDGE_CURVE('',#20370,#20358,#16396,.T.);
#26664=EDGE_CURVE('',#20437,#20427,#16397,.T.);
#26665=EDGE_CURVE('',#20361,#20349,#16398,.T.);
#26666=EDGE_CURVE('',#20428,#20418,#56,.T.);
#26667=EDGE_CURVE('',#20352,#20340,#16399,.T.);
#26668=EDGE_CURVE('',#20419,#20409,#16400,.T.);
#26669=EDGE_CURVE('',#20343,#20336,#16401,.T.);
#26670=EDGE_CURVE('',#20410,#20404,#16402,.T.);
#26671=EDGE_CURVE('',#20405,#20400,#16403,.T.);
#26672=EDGE_CURVE('',#20338,#17246,#16404,.T.);
#26673=EDGE_CURVE('',#17530,#20326,#2151,.T.);
#26674=EDGE_CURVE('',#20329,#20317,#16405,.T.);
#26675=EDGE_CURVE('',#20390,#20386,#16406,.T.);
#26676=EDGE_CURVE('',#20320,#20308,#16407,.T.);
#26677=EDGE_CURVE('',#20387,#20377,#16408,.T.);
#26678=EDGE_CURVE('',#20311,#20299,#16409,.T.);
#26679=EDGE_CURVE('',#20378,#20368,#16410,.T.);
#26680=EDGE_CURVE('',#20302,#20290,#16411,.T.);
#26681=EDGE_CURVE('',#20369,#20359,#57,.T.);
#26682=EDGE_CURVE('',#20293,#20281,#16412,.T.);
#26683=EDGE_CURVE('',#20360,#20350,#16413,.T.);
#26684=EDGE_CURVE('',#20284,#20273,#16414,.T.);
#26685=EDGE_CURVE('',#20351,#20341,#16415,.T.);
#26686=EDGE_CURVE('',#20342,#20337,#16416,.T.);
#26687=EDGE_CURVE('',#20275,#17250,#16417,.T.);
#26688=EDGE_CURVE('',#17524,#20267,#2152,.T.);
#26689=EDGE_CURVE('',#20270,#20258,#16418,.T.);
#26690=EDGE_CURVE('',#20331,#20327,#16419,.T.);
#26691=EDGE_CURVE('',#20261,#20249,#16420,.T.);
#26692=EDGE_CURVE('',#20328,#20318,#16421,.T.);
#26693=EDGE_CURVE('',#20252,#20240,#16422,.T.);
#26694=EDGE_CURVE('',#20319,#20309,#16423,.T.);
#26695=EDGE_CURVE('',#20243,#20231,#16424,.T.);
#26696=EDGE_CURVE('',#20310,#20300,#58,.T.);
#26697=EDGE_CURVE('',#20234,#20222,#16425,.T.);
#26698=EDGE_CURVE('',#20301,#20291,#16426,.T.);
#26699=EDGE_CURVE('',#20225,#20214,#16427,.T.);
#26700=EDGE_CURVE('',#20292,#20282,#16428,.T.);
#26701=EDGE_CURVE('',#20283,#20274,#16429,.T.);
#26702=EDGE_CURVE('',#20216,#17254,#16430,.T.);
#26703=EDGE_CURVE('',#17518,#20208,#2153,.T.);
#26704=EDGE_CURVE('',#20211,#20199,#16431,.T.);
#26705=EDGE_CURVE('',#20272,#20268,#16432,.T.);
#26706=EDGE_CURVE('',#20202,#20190,#16433,.T.);
#26707=EDGE_CURVE('',#20269,#20259,#16434,.T.);
#26708=EDGE_CURVE('',#20193,#20181,#16435,.T.);
#26709=EDGE_CURVE('',#20260,#20250,#16436,.T.);
#26710=EDGE_CURVE('',#20184,#20172,#16437,.T.);
#26711=EDGE_CURVE('',#20251,#20241,#59,.T.);
#26712=EDGE_CURVE('',#20175,#20163,#16438,.T.);
#26713=EDGE_CURVE('',#20242,#20232,#16439,.T.);
#26714=EDGE_CURVE('',#20166,#20155,#16440,.T.);
#26715=EDGE_CURVE('',#20233,#20223,#16441,.T.);
#26716=EDGE_CURVE('',#20224,#20215,#16442,.T.);
#26717=EDGE_CURVE('',#20157,#17258,#16443,.T.);
#26718=EDGE_CURVE('',#17512,#20149,#2154,.T.);
#26719=EDGE_CURVE('',#20152,#20140,#16444,.T.);
#26720=EDGE_CURVE('',#20213,#20209,#16445,.T.);
#26721=EDGE_CURVE('',#20143,#20131,#16446,.T.);
#26722=EDGE_CURVE('',#20210,#20200,#16447,.T.);
#26723=EDGE_CURVE('',#20134,#20122,#16448,.T.);
#26724=EDGE_CURVE('',#20201,#20191,#16449,.T.);
#26725=EDGE_CURVE('',#20125,#20113,#16450,.T.);
#26726=EDGE_CURVE('',#20192,#20182,#60,.T.);
#26727=EDGE_CURVE('',#20116,#20104,#16451,.T.);
#26728=EDGE_CURVE('',#20183,#20173,#16452,.T.);
#26729=EDGE_CURVE('',#20107,#20096,#16453,.T.);
#26730=EDGE_CURVE('',#20174,#20164,#16454,.T.);
#26731=EDGE_CURVE('',#20165,#20156,#16455,.T.);
#26732=EDGE_CURVE('',#20098,#17262,#16456,.T.);
#26733=EDGE_CURVE('',#17506,#20090,#2155,.T.);
#26734=EDGE_CURVE('',#20093,#20081,#16457,.T.);
#26735=EDGE_CURVE('',#20154,#20150,#16458,.T.);
#26736=EDGE_CURVE('',#20084,#20072,#16459,.T.);
#26737=EDGE_CURVE('',#20151,#20141,#16460,.T.);
#26738=EDGE_CURVE('',#20075,#20063,#16461,.T.);
#26739=EDGE_CURVE('',#20142,#20132,#16462,.T.);
#26740=EDGE_CURVE('',#20066,#20054,#16463,.T.);
#26741=EDGE_CURVE('',#20133,#20123,#61,.T.);
#26742=EDGE_CURVE('',#20057,#20045,#16464,.T.);
#26743=EDGE_CURVE('',#20124,#20114,#16465,.T.);
#26744=EDGE_CURVE('',#20048,#20037,#16466,.T.);
#26745=EDGE_CURVE('',#20115,#20105,#16467,.T.);
#26746=EDGE_CURVE('',#20106,#20097,#16468,.T.);
#26747=EDGE_CURVE('',#20039,#17266,#16469,.T.);
#26748=EDGE_CURVE('',#17500,#20031,#2156,.T.);
#26749=EDGE_CURVE('',#20034,#20022,#16470,.T.);
#26750=EDGE_CURVE('',#20095,#20091,#16471,.T.);
#26751=EDGE_CURVE('',#20025,#20013,#16472,.T.);
#26752=EDGE_CURVE('',#20092,#20082,#16473,.T.);
#26753=EDGE_CURVE('',#20016,#20004,#16474,.T.);
#26754=EDGE_CURVE('',#20083,#20073,#16475,.T.);
#26755=EDGE_CURVE('',#20007,#19995,#16476,.T.);
#26756=EDGE_CURVE('',#20074,#20064,#62,.T.);
#26757=EDGE_CURVE('',#19998,#19986,#16477,.T.);
#26758=EDGE_CURVE('',#20065,#20055,#16478,.T.);
#26759=EDGE_CURVE('',#19989,#19978,#16479,.T.);
#26760=EDGE_CURVE('',#20056,#20046,#16480,.T.);
#26761=EDGE_CURVE('',#20047,#20038,#16481,.T.);
#26762=EDGE_CURVE('',#19980,#17270,#16482,.T.);
#26763=EDGE_CURVE('',#17494,#19972,#2157,.T.);
#26764=EDGE_CURVE('',#19975,#19963,#16483,.T.);
#26765=EDGE_CURVE('',#20036,#20032,#16484,.T.);
#26766=EDGE_CURVE('',#19966,#19954,#16485,.T.);
#26767=EDGE_CURVE('',#20033,#20023,#16486,.T.);
#26768=EDGE_CURVE('',#19957,#19945,#16487,.T.);
#26769=EDGE_CURVE('',#20024,#20014,#16488,.T.);
#26770=EDGE_CURVE('',#19948,#19936,#16489,.T.);
#26771=EDGE_CURVE('',#20015,#20005,#63,.T.);
#26772=EDGE_CURVE('',#19939,#19927,#16490,.T.);
#26773=EDGE_CURVE('',#20006,#19996,#16491,.T.);
#26774=EDGE_CURVE('',#19930,#19919,#16492,.T.);
#26775=EDGE_CURVE('',#19997,#19987,#16493,.T.);
#26776=EDGE_CURVE('',#19988,#19979,#16494,.T.);
#26777=EDGE_CURVE('',#19921,#17274,#16495,.T.);
#26778=EDGE_CURVE('',#17488,#19913,#2158,.T.);
#26779=EDGE_CURVE('',#19916,#19904,#16496,.T.);
#26780=EDGE_CURVE('',#19977,#19973,#16497,.T.);
#26781=EDGE_CURVE('',#19907,#19895,#16498,.T.);
#26782=EDGE_CURVE('',#19974,#19964,#16499,.T.);
#26783=EDGE_CURVE('',#19898,#19886,#16500,.T.);
#26784=EDGE_CURVE('',#19965,#19955,#16501,.T.);
#26785=EDGE_CURVE('',#19889,#19877,#16502,.T.);
#26786=EDGE_CURVE('',#19956,#19946,#64,.T.);
#26787=EDGE_CURVE('',#19880,#19868,#16503,.T.);
#26788=EDGE_CURVE('',#19947,#19937,#16504,.T.);
#26789=EDGE_CURVE('',#19871,#19860,#16505,.T.);
#26790=EDGE_CURVE('',#19938,#19928,#16506,.T.);
#26791=EDGE_CURVE('',#19929,#19920,#16507,.T.);
#26792=EDGE_CURVE('',#19862,#17278,#16508,.T.);
#26793=EDGE_CURVE('',#17482,#19854,#2159,.T.);
#26794=EDGE_CURVE('',#19857,#19845,#16509,.T.);
#26795=EDGE_CURVE('',#19918,#19914,#16510,.T.);
#26796=EDGE_CURVE('',#19848,#19836,#16511,.T.);
#26797=EDGE_CURVE('',#19915,#19905,#16512,.T.);
#26798=EDGE_CURVE('',#19839,#19827,#16513,.T.);
#26799=EDGE_CURVE('',#19906,#19896,#16514,.T.);
#26800=EDGE_CURVE('',#19830,#19818,#16515,.T.);
#26801=EDGE_CURVE('',#19897,#19887,#65,.T.);
#26802=EDGE_CURVE('',#19821,#19809,#16516,.T.);
#26803=EDGE_CURVE('',#19888,#19878,#16517,.T.);
#26804=EDGE_CURVE('',#19812,#19801,#16518,.T.);
#26805=EDGE_CURVE('',#19879,#19869,#16519,.T.);
#26806=EDGE_CURVE('',#19870,#19861,#16520,.T.);
#26807=EDGE_CURVE('',#19803,#17282,#16521,.T.);
#26808=EDGE_CURVE('',#17476,#19795,#2160,.T.);
#26809=EDGE_CURVE('',#19798,#19786,#16522,.T.);
#26810=EDGE_CURVE('',#19859,#19855,#16523,.T.);
#26811=EDGE_CURVE('',#19789,#19777,#16524,.T.);
#26812=EDGE_CURVE('',#19856,#19846,#16525,.T.);
#26813=EDGE_CURVE('',#19780,#19768,#16526,.T.);
#26814=EDGE_CURVE('',#19847,#19837,#16527,.T.);
#26815=EDGE_CURVE('',#19771,#19759,#16528,.T.);
#26816=EDGE_CURVE('',#19838,#19828,#66,.T.);
#26817=EDGE_CURVE('',#19762,#19750,#16529,.T.);
#26818=EDGE_CURVE('',#19829,#19819,#16530,.T.);
#26819=EDGE_CURVE('',#19753,#19742,#16531,.T.);
#26820=EDGE_CURVE('',#19820,#19810,#16532,.T.);
#26821=EDGE_CURVE('',#19811,#19802,#16533,.T.);
#26822=EDGE_CURVE('',#19744,#17286,#16534,.T.);
#26823=EDGE_CURVE('',#17470,#19736,#2161,.T.);
#26824=EDGE_CURVE('',#19739,#19727,#16535,.T.);
#26825=EDGE_CURVE('',#19800,#19796,#16536,.T.);
#26826=EDGE_CURVE('',#19730,#19718,#16537,.T.);
#26827=EDGE_CURVE('',#19797,#19787,#16538,.T.);
#26828=EDGE_CURVE('',#19721,#19709,#16539,.T.);
#26829=EDGE_CURVE('',#19788,#19778,#16540,.T.);
#26830=EDGE_CURVE('',#19712,#19700,#16541,.T.);
#26831=EDGE_CURVE('',#19779,#19769,#67,.T.);
#26832=EDGE_CURVE('',#19703,#19691,#16542,.T.);
#26833=EDGE_CURVE('',#19770,#19760,#16543,.T.);
#26834=EDGE_CURVE('',#19694,#19683,#16544,.T.);
#26835=EDGE_CURVE('',#19761,#19751,#16545,.T.);
#26836=EDGE_CURVE('',#19752,#19743,#16546,.T.);
#26837=EDGE_CURVE('',#19685,#17290,#16547,.T.);
#26838=EDGE_CURVE('',#17464,#19677,#2162,.T.);
#26839=EDGE_CURVE('',#19680,#19668,#16548,.T.);
#26840=EDGE_CURVE('',#19741,#19737,#16549,.T.);
#26841=EDGE_CURVE('',#19671,#19659,#16550,.T.);
#26842=EDGE_CURVE('',#19738,#19728,#16551,.T.);
#26843=EDGE_CURVE('',#19662,#19650,#16552,.T.);
#26844=EDGE_CURVE('',#19729,#19719,#16553,.T.);
#26845=EDGE_CURVE('',#19653,#19641,#16554,.T.);
#26846=EDGE_CURVE('',#19720,#19710,#68,.T.);
#26847=EDGE_CURVE('',#19644,#19632,#16555,.T.);
#26848=EDGE_CURVE('',#19711,#19701,#16556,.T.);
#26849=EDGE_CURVE('',#19635,#19624,#16557,.T.);
#26850=EDGE_CURVE('',#19702,#19692,#16558,.T.);
#26851=EDGE_CURVE('',#19693,#19684,#16559,.T.);
#26852=EDGE_CURVE('',#19626,#17294,#16560,.T.);
#26853=EDGE_CURVE('',#17458,#19618,#2163,.T.);
#26854=EDGE_CURVE('',#19621,#19609,#16561,.T.);
#26855=EDGE_CURVE('',#19682,#19678,#16562,.T.);
#26856=EDGE_CURVE('',#19612,#19600,#16563,.T.);
#26857=EDGE_CURVE('',#19679,#19669,#16564,.T.);
#26858=EDGE_CURVE('',#19603,#19591,#16565,.T.);
#26859=EDGE_CURVE('',#19670,#19660,#16566,.T.);
#26860=EDGE_CURVE('',#19594,#19582,#16567,.T.);
#26861=EDGE_CURVE('',#19661,#19651,#69,.T.);
#26862=EDGE_CURVE('',#19585,#19573,#16568,.T.);
#26863=EDGE_CURVE('',#19652,#19642,#16569,.T.);
#26864=EDGE_CURVE('',#19576,#19565,#16570,.T.);
#26865=EDGE_CURVE('',#19643,#19633,#16571,.T.);
#26866=EDGE_CURVE('',#19634,#19625,#16572,.T.);
#26867=EDGE_CURVE('',#19567,#17298,#16573,.T.);
#26868=EDGE_CURVE('',#17452,#19559,#2164,.T.);
#26869=EDGE_CURVE('',#19562,#19550,#16574,.T.);
#26870=EDGE_CURVE('',#19623,#19619,#16575,.T.);
#26871=EDGE_CURVE('',#19553,#19541,#16576,.T.);
#26872=EDGE_CURVE('',#19620,#19610,#16577,.T.);
#26873=EDGE_CURVE('',#19544,#19532,#16578,.T.);
#26874=EDGE_CURVE('',#19611,#19601,#16579,.T.);
#26875=EDGE_CURVE('',#19535,#19523,#16580,.T.);
#26876=EDGE_CURVE('',#19602,#19592,#70,.T.);
#26877=EDGE_CURVE('',#19526,#19514,#16581,.T.);
#26878=EDGE_CURVE('',#19593,#19583,#16582,.T.);
#26879=EDGE_CURVE('',#19517,#19506,#16583,.T.);
#26880=EDGE_CURVE('',#19584,#19574,#16584,.T.);
#26881=EDGE_CURVE('',#19575,#19566,#16585,.T.);
#26882=EDGE_CURVE('',#19508,#17302,#16586,.T.);
#26883=EDGE_CURVE('',#17446,#19500,#2165,.T.);
#26884=EDGE_CURVE('',#19503,#19491,#16587,.T.);
#26885=EDGE_CURVE('',#19564,#19560,#16588,.T.);
#26886=EDGE_CURVE('',#19494,#19482,#16589,.T.);
#26887=EDGE_CURVE('',#19561,#19551,#16590,.T.);
#26888=EDGE_CURVE('',#19485,#19473,#16591,.T.);
#26889=EDGE_CURVE('',#19552,#19542,#16592,.T.);
#26890=EDGE_CURVE('',#19476,#19464,#16593,.T.);
#26891=EDGE_CURVE('',#19543,#19533,#71,.T.);
#26892=EDGE_CURVE('',#19467,#19455,#16594,.T.);
#26893=EDGE_CURVE('',#19534,#19524,#16595,.T.);
#26894=EDGE_CURVE('',#19458,#19447,#16596,.T.);
#26895=EDGE_CURVE('',#19525,#19515,#16597,.T.);
#26896=EDGE_CURVE('',#19516,#19507,#16598,.T.);
#26897=EDGE_CURVE('',#19449,#17306,#16599,.T.);
#26898=EDGE_CURVE('',#17440,#19441,#2166,.T.);
#26899=EDGE_CURVE('',#19444,#19432,#16600,.T.);
#26900=EDGE_CURVE('',#19505,#19501,#16601,.T.);
#26901=EDGE_CURVE('',#19435,#19423,#16602,.T.);
#26902=EDGE_CURVE('',#19502,#19492,#16603,.T.);
#26903=EDGE_CURVE('',#19426,#19414,#16604,.T.);
#26904=EDGE_CURVE('',#19493,#19483,#16605,.T.);
#26905=EDGE_CURVE('',#19417,#19405,#16606,.T.);
#26906=EDGE_CURVE('',#19484,#19474,#72,.T.);
#26907=EDGE_CURVE('',#19408,#19396,#16607,.T.);
#26908=EDGE_CURVE('',#19475,#19465,#16608,.T.);
#26909=EDGE_CURVE('',#19399,#19388,#16609,.T.);
#26910=EDGE_CURVE('',#19466,#19456,#16610,.T.);
#26911=EDGE_CURVE('',#19457,#19448,#16611,.T.);
#26912=EDGE_CURVE('',#19390,#17310,#16612,.T.);
#26913=EDGE_CURVE('',#17434,#19382,#2167,.T.);
#26914=EDGE_CURVE('',#19385,#19373,#16613,.T.);
#26915=EDGE_CURVE('',#19446,#19442,#16614,.T.);
#26916=EDGE_CURVE('',#19376,#19364,#16615,.T.);
#26917=EDGE_CURVE('',#19443,#19433,#16616,.T.);
#26918=EDGE_CURVE('',#19367,#19355,#16617,.T.);
#26919=EDGE_CURVE('',#19434,#19424,#16618,.T.);
#26920=EDGE_CURVE('',#19358,#19346,#16619,.T.);
#26921=EDGE_CURVE('',#19425,#19415,#73,.T.);
#26922=EDGE_CURVE('',#19349,#19337,#16620,.T.);
#26923=EDGE_CURVE('',#19416,#19406,#16621,.T.);
#26924=EDGE_CURVE('',#19340,#19329,#16622,.T.);
#26925=EDGE_CURVE('',#19407,#19397,#16623,.T.);
#26926=EDGE_CURVE('',#19398,#19389,#16624,.T.);
#26927=EDGE_CURVE('',#19331,#17314,#16625,.T.);
#26928=EDGE_CURVE('',#17728,#19323,#2168,.T.);
#26929=EDGE_CURVE('',#19326,#19314,#16626,.T.);
#26930=EDGE_CURVE('',#19387,#19383,#16627,.T.);
#26931=EDGE_CURVE('',#19317,#19305,#16628,.T.);
#26932=EDGE_CURVE('',#19384,#19374,#16629,.T.);
#26933=EDGE_CURVE('',#19308,#19296,#16630,.T.);
#26934=EDGE_CURVE('',#19375,#19365,#16631,.T.);
#26935=EDGE_CURVE('',#19299,#19287,#16632,.T.);
#26936=EDGE_CURVE('',#19366,#19356,#74,.T.);
#26937=EDGE_CURVE('',#19290,#19278,#16633,.T.);
#26938=EDGE_CURVE('',#19357,#19347,#16634,.T.);
#26939=EDGE_CURVE('',#19281,#19270,#16635,.T.);
#26940=EDGE_CURVE('',#19348,#19338,#16636,.T.);
#26941=EDGE_CURVE('',#19339,#19330,#16637,.T.);
#26942=EDGE_CURVE('',#19272,#17318,#16638,.T.);
#26943=EDGE_CURVE('',#17722,#19264,#2169,.T.);
#26944=EDGE_CURVE('',#19267,#19255,#16639,.T.);
#26945=EDGE_CURVE('',#19328,#19324,#16640,.T.);
#26946=EDGE_CURVE('',#19258,#19246,#16641,.T.);
#26947=EDGE_CURVE('',#19325,#19315,#16642,.T.);
#26948=EDGE_CURVE('',#19249,#19237,#16643,.T.);
#26949=EDGE_CURVE('',#19316,#19306,#16644,.T.);
#26950=EDGE_CURVE('',#19240,#19228,#16645,.T.);
#26951=EDGE_CURVE('',#19307,#19297,#75,.T.);
#26952=EDGE_CURVE('',#19231,#19219,#16646,.T.);
#26953=EDGE_CURVE('',#19298,#19288,#16647,.T.);
#26954=EDGE_CURVE('',#19222,#19211,#16648,.T.);
#26955=EDGE_CURVE('',#19289,#19279,#16649,.T.);
#26956=EDGE_CURVE('',#19280,#19271,#16650,.T.);
#26957=EDGE_CURVE('',#19213,#17322,#16651,.T.);
#26958=EDGE_CURVE('',#17716,#19205,#2170,.T.);
#26959=EDGE_CURVE('',#19208,#19196,#16652,.T.);
#26960=EDGE_CURVE('',#19269,#19265,#16653,.T.);
#26961=EDGE_CURVE('',#19199,#19187,#16654,.T.);
#26962=EDGE_CURVE('',#19266,#19256,#16655,.T.);
#26963=EDGE_CURVE('',#19190,#19178,#16656,.T.);
#26964=EDGE_CURVE('',#19257,#19247,#16657,.T.);
#26965=EDGE_CURVE('',#19181,#19169,#16658,.T.);
#26966=EDGE_CURVE('',#19248,#19238,#76,.T.);
#26967=EDGE_CURVE('',#19172,#19160,#16659,.T.);
#26968=EDGE_CURVE('',#19239,#19229,#16660,.T.);
#26969=EDGE_CURVE('',#19163,#19152,#16661,.T.);
#26970=EDGE_CURVE('',#19230,#19220,#16662,.T.);
#26971=EDGE_CURVE('',#19221,#19212,#16663,.T.);
#26972=EDGE_CURVE('',#19154,#17326,#16664,.T.);
#26973=EDGE_CURVE('',#17710,#19146,#2171,.T.);
#26974=EDGE_CURVE('',#19149,#19137,#16665,.T.);
#26975=EDGE_CURVE('',#19210,#19206,#16666,.T.);
#26976=EDGE_CURVE('',#19140,#19128,#16667,.T.);
#26977=EDGE_CURVE('',#19207,#19197,#16668,.T.);
#26978=EDGE_CURVE('',#19131,#19119,#16669,.T.);
#26979=EDGE_CURVE('',#19198,#19188,#16670,.T.);
#26980=EDGE_CURVE('',#19122,#19110,#16671,.T.);
#26981=EDGE_CURVE('',#19189,#19179,#77,.T.);
#26982=EDGE_CURVE('',#19113,#19101,#16672,.T.);
#26983=EDGE_CURVE('',#19180,#19170,#16673,.T.);
#26984=EDGE_CURVE('',#19104,#19093,#16674,.T.);
#26985=EDGE_CURVE('',#19171,#19161,#16675,.T.);
#26986=EDGE_CURVE('',#19162,#19153,#16676,.T.);
#26987=EDGE_CURVE('',#19095,#17330,#16677,.T.);
#26988=EDGE_CURVE('',#17704,#19087,#2172,.T.);
#26989=EDGE_CURVE('',#19090,#19078,#16678,.T.);
#26990=EDGE_CURVE('',#19151,#19147,#16679,.T.);
#26991=EDGE_CURVE('',#19081,#19069,#16680,.T.);
#26992=EDGE_CURVE('',#19148,#19138,#16681,.T.);
#26993=EDGE_CURVE('',#19072,#19060,#16682,.T.);
#26994=EDGE_CURVE('',#19139,#19129,#16683,.T.);
#26995=EDGE_CURVE('',#19063,#19051,#16684,.T.);
#26996=EDGE_CURVE('',#19130,#19120,#78,.T.);
#26997=EDGE_CURVE('',#19054,#19042,#16685,.T.);
#26998=EDGE_CURVE('',#19121,#19111,#16686,.T.);
#26999=EDGE_CURVE('',#19045,#19034,#16687,.T.);
#27000=EDGE_CURVE('',#19112,#19102,#16688,.T.);
#27001=EDGE_CURVE('',#19103,#19094,#16689,.T.);
#27002=EDGE_CURVE('',#19036,#17334,#16690,.T.);
#27003=EDGE_CURVE('',#17698,#19028,#2173,.T.);
#27004=EDGE_CURVE('',#19031,#19019,#16691,.T.);
#27005=EDGE_CURVE('',#19092,#19088,#16692,.T.);
#27006=EDGE_CURVE('',#19022,#19010,#16693,.T.);
#27007=EDGE_CURVE('',#19089,#19079,#16694,.T.);
#27008=EDGE_CURVE('',#19013,#19001,#16695,.T.);
#27009=EDGE_CURVE('',#19080,#19070,#16696,.T.);
#27010=EDGE_CURVE('',#19004,#18992,#16697,.T.);
#27011=EDGE_CURVE('',#19071,#19061,#79,.T.);
#27012=EDGE_CURVE('',#18995,#18983,#16698,.T.);
#27013=EDGE_CURVE('',#19062,#19052,#16699,.T.);
#27014=EDGE_CURVE('',#18986,#18975,#16700,.T.);
#27015=EDGE_CURVE('',#19053,#19043,#16701,.T.);
#27016=EDGE_CURVE('',#19044,#19035,#16702,.T.);
#27017=EDGE_CURVE('',#18977,#17338,#16703,.T.);
#27018=EDGE_CURVE('',#17692,#18969,#2174,.T.);
#27019=EDGE_CURVE('',#18972,#18960,#16704,.T.);
#27020=EDGE_CURVE('',#19033,#19029,#16705,.T.);
#27021=EDGE_CURVE('',#18963,#18951,#16706,.T.);
#27022=EDGE_CURVE('',#19030,#19020,#16707,.T.);
#27023=EDGE_CURVE('',#18954,#18942,#16708,.T.);
#27024=EDGE_CURVE('',#19021,#19011,#16709,.T.);
#27025=EDGE_CURVE('',#18945,#18933,#16710,.T.);
#27026=EDGE_CURVE('',#19012,#19002,#80,.T.);
#27027=EDGE_CURVE('',#18936,#18924,#16711,.T.);
#27028=EDGE_CURVE('',#19003,#18993,#16712,.T.);
#27029=EDGE_CURVE('',#18927,#18916,#16713,.T.);
#27030=EDGE_CURVE('',#18994,#18984,#16714,.T.);
#27031=EDGE_CURVE('',#18985,#18976,#16715,.T.);
#27032=EDGE_CURVE('',#18918,#17342,#16716,.T.);
#27033=EDGE_CURVE('',#17686,#18910,#2175,.T.);
#27034=EDGE_CURVE('',#18913,#18901,#16717,.T.);
#27035=EDGE_CURVE('',#18974,#18970,#16718,.T.);
#27036=EDGE_CURVE('',#18904,#18892,#16719,.T.);
#27037=EDGE_CURVE('',#18971,#18961,#16720,.T.);
#27038=EDGE_CURVE('',#18895,#18883,#16721,.T.);
#27039=EDGE_CURVE('',#18962,#18952,#16722,.T.);
#27040=EDGE_CURVE('',#18886,#18874,#16723,.T.);
#27041=EDGE_CURVE('',#18953,#18943,#81,.T.);
#27042=EDGE_CURVE('',#18877,#18865,#16724,.T.);
#27043=EDGE_CURVE('',#18944,#18934,#16725,.T.);
#27044=EDGE_CURVE('',#18868,#18857,#16726,.T.);
#27045=EDGE_CURVE('',#18935,#18925,#16727,.T.);
#27046=EDGE_CURVE('',#18926,#18917,#16728,.T.);
#27047=EDGE_CURVE('',#18859,#17346,#16729,.T.);
#27048=EDGE_CURVE('',#17680,#18851,#2176,.T.);
#27049=EDGE_CURVE('',#18854,#18842,#16730,.T.);
#27050=EDGE_CURVE('',#18915,#18911,#16731,.T.);
#27051=EDGE_CURVE('',#18845,#18833,#16732,.T.);
#27052=EDGE_CURVE('',#18912,#18902,#16733,.T.);
#27053=EDGE_CURVE('',#18836,#18824,#16734,.T.);
#27054=EDGE_CURVE('',#18903,#18893,#16735,.T.);
#27055=EDGE_CURVE('',#18827,#18815,#16736,.T.);
#27056=EDGE_CURVE('',#18894,#18884,#82,.T.);
#27057=EDGE_CURVE('',#18818,#18806,#16737,.T.);
#27058=EDGE_CURVE('',#18885,#18875,#16738,.T.);
#27059=EDGE_CURVE('',#18809,#18798,#16739,.T.);
#27060=EDGE_CURVE('',#18876,#18866,#16740,.T.);
#27061=EDGE_CURVE('',#18867,#18858,#16741,.T.);
#27062=EDGE_CURVE('',#18800,#17350,#16742,.T.);
#27063=EDGE_CURVE('',#17674,#18792,#2177,.T.);
#27064=EDGE_CURVE('',#18795,#18783,#16743,.T.);
#27065=EDGE_CURVE('',#18856,#18852,#16744,.T.);
#27066=EDGE_CURVE('',#18786,#18774,#16745,.T.);
#27067=EDGE_CURVE('',#18853,#18843,#16746,.T.);
#27068=EDGE_CURVE('',#18777,#18765,#16747,.T.);
#27069=EDGE_CURVE('',#18844,#18834,#16748,.T.);
#27070=EDGE_CURVE('',#18768,#18756,#16749,.T.);
#27071=EDGE_CURVE('',#18835,#18825,#83,.T.);
#27072=EDGE_CURVE('',#18759,#18747,#16750,.T.);
#27073=EDGE_CURVE('',#18826,#18816,#16751,.T.);
#27074=EDGE_CURVE('',#18750,#18739,#16752,.T.);
#27075=EDGE_CURVE('',#18817,#18807,#16753,.T.);
#27076=EDGE_CURVE('',#18808,#18799,#16754,.T.);
#27077=EDGE_CURVE('',#18741,#17354,#16755,.T.);
#27078=EDGE_CURVE('',#17668,#18733,#2178,.T.);
#27079=EDGE_CURVE('',#18736,#18724,#16756,.T.);
#27080=EDGE_CURVE('',#18797,#18793,#16757,.T.);
#27081=EDGE_CURVE('',#18727,#18715,#16758,.T.);
#27082=EDGE_CURVE('',#18794,#18784,#16759,.T.);
#27083=EDGE_CURVE('',#18718,#18706,#16760,.T.);
#27084=EDGE_CURVE('',#18785,#18775,#16761,.T.);
#27085=EDGE_CURVE('',#18709,#18697,#16762,.T.);
#27086=EDGE_CURVE('',#18776,#18766,#84,.T.);
#27087=EDGE_CURVE('',#18700,#18688,#16763,.T.);
#27088=EDGE_CURVE('',#18767,#18757,#16764,.T.);
#27089=EDGE_CURVE('',#18691,#18680,#16765,.T.);
#27090=EDGE_CURVE('',#18758,#18748,#16766,.T.);
#27091=EDGE_CURVE('',#18749,#18740,#16767,.T.);
#27092=EDGE_CURVE('',#18682,#17358,#16768,.T.);
#27093=EDGE_CURVE('',#17662,#18674,#2179,.T.);
#27094=EDGE_CURVE('',#18677,#18665,#16769,.T.);
#27095=EDGE_CURVE('',#18738,#18734,#16770,.T.);
#27096=EDGE_CURVE('',#18668,#18656,#16771,.T.);
#27097=EDGE_CURVE('',#18735,#18725,#16772,.T.);
#27098=EDGE_CURVE('',#18659,#18647,#16773,.T.);
#27099=EDGE_CURVE('',#18726,#18716,#16774,.T.);
#27100=EDGE_CURVE('',#18650,#18638,#16775,.T.);
#27101=EDGE_CURVE('',#18717,#18707,#85,.T.);
#27102=EDGE_CURVE('',#18641,#18629,#16776,.T.);
#27103=EDGE_CURVE('',#18708,#18698,#16777,.T.);
#27104=EDGE_CURVE('',#18632,#18621,#16778,.T.);
#27105=EDGE_CURVE('',#18699,#18689,#16779,.T.);
#27106=EDGE_CURVE('',#18690,#18681,#16780,.T.);
#27107=EDGE_CURVE('',#18623,#17362,#16781,.T.);
#27108=EDGE_CURVE('',#17656,#18615,#2180,.T.);
#27109=EDGE_CURVE('',#18618,#18606,#16782,.T.);
#27110=EDGE_CURVE('',#18679,#18675,#16783,.T.);
#27111=EDGE_CURVE('',#18609,#18597,#16784,.T.);
#27112=EDGE_CURVE('',#18676,#18666,#16785,.T.);
#27113=EDGE_CURVE('',#18600,#18588,#16786,.T.);
#27114=EDGE_CURVE('',#18667,#18657,#16787,.T.);
#27115=EDGE_CURVE('',#18591,#18579,#16788,.T.);
#27116=EDGE_CURVE('',#18658,#18648,#86,.T.);
#27117=EDGE_CURVE('',#18582,#18570,#16789,.T.);
#27118=EDGE_CURVE('',#18649,#18639,#16790,.T.);
#27119=EDGE_CURVE('',#18573,#18562,#16791,.T.);
#27120=EDGE_CURVE('',#18640,#18630,#16792,.T.);
#27121=EDGE_CURVE('',#18631,#18622,#16793,.T.);
#27122=EDGE_CURVE('',#18564,#17366,#16794,.T.);
#27123=EDGE_CURVE('',#17650,#18556,#2181,.T.);
#27124=EDGE_CURVE('',#18559,#18547,#16795,.T.);
#27125=EDGE_CURVE('',#18620,#18616,#16796,.T.);
#27126=EDGE_CURVE('',#18550,#18538,#16797,.T.);
#27127=EDGE_CURVE('',#18617,#18607,#16798,.T.);
#27128=EDGE_CURVE('',#18541,#18529,#16799,.T.);
#27129=EDGE_CURVE('',#18608,#18598,#16800,.T.);
#27130=EDGE_CURVE('',#18532,#18520,#16801,.T.);
#27131=EDGE_CURVE('',#18599,#18589,#87,.T.);
#27132=EDGE_CURVE('',#18523,#18511,#16802,.T.);
#27133=EDGE_CURVE('',#18590,#18580,#16803,.T.);
#27134=EDGE_CURVE('',#18514,#18503,#16804,.T.);
#27135=EDGE_CURVE('',#18581,#18571,#16805,.T.);
#27136=EDGE_CURVE('',#18572,#18563,#16806,.T.);
#27137=EDGE_CURVE('',#18505,#17370,#16807,.T.);
#27138=EDGE_CURVE('',#17644,#18497,#2182,.T.);
#27139=EDGE_CURVE('',#18500,#18488,#16808,.T.);
#27140=EDGE_CURVE('',#18561,#18557,#16809,.T.);
#27141=EDGE_CURVE('',#18491,#18479,#16810,.T.);
#27142=EDGE_CURVE('',#18558,#18548,#16811,.T.);
#27143=EDGE_CURVE('',#18482,#18470,#16812,.T.);
#27144=EDGE_CURVE('',#18549,#18539,#16813,.T.);
#27145=EDGE_CURVE('',#18473,#18461,#16814,.T.);
#27146=EDGE_CURVE('',#18540,#18530,#88,.T.);
#27147=EDGE_CURVE('',#18464,#18452,#16815,.T.);
#27148=EDGE_CURVE('',#18531,#18521,#16816,.T.);
#27149=EDGE_CURVE('',#18455,#18444,#16817,.T.);
#27150=EDGE_CURVE('',#18522,#18512,#16818,.T.);
#27151=EDGE_CURVE('',#18513,#18504,#16819,.T.);
#27152=EDGE_CURVE('',#18446,#17374,#16820,.T.);
#27153=EDGE_CURVE('',#17638,#18438,#2183,.T.);
#27154=EDGE_CURVE('',#18441,#18429,#16821,.T.);
#27155=EDGE_CURVE('',#18502,#18498,#16822,.T.);
#27156=EDGE_CURVE('',#18432,#18420,#16823,.T.);
#27157=EDGE_CURVE('',#18499,#18489,#16824,.T.);
#27158=EDGE_CURVE('',#18423,#18411,#16825,.T.);
#27159=EDGE_CURVE('',#18490,#18480,#16826,.T.);
#27160=EDGE_CURVE('',#18414,#18402,#16827,.T.);
#27161=EDGE_CURVE('',#18481,#18471,#89,.T.);
#27162=EDGE_CURVE('',#18405,#18393,#16828,.T.);
#27163=EDGE_CURVE('',#18472,#18462,#16829,.T.);
#27164=EDGE_CURVE('',#18396,#18385,#16830,.T.);
#27165=EDGE_CURVE('',#18463,#18453,#16831,.T.);
#27166=EDGE_CURVE('',#18454,#18445,#16832,.T.);
#27167=EDGE_CURVE('',#18387,#17378,#16833,.T.);
#27168=EDGE_CURVE('',#17632,#18379,#2184,.T.);
#27169=EDGE_CURVE('',#18382,#18370,#16834,.T.);
#27170=EDGE_CURVE('',#18443,#18439,#16835,.T.);
#27171=EDGE_CURVE('',#18373,#18361,#16836,.T.);
#27172=EDGE_CURVE('',#18440,#18430,#16837,.T.);
#27173=EDGE_CURVE('',#18364,#18352,#16838,.T.);
#27174=EDGE_CURVE('',#18431,#18421,#16839,.T.);
#27175=EDGE_CURVE('',#18355,#18343,#16840,.T.);
#27176=EDGE_CURVE('',#18422,#18412,#90,.T.);
#27177=EDGE_CURVE('',#18346,#18334,#16841,.T.);
#27178=EDGE_CURVE('',#18413,#18403,#16842,.T.);
#27179=EDGE_CURVE('',#18337,#18326,#16843,.T.);
#27180=EDGE_CURVE('',#18404,#18394,#16844,.T.);
#27181=EDGE_CURVE('',#18395,#18386,#16845,.T.);
#27182=EDGE_CURVE('',#18328,#17382,#16846,.T.);
#27183=EDGE_CURVE('',#17626,#18320,#2185,.T.);
#27184=EDGE_CURVE('',#18323,#18311,#16847,.T.);
#27185=EDGE_CURVE('',#18384,#18380,#16848,.T.);
#27186=EDGE_CURVE('',#18314,#18302,#16849,.T.);
#27187=EDGE_CURVE('',#18381,#18371,#16850,.T.);
#27188=EDGE_CURVE('',#18305,#18293,#16851,.T.);
#27189=EDGE_CURVE('',#18372,#18362,#16852,.T.);
#27190=EDGE_CURVE('',#18296,#18284,#16853,.T.);
#27191=EDGE_CURVE('',#18363,#18353,#91,.T.);
#27192=EDGE_CURVE('',#18287,#18275,#16854,.T.);
#27193=EDGE_CURVE('',#18354,#18344,#16855,.T.);
#27194=EDGE_CURVE('',#18278,#18267,#16856,.T.);
#27195=EDGE_CURVE('',#18345,#18335,#16857,.T.);
#27196=EDGE_CURVE('',#18336,#18327,#16858,.T.);
#27197=EDGE_CURVE('',#18269,#17386,#16859,.T.);
#27198=EDGE_CURVE('',#17620,#18261,#2186,.T.);
#27199=EDGE_CURVE('',#18264,#18252,#16860,.T.);
#27200=EDGE_CURVE('',#18325,#18321,#16861,.T.);
#27201=EDGE_CURVE('',#18255,#18243,#16862,.T.);
#27202=EDGE_CURVE('',#18322,#18312,#16863,.T.);
#27203=EDGE_CURVE('',#18246,#18234,#16864,.T.);
#27204=EDGE_CURVE('',#18313,#18303,#16865,.T.);
#27205=EDGE_CURVE('',#18237,#18225,#16866,.T.);
#27206=EDGE_CURVE('',#18304,#18294,#92,.T.);
#27207=EDGE_CURVE('',#18228,#18216,#16867,.T.);
#27208=EDGE_CURVE('',#18295,#18285,#16868,.T.);
#27209=EDGE_CURVE('',#18219,#18208,#16869,.T.);
#27210=EDGE_CURVE('',#18286,#18276,#16870,.T.);
#27211=EDGE_CURVE('',#18277,#18268,#16871,.T.);
#27212=EDGE_CURVE('',#18210,#17390,#16872,.T.);
#27213=EDGE_CURVE('',#17614,#18202,#2187,.T.);
#27214=EDGE_CURVE('',#18205,#18193,#16873,.T.);
#27215=EDGE_CURVE('',#18266,#18262,#16874,.T.);
#27216=EDGE_CURVE('',#18196,#18184,#16875,.T.);
#27217=EDGE_CURVE('',#18263,#18253,#16876,.T.);
#27218=EDGE_CURVE('',#18187,#18175,#16877,.T.);
#27219=EDGE_CURVE('',#18254,#18244,#16878,.T.);
#27220=EDGE_CURVE('',#18178,#18166,#16879,.T.);
#27221=EDGE_CURVE('',#18245,#18235,#93,.T.);
#27222=EDGE_CURVE('',#18169,#18157,#16880,.T.);
#27223=EDGE_CURVE('',#18236,#18226,#16881,.T.);
#27224=EDGE_CURVE('',#18160,#18149,#16882,.T.);
#27225=EDGE_CURVE('',#18227,#18217,#16883,.T.);
#27226=EDGE_CURVE('',#18218,#18209,#16884,.T.);
#27227=EDGE_CURVE('',#18151,#17394,#16885,.T.);
#27228=EDGE_CURVE('',#18144,#18134,#16886,.T.);
#27229=EDGE_CURVE('',#18207,#18203,#16887,.T.);
#27230=EDGE_CURVE('',#17608,#18141,#2188,.T.);
#27231=EDGE_CURVE('',#18137,#18125,#16888,.T.);
#27232=EDGE_CURVE('',#18204,#18194,#16889,.T.);
#27233=EDGE_CURVE('',#18128,#18116,#16890,.T.);
#27234=EDGE_CURVE('',#18195,#18185,#16891,.T.);
#27235=EDGE_CURVE('',#18119,#18107,#16892,.T.);
#27236=EDGE_CURVE('',#18186,#18176,#94,.T.);
#27237=EDGE_CURVE('',#18110,#18098,#16893,.T.);
#27238=EDGE_CURVE('',#18177,#18167,#16894,.T.);
#27239=EDGE_CURVE('',#18101,#18090,#16895,.T.);
#27240=EDGE_CURVE('',#18168,#18158,#16896,.T.);
#27241=EDGE_CURVE('',#18159,#18150,#16897,.T.);
#27242=EDGE_CURVE('',#18092,#17398,#16898,.T.);
#27243=EDGE_CURVE('',#17602,#18084,#2189,.T.);
#27244=EDGE_CURVE('',#18087,#18073,#16899,.T.);
#27245=EDGE_CURVE('',#18148,#18142,#16900,.T.);
#27246=EDGE_CURVE('',#18076,#18066,#16901,.T.);
#27247=EDGE_CURVE('',#18143,#18135,#16902,.T.);
#27248=EDGE_CURVE('',#18069,#18057,#16903,.T.);
#27249=EDGE_CURVE('',#18136,#18126,#16904,.T.);
#27250=EDGE_CURVE('',#18060,#18048,#16905,.T.);
#27251=EDGE_CURVE('',#18127,#18117,#95,.T.);
#27252=EDGE_CURVE('',#18051,#18039,#16906,.T.);
#27253=EDGE_CURVE('',#18118,#18108,#16907,.T.);
#27254=EDGE_CURVE('',#18042,#18031,#16908,.T.);
#27255=EDGE_CURVE('',#18109,#18099,#16909,.T.);
#27256=EDGE_CURVE('',#18100,#18091,#16910,.T.);
#27257=EDGE_CURVE('',#18033,#17402,#16911,.T.);
#27258=EDGE_CURVE('',#17596,#18025,#2190,.T.);
#27259=EDGE_CURVE('',#18028,#18016,#16912,.T.);
#27260=EDGE_CURVE('',#18089,#18085,#16913,.T.);
#27261=EDGE_CURVE('',#18019,#18005,#16914,.T.);
#27262=EDGE_CURVE('',#18086,#18074,#16915,.T.);
#27263=EDGE_CURVE('',#18008,#17998,#16916,.T.);
#27264=EDGE_CURVE('',#18075,#18067,#16917,.T.);
#27265=EDGE_CURVE('',#18001,#17989,#16918,.T.);
#27266=EDGE_CURVE('',#18068,#18058,#96,.T.);
#27267=EDGE_CURVE('',#17992,#17980,#16919,.T.);
#27268=EDGE_CURVE('',#18059,#18049,#16920,.T.);
#27269=EDGE_CURVE('',#17983,#17972,#16921,.T.);
#27270=EDGE_CURVE('',#18050,#18040,#16922,.T.);
#27271=EDGE_CURVE('',#18041,#18032,#16923,.T.);
#27272=EDGE_CURVE('',#17974,#17406,#16924,.T.);
#27273=EDGE_CURVE('',#17590,#17966,#2191,.T.);
#27274=EDGE_CURVE('',#17969,#17957,#16925,.T.);
#27275=EDGE_CURVE('',#18030,#18026,#16926,.T.);
#27276=EDGE_CURVE('',#17960,#17948,#16927,.T.);
#27277=EDGE_CURVE('',#18027,#18017,#16928,.T.);
#27278=EDGE_CURVE('',#17951,#17937,#16929,.T.);
#27279=EDGE_CURVE('',#18018,#18006,#16930,.T.);
#27280=EDGE_CURVE('',#17940,#17930,#16931,.T.);
#27281=EDGE_CURVE('',#18007,#17999,#97,.T.);
#27282=EDGE_CURVE('',#17933,#17921,#16932,.T.);
#27283=EDGE_CURVE('',#18000,#17990,#16933,.T.);
#27284=EDGE_CURVE('',#17924,#17913,#16934,.T.);
#27285=EDGE_CURVE('',#17991,#17981,#16935,.T.);
#27286=EDGE_CURVE('',#17982,#17973,#16936,.T.);
#27287=EDGE_CURVE('',#17915,#17410,#16937,.T.);
#27288=EDGE_CURVE('',#17584,#17907,#2192,.T.);
#27289=EDGE_CURVE('',#17910,#17898,#16938,.T.);
#27290=EDGE_CURVE('',#17971,#17967,#16939,.T.);
#27291=EDGE_CURVE('',#17901,#17889,#16940,.T.);
#27292=EDGE_CURVE('',#17968,#17958,#16941,.T.);
#27293=EDGE_CURVE('',#17892,#17880,#16942,.T.);
#27294=EDGE_CURVE('',#17959,#17949,#16943,.T.);
#27295=EDGE_CURVE('',#17883,#17869,#16944,.T.);
#27296=EDGE_CURVE('',#17950,#17938,#98,.T.);
#27297=EDGE_CURVE('',#17872,#17862,#16945,.T.);
#27298=EDGE_CURVE('',#17939,#17931,#16946,.T.);
#27299=EDGE_CURVE('',#17865,#17854,#16947,.T.);
#27300=EDGE_CURVE('',#17932,#17922,#16948,.T.);
#27301=EDGE_CURVE('',#17923,#17914,#16949,.T.);
#27302=EDGE_CURVE('',#17856,#17414,#16950,.T.);
#27303=EDGE_CURVE('',#17578,#17832,#2193,.T.);
#27304=EDGE_CURVE('',#17836,#17813,#16951,.T.);
#27305=EDGE_CURVE('',#17912,#17908,#16952,.T.);
#27306=EDGE_CURVE('',#17817,#17794,#16953,.T.);
#27307=EDGE_CURVE('',#17909,#17899,#16954,.T.);
#27308=EDGE_CURVE('',#17798,#17775,#16955,.T.);
#27309=EDGE_CURVE('',#17900,#17890,#16956,.T.);
#27310=EDGE_CURVE('',#17779,#17756,#16957,.T.);
#27311=EDGE_CURVE('',#17891,#17881,#99,.T.);
#27312=EDGE_CURVE('',#17760,#17737,#16958,.T.);
#27313=EDGE_CURVE('',#17882,#17870,#16959,.T.);
#27314=EDGE_CURVE('',#17741,#17731,#16960,.T.);
#27315=EDGE_CURVE('',#17871,#17863,#16961,.T.);
#27316=EDGE_CURVE('',#17864,#17855,#16962,.T.);
#27317=EDGE_CURVE('',#17733,#17418,#16963,.T.);
#27318=EDGE_CURVE('',#17572,#17851,#2194,.T.);
#27319=EDGE_CURVE('',#17849,#17840,#16964,.T.);
#27320=EDGE_CURVE('',#17848,#17833,#16965,.T.);
#27321=EDGE_CURVE('',#17838,#17821,#16966,.T.);
#27322=EDGE_CURVE('',#17835,#17814,#16967,.T.);
#27323=EDGE_CURVE('',#17819,#17802,#16968,.T.);
#27324=EDGE_CURVE('',#17816,#17795,#16969,.T.);
#27325=EDGE_CURVE('',#17800,#17783,#16970,.T.);
#27326=EDGE_CURVE('',#17797,#17776,#100,.T.);
#27327=EDGE_CURVE('',#17781,#17764,#16971,.T.);
#27328=EDGE_CURVE('',#17778,#17757,#16972,.T.);
#27329=EDGE_CURVE('',#17762,#17744,#16973,.T.);
#27330=EDGE_CURVE('',#17759,#17738,#16974,.T.);
#27331=EDGE_CURVE('',#17740,#17732,#16975,.T.);
#27332=EDGE_CURVE('',#17743,#17422,#16976,.T.);
#28264=ORIENTED_EDGE('',*,*,#21274,.T.);
#28265=ORIENTED_EDGE('',*,*,#21275,.T.);
#28266=ORIENTED_EDGE('',*,*,#21276,.F.);
#28267=ORIENTED_EDGE('',*,*,#21275,.F.);
#28268=ORIENTED_EDGE('',*,*,#21277,.T.);
#28269=ORIENTED_EDGE('',*,*,#21278,.T.);
#28270=ORIENTED_EDGE('',*,*,#21279,.F.);
#28271=ORIENTED_EDGE('',*,*,#21278,.F.);
#28272=ORIENTED_EDGE('',*,*,#21280,.T.);
#28273=ORIENTED_EDGE('',*,*,#21281,.T.);
#28274=ORIENTED_EDGE('',*,*,#21282,.T.);
#28275=ORIENTED_EDGE('',*,*,#21283,.T.);
#28276=ORIENTED_EDGE('',*,*,#21284,.T.);
#28277=ORIENTED_EDGE('',*,*,#21285,.T.);
#28278=ORIENTED_EDGE('',*,*,#21286,.T.);
#28279=ORIENTED_EDGE('',*,*,#21287,.T.);
#28280=ORIENTED_EDGE('',*,*,#21288,.T.);
#28281=ORIENTED_EDGE('',*,*,#21289,.T.);
#28282=ORIENTED_EDGE('',*,*,#21290,.T.);
#28283=ORIENTED_EDGE('',*,*,#21291,.T.);
#28284=ORIENTED_EDGE('',*,*,#21292,.T.);
#28285=ORIENTED_EDGE('',*,*,#21293,.T.);
#28286=ORIENTED_EDGE('',*,*,#21294,.T.);
#28287=ORIENTED_EDGE('',*,*,#21295,.T.);
#28288=ORIENTED_EDGE('',*,*,#21296,.T.);
#28289=ORIENTED_EDGE('',*,*,#21297,.T.);
#28290=ORIENTED_EDGE('',*,*,#21298,.T.);
#28291=ORIENTED_EDGE('',*,*,#21299,.T.);
#28292=ORIENTED_EDGE('',*,*,#21300,.T.);
#28293=ORIENTED_EDGE('',*,*,#21301,.T.);
#28294=ORIENTED_EDGE('',*,*,#21302,.T.);
#28295=ORIENTED_EDGE('',*,*,#21303,.T.);
#28296=ORIENTED_EDGE('',*,*,#21304,.T.);
#28297=ORIENTED_EDGE('',*,*,#21305,.T.);
#28298=ORIENTED_EDGE('',*,*,#21306,.T.);
#28299=ORIENTED_EDGE('',*,*,#21307,.T.);
#28300=ORIENTED_EDGE('',*,*,#21308,.T.);
#28301=ORIENTED_EDGE('',*,*,#21309,.T.);
#28302=ORIENTED_EDGE('',*,*,#21310,.T.);
#28303=ORIENTED_EDGE('',*,*,#21311,.T.);
#28304=ORIENTED_EDGE('',*,*,#21312,.T.);
#28305=ORIENTED_EDGE('',*,*,#21313,.T.);
#28306=ORIENTED_EDGE('',*,*,#21314,.T.);
#28307=ORIENTED_EDGE('',*,*,#21315,.T.);
#28308=ORIENTED_EDGE('',*,*,#21316,.T.);
#28309=ORIENTED_EDGE('',*,*,#21317,.T.);
#28310=ORIENTED_EDGE('',*,*,#21318,.T.);
#28311=ORIENTED_EDGE('',*,*,#21319,.T.);
#28312=ORIENTED_EDGE('',*,*,#21320,.T.);
#28313=ORIENTED_EDGE('',*,*,#21321,.T.);
#28314=ORIENTED_EDGE('',*,*,#21322,.T.);
#28315=ORIENTED_EDGE('',*,*,#21323,.T.);
#28316=ORIENTED_EDGE('',*,*,#21324,.T.);
#28317=ORIENTED_EDGE('',*,*,#21325,.T.);
#28318=ORIENTED_EDGE('',*,*,#21326,.T.);
#28319=ORIENTED_EDGE('',*,*,#21327,.T.);
#28320=ORIENTED_EDGE('',*,*,#21328,.T.);
#28321=ORIENTED_EDGE('',*,*,#21329,.T.);
#28322=ORIENTED_EDGE('',*,*,#21330,.T.);
#28323=ORIENTED_EDGE('',*,*,#21331,.T.);
#28324=ORIENTED_EDGE('',*,*,#21332,.T.);
#28325=ORIENTED_EDGE('',*,*,#21333,.T.);
#28326=ORIENTED_EDGE('',*,*,#21334,.T.);
#28327=ORIENTED_EDGE('',*,*,#21335,.T.);
#28328=ORIENTED_EDGE('',*,*,#21336,.T.);
#28329=ORIENTED_EDGE('',*,*,#21337,.T.);
#28330=ORIENTED_EDGE('',*,*,#21338,.T.);
#28331=ORIENTED_EDGE('',*,*,#21339,.T.);
#28332=ORIENTED_EDGE('',*,*,#21340,.T.);
#28333=ORIENTED_EDGE('',*,*,#21341,.T.);
#28334=ORIENTED_EDGE('',*,*,#21342,.T.);
#28335=ORIENTED_EDGE('',*,*,#21343,.T.);
#28336=ORIENTED_EDGE('',*,*,#21344,.T.);
#28337=ORIENTED_EDGE('',*,*,#21345,.T.);
#28338=ORIENTED_EDGE('',*,*,#21346,.T.);
#28339=ORIENTED_EDGE('',*,*,#21347,.T.);
#28340=ORIENTED_EDGE('',*,*,#21348,.T.);
#28341=ORIENTED_EDGE('',*,*,#21349,.T.);
#28342=ORIENTED_EDGE('',*,*,#21350,.T.);
#28343=ORIENTED_EDGE('',*,*,#21351,.T.);
#28344=ORIENTED_EDGE('',*,*,#21352,.T.);
#28345=ORIENTED_EDGE('',*,*,#21353,.T.);
#28346=ORIENTED_EDGE('',*,*,#21354,.T.);
#28347=ORIENTED_EDGE('',*,*,#21355,.T.);
#28348=ORIENTED_EDGE('',*,*,#21356,.T.);
#28349=ORIENTED_EDGE('',*,*,#21357,.T.);
#28350=ORIENTED_EDGE('',*,*,#21358,.T.);
#28351=ORIENTED_EDGE('',*,*,#21359,.T.);
#28352=ORIENTED_EDGE('',*,*,#21360,.T.);
#28353=ORIENTED_EDGE('',*,*,#21361,.T.);
#28354=ORIENTED_EDGE('',*,*,#21362,.T.);
#28355=ORIENTED_EDGE('',*,*,#21363,.T.);
#28356=ORIENTED_EDGE('',*,*,#21364,.T.);
#28357=ORIENTED_EDGE('',*,*,#21365,.T.);
#28358=ORIENTED_EDGE('',*,*,#21366,.T.);
#28359=ORIENTED_EDGE('',*,*,#21367,.T.);
#28360=ORIENTED_EDGE('',*,*,#21368,.T.);
#28361=ORIENTED_EDGE('',*,*,#21369,.T.);
#28362=ORIENTED_EDGE('',*,*,#21370,.T.);
#28363=ORIENTED_EDGE('',*,*,#21371,.T.);
#28364=ORIENTED_EDGE('',*,*,#21372,.T.);
#28365=ORIENTED_EDGE('',*,*,#21373,.T.);
#28366=ORIENTED_EDGE('',*,*,#21374,.T.);
#28367=ORIENTED_EDGE('',*,*,#21375,.T.);
#28368=ORIENTED_EDGE('',*,*,#21376,.T.);
#28369=ORIENTED_EDGE('',*,*,#21377,.T.);
#28370=ORIENTED_EDGE('',*,*,#21378,.T.);
#28371=ORIENTED_EDGE('',*,*,#21379,.T.);
#28372=ORIENTED_EDGE('',*,*,#21380,.T.);
#28373=ORIENTED_EDGE('',*,*,#21381,.T.);
#28374=ORIENTED_EDGE('',*,*,#21382,.T.);
#28375=ORIENTED_EDGE('',*,*,#21383,.T.);
#28376=ORIENTED_EDGE('',*,*,#21384,.T.);
#28377=ORIENTED_EDGE('',*,*,#21385,.T.);
#28378=ORIENTED_EDGE('',*,*,#21386,.T.);
#28379=ORIENTED_EDGE('',*,*,#21387,.T.);
#28380=ORIENTED_EDGE('',*,*,#21388,.T.);
#28381=ORIENTED_EDGE('',*,*,#21389,.T.);
#28382=ORIENTED_EDGE('',*,*,#21390,.T.);
#28383=ORIENTED_EDGE('',*,*,#21391,.T.);
#28384=ORIENTED_EDGE('',*,*,#21392,.T.);
#28385=ORIENTED_EDGE('',*,*,#21393,.T.);
#28386=ORIENTED_EDGE('',*,*,#21394,.T.);
#28387=ORIENTED_EDGE('',*,*,#21395,.T.);
#28388=ORIENTED_EDGE('',*,*,#21396,.T.);
#28389=ORIENTED_EDGE('',*,*,#21397,.T.);
#28390=ORIENTED_EDGE('',*,*,#21398,.T.);
#28391=ORIENTED_EDGE('',*,*,#21399,.T.);
#28392=ORIENTED_EDGE('',*,*,#21400,.T.);
#28393=ORIENTED_EDGE('',*,*,#21401,.T.);
#28394=ORIENTED_EDGE('',*,*,#21402,.T.);
#28395=ORIENTED_EDGE('',*,*,#21403,.T.);
#28396=ORIENTED_EDGE('',*,*,#21404,.T.);
#28397=ORIENTED_EDGE('',*,*,#21405,.T.);
#28398=ORIENTED_EDGE('',*,*,#21406,.T.);
#28399=ORIENTED_EDGE('',*,*,#21407,.T.);
#28400=ORIENTED_EDGE('',*,*,#21408,.T.);
#28401=ORIENTED_EDGE('',*,*,#21409,.T.);
#28402=ORIENTED_EDGE('',*,*,#21410,.T.);
#28403=ORIENTED_EDGE('',*,*,#21411,.T.);
#28404=ORIENTED_EDGE('',*,*,#21412,.T.);
#28405=ORIENTED_EDGE('',*,*,#21413,.T.);
#28406=ORIENTED_EDGE('',*,*,#21414,.T.);
#28407=ORIENTED_EDGE('',*,*,#21415,.T.);
#28408=ORIENTED_EDGE('',*,*,#21416,.T.);
#28409=ORIENTED_EDGE('',*,*,#21417,.T.);
#28410=ORIENTED_EDGE('',*,*,#21418,.T.);
#28411=ORIENTED_EDGE('',*,*,#21419,.T.);
#28412=ORIENTED_EDGE('',*,*,#21420,.T.);
#28413=ORIENTED_EDGE('',*,*,#21421,.T.);
#28414=ORIENTED_EDGE('',*,*,#21422,.T.);
#28415=ORIENTED_EDGE('',*,*,#21423,.T.);
#28416=ORIENTED_EDGE('',*,*,#21424,.T.);
#28417=ORIENTED_EDGE('',*,*,#21425,.T.);
#28418=ORIENTED_EDGE('',*,*,#21426,.T.);
#28419=ORIENTED_EDGE('',*,*,#21427,.T.);
#28420=ORIENTED_EDGE('',*,*,#21428,.T.);
#28421=ORIENTED_EDGE('',*,*,#21429,.T.);
#28422=ORIENTED_EDGE('',*,*,#21430,.T.);
#28423=ORIENTED_EDGE('',*,*,#21431,.T.);
#28424=ORIENTED_EDGE('',*,*,#21432,.T.);
#28425=ORIENTED_EDGE('',*,*,#21433,.T.);
#28426=ORIENTED_EDGE('',*,*,#21434,.T.);
#28427=ORIENTED_EDGE('',*,*,#21435,.T.);
#28428=ORIENTED_EDGE('',*,*,#21436,.T.);
#28429=ORIENTED_EDGE('',*,*,#21437,.T.);
#28430=ORIENTED_EDGE('',*,*,#21438,.T.);
#28431=ORIENTED_EDGE('',*,*,#21439,.T.);
#28432=ORIENTED_EDGE('',*,*,#21440,.T.);
#28433=ORIENTED_EDGE('',*,*,#21441,.T.);
#28434=ORIENTED_EDGE('',*,*,#21442,.T.);
#28435=ORIENTED_EDGE('',*,*,#21443,.T.);
#28436=ORIENTED_EDGE('',*,*,#21444,.T.);
#28437=ORIENTED_EDGE('',*,*,#21445,.T.);
#28438=ORIENTED_EDGE('',*,*,#21446,.T.);
#28439=ORIENTED_EDGE('',*,*,#21447,.T.);
#28440=ORIENTED_EDGE('',*,*,#21448,.T.);
#28441=ORIENTED_EDGE('',*,*,#21449,.T.);
#28442=ORIENTED_EDGE('',*,*,#21450,.T.);
#28443=ORIENTED_EDGE('',*,*,#21451,.T.);
#28444=ORIENTED_EDGE('',*,*,#21452,.T.);
#28445=ORIENTED_EDGE('',*,*,#21453,.T.);
#28446=ORIENTED_EDGE('',*,*,#21454,.T.);
#28447=ORIENTED_EDGE('',*,*,#21455,.T.);
#28448=ORIENTED_EDGE('',*,*,#21456,.T.);
#28449=ORIENTED_EDGE('',*,*,#21457,.T.);
#28450=ORIENTED_EDGE('',*,*,#21458,.T.);
#28451=ORIENTED_EDGE('',*,*,#21459,.T.);
#28452=ORIENTED_EDGE('',*,*,#21460,.T.);
#28453=ORIENTED_EDGE('',*,*,#21461,.T.);
#28454=ORIENTED_EDGE('',*,*,#21462,.T.);
#28455=ORIENTED_EDGE('',*,*,#21463,.T.);
#28456=ORIENTED_EDGE('',*,*,#21464,.T.);
#28457=ORIENTED_EDGE('',*,*,#21465,.T.);
#28458=ORIENTED_EDGE('',*,*,#21466,.T.);
#28459=ORIENTED_EDGE('',*,*,#21467,.T.);
#28460=ORIENTED_EDGE('',*,*,#21468,.T.);
#28461=ORIENTED_EDGE('',*,*,#21469,.T.);
#28462=ORIENTED_EDGE('',*,*,#21470,.T.);
#28463=ORIENTED_EDGE('',*,*,#21471,.T.);
#28464=ORIENTED_EDGE('',*,*,#21472,.T.);
#28465=ORIENTED_EDGE('',*,*,#21473,.T.);
#28466=ORIENTED_EDGE('',*,*,#21474,.T.);
#28467=ORIENTED_EDGE('',*,*,#21475,.T.);
#28468=ORIENTED_EDGE('',*,*,#21476,.T.);
#28469=ORIENTED_EDGE('',*,*,#21477,.T.);
#28470=ORIENTED_EDGE('',*,*,#21478,.T.);
#28471=ORIENTED_EDGE('',*,*,#21479,.T.);
#28472=ORIENTED_EDGE('',*,*,#21480,.T.);
#28473=ORIENTED_EDGE('',*,*,#21481,.T.);
#28474=ORIENTED_EDGE('',*,*,#21482,.F.);
#28475=ORIENTED_EDGE('',*,*,#21481,.F.);
#28476=ORIENTED_EDGE('',*,*,#21483,.T.);
#28477=ORIENTED_EDGE('',*,*,#21484,.T.);
#28478=ORIENTED_EDGE('',*,*,#21485,.T.);
#28479=ORIENTED_EDGE('',*,*,#21486,.T.);
#28480=ORIENTED_EDGE('',*,*,#21487,.T.);
#28481=ORIENTED_EDGE('',*,*,#21488,.T.);
#28482=ORIENTED_EDGE('',*,*,#21489,.T.);
#28483=ORIENTED_EDGE('',*,*,#21490,.T.);
#28484=ORIENTED_EDGE('',*,*,#21491,.T.);
#28485=ORIENTED_EDGE('',*,*,#21492,.T.);
#28486=ORIENTED_EDGE('',*,*,#21493,.T.);
#28487=ORIENTED_EDGE('',*,*,#21494,.T.);
#28488=ORIENTED_EDGE('',*,*,#21495,.T.);
#28489=ORIENTED_EDGE('',*,*,#21496,.T.);
#28490=ORIENTED_EDGE('',*,*,#21497,.T.);
#28491=ORIENTED_EDGE('',*,*,#21498,.T.);
#28492=ORIENTED_EDGE('',*,*,#21499,.T.);
#28493=ORIENTED_EDGE('',*,*,#21500,.T.);
#28494=ORIENTED_EDGE('',*,*,#21501,.T.);
#28495=ORIENTED_EDGE('',*,*,#21502,.T.);
#28496=ORIENTED_EDGE('',*,*,#21503,.T.);
#28497=ORIENTED_EDGE('',*,*,#21504,.T.);
#28498=ORIENTED_EDGE('',*,*,#21505,.T.);
#28499=ORIENTED_EDGE('',*,*,#21506,.T.);
#28500=ORIENTED_EDGE('',*,*,#21507,.T.);
#28501=ORIENTED_EDGE('',*,*,#21508,.T.);
#28502=ORIENTED_EDGE('',*,*,#21509,.T.);
#28503=ORIENTED_EDGE('',*,*,#21510,.T.);
#28504=ORIENTED_EDGE('',*,*,#21511,.T.);
#28505=ORIENTED_EDGE('',*,*,#21512,.T.);
#28506=ORIENTED_EDGE('',*,*,#21513,.T.);
#28507=ORIENTED_EDGE('',*,*,#21514,.T.);
#28508=ORIENTED_EDGE('',*,*,#21515,.T.);
#28509=ORIENTED_EDGE('',*,*,#21516,.T.);
#28510=ORIENTED_EDGE('',*,*,#21517,.T.);
#28511=ORIENTED_EDGE('',*,*,#21518,.T.);
#28512=ORIENTED_EDGE('',*,*,#21519,.T.);
#28513=ORIENTED_EDGE('',*,*,#21520,.T.);
#28514=ORIENTED_EDGE('',*,*,#21521,.T.);
#28515=ORIENTED_EDGE('',*,*,#21522,.T.);
#28516=ORIENTED_EDGE('',*,*,#21523,.T.);
#28517=ORIENTED_EDGE('',*,*,#21524,.T.);
#28518=ORIENTED_EDGE('',*,*,#21525,.T.);
#28519=ORIENTED_EDGE('',*,*,#21526,.T.);
#28520=ORIENTED_EDGE('',*,*,#21527,.T.);
#28521=ORIENTED_EDGE('',*,*,#21528,.T.);
#28522=ORIENTED_EDGE('',*,*,#21529,.T.);
#28523=ORIENTED_EDGE('',*,*,#21530,.T.);
#28524=ORIENTED_EDGE('',*,*,#21531,.T.);
#28525=ORIENTED_EDGE('',*,*,#21532,.T.);
#28526=ORIENTED_EDGE('',*,*,#21533,.T.);
#28527=ORIENTED_EDGE('',*,*,#21534,.T.);
#28528=ORIENTED_EDGE('',*,*,#21535,.T.);
#28529=ORIENTED_EDGE('',*,*,#21536,.T.);
#28530=ORIENTED_EDGE('',*,*,#21537,.T.);
#28531=ORIENTED_EDGE('',*,*,#21538,.T.);
#28532=ORIENTED_EDGE('',*,*,#21539,.T.);
#28533=ORIENTED_EDGE('',*,*,#21540,.T.);
#28534=ORIENTED_EDGE('',*,*,#21541,.T.);
#28535=ORIENTED_EDGE('',*,*,#21542,.T.);
#28536=ORIENTED_EDGE('',*,*,#21543,.T.);
#28537=ORIENTED_EDGE('',*,*,#21544,.T.);
#28538=ORIENTED_EDGE('',*,*,#21545,.T.);
#28539=ORIENTED_EDGE('',*,*,#21546,.T.);
#28540=ORIENTED_EDGE('',*,*,#21547,.T.);
#28541=ORIENTED_EDGE('',*,*,#21548,.T.);
#28542=ORIENTED_EDGE('',*,*,#21549,.T.);
#28543=ORIENTED_EDGE('',*,*,#21550,.T.);
#28544=ORIENTED_EDGE('',*,*,#21551,.T.);
#28545=ORIENTED_EDGE('',*,*,#21552,.T.);
#28546=ORIENTED_EDGE('',*,*,#21553,.T.);
#28547=ORIENTED_EDGE('',*,*,#21554,.T.);
#28548=ORIENTED_EDGE('',*,*,#21555,.T.);
#28549=ORIENTED_EDGE('',*,*,#21556,.T.);
#28550=ORIENTED_EDGE('',*,*,#21557,.T.);
#28551=ORIENTED_EDGE('',*,*,#21558,.T.);
#28552=ORIENTED_EDGE('',*,*,#21559,.T.);
#28553=ORIENTED_EDGE('',*,*,#21560,.T.);
#28554=ORIENTED_EDGE('',*,*,#21561,.T.);
#28555=ORIENTED_EDGE('',*,*,#21562,.T.);
#28556=ORIENTED_EDGE('',*,*,#21563,.T.);
#28557=ORIENTED_EDGE('',*,*,#21564,.T.);
#28558=ORIENTED_EDGE('',*,*,#21565,.T.);
#28559=ORIENTED_EDGE('',*,*,#21566,.T.);
#28560=ORIENTED_EDGE('',*,*,#21567,.T.);
#28561=ORIENTED_EDGE('',*,*,#21568,.T.);
#28562=ORIENTED_EDGE('',*,*,#21569,.T.);
#28563=ORIENTED_EDGE('',*,*,#21570,.T.);
#28564=ORIENTED_EDGE('',*,*,#21571,.T.);
#28565=ORIENTED_EDGE('',*,*,#21572,.T.);
#28566=ORIENTED_EDGE('',*,*,#21573,.T.);
#28567=ORIENTED_EDGE('',*,*,#21574,.T.);
#28568=ORIENTED_EDGE('',*,*,#21575,.T.);
#28569=ORIENTED_EDGE('',*,*,#21576,.T.);
#28570=ORIENTED_EDGE('',*,*,#21577,.T.);
#28571=ORIENTED_EDGE('',*,*,#21578,.T.);
#28572=ORIENTED_EDGE('',*,*,#21579,.T.);
#28573=ORIENTED_EDGE('',*,*,#21580,.T.);
#28574=ORIENTED_EDGE('',*,*,#21581,.T.);
#28575=ORIENTED_EDGE('',*,*,#21582,.T.);
#28576=ORIENTED_EDGE('',*,*,#21583,.T.);
#28577=ORIENTED_EDGE('',*,*,#21584,.T.);
#28578=ORIENTED_EDGE('',*,*,#21585,.T.);
#28579=ORIENTED_EDGE('',*,*,#21586,.T.);
#28580=ORIENTED_EDGE('',*,*,#21587,.T.);
#28581=ORIENTED_EDGE('',*,*,#21588,.T.);
#28582=ORIENTED_EDGE('',*,*,#21589,.T.);
#28583=ORIENTED_EDGE('',*,*,#21590,.T.);
#28584=ORIENTED_EDGE('',*,*,#21591,.T.);
#28585=ORIENTED_EDGE('',*,*,#21592,.T.);
#28586=ORIENTED_EDGE('',*,*,#21593,.T.);
#28587=ORIENTED_EDGE('',*,*,#21594,.T.);
#28588=ORIENTED_EDGE('',*,*,#21595,.T.);
#28589=ORIENTED_EDGE('',*,*,#21596,.T.);
#28590=ORIENTED_EDGE('',*,*,#21597,.T.);
#28591=ORIENTED_EDGE('',*,*,#21598,.T.);
#28592=ORIENTED_EDGE('',*,*,#21599,.T.);
#28593=ORIENTED_EDGE('',*,*,#21600,.T.);
#28594=ORIENTED_EDGE('',*,*,#21601,.T.);
#28595=ORIENTED_EDGE('',*,*,#21602,.T.);
#28596=ORIENTED_EDGE('',*,*,#21603,.T.);
#28597=ORIENTED_EDGE('',*,*,#21604,.T.);
#28598=ORIENTED_EDGE('',*,*,#21605,.T.);
#28599=ORIENTED_EDGE('',*,*,#21606,.T.);
#28600=ORIENTED_EDGE('',*,*,#21607,.T.);
#28601=ORIENTED_EDGE('',*,*,#21608,.T.);
#28602=ORIENTED_EDGE('',*,*,#21609,.T.);
#28603=ORIENTED_EDGE('',*,*,#21610,.T.);
#28604=ORIENTED_EDGE('',*,*,#21611,.T.);
#28605=ORIENTED_EDGE('',*,*,#21612,.T.);
#28606=ORIENTED_EDGE('',*,*,#21613,.T.);
#28607=ORIENTED_EDGE('',*,*,#21614,.T.);
#28608=ORIENTED_EDGE('',*,*,#21615,.T.);
#28609=ORIENTED_EDGE('',*,*,#21616,.T.);
#28610=ORIENTED_EDGE('',*,*,#21617,.T.);
#28611=ORIENTED_EDGE('',*,*,#21618,.T.);
#28612=ORIENTED_EDGE('',*,*,#21619,.T.);
#28613=ORIENTED_EDGE('',*,*,#21620,.T.);
#28614=ORIENTED_EDGE('',*,*,#21621,.T.);
#28615=ORIENTED_EDGE('',*,*,#21622,.T.);
#28616=ORIENTED_EDGE('',*,*,#21623,.T.);
#28617=ORIENTED_EDGE('',*,*,#21624,.T.);
#28618=ORIENTED_EDGE('',*,*,#21625,.T.);
#28619=ORIENTED_EDGE('',*,*,#21626,.T.);
#28620=ORIENTED_EDGE('',*,*,#21627,.T.);
#28621=ORIENTED_EDGE('',*,*,#21628,.T.);
#28622=ORIENTED_EDGE('',*,*,#21629,.T.);
#28623=ORIENTED_EDGE('',*,*,#21630,.T.);
#28624=ORIENTED_EDGE('',*,*,#21631,.T.);
#28625=ORIENTED_EDGE('',*,*,#21632,.T.);
#28626=ORIENTED_EDGE('',*,*,#21633,.T.);
#28627=ORIENTED_EDGE('',*,*,#21634,.T.);
#28628=ORIENTED_EDGE('',*,*,#21635,.T.);
#28629=ORIENTED_EDGE('',*,*,#21636,.T.);
#28630=ORIENTED_EDGE('',*,*,#21637,.T.);
#28631=ORIENTED_EDGE('',*,*,#21638,.T.);
#28632=ORIENTED_EDGE('',*,*,#21639,.T.);
#28633=ORIENTED_EDGE('',*,*,#21640,.T.);
#28634=ORIENTED_EDGE('',*,*,#21641,.T.);
#28635=ORIENTED_EDGE('',*,*,#21642,.T.);
#28636=ORIENTED_EDGE('',*,*,#21643,.T.);
#28637=ORIENTED_EDGE('',*,*,#21644,.T.);
#28638=ORIENTED_EDGE('',*,*,#21645,.T.);
#28639=ORIENTED_EDGE('',*,*,#21646,.T.);
#28640=ORIENTED_EDGE('',*,*,#21647,.T.);
#28641=ORIENTED_EDGE('',*,*,#21648,.T.);
#28642=ORIENTED_EDGE('',*,*,#21649,.T.);
#28643=ORIENTED_EDGE('',*,*,#21650,.T.);
#28644=ORIENTED_EDGE('',*,*,#21651,.T.);
#28645=ORIENTED_EDGE('',*,*,#21652,.T.);
#28646=ORIENTED_EDGE('',*,*,#21653,.T.);
#28647=ORIENTED_EDGE('',*,*,#21654,.T.);
#28648=ORIENTED_EDGE('',*,*,#21655,.T.);
#28649=ORIENTED_EDGE('',*,*,#21656,.T.);
#28650=ORIENTED_EDGE('',*,*,#21657,.T.);
#28651=ORIENTED_EDGE('',*,*,#21658,.T.);
#28652=ORIENTED_EDGE('',*,*,#21659,.T.);
#28653=ORIENTED_EDGE('',*,*,#21660,.T.);
#28654=ORIENTED_EDGE('',*,*,#21661,.T.);
#28655=ORIENTED_EDGE('',*,*,#21662,.T.);
#28656=ORIENTED_EDGE('',*,*,#21663,.T.);
#28657=ORIENTED_EDGE('',*,*,#21664,.T.);
#28658=ORIENTED_EDGE('',*,*,#21665,.T.);
#28659=ORIENTED_EDGE('',*,*,#21666,.T.);
#28660=ORIENTED_EDGE('',*,*,#21667,.T.);
#28661=ORIENTED_EDGE('',*,*,#21668,.T.);
#28662=ORIENTED_EDGE('',*,*,#21669,.T.);
#28663=ORIENTED_EDGE('',*,*,#21670,.T.);
#28664=ORIENTED_EDGE('',*,*,#21671,.T.);
#28665=ORIENTED_EDGE('',*,*,#21672,.T.);
#28666=ORIENTED_EDGE('',*,*,#21673,.T.);
#28667=ORIENTED_EDGE('',*,*,#21674,.T.);
#28668=ORIENTED_EDGE('',*,*,#21675,.T.);
#28669=ORIENTED_EDGE('',*,*,#21676,.T.);
#28670=ORIENTED_EDGE('',*,*,#21677,.T.);
#28671=ORIENTED_EDGE('',*,*,#21678,.T.);
#28672=ORIENTED_EDGE('',*,*,#21679,.T.);
#28673=ORIENTED_EDGE('',*,*,#21680,.T.);
#28674=ORIENTED_EDGE('',*,*,#21681,.T.);
#28675=ORIENTED_EDGE('',*,*,#21682,.T.);
#28676=ORIENTED_EDGE('',*,*,#21683,.T.);
#28677=ORIENTED_EDGE('',*,*,#21684,.T.);
#28678=ORIENTED_EDGE('',*,*,#21685,.T.);
#28679=ORIENTED_EDGE('',*,*,#21686,.T.);
#28680=ORIENTED_EDGE('',*,*,#21687,.T.);
#28681=ORIENTED_EDGE('',*,*,#21688,.T.);
#28682=ORIENTED_EDGE('',*,*,#21689,.T.);
#28683=ORIENTED_EDGE('',*,*,#21690,.T.);
#28684=ORIENTED_EDGE('',*,*,#21691,.T.);
#28685=ORIENTED_EDGE('',*,*,#21692,.T.);
#28686=ORIENTED_EDGE('',*,*,#21693,.T.);
#28687=ORIENTED_EDGE('',*,*,#21694,.T.);
#28688=ORIENTED_EDGE('',*,*,#21695,.T.);
#28689=ORIENTED_EDGE('',*,*,#21696,.T.);
#28690=ORIENTED_EDGE('',*,*,#21697,.T.);
#28691=ORIENTED_EDGE('',*,*,#21698,.T.);
#28692=ORIENTED_EDGE('',*,*,#21699,.T.);
#28693=ORIENTED_EDGE('',*,*,#21700,.T.);
#28694=ORIENTED_EDGE('',*,*,#21701,.T.);
#28695=ORIENTED_EDGE('',*,*,#21702,.T.);
#28696=ORIENTED_EDGE('',*,*,#21703,.T.);
#28697=ORIENTED_EDGE('',*,*,#21704,.T.);
#28698=ORIENTED_EDGE('',*,*,#21705,.T.);
#28699=ORIENTED_EDGE('',*,*,#21706,.T.);
#28700=ORIENTED_EDGE('',*,*,#21707,.T.);
#28701=ORIENTED_EDGE('',*,*,#21708,.T.);
#28702=ORIENTED_EDGE('',*,*,#21709,.T.);
#28703=ORIENTED_EDGE('',*,*,#21710,.T.);
#28704=ORIENTED_EDGE('',*,*,#21711,.T.);
#28705=ORIENTED_EDGE('',*,*,#21712,.T.);
#28706=ORIENTED_EDGE('',*,*,#21713,.T.);
#28707=ORIENTED_EDGE('',*,*,#21714,.T.);
#28708=ORIENTED_EDGE('',*,*,#21715,.T.);
#28709=ORIENTED_EDGE('',*,*,#21716,.T.);
#28710=ORIENTED_EDGE('',*,*,#21717,.T.);
#28711=ORIENTED_EDGE('',*,*,#21718,.T.);
#28712=ORIENTED_EDGE('',*,*,#21719,.T.);
#28713=ORIENTED_EDGE('',*,*,#21720,.T.);
#28714=ORIENTED_EDGE('',*,*,#21721,.T.);
#28715=ORIENTED_EDGE('',*,*,#21722,.T.);
#28716=ORIENTED_EDGE('',*,*,#21723,.T.);
#28717=ORIENTED_EDGE('',*,*,#21724,.T.);
#28718=ORIENTED_EDGE('',*,*,#21725,.T.);
#28719=ORIENTED_EDGE('',*,*,#21726,.T.);
#28720=ORIENTED_EDGE('',*,*,#21727,.T.);
#28721=ORIENTED_EDGE('',*,*,#21728,.T.);
#28722=ORIENTED_EDGE('',*,*,#21729,.T.);
#28723=ORIENTED_EDGE('',*,*,#21730,.T.);
#28724=ORIENTED_EDGE('',*,*,#21731,.T.);
#28725=ORIENTED_EDGE('',*,*,#21732,.T.);
#28726=ORIENTED_EDGE('',*,*,#21733,.T.);
#28727=ORIENTED_EDGE('',*,*,#21734,.T.);
#28728=ORIENTED_EDGE('',*,*,#21735,.T.);
#28729=ORIENTED_EDGE('',*,*,#21736,.T.);
#28730=ORIENTED_EDGE('',*,*,#21737,.T.);
#28731=ORIENTED_EDGE('',*,*,#21738,.T.);
#28732=ORIENTED_EDGE('',*,*,#21739,.T.);
#28733=ORIENTED_EDGE('',*,*,#21740,.T.);
#28734=ORIENTED_EDGE('',*,*,#21741,.T.);
#28735=ORIENTED_EDGE('',*,*,#21742,.T.);
#28736=ORIENTED_EDGE('',*,*,#21743,.T.);
#28737=ORIENTED_EDGE('',*,*,#21744,.T.);
#28738=ORIENTED_EDGE('',*,*,#21745,.T.);
#28739=ORIENTED_EDGE('',*,*,#21746,.T.);
#28740=ORIENTED_EDGE('',*,*,#21747,.T.);
#28741=ORIENTED_EDGE('',*,*,#21748,.T.);
#28742=ORIENTED_EDGE('',*,*,#21749,.T.);
#28743=ORIENTED_EDGE('',*,*,#21750,.T.);
#28744=ORIENTED_EDGE('',*,*,#21751,.T.);
#28745=ORIENTED_EDGE('',*,*,#21752,.T.);
#28746=ORIENTED_EDGE('',*,*,#21753,.T.);
#28747=ORIENTED_EDGE('',*,*,#21754,.T.);
#28748=ORIENTED_EDGE('',*,*,#21755,.T.);
#28749=ORIENTED_EDGE('',*,*,#21756,.T.);
#28750=ORIENTED_EDGE('',*,*,#21757,.T.);
#28751=ORIENTED_EDGE('',*,*,#21758,.T.);
#28752=ORIENTED_EDGE('',*,*,#21759,.T.);
#28753=ORIENTED_EDGE('',*,*,#21760,.T.);
#28754=ORIENTED_EDGE('',*,*,#21761,.T.);
#28755=ORIENTED_EDGE('',*,*,#21762,.T.);
#28756=ORIENTED_EDGE('',*,*,#21763,.T.);
#28757=ORIENTED_EDGE('',*,*,#21764,.T.);
#28758=ORIENTED_EDGE('',*,*,#21765,.T.);
#28759=ORIENTED_EDGE('',*,*,#21766,.T.);
#28760=ORIENTED_EDGE('',*,*,#21767,.T.);
#28761=ORIENTED_EDGE('',*,*,#21768,.T.);
#28762=ORIENTED_EDGE('',*,*,#21769,.T.);
#28763=ORIENTED_EDGE('',*,*,#21770,.T.);
#28764=ORIENTED_EDGE('',*,*,#21771,.T.);
#28765=ORIENTED_EDGE('',*,*,#21772,.T.);
#28766=ORIENTED_EDGE('',*,*,#21773,.T.);
#28767=ORIENTED_EDGE('',*,*,#21774,.T.);
#28768=ORIENTED_EDGE('',*,*,#21775,.T.);
#28769=ORIENTED_EDGE('',*,*,#21776,.T.);
#28770=ORIENTED_EDGE('',*,*,#21777,.T.);
#28771=ORIENTED_EDGE('',*,*,#21778,.T.);
#28772=ORIENTED_EDGE('',*,*,#21779,.T.);
#28773=ORIENTED_EDGE('',*,*,#21780,.T.);
#28774=ORIENTED_EDGE('',*,*,#21781,.T.);
#28775=ORIENTED_EDGE('',*,*,#21782,.T.);
#28776=ORIENTED_EDGE('',*,*,#21783,.T.);
#28777=ORIENTED_EDGE('',*,*,#21784,.T.);
#28778=ORIENTED_EDGE('',*,*,#21471,.F.);
#28779=ORIENTED_EDGE('',*,*,#21785,.F.);
#28780=ORIENTED_EDGE('',*,*,#21786,.T.);
#28781=ORIENTED_EDGE('',*,*,#21787,.T.);
#28782=ORIENTED_EDGE('',*,*,#21788,.F.);
#28783=ORIENTED_EDGE('',*,*,#21789,.T.);
#28784=ORIENTED_EDGE('',*,*,#21783,.F.);
#28785=ORIENTED_EDGE('',*,*,#21790,.T.);
#28786=ORIENTED_EDGE('',*,*,#21791,.T.);
#28787=ORIENTED_EDGE('',*,*,#21792,.T.);
#28788=ORIENTED_EDGE('',*,*,#21793,.T.);
#28789=ORIENTED_EDGE('',*,*,#21794,.F.);
#28790=ORIENTED_EDGE('',*,*,#21795,.T.);
#28791=ORIENTED_EDGE('',*,*,#21796,.T.);
#28792=ORIENTED_EDGE('',*,*,#21797,.F.);
#28793=ORIENTED_EDGE('',*,*,#21798,.T.);
#28794=ORIENTED_EDGE('',*,*,#21799,.T.);
#28795=ORIENTED_EDGE('',*,*,#21800,.T.);
#28796=ORIENTED_EDGE('',*,*,#21801,.T.);
#28797=ORIENTED_EDGE('',*,*,#21475,.F.);
#28798=ORIENTED_EDGE('',*,*,#21802,.F.);
#28799=ORIENTED_EDGE('',*,*,#21803,.T.);
#28800=ORIENTED_EDGE('',*,*,#21791,.F.);
#28801=ORIENTED_EDGE('',*,*,#21804,.T.);
#28802=ORIENTED_EDGE('',*,*,#21800,.F.);
#28803=ORIENTED_EDGE('',*,*,#21805,.T.);
#28804=ORIENTED_EDGE('',*,*,#21806,.F.);
#28805=ORIENTED_EDGE('',*,*,#21807,.T.);
#28806=ORIENTED_EDGE('',*,*,#21808,.T.);
#28807=ORIENTED_EDGE('',*,*,#21809,.T.);
#28808=ORIENTED_EDGE('',*,*,#21788,.T.);
#28809=ORIENTED_EDGE('',*,*,#21810,.T.);
#28810=ORIENTED_EDGE('',*,*,#21794,.T.);
#28811=ORIENTED_EDGE('',*,*,#21811,.T.);
#28812=ORIENTED_EDGE('',*,*,#21808,.F.);
#28813=ORIENTED_EDGE('',*,*,#21812,.T.);
#28814=ORIENTED_EDGE('',*,*,#21474,.F.);
#28815=ORIENTED_EDGE('',*,*,#21813,.T.);
#28816=ORIENTED_EDGE('',*,*,#21797,.T.);
#28817=ORIENTED_EDGE('',*,*,#21814,.T.);
#28818=ORIENTED_EDGE('',*,*,#21815,.T.);
#28819=ORIENTED_EDGE('',*,*,#21802,.T.);
#28820=ORIENTED_EDGE('',*,*,#21816,.T.);
#28821=ORIENTED_EDGE('',*,*,#21806,.T.);
#28822=ORIENTED_EDGE('',*,*,#21817,.T.);
#28823=ORIENTED_EDGE('',*,*,#21818,.T.);
#28824=ORIENTED_EDGE('',*,*,#21819,.T.);
#28825=ORIENTED_EDGE('',*,*,#21820,.T.);
#28826=ORIENTED_EDGE('',*,*,#21821,.T.);
#28827=ORIENTED_EDGE('',*,*,#21822,.T.);
#28828=ORIENTED_EDGE('',*,*,#21823,.F.);
#28829=ORIENTED_EDGE('',*,*,#21824,.T.);
#28830=ORIENTED_EDGE('',*,*,#21825,.T.);
#28831=ORIENTED_EDGE('',*,*,#21826,.F.);
#28832=ORIENTED_EDGE('',*,*,#21827,.T.);
#28833=ORIENTED_EDGE('',*,*,#21828,.T.);
#28834=ORIENTED_EDGE('',*,*,#21829,.T.);
#28835=ORIENTED_EDGE('',*,*,#21830,.T.);
#28836=ORIENTED_EDGE('',*,*,#21831,.T.);
#28837=ORIENTED_EDGE('',*,*,#21823,.T.);
#28838=ORIENTED_EDGE('',*,*,#21832,.T.);
#28839=ORIENTED_EDGE('',*,*,#21814,.F.);
#28840=ORIENTED_EDGE('',*,*,#21833,.T.);
#28841=ORIENTED_EDGE('',*,*,#21818,.F.);
#28842=ORIENTED_EDGE('',*,*,#21834,.T.);
#28843=ORIENTED_EDGE('',*,*,#21826,.T.);
#28844=ORIENTED_EDGE('',*,*,#21835,.T.);
#28845=ORIENTED_EDGE('',*,*,#21836,.F.);
#28846=ORIENTED_EDGE('',*,*,#21837,.T.);
#28847=ORIENTED_EDGE('',*,*,#21820,.F.);
#28848=ORIENTED_EDGE('',*,*,#21838,.T.);
#28849=ORIENTED_EDGE('',*,*,#21829,.F.);
#28850=ORIENTED_EDGE('',*,*,#21839,.T.);
#28851=ORIENTED_EDGE('',*,*,#21840,.F.);
#28852=ORIENTED_EDGE('',*,*,#21841,.T.);
#28853=ORIENTED_EDGE('',*,*,#21842,.T.);
#28854=ORIENTED_EDGE('',*,*,#21843,.T.);
#28855=ORIENTED_EDGE('',*,*,#21836,.T.);
#28856=ORIENTED_EDGE('',*,*,#21844,.T.);
#28857=ORIENTED_EDGE('',*,*,#21840,.T.);
#28858=ORIENTED_EDGE('',*,*,#21845,.T.);
#28859=ORIENTED_EDGE('',*,*,#21846,.T.);
#28860=ORIENTED_EDGE('',*,*,#21847,.T.);
#28861=ORIENTED_EDGE('',*,*,#21848,.T.);
#28862=ORIENTED_EDGE('',*,*,#21849,.T.);
#28863=ORIENTED_EDGE('',*,*,#21850,.T.);
#28864=ORIENTED_EDGE('',*,*,#21851,.F.);
#28865=ORIENTED_EDGE('',*,*,#21852,.T.);
#28866=ORIENTED_EDGE('',*,*,#21853,.T.);
#28867=ORIENTED_EDGE('',*,*,#21854,.F.);
#28868=ORIENTED_EDGE('',*,*,#21855,.T.);
#28869=ORIENTED_EDGE('',*,*,#21856,.T.);
#28870=ORIENTED_EDGE('',*,*,#21857,.T.);
#28871=ORIENTED_EDGE('',*,*,#21858,.T.);
#28872=ORIENTED_EDGE('',*,*,#21859,.T.);
#28873=ORIENTED_EDGE('',*,*,#21851,.T.);
#28874=ORIENTED_EDGE('',*,*,#21860,.T.);
#28875=ORIENTED_EDGE('',*,*,#21842,.F.);
#28876=ORIENTED_EDGE('',*,*,#21861,.T.);
#28877=ORIENTED_EDGE('',*,*,#21846,.F.);
#28878=ORIENTED_EDGE('',*,*,#21862,.T.);
#28879=ORIENTED_EDGE('',*,*,#21854,.T.);
#28880=ORIENTED_EDGE('',*,*,#21863,.T.);
#28881=ORIENTED_EDGE('',*,*,#21864,.F.);
#28882=ORIENTED_EDGE('',*,*,#21865,.T.);
#28883=ORIENTED_EDGE('',*,*,#21848,.F.);
#28884=ORIENTED_EDGE('',*,*,#21866,.T.);
#28885=ORIENTED_EDGE('',*,*,#21857,.F.);
#28886=ORIENTED_EDGE('',*,*,#21867,.T.);
#28887=ORIENTED_EDGE('',*,*,#21868,.F.);
#28888=ORIENTED_EDGE('',*,*,#21869,.T.);
#28889=ORIENTED_EDGE('',*,*,#21870,.T.);
#28890=ORIENTED_EDGE('',*,*,#21871,.T.);
#28891=ORIENTED_EDGE('',*,*,#21864,.T.);
#28892=ORIENTED_EDGE('',*,*,#21872,.T.);
#28893=ORIENTED_EDGE('',*,*,#21868,.T.);
#28894=ORIENTED_EDGE('',*,*,#21873,.T.);
#28895=ORIENTED_EDGE('',*,*,#21874,.T.);
#28896=ORIENTED_EDGE('',*,*,#21875,.T.);
#28897=ORIENTED_EDGE('',*,*,#21876,.T.);
#28898=ORIENTED_EDGE('',*,*,#21877,.T.);
#28899=ORIENTED_EDGE('',*,*,#21878,.T.);
#28900=ORIENTED_EDGE('',*,*,#21879,.F.);
#28901=ORIENTED_EDGE('',*,*,#21880,.T.);
#28902=ORIENTED_EDGE('',*,*,#21881,.T.);
#28903=ORIENTED_EDGE('',*,*,#21882,.F.);
#28904=ORIENTED_EDGE('',*,*,#21883,.T.);
#28905=ORIENTED_EDGE('',*,*,#21884,.T.);
#28906=ORIENTED_EDGE('',*,*,#21885,.T.);
#28907=ORIENTED_EDGE('',*,*,#21886,.T.);
#28908=ORIENTED_EDGE('',*,*,#21887,.T.);
#28909=ORIENTED_EDGE('',*,*,#21879,.T.);
#28910=ORIENTED_EDGE('',*,*,#21888,.T.);
#28911=ORIENTED_EDGE('',*,*,#21870,.F.);
#28912=ORIENTED_EDGE('',*,*,#21889,.T.);
#28913=ORIENTED_EDGE('',*,*,#21874,.F.);
#28914=ORIENTED_EDGE('',*,*,#21890,.T.);
#28915=ORIENTED_EDGE('',*,*,#21882,.T.);
#28916=ORIENTED_EDGE('',*,*,#21891,.T.);
#28917=ORIENTED_EDGE('',*,*,#21892,.F.);
#28918=ORIENTED_EDGE('',*,*,#21893,.T.);
#28919=ORIENTED_EDGE('',*,*,#21876,.F.);
#28920=ORIENTED_EDGE('',*,*,#21894,.T.);
#28921=ORIENTED_EDGE('',*,*,#21885,.F.);
#28922=ORIENTED_EDGE('',*,*,#21895,.T.);
#28923=ORIENTED_EDGE('',*,*,#21896,.F.);
#28924=ORIENTED_EDGE('',*,*,#21897,.T.);
#28925=ORIENTED_EDGE('',*,*,#21898,.T.);
#28926=ORIENTED_EDGE('',*,*,#21899,.T.);
#28927=ORIENTED_EDGE('',*,*,#21892,.T.);
#28928=ORIENTED_EDGE('',*,*,#21900,.T.);
#28929=ORIENTED_EDGE('',*,*,#21896,.T.);
#28930=ORIENTED_EDGE('',*,*,#21901,.T.);
#28931=ORIENTED_EDGE('',*,*,#21902,.T.);
#28932=ORIENTED_EDGE('',*,*,#21903,.T.);
#28933=ORIENTED_EDGE('',*,*,#21904,.T.);
#28934=ORIENTED_EDGE('',*,*,#21905,.T.);
#28935=ORIENTED_EDGE('',*,*,#21906,.T.);
#28936=ORIENTED_EDGE('',*,*,#21907,.F.);
#28937=ORIENTED_EDGE('',*,*,#21908,.T.);
#28938=ORIENTED_EDGE('',*,*,#21909,.T.);
#28939=ORIENTED_EDGE('',*,*,#21910,.F.);
#28940=ORIENTED_EDGE('',*,*,#21911,.T.);
#28941=ORIENTED_EDGE('',*,*,#21912,.T.);
#28942=ORIENTED_EDGE('',*,*,#21913,.T.);
#28943=ORIENTED_EDGE('',*,*,#21914,.T.);
#28944=ORIENTED_EDGE('',*,*,#21915,.T.);
#28945=ORIENTED_EDGE('',*,*,#21907,.T.);
#28946=ORIENTED_EDGE('',*,*,#21916,.T.);
#28947=ORIENTED_EDGE('',*,*,#21898,.F.);
#28948=ORIENTED_EDGE('',*,*,#21917,.T.);
#28949=ORIENTED_EDGE('',*,*,#21902,.F.);
#28950=ORIENTED_EDGE('',*,*,#21918,.T.);
#28951=ORIENTED_EDGE('',*,*,#21910,.T.);
#28952=ORIENTED_EDGE('',*,*,#21919,.T.);
#28953=ORIENTED_EDGE('',*,*,#21920,.F.);
#28954=ORIENTED_EDGE('',*,*,#21921,.T.);
#28955=ORIENTED_EDGE('',*,*,#21904,.F.);
#28956=ORIENTED_EDGE('',*,*,#21922,.T.);
#28957=ORIENTED_EDGE('',*,*,#21913,.F.);
#28958=ORIENTED_EDGE('',*,*,#21923,.T.);
#28959=ORIENTED_EDGE('',*,*,#21924,.F.);
#28960=ORIENTED_EDGE('',*,*,#21925,.T.);
#28961=ORIENTED_EDGE('',*,*,#21926,.T.);
#28962=ORIENTED_EDGE('',*,*,#21927,.T.);
#28963=ORIENTED_EDGE('',*,*,#21920,.T.);
#28964=ORIENTED_EDGE('',*,*,#21928,.T.);
#28965=ORIENTED_EDGE('',*,*,#21924,.T.);
#28966=ORIENTED_EDGE('',*,*,#21929,.T.);
#28967=ORIENTED_EDGE('',*,*,#21930,.T.);
#28968=ORIENTED_EDGE('',*,*,#21931,.T.);
#28969=ORIENTED_EDGE('',*,*,#21932,.T.);
#28970=ORIENTED_EDGE('',*,*,#21933,.T.);
#28971=ORIENTED_EDGE('',*,*,#21934,.T.);
#28972=ORIENTED_EDGE('',*,*,#21935,.F.);
#28973=ORIENTED_EDGE('',*,*,#21936,.T.);
#28974=ORIENTED_EDGE('',*,*,#21937,.T.);
#28975=ORIENTED_EDGE('',*,*,#21938,.F.);
#28976=ORIENTED_EDGE('',*,*,#21939,.T.);
#28977=ORIENTED_EDGE('',*,*,#21940,.T.);
#28978=ORIENTED_EDGE('',*,*,#21941,.T.);
#28979=ORIENTED_EDGE('',*,*,#21942,.T.);
#28980=ORIENTED_EDGE('',*,*,#21943,.T.);
#28981=ORIENTED_EDGE('',*,*,#21935,.T.);
#28982=ORIENTED_EDGE('',*,*,#21944,.T.);
#28983=ORIENTED_EDGE('',*,*,#21926,.F.);
#28984=ORIENTED_EDGE('',*,*,#21945,.T.);
#28985=ORIENTED_EDGE('',*,*,#21930,.F.);
#28986=ORIENTED_EDGE('',*,*,#21946,.T.);
#28987=ORIENTED_EDGE('',*,*,#21938,.T.);
#28988=ORIENTED_EDGE('',*,*,#21947,.T.);
#28989=ORIENTED_EDGE('',*,*,#21628,.F.);
#28990=ORIENTED_EDGE('',*,*,#21948,.T.);
#28991=ORIENTED_EDGE('',*,*,#21932,.F.);
#28992=ORIENTED_EDGE('',*,*,#21949,.T.);
#28993=ORIENTED_EDGE('',*,*,#21941,.F.);
#28994=ORIENTED_EDGE('',*,*,#21950,.T.);
#28995=ORIENTED_EDGE('',*,*,#21951,.F.);
#28996=ORIENTED_EDGE('',*,*,#21952,.T.);
#28997=ORIENTED_EDGE('',*,*,#21951,.T.);
#28998=ORIENTED_EDGE('',*,*,#21953,.T.);
#28999=ORIENTED_EDGE('',*,*,#21954,.T.);
#29000=ORIENTED_EDGE('',*,*,#21955,.T.);
#29001=ORIENTED_EDGE('',*,*,#21625,.F.);
#29002=ORIENTED_EDGE('',*,*,#21956,.T.);
#29003=ORIENTED_EDGE('',*,*,#21957,.T.);
#29004=ORIENTED_EDGE('',*,*,#21958,.F.);
#29005=ORIENTED_EDGE('',*,*,#21959,.F.);
#29006=ORIENTED_EDGE('',*,*,#21960,.T.);
#29007=ORIENTED_EDGE('',*,*,#21961,.T.);
#29008=ORIENTED_EDGE('',*,*,#21962,.T.);
#29009=ORIENTED_EDGE('',*,*,#21963,.T.);
#29010=ORIENTED_EDGE('',*,*,#21964,.T.);
#29011=ORIENTED_EDGE('',*,*,#21958,.T.);
#29012=ORIENTED_EDGE('',*,*,#21965,.T.);
#29013=ORIENTED_EDGE('',*,*,#21626,.F.);
#29014=ORIENTED_EDGE('',*,*,#21954,.F.);
#29015=ORIENTED_EDGE('',*,*,#21966,.T.);
#29016=ORIENTED_EDGE('',*,*,#21959,.T.);
#29017=ORIENTED_EDGE('',*,*,#21967,.T.);
#29018=ORIENTED_EDGE('',*,*,#21962,.F.);
#29019=ORIENTED_EDGE('',*,*,#21968,.T.);
#29020=ORIENTED_EDGE('',*,*,#21622,.F.);
#29021=ORIENTED_EDGE('',*,*,#21969,.T.);
#29022=ORIENTED_EDGE('',*,*,#21970,.T.);
#29023=ORIENTED_EDGE('',*,*,#21971,.T.);
#29024=ORIENTED_EDGE('',*,*,#21467,.F.);
#29025=ORIENTED_EDGE('',*,*,#21972,.F.);
#29026=ORIENTED_EDGE('',*,*,#21973,.T.);
#29027=ORIENTED_EDGE('',*,*,#21974,.T.);
#29028=ORIENTED_EDGE('',*,*,#21975,.F.);
#29029=ORIENTED_EDGE('',*,*,#21976,.T.);
#29030=ORIENTED_EDGE('',*,*,#21970,.F.);
#29031=ORIENTED_EDGE('',*,*,#21977,.T.);
#29032=ORIENTED_EDGE('',*,*,#21978,.T.);
#29033=ORIENTED_EDGE('',*,*,#21979,.T.);
#29034=ORIENTED_EDGE('',*,*,#21975,.T.);
#29035=ORIENTED_EDGE('',*,*,#21980,.T.);
#29036=ORIENTED_EDGE('',*,*,#21981,.T.);
#29037=ORIENTED_EDGE('',*,*,#21982,.T.);
#29038=ORIENTED_EDGE('',*,*,#21983,.T.);
#29039=ORIENTED_EDGE('',*,*,#21984,.F.);
#29040=ORIENTED_EDGE('',*,*,#21985,.T.);
#29041=ORIENTED_EDGE('',*,*,#21986,.T.);
#29042=ORIENTED_EDGE('',*,*,#21984,.T.);
#29043=ORIENTED_EDGE('',*,*,#21987,.T.);
#29044=ORIENTED_EDGE('',*,*,#21978,.F.);
#29045=ORIENTED_EDGE('',*,*,#21988,.T.);
#29046=ORIENTED_EDGE('',*,*,#21470,.F.);
#29047=ORIENTED_EDGE('',*,*,#21989,.T.);
#29048=ORIENTED_EDGE('',*,*,#21785,.T.);
#29049=ORIENTED_EDGE('',*,*,#21990,.F.);
#29050=ORIENTED_EDGE('',*,*,#21991,.T.);
#29051=ORIENTED_EDGE('',*,*,#21981,.F.);
#29052=ORIENTED_EDGE('',*,*,#21992,.T.);
#29053=ORIENTED_EDGE('',*,*,#21993,.T.);
#29054=ORIENTED_EDGE('',*,*,#21994,.T.);
#29055=ORIENTED_EDGE('',*,*,#21995,.T.);
#29056=ORIENTED_EDGE('',*,*,#21996,.F.);
#29057=ORIENTED_EDGE('',*,*,#21997,.T.);
#29058=ORIENTED_EDGE('',*,*,#21998,.T.);
#29059=ORIENTED_EDGE('',*,*,#21999,.F.);
#29060=ORIENTED_EDGE('',*,*,#22000,.T.);
#29061=ORIENTED_EDGE('',*,*,#21993,.F.);
#29062=ORIENTED_EDGE('',*,*,#22001,.T.);
#29063=ORIENTED_EDGE('',*,*,#22002,.T.);
#29064=ORIENTED_EDGE('',*,*,#22003,.T.);
#29065=ORIENTED_EDGE('',*,*,#21990,.T.);
#29066=ORIENTED_EDGE('',*,*,#22004,.T.);
#29067=ORIENTED_EDGE('',*,*,#21996,.T.);
#29068=ORIENTED_EDGE('',*,*,#22005,.T.);
#29069=ORIENTED_EDGE('',*,*,#22002,.F.);
#29070=ORIENTED_EDGE('',*,*,#22006,.T.);
#29071=ORIENTED_EDGE('',*,*,#22007,.T.);
#29072=ORIENTED_EDGE('',*,*,#22008,.T.);
#29073=ORIENTED_EDGE('',*,*,#21999,.T.);
#29074=ORIENTED_EDGE('',*,*,#22009,.T.);
#29075=ORIENTED_EDGE('',*,*,#22010,.T.);
#29076=ORIENTED_EDGE('',*,*,#22011,.T.);
#29077=ORIENTED_EDGE('',*,*,#22012,.T.);
#29078=ORIENTED_EDGE('',*,*,#22013,.F.);
#29079=ORIENTED_EDGE('',*,*,#22014,.T.);
#29080=ORIENTED_EDGE('',*,*,#22015,.T.);
#29081=ORIENTED_EDGE('',*,*,#22013,.T.);
#29082=ORIENTED_EDGE('',*,*,#22016,.T.);
#29083=ORIENTED_EDGE('',*,*,#22007,.F.);
#29084=ORIENTED_EDGE('',*,*,#22017,.T.);
#29085=ORIENTED_EDGE('',*,*,#22018,.F.);
#29086=ORIENTED_EDGE('',*,*,#22019,.T.);
#29087=ORIENTED_EDGE('',*,*,#22010,.F.);
#29088=ORIENTED_EDGE('',*,*,#22020,.T.);
#29089=ORIENTED_EDGE('',*,*,#22021,.T.);
#29090=ORIENTED_EDGE('',*,*,#22022,.T.);
#29091=ORIENTED_EDGE('',*,*,#22018,.T.);
#29092=ORIENTED_EDGE('',*,*,#22023,.T.);
#29093=ORIENTED_EDGE('',*,*,#22024,.T.);
#29094=ORIENTED_EDGE('',*,*,#22025,.T.);
#29095=ORIENTED_EDGE('',*,*,#22026,.T.);
#29096=ORIENTED_EDGE('',*,*,#22027,.F.);
#29097=ORIENTED_EDGE('',*,*,#22028,.T.);
#29098=ORIENTED_EDGE('',*,*,#22029,.T.);
#29099=ORIENTED_EDGE('',*,*,#22027,.T.);
#29100=ORIENTED_EDGE('',*,*,#22030,.T.);
#29101=ORIENTED_EDGE('',*,*,#22021,.F.);
#29102=ORIENTED_EDGE('',*,*,#22031,.T.);
#29103=ORIENTED_EDGE('',*,*,#22032,.F.);
#29104=ORIENTED_EDGE('',*,*,#22033,.T.);
#29105=ORIENTED_EDGE('',*,*,#22024,.F.);
#29106=ORIENTED_EDGE('',*,*,#22034,.T.);
#29107=ORIENTED_EDGE('',*,*,#22035,.T.);
#29108=ORIENTED_EDGE('',*,*,#22036,.T.);
#29109=ORIENTED_EDGE('',*,*,#22032,.T.);
#29110=ORIENTED_EDGE('',*,*,#22037,.T.);
#29111=ORIENTED_EDGE('',*,*,#22038,.T.);
#29112=ORIENTED_EDGE('',*,*,#22039,.T.);
#29113=ORIENTED_EDGE('',*,*,#22040,.T.);
#29114=ORIENTED_EDGE('',*,*,#22041,.F.);
#29115=ORIENTED_EDGE('',*,*,#22042,.T.);
#29116=ORIENTED_EDGE('',*,*,#22043,.T.);
#29117=ORIENTED_EDGE('',*,*,#22041,.T.);
#29118=ORIENTED_EDGE('',*,*,#22044,.T.);
#29119=ORIENTED_EDGE('',*,*,#22035,.F.);
#29120=ORIENTED_EDGE('',*,*,#22045,.T.);
#29121=ORIENTED_EDGE('',*,*,#22046,.F.);
#29122=ORIENTED_EDGE('',*,*,#22047,.T.);
#29123=ORIENTED_EDGE('',*,*,#22038,.F.);
#29124=ORIENTED_EDGE('',*,*,#22048,.T.);
#29125=ORIENTED_EDGE('',*,*,#22049,.T.);
#29126=ORIENTED_EDGE('',*,*,#22050,.T.);
#29127=ORIENTED_EDGE('',*,*,#22046,.T.);
#29128=ORIENTED_EDGE('',*,*,#22051,.T.);
#29129=ORIENTED_EDGE('',*,*,#22052,.T.);
#29130=ORIENTED_EDGE('',*,*,#22053,.T.);
#29131=ORIENTED_EDGE('',*,*,#22054,.T.);
#29132=ORIENTED_EDGE('',*,*,#22055,.F.);
#29133=ORIENTED_EDGE('',*,*,#22056,.T.);
#29134=ORIENTED_EDGE('',*,*,#22057,.T.);
#29135=ORIENTED_EDGE('',*,*,#22055,.T.);
#29136=ORIENTED_EDGE('',*,*,#22058,.T.);
#29137=ORIENTED_EDGE('',*,*,#22049,.F.);
#29138=ORIENTED_EDGE('',*,*,#22059,.T.);
#29139=ORIENTED_EDGE('',*,*,#21634,.F.);
#29140=ORIENTED_EDGE('',*,*,#22060,.T.);
#29141=ORIENTED_EDGE('',*,*,#22052,.F.);
#29142=ORIENTED_EDGE('',*,*,#22061,.T.);
#29143=ORIENTED_EDGE('',*,*,#21631,.F.);
#29144=ORIENTED_EDGE('',*,*,#22062,.T.);
#29145=ORIENTED_EDGE('',*,*,#22063,.T.);
#29146=ORIENTED_EDGE('',*,*,#22064,.F.);
#29147=ORIENTED_EDGE('',*,*,#22064,.T.);
#29148=ORIENTED_EDGE('',*,*,#22065,.T.);
#29149=ORIENTED_EDGE('',*,*,#21632,.F.);
#29150=ORIENTED_EDGE('',*,*,#22066,.T.);
#29151=ORIENTED_EDGE('',*,*,#22067,.T.);
#29152=ORIENTED_EDGE('',*,*,#21463,.F.);
#29153=ORIENTED_EDGE('',*,*,#22068,.F.);
#29154=ORIENTED_EDGE('',*,*,#22069,.T.);
#29155=ORIENTED_EDGE('',*,*,#22070,.T.);
#29156=ORIENTED_EDGE('',*,*,#22071,.F.);
#29157=ORIENTED_EDGE('',*,*,#22072,.T.);
#29158=ORIENTED_EDGE('',*,*,#22066,.F.);
#29159=ORIENTED_EDGE('',*,*,#22073,.T.);
#29160=ORIENTED_EDGE('',*,*,#22074,.T.);
#29161=ORIENTED_EDGE('',*,*,#22075,.T.);
#29162=ORIENTED_EDGE('',*,*,#22071,.T.);
#29163=ORIENTED_EDGE('',*,*,#22076,.T.);
#29164=ORIENTED_EDGE('',*,*,#22077,.T.);
#29165=ORIENTED_EDGE('',*,*,#22078,.T.);
#29166=ORIENTED_EDGE('',*,*,#22079,.T.);
#29167=ORIENTED_EDGE('',*,*,#22080,.F.);
#29168=ORIENTED_EDGE('',*,*,#22081,.T.);
#29169=ORIENTED_EDGE('',*,*,#22082,.T.);
#29170=ORIENTED_EDGE('',*,*,#22080,.T.);
#29171=ORIENTED_EDGE('',*,*,#22083,.T.);
#29172=ORIENTED_EDGE('',*,*,#22074,.F.);
#29173=ORIENTED_EDGE('',*,*,#22084,.T.);
#29174=ORIENTED_EDGE('',*,*,#21466,.F.);
#29175=ORIENTED_EDGE('',*,*,#22085,.T.);
#29176=ORIENTED_EDGE('',*,*,#21972,.T.);
#29177=ORIENTED_EDGE('',*,*,#22086,.F.);
#29178=ORIENTED_EDGE('',*,*,#22087,.T.);
#29179=ORIENTED_EDGE('',*,*,#22077,.F.);
#29180=ORIENTED_EDGE('',*,*,#22088,.T.);
#29181=ORIENTED_EDGE('',*,*,#22089,.T.);
#29182=ORIENTED_EDGE('',*,*,#22090,.T.);
#29183=ORIENTED_EDGE('',*,*,#22086,.T.);
#29184=ORIENTED_EDGE('',*,*,#22091,.T.);
#29185=ORIENTED_EDGE('',*,*,#22092,.T.);
#29186=ORIENTED_EDGE('',*,*,#22093,.T.);
#29187=ORIENTED_EDGE('',*,*,#22094,.T.);
#29188=ORIENTED_EDGE('',*,*,#22095,.F.);
#29189=ORIENTED_EDGE('',*,*,#22096,.T.);
#29190=ORIENTED_EDGE('',*,*,#22097,.T.);
#29191=ORIENTED_EDGE('',*,*,#22095,.T.);
#29192=ORIENTED_EDGE('',*,*,#22098,.T.);
#29193=ORIENTED_EDGE('',*,*,#22089,.F.);
#29194=ORIENTED_EDGE('',*,*,#22099,.T.);
#29195=ORIENTED_EDGE('',*,*,#22100,.F.);
#29196=ORIENTED_EDGE('',*,*,#22101,.T.);
#29197=ORIENTED_EDGE('',*,*,#22092,.F.);
#29198=ORIENTED_EDGE('',*,*,#22102,.T.);
#29199=ORIENTED_EDGE('',*,*,#22103,.T.);
#29200=ORIENTED_EDGE('',*,*,#22104,.T.);
#29201=ORIENTED_EDGE('',*,*,#22105,.T.);
#29202=ORIENTED_EDGE('',*,*,#22106,.F.);
#29203=ORIENTED_EDGE('',*,*,#22107,.T.);
#29204=ORIENTED_EDGE('',*,*,#22108,.T.);
#29205=ORIENTED_EDGE('',*,*,#22109,.F.);
#29206=ORIENTED_EDGE('',*,*,#22110,.T.);
#29207=ORIENTED_EDGE('',*,*,#22103,.F.);
#29208=ORIENTED_EDGE('',*,*,#22111,.T.);
#29209=ORIENTED_EDGE('',*,*,#22112,.T.);
#29210=ORIENTED_EDGE('',*,*,#22113,.T.);
#29211=ORIENTED_EDGE('',*,*,#22100,.T.);
#29212=ORIENTED_EDGE('',*,*,#22114,.T.);
#29213=ORIENTED_EDGE('',*,*,#22106,.T.);
#29214=ORIENTED_EDGE('',*,*,#22115,.T.);
#29215=ORIENTED_EDGE('',*,*,#22112,.F.);
#29216=ORIENTED_EDGE('',*,*,#22116,.T.);
#29217=ORIENTED_EDGE('',*,*,#22117,.T.);
#29218=ORIENTED_EDGE('',*,*,#22118,.T.);
#29219=ORIENTED_EDGE('',*,*,#22109,.T.);
#29220=ORIENTED_EDGE('',*,*,#22119,.T.);
#29221=ORIENTED_EDGE('',*,*,#22120,.T.);
#29222=ORIENTED_EDGE('',*,*,#22121,.T.);
#29223=ORIENTED_EDGE('',*,*,#22122,.T.);
#29224=ORIENTED_EDGE('',*,*,#22123,.F.);
#29225=ORIENTED_EDGE('',*,*,#22124,.T.);
#29226=ORIENTED_EDGE('',*,*,#22125,.T.);
#29227=ORIENTED_EDGE('',*,*,#22123,.T.);
#29228=ORIENTED_EDGE('',*,*,#22126,.T.);
#29229=ORIENTED_EDGE('',*,*,#22117,.F.);
#29230=ORIENTED_EDGE('',*,*,#22127,.T.);
#29231=ORIENTED_EDGE('',*,*,#22128,.F.);
#29232=ORIENTED_EDGE('',*,*,#22129,.T.);
#29233=ORIENTED_EDGE('',*,*,#22120,.F.);
#29234=ORIENTED_EDGE('',*,*,#22130,.T.);
#29235=ORIENTED_EDGE('',*,*,#22131,.T.);
#29236=ORIENTED_EDGE('',*,*,#22132,.T.);
#29237=ORIENTED_EDGE('',*,*,#22128,.T.);
#29238=ORIENTED_EDGE('',*,*,#22133,.T.);
#29239=ORIENTED_EDGE('',*,*,#22134,.T.);
#29240=ORIENTED_EDGE('',*,*,#22135,.T.);
#29241=ORIENTED_EDGE('',*,*,#22136,.T.);
#29242=ORIENTED_EDGE('',*,*,#22137,.F.);
#29243=ORIENTED_EDGE('',*,*,#22138,.T.);
#29244=ORIENTED_EDGE('',*,*,#22139,.T.);
#29245=ORIENTED_EDGE('',*,*,#22137,.T.);
#29246=ORIENTED_EDGE('',*,*,#22140,.T.);
#29247=ORIENTED_EDGE('',*,*,#22131,.F.);
#29248=ORIENTED_EDGE('',*,*,#22141,.T.);
#29249=ORIENTED_EDGE('',*,*,#22142,.F.);
#29250=ORIENTED_EDGE('',*,*,#22143,.T.);
#29251=ORIENTED_EDGE('',*,*,#22134,.F.);
#29252=ORIENTED_EDGE('',*,*,#22144,.T.);
#29253=ORIENTED_EDGE('',*,*,#22145,.T.);
#29254=ORIENTED_EDGE('',*,*,#22146,.T.);
#29255=ORIENTED_EDGE('',*,*,#22142,.T.);
#29256=ORIENTED_EDGE('',*,*,#22147,.T.);
#29257=ORIENTED_EDGE('',*,*,#22148,.T.);
#29258=ORIENTED_EDGE('',*,*,#22149,.T.);
#29259=ORIENTED_EDGE('',*,*,#22150,.T.);
#29260=ORIENTED_EDGE('',*,*,#22151,.F.);
#29261=ORIENTED_EDGE('',*,*,#22152,.T.);
#29262=ORIENTED_EDGE('',*,*,#22153,.T.);
#29263=ORIENTED_EDGE('',*,*,#22151,.T.);
#29264=ORIENTED_EDGE('',*,*,#22154,.T.);
#29265=ORIENTED_EDGE('',*,*,#22145,.F.);
#29266=ORIENTED_EDGE('',*,*,#22155,.T.);
#29267=ORIENTED_EDGE('',*,*,#21640,.F.);
#29268=ORIENTED_EDGE('',*,*,#22156,.T.);
#29269=ORIENTED_EDGE('',*,*,#22148,.F.);
#29270=ORIENTED_EDGE('',*,*,#22157,.T.);
#29271=ORIENTED_EDGE('',*,*,#21637,.F.);
#29272=ORIENTED_EDGE('',*,*,#22158,.T.);
#29273=ORIENTED_EDGE('',*,*,#22159,.T.);
#29274=ORIENTED_EDGE('',*,*,#22160,.F.);
#29275=ORIENTED_EDGE('',*,*,#22160,.T.);
#29276=ORIENTED_EDGE('',*,*,#22161,.T.);
#29277=ORIENTED_EDGE('',*,*,#21638,.F.);
#29278=ORIENTED_EDGE('',*,*,#22162,.T.);
#29279=ORIENTED_EDGE('',*,*,#22163,.T.);
#29280=ORIENTED_EDGE('',*,*,#21459,.F.);
#29281=ORIENTED_EDGE('',*,*,#22164,.F.);
#29282=ORIENTED_EDGE('',*,*,#22165,.T.);
#29283=ORIENTED_EDGE('',*,*,#22166,.T.);
#29284=ORIENTED_EDGE('',*,*,#22167,.F.);
#29285=ORIENTED_EDGE('',*,*,#22168,.T.);
#29286=ORIENTED_EDGE('',*,*,#22162,.F.);
#29287=ORIENTED_EDGE('',*,*,#22169,.T.);
#29288=ORIENTED_EDGE('',*,*,#22170,.T.);
#29289=ORIENTED_EDGE('',*,*,#22171,.T.);
#29290=ORIENTED_EDGE('',*,*,#22167,.T.);
#29291=ORIENTED_EDGE('',*,*,#22172,.T.);
#29292=ORIENTED_EDGE('',*,*,#22173,.T.);
#29293=ORIENTED_EDGE('',*,*,#22174,.T.);
#29294=ORIENTED_EDGE('',*,*,#22175,.T.);
#29295=ORIENTED_EDGE('',*,*,#22176,.F.);
#29296=ORIENTED_EDGE('',*,*,#22177,.T.);
#29297=ORIENTED_EDGE('',*,*,#22178,.T.);
#29298=ORIENTED_EDGE('',*,*,#22176,.T.);
#29299=ORIENTED_EDGE('',*,*,#22179,.T.);
#29300=ORIENTED_EDGE('',*,*,#22170,.F.);
#29301=ORIENTED_EDGE('',*,*,#22180,.T.);
#29302=ORIENTED_EDGE('',*,*,#21462,.F.);
#29303=ORIENTED_EDGE('',*,*,#22181,.T.);
#29304=ORIENTED_EDGE('',*,*,#22068,.T.);
#29305=ORIENTED_EDGE('',*,*,#22182,.F.);
#29306=ORIENTED_EDGE('',*,*,#22183,.T.);
#29307=ORIENTED_EDGE('',*,*,#22173,.F.);
#29308=ORIENTED_EDGE('',*,*,#22184,.T.);
#29309=ORIENTED_EDGE('',*,*,#22185,.T.);
#29310=ORIENTED_EDGE('',*,*,#22186,.T.);
#29311=ORIENTED_EDGE('',*,*,#22182,.T.);
#29312=ORIENTED_EDGE('',*,*,#22187,.T.);
#29313=ORIENTED_EDGE('',*,*,#22188,.T.);
#29314=ORIENTED_EDGE('',*,*,#22189,.T.);
#29315=ORIENTED_EDGE('',*,*,#22190,.T.);
#29316=ORIENTED_EDGE('',*,*,#22191,.F.);
#29317=ORIENTED_EDGE('',*,*,#22192,.T.);
#29318=ORIENTED_EDGE('',*,*,#22193,.T.);
#29319=ORIENTED_EDGE('',*,*,#22191,.T.);
#29320=ORIENTED_EDGE('',*,*,#22194,.T.);
#29321=ORIENTED_EDGE('',*,*,#22185,.F.);
#29322=ORIENTED_EDGE('',*,*,#22195,.T.);
#29323=ORIENTED_EDGE('',*,*,#22196,.F.);
#29324=ORIENTED_EDGE('',*,*,#22197,.T.);
#29325=ORIENTED_EDGE('',*,*,#22188,.F.);
#29326=ORIENTED_EDGE('',*,*,#22198,.T.);
#29327=ORIENTED_EDGE('',*,*,#22199,.T.);
#29328=ORIENTED_EDGE('',*,*,#22200,.T.);
#29329=ORIENTED_EDGE('',*,*,#22196,.T.);
#29330=ORIENTED_EDGE('',*,*,#22201,.T.);
#29331=ORIENTED_EDGE('',*,*,#22202,.T.);
#29332=ORIENTED_EDGE('',*,*,#22203,.T.);
#29333=ORIENTED_EDGE('',*,*,#22204,.T.);
#29334=ORIENTED_EDGE('',*,*,#22205,.F.);
#29335=ORIENTED_EDGE('',*,*,#22206,.T.);
#29336=ORIENTED_EDGE('',*,*,#22207,.T.);
#29337=ORIENTED_EDGE('',*,*,#22205,.T.);
#29338=ORIENTED_EDGE('',*,*,#22208,.T.);
#29339=ORIENTED_EDGE('',*,*,#22199,.F.);
#29340=ORIENTED_EDGE('',*,*,#22209,.T.);
#29341=ORIENTED_EDGE('',*,*,#22210,.F.);
#29342=ORIENTED_EDGE('',*,*,#22211,.T.);
#29343=ORIENTED_EDGE('',*,*,#22202,.F.);
#29344=ORIENTED_EDGE('',*,*,#22212,.T.);
#29345=ORIENTED_EDGE('',*,*,#22213,.T.);
#29346=ORIENTED_EDGE('',*,*,#22214,.T.);
#29347=ORIENTED_EDGE('',*,*,#22215,.T.);
#29348=ORIENTED_EDGE('',*,*,#22216,.F.);
#29349=ORIENTED_EDGE('',*,*,#22217,.T.);
#29350=ORIENTED_EDGE('',*,*,#22218,.T.);
#29351=ORIENTED_EDGE('',*,*,#22219,.F.);
#29352=ORIENTED_EDGE('',*,*,#22220,.T.);
#29353=ORIENTED_EDGE('',*,*,#22213,.F.);
#29354=ORIENTED_EDGE('',*,*,#22221,.T.);
#29355=ORIENTED_EDGE('',*,*,#22222,.T.);
#29356=ORIENTED_EDGE('',*,*,#22223,.T.);
#29357=ORIENTED_EDGE('',*,*,#22210,.T.);
#29358=ORIENTED_EDGE('',*,*,#22224,.T.);
#29359=ORIENTED_EDGE('',*,*,#22216,.T.);
#29360=ORIENTED_EDGE('',*,*,#22225,.T.);
#29361=ORIENTED_EDGE('',*,*,#22222,.F.);
#29362=ORIENTED_EDGE('',*,*,#22226,.T.);
#29363=ORIENTED_EDGE('',*,*,#22227,.T.);
#29364=ORIENTED_EDGE('',*,*,#22228,.T.);
#29365=ORIENTED_EDGE('',*,*,#22219,.T.);
#29366=ORIENTED_EDGE('',*,*,#22229,.T.);
#29367=ORIENTED_EDGE('',*,*,#22230,.T.);
#29368=ORIENTED_EDGE('',*,*,#22231,.T.);
#29369=ORIENTED_EDGE('',*,*,#22232,.T.);
#29370=ORIENTED_EDGE('',*,*,#22233,.F.);
#29371=ORIENTED_EDGE('',*,*,#22234,.T.);
#29372=ORIENTED_EDGE('',*,*,#22235,.T.);
#29373=ORIENTED_EDGE('',*,*,#22233,.T.);
#29374=ORIENTED_EDGE('',*,*,#22236,.T.);
#29375=ORIENTED_EDGE('',*,*,#22227,.F.);
#29376=ORIENTED_EDGE('',*,*,#22237,.T.);
#29377=ORIENTED_EDGE('',*,*,#22238,.F.);
#29378=ORIENTED_EDGE('',*,*,#22239,.T.);
#29379=ORIENTED_EDGE('',*,*,#22230,.F.);
#29380=ORIENTED_EDGE('',*,*,#22240,.T.);
#29381=ORIENTED_EDGE('',*,*,#22241,.T.);
#29382=ORIENTED_EDGE('',*,*,#22242,.T.);
#29383=ORIENTED_EDGE('',*,*,#22238,.T.);
#29384=ORIENTED_EDGE('',*,*,#22243,.T.);
#29385=ORIENTED_EDGE('',*,*,#22244,.T.);
#29386=ORIENTED_EDGE('',*,*,#22245,.T.);
#29387=ORIENTED_EDGE('',*,*,#22246,.T.);
#29388=ORIENTED_EDGE('',*,*,#22247,.F.);
#29389=ORIENTED_EDGE('',*,*,#22248,.T.);
#29390=ORIENTED_EDGE('',*,*,#22249,.T.);
#29391=ORIENTED_EDGE('',*,*,#22247,.T.);
#29392=ORIENTED_EDGE('',*,*,#22250,.T.);
#29393=ORIENTED_EDGE('',*,*,#22241,.F.);
#29394=ORIENTED_EDGE('',*,*,#22251,.T.);
#29395=ORIENTED_EDGE('',*,*,#21646,.F.);
#29396=ORIENTED_EDGE('',*,*,#22252,.T.);
#29397=ORIENTED_EDGE('',*,*,#22244,.F.);
#29398=ORIENTED_EDGE('',*,*,#22253,.T.);
#29399=ORIENTED_EDGE('',*,*,#21643,.F.);
#29400=ORIENTED_EDGE('',*,*,#22254,.T.);
#29401=ORIENTED_EDGE('',*,*,#22255,.T.);
#29402=ORIENTED_EDGE('',*,*,#22256,.F.);
#29403=ORIENTED_EDGE('',*,*,#22256,.T.);
#29404=ORIENTED_EDGE('',*,*,#22257,.T.);
#29405=ORIENTED_EDGE('',*,*,#21644,.F.);
#29406=ORIENTED_EDGE('',*,*,#22258,.T.);
#29407=ORIENTED_EDGE('',*,*,#22259,.T.);
#29408=ORIENTED_EDGE('',*,*,#21455,.F.);
#29409=ORIENTED_EDGE('',*,*,#22260,.F.);
#29410=ORIENTED_EDGE('',*,*,#22261,.T.);
#29411=ORIENTED_EDGE('',*,*,#22262,.T.);
#29412=ORIENTED_EDGE('',*,*,#22263,.F.);
#29413=ORIENTED_EDGE('',*,*,#22264,.T.);
#29414=ORIENTED_EDGE('',*,*,#22258,.F.);
#29415=ORIENTED_EDGE('',*,*,#22265,.T.);
#29416=ORIENTED_EDGE('',*,*,#22266,.T.);
#29417=ORIENTED_EDGE('',*,*,#22267,.T.);
#29418=ORIENTED_EDGE('',*,*,#22263,.T.);
#29419=ORIENTED_EDGE('',*,*,#22268,.T.);
#29420=ORIENTED_EDGE('',*,*,#22269,.T.);
#29421=ORIENTED_EDGE('',*,*,#22270,.T.);
#29422=ORIENTED_EDGE('',*,*,#22271,.T.);
#29423=ORIENTED_EDGE('',*,*,#22272,.F.);
#29424=ORIENTED_EDGE('',*,*,#22273,.T.);
#29425=ORIENTED_EDGE('',*,*,#22274,.T.);
#29426=ORIENTED_EDGE('',*,*,#22272,.T.);
#29427=ORIENTED_EDGE('',*,*,#22275,.T.);
#29428=ORIENTED_EDGE('',*,*,#22266,.F.);
#29429=ORIENTED_EDGE('',*,*,#22276,.T.);
#29430=ORIENTED_EDGE('',*,*,#21458,.F.);
#29431=ORIENTED_EDGE('',*,*,#22277,.T.);
#29432=ORIENTED_EDGE('',*,*,#22164,.T.);
#29433=ORIENTED_EDGE('',*,*,#22278,.F.);
#29434=ORIENTED_EDGE('',*,*,#22279,.T.);
#29435=ORIENTED_EDGE('',*,*,#22269,.F.);
#29436=ORIENTED_EDGE('',*,*,#22280,.T.);
#29437=ORIENTED_EDGE('',*,*,#22281,.T.);
#29438=ORIENTED_EDGE('',*,*,#22282,.T.);
#29439=ORIENTED_EDGE('',*,*,#22278,.T.);
#29440=ORIENTED_EDGE('',*,*,#22283,.T.);
#29441=ORIENTED_EDGE('',*,*,#22284,.T.);
#29442=ORIENTED_EDGE('',*,*,#22285,.T.);
#29443=ORIENTED_EDGE('',*,*,#22286,.T.);
#29444=ORIENTED_EDGE('',*,*,#22287,.F.);
#29445=ORIENTED_EDGE('',*,*,#22288,.T.);
#29446=ORIENTED_EDGE('',*,*,#22289,.T.);
#29447=ORIENTED_EDGE('',*,*,#22287,.T.);
#29448=ORIENTED_EDGE('',*,*,#22290,.T.);
#29449=ORIENTED_EDGE('',*,*,#22281,.F.);
#29450=ORIENTED_EDGE('',*,*,#22291,.T.);
#29451=ORIENTED_EDGE('',*,*,#22292,.F.);
#29452=ORIENTED_EDGE('',*,*,#22293,.T.);
#29453=ORIENTED_EDGE('',*,*,#22284,.F.);
#29454=ORIENTED_EDGE('',*,*,#22294,.T.);
#29455=ORIENTED_EDGE('',*,*,#22295,.T.);
#29456=ORIENTED_EDGE('',*,*,#22296,.T.);
#29457=ORIENTED_EDGE('',*,*,#22292,.T.);
#29458=ORIENTED_EDGE('',*,*,#22297,.T.);
#29459=ORIENTED_EDGE('',*,*,#22298,.T.);
#29460=ORIENTED_EDGE('',*,*,#22299,.T.);
#29461=ORIENTED_EDGE('',*,*,#22300,.T.);
#29462=ORIENTED_EDGE('',*,*,#22301,.F.);
#29463=ORIENTED_EDGE('',*,*,#22302,.T.);
#29464=ORIENTED_EDGE('',*,*,#22303,.T.);
#29465=ORIENTED_EDGE('',*,*,#22301,.T.);
#29466=ORIENTED_EDGE('',*,*,#22304,.T.);
#29467=ORIENTED_EDGE('',*,*,#22295,.F.);
#29468=ORIENTED_EDGE('',*,*,#22305,.T.);
#29469=ORIENTED_EDGE('',*,*,#22306,.F.);
#29470=ORIENTED_EDGE('',*,*,#22307,.T.);
#29471=ORIENTED_EDGE('',*,*,#22298,.F.);
#29472=ORIENTED_EDGE('',*,*,#22308,.T.);
#29473=ORIENTED_EDGE('',*,*,#22309,.T.);
#29474=ORIENTED_EDGE('',*,*,#22310,.T.);
#29475=ORIENTED_EDGE('',*,*,#22306,.T.);
#29476=ORIENTED_EDGE('',*,*,#22311,.T.);
#29477=ORIENTED_EDGE('',*,*,#22312,.T.);
#29478=ORIENTED_EDGE('',*,*,#22313,.T.);
#29479=ORIENTED_EDGE('',*,*,#22314,.T.);
#29480=ORIENTED_EDGE('',*,*,#22315,.F.);
#29481=ORIENTED_EDGE('',*,*,#22316,.T.);
#29482=ORIENTED_EDGE('',*,*,#22317,.T.);
#29483=ORIENTED_EDGE('',*,*,#22315,.T.);
#29484=ORIENTED_EDGE('',*,*,#22318,.T.);
#29485=ORIENTED_EDGE('',*,*,#22309,.F.);
#29486=ORIENTED_EDGE('',*,*,#22319,.T.);
#29487=ORIENTED_EDGE('',*,*,#22320,.F.);
#29488=ORIENTED_EDGE('',*,*,#22321,.T.);
#29489=ORIENTED_EDGE('',*,*,#22312,.F.);
#29490=ORIENTED_EDGE('',*,*,#22322,.T.);
#29491=ORIENTED_EDGE('',*,*,#22323,.T.);
#29492=ORIENTED_EDGE('',*,*,#22324,.T.);
#29493=ORIENTED_EDGE('',*,*,#22325,.T.);
#29494=ORIENTED_EDGE('',*,*,#22326,.F.);
#29495=ORIENTED_EDGE('',*,*,#22327,.T.);
#29496=ORIENTED_EDGE('',*,*,#22328,.T.);
#29497=ORIENTED_EDGE('',*,*,#22329,.F.);
#29498=ORIENTED_EDGE('',*,*,#22330,.T.);
#29499=ORIENTED_EDGE('',*,*,#22323,.F.);
#29500=ORIENTED_EDGE('',*,*,#22331,.T.);
#29501=ORIENTED_EDGE('',*,*,#22332,.T.);
#29502=ORIENTED_EDGE('',*,*,#22333,.T.);
#29503=ORIENTED_EDGE('',*,*,#22320,.T.);
#29504=ORIENTED_EDGE('',*,*,#22334,.T.);
#29505=ORIENTED_EDGE('',*,*,#22326,.T.);
#29506=ORIENTED_EDGE('',*,*,#22335,.T.);
#29507=ORIENTED_EDGE('',*,*,#22332,.F.);
#29508=ORIENTED_EDGE('',*,*,#22336,.T.);
#29509=ORIENTED_EDGE('',*,*,#22337,.T.);
#29510=ORIENTED_EDGE('',*,*,#22338,.T.);
#29511=ORIENTED_EDGE('',*,*,#22329,.T.);
#29512=ORIENTED_EDGE('',*,*,#22339,.T.);
#29513=ORIENTED_EDGE('',*,*,#22340,.T.);
#29514=ORIENTED_EDGE('',*,*,#22341,.T.);
#29515=ORIENTED_EDGE('',*,*,#22342,.T.);
#29516=ORIENTED_EDGE('',*,*,#22343,.F.);
#29517=ORIENTED_EDGE('',*,*,#22344,.T.);
#29518=ORIENTED_EDGE('',*,*,#22345,.T.);
#29519=ORIENTED_EDGE('',*,*,#22343,.T.);
#29520=ORIENTED_EDGE('',*,*,#22346,.T.);
#29521=ORIENTED_EDGE('',*,*,#22337,.F.);
#29522=ORIENTED_EDGE('',*,*,#22347,.T.);
#29523=ORIENTED_EDGE('',*,*,#21652,.F.);
#29524=ORIENTED_EDGE('',*,*,#22348,.T.);
#29525=ORIENTED_EDGE('',*,*,#22340,.F.);
#29526=ORIENTED_EDGE('',*,*,#22349,.T.);
#29527=ORIENTED_EDGE('',*,*,#21649,.F.);
#29528=ORIENTED_EDGE('',*,*,#22350,.T.);
#29529=ORIENTED_EDGE('',*,*,#22351,.T.);
#29530=ORIENTED_EDGE('',*,*,#22352,.F.);
#29531=ORIENTED_EDGE('',*,*,#22352,.T.);
#29532=ORIENTED_EDGE('',*,*,#22353,.T.);
#29533=ORIENTED_EDGE('',*,*,#21650,.F.);
#29534=ORIENTED_EDGE('',*,*,#22354,.T.);
#29535=ORIENTED_EDGE('',*,*,#22355,.T.);
#29536=ORIENTED_EDGE('',*,*,#21451,.F.);
#29537=ORIENTED_EDGE('',*,*,#22356,.F.);
#29538=ORIENTED_EDGE('',*,*,#22357,.T.);
#29539=ORIENTED_EDGE('',*,*,#22358,.T.);
#29540=ORIENTED_EDGE('',*,*,#22359,.F.);
#29541=ORIENTED_EDGE('',*,*,#22360,.T.);
#29542=ORIENTED_EDGE('',*,*,#22354,.F.);
#29543=ORIENTED_EDGE('',*,*,#22361,.T.);
#29544=ORIENTED_EDGE('',*,*,#22362,.T.);
#29545=ORIENTED_EDGE('',*,*,#22363,.T.);
#29546=ORIENTED_EDGE('',*,*,#22359,.T.);
#29547=ORIENTED_EDGE('',*,*,#22364,.T.);
#29548=ORIENTED_EDGE('',*,*,#22365,.T.);
#29549=ORIENTED_EDGE('',*,*,#22366,.T.);
#29550=ORIENTED_EDGE('',*,*,#22367,.T.);
#29551=ORIENTED_EDGE('',*,*,#22368,.F.);
#29552=ORIENTED_EDGE('',*,*,#22369,.T.);
#29553=ORIENTED_EDGE('',*,*,#22370,.T.);
#29554=ORIENTED_EDGE('',*,*,#22368,.T.);
#29555=ORIENTED_EDGE('',*,*,#22371,.T.);
#29556=ORIENTED_EDGE('',*,*,#22362,.F.);
#29557=ORIENTED_EDGE('',*,*,#22372,.T.);
#29558=ORIENTED_EDGE('',*,*,#21454,.F.);
#29559=ORIENTED_EDGE('',*,*,#22373,.T.);
#29560=ORIENTED_EDGE('',*,*,#22260,.T.);
#29561=ORIENTED_EDGE('',*,*,#22374,.F.);
#29562=ORIENTED_EDGE('',*,*,#22375,.T.);
#29563=ORIENTED_EDGE('',*,*,#22365,.F.);
#29564=ORIENTED_EDGE('',*,*,#22376,.T.);
#29565=ORIENTED_EDGE('',*,*,#22377,.T.);
#29566=ORIENTED_EDGE('',*,*,#22378,.T.);
#29567=ORIENTED_EDGE('',*,*,#22374,.T.);
#29568=ORIENTED_EDGE('',*,*,#22379,.T.);
#29569=ORIENTED_EDGE('',*,*,#22380,.T.);
#29570=ORIENTED_EDGE('',*,*,#22381,.T.);
#29571=ORIENTED_EDGE('',*,*,#22382,.T.);
#29572=ORIENTED_EDGE('',*,*,#22383,.F.);
#29573=ORIENTED_EDGE('',*,*,#22384,.T.);
#29574=ORIENTED_EDGE('',*,*,#22385,.T.);
#29575=ORIENTED_EDGE('',*,*,#22383,.T.);
#29576=ORIENTED_EDGE('',*,*,#22386,.T.);
#29577=ORIENTED_EDGE('',*,*,#22377,.F.);
#29578=ORIENTED_EDGE('',*,*,#22387,.T.);
#29579=ORIENTED_EDGE('',*,*,#22388,.F.);
#29580=ORIENTED_EDGE('',*,*,#22389,.T.);
#29581=ORIENTED_EDGE('',*,*,#22380,.F.);
#29582=ORIENTED_EDGE('',*,*,#22390,.T.);
#29583=ORIENTED_EDGE('',*,*,#22391,.T.);
#29584=ORIENTED_EDGE('',*,*,#22392,.T.);
#29585=ORIENTED_EDGE('',*,*,#22388,.T.);
#29586=ORIENTED_EDGE('',*,*,#22393,.T.);
#29587=ORIENTED_EDGE('',*,*,#22394,.T.);
#29588=ORIENTED_EDGE('',*,*,#22395,.T.);
#29589=ORIENTED_EDGE('',*,*,#22396,.T.);
#29590=ORIENTED_EDGE('',*,*,#22397,.F.);
#29591=ORIENTED_EDGE('',*,*,#22398,.T.);
#29592=ORIENTED_EDGE('',*,*,#22399,.T.);
#29593=ORIENTED_EDGE('',*,*,#22397,.T.);
#29594=ORIENTED_EDGE('',*,*,#22400,.T.);
#29595=ORIENTED_EDGE('',*,*,#22391,.F.);
#29596=ORIENTED_EDGE('',*,*,#22401,.T.);
#29597=ORIENTED_EDGE('',*,*,#22402,.F.);
#29598=ORIENTED_EDGE('',*,*,#22403,.T.);
#29599=ORIENTED_EDGE('',*,*,#22394,.F.);
#29600=ORIENTED_EDGE('',*,*,#22404,.T.);
#29601=ORIENTED_EDGE('',*,*,#22405,.T.);
#29602=ORIENTED_EDGE('',*,*,#22406,.T.);
#29603=ORIENTED_EDGE('',*,*,#22402,.T.);
#29604=ORIENTED_EDGE('',*,*,#22407,.T.);
#29605=ORIENTED_EDGE('',*,*,#22408,.T.);
#29606=ORIENTED_EDGE('',*,*,#22409,.T.);
#29607=ORIENTED_EDGE('',*,*,#22410,.T.);
#29608=ORIENTED_EDGE('',*,*,#22411,.F.);
#29609=ORIENTED_EDGE('',*,*,#22412,.T.);
#29610=ORIENTED_EDGE('',*,*,#22413,.T.);
#29611=ORIENTED_EDGE('',*,*,#22411,.T.);
#29612=ORIENTED_EDGE('',*,*,#22414,.T.);
#29613=ORIENTED_EDGE('',*,*,#22405,.F.);
#29614=ORIENTED_EDGE('',*,*,#22415,.T.);
#29615=ORIENTED_EDGE('',*,*,#22416,.F.);
#29616=ORIENTED_EDGE('',*,*,#22417,.T.);
#29617=ORIENTED_EDGE('',*,*,#22408,.F.);
#29618=ORIENTED_EDGE('',*,*,#22418,.T.);
#29619=ORIENTED_EDGE('',*,*,#22419,.T.);
#29620=ORIENTED_EDGE('',*,*,#22420,.T.);
#29621=ORIENTED_EDGE('',*,*,#22416,.T.);
#29622=ORIENTED_EDGE('',*,*,#22421,.T.);
#29623=ORIENTED_EDGE('',*,*,#22422,.T.);
#29624=ORIENTED_EDGE('',*,*,#22423,.T.);
#29625=ORIENTED_EDGE('',*,*,#22424,.T.);
#29626=ORIENTED_EDGE('',*,*,#22425,.F.);
#29627=ORIENTED_EDGE('',*,*,#22426,.T.);
#29628=ORIENTED_EDGE('',*,*,#22427,.T.);
#29629=ORIENTED_EDGE('',*,*,#22425,.T.);
#29630=ORIENTED_EDGE('',*,*,#22428,.T.);
#29631=ORIENTED_EDGE('',*,*,#22419,.F.);
#29632=ORIENTED_EDGE('',*,*,#22429,.T.);
#29633=ORIENTED_EDGE('',*,*,#22430,.F.);
#29634=ORIENTED_EDGE('',*,*,#22431,.T.);
#29635=ORIENTED_EDGE('',*,*,#22422,.F.);
#29636=ORIENTED_EDGE('',*,*,#22432,.T.);
#29637=ORIENTED_EDGE('',*,*,#22433,.T.);
#29638=ORIENTED_EDGE('',*,*,#22434,.T.);
#29639=ORIENTED_EDGE('',*,*,#22435,.T.);
#29640=ORIENTED_EDGE('',*,*,#22436,.F.);
#29641=ORIENTED_EDGE('',*,*,#22437,.T.);
#29642=ORIENTED_EDGE('',*,*,#22438,.T.);
#29643=ORIENTED_EDGE('',*,*,#21658,.F.);
#29644=ORIENTED_EDGE('',*,*,#22439,.T.);
#29645=ORIENTED_EDGE('',*,*,#22433,.F.);
#29646=ORIENTED_EDGE('',*,*,#22440,.T.);
#29647=ORIENTED_EDGE('',*,*,#22441,.T.);
#29648=ORIENTED_EDGE('',*,*,#22442,.T.);
#29649=ORIENTED_EDGE('',*,*,#22430,.T.);
#29650=ORIENTED_EDGE('',*,*,#22443,.T.);
#29651=ORIENTED_EDGE('',*,*,#22436,.T.);
#29652=ORIENTED_EDGE('',*,*,#22444,.T.);
#29653=ORIENTED_EDGE('',*,*,#22441,.F.);
#29654=ORIENTED_EDGE('',*,*,#22445,.T.);
#29655=ORIENTED_EDGE('',*,*,#21655,.F.);
#29656=ORIENTED_EDGE('',*,*,#22446,.T.);
#29657=ORIENTED_EDGE('',*,*,#22447,.T.);
#29658=ORIENTED_EDGE('',*,*,#22448,.F.);
#29659=ORIENTED_EDGE('',*,*,#22448,.T.);
#29660=ORIENTED_EDGE('',*,*,#22449,.T.);
#29661=ORIENTED_EDGE('',*,*,#21656,.F.);
#29662=ORIENTED_EDGE('',*,*,#22450,.T.);
#29663=ORIENTED_EDGE('',*,*,#22451,.T.);
#29664=ORIENTED_EDGE('',*,*,#21447,.F.);
#29665=ORIENTED_EDGE('',*,*,#22452,.F.);
#29666=ORIENTED_EDGE('',*,*,#22453,.T.);
#29667=ORIENTED_EDGE('',*,*,#22454,.T.);
#29668=ORIENTED_EDGE('',*,*,#22455,.F.);
#29669=ORIENTED_EDGE('',*,*,#22456,.T.);
#29670=ORIENTED_EDGE('',*,*,#22450,.F.);
#29671=ORIENTED_EDGE('',*,*,#22457,.T.);
#29672=ORIENTED_EDGE('',*,*,#22458,.T.);
#29673=ORIENTED_EDGE('',*,*,#22459,.T.);
#29674=ORIENTED_EDGE('',*,*,#22455,.T.);
#29675=ORIENTED_EDGE('',*,*,#22460,.T.);
#29676=ORIENTED_EDGE('',*,*,#22461,.T.);
#29677=ORIENTED_EDGE('',*,*,#22462,.T.);
#29678=ORIENTED_EDGE('',*,*,#22463,.T.);
#29679=ORIENTED_EDGE('',*,*,#22464,.F.);
#29680=ORIENTED_EDGE('',*,*,#22465,.T.);
#29681=ORIENTED_EDGE('',*,*,#22466,.T.);
#29682=ORIENTED_EDGE('',*,*,#22464,.T.);
#29683=ORIENTED_EDGE('',*,*,#22467,.T.);
#29684=ORIENTED_EDGE('',*,*,#22458,.F.);
#29685=ORIENTED_EDGE('',*,*,#22468,.T.);
#29686=ORIENTED_EDGE('',*,*,#21450,.F.);
#29687=ORIENTED_EDGE('',*,*,#22469,.T.);
#29688=ORIENTED_EDGE('',*,*,#22356,.T.);
#29689=ORIENTED_EDGE('',*,*,#22470,.F.);
#29690=ORIENTED_EDGE('',*,*,#22471,.T.);
#29691=ORIENTED_EDGE('',*,*,#22461,.F.);
#29692=ORIENTED_EDGE('',*,*,#22472,.T.);
#29693=ORIENTED_EDGE('',*,*,#22473,.T.);
#29694=ORIENTED_EDGE('',*,*,#22474,.T.);
#29695=ORIENTED_EDGE('',*,*,#22470,.T.);
#29696=ORIENTED_EDGE('',*,*,#22475,.T.);
#29697=ORIENTED_EDGE('',*,*,#22476,.T.);
#29698=ORIENTED_EDGE('',*,*,#22477,.T.);
#29699=ORIENTED_EDGE('',*,*,#22478,.T.);
#29700=ORIENTED_EDGE('',*,*,#22479,.F.);
#29701=ORIENTED_EDGE('',*,*,#22480,.T.);
#29702=ORIENTED_EDGE('',*,*,#22481,.T.);
#29703=ORIENTED_EDGE('',*,*,#22479,.T.);
#29704=ORIENTED_EDGE('',*,*,#22482,.T.);
#29705=ORIENTED_EDGE('',*,*,#22473,.F.);
#29706=ORIENTED_EDGE('',*,*,#22483,.T.);
#29707=ORIENTED_EDGE('',*,*,#22484,.F.);
#29708=ORIENTED_EDGE('',*,*,#22485,.T.);
#29709=ORIENTED_EDGE('',*,*,#22476,.F.);
#29710=ORIENTED_EDGE('',*,*,#22486,.T.);
#29711=ORIENTED_EDGE('',*,*,#22487,.T.);
#29712=ORIENTED_EDGE('',*,*,#22488,.T.);
#29713=ORIENTED_EDGE('',*,*,#22484,.T.);
#29714=ORIENTED_EDGE('',*,*,#22489,.T.);
#29715=ORIENTED_EDGE('',*,*,#22490,.T.);
#29716=ORIENTED_EDGE('',*,*,#22491,.T.);
#29717=ORIENTED_EDGE('',*,*,#22492,.T.);
#29718=ORIENTED_EDGE('',*,*,#22493,.F.);
#29719=ORIENTED_EDGE('',*,*,#22494,.T.);
#29720=ORIENTED_EDGE('',*,*,#22495,.T.);
#29721=ORIENTED_EDGE('',*,*,#22493,.T.);
#29722=ORIENTED_EDGE('',*,*,#22496,.T.);
#29723=ORIENTED_EDGE('',*,*,#22487,.F.);
#29724=ORIENTED_EDGE('',*,*,#22497,.T.);
#29725=ORIENTED_EDGE('',*,*,#22498,.F.);
#29726=ORIENTED_EDGE('',*,*,#22499,.T.);
#29727=ORIENTED_EDGE('',*,*,#22490,.F.);
#29728=ORIENTED_EDGE('',*,*,#22500,.T.);
#29729=ORIENTED_EDGE('',*,*,#22501,.T.);
#29730=ORIENTED_EDGE('',*,*,#22502,.T.);
#29731=ORIENTED_EDGE('',*,*,#22498,.T.);
#29732=ORIENTED_EDGE('',*,*,#22503,.T.);
#29733=ORIENTED_EDGE('',*,*,#22504,.T.);
#29734=ORIENTED_EDGE('',*,*,#22505,.T.);
#29735=ORIENTED_EDGE('',*,*,#22506,.T.);
#29736=ORIENTED_EDGE('',*,*,#22507,.F.);
#29737=ORIENTED_EDGE('',*,*,#22508,.T.);
#29738=ORIENTED_EDGE('',*,*,#22509,.T.);
#29739=ORIENTED_EDGE('',*,*,#22507,.T.);
#29740=ORIENTED_EDGE('',*,*,#22510,.T.);
#29741=ORIENTED_EDGE('',*,*,#22501,.F.);
#29742=ORIENTED_EDGE('',*,*,#22511,.T.);
#29743=ORIENTED_EDGE('',*,*,#22512,.F.);
#29744=ORIENTED_EDGE('',*,*,#22513,.T.);
#29745=ORIENTED_EDGE('',*,*,#22504,.F.);
#29746=ORIENTED_EDGE('',*,*,#22514,.T.);
#29747=ORIENTED_EDGE('',*,*,#22515,.T.);
#29748=ORIENTED_EDGE('',*,*,#22516,.T.);
#29749=ORIENTED_EDGE('',*,*,#22512,.T.);
#29750=ORIENTED_EDGE('',*,*,#22517,.T.);
#29751=ORIENTED_EDGE('',*,*,#22518,.T.);
#29752=ORIENTED_EDGE('',*,*,#22519,.T.);
#29753=ORIENTED_EDGE('',*,*,#22520,.T.);
#29754=ORIENTED_EDGE('',*,*,#22521,.F.);
#29755=ORIENTED_EDGE('',*,*,#22522,.T.);
#29756=ORIENTED_EDGE('',*,*,#22523,.T.);
#29757=ORIENTED_EDGE('',*,*,#22521,.T.);
#29758=ORIENTED_EDGE('',*,*,#22524,.T.);
#29759=ORIENTED_EDGE('',*,*,#22515,.F.);
#29760=ORIENTED_EDGE('',*,*,#22525,.T.);
#29761=ORIENTED_EDGE('',*,*,#22526,.F.);
#29762=ORIENTED_EDGE('',*,*,#22527,.T.);
#29763=ORIENTED_EDGE('',*,*,#22518,.F.);
#29764=ORIENTED_EDGE('',*,*,#22528,.T.);
#29765=ORIENTED_EDGE('',*,*,#22529,.T.);
#29766=ORIENTED_EDGE('',*,*,#22530,.T.);
#29767=ORIENTED_EDGE('',*,*,#22526,.T.);
#29768=ORIENTED_EDGE('',*,*,#22531,.T.);
#29769=ORIENTED_EDGE('',*,*,#22532,.T.);
#29770=ORIENTED_EDGE('',*,*,#22533,.T.);
#29771=ORIENTED_EDGE('',*,*,#22534,.T.);
#29772=ORIENTED_EDGE('',*,*,#22535,.F.);
#29773=ORIENTED_EDGE('',*,*,#22536,.T.);
#29774=ORIENTED_EDGE('',*,*,#22537,.T.);
#29775=ORIENTED_EDGE('',*,*,#22535,.T.);
#29776=ORIENTED_EDGE('',*,*,#22538,.T.);
#29777=ORIENTED_EDGE('',*,*,#22529,.F.);
#29778=ORIENTED_EDGE('',*,*,#22539,.T.);
#29779=ORIENTED_EDGE('',*,*,#21664,.F.);
#29780=ORIENTED_EDGE('',*,*,#22540,.T.);
#29781=ORIENTED_EDGE('',*,*,#22532,.F.);
#29782=ORIENTED_EDGE('',*,*,#22541,.T.);
#29783=ORIENTED_EDGE('',*,*,#21661,.F.);
#29784=ORIENTED_EDGE('',*,*,#22542,.T.);
#29785=ORIENTED_EDGE('',*,*,#22543,.T.);
#29786=ORIENTED_EDGE('',*,*,#22544,.F.);
#29787=ORIENTED_EDGE('',*,*,#22544,.T.);
#29788=ORIENTED_EDGE('',*,*,#22545,.T.);
#29789=ORIENTED_EDGE('',*,*,#21662,.F.);
#29790=ORIENTED_EDGE('',*,*,#22546,.T.);
#29791=ORIENTED_EDGE('',*,*,#22547,.T.);
#29792=ORIENTED_EDGE('',*,*,#21443,.F.);
#29793=ORIENTED_EDGE('',*,*,#22548,.F.);
#29794=ORIENTED_EDGE('',*,*,#22549,.T.);
#29795=ORIENTED_EDGE('',*,*,#22550,.T.);
#29796=ORIENTED_EDGE('',*,*,#22551,.F.);
#29797=ORIENTED_EDGE('',*,*,#22552,.T.);
#29798=ORIENTED_EDGE('',*,*,#22546,.F.);
#29799=ORIENTED_EDGE('',*,*,#22553,.T.);
#29800=ORIENTED_EDGE('',*,*,#22554,.T.);
#29801=ORIENTED_EDGE('',*,*,#22555,.T.);
#29802=ORIENTED_EDGE('',*,*,#22551,.T.);
#29803=ORIENTED_EDGE('',*,*,#22556,.T.);
#29804=ORIENTED_EDGE('',*,*,#22557,.T.);
#29805=ORIENTED_EDGE('',*,*,#22558,.T.);
#29806=ORIENTED_EDGE('',*,*,#22559,.T.);
#29807=ORIENTED_EDGE('',*,*,#22560,.F.);
#29808=ORIENTED_EDGE('',*,*,#22561,.T.);
#29809=ORIENTED_EDGE('',*,*,#22562,.T.);
#29810=ORIENTED_EDGE('',*,*,#22560,.T.);
#29811=ORIENTED_EDGE('',*,*,#22563,.T.);
#29812=ORIENTED_EDGE('',*,*,#22554,.F.);
#29813=ORIENTED_EDGE('',*,*,#22564,.T.);
#29814=ORIENTED_EDGE('',*,*,#21446,.F.);
#29815=ORIENTED_EDGE('',*,*,#22565,.T.);
#29816=ORIENTED_EDGE('',*,*,#22452,.T.);
#29817=ORIENTED_EDGE('',*,*,#22566,.F.);
#29818=ORIENTED_EDGE('',*,*,#22567,.T.);
#29819=ORIENTED_EDGE('',*,*,#22557,.F.);
#29820=ORIENTED_EDGE('',*,*,#22568,.T.);
#29821=ORIENTED_EDGE('',*,*,#22569,.T.);
#29822=ORIENTED_EDGE('',*,*,#22570,.T.);
#29823=ORIENTED_EDGE('',*,*,#22566,.T.);
#29824=ORIENTED_EDGE('',*,*,#22571,.T.);
#29825=ORIENTED_EDGE('',*,*,#22572,.T.);
#29826=ORIENTED_EDGE('',*,*,#22573,.T.);
#29827=ORIENTED_EDGE('',*,*,#22574,.T.);
#29828=ORIENTED_EDGE('',*,*,#22575,.F.);
#29829=ORIENTED_EDGE('',*,*,#22576,.T.);
#29830=ORIENTED_EDGE('',*,*,#22577,.T.);
#29831=ORIENTED_EDGE('',*,*,#22575,.T.);
#29832=ORIENTED_EDGE('',*,*,#22578,.T.);
#29833=ORIENTED_EDGE('',*,*,#22569,.F.);
#29834=ORIENTED_EDGE('',*,*,#22579,.T.);
#29835=ORIENTED_EDGE('',*,*,#22580,.F.);
#29836=ORIENTED_EDGE('',*,*,#22581,.T.);
#29837=ORIENTED_EDGE('',*,*,#22572,.F.);
#29838=ORIENTED_EDGE('',*,*,#22582,.T.);
#29839=ORIENTED_EDGE('',*,*,#22583,.T.);
#29840=ORIENTED_EDGE('',*,*,#22584,.T.);
#29841=ORIENTED_EDGE('',*,*,#22580,.T.);
#29842=ORIENTED_EDGE('',*,*,#22585,.T.);
#29843=ORIENTED_EDGE('',*,*,#22586,.T.);
#29844=ORIENTED_EDGE('',*,*,#22587,.T.);
#29845=ORIENTED_EDGE('',*,*,#22588,.T.);
#29846=ORIENTED_EDGE('',*,*,#22589,.F.);
#29847=ORIENTED_EDGE('',*,*,#22590,.T.);
#29848=ORIENTED_EDGE('',*,*,#22591,.T.);
#29849=ORIENTED_EDGE('',*,*,#22589,.T.);
#29850=ORIENTED_EDGE('',*,*,#22592,.T.);
#29851=ORIENTED_EDGE('',*,*,#22583,.F.);
#29852=ORIENTED_EDGE('',*,*,#22593,.T.);
#29853=ORIENTED_EDGE('',*,*,#22594,.F.);
#29854=ORIENTED_EDGE('',*,*,#22595,.T.);
#29855=ORIENTED_EDGE('',*,*,#22586,.F.);
#29856=ORIENTED_EDGE('',*,*,#22596,.T.);
#29857=ORIENTED_EDGE('',*,*,#22597,.T.);
#29858=ORIENTED_EDGE('',*,*,#22598,.T.);
#29859=ORIENTED_EDGE('',*,*,#22594,.T.);
#29860=ORIENTED_EDGE('',*,*,#22599,.T.);
#29861=ORIENTED_EDGE('',*,*,#22600,.T.);
#29862=ORIENTED_EDGE('',*,*,#22601,.T.);
#29863=ORIENTED_EDGE('',*,*,#22602,.T.);
#29864=ORIENTED_EDGE('',*,*,#22603,.F.);
#29865=ORIENTED_EDGE('',*,*,#22604,.T.);
#29866=ORIENTED_EDGE('',*,*,#22605,.T.);
#29867=ORIENTED_EDGE('',*,*,#22603,.T.);
#29868=ORIENTED_EDGE('',*,*,#22606,.T.);
#29869=ORIENTED_EDGE('',*,*,#22597,.F.);
#29870=ORIENTED_EDGE('',*,*,#22607,.T.);
#29871=ORIENTED_EDGE('',*,*,#22608,.F.);
#29872=ORIENTED_EDGE('',*,*,#22609,.T.);
#29873=ORIENTED_EDGE('',*,*,#22600,.F.);
#29874=ORIENTED_EDGE('',*,*,#22610,.T.);
#29875=ORIENTED_EDGE('',*,*,#22611,.T.);
#29876=ORIENTED_EDGE('',*,*,#22612,.T.);
#29877=ORIENTED_EDGE('',*,*,#22608,.T.);
#29878=ORIENTED_EDGE('',*,*,#22613,.T.);
#29879=ORIENTED_EDGE('',*,*,#22614,.T.);
#29880=ORIENTED_EDGE('',*,*,#22615,.T.);
#29881=ORIENTED_EDGE('',*,*,#22616,.T.);
#29882=ORIENTED_EDGE('',*,*,#22617,.F.);
#29883=ORIENTED_EDGE('',*,*,#22618,.T.);
#29884=ORIENTED_EDGE('',*,*,#22619,.T.);
#29885=ORIENTED_EDGE('',*,*,#22617,.T.);
#29886=ORIENTED_EDGE('',*,*,#22620,.T.);
#29887=ORIENTED_EDGE('',*,*,#22611,.F.);
#29888=ORIENTED_EDGE('',*,*,#22621,.T.);
#29889=ORIENTED_EDGE('',*,*,#22622,.F.);
#29890=ORIENTED_EDGE('',*,*,#22623,.T.);
#29891=ORIENTED_EDGE('',*,*,#22614,.F.);
#29892=ORIENTED_EDGE('',*,*,#22624,.T.);
#29893=ORIENTED_EDGE('',*,*,#22625,.T.);
#29894=ORIENTED_EDGE('',*,*,#22626,.T.);
#29895=ORIENTED_EDGE('',*,*,#22622,.T.);
#29896=ORIENTED_EDGE('',*,*,#22627,.T.);
#29897=ORIENTED_EDGE('',*,*,#22628,.T.);
#29898=ORIENTED_EDGE('',*,*,#22629,.T.);
#29899=ORIENTED_EDGE('',*,*,#22630,.T.);
#29900=ORIENTED_EDGE('',*,*,#22631,.F.);
#29901=ORIENTED_EDGE('',*,*,#22632,.T.);
#29902=ORIENTED_EDGE('',*,*,#22633,.T.);
#29903=ORIENTED_EDGE('',*,*,#22631,.T.);
#29904=ORIENTED_EDGE('',*,*,#22634,.T.);
#29905=ORIENTED_EDGE('',*,*,#22625,.F.);
#29906=ORIENTED_EDGE('',*,*,#22635,.T.);
#29907=ORIENTED_EDGE('',*,*,#21670,.F.);
#29908=ORIENTED_EDGE('',*,*,#22636,.T.);
#29909=ORIENTED_EDGE('',*,*,#22628,.F.);
#29910=ORIENTED_EDGE('',*,*,#22637,.T.);
#29911=ORIENTED_EDGE('',*,*,#21667,.F.);
#29912=ORIENTED_EDGE('',*,*,#22638,.T.);
#29913=ORIENTED_EDGE('',*,*,#22639,.T.);
#29914=ORIENTED_EDGE('',*,*,#22640,.F.);
#29915=ORIENTED_EDGE('',*,*,#22640,.T.);
#29916=ORIENTED_EDGE('',*,*,#22641,.T.);
#29917=ORIENTED_EDGE('',*,*,#21668,.F.);
#29918=ORIENTED_EDGE('',*,*,#22642,.T.);
#29919=ORIENTED_EDGE('',*,*,#22643,.T.);
#29920=ORIENTED_EDGE('',*,*,#21439,.F.);
#29921=ORIENTED_EDGE('',*,*,#22644,.F.);
#29922=ORIENTED_EDGE('',*,*,#22645,.T.);
#29923=ORIENTED_EDGE('',*,*,#22646,.T.);
#29924=ORIENTED_EDGE('',*,*,#22647,.F.);
#29925=ORIENTED_EDGE('',*,*,#22648,.T.);
#29926=ORIENTED_EDGE('',*,*,#22642,.F.);
#29927=ORIENTED_EDGE('',*,*,#22649,.T.);
#29928=ORIENTED_EDGE('',*,*,#22650,.T.);
#29929=ORIENTED_EDGE('',*,*,#22651,.T.);
#29930=ORIENTED_EDGE('',*,*,#22647,.T.);
#29931=ORIENTED_EDGE('',*,*,#22652,.T.);
#29932=ORIENTED_EDGE('',*,*,#22653,.T.);
#29933=ORIENTED_EDGE('',*,*,#22654,.T.);
#29934=ORIENTED_EDGE('',*,*,#22655,.T.);
#29935=ORIENTED_EDGE('',*,*,#22656,.F.);
#29936=ORIENTED_EDGE('',*,*,#22657,.T.);
#29937=ORIENTED_EDGE('',*,*,#22658,.T.);
#29938=ORIENTED_EDGE('',*,*,#22656,.T.);
#29939=ORIENTED_EDGE('',*,*,#22659,.T.);
#29940=ORIENTED_EDGE('',*,*,#22650,.F.);
#29941=ORIENTED_EDGE('',*,*,#22660,.T.);
#29942=ORIENTED_EDGE('',*,*,#21442,.F.);
#29943=ORIENTED_EDGE('',*,*,#22661,.T.);
#29944=ORIENTED_EDGE('',*,*,#22548,.T.);
#29945=ORIENTED_EDGE('',*,*,#22662,.F.);
#29946=ORIENTED_EDGE('',*,*,#22663,.T.);
#29947=ORIENTED_EDGE('',*,*,#22653,.F.);
#29948=ORIENTED_EDGE('',*,*,#22664,.T.);
#29949=ORIENTED_EDGE('',*,*,#22665,.T.);
#29950=ORIENTED_EDGE('',*,*,#22666,.T.);
#29951=ORIENTED_EDGE('',*,*,#22662,.T.);
#29952=ORIENTED_EDGE('',*,*,#22667,.T.);
#29953=ORIENTED_EDGE('',*,*,#22668,.T.);
#29954=ORIENTED_EDGE('',*,*,#22669,.T.);
#29955=ORIENTED_EDGE('',*,*,#22670,.T.);
#29956=ORIENTED_EDGE('',*,*,#22671,.F.);
#29957=ORIENTED_EDGE('',*,*,#22672,.T.);
#29958=ORIENTED_EDGE('',*,*,#22673,.T.);
#29959=ORIENTED_EDGE('',*,*,#22671,.T.);
#29960=ORIENTED_EDGE('',*,*,#22674,.T.);
#29961=ORIENTED_EDGE('',*,*,#22665,.F.);
#29962=ORIENTED_EDGE('',*,*,#22675,.T.);
#29963=ORIENTED_EDGE('',*,*,#22676,.F.);
#29964=ORIENTED_EDGE('',*,*,#22677,.T.);
#29965=ORIENTED_EDGE('',*,*,#22668,.F.);
#29966=ORIENTED_EDGE('',*,*,#22678,.T.);
#29967=ORIENTED_EDGE('',*,*,#22679,.T.);
#29968=ORIENTED_EDGE('',*,*,#22680,.T.);
#29969=ORIENTED_EDGE('',*,*,#22676,.T.);
#29970=ORIENTED_EDGE('',*,*,#22681,.T.);
#29971=ORIENTED_EDGE('',*,*,#22682,.T.);
#29972=ORIENTED_EDGE('',*,*,#22683,.T.);
#29973=ORIENTED_EDGE('',*,*,#22684,.T.);
#29974=ORIENTED_EDGE('',*,*,#22685,.F.);
#29975=ORIENTED_EDGE('',*,*,#22686,.T.);
#29976=ORIENTED_EDGE('',*,*,#22687,.T.);
#29977=ORIENTED_EDGE('',*,*,#22685,.T.);
#29978=ORIENTED_EDGE('',*,*,#22688,.T.);
#29979=ORIENTED_EDGE('',*,*,#22679,.F.);
#29980=ORIENTED_EDGE('',*,*,#22689,.T.);
#29981=ORIENTED_EDGE('',*,*,#22690,.F.);
#29982=ORIENTED_EDGE('',*,*,#22691,.T.);
#29983=ORIENTED_EDGE('',*,*,#22682,.F.);
#29984=ORIENTED_EDGE('',*,*,#22692,.T.);
#29985=ORIENTED_EDGE('',*,*,#22693,.T.);
#29986=ORIENTED_EDGE('',*,*,#22694,.T.);
#29987=ORIENTED_EDGE('',*,*,#22690,.T.);
#29988=ORIENTED_EDGE('',*,*,#22695,.T.);
#29989=ORIENTED_EDGE('',*,*,#22696,.T.);
#29990=ORIENTED_EDGE('',*,*,#22697,.T.);
#29991=ORIENTED_EDGE('',*,*,#22698,.T.);
#29992=ORIENTED_EDGE('',*,*,#22699,.F.);
#29993=ORIENTED_EDGE('',*,*,#22700,.T.);
#29994=ORIENTED_EDGE('',*,*,#22701,.T.);
#29995=ORIENTED_EDGE('',*,*,#22699,.T.);
#29996=ORIENTED_EDGE('',*,*,#22702,.T.);
#29997=ORIENTED_EDGE('',*,*,#22693,.F.);
#29998=ORIENTED_EDGE('',*,*,#22703,.T.);
#29999=ORIENTED_EDGE('',*,*,#22704,.F.);
#30000=ORIENTED_EDGE('',*,*,#22705,.T.);
#30001=ORIENTED_EDGE('',*,*,#22696,.F.);
#30002=ORIENTED_EDGE('',*,*,#22706,.T.);
#30003=ORIENTED_EDGE('',*,*,#22707,.T.);
#30004=ORIENTED_EDGE('',*,*,#22708,.T.);
#30005=ORIENTED_EDGE('',*,*,#22704,.T.);
#30006=ORIENTED_EDGE('',*,*,#22709,.T.);
#30007=ORIENTED_EDGE('',*,*,#22710,.T.);
#30008=ORIENTED_EDGE('',*,*,#22711,.T.);
#30009=ORIENTED_EDGE('',*,*,#22712,.T.);
#30010=ORIENTED_EDGE('',*,*,#22713,.F.);
#30011=ORIENTED_EDGE('',*,*,#22714,.T.);
#30012=ORIENTED_EDGE('',*,*,#22715,.T.);
#30013=ORIENTED_EDGE('',*,*,#22713,.T.);
#30014=ORIENTED_EDGE('',*,*,#22716,.T.);
#30015=ORIENTED_EDGE('',*,*,#22707,.F.);
#30016=ORIENTED_EDGE('',*,*,#22717,.T.);
#30017=ORIENTED_EDGE('',*,*,#22718,.F.);
#30018=ORIENTED_EDGE('',*,*,#22719,.T.);
#30019=ORIENTED_EDGE('',*,*,#22710,.F.);
#30020=ORIENTED_EDGE('',*,*,#22720,.T.);
#30021=ORIENTED_EDGE('',*,*,#22721,.T.);
#30022=ORIENTED_EDGE('',*,*,#22722,.T.);
#30023=ORIENTED_EDGE('',*,*,#22718,.T.);
#30024=ORIENTED_EDGE('',*,*,#22723,.T.);
#30025=ORIENTED_EDGE('',*,*,#22724,.T.);
#30026=ORIENTED_EDGE('',*,*,#22725,.T.);
#30027=ORIENTED_EDGE('',*,*,#22726,.T.);
#30028=ORIENTED_EDGE('',*,*,#22727,.F.);
#30029=ORIENTED_EDGE('',*,*,#22728,.T.);
#30030=ORIENTED_EDGE('',*,*,#22729,.T.);
#30031=ORIENTED_EDGE('',*,*,#22727,.T.);
#30032=ORIENTED_EDGE('',*,*,#22730,.T.);
#30033=ORIENTED_EDGE('',*,*,#22721,.F.);
#30034=ORIENTED_EDGE('',*,*,#22731,.T.);
#30035=ORIENTED_EDGE('',*,*,#21676,.F.);
#30036=ORIENTED_EDGE('',*,*,#22732,.T.);
#30037=ORIENTED_EDGE('',*,*,#22724,.F.);
#30038=ORIENTED_EDGE('',*,*,#22733,.T.);
#30039=ORIENTED_EDGE('',*,*,#21673,.F.);
#30040=ORIENTED_EDGE('',*,*,#22734,.T.);
#30041=ORIENTED_EDGE('',*,*,#22735,.T.);
#30042=ORIENTED_EDGE('',*,*,#22736,.F.);
#30043=ORIENTED_EDGE('',*,*,#22736,.T.);
#30044=ORIENTED_EDGE('',*,*,#22737,.T.);
#30045=ORIENTED_EDGE('',*,*,#21674,.F.);
#30046=ORIENTED_EDGE('',*,*,#22738,.T.);
#30047=ORIENTED_EDGE('',*,*,#22739,.T.);
#30048=ORIENTED_EDGE('',*,*,#21435,.F.);
#30049=ORIENTED_EDGE('',*,*,#22740,.F.);
#30050=ORIENTED_EDGE('',*,*,#22741,.T.);
#30051=ORIENTED_EDGE('',*,*,#22742,.T.);
#30052=ORIENTED_EDGE('',*,*,#22743,.F.);
#30053=ORIENTED_EDGE('',*,*,#22744,.T.);
#30054=ORIENTED_EDGE('',*,*,#22738,.F.);
#30055=ORIENTED_EDGE('',*,*,#22745,.T.);
#30056=ORIENTED_EDGE('',*,*,#22746,.T.);
#30057=ORIENTED_EDGE('',*,*,#22747,.T.);
#30058=ORIENTED_EDGE('',*,*,#22743,.T.);
#30059=ORIENTED_EDGE('',*,*,#22748,.T.);
#30060=ORIENTED_EDGE('',*,*,#22749,.T.);
#30061=ORIENTED_EDGE('',*,*,#22750,.T.);
#30062=ORIENTED_EDGE('',*,*,#22751,.T.);
#30063=ORIENTED_EDGE('',*,*,#22752,.F.);
#30064=ORIENTED_EDGE('',*,*,#22753,.T.);
#30065=ORIENTED_EDGE('',*,*,#22754,.T.);
#30066=ORIENTED_EDGE('',*,*,#22752,.T.);
#30067=ORIENTED_EDGE('',*,*,#22755,.T.);
#30068=ORIENTED_EDGE('',*,*,#22746,.F.);
#30069=ORIENTED_EDGE('',*,*,#22756,.T.);
#30070=ORIENTED_EDGE('',*,*,#21438,.F.);
#30071=ORIENTED_EDGE('',*,*,#22757,.T.);
#30072=ORIENTED_EDGE('',*,*,#22644,.T.);
#30073=ORIENTED_EDGE('',*,*,#22758,.F.);
#30074=ORIENTED_EDGE('',*,*,#22759,.T.);
#30075=ORIENTED_EDGE('',*,*,#22749,.F.);
#30076=ORIENTED_EDGE('',*,*,#22760,.T.);
#30077=ORIENTED_EDGE('',*,*,#22761,.T.);
#30078=ORIENTED_EDGE('',*,*,#22762,.T.);
#30079=ORIENTED_EDGE('',*,*,#22758,.T.);
#30080=ORIENTED_EDGE('',*,*,#22763,.T.);
#30081=ORIENTED_EDGE('',*,*,#22764,.T.);
#30082=ORIENTED_EDGE('',*,*,#22765,.T.);
#30083=ORIENTED_EDGE('',*,*,#22766,.T.);
#30084=ORIENTED_EDGE('',*,*,#22767,.F.);
#30085=ORIENTED_EDGE('',*,*,#22768,.T.);
#30086=ORIENTED_EDGE('',*,*,#22769,.T.);
#30087=ORIENTED_EDGE('',*,*,#22767,.T.);
#30088=ORIENTED_EDGE('',*,*,#22770,.T.);
#30089=ORIENTED_EDGE('',*,*,#22761,.F.);
#30090=ORIENTED_EDGE('',*,*,#22771,.T.);
#30091=ORIENTED_EDGE('',*,*,#22772,.F.);
#30092=ORIENTED_EDGE('',*,*,#22773,.T.);
#30093=ORIENTED_EDGE('',*,*,#22764,.F.);
#30094=ORIENTED_EDGE('',*,*,#22774,.T.);
#30095=ORIENTED_EDGE('',*,*,#22775,.T.);
#30096=ORIENTED_EDGE('',*,*,#22776,.T.);
#30097=ORIENTED_EDGE('',*,*,#22772,.T.);
#30098=ORIENTED_EDGE('',*,*,#22777,.T.);
#30099=ORIENTED_EDGE('',*,*,#22778,.T.);
#30100=ORIENTED_EDGE('',*,*,#22779,.T.);
#30101=ORIENTED_EDGE('',*,*,#22780,.T.);
#30102=ORIENTED_EDGE('',*,*,#22781,.F.);
#30103=ORIENTED_EDGE('',*,*,#22782,.T.);
#30104=ORIENTED_EDGE('',*,*,#22783,.T.);
#30105=ORIENTED_EDGE('',*,*,#22781,.T.);
#30106=ORIENTED_EDGE('',*,*,#22784,.T.);
#30107=ORIENTED_EDGE('',*,*,#22775,.F.);
#30108=ORIENTED_EDGE('',*,*,#22785,.T.);
#30109=ORIENTED_EDGE('',*,*,#22786,.F.);
#30110=ORIENTED_EDGE('',*,*,#22787,.T.);
#30111=ORIENTED_EDGE('',*,*,#22778,.F.);
#30112=ORIENTED_EDGE('',*,*,#22788,.T.);
#30113=ORIENTED_EDGE('',*,*,#22789,.T.);
#30114=ORIENTED_EDGE('',*,*,#22790,.T.);
#30115=ORIENTED_EDGE('',*,*,#22786,.T.);
#30116=ORIENTED_EDGE('',*,*,#22791,.T.);
#30117=ORIENTED_EDGE('',*,*,#22792,.T.);
#30118=ORIENTED_EDGE('',*,*,#22793,.T.);
#30119=ORIENTED_EDGE('',*,*,#22794,.T.);
#30120=ORIENTED_EDGE('',*,*,#22795,.F.);
#30121=ORIENTED_EDGE('',*,*,#22796,.T.);
#30122=ORIENTED_EDGE('',*,*,#22797,.T.);
#30123=ORIENTED_EDGE('',*,*,#22795,.T.);
#30124=ORIENTED_EDGE('',*,*,#22798,.T.);
#30125=ORIENTED_EDGE('',*,*,#22789,.F.);
#30126=ORIENTED_EDGE('',*,*,#22799,.T.);
#30127=ORIENTED_EDGE('',*,*,#22800,.F.);
#30128=ORIENTED_EDGE('',*,*,#22801,.T.);
#30129=ORIENTED_EDGE('',*,*,#22792,.F.);
#30130=ORIENTED_EDGE('',*,*,#22802,.T.);
#30131=ORIENTED_EDGE('',*,*,#22803,.T.);
#30132=ORIENTED_EDGE('',*,*,#22804,.T.);
#30133=ORIENTED_EDGE('',*,*,#22800,.T.);
#30134=ORIENTED_EDGE('',*,*,#22805,.T.);
#30135=ORIENTED_EDGE('',*,*,#22806,.T.);
#30136=ORIENTED_EDGE('',*,*,#22807,.T.);
#30137=ORIENTED_EDGE('',*,*,#22808,.T.);
#30138=ORIENTED_EDGE('',*,*,#22809,.F.);
#30139=ORIENTED_EDGE('',*,*,#22810,.T.);
#30140=ORIENTED_EDGE('',*,*,#22811,.T.);
#30141=ORIENTED_EDGE('',*,*,#22809,.T.);
#30142=ORIENTED_EDGE('',*,*,#22812,.T.);
#30143=ORIENTED_EDGE('',*,*,#22803,.F.);
#30144=ORIENTED_EDGE('',*,*,#22813,.T.);
#30145=ORIENTED_EDGE('',*,*,#22814,.F.);
#30146=ORIENTED_EDGE('',*,*,#22815,.T.);
#30147=ORIENTED_EDGE('',*,*,#22806,.F.);
#30148=ORIENTED_EDGE('',*,*,#22816,.T.);
#30149=ORIENTED_EDGE('',*,*,#22817,.T.);
#30150=ORIENTED_EDGE('',*,*,#22818,.T.);
#30151=ORIENTED_EDGE('',*,*,#22814,.T.);
#30152=ORIENTED_EDGE('',*,*,#22819,.T.);
#30153=ORIENTED_EDGE('',*,*,#22820,.T.);
#30154=ORIENTED_EDGE('',*,*,#22821,.T.);
#30155=ORIENTED_EDGE('',*,*,#22822,.T.);
#30156=ORIENTED_EDGE('',*,*,#22823,.F.);
#30157=ORIENTED_EDGE('',*,*,#22824,.T.);
#30158=ORIENTED_EDGE('',*,*,#22825,.T.);
#30159=ORIENTED_EDGE('',*,*,#22823,.T.);
#30160=ORIENTED_EDGE('',*,*,#22826,.T.);
#30161=ORIENTED_EDGE('',*,*,#22817,.F.);
#30162=ORIENTED_EDGE('',*,*,#22827,.T.);
#30163=ORIENTED_EDGE('',*,*,#21682,.F.);
#30164=ORIENTED_EDGE('',*,*,#22828,.T.);
#30165=ORIENTED_EDGE('',*,*,#22820,.F.);
#30166=ORIENTED_EDGE('',*,*,#22829,.T.);
#30167=ORIENTED_EDGE('',*,*,#21679,.F.);
#30168=ORIENTED_EDGE('',*,*,#22830,.T.);
#30169=ORIENTED_EDGE('',*,*,#22831,.T.);
#30170=ORIENTED_EDGE('',*,*,#22832,.F.);
#30171=ORIENTED_EDGE('',*,*,#22832,.T.);
#30172=ORIENTED_EDGE('',*,*,#22833,.T.);
#30173=ORIENTED_EDGE('',*,*,#21680,.F.);
#30174=ORIENTED_EDGE('',*,*,#22834,.T.);
#30175=ORIENTED_EDGE('',*,*,#22835,.T.);
#30176=ORIENTED_EDGE('',*,*,#21431,.F.);
#30177=ORIENTED_EDGE('',*,*,#22836,.F.);
#30178=ORIENTED_EDGE('',*,*,#22837,.T.);
#30179=ORIENTED_EDGE('',*,*,#22838,.T.);
#30180=ORIENTED_EDGE('',*,*,#22839,.F.);
#30181=ORIENTED_EDGE('',*,*,#22840,.T.);
#30182=ORIENTED_EDGE('',*,*,#22834,.F.);
#30183=ORIENTED_EDGE('',*,*,#22841,.T.);
#30184=ORIENTED_EDGE('',*,*,#22842,.T.);
#30185=ORIENTED_EDGE('',*,*,#22843,.T.);
#30186=ORIENTED_EDGE('',*,*,#22839,.T.);
#30187=ORIENTED_EDGE('',*,*,#22844,.T.);
#30188=ORIENTED_EDGE('',*,*,#22845,.T.);
#30189=ORIENTED_EDGE('',*,*,#22846,.T.);
#30190=ORIENTED_EDGE('',*,*,#22847,.T.);
#30191=ORIENTED_EDGE('',*,*,#22848,.F.);
#30192=ORIENTED_EDGE('',*,*,#22849,.T.);
#30193=ORIENTED_EDGE('',*,*,#22850,.T.);
#30194=ORIENTED_EDGE('',*,*,#22848,.T.);
#30195=ORIENTED_EDGE('',*,*,#22851,.T.);
#30196=ORIENTED_EDGE('',*,*,#22842,.F.);
#30197=ORIENTED_EDGE('',*,*,#22852,.T.);
#30198=ORIENTED_EDGE('',*,*,#21434,.F.);
#30199=ORIENTED_EDGE('',*,*,#22853,.T.);
#30200=ORIENTED_EDGE('',*,*,#22740,.T.);
#30201=ORIENTED_EDGE('',*,*,#22854,.F.);
#30202=ORIENTED_EDGE('',*,*,#22855,.T.);
#30203=ORIENTED_EDGE('',*,*,#22845,.F.);
#30204=ORIENTED_EDGE('',*,*,#22856,.T.);
#30205=ORIENTED_EDGE('',*,*,#22857,.T.);
#30206=ORIENTED_EDGE('',*,*,#22858,.T.);
#30207=ORIENTED_EDGE('',*,*,#22854,.T.);
#30208=ORIENTED_EDGE('',*,*,#22859,.T.);
#30209=ORIENTED_EDGE('',*,*,#22860,.T.);
#30210=ORIENTED_EDGE('',*,*,#22861,.T.);
#30211=ORIENTED_EDGE('',*,*,#22862,.T.);
#30212=ORIENTED_EDGE('',*,*,#22863,.F.);
#30213=ORIENTED_EDGE('',*,*,#22864,.T.);
#30214=ORIENTED_EDGE('',*,*,#22865,.T.);
#30215=ORIENTED_EDGE('',*,*,#22863,.T.);
#30216=ORIENTED_EDGE('',*,*,#22866,.T.);
#30217=ORIENTED_EDGE('',*,*,#22857,.F.);
#30218=ORIENTED_EDGE('',*,*,#22867,.T.);
#30219=ORIENTED_EDGE('',*,*,#22868,.F.);
#30220=ORIENTED_EDGE('',*,*,#22869,.T.);
#30221=ORIENTED_EDGE('',*,*,#22860,.F.);
#30222=ORIENTED_EDGE('',*,*,#22870,.T.);
#30223=ORIENTED_EDGE('',*,*,#22871,.T.);
#30224=ORIENTED_EDGE('',*,*,#22872,.T.);
#30225=ORIENTED_EDGE('',*,*,#22868,.T.);
#30226=ORIENTED_EDGE('',*,*,#22873,.T.);
#30227=ORIENTED_EDGE('',*,*,#22874,.T.);
#30228=ORIENTED_EDGE('',*,*,#22875,.T.);
#30229=ORIENTED_EDGE('',*,*,#22876,.T.);
#30230=ORIENTED_EDGE('',*,*,#22877,.F.);
#30231=ORIENTED_EDGE('',*,*,#22878,.T.);
#30232=ORIENTED_EDGE('',*,*,#22879,.T.);
#30233=ORIENTED_EDGE('',*,*,#22877,.T.);
#30234=ORIENTED_EDGE('',*,*,#22880,.T.);
#30235=ORIENTED_EDGE('',*,*,#22871,.F.);
#30236=ORIENTED_EDGE('',*,*,#22881,.T.);
#30237=ORIENTED_EDGE('',*,*,#22882,.F.);
#30238=ORIENTED_EDGE('',*,*,#22883,.T.);
#30239=ORIENTED_EDGE('',*,*,#22874,.F.);
#30240=ORIENTED_EDGE('',*,*,#22884,.T.);
#30241=ORIENTED_EDGE('',*,*,#22885,.T.);
#30242=ORIENTED_EDGE('',*,*,#22886,.T.);
#30243=ORIENTED_EDGE('',*,*,#22882,.T.);
#30244=ORIENTED_EDGE('',*,*,#22887,.T.);
#30245=ORIENTED_EDGE('',*,*,#22888,.T.);
#30246=ORIENTED_EDGE('',*,*,#22889,.T.);
#30247=ORIENTED_EDGE('',*,*,#22890,.T.);
#30248=ORIENTED_EDGE('',*,*,#22891,.F.);
#30249=ORIENTED_EDGE('',*,*,#22892,.T.);
#30250=ORIENTED_EDGE('',*,*,#22893,.T.);
#30251=ORIENTED_EDGE('',*,*,#22891,.T.);
#30252=ORIENTED_EDGE('',*,*,#22894,.T.);
#30253=ORIENTED_EDGE('',*,*,#22885,.F.);
#30254=ORIENTED_EDGE('',*,*,#22895,.T.);
#30255=ORIENTED_EDGE('',*,*,#22896,.F.);
#30256=ORIENTED_EDGE('',*,*,#22897,.T.);
#30257=ORIENTED_EDGE('',*,*,#22888,.F.);
#30258=ORIENTED_EDGE('',*,*,#22898,.T.);
#30259=ORIENTED_EDGE('',*,*,#22899,.T.);
#30260=ORIENTED_EDGE('',*,*,#22900,.T.);
#30261=ORIENTED_EDGE('',*,*,#22896,.T.);
#30262=ORIENTED_EDGE('',*,*,#22901,.T.);
#30263=ORIENTED_EDGE('',*,*,#22902,.T.);
#30264=ORIENTED_EDGE('',*,*,#22903,.T.);
#30265=ORIENTED_EDGE('',*,*,#22904,.T.);
#30266=ORIENTED_EDGE('',*,*,#22905,.F.);
#30267=ORIENTED_EDGE('',*,*,#22906,.T.);
#30268=ORIENTED_EDGE('',*,*,#22907,.T.);
#30269=ORIENTED_EDGE('',*,*,#22905,.T.);
#30270=ORIENTED_EDGE('',*,*,#22908,.T.);
#30271=ORIENTED_EDGE('',*,*,#22899,.F.);
#30272=ORIENTED_EDGE('',*,*,#22909,.T.);
#30273=ORIENTED_EDGE('',*,*,#22910,.F.);
#30274=ORIENTED_EDGE('',*,*,#22911,.T.);
#30275=ORIENTED_EDGE('',*,*,#22902,.F.);
#30276=ORIENTED_EDGE('',*,*,#22912,.T.);
#30277=ORIENTED_EDGE('',*,*,#22913,.T.);
#30278=ORIENTED_EDGE('',*,*,#22914,.T.);
#30279=ORIENTED_EDGE('',*,*,#22910,.T.);
#30280=ORIENTED_EDGE('',*,*,#22915,.T.);
#30281=ORIENTED_EDGE('',*,*,#22916,.T.);
#30282=ORIENTED_EDGE('',*,*,#22917,.T.);
#30283=ORIENTED_EDGE('',*,*,#22918,.T.);
#30284=ORIENTED_EDGE('',*,*,#22919,.F.);
#30285=ORIENTED_EDGE('',*,*,#22920,.T.);
#30286=ORIENTED_EDGE('',*,*,#22921,.T.);
#30287=ORIENTED_EDGE('',*,*,#22919,.T.);
#30288=ORIENTED_EDGE('',*,*,#22922,.T.);
#30289=ORIENTED_EDGE('',*,*,#22913,.F.);
#30290=ORIENTED_EDGE('',*,*,#22923,.T.);
#30291=ORIENTED_EDGE('',*,*,#21688,.F.);
#30292=ORIENTED_EDGE('',*,*,#22924,.T.);
#30293=ORIENTED_EDGE('',*,*,#22916,.F.);
#30294=ORIENTED_EDGE('',*,*,#22925,.T.);
#30295=ORIENTED_EDGE('',*,*,#21685,.F.);
#30296=ORIENTED_EDGE('',*,*,#22926,.T.);
#30297=ORIENTED_EDGE('',*,*,#22927,.T.);
#30298=ORIENTED_EDGE('',*,*,#22928,.F.);
#30299=ORIENTED_EDGE('',*,*,#22928,.T.);
#30300=ORIENTED_EDGE('',*,*,#22929,.T.);
#30301=ORIENTED_EDGE('',*,*,#21686,.F.);
#30302=ORIENTED_EDGE('',*,*,#22930,.T.);
#30303=ORIENTED_EDGE('',*,*,#22931,.T.);
#30304=ORIENTED_EDGE('',*,*,#21427,.F.);
#30305=ORIENTED_EDGE('',*,*,#22932,.F.);
#30306=ORIENTED_EDGE('',*,*,#22933,.T.);
#30307=ORIENTED_EDGE('',*,*,#22934,.T.);
#30308=ORIENTED_EDGE('',*,*,#22935,.F.);
#30309=ORIENTED_EDGE('',*,*,#22936,.T.);
#30310=ORIENTED_EDGE('',*,*,#22930,.F.);
#30311=ORIENTED_EDGE('',*,*,#22937,.T.);
#30312=ORIENTED_EDGE('',*,*,#22938,.T.);
#30313=ORIENTED_EDGE('',*,*,#22939,.T.);
#30314=ORIENTED_EDGE('',*,*,#22935,.T.);
#30315=ORIENTED_EDGE('',*,*,#22940,.T.);
#30316=ORIENTED_EDGE('',*,*,#22941,.T.);
#30317=ORIENTED_EDGE('',*,*,#22942,.T.);
#30318=ORIENTED_EDGE('',*,*,#22943,.T.);
#30319=ORIENTED_EDGE('',*,*,#22944,.F.);
#30320=ORIENTED_EDGE('',*,*,#22945,.T.);
#30321=ORIENTED_EDGE('',*,*,#22946,.T.);
#30322=ORIENTED_EDGE('',*,*,#22944,.T.);
#30323=ORIENTED_EDGE('',*,*,#22947,.T.);
#30324=ORIENTED_EDGE('',*,*,#22938,.F.);
#30325=ORIENTED_EDGE('',*,*,#22948,.T.);
#30326=ORIENTED_EDGE('',*,*,#21430,.F.);
#30327=ORIENTED_EDGE('',*,*,#22949,.T.);
#30328=ORIENTED_EDGE('',*,*,#22836,.T.);
#30329=ORIENTED_EDGE('',*,*,#22950,.F.);
#30330=ORIENTED_EDGE('',*,*,#22951,.T.);
#30331=ORIENTED_EDGE('',*,*,#22941,.F.);
#30332=ORIENTED_EDGE('',*,*,#22952,.T.);
#30333=ORIENTED_EDGE('',*,*,#22953,.T.);
#30334=ORIENTED_EDGE('',*,*,#22954,.T.);
#30335=ORIENTED_EDGE('',*,*,#22950,.T.);
#30336=ORIENTED_EDGE('',*,*,#22955,.T.);
#30337=ORIENTED_EDGE('',*,*,#22956,.T.);
#30338=ORIENTED_EDGE('',*,*,#22957,.T.);
#30339=ORIENTED_EDGE('',*,*,#22958,.T.);
#30340=ORIENTED_EDGE('',*,*,#22959,.F.);
#30341=ORIENTED_EDGE('',*,*,#22960,.T.);
#30342=ORIENTED_EDGE('',*,*,#22961,.T.);
#30343=ORIENTED_EDGE('',*,*,#22959,.T.);
#30344=ORIENTED_EDGE('',*,*,#22962,.T.);
#30345=ORIENTED_EDGE('',*,*,#22953,.F.);
#30346=ORIENTED_EDGE('',*,*,#22963,.T.);
#30347=ORIENTED_EDGE('',*,*,#22964,.F.);
#30348=ORIENTED_EDGE('',*,*,#22965,.T.);
#30349=ORIENTED_EDGE('',*,*,#22956,.F.);
#30350=ORIENTED_EDGE('',*,*,#22966,.T.);
#30351=ORIENTED_EDGE('',*,*,#22967,.T.);
#30352=ORIENTED_EDGE('',*,*,#22968,.T.);
#30353=ORIENTED_EDGE('',*,*,#22964,.T.);
#30354=ORIENTED_EDGE('',*,*,#22969,.T.);
#30355=ORIENTED_EDGE('',*,*,#22970,.T.);
#30356=ORIENTED_EDGE('',*,*,#22971,.T.);
#30357=ORIENTED_EDGE('',*,*,#22972,.T.);
#30358=ORIENTED_EDGE('',*,*,#22973,.F.);
#30359=ORIENTED_EDGE('',*,*,#22974,.T.);
#30360=ORIENTED_EDGE('',*,*,#22975,.T.);
#30361=ORIENTED_EDGE('',*,*,#22973,.T.);
#30362=ORIENTED_EDGE('',*,*,#22976,.T.);
#30363=ORIENTED_EDGE('',*,*,#22967,.F.);
#30364=ORIENTED_EDGE('',*,*,#22977,.T.);
#30365=ORIENTED_EDGE('',*,*,#22978,.F.);
#30366=ORIENTED_EDGE('',*,*,#22979,.T.);
#30367=ORIENTED_EDGE('',*,*,#22970,.F.);
#30368=ORIENTED_EDGE('',*,*,#22980,.T.);
#30369=ORIENTED_EDGE('',*,*,#22981,.T.);
#30370=ORIENTED_EDGE('',*,*,#22982,.T.);
#30371=ORIENTED_EDGE('',*,*,#22978,.T.);
#30372=ORIENTED_EDGE('',*,*,#22983,.T.);
#30373=ORIENTED_EDGE('',*,*,#22984,.T.);
#30374=ORIENTED_EDGE('',*,*,#22985,.T.);
#30375=ORIENTED_EDGE('',*,*,#22986,.T.);
#30376=ORIENTED_EDGE('',*,*,#22987,.F.);
#30377=ORIENTED_EDGE('',*,*,#22988,.T.);
#30378=ORIENTED_EDGE('',*,*,#22989,.T.);
#30379=ORIENTED_EDGE('',*,*,#22987,.T.);
#30380=ORIENTED_EDGE('',*,*,#22990,.T.);
#30381=ORIENTED_EDGE('',*,*,#22981,.F.);
#30382=ORIENTED_EDGE('',*,*,#22991,.T.);
#30383=ORIENTED_EDGE('',*,*,#22992,.F.);
#30384=ORIENTED_EDGE('',*,*,#22993,.T.);
#30385=ORIENTED_EDGE('',*,*,#22984,.F.);
#30386=ORIENTED_EDGE('',*,*,#22994,.T.);
#30387=ORIENTED_EDGE('',*,*,#22995,.T.);
#30388=ORIENTED_EDGE('',*,*,#22996,.T.);
#30389=ORIENTED_EDGE('',*,*,#22992,.T.);
#30390=ORIENTED_EDGE('',*,*,#22997,.T.);
#30391=ORIENTED_EDGE('',*,*,#22998,.T.);
#30392=ORIENTED_EDGE('',*,*,#22999,.T.);
#30393=ORIENTED_EDGE('',*,*,#23000,.T.);
#30394=ORIENTED_EDGE('',*,*,#23001,.F.);
#30395=ORIENTED_EDGE('',*,*,#23002,.T.);
#30396=ORIENTED_EDGE('',*,*,#23003,.T.);
#30397=ORIENTED_EDGE('',*,*,#23001,.T.);
#30398=ORIENTED_EDGE('',*,*,#23004,.T.);
#30399=ORIENTED_EDGE('',*,*,#22995,.F.);
#30400=ORIENTED_EDGE('',*,*,#23005,.T.);
#30401=ORIENTED_EDGE('',*,*,#23006,.F.);
#30402=ORIENTED_EDGE('',*,*,#23007,.T.);
#30403=ORIENTED_EDGE('',*,*,#22998,.F.);
#30404=ORIENTED_EDGE('',*,*,#23008,.T.);
#30405=ORIENTED_EDGE('',*,*,#23009,.T.);
#30406=ORIENTED_EDGE('',*,*,#23010,.T.);
#30407=ORIENTED_EDGE('',*,*,#23006,.T.);
#30408=ORIENTED_EDGE('',*,*,#23011,.T.);
#30409=ORIENTED_EDGE('',*,*,#23012,.T.);
#30410=ORIENTED_EDGE('',*,*,#23013,.T.);
#30411=ORIENTED_EDGE('',*,*,#23014,.T.);
#30412=ORIENTED_EDGE('',*,*,#23015,.F.);
#30413=ORIENTED_EDGE('',*,*,#23016,.T.);
#30414=ORIENTED_EDGE('',*,*,#23017,.T.);
#30415=ORIENTED_EDGE('',*,*,#23015,.T.);
#30416=ORIENTED_EDGE('',*,*,#23018,.T.);
#30417=ORIENTED_EDGE('',*,*,#23009,.F.);
#30418=ORIENTED_EDGE('',*,*,#23019,.T.);
#30419=ORIENTED_EDGE('',*,*,#21694,.F.);
#30420=ORIENTED_EDGE('',*,*,#23020,.T.);
#30421=ORIENTED_EDGE('',*,*,#23012,.F.);
#30422=ORIENTED_EDGE('',*,*,#23021,.T.);
#30423=ORIENTED_EDGE('',*,*,#21691,.F.);
#30424=ORIENTED_EDGE('',*,*,#23022,.T.);
#30425=ORIENTED_EDGE('',*,*,#23023,.T.);
#30426=ORIENTED_EDGE('',*,*,#23024,.F.);
#30427=ORIENTED_EDGE('',*,*,#23024,.T.);
#30428=ORIENTED_EDGE('',*,*,#23025,.T.);
#30429=ORIENTED_EDGE('',*,*,#21692,.F.);
#30430=ORIENTED_EDGE('',*,*,#23026,.T.);
#30431=ORIENTED_EDGE('',*,*,#23027,.T.);
#30432=ORIENTED_EDGE('',*,*,#21423,.F.);
#30433=ORIENTED_EDGE('',*,*,#23028,.F.);
#30434=ORIENTED_EDGE('',*,*,#23029,.T.);
#30435=ORIENTED_EDGE('',*,*,#23030,.T.);
#30436=ORIENTED_EDGE('',*,*,#23031,.F.);
#30437=ORIENTED_EDGE('',*,*,#23032,.T.);
#30438=ORIENTED_EDGE('',*,*,#23026,.F.);
#30439=ORIENTED_EDGE('',*,*,#23033,.T.);
#30440=ORIENTED_EDGE('',*,*,#23034,.T.);
#30441=ORIENTED_EDGE('',*,*,#23035,.T.);
#30442=ORIENTED_EDGE('',*,*,#23031,.T.);
#30443=ORIENTED_EDGE('',*,*,#23036,.T.);
#30444=ORIENTED_EDGE('',*,*,#23037,.T.);
#30445=ORIENTED_EDGE('',*,*,#23038,.T.);
#30446=ORIENTED_EDGE('',*,*,#23039,.T.);
#30447=ORIENTED_EDGE('',*,*,#23040,.F.);
#30448=ORIENTED_EDGE('',*,*,#23041,.T.);
#30449=ORIENTED_EDGE('',*,*,#23042,.T.);
#30450=ORIENTED_EDGE('',*,*,#23040,.T.);
#30451=ORIENTED_EDGE('',*,*,#23043,.T.);
#30452=ORIENTED_EDGE('',*,*,#23034,.F.);
#30453=ORIENTED_EDGE('',*,*,#23044,.T.);
#30454=ORIENTED_EDGE('',*,*,#21426,.F.);
#30455=ORIENTED_EDGE('',*,*,#23045,.T.);
#30456=ORIENTED_EDGE('',*,*,#22932,.T.);
#30457=ORIENTED_EDGE('',*,*,#23046,.F.);
#30458=ORIENTED_EDGE('',*,*,#23047,.T.);
#30459=ORIENTED_EDGE('',*,*,#23037,.F.);
#30460=ORIENTED_EDGE('',*,*,#23048,.T.);
#30461=ORIENTED_EDGE('',*,*,#23049,.T.);
#30462=ORIENTED_EDGE('',*,*,#23050,.T.);
#30463=ORIENTED_EDGE('',*,*,#23046,.T.);
#30464=ORIENTED_EDGE('',*,*,#23051,.T.);
#30465=ORIENTED_EDGE('',*,*,#23052,.T.);
#30466=ORIENTED_EDGE('',*,*,#23053,.T.);
#30467=ORIENTED_EDGE('',*,*,#23054,.T.);
#30468=ORIENTED_EDGE('',*,*,#23055,.F.);
#30469=ORIENTED_EDGE('',*,*,#23056,.T.);
#30470=ORIENTED_EDGE('',*,*,#23057,.T.);
#30471=ORIENTED_EDGE('',*,*,#23055,.T.);
#30472=ORIENTED_EDGE('',*,*,#23058,.T.);
#30473=ORIENTED_EDGE('',*,*,#23049,.F.);
#30474=ORIENTED_EDGE('',*,*,#23059,.T.);
#30475=ORIENTED_EDGE('',*,*,#23060,.F.);
#30476=ORIENTED_EDGE('',*,*,#23061,.T.);
#30477=ORIENTED_EDGE('',*,*,#23052,.F.);
#30478=ORIENTED_EDGE('',*,*,#23062,.T.);
#30479=ORIENTED_EDGE('',*,*,#23063,.T.);
#30480=ORIENTED_EDGE('',*,*,#23064,.T.);
#30481=ORIENTED_EDGE('',*,*,#23060,.T.);
#30482=ORIENTED_EDGE('',*,*,#23065,.T.);
#30483=ORIENTED_EDGE('',*,*,#23066,.T.);
#30484=ORIENTED_EDGE('',*,*,#23067,.T.);
#30485=ORIENTED_EDGE('',*,*,#23068,.T.);
#30486=ORIENTED_EDGE('',*,*,#23069,.F.);
#30487=ORIENTED_EDGE('',*,*,#23070,.T.);
#30488=ORIENTED_EDGE('',*,*,#23071,.T.);
#30489=ORIENTED_EDGE('',*,*,#23069,.T.);
#30490=ORIENTED_EDGE('',*,*,#23072,.T.);
#30491=ORIENTED_EDGE('',*,*,#23063,.F.);
#30492=ORIENTED_EDGE('',*,*,#23073,.T.);
#30493=ORIENTED_EDGE('',*,*,#23074,.F.);
#30494=ORIENTED_EDGE('',*,*,#23075,.T.);
#30495=ORIENTED_EDGE('',*,*,#23066,.F.);
#30496=ORIENTED_EDGE('',*,*,#23076,.T.);
#30497=ORIENTED_EDGE('',*,*,#23077,.T.);
#30498=ORIENTED_EDGE('',*,*,#23078,.T.);
#30499=ORIENTED_EDGE('',*,*,#23074,.T.);
#30500=ORIENTED_EDGE('',*,*,#23079,.T.);
#30501=ORIENTED_EDGE('',*,*,#23080,.T.);
#30502=ORIENTED_EDGE('',*,*,#23081,.T.);
#30503=ORIENTED_EDGE('',*,*,#23082,.T.);
#30504=ORIENTED_EDGE('',*,*,#23083,.F.);
#30505=ORIENTED_EDGE('',*,*,#23084,.T.);
#30506=ORIENTED_EDGE('',*,*,#23085,.T.);
#30507=ORIENTED_EDGE('',*,*,#23083,.T.);
#30508=ORIENTED_EDGE('',*,*,#23086,.T.);
#30509=ORIENTED_EDGE('',*,*,#23077,.F.);
#30510=ORIENTED_EDGE('',*,*,#23087,.T.);
#30511=ORIENTED_EDGE('',*,*,#23088,.F.);
#30512=ORIENTED_EDGE('',*,*,#23089,.T.);
#30513=ORIENTED_EDGE('',*,*,#23080,.F.);
#30514=ORIENTED_EDGE('',*,*,#23090,.T.);
#30515=ORIENTED_EDGE('',*,*,#23091,.T.);
#30516=ORIENTED_EDGE('',*,*,#23092,.T.);
#30517=ORIENTED_EDGE('',*,*,#23088,.T.);
#30518=ORIENTED_EDGE('',*,*,#23093,.T.);
#30519=ORIENTED_EDGE('',*,*,#23094,.T.);
#30520=ORIENTED_EDGE('',*,*,#23095,.T.);
#30521=ORIENTED_EDGE('',*,*,#23096,.T.);
#30522=ORIENTED_EDGE('',*,*,#23097,.F.);
#30523=ORIENTED_EDGE('',*,*,#23098,.T.);
#30524=ORIENTED_EDGE('',*,*,#23099,.T.);
#30525=ORIENTED_EDGE('',*,*,#23097,.T.);
#30526=ORIENTED_EDGE('',*,*,#23100,.T.);
#30527=ORIENTED_EDGE('',*,*,#23091,.F.);
#30528=ORIENTED_EDGE('',*,*,#23101,.T.);
#30529=ORIENTED_EDGE('',*,*,#23102,.F.);
#30530=ORIENTED_EDGE('',*,*,#23103,.T.);
#30531=ORIENTED_EDGE('',*,*,#23094,.F.);
#30532=ORIENTED_EDGE('',*,*,#23104,.T.);
#30533=ORIENTED_EDGE('',*,*,#23105,.T.);
#30534=ORIENTED_EDGE('',*,*,#23106,.T.);
#30535=ORIENTED_EDGE('',*,*,#23102,.T.);
#30536=ORIENTED_EDGE('',*,*,#23107,.T.);
#30537=ORIENTED_EDGE('',*,*,#23108,.T.);
#30538=ORIENTED_EDGE('',*,*,#23109,.T.);
#30539=ORIENTED_EDGE('',*,*,#23110,.T.);
#30540=ORIENTED_EDGE('',*,*,#23111,.F.);
#30541=ORIENTED_EDGE('',*,*,#23112,.T.);
#30542=ORIENTED_EDGE('',*,*,#23113,.T.);
#30543=ORIENTED_EDGE('',*,*,#23111,.T.);
#30544=ORIENTED_EDGE('',*,*,#23114,.T.);
#30545=ORIENTED_EDGE('',*,*,#23105,.F.);
#30546=ORIENTED_EDGE('',*,*,#23115,.T.);
#30547=ORIENTED_EDGE('',*,*,#21700,.F.);
#30548=ORIENTED_EDGE('',*,*,#23116,.T.);
#30549=ORIENTED_EDGE('',*,*,#23108,.F.);
#30550=ORIENTED_EDGE('',*,*,#23117,.T.);
#30551=ORIENTED_EDGE('',*,*,#21697,.F.);
#30552=ORIENTED_EDGE('',*,*,#23118,.T.);
#30553=ORIENTED_EDGE('',*,*,#23119,.T.);
#30554=ORIENTED_EDGE('',*,*,#23120,.F.);
#30555=ORIENTED_EDGE('',*,*,#23120,.T.);
#30556=ORIENTED_EDGE('',*,*,#23121,.T.);
#30557=ORIENTED_EDGE('',*,*,#21698,.F.);
#30558=ORIENTED_EDGE('',*,*,#23122,.T.);
#30559=ORIENTED_EDGE('',*,*,#23123,.T.);
#30560=ORIENTED_EDGE('',*,*,#21419,.F.);
#30561=ORIENTED_EDGE('',*,*,#23124,.F.);
#30562=ORIENTED_EDGE('',*,*,#23125,.T.);
#30563=ORIENTED_EDGE('',*,*,#23126,.T.);
#30564=ORIENTED_EDGE('',*,*,#23127,.F.);
#30565=ORIENTED_EDGE('',*,*,#23128,.T.);
#30566=ORIENTED_EDGE('',*,*,#23122,.F.);
#30567=ORIENTED_EDGE('',*,*,#23129,.T.);
#30568=ORIENTED_EDGE('',*,*,#23130,.T.);
#30569=ORIENTED_EDGE('',*,*,#23131,.T.);
#30570=ORIENTED_EDGE('',*,*,#23127,.T.);
#30571=ORIENTED_EDGE('',*,*,#23132,.T.);
#30572=ORIENTED_EDGE('',*,*,#23133,.T.);
#30573=ORIENTED_EDGE('',*,*,#23134,.T.);
#30574=ORIENTED_EDGE('',*,*,#23135,.T.);
#30575=ORIENTED_EDGE('',*,*,#23136,.F.);
#30576=ORIENTED_EDGE('',*,*,#23137,.T.);
#30577=ORIENTED_EDGE('',*,*,#23138,.T.);
#30578=ORIENTED_EDGE('',*,*,#23136,.T.);
#30579=ORIENTED_EDGE('',*,*,#23139,.T.);
#30580=ORIENTED_EDGE('',*,*,#23130,.F.);
#30581=ORIENTED_EDGE('',*,*,#23140,.T.);
#30582=ORIENTED_EDGE('',*,*,#21422,.F.);
#30583=ORIENTED_EDGE('',*,*,#23141,.T.);
#30584=ORIENTED_EDGE('',*,*,#23028,.T.);
#30585=ORIENTED_EDGE('',*,*,#23142,.F.);
#30586=ORIENTED_EDGE('',*,*,#23143,.T.);
#30587=ORIENTED_EDGE('',*,*,#23133,.F.);
#30588=ORIENTED_EDGE('',*,*,#23144,.T.);
#30589=ORIENTED_EDGE('',*,*,#23145,.T.);
#30590=ORIENTED_EDGE('',*,*,#23146,.T.);
#30591=ORIENTED_EDGE('',*,*,#23142,.T.);
#30592=ORIENTED_EDGE('',*,*,#23147,.T.);
#30593=ORIENTED_EDGE('',*,*,#23148,.T.);
#30594=ORIENTED_EDGE('',*,*,#23149,.T.);
#30595=ORIENTED_EDGE('',*,*,#23150,.T.);
#30596=ORIENTED_EDGE('',*,*,#23151,.F.);
#30597=ORIENTED_EDGE('',*,*,#23152,.T.);
#30598=ORIENTED_EDGE('',*,*,#23153,.T.);
#30599=ORIENTED_EDGE('',*,*,#23151,.T.);
#30600=ORIENTED_EDGE('',*,*,#23154,.T.);
#30601=ORIENTED_EDGE('',*,*,#23145,.F.);
#30602=ORIENTED_EDGE('',*,*,#23155,.T.);
#30603=ORIENTED_EDGE('',*,*,#23156,.F.);
#30604=ORIENTED_EDGE('',*,*,#23157,.T.);
#30605=ORIENTED_EDGE('',*,*,#23148,.F.);
#30606=ORIENTED_EDGE('',*,*,#23158,.T.);
#30607=ORIENTED_EDGE('',*,*,#23159,.T.);
#30608=ORIENTED_EDGE('',*,*,#23160,.T.);
#30609=ORIENTED_EDGE('',*,*,#23156,.T.);
#30610=ORIENTED_EDGE('',*,*,#23161,.T.);
#30611=ORIENTED_EDGE('',*,*,#23162,.T.);
#30612=ORIENTED_EDGE('',*,*,#23163,.T.);
#30613=ORIENTED_EDGE('',*,*,#23164,.T.);
#30614=ORIENTED_EDGE('',*,*,#23165,.F.);
#30615=ORIENTED_EDGE('',*,*,#23166,.T.);
#30616=ORIENTED_EDGE('',*,*,#23167,.T.);
#30617=ORIENTED_EDGE('',*,*,#23165,.T.);
#30618=ORIENTED_EDGE('',*,*,#23168,.T.);
#30619=ORIENTED_EDGE('',*,*,#23159,.F.);
#30620=ORIENTED_EDGE('',*,*,#23169,.T.);
#30621=ORIENTED_EDGE('',*,*,#23170,.F.);
#30622=ORIENTED_EDGE('',*,*,#23171,.T.);
#30623=ORIENTED_EDGE('',*,*,#23162,.F.);
#30624=ORIENTED_EDGE('',*,*,#23172,.T.);
#30625=ORIENTED_EDGE('',*,*,#23173,.T.);
#30626=ORIENTED_EDGE('',*,*,#23174,.T.);
#30627=ORIENTED_EDGE('',*,*,#23170,.T.);
#30628=ORIENTED_EDGE('',*,*,#23175,.T.);
#30629=ORIENTED_EDGE('',*,*,#23176,.T.);
#30630=ORIENTED_EDGE('',*,*,#23177,.T.);
#30631=ORIENTED_EDGE('',*,*,#23178,.T.);
#30632=ORIENTED_EDGE('',*,*,#23179,.F.);
#30633=ORIENTED_EDGE('',*,*,#23180,.T.);
#30634=ORIENTED_EDGE('',*,*,#23181,.T.);
#30635=ORIENTED_EDGE('',*,*,#23179,.T.);
#30636=ORIENTED_EDGE('',*,*,#23182,.T.);
#30637=ORIENTED_EDGE('',*,*,#23173,.F.);
#30638=ORIENTED_EDGE('',*,*,#23183,.T.);
#30639=ORIENTED_EDGE('',*,*,#23184,.F.);
#30640=ORIENTED_EDGE('',*,*,#23185,.T.);
#30641=ORIENTED_EDGE('',*,*,#23176,.F.);
#30642=ORIENTED_EDGE('',*,*,#23186,.T.);
#30643=ORIENTED_EDGE('',*,*,#23187,.T.);
#30644=ORIENTED_EDGE('',*,*,#23188,.T.);
#30645=ORIENTED_EDGE('',*,*,#23184,.T.);
#30646=ORIENTED_EDGE('',*,*,#23189,.T.);
#30647=ORIENTED_EDGE('',*,*,#23190,.T.);
#30648=ORIENTED_EDGE('',*,*,#23191,.T.);
#30649=ORIENTED_EDGE('',*,*,#23192,.T.);
#30650=ORIENTED_EDGE('',*,*,#23193,.F.);
#30651=ORIENTED_EDGE('',*,*,#23194,.T.);
#30652=ORIENTED_EDGE('',*,*,#23195,.T.);
#30653=ORIENTED_EDGE('',*,*,#23193,.T.);
#30654=ORIENTED_EDGE('',*,*,#23196,.T.);
#30655=ORIENTED_EDGE('',*,*,#23187,.F.);
#30656=ORIENTED_EDGE('',*,*,#23197,.T.);
#30657=ORIENTED_EDGE('',*,*,#23198,.F.);
#30658=ORIENTED_EDGE('',*,*,#23199,.T.);
#30659=ORIENTED_EDGE('',*,*,#23190,.F.);
#30660=ORIENTED_EDGE('',*,*,#23200,.T.);
#30661=ORIENTED_EDGE('',*,*,#23201,.T.);
#30662=ORIENTED_EDGE('',*,*,#23202,.T.);
#30663=ORIENTED_EDGE('',*,*,#23198,.T.);
#30664=ORIENTED_EDGE('',*,*,#23203,.T.);
#30665=ORIENTED_EDGE('',*,*,#23204,.T.);
#30666=ORIENTED_EDGE('',*,*,#23205,.T.);
#30667=ORIENTED_EDGE('',*,*,#23206,.T.);
#30668=ORIENTED_EDGE('',*,*,#23207,.F.);
#30669=ORIENTED_EDGE('',*,*,#23208,.T.);
#30670=ORIENTED_EDGE('',*,*,#23209,.T.);
#30671=ORIENTED_EDGE('',*,*,#23207,.T.);
#30672=ORIENTED_EDGE('',*,*,#23210,.T.);
#30673=ORIENTED_EDGE('',*,*,#23201,.F.);
#30674=ORIENTED_EDGE('',*,*,#23211,.T.);
#30675=ORIENTED_EDGE('',*,*,#21706,.F.);
#30676=ORIENTED_EDGE('',*,*,#23212,.T.);
#30677=ORIENTED_EDGE('',*,*,#23204,.F.);
#30678=ORIENTED_EDGE('',*,*,#23213,.T.);
#30679=ORIENTED_EDGE('',*,*,#21703,.F.);
#30680=ORIENTED_EDGE('',*,*,#23214,.T.);
#30681=ORIENTED_EDGE('',*,*,#23215,.T.);
#30682=ORIENTED_EDGE('',*,*,#23216,.F.);
#30683=ORIENTED_EDGE('',*,*,#23216,.T.);
#30684=ORIENTED_EDGE('',*,*,#23217,.T.);
#30685=ORIENTED_EDGE('',*,*,#21704,.F.);
#30686=ORIENTED_EDGE('',*,*,#23218,.T.);
#30687=ORIENTED_EDGE('',*,*,#23219,.T.);
#30688=ORIENTED_EDGE('',*,*,#21415,.F.);
#30689=ORIENTED_EDGE('',*,*,#23220,.F.);
#30690=ORIENTED_EDGE('',*,*,#23221,.T.);
#30691=ORIENTED_EDGE('',*,*,#23222,.T.);
#30692=ORIENTED_EDGE('',*,*,#23223,.F.);
#30693=ORIENTED_EDGE('',*,*,#23224,.T.);
#30694=ORIENTED_EDGE('',*,*,#23218,.F.);
#30695=ORIENTED_EDGE('',*,*,#23225,.T.);
#30696=ORIENTED_EDGE('',*,*,#23226,.T.);
#30697=ORIENTED_EDGE('',*,*,#23227,.T.);
#30698=ORIENTED_EDGE('',*,*,#23223,.T.);
#30699=ORIENTED_EDGE('',*,*,#23228,.T.);
#30700=ORIENTED_EDGE('',*,*,#23229,.T.);
#30701=ORIENTED_EDGE('',*,*,#23230,.T.);
#30702=ORIENTED_EDGE('',*,*,#23231,.T.);
#30703=ORIENTED_EDGE('',*,*,#23232,.F.);
#30704=ORIENTED_EDGE('',*,*,#23233,.T.);
#30705=ORIENTED_EDGE('',*,*,#23234,.T.);
#30706=ORIENTED_EDGE('',*,*,#23232,.T.);
#30707=ORIENTED_EDGE('',*,*,#23235,.T.);
#30708=ORIENTED_EDGE('',*,*,#23226,.F.);
#30709=ORIENTED_EDGE('',*,*,#23236,.T.);
#30710=ORIENTED_EDGE('',*,*,#21418,.F.);
#30711=ORIENTED_EDGE('',*,*,#23237,.T.);
#30712=ORIENTED_EDGE('',*,*,#23124,.T.);
#30713=ORIENTED_EDGE('',*,*,#23238,.F.);
#30714=ORIENTED_EDGE('',*,*,#23239,.T.);
#30715=ORIENTED_EDGE('',*,*,#23229,.F.);
#30716=ORIENTED_EDGE('',*,*,#23240,.T.);
#30717=ORIENTED_EDGE('',*,*,#23241,.T.);
#30718=ORIENTED_EDGE('',*,*,#23242,.T.);
#30719=ORIENTED_EDGE('',*,*,#23238,.T.);
#30720=ORIENTED_EDGE('',*,*,#23243,.T.);
#30721=ORIENTED_EDGE('',*,*,#23244,.T.);
#30722=ORIENTED_EDGE('',*,*,#23245,.T.);
#30723=ORIENTED_EDGE('',*,*,#23246,.T.);
#30724=ORIENTED_EDGE('',*,*,#23247,.F.);
#30725=ORIENTED_EDGE('',*,*,#23248,.T.);
#30726=ORIENTED_EDGE('',*,*,#23249,.T.);
#30727=ORIENTED_EDGE('',*,*,#23247,.T.);
#30728=ORIENTED_EDGE('',*,*,#23250,.T.);
#30729=ORIENTED_EDGE('',*,*,#23241,.F.);
#30730=ORIENTED_EDGE('',*,*,#23251,.T.);
#30731=ORIENTED_EDGE('',*,*,#23252,.F.);
#30732=ORIENTED_EDGE('',*,*,#23253,.T.);
#30733=ORIENTED_EDGE('',*,*,#23244,.F.);
#30734=ORIENTED_EDGE('',*,*,#23254,.T.);
#30735=ORIENTED_EDGE('',*,*,#23255,.T.);
#30736=ORIENTED_EDGE('',*,*,#23256,.T.);
#30737=ORIENTED_EDGE('',*,*,#23252,.T.);
#30738=ORIENTED_EDGE('',*,*,#23257,.T.);
#30739=ORIENTED_EDGE('',*,*,#23258,.T.);
#30740=ORIENTED_EDGE('',*,*,#23259,.T.);
#30741=ORIENTED_EDGE('',*,*,#23260,.T.);
#30742=ORIENTED_EDGE('',*,*,#23261,.F.);
#30743=ORIENTED_EDGE('',*,*,#23262,.T.);
#30744=ORIENTED_EDGE('',*,*,#23263,.T.);
#30745=ORIENTED_EDGE('',*,*,#23261,.T.);
#30746=ORIENTED_EDGE('',*,*,#23264,.T.);
#30747=ORIENTED_EDGE('',*,*,#23255,.F.);
#30748=ORIENTED_EDGE('',*,*,#23265,.T.);
#30749=ORIENTED_EDGE('',*,*,#23266,.F.);
#30750=ORIENTED_EDGE('',*,*,#23267,.T.);
#30751=ORIENTED_EDGE('',*,*,#23258,.F.);
#30752=ORIENTED_EDGE('',*,*,#23268,.T.);
#30753=ORIENTED_EDGE('',*,*,#23269,.T.);
#30754=ORIENTED_EDGE('',*,*,#23270,.T.);
#30755=ORIENTED_EDGE('',*,*,#23266,.T.);
#30756=ORIENTED_EDGE('',*,*,#23271,.T.);
#30757=ORIENTED_EDGE('',*,*,#23272,.T.);
#30758=ORIENTED_EDGE('',*,*,#23273,.T.);
#30759=ORIENTED_EDGE('',*,*,#23274,.T.);
#30760=ORIENTED_EDGE('',*,*,#23275,.F.);
#30761=ORIENTED_EDGE('',*,*,#23276,.T.);
#30762=ORIENTED_EDGE('',*,*,#23277,.T.);
#30763=ORIENTED_EDGE('',*,*,#23275,.T.);
#30764=ORIENTED_EDGE('',*,*,#23278,.T.);
#30765=ORIENTED_EDGE('',*,*,#23269,.F.);
#30766=ORIENTED_EDGE('',*,*,#23279,.T.);
#30767=ORIENTED_EDGE('',*,*,#23280,.F.);
#30768=ORIENTED_EDGE('',*,*,#23281,.T.);
#30769=ORIENTED_EDGE('',*,*,#23272,.F.);
#30770=ORIENTED_EDGE('',*,*,#23282,.T.);
#30771=ORIENTED_EDGE('',*,*,#23283,.T.);
#30772=ORIENTED_EDGE('',*,*,#23284,.T.);
#30773=ORIENTED_EDGE('',*,*,#23280,.T.);
#30774=ORIENTED_EDGE('',*,*,#23285,.T.);
#30775=ORIENTED_EDGE('',*,*,#23286,.T.);
#30776=ORIENTED_EDGE('',*,*,#23287,.T.);
#30777=ORIENTED_EDGE('',*,*,#23288,.T.);
#30778=ORIENTED_EDGE('',*,*,#23289,.F.);
#30779=ORIENTED_EDGE('',*,*,#23290,.T.);
#30780=ORIENTED_EDGE('',*,*,#23291,.T.);
#30781=ORIENTED_EDGE('',*,*,#23289,.T.);
#30782=ORIENTED_EDGE('',*,*,#23292,.T.);
#30783=ORIENTED_EDGE('',*,*,#23283,.F.);
#30784=ORIENTED_EDGE('',*,*,#23293,.T.);
#30785=ORIENTED_EDGE('',*,*,#23294,.F.);
#30786=ORIENTED_EDGE('',*,*,#23295,.T.);
#30787=ORIENTED_EDGE('',*,*,#23286,.F.);
#30788=ORIENTED_EDGE('',*,*,#23296,.T.);
#30789=ORIENTED_EDGE('',*,*,#23297,.T.);
#30790=ORIENTED_EDGE('',*,*,#23298,.T.);
#30791=ORIENTED_EDGE('',*,*,#23294,.T.);
#30792=ORIENTED_EDGE('',*,*,#23299,.T.);
#30793=ORIENTED_EDGE('',*,*,#23300,.T.);
#30794=ORIENTED_EDGE('',*,*,#23301,.T.);
#30795=ORIENTED_EDGE('',*,*,#23302,.T.);
#30796=ORIENTED_EDGE('',*,*,#23303,.F.);
#30797=ORIENTED_EDGE('',*,*,#23304,.T.);
#30798=ORIENTED_EDGE('',*,*,#23305,.T.);
#30799=ORIENTED_EDGE('',*,*,#23303,.T.);
#30800=ORIENTED_EDGE('',*,*,#23306,.T.);
#30801=ORIENTED_EDGE('',*,*,#23297,.F.);
#30802=ORIENTED_EDGE('',*,*,#23307,.T.);
#30803=ORIENTED_EDGE('',*,*,#21712,.F.);
#30804=ORIENTED_EDGE('',*,*,#23308,.T.);
#30805=ORIENTED_EDGE('',*,*,#23300,.F.);
#30806=ORIENTED_EDGE('',*,*,#23309,.T.);
#30807=ORIENTED_EDGE('',*,*,#21709,.F.);
#30808=ORIENTED_EDGE('',*,*,#23310,.T.);
#30809=ORIENTED_EDGE('',*,*,#23311,.T.);
#30810=ORIENTED_EDGE('',*,*,#23312,.F.);
#30811=ORIENTED_EDGE('',*,*,#23312,.T.);
#30812=ORIENTED_EDGE('',*,*,#23313,.T.);
#30813=ORIENTED_EDGE('',*,*,#21710,.F.);
#30814=ORIENTED_EDGE('',*,*,#23314,.T.);
#30815=ORIENTED_EDGE('',*,*,#23315,.T.);
#30816=ORIENTED_EDGE('',*,*,#21411,.F.);
#30817=ORIENTED_EDGE('',*,*,#23316,.F.);
#30818=ORIENTED_EDGE('',*,*,#23317,.T.);
#30819=ORIENTED_EDGE('',*,*,#23318,.T.);
#30820=ORIENTED_EDGE('',*,*,#23319,.F.);
#30821=ORIENTED_EDGE('',*,*,#23320,.T.);
#30822=ORIENTED_EDGE('',*,*,#23314,.F.);
#30823=ORIENTED_EDGE('',*,*,#23321,.T.);
#30824=ORIENTED_EDGE('',*,*,#23322,.T.);
#30825=ORIENTED_EDGE('',*,*,#23323,.T.);
#30826=ORIENTED_EDGE('',*,*,#23319,.T.);
#30827=ORIENTED_EDGE('',*,*,#23324,.T.);
#30828=ORIENTED_EDGE('',*,*,#23325,.T.);
#30829=ORIENTED_EDGE('',*,*,#23326,.T.);
#30830=ORIENTED_EDGE('',*,*,#23327,.T.);
#30831=ORIENTED_EDGE('',*,*,#23328,.F.);
#30832=ORIENTED_EDGE('',*,*,#23329,.T.);
#30833=ORIENTED_EDGE('',*,*,#23330,.T.);
#30834=ORIENTED_EDGE('',*,*,#23328,.T.);
#30835=ORIENTED_EDGE('',*,*,#23331,.T.);
#30836=ORIENTED_EDGE('',*,*,#23322,.F.);
#30837=ORIENTED_EDGE('',*,*,#23332,.T.);
#30838=ORIENTED_EDGE('',*,*,#21414,.F.);
#30839=ORIENTED_EDGE('',*,*,#23333,.T.);
#30840=ORIENTED_EDGE('',*,*,#23220,.T.);
#30841=ORIENTED_EDGE('',*,*,#23334,.F.);
#30842=ORIENTED_EDGE('',*,*,#23335,.T.);
#30843=ORIENTED_EDGE('',*,*,#23325,.F.);
#30844=ORIENTED_EDGE('',*,*,#23336,.T.);
#30845=ORIENTED_EDGE('',*,*,#23337,.T.);
#30846=ORIENTED_EDGE('',*,*,#23338,.T.);
#30847=ORIENTED_EDGE('',*,*,#23334,.T.);
#30848=ORIENTED_EDGE('',*,*,#23339,.T.);
#30849=ORIENTED_EDGE('',*,*,#23340,.T.);
#30850=ORIENTED_EDGE('',*,*,#23341,.T.);
#30851=ORIENTED_EDGE('',*,*,#23342,.T.);
#30852=ORIENTED_EDGE('',*,*,#23343,.F.);
#30853=ORIENTED_EDGE('',*,*,#23344,.T.);
#30854=ORIENTED_EDGE('',*,*,#23345,.T.);
#30855=ORIENTED_EDGE('',*,*,#23343,.T.);
#30856=ORIENTED_EDGE('',*,*,#23346,.T.);
#30857=ORIENTED_EDGE('',*,*,#23337,.F.);
#30858=ORIENTED_EDGE('',*,*,#23347,.T.);
#30859=ORIENTED_EDGE('',*,*,#23348,.F.);
#30860=ORIENTED_EDGE('',*,*,#23349,.T.);
#30861=ORIENTED_EDGE('',*,*,#23340,.F.);
#30862=ORIENTED_EDGE('',*,*,#23350,.T.);
#30863=ORIENTED_EDGE('',*,*,#23351,.T.);
#30864=ORIENTED_EDGE('',*,*,#23352,.T.);
#30865=ORIENTED_EDGE('',*,*,#23348,.T.);
#30866=ORIENTED_EDGE('',*,*,#23353,.T.);
#30867=ORIENTED_EDGE('',*,*,#23354,.T.);
#30868=ORIENTED_EDGE('',*,*,#23355,.T.);
#30869=ORIENTED_EDGE('',*,*,#23356,.T.);
#30870=ORIENTED_EDGE('',*,*,#23357,.F.);
#30871=ORIENTED_EDGE('',*,*,#23358,.T.);
#30872=ORIENTED_EDGE('',*,*,#23359,.T.);
#30873=ORIENTED_EDGE('',*,*,#23357,.T.);
#30874=ORIENTED_EDGE('',*,*,#23360,.T.);
#30875=ORIENTED_EDGE('',*,*,#23351,.F.);
#30876=ORIENTED_EDGE('',*,*,#23361,.T.);
#30877=ORIENTED_EDGE('',*,*,#23362,.F.);
#30878=ORIENTED_EDGE('',*,*,#23363,.T.);
#30879=ORIENTED_EDGE('',*,*,#23354,.F.);
#30880=ORIENTED_EDGE('',*,*,#23364,.T.);
#30881=ORIENTED_EDGE('',*,*,#23365,.T.);
#30882=ORIENTED_EDGE('',*,*,#23366,.T.);
#30883=ORIENTED_EDGE('',*,*,#23362,.T.);
#30884=ORIENTED_EDGE('',*,*,#23367,.T.);
#30885=ORIENTED_EDGE('',*,*,#23368,.T.);
#30886=ORIENTED_EDGE('',*,*,#23369,.T.);
#30887=ORIENTED_EDGE('',*,*,#23370,.T.);
#30888=ORIENTED_EDGE('',*,*,#23371,.F.);
#30889=ORIENTED_EDGE('',*,*,#23372,.T.);
#30890=ORIENTED_EDGE('',*,*,#23373,.T.);
#30891=ORIENTED_EDGE('',*,*,#23371,.T.);
#30892=ORIENTED_EDGE('',*,*,#23374,.T.);
#30893=ORIENTED_EDGE('',*,*,#23365,.F.);
#30894=ORIENTED_EDGE('',*,*,#23375,.T.);
#30895=ORIENTED_EDGE('',*,*,#23376,.F.);
#30896=ORIENTED_EDGE('',*,*,#23377,.T.);
#30897=ORIENTED_EDGE('',*,*,#23368,.F.);
#30898=ORIENTED_EDGE('',*,*,#23378,.T.);
#30899=ORIENTED_EDGE('',*,*,#23379,.T.);
#30900=ORIENTED_EDGE('',*,*,#23380,.T.);
#30901=ORIENTED_EDGE('',*,*,#23376,.T.);
#30902=ORIENTED_EDGE('',*,*,#23381,.T.);
#30903=ORIENTED_EDGE('',*,*,#23382,.T.);
#30904=ORIENTED_EDGE('',*,*,#23383,.T.);
#30905=ORIENTED_EDGE('',*,*,#23384,.T.);
#30906=ORIENTED_EDGE('',*,*,#23385,.F.);
#30907=ORIENTED_EDGE('',*,*,#23386,.T.);
#30908=ORIENTED_EDGE('',*,*,#23387,.T.);
#30909=ORIENTED_EDGE('',*,*,#23385,.T.);
#30910=ORIENTED_EDGE('',*,*,#23388,.T.);
#30911=ORIENTED_EDGE('',*,*,#23379,.F.);
#30912=ORIENTED_EDGE('',*,*,#23389,.T.);
#30913=ORIENTED_EDGE('',*,*,#23390,.F.);
#30914=ORIENTED_EDGE('',*,*,#23391,.T.);
#30915=ORIENTED_EDGE('',*,*,#23382,.F.);
#30916=ORIENTED_EDGE('',*,*,#23392,.T.);
#30917=ORIENTED_EDGE('',*,*,#23393,.T.);
#30918=ORIENTED_EDGE('',*,*,#23394,.T.);
#30919=ORIENTED_EDGE('',*,*,#23390,.T.);
#30920=ORIENTED_EDGE('',*,*,#23395,.T.);
#30921=ORIENTED_EDGE('',*,*,#23396,.T.);
#30922=ORIENTED_EDGE('',*,*,#23397,.T.);
#30923=ORIENTED_EDGE('',*,*,#23398,.T.);
#30924=ORIENTED_EDGE('',*,*,#23399,.F.);
#30925=ORIENTED_EDGE('',*,*,#23400,.T.);
#30926=ORIENTED_EDGE('',*,*,#23401,.T.);
#30927=ORIENTED_EDGE('',*,*,#23399,.T.);
#30928=ORIENTED_EDGE('',*,*,#23402,.T.);
#30929=ORIENTED_EDGE('',*,*,#23393,.F.);
#30930=ORIENTED_EDGE('',*,*,#23403,.T.);
#30931=ORIENTED_EDGE('',*,*,#21718,.F.);
#30932=ORIENTED_EDGE('',*,*,#23404,.T.);
#30933=ORIENTED_EDGE('',*,*,#23396,.F.);
#30934=ORIENTED_EDGE('',*,*,#23405,.T.);
#30935=ORIENTED_EDGE('',*,*,#21715,.F.);
#30936=ORIENTED_EDGE('',*,*,#23406,.T.);
#30937=ORIENTED_EDGE('',*,*,#23407,.T.);
#30938=ORIENTED_EDGE('',*,*,#23408,.F.);
#30939=ORIENTED_EDGE('',*,*,#23408,.T.);
#30940=ORIENTED_EDGE('',*,*,#23409,.T.);
#30941=ORIENTED_EDGE('',*,*,#21716,.F.);
#30942=ORIENTED_EDGE('',*,*,#23410,.T.);
#30943=ORIENTED_EDGE('',*,*,#23411,.T.);
#30944=ORIENTED_EDGE('',*,*,#21407,.F.);
#30945=ORIENTED_EDGE('',*,*,#23412,.F.);
#30946=ORIENTED_EDGE('',*,*,#23413,.T.);
#30947=ORIENTED_EDGE('',*,*,#23414,.T.);
#30948=ORIENTED_EDGE('',*,*,#23415,.F.);
#30949=ORIENTED_EDGE('',*,*,#23416,.T.);
#30950=ORIENTED_EDGE('',*,*,#23410,.F.);
#30951=ORIENTED_EDGE('',*,*,#23417,.T.);
#30952=ORIENTED_EDGE('',*,*,#23418,.T.);
#30953=ORIENTED_EDGE('',*,*,#23419,.T.);
#30954=ORIENTED_EDGE('',*,*,#23415,.T.);
#30955=ORIENTED_EDGE('',*,*,#23420,.T.);
#30956=ORIENTED_EDGE('',*,*,#23421,.T.);
#30957=ORIENTED_EDGE('',*,*,#23422,.T.);
#30958=ORIENTED_EDGE('',*,*,#23423,.T.);
#30959=ORIENTED_EDGE('',*,*,#23424,.F.);
#30960=ORIENTED_EDGE('',*,*,#23425,.T.);
#30961=ORIENTED_EDGE('',*,*,#23426,.T.);
#30962=ORIENTED_EDGE('',*,*,#23424,.T.);
#30963=ORIENTED_EDGE('',*,*,#23427,.T.);
#30964=ORIENTED_EDGE('',*,*,#23418,.F.);
#30965=ORIENTED_EDGE('',*,*,#23428,.T.);
#30966=ORIENTED_EDGE('',*,*,#21410,.F.);
#30967=ORIENTED_EDGE('',*,*,#23429,.T.);
#30968=ORIENTED_EDGE('',*,*,#23316,.T.);
#30969=ORIENTED_EDGE('',*,*,#23430,.F.);
#30970=ORIENTED_EDGE('',*,*,#23431,.T.);
#30971=ORIENTED_EDGE('',*,*,#23421,.F.);
#30972=ORIENTED_EDGE('',*,*,#23432,.T.);
#30973=ORIENTED_EDGE('',*,*,#23433,.T.);
#30974=ORIENTED_EDGE('',*,*,#23434,.T.);
#30975=ORIENTED_EDGE('',*,*,#23430,.T.);
#30976=ORIENTED_EDGE('',*,*,#23435,.T.);
#30977=ORIENTED_EDGE('',*,*,#23436,.T.);
#30978=ORIENTED_EDGE('',*,*,#23437,.T.);
#30979=ORIENTED_EDGE('',*,*,#23438,.T.);
#30980=ORIENTED_EDGE('',*,*,#23439,.F.);
#30981=ORIENTED_EDGE('',*,*,#23440,.T.);
#30982=ORIENTED_EDGE('',*,*,#23441,.T.);
#30983=ORIENTED_EDGE('',*,*,#23439,.T.);
#30984=ORIENTED_EDGE('',*,*,#23442,.T.);
#30985=ORIENTED_EDGE('',*,*,#23433,.F.);
#30986=ORIENTED_EDGE('',*,*,#23443,.T.);
#30987=ORIENTED_EDGE('',*,*,#23444,.F.);
#30988=ORIENTED_EDGE('',*,*,#23445,.T.);
#30989=ORIENTED_EDGE('',*,*,#23436,.F.);
#30990=ORIENTED_EDGE('',*,*,#23446,.T.);
#30991=ORIENTED_EDGE('',*,*,#23447,.T.);
#30992=ORIENTED_EDGE('',*,*,#23448,.T.);
#30993=ORIENTED_EDGE('',*,*,#23444,.T.);
#30994=ORIENTED_EDGE('',*,*,#23449,.T.);
#30995=ORIENTED_EDGE('',*,*,#23450,.T.);
#30996=ORIENTED_EDGE('',*,*,#23451,.T.);
#30997=ORIENTED_EDGE('',*,*,#23452,.T.);
#30998=ORIENTED_EDGE('',*,*,#23453,.F.);
#30999=ORIENTED_EDGE('',*,*,#23454,.T.);
#31000=ORIENTED_EDGE('',*,*,#23455,.T.);
#31001=ORIENTED_EDGE('',*,*,#23453,.T.);
#31002=ORIENTED_EDGE('',*,*,#23456,.T.);
#31003=ORIENTED_EDGE('',*,*,#23447,.F.);
#31004=ORIENTED_EDGE('',*,*,#23457,.T.);
#31005=ORIENTED_EDGE('',*,*,#23458,.F.);
#31006=ORIENTED_EDGE('',*,*,#23459,.T.);
#31007=ORIENTED_EDGE('',*,*,#23450,.F.);
#31008=ORIENTED_EDGE('',*,*,#23460,.T.);
#31009=ORIENTED_EDGE('',*,*,#23461,.T.);
#31010=ORIENTED_EDGE('',*,*,#23462,.T.);
#31011=ORIENTED_EDGE('',*,*,#23458,.T.);
#31012=ORIENTED_EDGE('',*,*,#23463,.T.);
#31013=ORIENTED_EDGE('',*,*,#23464,.T.);
#31014=ORIENTED_EDGE('',*,*,#23465,.T.);
#31015=ORIENTED_EDGE('',*,*,#23466,.T.);
#31016=ORIENTED_EDGE('',*,*,#23467,.F.);
#31017=ORIENTED_EDGE('',*,*,#23468,.T.);
#31018=ORIENTED_EDGE('',*,*,#23469,.T.);
#31019=ORIENTED_EDGE('',*,*,#23467,.T.);
#31020=ORIENTED_EDGE('',*,*,#23470,.T.);
#31021=ORIENTED_EDGE('',*,*,#23461,.F.);
#31022=ORIENTED_EDGE('',*,*,#23471,.T.);
#31023=ORIENTED_EDGE('',*,*,#23472,.F.);
#31024=ORIENTED_EDGE('',*,*,#23473,.T.);
#31025=ORIENTED_EDGE('',*,*,#23464,.F.);
#31026=ORIENTED_EDGE('',*,*,#23474,.T.);
#31027=ORIENTED_EDGE('',*,*,#23475,.T.);
#31028=ORIENTED_EDGE('',*,*,#23476,.T.);
#31029=ORIENTED_EDGE('',*,*,#23472,.T.);
#31030=ORIENTED_EDGE('',*,*,#23477,.T.);
#31031=ORIENTED_EDGE('',*,*,#23478,.T.);
#31032=ORIENTED_EDGE('',*,*,#23479,.T.);
#31033=ORIENTED_EDGE('',*,*,#23480,.T.);
#31034=ORIENTED_EDGE('',*,*,#23481,.F.);
#31035=ORIENTED_EDGE('',*,*,#23482,.T.);
#31036=ORIENTED_EDGE('',*,*,#23483,.T.);
#31037=ORIENTED_EDGE('',*,*,#23481,.T.);
#31038=ORIENTED_EDGE('',*,*,#23484,.T.);
#31039=ORIENTED_EDGE('',*,*,#23475,.F.);
#31040=ORIENTED_EDGE('',*,*,#23485,.T.);
#31041=ORIENTED_EDGE('',*,*,#23486,.F.);
#31042=ORIENTED_EDGE('',*,*,#23487,.T.);
#31043=ORIENTED_EDGE('',*,*,#23478,.F.);
#31044=ORIENTED_EDGE('',*,*,#23488,.T.);
#31045=ORIENTED_EDGE('',*,*,#23489,.T.);
#31046=ORIENTED_EDGE('',*,*,#23490,.T.);
#31047=ORIENTED_EDGE('',*,*,#23486,.T.);
#31048=ORIENTED_EDGE('',*,*,#23491,.T.);
#31049=ORIENTED_EDGE('',*,*,#23492,.T.);
#31050=ORIENTED_EDGE('',*,*,#23493,.T.);
#31051=ORIENTED_EDGE('',*,*,#23494,.T.);
#31052=ORIENTED_EDGE('',*,*,#23495,.F.);
#31053=ORIENTED_EDGE('',*,*,#23496,.T.);
#31054=ORIENTED_EDGE('',*,*,#23497,.T.);
#31055=ORIENTED_EDGE('',*,*,#23495,.T.);
#31056=ORIENTED_EDGE('',*,*,#23498,.T.);
#31057=ORIENTED_EDGE('',*,*,#23489,.F.);
#31058=ORIENTED_EDGE('',*,*,#23499,.T.);
#31059=ORIENTED_EDGE('',*,*,#21724,.F.);
#31060=ORIENTED_EDGE('',*,*,#23500,.T.);
#31061=ORIENTED_EDGE('',*,*,#23492,.F.);
#31062=ORIENTED_EDGE('',*,*,#23501,.T.);
#31063=ORIENTED_EDGE('',*,*,#21721,.F.);
#31064=ORIENTED_EDGE('',*,*,#23502,.T.);
#31065=ORIENTED_EDGE('',*,*,#23503,.T.);
#31066=ORIENTED_EDGE('',*,*,#23504,.F.);
#31067=ORIENTED_EDGE('',*,*,#23504,.T.);
#31068=ORIENTED_EDGE('',*,*,#23505,.T.);
#31069=ORIENTED_EDGE('',*,*,#21722,.F.);
#31070=ORIENTED_EDGE('',*,*,#23506,.T.);
#31071=ORIENTED_EDGE('',*,*,#23507,.T.);
#31072=ORIENTED_EDGE('',*,*,#21403,.F.);
#31073=ORIENTED_EDGE('',*,*,#23508,.F.);
#31074=ORIENTED_EDGE('',*,*,#23509,.T.);
#31075=ORIENTED_EDGE('',*,*,#23510,.T.);
#31076=ORIENTED_EDGE('',*,*,#23511,.F.);
#31077=ORIENTED_EDGE('',*,*,#23512,.T.);
#31078=ORIENTED_EDGE('',*,*,#23506,.F.);
#31079=ORIENTED_EDGE('',*,*,#23513,.T.);
#31080=ORIENTED_EDGE('',*,*,#23514,.T.);
#31081=ORIENTED_EDGE('',*,*,#23515,.T.);
#31082=ORIENTED_EDGE('',*,*,#23511,.T.);
#31083=ORIENTED_EDGE('',*,*,#23516,.T.);
#31084=ORIENTED_EDGE('',*,*,#23517,.T.);
#31085=ORIENTED_EDGE('',*,*,#23518,.T.);
#31086=ORIENTED_EDGE('',*,*,#23519,.T.);
#31087=ORIENTED_EDGE('',*,*,#23520,.F.);
#31088=ORIENTED_EDGE('',*,*,#23521,.T.);
#31089=ORIENTED_EDGE('',*,*,#23522,.T.);
#31090=ORIENTED_EDGE('',*,*,#23520,.T.);
#31091=ORIENTED_EDGE('',*,*,#23523,.T.);
#31092=ORIENTED_EDGE('',*,*,#23514,.F.);
#31093=ORIENTED_EDGE('',*,*,#23524,.T.);
#31094=ORIENTED_EDGE('',*,*,#21406,.F.);
#31095=ORIENTED_EDGE('',*,*,#23525,.T.);
#31096=ORIENTED_EDGE('',*,*,#23412,.T.);
#31097=ORIENTED_EDGE('',*,*,#23526,.F.);
#31098=ORIENTED_EDGE('',*,*,#23527,.T.);
#31099=ORIENTED_EDGE('',*,*,#23517,.F.);
#31100=ORIENTED_EDGE('',*,*,#23528,.T.);
#31101=ORIENTED_EDGE('',*,*,#23529,.T.);
#31102=ORIENTED_EDGE('',*,*,#23530,.T.);
#31103=ORIENTED_EDGE('',*,*,#23526,.T.);
#31104=ORIENTED_EDGE('',*,*,#23531,.T.);
#31105=ORIENTED_EDGE('',*,*,#23532,.T.);
#31106=ORIENTED_EDGE('',*,*,#23533,.T.);
#31107=ORIENTED_EDGE('',*,*,#23534,.T.);
#31108=ORIENTED_EDGE('',*,*,#23535,.F.);
#31109=ORIENTED_EDGE('',*,*,#23536,.T.);
#31110=ORIENTED_EDGE('',*,*,#23537,.T.);
#31111=ORIENTED_EDGE('',*,*,#23535,.T.);
#31112=ORIENTED_EDGE('',*,*,#23538,.T.);
#31113=ORIENTED_EDGE('',*,*,#23529,.F.);
#31114=ORIENTED_EDGE('',*,*,#23539,.T.);
#31115=ORIENTED_EDGE('',*,*,#23540,.F.);
#31116=ORIENTED_EDGE('',*,*,#23541,.T.);
#31117=ORIENTED_EDGE('',*,*,#23532,.F.);
#31118=ORIENTED_EDGE('',*,*,#23542,.T.);
#31119=ORIENTED_EDGE('',*,*,#23543,.T.);
#31120=ORIENTED_EDGE('',*,*,#23544,.T.);
#31121=ORIENTED_EDGE('',*,*,#23540,.T.);
#31122=ORIENTED_EDGE('',*,*,#23545,.T.);
#31123=ORIENTED_EDGE('',*,*,#23546,.T.);
#31124=ORIENTED_EDGE('',*,*,#23547,.T.);
#31125=ORIENTED_EDGE('',*,*,#23548,.T.);
#31126=ORIENTED_EDGE('',*,*,#23549,.F.);
#31127=ORIENTED_EDGE('',*,*,#23550,.T.);
#31128=ORIENTED_EDGE('',*,*,#23551,.T.);
#31129=ORIENTED_EDGE('',*,*,#23549,.T.);
#31130=ORIENTED_EDGE('',*,*,#23552,.T.);
#31131=ORIENTED_EDGE('',*,*,#23543,.F.);
#31132=ORIENTED_EDGE('',*,*,#23553,.T.);
#31133=ORIENTED_EDGE('',*,*,#23554,.F.);
#31134=ORIENTED_EDGE('',*,*,#23555,.T.);
#31135=ORIENTED_EDGE('',*,*,#23546,.F.);
#31136=ORIENTED_EDGE('',*,*,#23556,.T.);
#31137=ORIENTED_EDGE('',*,*,#23557,.T.);
#31138=ORIENTED_EDGE('',*,*,#23558,.T.);
#31139=ORIENTED_EDGE('',*,*,#23554,.T.);
#31140=ORIENTED_EDGE('',*,*,#23559,.T.);
#31141=ORIENTED_EDGE('',*,*,#23560,.T.);
#31142=ORIENTED_EDGE('',*,*,#23561,.T.);
#31143=ORIENTED_EDGE('',*,*,#23562,.T.);
#31144=ORIENTED_EDGE('',*,*,#23563,.F.);
#31145=ORIENTED_EDGE('',*,*,#23564,.T.);
#31146=ORIENTED_EDGE('',*,*,#23565,.T.);
#31147=ORIENTED_EDGE('',*,*,#23563,.T.);
#31148=ORIENTED_EDGE('',*,*,#23566,.T.);
#31149=ORIENTED_EDGE('',*,*,#23557,.F.);
#31150=ORIENTED_EDGE('',*,*,#23567,.T.);
#31151=ORIENTED_EDGE('',*,*,#23568,.F.);
#31152=ORIENTED_EDGE('',*,*,#23569,.T.);
#31153=ORIENTED_EDGE('',*,*,#23560,.F.);
#31154=ORIENTED_EDGE('',*,*,#23570,.T.);
#31155=ORIENTED_EDGE('',*,*,#23571,.T.);
#31156=ORIENTED_EDGE('',*,*,#23572,.T.);
#31157=ORIENTED_EDGE('',*,*,#23568,.T.);
#31158=ORIENTED_EDGE('',*,*,#23573,.T.);
#31159=ORIENTED_EDGE('',*,*,#23574,.T.);
#31160=ORIENTED_EDGE('',*,*,#23575,.T.);
#31161=ORIENTED_EDGE('',*,*,#23576,.T.);
#31162=ORIENTED_EDGE('',*,*,#23577,.F.);
#31163=ORIENTED_EDGE('',*,*,#23578,.T.);
#31164=ORIENTED_EDGE('',*,*,#23579,.T.);
#31165=ORIENTED_EDGE('',*,*,#23577,.T.);
#31166=ORIENTED_EDGE('',*,*,#23580,.T.);
#31167=ORIENTED_EDGE('',*,*,#23571,.F.);
#31168=ORIENTED_EDGE('',*,*,#23581,.T.);
#31169=ORIENTED_EDGE('',*,*,#23582,.F.);
#31170=ORIENTED_EDGE('',*,*,#23583,.T.);
#31171=ORIENTED_EDGE('',*,*,#23574,.F.);
#31172=ORIENTED_EDGE('',*,*,#23584,.T.);
#31173=ORIENTED_EDGE('',*,*,#23585,.T.);
#31174=ORIENTED_EDGE('',*,*,#23586,.T.);
#31175=ORIENTED_EDGE('',*,*,#23582,.T.);
#31176=ORIENTED_EDGE('',*,*,#23587,.T.);
#31177=ORIENTED_EDGE('',*,*,#23588,.T.);
#31178=ORIENTED_EDGE('',*,*,#23589,.T.);
#31179=ORIENTED_EDGE('',*,*,#23590,.T.);
#31180=ORIENTED_EDGE('',*,*,#23591,.F.);
#31181=ORIENTED_EDGE('',*,*,#23592,.T.);
#31182=ORIENTED_EDGE('',*,*,#23593,.T.);
#31183=ORIENTED_EDGE('',*,*,#23591,.T.);
#31184=ORIENTED_EDGE('',*,*,#23594,.T.);
#31185=ORIENTED_EDGE('',*,*,#23585,.F.);
#31186=ORIENTED_EDGE('',*,*,#23595,.T.);
#31187=ORIENTED_EDGE('',*,*,#21730,.F.);
#31188=ORIENTED_EDGE('',*,*,#23596,.T.);
#31189=ORIENTED_EDGE('',*,*,#23588,.F.);
#31190=ORIENTED_EDGE('',*,*,#23597,.T.);
#31191=ORIENTED_EDGE('',*,*,#21727,.F.);
#31192=ORIENTED_EDGE('',*,*,#23598,.T.);
#31193=ORIENTED_EDGE('',*,*,#23599,.T.);
#31194=ORIENTED_EDGE('',*,*,#23600,.F.);
#31195=ORIENTED_EDGE('',*,*,#23600,.T.);
#31196=ORIENTED_EDGE('',*,*,#23601,.T.);
#31197=ORIENTED_EDGE('',*,*,#21728,.F.);
#31198=ORIENTED_EDGE('',*,*,#23602,.T.);
#31199=ORIENTED_EDGE('',*,*,#23603,.T.);
#31200=ORIENTED_EDGE('',*,*,#21399,.F.);
#31201=ORIENTED_EDGE('',*,*,#23604,.F.);
#31202=ORIENTED_EDGE('',*,*,#23605,.T.);
#31203=ORIENTED_EDGE('',*,*,#23606,.T.);
#31204=ORIENTED_EDGE('',*,*,#23607,.F.);
#31205=ORIENTED_EDGE('',*,*,#23608,.T.);
#31206=ORIENTED_EDGE('',*,*,#23602,.F.);
#31207=ORIENTED_EDGE('',*,*,#23609,.T.);
#31208=ORIENTED_EDGE('',*,*,#23610,.T.);
#31209=ORIENTED_EDGE('',*,*,#23611,.T.);
#31210=ORIENTED_EDGE('',*,*,#23607,.T.);
#31211=ORIENTED_EDGE('',*,*,#23612,.T.);
#31212=ORIENTED_EDGE('',*,*,#23613,.T.);
#31213=ORIENTED_EDGE('',*,*,#23614,.T.);
#31214=ORIENTED_EDGE('',*,*,#23615,.T.);
#31215=ORIENTED_EDGE('',*,*,#23616,.F.);
#31216=ORIENTED_EDGE('',*,*,#23617,.T.);
#31217=ORIENTED_EDGE('',*,*,#23618,.T.);
#31218=ORIENTED_EDGE('',*,*,#23616,.T.);
#31219=ORIENTED_EDGE('',*,*,#23619,.T.);
#31220=ORIENTED_EDGE('',*,*,#23610,.F.);
#31221=ORIENTED_EDGE('',*,*,#23620,.T.);
#31222=ORIENTED_EDGE('',*,*,#21402,.F.);
#31223=ORIENTED_EDGE('',*,*,#23621,.T.);
#31224=ORIENTED_EDGE('',*,*,#23508,.T.);
#31225=ORIENTED_EDGE('',*,*,#23622,.F.);
#31226=ORIENTED_EDGE('',*,*,#23623,.T.);
#31227=ORIENTED_EDGE('',*,*,#23613,.F.);
#31228=ORIENTED_EDGE('',*,*,#23624,.T.);
#31229=ORIENTED_EDGE('',*,*,#23625,.T.);
#31230=ORIENTED_EDGE('',*,*,#23626,.T.);
#31231=ORIENTED_EDGE('',*,*,#23622,.T.);
#31232=ORIENTED_EDGE('',*,*,#23627,.T.);
#31233=ORIENTED_EDGE('',*,*,#23628,.T.);
#31234=ORIENTED_EDGE('',*,*,#23629,.T.);
#31235=ORIENTED_EDGE('',*,*,#23630,.T.);
#31236=ORIENTED_EDGE('',*,*,#23631,.F.);
#31237=ORIENTED_EDGE('',*,*,#23632,.T.);
#31238=ORIENTED_EDGE('',*,*,#23633,.T.);
#31239=ORIENTED_EDGE('',*,*,#23631,.T.);
#31240=ORIENTED_EDGE('',*,*,#23634,.T.);
#31241=ORIENTED_EDGE('',*,*,#23625,.F.);
#31242=ORIENTED_EDGE('',*,*,#23635,.T.);
#31243=ORIENTED_EDGE('',*,*,#23636,.F.);
#31244=ORIENTED_EDGE('',*,*,#23637,.T.);
#31245=ORIENTED_EDGE('',*,*,#23628,.F.);
#31246=ORIENTED_EDGE('',*,*,#23638,.T.);
#31247=ORIENTED_EDGE('',*,*,#23639,.T.);
#31248=ORIENTED_EDGE('',*,*,#23640,.T.);
#31249=ORIENTED_EDGE('',*,*,#23636,.T.);
#31250=ORIENTED_EDGE('',*,*,#23641,.T.);
#31251=ORIENTED_EDGE('',*,*,#23642,.T.);
#31252=ORIENTED_EDGE('',*,*,#23643,.T.);
#31253=ORIENTED_EDGE('',*,*,#23644,.T.);
#31254=ORIENTED_EDGE('',*,*,#23645,.F.);
#31255=ORIENTED_EDGE('',*,*,#23646,.T.);
#31256=ORIENTED_EDGE('',*,*,#23647,.T.);
#31257=ORIENTED_EDGE('',*,*,#23645,.T.);
#31258=ORIENTED_EDGE('',*,*,#23648,.T.);
#31259=ORIENTED_EDGE('',*,*,#23639,.F.);
#31260=ORIENTED_EDGE('',*,*,#23649,.T.);
#31261=ORIENTED_EDGE('',*,*,#23650,.F.);
#31262=ORIENTED_EDGE('',*,*,#23651,.T.);
#31263=ORIENTED_EDGE('',*,*,#23642,.F.);
#31264=ORIENTED_EDGE('',*,*,#23652,.T.);
#31265=ORIENTED_EDGE('',*,*,#23653,.T.);
#31266=ORIENTED_EDGE('',*,*,#23654,.T.);
#31267=ORIENTED_EDGE('',*,*,#23650,.T.);
#31268=ORIENTED_EDGE('',*,*,#23655,.T.);
#31269=ORIENTED_EDGE('',*,*,#23656,.T.);
#31270=ORIENTED_EDGE('',*,*,#23657,.T.);
#31271=ORIENTED_EDGE('',*,*,#23658,.T.);
#31272=ORIENTED_EDGE('',*,*,#23659,.F.);
#31273=ORIENTED_EDGE('',*,*,#23660,.T.);
#31274=ORIENTED_EDGE('',*,*,#23661,.T.);
#31275=ORIENTED_EDGE('',*,*,#23659,.T.);
#31276=ORIENTED_EDGE('',*,*,#23662,.T.);
#31277=ORIENTED_EDGE('',*,*,#23653,.F.);
#31278=ORIENTED_EDGE('',*,*,#23663,.T.);
#31279=ORIENTED_EDGE('',*,*,#23664,.F.);
#31280=ORIENTED_EDGE('',*,*,#23665,.T.);
#31281=ORIENTED_EDGE('',*,*,#23656,.F.);
#31282=ORIENTED_EDGE('',*,*,#23666,.T.);
#31283=ORIENTED_EDGE('',*,*,#23667,.T.);
#31284=ORIENTED_EDGE('',*,*,#23668,.T.);
#31285=ORIENTED_EDGE('',*,*,#23664,.T.);
#31286=ORIENTED_EDGE('',*,*,#23669,.T.);
#31287=ORIENTED_EDGE('',*,*,#23670,.T.);
#31288=ORIENTED_EDGE('',*,*,#23671,.T.);
#31289=ORIENTED_EDGE('',*,*,#23672,.T.);
#31290=ORIENTED_EDGE('',*,*,#23673,.F.);
#31291=ORIENTED_EDGE('',*,*,#23674,.T.);
#31292=ORIENTED_EDGE('',*,*,#23675,.T.);
#31293=ORIENTED_EDGE('',*,*,#23673,.T.);
#31294=ORIENTED_EDGE('',*,*,#23676,.T.);
#31295=ORIENTED_EDGE('',*,*,#23667,.F.);
#31296=ORIENTED_EDGE('',*,*,#23677,.T.);
#31297=ORIENTED_EDGE('',*,*,#23678,.F.);
#31298=ORIENTED_EDGE('',*,*,#23679,.T.);
#31299=ORIENTED_EDGE('',*,*,#23670,.F.);
#31300=ORIENTED_EDGE('',*,*,#23680,.T.);
#31301=ORIENTED_EDGE('',*,*,#23681,.T.);
#31302=ORIENTED_EDGE('',*,*,#23682,.T.);
#31303=ORIENTED_EDGE('',*,*,#23678,.T.);
#31304=ORIENTED_EDGE('',*,*,#23683,.T.);
#31305=ORIENTED_EDGE('',*,*,#23684,.T.);
#31306=ORIENTED_EDGE('',*,*,#23685,.T.);
#31307=ORIENTED_EDGE('',*,*,#23686,.T.);
#31308=ORIENTED_EDGE('',*,*,#23687,.F.);
#31309=ORIENTED_EDGE('',*,*,#23688,.T.);
#31310=ORIENTED_EDGE('',*,*,#23689,.T.);
#31311=ORIENTED_EDGE('',*,*,#23687,.T.);
#31312=ORIENTED_EDGE('',*,*,#23690,.T.);
#31313=ORIENTED_EDGE('',*,*,#23681,.F.);
#31314=ORIENTED_EDGE('',*,*,#23691,.T.);
#31315=ORIENTED_EDGE('',*,*,#21736,.F.);
#31316=ORIENTED_EDGE('',*,*,#23692,.T.);
#31317=ORIENTED_EDGE('',*,*,#23684,.F.);
#31318=ORIENTED_EDGE('',*,*,#23693,.T.);
#31319=ORIENTED_EDGE('',*,*,#21733,.F.);
#31320=ORIENTED_EDGE('',*,*,#23694,.T.);
#31321=ORIENTED_EDGE('',*,*,#23695,.T.);
#31322=ORIENTED_EDGE('',*,*,#23696,.F.);
#31323=ORIENTED_EDGE('',*,*,#23696,.T.);
#31324=ORIENTED_EDGE('',*,*,#23697,.T.);
#31325=ORIENTED_EDGE('',*,*,#21734,.F.);
#31326=ORIENTED_EDGE('',*,*,#23698,.T.);
#31327=ORIENTED_EDGE('',*,*,#23699,.T.);
#31328=ORIENTED_EDGE('',*,*,#21395,.F.);
#31329=ORIENTED_EDGE('',*,*,#23700,.F.);
#31330=ORIENTED_EDGE('',*,*,#23701,.T.);
#31331=ORIENTED_EDGE('',*,*,#23702,.T.);
#31332=ORIENTED_EDGE('',*,*,#23703,.F.);
#31333=ORIENTED_EDGE('',*,*,#23704,.T.);
#31334=ORIENTED_EDGE('',*,*,#23698,.F.);
#31335=ORIENTED_EDGE('',*,*,#23705,.T.);
#31336=ORIENTED_EDGE('',*,*,#23706,.T.);
#31337=ORIENTED_EDGE('',*,*,#23707,.T.);
#31338=ORIENTED_EDGE('',*,*,#23703,.T.);
#31339=ORIENTED_EDGE('',*,*,#23708,.T.);
#31340=ORIENTED_EDGE('',*,*,#23709,.T.);
#31341=ORIENTED_EDGE('',*,*,#23710,.T.);
#31342=ORIENTED_EDGE('',*,*,#23711,.T.);
#31343=ORIENTED_EDGE('',*,*,#23712,.F.);
#31344=ORIENTED_EDGE('',*,*,#23713,.T.);
#31345=ORIENTED_EDGE('',*,*,#23714,.T.);
#31346=ORIENTED_EDGE('',*,*,#23712,.T.);
#31347=ORIENTED_EDGE('',*,*,#23715,.T.);
#31348=ORIENTED_EDGE('',*,*,#23706,.F.);
#31349=ORIENTED_EDGE('',*,*,#23716,.T.);
#31350=ORIENTED_EDGE('',*,*,#21398,.F.);
#31351=ORIENTED_EDGE('',*,*,#23717,.T.);
#31352=ORIENTED_EDGE('',*,*,#23604,.T.);
#31353=ORIENTED_EDGE('',*,*,#23718,.F.);
#31354=ORIENTED_EDGE('',*,*,#23719,.T.);
#31355=ORIENTED_EDGE('',*,*,#23709,.F.);
#31356=ORIENTED_EDGE('',*,*,#23720,.T.);
#31357=ORIENTED_EDGE('',*,*,#23721,.T.);
#31358=ORIENTED_EDGE('',*,*,#23722,.T.);
#31359=ORIENTED_EDGE('',*,*,#23718,.T.);
#31360=ORIENTED_EDGE('',*,*,#23723,.T.);
#31361=ORIENTED_EDGE('',*,*,#23724,.T.);
#31362=ORIENTED_EDGE('',*,*,#23725,.T.);
#31363=ORIENTED_EDGE('',*,*,#23726,.T.);
#31364=ORIENTED_EDGE('',*,*,#23727,.F.);
#31365=ORIENTED_EDGE('',*,*,#23728,.T.);
#31366=ORIENTED_EDGE('',*,*,#23729,.T.);
#31367=ORIENTED_EDGE('',*,*,#23727,.T.);
#31368=ORIENTED_EDGE('',*,*,#23730,.T.);
#31369=ORIENTED_EDGE('',*,*,#23721,.F.);
#31370=ORIENTED_EDGE('',*,*,#23731,.T.);
#31371=ORIENTED_EDGE('',*,*,#23732,.F.);
#31372=ORIENTED_EDGE('',*,*,#23733,.T.);
#31373=ORIENTED_EDGE('',*,*,#23724,.F.);
#31374=ORIENTED_EDGE('',*,*,#23734,.T.);
#31375=ORIENTED_EDGE('',*,*,#23735,.T.);
#31376=ORIENTED_EDGE('',*,*,#23736,.T.);
#31377=ORIENTED_EDGE('',*,*,#23732,.T.);
#31378=ORIENTED_EDGE('',*,*,#23737,.T.);
#31379=ORIENTED_EDGE('',*,*,#23738,.T.);
#31380=ORIENTED_EDGE('',*,*,#23739,.T.);
#31381=ORIENTED_EDGE('',*,*,#23740,.T.);
#31382=ORIENTED_EDGE('',*,*,#23741,.F.);
#31383=ORIENTED_EDGE('',*,*,#23742,.T.);
#31384=ORIENTED_EDGE('',*,*,#23743,.T.);
#31385=ORIENTED_EDGE('',*,*,#23741,.T.);
#31386=ORIENTED_EDGE('',*,*,#23744,.T.);
#31387=ORIENTED_EDGE('',*,*,#23735,.F.);
#31388=ORIENTED_EDGE('',*,*,#23745,.T.);
#31389=ORIENTED_EDGE('',*,*,#23746,.F.);
#31390=ORIENTED_EDGE('',*,*,#23747,.T.);
#31391=ORIENTED_EDGE('',*,*,#23738,.F.);
#31392=ORIENTED_EDGE('',*,*,#23748,.T.);
#31393=ORIENTED_EDGE('',*,*,#23749,.T.);
#31394=ORIENTED_EDGE('',*,*,#23750,.T.);
#31395=ORIENTED_EDGE('',*,*,#23746,.T.);
#31396=ORIENTED_EDGE('',*,*,#23751,.T.);
#31397=ORIENTED_EDGE('',*,*,#23752,.T.);
#31398=ORIENTED_EDGE('',*,*,#23753,.T.);
#31399=ORIENTED_EDGE('',*,*,#23754,.T.);
#31400=ORIENTED_EDGE('',*,*,#23755,.F.);
#31401=ORIENTED_EDGE('',*,*,#23756,.T.);
#31402=ORIENTED_EDGE('',*,*,#23757,.T.);
#31403=ORIENTED_EDGE('',*,*,#23755,.T.);
#31404=ORIENTED_EDGE('',*,*,#23758,.T.);
#31405=ORIENTED_EDGE('',*,*,#23749,.F.);
#31406=ORIENTED_EDGE('',*,*,#23759,.T.);
#31407=ORIENTED_EDGE('',*,*,#23760,.F.);
#31408=ORIENTED_EDGE('',*,*,#23761,.T.);
#31409=ORIENTED_EDGE('',*,*,#23752,.F.);
#31410=ORIENTED_EDGE('',*,*,#23762,.T.);
#31411=ORIENTED_EDGE('',*,*,#23763,.T.);
#31412=ORIENTED_EDGE('',*,*,#23764,.T.);
#31413=ORIENTED_EDGE('',*,*,#23760,.T.);
#31414=ORIENTED_EDGE('',*,*,#23765,.T.);
#31415=ORIENTED_EDGE('',*,*,#23766,.T.);
#31416=ORIENTED_EDGE('',*,*,#23767,.T.);
#31417=ORIENTED_EDGE('',*,*,#23768,.T.);
#31418=ORIENTED_EDGE('',*,*,#23769,.F.);
#31419=ORIENTED_EDGE('',*,*,#23770,.T.);
#31420=ORIENTED_EDGE('',*,*,#23771,.T.);
#31421=ORIENTED_EDGE('',*,*,#23769,.T.);
#31422=ORIENTED_EDGE('',*,*,#23772,.T.);
#31423=ORIENTED_EDGE('',*,*,#23763,.F.);
#31424=ORIENTED_EDGE('',*,*,#23773,.T.);
#31425=ORIENTED_EDGE('',*,*,#23774,.F.);
#31426=ORIENTED_EDGE('',*,*,#23775,.T.);
#31427=ORIENTED_EDGE('',*,*,#23766,.F.);
#31428=ORIENTED_EDGE('',*,*,#23776,.T.);
#31429=ORIENTED_EDGE('',*,*,#23777,.T.);
#31430=ORIENTED_EDGE('',*,*,#23778,.T.);
#31431=ORIENTED_EDGE('',*,*,#23774,.T.);
#31432=ORIENTED_EDGE('',*,*,#23779,.T.);
#31433=ORIENTED_EDGE('',*,*,#23780,.T.);
#31434=ORIENTED_EDGE('',*,*,#23781,.T.);
#31435=ORIENTED_EDGE('',*,*,#23782,.T.);
#31436=ORIENTED_EDGE('',*,*,#23783,.F.);
#31437=ORIENTED_EDGE('',*,*,#23784,.T.);
#31438=ORIENTED_EDGE('',*,*,#23785,.T.);
#31439=ORIENTED_EDGE('',*,*,#23783,.T.);
#31440=ORIENTED_EDGE('',*,*,#23786,.T.);
#31441=ORIENTED_EDGE('',*,*,#23777,.F.);
#31442=ORIENTED_EDGE('',*,*,#23787,.T.);
#31443=ORIENTED_EDGE('',*,*,#21742,.F.);
#31444=ORIENTED_EDGE('',*,*,#23788,.T.);
#31445=ORIENTED_EDGE('',*,*,#23780,.F.);
#31446=ORIENTED_EDGE('',*,*,#23789,.T.);
#31447=ORIENTED_EDGE('',*,*,#21739,.F.);
#31448=ORIENTED_EDGE('',*,*,#23790,.T.);
#31449=ORIENTED_EDGE('',*,*,#23791,.T.);
#31450=ORIENTED_EDGE('',*,*,#23792,.F.);
#31451=ORIENTED_EDGE('',*,*,#23792,.T.);
#31452=ORIENTED_EDGE('',*,*,#23793,.T.);
#31453=ORIENTED_EDGE('',*,*,#21740,.F.);
#31454=ORIENTED_EDGE('',*,*,#23794,.T.);
#31455=ORIENTED_EDGE('',*,*,#23795,.T.);
#31456=ORIENTED_EDGE('',*,*,#21391,.F.);
#31457=ORIENTED_EDGE('',*,*,#23796,.F.);
#31458=ORIENTED_EDGE('',*,*,#23797,.T.);
#31459=ORIENTED_EDGE('',*,*,#23798,.T.);
#31460=ORIENTED_EDGE('',*,*,#23799,.F.);
#31461=ORIENTED_EDGE('',*,*,#23800,.T.);
#31462=ORIENTED_EDGE('',*,*,#23794,.F.);
#31463=ORIENTED_EDGE('',*,*,#23801,.T.);
#31464=ORIENTED_EDGE('',*,*,#23802,.T.);
#31465=ORIENTED_EDGE('',*,*,#23803,.T.);
#31466=ORIENTED_EDGE('',*,*,#23799,.T.);
#31467=ORIENTED_EDGE('',*,*,#23804,.T.);
#31468=ORIENTED_EDGE('',*,*,#23805,.T.);
#31469=ORIENTED_EDGE('',*,*,#23806,.T.);
#31470=ORIENTED_EDGE('',*,*,#23807,.T.);
#31471=ORIENTED_EDGE('',*,*,#23808,.F.);
#31472=ORIENTED_EDGE('',*,*,#23809,.T.);
#31473=ORIENTED_EDGE('',*,*,#23810,.T.);
#31474=ORIENTED_EDGE('',*,*,#23808,.T.);
#31475=ORIENTED_EDGE('',*,*,#23811,.T.);
#31476=ORIENTED_EDGE('',*,*,#23802,.F.);
#31477=ORIENTED_EDGE('',*,*,#23812,.T.);
#31478=ORIENTED_EDGE('',*,*,#21394,.F.);
#31479=ORIENTED_EDGE('',*,*,#23813,.T.);
#31480=ORIENTED_EDGE('',*,*,#23700,.T.);
#31481=ORIENTED_EDGE('',*,*,#23814,.F.);
#31482=ORIENTED_EDGE('',*,*,#23815,.T.);
#31483=ORIENTED_EDGE('',*,*,#23805,.F.);
#31484=ORIENTED_EDGE('',*,*,#23816,.T.);
#31485=ORIENTED_EDGE('',*,*,#23817,.T.);
#31486=ORIENTED_EDGE('',*,*,#23818,.T.);
#31487=ORIENTED_EDGE('',*,*,#23814,.T.);
#31488=ORIENTED_EDGE('',*,*,#23819,.T.);
#31489=ORIENTED_EDGE('',*,*,#23820,.T.);
#31490=ORIENTED_EDGE('',*,*,#23821,.T.);
#31491=ORIENTED_EDGE('',*,*,#23822,.T.);
#31492=ORIENTED_EDGE('',*,*,#23823,.F.);
#31493=ORIENTED_EDGE('',*,*,#23824,.T.);
#31494=ORIENTED_EDGE('',*,*,#23825,.T.);
#31495=ORIENTED_EDGE('',*,*,#23823,.T.);
#31496=ORIENTED_EDGE('',*,*,#23826,.T.);
#31497=ORIENTED_EDGE('',*,*,#23817,.F.);
#31498=ORIENTED_EDGE('',*,*,#23827,.T.);
#31499=ORIENTED_EDGE('',*,*,#23828,.F.);
#31500=ORIENTED_EDGE('',*,*,#23829,.T.);
#31501=ORIENTED_EDGE('',*,*,#23820,.F.);
#31502=ORIENTED_EDGE('',*,*,#23830,.T.);
#31503=ORIENTED_EDGE('',*,*,#23831,.T.);
#31504=ORIENTED_EDGE('',*,*,#23832,.T.);
#31505=ORIENTED_EDGE('',*,*,#23828,.T.);
#31506=ORIENTED_EDGE('',*,*,#23833,.T.);
#31507=ORIENTED_EDGE('',*,*,#23834,.T.);
#31508=ORIENTED_EDGE('',*,*,#23835,.T.);
#31509=ORIENTED_EDGE('',*,*,#23836,.T.);
#31510=ORIENTED_EDGE('',*,*,#23837,.F.);
#31511=ORIENTED_EDGE('',*,*,#23838,.T.);
#31512=ORIENTED_EDGE('',*,*,#23839,.T.);
#31513=ORIENTED_EDGE('',*,*,#23837,.T.);
#31514=ORIENTED_EDGE('',*,*,#23840,.T.);
#31515=ORIENTED_EDGE('',*,*,#23831,.F.);
#31516=ORIENTED_EDGE('',*,*,#23841,.T.);
#31517=ORIENTED_EDGE('',*,*,#23842,.F.);
#31518=ORIENTED_EDGE('',*,*,#23843,.T.);
#31519=ORIENTED_EDGE('',*,*,#23834,.F.);
#31520=ORIENTED_EDGE('',*,*,#23844,.T.);
#31521=ORIENTED_EDGE('',*,*,#23845,.T.);
#31522=ORIENTED_EDGE('',*,*,#23846,.T.);
#31523=ORIENTED_EDGE('',*,*,#23842,.T.);
#31524=ORIENTED_EDGE('',*,*,#23847,.T.);
#31525=ORIENTED_EDGE('',*,*,#23848,.T.);
#31526=ORIENTED_EDGE('',*,*,#23849,.T.);
#31527=ORIENTED_EDGE('',*,*,#23850,.T.);
#31528=ORIENTED_EDGE('',*,*,#23851,.F.);
#31529=ORIENTED_EDGE('',*,*,#23852,.T.);
#31530=ORIENTED_EDGE('',*,*,#23853,.T.);
#31531=ORIENTED_EDGE('',*,*,#23851,.T.);
#31532=ORIENTED_EDGE('',*,*,#23854,.T.);
#31533=ORIENTED_EDGE('',*,*,#23845,.F.);
#31534=ORIENTED_EDGE('',*,*,#23855,.T.);
#31535=ORIENTED_EDGE('',*,*,#23856,.F.);
#31536=ORIENTED_EDGE('',*,*,#23857,.T.);
#31537=ORIENTED_EDGE('',*,*,#23848,.F.);
#31538=ORIENTED_EDGE('',*,*,#23858,.T.);
#31539=ORIENTED_EDGE('',*,*,#23859,.T.);
#31540=ORIENTED_EDGE('',*,*,#23860,.T.);
#31541=ORIENTED_EDGE('',*,*,#23856,.T.);
#31542=ORIENTED_EDGE('',*,*,#23861,.T.);
#31543=ORIENTED_EDGE('',*,*,#23862,.T.);
#31544=ORIENTED_EDGE('',*,*,#23863,.T.);
#31545=ORIENTED_EDGE('',*,*,#23864,.T.);
#31546=ORIENTED_EDGE('',*,*,#23865,.F.);
#31547=ORIENTED_EDGE('',*,*,#23866,.T.);
#31548=ORIENTED_EDGE('',*,*,#23867,.T.);
#31549=ORIENTED_EDGE('',*,*,#23865,.T.);
#31550=ORIENTED_EDGE('',*,*,#23868,.T.);
#31551=ORIENTED_EDGE('',*,*,#23859,.F.);
#31552=ORIENTED_EDGE('',*,*,#23869,.T.);
#31553=ORIENTED_EDGE('',*,*,#23870,.F.);
#31554=ORIENTED_EDGE('',*,*,#23871,.T.);
#31555=ORIENTED_EDGE('',*,*,#23862,.F.);
#31556=ORIENTED_EDGE('',*,*,#23872,.T.);
#31557=ORIENTED_EDGE('',*,*,#23873,.T.);
#31558=ORIENTED_EDGE('',*,*,#23874,.T.);
#31559=ORIENTED_EDGE('',*,*,#23870,.T.);
#31560=ORIENTED_EDGE('',*,*,#23875,.T.);
#31561=ORIENTED_EDGE('',*,*,#23876,.T.);
#31562=ORIENTED_EDGE('',*,*,#23877,.T.);
#31563=ORIENTED_EDGE('',*,*,#23878,.T.);
#31564=ORIENTED_EDGE('',*,*,#23879,.F.);
#31565=ORIENTED_EDGE('',*,*,#23880,.T.);
#31566=ORIENTED_EDGE('',*,*,#23881,.T.);
#31567=ORIENTED_EDGE('',*,*,#23879,.T.);
#31568=ORIENTED_EDGE('',*,*,#23882,.T.);
#31569=ORIENTED_EDGE('',*,*,#23873,.F.);
#31570=ORIENTED_EDGE('',*,*,#23883,.T.);
#31571=ORIENTED_EDGE('',*,*,#21748,.F.);
#31572=ORIENTED_EDGE('',*,*,#23884,.T.);
#31573=ORIENTED_EDGE('',*,*,#23876,.F.);
#31574=ORIENTED_EDGE('',*,*,#23885,.T.);
#31575=ORIENTED_EDGE('',*,*,#21745,.F.);
#31576=ORIENTED_EDGE('',*,*,#23886,.T.);
#31577=ORIENTED_EDGE('',*,*,#23887,.T.);
#31578=ORIENTED_EDGE('',*,*,#23888,.F.);
#31579=ORIENTED_EDGE('',*,*,#23888,.T.);
#31580=ORIENTED_EDGE('',*,*,#23889,.T.);
#31581=ORIENTED_EDGE('',*,*,#21746,.F.);
#31582=ORIENTED_EDGE('',*,*,#23890,.T.);
#31583=ORIENTED_EDGE('',*,*,#23891,.T.);
#31584=ORIENTED_EDGE('',*,*,#21387,.F.);
#31585=ORIENTED_EDGE('',*,*,#23892,.F.);
#31586=ORIENTED_EDGE('',*,*,#23893,.T.);
#31587=ORIENTED_EDGE('',*,*,#23894,.T.);
#31588=ORIENTED_EDGE('',*,*,#23895,.F.);
#31589=ORIENTED_EDGE('',*,*,#23896,.T.);
#31590=ORIENTED_EDGE('',*,*,#23890,.F.);
#31591=ORIENTED_EDGE('',*,*,#23897,.T.);
#31592=ORIENTED_EDGE('',*,*,#23898,.T.);
#31593=ORIENTED_EDGE('',*,*,#23899,.T.);
#31594=ORIENTED_EDGE('',*,*,#23895,.T.);
#31595=ORIENTED_EDGE('',*,*,#23900,.T.);
#31596=ORIENTED_EDGE('',*,*,#23901,.T.);
#31597=ORIENTED_EDGE('',*,*,#23902,.T.);
#31598=ORIENTED_EDGE('',*,*,#23903,.T.);
#31599=ORIENTED_EDGE('',*,*,#23904,.F.);
#31600=ORIENTED_EDGE('',*,*,#23905,.T.);
#31601=ORIENTED_EDGE('',*,*,#23906,.T.);
#31602=ORIENTED_EDGE('',*,*,#23904,.T.);
#31603=ORIENTED_EDGE('',*,*,#23907,.T.);
#31604=ORIENTED_EDGE('',*,*,#23898,.F.);
#31605=ORIENTED_EDGE('',*,*,#23908,.T.);
#31606=ORIENTED_EDGE('',*,*,#21390,.F.);
#31607=ORIENTED_EDGE('',*,*,#23909,.T.);
#31608=ORIENTED_EDGE('',*,*,#23796,.T.);
#31609=ORIENTED_EDGE('',*,*,#23910,.F.);
#31610=ORIENTED_EDGE('',*,*,#23911,.T.);
#31611=ORIENTED_EDGE('',*,*,#23901,.F.);
#31612=ORIENTED_EDGE('',*,*,#23912,.T.);
#31613=ORIENTED_EDGE('',*,*,#23913,.T.);
#31614=ORIENTED_EDGE('',*,*,#23914,.T.);
#31615=ORIENTED_EDGE('',*,*,#23910,.T.);
#31616=ORIENTED_EDGE('',*,*,#23915,.T.);
#31617=ORIENTED_EDGE('',*,*,#23916,.T.);
#31618=ORIENTED_EDGE('',*,*,#23917,.T.);
#31619=ORIENTED_EDGE('',*,*,#23918,.T.);
#31620=ORIENTED_EDGE('',*,*,#23919,.F.);
#31621=ORIENTED_EDGE('',*,*,#23920,.T.);
#31622=ORIENTED_EDGE('',*,*,#23921,.T.);
#31623=ORIENTED_EDGE('',*,*,#23919,.T.);
#31624=ORIENTED_EDGE('',*,*,#23922,.T.);
#31625=ORIENTED_EDGE('',*,*,#23913,.F.);
#31626=ORIENTED_EDGE('',*,*,#23923,.T.);
#31627=ORIENTED_EDGE('',*,*,#23924,.F.);
#31628=ORIENTED_EDGE('',*,*,#23925,.T.);
#31629=ORIENTED_EDGE('',*,*,#23916,.F.);
#31630=ORIENTED_EDGE('',*,*,#23926,.T.);
#31631=ORIENTED_EDGE('',*,*,#23927,.T.);
#31632=ORIENTED_EDGE('',*,*,#23928,.T.);
#31633=ORIENTED_EDGE('',*,*,#23924,.T.);
#31634=ORIENTED_EDGE('',*,*,#23929,.T.);
#31635=ORIENTED_EDGE('',*,*,#23930,.T.);
#31636=ORIENTED_EDGE('',*,*,#23931,.T.);
#31637=ORIENTED_EDGE('',*,*,#23932,.T.);
#31638=ORIENTED_EDGE('',*,*,#23933,.F.);
#31639=ORIENTED_EDGE('',*,*,#23934,.T.);
#31640=ORIENTED_EDGE('',*,*,#23935,.T.);
#31641=ORIENTED_EDGE('',*,*,#23933,.T.);
#31642=ORIENTED_EDGE('',*,*,#23936,.T.);
#31643=ORIENTED_EDGE('',*,*,#23927,.F.);
#31644=ORIENTED_EDGE('',*,*,#23937,.T.);
#31645=ORIENTED_EDGE('',*,*,#23938,.F.);
#31646=ORIENTED_EDGE('',*,*,#23939,.T.);
#31647=ORIENTED_EDGE('',*,*,#23930,.F.);
#31648=ORIENTED_EDGE('',*,*,#23940,.T.);
#31649=ORIENTED_EDGE('',*,*,#23941,.T.);
#31650=ORIENTED_EDGE('',*,*,#23942,.T.);
#31651=ORIENTED_EDGE('',*,*,#23938,.T.);
#31652=ORIENTED_EDGE('',*,*,#23943,.T.);
#31653=ORIENTED_EDGE('',*,*,#23944,.T.);
#31654=ORIENTED_EDGE('',*,*,#23945,.T.);
#31655=ORIENTED_EDGE('',*,*,#23946,.T.);
#31656=ORIENTED_EDGE('',*,*,#23947,.F.);
#31657=ORIENTED_EDGE('',*,*,#23948,.T.);
#31658=ORIENTED_EDGE('',*,*,#23949,.T.);
#31659=ORIENTED_EDGE('',*,*,#23947,.T.);
#31660=ORIENTED_EDGE('',*,*,#23950,.T.);
#31661=ORIENTED_EDGE('',*,*,#23941,.F.);
#31662=ORIENTED_EDGE('',*,*,#23951,.T.);
#31663=ORIENTED_EDGE('',*,*,#23952,.F.);
#31664=ORIENTED_EDGE('',*,*,#23953,.T.);
#31665=ORIENTED_EDGE('',*,*,#23944,.F.);
#31666=ORIENTED_EDGE('',*,*,#23954,.T.);
#31667=ORIENTED_EDGE('',*,*,#23955,.T.);
#31668=ORIENTED_EDGE('',*,*,#23956,.T.);
#31669=ORIENTED_EDGE('',*,*,#23952,.T.);
#31670=ORIENTED_EDGE('',*,*,#23957,.T.);
#31671=ORIENTED_EDGE('',*,*,#23958,.T.);
#31672=ORIENTED_EDGE('',*,*,#23959,.T.);
#31673=ORIENTED_EDGE('',*,*,#23960,.T.);
#31674=ORIENTED_EDGE('',*,*,#23961,.F.);
#31675=ORIENTED_EDGE('',*,*,#23962,.T.);
#31676=ORIENTED_EDGE('',*,*,#23963,.T.);
#31677=ORIENTED_EDGE('',*,*,#23961,.T.);
#31678=ORIENTED_EDGE('',*,*,#23964,.T.);
#31679=ORIENTED_EDGE('',*,*,#23955,.F.);
#31680=ORIENTED_EDGE('',*,*,#23965,.T.);
#31681=ORIENTED_EDGE('',*,*,#23966,.F.);
#31682=ORIENTED_EDGE('',*,*,#23967,.T.);
#31683=ORIENTED_EDGE('',*,*,#23958,.F.);
#31684=ORIENTED_EDGE('',*,*,#23968,.T.);
#31685=ORIENTED_EDGE('',*,*,#23969,.T.);
#31686=ORIENTED_EDGE('',*,*,#23970,.T.);
#31687=ORIENTED_EDGE('',*,*,#23966,.T.);
#31688=ORIENTED_EDGE('',*,*,#23971,.T.);
#31689=ORIENTED_EDGE('',*,*,#23972,.T.);
#31690=ORIENTED_EDGE('',*,*,#23973,.T.);
#31691=ORIENTED_EDGE('',*,*,#23974,.T.);
#31692=ORIENTED_EDGE('',*,*,#23975,.F.);
#31693=ORIENTED_EDGE('',*,*,#23976,.T.);
#31694=ORIENTED_EDGE('',*,*,#23977,.T.);
#31695=ORIENTED_EDGE('',*,*,#23975,.T.);
#31696=ORIENTED_EDGE('',*,*,#23978,.T.);
#31697=ORIENTED_EDGE('',*,*,#23969,.F.);
#31698=ORIENTED_EDGE('',*,*,#23979,.T.);
#31699=ORIENTED_EDGE('',*,*,#21754,.F.);
#31700=ORIENTED_EDGE('',*,*,#23980,.T.);
#31701=ORIENTED_EDGE('',*,*,#23972,.F.);
#31702=ORIENTED_EDGE('',*,*,#23981,.T.);
#31703=ORIENTED_EDGE('',*,*,#21751,.F.);
#31704=ORIENTED_EDGE('',*,*,#23982,.T.);
#31705=ORIENTED_EDGE('',*,*,#23983,.T.);
#31706=ORIENTED_EDGE('',*,*,#23984,.F.);
#31707=ORIENTED_EDGE('',*,*,#23984,.T.);
#31708=ORIENTED_EDGE('',*,*,#23985,.T.);
#31709=ORIENTED_EDGE('',*,*,#21752,.F.);
#31710=ORIENTED_EDGE('',*,*,#23986,.T.);
#31711=ORIENTED_EDGE('',*,*,#23987,.T.);
#31712=ORIENTED_EDGE('',*,*,#21383,.F.);
#31713=ORIENTED_EDGE('',*,*,#23988,.F.);
#31714=ORIENTED_EDGE('',*,*,#23989,.T.);
#31715=ORIENTED_EDGE('',*,*,#23990,.T.);
#31716=ORIENTED_EDGE('',*,*,#23991,.F.);
#31717=ORIENTED_EDGE('',*,*,#23992,.T.);
#31718=ORIENTED_EDGE('',*,*,#23986,.F.);
#31719=ORIENTED_EDGE('',*,*,#23993,.T.);
#31720=ORIENTED_EDGE('',*,*,#23994,.T.);
#31721=ORIENTED_EDGE('',*,*,#23995,.T.);
#31722=ORIENTED_EDGE('',*,*,#23991,.T.);
#31723=ORIENTED_EDGE('',*,*,#23996,.T.);
#31724=ORIENTED_EDGE('',*,*,#23997,.T.);
#31725=ORIENTED_EDGE('',*,*,#23998,.T.);
#31726=ORIENTED_EDGE('',*,*,#23999,.T.);
#31727=ORIENTED_EDGE('',*,*,#24000,.F.);
#31728=ORIENTED_EDGE('',*,*,#24001,.T.);
#31729=ORIENTED_EDGE('',*,*,#24002,.T.);
#31730=ORIENTED_EDGE('',*,*,#24000,.T.);
#31731=ORIENTED_EDGE('',*,*,#24003,.T.);
#31732=ORIENTED_EDGE('',*,*,#23994,.F.);
#31733=ORIENTED_EDGE('',*,*,#24004,.T.);
#31734=ORIENTED_EDGE('',*,*,#21386,.F.);
#31735=ORIENTED_EDGE('',*,*,#24005,.T.);
#31736=ORIENTED_EDGE('',*,*,#23892,.T.);
#31737=ORIENTED_EDGE('',*,*,#24006,.F.);
#31738=ORIENTED_EDGE('',*,*,#24007,.T.);
#31739=ORIENTED_EDGE('',*,*,#23997,.F.);
#31740=ORIENTED_EDGE('',*,*,#24008,.T.);
#31741=ORIENTED_EDGE('',*,*,#24009,.T.);
#31742=ORIENTED_EDGE('',*,*,#24010,.T.);
#31743=ORIENTED_EDGE('',*,*,#24006,.T.);
#31744=ORIENTED_EDGE('',*,*,#24011,.T.);
#31745=ORIENTED_EDGE('',*,*,#24012,.T.);
#31746=ORIENTED_EDGE('',*,*,#24013,.T.);
#31747=ORIENTED_EDGE('',*,*,#24014,.T.);
#31748=ORIENTED_EDGE('',*,*,#24015,.F.);
#31749=ORIENTED_EDGE('',*,*,#24016,.T.);
#31750=ORIENTED_EDGE('',*,*,#24017,.T.);
#31751=ORIENTED_EDGE('',*,*,#24015,.T.);
#31752=ORIENTED_EDGE('',*,*,#24018,.T.);
#31753=ORIENTED_EDGE('',*,*,#24009,.F.);
#31754=ORIENTED_EDGE('',*,*,#24019,.T.);
#31755=ORIENTED_EDGE('',*,*,#24020,.F.);
#31756=ORIENTED_EDGE('',*,*,#24021,.T.);
#31757=ORIENTED_EDGE('',*,*,#24012,.F.);
#31758=ORIENTED_EDGE('',*,*,#24022,.T.);
#31759=ORIENTED_EDGE('',*,*,#24023,.T.);
#31760=ORIENTED_EDGE('',*,*,#24024,.T.);
#31761=ORIENTED_EDGE('',*,*,#24020,.T.);
#31762=ORIENTED_EDGE('',*,*,#24025,.T.);
#31763=ORIENTED_EDGE('',*,*,#24026,.T.);
#31764=ORIENTED_EDGE('',*,*,#24027,.T.);
#31765=ORIENTED_EDGE('',*,*,#24028,.T.);
#31766=ORIENTED_EDGE('',*,*,#24029,.F.);
#31767=ORIENTED_EDGE('',*,*,#24030,.T.);
#31768=ORIENTED_EDGE('',*,*,#24031,.T.);
#31769=ORIENTED_EDGE('',*,*,#24029,.T.);
#31770=ORIENTED_EDGE('',*,*,#24032,.T.);
#31771=ORIENTED_EDGE('',*,*,#24023,.F.);
#31772=ORIENTED_EDGE('',*,*,#24033,.T.);
#31773=ORIENTED_EDGE('',*,*,#24034,.F.);
#31774=ORIENTED_EDGE('',*,*,#24035,.T.);
#31775=ORIENTED_EDGE('',*,*,#24026,.F.);
#31776=ORIENTED_EDGE('',*,*,#24036,.T.);
#31777=ORIENTED_EDGE('',*,*,#24037,.T.);
#31778=ORIENTED_EDGE('',*,*,#24038,.T.);
#31779=ORIENTED_EDGE('',*,*,#24034,.T.);
#31780=ORIENTED_EDGE('',*,*,#24039,.T.);
#31781=ORIENTED_EDGE('',*,*,#24040,.T.);
#31782=ORIENTED_EDGE('',*,*,#24041,.T.);
#31783=ORIENTED_EDGE('',*,*,#24042,.T.);
#31784=ORIENTED_EDGE('',*,*,#24043,.F.);
#31785=ORIENTED_EDGE('',*,*,#24044,.T.);
#31786=ORIENTED_EDGE('',*,*,#24045,.T.);
#31787=ORIENTED_EDGE('',*,*,#24043,.T.);
#31788=ORIENTED_EDGE('',*,*,#24046,.T.);
#31789=ORIENTED_EDGE('',*,*,#24037,.F.);
#31790=ORIENTED_EDGE('',*,*,#24047,.T.);
#31791=ORIENTED_EDGE('',*,*,#24048,.F.);
#31792=ORIENTED_EDGE('',*,*,#24049,.T.);
#31793=ORIENTED_EDGE('',*,*,#24040,.F.);
#31794=ORIENTED_EDGE('',*,*,#24050,.T.);
#31795=ORIENTED_EDGE('',*,*,#24051,.T.);
#31796=ORIENTED_EDGE('',*,*,#24052,.T.);
#31797=ORIENTED_EDGE('',*,*,#24048,.T.);
#31798=ORIENTED_EDGE('',*,*,#24053,.T.);
#31799=ORIENTED_EDGE('',*,*,#24054,.T.);
#31800=ORIENTED_EDGE('',*,*,#24055,.T.);
#31801=ORIENTED_EDGE('',*,*,#24056,.T.);
#31802=ORIENTED_EDGE('',*,*,#24057,.F.);
#31803=ORIENTED_EDGE('',*,*,#24058,.T.);
#31804=ORIENTED_EDGE('',*,*,#24059,.T.);
#31805=ORIENTED_EDGE('',*,*,#24057,.T.);
#31806=ORIENTED_EDGE('',*,*,#24060,.T.);
#31807=ORIENTED_EDGE('',*,*,#24051,.F.);
#31808=ORIENTED_EDGE('',*,*,#24061,.T.);
#31809=ORIENTED_EDGE('',*,*,#24062,.F.);
#31810=ORIENTED_EDGE('',*,*,#24063,.T.);
#31811=ORIENTED_EDGE('',*,*,#24054,.F.);
#31812=ORIENTED_EDGE('',*,*,#24064,.T.);
#31813=ORIENTED_EDGE('',*,*,#24065,.T.);
#31814=ORIENTED_EDGE('',*,*,#24066,.T.);
#31815=ORIENTED_EDGE('',*,*,#24062,.T.);
#31816=ORIENTED_EDGE('',*,*,#24067,.T.);
#31817=ORIENTED_EDGE('',*,*,#24068,.T.);
#31818=ORIENTED_EDGE('',*,*,#24069,.T.);
#31819=ORIENTED_EDGE('',*,*,#24070,.T.);
#31820=ORIENTED_EDGE('',*,*,#24071,.F.);
#31821=ORIENTED_EDGE('',*,*,#24072,.T.);
#31822=ORIENTED_EDGE('',*,*,#24073,.T.);
#31823=ORIENTED_EDGE('',*,*,#24071,.T.);
#31824=ORIENTED_EDGE('',*,*,#24074,.T.);
#31825=ORIENTED_EDGE('',*,*,#24065,.F.);
#31826=ORIENTED_EDGE('',*,*,#24075,.T.);
#31827=ORIENTED_EDGE('',*,*,#21760,.F.);
#31828=ORIENTED_EDGE('',*,*,#24076,.T.);
#31829=ORIENTED_EDGE('',*,*,#24068,.F.);
#31830=ORIENTED_EDGE('',*,*,#24077,.T.);
#31831=ORIENTED_EDGE('',*,*,#21757,.F.);
#31832=ORIENTED_EDGE('',*,*,#24078,.T.);
#31833=ORIENTED_EDGE('',*,*,#24079,.T.);
#31834=ORIENTED_EDGE('',*,*,#24080,.F.);
#31835=ORIENTED_EDGE('',*,*,#24080,.T.);
#31836=ORIENTED_EDGE('',*,*,#24081,.T.);
#31837=ORIENTED_EDGE('',*,*,#21758,.F.);
#31838=ORIENTED_EDGE('',*,*,#24082,.T.);
#31839=ORIENTED_EDGE('',*,*,#24083,.T.);
#31840=ORIENTED_EDGE('',*,*,#21379,.F.);
#31841=ORIENTED_EDGE('',*,*,#24084,.F.);
#31842=ORIENTED_EDGE('',*,*,#24085,.T.);
#31843=ORIENTED_EDGE('',*,*,#24086,.T.);
#31844=ORIENTED_EDGE('',*,*,#24087,.F.);
#31845=ORIENTED_EDGE('',*,*,#24088,.T.);
#31846=ORIENTED_EDGE('',*,*,#24082,.F.);
#31847=ORIENTED_EDGE('',*,*,#24089,.T.);
#31848=ORIENTED_EDGE('',*,*,#24090,.T.);
#31849=ORIENTED_EDGE('',*,*,#24091,.T.);
#31850=ORIENTED_EDGE('',*,*,#24087,.T.);
#31851=ORIENTED_EDGE('',*,*,#24092,.T.);
#31852=ORIENTED_EDGE('',*,*,#24093,.T.);
#31853=ORIENTED_EDGE('',*,*,#24094,.T.);
#31854=ORIENTED_EDGE('',*,*,#24095,.T.);
#31855=ORIENTED_EDGE('',*,*,#24096,.F.);
#31856=ORIENTED_EDGE('',*,*,#24097,.T.);
#31857=ORIENTED_EDGE('',*,*,#24098,.T.);
#31858=ORIENTED_EDGE('',*,*,#24096,.T.);
#31859=ORIENTED_EDGE('',*,*,#24099,.T.);
#31860=ORIENTED_EDGE('',*,*,#24090,.F.);
#31861=ORIENTED_EDGE('',*,*,#24100,.T.);
#31862=ORIENTED_EDGE('',*,*,#21382,.F.);
#31863=ORIENTED_EDGE('',*,*,#24101,.T.);
#31864=ORIENTED_EDGE('',*,*,#23988,.T.);
#31865=ORIENTED_EDGE('',*,*,#24102,.F.);
#31866=ORIENTED_EDGE('',*,*,#24103,.T.);
#31867=ORIENTED_EDGE('',*,*,#24093,.F.);
#31868=ORIENTED_EDGE('',*,*,#24104,.T.);
#31869=ORIENTED_EDGE('',*,*,#24105,.T.);
#31870=ORIENTED_EDGE('',*,*,#24106,.T.);
#31871=ORIENTED_EDGE('',*,*,#24102,.T.);
#31872=ORIENTED_EDGE('',*,*,#24107,.T.);
#31873=ORIENTED_EDGE('',*,*,#24108,.T.);
#31874=ORIENTED_EDGE('',*,*,#24109,.T.);
#31875=ORIENTED_EDGE('',*,*,#24110,.T.);
#31876=ORIENTED_EDGE('',*,*,#24111,.F.);
#31877=ORIENTED_EDGE('',*,*,#24112,.T.);
#31878=ORIENTED_EDGE('',*,*,#24113,.T.);
#31879=ORIENTED_EDGE('',*,*,#24111,.T.);
#31880=ORIENTED_EDGE('',*,*,#24114,.T.);
#31881=ORIENTED_EDGE('',*,*,#24105,.F.);
#31882=ORIENTED_EDGE('',*,*,#24115,.T.);
#31883=ORIENTED_EDGE('',*,*,#24116,.F.);
#31884=ORIENTED_EDGE('',*,*,#24117,.T.);
#31885=ORIENTED_EDGE('',*,*,#24108,.F.);
#31886=ORIENTED_EDGE('',*,*,#24118,.T.);
#31887=ORIENTED_EDGE('',*,*,#24119,.T.);
#31888=ORIENTED_EDGE('',*,*,#24120,.T.);
#31889=ORIENTED_EDGE('',*,*,#24116,.T.);
#31890=ORIENTED_EDGE('',*,*,#24121,.T.);
#31891=ORIENTED_EDGE('',*,*,#24122,.T.);
#31892=ORIENTED_EDGE('',*,*,#24123,.T.);
#31893=ORIENTED_EDGE('',*,*,#24124,.T.);
#31894=ORIENTED_EDGE('',*,*,#24125,.F.);
#31895=ORIENTED_EDGE('',*,*,#24126,.T.);
#31896=ORIENTED_EDGE('',*,*,#24127,.T.);
#31897=ORIENTED_EDGE('',*,*,#24125,.T.);
#31898=ORIENTED_EDGE('',*,*,#24128,.T.);
#31899=ORIENTED_EDGE('',*,*,#24119,.F.);
#31900=ORIENTED_EDGE('',*,*,#24129,.T.);
#31901=ORIENTED_EDGE('',*,*,#24130,.F.);
#31902=ORIENTED_EDGE('',*,*,#24131,.T.);
#31903=ORIENTED_EDGE('',*,*,#24122,.F.);
#31904=ORIENTED_EDGE('',*,*,#24132,.T.);
#31905=ORIENTED_EDGE('',*,*,#24133,.T.);
#31906=ORIENTED_EDGE('',*,*,#24134,.T.);
#31907=ORIENTED_EDGE('',*,*,#24130,.T.);
#31908=ORIENTED_EDGE('',*,*,#24135,.T.);
#31909=ORIENTED_EDGE('',*,*,#24136,.T.);
#31910=ORIENTED_EDGE('',*,*,#24137,.T.);
#31911=ORIENTED_EDGE('',*,*,#24138,.T.);
#31912=ORIENTED_EDGE('',*,*,#24139,.F.);
#31913=ORIENTED_EDGE('',*,*,#24140,.T.);
#31914=ORIENTED_EDGE('',*,*,#24141,.T.);
#31915=ORIENTED_EDGE('',*,*,#24139,.T.);
#31916=ORIENTED_EDGE('',*,*,#24142,.T.);
#31917=ORIENTED_EDGE('',*,*,#24133,.F.);
#31918=ORIENTED_EDGE('',*,*,#24143,.T.);
#31919=ORIENTED_EDGE('',*,*,#24144,.F.);
#31920=ORIENTED_EDGE('',*,*,#24145,.T.);
#31921=ORIENTED_EDGE('',*,*,#24136,.F.);
#31922=ORIENTED_EDGE('',*,*,#24146,.T.);
#31923=ORIENTED_EDGE('',*,*,#24147,.T.);
#31924=ORIENTED_EDGE('',*,*,#24148,.T.);
#31925=ORIENTED_EDGE('',*,*,#24144,.T.);
#31926=ORIENTED_EDGE('',*,*,#24149,.T.);
#31927=ORIENTED_EDGE('',*,*,#24150,.T.);
#31928=ORIENTED_EDGE('',*,*,#24151,.T.);
#31929=ORIENTED_EDGE('',*,*,#24152,.T.);
#31930=ORIENTED_EDGE('',*,*,#24153,.F.);
#31931=ORIENTED_EDGE('',*,*,#24154,.T.);
#31932=ORIENTED_EDGE('',*,*,#24155,.T.);
#31933=ORIENTED_EDGE('',*,*,#24153,.T.);
#31934=ORIENTED_EDGE('',*,*,#24156,.T.);
#31935=ORIENTED_EDGE('',*,*,#24147,.F.);
#31936=ORIENTED_EDGE('',*,*,#24157,.T.);
#31937=ORIENTED_EDGE('',*,*,#24158,.F.);
#31938=ORIENTED_EDGE('',*,*,#24159,.T.);
#31939=ORIENTED_EDGE('',*,*,#24150,.F.);
#31940=ORIENTED_EDGE('',*,*,#24160,.T.);
#31941=ORIENTED_EDGE('',*,*,#24161,.T.);
#31942=ORIENTED_EDGE('',*,*,#24162,.T.);
#31943=ORIENTED_EDGE('',*,*,#24158,.T.);
#31944=ORIENTED_EDGE('',*,*,#24163,.T.);
#31945=ORIENTED_EDGE('',*,*,#24164,.T.);
#31946=ORIENTED_EDGE('',*,*,#24165,.T.);
#31947=ORIENTED_EDGE('',*,*,#24166,.T.);
#31948=ORIENTED_EDGE('',*,*,#24167,.F.);
#31949=ORIENTED_EDGE('',*,*,#24168,.T.);
#31950=ORIENTED_EDGE('',*,*,#24169,.T.);
#31951=ORIENTED_EDGE('',*,*,#24167,.T.);
#31952=ORIENTED_EDGE('',*,*,#24170,.T.);
#31953=ORIENTED_EDGE('',*,*,#24161,.F.);
#31954=ORIENTED_EDGE('',*,*,#24171,.T.);
#31955=ORIENTED_EDGE('',*,*,#21766,.F.);
#31956=ORIENTED_EDGE('',*,*,#24172,.T.);
#31957=ORIENTED_EDGE('',*,*,#24164,.F.);
#31958=ORIENTED_EDGE('',*,*,#24173,.T.);
#31959=ORIENTED_EDGE('',*,*,#21763,.F.);
#31960=ORIENTED_EDGE('',*,*,#24174,.T.);
#31961=ORIENTED_EDGE('',*,*,#24175,.T.);
#31962=ORIENTED_EDGE('',*,*,#24176,.F.);
#31963=ORIENTED_EDGE('',*,*,#24176,.T.);
#31964=ORIENTED_EDGE('',*,*,#24177,.T.);
#31965=ORIENTED_EDGE('',*,*,#21764,.F.);
#31966=ORIENTED_EDGE('',*,*,#24178,.T.);
#31967=ORIENTED_EDGE('',*,*,#24179,.T.);
#31968=ORIENTED_EDGE('',*,*,#21375,.F.);
#31969=ORIENTED_EDGE('',*,*,#24180,.F.);
#31970=ORIENTED_EDGE('',*,*,#24181,.T.);
#31971=ORIENTED_EDGE('',*,*,#24182,.T.);
#31972=ORIENTED_EDGE('',*,*,#24183,.F.);
#31973=ORIENTED_EDGE('',*,*,#24184,.T.);
#31974=ORIENTED_EDGE('',*,*,#24178,.F.);
#31975=ORIENTED_EDGE('',*,*,#24185,.T.);
#31976=ORIENTED_EDGE('',*,*,#24186,.T.);
#31977=ORIENTED_EDGE('',*,*,#24187,.T.);
#31978=ORIENTED_EDGE('',*,*,#24183,.T.);
#31979=ORIENTED_EDGE('',*,*,#24188,.T.);
#31980=ORIENTED_EDGE('',*,*,#24189,.T.);
#31981=ORIENTED_EDGE('',*,*,#24190,.T.);
#31982=ORIENTED_EDGE('',*,*,#24191,.T.);
#31983=ORIENTED_EDGE('',*,*,#24192,.F.);
#31984=ORIENTED_EDGE('',*,*,#24193,.T.);
#31985=ORIENTED_EDGE('',*,*,#24194,.T.);
#31986=ORIENTED_EDGE('',*,*,#24192,.T.);
#31987=ORIENTED_EDGE('',*,*,#24195,.T.);
#31988=ORIENTED_EDGE('',*,*,#24186,.F.);
#31989=ORIENTED_EDGE('',*,*,#24196,.T.);
#31990=ORIENTED_EDGE('',*,*,#21378,.F.);
#31991=ORIENTED_EDGE('',*,*,#24197,.T.);
#31992=ORIENTED_EDGE('',*,*,#24084,.T.);
#31993=ORIENTED_EDGE('',*,*,#24198,.F.);
#31994=ORIENTED_EDGE('',*,*,#24199,.T.);
#31995=ORIENTED_EDGE('',*,*,#24189,.F.);
#31996=ORIENTED_EDGE('',*,*,#24200,.T.);
#31997=ORIENTED_EDGE('',*,*,#24201,.T.);
#31998=ORIENTED_EDGE('',*,*,#24202,.T.);
#31999=ORIENTED_EDGE('',*,*,#24198,.T.);
#32000=ORIENTED_EDGE('',*,*,#24203,.T.);
#32001=ORIENTED_EDGE('',*,*,#24204,.T.);
#32002=ORIENTED_EDGE('',*,*,#24205,.T.);
#32003=ORIENTED_EDGE('',*,*,#24206,.T.);
#32004=ORIENTED_EDGE('',*,*,#24207,.F.);
#32005=ORIENTED_EDGE('',*,*,#24208,.T.);
#32006=ORIENTED_EDGE('',*,*,#24209,.T.);
#32007=ORIENTED_EDGE('',*,*,#24207,.T.);
#32008=ORIENTED_EDGE('',*,*,#24210,.T.);
#32009=ORIENTED_EDGE('',*,*,#24201,.F.);
#32010=ORIENTED_EDGE('',*,*,#24211,.T.);
#32011=ORIENTED_EDGE('',*,*,#24212,.F.);
#32012=ORIENTED_EDGE('',*,*,#24213,.T.);
#32013=ORIENTED_EDGE('',*,*,#24204,.F.);
#32014=ORIENTED_EDGE('',*,*,#24214,.T.);
#32015=ORIENTED_EDGE('',*,*,#24215,.T.);
#32016=ORIENTED_EDGE('',*,*,#24216,.T.);
#32017=ORIENTED_EDGE('',*,*,#24212,.T.);
#32018=ORIENTED_EDGE('',*,*,#24217,.T.);
#32019=ORIENTED_EDGE('',*,*,#24218,.T.);
#32020=ORIENTED_EDGE('',*,*,#24219,.T.);
#32021=ORIENTED_EDGE('',*,*,#24220,.T.);
#32022=ORIENTED_EDGE('',*,*,#24221,.F.);
#32023=ORIENTED_EDGE('',*,*,#24222,.T.);
#32024=ORIENTED_EDGE('',*,*,#24223,.T.);
#32025=ORIENTED_EDGE('',*,*,#24221,.T.);
#32026=ORIENTED_EDGE('',*,*,#24224,.T.);
#32027=ORIENTED_EDGE('',*,*,#24215,.F.);
#32028=ORIENTED_EDGE('',*,*,#24225,.T.);
#32029=ORIENTED_EDGE('',*,*,#24226,.F.);
#32030=ORIENTED_EDGE('',*,*,#24227,.T.);
#32031=ORIENTED_EDGE('',*,*,#24218,.F.);
#32032=ORIENTED_EDGE('',*,*,#24228,.T.);
#32033=ORIENTED_EDGE('',*,*,#24229,.T.);
#32034=ORIENTED_EDGE('',*,*,#24230,.T.);
#32035=ORIENTED_EDGE('',*,*,#24226,.T.);
#32036=ORIENTED_EDGE('',*,*,#24231,.T.);
#32037=ORIENTED_EDGE('',*,*,#24232,.T.);
#32038=ORIENTED_EDGE('',*,*,#24233,.T.);
#32039=ORIENTED_EDGE('',*,*,#24234,.T.);
#32040=ORIENTED_EDGE('',*,*,#24235,.F.);
#32041=ORIENTED_EDGE('',*,*,#24236,.T.);
#32042=ORIENTED_EDGE('',*,*,#24237,.T.);
#32043=ORIENTED_EDGE('',*,*,#24235,.T.);
#32044=ORIENTED_EDGE('',*,*,#24238,.T.);
#32045=ORIENTED_EDGE('',*,*,#24229,.F.);
#32046=ORIENTED_EDGE('',*,*,#24239,.T.);
#32047=ORIENTED_EDGE('',*,*,#24240,.F.);
#32048=ORIENTED_EDGE('',*,*,#24241,.T.);
#32049=ORIENTED_EDGE('',*,*,#24232,.F.);
#32050=ORIENTED_EDGE('',*,*,#24242,.T.);
#32051=ORIENTED_EDGE('',*,*,#24243,.T.);
#32052=ORIENTED_EDGE('',*,*,#24244,.T.);
#32053=ORIENTED_EDGE('',*,*,#24240,.T.);
#32054=ORIENTED_EDGE('',*,*,#24245,.T.);
#32055=ORIENTED_EDGE('',*,*,#24246,.T.);
#32056=ORIENTED_EDGE('',*,*,#24247,.T.);
#32057=ORIENTED_EDGE('',*,*,#24248,.T.);
#32058=ORIENTED_EDGE('',*,*,#24249,.F.);
#32059=ORIENTED_EDGE('',*,*,#24250,.T.);
#32060=ORIENTED_EDGE('',*,*,#24251,.T.);
#32061=ORIENTED_EDGE('',*,*,#24249,.T.);
#32062=ORIENTED_EDGE('',*,*,#24252,.T.);
#32063=ORIENTED_EDGE('',*,*,#24243,.F.);
#32064=ORIENTED_EDGE('',*,*,#24253,.T.);
#32065=ORIENTED_EDGE('',*,*,#24254,.F.);
#32066=ORIENTED_EDGE('',*,*,#24255,.T.);
#32067=ORIENTED_EDGE('',*,*,#24246,.F.);
#32068=ORIENTED_EDGE('',*,*,#24256,.T.);
#32069=ORIENTED_EDGE('',*,*,#24257,.T.);
#32070=ORIENTED_EDGE('',*,*,#24258,.T.);
#32071=ORIENTED_EDGE('',*,*,#24254,.T.);
#32072=ORIENTED_EDGE('',*,*,#24259,.T.);
#32073=ORIENTED_EDGE('',*,*,#24260,.T.);
#32074=ORIENTED_EDGE('',*,*,#24261,.T.);
#32075=ORIENTED_EDGE('',*,*,#24262,.T.);
#32076=ORIENTED_EDGE('',*,*,#24263,.F.);
#32077=ORIENTED_EDGE('',*,*,#24264,.T.);
#32078=ORIENTED_EDGE('',*,*,#24265,.T.);
#32079=ORIENTED_EDGE('',*,*,#24263,.T.);
#32080=ORIENTED_EDGE('',*,*,#24266,.T.);
#32081=ORIENTED_EDGE('',*,*,#24257,.F.);
#32082=ORIENTED_EDGE('',*,*,#24267,.T.);
#32083=ORIENTED_EDGE('',*,*,#21772,.F.);
#32084=ORIENTED_EDGE('',*,*,#24268,.T.);
#32085=ORIENTED_EDGE('',*,*,#24260,.F.);
#32086=ORIENTED_EDGE('',*,*,#24269,.T.);
#32087=ORIENTED_EDGE('',*,*,#21769,.F.);
#32088=ORIENTED_EDGE('',*,*,#24270,.T.);
#32089=ORIENTED_EDGE('',*,*,#24271,.T.);
#32090=ORIENTED_EDGE('',*,*,#24272,.F.);
#32091=ORIENTED_EDGE('',*,*,#24272,.T.);
#32092=ORIENTED_EDGE('',*,*,#24273,.T.);
#32093=ORIENTED_EDGE('',*,*,#21770,.F.);
#32094=ORIENTED_EDGE('',*,*,#24274,.T.);
#32095=ORIENTED_EDGE('',*,*,#24275,.T.);
#32096=ORIENTED_EDGE('',*,*,#21371,.F.);
#32097=ORIENTED_EDGE('',*,*,#24276,.F.);
#32098=ORIENTED_EDGE('',*,*,#24277,.T.);
#32099=ORIENTED_EDGE('',*,*,#24278,.T.);
#32100=ORIENTED_EDGE('',*,*,#24279,.F.);
#32101=ORIENTED_EDGE('',*,*,#24280,.T.);
#32102=ORIENTED_EDGE('',*,*,#24274,.F.);
#32103=ORIENTED_EDGE('',*,*,#24281,.T.);
#32104=ORIENTED_EDGE('',*,*,#24282,.T.);
#32105=ORIENTED_EDGE('',*,*,#24283,.T.);
#32106=ORIENTED_EDGE('',*,*,#24279,.T.);
#32107=ORIENTED_EDGE('',*,*,#24284,.T.);
#32108=ORIENTED_EDGE('',*,*,#24285,.T.);
#32109=ORIENTED_EDGE('',*,*,#24286,.T.);
#32110=ORIENTED_EDGE('',*,*,#24287,.T.);
#32111=ORIENTED_EDGE('',*,*,#24288,.F.);
#32112=ORIENTED_EDGE('',*,*,#24289,.T.);
#32113=ORIENTED_EDGE('',*,*,#24290,.T.);
#32114=ORIENTED_EDGE('',*,*,#24288,.T.);
#32115=ORIENTED_EDGE('',*,*,#24291,.T.);
#32116=ORIENTED_EDGE('',*,*,#24282,.F.);
#32117=ORIENTED_EDGE('',*,*,#24292,.T.);
#32118=ORIENTED_EDGE('',*,*,#21374,.F.);
#32119=ORIENTED_EDGE('',*,*,#24293,.T.);
#32120=ORIENTED_EDGE('',*,*,#24180,.T.);
#32121=ORIENTED_EDGE('',*,*,#24294,.F.);
#32122=ORIENTED_EDGE('',*,*,#24295,.T.);
#32123=ORIENTED_EDGE('',*,*,#24285,.F.);
#32124=ORIENTED_EDGE('',*,*,#24296,.T.);
#32125=ORIENTED_EDGE('',*,*,#24297,.T.);
#32126=ORIENTED_EDGE('',*,*,#24298,.T.);
#32127=ORIENTED_EDGE('',*,*,#24294,.T.);
#32128=ORIENTED_EDGE('',*,*,#24299,.T.);
#32129=ORIENTED_EDGE('',*,*,#24300,.T.);
#32130=ORIENTED_EDGE('',*,*,#24301,.T.);
#32131=ORIENTED_EDGE('',*,*,#24302,.T.);
#32132=ORIENTED_EDGE('',*,*,#24303,.F.);
#32133=ORIENTED_EDGE('',*,*,#24304,.T.);
#32134=ORIENTED_EDGE('',*,*,#24305,.T.);
#32135=ORIENTED_EDGE('',*,*,#24303,.T.);
#32136=ORIENTED_EDGE('',*,*,#24306,.T.);
#32137=ORIENTED_EDGE('',*,*,#24297,.F.);
#32138=ORIENTED_EDGE('',*,*,#24307,.T.);
#32139=ORIENTED_EDGE('',*,*,#24308,.F.);
#32140=ORIENTED_EDGE('',*,*,#24309,.T.);
#32141=ORIENTED_EDGE('',*,*,#24300,.F.);
#32142=ORIENTED_EDGE('',*,*,#24310,.T.);
#32143=ORIENTED_EDGE('',*,*,#24311,.T.);
#32144=ORIENTED_EDGE('',*,*,#24312,.T.);
#32145=ORIENTED_EDGE('',*,*,#24308,.T.);
#32146=ORIENTED_EDGE('',*,*,#24313,.T.);
#32147=ORIENTED_EDGE('',*,*,#24314,.T.);
#32148=ORIENTED_EDGE('',*,*,#24315,.T.);
#32149=ORIENTED_EDGE('',*,*,#24316,.T.);
#32150=ORIENTED_EDGE('',*,*,#24317,.F.);
#32151=ORIENTED_EDGE('',*,*,#24318,.T.);
#32152=ORIENTED_EDGE('',*,*,#24319,.T.);
#32153=ORIENTED_EDGE('',*,*,#24317,.T.);
#32154=ORIENTED_EDGE('',*,*,#24320,.T.);
#32155=ORIENTED_EDGE('',*,*,#24311,.F.);
#32156=ORIENTED_EDGE('',*,*,#24321,.T.);
#32157=ORIENTED_EDGE('',*,*,#24322,.F.);
#32158=ORIENTED_EDGE('',*,*,#24323,.T.);
#32159=ORIENTED_EDGE('',*,*,#24314,.F.);
#32160=ORIENTED_EDGE('',*,*,#24324,.T.);
#32161=ORIENTED_EDGE('',*,*,#24325,.T.);
#32162=ORIENTED_EDGE('',*,*,#24326,.T.);
#32163=ORIENTED_EDGE('',*,*,#24322,.T.);
#32164=ORIENTED_EDGE('',*,*,#24327,.T.);
#32165=ORIENTED_EDGE('',*,*,#24328,.T.);
#32166=ORIENTED_EDGE('',*,*,#24329,.T.);
#32167=ORIENTED_EDGE('',*,*,#24330,.T.);
#32168=ORIENTED_EDGE('',*,*,#24331,.F.);
#32169=ORIENTED_EDGE('',*,*,#24332,.T.);
#32170=ORIENTED_EDGE('',*,*,#24333,.T.);
#32171=ORIENTED_EDGE('',*,*,#24331,.T.);
#32172=ORIENTED_EDGE('',*,*,#24334,.T.);
#32173=ORIENTED_EDGE('',*,*,#24325,.F.);
#32174=ORIENTED_EDGE('',*,*,#24335,.T.);
#32175=ORIENTED_EDGE('',*,*,#24336,.F.);
#32176=ORIENTED_EDGE('',*,*,#24337,.T.);
#32177=ORIENTED_EDGE('',*,*,#24328,.F.);
#32178=ORIENTED_EDGE('',*,*,#24338,.T.);
#32179=ORIENTED_EDGE('',*,*,#24339,.T.);
#32180=ORIENTED_EDGE('',*,*,#24340,.T.);
#32181=ORIENTED_EDGE('',*,*,#24336,.T.);
#32182=ORIENTED_EDGE('',*,*,#24341,.T.);
#32183=ORIENTED_EDGE('',*,*,#24342,.T.);
#32184=ORIENTED_EDGE('',*,*,#24343,.T.);
#32185=ORIENTED_EDGE('',*,*,#24344,.T.);
#32186=ORIENTED_EDGE('',*,*,#24345,.F.);
#32187=ORIENTED_EDGE('',*,*,#24346,.T.);
#32188=ORIENTED_EDGE('',*,*,#24347,.T.);
#32189=ORIENTED_EDGE('',*,*,#24345,.T.);
#32190=ORIENTED_EDGE('',*,*,#24348,.T.);
#32191=ORIENTED_EDGE('',*,*,#24339,.F.);
#32192=ORIENTED_EDGE('',*,*,#24349,.T.);
#32193=ORIENTED_EDGE('',*,*,#24350,.F.);
#32194=ORIENTED_EDGE('',*,*,#24351,.T.);
#32195=ORIENTED_EDGE('',*,*,#24342,.F.);
#32196=ORIENTED_EDGE('',*,*,#24352,.T.);
#32197=ORIENTED_EDGE('',*,*,#24353,.T.);
#32198=ORIENTED_EDGE('',*,*,#24354,.T.);
#32199=ORIENTED_EDGE('',*,*,#24350,.T.);
#32200=ORIENTED_EDGE('',*,*,#24355,.T.);
#32201=ORIENTED_EDGE('',*,*,#24356,.T.);
#32202=ORIENTED_EDGE('',*,*,#24357,.T.);
#32203=ORIENTED_EDGE('',*,*,#24358,.T.);
#32204=ORIENTED_EDGE('',*,*,#24359,.F.);
#32205=ORIENTED_EDGE('',*,*,#24360,.T.);
#32206=ORIENTED_EDGE('',*,*,#24361,.T.);
#32207=ORIENTED_EDGE('',*,*,#24359,.T.);
#32208=ORIENTED_EDGE('',*,*,#24362,.T.);
#32209=ORIENTED_EDGE('',*,*,#24353,.F.);
#32210=ORIENTED_EDGE('',*,*,#24363,.T.);
#32211=ORIENTED_EDGE('',*,*,#21778,.F.);
#32212=ORIENTED_EDGE('',*,*,#24364,.T.);
#32213=ORIENTED_EDGE('',*,*,#24356,.F.);
#32214=ORIENTED_EDGE('',*,*,#24365,.T.);
#32215=ORIENTED_EDGE('',*,*,#21775,.F.);
#32216=ORIENTED_EDGE('',*,*,#24366,.T.);
#32217=ORIENTED_EDGE('',*,*,#24367,.T.);
#32218=ORIENTED_EDGE('',*,*,#24368,.F.);
#32219=ORIENTED_EDGE('',*,*,#24368,.T.);
#32220=ORIENTED_EDGE('',*,*,#24369,.T.);
#32221=ORIENTED_EDGE('',*,*,#21776,.F.);
#32222=ORIENTED_EDGE('',*,*,#24370,.T.);
#32223=ORIENTED_EDGE('',*,*,#24371,.T.);
#32224=ORIENTED_EDGE('',*,*,#21367,.F.);
#32225=ORIENTED_EDGE('',*,*,#24372,.F.);
#32226=ORIENTED_EDGE('',*,*,#24373,.T.);
#32227=ORIENTED_EDGE('',*,*,#24374,.T.);
#32228=ORIENTED_EDGE('',*,*,#24375,.F.);
#32229=ORIENTED_EDGE('',*,*,#24376,.T.);
#32230=ORIENTED_EDGE('',*,*,#24370,.F.);
#32231=ORIENTED_EDGE('',*,*,#24377,.T.);
#32232=ORIENTED_EDGE('',*,*,#24378,.T.);
#32233=ORIENTED_EDGE('',*,*,#24379,.T.);
#32234=ORIENTED_EDGE('',*,*,#24375,.T.);
#32235=ORIENTED_EDGE('',*,*,#24380,.T.);
#32236=ORIENTED_EDGE('',*,*,#24381,.T.);
#32237=ORIENTED_EDGE('',*,*,#24382,.T.);
#32238=ORIENTED_EDGE('',*,*,#24383,.T.);
#32239=ORIENTED_EDGE('',*,*,#24384,.F.);
#32240=ORIENTED_EDGE('',*,*,#24385,.T.);
#32241=ORIENTED_EDGE('',*,*,#24386,.T.);
#32242=ORIENTED_EDGE('',*,*,#24384,.T.);
#32243=ORIENTED_EDGE('',*,*,#24387,.T.);
#32244=ORIENTED_EDGE('',*,*,#24378,.F.);
#32245=ORIENTED_EDGE('',*,*,#24388,.T.);
#32246=ORIENTED_EDGE('',*,*,#21370,.F.);
#32247=ORIENTED_EDGE('',*,*,#24389,.T.);
#32248=ORIENTED_EDGE('',*,*,#24276,.T.);
#32249=ORIENTED_EDGE('',*,*,#24390,.F.);
#32250=ORIENTED_EDGE('',*,*,#24391,.T.);
#32251=ORIENTED_EDGE('',*,*,#24381,.F.);
#32252=ORIENTED_EDGE('',*,*,#24392,.T.);
#32253=ORIENTED_EDGE('',*,*,#24393,.T.);
#32254=ORIENTED_EDGE('',*,*,#24394,.T.);
#32255=ORIENTED_EDGE('',*,*,#24390,.T.);
#32256=ORIENTED_EDGE('',*,*,#24395,.T.);
#32257=ORIENTED_EDGE('',*,*,#24396,.T.);
#32258=ORIENTED_EDGE('',*,*,#24397,.T.);
#32259=ORIENTED_EDGE('',*,*,#24398,.T.);
#32260=ORIENTED_EDGE('',*,*,#24399,.F.);
#32261=ORIENTED_EDGE('',*,*,#24400,.T.);
#32262=ORIENTED_EDGE('',*,*,#24401,.T.);
#32263=ORIENTED_EDGE('',*,*,#24399,.T.);
#32264=ORIENTED_EDGE('',*,*,#24402,.T.);
#32265=ORIENTED_EDGE('',*,*,#24393,.F.);
#32266=ORIENTED_EDGE('',*,*,#24403,.T.);
#32267=ORIENTED_EDGE('',*,*,#24404,.F.);
#32268=ORIENTED_EDGE('',*,*,#24405,.T.);
#32269=ORIENTED_EDGE('',*,*,#24396,.F.);
#32270=ORIENTED_EDGE('',*,*,#24406,.T.);
#32271=ORIENTED_EDGE('',*,*,#24407,.T.);
#32272=ORIENTED_EDGE('',*,*,#24408,.T.);
#32273=ORIENTED_EDGE('',*,*,#24404,.T.);
#32274=ORIENTED_EDGE('',*,*,#24409,.T.);
#32275=ORIENTED_EDGE('',*,*,#24410,.T.);
#32276=ORIENTED_EDGE('',*,*,#24411,.T.);
#32277=ORIENTED_EDGE('',*,*,#24412,.T.);
#32278=ORIENTED_EDGE('',*,*,#24413,.F.);
#32279=ORIENTED_EDGE('',*,*,#24414,.T.);
#32280=ORIENTED_EDGE('',*,*,#24415,.T.);
#32281=ORIENTED_EDGE('',*,*,#24413,.T.);
#32282=ORIENTED_EDGE('',*,*,#24416,.T.);
#32283=ORIENTED_EDGE('',*,*,#24407,.F.);
#32284=ORIENTED_EDGE('',*,*,#24417,.T.);
#32285=ORIENTED_EDGE('',*,*,#24418,.F.);
#32286=ORIENTED_EDGE('',*,*,#24419,.T.);
#32287=ORIENTED_EDGE('',*,*,#24410,.F.);
#32288=ORIENTED_EDGE('',*,*,#24420,.T.);
#32289=ORIENTED_EDGE('',*,*,#24421,.T.);
#32290=ORIENTED_EDGE('',*,*,#24422,.T.);
#32291=ORIENTED_EDGE('',*,*,#24418,.T.);
#32292=ORIENTED_EDGE('',*,*,#24423,.T.);
#32293=ORIENTED_EDGE('',*,*,#24424,.T.);
#32294=ORIENTED_EDGE('',*,*,#24425,.T.);
#32295=ORIENTED_EDGE('',*,*,#24426,.T.);
#32296=ORIENTED_EDGE('',*,*,#24427,.F.);
#32297=ORIENTED_EDGE('',*,*,#24428,.T.);
#32298=ORIENTED_EDGE('',*,*,#24429,.T.);
#32299=ORIENTED_EDGE('',*,*,#24427,.T.);
#32300=ORIENTED_EDGE('',*,*,#24430,.T.);
#32301=ORIENTED_EDGE('',*,*,#24421,.F.);
#32302=ORIENTED_EDGE('',*,*,#24431,.T.);
#32303=ORIENTED_EDGE('',*,*,#24432,.F.);
#32304=ORIENTED_EDGE('',*,*,#24433,.T.);
#32305=ORIENTED_EDGE('',*,*,#24424,.F.);
#32306=ORIENTED_EDGE('',*,*,#24434,.T.);
#32307=ORIENTED_EDGE('',*,*,#24435,.T.);
#32308=ORIENTED_EDGE('',*,*,#24436,.T.);
#32309=ORIENTED_EDGE('',*,*,#24432,.T.);
#32310=ORIENTED_EDGE('',*,*,#24437,.T.);
#32311=ORIENTED_EDGE('',*,*,#24438,.T.);
#32312=ORIENTED_EDGE('',*,*,#24439,.T.);
#32313=ORIENTED_EDGE('',*,*,#24440,.T.);
#32314=ORIENTED_EDGE('',*,*,#24441,.F.);
#32315=ORIENTED_EDGE('',*,*,#24442,.T.);
#32316=ORIENTED_EDGE('',*,*,#24443,.T.);
#32317=ORIENTED_EDGE('',*,*,#24441,.T.);
#32318=ORIENTED_EDGE('',*,*,#24444,.T.);
#32319=ORIENTED_EDGE('',*,*,#24435,.F.);
#32320=ORIENTED_EDGE('',*,*,#24445,.T.);
#32321=ORIENTED_EDGE('',*,*,#24446,.F.);
#32322=ORIENTED_EDGE('',*,*,#24447,.T.);
#32323=ORIENTED_EDGE('',*,*,#24438,.F.);
#32324=ORIENTED_EDGE('',*,*,#24448,.T.);
#32325=ORIENTED_EDGE('',*,*,#24449,.T.);
#32326=ORIENTED_EDGE('',*,*,#24450,.T.);
#32327=ORIENTED_EDGE('',*,*,#24446,.T.);
#32328=ORIENTED_EDGE('',*,*,#24451,.T.);
#32329=ORIENTED_EDGE('',*,*,#24452,.T.);
#32330=ORIENTED_EDGE('',*,*,#24453,.T.);
#32331=ORIENTED_EDGE('',*,*,#24454,.T.);
#32332=ORIENTED_EDGE('',*,*,#24455,.F.);
#32333=ORIENTED_EDGE('',*,*,#24456,.T.);
#32334=ORIENTED_EDGE('',*,*,#24457,.T.);
#32335=ORIENTED_EDGE('',*,*,#24455,.T.);
#32336=ORIENTED_EDGE('',*,*,#24458,.T.);
#32337=ORIENTED_EDGE('',*,*,#24449,.F.);
#32338=ORIENTED_EDGE('',*,*,#24459,.T.);
#32339=ORIENTED_EDGE('',*,*,#21484,.F.);
#32340=ORIENTED_EDGE('',*,*,#24460,.T.);
#32341=ORIENTED_EDGE('',*,*,#24452,.F.);
#32342=ORIENTED_EDGE('',*,*,#24461,.T.);
#32343=ORIENTED_EDGE('',*,*,#21781,.F.);
#32344=ORIENTED_EDGE('',*,*,#24462,.T.);
#32345=ORIENTED_EDGE('',*,*,#24463,.T.);
#32346=ORIENTED_EDGE('',*,*,#24464,.F.);
#32347=ORIENTED_EDGE('',*,*,#24464,.T.);
#32348=ORIENTED_EDGE('',*,*,#24465,.T.);
#32349=ORIENTED_EDGE('',*,*,#21782,.F.);
#32350=ORIENTED_EDGE('',*,*,#24466,.T.);
#32351=ORIENTED_EDGE('',*,*,#24467,.T.);
#32352=ORIENTED_EDGE('',*,*,#21363,.F.);
#32353=ORIENTED_EDGE('',*,*,#24468,.F.);
#32354=ORIENTED_EDGE('',*,*,#24469,.T.);
#32355=ORIENTED_EDGE('',*,*,#24470,.T.);
#32356=ORIENTED_EDGE('',*,*,#24471,.F.);
#32357=ORIENTED_EDGE('',*,*,#24472,.T.);
#32358=ORIENTED_EDGE('',*,*,#24466,.F.);
#32359=ORIENTED_EDGE('',*,*,#24473,.T.);
#32360=ORIENTED_EDGE('',*,*,#24474,.T.);
#32361=ORIENTED_EDGE('',*,*,#24475,.T.);
#32362=ORIENTED_EDGE('',*,*,#24471,.T.);
#32363=ORIENTED_EDGE('',*,*,#24476,.T.);
#32364=ORIENTED_EDGE('',*,*,#24477,.T.);
#32365=ORIENTED_EDGE('',*,*,#24478,.T.);
#32366=ORIENTED_EDGE('',*,*,#24479,.T.);
#32367=ORIENTED_EDGE('',*,*,#24480,.F.);
#32368=ORIENTED_EDGE('',*,*,#24481,.T.);
#32369=ORIENTED_EDGE('',*,*,#24482,.T.);
#32370=ORIENTED_EDGE('',*,*,#24480,.T.);
#32371=ORIENTED_EDGE('',*,*,#24483,.T.);
#32372=ORIENTED_EDGE('',*,*,#24474,.F.);
#32373=ORIENTED_EDGE('',*,*,#24484,.T.);
#32374=ORIENTED_EDGE('',*,*,#21366,.F.);
#32375=ORIENTED_EDGE('',*,*,#24485,.T.);
#32376=ORIENTED_EDGE('',*,*,#24372,.T.);
#32377=ORIENTED_EDGE('',*,*,#24486,.F.);
#32378=ORIENTED_EDGE('',*,*,#24487,.T.);
#32379=ORIENTED_EDGE('',*,*,#24477,.F.);
#32380=ORIENTED_EDGE('',*,*,#24488,.T.);
#32381=ORIENTED_EDGE('',*,*,#24489,.T.);
#32382=ORIENTED_EDGE('',*,*,#24490,.T.);
#32383=ORIENTED_EDGE('',*,*,#24486,.T.);
#32384=ORIENTED_EDGE('',*,*,#24491,.T.);
#32385=ORIENTED_EDGE('',*,*,#24492,.T.);
#32386=ORIENTED_EDGE('',*,*,#24493,.T.);
#32387=ORIENTED_EDGE('',*,*,#24494,.T.);
#32388=ORIENTED_EDGE('',*,*,#24495,.F.);
#32389=ORIENTED_EDGE('',*,*,#24496,.T.);
#32390=ORIENTED_EDGE('',*,*,#24497,.T.);
#32391=ORIENTED_EDGE('',*,*,#24495,.T.);
#32392=ORIENTED_EDGE('',*,*,#24498,.T.);
#32393=ORIENTED_EDGE('',*,*,#24489,.F.);
#32394=ORIENTED_EDGE('',*,*,#24499,.T.);
#32395=ORIENTED_EDGE('',*,*,#24500,.F.);
#32396=ORIENTED_EDGE('',*,*,#24501,.T.);
#32397=ORIENTED_EDGE('',*,*,#24492,.F.);
#32398=ORIENTED_EDGE('',*,*,#24502,.T.);
#32399=ORIENTED_EDGE('',*,*,#24503,.T.);
#32400=ORIENTED_EDGE('',*,*,#24504,.T.);
#32401=ORIENTED_EDGE('',*,*,#24500,.T.);
#32402=ORIENTED_EDGE('',*,*,#24505,.T.);
#32403=ORIENTED_EDGE('',*,*,#24506,.T.);
#32404=ORIENTED_EDGE('',*,*,#24507,.T.);
#32405=ORIENTED_EDGE('',*,*,#24508,.T.);
#32406=ORIENTED_EDGE('',*,*,#24509,.F.);
#32407=ORIENTED_EDGE('',*,*,#24510,.T.);
#32408=ORIENTED_EDGE('',*,*,#24511,.T.);
#32409=ORIENTED_EDGE('',*,*,#24509,.T.);
#32410=ORIENTED_EDGE('',*,*,#24512,.T.);
#32411=ORIENTED_EDGE('',*,*,#24503,.F.);
#32412=ORIENTED_EDGE('',*,*,#24513,.T.);
#32413=ORIENTED_EDGE('',*,*,#24514,.F.);
#32414=ORIENTED_EDGE('',*,*,#24515,.T.);
#32415=ORIENTED_EDGE('',*,*,#24506,.F.);
#32416=ORIENTED_EDGE('',*,*,#24516,.T.);
#32417=ORIENTED_EDGE('',*,*,#24517,.T.);
#32418=ORIENTED_EDGE('',*,*,#24518,.T.);
#32419=ORIENTED_EDGE('',*,*,#24514,.T.);
#32420=ORIENTED_EDGE('',*,*,#24519,.T.);
#32421=ORIENTED_EDGE('',*,*,#24520,.T.);
#32422=ORIENTED_EDGE('',*,*,#24521,.T.);
#32423=ORIENTED_EDGE('',*,*,#24522,.T.);
#32424=ORIENTED_EDGE('',*,*,#24523,.F.);
#32425=ORIENTED_EDGE('',*,*,#24524,.T.);
#32426=ORIENTED_EDGE('',*,*,#24525,.T.);
#32427=ORIENTED_EDGE('',*,*,#24523,.T.);
#32428=ORIENTED_EDGE('',*,*,#24526,.T.);
#32429=ORIENTED_EDGE('',*,*,#24517,.F.);
#32430=ORIENTED_EDGE('',*,*,#24527,.T.);
#32431=ORIENTED_EDGE('',*,*,#24528,.F.);
#32432=ORIENTED_EDGE('',*,*,#24529,.T.);
#32433=ORIENTED_EDGE('',*,*,#24520,.F.);
#32434=ORIENTED_EDGE('',*,*,#24530,.T.);
#32435=ORIENTED_EDGE('',*,*,#24531,.T.);
#32436=ORIENTED_EDGE('',*,*,#24532,.T.);
#32437=ORIENTED_EDGE('',*,*,#24528,.T.);
#32438=ORIENTED_EDGE('',*,*,#24533,.T.);
#32439=ORIENTED_EDGE('',*,*,#24534,.T.);
#32440=ORIENTED_EDGE('',*,*,#24535,.T.);
#32441=ORIENTED_EDGE('',*,*,#24536,.T.);
#32442=ORIENTED_EDGE('',*,*,#24537,.F.);
#32443=ORIENTED_EDGE('',*,*,#24538,.T.);
#32444=ORIENTED_EDGE('',*,*,#24539,.T.);
#32445=ORIENTED_EDGE('',*,*,#24537,.T.);
#32446=ORIENTED_EDGE('',*,*,#24540,.T.);
#32447=ORIENTED_EDGE('',*,*,#24531,.F.);
#32448=ORIENTED_EDGE('',*,*,#24541,.T.);
#32449=ORIENTED_EDGE('',*,*,#24542,.F.);
#32450=ORIENTED_EDGE('',*,*,#24543,.T.);
#32451=ORIENTED_EDGE('',*,*,#24534,.F.);
#32452=ORIENTED_EDGE('',*,*,#24544,.T.);
#32453=ORIENTED_EDGE('',*,*,#24545,.T.);
#32454=ORIENTED_EDGE('',*,*,#24546,.T.);
#32455=ORIENTED_EDGE('',*,*,#24542,.T.);
#32456=ORIENTED_EDGE('',*,*,#24547,.T.);
#32457=ORIENTED_EDGE('',*,*,#24548,.T.);
#32458=ORIENTED_EDGE('',*,*,#24549,.T.);
#32459=ORIENTED_EDGE('',*,*,#24550,.T.);
#32460=ORIENTED_EDGE('',*,*,#24551,.F.);
#32461=ORIENTED_EDGE('',*,*,#24552,.T.);
#32462=ORIENTED_EDGE('',*,*,#24553,.T.);
#32463=ORIENTED_EDGE('',*,*,#24551,.T.);
#32464=ORIENTED_EDGE('',*,*,#24554,.T.);
#32465=ORIENTED_EDGE('',*,*,#24545,.F.);
#32466=ORIENTED_EDGE('',*,*,#24555,.T.);
#32467=ORIENTED_EDGE('',*,*,#21490,.F.);
#32468=ORIENTED_EDGE('',*,*,#24556,.T.);
#32469=ORIENTED_EDGE('',*,*,#24548,.F.);
#32470=ORIENTED_EDGE('',*,*,#24557,.T.);
#32471=ORIENTED_EDGE('',*,*,#21487,.F.);
#32472=ORIENTED_EDGE('',*,*,#24558,.T.);
#32473=ORIENTED_EDGE('',*,*,#24559,.T.);
#32474=ORIENTED_EDGE('',*,*,#24560,.F.);
#32475=ORIENTED_EDGE('',*,*,#24560,.T.);
#32476=ORIENTED_EDGE('',*,*,#24561,.T.);
#32477=ORIENTED_EDGE('',*,*,#21488,.F.);
#32478=ORIENTED_EDGE('',*,*,#24562,.T.);
#32479=ORIENTED_EDGE('',*,*,#24563,.T.);
#32480=ORIENTED_EDGE('',*,*,#21359,.F.);
#32481=ORIENTED_EDGE('',*,*,#24564,.F.);
#32482=ORIENTED_EDGE('',*,*,#24565,.T.);
#32483=ORIENTED_EDGE('',*,*,#24566,.T.);
#32484=ORIENTED_EDGE('',*,*,#24567,.F.);
#32485=ORIENTED_EDGE('',*,*,#24568,.T.);
#32486=ORIENTED_EDGE('',*,*,#24562,.F.);
#32487=ORIENTED_EDGE('',*,*,#24569,.T.);
#32488=ORIENTED_EDGE('',*,*,#24570,.T.);
#32489=ORIENTED_EDGE('',*,*,#24571,.T.);
#32490=ORIENTED_EDGE('',*,*,#24567,.T.);
#32491=ORIENTED_EDGE('',*,*,#24572,.T.);
#32492=ORIENTED_EDGE('',*,*,#24573,.T.);
#32493=ORIENTED_EDGE('',*,*,#24574,.T.);
#32494=ORIENTED_EDGE('',*,*,#24575,.T.);
#32495=ORIENTED_EDGE('',*,*,#24576,.F.);
#32496=ORIENTED_EDGE('',*,*,#24577,.T.);
#32497=ORIENTED_EDGE('',*,*,#24578,.T.);
#32498=ORIENTED_EDGE('',*,*,#24576,.T.);
#32499=ORIENTED_EDGE('',*,*,#24579,.T.);
#32500=ORIENTED_EDGE('',*,*,#24570,.F.);
#32501=ORIENTED_EDGE('',*,*,#24580,.T.);
#32502=ORIENTED_EDGE('',*,*,#21362,.F.);
#32503=ORIENTED_EDGE('',*,*,#24581,.T.);
#32504=ORIENTED_EDGE('',*,*,#24468,.T.);
#32505=ORIENTED_EDGE('',*,*,#24582,.F.);
#32506=ORIENTED_EDGE('',*,*,#24583,.T.);
#32507=ORIENTED_EDGE('',*,*,#24573,.F.);
#32508=ORIENTED_EDGE('',*,*,#24584,.T.);
#32509=ORIENTED_EDGE('',*,*,#24585,.T.);
#32510=ORIENTED_EDGE('',*,*,#24586,.T.);
#32511=ORIENTED_EDGE('',*,*,#24582,.T.);
#32512=ORIENTED_EDGE('',*,*,#24587,.T.);
#32513=ORIENTED_EDGE('',*,*,#24588,.T.);
#32514=ORIENTED_EDGE('',*,*,#24589,.T.);
#32515=ORIENTED_EDGE('',*,*,#24590,.T.);
#32516=ORIENTED_EDGE('',*,*,#24591,.F.);
#32517=ORIENTED_EDGE('',*,*,#24592,.T.);
#32518=ORIENTED_EDGE('',*,*,#24593,.T.);
#32519=ORIENTED_EDGE('',*,*,#24591,.T.);
#32520=ORIENTED_EDGE('',*,*,#24594,.T.);
#32521=ORIENTED_EDGE('',*,*,#24585,.F.);
#32522=ORIENTED_EDGE('',*,*,#24595,.T.);
#32523=ORIENTED_EDGE('',*,*,#24596,.F.);
#32524=ORIENTED_EDGE('',*,*,#24597,.T.);
#32525=ORIENTED_EDGE('',*,*,#24588,.F.);
#32526=ORIENTED_EDGE('',*,*,#24598,.T.);
#32527=ORIENTED_EDGE('',*,*,#24599,.T.);
#32528=ORIENTED_EDGE('',*,*,#24600,.T.);
#32529=ORIENTED_EDGE('',*,*,#24596,.T.);
#32530=ORIENTED_EDGE('',*,*,#24601,.T.);
#32531=ORIENTED_EDGE('',*,*,#24602,.T.);
#32532=ORIENTED_EDGE('',*,*,#24603,.T.);
#32533=ORIENTED_EDGE('',*,*,#24604,.T.);
#32534=ORIENTED_EDGE('',*,*,#24605,.F.);
#32535=ORIENTED_EDGE('',*,*,#24606,.T.);
#32536=ORIENTED_EDGE('',*,*,#24607,.T.);
#32537=ORIENTED_EDGE('',*,*,#24605,.T.);
#32538=ORIENTED_EDGE('',*,*,#24608,.T.);
#32539=ORIENTED_EDGE('',*,*,#24599,.F.);
#32540=ORIENTED_EDGE('',*,*,#24609,.T.);
#32541=ORIENTED_EDGE('',*,*,#24610,.F.);
#32542=ORIENTED_EDGE('',*,*,#24611,.T.);
#32543=ORIENTED_EDGE('',*,*,#24602,.F.);
#32544=ORIENTED_EDGE('',*,*,#24612,.T.);
#32545=ORIENTED_EDGE('',*,*,#24613,.T.);
#32546=ORIENTED_EDGE('',*,*,#24614,.T.);
#32547=ORIENTED_EDGE('',*,*,#24610,.T.);
#32548=ORIENTED_EDGE('',*,*,#24615,.T.);
#32549=ORIENTED_EDGE('',*,*,#24616,.T.);
#32550=ORIENTED_EDGE('',*,*,#24617,.T.);
#32551=ORIENTED_EDGE('',*,*,#24618,.T.);
#32552=ORIENTED_EDGE('',*,*,#24619,.F.);
#32553=ORIENTED_EDGE('',*,*,#24620,.T.);
#32554=ORIENTED_EDGE('',*,*,#24621,.T.);
#32555=ORIENTED_EDGE('',*,*,#24619,.T.);
#32556=ORIENTED_EDGE('',*,*,#24622,.T.);
#32557=ORIENTED_EDGE('',*,*,#24613,.F.);
#32558=ORIENTED_EDGE('',*,*,#24623,.T.);
#32559=ORIENTED_EDGE('',*,*,#24624,.F.);
#32560=ORIENTED_EDGE('',*,*,#24625,.T.);
#32561=ORIENTED_EDGE('',*,*,#24616,.F.);
#32562=ORIENTED_EDGE('',*,*,#24626,.T.);
#32563=ORIENTED_EDGE('',*,*,#24627,.T.);
#32564=ORIENTED_EDGE('',*,*,#24628,.T.);
#32565=ORIENTED_EDGE('',*,*,#24624,.T.);
#32566=ORIENTED_EDGE('',*,*,#24629,.T.);
#32567=ORIENTED_EDGE('',*,*,#24630,.T.);
#32568=ORIENTED_EDGE('',*,*,#24631,.T.);
#32569=ORIENTED_EDGE('',*,*,#24632,.T.);
#32570=ORIENTED_EDGE('',*,*,#24633,.F.);
#32571=ORIENTED_EDGE('',*,*,#24634,.T.);
#32572=ORIENTED_EDGE('',*,*,#24635,.T.);
#32573=ORIENTED_EDGE('',*,*,#24633,.T.);
#32574=ORIENTED_EDGE('',*,*,#24636,.T.);
#32575=ORIENTED_EDGE('',*,*,#24627,.F.);
#32576=ORIENTED_EDGE('',*,*,#24637,.T.);
#32577=ORIENTED_EDGE('',*,*,#24638,.F.);
#32578=ORIENTED_EDGE('',*,*,#24639,.T.);
#32579=ORIENTED_EDGE('',*,*,#24630,.F.);
#32580=ORIENTED_EDGE('',*,*,#24640,.T.);
#32581=ORIENTED_EDGE('',*,*,#24641,.T.);
#32582=ORIENTED_EDGE('',*,*,#24642,.T.);
#32583=ORIENTED_EDGE('',*,*,#24638,.T.);
#32584=ORIENTED_EDGE('',*,*,#24643,.T.);
#32585=ORIENTED_EDGE('',*,*,#24644,.T.);
#32586=ORIENTED_EDGE('',*,*,#24645,.T.);
#32587=ORIENTED_EDGE('',*,*,#24646,.T.);
#32588=ORIENTED_EDGE('',*,*,#24647,.F.);
#32589=ORIENTED_EDGE('',*,*,#24648,.T.);
#32590=ORIENTED_EDGE('',*,*,#24649,.T.);
#32591=ORIENTED_EDGE('',*,*,#24647,.T.);
#32592=ORIENTED_EDGE('',*,*,#24650,.T.);
#32593=ORIENTED_EDGE('',*,*,#24641,.F.);
#32594=ORIENTED_EDGE('',*,*,#24651,.T.);
#32595=ORIENTED_EDGE('',*,*,#21496,.F.);
#32596=ORIENTED_EDGE('',*,*,#24652,.T.);
#32597=ORIENTED_EDGE('',*,*,#24644,.F.);
#32598=ORIENTED_EDGE('',*,*,#24653,.T.);
#32599=ORIENTED_EDGE('',*,*,#21493,.F.);
#32600=ORIENTED_EDGE('',*,*,#24654,.T.);
#32601=ORIENTED_EDGE('',*,*,#24655,.T.);
#32602=ORIENTED_EDGE('',*,*,#24656,.F.);
#32603=ORIENTED_EDGE('',*,*,#24656,.T.);
#32604=ORIENTED_EDGE('',*,*,#24657,.T.);
#32605=ORIENTED_EDGE('',*,*,#21494,.F.);
#32606=ORIENTED_EDGE('',*,*,#24658,.T.);
#32607=ORIENTED_EDGE('',*,*,#24659,.T.);
#32608=ORIENTED_EDGE('',*,*,#21355,.F.);
#32609=ORIENTED_EDGE('',*,*,#24660,.F.);
#32610=ORIENTED_EDGE('',*,*,#24661,.T.);
#32611=ORIENTED_EDGE('',*,*,#24662,.T.);
#32612=ORIENTED_EDGE('',*,*,#24663,.F.);
#32613=ORIENTED_EDGE('',*,*,#24664,.T.);
#32614=ORIENTED_EDGE('',*,*,#24658,.F.);
#32615=ORIENTED_EDGE('',*,*,#24665,.T.);
#32616=ORIENTED_EDGE('',*,*,#24666,.T.);
#32617=ORIENTED_EDGE('',*,*,#24667,.T.);
#32618=ORIENTED_EDGE('',*,*,#24663,.T.);
#32619=ORIENTED_EDGE('',*,*,#24668,.T.);
#32620=ORIENTED_EDGE('',*,*,#24669,.T.);
#32621=ORIENTED_EDGE('',*,*,#24670,.T.);
#32622=ORIENTED_EDGE('',*,*,#24671,.T.);
#32623=ORIENTED_EDGE('',*,*,#24672,.F.);
#32624=ORIENTED_EDGE('',*,*,#24673,.T.);
#32625=ORIENTED_EDGE('',*,*,#24674,.T.);
#32626=ORIENTED_EDGE('',*,*,#24672,.T.);
#32627=ORIENTED_EDGE('',*,*,#24675,.T.);
#32628=ORIENTED_EDGE('',*,*,#24666,.F.);
#32629=ORIENTED_EDGE('',*,*,#24676,.T.);
#32630=ORIENTED_EDGE('',*,*,#21358,.F.);
#32631=ORIENTED_EDGE('',*,*,#24677,.T.);
#32632=ORIENTED_EDGE('',*,*,#24564,.T.);
#32633=ORIENTED_EDGE('',*,*,#24678,.F.);
#32634=ORIENTED_EDGE('',*,*,#24679,.T.);
#32635=ORIENTED_EDGE('',*,*,#24669,.F.);
#32636=ORIENTED_EDGE('',*,*,#24680,.T.);
#32637=ORIENTED_EDGE('',*,*,#24681,.T.);
#32638=ORIENTED_EDGE('',*,*,#24682,.T.);
#32639=ORIENTED_EDGE('',*,*,#24678,.T.);
#32640=ORIENTED_EDGE('',*,*,#24683,.T.);
#32641=ORIENTED_EDGE('',*,*,#24684,.T.);
#32642=ORIENTED_EDGE('',*,*,#24685,.T.);
#32643=ORIENTED_EDGE('',*,*,#24686,.T.);
#32644=ORIENTED_EDGE('',*,*,#24687,.F.);
#32645=ORIENTED_EDGE('',*,*,#24688,.T.);
#32646=ORIENTED_EDGE('',*,*,#24689,.T.);
#32647=ORIENTED_EDGE('',*,*,#24687,.T.);
#32648=ORIENTED_EDGE('',*,*,#24690,.T.);
#32649=ORIENTED_EDGE('',*,*,#24681,.F.);
#32650=ORIENTED_EDGE('',*,*,#24691,.T.);
#32651=ORIENTED_EDGE('',*,*,#24692,.F.);
#32652=ORIENTED_EDGE('',*,*,#24693,.T.);
#32653=ORIENTED_EDGE('',*,*,#24684,.F.);
#32654=ORIENTED_EDGE('',*,*,#24694,.T.);
#32655=ORIENTED_EDGE('',*,*,#24695,.T.);
#32656=ORIENTED_EDGE('',*,*,#24696,.T.);
#32657=ORIENTED_EDGE('',*,*,#24692,.T.);
#32658=ORIENTED_EDGE('',*,*,#24697,.T.);
#32659=ORIENTED_EDGE('',*,*,#24698,.T.);
#32660=ORIENTED_EDGE('',*,*,#24699,.T.);
#32661=ORIENTED_EDGE('',*,*,#24700,.T.);
#32662=ORIENTED_EDGE('',*,*,#24701,.F.);
#32663=ORIENTED_EDGE('',*,*,#24702,.T.);
#32664=ORIENTED_EDGE('',*,*,#24703,.T.);
#32665=ORIENTED_EDGE('',*,*,#24701,.T.);
#32666=ORIENTED_EDGE('',*,*,#24704,.T.);
#32667=ORIENTED_EDGE('',*,*,#24695,.F.);
#32668=ORIENTED_EDGE('',*,*,#24705,.T.);
#32669=ORIENTED_EDGE('',*,*,#24706,.F.);
#32670=ORIENTED_EDGE('',*,*,#24707,.T.);
#32671=ORIENTED_EDGE('',*,*,#24698,.F.);
#32672=ORIENTED_EDGE('',*,*,#24708,.T.);
#32673=ORIENTED_EDGE('',*,*,#24709,.T.);
#32674=ORIENTED_EDGE('',*,*,#24710,.T.);
#32675=ORIENTED_EDGE('',*,*,#24706,.T.);
#32676=ORIENTED_EDGE('',*,*,#24711,.T.);
#32677=ORIENTED_EDGE('',*,*,#24712,.T.);
#32678=ORIENTED_EDGE('',*,*,#24713,.T.);
#32679=ORIENTED_EDGE('',*,*,#24714,.T.);
#32680=ORIENTED_EDGE('',*,*,#24715,.F.);
#32681=ORIENTED_EDGE('',*,*,#24716,.T.);
#32682=ORIENTED_EDGE('',*,*,#24717,.T.);
#32683=ORIENTED_EDGE('',*,*,#24715,.T.);
#32684=ORIENTED_EDGE('',*,*,#24718,.T.);
#32685=ORIENTED_EDGE('',*,*,#24709,.F.);
#32686=ORIENTED_EDGE('',*,*,#24719,.T.);
#32687=ORIENTED_EDGE('',*,*,#24720,.F.);
#32688=ORIENTED_EDGE('',*,*,#24721,.T.);
#32689=ORIENTED_EDGE('',*,*,#24712,.F.);
#32690=ORIENTED_EDGE('',*,*,#24722,.T.);
#32691=ORIENTED_EDGE('',*,*,#24723,.T.);
#32692=ORIENTED_EDGE('',*,*,#24724,.T.);
#32693=ORIENTED_EDGE('',*,*,#24720,.T.);
#32694=ORIENTED_EDGE('',*,*,#24725,.T.);
#32695=ORIENTED_EDGE('',*,*,#24726,.T.);
#32696=ORIENTED_EDGE('',*,*,#24727,.T.);
#32697=ORIENTED_EDGE('',*,*,#24728,.T.);
#32698=ORIENTED_EDGE('',*,*,#24729,.F.);
#32699=ORIENTED_EDGE('',*,*,#24730,.T.);
#32700=ORIENTED_EDGE('',*,*,#24731,.T.);
#32701=ORIENTED_EDGE('',*,*,#24729,.T.);
#32702=ORIENTED_EDGE('',*,*,#24732,.T.);
#32703=ORIENTED_EDGE('',*,*,#24723,.F.);
#32704=ORIENTED_EDGE('',*,*,#24733,.T.);
#32705=ORIENTED_EDGE('',*,*,#24734,.F.);
#32706=ORIENTED_EDGE('',*,*,#24735,.T.);
#32707=ORIENTED_EDGE('',*,*,#24726,.F.);
#32708=ORIENTED_EDGE('',*,*,#24736,.T.);
#32709=ORIENTED_EDGE('',*,*,#24737,.T.);
#32710=ORIENTED_EDGE('',*,*,#24738,.T.);
#32711=ORIENTED_EDGE('',*,*,#24734,.T.);
#32712=ORIENTED_EDGE('',*,*,#24739,.T.);
#32713=ORIENTED_EDGE('',*,*,#24740,.T.);
#32714=ORIENTED_EDGE('',*,*,#24741,.T.);
#32715=ORIENTED_EDGE('',*,*,#24742,.T.);
#32716=ORIENTED_EDGE('',*,*,#24743,.F.);
#32717=ORIENTED_EDGE('',*,*,#24744,.T.);
#32718=ORIENTED_EDGE('',*,*,#24745,.T.);
#32719=ORIENTED_EDGE('',*,*,#24743,.T.);
#32720=ORIENTED_EDGE('',*,*,#24746,.T.);
#32721=ORIENTED_EDGE('',*,*,#24737,.F.);
#32722=ORIENTED_EDGE('',*,*,#24747,.T.);
#32723=ORIENTED_EDGE('',*,*,#21502,.F.);
#32724=ORIENTED_EDGE('',*,*,#24748,.T.);
#32725=ORIENTED_EDGE('',*,*,#24740,.F.);
#32726=ORIENTED_EDGE('',*,*,#24749,.T.);
#32727=ORIENTED_EDGE('',*,*,#21499,.F.);
#32728=ORIENTED_EDGE('',*,*,#24750,.T.);
#32729=ORIENTED_EDGE('',*,*,#24751,.T.);
#32730=ORIENTED_EDGE('',*,*,#24752,.F.);
#32731=ORIENTED_EDGE('',*,*,#24752,.T.);
#32732=ORIENTED_EDGE('',*,*,#24753,.T.);
#32733=ORIENTED_EDGE('',*,*,#21500,.F.);
#32734=ORIENTED_EDGE('',*,*,#24754,.T.);
#32735=ORIENTED_EDGE('',*,*,#24755,.T.);
#32736=ORIENTED_EDGE('',*,*,#21351,.F.);
#32737=ORIENTED_EDGE('',*,*,#24756,.F.);
#32738=ORIENTED_EDGE('',*,*,#24757,.T.);
#32739=ORIENTED_EDGE('',*,*,#24758,.T.);
#32740=ORIENTED_EDGE('',*,*,#24759,.F.);
#32741=ORIENTED_EDGE('',*,*,#24760,.T.);
#32742=ORIENTED_EDGE('',*,*,#24754,.F.);
#32743=ORIENTED_EDGE('',*,*,#24761,.T.);
#32744=ORIENTED_EDGE('',*,*,#24762,.T.);
#32745=ORIENTED_EDGE('',*,*,#24763,.T.);
#32746=ORIENTED_EDGE('',*,*,#24759,.T.);
#32747=ORIENTED_EDGE('',*,*,#24764,.T.);
#32748=ORIENTED_EDGE('',*,*,#24765,.T.);
#32749=ORIENTED_EDGE('',*,*,#24766,.T.);
#32750=ORIENTED_EDGE('',*,*,#24767,.T.);
#32751=ORIENTED_EDGE('',*,*,#24768,.F.);
#32752=ORIENTED_EDGE('',*,*,#24769,.T.);
#32753=ORIENTED_EDGE('',*,*,#24770,.T.);
#32754=ORIENTED_EDGE('',*,*,#24768,.T.);
#32755=ORIENTED_EDGE('',*,*,#24771,.T.);
#32756=ORIENTED_EDGE('',*,*,#24762,.F.);
#32757=ORIENTED_EDGE('',*,*,#24772,.T.);
#32758=ORIENTED_EDGE('',*,*,#21354,.F.);
#32759=ORIENTED_EDGE('',*,*,#24773,.T.);
#32760=ORIENTED_EDGE('',*,*,#24660,.T.);
#32761=ORIENTED_EDGE('',*,*,#24774,.F.);
#32762=ORIENTED_EDGE('',*,*,#24775,.T.);
#32763=ORIENTED_EDGE('',*,*,#24765,.F.);
#32764=ORIENTED_EDGE('',*,*,#24776,.T.);
#32765=ORIENTED_EDGE('',*,*,#24777,.T.);
#32766=ORIENTED_EDGE('',*,*,#24778,.T.);
#32767=ORIENTED_EDGE('',*,*,#24774,.T.);
#32768=ORIENTED_EDGE('',*,*,#24779,.T.);
#32769=ORIENTED_EDGE('',*,*,#24780,.T.);
#32770=ORIENTED_EDGE('',*,*,#24781,.T.);
#32771=ORIENTED_EDGE('',*,*,#24782,.T.);
#32772=ORIENTED_EDGE('',*,*,#24783,.F.);
#32773=ORIENTED_EDGE('',*,*,#24784,.T.);
#32774=ORIENTED_EDGE('',*,*,#24785,.T.);
#32775=ORIENTED_EDGE('',*,*,#24783,.T.);
#32776=ORIENTED_EDGE('',*,*,#24786,.T.);
#32777=ORIENTED_EDGE('',*,*,#24777,.F.);
#32778=ORIENTED_EDGE('',*,*,#24787,.T.);
#32779=ORIENTED_EDGE('',*,*,#24788,.F.);
#32780=ORIENTED_EDGE('',*,*,#24789,.T.);
#32781=ORIENTED_EDGE('',*,*,#24780,.F.);
#32782=ORIENTED_EDGE('',*,*,#24790,.T.);
#32783=ORIENTED_EDGE('',*,*,#24791,.T.);
#32784=ORIENTED_EDGE('',*,*,#24792,.T.);
#32785=ORIENTED_EDGE('',*,*,#24788,.T.);
#32786=ORIENTED_EDGE('',*,*,#24793,.T.);
#32787=ORIENTED_EDGE('',*,*,#24794,.T.);
#32788=ORIENTED_EDGE('',*,*,#24795,.T.);
#32789=ORIENTED_EDGE('',*,*,#24796,.T.);
#32790=ORIENTED_EDGE('',*,*,#24797,.F.);
#32791=ORIENTED_EDGE('',*,*,#24798,.T.);
#32792=ORIENTED_EDGE('',*,*,#24799,.T.);
#32793=ORIENTED_EDGE('',*,*,#24797,.T.);
#32794=ORIENTED_EDGE('',*,*,#24800,.T.);
#32795=ORIENTED_EDGE('',*,*,#24791,.F.);
#32796=ORIENTED_EDGE('',*,*,#24801,.T.);
#32797=ORIENTED_EDGE('',*,*,#24802,.F.);
#32798=ORIENTED_EDGE('',*,*,#24803,.T.);
#32799=ORIENTED_EDGE('',*,*,#24794,.F.);
#32800=ORIENTED_EDGE('',*,*,#24804,.T.);
#32801=ORIENTED_EDGE('',*,*,#24805,.T.);
#32802=ORIENTED_EDGE('',*,*,#24806,.T.);
#32803=ORIENTED_EDGE('',*,*,#24802,.T.);
#32804=ORIENTED_EDGE('',*,*,#24807,.T.);
#32805=ORIENTED_EDGE('',*,*,#24808,.T.);
#32806=ORIENTED_EDGE('',*,*,#24809,.T.);
#32807=ORIENTED_EDGE('',*,*,#24810,.T.);
#32808=ORIENTED_EDGE('',*,*,#24811,.F.);
#32809=ORIENTED_EDGE('',*,*,#24812,.T.);
#32810=ORIENTED_EDGE('',*,*,#24813,.T.);
#32811=ORIENTED_EDGE('',*,*,#24811,.T.);
#32812=ORIENTED_EDGE('',*,*,#24814,.T.);
#32813=ORIENTED_EDGE('',*,*,#24805,.F.);
#32814=ORIENTED_EDGE('',*,*,#24815,.T.);
#32815=ORIENTED_EDGE('',*,*,#24816,.F.);
#32816=ORIENTED_EDGE('',*,*,#24817,.T.);
#32817=ORIENTED_EDGE('',*,*,#24808,.F.);
#32818=ORIENTED_EDGE('',*,*,#24818,.T.);
#32819=ORIENTED_EDGE('',*,*,#24819,.T.);
#32820=ORIENTED_EDGE('',*,*,#24820,.T.);
#32821=ORIENTED_EDGE('',*,*,#24816,.T.);
#32822=ORIENTED_EDGE('',*,*,#24821,.T.);
#32823=ORIENTED_EDGE('',*,*,#24822,.T.);
#32824=ORIENTED_EDGE('',*,*,#24823,.T.);
#32825=ORIENTED_EDGE('',*,*,#24824,.T.);
#32826=ORIENTED_EDGE('',*,*,#24825,.F.);
#32827=ORIENTED_EDGE('',*,*,#24826,.T.);
#32828=ORIENTED_EDGE('',*,*,#24827,.T.);
#32829=ORIENTED_EDGE('',*,*,#24825,.T.);
#32830=ORIENTED_EDGE('',*,*,#24828,.T.);
#32831=ORIENTED_EDGE('',*,*,#24819,.F.);
#32832=ORIENTED_EDGE('',*,*,#24829,.T.);
#32833=ORIENTED_EDGE('',*,*,#24830,.F.);
#32834=ORIENTED_EDGE('',*,*,#24831,.T.);
#32835=ORIENTED_EDGE('',*,*,#24822,.F.);
#32836=ORIENTED_EDGE('',*,*,#24832,.T.);
#32837=ORIENTED_EDGE('',*,*,#24833,.T.);
#32838=ORIENTED_EDGE('',*,*,#24834,.T.);
#32839=ORIENTED_EDGE('',*,*,#24830,.T.);
#32840=ORIENTED_EDGE('',*,*,#24835,.T.);
#32841=ORIENTED_EDGE('',*,*,#24836,.T.);
#32842=ORIENTED_EDGE('',*,*,#24837,.T.);
#32843=ORIENTED_EDGE('',*,*,#24838,.T.);
#32844=ORIENTED_EDGE('',*,*,#24839,.F.);
#32845=ORIENTED_EDGE('',*,*,#24840,.T.);
#32846=ORIENTED_EDGE('',*,*,#24841,.T.);
#32847=ORIENTED_EDGE('',*,*,#24839,.T.);
#32848=ORIENTED_EDGE('',*,*,#24842,.T.);
#32849=ORIENTED_EDGE('',*,*,#24833,.F.);
#32850=ORIENTED_EDGE('',*,*,#24843,.T.);
#32851=ORIENTED_EDGE('',*,*,#21508,.F.);
#32852=ORIENTED_EDGE('',*,*,#24844,.T.);
#32853=ORIENTED_EDGE('',*,*,#24836,.F.);
#32854=ORIENTED_EDGE('',*,*,#24845,.T.);
#32855=ORIENTED_EDGE('',*,*,#21505,.F.);
#32856=ORIENTED_EDGE('',*,*,#24846,.T.);
#32857=ORIENTED_EDGE('',*,*,#24847,.T.);
#32858=ORIENTED_EDGE('',*,*,#24848,.F.);
#32859=ORIENTED_EDGE('',*,*,#24848,.T.);
#32860=ORIENTED_EDGE('',*,*,#24849,.T.);
#32861=ORIENTED_EDGE('',*,*,#21506,.F.);
#32862=ORIENTED_EDGE('',*,*,#24850,.T.);
#32863=ORIENTED_EDGE('',*,*,#24851,.T.);
#32864=ORIENTED_EDGE('',*,*,#21347,.F.);
#32865=ORIENTED_EDGE('',*,*,#24852,.F.);
#32866=ORIENTED_EDGE('',*,*,#24853,.T.);
#32867=ORIENTED_EDGE('',*,*,#24854,.T.);
#32868=ORIENTED_EDGE('',*,*,#24855,.F.);
#32869=ORIENTED_EDGE('',*,*,#24856,.T.);
#32870=ORIENTED_EDGE('',*,*,#24850,.F.);
#32871=ORIENTED_EDGE('',*,*,#24857,.T.);
#32872=ORIENTED_EDGE('',*,*,#24858,.T.);
#32873=ORIENTED_EDGE('',*,*,#24859,.T.);
#32874=ORIENTED_EDGE('',*,*,#24855,.T.);
#32875=ORIENTED_EDGE('',*,*,#24860,.T.);
#32876=ORIENTED_EDGE('',*,*,#24861,.T.);
#32877=ORIENTED_EDGE('',*,*,#24862,.T.);
#32878=ORIENTED_EDGE('',*,*,#24863,.T.);
#32879=ORIENTED_EDGE('',*,*,#24864,.F.);
#32880=ORIENTED_EDGE('',*,*,#24865,.T.);
#32881=ORIENTED_EDGE('',*,*,#24866,.T.);
#32882=ORIENTED_EDGE('',*,*,#24864,.T.);
#32883=ORIENTED_EDGE('',*,*,#24867,.T.);
#32884=ORIENTED_EDGE('',*,*,#24858,.F.);
#32885=ORIENTED_EDGE('',*,*,#24868,.T.);
#32886=ORIENTED_EDGE('',*,*,#21350,.F.);
#32887=ORIENTED_EDGE('',*,*,#24869,.T.);
#32888=ORIENTED_EDGE('',*,*,#24756,.T.);
#32889=ORIENTED_EDGE('',*,*,#24870,.F.);
#32890=ORIENTED_EDGE('',*,*,#24871,.T.);
#32891=ORIENTED_EDGE('',*,*,#24861,.F.);
#32892=ORIENTED_EDGE('',*,*,#24872,.T.);
#32893=ORIENTED_EDGE('',*,*,#24873,.T.);
#32894=ORIENTED_EDGE('',*,*,#24874,.T.);
#32895=ORIENTED_EDGE('',*,*,#24870,.T.);
#32896=ORIENTED_EDGE('',*,*,#24875,.T.);
#32897=ORIENTED_EDGE('',*,*,#24876,.T.);
#32898=ORIENTED_EDGE('',*,*,#24877,.T.);
#32899=ORIENTED_EDGE('',*,*,#24878,.T.);
#32900=ORIENTED_EDGE('',*,*,#24879,.F.);
#32901=ORIENTED_EDGE('',*,*,#24880,.T.);
#32902=ORIENTED_EDGE('',*,*,#24881,.T.);
#32903=ORIENTED_EDGE('',*,*,#24879,.T.);
#32904=ORIENTED_EDGE('',*,*,#24882,.T.);
#32905=ORIENTED_EDGE('',*,*,#24873,.F.);
#32906=ORIENTED_EDGE('',*,*,#24883,.T.);
#32907=ORIENTED_EDGE('',*,*,#24884,.F.);
#32908=ORIENTED_EDGE('',*,*,#24885,.T.);
#32909=ORIENTED_EDGE('',*,*,#24876,.F.);
#32910=ORIENTED_EDGE('',*,*,#24886,.T.);
#32911=ORIENTED_EDGE('',*,*,#24887,.T.);
#32912=ORIENTED_EDGE('',*,*,#24888,.T.);
#32913=ORIENTED_EDGE('',*,*,#24884,.T.);
#32914=ORIENTED_EDGE('',*,*,#24889,.T.);
#32915=ORIENTED_EDGE('',*,*,#24890,.T.);
#32916=ORIENTED_EDGE('',*,*,#24891,.T.);
#32917=ORIENTED_EDGE('',*,*,#24892,.T.);
#32918=ORIENTED_EDGE('',*,*,#24893,.F.);
#32919=ORIENTED_EDGE('',*,*,#24894,.T.);
#32920=ORIENTED_EDGE('',*,*,#24895,.T.);
#32921=ORIENTED_EDGE('',*,*,#24893,.T.);
#32922=ORIENTED_EDGE('',*,*,#24896,.T.);
#32923=ORIENTED_EDGE('',*,*,#24887,.F.);
#32924=ORIENTED_EDGE('',*,*,#24897,.T.);
#32925=ORIENTED_EDGE('',*,*,#24898,.F.);
#32926=ORIENTED_EDGE('',*,*,#24899,.T.);
#32927=ORIENTED_EDGE('',*,*,#24890,.F.);
#32928=ORIENTED_EDGE('',*,*,#24900,.T.);
#32929=ORIENTED_EDGE('',*,*,#24901,.T.);
#32930=ORIENTED_EDGE('',*,*,#24902,.T.);
#32931=ORIENTED_EDGE('',*,*,#24898,.T.);
#32932=ORIENTED_EDGE('',*,*,#24903,.T.);
#32933=ORIENTED_EDGE('',*,*,#24904,.T.);
#32934=ORIENTED_EDGE('',*,*,#24905,.T.);
#32935=ORIENTED_EDGE('',*,*,#24906,.T.);
#32936=ORIENTED_EDGE('',*,*,#24907,.F.);
#32937=ORIENTED_EDGE('',*,*,#24908,.T.);
#32938=ORIENTED_EDGE('',*,*,#24909,.T.);
#32939=ORIENTED_EDGE('',*,*,#24907,.T.);
#32940=ORIENTED_EDGE('',*,*,#24910,.T.);
#32941=ORIENTED_EDGE('',*,*,#24901,.F.);
#32942=ORIENTED_EDGE('',*,*,#24911,.T.);
#32943=ORIENTED_EDGE('',*,*,#24912,.F.);
#32944=ORIENTED_EDGE('',*,*,#24913,.T.);
#32945=ORIENTED_EDGE('',*,*,#24904,.F.);
#32946=ORIENTED_EDGE('',*,*,#24914,.T.);
#32947=ORIENTED_EDGE('',*,*,#24915,.T.);
#32948=ORIENTED_EDGE('',*,*,#24916,.T.);
#32949=ORIENTED_EDGE('',*,*,#24912,.T.);
#32950=ORIENTED_EDGE('',*,*,#24917,.T.);
#32951=ORIENTED_EDGE('',*,*,#24918,.T.);
#32952=ORIENTED_EDGE('',*,*,#24919,.T.);
#32953=ORIENTED_EDGE('',*,*,#24920,.T.);
#32954=ORIENTED_EDGE('',*,*,#24921,.F.);
#32955=ORIENTED_EDGE('',*,*,#24922,.T.);
#32956=ORIENTED_EDGE('',*,*,#24923,.T.);
#32957=ORIENTED_EDGE('',*,*,#24921,.T.);
#32958=ORIENTED_EDGE('',*,*,#24924,.T.);
#32959=ORIENTED_EDGE('',*,*,#24915,.F.);
#32960=ORIENTED_EDGE('',*,*,#24925,.T.);
#32961=ORIENTED_EDGE('',*,*,#24926,.F.);
#32962=ORIENTED_EDGE('',*,*,#24927,.T.);
#32963=ORIENTED_EDGE('',*,*,#24918,.F.);
#32964=ORIENTED_EDGE('',*,*,#24928,.T.);
#32965=ORIENTED_EDGE('',*,*,#24929,.T.);
#32966=ORIENTED_EDGE('',*,*,#24930,.T.);
#32967=ORIENTED_EDGE('',*,*,#24926,.T.);
#32968=ORIENTED_EDGE('',*,*,#24931,.T.);
#32969=ORIENTED_EDGE('',*,*,#24932,.T.);
#32970=ORIENTED_EDGE('',*,*,#24933,.T.);
#32971=ORIENTED_EDGE('',*,*,#24934,.T.);
#32972=ORIENTED_EDGE('',*,*,#24935,.F.);
#32973=ORIENTED_EDGE('',*,*,#24936,.T.);
#32974=ORIENTED_EDGE('',*,*,#24937,.T.);
#32975=ORIENTED_EDGE('',*,*,#24935,.T.);
#32976=ORIENTED_EDGE('',*,*,#24938,.T.);
#32977=ORIENTED_EDGE('',*,*,#24929,.F.);
#32978=ORIENTED_EDGE('',*,*,#24939,.T.);
#32979=ORIENTED_EDGE('',*,*,#21514,.F.);
#32980=ORIENTED_EDGE('',*,*,#24940,.T.);
#32981=ORIENTED_EDGE('',*,*,#24932,.F.);
#32982=ORIENTED_EDGE('',*,*,#24941,.T.);
#32983=ORIENTED_EDGE('',*,*,#21511,.F.);
#32984=ORIENTED_EDGE('',*,*,#24942,.T.);
#32985=ORIENTED_EDGE('',*,*,#24943,.T.);
#32986=ORIENTED_EDGE('',*,*,#24944,.F.);
#32987=ORIENTED_EDGE('',*,*,#24944,.T.);
#32988=ORIENTED_EDGE('',*,*,#24945,.T.);
#32989=ORIENTED_EDGE('',*,*,#21512,.F.);
#32990=ORIENTED_EDGE('',*,*,#24946,.T.);
#32991=ORIENTED_EDGE('',*,*,#24947,.T.);
#32992=ORIENTED_EDGE('',*,*,#21343,.F.);
#32993=ORIENTED_EDGE('',*,*,#24948,.F.);
#32994=ORIENTED_EDGE('',*,*,#24949,.T.);
#32995=ORIENTED_EDGE('',*,*,#24950,.T.);
#32996=ORIENTED_EDGE('',*,*,#24951,.F.);
#32997=ORIENTED_EDGE('',*,*,#24952,.T.);
#32998=ORIENTED_EDGE('',*,*,#24946,.F.);
#32999=ORIENTED_EDGE('',*,*,#24953,.T.);
#33000=ORIENTED_EDGE('',*,*,#24954,.T.);
#33001=ORIENTED_EDGE('',*,*,#24955,.T.);
#33002=ORIENTED_EDGE('',*,*,#24951,.T.);
#33003=ORIENTED_EDGE('',*,*,#24956,.T.);
#33004=ORIENTED_EDGE('',*,*,#24957,.T.);
#33005=ORIENTED_EDGE('',*,*,#24958,.T.);
#33006=ORIENTED_EDGE('',*,*,#24959,.T.);
#33007=ORIENTED_EDGE('',*,*,#24960,.F.);
#33008=ORIENTED_EDGE('',*,*,#24961,.T.);
#33009=ORIENTED_EDGE('',*,*,#24962,.T.);
#33010=ORIENTED_EDGE('',*,*,#24960,.T.);
#33011=ORIENTED_EDGE('',*,*,#24963,.T.);
#33012=ORIENTED_EDGE('',*,*,#24954,.F.);
#33013=ORIENTED_EDGE('',*,*,#24964,.T.);
#33014=ORIENTED_EDGE('',*,*,#21346,.F.);
#33015=ORIENTED_EDGE('',*,*,#24965,.T.);
#33016=ORIENTED_EDGE('',*,*,#24852,.T.);
#33017=ORIENTED_EDGE('',*,*,#24966,.F.);
#33018=ORIENTED_EDGE('',*,*,#24967,.T.);
#33019=ORIENTED_EDGE('',*,*,#24957,.F.);
#33020=ORIENTED_EDGE('',*,*,#24968,.T.);
#33021=ORIENTED_EDGE('',*,*,#24969,.T.);
#33022=ORIENTED_EDGE('',*,*,#24970,.T.);
#33023=ORIENTED_EDGE('',*,*,#24966,.T.);
#33024=ORIENTED_EDGE('',*,*,#24971,.T.);
#33025=ORIENTED_EDGE('',*,*,#24972,.T.);
#33026=ORIENTED_EDGE('',*,*,#24973,.T.);
#33027=ORIENTED_EDGE('',*,*,#24974,.T.);
#33028=ORIENTED_EDGE('',*,*,#24975,.F.);
#33029=ORIENTED_EDGE('',*,*,#24976,.T.);
#33030=ORIENTED_EDGE('',*,*,#24977,.T.);
#33031=ORIENTED_EDGE('',*,*,#24975,.T.);
#33032=ORIENTED_EDGE('',*,*,#24978,.T.);
#33033=ORIENTED_EDGE('',*,*,#24969,.F.);
#33034=ORIENTED_EDGE('',*,*,#24979,.T.);
#33035=ORIENTED_EDGE('',*,*,#24980,.F.);
#33036=ORIENTED_EDGE('',*,*,#24981,.T.);
#33037=ORIENTED_EDGE('',*,*,#24972,.F.);
#33038=ORIENTED_EDGE('',*,*,#24982,.T.);
#33039=ORIENTED_EDGE('',*,*,#24983,.T.);
#33040=ORIENTED_EDGE('',*,*,#24984,.T.);
#33041=ORIENTED_EDGE('',*,*,#24980,.T.);
#33042=ORIENTED_EDGE('',*,*,#24985,.T.);
#33043=ORIENTED_EDGE('',*,*,#24986,.T.);
#33044=ORIENTED_EDGE('',*,*,#24987,.T.);
#33045=ORIENTED_EDGE('',*,*,#24988,.T.);
#33046=ORIENTED_EDGE('',*,*,#24989,.F.);
#33047=ORIENTED_EDGE('',*,*,#24990,.T.);
#33048=ORIENTED_EDGE('',*,*,#24991,.T.);
#33049=ORIENTED_EDGE('',*,*,#24989,.T.);
#33050=ORIENTED_EDGE('',*,*,#24992,.T.);
#33051=ORIENTED_EDGE('',*,*,#24983,.F.);
#33052=ORIENTED_EDGE('',*,*,#24993,.T.);
#33053=ORIENTED_EDGE('',*,*,#24994,.F.);
#33054=ORIENTED_EDGE('',*,*,#24995,.T.);
#33055=ORIENTED_EDGE('',*,*,#24986,.F.);
#33056=ORIENTED_EDGE('',*,*,#24996,.T.);
#33057=ORIENTED_EDGE('',*,*,#24997,.T.);
#33058=ORIENTED_EDGE('',*,*,#24998,.T.);
#33059=ORIENTED_EDGE('',*,*,#24994,.T.);
#33060=ORIENTED_EDGE('',*,*,#24999,.T.);
#33061=ORIENTED_EDGE('',*,*,#25000,.T.);
#33062=ORIENTED_EDGE('',*,*,#25001,.T.);
#33063=ORIENTED_EDGE('',*,*,#25002,.T.);
#33064=ORIENTED_EDGE('',*,*,#25003,.F.);
#33065=ORIENTED_EDGE('',*,*,#25004,.T.);
#33066=ORIENTED_EDGE('',*,*,#25005,.T.);
#33067=ORIENTED_EDGE('',*,*,#25003,.T.);
#33068=ORIENTED_EDGE('',*,*,#25006,.T.);
#33069=ORIENTED_EDGE('',*,*,#24997,.F.);
#33070=ORIENTED_EDGE('',*,*,#25007,.T.);
#33071=ORIENTED_EDGE('',*,*,#25008,.F.);
#33072=ORIENTED_EDGE('',*,*,#25009,.T.);
#33073=ORIENTED_EDGE('',*,*,#25000,.F.);
#33074=ORIENTED_EDGE('',*,*,#25010,.T.);
#33075=ORIENTED_EDGE('',*,*,#25011,.T.);
#33076=ORIENTED_EDGE('',*,*,#25012,.T.);
#33077=ORIENTED_EDGE('',*,*,#25008,.T.);
#33078=ORIENTED_EDGE('',*,*,#25013,.T.);
#33079=ORIENTED_EDGE('',*,*,#25014,.T.);
#33080=ORIENTED_EDGE('',*,*,#25015,.T.);
#33081=ORIENTED_EDGE('',*,*,#25016,.T.);
#33082=ORIENTED_EDGE('',*,*,#25017,.F.);
#33083=ORIENTED_EDGE('',*,*,#25018,.T.);
#33084=ORIENTED_EDGE('',*,*,#25019,.T.);
#33085=ORIENTED_EDGE('',*,*,#25017,.T.);
#33086=ORIENTED_EDGE('',*,*,#25020,.T.);
#33087=ORIENTED_EDGE('',*,*,#25011,.F.);
#33088=ORIENTED_EDGE('',*,*,#25021,.T.);
#33089=ORIENTED_EDGE('',*,*,#25022,.F.);
#33090=ORIENTED_EDGE('',*,*,#25023,.T.);
#33091=ORIENTED_EDGE('',*,*,#25014,.F.);
#33092=ORIENTED_EDGE('',*,*,#25024,.T.);
#33093=ORIENTED_EDGE('',*,*,#25025,.T.);
#33094=ORIENTED_EDGE('',*,*,#25026,.T.);
#33095=ORIENTED_EDGE('',*,*,#25022,.T.);
#33096=ORIENTED_EDGE('',*,*,#25027,.T.);
#33097=ORIENTED_EDGE('',*,*,#25028,.T.);
#33098=ORIENTED_EDGE('',*,*,#25029,.T.);
#33099=ORIENTED_EDGE('',*,*,#25030,.T.);
#33100=ORIENTED_EDGE('',*,*,#25031,.F.);
#33101=ORIENTED_EDGE('',*,*,#25032,.T.);
#33102=ORIENTED_EDGE('',*,*,#25033,.T.);
#33103=ORIENTED_EDGE('',*,*,#25031,.T.);
#33104=ORIENTED_EDGE('',*,*,#25034,.T.);
#33105=ORIENTED_EDGE('',*,*,#25025,.F.);
#33106=ORIENTED_EDGE('',*,*,#25035,.T.);
#33107=ORIENTED_EDGE('',*,*,#21520,.F.);
#33108=ORIENTED_EDGE('',*,*,#25036,.T.);
#33109=ORIENTED_EDGE('',*,*,#25028,.F.);
#33110=ORIENTED_EDGE('',*,*,#25037,.T.);
#33111=ORIENTED_EDGE('',*,*,#21517,.F.);
#33112=ORIENTED_EDGE('',*,*,#25038,.T.);
#33113=ORIENTED_EDGE('',*,*,#25039,.T.);
#33114=ORIENTED_EDGE('',*,*,#25040,.F.);
#33115=ORIENTED_EDGE('',*,*,#25040,.T.);
#33116=ORIENTED_EDGE('',*,*,#25041,.T.);
#33117=ORIENTED_EDGE('',*,*,#21518,.F.);
#33118=ORIENTED_EDGE('',*,*,#25042,.T.);
#33119=ORIENTED_EDGE('',*,*,#25043,.T.);
#33120=ORIENTED_EDGE('',*,*,#21339,.F.);
#33121=ORIENTED_EDGE('',*,*,#25044,.F.);
#33122=ORIENTED_EDGE('',*,*,#25045,.T.);
#33123=ORIENTED_EDGE('',*,*,#25046,.T.);
#33124=ORIENTED_EDGE('',*,*,#25047,.F.);
#33125=ORIENTED_EDGE('',*,*,#25048,.T.);
#33126=ORIENTED_EDGE('',*,*,#25042,.F.);
#33127=ORIENTED_EDGE('',*,*,#25049,.T.);
#33128=ORIENTED_EDGE('',*,*,#25050,.T.);
#33129=ORIENTED_EDGE('',*,*,#25051,.T.);
#33130=ORIENTED_EDGE('',*,*,#25047,.T.);
#33131=ORIENTED_EDGE('',*,*,#25052,.T.);
#33132=ORIENTED_EDGE('',*,*,#25053,.T.);
#33133=ORIENTED_EDGE('',*,*,#25054,.T.);
#33134=ORIENTED_EDGE('',*,*,#25055,.T.);
#33135=ORIENTED_EDGE('',*,*,#25056,.F.);
#33136=ORIENTED_EDGE('',*,*,#25057,.T.);
#33137=ORIENTED_EDGE('',*,*,#25058,.T.);
#33138=ORIENTED_EDGE('',*,*,#25056,.T.);
#33139=ORIENTED_EDGE('',*,*,#25059,.T.);
#33140=ORIENTED_EDGE('',*,*,#25050,.F.);
#33141=ORIENTED_EDGE('',*,*,#25060,.T.);
#33142=ORIENTED_EDGE('',*,*,#21342,.F.);
#33143=ORIENTED_EDGE('',*,*,#25061,.T.);
#33144=ORIENTED_EDGE('',*,*,#24948,.T.);
#33145=ORIENTED_EDGE('',*,*,#25062,.F.);
#33146=ORIENTED_EDGE('',*,*,#25063,.T.);
#33147=ORIENTED_EDGE('',*,*,#25053,.F.);
#33148=ORIENTED_EDGE('',*,*,#25064,.T.);
#33149=ORIENTED_EDGE('',*,*,#25065,.T.);
#33150=ORIENTED_EDGE('',*,*,#25066,.T.);
#33151=ORIENTED_EDGE('',*,*,#25062,.T.);
#33152=ORIENTED_EDGE('',*,*,#25067,.T.);
#33153=ORIENTED_EDGE('',*,*,#25068,.T.);
#33154=ORIENTED_EDGE('',*,*,#25069,.T.);
#33155=ORIENTED_EDGE('',*,*,#25070,.T.);
#33156=ORIENTED_EDGE('',*,*,#25071,.F.);
#33157=ORIENTED_EDGE('',*,*,#25072,.T.);
#33158=ORIENTED_EDGE('',*,*,#25073,.T.);
#33159=ORIENTED_EDGE('',*,*,#25071,.T.);
#33160=ORIENTED_EDGE('',*,*,#25074,.T.);
#33161=ORIENTED_EDGE('',*,*,#25065,.F.);
#33162=ORIENTED_EDGE('',*,*,#25075,.T.);
#33163=ORIENTED_EDGE('',*,*,#25076,.F.);
#33164=ORIENTED_EDGE('',*,*,#25077,.T.);
#33165=ORIENTED_EDGE('',*,*,#25068,.F.);
#33166=ORIENTED_EDGE('',*,*,#25078,.T.);
#33167=ORIENTED_EDGE('',*,*,#25079,.T.);
#33168=ORIENTED_EDGE('',*,*,#25080,.T.);
#33169=ORIENTED_EDGE('',*,*,#25076,.T.);
#33170=ORIENTED_EDGE('',*,*,#25081,.T.);
#33171=ORIENTED_EDGE('',*,*,#25082,.T.);
#33172=ORIENTED_EDGE('',*,*,#25083,.T.);
#33173=ORIENTED_EDGE('',*,*,#25084,.T.);
#33174=ORIENTED_EDGE('',*,*,#25085,.F.);
#33175=ORIENTED_EDGE('',*,*,#25086,.T.);
#33176=ORIENTED_EDGE('',*,*,#25087,.T.);
#33177=ORIENTED_EDGE('',*,*,#25085,.T.);
#33178=ORIENTED_EDGE('',*,*,#25088,.T.);
#33179=ORIENTED_EDGE('',*,*,#25079,.F.);
#33180=ORIENTED_EDGE('',*,*,#25089,.T.);
#33181=ORIENTED_EDGE('',*,*,#25090,.F.);
#33182=ORIENTED_EDGE('',*,*,#25091,.T.);
#33183=ORIENTED_EDGE('',*,*,#25082,.F.);
#33184=ORIENTED_EDGE('',*,*,#25092,.T.);
#33185=ORIENTED_EDGE('',*,*,#25093,.T.);
#33186=ORIENTED_EDGE('',*,*,#25094,.T.);
#33187=ORIENTED_EDGE('',*,*,#25090,.T.);
#33188=ORIENTED_EDGE('',*,*,#25095,.T.);
#33189=ORIENTED_EDGE('',*,*,#25096,.T.);
#33190=ORIENTED_EDGE('',*,*,#25097,.T.);
#33191=ORIENTED_EDGE('',*,*,#25098,.T.);
#33192=ORIENTED_EDGE('',*,*,#25099,.F.);
#33193=ORIENTED_EDGE('',*,*,#25100,.T.);
#33194=ORIENTED_EDGE('',*,*,#25101,.T.);
#33195=ORIENTED_EDGE('',*,*,#25099,.T.);
#33196=ORIENTED_EDGE('',*,*,#25102,.T.);
#33197=ORIENTED_EDGE('',*,*,#25093,.F.);
#33198=ORIENTED_EDGE('',*,*,#25103,.T.);
#33199=ORIENTED_EDGE('',*,*,#25104,.F.);
#33200=ORIENTED_EDGE('',*,*,#25105,.T.);
#33201=ORIENTED_EDGE('',*,*,#25096,.F.);
#33202=ORIENTED_EDGE('',*,*,#25106,.T.);
#33203=ORIENTED_EDGE('',*,*,#25107,.T.);
#33204=ORIENTED_EDGE('',*,*,#25108,.T.);
#33205=ORIENTED_EDGE('',*,*,#25104,.T.);
#33206=ORIENTED_EDGE('',*,*,#25109,.T.);
#33207=ORIENTED_EDGE('',*,*,#25110,.T.);
#33208=ORIENTED_EDGE('',*,*,#25111,.T.);
#33209=ORIENTED_EDGE('',*,*,#25112,.T.);
#33210=ORIENTED_EDGE('',*,*,#25113,.F.);
#33211=ORIENTED_EDGE('',*,*,#25114,.T.);
#33212=ORIENTED_EDGE('',*,*,#25115,.T.);
#33213=ORIENTED_EDGE('',*,*,#25113,.T.);
#33214=ORIENTED_EDGE('',*,*,#25116,.T.);
#33215=ORIENTED_EDGE('',*,*,#25107,.F.);
#33216=ORIENTED_EDGE('',*,*,#25117,.T.);
#33217=ORIENTED_EDGE('',*,*,#25118,.F.);
#33218=ORIENTED_EDGE('',*,*,#25119,.T.);
#33219=ORIENTED_EDGE('',*,*,#25110,.F.);
#33220=ORIENTED_EDGE('',*,*,#25120,.T.);
#33221=ORIENTED_EDGE('',*,*,#25121,.T.);
#33222=ORIENTED_EDGE('',*,*,#25122,.T.);
#33223=ORIENTED_EDGE('',*,*,#25118,.T.);
#33224=ORIENTED_EDGE('',*,*,#25123,.T.);
#33225=ORIENTED_EDGE('',*,*,#25124,.T.);
#33226=ORIENTED_EDGE('',*,*,#25125,.T.);
#33227=ORIENTED_EDGE('',*,*,#25126,.T.);
#33228=ORIENTED_EDGE('',*,*,#25127,.F.);
#33229=ORIENTED_EDGE('',*,*,#25128,.T.);
#33230=ORIENTED_EDGE('',*,*,#25129,.T.);
#33231=ORIENTED_EDGE('',*,*,#25127,.T.);
#33232=ORIENTED_EDGE('',*,*,#25130,.T.);
#33233=ORIENTED_EDGE('',*,*,#25121,.F.);
#33234=ORIENTED_EDGE('',*,*,#25131,.T.);
#33235=ORIENTED_EDGE('',*,*,#21526,.F.);
#33236=ORIENTED_EDGE('',*,*,#25132,.T.);
#33237=ORIENTED_EDGE('',*,*,#25124,.F.);
#33238=ORIENTED_EDGE('',*,*,#25133,.T.);
#33239=ORIENTED_EDGE('',*,*,#21523,.F.);
#33240=ORIENTED_EDGE('',*,*,#25134,.T.);
#33241=ORIENTED_EDGE('',*,*,#25135,.T.);
#33242=ORIENTED_EDGE('',*,*,#25136,.F.);
#33243=ORIENTED_EDGE('',*,*,#25136,.T.);
#33244=ORIENTED_EDGE('',*,*,#25137,.T.);
#33245=ORIENTED_EDGE('',*,*,#21524,.F.);
#33246=ORIENTED_EDGE('',*,*,#25138,.T.);
#33247=ORIENTED_EDGE('',*,*,#25139,.T.);
#33248=ORIENTED_EDGE('',*,*,#21335,.F.);
#33249=ORIENTED_EDGE('',*,*,#25140,.F.);
#33250=ORIENTED_EDGE('',*,*,#25141,.T.);
#33251=ORIENTED_EDGE('',*,*,#25142,.T.);
#33252=ORIENTED_EDGE('',*,*,#25143,.F.);
#33253=ORIENTED_EDGE('',*,*,#25144,.T.);
#33254=ORIENTED_EDGE('',*,*,#25138,.F.);
#33255=ORIENTED_EDGE('',*,*,#25145,.T.);
#33256=ORIENTED_EDGE('',*,*,#25146,.T.);
#33257=ORIENTED_EDGE('',*,*,#25147,.T.);
#33258=ORIENTED_EDGE('',*,*,#25143,.T.);
#33259=ORIENTED_EDGE('',*,*,#25148,.T.);
#33260=ORIENTED_EDGE('',*,*,#25149,.T.);
#33261=ORIENTED_EDGE('',*,*,#25150,.T.);
#33262=ORIENTED_EDGE('',*,*,#25151,.T.);
#33263=ORIENTED_EDGE('',*,*,#25152,.F.);
#33264=ORIENTED_EDGE('',*,*,#25153,.T.);
#33265=ORIENTED_EDGE('',*,*,#25154,.T.);
#33266=ORIENTED_EDGE('',*,*,#25152,.T.);
#33267=ORIENTED_EDGE('',*,*,#25155,.T.);
#33268=ORIENTED_EDGE('',*,*,#25146,.F.);
#33269=ORIENTED_EDGE('',*,*,#25156,.T.);
#33270=ORIENTED_EDGE('',*,*,#21338,.F.);
#33271=ORIENTED_EDGE('',*,*,#25157,.T.);
#33272=ORIENTED_EDGE('',*,*,#25044,.T.);
#33273=ORIENTED_EDGE('',*,*,#25158,.F.);
#33274=ORIENTED_EDGE('',*,*,#25159,.T.);
#33275=ORIENTED_EDGE('',*,*,#25149,.F.);
#33276=ORIENTED_EDGE('',*,*,#25160,.T.);
#33277=ORIENTED_EDGE('',*,*,#25161,.T.);
#33278=ORIENTED_EDGE('',*,*,#25162,.T.);
#33279=ORIENTED_EDGE('',*,*,#25158,.T.);
#33280=ORIENTED_EDGE('',*,*,#25163,.T.);
#33281=ORIENTED_EDGE('',*,*,#25164,.T.);
#33282=ORIENTED_EDGE('',*,*,#25165,.T.);
#33283=ORIENTED_EDGE('',*,*,#25166,.T.);
#33284=ORIENTED_EDGE('',*,*,#25167,.F.);
#33285=ORIENTED_EDGE('',*,*,#25168,.T.);
#33286=ORIENTED_EDGE('',*,*,#25169,.T.);
#33287=ORIENTED_EDGE('',*,*,#25167,.T.);
#33288=ORIENTED_EDGE('',*,*,#25170,.T.);
#33289=ORIENTED_EDGE('',*,*,#25161,.F.);
#33290=ORIENTED_EDGE('',*,*,#25171,.T.);
#33291=ORIENTED_EDGE('',*,*,#25172,.F.);
#33292=ORIENTED_EDGE('',*,*,#25173,.T.);
#33293=ORIENTED_EDGE('',*,*,#25164,.F.);
#33294=ORIENTED_EDGE('',*,*,#25174,.T.);
#33295=ORIENTED_EDGE('',*,*,#25175,.T.);
#33296=ORIENTED_EDGE('',*,*,#25176,.T.);
#33297=ORIENTED_EDGE('',*,*,#25172,.T.);
#33298=ORIENTED_EDGE('',*,*,#25177,.T.);
#33299=ORIENTED_EDGE('',*,*,#25178,.T.);
#33300=ORIENTED_EDGE('',*,*,#25179,.T.);
#33301=ORIENTED_EDGE('',*,*,#25180,.T.);
#33302=ORIENTED_EDGE('',*,*,#25181,.F.);
#33303=ORIENTED_EDGE('',*,*,#25182,.T.);
#33304=ORIENTED_EDGE('',*,*,#25183,.T.);
#33305=ORIENTED_EDGE('',*,*,#25181,.T.);
#33306=ORIENTED_EDGE('',*,*,#25184,.T.);
#33307=ORIENTED_EDGE('',*,*,#25175,.F.);
#33308=ORIENTED_EDGE('',*,*,#25185,.T.);
#33309=ORIENTED_EDGE('',*,*,#25186,.F.);
#33310=ORIENTED_EDGE('',*,*,#25187,.T.);
#33311=ORIENTED_EDGE('',*,*,#25178,.F.);
#33312=ORIENTED_EDGE('',*,*,#25188,.T.);
#33313=ORIENTED_EDGE('',*,*,#25189,.T.);
#33314=ORIENTED_EDGE('',*,*,#25190,.T.);
#33315=ORIENTED_EDGE('',*,*,#25186,.T.);
#33316=ORIENTED_EDGE('',*,*,#25191,.T.);
#33317=ORIENTED_EDGE('',*,*,#25192,.T.);
#33318=ORIENTED_EDGE('',*,*,#25193,.T.);
#33319=ORIENTED_EDGE('',*,*,#25194,.T.);
#33320=ORIENTED_EDGE('',*,*,#25195,.F.);
#33321=ORIENTED_EDGE('',*,*,#25196,.T.);
#33322=ORIENTED_EDGE('',*,*,#25197,.T.);
#33323=ORIENTED_EDGE('',*,*,#25195,.T.);
#33324=ORIENTED_EDGE('',*,*,#25198,.T.);
#33325=ORIENTED_EDGE('',*,*,#25189,.F.);
#33326=ORIENTED_EDGE('',*,*,#25199,.T.);
#33327=ORIENTED_EDGE('',*,*,#25200,.F.);
#33328=ORIENTED_EDGE('',*,*,#25201,.T.);
#33329=ORIENTED_EDGE('',*,*,#25192,.F.);
#33330=ORIENTED_EDGE('',*,*,#25202,.T.);
#33331=ORIENTED_EDGE('',*,*,#25203,.T.);
#33332=ORIENTED_EDGE('',*,*,#25204,.T.);
#33333=ORIENTED_EDGE('',*,*,#25200,.T.);
#33334=ORIENTED_EDGE('',*,*,#25205,.T.);
#33335=ORIENTED_EDGE('',*,*,#25206,.T.);
#33336=ORIENTED_EDGE('',*,*,#25207,.T.);
#33337=ORIENTED_EDGE('',*,*,#25208,.T.);
#33338=ORIENTED_EDGE('',*,*,#25209,.F.);
#33339=ORIENTED_EDGE('',*,*,#25210,.T.);
#33340=ORIENTED_EDGE('',*,*,#25211,.T.);
#33341=ORIENTED_EDGE('',*,*,#25209,.T.);
#33342=ORIENTED_EDGE('',*,*,#25212,.T.);
#33343=ORIENTED_EDGE('',*,*,#25203,.F.);
#33344=ORIENTED_EDGE('',*,*,#25213,.T.);
#33345=ORIENTED_EDGE('',*,*,#25214,.F.);
#33346=ORIENTED_EDGE('',*,*,#25215,.T.);
#33347=ORIENTED_EDGE('',*,*,#25206,.F.);
#33348=ORIENTED_EDGE('',*,*,#25216,.T.);
#33349=ORIENTED_EDGE('',*,*,#25217,.T.);
#33350=ORIENTED_EDGE('',*,*,#25218,.T.);
#33351=ORIENTED_EDGE('',*,*,#25214,.T.);
#33352=ORIENTED_EDGE('',*,*,#25219,.T.);
#33353=ORIENTED_EDGE('',*,*,#25220,.T.);
#33354=ORIENTED_EDGE('',*,*,#25221,.T.);
#33355=ORIENTED_EDGE('',*,*,#25222,.T.);
#33356=ORIENTED_EDGE('',*,*,#25223,.F.);
#33357=ORIENTED_EDGE('',*,*,#25224,.T.);
#33358=ORIENTED_EDGE('',*,*,#25225,.T.);
#33359=ORIENTED_EDGE('',*,*,#25223,.T.);
#33360=ORIENTED_EDGE('',*,*,#25226,.T.);
#33361=ORIENTED_EDGE('',*,*,#25217,.F.);
#33362=ORIENTED_EDGE('',*,*,#25227,.T.);
#33363=ORIENTED_EDGE('',*,*,#21532,.F.);
#33364=ORIENTED_EDGE('',*,*,#25228,.T.);
#33365=ORIENTED_EDGE('',*,*,#25220,.F.);
#33366=ORIENTED_EDGE('',*,*,#25229,.T.);
#33367=ORIENTED_EDGE('',*,*,#21529,.F.);
#33368=ORIENTED_EDGE('',*,*,#25230,.T.);
#33369=ORIENTED_EDGE('',*,*,#25231,.T.);
#33370=ORIENTED_EDGE('',*,*,#25232,.F.);
#33371=ORIENTED_EDGE('',*,*,#25232,.T.);
#33372=ORIENTED_EDGE('',*,*,#25233,.T.);
#33373=ORIENTED_EDGE('',*,*,#21530,.F.);
#33374=ORIENTED_EDGE('',*,*,#25234,.T.);
#33375=ORIENTED_EDGE('',*,*,#25235,.T.);
#33376=ORIENTED_EDGE('',*,*,#21331,.F.);
#33377=ORIENTED_EDGE('',*,*,#25236,.F.);
#33378=ORIENTED_EDGE('',*,*,#25237,.T.);
#33379=ORIENTED_EDGE('',*,*,#25238,.T.);
#33380=ORIENTED_EDGE('',*,*,#25239,.F.);
#33381=ORIENTED_EDGE('',*,*,#25240,.T.);
#33382=ORIENTED_EDGE('',*,*,#25234,.F.);
#33383=ORIENTED_EDGE('',*,*,#25241,.T.);
#33384=ORIENTED_EDGE('',*,*,#25242,.T.);
#33385=ORIENTED_EDGE('',*,*,#25243,.T.);
#33386=ORIENTED_EDGE('',*,*,#25239,.T.);
#33387=ORIENTED_EDGE('',*,*,#25244,.T.);
#33388=ORIENTED_EDGE('',*,*,#25245,.T.);
#33389=ORIENTED_EDGE('',*,*,#25246,.T.);
#33390=ORIENTED_EDGE('',*,*,#25247,.T.);
#33391=ORIENTED_EDGE('',*,*,#25248,.F.);
#33392=ORIENTED_EDGE('',*,*,#25249,.T.);
#33393=ORIENTED_EDGE('',*,*,#25250,.T.);
#33394=ORIENTED_EDGE('',*,*,#25248,.T.);
#33395=ORIENTED_EDGE('',*,*,#25251,.T.);
#33396=ORIENTED_EDGE('',*,*,#25242,.F.);
#33397=ORIENTED_EDGE('',*,*,#25252,.T.);
#33398=ORIENTED_EDGE('',*,*,#21334,.F.);
#33399=ORIENTED_EDGE('',*,*,#25253,.T.);
#33400=ORIENTED_EDGE('',*,*,#25140,.T.);
#33401=ORIENTED_EDGE('',*,*,#25254,.F.);
#33402=ORIENTED_EDGE('',*,*,#25255,.T.);
#33403=ORIENTED_EDGE('',*,*,#25245,.F.);
#33404=ORIENTED_EDGE('',*,*,#25256,.T.);
#33405=ORIENTED_EDGE('',*,*,#25257,.T.);
#33406=ORIENTED_EDGE('',*,*,#25258,.T.);
#33407=ORIENTED_EDGE('',*,*,#25254,.T.);
#33408=ORIENTED_EDGE('',*,*,#25259,.T.);
#33409=ORIENTED_EDGE('',*,*,#25260,.T.);
#33410=ORIENTED_EDGE('',*,*,#25261,.T.);
#33411=ORIENTED_EDGE('',*,*,#25262,.T.);
#33412=ORIENTED_EDGE('',*,*,#25263,.F.);
#33413=ORIENTED_EDGE('',*,*,#25264,.T.);
#33414=ORIENTED_EDGE('',*,*,#25265,.T.);
#33415=ORIENTED_EDGE('',*,*,#25263,.T.);
#33416=ORIENTED_EDGE('',*,*,#25266,.T.);
#33417=ORIENTED_EDGE('',*,*,#25257,.F.);
#33418=ORIENTED_EDGE('',*,*,#25267,.T.);
#33419=ORIENTED_EDGE('',*,*,#25268,.F.);
#33420=ORIENTED_EDGE('',*,*,#25269,.T.);
#33421=ORIENTED_EDGE('',*,*,#25260,.F.);
#33422=ORIENTED_EDGE('',*,*,#25270,.T.);
#33423=ORIENTED_EDGE('',*,*,#25271,.T.);
#33424=ORIENTED_EDGE('',*,*,#25272,.T.);
#33425=ORIENTED_EDGE('',*,*,#25268,.T.);
#33426=ORIENTED_EDGE('',*,*,#25273,.T.);
#33427=ORIENTED_EDGE('',*,*,#25274,.T.);
#33428=ORIENTED_EDGE('',*,*,#25275,.T.);
#33429=ORIENTED_EDGE('',*,*,#25276,.T.);
#33430=ORIENTED_EDGE('',*,*,#25277,.F.);
#33431=ORIENTED_EDGE('',*,*,#25278,.T.);
#33432=ORIENTED_EDGE('',*,*,#25279,.T.);
#33433=ORIENTED_EDGE('',*,*,#25277,.T.);
#33434=ORIENTED_EDGE('',*,*,#25280,.T.);
#33435=ORIENTED_EDGE('',*,*,#25271,.F.);
#33436=ORIENTED_EDGE('',*,*,#25281,.T.);
#33437=ORIENTED_EDGE('',*,*,#25282,.F.);
#33438=ORIENTED_EDGE('',*,*,#25283,.T.);
#33439=ORIENTED_EDGE('',*,*,#25274,.F.);
#33440=ORIENTED_EDGE('',*,*,#25284,.T.);
#33441=ORIENTED_EDGE('',*,*,#25285,.T.);
#33442=ORIENTED_EDGE('',*,*,#25286,.T.);
#33443=ORIENTED_EDGE('',*,*,#25282,.T.);
#33444=ORIENTED_EDGE('',*,*,#25287,.T.);
#33445=ORIENTED_EDGE('',*,*,#25288,.T.);
#33446=ORIENTED_EDGE('',*,*,#25289,.T.);
#33447=ORIENTED_EDGE('',*,*,#25290,.T.);
#33448=ORIENTED_EDGE('',*,*,#25291,.F.);
#33449=ORIENTED_EDGE('',*,*,#25292,.T.);
#33450=ORIENTED_EDGE('',*,*,#25293,.T.);
#33451=ORIENTED_EDGE('',*,*,#25291,.T.);
#33452=ORIENTED_EDGE('',*,*,#25294,.T.);
#33453=ORIENTED_EDGE('',*,*,#25285,.F.);
#33454=ORIENTED_EDGE('',*,*,#25295,.T.);
#33455=ORIENTED_EDGE('',*,*,#25296,.F.);
#33456=ORIENTED_EDGE('',*,*,#25297,.T.);
#33457=ORIENTED_EDGE('',*,*,#25288,.F.);
#33458=ORIENTED_EDGE('',*,*,#25298,.T.);
#33459=ORIENTED_EDGE('',*,*,#25299,.T.);
#33460=ORIENTED_EDGE('',*,*,#25300,.T.);
#33461=ORIENTED_EDGE('',*,*,#25296,.T.);
#33462=ORIENTED_EDGE('',*,*,#25301,.T.);
#33463=ORIENTED_EDGE('',*,*,#25302,.T.);
#33464=ORIENTED_EDGE('',*,*,#25303,.T.);
#33465=ORIENTED_EDGE('',*,*,#25304,.T.);
#33466=ORIENTED_EDGE('',*,*,#25305,.F.);
#33467=ORIENTED_EDGE('',*,*,#25306,.T.);
#33468=ORIENTED_EDGE('',*,*,#25307,.T.);
#33469=ORIENTED_EDGE('',*,*,#25305,.T.);
#33470=ORIENTED_EDGE('',*,*,#25308,.T.);
#33471=ORIENTED_EDGE('',*,*,#25299,.F.);
#33472=ORIENTED_EDGE('',*,*,#25309,.T.);
#33473=ORIENTED_EDGE('',*,*,#25310,.F.);
#33474=ORIENTED_EDGE('',*,*,#25311,.T.);
#33475=ORIENTED_EDGE('',*,*,#25302,.F.);
#33476=ORIENTED_EDGE('',*,*,#25312,.T.);
#33477=ORIENTED_EDGE('',*,*,#25313,.T.);
#33478=ORIENTED_EDGE('',*,*,#25314,.T.);
#33479=ORIENTED_EDGE('',*,*,#25310,.T.);
#33480=ORIENTED_EDGE('',*,*,#25315,.T.);
#33481=ORIENTED_EDGE('',*,*,#25316,.T.);
#33482=ORIENTED_EDGE('',*,*,#25317,.T.);
#33483=ORIENTED_EDGE('',*,*,#25318,.T.);
#33484=ORIENTED_EDGE('',*,*,#25319,.F.);
#33485=ORIENTED_EDGE('',*,*,#25320,.T.);
#33486=ORIENTED_EDGE('',*,*,#25321,.T.);
#33487=ORIENTED_EDGE('',*,*,#25319,.T.);
#33488=ORIENTED_EDGE('',*,*,#25322,.T.);
#33489=ORIENTED_EDGE('',*,*,#25313,.F.);
#33490=ORIENTED_EDGE('',*,*,#25323,.T.);
#33491=ORIENTED_EDGE('',*,*,#21538,.F.);
#33492=ORIENTED_EDGE('',*,*,#25324,.T.);
#33493=ORIENTED_EDGE('',*,*,#25316,.F.);
#33494=ORIENTED_EDGE('',*,*,#25325,.T.);
#33495=ORIENTED_EDGE('',*,*,#21535,.F.);
#33496=ORIENTED_EDGE('',*,*,#25326,.T.);
#33497=ORIENTED_EDGE('',*,*,#25327,.T.);
#33498=ORIENTED_EDGE('',*,*,#25328,.F.);
#33499=ORIENTED_EDGE('',*,*,#25328,.T.);
#33500=ORIENTED_EDGE('',*,*,#25329,.T.);
#33501=ORIENTED_EDGE('',*,*,#21536,.F.);
#33502=ORIENTED_EDGE('',*,*,#25330,.T.);
#33503=ORIENTED_EDGE('',*,*,#25331,.T.);
#33504=ORIENTED_EDGE('',*,*,#21327,.F.);
#33505=ORIENTED_EDGE('',*,*,#25332,.F.);
#33506=ORIENTED_EDGE('',*,*,#25333,.T.);
#33507=ORIENTED_EDGE('',*,*,#25334,.T.);
#33508=ORIENTED_EDGE('',*,*,#25335,.F.);
#33509=ORIENTED_EDGE('',*,*,#25336,.T.);
#33510=ORIENTED_EDGE('',*,*,#25330,.F.);
#33511=ORIENTED_EDGE('',*,*,#25337,.T.);
#33512=ORIENTED_EDGE('',*,*,#25338,.T.);
#33513=ORIENTED_EDGE('',*,*,#25339,.T.);
#33514=ORIENTED_EDGE('',*,*,#25335,.T.);
#33515=ORIENTED_EDGE('',*,*,#25340,.T.);
#33516=ORIENTED_EDGE('',*,*,#25341,.T.);
#33517=ORIENTED_EDGE('',*,*,#25342,.T.);
#33518=ORIENTED_EDGE('',*,*,#25343,.T.);
#33519=ORIENTED_EDGE('',*,*,#25344,.F.);
#33520=ORIENTED_EDGE('',*,*,#25345,.T.);
#33521=ORIENTED_EDGE('',*,*,#25346,.T.);
#33522=ORIENTED_EDGE('',*,*,#25344,.T.);
#33523=ORIENTED_EDGE('',*,*,#25347,.T.);
#33524=ORIENTED_EDGE('',*,*,#25338,.F.);
#33525=ORIENTED_EDGE('',*,*,#25348,.T.);
#33526=ORIENTED_EDGE('',*,*,#21330,.F.);
#33527=ORIENTED_EDGE('',*,*,#25349,.T.);
#33528=ORIENTED_EDGE('',*,*,#25236,.T.);
#33529=ORIENTED_EDGE('',*,*,#25350,.F.);
#33530=ORIENTED_EDGE('',*,*,#25351,.T.);
#33531=ORIENTED_EDGE('',*,*,#25341,.F.);
#33532=ORIENTED_EDGE('',*,*,#25352,.T.);
#33533=ORIENTED_EDGE('',*,*,#25353,.T.);
#33534=ORIENTED_EDGE('',*,*,#25354,.T.);
#33535=ORIENTED_EDGE('',*,*,#25350,.T.);
#33536=ORIENTED_EDGE('',*,*,#25355,.T.);
#33537=ORIENTED_EDGE('',*,*,#25356,.T.);
#33538=ORIENTED_EDGE('',*,*,#25357,.T.);
#33539=ORIENTED_EDGE('',*,*,#25358,.T.);
#33540=ORIENTED_EDGE('',*,*,#25359,.F.);
#33541=ORIENTED_EDGE('',*,*,#25360,.T.);
#33542=ORIENTED_EDGE('',*,*,#25361,.T.);
#33543=ORIENTED_EDGE('',*,*,#25359,.T.);
#33544=ORIENTED_EDGE('',*,*,#25362,.T.);
#33545=ORIENTED_EDGE('',*,*,#25353,.F.);
#33546=ORIENTED_EDGE('',*,*,#25363,.T.);
#33547=ORIENTED_EDGE('',*,*,#25364,.F.);
#33548=ORIENTED_EDGE('',*,*,#25365,.T.);
#33549=ORIENTED_EDGE('',*,*,#25356,.F.);
#33550=ORIENTED_EDGE('',*,*,#25366,.T.);
#33551=ORIENTED_EDGE('',*,*,#25367,.T.);
#33552=ORIENTED_EDGE('',*,*,#25368,.T.);
#33553=ORIENTED_EDGE('',*,*,#25364,.T.);
#33554=ORIENTED_EDGE('',*,*,#25369,.T.);
#33555=ORIENTED_EDGE('',*,*,#25370,.T.);
#33556=ORIENTED_EDGE('',*,*,#25371,.T.);
#33557=ORIENTED_EDGE('',*,*,#25372,.T.);
#33558=ORIENTED_EDGE('',*,*,#25373,.F.);
#33559=ORIENTED_EDGE('',*,*,#25374,.T.);
#33560=ORIENTED_EDGE('',*,*,#25375,.T.);
#33561=ORIENTED_EDGE('',*,*,#25373,.T.);
#33562=ORIENTED_EDGE('',*,*,#25376,.T.);
#33563=ORIENTED_EDGE('',*,*,#25367,.F.);
#33564=ORIENTED_EDGE('',*,*,#25377,.T.);
#33565=ORIENTED_EDGE('',*,*,#25378,.F.);
#33566=ORIENTED_EDGE('',*,*,#25379,.T.);
#33567=ORIENTED_EDGE('',*,*,#25370,.F.);
#33568=ORIENTED_EDGE('',*,*,#25380,.T.);
#33569=ORIENTED_EDGE('',*,*,#25381,.T.);
#33570=ORIENTED_EDGE('',*,*,#25382,.T.);
#33571=ORIENTED_EDGE('',*,*,#25378,.T.);
#33572=ORIENTED_EDGE('',*,*,#25383,.T.);
#33573=ORIENTED_EDGE('',*,*,#25384,.T.);
#33574=ORIENTED_EDGE('',*,*,#25385,.T.);
#33575=ORIENTED_EDGE('',*,*,#25386,.T.);
#33576=ORIENTED_EDGE('',*,*,#25387,.F.);
#33577=ORIENTED_EDGE('',*,*,#25388,.T.);
#33578=ORIENTED_EDGE('',*,*,#25389,.T.);
#33579=ORIENTED_EDGE('',*,*,#25387,.T.);
#33580=ORIENTED_EDGE('',*,*,#25390,.T.);
#33581=ORIENTED_EDGE('',*,*,#25381,.F.);
#33582=ORIENTED_EDGE('',*,*,#25391,.T.);
#33583=ORIENTED_EDGE('',*,*,#25392,.F.);
#33584=ORIENTED_EDGE('',*,*,#25393,.T.);
#33585=ORIENTED_EDGE('',*,*,#25384,.F.);
#33586=ORIENTED_EDGE('',*,*,#25394,.T.);
#33587=ORIENTED_EDGE('',*,*,#25395,.T.);
#33588=ORIENTED_EDGE('',*,*,#25396,.T.);
#33589=ORIENTED_EDGE('',*,*,#25392,.T.);
#33590=ORIENTED_EDGE('',*,*,#25397,.T.);
#33591=ORIENTED_EDGE('',*,*,#25398,.T.);
#33592=ORIENTED_EDGE('',*,*,#25399,.T.);
#33593=ORIENTED_EDGE('',*,*,#25400,.T.);
#33594=ORIENTED_EDGE('',*,*,#25401,.F.);
#33595=ORIENTED_EDGE('',*,*,#25402,.T.);
#33596=ORIENTED_EDGE('',*,*,#25403,.T.);
#33597=ORIENTED_EDGE('',*,*,#25401,.T.);
#33598=ORIENTED_EDGE('',*,*,#25404,.T.);
#33599=ORIENTED_EDGE('',*,*,#25395,.F.);
#33600=ORIENTED_EDGE('',*,*,#25405,.T.);
#33601=ORIENTED_EDGE('',*,*,#25406,.F.);
#33602=ORIENTED_EDGE('',*,*,#25407,.T.);
#33603=ORIENTED_EDGE('',*,*,#25398,.F.);
#33604=ORIENTED_EDGE('',*,*,#25408,.T.);
#33605=ORIENTED_EDGE('',*,*,#25409,.T.);
#33606=ORIENTED_EDGE('',*,*,#25410,.T.);
#33607=ORIENTED_EDGE('',*,*,#25406,.T.);
#33608=ORIENTED_EDGE('',*,*,#25411,.T.);
#33609=ORIENTED_EDGE('',*,*,#25412,.T.);
#33610=ORIENTED_EDGE('',*,*,#25413,.T.);
#33611=ORIENTED_EDGE('',*,*,#25414,.T.);
#33612=ORIENTED_EDGE('',*,*,#25415,.F.);
#33613=ORIENTED_EDGE('',*,*,#25416,.T.);
#33614=ORIENTED_EDGE('',*,*,#25417,.T.);
#33615=ORIENTED_EDGE('',*,*,#25415,.T.);
#33616=ORIENTED_EDGE('',*,*,#25418,.T.);
#33617=ORIENTED_EDGE('',*,*,#25409,.F.);
#33618=ORIENTED_EDGE('',*,*,#25419,.T.);
#33619=ORIENTED_EDGE('',*,*,#21544,.F.);
#33620=ORIENTED_EDGE('',*,*,#25420,.T.);
#33621=ORIENTED_EDGE('',*,*,#25412,.F.);
#33622=ORIENTED_EDGE('',*,*,#25421,.T.);
#33623=ORIENTED_EDGE('',*,*,#21541,.F.);
#33624=ORIENTED_EDGE('',*,*,#25422,.T.);
#33625=ORIENTED_EDGE('',*,*,#25423,.T.);
#33626=ORIENTED_EDGE('',*,*,#25424,.F.);
#33627=ORIENTED_EDGE('',*,*,#25424,.T.);
#33628=ORIENTED_EDGE('',*,*,#25425,.T.);
#33629=ORIENTED_EDGE('',*,*,#21542,.F.);
#33630=ORIENTED_EDGE('',*,*,#25426,.T.);
#33631=ORIENTED_EDGE('',*,*,#25427,.T.);
#33632=ORIENTED_EDGE('',*,*,#21323,.F.);
#33633=ORIENTED_EDGE('',*,*,#25428,.F.);
#33634=ORIENTED_EDGE('',*,*,#25429,.T.);
#33635=ORIENTED_EDGE('',*,*,#25430,.T.);
#33636=ORIENTED_EDGE('',*,*,#25431,.F.);
#33637=ORIENTED_EDGE('',*,*,#25432,.T.);
#33638=ORIENTED_EDGE('',*,*,#25426,.F.);
#33639=ORIENTED_EDGE('',*,*,#25433,.T.);
#33640=ORIENTED_EDGE('',*,*,#25434,.T.);
#33641=ORIENTED_EDGE('',*,*,#25435,.T.);
#33642=ORIENTED_EDGE('',*,*,#25431,.T.);
#33643=ORIENTED_EDGE('',*,*,#25436,.T.);
#33644=ORIENTED_EDGE('',*,*,#25437,.T.);
#33645=ORIENTED_EDGE('',*,*,#25438,.T.);
#33646=ORIENTED_EDGE('',*,*,#25439,.T.);
#33647=ORIENTED_EDGE('',*,*,#25440,.F.);
#33648=ORIENTED_EDGE('',*,*,#25441,.T.);
#33649=ORIENTED_EDGE('',*,*,#25442,.T.);
#33650=ORIENTED_EDGE('',*,*,#25440,.T.);
#33651=ORIENTED_EDGE('',*,*,#25443,.T.);
#33652=ORIENTED_EDGE('',*,*,#25434,.F.);
#33653=ORIENTED_EDGE('',*,*,#25444,.T.);
#33654=ORIENTED_EDGE('',*,*,#21326,.F.);
#33655=ORIENTED_EDGE('',*,*,#25445,.T.);
#33656=ORIENTED_EDGE('',*,*,#25332,.T.);
#33657=ORIENTED_EDGE('',*,*,#25446,.F.);
#33658=ORIENTED_EDGE('',*,*,#25447,.T.);
#33659=ORIENTED_EDGE('',*,*,#25437,.F.);
#33660=ORIENTED_EDGE('',*,*,#25448,.T.);
#33661=ORIENTED_EDGE('',*,*,#25449,.T.);
#33662=ORIENTED_EDGE('',*,*,#25450,.T.);
#33663=ORIENTED_EDGE('',*,*,#25446,.T.);
#33664=ORIENTED_EDGE('',*,*,#25451,.T.);
#33665=ORIENTED_EDGE('',*,*,#25452,.T.);
#33666=ORIENTED_EDGE('',*,*,#25453,.T.);
#33667=ORIENTED_EDGE('',*,*,#25454,.T.);
#33668=ORIENTED_EDGE('',*,*,#25455,.F.);
#33669=ORIENTED_EDGE('',*,*,#25456,.T.);
#33670=ORIENTED_EDGE('',*,*,#25457,.T.);
#33671=ORIENTED_EDGE('',*,*,#25455,.T.);
#33672=ORIENTED_EDGE('',*,*,#25458,.T.);
#33673=ORIENTED_EDGE('',*,*,#25449,.F.);
#33674=ORIENTED_EDGE('',*,*,#25459,.T.);
#33675=ORIENTED_EDGE('',*,*,#25460,.F.);
#33676=ORIENTED_EDGE('',*,*,#25461,.T.);
#33677=ORIENTED_EDGE('',*,*,#25452,.F.);
#33678=ORIENTED_EDGE('',*,*,#25462,.T.);
#33679=ORIENTED_EDGE('',*,*,#25463,.T.);
#33680=ORIENTED_EDGE('',*,*,#25464,.T.);
#33681=ORIENTED_EDGE('',*,*,#25460,.T.);
#33682=ORIENTED_EDGE('',*,*,#25465,.T.);
#33683=ORIENTED_EDGE('',*,*,#25466,.T.);
#33684=ORIENTED_EDGE('',*,*,#25467,.T.);
#33685=ORIENTED_EDGE('',*,*,#25468,.T.);
#33686=ORIENTED_EDGE('',*,*,#25469,.F.);
#33687=ORIENTED_EDGE('',*,*,#25470,.T.);
#33688=ORIENTED_EDGE('',*,*,#25471,.T.);
#33689=ORIENTED_EDGE('',*,*,#25469,.T.);
#33690=ORIENTED_EDGE('',*,*,#25472,.T.);
#33691=ORIENTED_EDGE('',*,*,#25463,.F.);
#33692=ORIENTED_EDGE('',*,*,#25473,.T.);
#33693=ORIENTED_EDGE('',*,*,#25474,.F.);
#33694=ORIENTED_EDGE('',*,*,#25475,.T.);
#33695=ORIENTED_EDGE('',*,*,#25466,.F.);
#33696=ORIENTED_EDGE('',*,*,#25476,.T.);
#33697=ORIENTED_EDGE('',*,*,#25477,.T.);
#33698=ORIENTED_EDGE('',*,*,#25478,.T.);
#33699=ORIENTED_EDGE('',*,*,#25474,.T.);
#33700=ORIENTED_EDGE('',*,*,#25479,.T.);
#33701=ORIENTED_EDGE('',*,*,#25480,.T.);
#33702=ORIENTED_EDGE('',*,*,#25481,.T.);
#33703=ORIENTED_EDGE('',*,*,#25482,.T.);
#33704=ORIENTED_EDGE('',*,*,#25483,.F.);
#33705=ORIENTED_EDGE('',*,*,#25484,.T.);
#33706=ORIENTED_EDGE('',*,*,#25485,.T.);
#33707=ORIENTED_EDGE('',*,*,#25483,.T.);
#33708=ORIENTED_EDGE('',*,*,#25486,.T.);
#33709=ORIENTED_EDGE('',*,*,#25477,.F.);
#33710=ORIENTED_EDGE('',*,*,#25487,.T.);
#33711=ORIENTED_EDGE('',*,*,#25488,.F.);
#33712=ORIENTED_EDGE('',*,*,#25489,.T.);
#33713=ORIENTED_EDGE('',*,*,#25480,.F.);
#33714=ORIENTED_EDGE('',*,*,#25490,.T.);
#33715=ORIENTED_EDGE('',*,*,#25491,.T.);
#33716=ORIENTED_EDGE('',*,*,#25492,.T.);
#33717=ORIENTED_EDGE('',*,*,#25488,.T.);
#33718=ORIENTED_EDGE('',*,*,#25493,.T.);
#33719=ORIENTED_EDGE('',*,*,#25494,.T.);
#33720=ORIENTED_EDGE('',*,*,#25495,.T.);
#33721=ORIENTED_EDGE('',*,*,#25496,.T.);
#33722=ORIENTED_EDGE('',*,*,#25497,.F.);
#33723=ORIENTED_EDGE('',*,*,#25498,.T.);
#33724=ORIENTED_EDGE('',*,*,#25499,.T.);
#33725=ORIENTED_EDGE('',*,*,#25497,.T.);
#33726=ORIENTED_EDGE('',*,*,#25500,.T.);
#33727=ORIENTED_EDGE('',*,*,#25491,.F.);
#33728=ORIENTED_EDGE('',*,*,#25501,.T.);
#33729=ORIENTED_EDGE('',*,*,#25502,.F.);
#33730=ORIENTED_EDGE('',*,*,#25503,.T.);
#33731=ORIENTED_EDGE('',*,*,#25494,.F.);
#33732=ORIENTED_EDGE('',*,*,#25504,.T.);
#33733=ORIENTED_EDGE('',*,*,#25505,.T.);
#33734=ORIENTED_EDGE('',*,*,#25506,.T.);
#33735=ORIENTED_EDGE('',*,*,#25502,.T.);
#33736=ORIENTED_EDGE('',*,*,#25507,.T.);
#33737=ORIENTED_EDGE('',*,*,#25508,.T.);
#33738=ORIENTED_EDGE('',*,*,#25509,.T.);
#33739=ORIENTED_EDGE('',*,*,#25510,.T.);
#33740=ORIENTED_EDGE('',*,*,#25511,.F.);
#33741=ORIENTED_EDGE('',*,*,#25512,.T.);
#33742=ORIENTED_EDGE('',*,*,#25513,.T.);
#33743=ORIENTED_EDGE('',*,*,#25511,.T.);
#33744=ORIENTED_EDGE('',*,*,#25514,.T.);
#33745=ORIENTED_EDGE('',*,*,#25505,.F.);
#33746=ORIENTED_EDGE('',*,*,#25515,.T.);
#33747=ORIENTED_EDGE('',*,*,#21550,.F.);
#33748=ORIENTED_EDGE('',*,*,#25516,.T.);
#33749=ORIENTED_EDGE('',*,*,#25508,.F.);
#33750=ORIENTED_EDGE('',*,*,#25517,.T.);
#33751=ORIENTED_EDGE('',*,*,#21547,.F.);
#33752=ORIENTED_EDGE('',*,*,#25518,.T.);
#33753=ORIENTED_EDGE('',*,*,#25519,.T.);
#33754=ORIENTED_EDGE('',*,*,#25520,.F.);
#33755=ORIENTED_EDGE('',*,*,#25520,.T.);
#33756=ORIENTED_EDGE('',*,*,#25521,.T.);
#33757=ORIENTED_EDGE('',*,*,#21548,.F.);
#33758=ORIENTED_EDGE('',*,*,#25522,.T.);
#33759=ORIENTED_EDGE('',*,*,#25523,.T.);
#33760=ORIENTED_EDGE('',*,*,#21319,.F.);
#33761=ORIENTED_EDGE('',*,*,#25524,.F.);
#33762=ORIENTED_EDGE('',*,*,#25525,.T.);
#33763=ORIENTED_EDGE('',*,*,#25526,.T.);
#33764=ORIENTED_EDGE('',*,*,#25527,.F.);
#33765=ORIENTED_EDGE('',*,*,#25528,.T.);
#33766=ORIENTED_EDGE('',*,*,#25522,.F.);
#33767=ORIENTED_EDGE('',*,*,#25529,.T.);
#33768=ORIENTED_EDGE('',*,*,#25530,.T.);
#33769=ORIENTED_EDGE('',*,*,#25531,.T.);
#33770=ORIENTED_EDGE('',*,*,#25527,.T.);
#33771=ORIENTED_EDGE('',*,*,#25532,.T.);
#33772=ORIENTED_EDGE('',*,*,#25533,.T.);
#33773=ORIENTED_EDGE('',*,*,#25534,.T.);
#33774=ORIENTED_EDGE('',*,*,#25535,.T.);
#33775=ORIENTED_EDGE('',*,*,#25536,.F.);
#33776=ORIENTED_EDGE('',*,*,#25537,.T.);
#33777=ORIENTED_EDGE('',*,*,#25538,.T.);
#33778=ORIENTED_EDGE('',*,*,#25536,.T.);
#33779=ORIENTED_EDGE('',*,*,#25539,.T.);
#33780=ORIENTED_EDGE('',*,*,#25530,.F.);
#33781=ORIENTED_EDGE('',*,*,#25540,.T.);
#33782=ORIENTED_EDGE('',*,*,#21322,.F.);
#33783=ORIENTED_EDGE('',*,*,#25541,.T.);
#33784=ORIENTED_EDGE('',*,*,#25428,.T.);
#33785=ORIENTED_EDGE('',*,*,#25542,.F.);
#33786=ORIENTED_EDGE('',*,*,#25543,.T.);
#33787=ORIENTED_EDGE('',*,*,#25533,.F.);
#33788=ORIENTED_EDGE('',*,*,#25544,.T.);
#33789=ORIENTED_EDGE('',*,*,#25545,.T.);
#33790=ORIENTED_EDGE('',*,*,#25546,.T.);
#33791=ORIENTED_EDGE('',*,*,#25542,.T.);
#33792=ORIENTED_EDGE('',*,*,#25547,.T.);
#33793=ORIENTED_EDGE('',*,*,#25548,.T.);
#33794=ORIENTED_EDGE('',*,*,#25549,.T.);
#33795=ORIENTED_EDGE('',*,*,#25550,.T.);
#33796=ORIENTED_EDGE('',*,*,#25551,.F.);
#33797=ORIENTED_EDGE('',*,*,#25552,.T.);
#33798=ORIENTED_EDGE('',*,*,#25553,.T.);
#33799=ORIENTED_EDGE('',*,*,#25551,.T.);
#33800=ORIENTED_EDGE('',*,*,#25554,.T.);
#33801=ORIENTED_EDGE('',*,*,#25545,.F.);
#33802=ORIENTED_EDGE('',*,*,#25555,.T.);
#33803=ORIENTED_EDGE('',*,*,#25556,.F.);
#33804=ORIENTED_EDGE('',*,*,#25557,.T.);
#33805=ORIENTED_EDGE('',*,*,#25548,.F.);
#33806=ORIENTED_EDGE('',*,*,#25558,.T.);
#33807=ORIENTED_EDGE('',*,*,#25559,.T.);
#33808=ORIENTED_EDGE('',*,*,#25560,.T.);
#33809=ORIENTED_EDGE('',*,*,#25556,.T.);
#33810=ORIENTED_EDGE('',*,*,#25561,.T.);
#33811=ORIENTED_EDGE('',*,*,#25562,.T.);
#33812=ORIENTED_EDGE('',*,*,#25563,.T.);
#33813=ORIENTED_EDGE('',*,*,#25564,.T.);
#33814=ORIENTED_EDGE('',*,*,#25565,.F.);
#33815=ORIENTED_EDGE('',*,*,#25566,.T.);
#33816=ORIENTED_EDGE('',*,*,#25567,.T.);
#33817=ORIENTED_EDGE('',*,*,#25565,.T.);
#33818=ORIENTED_EDGE('',*,*,#25568,.T.);
#33819=ORIENTED_EDGE('',*,*,#25559,.F.);
#33820=ORIENTED_EDGE('',*,*,#25569,.T.);
#33821=ORIENTED_EDGE('',*,*,#25570,.F.);
#33822=ORIENTED_EDGE('',*,*,#25571,.T.);
#33823=ORIENTED_EDGE('',*,*,#25562,.F.);
#33824=ORIENTED_EDGE('',*,*,#25572,.T.);
#33825=ORIENTED_EDGE('',*,*,#25573,.T.);
#33826=ORIENTED_EDGE('',*,*,#25574,.T.);
#33827=ORIENTED_EDGE('',*,*,#25570,.T.);
#33828=ORIENTED_EDGE('',*,*,#25575,.T.);
#33829=ORIENTED_EDGE('',*,*,#25576,.T.);
#33830=ORIENTED_EDGE('',*,*,#25577,.T.);
#33831=ORIENTED_EDGE('',*,*,#25578,.T.);
#33832=ORIENTED_EDGE('',*,*,#25579,.F.);
#33833=ORIENTED_EDGE('',*,*,#25580,.T.);
#33834=ORIENTED_EDGE('',*,*,#25581,.T.);
#33835=ORIENTED_EDGE('',*,*,#25579,.T.);
#33836=ORIENTED_EDGE('',*,*,#25582,.T.);
#33837=ORIENTED_EDGE('',*,*,#25573,.F.);
#33838=ORIENTED_EDGE('',*,*,#25583,.T.);
#33839=ORIENTED_EDGE('',*,*,#25584,.F.);
#33840=ORIENTED_EDGE('',*,*,#25585,.T.);
#33841=ORIENTED_EDGE('',*,*,#25576,.F.);
#33842=ORIENTED_EDGE('',*,*,#25586,.T.);
#33843=ORIENTED_EDGE('',*,*,#25587,.T.);
#33844=ORIENTED_EDGE('',*,*,#25588,.T.);
#33845=ORIENTED_EDGE('',*,*,#25584,.T.);
#33846=ORIENTED_EDGE('',*,*,#25589,.T.);
#33847=ORIENTED_EDGE('',*,*,#25590,.T.);
#33848=ORIENTED_EDGE('',*,*,#25591,.T.);
#33849=ORIENTED_EDGE('',*,*,#25592,.T.);
#33850=ORIENTED_EDGE('',*,*,#25593,.F.);
#33851=ORIENTED_EDGE('',*,*,#25594,.T.);
#33852=ORIENTED_EDGE('',*,*,#25595,.T.);
#33853=ORIENTED_EDGE('',*,*,#25593,.T.);
#33854=ORIENTED_EDGE('',*,*,#25596,.T.);
#33855=ORIENTED_EDGE('',*,*,#25587,.F.);
#33856=ORIENTED_EDGE('',*,*,#25597,.T.);
#33857=ORIENTED_EDGE('',*,*,#25598,.F.);
#33858=ORIENTED_EDGE('',*,*,#25599,.T.);
#33859=ORIENTED_EDGE('',*,*,#25590,.F.);
#33860=ORIENTED_EDGE('',*,*,#25600,.T.);
#33861=ORIENTED_EDGE('',*,*,#25601,.T.);
#33862=ORIENTED_EDGE('',*,*,#25602,.T.);
#33863=ORIENTED_EDGE('',*,*,#25598,.T.);
#33864=ORIENTED_EDGE('',*,*,#25603,.T.);
#33865=ORIENTED_EDGE('',*,*,#25604,.T.);
#33866=ORIENTED_EDGE('',*,*,#25605,.T.);
#33867=ORIENTED_EDGE('',*,*,#25606,.T.);
#33868=ORIENTED_EDGE('',*,*,#25607,.F.);
#33869=ORIENTED_EDGE('',*,*,#25608,.T.);
#33870=ORIENTED_EDGE('',*,*,#25609,.T.);
#33871=ORIENTED_EDGE('',*,*,#25607,.T.);
#33872=ORIENTED_EDGE('',*,*,#25610,.T.);
#33873=ORIENTED_EDGE('',*,*,#25601,.F.);
#33874=ORIENTED_EDGE('',*,*,#25611,.T.);
#33875=ORIENTED_EDGE('',*,*,#21556,.F.);
#33876=ORIENTED_EDGE('',*,*,#25612,.T.);
#33877=ORIENTED_EDGE('',*,*,#25604,.F.);
#33878=ORIENTED_EDGE('',*,*,#25613,.T.);
#33879=ORIENTED_EDGE('',*,*,#21553,.F.);
#33880=ORIENTED_EDGE('',*,*,#25614,.T.);
#33881=ORIENTED_EDGE('',*,*,#25615,.T.);
#33882=ORIENTED_EDGE('',*,*,#25616,.F.);
#33883=ORIENTED_EDGE('',*,*,#25616,.T.);
#33884=ORIENTED_EDGE('',*,*,#25617,.T.);
#33885=ORIENTED_EDGE('',*,*,#21554,.F.);
#33886=ORIENTED_EDGE('',*,*,#25618,.T.);
#33887=ORIENTED_EDGE('',*,*,#25619,.T.);
#33888=ORIENTED_EDGE('',*,*,#21315,.F.);
#33889=ORIENTED_EDGE('',*,*,#25620,.F.);
#33890=ORIENTED_EDGE('',*,*,#25621,.T.);
#33891=ORIENTED_EDGE('',*,*,#25622,.T.);
#33892=ORIENTED_EDGE('',*,*,#25623,.F.);
#33893=ORIENTED_EDGE('',*,*,#25624,.T.);
#33894=ORIENTED_EDGE('',*,*,#25618,.F.);
#33895=ORIENTED_EDGE('',*,*,#25625,.T.);
#33896=ORIENTED_EDGE('',*,*,#25626,.T.);
#33897=ORIENTED_EDGE('',*,*,#25627,.T.);
#33898=ORIENTED_EDGE('',*,*,#25623,.T.);
#33899=ORIENTED_EDGE('',*,*,#25628,.T.);
#33900=ORIENTED_EDGE('',*,*,#25629,.T.);
#33901=ORIENTED_EDGE('',*,*,#25630,.T.);
#33902=ORIENTED_EDGE('',*,*,#25631,.T.);
#33903=ORIENTED_EDGE('',*,*,#25632,.F.);
#33904=ORIENTED_EDGE('',*,*,#25633,.T.);
#33905=ORIENTED_EDGE('',*,*,#25634,.T.);
#33906=ORIENTED_EDGE('',*,*,#25632,.T.);
#33907=ORIENTED_EDGE('',*,*,#25635,.T.);
#33908=ORIENTED_EDGE('',*,*,#25626,.F.);
#33909=ORIENTED_EDGE('',*,*,#25636,.T.);
#33910=ORIENTED_EDGE('',*,*,#21318,.F.);
#33911=ORIENTED_EDGE('',*,*,#25637,.T.);
#33912=ORIENTED_EDGE('',*,*,#25524,.T.);
#33913=ORIENTED_EDGE('',*,*,#25638,.F.);
#33914=ORIENTED_EDGE('',*,*,#25639,.T.);
#33915=ORIENTED_EDGE('',*,*,#25629,.F.);
#33916=ORIENTED_EDGE('',*,*,#25640,.T.);
#33917=ORIENTED_EDGE('',*,*,#25641,.T.);
#33918=ORIENTED_EDGE('',*,*,#25642,.T.);
#33919=ORIENTED_EDGE('',*,*,#25638,.T.);
#33920=ORIENTED_EDGE('',*,*,#25643,.T.);
#33921=ORIENTED_EDGE('',*,*,#25644,.T.);
#33922=ORIENTED_EDGE('',*,*,#25645,.T.);
#33923=ORIENTED_EDGE('',*,*,#25646,.T.);
#33924=ORIENTED_EDGE('',*,*,#25647,.F.);
#33925=ORIENTED_EDGE('',*,*,#25648,.T.);
#33926=ORIENTED_EDGE('',*,*,#25649,.T.);
#33927=ORIENTED_EDGE('',*,*,#25647,.T.);
#33928=ORIENTED_EDGE('',*,*,#25650,.T.);
#33929=ORIENTED_EDGE('',*,*,#25641,.F.);
#33930=ORIENTED_EDGE('',*,*,#25651,.T.);
#33931=ORIENTED_EDGE('',*,*,#25652,.F.);
#33932=ORIENTED_EDGE('',*,*,#25653,.T.);
#33933=ORIENTED_EDGE('',*,*,#25644,.F.);
#33934=ORIENTED_EDGE('',*,*,#25654,.T.);
#33935=ORIENTED_EDGE('',*,*,#25655,.T.);
#33936=ORIENTED_EDGE('',*,*,#25656,.T.);
#33937=ORIENTED_EDGE('',*,*,#25652,.T.);
#33938=ORIENTED_EDGE('',*,*,#25657,.T.);
#33939=ORIENTED_EDGE('',*,*,#25658,.T.);
#33940=ORIENTED_EDGE('',*,*,#25659,.T.);
#33941=ORIENTED_EDGE('',*,*,#25660,.T.);
#33942=ORIENTED_EDGE('',*,*,#25661,.F.);
#33943=ORIENTED_EDGE('',*,*,#25662,.T.);
#33944=ORIENTED_EDGE('',*,*,#25663,.T.);
#33945=ORIENTED_EDGE('',*,*,#25661,.T.);
#33946=ORIENTED_EDGE('',*,*,#25664,.T.);
#33947=ORIENTED_EDGE('',*,*,#25655,.F.);
#33948=ORIENTED_EDGE('',*,*,#25665,.T.);
#33949=ORIENTED_EDGE('',*,*,#25666,.F.);
#33950=ORIENTED_EDGE('',*,*,#25667,.T.);
#33951=ORIENTED_EDGE('',*,*,#25658,.F.);
#33952=ORIENTED_EDGE('',*,*,#25668,.T.);
#33953=ORIENTED_EDGE('',*,*,#25669,.T.);
#33954=ORIENTED_EDGE('',*,*,#25670,.T.);
#33955=ORIENTED_EDGE('',*,*,#25666,.T.);
#33956=ORIENTED_EDGE('',*,*,#25671,.T.);
#33957=ORIENTED_EDGE('',*,*,#25672,.T.);
#33958=ORIENTED_EDGE('',*,*,#25673,.T.);
#33959=ORIENTED_EDGE('',*,*,#25674,.T.);
#33960=ORIENTED_EDGE('',*,*,#25675,.F.);
#33961=ORIENTED_EDGE('',*,*,#25676,.T.);
#33962=ORIENTED_EDGE('',*,*,#25677,.T.);
#33963=ORIENTED_EDGE('',*,*,#25675,.T.);
#33964=ORIENTED_EDGE('',*,*,#25678,.T.);
#33965=ORIENTED_EDGE('',*,*,#25669,.F.);
#33966=ORIENTED_EDGE('',*,*,#25679,.T.);
#33967=ORIENTED_EDGE('',*,*,#25680,.F.);
#33968=ORIENTED_EDGE('',*,*,#25681,.T.);
#33969=ORIENTED_EDGE('',*,*,#25672,.F.);
#33970=ORIENTED_EDGE('',*,*,#25682,.T.);
#33971=ORIENTED_EDGE('',*,*,#25683,.T.);
#33972=ORIENTED_EDGE('',*,*,#25684,.T.);
#33973=ORIENTED_EDGE('',*,*,#25680,.T.);
#33974=ORIENTED_EDGE('',*,*,#25685,.T.);
#33975=ORIENTED_EDGE('',*,*,#25686,.T.);
#33976=ORIENTED_EDGE('',*,*,#25687,.T.);
#33977=ORIENTED_EDGE('',*,*,#25688,.T.);
#33978=ORIENTED_EDGE('',*,*,#25689,.F.);
#33979=ORIENTED_EDGE('',*,*,#25690,.T.);
#33980=ORIENTED_EDGE('',*,*,#25691,.T.);
#33981=ORIENTED_EDGE('',*,*,#25689,.T.);
#33982=ORIENTED_EDGE('',*,*,#25692,.T.);
#33983=ORIENTED_EDGE('',*,*,#25683,.F.);
#33984=ORIENTED_EDGE('',*,*,#25693,.T.);
#33985=ORIENTED_EDGE('',*,*,#25694,.F.);
#33986=ORIENTED_EDGE('',*,*,#25695,.T.);
#33987=ORIENTED_EDGE('',*,*,#25686,.F.);
#33988=ORIENTED_EDGE('',*,*,#25696,.T.);
#33989=ORIENTED_EDGE('',*,*,#25697,.T.);
#33990=ORIENTED_EDGE('',*,*,#25698,.T.);
#33991=ORIENTED_EDGE('',*,*,#25694,.T.);
#33992=ORIENTED_EDGE('',*,*,#25699,.T.);
#33993=ORIENTED_EDGE('',*,*,#25700,.T.);
#33994=ORIENTED_EDGE('',*,*,#25701,.T.);
#33995=ORIENTED_EDGE('',*,*,#25702,.T.);
#33996=ORIENTED_EDGE('',*,*,#25703,.F.);
#33997=ORIENTED_EDGE('',*,*,#25704,.T.);
#33998=ORIENTED_EDGE('',*,*,#25705,.T.);
#33999=ORIENTED_EDGE('',*,*,#25703,.T.);
#34000=ORIENTED_EDGE('',*,*,#25706,.T.);
#34001=ORIENTED_EDGE('',*,*,#25697,.F.);
#34002=ORIENTED_EDGE('',*,*,#25707,.T.);
#34003=ORIENTED_EDGE('',*,*,#21562,.F.);
#34004=ORIENTED_EDGE('',*,*,#25708,.T.);
#34005=ORIENTED_EDGE('',*,*,#25700,.F.);
#34006=ORIENTED_EDGE('',*,*,#25709,.T.);
#34007=ORIENTED_EDGE('',*,*,#21559,.F.);
#34008=ORIENTED_EDGE('',*,*,#25710,.T.);
#34009=ORIENTED_EDGE('',*,*,#25711,.T.);
#34010=ORIENTED_EDGE('',*,*,#25712,.F.);
#34011=ORIENTED_EDGE('',*,*,#25712,.T.);
#34012=ORIENTED_EDGE('',*,*,#25713,.T.);
#34013=ORIENTED_EDGE('',*,*,#21560,.F.);
#34014=ORIENTED_EDGE('',*,*,#25714,.T.);
#34015=ORIENTED_EDGE('',*,*,#25715,.T.);
#34016=ORIENTED_EDGE('',*,*,#21311,.F.);
#34017=ORIENTED_EDGE('',*,*,#25716,.F.);
#34018=ORIENTED_EDGE('',*,*,#25717,.T.);
#34019=ORIENTED_EDGE('',*,*,#25718,.T.);
#34020=ORIENTED_EDGE('',*,*,#25719,.F.);
#34021=ORIENTED_EDGE('',*,*,#25720,.T.);
#34022=ORIENTED_EDGE('',*,*,#25714,.F.);
#34023=ORIENTED_EDGE('',*,*,#25721,.T.);
#34024=ORIENTED_EDGE('',*,*,#25722,.T.);
#34025=ORIENTED_EDGE('',*,*,#25723,.T.);
#34026=ORIENTED_EDGE('',*,*,#25719,.T.);
#34027=ORIENTED_EDGE('',*,*,#25724,.T.);
#34028=ORIENTED_EDGE('',*,*,#25725,.T.);
#34029=ORIENTED_EDGE('',*,*,#25726,.T.);
#34030=ORIENTED_EDGE('',*,*,#25727,.T.);
#34031=ORIENTED_EDGE('',*,*,#25728,.F.);
#34032=ORIENTED_EDGE('',*,*,#25729,.T.);
#34033=ORIENTED_EDGE('',*,*,#25730,.T.);
#34034=ORIENTED_EDGE('',*,*,#25728,.T.);
#34035=ORIENTED_EDGE('',*,*,#25731,.T.);
#34036=ORIENTED_EDGE('',*,*,#25722,.F.);
#34037=ORIENTED_EDGE('',*,*,#25732,.T.);
#34038=ORIENTED_EDGE('',*,*,#21314,.F.);
#34039=ORIENTED_EDGE('',*,*,#25733,.T.);
#34040=ORIENTED_EDGE('',*,*,#25620,.T.);
#34041=ORIENTED_EDGE('',*,*,#25734,.F.);
#34042=ORIENTED_EDGE('',*,*,#25735,.T.);
#34043=ORIENTED_EDGE('',*,*,#25725,.F.);
#34044=ORIENTED_EDGE('',*,*,#25736,.T.);
#34045=ORIENTED_EDGE('',*,*,#25737,.T.);
#34046=ORIENTED_EDGE('',*,*,#25738,.T.);
#34047=ORIENTED_EDGE('',*,*,#25734,.T.);
#34048=ORIENTED_EDGE('',*,*,#25739,.T.);
#34049=ORIENTED_EDGE('',*,*,#25740,.T.);
#34050=ORIENTED_EDGE('',*,*,#25741,.T.);
#34051=ORIENTED_EDGE('',*,*,#25742,.T.);
#34052=ORIENTED_EDGE('',*,*,#25743,.F.);
#34053=ORIENTED_EDGE('',*,*,#25744,.T.);
#34054=ORIENTED_EDGE('',*,*,#25745,.T.);
#34055=ORIENTED_EDGE('',*,*,#25743,.T.);
#34056=ORIENTED_EDGE('',*,*,#25746,.T.);
#34057=ORIENTED_EDGE('',*,*,#25737,.F.);
#34058=ORIENTED_EDGE('',*,*,#25747,.T.);
#34059=ORIENTED_EDGE('',*,*,#25748,.F.);
#34060=ORIENTED_EDGE('',*,*,#25749,.T.);
#34061=ORIENTED_EDGE('',*,*,#25740,.F.);
#34062=ORIENTED_EDGE('',*,*,#25750,.T.);
#34063=ORIENTED_EDGE('',*,*,#25751,.T.);
#34064=ORIENTED_EDGE('',*,*,#25752,.T.);
#34065=ORIENTED_EDGE('',*,*,#25748,.T.);
#34066=ORIENTED_EDGE('',*,*,#25753,.T.);
#34067=ORIENTED_EDGE('',*,*,#25754,.T.);
#34068=ORIENTED_EDGE('',*,*,#25755,.T.);
#34069=ORIENTED_EDGE('',*,*,#25756,.T.);
#34070=ORIENTED_EDGE('',*,*,#25757,.F.);
#34071=ORIENTED_EDGE('',*,*,#25758,.T.);
#34072=ORIENTED_EDGE('',*,*,#25759,.T.);
#34073=ORIENTED_EDGE('',*,*,#25757,.T.);
#34074=ORIENTED_EDGE('',*,*,#25760,.T.);
#34075=ORIENTED_EDGE('',*,*,#25751,.F.);
#34076=ORIENTED_EDGE('',*,*,#25761,.T.);
#34077=ORIENTED_EDGE('',*,*,#25762,.F.);
#34078=ORIENTED_EDGE('',*,*,#25763,.T.);
#34079=ORIENTED_EDGE('',*,*,#25754,.F.);
#34080=ORIENTED_EDGE('',*,*,#25764,.T.);
#34081=ORIENTED_EDGE('',*,*,#25765,.T.);
#34082=ORIENTED_EDGE('',*,*,#25766,.T.);
#34083=ORIENTED_EDGE('',*,*,#25762,.T.);
#34084=ORIENTED_EDGE('',*,*,#25767,.T.);
#34085=ORIENTED_EDGE('',*,*,#25768,.T.);
#34086=ORIENTED_EDGE('',*,*,#25769,.T.);
#34087=ORIENTED_EDGE('',*,*,#25770,.T.);
#34088=ORIENTED_EDGE('',*,*,#25771,.F.);
#34089=ORIENTED_EDGE('',*,*,#25772,.T.);
#34090=ORIENTED_EDGE('',*,*,#25773,.T.);
#34091=ORIENTED_EDGE('',*,*,#25771,.T.);
#34092=ORIENTED_EDGE('',*,*,#25774,.T.);
#34093=ORIENTED_EDGE('',*,*,#25765,.F.);
#34094=ORIENTED_EDGE('',*,*,#25775,.T.);
#34095=ORIENTED_EDGE('',*,*,#25776,.F.);
#34096=ORIENTED_EDGE('',*,*,#25777,.T.);
#34097=ORIENTED_EDGE('',*,*,#25768,.F.);
#34098=ORIENTED_EDGE('',*,*,#25778,.T.);
#34099=ORIENTED_EDGE('',*,*,#25779,.T.);
#34100=ORIENTED_EDGE('',*,*,#25780,.T.);
#34101=ORIENTED_EDGE('',*,*,#25776,.T.);
#34102=ORIENTED_EDGE('',*,*,#25781,.T.);
#34103=ORIENTED_EDGE('',*,*,#25782,.T.);
#34104=ORIENTED_EDGE('',*,*,#25783,.T.);
#34105=ORIENTED_EDGE('',*,*,#25784,.T.);
#34106=ORIENTED_EDGE('',*,*,#25785,.F.);
#34107=ORIENTED_EDGE('',*,*,#25786,.T.);
#34108=ORIENTED_EDGE('',*,*,#25787,.T.);
#34109=ORIENTED_EDGE('',*,*,#25785,.T.);
#34110=ORIENTED_EDGE('',*,*,#25788,.T.);
#34111=ORIENTED_EDGE('',*,*,#25779,.F.);
#34112=ORIENTED_EDGE('',*,*,#25789,.T.);
#34113=ORIENTED_EDGE('',*,*,#25790,.F.);
#34114=ORIENTED_EDGE('',*,*,#25791,.T.);
#34115=ORIENTED_EDGE('',*,*,#25782,.F.);
#34116=ORIENTED_EDGE('',*,*,#25792,.T.);
#34117=ORIENTED_EDGE('',*,*,#25793,.T.);
#34118=ORIENTED_EDGE('',*,*,#25794,.T.);
#34119=ORIENTED_EDGE('',*,*,#25790,.T.);
#34120=ORIENTED_EDGE('',*,*,#25795,.T.);
#34121=ORIENTED_EDGE('',*,*,#25796,.T.);
#34122=ORIENTED_EDGE('',*,*,#25797,.T.);
#34123=ORIENTED_EDGE('',*,*,#25798,.T.);
#34124=ORIENTED_EDGE('',*,*,#25799,.F.);
#34125=ORIENTED_EDGE('',*,*,#25800,.T.);
#34126=ORIENTED_EDGE('',*,*,#25801,.T.);
#34127=ORIENTED_EDGE('',*,*,#25799,.T.);
#34128=ORIENTED_EDGE('',*,*,#25802,.T.);
#34129=ORIENTED_EDGE('',*,*,#25793,.F.);
#34130=ORIENTED_EDGE('',*,*,#25803,.T.);
#34131=ORIENTED_EDGE('',*,*,#21568,.F.);
#34132=ORIENTED_EDGE('',*,*,#25804,.T.);
#34133=ORIENTED_EDGE('',*,*,#25796,.F.);
#34134=ORIENTED_EDGE('',*,*,#25805,.T.);
#34135=ORIENTED_EDGE('',*,*,#21565,.F.);
#34136=ORIENTED_EDGE('',*,*,#25806,.T.);
#34137=ORIENTED_EDGE('',*,*,#25807,.T.);
#34138=ORIENTED_EDGE('',*,*,#25808,.F.);
#34139=ORIENTED_EDGE('',*,*,#25808,.T.);
#34140=ORIENTED_EDGE('',*,*,#25809,.T.);
#34141=ORIENTED_EDGE('',*,*,#21566,.F.);
#34142=ORIENTED_EDGE('',*,*,#25810,.T.);
#34143=ORIENTED_EDGE('',*,*,#25811,.T.);
#34144=ORIENTED_EDGE('',*,*,#21307,.F.);
#34145=ORIENTED_EDGE('',*,*,#25812,.F.);
#34146=ORIENTED_EDGE('',*,*,#25813,.T.);
#34147=ORIENTED_EDGE('',*,*,#25814,.T.);
#34148=ORIENTED_EDGE('',*,*,#25815,.F.);
#34149=ORIENTED_EDGE('',*,*,#25816,.T.);
#34150=ORIENTED_EDGE('',*,*,#25810,.F.);
#34151=ORIENTED_EDGE('',*,*,#25817,.T.);
#34152=ORIENTED_EDGE('',*,*,#25818,.T.);
#34153=ORIENTED_EDGE('',*,*,#25819,.T.);
#34154=ORIENTED_EDGE('',*,*,#25815,.T.);
#34155=ORIENTED_EDGE('',*,*,#25820,.T.);
#34156=ORIENTED_EDGE('',*,*,#25821,.T.);
#34157=ORIENTED_EDGE('',*,*,#25822,.T.);
#34158=ORIENTED_EDGE('',*,*,#25823,.T.);
#34159=ORIENTED_EDGE('',*,*,#25824,.F.);
#34160=ORIENTED_EDGE('',*,*,#25825,.T.);
#34161=ORIENTED_EDGE('',*,*,#25826,.T.);
#34162=ORIENTED_EDGE('',*,*,#25824,.T.);
#34163=ORIENTED_EDGE('',*,*,#25827,.T.);
#34164=ORIENTED_EDGE('',*,*,#25818,.F.);
#34165=ORIENTED_EDGE('',*,*,#25828,.T.);
#34166=ORIENTED_EDGE('',*,*,#21310,.F.);
#34167=ORIENTED_EDGE('',*,*,#25829,.T.);
#34168=ORIENTED_EDGE('',*,*,#25716,.T.);
#34169=ORIENTED_EDGE('',*,*,#25830,.F.);
#34170=ORIENTED_EDGE('',*,*,#25831,.T.);
#34171=ORIENTED_EDGE('',*,*,#25821,.F.);
#34172=ORIENTED_EDGE('',*,*,#25832,.T.);
#34173=ORIENTED_EDGE('',*,*,#25833,.T.);
#34174=ORIENTED_EDGE('',*,*,#25834,.T.);
#34175=ORIENTED_EDGE('',*,*,#25830,.T.);
#34176=ORIENTED_EDGE('',*,*,#25835,.T.);
#34177=ORIENTED_EDGE('',*,*,#25836,.T.);
#34178=ORIENTED_EDGE('',*,*,#25837,.T.);
#34179=ORIENTED_EDGE('',*,*,#25838,.T.);
#34180=ORIENTED_EDGE('',*,*,#25839,.F.);
#34181=ORIENTED_EDGE('',*,*,#25840,.T.);
#34182=ORIENTED_EDGE('',*,*,#25841,.T.);
#34183=ORIENTED_EDGE('',*,*,#25839,.T.);
#34184=ORIENTED_EDGE('',*,*,#25842,.T.);
#34185=ORIENTED_EDGE('',*,*,#25833,.F.);
#34186=ORIENTED_EDGE('',*,*,#25843,.T.);
#34187=ORIENTED_EDGE('',*,*,#25844,.F.);
#34188=ORIENTED_EDGE('',*,*,#25845,.T.);
#34189=ORIENTED_EDGE('',*,*,#25836,.F.);
#34190=ORIENTED_EDGE('',*,*,#25846,.T.);
#34191=ORIENTED_EDGE('',*,*,#25847,.T.);
#34192=ORIENTED_EDGE('',*,*,#25848,.T.);
#34193=ORIENTED_EDGE('',*,*,#25844,.T.);
#34194=ORIENTED_EDGE('',*,*,#25849,.T.);
#34195=ORIENTED_EDGE('',*,*,#25850,.T.);
#34196=ORIENTED_EDGE('',*,*,#25851,.T.);
#34197=ORIENTED_EDGE('',*,*,#25852,.T.);
#34198=ORIENTED_EDGE('',*,*,#25853,.F.);
#34199=ORIENTED_EDGE('',*,*,#25854,.T.);
#34200=ORIENTED_EDGE('',*,*,#25855,.T.);
#34201=ORIENTED_EDGE('',*,*,#25853,.T.);
#34202=ORIENTED_EDGE('',*,*,#25856,.T.);
#34203=ORIENTED_EDGE('',*,*,#25847,.F.);
#34204=ORIENTED_EDGE('',*,*,#25857,.T.);
#34205=ORIENTED_EDGE('',*,*,#25858,.F.);
#34206=ORIENTED_EDGE('',*,*,#25859,.T.);
#34207=ORIENTED_EDGE('',*,*,#25850,.F.);
#34208=ORIENTED_EDGE('',*,*,#25860,.T.);
#34209=ORIENTED_EDGE('',*,*,#25861,.T.);
#34210=ORIENTED_EDGE('',*,*,#25862,.T.);
#34211=ORIENTED_EDGE('',*,*,#25858,.T.);
#34212=ORIENTED_EDGE('',*,*,#25863,.T.);
#34213=ORIENTED_EDGE('',*,*,#25864,.T.);
#34214=ORIENTED_EDGE('',*,*,#25865,.T.);
#34215=ORIENTED_EDGE('',*,*,#25866,.T.);
#34216=ORIENTED_EDGE('',*,*,#25867,.F.);
#34217=ORIENTED_EDGE('',*,*,#25868,.T.);
#34218=ORIENTED_EDGE('',*,*,#25869,.T.);
#34219=ORIENTED_EDGE('',*,*,#25867,.T.);
#34220=ORIENTED_EDGE('',*,*,#25870,.T.);
#34221=ORIENTED_EDGE('',*,*,#25861,.F.);
#34222=ORIENTED_EDGE('',*,*,#25871,.T.);
#34223=ORIENTED_EDGE('',*,*,#25872,.F.);
#34224=ORIENTED_EDGE('',*,*,#25873,.T.);
#34225=ORIENTED_EDGE('',*,*,#25864,.F.);
#34226=ORIENTED_EDGE('',*,*,#25874,.T.);
#34227=ORIENTED_EDGE('',*,*,#25875,.T.);
#34228=ORIENTED_EDGE('',*,*,#25876,.T.);
#34229=ORIENTED_EDGE('',*,*,#25872,.T.);
#34230=ORIENTED_EDGE('',*,*,#25877,.T.);
#34231=ORIENTED_EDGE('',*,*,#25878,.T.);
#34232=ORIENTED_EDGE('',*,*,#25879,.T.);
#34233=ORIENTED_EDGE('',*,*,#25880,.T.);
#34234=ORIENTED_EDGE('',*,*,#25881,.F.);
#34235=ORIENTED_EDGE('',*,*,#25882,.T.);
#34236=ORIENTED_EDGE('',*,*,#25883,.T.);
#34237=ORIENTED_EDGE('',*,*,#25881,.T.);
#34238=ORIENTED_EDGE('',*,*,#25884,.T.);
#34239=ORIENTED_EDGE('',*,*,#25875,.F.);
#34240=ORIENTED_EDGE('',*,*,#25885,.T.);
#34241=ORIENTED_EDGE('',*,*,#25886,.F.);
#34242=ORIENTED_EDGE('',*,*,#25887,.T.);
#34243=ORIENTED_EDGE('',*,*,#25878,.F.);
#34244=ORIENTED_EDGE('',*,*,#25888,.T.);
#34245=ORIENTED_EDGE('',*,*,#25889,.T.);
#34246=ORIENTED_EDGE('',*,*,#25890,.T.);
#34247=ORIENTED_EDGE('',*,*,#25886,.T.);
#34248=ORIENTED_EDGE('',*,*,#25891,.T.);
#34249=ORIENTED_EDGE('',*,*,#25892,.T.);
#34250=ORIENTED_EDGE('',*,*,#25893,.T.);
#34251=ORIENTED_EDGE('',*,*,#25894,.T.);
#34252=ORIENTED_EDGE('',*,*,#25895,.F.);
#34253=ORIENTED_EDGE('',*,*,#25896,.T.);
#34254=ORIENTED_EDGE('',*,*,#25897,.T.);
#34255=ORIENTED_EDGE('',*,*,#25895,.T.);
#34256=ORIENTED_EDGE('',*,*,#25898,.T.);
#34257=ORIENTED_EDGE('',*,*,#25889,.F.);
#34258=ORIENTED_EDGE('',*,*,#25899,.T.);
#34259=ORIENTED_EDGE('',*,*,#21574,.F.);
#34260=ORIENTED_EDGE('',*,*,#25900,.T.);
#34261=ORIENTED_EDGE('',*,*,#25892,.F.);
#34262=ORIENTED_EDGE('',*,*,#25901,.T.);
#34263=ORIENTED_EDGE('',*,*,#21571,.F.);
#34264=ORIENTED_EDGE('',*,*,#25902,.T.);
#34265=ORIENTED_EDGE('',*,*,#25903,.T.);
#34266=ORIENTED_EDGE('',*,*,#25904,.F.);
#34267=ORIENTED_EDGE('',*,*,#25904,.T.);
#34268=ORIENTED_EDGE('',*,*,#25905,.T.);
#34269=ORIENTED_EDGE('',*,*,#21572,.F.);
#34270=ORIENTED_EDGE('',*,*,#25906,.T.);
#34271=ORIENTED_EDGE('',*,*,#25907,.T.);
#34272=ORIENTED_EDGE('',*,*,#21303,.F.);
#34273=ORIENTED_EDGE('',*,*,#25908,.F.);
#34274=ORIENTED_EDGE('',*,*,#25909,.T.);
#34275=ORIENTED_EDGE('',*,*,#25910,.T.);
#34276=ORIENTED_EDGE('',*,*,#25911,.F.);
#34277=ORIENTED_EDGE('',*,*,#25912,.T.);
#34278=ORIENTED_EDGE('',*,*,#25906,.F.);
#34279=ORIENTED_EDGE('',*,*,#25913,.T.);
#34280=ORIENTED_EDGE('',*,*,#25914,.T.);
#34281=ORIENTED_EDGE('',*,*,#25915,.T.);
#34282=ORIENTED_EDGE('',*,*,#25911,.T.);
#34283=ORIENTED_EDGE('',*,*,#25916,.T.);
#34284=ORIENTED_EDGE('',*,*,#25917,.T.);
#34285=ORIENTED_EDGE('',*,*,#25918,.T.);
#34286=ORIENTED_EDGE('',*,*,#25919,.T.);
#34287=ORIENTED_EDGE('',*,*,#25920,.F.);
#34288=ORIENTED_EDGE('',*,*,#25921,.T.);
#34289=ORIENTED_EDGE('',*,*,#25922,.T.);
#34290=ORIENTED_EDGE('',*,*,#25920,.T.);
#34291=ORIENTED_EDGE('',*,*,#25923,.T.);
#34292=ORIENTED_EDGE('',*,*,#25914,.F.);
#34293=ORIENTED_EDGE('',*,*,#25924,.T.);
#34294=ORIENTED_EDGE('',*,*,#21306,.F.);
#34295=ORIENTED_EDGE('',*,*,#25925,.T.);
#34296=ORIENTED_EDGE('',*,*,#25812,.T.);
#34297=ORIENTED_EDGE('',*,*,#25926,.F.);
#34298=ORIENTED_EDGE('',*,*,#25927,.T.);
#34299=ORIENTED_EDGE('',*,*,#25917,.F.);
#34300=ORIENTED_EDGE('',*,*,#25928,.T.);
#34301=ORIENTED_EDGE('',*,*,#25929,.T.);
#34302=ORIENTED_EDGE('',*,*,#25930,.T.);
#34303=ORIENTED_EDGE('',*,*,#25926,.T.);
#34304=ORIENTED_EDGE('',*,*,#25931,.T.);
#34305=ORIENTED_EDGE('',*,*,#25932,.T.);
#34306=ORIENTED_EDGE('',*,*,#25933,.T.);
#34307=ORIENTED_EDGE('',*,*,#25934,.T.);
#34308=ORIENTED_EDGE('',*,*,#25935,.F.);
#34309=ORIENTED_EDGE('',*,*,#25936,.T.);
#34310=ORIENTED_EDGE('',*,*,#25937,.T.);
#34311=ORIENTED_EDGE('',*,*,#25935,.T.);
#34312=ORIENTED_EDGE('',*,*,#25938,.T.);
#34313=ORIENTED_EDGE('',*,*,#25929,.F.);
#34314=ORIENTED_EDGE('',*,*,#25939,.T.);
#34315=ORIENTED_EDGE('',*,*,#25940,.F.);
#34316=ORIENTED_EDGE('',*,*,#25941,.T.);
#34317=ORIENTED_EDGE('',*,*,#25932,.F.);
#34318=ORIENTED_EDGE('',*,*,#25942,.T.);
#34319=ORIENTED_EDGE('',*,*,#25943,.T.);
#34320=ORIENTED_EDGE('',*,*,#25944,.T.);
#34321=ORIENTED_EDGE('',*,*,#25940,.T.);
#34322=ORIENTED_EDGE('',*,*,#25945,.T.);
#34323=ORIENTED_EDGE('',*,*,#25946,.T.);
#34324=ORIENTED_EDGE('',*,*,#25947,.T.);
#34325=ORIENTED_EDGE('',*,*,#25948,.T.);
#34326=ORIENTED_EDGE('',*,*,#25949,.F.);
#34327=ORIENTED_EDGE('',*,*,#25950,.T.);
#34328=ORIENTED_EDGE('',*,*,#25951,.T.);
#34329=ORIENTED_EDGE('',*,*,#25949,.T.);
#34330=ORIENTED_EDGE('',*,*,#25952,.T.);
#34331=ORIENTED_EDGE('',*,*,#25943,.F.);
#34332=ORIENTED_EDGE('',*,*,#25953,.T.);
#34333=ORIENTED_EDGE('',*,*,#25954,.F.);
#34334=ORIENTED_EDGE('',*,*,#25955,.T.);
#34335=ORIENTED_EDGE('',*,*,#25946,.F.);
#34336=ORIENTED_EDGE('',*,*,#25956,.T.);
#34337=ORIENTED_EDGE('',*,*,#25957,.T.);
#34338=ORIENTED_EDGE('',*,*,#25958,.T.);
#34339=ORIENTED_EDGE('',*,*,#25954,.T.);
#34340=ORIENTED_EDGE('',*,*,#25959,.T.);
#34341=ORIENTED_EDGE('',*,*,#25960,.T.);
#34342=ORIENTED_EDGE('',*,*,#25961,.T.);
#34343=ORIENTED_EDGE('',*,*,#25962,.T.);
#34344=ORIENTED_EDGE('',*,*,#25963,.F.);
#34345=ORIENTED_EDGE('',*,*,#25964,.T.);
#34346=ORIENTED_EDGE('',*,*,#25965,.T.);
#34347=ORIENTED_EDGE('',*,*,#25963,.T.);
#34348=ORIENTED_EDGE('',*,*,#25966,.T.);
#34349=ORIENTED_EDGE('',*,*,#25957,.F.);
#34350=ORIENTED_EDGE('',*,*,#25967,.T.);
#34351=ORIENTED_EDGE('',*,*,#25968,.F.);
#34352=ORIENTED_EDGE('',*,*,#25969,.T.);
#34353=ORIENTED_EDGE('',*,*,#25960,.F.);
#34354=ORIENTED_EDGE('',*,*,#25970,.T.);
#34355=ORIENTED_EDGE('',*,*,#25971,.T.);
#34356=ORIENTED_EDGE('',*,*,#25972,.T.);
#34357=ORIENTED_EDGE('',*,*,#25968,.T.);
#34358=ORIENTED_EDGE('',*,*,#25973,.T.);
#34359=ORIENTED_EDGE('',*,*,#25974,.T.);
#34360=ORIENTED_EDGE('',*,*,#25975,.T.);
#34361=ORIENTED_EDGE('',*,*,#25976,.T.);
#34362=ORIENTED_EDGE('',*,*,#25977,.F.);
#34363=ORIENTED_EDGE('',*,*,#25978,.T.);
#34364=ORIENTED_EDGE('',*,*,#25979,.T.);
#34365=ORIENTED_EDGE('',*,*,#25977,.T.);
#34366=ORIENTED_EDGE('',*,*,#25980,.T.);
#34367=ORIENTED_EDGE('',*,*,#25971,.F.);
#34368=ORIENTED_EDGE('',*,*,#25981,.T.);
#34369=ORIENTED_EDGE('',*,*,#25982,.F.);
#34370=ORIENTED_EDGE('',*,*,#25983,.T.);
#34371=ORIENTED_EDGE('',*,*,#25974,.F.);
#34372=ORIENTED_EDGE('',*,*,#25984,.T.);
#34373=ORIENTED_EDGE('',*,*,#25985,.T.);
#34374=ORIENTED_EDGE('',*,*,#25986,.T.);
#34375=ORIENTED_EDGE('',*,*,#25982,.T.);
#34376=ORIENTED_EDGE('',*,*,#25987,.T.);
#34377=ORIENTED_EDGE('',*,*,#25988,.T.);
#34378=ORIENTED_EDGE('',*,*,#25989,.T.);
#34379=ORIENTED_EDGE('',*,*,#25990,.T.);
#34380=ORIENTED_EDGE('',*,*,#25991,.F.);
#34381=ORIENTED_EDGE('',*,*,#25992,.T.);
#34382=ORIENTED_EDGE('',*,*,#25993,.T.);
#34383=ORIENTED_EDGE('',*,*,#25991,.T.);
#34384=ORIENTED_EDGE('',*,*,#25994,.T.);
#34385=ORIENTED_EDGE('',*,*,#25985,.F.);
#34386=ORIENTED_EDGE('',*,*,#25995,.T.);
#34387=ORIENTED_EDGE('',*,*,#21580,.F.);
#34388=ORIENTED_EDGE('',*,*,#25996,.T.);
#34389=ORIENTED_EDGE('',*,*,#25988,.F.);
#34390=ORIENTED_EDGE('',*,*,#25997,.T.);
#34391=ORIENTED_EDGE('',*,*,#21577,.F.);
#34392=ORIENTED_EDGE('',*,*,#25998,.T.);
#34393=ORIENTED_EDGE('',*,*,#25999,.T.);
#34394=ORIENTED_EDGE('',*,*,#26000,.F.);
#34395=ORIENTED_EDGE('',*,*,#26000,.T.);
#34396=ORIENTED_EDGE('',*,*,#26001,.T.);
#34397=ORIENTED_EDGE('',*,*,#21578,.F.);
#34398=ORIENTED_EDGE('',*,*,#26002,.T.);
#34399=ORIENTED_EDGE('',*,*,#26003,.T.);
#34400=ORIENTED_EDGE('',*,*,#26004,.T.);
#34401=ORIENTED_EDGE('',*,*,#26005,.T.);
#34402=ORIENTED_EDGE('',*,*,#26006,.T.);
#34403=ORIENTED_EDGE('',*,*,#26007,.T.);
#34404=ORIENTED_EDGE('',*,*,#21299,.F.);
#34405=ORIENTED_EDGE('',*,*,#26008,.F.);
#34406=ORIENTED_EDGE('',*,*,#26009,.T.);
#34407=ORIENTED_EDGE('',*,*,#26010,.T.);
#34408=ORIENTED_EDGE('',*,*,#26004,.F.);
#34409=ORIENTED_EDGE('',*,*,#26011,.T.);
#34410=ORIENTED_EDGE('',*,*,#26006,.F.);
#34411=ORIENTED_EDGE('',*,*,#26012,.T.);
#34412=ORIENTED_EDGE('',*,*,#26013,.T.);
#34413=ORIENTED_EDGE('',*,*,#26014,.T.);
#34414=ORIENTED_EDGE('',*,*,#26015,.T.);
#34415=ORIENTED_EDGE('',*,*,#26016,.F.);
#34416=ORIENTED_EDGE('',*,*,#26017,.T.);
#34417=ORIENTED_EDGE('',*,*,#26018,.T.);
#34418=ORIENTED_EDGE('',*,*,#26016,.T.);
#34419=ORIENTED_EDGE('',*,*,#26019,.T.);
#34420=ORIENTED_EDGE('',*,*,#26002,.F.);
#34421=ORIENTED_EDGE('',*,*,#26020,.T.);
#34422=ORIENTED_EDGE('',*,*,#21302,.F.);
#34423=ORIENTED_EDGE('',*,*,#26021,.T.);
#34424=ORIENTED_EDGE('',*,*,#25908,.T.);
#34425=ORIENTED_EDGE('',*,*,#26022,.F.);
#34426=ORIENTED_EDGE('',*,*,#26023,.T.);
#34427=ORIENTED_EDGE('',*,*,#26013,.F.);
#34428=ORIENTED_EDGE('',*,*,#26024,.T.);
#34429=ORIENTED_EDGE('',*,*,#26025,.T.);
#34430=ORIENTED_EDGE('',*,*,#26026,.T.);
#34431=ORIENTED_EDGE('',*,*,#26022,.T.);
#34432=ORIENTED_EDGE('',*,*,#26027,.T.);
#34433=ORIENTED_EDGE('',*,*,#26028,.T.);
#34434=ORIENTED_EDGE('',*,*,#26029,.T.);
#34435=ORIENTED_EDGE('',*,*,#26030,.T.);
#34436=ORIENTED_EDGE('',*,*,#26031,.F.);
#34437=ORIENTED_EDGE('',*,*,#26032,.T.);
#34438=ORIENTED_EDGE('',*,*,#26033,.T.);
#34439=ORIENTED_EDGE('',*,*,#26031,.T.);
#34440=ORIENTED_EDGE('',*,*,#26034,.T.);
#34441=ORIENTED_EDGE('',*,*,#26025,.F.);
#34442=ORIENTED_EDGE('',*,*,#26035,.T.);
#34443=ORIENTED_EDGE('',*,*,#26036,.F.);
#34444=ORIENTED_EDGE('',*,*,#26037,.T.);
#34445=ORIENTED_EDGE('',*,*,#26028,.F.);
#34446=ORIENTED_EDGE('',*,*,#26038,.T.);
#34447=ORIENTED_EDGE('',*,*,#26039,.T.);
#34448=ORIENTED_EDGE('',*,*,#26040,.T.);
#34449=ORIENTED_EDGE('',*,*,#26036,.T.);
#34450=ORIENTED_EDGE('',*,*,#26041,.T.);
#34451=ORIENTED_EDGE('',*,*,#26042,.T.);
#34452=ORIENTED_EDGE('',*,*,#26043,.T.);
#34453=ORIENTED_EDGE('',*,*,#26044,.T.);
#34454=ORIENTED_EDGE('',*,*,#26045,.F.);
#34455=ORIENTED_EDGE('',*,*,#26046,.T.);
#34456=ORIENTED_EDGE('',*,*,#26047,.T.);
#34457=ORIENTED_EDGE('',*,*,#26045,.T.);
#34458=ORIENTED_EDGE('',*,*,#26048,.T.);
#34459=ORIENTED_EDGE('',*,*,#26039,.F.);
#34460=ORIENTED_EDGE('',*,*,#26049,.T.);
#34461=ORIENTED_EDGE('',*,*,#26050,.F.);
#34462=ORIENTED_EDGE('',*,*,#26051,.T.);
#34463=ORIENTED_EDGE('',*,*,#26042,.F.);
#34464=ORIENTED_EDGE('',*,*,#26052,.T.);
#34465=ORIENTED_EDGE('',*,*,#26053,.T.);
#34466=ORIENTED_EDGE('',*,*,#26054,.T.);
#34467=ORIENTED_EDGE('',*,*,#26050,.T.);
#34468=ORIENTED_EDGE('',*,*,#26055,.T.);
#34469=ORIENTED_EDGE('',*,*,#26056,.T.);
#34470=ORIENTED_EDGE('',*,*,#26057,.T.);
#34471=ORIENTED_EDGE('',*,*,#26058,.T.);
#34472=ORIENTED_EDGE('',*,*,#26059,.F.);
#34473=ORIENTED_EDGE('',*,*,#26060,.T.);
#34474=ORIENTED_EDGE('',*,*,#26061,.T.);
#34475=ORIENTED_EDGE('',*,*,#26059,.T.);
#34476=ORIENTED_EDGE('',*,*,#26062,.T.);
#34477=ORIENTED_EDGE('',*,*,#26053,.F.);
#34478=ORIENTED_EDGE('',*,*,#26063,.T.);
#34479=ORIENTED_EDGE('',*,*,#26064,.F.);
#34480=ORIENTED_EDGE('',*,*,#26065,.T.);
#34481=ORIENTED_EDGE('',*,*,#26056,.F.);
#34482=ORIENTED_EDGE('',*,*,#26066,.T.);
#34483=ORIENTED_EDGE('',*,*,#26067,.T.);
#34484=ORIENTED_EDGE('',*,*,#26068,.T.);
#34485=ORIENTED_EDGE('',*,*,#26064,.T.);
#34486=ORIENTED_EDGE('',*,*,#26069,.T.);
#34487=ORIENTED_EDGE('',*,*,#26070,.T.);
#34488=ORIENTED_EDGE('',*,*,#26071,.T.);
#34489=ORIENTED_EDGE('',*,*,#26072,.T.);
#34490=ORIENTED_EDGE('',*,*,#26073,.F.);
#34491=ORIENTED_EDGE('',*,*,#26074,.T.);
#34492=ORIENTED_EDGE('',*,*,#26075,.T.);
#34493=ORIENTED_EDGE('',*,*,#26073,.T.);
#34494=ORIENTED_EDGE('',*,*,#26076,.T.);
#34495=ORIENTED_EDGE('',*,*,#26067,.F.);
#34496=ORIENTED_EDGE('',*,*,#26077,.T.);
#34497=ORIENTED_EDGE('',*,*,#26078,.F.);
#34498=ORIENTED_EDGE('',*,*,#26079,.T.);
#34499=ORIENTED_EDGE('',*,*,#26070,.F.);
#34500=ORIENTED_EDGE('',*,*,#26080,.T.);
#34501=ORIENTED_EDGE('',*,*,#26081,.T.);
#34502=ORIENTED_EDGE('',*,*,#26082,.T.);
#34503=ORIENTED_EDGE('',*,*,#26078,.T.);
#34504=ORIENTED_EDGE('',*,*,#26083,.T.);
#34505=ORIENTED_EDGE('',*,*,#26084,.T.);
#34506=ORIENTED_EDGE('',*,*,#26085,.T.);
#34507=ORIENTED_EDGE('',*,*,#26086,.T.);
#34508=ORIENTED_EDGE('',*,*,#26087,.F.);
#34509=ORIENTED_EDGE('',*,*,#26088,.T.);
#34510=ORIENTED_EDGE('',*,*,#26089,.T.);
#34511=ORIENTED_EDGE('',*,*,#26087,.T.);
#34512=ORIENTED_EDGE('',*,*,#26090,.T.);
#34513=ORIENTED_EDGE('',*,*,#26081,.F.);
#34514=ORIENTED_EDGE('',*,*,#26091,.T.);
#34515=ORIENTED_EDGE('',*,*,#21586,.F.);
#34516=ORIENTED_EDGE('',*,*,#26092,.T.);
#34517=ORIENTED_EDGE('',*,*,#26084,.F.);
#34518=ORIENTED_EDGE('',*,*,#26093,.T.);
#34519=ORIENTED_EDGE('',*,*,#21583,.F.);
#34520=ORIENTED_EDGE('',*,*,#26094,.T.);
#34521=ORIENTED_EDGE('',*,*,#26095,.T.);
#34522=ORIENTED_EDGE('',*,*,#26096,.F.);
#34523=ORIENTED_EDGE('',*,*,#26096,.T.);
#34524=ORIENTED_EDGE('',*,*,#26097,.T.);
#34525=ORIENTED_EDGE('',*,*,#21584,.F.);
#34526=ORIENTED_EDGE('',*,*,#26098,.T.);
#34527=ORIENTED_EDGE('',*,*,#26099,.T.);
#34528=ORIENTED_EDGE('',*,*,#26100,.T.);
#34529=ORIENTED_EDGE('',*,*,#26101,.T.);
#34530=ORIENTED_EDGE('',*,*,#26102,.T.);
#34531=ORIENTED_EDGE('',*,*,#26103,.T.);
#34532=ORIENTED_EDGE('',*,*,#26104,.T.);
#34533=ORIENTED_EDGE('',*,*,#26105,.T.);
#34534=ORIENTED_EDGE('',*,*,#26106,.T.);
#34535=ORIENTED_EDGE('',*,*,#26107,.T.);
#34536=ORIENTED_EDGE('',*,*,#21295,.F.);
#34537=ORIENTED_EDGE('',*,*,#26108,.F.);
#34538=ORIENTED_EDGE('',*,*,#26109,.T.);
#34539=ORIENTED_EDGE('',*,*,#26110,.T.);
#34540=ORIENTED_EDGE('',*,*,#26104,.F.);
#34541=ORIENTED_EDGE('',*,*,#26111,.T.);
#34542=ORIENTED_EDGE('',*,*,#26106,.F.);
#34543=ORIENTED_EDGE('',*,*,#26112,.T.);
#34544=ORIENTED_EDGE('',*,*,#26113,.T.);
#34545=ORIENTED_EDGE('',*,*,#26114,.T.);
#34546=ORIENTED_EDGE('',*,*,#26115,.T.);
#34547=ORIENTED_EDGE('',*,*,#26116,.F.);
#34548=ORIENTED_EDGE('',*,*,#26117,.T.);
#34549=ORIENTED_EDGE('',*,*,#26118,.T.);
#34550=ORIENTED_EDGE('',*,*,#26116,.T.);
#34551=ORIENTED_EDGE('',*,*,#26119,.T.);
#34552=ORIENTED_EDGE('',*,*,#26102,.F.);
#34553=ORIENTED_EDGE('',*,*,#26120,.T.);
#34554=ORIENTED_EDGE('',*,*,#21298,.F.);
#34555=ORIENTED_EDGE('',*,*,#26121,.T.);
#34556=ORIENTED_EDGE('',*,*,#26008,.T.);
#34557=ORIENTED_EDGE('',*,*,#26100,.F.);
#34558=ORIENTED_EDGE('',*,*,#26122,.T.);
#34559=ORIENTED_EDGE('',*,*,#26113,.F.);
#34560=ORIENTED_EDGE('',*,*,#26123,.T.);
#34561=ORIENTED_EDGE('',*,*,#26124,.T.);
#34562=ORIENTED_EDGE('',*,*,#26125,.T.);
#34563=ORIENTED_EDGE('',*,*,#26126,.T.);
#34564=ORIENTED_EDGE('',*,*,#26127,.F.);
#34565=ORIENTED_EDGE('',*,*,#26128,.T.);
#34566=ORIENTED_EDGE('',*,*,#26129,.T.);
#34567=ORIENTED_EDGE('',*,*,#26127,.T.);
#34568=ORIENTED_EDGE('',*,*,#26130,.T.);
#34569=ORIENTED_EDGE('',*,*,#26098,.F.);
#34570=ORIENTED_EDGE('',*,*,#26131,.T.);
#34571=ORIENTED_EDGE('',*,*,#26132,.F.);
#34572=ORIENTED_EDGE('',*,*,#26133,.T.);
#34573=ORIENTED_EDGE('',*,*,#26124,.F.);
#34574=ORIENTED_EDGE('',*,*,#26134,.T.);
#34575=ORIENTED_EDGE('',*,*,#26135,.T.);
#34576=ORIENTED_EDGE('',*,*,#26136,.T.);
#34577=ORIENTED_EDGE('',*,*,#26132,.T.);
#34578=ORIENTED_EDGE('',*,*,#26137,.T.);
#34579=ORIENTED_EDGE('',*,*,#26138,.T.);
#34580=ORIENTED_EDGE('',*,*,#26139,.T.);
#34581=ORIENTED_EDGE('',*,*,#26140,.T.);
#34582=ORIENTED_EDGE('',*,*,#26141,.F.);
#34583=ORIENTED_EDGE('',*,*,#26142,.T.);
#34584=ORIENTED_EDGE('',*,*,#26143,.T.);
#34585=ORIENTED_EDGE('',*,*,#26141,.T.);
#34586=ORIENTED_EDGE('',*,*,#26144,.T.);
#34587=ORIENTED_EDGE('',*,*,#26135,.F.);
#34588=ORIENTED_EDGE('',*,*,#26145,.T.);
#34589=ORIENTED_EDGE('',*,*,#26146,.F.);
#34590=ORIENTED_EDGE('',*,*,#26147,.T.);
#34591=ORIENTED_EDGE('',*,*,#26138,.F.);
#34592=ORIENTED_EDGE('',*,*,#26148,.T.);
#34593=ORIENTED_EDGE('',*,*,#26149,.T.);
#34594=ORIENTED_EDGE('',*,*,#26150,.T.);
#34595=ORIENTED_EDGE('',*,*,#26146,.T.);
#34596=ORIENTED_EDGE('',*,*,#26151,.T.);
#34597=ORIENTED_EDGE('',*,*,#26152,.T.);
#34598=ORIENTED_EDGE('',*,*,#26153,.T.);
#34599=ORIENTED_EDGE('',*,*,#26154,.T.);
#34600=ORIENTED_EDGE('',*,*,#26155,.F.);
#34601=ORIENTED_EDGE('',*,*,#26156,.T.);
#34602=ORIENTED_EDGE('',*,*,#26157,.T.);
#34603=ORIENTED_EDGE('',*,*,#26155,.T.);
#34604=ORIENTED_EDGE('',*,*,#26158,.T.);
#34605=ORIENTED_EDGE('',*,*,#26149,.F.);
#34606=ORIENTED_EDGE('',*,*,#26159,.T.);
#34607=ORIENTED_EDGE('',*,*,#26160,.F.);
#34608=ORIENTED_EDGE('',*,*,#26161,.T.);
#34609=ORIENTED_EDGE('',*,*,#26152,.F.);
#34610=ORIENTED_EDGE('',*,*,#26162,.T.);
#34611=ORIENTED_EDGE('',*,*,#26163,.T.);
#34612=ORIENTED_EDGE('',*,*,#26164,.T.);
#34613=ORIENTED_EDGE('',*,*,#26160,.T.);
#34614=ORIENTED_EDGE('',*,*,#26165,.T.);
#34615=ORIENTED_EDGE('',*,*,#26166,.T.);
#34616=ORIENTED_EDGE('',*,*,#26167,.T.);
#34617=ORIENTED_EDGE('',*,*,#26168,.T.);
#34618=ORIENTED_EDGE('',*,*,#26169,.F.);
#34619=ORIENTED_EDGE('',*,*,#26170,.T.);
#34620=ORIENTED_EDGE('',*,*,#26171,.T.);
#34621=ORIENTED_EDGE('',*,*,#26169,.T.);
#34622=ORIENTED_EDGE('',*,*,#26172,.T.);
#34623=ORIENTED_EDGE('',*,*,#26163,.F.);
#34624=ORIENTED_EDGE('',*,*,#26173,.T.);
#34625=ORIENTED_EDGE('',*,*,#26174,.F.);
#34626=ORIENTED_EDGE('',*,*,#26175,.T.);
#34627=ORIENTED_EDGE('',*,*,#26166,.F.);
#34628=ORIENTED_EDGE('',*,*,#26176,.T.);
#34629=ORIENTED_EDGE('',*,*,#26177,.T.);
#34630=ORIENTED_EDGE('',*,*,#26178,.T.);
#34631=ORIENTED_EDGE('',*,*,#26174,.T.);
#34632=ORIENTED_EDGE('',*,*,#26179,.T.);
#34633=ORIENTED_EDGE('',*,*,#26180,.T.);
#34634=ORIENTED_EDGE('',*,*,#26181,.T.);
#34635=ORIENTED_EDGE('',*,*,#26182,.T.);
#34636=ORIENTED_EDGE('',*,*,#26183,.F.);
#34637=ORIENTED_EDGE('',*,*,#26184,.T.);
#34638=ORIENTED_EDGE('',*,*,#26185,.T.);
#34639=ORIENTED_EDGE('',*,*,#26183,.T.);
#34640=ORIENTED_EDGE('',*,*,#26186,.T.);
#34641=ORIENTED_EDGE('',*,*,#26177,.F.);
#34642=ORIENTED_EDGE('',*,*,#26187,.T.);
#34643=ORIENTED_EDGE('',*,*,#21592,.F.);
#34644=ORIENTED_EDGE('',*,*,#26188,.T.);
#34645=ORIENTED_EDGE('',*,*,#26180,.F.);
#34646=ORIENTED_EDGE('',*,*,#26189,.T.);
#34647=ORIENTED_EDGE('',*,*,#21589,.F.);
#34648=ORIENTED_EDGE('',*,*,#26190,.T.);
#34649=ORIENTED_EDGE('',*,*,#26191,.T.);
#34650=ORIENTED_EDGE('',*,*,#26192,.F.);
#34651=ORIENTED_EDGE('',*,*,#26192,.T.);
#34652=ORIENTED_EDGE('',*,*,#26193,.T.);
#34653=ORIENTED_EDGE('',*,*,#21590,.F.);
#34654=ORIENTED_EDGE('',*,*,#26194,.T.);
#34655=ORIENTED_EDGE('',*,*,#26195,.T.);
#34656=ORIENTED_EDGE('',*,*,#26196,.T.);
#34657=ORIENTED_EDGE('',*,*,#26197,.T.);
#34658=ORIENTED_EDGE('',*,*,#26198,.T.);
#34659=ORIENTED_EDGE('',*,*,#26199,.T.);
#34660=ORIENTED_EDGE('',*,*,#26200,.T.);
#34661=ORIENTED_EDGE('',*,*,#26201,.T.);
#34662=ORIENTED_EDGE('',*,*,#26202,.T.);
#34663=ORIENTED_EDGE('',*,*,#26203,.T.);
#34664=ORIENTED_EDGE('',*,*,#26204,.T.);
#34665=ORIENTED_EDGE('',*,*,#26205,.T.);
#34666=ORIENTED_EDGE('',*,*,#26206,.T.);
#34667=ORIENTED_EDGE('',*,*,#26207,.T.);
#34668=ORIENTED_EDGE('',*,*,#26208,.T.);
#34669=ORIENTED_EDGE('',*,*,#26209,.F.);
#34670=ORIENTED_EDGE('',*,*,#26210,.T.);
#34671=ORIENTED_EDGE('',*,*,#26211,.T.);
#34672=ORIENTED_EDGE('',*,*,#26209,.T.);
#34673=ORIENTED_EDGE('',*,*,#26212,.T.);
#34674=ORIENTED_EDGE('',*,*,#26194,.F.);
#34675=ORIENTED_EDGE('',*,*,#26213,.T.);
#34676=ORIENTED_EDGE('',*,*,#21294,.F.);
#34677=ORIENTED_EDGE('',*,*,#26214,.T.);
#34678=ORIENTED_EDGE('',*,*,#26108,.T.);
#34679=ORIENTED_EDGE('',*,*,#26204,.F.);
#34680=ORIENTED_EDGE('',*,*,#26215,.T.);
#34681=ORIENTED_EDGE('',*,*,#26206,.F.);
#34682=ORIENTED_EDGE('',*,*,#26216,.T.);
#34683=ORIENTED_EDGE('',*,*,#26217,.T.);
#34684=ORIENTED_EDGE('',*,*,#26218,.T.);
#34685=ORIENTED_EDGE('',*,*,#26219,.T.);
#34686=ORIENTED_EDGE('',*,*,#26220,.F.);
#34687=ORIENTED_EDGE('',*,*,#26221,.T.);
#34688=ORIENTED_EDGE('',*,*,#26222,.T.);
#34689=ORIENTED_EDGE('',*,*,#26220,.T.);
#34690=ORIENTED_EDGE('',*,*,#26223,.T.);
#34691=ORIENTED_EDGE('',*,*,#26202,.F.);
#34692=ORIENTED_EDGE('',*,*,#26224,.T.);
#34693=ORIENTED_EDGE('',*,*,#26200,.F.);
#34694=ORIENTED_EDGE('',*,*,#26225,.T.);
#34695=ORIENTED_EDGE('',*,*,#26217,.F.);
#34696=ORIENTED_EDGE('',*,*,#26226,.T.);
#34697=ORIENTED_EDGE('',*,*,#26227,.T.);
#34698=ORIENTED_EDGE('',*,*,#26228,.T.);
#34699=ORIENTED_EDGE('',*,*,#26229,.T.);
#34700=ORIENTED_EDGE('',*,*,#26230,.F.);
#34701=ORIENTED_EDGE('',*,*,#26231,.T.);
#34702=ORIENTED_EDGE('',*,*,#26232,.T.);
#34703=ORIENTED_EDGE('',*,*,#26230,.T.);
#34704=ORIENTED_EDGE('',*,*,#26233,.T.);
#34705=ORIENTED_EDGE('',*,*,#26198,.F.);
#34706=ORIENTED_EDGE('',*,*,#26234,.T.);
#34707=ORIENTED_EDGE('',*,*,#26235,.F.);
#34708=ORIENTED_EDGE('',*,*,#26236,.T.);
#34709=ORIENTED_EDGE('',*,*,#26227,.F.);
#34710=ORIENTED_EDGE('',*,*,#26237,.T.);
#34711=ORIENTED_EDGE('',*,*,#26238,.T.);
#34712=ORIENTED_EDGE('',*,*,#26239,.T.);
#34713=ORIENTED_EDGE('',*,*,#21291,.F.);
#34714=ORIENTED_EDGE('',*,*,#26240,.F.);
#34715=ORIENTED_EDGE('',*,*,#26241,.T.);
#34716=ORIENTED_EDGE('',*,*,#26242,.T.);
#34717=ORIENTED_EDGE('',*,*,#26196,.F.);
#34718=ORIENTED_EDGE('',*,*,#26243,.T.);
#34719=ORIENTED_EDGE('',*,*,#26238,.F.);
#34720=ORIENTED_EDGE('',*,*,#26244,.T.);
#34721=ORIENTED_EDGE('',*,*,#26245,.T.);
#34722=ORIENTED_EDGE('',*,*,#26246,.T.);
#34723=ORIENTED_EDGE('',*,*,#26235,.T.);
#34724=ORIENTED_EDGE('',*,*,#26247,.T.);
#34725=ORIENTED_EDGE('',*,*,#26248,.T.);
#34726=ORIENTED_EDGE('',*,*,#26249,.T.);
#34727=ORIENTED_EDGE('',*,*,#26250,.T.);
#34728=ORIENTED_EDGE('',*,*,#26251,.F.);
#34729=ORIENTED_EDGE('',*,*,#26252,.T.);
#34730=ORIENTED_EDGE('',*,*,#26253,.T.);
#34731=ORIENTED_EDGE('',*,*,#26251,.T.);
#34732=ORIENTED_EDGE('',*,*,#26254,.T.);
#34733=ORIENTED_EDGE('',*,*,#26245,.F.);
#34734=ORIENTED_EDGE('',*,*,#26255,.T.);
#34735=ORIENTED_EDGE('',*,*,#26256,.F.);
#34736=ORIENTED_EDGE('',*,*,#26257,.T.);
#34737=ORIENTED_EDGE('',*,*,#26248,.F.);
#34738=ORIENTED_EDGE('',*,*,#26258,.T.);
#34739=ORIENTED_EDGE('',*,*,#26259,.T.);
#34740=ORIENTED_EDGE('',*,*,#26260,.T.);
#34741=ORIENTED_EDGE('',*,*,#26256,.T.);
#34742=ORIENTED_EDGE('',*,*,#26261,.T.);
#34743=ORIENTED_EDGE('',*,*,#26262,.T.);
#34744=ORIENTED_EDGE('',*,*,#26263,.T.);
#34745=ORIENTED_EDGE('',*,*,#26264,.T.);
#34746=ORIENTED_EDGE('',*,*,#26265,.F.);
#34747=ORIENTED_EDGE('',*,*,#26266,.T.);
#34748=ORIENTED_EDGE('',*,*,#26267,.T.);
#34749=ORIENTED_EDGE('',*,*,#26265,.T.);
#34750=ORIENTED_EDGE('',*,*,#26268,.T.);
#34751=ORIENTED_EDGE('',*,*,#26259,.F.);
#34752=ORIENTED_EDGE('',*,*,#26269,.T.);
#34753=ORIENTED_EDGE('',*,*,#26270,.F.);
#34754=ORIENTED_EDGE('',*,*,#26271,.T.);
#34755=ORIENTED_EDGE('',*,*,#26262,.F.);
#34756=ORIENTED_EDGE('',*,*,#26272,.T.);
#34757=ORIENTED_EDGE('',*,*,#26273,.T.);
#34758=ORIENTED_EDGE('',*,*,#26274,.T.);
#34759=ORIENTED_EDGE('',*,*,#26270,.T.);
#34760=ORIENTED_EDGE('',*,*,#26275,.T.);
#34761=ORIENTED_EDGE('',*,*,#26276,.T.);
#34762=ORIENTED_EDGE('',*,*,#26277,.T.);
#34763=ORIENTED_EDGE('',*,*,#26278,.T.);
#34764=ORIENTED_EDGE('',*,*,#26279,.F.);
#34765=ORIENTED_EDGE('',*,*,#26280,.T.);
#34766=ORIENTED_EDGE('',*,*,#26281,.T.);
#34767=ORIENTED_EDGE('',*,*,#26279,.T.);
#34768=ORIENTED_EDGE('',*,*,#26282,.T.);
#34769=ORIENTED_EDGE('',*,*,#26273,.F.);
#34770=ORIENTED_EDGE('',*,*,#26283,.T.);
#34771=ORIENTED_EDGE('',*,*,#21598,.F.);
#34772=ORIENTED_EDGE('',*,*,#26284,.T.);
#34773=ORIENTED_EDGE('',*,*,#26276,.F.);
#34774=ORIENTED_EDGE('',*,*,#26285,.T.);
#34775=ORIENTED_EDGE('',*,*,#21595,.F.);
#34776=ORIENTED_EDGE('',*,*,#26286,.T.);
#34777=ORIENTED_EDGE('',*,*,#26287,.T.);
#34778=ORIENTED_EDGE('',*,*,#26288,.F.);
#34779=ORIENTED_EDGE('',*,*,#26288,.T.);
#34780=ORIENTED_EDGE('',*,*,#26289,.T.);
#34781=ORIENTED_EDGE('',*,*,#21596,.F.);
#34782=ORIENTED_EDGE('',*,*,#26290,.T.);
#34783=ORIENTED_EDGE('',*,*,#26291,.T.);
#34784=ORIENTED_EDGE('',*,*,#26292,.T.);
#34785=ORIENTED_EDGE('',*,*,#26293,.T.);
#34786=ORIENTED_EDGE('',*,*,#26294,.T.);
#34787=ORIENTED_EDGE('',*,*,#26295,.T.);
#34788=ORIENTED_EDGE('',*,*,#26296,.T.);
#34789=ORIENTED_EDGE('',*,*,#26297,.T.);
#34790=ORIENTED_EDGE('',*,*,#26298,.T.);
#34791=ORIENTED_EDGE('',*,*,#26299,.T.);
#34792=ORIENTED_EDGE('',*,*,#26300,.T.);
#34793=ORIENTED_EDGE('',*,*,#26301,.T.);
#34794=ORIENTED_EDGE('',*,*,#26302,.T.);
#34795=ORIENTED_EDGE('',*,*,#26303,.T.);
#34796=ORIENTED_EDGE('',*,*,#26304,.T.);
#34797=ORIENTED_EDGE('',*,*,#26305,.T.);
#34798=ORIENTED_EDGE('',*,*,#26306,.T.);
#34799=ORIENTED_EDGE('',*,*,#26307,.T.);
#34800=ORIENTED_EDGE('',*,*,#26308,.T.);
#34801=ORIENTED_EDGE('',*,*,#26309,.F.);
#34802=ORIENTED_EDGE('',*,*,#26310,.T.);
#34803=ORIENTED_EDGE('',*,*,#26311,.T.);
#34804=ORIENTED_EDGE('',*,*,#26309,.T.);
#34805=ORIENTED_EDGE('',*,*,#26312,.T.);
#34806=ORIENTED_EDGE('',*,*,#26294,.F.);
#34807=ORIENTED_EDGE('',*,*,#26313,.T.);
#34808=ORIENTED_EDGE('',*,*,#26304,.F.);
#34809=ORIENTED_EDGE('',*,*,#26314,.T.);
#34810=ORIENTED_EDGE('',*,*,#26306,.F.);
#34811=ORIENTED_EDGE('',*,*,#26315,.T.);
#34812=ORIENTED_EDGE('',*,*,#26316,.T.);
#34813=ORIENTED_EDGE('',*,*,#26317,.T.);
#34814=ORIENTED_EDGE('',*,*,#26318,.T.);
#34815=ORIENTED_EDGE('',*,*,#26319,.F.);
#34816=ORIENTED_EDGE('',*,*,#26320,.T.);
#34817=ORIENTED_EDGE('',*,*,#26321,.T.);
#34818=ORIENTED_EDGE('',*,*,#26319,.T.);
#34819=ORIENTED_EDGE('',*,*,#26322,.T.);
#34820=ORIENTED_EDGE('',*,*,#26302,.F.);
#34821=ORIENTED_EDGE('',*,*,#26323,.T.);
#34822=ORIENTED_EDGE('',*,*,#26300,.F.);
#34823=ORIENTED_EDGE('',*,*,#26324,.T.);
#34824=ORIENTED_EDGE('',*,*,#26316,.F.);
#34825=ORIENTED_EDGE('',*,*,#26325,.T.);
#34826=ORIENTED_EDGE('',*,*,#26326,.T.);
#34827=ORIENTED_EDGE('',*,*,#26327,.T.);
#34828=ORIENTED_EDGE('',*,*,#26328,.T.);
#34829=ORIENTED_EDGE('',*,*,#26329,.F.);
#34830=ORIENTED_EDGE('',*,*,#26330,.T.);
#34831=ORIENTED_EDGE('',*,*,#26331,.T.);
#34832=ORIENTED_EDGE('',*,*,#26329,.T.);
#34833=ORIENTED_EDGE('',*,*,#26332,.T.);
#34834=ORIENTED_EDGE('',*,*,#26298,.F.);
#34835=ORIENTED_EDGE('',*,*,#26333,.T.);
#34836=ORIENTED_EDGE('',*,*,#26334,.F.);
#34837=ORIENTED_EDGE('',*,*,#26335,.T.);
#34838=ORIENTED_EDGE('',*,*,#26326,.F.);
#34839=ORIENTED_EDGE('',*,*,#26336,.T.);
#34840=ORIENTED_EDGE('',*,*,#26337,.T.);
#34841=ORIENTED_EDGE('',*,*,#26338,.T.);
#34842=ORIENTED_EDGE('',*,*,#21287,.F.);
#34843=ORIENTED_EDGE('',*,*,#26339,.F.);
#34844=ORIENTED_EDGE('',*,*,#26340,.T.);
#34845=ORIENTED_EDGE('',*,*,#26341,.T.);
#34846=ORIENTED_EDGE('',*,*,#26292,.F.);
#34847=ORIENTED_EDGE('',*,*,#26342,.T.);
#34848=ORIENTED_EDGE('',*,*,#26337,.F.);
#34849=ORIENTED_EDGE('',*,*,#26343,.T.);
#34850=ORIENTED_EDGE('',*,*,#26344,.T.);
#34851=ORIENTED_EDGE('',*,*,#26345,.T.);
#34852=ORIENTED_EDGE('',*,*,#26346,.T.);
#34853=ORIENTED_EDGE('',*,*,#26347,.F.);
#34854=ORIENTED_EDGE('',*,*,#26348,.T.);
#34855=ORIENTED_EDGE('',*,*,#26349,.T.);
#34856=ORIENTED_EDGE('',*,*,#26347,.T.);
#34857=ORIENTED_EDGE('',*,*,#26350,.T.);
#34858=ORIENTED_EDGE('',*,*,#26290,.F.);
#34859=ORIENTED_EDGE('',*,*,#26351,.T.);
#34860=ORIENTED_EDGE('',*,*,#21290,.F.);
#34861=ORIENTED_EDGE('',*,*,#26352,.T.);
#34862=ORIENTED_EDGE('',*,*,#26240,.T.);
#34863=ORIENTED_EDGE('',*,*,#26296,.F.);
#34864=ORIENTED_EDGE('',*,*,#26353,.T.);
#34865=ORIENTED_EDGE('',*,*,#26344,.F.);
#34866=ORIENTED_EDGE('',*,*,#26354,.T.);
#34867=ORIENTED_EDGE('',*,*,#26355,.T.);
#34868=ORIENTED_EDGE('',*,*,#26356,.T.);
#34869=ORIENTED_EDGE('',*,*,#26334,.T.);
#34870=ORIENTED_EDGE('',*,*,#26357,.T.);
#34871=ORIENTED_EDGE('',*,*,#26358,.T.);
#34872=ORIENTED_EDGE('',*,*,#26359,.T.);
#34873=ORIENTED_EDGE('',*,*,#26360,.T.);
#34874=ORIENTED_EDGE('',*,*,#26361,.F.);
#34875=ORIENTED_EDGE('',*,*,#26362,.T.);
#34876=ORIENTED_EDGE('',*,*,#26363,.T.);
#34877=ORIENTED_EDGE('',*,*,#26361,.T.);
#34878=ORIENTED_EDGE('',*,*,#26364,.T.);
#34879=ORIENTED_EDGE('',*,*,#26355,.F.);
#34880=ORIENTED_EDGE('',*,*,#26365,.T.);
#34881=ORIENTED_EDGE('',*,*,#26366,.F.);
#34882=ORIENTED_EDGE('',*,*,#26367,.T.);
#34883=ORIENTED_EDGE('',*,*,#26358,.F.);
#34884=ORIENTED_EDGE('',*,*,#26368,.T.);
#34885=ORIENTED_EDGE('',*,*,#26369,.T.);
#34886=ORIENTED_EDGE('',*,*,#26370,.T.);
#34887=ORIENTED_EDGE('',*,*,#26366,.T.);
#34888=ORIENTED_EDGE('',*,*,#26371,.T.);
#34889=ORIENTED_EDGE('',*,*,#26372,.T.);
#34890=ORIENTED_EDGE('',*,*,#26373,.T.);
#34891=ORIENTED_EDGE('',*,*,#26374,.T.);
#34892=ORIENTED_EDGE('',*,*,#26375,.F.);
#34893=ORIENTED_EDGE('',*,*,#26376,.T.);
#34894=ORIENTED_EDGE('',*,*,#26377,.T.);
#34895=ORIENTED_EDGE('',*,*,#26375,.T.);
#34896=ORIENTED_EDGE('',*,*,#26378,.T.);
#34897=ORIENTED_EDGE('',*,*,#26369,.F.);
#34898=ORIENTED_EDGE('',*,*,#26379,.T.);
#34899=ORIENTED_EDGE('',*,*,#21604,.F.);
#34900=ORIENTED_EDGE('',*,*,#26380,.T.);
#34901=ORIENTED_EDGE('',*,*,#26372,.F.);
#34902=ORIENTED_EDGE('',*,*,#26381,.T.);
#34903=ORIENTED_EDGE('',*,*,#21601,.F.);
#34904=ORIENTED_EDGE('',*,*,#26382,.T.);
#34905=ORIENTED_EDGE('',*,*,#26383,.T.);
#34906=ORIENTED_EDGE('',*,*,#26384,.F.);
#34907=ORIENTED_EDGE('',*,*,#26384,.T.);
#34908=ORIENTED_EDGE('',*,*,#26385,.T.);
#34909=ORIENTED_EDGE('',*,*,#21602,.F.);
#34910=ORIENTED_EDGE('',*,*,#26386,.T.);
#34911=ORIENTED_EDGE('',*,*,#26387,.T.);
#34912=ORIENTED_EDGE('',*,*,#26388,.T.);
#34913=ORIENTED_EDGE('',*,*,#26389,.T.);
#34914=ORIENTED_EDGE('',*,*,#26390,.T.);
#34915=ORIENTED_EDGE('',*,*,#26391,.T.);
#34916=ORIENTED_EDGE('',*,*,#26392,.T.);
#34917=ORIENTED_EDGE('',*,*,#26393,.T.);
#34918=ORIENTED_EDGE('',*,*,#26394,.T.);
#34919=ORIENTED_EDGE('',*,*,#26395,.T.);
#34920=ORIENTED_EDGE('',*,*,#26396,.T.);
#34921=ORIENTED_EDGE('',*,*,#26397,.T.);
#34922=ORIENTED_EDGE('',*,*,#26398,.T.);
#34923=ORIENTED_EDGE('',*,*,#26399,.T.);
#34924=ORIENTED_EDGE('',*,*,#26400,.T.);
#34925=ORIENTED_EDGE('',*,*,#26401,.T.);
#34926=ORIENTED_EDGE('',*,*,#26402,.T.);
#34927=ORIENTED_EDGE('',*,*,#26403,.T.);
#34928=ORIENTED_EDGE('',*,*,#26404,.T.);
#34929=ORIENTED_EDGE('',*,*,#26405,.T.);
#34930=ORIENTED_EDGE('',*,*,#26406,.T.);
#34931=ORIENTED_EDGE('',*,*,#26407,.T.);
#34932=ORIENTED_EDGE('',*,*,#26408,.T.);
#34933=ORIENTED_EDGE('',*,*,#26409,.F.);
#34934=ORIENTED_EDGE('',*,*,#26410,.T.);
#34935=ORIENTED_EDGE('',*,*,#26411,.T.);
#34936=ORIENTED_EDGE('',*,*,#26409,.T.);
#34937=ORIENTED_EDGE('',*,*,#26412,.T.);
#34938=ORIENTED_EDGE('',*,*,#26390,.F.);
#34939=ORIENTED_EDGE('',*,*,#26413,.T.);
#34940=ORIENTED_EDGE('',*,*,#26404,.F.);
#34941=ORIENTED_EDGE('',*,*,#26414,.T.);
#34942=ORIENTED_EDGE('',*,*,#26406,.F.);
#34943=ORIENTED_EDGE('',*,*,#26415,.T.);
#34944=ORIENTED_EDGE('',*,*,#26416,.T.);
#34945=ORIENTED_EDGE('',*,*,#26417,.T.);
#34946=ORIENTED_EDGE('',*,*,#26418,.T.);
#34947=ORIENTED_EDGE('',*,*,#26419,.F.);
#34948=ORIENTED_EDGE('',*,*,#26420,.T.);
#34949=ORIENTED_EDGE('',*,*,#26421,.T.);
#34950=ORIENTED_EDGE('',*,*,#26419,.T.);
#34951=ORIENTED_EDGE('',*,*,#26422,.T.);
#34952=ORIENTED_EDGE('',*,*,#26402,.F.);
#34953=ORIENTED_EDGE('',*,*,#26423,.T.);
#34954=ORIENTED_EDGE('',*,*,#26400,.F.);
#34955=ORIENTED_EDGE('',*,*,#26424,.T.);
#34956=ORIENTED_EDGE('',*,*,#26416,.F.);
#34957=ORIENTED_EDGE('',*,*,#26425,.T.);
#34958=ORIENTED_EDGE('',*,*,#26426,.T.);
#34959=ORIENTED_EDGE('',*,*,#26427,.T.);
#34960=ORIENTED_EDGE('',*,*,#26428,.T.);
#34961=ORIENTED_EDGE('',*,*,#26429,.F.);
#34962=ORIENTED_EDGE('',*,*,#26430,.T.);
#34963=ORIENTED_EDGE('',*,*,#26431,.T.);
#34964=ORIENTED_EDGE('',*,*,#26429,.T.);
#34965=ORIENTED_EDGE('',*,*,#26432,.T.);
#34966=ORIENTED_EDGE('',*,*,#26398,.F.);
#34967=ORIENTED_EDGE('',*,*,#26433,.T.);
#34968=ORIENTED_EDGE('',*,*,#26434,.F.);
#34969=ORIENTED_EDGE('',*,*,#26435,.T.);
#34970=ORIENTED_EDGE('',*,*,#26426,.F.);
#34971=ORIENTED_EDGE('',*,*,#26436,.T.);
#34972=ORIENTED_EDGE('',*,*,#26437,.T.);
#34973=ORIENTED_EDGE('',*,*,#26438,.T.);
#34974=ORIENTED_EDGE('',*,*,#21283,.F.);
#34975=ORIENTED_EDGE('',*,*,#26439,.F.);
#34976=ORIENTED_EDGE('',*,*,#26440,.T.);
#34977=ORIENTED_EDGE('',*,*,#26441,.T.);
#34978=ORIENTED_EDGE('',*,*,#26396,.F.);
#34979=ORIENTED_EDGE('',*,*,#26442,.T.);
#34980=ORIENTED_EDGE('',*,*,#26437,.F.);
#34981=ORIENTED_EDGE('',*,*,#26443,.T.);
#34982=ORIENTED_EDGE('',*,*,#26444,.T.);
#34983=ORIENTED_EDGE('',*,*,#26445,.T.);
#34984=ORIENTED_EDGE('',*,*,#26446,.T.);
#34985=ORIENTED_EDGE('',*,*,#26447,.F.);
#34986=ORIENTED_EDGE('',*,*,#26448,.T.);
#34987=ORIENTED_EDGE('',*,*,#26449,.T.);
#34988=ORIENTED_EDGE('',*,*,#26447,.T.);
#34989=ORIENTED_EDGE('',*,*,#26450,.T.);
#34990=ORIENTED_EDGE('',*,*,#26394,.F.);
#34991=ORIENTED_EDGE('',*,*,#26451,.T.);
#34992=ORIENTED_EDGE('',*,*,#21286,.F.);
#34993=ORIENTED_EDGE('',*,*,#26452,.T.);
#34994=ORIENTED_EDGE('',*,*,#26339,.T.);
#34995=ORIENTED_EDGE('',*,*,#26388,.F.);
#34996=ORIENTED_EDGE('',*,*,#26453,.T.);
#34997=ORIENTED_EDGE('',*,*,#26444,.F.);
#34998=ORIENTED_EDGE('',*,*,#26454,.T.);
#34999=ORIENTED_EDGE('',*,*,#26455,.T.);
#35000=ORIENTED_EDGE('',*,*,#26456,.T.);
#35001=ORIENTED_EDGE('',*,*,#26457,.T.);
#35002=ORIENTED_EDGE('',*,*,#26458,.F.);
#35003=ORIENTED_EDGE('',*,*,#26459,.T.);
#35004=ORIENTED_EDGE('',*,*,#26460,.T.);
#35005=ORIENTED_EDGE('',*,*,#26458,.T.);
#35006=ORIENTED_EDGE('',*,*,#26461,.T.);
#35007=ORIENTED_EDGE('',*,*,#26386,.F.);
#35008=ORIENTED_EDGE('',*,*,#26462,.T.);
#35009=ORIENTED_EDGE('',*,*,#26392,.F.);
#35010=ORIENTED_EDGE('',*,*,#26463,.T.);
#35011=ORIENTED_EDGE('',*,*,#26455,.F.);
#35012=ORIENTED_EDGE('',*,*,#26464,.T.);
#35013=ORIENTED_EDGE('',*,*,#26465,.T.);
#35014=ORIENTED_EDGE('',*,*,#26466,.T.);
#35015=ORIENTED_EDGE('',*,*,#26434,.T.);
#35016=ORIENTED_EDGE('',*,*,#26467,.T.);
#35017=ORIENTED_EDGE('',*,*,#26468,.T.);
#35018=ORIENTED_EDGE('',*,*,#26469,.T.);
#35019=ORIENTED_EDGE('',*,*,#26470,.T.);
#35020=ORIENTED_EDGE('',*,*,#26471,.F.);
#35021=ORIENTED_EDGE('',*,*,#26472,.T.);
#35022=ORIENTED_EDGE('',*,*,#26473,.T.);
#35023=ORIENTED_EDGE('',*,*,#26471,.T.);
#35024=ORIENTED_EDGE('',*,*,#26474,.T.);
#35025=ORIENTED_EDGE('',*,*,#26465,.F.);
#35026=ORIENTED_EDGE('',*,*,#26475,.T.);
#35027=ORIENTED_EDGE('',*,*,#21610,.F.);
#35028=ORIENTED_EDGE('',*,*,#26476,.T.);
#35029=ORIENTED_EDGE('',*,*,#26468,.F.);
#35030=ORIENTED_EDGE('',*,*,#26477,.T.);
#35031=ORIENTED_EDGE('',*,*,#21607,.F.);
#35032=ORIENTED_EDGE('',*,*,#26478,.T.);
#35033=ORIENTED_EDGE('',*,*,#26479,.T.);
#35034=ORIENTED_EDGE('',*,*,#26480,.F.);
#35035=ORIENTED_EDGE('',*,*,#26480,.T.);
#35036=ORIENTED_EDGE('',*,*,#26481,.T.);
#35037=ORIENTED_EDGE('',*,*,#21608,.F.);
#35038=ORIENTED_EDGE('',*,*,#26482,.T.);
#35039=ORIENTED_EDGE('',*,*,#26483,.T.);
#35040=ORIENTED_EDGE('',*,*,#26484,.T.);
#35041=ORIENTED_EDGE('',*,*,#26485,.T.);
#35042=ORIENTED_EDGE('',*,*,#26486,.T.);
#35043=ORIENTED_EDGE('',*,*,#26487,.T.);
#35044=ORIENTED_EDGE('',*,*,#26488,.T.);
#35045=ORIENTED_EDGE('',*,*,#26489,.T.);
#35046=ORIENTED_EDGE('',*,*,#26490,.T.);
#35047=ORIENTED_EDGE('',*,*,#26491,.T.);
#35048=ORIENTED_EDGE('',*,*,#26492,.T.);
#35049=ORIENTED_EDGE('',*,*,#26493,.T.);
#35050=ORIENTED_EDGE('',*,*,#26494,.T.);
#35051=ORIENTED_EDGE('',*,*,#26495,.T.);
#35052=ORIENTED_EDGE('',*,*,#26496,.T.);
#35053=ORIENTED_EDGE('',*,*,#26497,.T.);
#35054=ORIENTED_EDGE('',*,*,#26498,.T.);
#35055=ORIENTED_EDGE('',*,*,#26499,.T.);
#35056=ORIENTED_EDGE('',*,*,#26500,.T.);
#35057=ORIENTED_EDGE('',*,*,#26501,.T.);
#35058=ORIENTED_EDGE('',*,*,#26502,.T.);
#35059=ORIENTED_EDGE('',*,*,#26503,.T.);
#35060=ORIENTED_EDGE('',*,*,#26504,.T.);
#35061=ORIENTED_EDGE('',*,*,#26505,.T.);
#35062=ORIENTED_EDGE('',*,*,#26506,.T.);
#35063=ORIENTED_EDGE('',*,*,#26507,.T.);
#35064=ORIENTED_EDGE('',*,*,#26508,.T.);
#35065=ORIENTED_EDGE('',*,*,#26509,.F.);
#35066=ORIENTED_EDGE('',*,*,#26510,.T.);
#35067=ORIENTED_EDGE('',*,*,#26511,.T.);
#35068=ORIENTED_EDGE('',*,*,#26509,.T.);
#35069=ORIENTED_EDGE('',*,*,#26512,.T.);
#35070=ORIENTED_EDGE('',*,*,#26486,.F.);
#35071=ORIENTED_EDGE('',*,*,#26513,.T.);
#35072=ORIENTED_EDGE('',*,*,#26504,.F.);
#35073=ORIENTED_EDGE('',*,*,#26514,.T.);
#35074=ORIENTED_EDGE('',*,*,#26506,.F.);
#35075=ORIENTED_EDGE('',*,*,#26515,.T.);
#35076=ORIENTED_EDGE('',*,*,#26516,.T.);
#35077=ORIENTED_EDGE('',*,*,#26517,.T.);
#35078=ORIENTED_EDGE('',*,*,#26518,.T.);
#35079=ORIENTED_EDGE('',*,*,#26519,.F.);
#35080=ORIENTED_EDGE('',*,*,#26520,.T.);
#35081=ORIENTED_EDGE('',*,*,#26521,.T.);
#35082=ORIENTED_EDGE('',*,*,#26519,.T.);
#35083=ORIENTED_EDGE('',*,*,#26522,.T.);
#35084=ORIENTED_EDGE('',*,*,#26502,.F.);
#35085=ORIENTED_EDGE('',*,*,#26523,.T.);
#35086=ORIENTED_EDGE('',*,*,#26500,.F.);
#35087=ORIENTED_EDGE('',*,*,#26524,.T.);
#35088=ORIENTED_EDGE('',*,*,#26516,.F.);
#35089=ORIENTED_EDGE('',*,*,#26525,.T.);
#35090=ORIENTED_EDGE('',*,*,#26526,.T.);
#35091=ORIENTED_EDGE('',*,*,#26527,.T.);
#35092=ORIENTED_EDGE('',*,*,#26528,.T.);
#35093=ORIENTED_EDGE('',*,*,#26529,.F.);
#35094=ORIENTED_EDGE('',*,*,#26530,.T.);
#35095=ORIENTED_EDGE('',*,*,#26531,.T.);
#35096=ORIENTED_EDGE('',*,*,#26529,.T.);
#35097=ORIENTED_EDGE('',*,*,#26532,.T.);
#35098=ORIENTED_EDGE('',*,*,#26498,.F.);
#35099=ORIENTED_EDGE('',*,*,#26533,.T.);
#35100=ORIENTED_EDGE('',*,*,#21616,.F.);
#35101=ORIENTED_EDGE('',*,*,#26534,.T.);
#35102=ORIENTED_EDGE('',*,*,#26526,.F.);
#35103=ORIENTED_EDGE('',*,*,#26535,.T.);
#35104=ORIENTED_EDGE('',*,*,#26536,.T.);
#35105=ORIENTED_EDGE('',*,*,#26537,.T.);
#35106=ORIENTED_EDGE('',*,*,#21479,.F.);
#35107=ORIENTED_EDGE('',*,*,#26538,.F.);
#35108=ORIENTED_EDGE('',*,*,#26539,.T.);
#35109=ORIENTED_EDGE('',*,*,#26540,.T.);
#35110=ORIENTED_EDGE('',*,*,#26496,.F.);
#35111=ORIENTED_EDGE('',*,*,#26541,.T.);
#35112=ORIENTED_EDGE('',*,*,#26536,.F.);
#35113=ORIENTED_EDGE('',*,*,#26542,.T.);
#35114=ORIENTED_EDGE('',*,*,#26543,.T.);
#35115=ORIENTED_EDGE('',*,*,#26544,.T.);
#35116=ORIENTED_EDGE('',*,*,#26545,.T.);
#35117=ORIENTED_EDGE('',*,*,#26546,.F.);
#35118=ORIENTED_EDGE('',*,*,#26547,.T.);
#35119=ORIENTED_EDGE('',*,*,#26548,.T.);
#35120=ORIENTED_EDGE('',*,*,#26546,.T.);
#35121=ORIENTED_EDGE('',*,*,#26549,.T.);
#35122=ORIENTED_EDGE('',*,*,#26494,.F.);
#35123=ORIENTED_EDGE('',*,*,#26550,.T.);
#35124=ORIENTED_EDGE('',*,*,#21282,.F.);
#35125=ORIENTED_EDGE('',*,*,#26551,.T.);
#35126=ORIENTED_EDGE('',*,*,#26439,.T.);
#35127=ORIENTED_EDGE('',*,*,#26492,.F.);
#35128=ORIENTED_EDGE('',*,*,#26552,.T.);
#35129=ORIENTED_EDGE('',*,*,#26543,.F.);
#35130=ORIENTED_EDGE('',*,*,#26553,.T.);
#35131=ORIENTED_EDGE('',*,*,#26554,.T.);
#35132=ORIENTED_EDGE('',*,*,#26555,.T.);
#35133=ORIENTED_EDGE('',*,*,#26556,.T.);
#35134=ORIENTED_EDGE('',*,*,#26557,.F.);
#35135=ORIENTED_EDGE('',*,*,#26558,.T.);
#35136=ORIENTED_EDGE('',*,*,#26559,.T.);
#35137=ORIENTED_EDGE('',*,*,#26557,.T.);
#35138=ORIENTED_EDGE('',*,*,#26560,.T.);
#35139=ORIENTED_EDGE('',*,*,#26490,.F.);
#35140=ORIENTED_EDGE('',*,*,#26561,.T.);
#35141=ORIENTED_EDGE('',*,*,#26484,.F.);
#35142=ORIENTED_EDGE('',*,*,#26562,.T.);
#35143=ORIENTED_EDGE('',*,*,#26554,.F.);
#35144=ORIENTED_EDGE('',*,*,#26563,.T.);
#35145=ORIENTED_EDGE('',*,*,#26564,.T.);
#35146=ORIENTED_EDGE('',*,*,#26565,.T.);
#35147=ORIENTED_EDGE('',*,*,#26566,.T.);
#35148=ORIENTED_EDGE('',*,*,#26567,.F.);
#35149=ORIENTED_EDGE('',*,*,#26568,.T.);
#35150=ORIENTED_EDGE('',*,*,#26569,.T.);
#35151=ORIENTED_EDGE('',*,*,#26567,.T.);
#35152=ORIENTED_EDGE('',*,*,#26570,.T.);
#35153=ORIENTED_EDGE('',*,*,#26482,.F.);
#35154=ORIENTED_EDGE('',*,*,#26571,.T.);
#35155=ORIENTED_EDGE('',*,*,#26488,.F.);
#35156=ORIENTED_EDGE('',*,*,#26572,.T.);
#35157=ORIENTED_EDGE('',*,*,#26564,.F.);
#35158=ORIENTED_EDGE('',*,*,#26573,.T.);
#35159=ORIENTED_EDGE('',*,*,#21613,.F.);
#35160=ORIENTED_EDGE('',*,*,#26574,.T.);
#35161=ORIENTED_EDGE('',*,*,#26575,.T.);
#35162=ORIENTED_EDGE('',*,*,#26576,.F.);
#35163=ORIENTED_EDGE('',*,*,#26576,.T.);
#35164=ORIENTED_EDGE('',*,*,#26577,.T.);
#35165=ORIENTED_EDGE('',*,*,#21614,.F.);
#35166=ORIENTED_EDGE('',*,*,#21619,.F.);
#35167=ORIENTED_EDGE('',*,*,#26578,.T.);
#35168=ORIENTED_EDGE('',*,*,#26579,.T.);
#35169=ORIENTED_EDGE('',*,*,#26580,.F.);
#35170=ORIENTED_EDGE('',*,*,#26580,.T.);
#35171=ORIENTED_EDGE('',*,*,#26581,.T.);
#35172=ORIENTED_EDGE('',*,*,#21620,.F.);
#35173=ORIENTED_EDGE('',*,*,#21478,.F.);
#35174=ORIENTED_EDGE('',*,*,#26582,.T.);
#35175=ORIENTED_EDGE('',*,*,#26538,.T.);
#35176=ORIENTED_EDGE('',*,*,#21274,.F.);
#35177=ORIENTED_EDGE('',*,*,#21279,.T.);
#35178=ORIENTED_EDGE('',*,*,#21276,.T.);
#35179=ORIENTED_EDGE('',*,*,#21482,.T.);
#35180=ORIENTED_EDGE('',*,*,#26583,.T.);
#35181=ORIENTED_EDGE('',*,*,#21925,.F.);
#35182=ORIENTED_EDGE('',*,*,#21931,.F.);
#35183=ORIENTED_EDGE('',*,*,#21947,.F.);
#35184=ORIENTED_EDGE('',*,*,#26489,.F.);
#35185=ORIENTED_EDGE('',*,*,#26573,.F.);
#35186=ORIENTED_EDGE('',*,*,#26584,.F.);
#35187=ORIENTED_EDGE('',*,*,#26513,.F.);
#35188=ORIENTED_EDGE('',*,*,#26584,.T.);
#35189=ORIENTED_EDGE('',*,*,#26569,.F.);
#35190=ORIENTED_EDGE('',*,*,#21914,.F.);
#35191=ORIENTED_EDGE('',*,*,#26583,.F.);
#35192=ORIENTED_EDGE('',*,*,#21943,.F.);
#35193=ORIENTED_EDGE('',*,*,#26510,.F.);
#35194=ORIENTED_EDGE('',*,*,#26585,.F.);
#35195=ORIENTED_EDGE('',*,*,#26571,.F.);
#35196=ORIENTED_EDGE('',*,*,#26485,.F.);
#35197=ORIENTED_EDGE('',*,*,#26563,.F.);
#35198=ORIENTED_EDGE('',*,*,#21903,.F.);
#35199=ORIENTED_EDGE('',*,*,#21919,.F.);
#35200=ORIENTED_EDGE('',*,*,#26586,.T.);
#35201=ORIENTED_EDGE('',*,*,#21897,.F.);
#35202=ORIENTED_EDGE('',*,*,#26586,.F.);
#35203=ORIENTED_EDGE('',*,*,#21915,.F.);
#35204=ORIENTED_EDGE('',*,*,#26568,.F.);
#35205=ORIENTED_EDGE('',*,*,#26585,.T.);
#35206=ORIENTED_EDGE('',*,*,#26559,.F.);
#35207=ORIENTED_EDGE('',*,*,#21886,.F.);
#35208=ORIENTED_EDGE('',*,*,#26587,.F.);
#35209=ORIENTED_EDGE('',*,*,#26561,.F.);
#35210=ORIENTED_EDGE('',*,*,#26493,.F.);
#35211=ORIENTED_EDGE('',*,*,#26553,.F.);
#35212=ORIENTED_EDGE('',*,*,#21875,.F.);
#35213=ORIENTED_EDGE('',*,*,#21891,.F.);
#35214=ORIENTED_EDGE('',*,*,#26588,.T.);
#35215=ORIENTED_EDGE('',*,*,#21869,.F.);
#35216=ORIENTED_EDGE('',*,*,#26588,.F.);
#35217=ORIENTED_EDGE('',*,*,#21887,.F.);
#35218=ORIENTED_EDGE('',*,*,#26558,.F.);
#35219=ORIENTED_EDGE('',*,*,#26587,.T.);
#35220=ORIENTED_EDGE('',*,*,#26548,.F.);
#35221=ORIENTED_EDGE('',*,*,#21858,.F.);
#35222=ORIENTED_EDGE('',*,*,#26589,.F.);
#35223=ORIENTED_EDGE('',*,*,#26550,.F.);
#35224=ORIENTED_EDGE('',*,*,#26497,.F.);
#35225=ORIENTED_EDGE('',*,*,#26542,.F.);
#35226=ORIENTED_EDGE('',*,*,#21847,.F.);
#35227=ORIENTED_EDGE('',*,*,#21863,.F.);
#35228=ORIENTED_EDGE('',*,*,#26590,.T.);
#35229=ORIENTED_EDGE('',*,*,#21841,.F.);
#35230=ORIENTED_EDGE('',*,*,#26590,.F.);
#35231=ORIENTED_EDGE('',*,*,#21859,.F.);
#35232=ORIENTED_EDGE('',*,*,#26547,.F.);
#35233=ORIENTED_EDGE('',*,*,#26589,.T.);
#35234=ORIENTED_EDGE('',*,*,#26540,.F.);
#35235=ORIENTED_EDGE('',*,*,#21830,.F.);
#35236=ORIENTED_EDGE('',*,*,#21819,.F.);
#35237=ORIENTED_EDGE('',*,*,#21835,.F.);
#35238=ORIENTED_EDGE('',*,*,#26591,.T.);
#35239=ORIENTED_EDGE('',*,*,#21807,.F.);
#35240=ORIENTED_EDGE('',*,*,#26592,.F.);
#35241=ORIENTED_EDGE('',*,*,#26582,.F.);
#35242=ORIENTED_EDGE('',*,*,#21477,.F.);
#35243=ORIENTED_EDGE('',*,*,#21801,.F.);
#35244=ORIENTED_EDGE('',*,*,#26591,.F.);
#35245=ORIENTED_EDGE('',*,*,#21831,.F.);
#35246=ORIENTED_EDGE('',*,*,#26539,.F.);
#35247=ORIENTED_EDGE('',*,*,#26592,.T.);
#35248=ORIENTED_EDGE('',*,*,#21476,.F.);
#35249=ORIENTED_EDGE('',*,*,#26535,.F.);
#35250=ORIENTED_EDGE('',*,*,#26593,.F.);
#35251=ORIENTED_EDGE('',*,*,#21617,.F.);
#35252=ORIENTED_EDGE('',*,*,#26593,.T.);
#35253=ORIENTED_EDGE('',*,*,#26531,.F.);
#35254=ORIENTED_EDGE('',*,*,#26578,.F.);
#35255=ORIENTED_EDGE('',*,*,#21618,.F.);
#35256=ORIENTED_EDGE('',*,*,#26594,.F.);
#35257=ORIENTED_EDGE('',*,*,#26533,.F.);
#35258=ORIENTED_EDGE('',*,*,#26501,.F.);
#35259=ORIENTED_EDGE('',*,*,#26525,.F.);
#35260=ORIENTED_EDGE('',*,*,#21621,.F.);
#35261=ORIENTED_EDGE('',*,*,#26581,.F.);
#35262=ORIENTED_EDGE('',*,*,#26595,.T.);
#35263=ORIENTED_EDGE('',*,*,#21969,.F.);
#35264=ORIENTED_EDGE('',*,*,#26595,.F.);
#35265=ORIENTED_EDGE('',*,*,#26579,.F.);
#35266=ORIENTED_EDGE('',*,*,#26530,.F.);
#35267=ORIENTED_EDGE('',*,*,#26594,.T.);
#35268=ORIENTED_EDGE('',*,*,#26521,.F.);
#35269=ORIENTED_EDGE('',*,*,#21963,.F.);
#35270=ORIENTED_EDGE('',*,*,#26596,.F.);
#35271=ORIENTED_EDGE('',*,*,#21964,.F.);
#35272=ORIENTED_EDGE('',*,*,#26520,.F.);
#35273=ORIENTED_EDGE('',*,*,#26597,.T.);
#35274=ORIENTED_EDGE('',*,*,#26511,.F.);
#35275=ORIENTED_EDGE('',*,*,#21942,.F.);
#35276=ORIENTED_EDGE('',*,*,#21955,.F.);
#35277=ORIENTED_EDGE('',*,*,#21967,.F.);
#35278=ORIENTED_EDGE('',*,*,#26596,.T.);
#35279=ORIENTED_EDGE('',*,*,#21952,.F.);
#35280=ORIENTED_EDGE('',*,*,#26597,.F.);
#35281=ORIENTED_EDGE('',*,*,#26523,.F.);
#35282=ORIENTED_EDGE('',*,*,#26505,.F.);
#35283=ORIENTED_EDGE('',*,*,#26515,.F.);
#35284=ORIENTED_EDGE('',*,*,#26477,.F.);
#35285=ORIENTED_EDGE('',*,*,#26598,.F.);
#35286=ORIENTED_EDGE('',*,*,#21611,.F.);
#35287=ORIENTED_EDGE('',*,*,#26598,.T.);
#35288=ORIENTED_EDGE('',*,*,#26473,.F.);
#35289=ORIENTED_EDGE('',*,*,#26574,.F.);
#35290=ORIENTED_EDGE('',*,*,#21612,.F.);
#35291=ORIENTED_EDGE('',*,*,#26599,.F.);
#35292=ORIENTED_EDGE('',*,*,#26475,.F.);
#35293=ORIENTED_EDGE('',*,*,#26467,.F.);
#35294=ORIENTED_EDGE('',*,*,#26436,.F.);
#35295=ORIENTED_EDGE('',*,*,#21615,.F.);
#35296=ORIENTED_EDGE('',*,*,#26577,.F.);
#35297=ORIENTED_EDGE('',*,*,#26600,.T.);
#35298=ORIENTED_EDGE('',*,*,#26534,.F.);
#35299=ORIENTED_EDGE('',*,*,#26600,.F.);
#35300=ORIENTED_EDGE('',*,*,#26575,.F.);
#35301=ORIENTED_EDGE('',*,*,#26472,.F.);
#35302=ORIENTED_EDGE('',*,*,#26599,.T.);
#35303=ORIENTED_EDGE('',*,*,#26431,.F.);
#35304=ORIENTED_EDGE('',*,*,#26527,.F.);
#35305=ORIENTED_EDGE('',*,*,#26601,.T.);
#35306=ORIENTED_EDGE('',*,*,#26572,.F.);
#35307=ORIENTED_EDGE('',*,*,#26487,.F.);
#35308=ORIENTED_EDGE('',*,*,#26512,.F.);
#35309=ORIENTED_EDGE('',*,*,#26393,.F.);
#35310=ORIENTED_EDGE('',*,*,#26464,.F.);
#35311=ORIENTED_EDGE('',*,*,#26602,.F.);
#35312=ORIENTED_EDGE('',*,*,#26413,.F.);
#35313=ORIENTED_EDGE('',*,*,#26602,.T.);
#35314=ORIENTED_EDGE('',*,*,#26460,.F.);
#35315=ORIENTED_EDGE('',*,*,#26565,.F.);
#35316=ORIENTED_EDGE('',*,*,#26601,.F.);
#35317=ORIENTED_EDGE('',*,*,#26508,.F.);
#35318=ORIENTED_EDGE('',*,*,#26410,.F.);
#35319=ORIENTED_EDGE('',*,*,#26603,.F.);
#35320=ORIENTED_EDGE('',*,*,#26462,.F.);
#35321=ORIENTED_EDGE('',*,*,#26389,.F.);
#35322=ORIENTED_EDGE('',*,*,#26454,.F.);
#35323=ORIENTED_EDGE('',*,*,#26483,.F.);
#35324=ORIENTED_EDGE('',*,*,#26570,.F.);
#35325=ORIENTED_EDGE('',*,*,#26604,.T.);
#35326=ORIENTED_EDGE('',*,*,#26562,.F.);
#35327=ORIENTED_EDGE('',*,*,#26604,.F.);
#35328=ORIENTED_EDGE('',*,*,#26566,.F.);
#35329=ORIENTED_EDGE('',*,*,#26459,.F.);
#35330=ORIENTED_EDGE('',*,*,#26603,.T.);
#35331=ORIENTED_EDGE('',*,*,#26449,.F.);
#35332=ORIENTED_EDGE('',*,*,#26555,.F.);
#35333=ORIENTED_EDGE('',*,*,#26605,.F.);
#35334=ORIENTED_EDGE('',*,*,#26451,.F.);
#35335=ORIENTED_EDGE('',*,*,#26397,.F.);
#35336=ORIENTED_EDGE('',*,*,#26443,.F.);
#35337=ORIENTED_EDGE('',*,*,#26491,.F.);
#35338=ORIENTED_EDGE('',*,*,#26560,.F.);
#35339=ORIENTED_EDGE('',*,*,#26606,.T.);
#35340=ORIENTED_EDGE('',*,*,#26552,.F.);
#35341=ORIENTED_EDGE('',*,*,#26606,.F.);
#35342=ORIENTED_EDGE('',*,*,#26556,.F.);
#35343=ORIENTED_EDGE('',*,*,#26448,.F.);
#35344=ORIENTED_EDGE('',*,*,#26605,.T.);
#35345=ORIENTED_EDGE('',*,*,#26441,.F.);
#35346=ORIENTED_EDGE('',*,*,#26544,.F.);
#35347=ORIENTED_EDGE('',*,*,#26495,.F.);
#35348=ORIENTED_EDGE('',*,*,#26549,.F.);
#35349=ORIENTED_EDGE('',*,*,#26607,.T.);
#35350=ORIENTED_EDGE('',*,*,#26541,.F.);
#35351=ORIENTED_EDGE('',*,*,#26608,.F.);
#35352=ORIENTED_EDGE('',*,*,#26551,.F.);
#35353=ORIENTED_EDGE('',*,*,#21281,.F.);
#35354=ORIENTED_EDGE('',*,*,#26537,.F.);
#35355=ORIENTED_EDGE('',*,*,#26607,.F.);
#35356=ORIENTED_EDGE('',*,*,#26545,.F.);
#35357=ORIENTED_EDGE('',*,*,#26440,.F.);
#35358=ORIENTED_EDGE('',*,*,#26608,.T.);
#35359=ORIENTED_EDGE('',*,*,#21280,.F.);
#35360=ORIENTED_EDGE('',*,*,#21277,.F.);
#35361=ORIENTED_EDGE('',*,*,#26609,.F.);
#35362=ORIENTED_EDGE('',*,*,#26433,.F.);
#35363=ORIENTED_EDGE('',*,*,#26401,.F.);
#35364=ORIENTED_EDGE('',*,*,#26425,.F.);
#35365=ORIENTED_EDGE('',*,*,#26499,.F.);
#35366=ORIENTED_EDGE('',*,*,#26532,.F.);
#35367=ORIENTED_EDGE('',*,*,#26610,.T.);
#35368=ORIENTED_EDGE('',*,*,#26524,.F.);
#35369=ORIENTED_EDGE('',*,*,#26610,.F.);
#35370=ORIENTED_EDGE('',*,*,#26528,.F.);
#35371=ORIENTED_EDGE('',*,*,#26430,.F.);
#35372=ORIENTED_EDGE('',*,*,#26609,.T.);
#35373=ORIENTED_EDGE('',*,*,#26421,.F.);
#35374=ORIENTED_EDGE('',*,*,#26517,.F.);
#35375=ORIENTED_EDGE('',*,*,#26611,.F.);
#35376=ORIENTED_EDGE('',*,*,#26518,.F.);
#35377=ORIENTED_EDGE('',*,*,#26420,.F.);
#35378=ORIENTED_EDGE('',*,*,#26612,.T.);
#35379=ORIENTED_EDGE('',*,*,#26411,.F.);
#35380=ORIENTED_EDGE('',*,*,#26507,.F.);
#35381=ORIENTED_EDGE('',*,*,#26503,.F.);
#35382=ORIENTED_EDGE('',*,*,#26522,.F.);
#35383=ORIENTED_EDGE('',*,*,#26611,.T.);
#35384=ORIENTED_EDGE('',*,*,#26514,.F.);
#35385=ORIENTED_EDGE('',*,*,#26612,.F.);
#35386=ORIENTED_EDGE('',*,*,#26423,.F.);
#35387=ORIENTED_EDGE('',*,*,#26405,.F.);
#35388=ORIENTED_EDGE('',*,*,#26415,.F.);
#35389=ORIENTED_EDGE('',*,*,#26381,.F.);
#35390=ORIENTED_EDGE('',*,*,#26613,.F.);
#35391=ORIENTED_EDGE('',*,*,#21605,.F.);
#35392=ORIENTED_EDGE('',*,*,#26613,.T.);
#35393=ORIENTED_EDGE('',*,*,#26377,.F.);
#35394=ORIENTED_EDGE('',*,*,#26478,.F.);
#35395=ORIENTED_EDGE('',*,*,#21606,.F.);
#35396=ORIENTED_EDGE('',*,*,#26614,.F.);
#35397=ORIENTED_EDGE('',*,*,#26379,.F.);
#35398=ORIENTED_EDGE('',*,*,#26371,.F.);
#35399=ORIENTED_EDGE('',*,*,#26368,.F.);
#35400=ORIENTED_EDGE('',*,*,#21609,.F.);
#35401=ORIENTED_EDGE('',*,*,#26481,.F.);
#35402=ORIENTED_EDGE('',*,*,#26615,.T.);
#35403=ORIENTED_EDGE('',*,*,#26476,.F.);
#35404=ORIENTED_EDGE('',*,*,#26615,.F.);
#35405=ORIENTED_EDGE('',*,*,#26479,.F.);
#35406=ORIENTED_EDGE('',*,*,#26376,.F.);
#35407=ORIENTED_EDGE('',*,*,#26614,.T.);
#35408=ORIENTED_EDGE('',*,*,#26363,.F.);
#35409=ORIENTED_EDGE('',*,*,#26469,.F.);
#35410=ORIENTED_EDGE('',*,*,#26616,.F.);
#35411=ORIENTED_EDGE('',*,*,#26365,.F.);
#35412=ORIENTED_EDGE('',*,*,#26357,.F.);
#35413=ORIENTED_EDGE('',*,*,#26336,.F.);
#35414=ORIENTED_EDGE('',*,*,#26466,.F.);
#35415=ORIENTED_EDGE('',*,*,#26474,.F.);
#35416=ORIENTED_EDGE('',*,*,#26617,.T.);
#35417=ORIENTED_EDGE('',*,*,#26435,.F.);
#35418=ORIENTED_EDGE('',*,*,#26617,.F.);
#35419=ORIENTED_EDGE('',*,*,#26470,.F.);
#35420=ORIENTED_EDGE('',*,*,#26362,.F.);
#35421=ORIENTED_EDGE('',*,*,#26616,.T.);
#35422=ORIENTED_EDGE('',*,*,#26331,.F.);
#35423=ORIENTED_EDGE('',*,*,#26427,.F.);
#35424=ORIENTED_EDGE('',*,*,#26618,.T.);
#35425=ORIENTED_EDGE('',*,*,#26463,.F.);
#35426=ORIENTED_EDGE('',*,*,#26391,.F.);
#35427=ORIENTED_EDGE('',*,*,#26412,.F.);
#35428=ORIENTED_EDGE('',*,*,#26297,.F.);
#35429=ORIENTED_EDGE('',*,*,#26354,.F.);
#35430=ORIENTED_EDGE('',*,*,#26619,.F.);
#35431=ORIENTED_EDGE('',*,*,#26313,.F.);
#35432=ORIENTED_EDGE('',*,*,#26619,.T.);
#35433=ORIENTED_EDGE('',*,*,#26349,.F.);
#35434=ORIENTED_EDGE('',*,*,#26456,.F.);
#35435=ORIENTED_EDGE('',*,*,#26618,.F.);
#35436=ORIENTED_EDGE('',*,*,#26408,.F.);
#35437=ORIENTED_EDGE('',*,*,#26310,.F.);
#35438=ORIENTED_EDGE('',*,*,#26620,.F.);
#35439=ORIENTED_EDGE('',*,*,#26351,.F.);
#35440=ORIENTED_EDGE('',*,*,#26293,.F.);
#35441=ORIENTED_EDGE('',*,*,#26343,.F.);
#35442=ORIENTED_EDGE('',*,*,#26387,.F.);
#35443=ORIENTED_EDGE('',*,*,#26461,.F.);
#35444=ORIENTED_EDGE('',*,*,#26621,.T.);
#35445=ORIENTED_EDGE('',*,*,#26453,.F.);
#35446=ORIENTED_EDGE('',*,*,#26621,.F.);
#35447=ORIENTED_EDGE('',*,*,#26457,.F.);
#35448=ORIENTED_EDGE('',*,*,#26348,.F.);
#35449=ORIENTED_EDGE('',*,*,#26620,.T.);
#35450=ORIENTED_EDGE('',*,*,#26341,.F.);
#35451=ORIENTED_EDGE('',*,*,#26445,.F.);
#35452=ORIENTED_EDGE('',*,*,#26395,.F.);
#35453=ORIENTED_EDGE('',*,*,#26450,.F.);
#35454=ORIENTED_EDGE('',*,*,#26622,.T.);
#35455=ORIENTED_EDGE('',*,*,#26442,.F.);
#35456=ORIENTED_EDGE('',*,*,#26623,.F.);
#35457=ORIENTED_EDGE('',*,*,#26452,.F.);
#35458=ORIENTED_EDGE('',*,*,#21285,.F.);
#35459=ORIENTED_EDGE('',*,*,#26438,.F.);
#35460=ORIENTED_EDGE('',*,*,#26622,.F.);
#35461=ORIENTED_EDGE('',*,*,#26446,.F.);
#35462=ORIENTED_EDGE('',*,*,#26340,.F.);
#35463=ORIENTED_EDGE('',*,*,#26623,.T.);
#35464=ORIENTED_EDGE('',*,*,#21284,.F.);
#35465=ORIENTED_EDGE('',*,*,#26624,.F.);
#35466=ORIENTED_EDGE('',*,*,#26333,.F.);
#35467=ORIENTED_EDGE('',*,*,#26301,.F.);
#35468=ORIENTED_EDGE('',*,*,#26325,.F.);
#35469=ORIENTED_EDGE('',*,*,#26399,.F.);
#35470=ORIENTED_EDGE('',*,*,#26432,.F.);
#35471=ORIENTED_EDGE('',*,*,#26625,.T.);
#35472=ORIENTED_EDGE('',*,*,#26424,.F.);
#35473=ORIENTED_EDGE('',*,*,#26625,.F.);
#35474=ORIENTED_EDGE('',*,*,#26428,.F.);
#35475=ORIENTED_EDGE('',*,*,#26330,.F.);
#35476=ORIENTED_EDGE('',*,*,#26624,.T.);
#35477=ORIENTED_EDGE('',*,*,#26321,.F.);
#35478=ORIENTED_EDGE('',*,*,#26417,.F.);
#35479=ORIENTED_EDGE('',*,*,#26626,.F.);
#35480=ORIENTED_EDGE('',*,*,#26418,.F.);
#35481=ORIENTED_EDGE('',*,*,#26320,.F.);
#35482=ORIENTED_EDGE('',*,*,#26627,.T.);
#35483=ORIENTED_EDGE('',*,*,#26311,.F.);
#35484=ORIENTED_EDGE('',*,*,#26407,.F.);
#35485=ORIENTED_EDGE('',*,*,#26403,.F.);
#35486=ORIENTED_EDGE('',*,*,#26422,.F.);
#35487=ORIENTED_EDGE('',*,*,#26626,.T.);
#35488=ORIENTED_EDGE('',*,*,#26414,.F.);
#35489=ORIENTED_EDGE('',*,*,#26627,.F.);
#35490=ORIENTED_EDGE('',*,*,#26323,.F.);
#35491=ORIENTED_EDGE('',*,*,#26305,.F.);
#35492=ORIENTED_EDGE('',*,*,#26315,.F.);
#35493=ORIENTED_EDGE('',*,*,#26285,.F.);
#35494=ORIENTED_EDGE('',*,*,#26628,.F.);
#35495=ORIENTED_EDGE('',*,*,#21599,.F.);
#35496=ORIENTED_EDGE('',*,*,#26628,.T.);
#35497=ORIENTED_EDGE('',*,*,#26281,.F.);
#35498=ORIENTED_EDGE('',*,*,#26382,.F.);
#35499=ORIENTED_EDGE('',*,*,#21600,.F.);
#35500=ORIENTED_EDGE('',*,*,#26629,.F.);
#35501=ORIENTED_EDGE('',*,*,#26283,.F.);
#35502=ORIENTED_EDGE('',*,*,#26275,.F.);
#35503=ORIENTED_EDGE('',*,*,#26272,.F.);
#35504=ORIENTED_EDGE('',*,*,#21603,.F.);
#35505=ORIENTED_EDGE('',*,*,#26385,.F.);
#35506=ORIENTED_EDGE('',*,*,#26630,.T.);
#35507=ORIENTED_EDGE('',*,*,#26380,.F.);
#35508=ORIENTED_EDGE('',*,*,#26630,.F.);
#35509=ORIENTED_EDGE('',*,*,#26383,.F.);
#35510=ORIENTED_EDGE('',*,*,#26280,.F.);
#35511=ORIENTED_EDGE('',*,*,#26629,.T.);
#35512=ORIENTED_EDGE('',*,*,#26267,.F.);
#35513=ORIENTED_EDGE('',*,*,#26373,.F.);
#35514=ORIENTED_EDGE('',*,*,#26631,.F.);
#35515=ORIENTED_EDGE('',*,*,#26269,.F.);
#35516=ORIENTED_EDGE('',*,*,#26261,.F.);
#35517=ORIENTED_EDGE('',*,*,#26258,.F.);
#35518=ORIENTED_EDGE('',*,*,#26370,.F.);
#35519=ORIENTED_EDGE('',*,*,#26378,.F.);
#35520=ORIENTED_EDGE('',*,*,#26632,.T.);
#35521=ORIENTED_EDGE('',*,*,#26367,.F.);
#35522=ORIENTED_EDGE('',*,*,#26632,.F.);
#35523=ORIENTED_EDGE('',*,*,#26374,.F.);
#35524=ORIENTED_EDGE('',*,*,#26266,.F.);
#35525=ORIENTED_EDGE('',*,*,#26631,.T.);
#35526=ORIENTED_EDGE('',*,*,#26253,.F.);
#35527=ORIENTED_EDGE('',*,*,#26359,.F.);
#35528=ORIENTED_EDGE('',*,*,#26633,.F.);
#35529=ORIENTED_EDGE('',*,*,#26255,.F.);
#35530=ORIENTED_EDGE('',*,*,#26247,.F.);
#35531=ORIENTED_EDGE('',*,*,#26237,.F.);
#35532=ORIENTED_EDGE('',*,*,#26356,.F.);
#35533=ORIENTED_EDGE('',*,*,#26364,.F.);
#35534=ORIENTED_EDGE('',*,*,#26634,.T.);
#35535=ORIENTED_EDGE('',*,*,#26335,.F.);
#35536=ORIENTED_EDGE('',*,*,#26634,.F.);
#35537=ORIENTED_EDGE('',*,*,#26360,.F.);
#35538=ORIENTED_EDGE('',*,*,#26252,.F.);
#35539=ORIENTED_EDGE('',*,*,#26633,.T.);
#35540=ORIENTED_EDGE('',*,*,#26232,.F.);
#35541=ORIENTED_EDGE('',*,*,#26327,.F.);
#35542=ORIENTED_EDGE('',*,*,#26635,.T.);
#35543=ORIENTED_EDGE('',*,*,#26353,.F.);
#35544=ORIENTED_EDGE('',*,*,#26295,.F.);
#35545=ORIENTED_EDGE('',*,*,#26312,.F.);
#35546=ORIENTED_EDGE('',*,*,#26197,.F.);
#35547=ORIENTED_EDGE('',*,*,#26244,.F.);
#35548=ORIENTED_EDGE('',*,*,#26636,.F.);
#35549=ORIENTED_EDGE('',*,*,#26213,.F.);
#35550=ORIENTED_EDGE('',*,*,#26636,.T.);
#35551=ORIENTED_EDGE('',*,*,#26242,.F.);
#35552=ORIENTED_EDGE('',*,*,#26345,.F.);
#35553=ORIENTED_EDGE('',*,*,#26635,.F.);
#35554=ORIENTED_EDGE('',*,*,#26308,.F.);
#35555=ORIENTED_EDGE('',*,*,#26210,.F.);
#35556=ORIENTED_EDGE('',*,*,#26291,.F.);
#35557=ORIENTED_EDGE('',*,*,#26350,.F.);
#35558=ORIENTED_EDGE('',*,*,#26637,.T.);
#35559=ORIENTED_EDGE('',*,*,#26342,.F.);
#35560=ORIENTED_EDGE('',*,*,#26638,.F.);
#35561=ORIENTED_EDGE('',*,*,#26352,.F.);
#35562=ORIENTED_EDGE('',*,*,#21289,.F.);
#35563=ORIENTED_EDGE('',*,*,#26338,.F.);
#35564=ORIENTED_EDGE('',*,*,#26637,.F.);
#35565=ORIENTED_EDGE('',*,*,#26346,.F.);
#35566=ORIENTED_EDGE('',*,*,#26241,.F.);
#35567=ORIENTED_EDGE('',*,*,#26638,.T.);
#35568=ORIENTED_EDGE('',*,*,#21288,.F.);
#35569=ORIENTED_EDGE('',*,*,#26639,.F.);
#35570=ORIENTED_EDGE('',*,*,#26234,.F.);
#35571=ORIENTED_EDGE('',*,*,#26201,.F.);
#35572=ORIENTED_EDGE('',*,*,#26226,.F.);
#35573=ORIENTED_EDGE('',*,*,#26299,.F.);
#35574=ORIENTED_EDGE('',*,*,#26332,.F.);
#35575=ORIENTED_EDGE('',*,*,#26640,.T.);
#35576=ORIENTED_EDGE('',*,*,#26324,.F.);
#35577=ORIENTED_EDGE('',*,*,#26640,.F.);
#35578=ORIENTED_EDGE('',*,*,#26328,.F.);
#35579=ORIENTED_EDGE('',*,*,#26231,.F.);
#35580=ORIENTED_EDGE('',*,*,#26639,.T.);
#35581=ORIENTED_EDGE('',*,*,#26222,.F.);
#35582=ORIENTED_EDGE('',*,*,#26317,.F.);
#35583=ORIENTED_EDGE('',*,*,#26641,.F.);
#35584=ORIENTED_EDGE('',*,*,#26318,.F.);
#35585=ORIENTED_EDGE('',*,*,#26221,.F.);
#35586=ORIENTED_EDGE('',*,*,#26642,.T.);
#35587=ORIENTED_EDGE('',*,*,#26211,.F.);
#35588=ORIENTED_EDGE('',*,*,#26307,.F.);
#35589=ORIENTED_EDGE('',*,*,#26303,.F.);
#35590=ORIENTED_EDGE('',*,*,#26322,.F.);
#35591=ORIENTED_EDGE('',*,*,#26641,.T.);
#35592=ORIENTED_EDGE('',*,*,#26314,.F.);
#35593=ORIENTED_EDGE('',*,*,#26642,.F.);
#35594=ORIENTED_EDGE('',*,*,#26224,.F.);
#35595=ORIENTED_EDGE('',*,*,#26205,.F.);
#35596=ORIENTED_EDGE('',*,*,#26216,.F.);
#35597=ORIENTED_EDGE('',*,*,#26189,.F.);
#35598=ORIENTED_EDGE('',*,*,#26643,.F.);
#35599=ORIENTED_EDGE('',*,*,#21593,.F.);
#35600=ORIENTED_EDGE('',*,*,#26643,.T.);
#35601=ORIENTED_EDGE('',*,*,#26185,.F.);
#35602=ORIENTED_EDGE('',*,*,#26286,.F.);
#35603=ORIENTED_EDGE('',*,*,#21594,.F.);
#35604=ORIENTED_EDGE('',*,*,#26644,.F.);
#35605=ORIENTED_EDGE('',*,*,#26187,.F.);
#35606=ORIENTED_EDGE('',*,*,#26179,.F.);
#35607=ORIENTED_EDGE('',*,*,#26176,.F.);
#35608=ORIENTED_EDGE('',*,*,#21597,.F.);
#35609=ORIENTED_EDGE('',*,*,#26289,.F.);
#35610=ORIENTED_EDGE('',*,*,#26645,.T.);
#35611=ORIENTED_EDGE('',*,*,#26284,.F.);
#35612=ORIENTED_EDGE('',*,*,#26645,.F.);
#35613=ORIENTED_EDGE('',*,*,#26287,.F.);
#35614=ORIENTED_EDGE('',*,*,#26184,.F.);
#35615=ORIENTED_EDGE('',*,*,#26644,.T.);
#35616=ORIENTED_EDGE('',*,*,#26171,.F.);
#35617=ORIENTED_EDGE('',*,*,#26277,.F.);
#35618=ORIENTED_EDGE('',*,*,#26646,.F.);
#35619=ORIENTED_EDGE('',*,*,#26173,.F.);
#35620=ORIENTED_EDGE('',*,*,#26165,.F.);
#35621=ORIENTED_EDGE('',*,*,#26162,.F.);
#35622=ORIENTED_EDGE('',*,*,#26274,.F.);
#35623=ORIENTED_EDGE('',*,*,#26282,.F.);
#35624=ORIENTED_EDGE('',*,*,#26647,.T.);
#35625=ORIENTED_EDGE('',*,*,#26271,.F.);
#35626=ORIENTED_EDGE('',*,*,#26647,.F.);
#35627=ORIENTED_EDGE('',*,*,#26278,.F.);
#35628=ORIENTED_EDGE('',*,*,#26170,.F.);
#35629=ORIENTED_EDGE('',*,*,#26646,.T.);
#35630=ORIENTED_EDGE('',*,*,#26157,.F.);
#35631=ORIENTED_EDGE('',*,*,#26263,.F.);
#35632=ORIENTED_EDGE('',*,*,#26648,.F.);
#35633=ORIENTED_EDGE('',*,*,#26159,.F.);
#35634=ORIENTED_EDGE('',*,*,#26151,.F.);
#35635=ORIENTED_EDGE('',*,*,#26148,.F.);
#35636=ORIENTED_EDGE('',*,*,#26260,.F.);
#35637=ORIENTED_EDGE('',*,*,#26268,.F.);
#35638=ORIENTED_EDGE('',*,*,#26649,.T.);
#35639=ORIENTED_EDGE('',*,*,#26257,.F.);
#35640=ORIENTED_EDGE('',*,*,#26649,.F.);
#35641=ORIENTED_EDGE('',*,*,#26264,.F.);
#35642=ORIENTED_EDGE('',*,*,#26156,.F.);
#35643=ORIENTED_EDGE('',*,*,#26648,.T.);
#35644=ORIENTED_EDGE('',*,*,#26143,.F.);
#35645=ORIENTED_EDGE('',*,*,#26249,.F.);
#35646=ORIENTED_EDGE('',*,*,#26650,.F.);
#35647=ORIENTED_EDGE('',*,*,#26145,.F.);
#35648=ORIENTED_EDGE('',*,*,#26137,.F.);
#35649=ORIENTED_EDGE('',*,*,#26134,.F.);
#35650=ORIENTED_EDGE('',*,*,#26246,.F.);
#35651=ORIENTED_EDGE('',*,*,#26254,.F.);
#35652=ORIENTED_EDGE('',*,*,#26651,.T.);
#35653=ORIENTED_EDGE('',*,*,#26236,.F.);
#35654=ORIENTED_EDGE('',*,*,#26651,.F.);
#35655=ORIENTED_EDGE('',*,*,#26250,.F.);
#35656=ORIENTED_EDGE('',*,*,#26142,.F.);
#35657=ORIENTED_EDGE('',*,*,#26650,.T.);
#35658=ORIENTED_EDGE('',*,*,#26129,.F.);
#35659=ORIENTED_EDGE('',*,*,#26228,.F.);
#35660=ORIENTED_EDGE('',*,*,#26652,.T.);
#35661=ORIENTED_EDGE('',*,*,#26243,.F.);
#35662=ORIENTED_EDGE('',*,*,#26195,.F.);
#35663=ORIENTED_EDGE('',*,*,#26212,.F.);
#35664=ORIENTED_EDGE('',*,*,#26653,.T.);
#35665=ORIENTED_EDGE('',*,*,#21292,.F.);
#35666=ORIENTED_EDGE('',*,*,#26239,.F.);
#35667=ORIENTED_EDGE('',*,*,#26652,.F.);
#35668=ORIENTED_EDGE('',*,*,#26208,.F.);
#35669=ORIENTED_EDGE('',*,*,#26109,.F.);
#35670=ORIENTED_EDGE('',*,*,#26653,.F.);
#35671=ORIENTED_EDGE('',*,*,#26214,.F.);
#35672=ORIENTED_EDGE('',*,*,#21293,.F.);
#35673=ORIENTED_EDGE('',*,*,#26654,.F.);
#35674=ORIENTED_EDGE('',*,*,#26131,.F.);
#35675=ORIENTED_EDGE('',*,*,#26101,.F.);
#35676=ORIENTED_EDGE('',*,*,#26123,.F.);
#35677=ORIENTED_EDGE('',*,*,#26199,.F.);
#35678=ORIENTED_EDGE('',*,*,#26233,.F.);
#35679=ORIENTED_EDGE('',*,*,#26655,.T.);
#35680=ORIENTED_EDGE('',*,*,#26225,.F.);
#35681=ORIENTED_EDGE('',*,*,#26655,.F.);
#35682=ORIENTED_EDGE('',*,*,#26229,.F.);
#35683=ORIENTED_EDGE('',*,*,#26128,.F.);
#35684=ORIENTED_EDGE('',*,*,#26654,.T.);
#35685=ORIENTED_EDGE('',*,*,#26118,.F.);
#35686=ORIENTED_EDGE('',*,*,#26218,.F.);
#35687=ORIENTED_EDGE('',*,*,#26656,.F.);
#35688=ORIENTED_EDGE('',*,*,#26219,.F.);
#35689=ORIENTED_EDGE('',*,*,#26117,.F.);
#35690=ORIENTED_EDGE('',*,*,#26657,.T.);
#35691=ORIENTED_EDGE('',*,*,#26110,.F.);
#35692=ORIENTED_EDGE('',*,*,#26207,.F.);
#35693=ORIENTED_EDGE('',*,*,#26203,.F.);
#35694=ORIENTED_EDGE('',*,*,#26223,.F.);
#35695=ORIENTED_EDGE('',*,*,#26656,.T.);
#35696=ORIENTED_EDGE('',*,*,#26215,.F.);
#35697=ORIENTED_EDGE('',*,*,#26657,.F.);
#35698=ORIENTED_EDGE('',*,*,#26120,.F.);
#35699=ORIENTED_EDGE('',*,*,#26105,.F.);
#35700=ORIENTED_EDGE('',*,*,#26112,.F.);
#35701=ORIENTED_EDGE('',*,*,#26093,.F.);
#35702=ORIENTED_EDGE('',*,*,#26658,.F.);
#35703=ORIENTED_EDGE('',*,*,#21587,.F.);
#35704=ORIENTED_EDGE('',*,*,#26658,.T.);
#35705=ORIENTED_EDGE('',*,*,#26089,.F.);
#35706=ORIENTED_EDGE('',*,*,#26190,.F.);
#35707=ORIENTED_EDGE('',*,*,#21588,.F.);
#35708=ORIENTED_EDGE('',*,*,#26659,.F.);
#35709=ORIENTED_EDGE('',*,*,#26091,.F.);
#35710=ORIENTED_EDGE('',*,*,#26083,.F.);
#35711=ORIENTED_EDGE('',*,*,#26080,.F.);
#35712=ORIENTED_EDGE('',*,*,#21591,.F.);
#35713=ORIENTED_EDGE('',*,*,#26193,.F.);
#35714=ORIENTED_EDGE('',*,*,#26660,.T.);
#35715=ORIENTED_EDGE('',*,*,#26188,.F.);
#35716=ORIENTED_EDGE('',*,*,#26660,.F.);
#35717=ORIENTED_EDGE('',*,*,#26191,.F.);
#35718=ORIENTED_EDGE('',*,*,#26088,.F.);
#35719=ORIENTED_EDGE('',*,*,#26659,.T.);
#35720=ORIENTED_EDGE('',*,*,#26075,.F.);
#35721=ORIENTED_EDGE('',*,*,#26181,.F.);
#35722=ORIENTED_EDGE('',*,*,#26661,.F.);
#35723=ORIENTED_EDGE('',*,*,#26077,.F.);
#35724=ORIENTED_EDGE('',*,*,#26069,.F.);
#35725=ORIENTED_EDGE('',*,*,#26066,.F.);
#35726=ORIENTED_EDGE('',*,*,#26178,.F.);
#35727=ORIENTED_EDGE('',*,*,#26186,.F.);
#35728=ORIENTED_EDGE('',*,*,#26662,.T.);
#35729=ORIENTED_EDGE('',*,*,#26175,.F.);
#35730=ORIENTED_EDGE('',*,*,#26662,.F.);
#35731=ORIENTED_EDGE('',*,*,#26182,.F.);
#35732=ORIENTED_EDGE('',*,*,#26074,.F.);
#35733=ORIENTED_EDGE('',*,*,#26661,.T.);
#35734=ORIENTED_EDGE('',*,*,#26061,.F.);
#35735=ORIENTED_EDGE('',*,*,#26167,.F.);
#35736=ORIENTED_EDGE('',*,*,#26663,.F.);
#35737=ORIENTED_EDGE('',*,*,#26063,.F.);
#35738=ORIENTED_EDGE('',*,*,#26055,.F.);
#35739=ORIENTED_EDGE('',*,*,#26052,.F.);
#35740=ORIENTED_EDGE('',*,*,#26164,.F.);
#35741=ORIENTED_EDGE('',*,*,#26172,.F.);
#35742=ORIENTED_EDGE('',*,*,#26664,.T.);
#35743=ORIENTED_EDGE('',*,*,#26161,.F.);
#35744=ORIENTED_EDGE('',*,*,#26664,.F.);
#35745=ORIENTED_EDGE('',*,*,#26168,.F.);
#35746=ORIENTED_EDGE('',*,*,#26060,.F.);
#35747=ORIENTED_EDGE('',*,*,#26663,.T.);
#35748=ORIENTED_EDGE('',*,*,#26047,.F.);
#35749=ORIENTED_EDGE('',*,*,#26153,.F.);
#35750=ORIENTED_EDGE('',*,*,#26665,.F.);
#35751=ORIENTED_EDGE('',*,*,#26049,.F.);
#35752=ORIENTED_EDGE('',*,*,#26041,.F.);
#35753=ORIENTED_EDGE('',*,*,#26038,.F.);
#35754=ORIENTED_EDGE('',*,*,#26150,.F.);
#35755=ORIENTED_EDGE('',*,*,#26158,.F.);
#35756=ORIENTED_EDGE('',*,*,#26666,.T.);
#35757=ORIENTED_EDGE('',*,*,#26147,.F.);
#35758=ORIENTED_EDGE('',*,*,#26666,.F.);
#35759=ORIENTED_EDGE('',*,*,#26154,.F.);
#35760=ORIENTED_EDGE('',*,*,#26046,.F.);
#35761=ORIENTED_EDGE('',*,*,#26665,.T.);
#35762=ORIENTED_EDGE('',*,*,#26033,.F.);
#35763=ORIENTED_EDGE('',*,*,#26139,.F.);
#35764=ORIENTED_EDGE('',*,*,#26667,.F.);
#35765=ORIENTED_EDGE('',*,*,#26035,.F.);
#35766=ORIENTED_EDGE('',*,*,#26027,.F.);
#35767=ORIENTED_EDGE('',*,*,#26024,.F.);
#35768=ORIENTED_EDGE('',*,*,#26136,.F.);
#35769=ORIENTED_EDGE('',*,*,#26144,.F.);
#35770=ORIENTED_EDGE('',*,*,#26668,.T.);
#35771=ORIENTED_EDGE('',*,*,#26133,.F.);
#35772=ORIENTED_EDGE('',*,*,#26668,.F.);
#35773=ORIENTED_EDGE('',*,*,#26140,.F.);
#35774=ORIENTED_EDGE('',*,*,#26032,.F.);
#35775=ORIENTED_EDGE('',*,*,#26667,.T.);
#35776=ORIENTED_EDGE('',*,*,#26018,.F.);
#35777=ORIENTED_EDGE('',*,*,#26125,.F.);
#35778=ORIENTED_EDGE('',*,*,#26669,.F.);
#35779=ORIENTED_EDGE('',*,*,#26020,.F.);
#35780=ORIENTED_EDGE('',*,*,#26005,.F.);
#35781=ORIENTED_EDGE('',*,*,#26012,.F.);
#35782=ORIENTED_EDGE('',*,*,#26099,.F.);
#35783=ORIENTED_EDGE('',*,*,#26130,.F.);
#35784=ORIENTED_EDGE('',*,*,#26670,.T.);
#35785=ORIENTED_EDGE('',*,*,#26122,.F.);
#35786=ORIENTED_EDGE('',*,*,#26670,.F.);
#35787=ORIENTED_EDGE('',*,*,#26126,.F.);
#35788=ORIENTED_EDGE('',*,*,#26017,.F.);
#35789=ORIENTED_EDGE('',*,*,#26669,.T.);
#35790=ORIENTED_EDGE('',*,*,#26010,.F.);
#35791=ORIENTED_EDGE('',*,*,#26114,.F.);
#35792=ORIENTED_EDGE('',*,*,#26107,.F.);
#35793=ORIENTED_EDGE('',*,*,#26671,.F.);
#35794=ORIENTED_EDGE('',*,*,#26115,.F.);
#35795=ORIENTED_EDGE('',*,*,#26009,.F.);
#35796=ORIENTED_EDGE('',*,*,#26672,.T.);
#35797=ORIENTED_EDGE('',*,*,#21296,.F.);
#35798=ORIENTED_EDGE('',*,*,#26103,.F.);
#35799=ORIENTED_EDGE('',*,*,#26119,.F.);
#35800=ORIENTED_EDGE('',*,*,#26671,.T.);
#35801=ORIENTED_EDGE('',*,*,#26111,.F.);
#35802=ORIENTED_EDGE('',*,*,#26672,.F.);
#35803=ORIENTED_EDGE('',*,*,#26121,.F.);
#35804=ORIENTED_EDGE('',*,*,#21297,.F.);
#35805=ORIENTED_EDGE('',*,*,#25997,.F.);
#35806=ORIENTED_EDGE('',*,*,#26673,.F.);
#35807=ORIENTED_EDGE('',*,*,#21581,.F.);
#35808=ORIENTED_EDGE('',*,*,#26673,.T.);
#35809=ORIENTED_EDGE('',*,*,#25993,.F.);
#35810=ORIENTED_EDGE('',*,*,#26094,.F.);
#35811=ORIENTED_EDGE('',*,*,#21582,.F.);
#35812=ORIENTED_EDGE('',*,*,#26674,.F.);
#35813=ORIENTED_EDGE('',*,*,#25995,.F.);
#35814=ORIENTED_EDGE('',*,*,#25987,.F.);
#35815=ORIENTED_EDGE('',*,*,#25984,.F.);
#35816=ORIENTED_EDGE('',*,*,#21585,.F.);
#35817=ORIENTED_EDGE('',*,*,#26097,.F.);
#35818=ORIENTED_EDGE('',*,*,#26675,.T.);
#35819=ORIENTED_EDGE('',*,*,#26092,.F.);
#35820=ORIENTED_EDGE('',*,*,#26675,.F.);
#35821=ORIENTED_EDGE('',*,*,#26095,.F.);
#35822=ORIENTED_EDGE('',*,*,#25992,.F.);
#35823=ORIENTED_EDGE('',*,*,#26674,.T.);
#35824=ORIENTED_EDGE('',*,*,#25979,.F.);
#35825=ORIENTED_EDGE('',*,*,#26085,.F.);
#35826=ORIENTED_EDGE('',*,*,#26676,.F.);
#35827=ORIENTED_EDGE('',*,*,#25981,.F.);
#35828=ORIENTED_EDGE('',*,*,#25973,.F.);
#35829=ORIENTED_EDGE('',*,*,#25970,.F.);
#35830=ORIENTED_EDGE('',*,*,#26082,.F.);
#35831=ORIENTED_EDGE('',*,*,#26090,.F.);
#35832=ORIENTED_EDGE('',*,*,#26677,.T.);
#35833=ORIENTED_EDGE('',*,*,#26079,.F.);
#35834=ORIENTED_EDGE('',*,*,#26677,.F.);
#35835=ORIENTED_EDGE('',*,*,#26086,.F.);
#35836=ORIENTED_EDGE('',*,*,#25978,.F.);
#35837=ORIENTED_EDGE('',*,*,#26676,.T.);
#35838=ORIENTED_EDGE('',*,*,#25965,.F.);
#35839=ORIENTED_EDGE('',*,*,#26071,.F.);
#35840=ORIENTED_EDGE('',*,*,#26678,.F.);
#35841=ORIENTED_EDGE('',*,*,#25967,.F.);
#35842=ORIENTED_EDGE('',*,*,#25959,.F.);
#35843=ORIENTED_EDGE('',*,*,#25956,.F.);
#35844=ORIENTED_EDGE('',*,*,#26068,.F.);
#35845=ORIENTED_EDGE('',*,*,#26076,.F.);
#35846=ORIENTED_EDGE('',*,*,#26679,.T.);
#35847=ORIENTED_EDGE('',*,*,#26065,.F.);
#35848=ORIENTED_EDGE('',*,*,#26679,.F.);
#35849=ORIENTED_EDGE('',*,*,#26072,.F.);
#35850=ORIENTED_EDGE('',*,*,#25964,.F.);
#35851=ORIENTED_EDGE('',*,*,#26678,.T.);
#35852=ORIENTED_EDGE('',*,*,#25951,.F.);
#35853=ORIENTED_EDGE('',*,*,#26057,.F.);
#35854=ORIENTED_EDGE('',*,*,#26680,.F.);
#35855=ORIENTED_EDGE('',*,*,#25953,.F.);
#35856=ORIENTED_EDGE('',*,*,#25945,.F.);
#35857=ORIENTED_EDGE('',*,*,#25942,.F.);
#35858=ORIENTED_EDGE('',*,*,#26054,.F.);
#35859=ORIENTED_EDGE('',*,*,#26062,.F.);
#35860=ORIENTED_EDGE('',*,*,#26681,.T.);
#35861=ORIENTED_EDGE('',*,*,#26051,.F.);
#35862=ORIENTED_EDGE('',*,*,#26681,.F.);
#35863=ORIENTED_EDGE('',*,*,#26058,.F.);
#35864=ORIENTED_EDGE('',*,*,#25950,.F.);
#35865=ORIENTED_EDGE('',*,*,#26680,.T.);
#35866=ORIENTED_EDGE('',*,*,#25937,.F.);
#35867=ORIENTED_EDGE('',*,*,#26043,.F.);
#35868=ORIENTED_EDGE('',*,*,#26682,.F.);
#35869=ORIENTED_EDGE('',*,*,#25939,.F.);
#35870=ORIENTED_EDGE('',*,*,#25931,.F.);
#35871=ORIENTED_EDGE('',*,*,#25928,.F.);
#35872=ORIENTED_EDGE('',*,*,#26040,.F.);
#35873=ORIENTED_EDGE('',*,*,#26048,.F.);
#35874=ORIENTED_EDGE('',*,*,#26683,.T.);
#35875=ORIENTED_EDGE('',*,*,#26037,.F.);
#35876=ORIENTED_EDGE('',*,*,#26683,.F.);
#35877=ORIENTED_EDGE('',*,*,#26044,.F.);
#35878=ORIENTED_EDGE('',*,*,#25936,.F.);
#35879=ORIENTED_EDGE('',*,*,#26682,.T.);
#35880=ORIENTED_EDGE('',*,*,#25922,.F.);
#35881=ORIENTED_EDGE('',*,*,#26029,.F.);
#35882=ORIENTED_EDGE('',*,*,#26684,.F.);
#35883=ORIENTED_EDGE('',*,*,#25924,.F.);
#35884=ORIENTED_EDGE('',*,*,#25916,.F.);
#35885=ORIENTED_EDGE('',*,*,#25913,.F.);
#35886=ORIENTED_EDGE('',*,*,#26026,.F.);
#35887=ORIENTED_EDGE('',*,*,#26034,.F.);
#35888=ORIENTED_EDGE('',*,*,#26685,.T.);
#35889=ORIENTED_EDGE('',*,*,#26023,.F.);
#35890=ORIENTED_EDGE('',*,*,#26685,.F.);
#35891=ORIENTED_EDGE('',*,*,#26030,.F.);
#35892=ORIENTED_EDGE('',*,*,#25921,.F.);
#35893=ORIENTED_EDGE('',*,*,#26684,.T.);
#35894=ORIENTED_EDGE('',*,*,#25910,.F.);
#35895=ORIENTED_EDGE('',*,*,#26014,.F.);
#35896=ORIENTED_EDGE('',*,*,#26007,.F.);
#35897=ORIENTED_EDGE('',*,*,#26686,.F.);
#35898=ORIENTED_EDGE('',*,*,#26015,.F.);
#35899=ORIENTED_EDGE('',*,*,#25909,.F.);
#35900=ORIENTED_EDGE('',*,*,#26687,.T.);
#35901=ORIENTED_EDGE('',*,*,#21300,.F.);
#35902=ORIENTED_EDGE('',*,*,#26003,.F.);
#35903=ORIENTED_EDGE('',*,*,#26019,.F.);
#35904=ORIENTED_EDGE('',*,*,#26686,.T.);
#35905=ORIENTED_EDGE('',*,*,#26011,.F.);
#35906=ORIENTED_EDGE('',*,*,#26687,.F.);
#35907=ORIENTED_EDGE('',*,*,#26021,.F.);
#35908=ORIENTED_EDGE('',*,*,#21301,.F.);
#35909=ORIENTED_EDGE('',*,*,#25901,.F.);
#35910=ORIENTED_EDGE('',*,*,#26688,.F.);
#35911=ORIENTED_EDGE('',*,*,#21575,.F.);
#35912=ORIENTED_EDGE('',*,*,#26688,.T.);
#35913=ORIENTED_EDGE('',*,*,#25897,.F.);
#35914=ORIENTED_EDGE('',*,*,#25998,.F.);
#35915=ORIENTED_EDGE('',*,*,#21576,.F.);
#35916=ORIENTED_EDGE('',*,*,#26689,.F.);
#35917=ORIENTED_EDGE('',*,*,#25899,.F.);
#35918=ORIENTED_EDGE('',*,*,#25891,.F.);
#35919=ORIENTED_EDGE('',*,*,#25888,.F.);
#35920=ORIENTED_EDGE('',*,*,#21579,.F.);
#35921=ORIENTED_EDGE('',*,*,#26001,.F.);
#35922=ORIENTED_EDGE('',*,*,#26690,.T.);
#35923=ORIENTED_EDGE('',*,*,#25996,.F.);
#35924=ORIENTED_EDGE('',*,*,#26690,.F.);
#35925=ORIENTED_EDGE('',*,*,#25999,.F.);
#35926=ORIENTED_EDGE('',*,*,#25896,.F.);
#35927=ORIENTED_EDGE('',*,*,#26689,.T.);
#35928=ORIENTED_EDGE('',*,*,#25883,.F.);
#35929=ORIENTED_EDGE('',*,*,#25989,.F.);
#35930=ORIENTED_EDGE('',*,*,#26691,.F.);
#35931=ORIENTED_EDGE('',*,*,#25885,.F.);
#35932=ORIENTED_EDGE('',*,*,#25877,.F.);
#35933=ORIENTED_EDGE('',*,*,#25874,.F.);
#35934=ORIENTED_EDGE('',*,*,#25986,.F.);
#35935=ORIENTED_EDGE('',*,*,#25994,.F.);
#35936=ORIENTED_EDGE('',*,*,#26692,.T.);
#35937=ORIENTED_EDGE('',*,*,#25983,.F.);
#35938=ORIENTED_EDGE('',*,*,#26692,.F.);
#35939=ORIENTED_EDGE('',*,*,#25990,.F.);
#35940=ORIENTED_EDGE('',*,*,#25882,.F.);
#35941=ORIENTED_EDGE('',*,*,#26691,.T.);
#35942=ORIENTED_EDGE('',*,*,#25869,.F.);
#35943=ORIENTED_EDGE('',*,*,#25975,.F.);
#35944=ORIENTED_EDGE('',*,*,#26693,.F.);
#35945=ORIENTED_EDGE('',*,*,#25871,.F.);
#35946=ORIENTED_EDGE('',*,*,#25863,.F.);
#35947=ORIENTED_EDGE('',*,*,#25860,.F.);
#35948=ORIENTED_EDGE('',*,*,#25972,.F.);
#35949=ORIENTED_EDGE('',*,*,#25980,.F.);
#35950=ORIENTED_EDGE('',*,*,#26694,.T.);
#35951=ORIENTED_EDGE('',*,*,#25969,.F.);
#35952=ORIENTED_EDGE('',*,*,#26694,.F.);
#35953=ORIENTED_EDGE('',*,*,#25976,.F.);
#35954=ORIENTED_EDGE('',*,*,#25868,.F.);
#35955=ORIENTED_EDGE('',*,*,#26693,.T.);
#35956=ORIENTED_EDGE('',*,*,#25855,.F.);
#35957=ORIENTED_EDGE('',*,*,#25961,.F.);
#35958=ORIENTED_EDGE('',*,*,#26695,.F.);
#35959=ORIENTED_EDGE('',*,*,#25857,.F.);
#35960=ORIENTED_EDGE('',*,*,#25849,.F.);
#35961=ORIENTED_EDGE('',*,*,#25846,.F.);
#35962=ORIENTED_EDGE('',*,*,#25958,.F.);
#35963=ORIENTED_EDGE('',*,*,#25966,.F.);
#35964=ORIENTED_EDGE('',*,*,#26696,.T.);
#35965=ORIENTED_EDGE('',*,*,#25955,.F.);
#35966=ORIENTED_EDGE('',*,*,#26696,.F.);
#35967=ORIENTED_EDGE('',*,*,#25962,.F.);
#35968=ORIENTED_EDGE('',*,*,#25854,.F.);
#35969=ORIENTED_EDGE('',*,*,#26695,.T.);
#35970=ORIENTED_EDGE('',*,*,#25841,.F.);
#35971=ORIENTED_EDGE('',*,*,#25947,.F.);
#35972=ORIENTED_EDGE('',*,*,#26697,.F.);
#35973=ORIENTED_EDGE('',*,*,#25843,.F.);
#35974=ORIENTED_EDGE('',*,*,#25835,.F.);
#35975=ORIENTED_EDGE('',*,*,#25832,.F.);
#35976=ORIENTED_EDGE('',*,*,#25944,.F.);
#35977=ORIENTED_EDGE('',*,*,#25952,.F.);
#35978=ORIENTED_EDGE('',*,*,#26698,.T.);
#35979=ORIENTED_EDGE('',*,*,#25941,.F.);
#35980=ORIENTED_EDGE('',*,*,#26698,.F.);
#35981=ORIENTED_EDGE('',*,*,#25948,.F.);
#35982=ORIENTED_EDGE('',*,*,#25840,.F.);
#35983=ORIENTED_EDGE('',*,*,#26697,.T.);
#35984=ORIENTED_EDGE('',*,*,#25826,.F.);
#35985=ORIENTED_EDGE('',*,*,#25933,.F.);
#35986=ORIENTED_EDGE('',*,*,#26699,.F.);
#35987=ORIENTED_EDGE('',*,*,#25828,.F.);
#35988=ORIENTED_EDGE('',*,*,#25820,.F.);
#35989=ORIENTED_EDGE('',*,*,#25817,.F.);
#35990=ORIENTED_EDGE('',*,*,#25930,.F.);
#35991=ORIENTED_EDGE('',*,*,#25938,.F.);
#35992=ORIENTED_EDGE('',*,*,#26700,.T.);
#35993=ORIENTED_EDGE('',*,*,#25927,.F.);
#35994=ORIENTED_EDGE('',*,*,#26700,.F.);
#35995=ORIENTED_EDGE('',*,*,#25934,.F.);
#35996=ORIENTED_EDGE('',*,*,#25825,.F.);
#35997=ORIENTED_EDGE('',*,*,#26699,.T.);
#35998=ORIENTED_EDGE('',*,*,#25814,.F.);
#35999=ORIENTED_EDGE('',*,*,#25918,.F.);
#36000=ORIENTED_EDGE('',*,*,#25907,.F.);
#36001=ORIENTED_EDGE('',*,*,#26701,.F.);
#36002=ORIENTED_EDGE('',*,*,#25919,.F.);
#36003=ORIENTED_EDGE('',*,*,#25813,.F.);
#36004=ORIENTED_EDGE('',*,*,#26702,.T.);
#36005=ORIENTED_EDGE('',*,*,#21304,.F.);
#36006=ORIENTED_EDGE('',*,*,#25915,.F.);
#36007=ORIENTED_EDGE('',*,*,#25923,.F.);
#36008=ORIENTED_EDGE('',*,*,#26701,.T.);
#36009=ORIENTED_EDGE('',*,*,#25912,.F.);
#36010=ORIENTED_EDGE('',*,*,#26702,.F.);
#36011=ORIENTED_EDGE('',*,*,#25925,.F.);
#36012=ORIENTED_EDGE('',*,*,#21305,.F.);
#36013=ORIENTED_EDGE('',*,*,#25805,.F.);
#36014=ORIENTED_EDGE('',*,*,#26703,.F.);
#36015=ORIENTED_EDGE('',*,*,#21569,.F.);
#36016=ORIENTED_EDGE('',*,*,#26703,.T.);
#36017=ORIENTED_EDGE('',*,*,#25801,.F.);
#36018=ORIENTED_EDGE('',*,*,#25902,.F.);
#36019=ORIENTED_EDGE('',*,*,#21570,.F.);
#36020=ORIENTED_EDGE('',*,*,#26704,.F.);
#36021=ORIENTED_EDGE('',*,*,#25803,.F.);
#36022=ORIENTED_EDGE('',*,*,#25795,.F.);
#36023=ORIENTED_EDGE('',*,*,#25792,.F.);
#36024=ORIENTED_EDGE('',*,*,#21573,.F.);
#36025=ORIENTED_EDGE('',*,*,#25905,.F.);
#36026=ORIENTED_EDGE('',*,*,#26705,.T.);
#36027=ORIENTED_EDGE('',*,*,#25900,.F.);
#36028=ORIENTED_EDGE('',*,*,#26705,.F.);
#36029=ORIENTED_EDGE('',*,*,#25903,.F.);
#36030=ORIENTED_EDGE('',*,*,#25800,.F.);
#36031=ORIENTED_EDGE('',*,*,#26704,.T.);
#36032=ORIENTED_EDGE('',*,*,#25787,.F.);
#36033=ORIENTED_EDGE('',*,*,#25893,.F.);
#36034=ORIENTED_EDGE('',*,*,#26706,.F.);
#36035=ORIENTED_EDGE('',*,*,#25789,.F.);
#36036=ORIENTED_EDGE('',*,*,#25781,.F.);
#36037=ORIENTED_EDGE('',*,*,#25778,.F.);
#36038=ORIENTED_EDGE('',*,*,#25890,.F.);
#36039=ORIENTED_EDGE('',*,*,#25898,.F.);
#36040=ORIENTED_EDGE('',*,*,#26707,.T.);
#36041=ORIENTED_EDGE('',*,*,#25887,.F.);
#36042=ORIENTED_EDGE('',*,*,#26707,.F.);
#36043=ORIENTED_EDGE('',*,*,#25894,.F.);
#36044=ORIENTED_EDGE('',*,*,#25786,.F.);
#36045=ORIENTED_EDGE('',*,*,#26706,.T.);
#36046=ORIENTED_EDGE('',*,*,#25773,.F.);
#36047=ORIENTED_EDGE('',*,*,#25879,.F.);
#36048=ORIENTED_EDGE('',*,*,#26708,.F.);
#36049=ORIENTED_EDGE('',*,*,#25775,.F.);
#36050=ORIENTED_EDGE('',*,*,#25767,.F.);
#36051=ORIENTED_EDGE('',*,*,#25764,.F.);
#36052=ORIENTED_EDGE('',*,*,#25876,.F.);
#36053=ORIENTED_EDGE('',*,*,#25884,.F.);
#36054=ORIENTED_EDGE('',*,*,#26709,.T.);
#36055=ORIENTED_EDGE('',*,*,#25873,.F.);
#36056=ORIENTED_EDGE('',*,*,#26709,.F.);
#36057=ORIENTED_EDGE('',*,*,#25880,.F.);
#36058=ORIENTED_EDGE('',*,*,#25772,.F.);
#36059=ORIENTED_EDGE('',*,*,#26708,.T.);
#36060=ORIENTED_EDGE('',*,*,#25759,.F.);
#36061=ORIENTED_EDGE('',*,*,#25865,.F.);
#36062=ORIENTED_EDGE('',*,*,#26710,.F.);
#36063=ORIENTED_EDGE('',*,*,#25761,.F.);
#36064=ORIENTED_EDGE('',*,*,#25753,.F.);
#36065=ORIENTED_EDGE('',*,*,#25750,.F.);
#36066=ORIENTED_EDGE('',*,*,#25862,.F.);
#36067=ORIENTED_EDGE('',*,*,#25870,.F.);
#36068=ORIENTED_EDGE('',*,*,#26711,.T.);
#36069=ORIENTED_EDGE('',*,*,#25859,.F.);
#36070=ORIENTED_EDGE('',*,*,#26711,.F.);
#36071=ORIENTED_EDGE('',*,*,#25866,.F.);
#36072=ORIENTED_EDGE('',*,*,#25758,.F.);
#36073=ORIENTED_EDGE('',*,*,#26710,.T.);
#36074=ORIENTED_EDGE('',*,*,#25745,.F.);
#36075=ORIENTED_EDGE('',*,*,#25851,.F.);
#36076=ORIENTED_EDGE('',*,*,#26712,.F.);
#36077=ORIENTED_EDGE('',*,*,#25747,.F.);
#36078=ORIENTED_EDGE('',*,*,#25739,.F.);
#36079=ORIENTED_EDGE('',*,*,#25736,.F.);
#36080=ORIENTED_EDGE('',*,*,#25848,.F.);
#36081=ORIENTED_EDGE('',*,*,#25856,.F.);
#36082=ORIENTED_EDGE('',*,*,#26713,.T.);
#36083=ORIENTED_EDGE('',*,*,#25845,.F.);
#36084=ORIENTED_EDGE('',*,*,#26713,.F.);
#36085=ORIENTED_EDGE('',*,*,#25852,.F.);
#36086=ORIENTED_EDGE('',*,*,#25744,.F.);
#36087=ORIENTED_EDGE('',*,*,#26712,.T.);
#36088=ORIENTED_EDGE('',*,*,#25730,.F.);
#36089=ORIENTED_EDGE('',*,*,#25837,.F.);
#36090=ORIENTED_EDGE('',*,*,#26714,.F.);
#36091=ORIENTED_EDGE('',*,*,#25732,.F.);
#36092=ORIENTED_EDGE('',*,*,#25724,.F.);
#36093=ORIENTED_EDGE('',*,*,#25721,.F.);
#36094=ORIENTED_EDGE('',*,*,#25834,.F.);
#36095=ORIENTED_EDGE('',*,*,#25842,.F.);
#36096=ORIENTED_EDGE('',*,*,#26715,.T.);
#36097=ORIENTED_EDGE('',*,*,#25831,.F.);
#36098=ORIENTED_EDGE('',*,*,#26715,.F.);
#36099=ORIENTED_EDGE('',*,*,#25838,.F.);
#36100=ORIENTED_EDGE('',*,*,#25729,.F.);
#36101=ORIENTED_EDGE('',*,*,#26714,.T.);
#36102=ORIENTED_EDGE('',*,*,#25718,.F.);
#36103=ORIENTED_EDGE('',*,*,#25822,.F.);
#36104=ORIENTED_EDGE('',*,*,#25811,.F.);
#36105=ORIENTED_EDGE('',*,*,#26716,.F.);
#36106=ORIENTED_EDGE('',*,*,#25823,.F.);
#36107=ORIENTED_EDGE('',*,*,#25717,.F.);
#36108=ORIENTED_EDGE('',*,*,#26717,.T.);
#36109=ORIENTED_EDGE('',*,*,#21308,.F.);
#36110=ORIENTED_EDGE('',*,*,#25819,.F.);
#36111=ORIENTED_EDGE('',*,*,#25827,.F.);
#36112=ORIENTED_EDGE('',*,*,#26716,.T.);
#36113=ORIENTED_EDGE('',*,*,#25816,.F.);
#36114=ORIENTED_EDGE('',*,*,#26717,.F.);
#36115=ORIENTED_EDGE('',*,*,#25829,.F.);
#36116=ORIENTED_EDGE('',*,*,#21309,.F.);
#36117=ORIENTED_EDGE('',*,*,#25709,.F.);
#36118=ORIENTED_EDGE('',*,*,#26718,.F.);
#36119=ORIENTED_EDGE('',*,*,#21563,.F.);
#36120=ORIENTED_EDGE('',*,*,#26718,.T.);
#36121=ORIENTED_EDGE('',*,*,#25705,.F.);
#36122=ORIENTED_EDGE('',*,*,#25806,.F.);
#36123=ORIENTED_EDGE('',*,*,#21564,.F.);
#36124=ORIENTED_EDGE('',*,*,#26719,.F.);
#36125=ORIENTED_EDGE('',*,*,#25707,.F.);
#36126=ORIENTED_EDGE('',*,*,#25699,.F.);
#36127=ORIENTED_EDGE('',*,*,#25696,.F.);
#36128=ORIENTED_EDGE('',*,*,#21567,.F.);
#36129=ORIENTED_EDGE('',*,*,#25809,.F.);
#36130=ORIENTED_EDGE('',*,*,#26720,.T.);
#36131=ORIENTED_EDGE('',*,*,#25804,.F.);
#36132=ORIENTED_EDGE('',*,*,#26720,.F.);
#36133=ORIENTED_EDGE('',*,*,#25807,.F.);
#36134=ORIENTED_EDGE('',*,*,#25704,.F.);
#36135=ORIENTED_EDGE('',*,*,#26719,.T.);
#36136=ORIENTED_EDGE('',*,*,#25691,.F.);
#36137=ORIENTED_EDGE('',*,*,#25797,.F.);
#36138=ORIENTED_EDGE('',*,*,#26721,.F.);
#36139=ORIENTED_EDGE('',*,*,#25693,.F.);
#36140=ORIENTED_EDGE('',*,*,#25685,.F.);
#36141=ORIENTED_EDGE('',*,*,#25682,.F.);
#36142=ORIENTED_EDGE('',*,*,#25794,.F.);
#36143=ORIENTED_EDGE('',*,*,#25802,.F.);
#36144=ORIENTED_EDGE('',*,*,#26722,.T.);
#36145=ORIENTED_EDGE('',*,*,#25791,.F.);
#36146=ORIENTED_EDGE('',*,*,#26722,.F.);
#36147=ORIENTED_EDGE('',*,*,#25798,.F.);
#36148=ORIENTED_EDGE('',*,*,#25690,.F.);
#36149=ORIENTED_EDGE('',*,*,#26721,.T.);
#36150=ORIENTED_EDGE('',*,*,#25677,.F.);
#36151=ORIENTED_EDGE('',*,*,#25783,.F.);
#36152=ORIENTED_EDGE('',*,*,#26723,.F.);
#36153=ORIENTED_EDGE('',*,*,#25679,.F.);
#36154=ORIENTED_EDGE('',*,*,#25671,.F.);
#36155=ORIENTED_EDGE('',*,*,#25668,.F.);
#36156=ORIENTED_EDGE('',*,*,#25780,.F.);
#36157=ORIENTED_EDGE('',*,*,#25788,.F.);
#36158=ORIENTED_EDGE('',*,*,#26724,.T.);
#36159=ORIENTED_EDGE('',*,*,#25777,.F.);
#36160=ORIENTED_EDGE('',*,*,#26724,.F.);
#36161=ORIENTED_EDGE('',*,*,#25784,.F.);
#36162=ORIENTED_EDGE('',*,*,#25676,.F.);
#36163=ORIENTED_EDGE('',*,*,#26723,.T.);
#36164=ORIENTED_EDGE('',*,*,#25663,.F.);
#36165=ORIENTED_EDGE('',*,*,#25769,.F.);
#36166=ORIENTED_EDGE('',*,*,#26725,.F.);
#36167=ORIENTED_EDGE('',*,*,#25665,.F.);
#36168=ORIENTED_EDGE('',*,*,#25657,.F.);
#36169=ORIENTED_EDGE('',*,*,#25654,.F.);
#36170=ORIENTED_EDGE('',*,*,#25766,.F.);
#36171=ORIENTED_EDGE('',*,*,#25774,.F.);
#36172=ORIENTED_EDGE('',*,*,#26726,.T.);
#36173=ORIENTED_EDGE('',*,*,#25763,.F.);
#36174=ORIENTED_EDGE('',*,*,#26726,.F.);
#36175=ORIENTED_EDGE('',*,*,#25770,.F.);
#36176=ORIENTED_EDGE('',*,*,#25662,.F.);
#36177=ORIENTED_EDGE('',*,*,#26725,.T.);
#36178=ORIENTED_EDGE('',*,*,#25649,.F.);
#36179=ORIENTED_EDGE('',*,*,#25755,.F.);
#36180=ORIENTED_EDGE('',*,*,#26727,.F.);
#36181=ORIENTED_EDGE('',*,*,#25651,.F.);
#36182=ORIENTED_EDGE('',*,*,#25643,.F.);
#36183=ORIENTED_EDGE('',*,*,#25640,.F.);
#36184=ORIENTED_EDGE('',*,*,#25752,.F.);
#36185=ORIENTED_EDGE('',*,*,#25760,.F.);
#36186=ORIENTED_EDGE('',*,*,#26728,.T.);
#36187=ORIENTED_EDGE('',*,*,#25749,.F.);
#36188=ORIENTED_EDGE('',*,*,#26728,.F.);
#36189=ORIENTED_EDGE('',*,*,#25756,.F.);
#36190=ORIENTED_EDGE('',*,*,#25648,.F.);
#36191=ORIENTED_EDGE('',*,*,#26727,.T.);
#36192=ORIENTED_EDGE('',*,*,#25634,.F.);
#36193=ORIENTED_EDGE('',*,*,#25741,.F.);
#36194=ORIENTED_EDGE('',*,*,#26729,.F.);
#36195=ORIENTED_EDGE('',*,*,#25636,.F.);
#36196=ORIENTED_EDGE('',*,*,#25628,.F.);
#36197=ORIENTED_EDGE('',*,*,#25625,.F.);
#36198=ORIENTED_EDGE('',*,*,#25738,.F.);
#36199=ORIENTED_EDGE('',*,*,#25746,.F.);
#36200=ORIENTED_EDGE('',*,*,#26730,.T.);
#36201=ORIENTED_EDGE('',*,*,#25735,.F.);
#36202=ORIENTED_EDGE('',*,*,#26730,.F.);
#36203=ORIENTED_EDGE('',*,*,#25742,.F.);
#36204=ORIENTED_EDGE('',*,*,#25633,.F.);
#36205=ORIENTED_EDGE('',*,*,#26729,.T.);
#36206=ORIENTED_EDGE('',*,*,#25622,.F.);
#36207=ORIENTED_EDGE('',*,*,#25726,.F.);
#36208=ORIENTED_EDGE('',*,*,#25715,.F.);
#36209=ORIENTED_EDGE('',*,*,#26731,.F.);
#36210=ORIENTED_EDGE('',*,*,#25727,.F.);
#36211=ORIENTED_EDGE('',*,*,#25621,.F.);
#36212=ORIENTED_EDGE('',*,*,#26732,.T.);
#36213=ORIENTED_EDGE('',*,*,#21312,.F.);
#36214=ORIENTED_EDGE('',*,*,#25723,.F.);
#36215=ORIENTED_EDGE('',*,*,#25731,.F.);
#36216=ORIENTED_EDGE('',*,*,#26731,.T.);
#36217=ORIENTED_EDGE('',*,*,#25720,.F.);
#36218=ORIENTED_EDGE('',*,*,#26732,.F.);
#36219=ORIENTED_EDGE('',*,*,#25733,.F.);
#36220=ORIENTED_EDGE('',*,*,#21313,.F.);
#36221=ORIENTED_EDGE('',*,*,#25613,.F.);
#36222=ORIENTED_EDGE('',*,*,#26733,.F.);
#36223=ORIENTED_EDGE('',*,*,#21557,.F.);
#36224=ORIENTED_EDGE('',*,*,#26733,.T.);
#36225=ORIENTED_EDGE('',*,*,#25609,.F.);
#36226=ORIENTED_EDGE('',*,*,#25710,.F.);
#36227=ORIENTED_EDGE('',*,*,#21558,.F.);
#36228=ORIENTED_EDGE('',*,*,#26734,.F.);
#36229=ORIENTED_EDGE('',*,*,#25611,.F.);
#36230=ORIENTED_EDGE('',*,*,#25603,.F.);
#36231=ORIENTED_EDGE('',*,*,#25600,.F.);
#36232=ORIENTED_EDGE('',*,*,#21561,.F.);
#36233=ORIENTED_EDGE('',*,*,#25713,.F.);
#36234=ORIENTED_EDGE('',*,*,#26735,.T.);
#36235=ORIENTED_EDGE('',*,*,#25708,.F.);
#36236=ORIENTED_EDGE('',*,*,#26735,.F.);
#36237=ORIENTED_EDGE('',*,*,#25711,.F.);
#36238=ORIENTED_EDGE('',*,*,#25608,.F.);
#36239=ORIENTED_EDGE('',*,*,#26734,.T.);
#36240=ORIENTED_EDGE('',*,*,#25595,.F.);
#36241=ORIENTED_EDGE('',*,*,#25701,.F.);
#36242=ORIENTED_EDGE('',*,*,#26736,.F.);
#36243=ORIENTED_EDGE('',*,*,#25597,.F.);
#36244=ORIENTED_EDGE('',*,*,#25589,.F.);
#36245=ORIENTED_EDGE('',*,*,#25586,.F.);
#36246=ORIENTED_EDGE('',*,*,#25698,.F.);
#36247=ORIENTED_EDGE('',*,*,#25706,.F.);
#36248=ORIENTED_EDGE('',*,*,#26737,.T.);
#36249=ORIENTED_EDGE('',*,*,#25695,.F.);
#36250=ORIENTED_EDGE('',*,*,#26737,.F.);
#36251=ORIENTED_EDGE('',*,*,#25702,.F.);
#36252=ORIENTED_EDGE('',*,*,#25594,.F.);
#36253=ORIENTED_EDGE('',*,*,#26736,.T.);
#36254=ORIENTED_EDGE('',*,*,#25581,.F.);
#36255=ORIENTED_EDGE('',*,*,#25687,.F.);
#36256=ORIENTED_EDGE('',*,*,#26738,.F.);
#36257=ORIENTED_EDGE('',*,*,#25583,.F.);
#36258=ORIENTED_EDGE('',*,*,#25575,.F.);
#36259=ORIENTED_EDGE('',*,*,#25572,.F.);
#36260=ORIENTED_EDGE('',*,*,#25684,.F.);
#36261=ORIENTED_EDGE('',*,*,#25692,.F.);
#36262=ORIENTED_EDGE('',*,*,#26739,.T.);
#36263=ORIENTED_EDGE('',*,*,#25681,.F.);
#36264=ORIENTED_EDGE('',*,*,#26739,.F.);
#36265=ORIENTED_EDGE('',*,*,#25688,.F.);
#36266=ORIENTED_EDGE('',*,*,#25580,.F.);
#36267=ORIENTED_EDGE('',*,*,#26738,.T.);
#36268=ORIENTED_EDGE('',*,*,#25567,.F.);
#36269=ORIENTED_EDGE('',*,*,#25673,.F.);
#36270=ORIENTED_EDGE('',*,*,#26740,.F.);
#36271=ORIENTED_EDGE('',*,*,#25569,.F.);
#36272=ORIENTED_EDGE('',*,*,#25561,.F.);
#36273=ORIENTED_EDGE('',*,*,#25558,.F.);
#36274=ORIENTED_EDGE('',*,*,#25670,.F.);
#36275=ORIENTED_EDGE('',*,*,#25678,.F.);
#36276=ORIENTED_EDGE('',*,*,#26741,.T.);
#36277=ORIENTED_EDGE('',*,*,#25667,.F.);
#36278=ORIENTED_EDGE('',*,*,#26741,.F.);
#36279=ORIENTED_EDGE('',*,*,#25674,.F.);
#36280=ORIENTED_EDGE('',*,*,#25566,.F.);
#36281=ORIENTED_EDGE('',*,*,#26740,.T.);
#36282=ORIENTED_EDGE('',*,*,#25553,.F.);
#36283=ORIENTED_EDGE('',*,*,#25659,.F.);
#36284=ORIENTED_EDGE('',*,*,#26742,.F.);
#36285=ORIENTED_EDGE('',*,*,#25555,.F.);
#36286=ORIENTED_EDGE('',*,*,#25547,.F.);
#36287=ORIENTED_EDGE('',*,*,#25544,.F.);
#36288=ORIENTED_EDGE('',*,*,#25656,.F.);
#36289=ORIENTED_EDGE('',*,*,#25664,.F.);
#36290=ORIENTED_EDGE('',*,*,#26743,.T.);
#36291=ORIENTED_EDGE('',*,*,#25653,.F.);
#36292=ORIENTED_EDGE('',*,*,#26743,.F.);
#36293=ORIENTED_EDGE('',*,*,#25660,.F.);
#36294=ORIENTED_EDGE('',*,*,#25552,.F.);
#36295=ORIENTED_EDGE('',*,*,#26742,.T.);
#36296=ORIENTED_EDGE('',*,*,#25538,.F.);
#36297=ORIENTED_EDGE('',*,*,#25645,.F.);
#36298=ORIENTED_EDGE('',*,*,#26744,.F.);
#36299=ORIENTED_EDGE('',*,*,#25540,.F.);
#36300=ORIENTED_EDGE('',*,*,#25532,.F.);
#36301=ORIENTED_EDGE('',*,*,#25529,.F.);
#36302=ORIENTED_EDGE('',*,*,#25642,.F.);
#36303=ORIENTED_EDGE('',*,*,#25650,.F.);
#36304=ORIENTED_EDGE('',*,*,#26745,.T.);
#36305=ORIENTED_EDGE('',*,*,#25639,.F.);
#36306=ORIENTED_EDGE('',*,*,#26745,.F.);
#36307=ORIENTED_EDGE('',*,*,#25646,.F.);
#36308=ORIENTED_EDGE('',*,*,#25537,.F.);
#36309=ORIENTED_EDGE('',*,*,#26744,.T.);
#36310=ORIENTED_EDGE('',*,*,#25526,.F.);
#36311=ORIENTED_EDGE('',*,*,#25630,.F.);
#36312=ORIENTED_EDGE('',*,*,#25619,.F.);
#36313=ORIENTED_EDGE('',*,*,#26746,.F.);
#36314=ORIENTED_EDGE('',*,*,#25631,.F.);
#36315=ORIENTED_EDGE('',*,*,#25525,.F.);
#36316=ORIENTED_EDGE('',*,*,#26747,.T.);
#36317=ORIENTED_EDGE('',*,*,#21316,.F.);
#36318=ORIENTED_EDGE('',*,*,#25627,.F.);
#36319=ORIENTED_EDGE('',*,*,#25635,.F.);
#36320=ORIENTED_EDGE('',*,*,#26746,.T.);
#36321=ORIENTED_EDGE('',*,*,#25624,.F.);
#36322=ORIENTED_EDGE('',*,*,#26747,.F.);
#36323=ORIENTED_EDGE('',*,*,#25637,.F.);
#36324=ORIENTED_EDGE('',*,*,#21317,.F.);
#36325=ORIENTED_EDGE('',*,*,#25517,.F.);
#36326=ORIENTED_EDGE('',*,*,#26748,.F.);
#36327=ORIENTED_EDGE('',*,*,#21551,.F.);
#36328=ORIENTED_EDGE('',*,*,#26748,.T.);
#36329=ORIENTED_EDGE('',*,*,#25513,.F.);
#36330=ORIENTED_EDGE('',*,*,#25614,.F.);
#36331=ORIENTED_EDGE('',*,*,#21552,.F.);
#36332=ORIENTED_EDGE('',*,*,#26749,.F.);
#36333=ORIENTED_EDGE('',*,*,#25515,.F.);
#36334=ORIENTED_EDGE('',*,*,#25507,.F.);
#36335=ORIENTED_EDGE('',*,*,#25504,.F.);
#36336=ORIENTED_EDGE('',*,*,#21555,.F.);
#36337=ORIENTED_EDGE('',*,*,#25617,.F.);
#36338=ORIENTED_EDGE('',*,*,#26750,.T.);
#36339=ORIENTED_EDGE('',*,*,#25612,.F.);
#36340=ORIENTED_EDGE('',*,*,#26750,.F.);
#36341=ORIENTED_EDGE('',*,*,#25615,.F.);
#36342=ORIENTED_EDGE('',*,*,#25512,.F.);
#36343=ORIENTED_EDGE('',*,*,#26749,.T.);
#36344=ORIENTED_EDGE('',*,*,#25499,.F.);
#36345=ORIENTED_EDGE('',*,*,#25605,.F.);
#36346=ORIENTED_EDGE('',*,*,#26751,.F.);
#36347=ORIENTED_EDGE('',*,*,#25501,.F.);
#36348=ORIENTED_EDGE('',*,*,#25493,.F.);
#36349=ORIENTED_EDGE('',*,*,#25490,.F.);
#36350=ORIENTED_EDGE('',*,*,#25602,.F.);
#36351=ORIENTED_EDGE('',*,*,#25610,.F.);
#36352=ORIENTED_EDGE('',*,*,#26752,.T.);
#36353=ORIENTED_EDGE('',*,*,#25599,.F.);
#36354=ORIENTED_EDGE('',*,*,#26752,.F.);
#36355=ORIENTED_EDGE('',*,*,#25606,.F.);
#36356=ORIENTED_EDGE('',*,*,#25498,.F.);
#36357=ORIENTED_EDGE('',*,*,#26751,.T.);
#36358=ORIENTED_EDGE('',*,*,#25485,.F.);
#36359=ORIENTED_EDGE('',*,*,#25591,.F.);
#36360=ORIENTED_EDGE('',*,*,#26753,.F.);
#36361=ORIENTED_EDGE('',*,*,#25487,.F.);
#36362=ORIENTED_EDGE('',*,*,#25479,.F.);
#36363=ORIENTED_EDGE('',*,*,#25476,.F.);
#36364=ORIENTED_EDGE('',*,*,#25588,.F.);
#36365=ORIENTED_EDGE('',*,*,#25596,.F.);
#36366=ORIENTED_EDGE('',*,*,#26754,.T.);
#36367=ORIENTED_EDGE('',*,*,#25585,.F.);
#36368=ORIENTED_EDGE('',*,*,#26754,.F.);
#36369=ORIENTED_EDGE('',*,*,#25592,.F.);
#36370=ORIENTED_EDGE('',*,*,#25484,.F.);
#36371=ORIENTED_EDGE('',*,*,#26753,.T.);
#36372=ORIENTED_EDGE('',*,*,#25471,.F.);
#36373=ORIENTED_EDGE('',*,*,#25577,.F.);
#36374=ORIENTED_EDGE('',*,*,#26755,.F.);
#36375=ORIENTED_EDGE('',*,*,#25473,.F.);
#36376=ORIENTED_EDGE('',*,*,#25465,.F.);
#36377=ORIENTED_EDGE('',*,*,#25462,.F.);
#36378=ORIENTED_EDGE('',*,*,#25574,.F.);
#36379=ORIENTED_EDGE('',*,*,#25582,.F.);
#36380=ORIENTED_EDGE('',*,*,#26756,.T.);
#36381=ORIENTED_EDGE('',*,*,#25571,.F.);
#36382=ORIENTED_EDGE('',*,*,#26756,.F.);
#36383=ORIENTED_EDGE('',*,*,#25578,.F.);
#36384=ORIENTED_EDGE('',*,*,#25470,.F.);
#36385=ORIENTED_EDGE('',*,*,#26755,.T.);
#36386=ORIENTED_EDGE('',*,*,#25457,.F.);
#36387=ORIENTED_EDGE('',*,*,#25563,.F.);
#36388=ORIENTED_EDGE('',*,*,#26757,.F.);
#36389=ORIENTED_EDGE('',*,*,#25459,.F.);
#36390=ORIENTED_EDGE('',*,*,#25451,.F.);
#36391=ORIENTED_EDGE('',*,*,#25448,.F.);
#36392=ORIENTED_EDGE('',*,*,#25560,.F.);
#36393=ORIENTED_EDGE('',*,*,#25568,.F.);
#36394=ORIENTED_EDGE('',*,*,#26758,.T.);
#36395=ORIENTED_EDGE('',*,*,#25557,.F.);
#36396=ORIENTED_EDGE('',*,*,#26758,.F.);
#36397=ORIENTED_EDGE('',*,*,#25564,.F.);
#36398=ORIENTED_EDGE('',*,*,#25456,.F.);
#36399=ORIENTED_EDGE('',*,*,#26757,.T.);
#36400=ORIENTED_EDGE('',*,*,#25442,.F.);
#36401=ORIENTED_EDGE('',*,*,#25549,.F.);
#36402=ORIENTED_EDGE('',*,*,#26759,.F.);
#36403=ORIENTED_EDGE('',*,*,#25444,.F.);
#36404=ORIENTED_EDGE('',*,*,#25436,.F.);
#36405=ORIENTED_EDGE('',*,*,#25433,.F.);
#36406=ORIENTED_EDGE('',*,*,#25546,.F.);
#36407=ORIENTED_EDGE('',*,*,#25554,.F.);
#36408=ORIENTED_EDGE('',*,*,#26760,.T.);
#36409=ORIENTED_EDGE('',*,*,#25543,.F.);
#36410=ORIENTED_EDGE('',*,*,#26760,.F.);
#36411=ORIENTED_EDGE('',*,*,#25550,.F.);
#36412=ORIENTED_EDGE('',*,*,#25441,.F.);
#36413=ORIENTED_EDGE('',*,*,#26759,.T.);
#36414=ORIENTED_EDGE('',*,*,#25430,.F.);
#36415=ORIENTED_EDGE('',*,*,#25534,.F.);
#36416=ORIENTED_EDGE('',*,*,#25523,.F.);
#36417=ORIENTED_EDGE('',*,*,#26761,.F.);
#36418=ORIENTED_EDGE('',*,*,#25535,.F.);
#36419=ORIENTED_EDGE('',*,*,#25429,.F.);
#36420=ORIENTED_EDGE('',*,*,#26762,.T.);
#36421=ORIENTED_EDGE('',*,*,#21320,.F.);
#36422=ORIENTED_EDGE('',*,*,#25531,.F.);
#36423=ORIENTED_EDGE('',*,*,#25539,.F.);
#36424=ORIENTED_EDGE('',*,*,#26761,.T.);
#36425=ORIENTED_EDGE('',*,*,#25528,.F.);
#36426=ORIENTED_EDGE('',*,*,#26762,.F.);
#36427=ORIENTED_EDGE('',*,*,#25541,.F.);
#36428=ORIENTED_EDGE('',*,*,#21321,.F.);
#36429=ORIENTED_EDGE('',*,*,#25421,.F.);
#36430=ORIENTED_EDGE('',*,*,#26763,.F.);
#36431=ORIENTED_EDGE('',*,*,#21545,.F.);
#36432=ORIENTED_EDGE('',*,*,#26763,.T.);
#36433=ORIENTED_EDGE('',*,*,#25417,.F.);
#36434=ORIENTED_EDGE('',*,*,#25518,.F.);
#36435=ORIENTED_EDGE('',*,*,#21546,.F.);
#36436=ORIENTED_EDGE('',*,*,#26764,.F.);
#36437=ORIENTED_EDGE('',*,*,#25419,.F.);
#36438=ORIENTED_EDGE('',*,*,#25411,.F.);
#36439=ORIENTED_EDGE('',*,*,#25408,.F.);
#36440=ORIENTED_EDGE('',*,*,#21549,.F.);
#36441=ORIENTED_EDGE('',*,*,#25521,.F.);
#36442=ORIENTED_EDGE('',*,*,#26765,.T.);
#36443=ORIENTED_EDGE('',*,*,#25516,.F.);
#36444=ORIENTED_EDGE('',*,*,#26765,.F.);
#36445=ORIENTED_EDGE('',*,*,#25519,.F.);
#36446=ORIENTED_EDGE('',*,*,#25416,.F.);
#36447=ORIENTED_EDGE('',*,*,#26764,.T.);
#36448=ORIENTED_EDGE('',*,*,#25403,.F.);
#36449=ORIENTED_EDGE('',*,*,#25509,.F.);
#36450=ORIENTED_EDGE('',*,*,#26766,.F.);
#36451=ORIENTED_EDGE('',*,*,#25405,.F.);
#36452=ORIENTED_EDGE('',*,*,#25397,.F.);
#36453=ORIENTED_EDGE('',*,*,#25394,.F.);
#36454=ORIENTED_EDGE('',*,*,#25506,.F.);
#36455=ORIENTED_EDGE('',*,*,#25514,.F.);
#36456=ORIENTED_EDGE('',*,*,#26767,.T.);
#36457=ORIENTED_EDGE('',*,*,#25503,.F.);
#36458=ORIENTED_EDGE('',*,*,#26767,.F.);
#36459=ORIENTED_EDGE('',*,*,#25510,.F.);
#36460=ORIENTED_EDGE('',*,*,#25402,.F.);
#36461=ORIENTED_EDGE('',*,*,#26766,.T.);
#36462=ORIENTED_EDGE('',*,*,#25389,.F.);
#36463=ORIENTED_EDGE('',*,*,#25495,.F.);
#36464=ORIENTED_EDGE('',*,*,#26768,.F.);
#36465=ORIENTED_EDGE('',*,*,#25391,.F.);
#36466=ORIENTED_EDGE('',*,*,#25383,.F.);
#36467=ORIENTED_EDGE('',*,*,#25380,.F.);
#36468=ORIENTED_EDGE('',*,*,#25492,.F.);
#36469=ORIENTED_EDGE('',*,*,#25500,.F.);
#36470=ORIENTED_EDGE('',*,*,#26769,.T.);
#36471=ORIENTED_EDGE('',*,*,#25489,.F.);
#36472=ORIENTED_EDGE('',*,*,#26769,.F.);
#36473=ORIENTED_EDGE('',*,*,#25496,.F.);
#36474=ORIENTED_EDGE('',*,*,#25388,.F.);
#36475=ORIENTED_EDGE('',*,*,#26768,.T.);
#36476=ORIENTED_EDGE('',*,*,#25375,.F.);
#36477=ORIENTED_EDGE('',*,*,#25481,.F.);
#36478=ORIENTED_EDGE('',*,*,#26770,.F.);
#36479=ORIENTED_EDGE('',*,*,#25377,.F.);
#36480=ORIENTED_EDGE('',*,*,#25369,.F.);
#36481=ORIENTED_EDGE('',*,*,#25366,.F.);
#36482=ORIENTED_EDGE('',*,*,#25478,.F.);
#36483=ORIENTED_EDGE('',*,*,#25486,.F.);
#36484=ORIENTED_EDGE('',*,*,#26771,.T.);
#36485=ORIENTED_EDGE('',*,*,#25475,.F.);
#36486=ORIENTED_EDGE('',*,*,#26771,.F.);
#36487=ORIENTED_EDGE('',*,*,#25482,.F.);
#36488=ORIENTED_EDGE('',*,*,#25374,.F.);
#36489=ORIENTED_EDGE('',*,*,#26770,.T.);
#36490=ORIENTED_EDGE('',*,*,#25361,.F.);
#36491=ORIENTED_EDGE('',*,*,#25467,.F.);
#36492=ORIENTED_EDGE('',*,*,#26772,.F.);
#36493=ORIENTED_EDGE('',*,*,#25363,.F.);
#36494=ORIENTED_EDGE('',*,*,#25355,.F.);
#36495=ORIENTED_EDGE('',*,*,#25352,.F.);
#36496=ORIENTED_EDGE('',*,*,#25464,.F.);
#36497=ORIENTED_EDGE('',*,*,#25472,.F.);
#36498=ORIENTED_EDGE('',*,*,#26773,.T.);
#36499=ORIENTED_EDGE('',*,*,#25461,.F.);
#36500=ORIENTED_EDGE('',*,*,#26773,.F.);
#36501=ORIENTED_EDGE('',*,*,#25468,.F.);
#36502=ORIENTED_EDGE('',*,*,#25360,.F.);
#36503=ORIENTED_EDGE('',*,*,#26772,.T.);
#36504=ORIENTED_EDGE('',*,*,#25346,.F.);
#36505=ORIENTED_EDGE('',*,*,#25453,.F.);
#36506=ORIENTED_EDGE('',*,*,#26774,.F.);
#36507=ORIENTED_EDGE('',*,*,#25348,.F.);
#36508=ORIENTED_EDGE('',*,*,#25340,.F.);
#36509=ORIENTED_EDGE('',*,*,#25337,.F.);
#36510=ORIENTED_EDGE('',*,*,#25450,.F.);
#36511=ORIENTED_EDGE('',*,*,#25458,.F.);
#36512=ORIENTED_EDGE('',*,*,#26775,.T.);
#36513=ORIENTED_EDGE('',*,*,#25447,.F.);
#36514=ORIENTED_EDGE('',*,*,#26775,.F.);
#36515=ORIENTED_EDGE('',*,*,#25454,.F.);
#36516=ORIENTED_EDGE('',*,*,#25345,.F.);
#36517=ORIENTED_EDGE('',*,*,#26774,.T.);
#36518=ORIENTED_EDGE('',*,*,#25334,.F.);
#36519=ORIENTED_EDGE('',*,*,#25438,.F.);
#36520=ORIENTED_EDGE('',*,*,#25427,.F.);
#36521=ORIENTED_EDGE('',*,*,#26776,.F.);
#36522=ORIENTED_EDGE('',*,*,#25439,.F.);
#36523=ORIENTED_EDGE('',*,*,#25333,.F.);
#36524=ORIENTED_EDGE('',*,*,#26777,.T.);
#36525=ORIENTED_EDGE('',*,*,#21324,.F.);
#36526=ORIENTED_EDGE('',*,*,#25435,.F.);
#36527=ORIENTED_EDGE('',*,*,#25443,.F.);
#36528=ORIENTED_EDGE('',*,*,#26776,.T.);
#36529=ORIENTED_EDGE('',*,*,#25432,.F.);
#36530=ORIENTED_EDGE('',*,*,#26777,.F.);
#36531=ORIENTED_EDGE('',*,*,#25445,.F.);
#36532=ORIENTED_EDGE('',*,*,#21325,.F.);
#36533=ORIENTED_EDGE('',*,*,#25325,.F.);
#36534=ORIENTED_EDGE('',*,*,#26778,.F.);
#36535=ORIENTED_EDGE('',*,*,#21539,.F.);
#36536=ORIENTED_EDGE('',*,*,#26778,.T.);
#36537=ORIENTED_EDGE('',*,*,#25321,.F.);
#36538=ORIENTED_EDGE('',*,*,#25422,.F.);
#36539=ORIENTED_EDGE('',*,*,#21540,.F.);
#36540=ORIENTED_EDGE('',*,*,#26779,.F.);
#36541=ORIENTED_EDGE('',*,*,#25323,.F.);
#36542=ORIENTED_EDGE('',*,*,#25315,.F.);
#36543=ORIENTED_EDGE('',*,*,#25312,.F.);
#36544=ORIENTED_EDGE('',*,*,#21543,.F.);
#36545=ORIENTED_EDGE('',*,*,#25425,.F.);
#36546=ORIENTED_EDGE('',*,*,#26780,.T.);
#36547=ORIENTED_EDGE('',*,*,#25420,.F.);
#36548=ORIENTED_EDGE('',*,*,#26780,.F.);
#36549=ORIENTED_EDGE('',*,*,#25423,.F.);
#36550=ORIENTED_EDGE('',*,*,#25320,.F.);
#36551=ORIENTED_EDGE('',*,*,#26779,.T.);
#36552=ORIENTED_EDGE('',*,*,#25307,.F.);
#36553=ORIENTED_EDGE('',*,*,#25413,.F.);
#36554=ORIENTED_EDGE('',*,*,#26781,.F.);
#36555=ORIENTED_EDGE('',*,*,#25309,.F.);
#36556=ORIENTED_EDGE('',*,*,#25301,.F.);
#36557=ORIENTED_EDGE('',*,*,#25298,.F.);
#36558=ORIENTED_EDGE('',*,*,#25410,.F.);
#36559=ORIENTED_EDGE('',*,*,#25418,.F.);
#36560=ORIENTED_EDGE('',*,*,#26782,.T.);
#36561=ORIENTED_EDGE('',*,*,#25407,.F.);
#36562=ORIENTED_EDGE('',*,*,#26782,.F.);
#36563=ORIENTED_EDGE('',*,*,#25414,.F.);
#36564=ORIENTED_EDGE('',*,*,#25306,.F.);
#36565=ORIENTED_EDGE('',*,*,#26781,.T.);
#36566=ORIENTED_EDGE('',*,*,#25293,.F.);
#36567=ORIENTED_EDGE('',*,*,#25399,.F.);
#36568=ORIENTED_EDGE('',*,*,#26783,.F.);
#36569=ORIENTED_EDGE('',*,*,#25295,.F.);
#36570=ORIENTED_EDGE('',*,*,#25287,.F.);
#36571=ORIENTED_EDGE('',*,*,#25284,.F.);
#36572=ORIENTED_EDGE('',*,*,#25396,.F.);
#36573=ORIENTED_EDGE('',*,*,#25404,.F.);
#36574=ORIENTED_EDGE('',*,*,#26784,.T.);
#36575=ORIENTED_EDGE('',*,*,#25393,.F.);
#36576=ORIENTED_EDGE('',*,*,#26784,.F.);
#36577=ORIENTED_EDGE('',*,*,#25400,.F.);
#36578=ORIENTED_EDGE('',*,*,#25292,.F.);
#36579=ORIENTED_EDGE('',*,*,#26783,.T.);
#36580=ORIENTED_EDGE('',*,*,#25279,.F.);
#36581=ORIENTED_EDGE('',*,*,#25385,.F.);
#36582=ORIENTED_EDGE('',*,*,#26785,.F.);
#36583=ORIENTED_EDGE('',*,*,#25281,.F.);
#36584=ORIENTED_EDGE('',*,*,#25273,.F.);
#36585=ORIENTED_EDGE('',*,*,#25270,.F.);
#36586=ORIENTED_EDGE('',*,*,#25382,.F.);
#36587=ORIENTED_EDGE('',*,*,#25390,.F.);
#36588=ORIENTED_EDGE('',*,*,#26786,.T.);
#36589=ORIENTED_EDGE('',*,*,#25379,.F.);
#36590=ORIENTED_EDGE('',*,*,#26786,.F.);
#36591=ORIENTED_EDGE('',*,*,#25386,.F.);
#36592=ORIENTED_EDGE('',*,*,#25278,.F.);
#36593=ORIENTED_EDGE('',*,*,#26785,.T.);
#36594=ORIENTED_EDGE('',*,*,#25265,.F.);
#36595=ORIENTED_EDGE('',*,*,#25371,.F.);
#36596=ORIENTED_EDGE('',*,*,#26787,.F.);
#36597=ORIENTED_EDGE('',*,*,#25267,.F.);
#36598=ORIENTED_EDGE('',*,*,#25259,.F.);
#36599=ORIENTED_EDGE('',*,*,#25256,.F.);
#36600=ORIENTED_EDGE('',*,*,#25368,.F.);
#36601=ORIENTED_EDGE('',*,*,#25376,.F.);
#36602=ORIENTED_EDGE('',*,*,#26788,.T.);
#36603=ORIENTED_EDGE('',*,*,#25365,.F.);
#36604=ORIENTED_EDGE('',*,*,#26788,.F.);
#36605=ORIENTED_EDGE('',*,*,#25372,.F.);
#36606=ORIENTED_EDGE('',*,*,#25264,.F.);
#36607=ORIENTED_EDGE('',*,*,#26787,.T.);
#36608=ORIENTED_EDGE('',*,*,#25250,.F.);
#36609=ORIENTED_EDGE('',*,*,#25357,.F.);
#36610=ORIENTED_EDGE('',*,*,#26789,.F.);
#36611=ORIENTED_EDGE('',*,*,#25252,.F.);
#36612=ORIENTED_EDGE('',*,*,#25244,.F.);
#36613=ORIENTED_EDGE('',*,*,#25241,.F.);
#36614=ORIENTED_EDGE('',*,*,#25354,.F.);
#36615=ORIENTED_EDGE('',*,*,#25362,.F.);
#36616=ORIENTED_EDGE('',*,*,#26790,.T.);
#36617=ORIENTED_EDGE('',*,*,#25351,.F.);
#36618=ORIENTED_EDGE('',*,*,#26790,.F.);
#36619=ORIENTED_EDGE('',*,*,#25358,.F.);
#36620=ORIENTED_EDGE('',*,*,#25249,.F.);
#36621=ORIENTED_EDGE('',*,*,#26789,.T.);
#36622=ORIENTED_EDGE('',*,*,#25238,.F.);
#36623=ORIENTED_EDGE('',*,*,#25342,.F.);
#36624=ORIENTED_EDGE('',*,*,#25331,.F.);
#36625=ORIENTED_EDGE('',*,*,#26791,.F.);
#36626=ORIENTED_EDGE('',*,*,#25343,.F.);
#36627=ORIENTED_EDGE('',*,*,#25237,.F.);
#36628=ORIENTED_EDGE('',*,*,#26792,.T.);
#36629=ORIENTED_EDGE('',*,*,#21328,.F.);
#36630=ORIENTED_EDGE('',*,*,#25339,.F.);
#36631=ORIENTED_EDGE('',*,*,#25347,.F.);
#36632=ORIENTED_EDGE('',*,*,#26791,.T.);
#36633=ORIENTED_EDGE('',*,*,#25336,.F.);
#36634=ORIENTED_EDGE('',*,*,#26792,.F.);
#36635=ORIENTED_EDGE('',*,*,#25349,.F.);
#36636=ORIENTED_EDGE('',*,*,#21329,.F.);
#36637=ORIENTED_EDGE('',*,*,#25229,.F.);
#36638=ORIENTED_EDGE('',*,*,#26793,.F.);
#36639=ORIENTED_EDGE('',*,*,#21533,.F.);
#36640=ORIENTED_EDGE('',*,*,#26793,.T.);
#36641=ORIENTED_EDGE('',*,*,#25225,.F.);
#36642=ORIENTED_EDGE('',*,*,#25326,.F.);
#36643=ORIENTED_EDGE('',*,*,#21534,.F.);
#36644=ORIENTED_EDGE('',*,*,#26794,.F.);
#36645=ORIENTED_EDGE('',*,*,#25227,.F.);
#36646=ORIENTED_EDGE('',*,*,#25219,.F.);
#36647=ORIENTED_EDGE('',*,*,#25216,.F.);
#36648=ORIENTED_EDGE('',*,*,#21537,.F.);
#36649=ORIENTED_EDGE('',*,*,#25329,.F.);
#36650=ORIENTED_EDGE('',*,*,#26795,.T.);
#36651=ORIENTED_EDGE('',*,*,#25324,.F.);
#36652=ORIENTED_EDGE('',*,*,#26795,.F.);
#36653=ORIENTED_EDGE('',*,*,#25327,.F.);
#36654=ORIENTED_EDGE('',*,*,#25224,.F.);
#36655=ORIENTED_EDGE('',*,*,#26794,.T.);
#36656=ORIENTED_EDGE('',*,*,#25211,.F.);
#36657=ORIENTED_EDGE('',*,*,#25317,.F.);
#36658=ORIENTED_EDGE('',*,*,#26796,.F.);
#36659=ORIENTED_EDGE('',*,*,#25213,.F.);
#36660=ORIENTED_EDGE('',*,*,#25205,.F.);
#36661=ORIENTED_EDGE('',*,*,#25202,.F.);
#36662=ORIENTED_EDGE('',*,*,#25314,.F.);
#36663=ORIENTED_EDGE('',*,*,#25322,.F.);
#36664=ORIENTED_EDGE('',*,*,#26797,.T.);
#36665=ORIENTED_EDGE('',*,*,#25311,.F.);
#36666=ORIENTED_EDGE('',*,*,#26797,.F.);
#36667=ORIENTED_EDGE('',*,*,#25318,.F.);
#36668=ORIENTED_EDGE('',*,*,#25210,.F.);
#36669=ORIENTED_EDGE('',*,*,#26796,.T.);
#36670=ORIENTED_EDGE('',*,*,#25197,.F.);
#36671=ORIENTED_EDGE('',*,*,#25303,.F.);
#36672=ORIENTED_EDGE('',*,*,#26798,.F.);
#36673=ORIENTED_EDGE('',*,*,#25199,.F.);
#36674=ORIENTED_EDGE('',*,*,#25191,.F.);
#36675=ORIENTED_EDGE('',*,*,#25188,.F.);
#36676=ORIENTED_EDGE('',*,*,#25300,.F.);
#36677=ORIENTED_EDGE('',*,*,#25308,.F.);
#36678=ORIENTED_EDGE('',*,*,#26799,.T.);
#36679=ORIENTED_EDGE('',*,*,#25297,.F.);
#36680=ORIENTED_EDGE('',*,*,#26799,.F.);
#36681=ORIENTED_EDGE('',*,*,#25304,.F.);
#36682=ORIENTED_EDGE('',*,*,#25196,.F.);
#36683=ORIENTED_EDGE('',*,*,#26798,.T.);
#36684=ORIENTED_EDGE('',*,*,#25183,.F.);
#36685=ORIENTED_EDGE('',*,*,#25289,.F.);
#36686=ORIENTED_EDGE('',*,*,#26800,.F.);
#36687=ORIENTED_EDGE('',*,*,#25185,.F.);
#36688=ORIENTED_EDGE('',*,*,#25177,.F.);
#36689=ORIENTED_EDGE('',*,*,#25174,.F.);
#36690=ORIENTED_EDGE('',*,*,#25286,.F.);
#36691=ORIENTED_EDGE('',*,*,#25294,.F.);
#36692=ORIENTED_EDGE('',*,*,#26801,.T.);
#36693=ORIENTED_EDGE('',*,*,#25283,.F.);
#36694=ORIENTED_EDGE('',*,*,#26801,.F.);
#36695=ORIENTED_EDGE('',*,*,#25290,.F.);
#36696=ORIENTED_EDGE('',*,*,#25182,.F.);
#36697=ORIENTED_EDGE('',*,*,#26800,.T.);
#36698=ORIENTED_EDGE('',*,*,#25169,.F.);
#36699=ORIENTED_EDGE('',*,*,#25275,.F.);
#36700=ORIENTED_EDGE('',*,*,#26802,.F.);
#36701=ORIENTED_EDGE('',*,*,#25171,.F.);
#36702=ORIENTED_EDGE('',*,*,#25163,.F.);
#36703=ORIENTED_EDGE('',*,*,#25160,.F.);
#36704=ORIENTED_EDGE('',*,*,#25272,.F.);
#36705=ORIENTED_EDGE('',*,*,#25280,.F.);
#36706=ORIENTED_EDGE('',*,*,#26803,.T.);
#36707=ORIENTED_EDGE('',*,*,#25269,.F.);
#36708=ORIENTED_EDGE('',*,*,#26803,.F.);
#36709=ORIENTED_EDGE('',*,*,#25276,.F.);
#36710=ORIENTED_EDGE('',*,*,#25168,.F.);
#36711=ORIENTED_EDGE('',*,*,#26802,.T.);
#36712=ORIENTED_EDGE('',*,*,#25154,.F.);
#36713=ORIENTED_EDGE('',*,*,#25261,.F.);
#36714=ORIENTED_EDGE('',*,*,#26804,.F.);
#36715=ORIENTED_EDGE('',*,*,#25156,.F.);
#36716=ORIENTED_EDGE('',*,*,#25148,.F.);
#36717=ORIENTED_EDGE('',*,*,#25145,.F.);
#36718=ORIENTED_EDGE('',*,*,#25258,.F.);
#36719=ORIENTED_EDGE('',*,*,#25266,.F.);
#36720=ORIENTED_EDGE('',*,*,#26805,.T.);
#36721=ORIENTED_EDGE('',*,*,#25255,.F.);
#36722=ORIENTED_EDGE('',*,*,#26805,.F.);
#36723=ORIENTED_EDGE('',*,*,#25262,.F.);
#36724=ORIENTED_EDGE('',*,*,#25153,.F.);
#36725=ORIENTED_EDGE('',*,*,#26804,.T.);
#36726=ORIENTED_EDGE('',*,*,#25142,.F.);
#36727=ORIENTED_EDGE('',*,*,#25246,.F.);
#36728=ORIENTED_EDGE('',*,*,#25235,.F.);
#36729=ORIENTED_EDGE('',*,*,#26806,.F.);
#36730=ORIENTED_EDGE('',*,*,#25247,.F.);
#36731=ORIENTED_EDGE('',*,*,#25141,.F.);
#36732=ORIENTED_EDGE('',*,*,#26807,.T.);
#36733=ORIENTED_EDGE('',*,*,#21332,.F.);
#36734=ORIENTED_EDGE('',*,*,#25243,.F.);
#36735=ORIENTED_EDGE('',*,*,#25251,.F.);
#36736=ORIENTED_EDGE('',*,*,#26806,.T.);
#36737=ORIENTED_EDGE('',*,*,#25240,.F.);
#36738=ORIENTED_EDGE('',*,*,#26807,.F.);
#36739=ORIENTED_EDGE('',*,*,#25253,.F.);
#36740=ORIENTED_EDGE('',*,*,#21333,.F.);
#36741=ORIENTED_EDGE('',*,*,#25133,.F.);
#36742=ORIENTED_EDGE('',*,*,#26808,.F.);
#36743=ORIENTED_EDGE('',*,*,#21527,.F.);
#36744=ORIENTED_EDGE('',*,*,#26808,.T.);
#36745=ORIENTED_EDGE('',*,*,#25129,.F.);
#36746=ORIENTED_EDGE('',*,*,#25230,.F.);
#36747=ORIENTED_EDGE('',*,*,#21528,.F.);
#36748=ORIENTED_EDGE('',*,*,#26809,.F.);
#36749=ORIENTED_EDGE('',*,*,#25131,.F.);
#36750=ORIENTED_EDGE('',*,*,#25123,.F.);
#36751=ORIENTED_EDGE('',*,*,#25120,.F.);
#36752=ORIENTED_EDGE('',*,*,#21531,.F.);
#36753=ORIENTED_EDGE('',*,*,#25233,.F.);
#36754=ORIENTED_EDGE('',*,*,#26810,.T.);
#36755=ORIENTED_EDGE('',*,*,#25228,.F.);
#36756=ORIENTED_EDGE('',*,*,#26810,.F.);
#36757=ORIENTED_EDGE('',*,*,#25231,.F.);
#36758=ORIENTED_EDGE('',*,*,#25128,.F.);
#36759=ORIENTED_EDGE('',*,*,#26809,.T.);
#36760=ORIENTED_EDGE('',*,*,#25115,.F.);
#36761=ORIENTED_EDGE('',*,*,#25221,.F.);
#36762=ORIENTED_EDGE('',*,*,#26811,.F.);
#36763=ORIENTED_EDGE('',*,*,#25117,.F.);
#36764=ORIENTED_EDGE('',*,*,#25109,.F.);
#36765=ORIENTED_EDGE('',*,*,#25106,.F.);
#36766=ORIENTED_EDGE('',*,*,#25218,.F.);
#36767=ORIENTED_EDGE('',*,*,#25226,.F.);
#36768=ORIENTED_EDGE('',*,*,#26812,.T.);
#36769=ORIENTED_EDGE('',*,*,#25215,.F.);
#36770=ORIENTED_EDGE('',*,*,#26812,.F.);
#36771=ORIENTED_EDGE('',*,*,#25222,.F.);
#36772=ORIENTED_EDGE('',*,*,#25114,.F.);
#36773=ORIENTED_EDGE('',*,*,#26811,.T.);
#36774=ORIENTED_EDGE('',*,*,#25101,.F.);
#36775=ORIENTED_EDGE('',*,*,#25207,.F.);
#36776=ORIENTED_EDGE('',*,*,#26813,.F.);
#36777=ORIENTED_EDGE('',*,*,#25103,.F.);
#36778=ORIENTED_EDGE('',*,*,#25095,.F.);
#36779=ORIENTED_EDGE('',*,*,#25092,.F.);
#36780=ORIENTED_EDGE('',*,*,#25204,.F.);
#36781=ORIENTED_EDGE('',*,*,#25212,.F.);
#36782=ORIENTED_EDGE('',*,*,#26814,.T.);
#36783=ORIENTED_EDGE('',*,*,#25201,.F.);
#36784=ORIENTED_EDGE('',*,*,#26814,.F.);
#36785=ORIENTED_EDGE('',*,*,#25208,.F.);
#36786=ORIENTED_EDGE('',*,*,#25100,.F.);
#36787=ORIENTED_EDGE('',*,*,#26813,.T.);
#36788=ORIENTED_EDGE('',*,*,#25087,.F.);
#36789=ORIENTED_EDGE('',*,*,#25193,.F.);
#36790=ORIENTED_EDGE('',*,*,#26815,.F.);
#36791=ORIENTED_EDGE('',*,*,#25089,.F.);
#36792=ORIENTED_EDGE('',*,*,#25081,.F.);
#36793=ORIENTED_EDGE('',*,*,#25078,.F.);
#36794=ORIENTED_EDGE('',*,*,#25190,.F.);
#36795=ORIENTED_EDGE('',*,*,#25198,.F.);
#36796=ORIENTED_EDGE('',*,*,#26816,.T.);
#36797=ORIENTED_EDGE('',*,*,#25187,.F.);
#36798=ORIENTED_EDGE('',*,*,#26816,.F.);
#36799=ORIENTED_EDGE('',*,*,#25194,.F.);
#36800=ORIENTED_EDGE('',*,*,#25086,.F.);
#36801=ORIENTED_EDGE('',*,*,#26815,.T.);
#36802=ORIENTED_EDGE('',*,*,#25073,.F.);
#36803=ORIENTED_EDGE('',*,*,#25179,.F.);
#36804=ORIENTED_EDGE('',*,*,#26817,.F.);
#36805=ORIENTED_EDGE('',*,*,#25075,.F.);
#36806=ORIENTED_EDGE('',*,*,#25067,.F.);
#36807=ORIENTED_EDGE('',*,*,#25064,.F.);
#36808=ORIENTED_EDGE('',*,*,#25176,.F.);
#36809=ORIENTED_EDGE('',*,*,#25184,.F.);
#36810=ORIENTED_EDGE('',*,*,#26818,.T.);
#36811=ORIENTED_EDGE('',*,*,#25173,.F.);
#36812=ORIENTED_EDGE('',*,*,#26818,.F.);
#36813=ORIENTED_EDGE('',*,*,#25180,.F.);
#36814=ORIENTED_EDGE('',*,*,#25072,.F.);
#36815=ORIENTED_EDGE('',*,*,#26817,.T.);
#36816=ORIENTED_EDGE('',*,*,#25058,.F.);
#36817=ORIENTED_EDGE('',*,*,#25165,.F.);
#36818=ORIENTED_EDGE('',*,*,#26819,.F.);
#36819=ORIENTED_EDGE('',*,*,#25060,.F.);
#36820=ORIENTED_EDGE('',*,*,#25052,.F.);
#36821=ORIENTED_EDGE('',*,*,#25049,.F.);
#36822=ORIENTED_EDGE('',*,*,#25162,.F.);
#36823=ORIENTED_EDGE('',*,*,#25170,.F.);
#36824=ORIENTED_EDGE('',*,*,#26820,.T.);
#36825=ORIENTED_EDGE('',*,*,#25159,.F.);
#36826=ORIENTED_EDGE('',*,*,#26820,.F.);
#36827=ORIENTED_EDGE('',*,*,#25166,.F.);
#36828=ORIENTED_EDGE('',*,*,#25057,.F.);
#36829=ORIENTED_EDGE('',*,*,#26819,.T.);
#36830=ORIENTED_EDGE('',*,*,#25046,.F.);
#36831=ORIENTED_EDGE('',*,*,#25150,.F.);
#36832=ORIENTED_EDGE('',*,*,#25139,.F.);
#36833=ORIENTED_EDGE('',*,*,#26821,.F.);
#36834=ORIENTED_EDGE('',*,*,#25151,.F.);
#36835=ORIENTED_EDGE('',*,*,#25045,.F.);
#36836=ORIENTED_EDGE('',*,*,#26822,.T.);
#36837=ORIENTED_EDGE('',*,*,#21336,.F.);
#36838=ORIENTED_EDGE('',*,*,#25147,.F.);
#36839=ORIENTED_EDGE('',*,*,#25155,.F.);
#36840=ORIENTED_EDGE('',*,*,#26821,.T.);
#36841=ORIENTED_EDGE('',*,*,#25144,.F.);
#36842=ORIENTED_EDGE('',*,*,#26822,.F.);
#36843=ORIENTED_EDGE('',*,*,#25157,.F.);
#36844=ORIENTED_EDGE('',*,*,#21337,.F.);
#36845=ORIENTED_EDGE('',*,*,#25037,.F.);
#36846=ORIENTED_EDGE('',*,*,#26823,.F.);
#36847=ORIENTED_EDGE('',*,*,#21521,.F.);
#36848=ORIENTED_EDGE('',*,*,#26823,.T.);
#36849=ORIENTED_EDGE('',*,*,#25033,.F.);
#36850=ORIENTED_EDGE('',*,*,#25134,.F.);
#36851=ORIENTED_EDGE('',*,*,#21522,.F.);
#36852=ORIENTED_EDGE('',*,*,#26824,.F.);
#36853=ORIENTED_EDGE('',*,*,#25035,.F.);
#36854=ORIENTED_EDGE('',*,*,#25027,.F.);
#36855=ORIENTED_EDGE('',*,*,#25024,.F.);
#36856=ORIENTED_EDGE('',*,*,#21525,.F.);
#36857=ORIENTED_EDGE('',*,*,#25137,.F.);
#36858=ORIENTED_EDGE('',*,*,#26825,.T.);
#36859=ORIENTED_EDGE('',*,*,#25132,.F.);
#36860=ORIENTED_EDGE('',*,*,#26825,.F.);
#36861=ORIENTED_EDGE('',*,*,#25135,.F.);
#36862=ORIENTED_EDGE('',*,*,#25032,.F.);
#36863=ORIENTED_EDGE('',*,*,#26824,.T.);
#36864=ORIENTED_EDGE('',*,*,#25019,.F.);
#36865=ORIENTED_EDGE('',*,*,#25125,.F.);
#36866=ORIENTED_EDGE('',*,*,#26826,.F.);
#36867=ORIENTED_EDGE('',*,*,#25021,.F.);
#36868=ORIENTED_EDGE('',*,*,#25013,.F.);
#36869=ORIENTED_EDGE('',*,*,#25010,.F.);
#36870=ORIENTED_EDGE('',*,*,#25122,.F.);
#36871=ORIENTED_EDGE('',*,*,#25130,.F.);
#36872=ORIENTED_EDGE('',*,*,#26827,.T.);
#36873=ORIENTED_EDGE('',*,*,#25119,.F.);
#36874=ORIENTED_EDGE('',*,*,#26827,.F.);
#36875=ORIENTED_EDGE('',*,*,#25126,.F.);
#36876=ORIENTED_EDGE('',*,*,#25018,.F.);
#36877=ORIENTED_EDGE('',*,*,#26826,.T.);
#36878=ORIENTED_EDGE('',*,*,#25005,.F.);
#36879=ORIENTED_EDGE('',*,*,#25111,.F.);
#36880=ORIENTED_EDGE('',*,*,#26828,.F.);
#36881=ORIENTED_EDGE('',*,*,#25007,.F.);
#36882=ORIENTED_EDGE('',*,*,#24999,.F.);
#36883=ORIENTED_EDGE('',*,*,#24996,.F.);
#36884=ORIENTED_EDGE('',*,*,#25108,.F.);
#36885=ORIENTED_EDGE('',*,*,#25116,.F.);
#36886=ORIENTED_EDGE('',*,*,#26829,.T.);
#36887=ORIENTED_EDGE('',*,*,#25105,.F.);
#36888=ORIENTED_EDGE('',*,*,#26829,.F.);
#36889=ORIENTED_EDGE('',*,*,#25112,.F.);
#36890=ORIENTED_EDGE('',*,*,#25004,.F.);
#36891=ORIENTED_EDGE('',*,*,#26828,.T.);
#36892=ORIENTED_EDGE('',*,*,#24991,.F.);
#36893=ORIENTED_EDGE('',*,*,#25097,.F.);
#36894=ORIENTED_EDGE('',*,*,#26830,.F.);
#36895=ORIENTED_EDGE('',*,*,#24993,.F.);
#36896=ORIENTED_EDGE('',*,*,#24985,.F.);
#36897=ORIENTED_EDGE('',*,*,#24982,.F.);
#36898=ORIENTED_EDGE('',*,*,#25094,.F.);
#36899=ORIENTED_EDGE('',*,*,#25102,.F.);
#36900=ORIENTED_EDGE('',*,*,#26831,.T.);
#36901=ORIENTED_EDGE('',*,*,#25091,.F.);
#36902=ORIENTED_EDGE('',*,*,#26831,.F.);
#36903=ORIENTED_EDGE('',*,*,#25098,.F.);
#36904=ORIENTED_EDGE('',*,*,#24990,.F.);
#36905=ORIENTED_EDGE('',*,*,#26830,.T.);
#36906=ORIENTED_EDGE('',*,*,#24977,.F.);
#36907=ORIENTED_EDGE('',*,*,#25083,.F.);
#36908=ORIENTED_EDGE('',*,*,#26832,.F.);
#36909=ORIENTED_EDGE('',*,*,#24979,.F.);
#36910=ORIENTED_EDGE('',*,*,#24971,.F.);
#36911=ORIENTED_EDGE('',*,*,#24968,.F.);
#36912=ORIENTED_EDGE('',*,*,#25080,.F.);
#36913=ORIENTED_EDGE('',*,*,#25088,.F.);
#36914=ORIENTED_EDGE('',*,*,#26833,.T.);
#36915=ORIENTED_EDGE('',*,*,#25077,.F.);
#36916=ORIENTED_EDGE('',*,*,#26833,.F.);
#36917=ORIENTED_EDGE('',*,*,#25084,.F.);
#36918=ORIENTED_EDGE('',*,*,#24976,.F.);
#36919=ORIENTED_EDGE('',*,*,#26832,.T.);
#36920=ORIENTED_EDGE('',*,*,#24962,.F.);
#36921=ORIENTED_EDGE('',*,*,#25069,.F.);
#36922=ORIENTED_EDGE('',*,*,#26834,.F.);
#36923=ORIENTED_EDGE('',*,*,#24964,.F.);
#36924=ORIENTED_EDGE('',*,*,#24956,.F.);
#36925=ORIENTED_EDGE('',*,*,#24953,.F.);
#36926=ORIENTED_EDGE('',*,*,#25066,.F.);
#36927=ORIENTED_EDGE('',*,*,#25074,.F.);
#36928=ORIENTED_EDGE('',*,*,#26835,.T.);
#36929=ORIENTED_EDGE('',*,*,#25063,.F.);
#36930=ORIENTED_EDGE('',*,*,#26835,.F.);
#36931=ORIENTED_EDGE('',*,*,#25070,.F.);
#36932=ORIENTED_EDGE('',*,*,#24961,.F.);
#36933=ORIENTED_EDGE('',*,*,#26834,.T.);
#36934=ORIENTED_EDGE('',*,*,#24950,.F.);
#36935=ORIENTED_EDGE('',*,*,#25054,.F.);
#36936=ORIENTED_EDGE('',*,*,#25043,.F.);
#36937=ORIENTED_EDGE('',*,*,#26836,.F.);
#36938=ORIENTED_EDGE('',*,*,#25055,.F.);
#36939=ORIENTED_EDGE('',*,*,#24949,.F.);
#36940=ORIENTED_EDGE('',*,*,#26837,.T.);
#36941=ORIENTED_EDGE('',*,*,#21340,.F.);
#36942=ORIENTED_EDGE('',*,*,#25051,.F.);
#36943=ORIENTED_EDGE('',*,*,#25059,.F.);
#36944=ORIENTED_EDGE('',*,*,#26836,.T.);
#36945=ORIENTED_EDGE('',*,*,#25048,.F.);
#36946=ORIENTED_EDGE('',*,*,#26837,.F.);
#36947=ORIENTED_EDGE('',*,*,#25061,.F.);
#36948=ORIENTED_EDGE('',*,*,#21341,.F.);
#36949=ORIENTED_EDGE('',*,*,#24941,.F.);
#36950=ORIENTED_EDGE('',*,*,#26838,.F.);
#36951=ORIENTED_EDGE('',*,*,#21515,.F.);
#36952=ORIENTED_EDGE('',*,*,#26838,.T.);
#36953=ORIENTED_EDGE('',*,*,#24937,.F.);
#36954=ORIENTED_EDGE('',*,*,#25038,.F.);
#36955=ORIENTED_EDGE('',*,*,#21516,.F.);
#36956=ORIENTED_EDGE('',*,*,#26839,.F.);
#36957=ORIENTED_EDGE('',*,*,#24939,.F.);
#36958=ORIENTED_EDGE('',*,*,#24931,.F.);
#36959=ORIENTED_EDGE('',*,*,#24928,.F.);
#36960=ORIENTED_EDGE('',*,*,#21519,.F.);
#36961=ORIENTED_EDGE('',*,*,#25041,.F.);
#36962=ORIENTED_EDGE('',*,*,#26840,.T.);
#36963=ORIENTED_EDGE('',*,*,#25036,.F.);
#36964=ORIENTED_EDGE('',*,*,#26840,.F.);
#36965=ORIENTED_EDGE('',*,*,#25039,.F.);
#36966=ORIENTED_EDGE('',*,*,#24936,.F.);
#36967=ORIENTED_EDGE('',*,*,#26839,.T.);
#36968=ORIENTED_EDGE('',*,*,#24923,.F.);
#36969=ORIENTED_EDGE('',*,*,#25029,.F.);
#36970=ORIENTED_EDGE('',*,*,#26841,.F.);
#36971=ORIENTED_EDGE('',*,*,#24925,.F.);
#36972=ORIENTED_EDGE('',*,*,#24917,.F.);
#36973=ORIENTED_EDGE('',*,*,#24914,.F.);
#36974=ORIENTED_EDGE('',*,*,#25026,.F.);
#36975=ORIENTED_EDGE('',*,*,#25034,.F.);
#36976=ORIENTED_EDGE('',*,*,#26842,.T.);
#36977=ORIENTED_EDGE('',*,*,#25023,.F.);
#36978=ORIENTED_EDGE('',*,*,#26842,.F.);
#36979=ORIENTED_EDGE('',*,*,#25030,.F.);
#36980=ORIENTED_EDGE('',*,*,#24922,.F.);
#36981=ORIENTED_EDGE('',*,*,#26841,.T.);
#36982=ORIENTED_EDGE('',*,*,#24909,.F.);
#36983=ORIENTED_EDGE('',*,*,#25015,.F.);
#36984=ORIENTED_EDGE('',*,*,#26843,.F.);
#36985=ORIENTED_EDGE('',*,*,#24911,.F.);
#36986=ORIENTED_EDGE('',*,*,#24903,.F.);
#36987=ORIENTED_EDGE('',*,*,#24900,.F.);
#36988=ORIENTED_EDGE('',*,*,#25012,.F.);
#36989=ORIENTED_EDGE('',*,*,#25020,.F.);
#36990=ORIENTED_EDGE('',*,*,#26844,.T.);
#36991=ORIENTED_EDGE('',*,*,#25009,.F.);
#36992=ORIENTED_EDGE('',*,*,#26844,.F.);
#36993=ORIENTED_EDGE('',*,*,#25016,.F.);
#36994=ORIENTED_EDGE('',*,*,#24908,.F.);
#36995=ORIENTED_EDGE('',*,*,#26843,.T.);
#36996=ORIENTED_EDGE('',*,*,#24895,.F.);
#36997=ORIENTED_EDGE('',*,*,#25001,.F.);
#36998=ORIENTED_EDGE('',*,*,#26845,.F.);
#36999=ORIENTED_EDGE('',*,*,#24897,.F.);
#37000=ORIENTED_EDGE('',*,*,#24889,.F.);
#37001=ORIENTED_EDGE('',*,*,#24886,.F.);
#37002=ORIENTED_EDGE('',*,*,#24998,.F.);
#37003=ORIENTED_EDGE('',*,*,#25006,.F.);
#37004=ORIENTED_EDGE('',*,*,#26846,.T.);
#37005=ORIENTED_EDGE('',*,*,#24995,.F.);
#37006=ORIENTED_EDGE('',*,*,#26846,.F.);
#37007=ORIENTED_EDGE('',*,*,#25002,.F.);
#37008=ORIENTED_EDGE('',*,*,#24894,.F.);
#37009=ORIENTED_EDGE('',*,*,#26845,.T.);
#37010=ORIENTED_EDGE('',*,*,#24881,.F.);
#37011=ORIENTED_EDGE('',*,*,#24987,.F.);
#37012=ORIENTED_EDGE('',*,*,#26847,.F.);
#37013=ORIENTED_EDGE('',*,*,#24883,.F.);
#37014=ORIENTED_EDGE('',*,*,#24875,.F.);
#37015=ORIENTED_EDGE('',*,*,#24872,.F.);
#37016=ORIENTED_EDGE('',*,*,#24984,.F.);
#37017=ORIENTED_EDGE('',*,*,#24992,.F.);
#37018=ORIENTED_EDGE('',*,*,#26848,.T.);
#37019=ORIENTED_EDGE('',*,*,#24981,.F.);
#37020=ORIENTED_EDGE('',*,*,#26848,.F.);
#37021=ORIENTED_EDGE('',*,*,#24988,.F.);
#37022=ORIENTED_EDGE('',*,*,#24880,.F.);
#37023=ORIENTED_EDGE('',*,*,#26847,.T.);
#37024=ORIENTED_EDGE('',*,*,#24866,.F.);
#37025=ORIENTED_EDGE('',*,*,#24973,.F.);
#37026=ORIENTED_EDGE('',*,*,#26849,.F.);
#37027=ORIENTED_EDGE('',*,*,#24868,.F.);
#37028=ORIENTED_EDGE('',*,*,#24860,.F.);
#37029=ORIENTED_EDGE('',*,*,#24857,.F.);
#37030=ORIENTED_EDGE('',*,*,#24970,.F.);
#37031=ORIENTED_EDGE('',*,*,#24978,.F.);
#37032=ORIENTED_EDGE('',*,*,#26850,.T.);
#37033=ORIENTED_EDGE('',*,*,#24967,.F.);
#37034=ORIENTED_EDGE('',*,*,#26850,.F.);
#37035=ORIENTED_EDGE('',*,*,#24974,.F.);
#37036=ORIENTED_EDGE('',*,*,#24865,.F.);
#37037=ORIENTED_EDGE('',*,*,#26849,.T.);
#37038=ORIENTED_EDGE('',*,*,#24854,.F.);
#37039=ORIENTED_EDGE('',*,*,#24958,.F.);
#37040=ORIENTED_EDGE('',*,*,#24947,.F.);
#37041=ORIENTED_EDGE('',*,*,#26851,.F.);
#37042=ORIENTED_EDGE('',*,*,#24959,.F.);
#37043=ORIENTED_EDGE('',*,*,#24853,.F.);
#37044=ORIENTED_EDGE('',*,*,#26852,.T.);
#37045=ORIENTED_EDGE('',*,*,#21344,.F.);
#37046=ORIENTED_EDGE('',*,*,#24955,.F.);
#37047=ORIENTED_EDGE('',*,*,#24963,.F.);
#37048=ORIENTED_EDGE('',*,*,#26851,.T.);
#37049=ORIENTED_EDGE('',*,*,#24952,.F.);
#37050=ORIENTED_EDGE('',*,*,#26852,.F.);
#37051=ORIENTED_EDGE('',*,*,#24965,.F.);
#37052=ORIENTED_EDGE('',*,*,#21345,.F.);
#37053=ORIENTED_EDGE('',*,*,#24845,.F.);
#37054=ORIENTED_EDGE('',*,*,#26853,.F.);
#37055=ORIENTED_EDGE('',*,*,#21509,.F.);
#37056=ORIENTED_EDGE('',*,*,#26853,.T.);
#37057=ORIENTED_EDGE('',*,*,#24841,.F.);
#37058=ORIENTED_EDGE('',*,*,#24942,.F.);
#37059=ORIENTED_EDGE('',*,*,#21510,.F.);
#37060=ORIENTED_EDGE('',*,*,#26854,.F.);
#37061=ORIENTED_EDGE('',*,*,#24843,.F.);
#37062=ORIENTED_EDGE('',*,*,#24835,.F.);
#37063=ORIENTED_EDGE('',*,*,#24832,.F.);
#37064=ORIENTED_EDGE('',*,*,#21513,.F.);
#37065=ORIENTED_EDGE('',*,*,#24945,.F.);
#37066=ORIENTED_EDGE('',*,*,#26855,.T.);
#37067=ORIENTED_EDGE('',*,*,#24940,.F.);
#37068=ORIENTED_EDGE('',*,*,#26855,.F.);
#37069=ORIENTED_EDGE('',*,*,#24943,.F.);
#37070=ORIENTED_EDGE('',*,*,#24840,.F.);
#37071=ORIENTED_EDGE('',*,*,#26854,.T.);
#37072=ORIENTED_EDGE('',*,*,#24827,.F.);
#37073=ORIENTED_EDGE('',*,*,#24933,.F.);
#37074=ORIENTED_EDGE('',*,*,#26856,.F.);
#37075=ORIENTED_EDGE('',*,*,#24829,.F.);
#37076=ORIENTED_EDGE('',*,*,#24821,.F.);
#37077=ORIENTED_EDGE('',*,*,#24818,.F.);
#37078=ORIENTED_EDGE('',*,*,#24930,.F.);
#37079=ORIENTED_EDGE('',*,*,#24938,.F.);
#37080=ORIENTED_EDGE('',*,*,#26857,.T.);
#37081=ORIENTED_EDGE('',*,*,#24927,.F.);
#37082=ORIENTED_EDGE('',*,*,#26857,.F.);
#37083=ORIENTED_EDGE('',*,*,#24934,.F.);
#37084=ORIENTED_EDGE('',*,*,#24826,.F.);
#37085=ORIENTED_EDGE('',*,*,#26856,.T.);
#37086=ORIENTED_EDGE('',*,*,#24813,.F.);
#37087=ORIENTED_EDGE('',*,*,#24919,.F.);
#37088=ORIENTED_EDGE('',*,*,#26858,.F.);
#37089=ORIENTED_EDGE('',*,*,#24815,.F.);
#37090=ORIENTED_EDGE('',*,*,#24807,.F.);
#37091=ORIENTED_EDGE('',*,*,#24804,.F.);
#37092=ORIENTED_EDGE('',*,*,#24916,.F.);
#37093=ORIENTED_EDGE('',*,*,#24924,.F.);
#37094=ORIENTED_EDGE('',*,*,#26859,.T.);
#37095=ORIENTED_EDGE('',*,*,#24913,.F.);
#37096=ORIENTED_EDGE('',*,*,#26859,.F.);
#37097=ORIENTED_EDGE('',*,*,#24920,.F.);
#37098=ORIENTED_EDGE('',*,*,#24812,.F.);
#37099=ORIENTED_EDGE('',*,*,#26858,.T.);
#37100=ORIENTED_EDGE('',*,*,#24799,.F.);
#37101=ORIENTED_EDGE('',*,*,#24905,.F.);
#37102=ORIENTED_EDGE('',*,*,#26860,.F.);
#37103=ORIENTED_EDGE('',*,*,#24801,.F.);
#37104=ORIENTED_EDGE('',*,*,#24793,.F.);
#37105=ORIENTED_EDGE('',*,*,#24790,.F.);
#37106=ORIENTED_EDGE('',*,*,#24902,.F.);
#37107=ORIENTED_EDGE('',*,*,#24910,.F.);
#37108=ORIENTED_EDGE('',*,*,#26861,.T.);
#37109=ORIENTED_EDGE('',*,*,#24899,.F.);
#37110=ORIENTED_EDGE('',*,*,#26861,.F.);
#37111=ORIENTED_EDGE('',*,*,#24906,.F.);
#37112=ORIENTED_EDGE('',*,*,#24798,.F.);
#37113=ORIENTED_EDGE('',*,*,#26860,.T.);
#37114=ORIENTED_EDGE('',*,*,#24785,.F.);
#37115=ORIENTED_EDGE('',*,*,#24891,.F.);
#37116=ORIENTED_EDGE('',*,*,#26862,.F.);
#37117=ORIENTED_EDGE('',*,*,#24787,.F.);
#37118=ORIENTED_EDGE('',*,*,#24779,.F.);
#37119=ORIENTED_EDGE('',*,*,#24776,.F.);
#37120=ORIENTED_EDGE('',*,*,#24888,.F.);
#37121=ORIENTED_EDGE('',*,*,#24896,.F.);
#37122=ORIENTED_EDGE('',*,*,#26863,.T.);
#37123=ORIENTED_EDGE('',*,*,#24885,.F.);
#37124=ORIENTED_EDGE('',*,*,#26863,.F.);
#37125=ORIENTED_EDGE('',*,*,#24892,.F.);
#37126=ORIENTED_EDGE('',*,*,#24784,.F.);
#37127=ORIENTED_EDGE('',*,*,#26862,.T.);
#37128=ORIENTED_EDGE('',*,*,#24770,.F.);
#37129=ORIENTED_EDGE('',*,*,#24877,.F.);
#37130=ORIENTED_EDGE('',*,*,#26864,.F.);
#37131=ORIENTED_EDGE('',*,*,#24772,.F.);
#37132=ORIENTED_EDGE('',*,*,#24764,.F.);
#37133=ORIENTED_EDGE('',*,*,#24761,.F.);
#37134=ORIENTED_EDGE('',*,*,#24874,.F.);
#37135=ORIENTED_EDGE('',*,*,#24882,.F.);
#37136=ORIENTED_EDGE('',*,*,#26865,.T.);
#37137=ORIENTED_EDGE('',*,*,#24871,.F.);
#37138=ORIENTED_EDGE('',*,*,#26865,.F.);
#37139=ORIENTED_EDGE('',*,*,#24878,.F.);
#37140=ORIENTED_EDGE('',*,*,#24769,.F.);
#37141=ORIENTED_EDGE('',*,*,#26864,.T.);
#37142=ORIENTED_EDGE('',*,*,#24758,.F.);
#37143=ORIENTED_EDGE('',*,*,#24862,.F.);
#37144=ORIENTED_EDGE('',*,*,#24851,.F.);
#37145=ORIENTED_EDGE('',*,*,#26866,.F.);
#37146=ORIENTED_EDGE('',*,*,#24863,.F.);
#37147=ORIENTED_EDGE('',*,*,#24757,.F.);
#37148=ORIENTED_EDGE('',*,*,#26867,.T.);
#37149=ORIENTED_EDGE('',*,*,#21348,.F.);
#37150=ORIENTED_EDGE('',*,*,#24859,.F.);
#37151=ORIENTED_EDGE('',*,*,#24867,.F.);
#37152=ORIENTED_EDGE('',*,*,#26866,.T.);
#37153=ORIENTED_EDGE('',*,*,#24856,.F.);
#37154=ORIENTED_EDGE('',*,*,#26867,.F.);
#37155=ORIENTED_EDGE('',*,*,#24869,.F.);
#37156=ORIENTED_EDGE('',*,*,#21349,.F.);
#37157=ORIENTED_EDGE('',*,*,#24749,.F.);
#37158=ORIENTED_EDGE('',*,*,#26868,.F.);
#37159=ORIENTED_EDGE('',*,*,#21503,.F.);
#37160=ORIENTED_EDGE('',*,*,#26868,.T.);
#37161=ORIENTED_EDGE('',*,*,#24745,.F.);
#37162=ORIENTED_EDGE('',*,*,#24846,.F.);
#37163=ORIENTED_EDGE('',*,*,#21504,.F.);
#37164=ORIENTED_EDGE('',*,*,#26869,.F.);
#37165=ORIENTED_EDGE('',*,*,#24747,.F.);
#37166=ORIENTED_EDGE('',*,*,#24739,.F.);
#37167=ORIENTED_EDGE('',*,*,#24736,.F.);
#37168=ORIENTED_EDGE('',*,*,#21507,.F.);
#37169=ORIENTED_EDGE('',*,*,#24849,.F.);
#37170=ORIENTED_EDGE('',*,*,#26870,.T.);
#37171=ORIENTED_EDGE('',*,*,#24844,.F.);
#37172=ORIENTED_EDGE('',*,*,#26870,.F.);
#37173=ORIENTED_EDGE('',*,*,#24847,.F.);
#37174=ORIENTED_EDGE('',*,*,#24744,.F.);
#37175=ORIENTED_EDGE('',*,*,#26869,.T.);
#37176=ORIENTED_EDGE('',*,*,#24731,.F.);
#37177=ORIENTED_EDGE('',*,*,#24837,.F.);
#37178=ORIENTED_EDGE('',*,*,#26871,.F.);
#37179=ORIENTED_EDGE('',*,*,#24733,.F.);
#37180=ORIENTED_EDGE('',*,*,#24725,.F.);
#37181=ORIENTED_EDGE('',*,*,#24722,.F.);
#37182=ORIENTED_EDGE('',*,*,#24834,.F.);
#37183=ORIENTED_EDGE('',*,*,#24842,.F.);
#37184=ORIENTED_EDGE('',*,*,#26872,.T.);
#37185=ORIENTED_EDGE('',*,*,#24831,.F.);
#37186=ORIENTED_EDGE('',*,*,#26872,.F.);
#37187=ORIENTED_EDGE('',*,*,#24838,.F.);
#37188=ORIENTED_EDGE('',*,*,#24730,.F.);
#37189=ORIENTED_EDGE('',*,*,#26871,.T.);
#37190=ORIENTED_EDGE('',*,*,#24717,.F.);
#37191=ORIENTED_EDGE('',*,*,#24823,.F.);
#37192=ORIENTED_EDGE('',*,*,#26873,.F.);
#37193=ORIENTED_EDGE('',*,*,#24719,.F.);
#37194=ORIENTED_EDGE('',*,*,#24711,.F.);
#37195=ORIENTED_EDGE('',*,*,#24708,.F.);
#37196=ORIENTED_EDGE('',*,*,#24820,.F.);
#37197=ORIENTED_EDGE('',*,*,#24828,.F.);
#37198=ORIENTED_EDGE('',*,*,#26874,.T.);
#37199=ORIENTED_EDGE('',*,*,#24817,.F.);
#37200=ORIENTED_EDGE('',*,*,#26874,.F.);
#37201=ORIENTED_EDGE('',*,*,#24824,.F.);
#37202=ORIENTED_EDGE('',*,*,#24716,.F.);
#37203=ORIENTED_EDGE('',*,*,#26873,.T.);
#37204=ORIENTED_EDGE('',*,*,#24703,.F.);
#37205=ORIENTED_EDGE('',*,*,#24809,.F.);
#37206=ORIENTED_EDGE('',*,*,#26875,.F.);
#37207=ORIENTED_EDGE('',*,*,#24705,.F.);
#37208=ORIENTED_EDGE('',*,*,#24697,.F.);
#37209=ORIENTED_EDGE('',*,*,#24694,.F.);
#37210=ORIENTED_EDGE('',*,*,#24806,.F.);
#37211=ORIENTED_EDGE('',*,*,#24814,.F.);
#37212=ORIENTED_EDGE('',*,*,#26876,.T.);
#37213=ORIENTED_EDGE('',*,*,#24803,.F.);
#37214=ORIENTED_EDGE('',*,*,#26876,.F.);
#37215=ORIENTED_EDGE('',*,*,#24810,.F.);
#37216=ORIENTED_EDGE('',*,*,#24702,.F.);
#37217=ORIENTED_EDGE('',*,*,#26875,.T.);
#37218=ORIENTED_EDGE('',*,*,#24689,.F.);
#37219=ORIENTED_EDGE('',*,*,#24795,.F.);
#37220=ORIENTED_EDGE('',*,*,#26877,.F.);
#37221=ORIENTED_EDGE('',*,*,#24691,.F.);
#37222=ORIENTED_EDGE('',*,*,#24683,.F.);
#37223=ORIENTED_EDGE('',*,*,#24680,.F.);
#37224=ORIENTED_EDGE('',*,*,#24792,.F.);
#37225=ORIENTED_EDGE('',*,*,#24800,.F.);
#37226=ORIENTED_EDGE('',*,*,#26878,.T.);
#37227=ORIENTED_EDGE('',*,*,#24789,.F.);
#37228=ORIENTED_EDGE('',*,*,#26878,.F.);
#37229=ORIENTED_EDGE('',*,*,#24796,.F.);
#37230=ORIENTED_EDGE('',*,*,#24688,.F.);
#37231=ORIENTED_EDGE('',*,*,#26877,.T.);
#37232=ORIENTED_EDGE('',*,*,#24674,.F.);
#37233=ORIENTED_EDGE('',*,*,#24781,.F.);
#37234=ORIENTED_EDGE('',*,*,#26879,.F.);
#37235=ORIENTED_EDGE('',*,*,#24676,.F.);
#37236=ORIENTED_EDGE('',*,*,#24668,.F.);
#37237=ORIENTED_EDGE('',*,*,#24665,.F.);
#37238=ORIENTED_EDGE('',*,*,#24778,.F.);
#37239=ORIENTED_EDGE('',*,*,#24786,.F.);
#37240=ORIENTED_EDGE('',*,*,#26880,.T.);
#37241=ORIENTED_EDGE('',*,*,#24775,.F.);
#37242=ORIENTED_EDGE('',*,*,#26880,.F.);
#37243=ORIENTED_EDGE('',*,*,#24782,.F.);
#37244=ORIENTED_EDGE('',*,*,#24673,.F.);
#37245=ORIENTED_EDGE('',*,*,#26879,.T.);
#37246=ORIENTED_EDGE('',*,*,#24662,.F.);
#37247=ORIENTED_EDGE('',*,*,#24766,.F.);
#37248=ORIENTED_EDGE('',*,*,#24755,.F.);
#37249=ORIENTED_EDGE('',*,*,#26881,.F.);
#37250=ORIENTED_EDGE('',*,*,#24767,.F.);
#37251=ORIENTED_EDGE('',*,*,#24661,.F.);
#37252=ORIENTED_EDGE('',*,*,#26882,.T.);
#37253=ORIENTED_EDGE('',*,*,#21352,.F.);
#37254=ORIENTED_EDGE('',*,*,#24763,.F.);
#37255=ORIENTED_EDGE('',*,*,#24771,.F.);
#37256=ORIENTED_EDGE('',*,*,#26881,.T.);
#37257=ORIENTED_EDGE('',*,*,#24760,.F.);
#37258=ORIENTED_EDGE('',*,*,#26882,.F.);
#37259=ORIENTED_EDGE('',*,*,#24773,.F.);
#37260=ORIENTED_EDGE('',*,*,#21353,.F.);
#37261=ORIENTED_EDGE('',*,*,#24653,.F.);
#37262=ORIENTED_EDGE('',*,*,#26883,.F.);
#37263=ORIENTED_EDGE('',*,*,#21497,.F.);
#37264=ORIENTED_EDGE('',*,*,#26883,.T.);
#37265=ORIENTED_EDGE('',*,*,#24649,.F.);
#37266=ORIENTED_EDGE('',*,*,#24750,.F.);
#37267=ORIENTED_EDGE('',*,*,#21498,.F.);
#37268=ORIENTED_EDGE('',*,*,#26884,.F.);
#37269=ORIENTED_EDGE('',*,*,#24651,.F.);
#37270=ORIENTED_EDGE('',*,*,#24643,.F.);
#37271=ORIENTED_EDGE('',*,*,#24640,.F.);
#37272=ORIENTED_EDGE('',*,*,#21501,.F.);
#37273=ORIENTED_EDGE('',*,*,#24753,.F.);
#37274=ORIENTED_EDGE('',*,*,#26885,.T.);
#37275=ORIENTED_EDGE('',*,*,#24748,.F.);
#37276=ORIENTED_EDGE('',*,*,#26885,.F.);
#37277=ORIENTED_EDGE('',*,*,#24751,.F.);
#37278=ORIENTED_EDGE('',*,*,#24648,.F.);
#37279=ORIENTED_EDGE('',*,*,#26884,.T.);
#37280=ORIENTED_EDGE('',*,*,#24635,.F.);
#37281=ORIENTED_EDGE('',*,*,#24741,.F.);
#37282=ORIENTED_EDGE('',*,*,#26886,.F.);
#37283=ORIENTED_EDGE('',*,*,#24637,.F.);
#37284=ORIENTED_EDGE('',*,*,#24629,.F.);
#37285=ORIENTED_EDGE('',*,*,#24626,.F.);
#37286=ORIENTED_EDGE('',*,*,#24738,.F.);
#37287=ORIENTED_EDGE('',*,*,#24746,.F.);
#37288=ORIENTED_EDGE('',*,*,#26887,.T.);
#37289=ORIENTED_EDGE('',*,*,#24735,.F.);
#37290=ORIENTED_EDGE('',*,*,#26887,.F.);
#37291=ORIENTED_EDGE('',*,*,#24742,.F.);
#37292=ORIENTED_EDGE('',*,*,#24634,.F.);
#37293=ORIENTED_EDGE('',*,*,#26886,.T.);
#37294=ORIENTED_EDGE('',*,*,#24621,.F.);
#37295=ORIENTED_EDGE('',*,*,#24727,.F.);
#37296=ORIENTED_EDGE('',*,*,#26888,.F.);
#37297=ORIENTED_EDGE('',*,*,#24623,.F.);
#37298=ORIENTED_EDGE('',*,*,#24615,.F.);
#37299=ORIENTED_EDGE('',*,*,#24612,.F.);
#37300=ORIENTED_EDGE('',*,*,#24724,.F.);
#37301=ORIENTED_EDGE('',*,*,#24732,.F.);
#37302=ORIENTED_EDGE('',*,*,#26889,.T.);
#37303=ORIENTED_EDGE('',*,*,#24721,.F.);
#37304=ORIENTED_EDGE('',*,*,#26889,.F.);
#37305=ORIENTED_EDGE('',*,*,#24728,.F.);
#37306=ORIENTED_EDGE('',*,*,#24620,.F.);
#37307=ORIENTED_EDGE('',*,*,#26888,.T.);
#37308=ORIENTED_EDGE('',*,*,#24607,.F.);
#37309=ORIENTED_EDGE('',*,*,#24713,.F.);
#37310=ORIENTED_EDGE('',*,*,#26890,.F.);
#37311=ORIENTED_EDGE('',*,*,#24609,.F.);
#37312=ORIENTED_EDGE('',*,*,#24601,.F.);
#37313=ORIENTED_EDGE('',*,*,#24598,.F.);
#37314=ORIENTED_EDGE('',*,*,#24710,.F.);
#37315=ORIENTED_EDGE('',*,*,#24718,.F.);
#37316=ORIENTED_EDGE('',*,*,#26891,.T.);
#37317=ORIENTED_EDGE('',*,*,#24707,.F.);
#37318=ORIENTED_EDGE('',*,*,#26891,.F.);
#37319=ORIENTED_EDGE('',*,*,#24714,.F.);
#37320=ORIENTED_EDGE('',*,*,#24606,.F.);
#37321=ORIENTED_EDGE('',*,*,#26890,.T.);
#37322=ORIENTED_EDGE('',*,*,#24593,.F.);
#37323=ORIENTED_EDGE('',*,*,#24699,.F.);
#37324=ORIENTED_EDGE('',*,*,#26892,.F.);
#37325=ORIENTED_EDGE('',*,*,#24595,.F.);
#37326=ORIENTED_EDGE('',*,*,#24587,.F.);
#37327=ORIENTED_EDGE('',*,*,#24584,.F.);
#37328=ORIENTED_EDGE('',*,*,#24696,.F.);
#37329=ORIENTED_EDGE('',*,*,#24704,.F.);
#37330=ORIENTED_EDGE('',*,*,#26893,.T.);
#37331=ORIENTED_EDGE('',*,*,#24693,.F.);
#37332=ORIENTED_EDGE('',*,*,#26893,.F.);
#37333=ORIENTED_EDGE('',*,*,#24700,.F.);
#37334=ORIENTED_EDGE('',*,*,#24592,.F.);
#37335=ORIENTED_EDGE('',*,*,#26892,.T.);
#37336=ORIENTED_EDGE('',*,*,#24578,.F.);
#37337=ORIENTED_EDGE('',*,*,#24685,.F.);
#37338=ORIENTED_EDGE('',*,*,#26894,.F.);
#37339=ORIENTED_EDGE('',*,*,#24580,.F.);
#37340=ORIENTED_EDGE('',*,*,#24572,.F.);
#37341=ORIENTED_EDGE('',*,*,#24569,.F.);
#37342=ORIENTED_EDGE('',*,*,#24682,.F.);
#37343=ORIENTED_EDGE('',*,*,#24690,.F.);
#37344=ORIENTED_EDGE('',*,*,#26895,.T.);
#37345=ORIENTED_EDGE('',*,*,#24679,.F.);
#37346=ORIENTED_EDGE('',*,*,#26895,.F.);
#37347=ORIENTED_EDGE('',*,*,#24686,.F.);
#37348=ORIENTED_EDGE('',*,*,#24577,.F.);
#37349=ORIENTED_EDGE('',*,*,#26894,.T.);
#37350=ORIENTED_EDGE('',*,*,#24566,.F.);
#37351=ORIENTED_EDGE('',*,*,#24670,.F.);
#37352=ORIENTED_EDGE('',*,*,#24659,.F.);
#37353=ORIENTED_EDGE('',*,*,#26896,.F.);
#37354=ORIENTED_EDGE('',*,*,#24671,.F.);
#37355=ORIENTED_EDGE('',*,*,#24565,.F.);
#37356=ORIENTED_EDGE('',*,*,#26897,.T.);
#37357=ORIENTED_EDGE('',*,*,#21356,.F.);
#37358=ORIENTED_EDGE('',*,*,#24667,.F.);
#37359=ORIENTED_EDGE('',*,*,#24675,.F.);
#37360=ORIENTED_EDGE('',*,*,#26896,.T.);
#37361=ORIENTED_EDGE('',*,*,#24664,.F.);
#37362=ORIENTED_EDGE('',*,*,#26897,.F.);
#37363=ORIENTED_EDGE('',*,*,#24677,.F.);
#37364=ORIENTED_EDGE('',*,*,#21357,.F.);
#37365=ORIENTED_EDGE('',*,*,#24557,.F.);
#37366=ORIENTED_EDGE('',*,*,#26898,.F.);
#37367=ORIENTED_EDGE('',*,*,#21491,.F.);
#37368=ORIENTED_EDGE('',*,*,#26898,.T.);
#37369=ORIENTED_EDGE('',*,*,#24553,.F.);
#37370=ORIENTED_EDGE('',*,*,#24654,.F.);
#37371=ORIENTED_EDGE('',*,*,#21492,.F.);
#37372=ORIENTED_EDGE('',*,*,#26899,.F.);
#37373=ORIENTED_EDGE('',*,*,#24555,.F.);
#37374=ORIENTED_EDGE('',*,*,#24547,.F.);
#37375=ORIENTED_EDGE('',*,*,#24544,.F.);
#37376=ORIENTED_EDGE('',*,*,#21495,.F.);
#37377=ORIENTED_EDGE('',*,*,#24657,.F.);
#37378=ORIENTED_EDGE('',*,*,#26900,.T.);
#37379=ORIENTED_EDGE('',*,*,#24652,.F.);
#37380=ORIENTED_EDGE('',*,*,#26900,.F.);
#37381=ORIENTED_EDGE('',*,*,#24655,.F.);
#37382=ORIENTED_EDGE('',*,*,#24552,.F.);
#37383=ORIENTED_EDGE('',*,*,#26899,.T.);
#37384=ORIENTED_EDGE('',*,*,#24539,.F.);
#37385=ORIENTED_EDGE('',*,*,#24645,.F.);
#37386=ORIENTED_EDGE('',*,*,#26901,.F.);
#37387=ORIENTED_EDGE('',*,*,#24541,.F.);
#37388=ORIENTED_EDGE('',*,*,#24533,.F.);
#37389=ORIENTED_EDGE('',*,*,#24530,.F.);
#37390=ORIENTED_EDGE('',*,*,#24642,.F.);
#37391=ORIENTED_EDGE('',*,*,#24650,.F.);
#37392=ORIENTED_EDGE('',*,*,#26902,.T.);
#37393=ORIENTED_EDGE('',*,*,#24639,.F.);
#37394=ORIENTED_EDGE('',*,*,#26902,.F.);
#37395=ORIENTED_EDGE('',*,*,#24646,.F.);
#37396=ORIENTED_EDGE('',*,*,#24538,.F.);
#37397=ORIENTED_EDGE('',*,*,#26901,.T.);
#37398=ORIENTED_EDGE('',*,*,#24525,.F.);
#37399=ORIENTED_EDGE('',*,*,#24631,.F.);
#37400=ORIENTED_EDGE('',*,*,#26903,.F.);
#37401=ORIENTED_EDGE('',*,*,#24527,.F.);
#37402=ORIENTED_EDGE('',*,*,#24519,.F.);
#37403=ORIENTED_EDGE('',*,*,#24516,.F.);
#37404=ORIENTED_EDGE('',*,*,#24628,.F.);
#37405=ORIENTED_EDGE('',*,*,#24636,.F.);
#37406=ORIENTED_EDGE('',*,*,#26904,.T.);
#37407=ORIENTED_EDGE('',*,*,#24625,.F.);
#37408=ORIENTED_EDGE('',*,*,#26904,.F.);
#37409=ORIENTED_EDGE('',*,*,#24632,.F.);
#37410=ORIENTED_EDGE('',*,*,#24524,.F.);
#37411=ORIENTED_EDGE('',*,*,#26903,.T.);
#37412=ORIENTED_EDGE('',*,*,#24511,.F.);
#37413=ORIENTED_EDGE('',*,*,#24617,.F.);
#37414=ORIENTED_EDGE('',*,*,#26905,.F.);
#37415=ORIENTED_EDGE('',*,*,#24513,.F.);
#37416=ORIENTED_EDGE('',*,*,#24505,.F.);
#37417=ORIENTED_EDGE('',*,*,#24502,.F.);
#37418=ORIENTED_EDGE('',*,*,#24614,.F.);
#37419=ORIENTED_EDGE('',*,*,#24622,.F.);
#37420=ORIENTED_EDGE('',*,*,#26906,.T.);
#37421=ORIENTED_EDGE('',*,*,#24611,.F.);
#37422=ORIENTED_EDGE('',*,*,#26906,.F.);
#37423=ORIENTED_EDGE('',*,*,#24618,.F.);
#37424=ORIENTED_EDGE('',*,*,#24510,.F.);
#37425=ORIENTED_EDGE('',*,*,#26905,.T.);
#37426=ORIENTED_EDGE('',*,*,#24497,.F.);
#37427=ORIENTED_EDGE('',*,*,#24603,.F.);
#37428=ORIENTED_EDGE('',*,*,#26907,.F.);
#37429=ORIENTED_EDGE('',*,*,#24499,.F.);
#37430=ORIENTED_EDGE('',*,*,#24491,.F.);
#37431=ORIENTED_EDGE('',*,*,#24488,.F.);
#37432=ORIENTED_EDGE('',*,*,#24600,.F.);
#37433=ORIENTED_EDGE('',*,*,#24608,.F.);
#37434=ORIENTED_EDGE('',*,*,#26908,.T.);
#37435=ORIENTED_EDGE('',*,*,#24597,.F.);
#37436=ORIENTED_EDGE('',*,*,#26908,.F.);
#37437=ORIENTED_EDGE('',*,*,#24604,.F.);
#37438=ORIENTED_EDGE('',*,*,#24496,.F.);
#37439=ORIENTED_EDGE('',*,*,#26907,.T.);
#37440=ORIENTED_EDGE('',*,*,#24482,.F.);
#37441=ORIENTED_EDGE('',*,*,#24589,.F.);
#37442=ORIENTED_EDGE('',*,*,#26909,.F.);
#37443=ORIENTED_EDGE('',*,*,#24484,.F.);
#37444=ORIENTED_EDGE('',*,*,#24476,.F.);
#37445=ORIENTED_EDGE('',*,*,#24473,.F.);
#37446=ORIENTED_EDGE('',*,*,#24586,.F.);
#37447=ORIENTED_EDGE('',*,*,#24594,.F.);
#37448=ORIENTED_EDGE('',*,*,#26910,.T.);
#37449=ORIENTED_EDGE('',*,*,#24583,.F.);
#37450=ORIENTED_EDGE('',*,*,#26910,.F.);
#37451=ORIENTED_EDGE('',*,*,#24590,.F.);
#37452=ORIENTED_EDGE('',*,*,#24481,.F.);
#37453=ORIENTED_EDGE('',*,*,#26909,.T.);
#37454=ORIENTED_EDGE('',*,*,#24470,.F.);
#37455=ORIENTED_EDGE('',*,*,#24574,.F.);
#37456=ORIENTED_EDGE('',*,*,#24563,.F.);
#37457=ORIENTED_EDGE('',*,*,#26911,.F.);
#37458=ORIENTED_EDGE('',*,*,#24575,.F.);
#37459=ORIENTED_EDGE('',*,*,#24469,.F.);
#37460=ORIENTED_EDGE('',*,*,#26912,.T.);
#37461=ORIENTED_EDGE('',*,*,#21360,.F.);
#37462=ORIENTED_EDGE('',*,*,#24571,.F.);
#37463=ORIENTED_EDGE('',*,*,#24579,.F.);
#37464=ORIENTED_EDGE('',*,*,#26911,.T.);
#37465=ORIENTED_EDGE('',*,*,#24568,.F.);
#37466=ORIENTED_EDGE('',*,*,#26912,.F.);
#37467=ORIENTED_EDGE('',*,*,#24581,.F.);
#37468=ORIENTED_EDGE('',*,*,#21361,.F.);
#37469=ORIENTED_EDGE('',*,*,#24461,.F.);
#37470=ORIENTED_EDGE('',*,*,#26913,.F.);
#37471=ORIENTED_EDGE('',*,*,#21485,.F.);
#37472=ORIENTED_EDGE('',*,*,#26913,.T.);
#37473=ORIENTED_EDGE('',*,*,#24457,.F.);
#37474=ORIENTED_EDGE('',*,*,#24558,.F.);
#37475=ORIENTED_EDGE('',*,*,#21486,.F.);
#37476=ORIENTED_EDGE('',*,*,#26914,.F.);
#37477=ORIENTED_EDGE('',*,*,#24459,.F.);
#37478=ORIENTED_EDGE('',*,*,#24451,.F.);
#37479=ORIENTED_EDGE('',*,*,#24448,.F.);
#37480=ORIENTED_EDGE('',*,*,#21489,.F.);
#37481=ORIENTED_EDGE('',*,*,#24561,.F.);
#37482=ORIENTED_EDGE('',*,*,#26915,.T.);
#37483=ORIENTED_EDGE('',*,*,#24556,.F.);
#37484=ORIENTED_EDGE('',*,*,#26915,.F.);
#37485=ORIENTED_EDGE('',*,*,#24559,.F.);
#37486=ORIENTED_EDGE('',*,*,#24456,.F.);
#37487=ORIENTED_EDGE('',*,*,#26914,.T.);
#37488=ORIENTED_EDGE('',*,*,#24443,.F.);
#37489=ORIENTED_EDGE('',*,*,#24549,.F.);
#37490=ORIENTED_EDGE('',*,*,#26916,.F.);
#37491=ORIENTED_EDGE('',*,*,#24445,.F.);
#37492=ORIENTED_EDGE('',*,*,#24437,.F.);
#37493=ORIENTED_EDGE('',*,*,#24434,.F.);
#37494=ORIENTED_EDGE('',*,*,#24546,.F.);
#37495=ORIENTED_EDGE('',*,*,#24554,.F.);
#37496=ORIENTED_EDGE('',*,*,#26917,.T.);
#37497=ORIENTED_EDGE('',*,*,#24543,.F.);
#37498=ORIENTED_EDGE('',*,*,#26917,.F.);
#37499=ORIENTED_EDGE('',*,*,#24550,.F.);
#37500=ORIENTED_EDGE('',*,*,#24442,.F.);
#37501=ORIENTED_EDGE('',*,*,#26916,.T.);
#37502=ORIENTED_EDGE('',*,*,#24429,.F.);
#37503=ORIENTED_EDGE('',*,*,#24535,.F.);
#37504=ORIENTED_EDGE('',*,*,#26918,.F.);
#37505=ORIENTED_EDGE('',*,*,#24431,.F.);
#37506=ORIENTED_EDGE('',*,*,#24423,.F.);
#37507=ORIENTED_EDGE('',*,*,#24420,.F.);
#37508=ORIENTED_EDGE('',*,*,#24532,.F.);
#37509=ORIENTED_EDGE('',*,*,#24540,.F.);
#37510=ORIENTED_EDGE('',*,*,#26919,.T.);
#37511=ORIENTED_EDGE('',*,*,#24529,.F.);
#37512=ORIENTED_EDGE('',*,*,#26919,.F.);
#37513=ORIENTED_EDGE('',*,*,#24536,.F.);
#37514=ORIENTED_EDGE('',*,*,#24428,.F.);
#37515=ORIENTED_EDGE('',*,*,#26918,.T.);
#37516=ORIENTED_EDGE('',*,*,#24415,.F.);
#37517=ORIENTED_EDGE('',*,*,#24521,.F.);
#37518=ORIENTED_EDGE('',*,*,#26920,.F.);
#37519=ORIENTED_EDGE('',*,*,#24417,.F.);
#37520=ORIENTED_EDGE('',*,*,#24409,.F.);
#37521=ORIENTED_EDGE('',*,*,#24406,.F.);
#37522=ORIENTED_EDGE('',*,*,#24518,.F.);
#37523=ORIENTED_EDGE('',*,*,#24526,.F.);
#37524=ORIENTED_EDGE('',*,*,#26921,.T.);
#37525=ORIENTED_EDGE('',*,*,#24515,.F.);
#37526=ORIENTED_EDGE('',*,*,#26921,.F.);
#37527=ORIENTED_EDGE('',*,*,#24522,.F.);
#37528=ORIENTED_EDGE('',*,*,#24414,.F.);
#37529=ORIENTED_EDGE('',*,*,#26920,.T.);
#37530=ORIENTED_EDGE('',*,*,#24401,.F.);
#37531=ORIENTED_EDGE('',*,*,#24507,.F.);
#37532=ORIENTED_EDGE('',*,*,#26922,.F.);
#37533=ORIENTED_EDGE('',*,*,#24403,.F.);
#37534=ORIENTED_EDGE('',*,*,#24395,.F.);
#37535=ORIENTED_EDGE('',*,*,#24392,.F.);
#37536=ORIENTED_EDGE('',*,*,#24504,.F.);
#37537=ORIENTED_EDGE('',*,*,#24512,.F.);
#37538=ORIENTED_EDGE('',*,*,#26923,.T.);
#37539=ORIENTED_EDGE('',*,*,#24501,.F.);
#37540=ORIENTED_EDGE('',*,*,#26923,.F.);
#37541=ORIENTED_EDGE('',*,*,#24508,.F.);
#37542=ORIENTED_EDGE('',*,*,#24400,.F.);
#37543=ORIENTED_EDGE('',*,*,#26922,.T.);
#37544=ORIENTED_EDGE('',*,*,#24386,.F.);
#37545=ORIENTED_EDGE('',*,*,#24493,.F.);
#37546=ORIENTED_EDGE('',*,*,#26924,.F.);
#37547=ORIENTED_EDGE('',*,*,#24388,.F.);
#37548=ORIENTED_EDGE('',*,*,#24380,.F.);
#37549=ORIENTED_EDGE('',*,*,#24377,.F.);
#37550=ORIENTED_EDGE('',*,*,#24490,.F.);
#37551=ORIENTED_EDGE('',*,*,#24498,.F.);
#37552=ORIENTED_EDGE('',*,*,#26925,.T.);
#37553=ORIENTED_EDGE('',*,*,#24487,.F.);
#37554=ORIENTED_EDGE('',*,*,#26925,.F.);
#37555=ORIENTED_EDGE('',*,*,#24494,.F.);
#37556=ORIENTED_EDGE('',*,*,#24385,.F.);
#37557=ORIENTED_EDGE('',*,*,#26924,.T.);
#37558=ORIENTED_EDGE('',*,*,#24374,.F.);
#37559=ORIENTED_EDGE('',*,*,#24478,.F.);
#37560=ORIENTED_EDGE('',*,*,#24467,.F.);
#37561=ORIENTED_EDGE('',*,*,#26926,.F.);
#37562=ORIENTED_EDGE('',*,*,#24479,.F.);
#37563=ORIENTED_EDGE('',*,*,#24373,.F.);
#37564=ORIENTED_EDGE('',*,*,#26927,.T.);
#37565=ORIENTED_EDGE('',*,*,#21364,.F.);
#37566=ORIENTED_EDGE('',*,*,#24475,.F.);
#37567=ORIENTED_EDGE('',*,*,#24483,.F.);
#37568=ORIENTED_EDGE('',*,*,#26926,.T.);
#37569=ORIENTED_EDGE('',*,*,#24472,.F.);
#37570=ORIENTED_EDGE('',*,*,#26927,.F.);
#37571=ORIENTED_EDGE('',*,*,#24485,.F.);
#37572=ORIENTED_EDGE('',*,*,#21365,.F.);
#37573=ORIENTED_EDGE('',*,*,#24365,.F.);
#37574=ORIENTED_EDGE('',*,*,#26928,.F.);
#37575=ORIENTED_EDGE('',*,*,#21779,.F.);
#37576=ORIENTED_EDGE('',*,*,#26928,.T.);
#37577=ORIENTED_EDGE('',*,*,#24361,.F.);
#37578=ORIENTED_EDGE('',*,*,#24462,.F.);
#37579=ORIENTED_EDGE('',*,*,#21780,.F.);
#37580=ORIENTED_EDGE('',*,*,#26929,.F.);
#37581=ORIENTED_EDGE('',*,*,#24363,.F.);
#37582=ORIENTED_EDGE('',*,*,#24355,.F.);
#37583=ORIENTED_EDGE('',*,*,#24352,.F.);
#37584=ORIENTED_EDGE('',*,*,#21480,.F.);
#37585=ORIENTED_EDGE('',*,*,#24465,.F.);
#37586=ORIENTED_EDGE('',*,*,#26930,.T.);
#37587=ORIENTED_EDGE('',*,*,#24460,.F.);
#37588=ORIENTED_EDGE('',*,*,#21483,.F.);
#37589=ORIENTED_EDGE('',*,*,#26930,.F.);
#37590=ORIENTED_EDGE('',*,*,#24463,.F.);
#37591=ORIENTED_EDGE('',*,*,#24360,.F.);
#37592=ORIENTED_EDGE('',*,*,#26929,.T.);
#37593=ORIENTED_EDGE('',*,*,#24347,.F.);
#37594=ORIENTED_EDGE('',*,*,#24453,.F.);
#37595=ORIENTED_EDGE('',*,*,#26931,.F.);
#37596=ORIENTED_EDGE('',*,*,#24349,.F.);
#37597=ORIENTED_EDGE('',*,*,#24341,.F.);
#37598=ORIENTED_EDGE('',*,*,#24338,.F.);
#37599=ORIENTED_EDGE('',*,*,#24450,.F.);
#37600=ORIENTED_EDGE('',*,*,#24458,.F.);
#37601=ORIENTED_EDGE('',*,*,#26932,.T.);
#37602=ORIENTED_EDGE('',*,*,#24447,.F.);
#37603=ORIENTED_EDGE('',*,*,#26932,.F.);
#37604=ORIENTED_EDGE('',*,*,#24454,.F.);
#37605=ORIENTED_EDGE('',*,*,#24346,.F.);
#37606=ORIENTED_EDGE('',*,*,#26931,.T.);
#37607=ORIENTED_EDGE('',*,*,#24333,.F.);
#37608=ORIENTED_EDGE('',*,*,#24439,.F.);
#37609=ORIENTED_EDGE('',*,*,#26933,.F.);
#37610=ORIENTED_EDGE('',*,*,#24335,.F.);
#37611=ORIENTED_EDGE('',*,*,#24327,.F.);
#37612=ORIENTED_EDGE('',*,*,#24324,.F.);
#37613=ORIENTED_EDGE('',*,*,#24436,.F.);
#37614=ORIENTED_EDGE('',*,*,#24444,.F.);
#37615=ORIENTED_EDGE('',*,*,#26934,.T.);
#37616=ORIENTED_EDGE('',*,*,#24433,.F.);
#37617=ORIENTED_EDGE('',*,*,#26934,.F.);
#37618=ORIENTED_EDGE('',*,*,#24440,.F.);
#37619=ORIENTED_EDGE('',*,*,#24332,.F.);
#37620=ORIENTED_EDGE('',*,*,#26933,.T.);
#37621=ORIENTED_EDGE('',*,*,#24319,.F.);
#37622=ORIENTED_EDGE('',*,*,#24425,.F.);
#37623=ORIENTED_EDGE('',*,*,#26935,.F.);
#37624=ORIENTED_EDGE('',*,*,#24321,.F.);
#37625=ORIENTED_EDGE('',*,*,#24313,.F.);
#37626=ORIENTED_EDGE('',*,*,#24310,.F.);
#37627=ORIENTED_EDGE('',*,*,#24422,.F.);
#37628=ORIENTED_EDGE('',*,*,#24430,.F.);
#37629=ORIENTED_EDGE('',*,*,#26936,.T.);
#37630=ORIENTED_EDGE('',*,*,#24419,.F.);
#37631=ORIENTED_EDGE('',*,*,#26936,.F.);
#37632=ORIENTED_EDGE('',*,*,#24426,.F.);
#37633=ORIENTED_EDGE('',*,*,#24318,.F.);
#37634=ORIENTED_EDGE('',*,*,#26935,.T.);
#37635=ORIENTED_EDGE('',*,*,#24305,.F.);
#37636=ORIENTED_EDGE('',*,*,#24411,.F.);
#37637=ORIENTED_EDGE('',*,*,#26937,.F.);
#37638=ORIENTED_EDGE('',*,*,#24307,.F.);
#37639=ORIENTED_EDGE('',*,*,#24299,.F.);
#37640=ORIENTED_EDGE('',*,*,#24296,.F.);
#37641=ORIENTED_EDGE('',*,*,#24408,.F.);
#37642=ORIENTED_EDGE('',*,*,#24416,.F.);
#37643=ORIENTED_EDGE('',*,*,#26938,.T.);
#37644=ORIENTED_EDGE('',*,*,#24405,.F.);
#37645=ORIENTED_EDGE('',*,*,#26938,.F.);
#37646=ORIENTED_EDGE('',*,*,#24412,.F.);
#37647=ORIENTED_EDGE('',*,*,#24304,.F.);
#37648=ORIENTED_EDGE('',*,*,#26937,.T.);
#37649=ORIENTED_EDGE('',*,*,#24290,.F.);
#37650=ORIENTED_EDGE('',*,*,#24397,.F.);
#37651=ORIENTED_EDGE('',*,*,#26939,.F.);
#37652=ORIENTED_EDGE('',*,*,#24292,.F.);
#37653=ORIENTED_EDGE('',*,*,#24284,.F.);
#37654=ORIENTED_EDGE('',*,*,#24281,.F.);
#37655=ORIENTED_EDGE('',*,*,#24394,.F.);
#37656=ORIENTED_EDGE('',*,*,#24402,.F.);
#37657=ORIENTED_EDGE('',*,*,#26940,.T.);
#37658=ORIENTED_EDGE('',*,*,#24391,.F.);
#37659=ORIENTED_EDGE('',*,*,#26940,.F.);
#37660=ORIENTED_EDGE('',*,*,#24398,.F.);
#37661=ORIENTED_EDGE('',*,*,#24289,.F.);
#37662=ORIENTED_EDGE('',*,*,#26939,.T.);
#37663=ORIENTED_EDGE('',*,*,#24278,.F.);
#37664=ORIENTED_EDGE('',*,*,#24382,.F.);
#37665=ORIENTED_EDGE('',*,*,#24371,.F.);
#37666=ORIENTED_EDGE('',*,*,#26941,.F.);
#37667=ORIENTED_EDGE('',*,*,#24383,.F.);
#37668=ORIENTED_EDGE('',*,*,#24277,.F.);
#37669=ORIENTED_EDGE('',*,*,#26942,.T.);
#37670=ORIENTED_EDGE('',*,*,#21368,.F.);
#37671=ORIENTED_EDGE('',*,*,#24379,.F.);
#37672=ORIENTED_EDGE('',*,*,#24387,.F.);
#37673=ORIENTED_EDGE('',*,*,#26941,.T.);
#37674=ORIENTED_EDGE('',*,*,#24376,.F.);
#37675=ORIENTED_EDGE('',*,*,#26942,.F.);
#37676=ORIENTED_EDGE('',*,*,#24389,.F.);
#37677=ORIENTED_EDGE('',*,*,#21369,.F.);
#37678=ORIENTED_EDGE('',*,*,#24269,.F.);
#37679=ORIENTED_EDGE('',*,*,#26943,.F.);
#37680=ORIENTED_EDGE('',*,*,#21773,.F.);
#37681=ORIENTED_EDGE('',*,*,#26943,.T.);
#37682=ORIENTED_EDGE('',*,*,#24265,.F.);
#37683=ORIENTED_EDGE('',*,*,#24366,.F.);
#37684=ORIENTED_EDGE('',*,*,#21774,.F.);
#37685=ORIENTED_EDGE('',*,*,#26944,.F.);
#37686=ORIENTED_EDGE('',*,*,#24267,.F.);
#37687=ORIENTED_EDGE('',*,*,#24259,.F.);
#37688=ORIENTED_EDGE('',*,*,#24256,.F.);
#37689=ORIENTED_EDGE('',*,*,#21777,.F.);
#37690=ORIENTED_EDGE('',*,*,#24369,.F.);
#37691=ORIENTED_EDGE('',*,*,#26945,.T.);
#37692=ORIENTED_EDGE('',*,*,#24364,.F.);
#37693=ORIENTED_EDGE('',*,*,#26945,.F.);
#37694=ORIENTED_EDGE('',*,*,#24367,.F.);
#37695=ORIENTED_EDGE('',*,*,#24264,.F.);
#37696=ORIENTED_EDGE('',*,*,#26944,.T.);
#37697=ORIENTED_EDGE('',*,*,#24251,.F.);
#37698=ORIENTED_EDGE('',*,*,#24357,.F.);
#37699=ORIENTED_EDGE('',*,*,#26946,.F.);
#37700=ORIENTED_EDGE('',*,*,#24253,.F.);
#37701=ORIENTED_EDGE('',*,*,#24245,.F.);
#37702=ORIENTED_EDGE('',*,*,#24242,.F.);
#37703=ORIENTED_EDGE('',*,*,#24354,.F.);
#37704=ORIENTED_EDGE('',*,*,#24362,.F.);
#37705=ORIENTED_EDGE('',*,*,#26947,.T.);
#37706=ORIENTED_EDGE('',*,*,#24351,.F.);
#37707=ORIENTED_EDGE('',*,*,#26947,.F.);
#37708=ORIENTED_EDGE('',*,*,#24358,.F.);
#37709=ORIENTED_EDGE('',*,*,#24250,.F.);
#37710=ORIENTED_EDGE('',*,*,#26946,.T.);
#37711=ORIENTED_EDGE('',*,*,#24237,.F.);
#37712=ORIENTED_EDGE('',*,*,#24343,.F.);
#37713=ORIENTED_EDGE('',*,*,#26948,.F.);
#37714=ORIENTED_EDGE('',*,*,#24239,.F.);
#37715=ORIENTED_EDGE('',*,*,#24231,.F.);
#37716=ORIENTED_EDGE('',*,*,#24228,.F.);
#37717=ORIENTED_EDGE('',*,*,#24340,.F.);
#37718=ORIENTED_EDGE('',*,*,#24348,.F.);
#37719=ORIENTED_EDGE('',*,*,#26949,.T.);
#37720=ORIENTED_EDGE('',*,*,#24337,.F.);
#37721=ORIENTED_EDGE('',*,*,#26949,.F.);
#37722=ORIENTED_EDGE('',*,*,#24344,.F.);
#37723=ORIENTED_EDGE('',*,*,#24236,.F.);
#37724=ORIENTED_EDGE('',*,*,#26948,.T.);
#37725=ORIENTED_EDGE('',*,*,#24223,.F.);
#37726=ORIENTED_EDGE('',*,*,#24329,.F.);
#37727=ORIENTED_EDGE('',*,*,#26950,.F.);
#37728=ORIENTED_EDGE('',*,*,#24225,.F.);
#37729=ORIENTED_EDGE('',*,*,#24217,.F.);
#37730=ORIENTED_EDGE('',*,*,#24214,.F.);
#37731=ORIENTED_EDGE('',*,*,#24326,.F.);
#37732=ORIENTED_EDGE('',*,*,#24334,.F.);
#37733=ORIENTED_EDGE('',*,*,#26951,.T.);
#37734=ORIENTED_EDGE('',*,*,#24323,.F.);
#37735=ORIENTED_EDGE('',*,*,#26951,.F.);
#37736=ORIENTED_EDGE('',*,*,#24330,.F.);
#37737=ORIENTED_EDGE('',*,*,#24222,.F.);
#37738=ORIENTED_EDGE('',*,*,#26950,.T.);
#37739=ORIENTED_EDGE('',*,*,#24209,.F.);
#37740=ORIENTED_EDGE('',*,*,#24315,.F.);
#37741=ORIENTED_EDGE('',*,*,#26952,.F.);
#37742=ORIENTED_EDGE('',*,*,#24211,.F.);
#37743=ORIENTED_EDGE('',*,*,#24203,.F.);
#37744=ORIENTED_EDGE('',*,*,#24200,.F.);
#37745=ORIENTED_EDGE('',*,*,#24312,.F.);
#37746=ORIENTED_EDGE('',*,*,#24320,.F.);
#37747=ORIENTED_EDGE('',*,*,#26953,.T.);
#37748=ORIENTED_EDGE('',*,*,#24309,.F.);
#37749=ORIENTED_EDGE('',*,*,#26953,.F.);
#37750=ORIENTED_EDGE('',*,*,#24316,.F.);
#37751=ORIENTED_EDGE('',*,*,#24208,.F.);
#37752=ORIENTED_EDGE('',*,*,#26952,.T.);
#37753=ORIENTED_EDGE('',*,*,#24194,.F.);
#37754=ORIENTED_EDGE('',*,*,#24301,.F.);
#37755=ORIENTED_EDGE('',*,*,#26954,.F.);
#37756=ORIENTED_EDGE('',*,*,#24196,.F.);
#37757=ORIENTED_EDGE('',*,*,#24188,.F.);
#37758=ORIENTED_EDGE('',*,*,#24185,.F.);
#37759=ORIENTED_EDGE('',*,*,#24298,.F.);
#37760=ORIENTED_EDGE('',*,*,#24306,.F.);
#37761=ORIENTED_EDGE('',*,*,#26955,.T.);
#37762=ORIENTED_EDGE('',*,*,#24295,.F.);
#37763=ORIENTED_EDGE('',*,*,#26955,.F.);
#37764=ORIENTED_EDGE('',*,*,#24302,.F.);
#37765=ORIENTED_EDGE('',*,*,#24193,.F.);
#37766=ORIENTED_EDGE('',*,*,#26954,.T.);
#37767=ORIENTED_EDGE('',*,*,#24182,.F.);
#37768=ORIENTED_EDGE('',*,*,#24286,.F.);
#37769=ORIENTED_EDGE('',*,*,#24275,.F.);
#37770=ORIENTED_EDGE('',*,*,#26956,.F.);
#37771=ORIENTED_EDGE('',*,*,#24287,.F.);
#37772=ORIENTED_EDGE('',*,*,#24181,.F.);
#37773=ORIENTED_EDGE('',*,*,#26957,.T.);
#37774=ORIENTED_EDGE('',*,*,#21372,.F.);
#37775=ORIENTED_EDGE('',*,*,#24283,.F.);
#37776=ORIENTED_EDGE('',*,*,#24291,.F.);
#37777=ORIENTED_EDGE('',*,*,#26956,.T.);
#37778=ORIENTED_EDGE('',*,*,#24280,.F.);
#37779=ORIENTED_EDGE('',*,*,#26957,.F.);
#37780=ORIENTED_EDGE('',*,*,#24293,.F.);
#37781=ORIENTED_EDGE('',*,*,#21373,.F.);
#37782=ORIENTED_EDGE('',*,*,#24173,.F.);
#37783=ORIENTED_EDGE('',*,*,#26958,.F.);
#37784=ORIENTED_EDGE('',*,*,#21767,.F.);
#37785=ORIENTED_EDGE('',*,*,#26958,.T.);
#37786=ORIENTED_EDGE('',*,*,#24169,.F.);
#37787=ORIENTED_EDGE('',*,*,#24270,.F.);
#37788=ORIENTED_EDGE('',*,*,#21768,.F.);
#37789=ORIENTED_EDGE('',*,*,#26959,.F.);
#37790=ORIENTED_EDGE('',*,*,#24171,.F.);
#37791=ORIENTED_EDGE('',*,*,#24163,.F.);
#37792=ORIENTED_EDGE('',*,*,#24160,.F.);
#37793=ORIENTED_EDGE('',*,*,#21771,.F.);
#37794=ORIENTED_EDGE('',*,*,#24273,.F.);
#37795=ORIENTED_EDGE('',*,*,#26960,.T.);
#37796=ORIENTED_EDGE('',*,*,#24268,.F.);
#37797=ORIENTED_EDGE('',*,*,#26960,.F.);
#37798=ORIENTED_EDGE('',*,*,#24271,.F.);
#37799=ORIENTED_EDGE('',*,*,#24168,.F.);
#37800=ORIENTED_EDGE('',*,*,#26959,.T.);
#37801=ORIENTED_EDGE('',*,*,#24155,.F.);
#37802=ORIENTED_EDGE('',*,*,#24261,.F.);
#37803=ORIENTED_EDGE('',*,*,#26961,.F.);
#37804=ORIENTED_EDGE('',*,*,#24157,.F.);
#37805=ORIENTED_EDGE('',*,*,#24149,.F.);
#37806=ORIENTED_EDGE('',*,*,#24146,.F.);
#37807=ORIENTED_EDGE('',*,*,#24258,.F.);
#37808=ORIENTED_EDGE('',*,*,#24266,.F.);
#37809=ORIENTED_EDGE('',*,*,#26962,.T.);
#37810=ORIENTED_EDGE('',*,*,#24255,.F.);
#37811=ORIENTED_EDGE('',*,*,#26962,.F.);
#37812=ORIENTED_EDGE('',*,*,#24262,.F.);
#37813=ORIENTED_EDGE('',*,*,#24154,.F.);
#37814=ORIENTED_EDGE('',*,*,#26961,.T.);
#37815=ORIENTED_EDGE('',*,*,#24141,.F.);
#37816=ORIENTED_EDGE('',*,*,#24247,.F.);
#37817=ORIENTED_EDGE('',*,*,#26963,.F.);
#37818=ORIENTED_EDGE('',*,*,#24143,.F.);
#37819=ORIENTED_EDGE('',*,*,#24135,.F.);
#37820=ORIENTED_EDGE('',*,*,#24132,.F.);
#37821=ORIENTED_EDGE('',*,*,#24244,.F.);
#37822=ORIENTED_EDGE('',*,*,#24252,.F.);
#37823=ORIENTED_EDGE('',*,*,#26964,.T.);
#37824=ORIENTED_EDGE('',*,*,#24241,.F.);
#37825=ORIENTED_EDGE('',*,*,#26964,.F.);
#37826=ORIENTED_EDGE('',*,*,#24248,.F.);
#37827=ORIENTED_EDGE('',*,*,#24140,.F.);
#37828=ORIENTED_EDGE('',*,*,#26963,.T.);
#37829=ORIENTED_EDGE('',*,*,#24127,.F.);
#37830=ORIENTED_EDGE('',*,*,#24233,.F.);
#37831=ORIENTED_EDGE('',*,*,#26965,.F.);
#37832=ORIENTED_EDGE('',*,*,#24129,.F.);
#37833=ORIENTED_EDGE('',*,*,#24121,.F.);
#37834=ORIENTED_EDGE('',*,*,#24118,.F.);
#37835=ORIENTED_EDGE('',*,*,#24230,.F.);
#37836=ORIENTED_EDGE('',*,*,#24238,.F.);
#37837=ORIENTED_EDGE('',*,*,#26966,.T.);
#37838=ORIENTED_EDGE('',*,*,#24227,.F.);
#37839=ORIENTED_EDGE('',*,*,#26966,.F.);
#37840=ORIENTED_EDGE('',*,*,#24234,.F.);
#37841=ORIENTED_EDGE('',*,*,#24126,.F.);
#37842=ORIENTED_EDGE('',*,*,#26965,.T.);
#37843=ORIENTED_EDGE('',*,*,#24113,.F.);
#37844=ORIENTED_EDGE('',*,*,#24219,.F.);
#37845=ORIENTED_EDGE('',*,*,#26967,.F.);
#37846=ORIENTED_EDGE('',*,*,#24115,.F.);
#37847=ORIENTED_EDGE('',*,*,#24107,.F.);
#37848=ORIENTED_EDGE('',*,*,#24104,.F.);
#37849=ORIENTED_EDGE('',*,*,#24216,.F.);
#37850=ORIENTED_EDGE('',*,*,#24224,.F.);
#37851=ORIENTED_EDGE('',*,*,#26968,.T.);
#37852=ORIENTED_EDGE('',*,*,#24213,.F.);
#37853=ORIENTED_EDGE('',*,*,#26968,.F.);
#37854=ORIENTED_EDGE('',*,*,#24220,.F.);
#37855=ORIENTED_EDGE('',*,*,#24112,.F.);
#37856=ORIENTED_EDGE('',*,*,#26967,.T.);
#37857=ORIENTED_EDGE('',*,*,#24098,.F.);
#37858=ORIENTED_EDGE('',*,*,#24205,.F.);
#37859=ORIENTED_EDGE('',*,*,#26969,.F.);
#37860=ORIENTED_EDGE('',*,*,#24100,.F.);
#37861=ORIENTED_EDGE('',*,*,#24092,.F.);
#37862=ORIENTED_EDGE('',*,*,#24089,.F.);
#37863=ORIENTED_EDGE('',*,*,#24202,.F.);
#37864=ORIENTED_EDGE('',*,*,#24210,.F.);
#37865=ORIENTED_EDGE('',*,*,#26970,.T.);
#37866=ORIENTED_EDGE('',*,*,#24199,.F.);
#37867=ORIENTED_EDGE('',*,*,#26970,.F.);
#37868=ORIENTED_EDGE('',*,*,#24206,.F.);
#37869=ORIENTED_EDGE('',*,*,#24097,.F.);
#37870=ORIENTED_EDGE('',*,*,#26969,.T.);
#37871=ORIENTED_EDGE('',*,*,#24086,.F.);
#37872=ORIENTED_EDGE('',*,*,#24190,.F.);
#37873=ORIENTED_EDGE('',*,*,#24179,.F.);
#37874=ORIENTED_EDGE('',*,*,#26971,.F.);
#37875=ORIENTED_EDGE('',*,*,#24191,.F.);
#37876=ORIENTED_EDGE('',*,*,#24085,.F.);
#37877=ORIENTED_EDGE('',*,*,#26972,.T.);
#37878=ORIENTED_EDGE('',*,*,#21376,.F.);
#37879=ORIENTED_EDGE('',*,*,#24187,.F.);
#37880=ORIENTED_EDGE('',*,*,#24195,.F.);
#37881=ORIENTED_EDGE('',*,*,#26971,.T.);
#37882=ORIENTED_EDGE('',*,*,#24184,.F.);
#37883=ORIENTED_EDGE('',*,*,#26972,.F.);
#37884=ORIENTED_EDGE('',*,*,#24197,.F.);
#37885=ORIENTED_EDGE('',*,*,#21377,.F.);
#37886=ORIENTED_EDGE('',*,*,#24077,.F.);
#37887=ORIENTED_EDGE('',*,*,#26973,.F.);
#37888=ORIENTED_EDGE('',*,*,#21761,.F.);
#37889=ORIENTED_EDGE('',*,*,#26973,.T.);
#37890=ORIENTED_EDGE('',*,*,#24073,.F.);
#37891=ORIENTED_EDGE('',*,*,#24174,.F.);
#37892=ORIENTED_EDGE('',*,*,#21762,.F.);
#37893=ORIENTED_EDGE('',*,*,#26974,.F.);
#37894=ORIENTED_EDGE('',*,*,#24075,.F.);
#37895=ORIENTED_EDGE('',*,*,#24067,.F.);
#37896=ORIENTED_EDGE('',*,*,#24064,.F.);
#37897=ORIENTED_EDGE('',*,*,#21765,.F.);
#37898=ORIENTED_EDGE('',*,*,#24177,.F.);
#37899=ORIENTED_EDGE('',*,*,#26975,.T.);
#37900=ORIENTED_EDGE('',*,*,#24172,.F.);
#37901=ORIENTED_EDGE('',*,*,#26975,.F.);
#37902=ORIENTED_EDGE('',*,*,#24175,.F.);
#37903=ORIENTED_EDGE('',*,*,#24072,.F.);
#37904=ORIENTED_EDGE('',*,*,#26974,.T.);
#37905=ORIENTED_EDGE('',*,*,#24059,.F.);
#37906=ORIENTED_EDGE('',*,*,#24165,.F.);
#37907=ORIENTED_EDGE('',*,*,#26976,.F.);
#37908=ORIENTED_EDGE('',*,*,#24061,.F.);
#37909=ORIENTED_EDGE('',*,*,#24053,.F.);
#37910=ORIENTED_EDGE('',*,*,#24050,.F.);
#37911=ORIENTED_EDGE('',*,*,#24162,.F.);
#37912=ORIENTED_EDGE('',*,*,#24170,.F.);
#37913=ORIENTED_EDGE('',*,*,#26977,.T.);
#37914=ORIENTED_EDGE('',*,*,#24159,.F.);
#37915=ORIENTED_EDGE('',*,*,#26977,.F.);
#37916=ORIENTED_EDGE('',*,*,#24166,.F.);
#37917=ORIENTED_EDGE('',*,*,#24058,.F.);
#37918=ORIENTED_EDGE('',*,*,#26976,.T.);
#37919=ORIENTED_EDGE('',*,*,#24045,.F.);
#37920=ORIENTED_EDGE('',*,*,#24151,.F.);
#37921=ORIENTED_EDGE('',*,*,#26978,.F.);
#37922=ORIENTED_EDGE('',*,*,#24047,.F.);
#37923=ORIENTED_EDGE('',*,*,#24039,.F.);
#37924=ORIENTED_EDGE('',*,*,#24036,.F.);
#37925=ORIENTED_EDGE('',*,*,#24148,.F.);
#37926=ORIENTED_EDGE('',*,*,#24156,.F.);
#37927=ORIENTED_EDGE('',*,*,#26979,.T.);
#37928=ORIENTED_EDGE('',*,*,#24145,.F.);
#37929=ORIENTED_EDGE('',*,*,#26979,.F.);
#37930=ORIENTED_EDGE('',*,*,#24152,.F.);
#37931=ORIENTED_EDGE('',*,*,#24044,.F.);
#37932=ORIENTED_EDGE('',*,*,#26978,.T.);
#37933=ORIENTED_EDGE('',*,*,#24031,.F.);
#37934=ORIENTED_EDGE('',*,*,#24137,.F.);
#37935=ORIENTED_EDGE('',*,*,#26980,.F.);
#37936=ORIENTED_EDGE('',*,*,#24033,.F.);
#37937=ORIENTED_EDGE('',*,*,#24025,.F.);
#37938=ORIENTED_EDGE('',*,*,#24022,.F.);
#37939=ORIENTED_EDGE('',*,*,#24134,.F.);
#37940=ORIENTED_EDGE('',*,*,#24142,.F.);
#37941=ORIENTED_EDGE('',*,*,#26981,.T.);
#37942=ORIENTED_EDGE('',*,*,#24131,.F.);
#37943=ORIENTED_EDGE('',*,*,#26981,.F.);
#37944=ORIENTED_EDGE('',*,*,#24138,.F.);
#37945=ORIENTED_EDGE('',*,*,#24030,.F.);
#37946=ORIENTED_EDGE('',*,*,#26980,.T.);
#37947=ORIENTED_EDGE('',*,*,#24017,.F.);
#37948=ORIENTED_EDGE('',*,*,#24123,.F.);
#37949=ORIENTED_EDGE('',*,*,#26982,.F.);
#37950=ORIENTED_EDGE('',*,*,#24019,.F.);
#37951=ORIENTED_EDGE('',*,*,#24011,.F.);
#37952=ORIENTED_EDGE('',*,*,#24008,.F.);
#37953=ORIENTED_EDGE('',*,*,#24120,.F.);
#37954=ORIENTED_EDGE('',*,*,#24128,.F.);
#37955=ORIENTED_EDGE('',*,*,#26983,.T.);
#37956=ORIENTED_EDGE('',*,*,#24117,.F.);
#37957=ORIENTED_EDGE('',*,*,#26983,.F.);
#37958=ORIENTED_EDGE('',*,*,#24124,.F.);
#37959=ORIENTED_EDGE('',*,*,#24016,.F.);
#37960=ORIENTED_EDGE('',*,*,#26982,.T.);
#37961=ORIENTED_EDGE('',*,*,#24002,.F.);
#37962=ORIENTED_EDGE('',*,*,#24109,.F.);
#37963=ORIENTED_EDGE('',*,*,#26984,.F.);
#37964=ORIENTED_EDGE('',*,*,#24004,.F.);
#37965=ORIENTED_EDGE('',*,*,#23996,.F.);
#37966=ORIENTED_EDGE('',*,*,#23993,.F.);
#37967=ORIENTED_EDGE('',*,*,#24106,.F.);
#37968=ORIENTED_EDGE('',*,*,#24114,.F.);
#37969=ORIENTED_EDGE('',*,*,#26985,.T.);
#37970=ORIENTED_EDGE('',*,*,#24103,.F.);
#37971=ORIENTED_EDGE('',*,*,#26985,.F.);
#37972=ORIENTED_EDGE('',*,*,#24110,.F.);
#37973=ORIENTED_EDGE('',*,*,#24001,.F.);
#37974=ORIENTED_EDGE('',*,*,#26984,.T.);
#37975=ORIENTED_EDGE('',*,*,#23990,.F.);
#37976=ORIENTED_EDGE('',*,*,#24094,.F.);
#37977=ORIENTED_EDGE('',*,*,#24083,.F.);
#37978=ORIENTED_EDGE('',*,*,#26986,.F.);
#37979=ORIENTED_EDGE('',*,*,#24095,.F.);
#37980=ORIENTED_EDGE('',*,*,#23989,.F.);
#37981=ORIENTED_EDGE('',*,*,#26987,.T.);
#37982=ORIENTED_EDGE('',*,*,#21380,.F.);
#37983=ORIENTED_EDGE('',*,*,#24091,.F.);
#37984=ORIENTED_EDGE('',*,*,#24099,.F.);
#37985=ORIENTED_EDGE('',*,*,#26986,.T.);
#37986=ORIENTED_EDGE('',*,*,#24088,.F.);
#37987=ORIENTED_EDGE('',*,*,#26987,.F.);
#37988=ORIENTED_EDGE('',*,*,#24101,.F.);
#37989=ORIENTED_EDGE('',*,*,#21381,.F.);
#37990=ORIENTED_EDGE('',*,*,#23981,.F.);
#37991=ORIENTED_EDGE('',*,*,#26988,.F.);
#37992=ORIENTED_EDGE('',*,*,#21755,.F.);
#37993=ORIENTED_EDGE('',*,*,#26988,.T.);
#37994=ORIENTED_EDGE('',*,*,#23977,.F.);
#37995=ORIENTED_EDGE('',*,*,#24078,.F.);
#37996=ORIENTED_EDGE('',*,*,#21756,.F.);
#37997=ORIENTED_EDGE('',*,*,#26989,.F.);
#37998=ORIENTED_EDGE('',*,*,#23979,.F.);
#37999=ORIENTED_EDGE('',*,*,#23971,.F.);
#38000=ORIENTED_EDGE('',*,*,#23968,.F.);
#38001=ORIENTED_EDGE('',*,*,#21759,.F.);
#38002=ORIENTED_EDGE('',*,*,#24081,.F.);
#38003=ORIENTED_EDGE('',*,*,#26990,.T.);
#38004=ORIENTED_EDGE('',*,*,#24076,.F.);
#38005=ORIENTED_EDGE('',*,*,#26990,.F.);
#38006=ORIENTED_EDGE('',*,*,#24079,.F.);
#38007=ORIENTED_EDGE('',*,*,#23976,.F.);
#38008=ORIENTED_EDGE('',*,*,#26989,.T.);
#38009=ORIENTED_EDGE('',*,*,#23963,.F.);
#38010=ORIENTED_EDGE('',*,*,#24069,.F.);
#38011=ORIENTED_EDGE('',*,*,#26991,.F.);
#38012=ORIENTED_EDGE('',*,*,#23965,.F.);
#38013=ORIENTED_EDGE('',*,*,#23957,.F.);
#38014=ORIENTED_EDGE('',*,*,#23954,.F.);
#38015=ORIENTED_EDGE('',*,*,#24066,.F.);
#38016=ORIENTED_EDGE('',*,*,#24074,.F.);
#38017=ORIENTED_EDGE('',*,*,#26992,.T.);
#38018=ORIENTED_EDGE('',*,*,#24063,.F.);
#38019=ORIENTED_EDGE('',*,*,#26992,.F.);
#38020=ORIENTED_EDGE('',*,*,#24070,.F.);
#38021=ORIENTED_EDGE('',*,*,#23962,.F.);
#38022=ORIENTED_EDGE('',*,*,#26991,.T.);
#38023=ORIENTED_EDGE('',*,*,#23949,.F.);
#38024=ORIENTED_EDGE('',*,*,#24055,.F.);
#38025=ORIENTED_EDGE('',*,*,#26993,.F.);
#38026=ORIENTED_EDGE('',*,*,#23951,.F.);
#38027=ORIENTED_EDGE('',*,*,#23943,.F.);
#38028=ORIENTED_EDGE('',*,*,#23940,.F.);
#38029=ORIENTED_EDGE('',*,*,#24052,.F.);
#38030=ORIENTED_EDGE('',*,*,#24060,.F.);
#38031=ORIENTED_EDGE('',*,*,#26994,.T.);
#38032=ORIENTED_EDGE('',*,*,#24049,.F.);
#38033=ORIENTED_EDGE('',*,*,#26994,.F.);
#38034=ORIENTED_EDGE('',*,*,#24056,.F.);
#38035=ORIENTED_EDGE('',*,*,#23948,.F.);
#38036=ORIENTED_EDGE('',*,*,#26993,.T.);
#38037=ORIENTED_EDGE('',*,*,#23935,.F.);
#38038=ORIENTED_EDGE('',*,*,#24041,.F.);
#38039=ORIENTED_EDGE('',*,*,#26995,.F.);
#38040=ORIENTED_EDGE('',*,*,#23937,.F.);
#38041=ORIENTED_EDGE('',*,*,#23929,.F.);
#38042=ORIENTED_EDGE('',*,*,#23926,.F.);
#38043=ORIENTED_EDGE('',*,*,#24038,.F.);
#38044=ORIENTED_EDGE('',*,*,#24046,.F.);
#38045=ORIENTED_EDGE('',*,*,#26996,.T.);
#38046=ORIENTED_EDGE('',*,*,#24035,.F.);
#38047=ORIENTED_EDGE('',*,*,#26996,.F.);
#38048=ORIENTED_EDGE('',*,*,#24042,.F.);
#38049=ORIENTED_EDGE('',*,*,#23934,.F.);
#38050=ORIENTED_EDGE('',*,*,#26995,.T.);
#38051=ORIENTED_EDGE('',*,*,#23921,.F.);
#38052=ORIENTED_EDGE('',*,*,#24027,.F.);
#38053=ORIENTED_EDGE('',*,*,#26997,.F.);
#38054=ORIENTED_EDGE('',*,*,#23923,.F.);
#38055=ORIENTED_EDGE('',*,*,#23915,.F.);
#38056=ORIENTED_EDGE('',*,*,#23912,.F.);
#38057=ORIENTED_EDGE('',*,*,#24024,.F.);
#38058=ORIENTED_EDGE('',*,*,#24032,.F.);
#38059=ORIENTED_EDGE('',*,*,#26998,.T.);
#38060=ORIENTED_EDGE('',*,*,#24021,.F.);
#38061=ORIENTED_EDGE('',*,*,#26998,.F.);
#38062=ORIENTED_EDGE('',*,*,#24028,.F.);
#38063=ORIENTED_EDGE('',*,*,#23920,.F.);
#38064=ORIENTED_EDGE('',*,*,#26997,.T.);
#38065=ORIENTED_EDGE('',*,*,#23906,.F.);
#38066=ORIENTED_EDGE('',*,*,#24013,.F.);
#38067=ORIENTED_EDGE('',*,*,#26999,.F.);
#38068=ORIENTED_EDGE('',*,*,#23908,.F.);
#38069=ORIENTED_EDGE('',*,*,#23900,.F.);
#38070=ORIENTED_EDGE('',*,*,#23897,.F.);
#38071=ORIENTED_EDGE('',*,*,#24010,.F.);
#38072=ORIENTED_EDGE('',*,*,#24018,.F.);
#38073=ORIENTED_EDGE('',*,*,#27000,.T.);
#38074=ORIENTED_EDGE('',*,*,#24007,.F.);
#38075=ORIENTED_EDGE('',*,*,#27000,.F.);
#38076=ORIENTED_EDGE('',*,*,#24014,.F.);
#38077=ORIENTED_EDGE('',*,*,#23905,.F.);
#38078=ORIENTED_EDGE('',*,*,#26999,.T.);
#38079=ORIENTED_EDGE('',*,*,#23894,.F.);
#38080=ORIENTED_EDGE('',*,*,#23998,.F.);
#38081=ORIENTED_EDGE('',*,*,#23987,.F.);
#38082=ORIENTED_EDGE('',*,*,#27001,.F.);
#38083=ORIENTED_EDGE('',*,*,#23999,.F.);
#38084=ORIENTED_EDGE('',*,*,#23893,.F.);
#38085=ORIENTED_EDGE('',*,*,#27002,.T.);
#38086=ORIENTED_EDGE('',*,*,#21384,.F.);
#38087=ORIENTED_EDGE('',*,*,#23995,.F.);
#38088=ORIENTED_EDGE('',*,*,#24003,.F.);
#38089=ORIENTED_EDGE('',*,*,#27001,.T.);
#38090=ORIENTED_EDGE('',*,*,#23992,.F.);
#38091=ORIENTED_EDGE('',*,*,#27002,.F.);
#38092=ORIENTED_EDGE('',*,*,#24005,.F.);
#38093=ORIENTED_EDGE('',*,*,#21385,.F.);
#38094=ORIENTED_EDGE('',*,*,#23885,.F.);
#38095=ORIENTED_EDGE('',*,*,#27003,.F.);
#38096=ORIENTED_EDGE('',*,*,#21749,.F.);
#38097=ORIENTED_EDGE('',*,*,#27003,.T.);
#38098=ORIENTED_EDGE('',*,*,#23881,.F.);
#38099=ORIENTED_EDGE('',*,*,#23982,.F.);
#38100=ORIENTED_EDGE('',*,*,#21750,.F.);
#38101=ORIENTED_EDGE('',*,*,#27004,.F.);
#38102=ORIENTED_EDGE('',*,*,#23883,.F.);
#38103=ORIENTED_EDGE('',*,*,#23875,.F.);
#38104=ORIENTED_EDGE('',*,*,#23872,.F.);
#38105=ORIENTED_EDGE('',*,*,#21753,.F.);
#38106=ORIENTED_EDGE('',*,*,#23985,.F.);
#38107=ORIENTED_EDGE('',*,*,#27005,.T.);
#38108=ORIENTED_EDGE('',*,*,#23980,.F.);
#38109=ORIENTED_EDGE('',*,*,#27005,.F.);
#38110=ORIENTED_EDGE('',*,*,#23983,.F.);
#38111=ORIENTED_EDGE('',*,*,#23880,.F.);
#38112=ORIENTED_EDGE('',*,*,#27004,.T.);
#38113=ORIENTED_EDGE('',*,*,#23867,.F.);
#38114=ORIENTED_EDGE('',*,*,#23973,.F.);
#38115=ORIENTED_EDGE('',*,*,#27006,.F.);
#38116=ORIENTED_EDGE('',*,*,#23869,.F.);
#38117=ORIENTED_EDGE('',*,*,#23861,.F.);
#38118=ORIENTED_EDGE('',*,*,#23858,.F.);
#38119=ORIENTED_EDGE('',*,*,#23970,.F.);
#38120=ORIENTED_EDGE('',*,*,#23978,.F.);
#38121=ORIENTED_EDGE('',*,*,#27007,.T.);
#38122=ORIENTED_EDGE('',*,*,#23967,.F.);
#38123=ORIENTED_EDGE('',*,*,#27007,.F.);
#38124=ORIENTED_EDGE('',*,*,#23974,.F.);
#38125=ORIENTED_EDGE('',*,*,#23866,.F.);
#38126=ORIENTED_EDGE('',*,*,#27006,.T.);
#38127=ORIENTED_EDGE('',*,*,#23853,.F.);
#38128=ORIENTED_EDGE('',*,*,#23959,.F.);
#38129=ORIENTED_EDGE('',*,*,#27008,.F.);
#38130=ORIENTED_EDGE('',*,*,#23855,.F.);
#38131=ORIENTED_EDGE('',*,*,#23847,.F.);
#38132=ORIENTED_EDGE('',*,*,#23844,.F.);
#38133=ORIENTED_EDGE('',*,*,#23956,.F.);
#38134=ORIENTED_EDGE('',*,*,#23964,.F.);
#38135=ORIENTED_EDGE('',*,*,#27009,.T.);
#38136=ORIENTED_EDGE('',*,*,#23953,.F.);
#38137=ORIENTED_EDGE('',*,*,#27009,.F.);
#38138=ORIENTED_EDGE('',*,*,#23960,.F.);
#38139=ORIENTED_EDGE('',*,*,#23852,.F.);
#38140=ORIENTED_EDGE('',*,*,#27008,.T.);
#38141=ORIENTED_EDGE('',*,*,#23839,.F.);
#38142=ORIENTED_EDGE('',*,*,#23945,.F.);
#38143=ORIENTED_EDGE('',*,*,#27010,.F.);
#38144=ORIENTED_EDGE('',*,*,#23841,.F.);
#38145=ORIENTED_EDGE('',*,*,#23833,.F.);
#38146=ORIENTED_EDGE('',*,*,#23830,.F.);
#38147=ORIENTED_EDGE('',*,*,#23942,.F.);
#38148=ORIENTED_EDGE('',*,*,#23950,.F.);
#38149=ORIENTED_EDGE('',*,*,#27011,.T.);
#38150=ORIENTED_EDGE('',*,*,#23939,.F.);
#38151=ORIENTED_EDGE('',*,*,#27011,.F.);
#38152=ORIENTED_EDGE('',*,*,#23946,.F.);
#38153=ORIENTED_EDGE('',*,*,#23838,.F.);
#38154=ORIENTED_EDGE('',*,*,#27010,.T.);
#38155=ORIENTED_EDGE('',*,*,#23825,.F.);
#38156=ORIENTED_EDGE('',*,*,#23931,.F.);
#38157=ORIENTED_EDGE('',*,*,#27012,.F.);
#38158=ORIENTED_EDGE('',*,*,#23827,.F.);
#38159=ORIENTED_EDGE('',*,*,#23819,.F.);
#38160=ORIENTED_EDGE('',*,*,#23816,.F.);
#38161=ORIENTED_EDGE('',*,*,#23928,.F.);
#38162=ORIENTED_EDGE('',*,*,#23936,.F.);
#38163=ORIENTED_EDGE('',*,*,#27013,.T.);
#38164=ORIENTED_EDGE('',*,*,#23925,.F.);
#38165=ORIENTED_EDGE('',*,*,#27013,.F.);
#38166=ORIENTED_EDGE('',*,*,#23932,.F.);
#38167=ORIENTED_EDGE('',*,*,#23824,.F.);
#38168=ORIENTED_EDGE('',*,*,#27012,.T.);
#38169=ORIENTED_EDGE('',*,*,#23810,.F.);
#38170=ORIENTED_EDGE('',*,*,#23917,.F.);
#38171=ORIENTED_EDGE('',*,*,#27014,.F.);
#38172=ORIENTED_EDGE('',*,*,#23812,.F.);
#38173=ORIENTED_EDGE('',*,*,#23804,.F.);
#38174=ORIENTED_EDGE('',*,*,#23801,.F.);
#38175=ORIENTED_EDGE('',*,*,#23914,.F.);
#38176=ORIENTED_EDGE('',*,*,#23922,.F.);
#38177=ORIENTED_EDGE('',*,*,#27015,.T.);
#38178=ORIENTED_EDGE('',*,*,#23911,.F.);
#38179=ORIENTED_EDGE('',*,*,#27015,.F.);
#38180=ORIENTED_EDGE('',*,*,#23918,.F.);
#38181=ORIENTED_EDGE('',*,*,#23809,.F.);
#38182=ORIENTED_EDGE('',*,*,#27014,.T.);
#38183=ORIENTED_EDGE('',*,*,#23798,.F.);
#38184=ORIENTED_EDGE('',*,*,#23902,.F.);
#38185=ORIENTED_EDGE('',*,*,#23891,.F.);
#38186=ORIENTED_EDGE('',*,*,#27016,.F.);
#38187=ORIENTED_EDGE('',*,*,#23903,.F.);
#38188=ORIENTED_EDGE('',*,*,#23797,.F.);
#38189=ORIENTED_EDGE('',*,*,#27017,.T.);
#38190=ORIENTED_EDGE('',*,*,#21388,.F.);
#38191=ORIENTED_EDGE('',*,*,#23899,.F.);
#38192=ORIENTED_EDGE('',*,*,#23907,.F.);
#38193=ORIENTED_EDGE('',*,*,#27016,.T.);
#38194=ORIENTED_EDGE('',*,*,#23896,.F.);
#38195=ORIENTED_EDGE('',*,*,#27017,.F.);
#38196=ORIENTED_EDGE('',*,*,#23909,.F.);
#38197=ORIENTED_EDGE('',*,*,#21389,.F.);
#38198=ORIENTED_EDGE('',*,*,#23789,.F.);
#38199=ORIENTED_EDGE('',*,*,#27018,.F.);
#38200=ORIENTED_EDGE('',*,*,#21743,.F.);
#38201=ORIENTED_EDGE('',*,*,#27018,.T.);
#38202=ORIENTED_EDGE('',*,*,#23785,.F.);
#38203=ORIENTED_EDGE('',*,*,#23886,.F.);
#38204=ORIENTED_EDGE('',*,*,#21744,.F.);
#38205=ORIENTED_EDGE('',*,*,#27019,.F.);
#38206=ORIENTED_EDGE('',*,*,#23787,.F.);
#38207=ORIENTED_EDGE('',*,*,#23779,.F.);
#38208=ORIENTED_EDGE('',*,*,#23776,.F.);
#38209=ORIENTED_EDGE('',*,*,#21747,.F.);
#38210=ORIENTED_EDGE('',*,*,#23889,.F.);
#38211=ORIENTED_EDGE('',*,*,#27020,.T.);
#38212=ORIENTED_EDGE('',*,*,#23884,.F.);
#38213=ORIENTED_EDGE('',*,*,#27020,.F.);
#38214=ORIENTED_EDGE('',*,*,#23887,.F.);
#38215=ORIENTED_EDGE('',*,*,#23784,.F.);
#38216=ORIENTED_EDGE('',*,*,#27019,.T.);
#38217=ORIENTED_EDGE('',*,*,#23771,.F.);
#38218=ORIENTED_EDGE('',*,*,#23877,.F.);
#38219=ORIENTED_EDGE('',*,*,#27021,.F.);
#38220=ORIENTED_EDGE('',*,*,#23773,.F.);
#38221=ORIENTED_EDGE('',*,*,#23765,.F.);
#38222=ORIENTED_EDGE('',*,*,#23762,.F.);
#38223=ORIENTED_EDGE('',*,*,#23874,.F.);
#38224=ORIENTED_EDGE('',*,*,#23882,.F.);
#38225=ORIENTED_EDGE('',*,*,#27022,.T.);
#38226=ORIENTED_EDGE('',*,*,#23871,.F.);
#38227=ORIENTED_EDGE('',*,*,#27022,.F.);
#38228=ORIENTED_EDGE('',*,*,#23878,.F.);
#38229=ORIENTED_EDGE('',*,*,#23770,.F.);
#38230=ORIENTED_EDGE('',*,*,#27021,.T.);
#38231=ORIENTED_EDGE('',*,*,#23757,.F.);
#38232=ORIENTED_EDGE('',*,*,#23863,.F.);
#38233=ORIENTED_EDGE('',*,*,#27023,.F.);
#38234=ORIENTED_EDGE('',*,*,#23759,.F.);
#38235=ORIENTED_EDGE('',*,*,#23751,.F.);
#38236=ORIENTED_EDGE('',*,*,#23748,.F.);
#38237=ORIENTED_EDGE('',*,*,#23860,.F.);
#38238=ORIENTED_EDGE('',*,*,#23868,.F.);
#38239=ORIENTED_EDGE('',*,*,#27024,.T.);
#38240=ORIENTED_EDGE('',*,*,#23857,.F.);
#38241=ORIENTED_EDGE('',*,*,#27024,.F.);
#38242=ORIENTED_EDGE('',*,*,#23864,.F.);
#38243=ORIENTED_EDGE('',*,*,#23756,.F.);
#38244=ORIENTED_EDGE('',*,*,#27023,.T.);
#38245=ORIENTED_EDGE('',*,*,#23743,.F.);
#38246=ORIENTED_EDGE('',*,*,#23849,.F.);
#38247=ORIENTED_EDGE('',*,*,#27025,.F.);
#38248=ORIENTED_EDGE('',*,*,#23745,.F.);
#38249=ORIENTED_EDGE('',*,*,#23737,.F.);
#38250=ORIENTED_EDGE('',*,*,#23734,.F.);
#38251=ORIENTED_EDGE('',*,*,#23846,.F.);
#38252=ORIENTED_EDGE('',*,*,#23854,.F.);
#38253=ORIENTED_EDGE('',*,*,#27026,.T.);
#38254=ORIENTED_EDGE('',*,*,#23843,.F.);
#38255=ORIENTED_EDGE('',*,*,#27026,.F.);
#38256=ORIENTED_EDGE('',*,*,#23850,.F.);
#38257=ORIENTED_EDGE('',*,*,#23742,.F.);
#38258=ORIENTED_EDGE('',*,*,#27025,.T.);
#38259=ORIENTED_EDGE('',*,*,#23729,.F.);
#38260=ORIENTED_EDGE('',*,*,#23835,.F.);
#38261=ORIENTED_EDGE('',*,*,#27027,.F.);
#38262=ORIENTED_EDGE('',*,*,#23731,.F.);
#38263=ORIENTED_EDGE('',*,*,#23723,.F.);
#38264=ORIENTED_EDGE('',*,*,#23720,.F.);
#38265=ORIENTED_EDGE('',*,*,#23832,.F.);
#38266=ORIENTED_EDGE('',*,*,#23840,.F.);
#38267=ORIENTED_EDGE('',*,*,#27028,.T.);
#38268=ORIENTED_EDGE('',*,*,#23829,.F.);
#38269=ORIENTED_EDGE('',*,*,#27028,.F.);
#38270=ORIENTED_EDGE('',*,*,#23836,.F.);
#38271=ORIENTED_EDGE('',*,*,#23728,.F.);
#38272=ORIENTED_EDGE('',*,*,#27027,.T.);
#38273=ORIENTED_EDGE('',*,*,#23714,.F.);
#38274=ORIENTED_EDGE('',*,*,#23821,.F.);
#38275=ORIENTED_EDGE('',*,*,#27029,.F.);
#38276=ORIENTED_EDGE('',*,*,#23716,.F.);
#38277=ORIENTED_EDGE('',*,*,#23708,.F.);
#38278=ORIENTED_EDGE('',*,*,#23705,.F.);
#38279=ORIENTED_EDGE('',*,*,#23818,.F.);
#38280=ORIENTED_EDGE('',*,*,#23826,.F.);
#38281=ORIENTED_EDGE('',*,*,#27030,.T.);
#38282=ORIENTED_EDGE('',*,*,#23815,.F.);
#38283=ORIENTED_EDGE('',*,*,#27030,.F.);
#38284=ORIENTED_EDGE('',*,*,#23822,.F.);
#38285=ORIENTED_EDGE('',*,*,#23713,.F.);
#38286=ORIENTED_EDGE('',*,*,#27029,.T.);
#38287=ORIENTED_EDGE('',*,*,#23702,.F.);
#38288=ORIENTED_EDGE('',*,*,#23806,.F.);
#38289=ORIENTED_EDGE('',*,*,#23795,.F.);
#38290=ORIENTED_EDGE('',*,*,#27031,.F.);
#38291=ORIENTED_EDGE('',*,*,#23807,.F.);
#38292=ORIENTED_EDGE('',*,*,#23701,.F.);
#38293=ORIENTED_EDGE('',*,*,#27032,.T.);
#38294=ORIENTED_EDGE('',*,*,#21392,.F.);
#38295=ORIENTED_EDGE('',*,*,#23803,.F.);
#38296=ORIENTED_EDGE('',*,*,#23811,.F.);
#38297=ORIENTED_EDGE('',*,*,#27031,.T.);
#38298=ORIENTED_EDGE('',*,*,#23800,.F.);
#38299=ORIENTED_EDGE('',*,*,#27032,.F.);
#38300=ORIENTED_EDGE('',*,*,#23813,.F.);
#38301=ORIENTED_EDGE('',*,*,#21393,.F.);
#38302=ORIENTED_EDGE('',*,*,#23693,.F.);
#38303=ORIENTED_EDGE('',*,*,#27033,.F.);
#38304=ORIENTED_EDGE('',*,*,#21737,.F.);
#38305=ORIENTED_EDGE('',*,*,#27033,.T.);
#38306=ORIENTED_EDGE('',*,*,#23689,.F.);
#38307=ORIENTED_EDGE('',*,*,#23790,.F.);
#38308=ORIENTED_EDGE('',*,*,#21738,.F.);
#38309=ORIENTED_EDGE('',*,*,#27034,.F.);
#38310=ORIENTED_EDGE('',*,*,#23691,.F.);
#38311=ORIENTED_EDGE('',*,*,#23683,.F.);
#38312=ORIENTED_EDGE('',*,*,#23680,.F.);
#38313=ORIENTED_EDGE('',*,*,#21741,.F.);
#38314=ORIENTED_EDGE('',*,*,#23793,.F.);
#38315=ORIENTED_EDGE('',*,*,#27035,.T.);
#38316=ORIENTED_EDGE('',*,*,#23788,.F.);
#38317=ORIENTED_EDGE('',*,*,#27035,.F.);
#38318=ORIENTED_EDGE('',*,*,#23791,.F.);
#38319=ORIENTED_EDGE('',*,*,#23688,.F.);
#38320=ORIENTED_EDGE('',*,*,#27034,.T.);
#38321=ORIENTED_EDGE('',*,*,#23675,.F.);
#38322=ORIENTED_EDGE('',*,*,#23781,.F.);
#38323=ORIENTED_EDGE('',*,*,#27036,.F.);
#38324=ORIENTED_EDGE('',*,*,#23677,.F.);
#38325=ORIENTED_EDGE('',*,*,#23669,.F.);
#38326=ORIENTED_EDGE('',*,*,#23666,.F.);
#38327=ORIENTED_EDGE('',*,*,#23778,.F.);
#38328=ORIENTED_EDGE('',*,*,#23786,.F.);
#38329=ORIENTED_EDGE('',*,*,#27037,.T.);
#38330=ORIENTED_EDGE('',*,*,#23775,.F.);
#38331=ORIENTED_EDGE('',*,*,#27037,.F.);
#38332=ORIENTED_EDGE('',*,*,#23782,.F.);
#38333=ORIENTED_EDGE('',*,*,#23674,.F.);
#38334=ORIENTED_EDGE('',*,*,#27036,.T.);
#38335=ORIENTED_EDGE('',*,*,#23661,.F.);
#38336=ORIENTED_EDGE('',*,*,#23767,.F.);
#38337=ORIENTED_EDGE('',*,*,#27038,.F.);
#38338=ORIENTED_EDGE('',*,*,#23663,.F.);
#38339=ORIENTED_EDGE('',*,*,#23655,.F.);
#38340=ORIENTED_EDGE('',*,*,#23652,.F.);
#38341=ORIENTED_EDGE('',*,*,#23764,.F.);
#38342=ORIENTED_EDGE('',*,*,#23772,.F.);
#38343=ORIENTED_EDGE('',*,*,#27039,.T.);
#38344=ORIENTED_EDGE('',*,*,#23761,.F.);
#38345=ORIENTED_EDGE('',*,*,#27039,.F.);
#38346=ORIENTED_EDGE('',*,*,#23768,.F.);
#38347=ORIENTED_EDGE('',*,*,#23660,.F.);
#38348=ORIENTED_EDGE('',*,*,#27038,.T.);
#38349=ORIENTED_EDGE('',*,*,#23647,.F.);
#38350=ORIENTED_EDGE('',*,*,#23753,.F.);
#38351=ORIENTED_EDGE('',*,*,#27040,.F.);
#38352=ORIENTED_EDGE('',*,*,#23649,.F.);
#38353=ORIENTED_EDGE('',*,*,#23641,.F.);
#38354=ORIENTED_EDGE('',*,*,#23638,.F.);
#38355=ORIENTED_EDGE('',*,*,#23750,.F.);
#38356=ORIENTED_EDGE('',*,*,#23758,.F.);
#38357=ORIENTED_EDGE('',*,*,#27041,.T.);
#38358=ORIENTED_EDGE('',*,*,#23747,.F.);
#38359=ORIENTED_EDGE('',*,*,#27041,.F.);
#38360=ORIENTED_EDGE('',*,*,#23754,.F.);
#38361=ORIENTED_EDGE('',*,*,#23646,.F.);
#38362=ORIENTED_EDGE('',*,*,#27040,.T.);
#38363=ORIENTED_EDGE('',*,*,#23633,.F.);
#38364=ORIENTED_EDGE('',*,*,#23739,.F.);
#38365=ORIENTED_EDGE('',*,*,#27042,.F.);
#38366=ORIENTED_EDGE('',*,*,#23635,.F.);
#38367=ORIENTED_EDGE('',*,*,#23627,.F.);
#38368=ORIENTED_EDGE('',*,*,#23624,.F.);
#38369=ORIENTED_EDGE('',*,*,#23736,.F.);
#38370=ORIENTED_EDGE('',*,*,#23744,.F.);
#38371=ORIENTED_EDGE('',*,*,#27043,.T.);
#38372=ORIENTED_EDGE('',*,*,#23733,.F.);
#38373=ORIENTED_EDGE('',*,*,#27043,.F.);
#38374=ORIENTED_EDGE('',*,*,#23740,.F.);
#38375=ORIENTED_EDGE('',*,*,#23632,.F.);
#38376=ORIENTED_EDGE('',*,*,#27042,.T.);
#38377=ORIENTED_EDGE('',*,*,#23618,.F.);
#38378=ORIENTED_EDGE('',*,*,#23725,.F.);
#38379=ORIENTED_EDGE('',*,*,#27044,.F.);
#38380=ORIENTED_EDGE('',*,*,#23620,.F.);
#38381=ORIENTED_EDGE('',*,*,#23612,.F.);
#38382=ORIENTED_EDGE('',*,*,#23609,.F.);
#38383=ORIENTED_EDGE('',*,*,#23722,.F.);
#38384=ORIENTED_EDGE('',*,*,#23730,.F.);
#38385=ORIENTED_EDGE('',*,*,#27045,.T.);
#38386=ORIENTED_EDGE('',*,*,#23719,.F.);
#38387=ORIENTED_EDGE('',*,*,#27045,.F.);
#38388=ORIENTED_EDGE('',*,*,#23726,.F.);
#38389=ORIENTED_EDGE('',*,*,#23617,.F.);
#38390=ORIENTED_EDGE('',*,*,#27044,.T.);
#38391=ORIENTED_EDGE('',*,*,#23606,.F.);
#38392=ORIENTED_EDGE('',*,*,#23710,.F.);
#38393=ORIENTED_EDGE('',*,*,#23699,.F.);
#38394=ORIENTED_EDGE('',*,*,#27046,.F.);
#38395=ORIENTED_EDGE('',*,*,#23711,.F.);
#38396=ORIENTED_EDGE('',*,*,#23605,.F.);
#38397=ORIENTED_EDGE('',*,*,#27047,.T.);
#38398=ORIENTED_EDGE('',*,*,#21396,.F.);
#38399=ORIENTED_EDGE('',*,*,#23707,.F.);
#38400=ORIENTED_EDGE('',*,*,#23715,.F.);
#38401=ORIENTED_EDGE('',*,*,#27046,.T.);
#38402=ORIENTED_EDGE('',*,*,#23704,.F.);
#38403=ORIENTED_EDGE('',*,*,#27047,.F.);
#38404=ORIENTED_EDGE('',*,*,#23717,.F.);
#38405=ORIENTED_EDGE('',*,*,#21397,.F.);
#38406=ORIENTED_EDGE('',*,*,#23597,.F.);
#38407=ORIENTED_EDGE('',*,*,#27048,.F.);
#38408=ORIENTED_EDGE('',*,*,#21731,.F.);
#38409=ORIENTED_EDGE('',*,*,#27048,.T.);
#38410=ORIENTED_EDGE('',*,*,#23593,.F.);
#38411=ORIENTED_EDGE('',*,*,#23694,.F.);
#38412=ORIENTED_EDGE('',*,*,#21732,.F.);
#38413=ORIENTED_EDGE('',*,*,#27049,.F.);
#38414=ORIENTED_EDGE('',*,*,#23595,.F.);
#38415=ORIENTED_EDGE('',*,*,#23587,.F.);
#38416=ORIENTED_EDGE('',*,*,#23584,.F.);
#38417=ORIENTED_EDGE('',*,*,#21735,.F.);
#38418=ORIENTED_EDGE('',*,*,#23697,.F.);
#38419=ORIENTED_EDGE('',*,*,#27050,.T.);
#38420=ORIENTED_EDGE('',*,*,#23692,.F.);
#38421=ORIENTED_EDGE('',*,*,#27050,.F.);
#38422=ORIENTED_EDGE('',*,*,#23695,.F.);
#38423=ORIENTED_EDGE('',*,*,#23592,.F.);
#38424=ORIENTED_EDGE('',*,*,#27049,.T.);
#38425=ORIENTED_EDGE('',*,*,#23579,.F.);
#38426=ORIENTED_EDGE('',*,*,#23685,.F.);
#38427=ORIENTED_EDGE('',*,*,#27051,.F.);
#38428=ORIENTED_EDGE('',*,*,#23581,.F.);
#38429=ORIENTED_EDGE('',*,*,#23573,.F.);
#38430=ORIENTED_EDGE('',*,*,#23570,.F.);
#38431=ORIENTED_EDGE('',*,*,#23682,.F.);
#38432=ORIENTED_EDGE('',*,*,#23690,.F.);
#38433=ORIENTED_EDGE('',*,*,#27052,.T.);
#38434=ORIENTED_EDGE('',*,*,#23679,.F.);
#38435=ORIENTED_EDGE('',*,*,#27052,.F.);
#38436=ORIENTED_EDGE('',*,*,#23686,.F.);
#38437=ORIENTED_EDGE('',*,*,#23578,.F.);
#38438=ORIENTED_EDGE('',*,*,#27051,.T.);
#38439=ORIENTED_EDGE('',*,*,#23565,.F.);
#38440=ORIENTED_EDGE('',*,*,#23671,.F.);
#38441=ORIENTED_EDGE('',*,*,#27053,.F.);
#38442=ORIENTED_EDGE('',*,*,#23567,.F.);
#38443=ORIENTED_EDGE('',*,*,#23559,.F.);
#38444=ORIENTED_EDGE('',*,*,#23556,.F.);
#38445=ORIENTED_EDGE('',*,*,#23668,.F.);
#38446=ORIENTED_EDGE('',*,*,#23676,.F.);
#38447=ORIENTED_EDGE('',*,*,#27054,.T.);
#38448=ORIENTED_EDGE('',*,*,#23665,.F.);
#38449=ORIENTED_EDGE('',*,*,#27054,.F.);
#38450=ORIENTED_EDGE('',*,*,#23672,.F.);
#38451=ORIENTED_EDGE('',*,*,#23564,.F.);
#38452=ORIENTED_EDGE('',*,*,#27053,.T.);
#38453=ORIENTED_EDGE('',*,*,#23551,.F.);
#38454=ORIENTED_EDGE('',*,*,#23657,.F.);
#38455=ORIENTED_EDGE('',*,*,#27055,.F.);
#38456=ORIENTED_EDGE('',*,*,#23553,.F.);
#38457=ORIENTED_EDGE('',*,*,#23545,.F.);
#38458=ORIENTED_EDGE('',*,*,#23542,.F.);
#38459=ORIENTED_EDGE('',*,*,#23654,.F.);
#38460=ORIENTED_EDGE('',*,*,#23662,.F.);
#38461=ORIENTED_EDGE('',*,*,#27056,.T.);
#38462=ORIENTED_EDGE('',*,*,#23651,.F.);
#38463=ORIENTED_EDGE('',*,*,#27056,.F.);
#38464=ORIENTED_EDGE('',*,*,#23658,.F.);
#38465=ORIENTED_EDGE('',*,*,#23550,.F.);
#38466=ORIENTED_EDGE('',*,*,#27055,.T.);
#38467=ORIENTED_EDGE('',*,*,#23537,.F.);
#38468=ORIENTED_EDGE('',*,*,#23643,.F.);
#38469=ORIENTED_EDGE('',*,*,#27057,.F.);
#38470=ORIENTED_EDGE('',*,*,#23539,.F.);
#38471=ORIENTED_EDGE('',*,*,#23531,.F.);
#38472=ORIENTED_EDGE('',*,*,#23528,.F.);
#38473=ORIENTED_EDGE('',*,*,#23640,.F.);
#38474=ORIENTED_EDGE('',*,*,#23648,.F.);
#38475=ORIENTED_EDGE('',*,*,#27058,.T.);
#38476=ORIENTED_EDGE('',*,*,#23637,.F.);
#38477=ORIENTED_EDGE('',*,*,#27058,.F.);
#38478=ORIENTED_EDGE('',*,*,#23644,.F.);
#38479=ORIENTED_EDGE('',*,*,#23536,.F.);
#38480=ORIENTED_EDGE('',*,*,#27057,.T.);
#38481=ORIENTED_EDGE('',*,*,#23522,.F.);
#38482=ORIENTED_EDGE('',*,*,#23629,.F.);
#38483=ORIENTED_EDGE('',*,*,#27059,.F.);
#38484=ORIENTED_EDGE('',*,*,#23524,.F.);
#38485=ORIENTED_EDGE('',*,*,#23516,.F.);
#38486=ORIENTED_EDGE('',*,*,#23513,.F.);
#38487=ORIENTED_EDGE('',*,*,#23626,.F.);
#38488=ORIENTED_EDGE('',*,*,#23634,.F.);
#38489=ORIENTED_EDGE('',*,*,#27060,.T.);
#38490=ORIENTED_EDGE('',*,*,#23623,.F.);
#38491=ORIENTED_EDGE('',*,*,#27060,.F.);
#38492=ORIENTED_EDGE('',*,*,#23630,.F.);
#38493=ORIENTED_EDGE('',*,*,#23521,.F.);
#38494=ORIENTED_EDGE('',*,*,#27059,.T.);
#38495=ORIENTED_EDGE('',*,*,#23510,.F.);
#38496=ORIENTED_EDGE('',*,*,#23614,.F.);
#38497=ORIENTED_EDGE('',*,*,#23603,.F.);
#38498=ORIENTED_EDGE('',*,*,#27061,.F.);
#38499=ORIENTED_EDGE('',*,*,#23615,.F.);
#38500=ORIENTED_EDGE('',*,*,#23509,.F.);
#38501=ORIENTED_EDGE('',*,*,#27062,.T.);
#38502=ORIENTED_EDGE('',*,*,#21400,.F.);
#38503=ORIENTED_EDGE('',*,*,#23611,.F.);
#38504=ORIENTED_EDGE('',*,*,#23619,.F.);
#38505=ORIENTED_EDGE('',*,*,#27061,.T.);
#38506=ORIENTED_EDGE('',*,*,#23608,.F.);
#38507=ORIENTED_EDGE('',*,*,#27062,.F.);
#38508=ORIENTED_EDGE('',*,*,#23621,.F.);
#38509=ORIENTED_EDGE('',*,*,#21401,.F.);
#38510=ORIENTED_EDGE('',*,*,#23501,.F.);
#38511=ORIENTED_EDGE('',*,*,#27063,.F.);
#38512=ORIENTED_EDGE('',*,*,#21725,.F.);
#38513=ORIENTED_EDGE('',*,*,#27063,.T.);
#38514=ORIENTED_EDGE('',*,*,#23497,.F.);
#38515=ORIENTED_EDGE('',*,*,#23598,.F.);
#38516=ORIENTED_EDGE('',*,*,#21726,.F.);
#38517=ORIENTED_EDGE('',*,*,#27064,.F.);
#38518=ORIENTED_EDGE('',*,*,#23499,.F.);
#38519=ORIENTED_EDGE('',*,*,#23491,.F.);
#38520=ORIENTED_EDGE('',*,*,#23488,.F.);
#38521=ORIENTED_EDGE('',*,*,#21729,.F.);
#38522=ORIENTED_EDGE('',*,*,#23601,.F.);
#38523=ORIENTED_EDGE('',*,*,#27065,.T.);
#38524=ORIENTED_EDGE('',*,*,#23596,.F.);
#38525=ORIENTED_EDGE('',*,*,#27065,.F.);
#38526=ORIENTED_EDGE('',*,*,#23599,.F.);
#38527=ORIENTED_EDGE('',*,*,#23496,.F.);
#38528=ORIENTED_EDGE('',*,*,#27064,.T.);
#38529=ORIENTED_EDGE('',*,*,#23483,.F.);
#38530=ORIENTED_EDGE('',*,*,#23589,.F.);
#38531=ORIENTED_EDGE('',*,*,#27066,.F.);
#38532=ORIENTED_EDGE('',*,*,#23485,.F.);
#38533=ORIENTED_EDGE('',*,*,#23477,.F.);
#38534=ORIENTED_EDGE('',*,*,#23474,.F.);
#38535=ORIENTED_EDGE('',*,*,#23586,.F.);
#38536=ORIENTED_EDGE('',*,*,#23594,.F.);
#38537=ORIENTED_EDGE('',*,*,#27067,.T.);
#38538=ORIENTED_EDGE('',*,*,#23583,.F.);
#38539=ORIENTED_EDGE('',*,*,#27067,.F.);
#38540=ORIENTED_EDGE('',*,*,#23590,.F.);
#38541=ORIENTED_EDGE('',*,*,#23482,.F.);
#38542=ORIENTED_EDGE('',*,*,#27066,.T.);
#38543=ORIENTED_EDGE('',*,*,#23469,.F.);
#38544=ORIENTED_EDGE('',*,*,#23575,.F.);
#38545=ORIENTED_EDGE('',*,*,#27068,.F.);
#38546=ORIENTED_EDGE('',*,*,#23471,.F.);
#38547=ORIENTED_EDGE('',*,*,#23463,.F.);
#38548=ORIENTED_EDGE('',*,*,#23460,.F.);
#38549=ORIENTED_EDGE('',*,*,#23572,.F.);
#38550=ORIENTED_EDGE('',*,*,#23580,.F.);
#38551=ORIENTED_EDGE('',*,*,#27069,.T.);
#38552=ORIENTED_EDGE('',*,*,#23569,.F.);
#38553=ORIENTED_EDGE('',*,*,#27069,.F.);
#38554=ORIENTED_EDGE('',*,*,#23576,.F.);
#38555=ORIENTED_EDGE('',*,*,#23468,.F.);
#38556=ORIENTED_EDGE('',*,*,#27068,.T.);
#38557=ORIENTED_EDGE('',*,*,#23455,.F.);
#38558=ORIENTED_EDGE('',*,*,#23561,.F.);
#38559=ORIENTED_EDGE('',*,*,#27070,.F.);
#38560=ORIENTED_EDGE('',*,*,#23457,.F.);
#38561=ORIENTED_EDGE('',*,*,#23449,.F.);
#38562=ORIENTED_EDGE('',*,*,#23446,.F.);
#38563=ORIENTED_EDGE('',*,*,#23558,.F.);
#38564=ORIENTED_EDGE('',*,*,#23566,.F.);
#38565=ORIENTED_EDGE('',*,*,#27071,.T.);
#38566=ORIENTED_EDGE('',*,*,#23555,.F.);
#38567=ORIENTED_EDGE('',*,*,#27071,.F.);
#38568=ORIENTED_EDGE('',*,*,#23562,.F.);
#38569=ORIENTED_EDGE('',*,*,#23454,.F.);
#38570=ORIENTED_EDGE('',*,*,#27070,.T.);
#38571=ORIENTED_EDGE('',*,*,#23441,.F.);
#38572=ORIENTED_EDGE('',*,*,#23547,.F.);
#38573=ORIENTED_EDGE('',*,*,#27072,.F.);
#38574=ORIENTED_EDGE('',*,*,#23443,.F.);
#38575=ORIENTED_EDGE('',*,*,#23435,.F.);
#38576=ORIENTED_EDGE('',*,*,#23432,.F.);
#38577=ORIENTED_EDGE('',*,*,#23544,.F.);
#38578=ORIENTED_EDGE('',*,*,#23552,.F.);
#38579=ORIENTED_EDGE('',*,*,#27073,.T.);
#38580=ORIENTED_EDGE('',*,*,#23541,.F.);
#38581=ORIENTED_EDGE('',*,*,#27073,.F.);
#38582=ORIENTED_EDGE('',*,*,#23548,.F.);
#38583=ORIENTED_EDGE('',*,*,#23440,.F.);
#38584=ORIENTED_EDGE('',*,*,#27072,.T.);
#38585=ORIENTED_EDGE('',*,*,#23426,.F.);
#38586=ORIENTED_EDGE('',*,*,#23533,.F.);
#38587=ORIENTED_EDGE('',*,*,#27074,.F.);
#38588=ORIENTED_EDGE('',*,*,#23428,.F.);
#38589=ORIENTED_EDGE('',*,*,#23420,.F.);
#38590=ORIENTED_EDGE('',*,*,#23417,.F.);
#38591=ORIENTED_EDGE('',*,*,#23530,.F.);
#38592=ORIENTED_EDGE('',*,*,#23538,.F.);
#38593=ORIENTED_EDGE('',*,*,#27075,.T.);
#38594=ORIENTED_EDGE('',*,*,#23527,.F.);
#38595=ORIENTED_EDGE('',*,*,#27075,.F.);
#38596=ORIENTED_EDGE('',*,*,#23534,.F.);
#38597=ORIENTED_EDGE('',*,*,#23425,.F.);
#38598=ORIENTED_EDGE('',*,*,#27074,.T.);
#38599=ORIENTED_EDGE('',*,*,#23414,.F.);
#38600=ORIENTED_EDGE('',*,*,#23518,.F.);
#38601=ORIENTED_EDGE('',*,*,#23507,.F.);
#38602=ORIENTED_EDGE('',*,*,#27076,.F.);
#38603=ORIENTED_EDGE('',*,*,#23519,.F.);
#38604=ORIENTED_EDGE('',*,*,#23413,.F.);
#38605=ORIENTED_EDGE('',*,*,#27077,.T.);
#38606=ORIENTED_EDGE('',*,*,#21404,.F.);
#38607=ORIENTED_EDGE('',*,*,#23515,.F.);
#38608=ORIENTED_EDGE('',*,*,#23523,.F.);
#38609=ORIENTED_EDGE('',*,*,#27076,.T.);
#38610=ORIENTED_EDGE('',*,*,#23512,.F.);
#38611=ORIENTED_EDGE('',*,*,#27077,.F.);
#38612=ORIENTED_EDGE('',*,*,#23525,.F.);
#38613=ORIENTED_EDGE('',*,*,#21405,.F.);
#38614=ORIENTED_EDGE('',*,*,#23405,.F.);
#38615=ORIENTED_EDGE('',*,*,#27078,.F.);
#38616=ORIENTED_EDGE('',*,*,#21719,.F.);
#38617=ORIENTED_EDGE('',*,*,#27078,.T.);
#38618=ORIENTED_EDGE('',*,*,#23401,.F.);
#38619=ORIENTED_EDGE('',*,*,#23502,.F.);
#38620=ORIENTED_EDGE('',*,*,#21720,.F.);
#38621=ORIENTED_EDGE('',*,*,#27079,.F.);
#38622=ORIENTED_EDGE('',*,*,#23403,.F.);
#38623=ORIENTED_EDGE('',*,*,#23395,.F.);
#38624=ORIENTED_EDGE('',*,*,#23392,.F.);
#38625=ORIENTED_EDGE('',*,*,#21723,.F.);
#38626=ORIENTED_EDGE('',*,*,#23505,.F.);
#38627=ORIENTED_EDGE('',*,*,#27080,.T.);
#38628=ORIENTED_EDGE('',*,*,#23500,.F.);
#38629=ORIENTED_EDGE('',*,*,#27080,.F.);
#38630=ORIENTED_EDGE('',*,*,#23503,.F.);
#38631=ORIENTED_EDGE('',*,*,#23400,.F.);
#38632=ORIENTED_EDGE('',*,*,#27079,.T.);
#38633=ORIENTED_EDGE('',*,*,#23387,.F.);
#38634=ORIENTED_EDGE('',*,*,#23493,.F.);
#38635=ORIENTED_EDGE('',*,*,#27081,.F.);
#38636=ORIENTED_EDGE('',*,*,#23389,.F.);
#38637=ORIENTED_EDGE('',*,*,#23381,.F.);
#38638=ORIENTED_EDGE('',*,*,#23378,.F.);
#38639=ORIENTED_EDGE('',*,*,#23490,.F.);
#38640=ORIENTED_EDGE('',*,*,#23498,.F.);
#38641=ORIENTED_EDGE('',*,*,#27082,.T.);
#38642=ORIENTED_EDGE('',*,*,#23487,.F.);
#38643=ORIENTED_EDGE('',*,*,#27082,.F.);
#38644=ORIENTED_EDGE('',*,*,#23494,.F.);
#38645=ORIENTED_EDGE('',*,*,#23386,.F.);
#38646=ORIENTED_EDGE('',*,*,#27081,.T.);
#38647=ORIENTED_EDGE('',*,*,#23373,.F.);
#38648=ORIENTED_EDGE('',*,*,#23479,.F.);
#38649=ORIENTED_EDGE('',*,*,#27083,.F.);
#38650=ORIENTED_EDGE('',*,*,#23375,.F.);
#38651=ORIENTED_EDGE('',*,*,#23367,.F.);
#38652=ORIENTED_EDGE('',*,*,#23364,.F.);
#38653=ORIENTED_EDGE('',*,*,#23476,.F.);
#38654=ORIENTED_EDGE('',*,*,#23484,.F.);
#38655=ORIENTED_EDGE('',*,*,#27084,.T.);
#38656=ORIENTED_EDGE('',*,*,#23473,.F.);
#38657=ORIENTED_EDGE('',*,*,#27084,.F.);
#38658=ORIENTED_EDGE('',*,*,#23480,.F.);
#38659=ORIENTED_EDGE('',*,*,#23372,.F.);
#38660=ORIENTED_EDGE('',*,*,#27083,.T.);
#38661=ORIENTED_EDGE('',*,*,#23359,.F.);
#38662=ORIENTED_EDGE('',*,*,#23465,.F.);
#38663=ORIENTED_EDGE('',*,*,#27085,.F.);
#38664=ORIENTED_EDGE('',*,*,#23361,.F.);
#38665=ORIENTED_EDGE('',*,*,#23353,.F.);
#38666=ORIENTED_EDGE('',*,*,#23350,.F.);
#38667=ORIENTED_EDGE('',*,*,#23462,.F.);
#38668=ORIENTED_EDGE('',*,*,#23470,.F.);
#38669=ORIENTED_EDGE('',*,*,#27086,.T.);
#38670=ORIENTED_EDGE('',*,*,#23459,.F.);
#38671=ORIENTED_EDGE('',*,*,#27086,.F.);
#38672=ORIENTED_EDGE('',*,*,#23466,.F.);
#38673=ORIENTED_EDGE('',*,*,#23358,.F.);
#38674=ORIENTED_EDGE('',*,*,#27085,.T.);
#38675=ORIENTED_EDGE('',*,*,#23345,.F.);
#38676=ORIENTED_EDGE('',*,*,#23451,.F.);
#38677=ORIENTED_EDGE('',*,*,#27087,.F.);
#38678=ORIENTED_EDGE('',*,*,#23347,.F.);
#38679=ORIENTED_EDGE('',*,*,#23339,.F.);
#38680=ORIENTED_EDGE('',*,*,#23336,.F.);
#38681=ORIENTED_EDGE('',*,*,#23448,.F.);
#38682=ORIENTED_EDGE('',*,*,#23456,.F.);
#38683=ORIENTED_EDGE('',*,*,#27088,.T.);
#38684=ORIENTED_EDGE('',*,*,#23445,.F.);
#38685=ORIENTED_EDGE('',*,*,#27088,.F.);
#38686=ORIENTED_EDGE('',*,*,#23452,.F.);
#38687=ORIENTED_EDGE('',*,*,#23344,.F.);
#38688=ORIENTED_EDGE('',*,*,#27087,.T.);
#38689=ORIENTED_EDGE('',*,*,#23330,.F.);
#38690=ORIENTED_EDGE('',*,*,#23437,.F.);
#38691=ORIENTED_EDGE('',*,*,#27089,.F.);
#38692=ORIENTED_EDGE('',*,*,#23332,.F.);
#38693=ORIENTED_EDGE('',*,*,#23324,.F.);
#38694=ORIENTED_EDGE('',*,*,#23321,.F.);
#38695=ORIENTED_EDGE('',*,*,#23434,.F.);
#38696=ORIENTED_EDGE('',*,*,#23442,.F.);
#38697=ORIENTED_EDGE('',*,*,#27090,.T.);
#38698=ORIENTED_EDGE('',*,*,#23431,.F.);
#38699=ORIENTED_EDGE('',*,*,#27090,.F.);
#38700=ORIENTED_EDGE('',*,*,#23438,.F.);
#38701=ORIENTED_EDGE('',*,*,#23329,.F.);
#38702=ORIENTED_EDGE('',*,*,#27089,.T.);
#38703=ORIENTED_EDGE('',*,*,#23318,.F.);
#38704=ORIENTED_EDGE('',*,*,#23422,.F.);
#38705=ORIENTED_EDGE('',*,*,#23411,.F.);
#38706=ORIENTED_EDGE('',*,*,#27091,.F.);
#38707=ORIENTED_EDGE('',*,*,#23423,.F.);
#38708=ORIENTED_EDGE('',*,*,#23317,.F.);
#38709=ORIENTED_EDGE('',*,*,#27092,.T.);
#38710=ORIENTED_EDGE('',*,*,#21408,.F.);
#38711=ORIENTED_EDGE('',*,*,#23419,.F.);
#38712=ORIENTED_EDGE('',*,*,#23427,.F.);
#38713=ORIENTED_EDGE('',*,*,#27091,.T.);
#38714=ORIENTED_EDGE('',*,*,#23416,.F.);
#38715=ORIENTED_EDGE('',*,*,#27092,.F.);
#38716=ORIENTED_EDGE('',*,*,#23429,.F.);
#38717=ORIENTED_EDGE('',*,*,#21409,.F.);
#38718=ORIENTED_EDGE('',*,*,#23309,.F.);
#38719=ORIENTED_EDGE('',*,*,#27093,.F.);
#38720=ORIENTED_EDGE('',*,*,#21713,.F.);
#38721=ORIENTED_EDGE('',*,*,#27093,.T.);
#38722=ORIENTED_EDGE('',*,*,#23305,.F.);
#38723=ORIENTED_EDGE('',*,*,#23406,.F.);
#38724=ORIENTED_EDGE('',*,*,#21714,.F.);
#38725=ORIENTED_EDGE('',*,*,#27094,.F.);
#38726=ORIENTED_EDGE('',*,*,#23307,.F.);
#38727=ORIENTED_EDGE('',*,*,#23299,.F.);
#38728=ORIENTED_EDGE('',*,*,#23296,.F.);
#38729=ORIENTED_EDGE('',*,*,#21717,.F.);
#38730=ORIENTED_EDGE('',*,*,#23409,.F.);
#38731=ORIENTED_EDGE('',*,*,#27095,.T.);
#38732=ORIENTED_EDGE('',*,*,#23404,.F.);
#38733=ORIENTED_EDGE('',*,*,#27095,.F.);
#38734=ORIENTED_EDGE('',*,*,#23407,.F.);
#38735=ORIENTED_EDGE('',*,*,#23304,.F.);
#38736=ORIENTED_EDGE('',*,*,#27094,.T.);
#38737=ORIENTED_EDGE('',*,*,#23291,.F.);
#38738=ORIENTED_EDGE('',*,*,#23397,.F.);
#38739=ORIENTED_EDGE('',*,*,#27096,.F.);
#38740=ORIENTED_EDGE('',*,*,#23293,.F.);
#38741=ORIENTED_EDGE('',*,*,#23285,.F.);
#38742=ORIENTED_EDGE('',*,*,#23282,.F.);
#38743=ORIENTED_EDGE('',*,*,#23394,.F.);
#38744=ORIENTED_EDGE('',*,*,#23402,.F.);
#38745=ORIENTED_EDGE('',*,*,#27097,.T.);
#38746=ORIENTED_EDGE('',*,*,#23391,.F.);
#38747=ORIENTED_EDGE('',*,*,#27097,.F.);
#38748=ORIENTED_EDGE('',*,*,#23398,.F.);
#38749=ORIENTED_EDGE('',*,*,#23290,.F.);
#38750=ORIENTED_EDGE('',*,*,#27096,.T.);
#38751=ORIENTED_EDGE('',*,*,#23277,.F.);
#38752=ORIENTED_EDGE('',*,*,#23383,.F.);
#38753=ORIENTED_EDGE('',*,*,#27098,.F.);
#38754=ORIENTED_EDGE('',*,*,#23279,.F.);
#38755=ORIENTED_EDGE('',*,*,#23271,.F.);
#38756=ORIENTED_EDGE('',*,*,#23268,.F.);
#38757=ORIENTED_EDGE('',*,*,#23380,.F.);
#38758=ORIENTED_EDGE('',*,*,#23388,.F.);
#38759=ORIENTED_EDGE('',*,*,#27099,.T.);
#38760=ORIENTED_EDGE('',*,*,#23377,.F.);
#38761=ORIENTED_EDGE('',*,*,#27099,.F.);
#38762=ORIENTED_EDGE('',*,*,#23384,.F.);
#38763=ORIENTED_EDGE('',*,*,#23276,.F.);
#38764=ORIENTED_EDGE('',*,*,#27098,.T.);
#38765=ORIENTED_EDGE('',*,*,#23263,.F.);
#38766=ORIENTED_EDGE('',*,*,#23369,.F.);
#38767=ORIENTED_EDGE('',*,*,#27100,.F.);
#38768=ORIENTED_EDGE('',*,*,#23265,.F.);
#38769=ORIENTED_EDGE('',*,*,#23257,.F.);
#38770=ORIENTED_EDGE('',*,*,#23254,.F.);
#38771=ORIENTED_EDGE('',*,*,#23366,.F.);
#38772=ORIENTED_EDGE('',*,*,#23374,.F.);
#38773=ORIENTED_EDGE('',*,*,#27101,.T.);
#38774=ORIENTED_EDGE('',*,*,#23363,.F.);
#38775=ORIENTED_EDGE('',*,*,#27101,.F.);
#38776=ORIENTED_EDGE('',*,*,#23370,.F.);
#38777=ORIENTED_EDGE('',*,*,#23262,.F.);
#38778=ORIENTED_EDGE('',*,*,#27100,.T.);
#38779=ORIENTED_EDGE('',*,*,#23249,.F.);
#38780=ORIENTED_EDGE('',*,*,#23355,.F.);
#38781=ORIENTED_EDGE('',*,*,#27102,.F.);
#38782=ORIENTED_EDGE('',*,*,#23251,.F.);
#38783=ORIENTED_EDGE('',*,*,#23243,.F.);
#38784=ORIENTED_EDGE('',*,*,#23240,.F.);
#38785=ORIENTED_EDGE('',*,*,#23352,.F.);
#38786=ORIENTED_EDGE('',*,*,#23360,.F.);
#38787=ORIENTED_EDGE('',*,*,#27103,.T.);
#38788=ORIENTED_EDGE('',*,*,#23349,.F.);
#38789=ORIENTED_EDGE('',*,*,#27103,.F.);
#38790=ORIENTED_EDGE('',*,*,#23356,.F.);
#38791=ORIENTED_EDGE('',*,*,#23248,.F.);
#38792=ORIENTED_EDGE('',*,*,#27102,.T.);
#38793=ORIENTED_EDGE('',*,*,#23234,.F.);
#38794=ORIENTED_EDGE('',*,*,#23341,.F.);
#38795=ORIENTED_EDGE('',*,*,#27104,.F.);
#38796=ORIENTED_EDGE('',*,*,#23236,.F.);
#38797=ORIENTED_EDGE('',*,*,#23228,.F.);
#38798=ORIENTED_EDGE('',*,*,#23225,.F.);
#38799=ORIENTED_EDGE('',*,*,#23338,.F.);
#38800=ORIENTED_EDGE('',*,*,#23346,.F.);
#38801=ORIENTED_EDGE('',*,*,#27105,.T.);
#38802=ORIENTED_EDGE('',*,*,#23335,.F.);
#38803=ORIENTED_EDGE('',*,*,#27105,.F.);
#38804=ORIENTED_EDGE('',*,*,#23342,.F.);
#38805=ORIENTED_EDGE('',*,*,#23233,.F.);
#38806=ORIENTED_EDGE('',*,*,#27104,.T.);
#38807=ORIENTED_EDGE('',*,*,#23222,.F.);
#38808=ORIENTED_EDGE('',*,*,#23326,.F.);
#38809=ORIENTED_EDGE('',*,*,#23315,.F.);
#38810=ORIENTED_EDGE('',*,*,#27106,.F.);
#38811=ORIENTED_EDGE('',*,*,#23327,.F.);
#38812=ORIENTED_EDGE('',*,*,#23221,.F.);
#38813=ORIENTED_EDGE('',*,*,#27107,.T.);
#38814=ORIENTED_EDGE('',*,*,#21412,.F.);
#38815=ORIENTED_EDGE('',*,*,#23323,.F.);
#38816=ORIENTED_EDGE('',*,*,#23331,.F.);
#38817=ORIENTED_EDGE('',*,*,#27106,.T.);
#38818=ORIENTED_EDGE('',*,*,#23320,.F.);
#38819=ORIENTED_EDGE('',*,*,#27107,.F.);
#38820=ORIENTED_EDGE('',*,*,#23333,.F.);
#38821=ORIENTED_EDGE('',*,*,#21413,.F.);
#38822=ORIENTED_EDGE('',*,*,#23213,.F.);
#38823=ORIENTED_EDGE('',*,*,#27108,.F.);
#38824=ORIENTED_EDGE('',*,*,#21707,.F.);
#38825=ORIENTED_EDGE('',*,*,#27108,.T.);
#38826=ORIENTED_EDGE('',*,*,#23209,.F.);
#38827=ORIENTED_EDGE('',*,*,#23310,.F.);
#38828=ORIENTED_EDGE('',*,*,#21708,.F.);
#38829=ORIENTED_EDGE('',*,*,#27109,.F.);
#38830=ORIENTED_EDGE('',*,*,#23211,.F.);
#38831=ORIENTED_EDGE('',*,*,#23203,.F.);
#38832=ORIENTED_EDGE('',*,*,#23200,.F.);
#38833=ORIENTED_EDGE('',*,*,#21711,.F.);
#38834=ORIENTED_EDGE('',*,*,#23313,.F.);
#38835=ORIENTED_EDGE('',*,*,#27110,.T.);
#38836=ORIENTED_EDGE('',*,*,#23308,.F.);
#38837=ORIENTED_EDGE('',*,*,#27110,.F.);
#38838=ORIENTED_EDGE('',*,*,#23311,.F.);
#38839=ORIENTED_EDGE('',*,*,#23208,.F.);
#38840=ORIENTED_EDGE('',*,*,#27109,.T.);
#38841=ORIENTED_EDGE('',*,*,#23195,.F.);
#38842=ORIENTED_EDGE('',*,*,#23301,.F.);
#38843=ORIENTED_EDGE('',*,*,#27111,.F.);
#38844=ORIENTED_EDGE('',*,*,#23197,.F.);
#38845=ORIENTED_EDGE('',*,*,#23189,.F.);
#38846=ORIENTED_EDGE('',*,*,#23186,.F.);
#38847=ORIENTED_EDGE('',*,*,#23298,.F.);
#38848=ORIENTED_EDGE('',*,*,#23306,.F.);
#38849=ORIENTED_EDGE('',*,*,#27112,.T.);
#38850=ORIENTED_EDGE('',*,*,#23295,.F.);
#38851=ORIENTED_EDGE('',*,*,#27112,.F.);
#38852=ORIENTED_EDGE('',*,*,#23302,.F.);
#38853=ORIENTED_EDGE('',*,*,#23194,.F.);
#38854=ORIENTED_EDGE('',*,*,#27111,.T.);
#38855=ORIENTED_EDGE('',*,*,#23181,.F.);
#38856=ORIENTED_EDGE('',*,*,#23287,.F.);
#38857=ORIENTED_EDGE('',*,*,#27113,.F.);
#38858=ORIENTED_EDGE('',*,*,#23183,.F.);
#38859=ORIENTED_EDGE('',*,*,#23175,.F.);
#38860=ORIENTED_EDGE('',*,*,#23172,.F.);
#38861=ORIENTED_EDGE('',*,*,#23284,.F.);
#38862=ORIENTED_EDGE('',*,*,#23292,.F.);
#38863=ORIENTED_EDGE('',*,*,#27114,.T.);
#38864=ORIENTED_EDGE('',*,*,#23281,.F.);
#38865=ORIENTED_EDGE('',*,*,#27114,.F.);
#38866=ORIENTED_EDGE('',*,*,#23288,.F.);
#38867=ORIENTED_EDGE('',*,*,#23180,.F.);
#38868=ORIENTED_EDGE('',*,*,#27113,.T.);
#38869=ORIENTED_EDGE('',*,*,#23167,.F.);
#38870=ORIENTED_EDGE('',*,*,#23273,.F.);
#38871=ORIENTED_EDGE('',*,*,#27115,.F.);
#38872=ORIENTED_EDGE('',*,*,#23169,.F.);
#38873=ORIENTED_EDGE('',*,*,#23161,.F.);
#38874=ORIENTED_EDGE('',*,*,#23158,.F.);
#38875=ORIENTED_EDGE('',*,*,#23270,.F.);
#38876=ORIENTED_EDGE('',*,*,#23278,.F.);
#38877=ORIENTED_EDGE('',*,*,#27116,.T.);
#38878=ORIENTED_EDGE('',*,*,#23267,.F.);
#38879=ORIENTED_EDGE('',*,*,#27116,.F.);
#38880=ORIENTED_EDGE('',*,*,#23274,.F.);
#38881=ORIENTED_EDGE('',*,*,#23166,.F.);
#38882=ORIENTED_EDGE('',*,*,#27115,.T.);
#38883=ORIENTED_EDGE('',*,*,#23153,.F.);
#38884=ORIENTED_EDGE('',*,*,#23259,.F.);
#38885=ORIENTED_EDGE('',*,*,#27117,.F.);
#38886=ORIENTED_EDGE('',*,*,#23155,.F.);
#38887=ORIENTED_EDGE('',*,*,#23147,.F.);
#38888=ORIENTED_EDGE('',*,*,#23144,.F.);
#38889=ORIENTED_EDGE('',*,*,#23256,.F.);
#38890=ORIENTED_EDGE('',*,*,#23264,.F.);
#38891=ORIENTED_EDGE('',*,*,#27118,.T.);
#38892=ORIENTED_EDGE('',*,*,#23253,.F.);
#38893=ORIENTED_EDGE('',*,*,#27118,.F.);
#38894=ORIENTED_EDGE('',*,*,#23260,.F.);
#38895=ORIENTED_EDGE('',*,*,#23152,.F.);
#38896=ORIENTED_EDGE('',*,*,#27117,.T.);
#38897=ORIENTED_EDGE('',*,*,#23138,.F.);
#38898=ORIENTED_EDGE('',*,*,#23245,.F.);
#38899=ORIENTED_EDGE('',*,*,#27119,.F.);
#38900=ORIENTED_EDGE('',*,*,#23140,.F.);
#38901=ORIENTED_EDGE('',*,*,#23132,.F.);
#38902=ORIENTED_EDGE('',*,*,#23129,.F.);
#38903=ORIENTED_EDGE('',*,*,#23242,.F.);
#38904=ORIENTED_EDGE('',*,*,#23250,.F.);
#38905=ORIENTED_EDGE('',*,*,#27120,.T.);
#38906=ORIENTED_EDGE('',*,*,#23239,.F.);
#38907=ORIENTED_EDGE('',*,*,#27120,.F.);
#38908=ORIENTED_EDGE('',*,*,#23246,.F.);
#38909=ORIENTED_EDGE('',*,*,#23137,.F.);
#38910=ORIENTED_EDGE('',*,*,#27119,.T.);
#38911=ORIENTED_EDGE('',*,*,#23126,.F.);
#38912=ORIENTED_EDGE('',*,*,#23230,.F.);
#38913=ORIENTED_EDGE('',*,*,#23219,.F.);
#38914=ORIENTED_EDGE('',*,*,#27121,.F.);
#38915=ORIENTED_EDGE('',*,*,#23231,.F.);
#38916=ORIENTED_EDGE('',*,*,#23125,.F.);
#38917=ORIENTED_EDGE('',*,*,#27122,.T.);
#38918=ORIENTED_EDGE('',*,*,#21416,.F.);
#38919=ORIENTED_EDGE('',*,*,#23227,.F.);
#38920=ORIENTED_EDGE('',*,*,#23235,.F.);
#38921=ORIENTED_EDGE('',*,*,#27121,.T.);
#38922=ORIENTED_EDGE('',*,*,#23224,.F.);
#38923=ORIENTED_EDGE('',*,*,#27122,.F.);
#38924=ORIENTED_EDGE('',*,*,#23237,.F.);
#38925=ORIENTED_EDGE('',*,*,#21417,.F.);
#38926=ORIENTED_EDGE('',*,*,#23117,.F.);
#38927=ORIENTED_EDGE('',*,*,#27123,.F.);
#38928=ORIENTED_EDGE('',*,*,#21701,.F.);
#38929=ORIENTED_EDGE('',*,*,#27123,.T.);
#38930=ORIENTED_EDGE('',*,*,#23113,.F.);
#38931=ORIENTED_EDGE('',*,*,#23214,.F.);
#38932=ORIENTED_EDGE('',*,*,#21702,.F.);
#38933=ORIENTED_EDGE('',*,*,#27124,.F.);
#38934=ORIENTED_EDGE('',*,*,#23115,.F.);
#38935=ORIENTED_EDGE('',*,*,#23107,.F.);
#38936=ORIENTED_EDGE('',*,*,#23104,.F.);
#38937=ORIENTED_EDGE('',*,*,#21705,.F.);
#38938=ORIENTED_EDGE('',*,*,#23217,.F.);
#38939=ORIENTED_EDGE('',*,*,#27125,.T.);
#38940=ORIENTED_EDGE('',*,*,#23212,.F.);
#38941=ORIENTED_EDGE('',*,*,#27125,.F.);
#38942=ORIENTED_EDGE('',*,*,#23215,.F.);
#38943=ORIENTED_EDGE('',*,*,#23112,.F.);
#38944=ORIENTED_EDGE('',*,*,#27124,.T.);
#38945=ORIENTED_EDGE('',*,*,#23099,.F.);
#38946=ORIENTED_EDGE('',*,*,#23205,.F.);
#38947=ORIENTED_EDGE('',*,*,#27126,.F.);
#38948=ORIENTED_EDGE('',*,*,#23101,.F.);
#38949=ORIENTED_EDGE('',*,*,#23093,.F.);
#38950=ORIENTED_EDGE('',*,*,#23090,.F.);
#38951=ORIENTED_EDGE('',*,*,#23202,.F.);
#38952=ORIENTED_EDGE('',*,*,#23210,.F.);
#38953=ORIENTED_EDGE('',*,*,#27127,.T.);
#38954=ORIENTED_EDGE('',*,*,#23199,.F.);
#38955=ORIENTED_EDGE('',*,*,#27127,.F.);
#38956=ORIENTED_EDGE('',*,*,#23206,.F.);
#38957=ORIENTED_EDGE('',*,*,#23098,.F.);
#38958=ORIENTED_EDGE('',*,*,#27126,.T.);
#38959=ORIENTED_EDGE('',*,*,#23085,.F.);
#38960=ORIENTED_EDGE('',*,*,#23191,.F.);
#38961=ORIENTED_EDGE('',*,*,#27128,.F.);
#38962=ORIENTED_EDGE('',*,*,#23087,.F.);
#38963=ORIENTED_EDGE('',*,*,#23079,.F.);
#38964=ORIENTED_EDGE('',*,*,#23076,.F.);
#38965=ORIENTED_EDGE('',*,*,#23188,.F.);
#38966=ORIENTED_EDGE('',*,*,#23196,.F.);
#38967=ORIENTED_EDGE('',*,*,#27129,.T.);
#38968=ORIENTED_EDGE('',*,*,#23185,.F.);
#38969=ORIENTED_EDGE('',*,*,#27129,.F.);
#38970=ORIENTED_EDGE('',*,*,#23192,.F.);
#38971=ORIENTED_EDGE('',*,*,#23084,.F.);
#38972=ORIENTED_EDGE('',*,*,#27128,.T.);
#38973=ORIENTED_EDGE('',*,*,#23071,.F.);
#38974=ORIENTED_EDGE('',*,*,#23177,.F.);
#38975=ORIENTED_EDGE('',*,*,#27130,.F.);
#38976=ORIENTED_EDGE('',*,*,#23073,.F.);
#38977=ORIENTED_EDGE('',*,*,#23065,.F.);
#38978=ORIENTED_EDGE('',*,*,#23062,.F.);
#38979=ORIENTED_EDGE('',*,*,#23174,.F.);
#38980=ORIENTED_EDGE('',*,*,#23182,.F.);
#38981=ORIENTED_EDGE('',*,*,#27131,.T.);
#38982=ORIENTED_EDGE('',*,*,#23171,.F.);
#38983=ORIENTED_EDGE('',*,*,#27131,.F.);
#38984=ORIENTED_EDGE('',*,*,#23178,.F.);
#38985=ORIENTED_EDGE('',*,*,#23070,.F.);
#38986=ORIENTED_EDGE('',*,*,#27130,.T.);
#38987=ORIENTED_EDGE('',*,*,#23057,.F.);
#38988=ORIENTED_EDGE('',*,*,#23163,.F.);
#38989=ORIENTED_EDGE('',*,*,#27132,.F.);
#38990=ORIENTED_EDGE('',*,*,#23059,.F.);
#38991=ORIENTED_EDGE('',*,*,#23051,.F.);
#38992=ORIENTED_EDGE('',*,*,#23048,.F.);
#38993=ORIENTED_EDGE('',*,*,#23160,.F.);
#38994=ORIENTED_EDGE('',*,*,#23168,.F.);
#38995=ORIENTED_EDGE('',*,*,#27133,.T.);
#38996=ORIENTED_EDGE('',*,*,#23157,.F.);
#38997=ORIENTED_EDGE('',*,*,#27133,.F.);
#38998=ORIENTED_EDGE('',*,*,#23164,.F.);
#38999=ORIENTED_EDGE('',*,*,#23056,.F.);
#39000=ORIENTED_EDGE('',*,*,#27132,.T.);
#39001=ORIENTED_EDGE('',*,*,#23042,.F.);
#39002=ORIENTED_EDGE('',*,*,#23149,.F.);
#39003=ORIENTED_EDGE('',*,*,#27134,.F.);
#39004=ORIENTED_EDGE('',*,*,#23044,.F.);
#39005=ORIENTED_EDGE('',*,*,#23036,.F.);
#39006=ORIENTED_EDGE('',*,*,#23033,.F.);
#39007=ORIENTED_EDGE('',*,*,#23146,.F.);
#39008=ORIENTED_EDGE('',*,*,#23154,.F.);
#39009=ORIENTED_EDGE('',*,*,#27135,.T.);
#39010=ORIENTED_EDGE('',*,*,#23143,.F.);
#39011=ORIENTED_EDGE('',*,*,#27135,.F.);
#39012=ORIENTED_EDGE('',*,*,#23150,.F.);
#39013=ORIENTED_EDGE('',*,*,#23041,.F.);
#39014=ORIENTED_EDGE('',*,*,#27134,.T.);
#39015=ORIENTED_EDGE('',*,*,#23030,.F.);
#39016=ORIENTED_EDGE('',*,*,#23134,.F.);
#39017=ORIENTED_EDGE('',*,*,#23123,.F.);
#39018=ORIENTED_EDGE('',*,*,#27136,.F.);
#39019=ORIENTED_EDGE('',*,*,#23135,.F.);
#39020=ORIENTED_EDGE('',*,*,#23029,.F.);
#39021=ORIENTED_EDGE('',*,*,#27137,.T.);
#39022=ORIENTED_EDGE('',*,*,#21420,.F.);
#39023=ORIENTED_EDGE('',*,*,#23131,.F.);
#39024=ORIENTED_EDGE('',*,*,#23139,.F.);
#39025=ORIENTED_EDGE('',*,*,#27136,.T.);
#39026=ORIENTED_EDGE('',*,*,#23128,.F.);
#39027=ORIENTED_EDGE('',*,*,#27137,.F.);
#39028=ORIENTED_EDGE('',*,*,#23141,.F.);
#39029=ORIENTED_EDGE('',*,*,#21421,.F.);
#39030=ORIENTED_EDGE('',*,*,#23021,.F.);
#39031=ORIENTED_EDGE('',*,*,#27138,.F.);
#39032=ORIENTED_EDGE('',*,*,#21695,.F.);
#39033=ORIENTED_EDGE('',*,*,#27138,.T.);
#39034=ORIENTED_EDGE('',*,*,#23017,.F.);
#39035=ORIENTED_EDGE('',*,*,#23118,.F.);
#39036=ORIENTED_EDGE('',*,*,#21696,.F.);
#39037=ORIENTED_EDGE('',*,*,#27139,.F.);
#39038=ORIENTED_EDGE('',*,*,#23019,.F.);
#39039=ORIENTED_EDGE('',*,*,#23011,.F.);
#39040=ORIENTED_EDGE('',*,*,#23008,.F.);
#39041=ORIENTED_EDGE('',*,*,#21699,.F.);
#39042=ORIENTED_EDGE('',*,*,#23121,.F.);
#39043=ORIENTED_EDGE('',*,*,#27140,.T.);
#39044=ORIENTED_EDGE('',*,*,#23116,.F.);
#39045=ORIENTED_EDGE('',*,*,#27140,.F.);
#39046=ORIENTED_EDGE('',*,*,#23119,.F.);
#39047=ORIENTED_EDGE('',*,*,#23016,.F.);
#39048=ORIENTED_EDGE('',*,*,#27139,.T.);
#39049=ORIENTED_EDGE('',*,*,#23003,.F.);
#39050=ORIENTED_EDGE('',*,*,#23109,.F.);
#39051=ORIENTED_EDGE('',*,*,#27141,.F.);
#39052=ORIENTED_EDGE('',*,*,#23005,.F.);
#39053=ORIENTED_EDGE('',*,*,#22997,.F.);
#39054=ORIENTED_EDGE('',*,*,#22994,.F.);
#39055=ORIENTED_EDGE('',*,*,#23106,.F.);
#39056=ORIENTED_EDGE('',*,*,#23114,.F.);
#39057=ORIENTED_EDGE('',*,*,#27142,.T.);
#39058=ORIENTED_EDGE('',*,*,#23103,.F.);
#39059=ORIENTED_EDGE('',*,*,#27142,.F.);
#39060=ORIENTED_EDGE('',*,*,#23110,.F.);
#39061=ORIENTED_EDGE('',*,*,#23002,.F.);
#39062=ORIENTED_EDGE('',*,*,#27141,.T.);
#39063=ORIENTED_EDGE('',*,*,#22989,.F.);
#39064=ORIENTED_EDGE('',*,*,#23095,.F.);
#39065=ORIENTED_EDGE('',*,*,#27143,.F.);
#39066=ORIENTED_EDGE('',*,*,#22991,.F.);
#39067=ORIENTED_EDGE('',*,*,#22983,.F.);
#39068=ORIENTED_EDGE('',*,*,#22980,.F.);
#39069=ORIENTED_EDGE('',*,*,#23092,.F.);
#39070=ORIENTED_EDGE('',*,*,#23100,.F.);
#39071=ORIENTED_EDGE('',*,*,#27144,.T.);
#39072=ORIENTED_EDGE('',*,*,#23089,.F.);
#39073=ORIENTED_EDGE('',*,*,#27144,.F.);
#39074=ORIENTED_EDGE('',*,*,#23096,.F.);
#39075=ORIENTED_EDGE('',*,*,#22988,.F.);
#39076=ORIENTED_EDGE('',*,*,#27143,.T.);
#39077=ORIENTED_EDGE('',*,*,#22975,.F.);
#39078=ORIENTED_EDGE('',*,*,#23081,.F.);
#39079=ORIENTED_EDGE('',*,*,#27145,.F.);
#39080=ORIENTED_EDGE('',*,*,#22977,.F.);
#39081=ORIENTED_EDGE('',*,*,#22969,.F.);
#39082=ORIENTED_EDGE('',*,*,#22966,.F.);
#39083=ORIENTED_EDGE('',*,*,#23078,.F.);
#39084=ORIENTED_EDGE('',*,*,#23086,.F.);
#39085=ORIENTED_EDGE('',*,*,#27146,.T.);
#39086=ORIENTED_EDGE('',*,*,#23075,.F.);
#39087=ORIENTED_EDGE('',*,*,#27146,.F.);
#39088=ORIENTED_EDGE('',*,*,#23082,.F.);
#39089=ORIENTED_EDGE('',*,*,#22974,.F.);
#39090=ORIENTED_EDGE('',*,*,#27145,.T.);
#39091=ORIENTED_EDGE('',*,*,#22961,.F.);
#39092=ORIENTED_EDGE('',*,*,#23067,.F.);
#39093=ORIENTED_EDGE('',*,*,#27147,.F.);
#39094=ORIENTED_EDGE('',*,*,#22963,.F.);
#39095=ORIENTED_EDGE('',*,*,#22955,.F.);
#39096=ORIENTED_EDGE('',*,*,#22952,.F.);
#39097=ORIENTED_EDGE('',*,*,#23064,.F.);
#39098=ORIENTED_EDGE('',*,*,#23072,.F.);
#39099=ORIENTED_EDGE('',*,*,#27148,.T.);
#39100=ORIENTED_EDGE('',*,*,#23061,.F.);
#39101=ORIENTED_EDGE('',*,*,#27148,.F.);
#39102=ORIENTED_EDGE('',*,*,#23068,.F.);
#39103=ORIENTED_EDGE('',*,*,#22960,.F.);
#39104=ORIENTED_EDGE('',*,*,#27147,.T.);
#39105=ORIENTED_EDGE('',*,*,#22946,.F.);
#39106=ORIENTED_EDGE('',*,*,#23053,.F.);
#39107=ORIENTED_EDGE('',*,*,#27149,.F.);
#39108=ORIENTED_EDGE('',*,*,#22948,.F.);
#39109=ORIENTED_EDGE('',*,*,#22940,.F.);
#39110=ORIENTED_EDGE('',*,*,#22937,.F.);
#39111=ORIENTED_EDGE('',*,*,#23050,.F.);
#39112=ORIENTED_EDGE('',*,*,#23058,.F.);
#39113=ORIENTED_EDGE('',*,*,#27150,.T.);
#39114=ORIENTED_EDGE('',*,*,#23047,.F.);
#39115=ORIENTED_EDGE('',*,*,#27150,.F.);
#39116=ORIENTED_EDGE('',*,*,#23054,.F.);
#39117=ORIENTED_EDGE('',*,*,#22945,.F.);
#39118=ORIENTED_EDGE('',*,*,#27149,.T.);
#39119=ORIENTED_EDGE('',*,*,#22934,.F.);
#39120=ORIENTED_EDGE('',*,*,#23038,.F.);
#39121=ORIENTED_EDGE('',*,*,#23027,.F.);
#39122=ORIENTED_EDGE('',*,*,#27151,.F.);
#39123=ORIENTED_EDGE('',*,*,#23039,.F.);
#39124=ORIENTED_EDGE('',*,*,#22933,.F.);
#39125=ORIENTED_EDGE('',*,*,#27152,.T.);
#39126=ORIENTED_EDGE('',*,*,#21424,.F.);
#39127=ORIENTED_EDGE('',*,*,#23035,.F.);
#39128=ORIENTED_EDGE('',*,*,#23043,.F.);
#39129=ORIENTED_EDGE('',*,*,#27151,.T.);
#39130=ORIENTED_EDGE('',*,*,#23032,.F.);
#39131=ORIENTED_EDGE('',*,*,#27152,.F.);
#39132=ORIENTED_EDGE('',*,*,#23045,.F.);
#39133=ORIENTED_EDGE('',*,*,#21425,.F.);
#39134=ORIENTED_EDGE('',*,*,#22925,.F.);
#39135=ORIENTED_EDGE('',*,*,#27153,.F.);
#39136=ORIENTED_EDGE('',*,*,#21689,.F.);
#39137=ORIENTED_EDGE('',*,*,#27153,.T.);
#39138=ORIENTED_EDGE('',*,*,#22921,.F.);
#39139=ORIENTED_EDGE('',*,*,#23022,.F.);
#39140=ORIENTED_EDGE('',*,*,#21690,.F.);
#39141=ORIENTED_EDGE('',*,*,#27154,.F.);
#39142=ORIENTED_EDGE('',*,*,#22923,.F.);
#39143=ORIENTED_EDGE('',*,*,#22915,.F.);
#39144=ORIENTED_EDGE('',*,*,#22912,.F.);
#39145=ORIENTED_EDGE('',*,*,#21693,.F.);
#39146=ORIENTED_EDGE('',*,*,#23025,.F.);
#39147=ORIENTED_EDGE('',*,*,#27155,.T.);
#39148=ORIENTED_EDGE('',*,*,#23020,.F.);
#39149=ORIENTED_EDGE('',*,*,#27155,.F.);
#39150=ORIENTED_EDGE('',*,*,#23023,.F.);
#39151=ORIENTED_EDGE('',*,*,#22920,.F.);
#39152=ORIENTED_EDGE('',*,*,#27154,.T.);
#39153=ORIENTED_EDGE('',*,*,#22907,.F.);
#39154=ORIENTED_EDGE('',*,*,#23013,.F.);
#39155=ORIENTED_EDGE('',*,*,#27156,.F.);
#39156=ORIENTED_EDGE('',*,*,#22909,.F.);
#39157=ORIENTED_EDGE('',*,*,#22901,.F.);
#39158=ORIENTED_EDGE('',*,*,#22898,.F.);
#39159=ORIENTED_EDGE('',*,*,#23010,.F.);
#39160=ORIENTED_EDGE('',*,*,#23018,.F.);
#39161=ORIENTED_EDGE('',*,*,#27157,.T.);
#39162=ORIENTED_EDGE('',*,*,#23007,.F.);
#39163=ORIENTED_EDGE('',*,*,#27157,.F.);
#39164=ORIENTED_EDGE('',*,*,#23014,.F.);
#39165=ORIENTED_EDGE('',*,*,#22906,.F.);
#39166=ORIENTED_EDGE('',*,*,#27156,.T.);
#39167=ORIENTED_EDGE('',*,*,#22893,.F.);
#39168=ORIENTED_EDGE('',*,*,#22999,.F.);
#39169=ORIENTED_EDGE('',*,*,#27158,.F.);
#39170=ORIENTED_EDGE('',*,*,#22895,.F.);
#39171=ORIENTED_EDGE('',*,*,#22887,.F.);
#39172=ORIENTED_EDGE('',*,*,#22884,.F.);
#39173=ORIENTED_EDGE('',*,*,#22996,.F.);
#39174=ORIENTED_EDGE('',*,*,#23004,.F.);
#39175=ORIENTED_EDGE('',*,*,#27159,.T.);
#39176=ORIENTED_EDGE('',*,*,#22993,.F.);
#39177=ORIENTED_EDGE('',*,*,#27159,.F.);
#39178=ORIENTED_EDGE('',*,*,#23000,.F.);
#39179=ORIENTED_EDGE('',*,*,#22892,.F.);
#39180=ORIENTED_EDGE('',*,*,#27158,.T.);
#39181=ORIENTED_EDGE('',*,*,#22879,.F.);
#39182=ORIENTED_EDGE('',*,*,#22985,.F.);
#39183=ORIENTED_EDGE('',*,*,#27160,.F.);
#39184=ORIENTED_EDGE('',*,*,#22881,.F.);
#39185=ORIENTED_EDGE('',*,*,#22873,.F.);
#39186=ORIENTED_EDGE('',*,*,#22870,.F.);
#39187=ORIENTED_EDGE('',*,*,#22982,.F.);
#39188=ORIENTED_EDGE('',*,*,#22990,.F.);
#39189=ORIENTED_EDGE('',*,*,#27161,.T.);
#39190=ORIENTED_EDGE('',*,*,#22979,.F.);
#39191=ORIENTED_EDGE('',*,*,#27161,.F.);
#39192=ORIENTED_EDGE('',*,*,#22986,.F.);
#39193=ORIENTED_EDGE('',*,*,#22878,.F.);
#39194=ORIENTED_EDGE('',*,*,#27160,.T.);
#39195=ORIENTED_EDGE('',*,*,#22865,.F.);
#39196=ORIENTED_EDGE('',*,*,#22971,.F.);
#39197=ORIENTED_EDGE('',*,*,#27162,.F.);
#39198=ORIENTED_EDGE('',*,*,#22867,.F.);
#39199=ORIENTED_EDGE('',*,*,#22859,.F.);
#39200=ORIENTED_EDGE('',*,*,#22856,.F.);
#39201=ORIENTED_EDGE('',*,*,#22968,.F.);
#39202=ORIENTED_EDGE('',*,*,#22976,.F.);
#39203=ORIENTED_EDGE('',*,*,#27163,.T.);
#39204=ORIENTED_EDGE('',*,*,#22965,.F.);
#39205=ORIENTED_EDGE('',*,*,#27163,.F.);
#39206=ORIENTED_EDGE('',*,*,#22972,.F.);
#39207=ORIENTED_EDGE('',*,*,#22864,.F.);
#39208=ORIENTED_EDGE('',*,*,#27162,.T.);
#39209=ORIENTED_EDGE('',*,*,#22850,.F.);
#39210=ORIENTED_EDGE('',*,*,#22957,.F.);
#39211=ORIENTED_EDGE('',*,*,#27164,.F.);
#39212=ORIENTED_EDGE('',*,*,#22852,.F.);
#39213=ORIENTED_EDGE('',*,*,#22844,.F.);
#39214=ORIENTED_EDGE('',*,*,#22841,.F.);
#39215=ORIENTED_EDGE('',*,*,#22954,.F.);
#39216=ORIENTED_EDGE('',*,*,#22962,.F.);
#39217=ORIENTED_EDGE('',*,*,#27165,.T.);
#39218=ORIENTED_EDGE('',*,*,#22951,.F.);
#39219=ORIENTED_EDGE('',*,*,#27165,.F.);
#39220=ORIENTED_EDGE('',*,*,#22958,.F.);
#39221=ORIENTED_EDGE('',*,*,#22849,.F.);
#39222=ORIENTED_EDGE('',*,*,#27164,.T.);
#39223=ORIENTED_EDGE('',*,*,#22838,.F.);
#39224=ORIENTED_EDGE('',*,*,#22942,.F.);
#39225=ORIENTED_EDGE('',*,*,#22931,.F.);
#39226=ORIENTED_EDGE('',*,*,#27166,.F.);
#39227=ORIENTED_EDGE('',*,*,#22943,.F.);
#39228=ORIENTED_EDGE('',*,*,#22837,.F.);
#39229=ORIENTED_EDGE('',*,*,#27167,.T.);
#39230=ORIENTED_EDGE('',*,*,#21428,.F.);
#39231=ORIENTED_EDGE('',*,*,#22939,.F.);
#39232=ORIENTED_EDGE('',*,*,#22947,.F.);
#39233=ORIENTED_EDGE('',*,*,#27166,.T.);
#39234=ORIENTED_EDGE('',*,*,#22936,.F.);
#39235=ORIENTED_EDGE('',*,*,#27167,.F.);
#39236=ORIENTED_EDGE('',*,*,#22949,.F.);
#39237=ORIENTED_EDGE('',*,*,#21429,.F.);
#39238=ORIENTED_EDGE('',*,*,#22829,.F.);
#39239=ORIENTED_EDGE('',*,*,#27168,.F.);
#39240=ORIENTED_EDGE('',*,*,#21683,.F.);
#39241=ORIENTED_EDGE('',*,*,#27168,.T.);
#39242=ORIENTED_EDGE('',*,*,#22825,.F.);
#39243=ORIENTED_EDGE('',*,*,#22926,.F.);
#39244=ORIENTED_EDGE('',*,*,#21684,.F.);
#39245=ORIENTED_EDGE('',*,*,#27169,.F.);
#39246=ORIENTED_EDGE('',*,*,#22827,.F.);
#39247=ORIENTED_EDGE('',*,*,#22819,.F.);
#39248=ORIENTED_EDGE('',*,*,#22816,.F.);
#39249=ORIENTED_EDGE('',*,*,#21687,.F.);
#39250=ORIENTED_EDGE('',*,*,#22929,.F.);
#39251=ORIENTED_EDGE('',*,*,#27170,.T.);
#39252=ORIENTED_EDGE('',*,*,#22924,.F.);
#39253=ORIENTED_EDGE('',*,*,#27170,.F.);
#39254=ORIENTED_EDGE('',*,*,#22927,.F.);
#39255=ORIENTED_EDGE('',*,*,#22824,.F.);
#39256=ORIENTED_EDGE('',*,*,#27169,.T.);
#39257=ORIENTED_EDGE('',*,*,#22811,.F.);
#39258=ORIENTED_EDGE('',*,*,#22917,.F.);
#39259=ORIENTED_EDGE('',*,*,#27171,.F.);
#39260=ORIENTED_EDGE('',*,*,#22813,.F.);
#39261=ORIENTED_EDGE('',*,*,#22805,.F.);
#39262=ORIENTED_EDGE('',*,*,#22802,.F.);
#39263=ORIENTED_EDGE('',*,*,#22914,.F.);
#39264=ORIENTED_EDGE('',*,*,#22922,.F.);
#39265=ORIENTED_EDGE('',*,*,#27172,.T.);
#39266=ORIENTED_EDGE('',*,*,#22911,.F.);
#39267=ORIENTED_EDGE('',*,*,#27172,.F.);
#39268=ORIENTED_EDGE('',*,*,#22918,.F.);
#39269=ORIENTED_EDGE('',*,*,#22810,.F.);
#39270=ORIENTED_EDGE('',*,*,#27171,.T.);
#39271=ORIENTED_EDGE('',*,*,#22797,.F.);
#39272=ORIENTED_EDGE('',*,*,#22903,.F.);
#39273=ORIENTED_EDGE('',*,*,#27173,.F.);
#39274=ORIENTED_EDGE('',*,*,#22799,.F.);
#39275=ORIENTED_EDGE('',*,*,#22791,.F.);
#39276=ORIENTED_EDGE('',*,*,#22788,.F.);
#39277=ORIENTED_EDGE('',*,*,#22900,.F.);
#39278=ORIENTED_EDGE('',*,*,#22908,.F.);
#39279=ORIENTED_EDGE('',*,*,#27174,.T.);
#39280=ORIENTED_EDGE('',*,*,#22897,.F.);
#39281=ORIENTED_EDGE('',*,*,#27174,.F.);
#39282=ORIENTED_EDGE('',*,*,#22904,.F.);
#39283=ORIENTED_EDGE('',*,*,#22796,.F.);
#39284=ORIENTED_EDGE('',*,*,#27173,.T.);
#39285=ORIENTED_EDGE('',*,*,#22783,.F.);
#39286=ORIENTED_EDGE('',*,*,#22889,.F.);
#39287=ORIENTED_EDGE('',*,*,#27175,.F.);
#39288=ORIENTED_EDGE('',*,*,#22785,.F.);
#39289=ORIENTED_EDGE('',*,*,#22777,.F.);
#39290=ORIENTED_EDGE('',*,*,#22774,.F.);
#39291=ORIENTED_EDGE('',*,*,#22886,.F.);
#39292=ORIENTED_EDGE('',*,*,#22894,.F.);
#39293=ORIENTED_EDGE('',*,*,#27176,.T.);
#39294=ORIENTED_EDGE('',*,*,#22883,.F.);
#39295=ORIENTED_EDGE('',*,*,#27176,.F.);
#39296=ORIENTED_EDGE('',*,*,#22890,.F.);
#39297=ORIENTED_EDGE('',*,*,#22782,.F.);
#39298=ORIENTED_EDGE('',*,*,#27175,.T.);
#39299=ORIENTED_EDGE('',*,*,#22769,.F.);
#39300=ORIENTED_EDGE('',*,*,#22875,.F.);
#39301=ORIENTED_EDGE('',*,*,#27177,.F.);
#39302=ORIENTED_EDGE('',*,*,#22771,.F.);
#39303=ORIENTED_EDGE('',*,*,#22763,.F.);
#39304=ORIENTED_EDGE('',*,*,#22760,.F.);
#39305=ORIENTED_EDGE('',*,*,#22872,.F.);
#39306=ORIENTED_EDGE('',*,*,#22880,.F.);
#39307=ORIENTED_EDGE('',*,*,#27178,.T.);
#39308=ORIENTED_EDGE('',*,*,#22869,.F.);
#39309=ORIENTED_EDGE('',*,*,#27178,.F.);
#39310=ORIENTED_EDGE('',*,*,#22876,.F.);
#39311=ORIENTED_EDGE('',*,*,#22768,.F.);
#39312=ORIENTED_EDGE('',*,*,#27177,.T.);
#39313=ORIENTED_EDGE('',*,*,#22754,.F.);
#39314=ORIENTED_EDGE('',*,*,#22861,.F.);
#39315=ORIENTED_EDGE('',*,*,#27179,.F.);
#39316=ORIENTED_EDGE('',*,*,#22756,.F.);
#39317=ORIENTED_EDGE('',*,*,#22748,.F.);
#39318=ORIENTED_EDGE('',*,*,#22745,.F.);
#39319=ORIENTED_EDGE('',*,*,#22858,.F.);
#39320=ORIENTED_EDGE('',*,*,#22866,.F.);
#39321=ORIENTED_EDGE('',*,*,#27180,.T.);
#39322=ORIENTED_EDGE('',*,*,#22855,.F.);
#39323=ORIENTED_EDGE('',*,*,#27180,.F.);
#39324=ORIENTED_EDGE('',*,*,#22862,.F.);
#39325=ORIENTED_EDGE('',*,*,#22753,.F.);
#39326=ORIENTED_EDGE('',*,*,#27179,.T.);
#39327=ORIENTED_EDGE('',*,*,#22742,.F.);
#39328=ORIENTED_EDGE('',*,*,#22846,.F.);
#39329=ORIENTED_EDGE('',*,*,#22835,.F.);
#39330=ORIENTED_EDGE('',*,*,#27181,.F.);
#39331=ORIENTED_EDGE('',*,*,#22847,.F.);
#39332=ORIENTED_EDGE('',*,*,#22741,.F.);
#39333=ORIENTED_EDGE('',*,*,#27182,.T.);
#39334=ORIENTED_EDGE('',*,*,#21432,.F.);
#39335=ORIENTED_EDGE('',*,*,#22843,.F.);
#39336=ORIENTED_EDGE('',*,*,#22851,.F.);
#39337=ORIENTED_EDGE('',*,*,#27181,.T.);
#39338=ORIENTED_EDGE('',*,*,#22840,.F.);
#39339=ORIENTED_EDGE('',*,*,#27182,.F.);
#39340=ORIENTED_EDGE('',*,*,#22853,.F.);
#39341=ORIENTED_EDGE('',*,*,#21433,.F.);
#39342=ORIENTED_EDGE('',*,*,#22733,.F.);
#39343=ORIENTED_EDGE('',*,*,#27183,.F.);
#39344=ORIENTED_EDGE('',*,*,#21677,.F.);
#39345=ORIENTED_EDGE('',*,*,#27183,.T.);
#39346=ORIENTED_EDGE('',*,*,#22729,.F.);
#39347=ORIENTED_EDGE('',*,*,#22830,.F.);
#39348=ORIENTED_EDGE('',*,*,#21678,.F.);
#39349=ORIENTED_EDGE('',*,*,#27184,.F.);
#39350=ORIENTED_EDGE('',*,*,#22731,.F.);
#39351=ORIENTED_EDGE('',*,*,#22723,.F.);
#39352=ORIENTED_EDGE('',*,*,#22720,.F.);
#39353=ORIENTED_EDGE('',*,*,#21681,.F.);
#39354=ORIENTED_EDGE('',*,*,#22833,.F.);
#39355=ORIENTED_EDGE('',*,*,#27185,.T.);
#39356=ORIENTED_EDGE('',*,*,#22828,.F.);
#39357=ORIENTED_EDGE('',*,*,#27185,.F.);
#39358=ORIENTED_EDGE('',*,*,#22831,.F.);
#39359=ORIENTED_EDGE('',*,*,#22728,.F.);
#39360=ORIENTED_EDGE('',*,*,#27184,.T.);
#39361=ORIENTED_EDGE('',*,*,#22715,.F.);
#39362=ORIENTED_EDGE('',*,*,#22821,.F.);
#39363=ORIENTED_EDGE('',*,*,#27186,.F.);
#39364=ORIENTED_EDGE('',*,*,#22717,.F.);
#39365=ORIENTED_EDGE('',*,*,#22709,.F.);
#39366=ORIENTED_EDGE('',*,*,#22706,.F.);
#39367=ORIENTED_EDGE('',*,*,#22818,.F.);
#39368=ORIENTED_EDGE('',*,*,#22826,.F.);
#39369=ORIENTED_EDGE('',*,*,#27187,.T.);
#39370=ORIENTED_EDGE('',*,*,#22815,.F.);
#39371=ORIENTED_EDGE('',*,*,#27187,.F.);
#39372=ORIENTED_EDGE('',*,*,#22822,.F.);
#39373=ORIENTED_EDGE('',*,*,#22714,.F.);
#39374=ORIENTED_EDGE('',*,*,#27186,.T.);
#39375=ORIENTED_EDGE('',*,*,#22701,.F.);
#39376=ORIENTED_EDGE('',*,*,#22807,.F.);
#39377=ORIENTED_EDGE('',*,*,#27188,.F.);
#39378=ORIENTED_EDGE('',*,*,#22703,.F.);
#39379=ORIENTED_EDGE('',*,*,#22695,.F.);
#39380=ORIENTED_EDGE('',*,*,#22692,.F.);
#39381=ORIENTED_EDGE('',*,*,#22804,.F.);
#39382=ORIENTED_EDGE('',*,*,#22812,.F.);
#39383=ORIENTED_EDGE('',*,*,#27189,.T.);
#39384=ORIENTED_EDGE('',*,*,#22801,.F.);
#39385=ORIENTED_EDGE('',*,*,#27189,.F.);
#39386=ORIENTED_EDGE('',*,*,#22808,.F.);
#39387=ORIENTED_EDGE('',*,*,#22700,.F.);
#39388=ORIENTED_EDGE('',*,*,#27188,.T.);
#39389=ORIENTED_EDGE('',*,*,#22687,.F.);
#39390=ORIENTED_EDGE('',*,*,#22793,.F.);
#39391=ORIENTED_EDGE('',*,*,#27190,.F.);
#39392=ORIENTED_EDGE('',*,*,#22689,.F.);
#39393=ORIENTED_EDGE('',*,*,#22681,.F.);
#39394=ORIENTED_EDGE('',*,*,#22678,.F.);
#39395=ORIENTED_EDGE('',*,*,#22790,.F.);
#39396=ORIENTED_EDGE('',*,*,#22798,.F.);
#39397=ORIENTED_EDGE('',*,*,#27191,.T.);
#39398=ORIENTED_EDGE('',*,*,#22787,.F.);
#39399=ORIENTED_EDGE('',*,*,#27191,.F.);
#39400=ORIENTED_EDGE('',*,*,#22794,.F.);
#39401=ORIENTED_EDGE('',*,*,#22686,.F.);
#39402=ORIENTED_EDGE('',*,*,#27190,.T.);
#39403=ORIENTED_EDGE('',*,*,#22673,.F.);
#39404=ORIENTED_EDGE('',*,*,#22779,.F.);
#39405=ORIENTED_EDGE('',*,*,#27192,.F.);
#39406=ORIENTED_EDGE('',*,*,#22675,.F.);
#39407=ORIENTED_EDGE('',*,*,#22667,.F.);
#39408=ORIENTED_EDGE('',*,*,#22664,.F.);
#39409=ORIENTED_EDGE('',*,*,#22776,.F.);
#39410=ORIENTED_EDGE('',*,*,#22784,.F.);
#39411=ORIENTED_EDGE('',*,*,#27193,.T.);
#39412=ORIENTED_EDGE('',*,*,#22773,.F.);
#39413=ORIENTED_EDGE('',*,*,#27193,.F.);
#39414=ORIENTED_EDGE('',*,*,#22780,.F.);
#39415=ORIENTED_EDGE('',*,*,#22672,.F.);
#39416=ORIENTED_EDGE('',*,*,#27192,.T.);
#39417=ORIENTED_EDGE('',*,*,#22658,.F.);
#39418=ORIENTED_EDGE('',*,*,#22765,.F.);
#39419=ORIENTED_EDGE('',*,*,#27194,.F.);
#39420=ORIENTED_EDGE('',*,*,#22660,.F.);
#39421=ORIENTED_EDGE('',*,*,#22652,.F.);
#39422=ORIENTED_EDGE('',*,*,#22649,.F.);
#39423=ORIENTED_EDGE('',*,*,#22762,.F.);
#39424=ORIENTED_EDGE('',*,*,#22770,.F.);
#39425=ORIENTED_EDGE('',*,*,#27195,.T.);
#39426=ORIENTED_EDGE('',*,*,#22759,.F.);
#39427=ORIENTED_EDGE('',*,*,#27195,.F.);
#39428=ORIENTED_EDGE('',*,*,#22766,.F.);
#39429=ORIENTED_EDGE('',*,*,#22657,.F.);
#39430=ORIENTED_EDGE('',*,*,#27194,.T.);
#39431=ORIENTED_EDGE('',*,*,#22646,.F.);
#39432=ORIENTED_EDGE('',*,*,#22750,.F.);
#39433=ORIENTED_EDGE('',*,*,#22739,.F.);
#39434=ORIENTED_EDGE('',*,*,#27196,.F.);
#39435=ORIENTED_EDGE('',*,*,#22751,.F.);
#39436=ORIENTED_EDGE('',*,*,#22645,.F.);
#39437=ORIENTED_EDGE('',*,*,#27197,.T.);
#39438=ORIENTED_EDGE('',*,*,#21436,.F.);
#39439=ORIENTED_EDGE('',*,*,#22747,.F.);
#39440=ORIENTED_EDGE('',*,*,#22755,.F.);
#39441=ORIENTED_EDGE('',*,*,#27196,.T.);
#39442=ORIENTED_EDGE('',*,*,#22744,.F.);
#39443=ORIENTED_EDGE('',*,*,#27197,.F.);
#39444=ORIENTED_EDGE('',*,*,#22757,.F.);
#39445=ORIENTED_EDGE('',*,*,#21437,.F.);
#39446=ORIENTED_EDGE('',*,*,#22637,.F.);
#39447=ORIENTED_EDGE('',*,*,#27198,.F.);
#39448=ORIENTED_EDGE('',*,*,#21671,.F.);
#39449=ORIENTED_EDGE('',*,*,#27198,.T.);
#39450=ORIENTED_EDGE('',*,*,#22633,.F.);
#39451=ORIENTED_EDGE('',*,*,#22734,.F.);
#39452=ORIENTED_EDGE('',*,*,#21672,.F.);
#39453=ORIENTED_EDGE('',*,*,#27199,.F.);
#39454=ORIENTED_EDGE('',*,*,#22635,.F.);
#39455=ORIENTED_EDGE('',*,*,#22627,.F.);
#39456=ORIENTED_EDGE('',*,*,#22624,.F.);
#39457=ORIENTED_EDGE('',*,*,#21675,.F.);
#39458=ORIENTED_EDGE('',*,*,#22737,.F.);
#39459=ORIENTED_EDGE('',*,*,#27200,.T.);
#39460=ORIENTED_EDGE('',*,*,#22732,.F.);
#39461=ORIENTED_EDGE('',*,*,#27200,.F.);
#39462=ORIENTED_EDGE('',*,*,#22735,.F.);
#39463=ORIENTED_EDGE('',*,*,#22632,.F.);
#39464=ORIENTED_EDGE('',*,*,#27199,.T.);
#39465=ORIENTED_EDGE('',*,*,#22619,.F.);
#39466=ORIENTED_EDGE('',*,*,#22725,.F.);
#39467=ORIENTED_EDGE('',*,*,#27201,.F.);
#39468=ORIENTED_EDGE('',*,*,#22621,.F.);
#39469=ORIENTED_EDGE('',*,*,#22613,.F.);
#39470=ORIENTED_EDGE('',*,*,#22610,.F.);
#39471=ORIENTED_EDGE('',*,*,#22722,.F.);
#39472=ORIENTED_EDGE('',*,*,#22730,.F.);
#39473=ORIENTED_EDGE('',*,*,#27202,.T.);
#39474=ORIENTED_EDGE('',*,*,#22719,.F.);
#39475=ORIENTED_EDGE('',*,*,#27202,.F.);
#39476=ORIENTED_EDGE('',*,*,#22726,.F.);
#39477=ORIENTED_EDGE('',*,*,#22618,.F.);
#39478=ORIENTED_EDGE('',*,*,#27201,.T.);
#39479=ORIENTED_EDGE('',*,*,#22605,.F.);
#39480=ORIENTED_EDGE('',*,*,#22711,.F.);
#39481=ORIENTED_EDGE('',*,*,#27203,.F.);
#39482=ORIENTED_EDGE('',*,*,#22607,.F.);
#39483=ORIENTED_EDGE('',*,*,#22599,.F.);
#39484=ORIENTED_EDGE('',*,*,#22596,.F.);
#39485=ORIENTED_EDGE('',*,*,#22708,.F.);
#39486=ORIENTED_EDGE('',*,*,#22716,.F.);
#39487=ORIENTED_EDGE('',*,*,#27204,.T.);
#39488=ORIENTED_EDGE('',*,*,#22705,.F.);
#39489=ORIENTED_EDGE('',*,*,#27204,.F.);
#39490=ORIENTED_EDGE('',*,*,#22712,.F.);
#39491=ORIENTED_EDGE('',*,*,#22604,.F.);
#39492=ORIENTED_EDGE('',*,*,#27203,.T.);
#39493=ORIENTED_EDGE('',*,*,#22591,.F.);
#39494=ORIENTED_EDGE('',*,*,#22697,.F.);
#39495=ORIENTED_EDGE('',*,*,#27205,.F.);
#39496=ORIENTED_EDGE('',*,*,#22593,.F.);
#39497=ORIENTED_EDGE('',*,*,#22585,.F.);
#39498=ORIENTED_EDGE('',*,*,#22582,.F.);
#39499=ORIENTED_EDGE('',*,*,#22694,.F.);
#39500=ORIENTED_EDGE('',*,*,#22702,.F.);
#39501=ORIENTED_EDGE('',*,*,#27206,.T.);
#39502=ORIENTED_EDGE('',*,*,#22691,.F.);
#39503=ORIENTED_EDGE('',*,*,#27206,.F.);
#39504=ORIENTED_EDGE('',*,*,#22698,.F.);
#39505=ORIENTED_EDGE('',*,*,#22590,.F.);
#39506=ORIENTED_EDGE('',*,*,#27205,.T.);
#39507=ORIENTED_EDGE('',*,*,#22577,.F.);
#39508=ORIENTED_EDGE('',*,*,#22683,.F.);
#39509=ORIENTED_EDGE('',*,*,#27207,.F.);
#39510=ORIENTED_EDGE('',*,*,#22579,.F.);
#39511=ORIENTED_EDGE('',*,*,#22571,.F.);
#39512=ORIENTED_EDGE('',*,*,#22568,.F.);
#39513=ORIENTED_EDGE('',*,*,#22680,.F.);
#39514=ORIENTED_EDGE('',*,*,#22688,.F.);
#39515=ORIENTED_EDGE('',*,*,#27208,.T.);
#39516=ORIENTED_EDGE('',*,*,#22677,.F.);
#39517=ORIENTED_EDGE('',*,*,#27208,.F.);
#39518=ORIENTED_EDGE('',*,*,#22684,.F.);
#39519=ORIENTED_EDGE('',*,*,#22576,.F.);
#39520=ORIENTED_EDGE('',*,*,#27207,.T.);
#39521=ORIENTED_EDGE('',*,*,#22562,.F.);
#39522=ORIENTED_EDGE('',*,*,#22669,.F.);
#39523=ORIENTED_EDGE('',*,*,#27209,.F.);
#39524=ORIENTED_EDGE('',*,*,#22564,.F.);
#39525=ORIENTED_EDGE('',*,*,#22556,.F.);
#39526=ORIENTED_EDGE('',*,*,#22553,.F.);
#39527=ORIENTED_EDGE('',*,*,#22666,.F.);
#39528=ORIENTED_EDGE('',*,*,#22674,.F.);
#39529=ORIENTED_EDGE('',*,*,#27210,.T.);
#39530=ORIENTED_EDGE('',*,*,#22663,.F.);
#39531=ORIENTED_EDGE('',*,*,#27210,.F.);
#39532=ORIENTED_EDGE('',*,*,#22670,.F.);
#39533=ORIENTED_EDGE('',*,*,#22561,.F.);
#39534=ORIENTED_EDGE('',*,*,#27209,.T.);
#39535=ORIENTED_EDGE('',*,*,#22550,.F.);
#39536=ORIENTED_EDGE('',*,*,#22654,.F.);
#39537=ORIENTED_EDGE('',*,*,#22643,.F.);
#39538=ORIENTED_EDGE('',*,*,#27211,.F.);
#39539=ORIENTED_EDGE('',*,*,#22655,.F.);
#39540=ORIENTED_EDGE('',*,*,#22549,.F.);
#39541=ORIENTED_EDGE('',*,*,#27212,.T.);
#39542=ORIENTED_EDGE('',*,*,#21440,.F.);
#39543=ORIENTED_EDGE('',*,*,#22651,.F.);
#39544=ORIENTED_EDGE('',*,*,#22659,.F.);
#39545=ORIENTED_EDGE('',*,*,#27211,.T.);
#39546=ORIENTED_EDGE('',*,*,#22648,.F.);
#39547=ORIENTED_EDGE('',*,*,#27212,.F.);
#39548=ORIENTED_EDGE('',*,*,#22661,.F.);
#39549=ORIENTED_EDGE('',*,*,#21441,.F.);
#39550=ORIENTED_EDGE('',*,*,#22541,.F.);
#39551=ORIENTED_EDGE('',*,*,#27213,.F.);
#39552=ORIENTED_EDGE('',*,*,#21665,.F.);
#39553=ORIENTED_EDGE('',*,*,#27213,.T.);
#39554=ORIENTED_EDGE('',*,*,#22537,.F.);
#39555=ORIENTED_EDGE('',*,*,#22638,.F.);
#39556=ORIENTED_EDGE('',*,*,#21666,.F.);
#39557=ORIENTED_EDGE('',*,*,#27214,.F.);
#39558=ORIENTED_EDGE('',*,*,#22539,.F.);
#39559=ORIENTED_EDGE('',*,*,#22531,.F.);
#39560=ORIENTED_EDGE('',*,*,#22528,.F.);
#39561=ORIENTED_EDGE('',*,*,#21669,.F.);
#39562=ORIENTED_EDGE('',*,*,#22641,.F.);
#39563=ORIENTED_EDGE('',*,*,#27215,.T.);
#39564=ORIENTED_EDGE('',*,*,#22636,.F.);
#39565=ORIENTED_EDGE('',*,*,#27215,.F.);
#39566=ORIENTED_EDGE('',*,*,#22639,.F.);
#39567=ORIENTED_EDGE('',*,*,#22536,.F.);
#39568=ORIENTED_EDGE('',*,*,#27214,.T.);
#39569=ORIENTED_EDGE('',*,*,#22523,.F.);
#39570=ORIENTED_EDGE('',*,*,#22629,.F.);
#39571=ORIENTED_EDGE('',*,*,#27216,.F.);
#39572=ORIENTED_EDGE('',*,*,#22525,.F.);
#39573=ORIENTED_EDGE('',*,*,#22517,.F.);
#39574=ORIENTED_EDGE('',*,*,#22514,.F.);
#39575=ORIENTED_EDGE('',*,*,#22626,.F.);
#39576=ORIENTED_EDGE('',*,*,#22634,.F.);
#39577=ORIENTED_EDGE('',*,*,#27217,.T.);
#39578=ORIENTED_EDGE('',*,*,#22623,.F.);
#39579=ORIENTED_EDGE('',*,*,#27217,.F.);
#39580=ORIENTED_EDGE('',*,*,#22630,.F.);
#39581=ORIENTED_EDGE('',*,*,#22522,.F.);
#39582=ORIENTED_EDGE('',*,*,#27216,.T.);
#39583=ORIENTED_EDGE('',*,*,#22509,.F.);
#39584=ORIENTED_EDGE('',*,*,#22615,.F.);
#39585=ORIENTED_EDGE('',*,*,#27218,.F.);
#39586=ORIENTED_EDGE('',*,*,#22511,.F.);
#39587=ORIENTED_EDGE('',*,*,#22503,.F.);
#39588=ORIENTED_EDGE('',*,*,#22500,.F.);
#39589=ORIENTED_EDGE('',*,*,#22612,.F.);
#39590=ORIENTED_EDGE('',*,*,#22620,.F.);
#39591=ORIENTED_EDGE('',*,*,#27219,.T.);
#39592=ORIENTED_EDGE('',*,*,#22609,.F.);
#39593=ORIENTED_EDGE('',*,*,#27219,.F.);
#39594=ORIENTED_EDGE('',*,*,#22616,.F.);
#39595=ORIENTED_EDGE('',*,*,#22508,.F.);
#39596=ORIENTED_EDGE('',*,*,#27218,.T.);
#39597=ORIENTED_EDGE('',*,*,#22495,.F.);
#39598=ORIENTED_EDGE('',*,*,#22601,.F.);
#39599=ORIENTED_EDGE('',*,*,#27220,.F.);
#39600=ORIENTED_EDGE('',*,*,#22497,.F.);
#39601=ORIENTED_EDGE('',*,*,#22489,.F.);
#39602=ORIENTED_EDGE('',*,*,#22486,.F.);
#39603=ORIENTED_EDGE('',*,*,#22598,.F.);
#39604=ORIENTED_EDGE('',*,*,#22606,.F.);
#39605=ORIENTED_EDGE('',*,*,#27221,.T.);
#39606=ORIENTED_EDGE('',*,*,#22595,.F.);
#39607=ORIENTED_EDGE('',*,*,#27221,.F.);
#39608=ORIENTED_EDGE('',*,*,#22602,.F.);
#39609=ORIENTED_EDGE('',*,*,#22494,.F.);
#39610=ORIENTED_EDGE('',*,*,#27220,.T.);
#39611=ORIENTED_EDGE('',*,*,#22481,.F.);
#39612=ORIENTED_EDGE('',*,*,#22587,.F.);
#39613=ORIENTED_EDGE('',*,*,#27222,.F.);
#39614=ORIENTED_EDGE('',*,*,#22483,.F.);
#39615=ORIENTED_EDGE('',*,*,#22475,.F.);
#39616=ORIENTED_EDGE('',*,*,#22472,.F.);
#39617=ORIENTED_EDGE('',*,*,#22584,.F.);
#39618=ORIENTED_EDGE('',*,*,#22592,.F.);
#39619=ORIENTED_EDGE('',*,*,#27223,.T.);
#39620=ORIENTED_EDGE('',*,*,#22581,.F.);
#39621=ORIENTED_EDGE('',*,*,#27223,.F.);
#39622=ORIENTED_EDGE('',*,*,#22588,.F.);
#39623=ORIENTED_EDGE('',*,*,#22480,.F.);
#39624=ORIENTED_EDGE('',*,*,#27222,.T.);
#39625=ORIENTED_EDGE('',*,*,#22466,.F.);
#39626=ORIENTED_EDGE('',*,*,#22573,.F.);
#39627=ORIENTED_EDGE('',*,*,#27224,.F.);
#39628=ORIENTED_EDGE('',*,*,#22468,.F.);
#39629=ORIENTED_EDGE('',*,*,#22460,.F.);
#39630=ORIENTED_EDGE('',*,*,#22457,.F.);
#39631=ORIENTED_EDGE('',*,*,#22570,.F.);
#39632=ORIENTED_EDGE('',*,*,#22578,.F.);
#39633=ORIENTED_EDGE('',*,*,#27225,.T.);
#39634=ORIENTED_EDGE('',*,*,#22567,.F.);
#39635=ORIENTED_EDGE('',*,*,#27225,.F.);
#39636=ORIENTED_EDGE('',*,*,#22574,.F.);
#39637=ORIENTED_EDGE('',*,*,#22465,.F.);
#39638=ORIENTED_EDGE('',*,*,#27224,.T.);
#39639=ORIENTED_EDGE('',*,*,#22454,.F.);
#39640=ORIENTED_EDGE('',*,*,#22558,.F.);
#39641=ORIENTED_EDGE('',*,*,#22547,.F.);
#39642=ORIENTED_EDGE('',*,*,#27226,.F.);
#39643=ORIENTED_EDGE('',*,*,#22559,.F.);
#39644=ORIENTED_EDGE('',*,*,#22453,.F.);
#39645=ORIENTED_EDGE('',*,*,#27227,.T.);
#39646=ORIENTED_EDGE('',*,*,#21444,.F.);
#39647=ORIENTED_EDGE('',*,*,#22555,.F.);
#39648=ORIENTED_EDGE('',*,*,#22563,.F.);
#39649=ORIENTED_EDGE('',*,*,#27226,.T.);
#39650=ORIENTED_EDGE('',*,*,#22552,.F.);
#39651=ORIENTED_EDGE('',*,*,#27227,.F.);
#39652=ORIENTED_EDGE('',*,*,#22565,.F.);
#39653=ORIENTED_EDGE('',*,*,#21445,.F.);
#39654=ORIENTED_EDGE('',*,*,#27228,.F.);
#39655=ORIENTED_EDGE('',*,*,#22445,.F.);
#39656=ORIENTED_EDGE('',*,*,#22443,.F.);
#39657=ORIENTED_EDGE('',*,*,#22432,.F.);
#39658=ORIENTED_EDGE('',*,*,#21663,.F.);
#39659=ORIENTED_EDGE('',*,*,#22545,.F.);
#39660=ORIENTED_EDGE('',*,*,#27229,.T.);
#39661=ORIENTED_EDGE('',*,*,#22540,.F.);
#39662=ORIENTED_EDGE('',*,*,#27229,.F.);
#39663=ORIENTED_EDGE('',*,*,#22543,.F.);
#39664=ORIENTED_EDGE('',*,*,#22437,.F.);
#39665=ORIENTED_EDGE('',*,*,#27228,.T.);
#39666=ORIENTED_EDGE('',*,*,#22427,.F.);
#39667=ORIENTED_EDGE('',*,*,#22533,.F.);
#39668=ORIENTED_EDGE('',*,*,#22440,.F.);
#39669=ORIENTED_EDGE('',*,*,#27230,.F.);
#39670=ORIENTED_EDGE('',*,*,#21659,.F.);
#39671=ORIENTED_EDGE('',*,*,#27230,.T.);
#39672=ORIENTED_EDGE('',*,*,#22438,.F.);
#39673=ORIENTED_EDGE('',*,*,#22542,.F.);
#39674=ORIENTED_EDGE('',*,*,#21660,.F.);
#39675=ORIENTED_EDGE('',*,*,#27231,.F.);
#39676=ORIENTED_EDGE('',*,*,#22429,.F.);
#39677=ORIENTED_EDGE('',*,*,#22421,.F.);
#39678=ORIENTED_EDGE('',*,*,#22418,.F.);
#39679=ORIENTED_EDGE('',*,*,#22530,.F.);
#39680=ORIENTED_EDGE('',*,*,#22538,.F.);
#39681=ORIENTED_EDGE('',*,*,#27232,.T.);
#39682=ORIENTED_EDGE('',*,*,#22527,.F.);
#39683=ORIENTED_EDGE('',*,*,#27232,.F.);
#39684=ORIENTED_EDGE('',*,*,#22534,.F.);
#39685=ORIENTED_EDGE('',*,*,#22426,.F.);
#39686=ORIENTED_EDGE('',*,*,#27231,.T.);
#39687=ORIENTED_EDGE('',*,*,#22413,.F.);
#39688=ORIENTED_EDGE('',*,*,#22519,.F.);
#39689=ORIENTED_EDGE('',*,*,#27233,.F.);
#39690=ORIENTED_EDGE('',*,*,#22415,.F.);
#39691=ORIENTED_EDGE('',*,*,#22407,.F.);
#39692=ORIENTED_EDGE('',*,*,#22404,.F.);
#39693=ORIENTED_EDGE('',*,*,#22516,.F.);
#39694=ORIENTED_EDGE('',*,*,#22524,.F.);
#39695=ORIENTED_EDGE('',*,*,#27234,.T.);
#39696=ORIENTED_EDGE('',*,*,#22513,.F.);
#39697=ORIENTED_EDGE('',*,*,#27234,.F.);
#39698=ORIENTED_EDGE('',*,*,#22520,.F.);
#39699=ORIENTED_EDGE('',*,*,#22412,.F.);
#39700=ORIENTED_EDGE('',*,*,#27233,.T.);
#39701=ORIENTED_EDGE('',*,*,#22399,.F.);
#39702=ORIENTED_EDGE('',*,*,#22505,.F.);
#39703=ORIENTED_EDGE('',*,*,#27235,.F.);
#39704=ORIENTED_EDGE('',*,*,#22401,.F.);
#39705=ORIENTED_EDGE('',*,*,#22393,.F.);
#39706=ORIENTED_EDGE('',*,*,#22390,.F.);
#39707=ORIENTED_EDGE('',*,*,#22502,.F.);
#39708=ORIENTED_EDGE('',*,*,#22510,.F.);
#39709=ORIENTED_EDGE('',*,*,#27236,.T.);
#39710=ORIENTED_EDGE('',*,*,#22499,.F.);
#39711=ORIENTED_EDGE('',*,*,#27236,.F.);
#39712=ORIENTED_EDGE('',*,*,#22506,.F.);
#39713=ORIENTED_EDGE('',*,*,#22398,.F.);
#39714=ORIENTED_EDGE('',*,*,#27235,.T.);
#39715=ORIENTED_EDGE('',*,*,#22385,.F.);
#39716=ORIENTED_EDGE('',*,*,#22491,.F.);
#39717=ORIENTED_EDGE('',*,*,#27237,.F.);
#39718=ORIENTED_EDGE('',*,*,#22387,.F.);
#39719=ORIENTED_EDGE('',*,*,#22379,.F.);
#39720=ORIENTED_EDGE('',*,*,#22376,.F.);
#39721=ORIENTED_EDGE('',*,*,#22488,.F.);
#39722=ORIENTED_EDGE('',*,*,#22496,.F.);
#39723=ORIENTED_EDGE('',*,*,#27238,.T.);
#39724=ORIENTED_EDGE('',*,*,#22485,.F.);
#39725=ORIENTED_EDGE('',*,*,#27238,.F.);
#39726=ORIENTED_EDGE('',*,*,#22492,.F.);
#39727=ORIENTED_EDGE('',*,*,#22384,.F.);
#39728=ORIENTED_EDGE('',*,*,#27237,.T.);
#39729=ORIENTED_EDGE('',*,*,#22370,.F.);
#39730=ORIENTED_EDGE('',*,*,#22477,.F.);
#39731=ORIENTED_EDGE('',*,*,#27239,.F.);
#39732=ORIENTED_EDGE('',*,*,#22372,.F.);
#39733=ORIENTED_EDGE('',*,*,#22364,.F.);
#39734=ORIENTED_EDGE('',*,*,#22361,.F.);
#39735=ORIENTED_EDGE('',*,*,#22474,.F.);
#39736=ORIENTED_EDGE('',*,*,#22482,.F.);
#39737=ORIENTED_EDGE('',*,*,#27240,.T.);
#39738=ORIENTED_EDGE('',*,*,#22471,.F.);
#39739=ORIENTED_EDGE('',*,*,#27240,.F.);
#39740=ORIENTED_EDGE('',*,*,#22478,.F.);
#39741=ORIENTED_EDGE('',*,*,#22369,.F.);
#39742=ORIENTED_EDGE('',*,*,#27239,.T.);
#39743=ORIENTED_EDGE('',*,*,#22358,.F.);
#39744=ORIENTED_EDGE('',*,*,#22462,.F.);
#39745=ORIENTED_EDGE('',*,*,#22451,.F.);
#39746=ORIENTED_EDGE('',*,*,#27241,.F.);
#39747=ORIENTED_EDGE('',*,*,#22463,.F.);
#39748=ORIENTED_EDGE('',*,*,#22357,.F.);
#39749=ORIENTED_EDGE('',*,*,#27242,.T.);
#39750=ORIENTED_EDGE('',*,*,#21448,.F.);
#39751=ORIENTED_EDGE('',*,*,#22459,.F.);
#39752=ORIENTED_EDGE('',*,*,#22467,.F.);
#39753=ORIENTED_EDGE('',*,*,#27241,.T.);
#39754=ORIENTED_EDGE('',*,*,#22456,.F.);
#39755=ORIENTED_EDGE('',*,*,#27242,.F.);
#39756=ORIENTED_EDGE('',*,*,#22469,.F.);
#39757=ORIENTED_EDGE('',*,*,#21449,.F.);
#39758=ORIENTED_EDGE('',*,*,#22349,.F.);
#39759=ORIENTED_EDGE('',*,*,#27243,.F.);
#39760=ORIENTED_EDGE('',*,*,#21653,.F.);
#39761=ORIENTED_EDGE('',*,*,#27243,.T.);
#39762=ORIENTED_EDGE('',*,*,#22345,.F.);
#39763=ORIENTED_EDGE('',*,*,#22446,.F.);
#39764=ORIENTED_EDGE('',*,*,#21654,.F.);
#39765=ORIENTED_EDGE('',*,*,#27244,.F.);
#39766=ORIENTED_EDGE('',*,*,#22347,.F.);
#39767=ORIENTED_EDGE('',*,*,#22339,.F.);
#39768=ORIENTED_EDGE('',*,*,#22331,.F.);
#39769=ORIENTED_EDGE('',*,*,#21657,.F.);
#39770=ORIENTED_EDGE('',*,*,#22449,.F.);
#39771=ORIENTED_EDGE('',*,*,#27245,.T.);
#39772=ORIENTED_EDGE('',*,*,#22439,.F.);
#39773=ORIENTED_EDGE('',*,*,#27245,.F.);
#39774=ORIENTED_EDGE('',*,*,#22447,.F.);
#39775=ORIENTED_EDGE('',*,*,#22344,.F.);
#39776=ORIENTED_EDGE('',*,*,#27244,.T.);
#39777=ORIENTED_EDGE('',*,*,#22328,.F.);
#39778=ORIENTED_EDGE('',*,*,#22434,.F.);
#39779=ORIENTED_EDGE('',*,*,#27246,.F.);
#39780=ORIENTED_EDGE('',*,*,#22336,.F.);
#39781=ORIENTED_EDGE('',*,*,#22334,.F.);
#39782=ORIENTED_EDGE('',*,*,#22322,.F.);
#39783=ORIENTED_EDGE('',*,*,#22442,.F.);
#39784=ORIENTED_EDGE('',*,*,#22444,.F.);
#39785=ORIENTED_EDGE('',*,*,#27247,.T.);
#39786=ORIENTED_EDGE('',*,*,#22431,.F.);
#39787=ORIENTED_EDGE('',*,*,#27247,.F.);
#39788=ORIENTED_EDGE('',*,*,#22435,.F.);
#39789=ORIENTED_EDGE('',*,*,#22327,.F.);
#39790=ORIENTED_EDGE('',*,*,#27246,.T.);
#39791=ORIENTED_EDGE('',*,*,#22317,.F.);
#39792=ORIENTED_EDGE('',*,*,#22423,.F.);
#39793=ORIENTED_EDGE('',*,*,#27248,.F.);
#39794=ORIENTED_EDGE('',*,*,#22319,.F.);
#39795=ORIENTED_EDGE('',*,*,#22311,.F.);
#39796=ORIENTED_EDGE('',*,*,#22308,.F.);
#39797=ORIENTED_EDGE('',*,*,#22420,.F.);
#39798=ORIENTED_EDGE('',*,*,#22428,.F.);
#39799=ORIENTED_EDGE('',*,*,#27249,.T.);
#39800=ORIENTED_EDGE('',*,*,#22417,.F.);
#39801=ORIENTED_EDGE('',*,*,#27249,.F.);
#39802=ORIENTED_EDGE('',*,*,#22424,.F.);
#39803=ORIENTED_EDGE('',*,*,#22316,.F.);
#39804=ORIENTED_EDGE('',*,*,#27248,.T.);
#39805=ORIENTED_EDGE('',*,*,#22303,.F.);
#39806=ORIENTED_EDGE('',*,*,#22409,.F.);
#39807=ORIENTED_EDGE('',*,*,#27250,.F.);
#39808=ORIENTED_EDGE('',*,*,#22305,.F.);
#39809=ORIENTED_EDGE('',*,*,#22297,.F.);
#39810=ORIENTED_EDGE('',*,*,#22294,.F.);
#39811=ORIENTED_EDGE('',*,*,#22406,.F.);
#39812=ORIENTED_EDGE('',*,*,#22414,.F.);
#39813=ORIENTED_EDGE('',*,*,#27251,.T.);
#39814=ORIENTED_EDGE('',*,*,#22403,.F.);
#39815=ORIENTED_EDGE('',*,*,#27251,.F.);
#39816=ORIENTED_EDGE('',*,*,#22410,.F.);
#39817=ORIENTED_EDGE('',*,*,#22302,.F.);
#39818=ORIENTED_EDGE('',*,*,#27250,.T.);
#39819=ORIENTED_EDGE('',*,*,#22289,.F.);
#39820=ORIENTED_EDGE('',*,*,#22395,.F.);
#39821=ORIENTED_EDGE('',*,*,#27252,.F.);
#39822=ORIENTED_EDGE('',*,*,#22291,.F.);
#39823=ORIENTED_EDGE('',*,*,#22283,.F.);
#39824=ORIENTED_EDGE('',*,*,#22280,.F.);
#39825=ORIENTED_EDGE('',*,*,#22392,.F.);
#39826=ORIENTED_EDGE('',*,*,#22400,.F.);
#39827=ORIENTED_EDGE('',*,*,#27253,.T.);
#39828=ORIENTED_EDGE('',*,*,#22389,.F.);
#39829=ORIENTED_EDGE('',*,*,#27253,.F.);
#39830=ORIENTED_EDGE('',*,*,#22396,.F.);
#39831=ORIENTED_EDGE('',*,*,#22288,.F.);
#39832=ORIENTED_EDGE('',*,*,#27252,.T.);
#39833=ORIENTED_EDGE('',*,*,#22274,.F.);
#39834=ORIENTED_EDGE('',*,*,#22381,.F.);
#39835=ORIENTED_EDGE('',*,*,#27254,.F.);
#39836=ORIENTED_EDGE('',*,*,#22276,.F.);
#39837=ORIENTED_EDGE('',*,*,#22268,.F.);
#39838=ORIENTED_EDGE('',*,*,#22265,.F.);
#39839=ORIENTED_EDGE('',*,*,#22378,.F.);
#39840=ORIENTED_EDGE('',*,*,#22386,.F.);
#39841=ORIENTED_EDGE('',*,*,#27255,.T.);
#39842=ORIENTED_EDGE('',*,*,#22375,.F.);
#39843=ORIENTED_EDGE('',*,*,#27255,.F.);
#39844=ORIENTED_EDGE('',*,*,#22382,.F.);
#39845=ORIENTED_EDGE('',*,*,#22273,.F.);
#39846=ORIENTED_EDGE('',*,*,#27254,.T.);
#39847=ORIENTED_EDGE('',*,*,#22262,.F.);
#39848=ORIENTED_EDGE('',*,*,#22366,.F.);
#39849=ORIENTED_EDGE('',*,*,#22355,.F.);
#39850=ORIENTED_EDGE('',*,*,#27256,.F.);
#39851=ORIENTED_EDGE('',*,*,#22367,.F.);
#39852=ORIENTED_EDGE('',*,*,#22261,.F.);
#39853=ORIENTED_EDGE('',*,*,#27257,.T.);
#39854=ORIENTED_EDGE('',*,*,#21452,.F.);
#39855=ORIENTED_EDGE('',*,*,#22363,.F.);
#39856=ORIENTED_EDGE('',*,*,#22371,.F.);
#39857=ORIENTED_EDGE('',*,*,#27256,.T.);
#39858=ORIENTED_EDGE('',*,*,#22360,.F.);
#39859=ORIENTED_EDGE('',*,*,#27257,.F.);
#39860=ORIENTED_EDGE('',*,*,#22373,.F.);
#39861=ORIENTED_EDGE('',*,*,#21453,.F.);
#39862=ORIENTED_EDGE('',*,*,#22253,.F.);
#39863=ORIENTED_EDGE('',*,*,#27258,.F.);
#39864=ORIENTED_EDGE('',*,*,#21647,.F.);
#39865=ORIENTED_EDGE('',*,*,#27258,.T.);
#39866=ORIENTED_EDGE('',*,*,#22249,.F.);
#39867=ORIENTED_EDGE('',*,*,#22350,.F.);
#39868=ORIENTED_EDGE('',*,*,#21648,.F.);
#39869=ORIENTED_EDGE('',*,*,#27259,.F.);
#39870=ORIENTED_EDGE('',*,*,#22251,.F.);
#39871=ORIENTED_EDGE('',*,*,#22243,.F.);
#39872=ORIENTED_EDGE('',*,*,#22240,.F.);
#39873=ORIENTED_EDGE('',*,*,#21651,.F.);
#39874=ORIENTED_EDGE('',*,*,#22353,.F.);
#39875=ORIENTED_EDGE('',*,*,#27260,.T.);
#39876=ORIENTED_EDGE('',*,*,#22348,.F.);
#39877=ORIENTED_EDGE('',*,*,#27260,.F.);
#39878=ORIENTED_EDGE('',*,*,#22351,.F.);
#39879=ORIENTED_EDGE('',*,*,#22248,.F.);
#39880=ORIENTED_EDGE('',*,*,#27259,.T.);
#39881=ORIENTED_EDGE('',*,*,#22235,.F.);
#39882=ORIENTED_EDGE('',*,*,#22341,.F.);
#39883=ORIENTED_EDGE('',*,*,#27261,.F.);
#39884=ORIENTED_EDGE('',*,*,#22237,.F.);
#39885=ORIENTED_EDGE('',*,*,#22229,.F.);
#39886=ORIENTED_EDGE('',*,*,#22221,.F.);
#39887=ORIENTED_EDGE('',*,*,#22338,.F.);
#39888=ORIENTED_EDGE('',*,*,#22346,.F.);
#39889=ORIENTED_EDGE('',*,*,#27262,.T.);
#39890=ORIENTED_EDGE('',*,*,#22330,.F.);
#39891=ORIENTED_EDGE('',*,*,#27262,.F.);
#39892=ORIENTED_EDGE('',*,*,#22342,.F.);
#39893=ORIENTED_EDGE('',*,*,#22234,.F.);
#39894=ORIENTED_EDGE('',*,*,#27261,.T.);
#39895=ORIENTED_EDGE('',*,*,#22218,.F.);
#39896=ORIENTED_EDGE('',*,*,#22324,.F.);
#39897=ORIENTED_EDGE('',*,*,#27263,.F.);
#39898=ORIENTED_EDGE('',*,*,#22226,.F.);
#39899=ORIENTED_EDGE('',*,*,#22224,.F.);
#39900=ORIENTED_EDGE('',*,*,#22212,.F.);
#39901=ORIENTED_EDGE('',*,*,#22333,.F.);
#39902=ORIENTED_EDGE('',*,*,#22335,.F.);
#39903=ORIENTED_EDGE('',*,*,#27264,.T.);
#39904=ORIENTED_EDGE('',*,*,#22321,.F.);
#39905=ORIENTED_EDGE('',*,*,#27264,.F.);
#39906=ORIENTED_EDGE('',*,*,#22325,.F.);
#39907=ORIENTED_EDGE('',*,*,#22217,.F.);
#39908=ORIENTED_EDGE('',*,*,#27263,.T.);
#39909=ORIENTED_EDGE('',*,*,#22207,.F.);
#39910=ORIENTED_EDGE('',*,*,#22313,.F.);
#39911=ORIENTED_EDGE('',*,*,#27265,.F.);
#39912=ORIENTED_EDGE('',*,*,#22209,.F.);
#39913=ORIENTED_EDGE('',*,*,#22201,.F.);
#39914=ORIENTED_EDGE('',*,*,#22198,.F.);
#39915=ORIENTED_EDGE('',*,*,#22310,.F.);
#39916=ORIENTED_EDGE('',*,*,#22318,.F.);
#39917=ORIENTED_EDGE('',*,*,#27266,.T.);
#39918=ORIENTED_EDGE('',*,*,#22307,.F.);
#39919=ORIENTED_EDGE('',*,*,#27266,.F.);
#39920=ORIENTED_EDGE('',*,*,#22314,.F.);
#39921=ORIENTED_EDGE('',*,*,#22206,.F.);
#39922=ORIENTED_EDGE('',*,*,#27265,.T.);
#39923=ORIENTED_EDGE('',*,*,#22193,.F.);
#39924=ORIENTED_EDGE('',*,*,#22299,.F.);
#39925=ORIENTED_EDGE('',*,*,#27267,.F.);
#39926=ORIENTED_EDGE('',*,*,#22195,.F.);
#39927=ORIENTED_EDGE('',*,*,#22187,.F.);
#39928=ORIENTED_EDGE('',*,*,#22184,.F.);
#39929=ORIENTED_EDGE('',*,*,#22296,.F.);
#39930=ORIENTED_EDGE('',*,*,#22304,.F.);
#39931=ORIENTED_EDGE('',*,*,#27268,.T.);
#39932=ORIENTED_EDGE('',*,*,#22293,.F.);
#39933=ORIENTED_EDGE('',*,*,#27268,.F.);
#39934=ORIENTED_EDGE('',*,*,#22300,.F.);
#39935=ORIENTED_EDGE('',*,*,#22192,.F.);
#39936=ORIENTED_EDGE('',*,*,#27267,.T.);
#39937=ORIENTED_EDGE('',*,*,#22178,.F.);
#39938=ORIENTED_EDGE('',*,*,#22285,.F.);
#39939=ORIENTED_EDGE('',*,*,#27269,.F.);
#39940=ORIENTED_EDGE('',*,*,#22180,.F.);
#39941=ORIENTED_EDGE('',*,*,#22172,.F.);
#39942=ORIENTED_EDGE('',*,*,#22169,.F.);
#39943=ORIENTED_EDGE('',*,*,#22282,.F.);
#39944=ORIENTED_EDGE('',*,*,#22290,.F.);
#39945=ORIENTED_EDGE('',*,*,#27270,.T.);
#39946=ORIENTED_EDGE('',*,*,#22279,.F.);
#39947=ORIENTED_EDGE('',*,*,#27270,.F.);
#39948=ORIENTED_EDGE('',*,*,#22286,.F.);
#39949=ORIENTED_EDGE('',*,*,#22177,.F.);
#39950=ORIENTED_EDGE('',*,*,#27269,.T.);
#39951=ORIENTED_EDGE('',*,*,#22166,.F.);
#39952=ORIENTED_EDGE('',*,*,#22270,.F.);
#39953=ORIENTED_EDGE('',*,*,#22259,.F.);
#39954=ORIENTED_EDGE('',*,*,#27271,.F.);
#39955=ORIENTED_EDGE('',*,*,#22271,.F.);
#39956=ORIENTED_EDGE('',*,*,#22165,.F.);
#39957=ORIENTED_EDGE('',*,*,#27272,.T.);
#39958=ORIENTED_EDGE('',*,*,#21456,.F.);
#39959=ORIENTED_EDGE('',*,*,#22267,.F.);
#39960=ORIENTED_EDGE('',*,*,#22275,.F.);
#39961=ORIENTED_EDGE('',*,*,#27271,.T.);
#39962=ORIENTED_EDGE('',*,*,#22264,.F.);
#39963=ORIENTED_EDGE('',*,*,#27272,.F.);
#39964=ORIENTED_EDGE('',*,*,#22277,.F.);
#39965=ORIENTED_EDGE('',*,*,#21457,.F.);
#39966=ORIENTED_EDGE('',*,*,#22157,.F.);
#39967=ORIENTED_EDGE('',*,*,#27273,.F.);
#39968=ORIENTED_EDGE('',*,*,#21641,.F.);
#39969=ORIENTED_EDGE('',*,*,#27273,.T.);
#39970=ORIENTED_EDGE('',*,*,#22153,.F.);
#39971=ORIENTED_EDGE('',*,*,#22254,.F.);
#39972=ORIENTED_EDGE('',*,*,#21642,.F.);
#39973=ORIENTED_EDGE('',*,*,#27274,.F.);
#39974=ORIENTED_EDGE('',*,*,#22155,.F.);
#39975=ORIENTED_EDGE('',*,*,#22147,.F.);
#39976=ORIENTED_EDGE('',*,*,#22144,.F.);
#39977=ORIENTED_EDGE('',*,*,#21645,.F.);
#39978=ORIENTED_EDGE('',*,*,#22257,.F.);
#39979=ORIENTED_EDGE('',*,*,#27275,.T.);
#39980=ORIENTED_EDGE('',*,*,#22252,.F.);
#39981=ORIENTED_EDGE('',*,*,#27275,.F.);
#39982=ORIENTED_EDGE('',*,*,#22255,.F.);
#39983=ORIENTED_EDGE('',*,*,#22152,.F.);
#39984=ORIENTED_EDGE('',*,*,#27274,.T.);
#39985=ORIENTED_EDGE('',*,*,#22139,.F.);
#39986=ORIENTED_EDGE('',*,*,#22245,.F.);
#39987=ORIENTED_EDGE('',*,*,#27276,.F.);
#39988=ORIENTED_EDGE('',*,*,#22141,.F.);
#39989=ORIENTED_EDGE('',*,*,#22133,.F.);
#39990=ORIENTED_EDGE('',*,*,#22130,.F.);
#39991=ORIENTED_EDGE('',*,*,#22242,.F.);
#39992=ORIENTED_EDGE('',*,*,#22250,.F.);
#39993=ORIENTED_EDGE('',*,*,#27277,.T.);
#39994=ORIENTED_EDGE('',*,*,#22239,.F.);
#39995=ORIENTED_EDGE('',*,*,#27277,.F.);
#39996=ORIENTED_EDGE('',*,*,#22246,.F.);
#39997=ORIENTED_EDGE('',*,*,#22138,.F.);
#39998=ORIENTED_EDGE('',*,*,#27276,.T.);
#39999=ORIENTED_EDGE('',*,*,#22125,.F.);
#40000=ORIENTED_EDGE('',*,*,#22231,.F.);
#40001=ORIENTED_EDGE('',*,*,#27278,.F.);
#40002=ORIENTED_EDGE('',*,*,#22127,.F.);
#40003=ORIENTED_EDGE('',*,*,#22119,.F.);
#40004=ORIENTED_EDGE('',*,*,#22111,.F.);
#40005=ORIENTED_EDGE('',*,*,#22228,.F.);
#40006=ORIENTED_EDGE('',*,*,#22236,.F.);
#40007=ORIENTED_EDGE('',*,*,#27279,.T.);
#40008=ORIENTED_EDGE('',*,*,#22220,.F.);
#40009=ORIENTED_EDGE('',*,*,#27279,.F.);
#40010=ORIENTED_EDGE('',*,*,#22232,.F.);
#40011=ORIENTED_EDGE('',*,*,#22124,.F.);
#40012=ORIENTED_EDGE('',*,*,#27278,.T.);
#40013=ORIENTED_EDGE('',*,*,#22108,.F.);
#40014=ORIENTED_EDGE('',*,*,#22214,.F.);
#40015=ORIENTED_EDGE('',*,*,#27280,.F.);
#40016=ORIENTED_EDGE('',*,*,#22116,.F.);
#40017=ORIENTED_EDGE('',*,*,#22114,.F.);
#40018=ORIENTED_EDGE('',*,*,#22102,.F.);
#40019=ORIENTED_EDGE('',*,*,#22223,.F.);
#40020=ORIENTED_EDGE('',*,*,#22225,.F.);
#40021=ORIENTED_EDGE('',*,*,#27281,.T.);
#40022=ORIENTED_EDGE('',*,*,#22211,.F.);
#40023=ORIENTED_EDGE('',*,*,#27281,.F.);
#40024=ORIENTED_EDGE('',*,*,#22215,.F.);
#40025=ORIENTED_EDGE('',*,*,#22107,.F.);
#40026=ORIENTED_EDGE('',*,*,#27280,.T.);
#40027=ORIENTED_EDGE('',*,*,#22097,.F.);
#40028=ORIENTED_EDGE('',*,*,#22203,.F.);
#40029=ORIENTED_EDGE('',*,*,#27282,.F.);
#40030=ORIENTED_EDGE('',*,*,#22099,.F.);
#40031=ORIENTED_EDGE('',*,*,#22091,.F.);
#40032=ORIENTED_EDGE('',*,*,#22088,.F.);
#40033=ORIENTED_EDGE('',*,*,#22200,.F.);
#40034=ORIENTED_EDGE('',*,*,#22208,.F.);
#40035=ORIENTED_EDGE('',*,*,#27283,.T.);
#40036=ORIENTED_EDGE('',*,*,#22197,.F.);
#40037=ORIENTED_EDGE('',*,*,#27283,.F.);
#40038=ORIENTED_EDGE('',*,*,#22204,.F.);
#40039=ORIENTED_EDGE('',*,*,#22096,.F.);
#40040=ORIENTED_EDGE('',*,*,#27282,.T.);
#40041=ORIENTED_EDGE('',*,*,#22082,.F.);
#40042=ORIENTED_EDGE('',*,*,#22189,.F.);
#40043=ORIENTED_EDGE('',*,*,#27284,.F.);
#40044=ORIENTED_EDGE('',*,*,#22084,.F.);
#40045=ORIENTED_EDGE('',*,*,#22076,.F.);
#40046=ORIENTED_EDGE('',*,*,#22073,.F.);
#40047=ORIENTED_EDGE('',*,*,#22186,.F.);
#40048=ORIENTED_EDGE('',*,*,#22194,.F.);
#40049=ORIENTED_EDGE('',*,*,#27285,.T.);
#40050=ORIENTED_EDGE('',*,*,#22183,.F.);
#40051=ORIENTED_EDGE('',*,*,#27285,.F.);
#40052=ORIENTED_EDGE('',*,*,#22190,.F.);
#40053=ORIENTED_EDGE('',*,*,#22081,.F.);
#40054=ORIENTED_EDGE('',*,*,#27284,.T.);
#40055=ORIENTED_EDGE('',*,*,#22070,.F.);
#40056=ORIENTED_EDGE('',*,*,#22174,.F.);
#40057=ORIENTED_EDGE('',*,*,#22163,.F.);
#40058=ORIENTED_EDGE('',*,*,#27286,.F.);
#40059=ORIENTED_EDGE('',*,*,#22175,.F.);
#40060=ORIENTED_EDGE('',*,*,#22069,.F.);
#40061=ORIENTED_EDGE('',*,*,#27287,.T.);
#40062=ORIENTED_EDGE('',*,*,#21460,.F.);
#40063=ORIENTED_EDGE('',*,*,#22171,.F.);
#40064=ORIENTED_EDGE('',*,*,#22179,.F.);
#40065=ORIENTED_EDGE('',*,*,#27286,.T.);
#40066=ORIENTED_EDGE('',*,*,#22168,.F.);
#40067=ORIENTED_EDGE('',*,*,#27287,.F.);
#40068=ORIENTED_EDGE('',*,*,#22181,.F.);
#40069=ORIENTED_EDGE('',*,*,#21461,.F.);
#40070=ORIENTED_EDGE('',*,*,#22061,.F.);
#40071=ORIENTED_EDGE('',*,*,#27288,.F.);
#40072=ORIENTED_EDGE('',*,*,#21635,.F.);
#40073=ORIENTED_EDGE('',*,*,#27288,.T.);
#40074=ORIENTED_EDGE('',*,*,#22057,.F.);
#40075=ORIENTED_EDGE('',*,*,#22158,.F.);
#40076=ORIENTED_EDGE('',*,*,#21636,.F.);
#40077=ORIENTED_EDGE('',*,*,#27289,.F.);
#40078=ORIENTED_EDGE('',*,*,#22059,.F.);
#40079=ORIENTED_EDGE('',*,*,#22051,.F.);
#40080=ORIENTED_EDGE('',*,*,#22048,.F.);
#40081=ORIENTED_EDGE('',*,*,#21639,.F.);
#40082=ORIENTED_EDGE('',*,*,#22161,.F.);
#40083=ORIENTED_EDGE('',*,*,#27290,.T.);
#40084=ORIENTED_EDGE('',*,*,#22156,.F.);
#40085=ORIENTED_EDGE('',*,*,#27290,.F.);
#40086=ORIENTED_EDGE('',*,*,#22159,.F.);
#40087=ORIENTED_EDGE('',*,*,#22056,.F.);
#40088=ORIENTED_EDGE('',*,*,#27289,.T.);
#40089=ORIENTED_EDGE('',*,*,#22043,.F.);
#40090=ORIENTED_EDGE('',*,*,#22149,.F.);
#40091=ORIENTED_EDGE('',*,*,#27291,.F.);
#40092=ORIENTED_EDGE('',*,*,#22045,.F.);
#40093=ORIENTED_EDGE('',*,*,#22037,.F.);
#40094=ORIENTED_EDGE('',*,*,#22034,.F.);
#40095=ORIENTED_EDGE('',*,*,#22146,.F.);
#40096=ORIENTED_EDGE('',*,*,#22154,.F.);
#40097=ORIENTED_EDGE('',*,*,#27292,.T.);
#40098=ORIENTED_EDGE('',*,*,#22143,.F.);
#40099=ORIENTED_EDGE('',*,*,#27292,.F.);
#40100=ORIENTED_EDGE('',*,*,#22150,.F.);
#40101=ORIENTED_EDGE('',*,*,#22042,.F.);
#40102=ORIENTED_EDGE('',*,*,#27291,.T.);
#40103=ORIENTED_EDGE('',*,*,#22029,.F.);
#40104=ORIENTED_EDGE('',*,*,#22135,.F.);
#40105=ORIENTED_EDGE('',*,*,#27293,.F.);
#40106=ORIENTED_EDGE('',*,*,#22031,.F.);
#40107=ORIENTED_EDGE('',*,*,#22023,.F.);
#40108=ORIENTED_EDGE('',*,*,#22020,.F.);
#40109=ORIENTED_EDGE('',*,*,#22132,.F.);
#40110=ORIENTED_EDGE('',*,*,#22140,.F.);
#40111=ORIENTED_EDGE('',*,*,#27294,.T.);
#40112=ORIENTED_EDGE('',*,*,#22129,.F.);
#40113=ORIENTED_EDGE('',*,*,#27294,.F.);
#40114=ORIENTED_EDGE('',*,*,#22136,.F.);
#40115=ORIENTED_EDGE('',*,*,#22028,.F.);
#40116=ORIENTED_EDGE('',*,*,#27293,.T.);
#40117=ORIENTED_EDGE('',*,*,#22015,.F.);
#40118=ORIENTED_EDGE('',*,*,#22121,.F.);
#40119=ORIENTED_EDGE('',*,*,#27295,.F.);
#40120=ORIENTED_EDGE('',*,*,#22017,.F.);
#40121=ORIENTED_EDGE('',*,*,#22009,.F.);
#40122=ORIENTED_EDGE('',*,*,#22001,.F.);
#40123=ORIENTED_EDGE('',*,*,#22118,.F.);
#40124=ORIENTED_EDGE('',*,*,#22126,.F.);
#40125=ORIENTED_EDGE('',*,*,#27296,.T.);
#40126=ORIENTED_EDGE('',*,*,#22110,.F.);
#40127=ORIENTED_EDGE('',*,*,#27296,.F.);
#40128=ORIENTED_EDGE('',*,*,#22122,.F.);
#40129=ORIENTED_EDGE('',*,*,#22014,.F.);
#40130=ORIENTED_EDGE('',*,*,#27295,.T.);
#40131=ORIENTED_EDGE('',*,*,#21998,.F.);
#40132=ORIENTED_EDGE('',*,*,#22104,.F.);
#40133=ORIENTED_EDGE('',*,*,#27297,.F.);
#40134=ORIENTED_EDGE('',*,*,#22006,.F.);
#40135=ORIENTED_EDGE('',*,*,#22004,.F.);
#40136=ORIENTED_EDGE('',*,*,#21992,.F.);
#40137=ORIENTED_EDGE('',*,*,#22113,.F.);
#40138=ORIENTED_EDGE('',*,*,#22115,.F.);
#40139=ORIENTED_EDGE('',*,*,#27298,.T.);
#40140=ORIENTED_EDGE('',*,*,#22101,.F.);
#40141=ORIENTED_EDGE('',*,*,#27298,.F.);
#40142=ORIENTED_EDGE('',*,*,#22105,.F.);
#40143=ORIENTED_EDGE('',*,*,#21997,.F.);
#40144=ORIENTED_EDGE('',*,*,#27297,.T.);
#40145=ORIENTED_EDGE('',*,*,#21986,.F.);
#40146=ORIENTED_EDGE('',*,*,#22093,.F.);
#40147=ORIENTED_EDGE('',*,*,#27299,.F.);
#40148=ORIENTED_EDGE('',*,*,#21988,.F.);
#40149=ORIENTED_EDGE('',*,*,#21980,.F.);
#40150=ORIENTED_EDGE('',*,*,#21977,.F.);
#40151=ORIENTED_EDGE('',*,*,#22090,.F.);
#40152=ORIENTED_EDGE('',*,*,#22098,.F.);
#40153=ORIENTED_EDGE('',*,*,#27300,.T.);
#40154=ORIENTED_EDGE('',*,*,#22087,.F.);
#40155=ORIENTED_EDGE('',*,*,#27300,.F.);
#40156=ORIENTED_EDGE('',*,*,#22094,.F.);
#40157=ORIENTED_EDGE('',*,*,#21985,.F.);
#40158=ORIENTED_EDGE('',*,*,#27299,.T.);
#40159=ORIENTED_EDGE('',*,*,#21974,.F.);
#40160=ORIENTED_EDGE('',*,*,#22078,.F.);
#40161=ORIENTED_EDGE('',*,*,#22067,.F.);
#40162=ORIENTED_EDGE('',*,*,#27301,.F.);
#40163=ORIENTED_EDGE('',*,*,#22079,.F.);
#40164=ORIENTED_EDGE('',*,*,#21973,.F.);
#40165=ORIENTED_EDGE('',*,*,#27302,.T.);
#40166=ORIENTED_EDGE('',*,*,#21464,.F.);
#40167=ORIENTED_EDGE('',*,*,#22075,.F.);
#40168=ORIENTED_EDGE('',*,*,#22083,.F.);
#40169=ORIENTED_EDGE('',*,*,#27301,.T.);
#40170=ORIENTED_EDGE('',*,*,#22072,.F.);
#40171=ORIENTED_EDGE('',*,*,#27302,.F.);
#40172=ORIENTED_EDGE('',*,*,#22085,.F.);
#40173=ORIENTED_EDGE('',*,*,#21465,.F.);
#40174=ORIENTED_EDGE('',*,*,#21949,.F.);
#40175=ORIENTED_EDGE('',*,*,#27303,.F.);
#40176=ORIENTED_EDGE('',*,*,#21629,.F.);
#40177=ORIENTED_EDGE('',*,*,#27303,.T.);
#40178=ORIENTED_EDGE('',*,*,#21937,.F.);
#40179=ORIENTED_EDGE('',*,*,#22062,.F.);
#40180=ORIENTED_EDGE('',*,*,#21630,.F.);
#40181=ORIENTED_EDGE('',*,*,#27304,.F.);
#40182=ORIENTED_EDGE('',*,*,#21945,.F.);
#40183=ORIENTED_EDGE('',*,*,#21928,.F.);
#40184=ORIENTED_EDGE('',*,*,#21922,.F.);
#40185=ORIENTED_EDGE('',*,*,#21633,.F.);
#40186=ORIENTED_EDGE('',*,*,#22065,.F.);
#40187=ORIENTED_EDGE('',*,*,#27305,.T.);
#40188=ORIENTED_EDGE('',*,*,#22060,.F.);
#40189=ORIENTED_EDGE('',*,*,#27305,.F.);
#40190=ORIENTED_EDGE('',*,*,#22063,.F.);
#40191=ORIENTED_EDGE('',*,*,#21936,.F.);
#40192=ORIENTED_EDGE('',*,*,#27304,.T.);
#40193=ORIENTED_EDGE('',*,*,#21909,.F.);
#40194=ORIENTED_EDGE('',*,*,#22053,.F.);
#40195=ORIENTED_EDGE('',*,*,#27306,.F.);
#40196=ORIENTED_EDGE('',*,*,#21917,.F.);
#40197=ORIENTED_EDGE('',*,*,#21900,.F.);
#40198=ORIENTED_EDGE('',*,*,#21894,.F.);
#40199=ORIENTED_EDGE('',*,*,#22050,.F.);
#40200=ORIENTED_EDGE('',*,*,#22058,.F.);
#40201=ORIENTED_EDGE('',*,*,#27307,.T.);
#40202=ORIENTED_EDGE('',*,*,#22047,.F.);
#40203=ORIENTED_EDGE('',*,*,#27307,.F.);
#40204=ORIENTED_EDGE('',*,*,#22054,.F.);
#40205=ORIENTED_EDGE('',*,*,#21908,.F.);
#40206=ORIENTED_EDGE('',*,*,#27306,.T.);
#40207=ORIENTED_EDGE('',*,*,#21881,.F.);
#40208=ORIENTED_EDGE('',*,*,#22039,.F.);
#40209=ORIENTED_EDGE('',*,*,#27308,.F.);
#40210=ORIENTED_EDGE('',*,*,#21889,.F.);
#40211=ORIENTED_EDGE('',*,*,#21872,.F.);
#40212=ORIENTED_EDGE('',*,*,#21866,.F.);
#40213=ORIENTED_EDGE('',*,*,#22036,.F.);
#40214=ORIENTED_EDGE('',*,*,#22044,.F.);
#40215=ORIENTED_EDGE('',*,*,#27309,.T.);
#40216=ORIENTED_EDGE('',*,*,#22033,.F.);
#40217=ORIENTED_EDGE('',*,*,#27309,.F.);
#40218=ORIENTED_EDGE('',*,*,#22040,.F.);
#40219=ORIENTED_EDGE('',*,*,#21880,.F.);
#40220=ORIENTED_EDGE('',*,*,#27308,.T.);
#40221=ORIENTED_EDGE('',*,*,#21853,.F.);
#40222=ORIENTED_EDGE('',*,*,#22025,.F.);
#40223=ORIENTED_EDGE('',*,*,#27310,.F.);
#40224=ORIENTED_EDGE('',*,*,#21861,.F.);
#40225=ORIENTED_EDGE('',*,*,#21844,.F.);
#40226=ORIENTED_EDGE('',*,*,#21838,.F.);
#40227=ORIENTED_EDGE('',*,*,#22022,.F.);
#40228=ORIENTED_EDGE('',*,*,#22030,.F.);
#40229=ORIENTED_EDGE('',*,*,#27311,.T.);
#40230=ORIENTED_EDGE('',*,*,#22019,.F.);
#40231=ORIENTED_EDGE('',*,*,#27311,.F.);
#40232=ORIENTED_EDGE('',*,*,#22026,.F.);
#40233=ORIENTED_EDGE('',*,*,#21852,.F.);
#40234=ORIENTED_EDGE('',*,*,#27310,.T.);
#40235=ORIENTED_EDGE('',*,*,#21825,.F.);
#40236=ORIENTED_EDGE('',*,*,#22011,.F.);
#40237=ORIENTED_EDGE('',*,*,#27312,.F.);
#40238=ORIENTED_EDGE('',*,*,#21833,.F.);
#40239=ORIENTED_EDGE('',*,*,#21816,.F.);
#40240=ORIENTED_EDGE('',*,*,#21804,.F.);
#40241=ORIENTED_EDGE('',*,*,#22008,.F.);
#40242=ORIENTED_EDGE('',*,*,#22016,.F.);
#40243=ORIENTED_EDGE('',*,*,#27313,.T.);
#40244=ORIENTED_EDGE('',*,*,#22000,.F.);
#40245=ORIENTED_EDGE('',*,*,#27313,.F.);
#40246=ORIENTED_EDGE('',*,*,#22012,.F.);
#40247=ORIENTED_EDGE('',*,*,#21824,.F.);
#40248=ORIENTED_EDGE('',*,*,#27312,.T.);
#40249=ORIENTED_EDGE('',*,*,#21796,.F.);
#40250=ORIENTED_EDGE('',*,*,#21994,.F.);
#40251=ORIENTED_EDGE('',*,*,#27314,.F.);
#40252=ORIENTED_EDGE('',*,*,#21812,.F.);
#40253=ORIENTED_EDGE('',*,*,#21810,.F.);
#40254=ORIENTED_EDGE('',*,*,#21790,.F.);
#40255=ORIENTED_EDGE('',*,*,#22003,.F.);
#40256=ORIENTED_EDGE('',*,*,#22005,.F.);
#40257=ORIENTED_EDGE('',*,*,#27315,.T.);
#40258=ORIENTED_EDGE('',*,*,#21991,.F.);
#40259=ORIENTED_EDGE('',*,*,#27315,.F.);
#40260=ORIENTED_EDGE('',*,*,#21995,.F.);
#40261=ORIENTED_EDGE('',*,*,#21795,.F.);
#40262=ORIENTED_EDGE('',*,*,#27314,.T.);
#40263=ORIENTED_EDGE('',*,*,#21787,.F.);
#40264=ORIENTED_EDGE('',*,*,#21982,.F.);
#40265=ORIENTED_EDGE('',*,*,#21971,.F.);
#40266=ORIENTED_EDGE('',*,*,#27316,.F.);
#40267=ORIENTED_EDGE('',*,*,#21983,.F.);
#40268=ORIENTED_EDGE('',*,*,#21786,.F.);
#40269=ORIENTED_EDGE('',*,*,#27317,.T.);
#40270=ORIENTED_EDGE('',*,*,#21468,.F.);
#40271=ORIENTED_EDGE('',*,*,#21979,.F.);
#40272=ORIENTED_EDGE('',*,*,#21987,.F.);
#40273=ORIENTED_EDGE('',*,*,#27316,.T.);
#40274=ORIENTED_EDGE('',*,*,#21976,.F.);
#40275=ORIENTED_EDGE('',*,*,#27317,.F.);
#40276=ORIENTED_EDGE('',*,*,#21989,.F.);
#40277=ORIENTED_EDGE('',*,*,#21469,.F.);
#40278=ORIENTED_EDGE('',*,*,#21968,.F.);
#40279=ORIENTED_EDGE('',*,*,#27318,.F.);
#40280=ORIENTED_EDGE('',*,*,#21623,.F.);
#40281=ORIENTED_EDGE('',*,*,#27318,.T.);
#40282=ORIENTED_EDGE('',*,*,#21961,.F.);
#40283=ORIENTED_EDGE('',*,*,#21956,.F.);
#40284=ORIENTED_EDGE('',*,*,#21624,.F.);
#40285=ORIENTED_EDGE('',*,*,#27319,.F.);
#40286=ORIENTED_EDGE('',*,*,#21966,.F.);
#40287=ORIENTED_EDGE('',*,*,#21953,.F.);
#40288=ORIENTED_EDGE('',*,*,#21950,.F.);
#40289=ORIENTED_EDGE('',*,*,#21627,.F.);
#40290=ORIENTED_EDGE('',*,*,#21965,.F.);
#40291=ORIENTED_EDGE('',*,*,#27320,.T.);
#40292=ORIENTED_EDGE('',*,*,#21948,.F.);
#40293=ORIENTED_EDGE('',*,*,#27320,.F.);
#40294=ORIENTED_EDGE('',*,*,#21957,.F.);
#40295=ORIENTED_EDGE('',*,*,#21960,.F.);
#40296=ORIENTED_EDGE('',*,*,#27319,.T.);
#40297=ORIENTED_EDGE('',*,*,#21940,.F.);
#40298=ORIENTED_EDGE('',*,*,#21933,.F.);
#40299=ORIENTED_EDGE('',*,*,#27321,.F.);
#40300=ORIENTED_EDGE('',*,*,#21946,.F.);
#40301=ORIENTED_EDGE('',*,*,#21929,.F.);
#40302=ORIENTED_EDGE('',*,*,#21923,.F.);
#40303=ORIENTED_EDGE('',*,*,#21927,.F.);
#40304=ORIENTED_EDGE('',*,*,#21944,.F.);
#40305=ORIENTED_EDGE('',*,*,#27322,.T.);
#40306=ORIENTED_EDGE('',*,*,#21921,.F.);
#40307=ORIENTED_EDGE('',*,*,#27322,.F.);
#40308=ORIENTED_EDGE('',*,*,#21934,.F.);
#40309=ORIENTED_EDGE('',*,*,#21939,.F.);
#40310=ORIENTED_EDGE('',*,*,#27321,.T.);
#40311=ORIENTED_EDGE('',*,*,#21912,.F.);
#40312=ORIENTED_EDGE('',*,*,#21905,.F.);
#40313=ORIENTED_EDGE('',*,*,#27323,.F.);
#40314=ORIENTED_EDGE('',*,*,#21918,.F.);
#40315=ORIENTED_EDGE('',*,*,#21901,.F.);
#40316=ORIENTED_EDGE('',*,*,#21895,.F.);
#40317=ORIENTED_EDGE('',*,*,#21899,.F.);
#40318=ORIENTED_EDGE('',*,*,#21916,.F.);
#40319=ORIENTED_EDGE('',*,*,#27324,.T.);
#40320=ORIENTED_EDGE('',*,*,#21893,.F.);
#40321=ORIENTED_EDGE('',*,*,#27324,.F.);
#40322=ORIENTED_EDGE('',*,*,#21906,.F.);
#40323=ORIENTED_EDGE('',*,*,#21911,.F.);
#40324=ORIENTED_EDGE('',*,*,#27323,.T.);
#40325=ORIENTED_EDGE('',*,*,#21884,.F.);
#40326=ORIENTED_EDGE('',*,*,#21877,.F.);
#40327=ORIENTED_EDGE('',*,*,#27325,.F.);
#40328=ORIENTED_EDGE('',*,*,#21890,.F.);
#40329=ORIENTED_EDGE('',*,*,#21873,.F.);
#40330=ORIENTED_EDGE('',*,*,#21867,.F.);
#40331=ORIENTED_EDGE('',*,*,#21871,.F.);
#40332=ORIENTED_EDGE('',*,*,#21888,.F.);
#40333=ORIENTED_EDGE('',*,*,#27326,.T.);
#40334=ORIENTED_EDGE('',*,*,#21865,.F.);
#40335=ORIENTED_EDGE('',*,*,#27326,.F.);
#40336=ORIENTED_EDGE('',*,*,#21878,.F.);
#40337=ORIENTED_EDGE('',*,*,#21883,.F.);
#40338=ORIENTED_EDGE('',*,*,#27325,.T.);
#40339=ORIENTED_EDGE('',*,*,#21856,.F.);
#40340=ORIENTED_EDGE('',*,*,#21849,.F.);
#40341=ORIENTED_EDGE('',*,*,#27327,.F.);
#40342=ORIENTED_EDGE('',*,*,#21862,.F.);
#40343=ORIENTED_EDGE('',*,*,#21845,.F.);
#40344=ORIENTED_EDGE('',*,*,#21839,.F.);
#40345=ORIENTED_EDGE('',*,*,#21843,.F.);
#40346=ORIENTED_EDGE('',*,*,#21860,.F.);
#40347=ORIENTED_EDGE('',*,*,#27328,.T.);
#40348=ORIENTED_EDGE('',*,*,#21837,.F.);
#40349=ORIENTED_EDGE('',*,*,#27328,.F.);
#40350=ORIENTED_EDGE('',*,*,#21850,.F.);
#40351=ORIENTED_EDGE('',*,*,#21855,.F.);
#40352=ORIENTED_EDGE('',*,*,#27327,.T.);
#40353=ORIENTED_EDGE('',*,*,#21828,.F.);
#40354=ORIENTED_EDGE('',*,*,#21821,.F.);
#40355=ORIENTED_EDGE('',*,*,#27329,.F.);
#40356=ORIENTED_EDGE('',*,*,#21834,.F.);
#40357=ORIENTED_EDGE('',*,*,#21817,.F.);
#40358=ORIENTED_EDGE('',*,*,#21805,.F.);
#40359=ORIENTED_EDGE('',*,*,#21815,.F.);
#40360=ORIENTED_EDGE('',*,*,#21832,.F.);
#40361=ORIENTED_EDGE('',*,*,#27330,.T.);
#40362=ORIENTED_EDGE('',*,*,#21803,.F.);
#40363=ORIENTED_EDGE('',*,*,#27330,.F.);
#40364=ORIENTED_EDGE('',*,*,#21822,.F.);
#40365=ORIENTED_EDGE('',*,*,#21827,.F.);
#40366=ORIENTED_EDGE('',*,*,#27329,.T.);
#40367=ORIENTED_EDGE('',*,*,#21799,.F.);
#40368=ORIENTED_EDGE('',*,*,#21792,.F.);
#40369=ORIENTED_EDGE('',*,*,#21784,.F.);
#40370=ORIENTED_EDGE('',*,*,#27331,.F.);
#40371=ORIENTED_EDGE('',*,*,#21793,.F.);
#40372=ORIENTED_EDGE('',*,*,#21798,.F.);
#40373=ORIENTED_EDGE('',*,*,#27332,.T.);
#40374=ORIENTED_EDGE('',*,*,#21472,.F.);
#40375=ORIENTED_EDGE('',*,*,#21809,.F.);
#40376=ORIENTED_EDGE('',*,*,#21811,.F.);
#40377=ORIENTED_EDGE('',*,*,#27331,.T.);
#40378=ORIENTED_EDGE('',*,*,#21789,.F.);
#40379=ORIENTED_EDGE('',*,*,#27332,.F.);
#40380=ORIENTED_EDGE('',*,*,#21813,.F.);
#40381=ORIENTED_EDGE('',*,*,#21473,.F.);
#41969=CYLINDRICAL_SURFACE('',#45718,0.0015);
#41970=CYLINDRICAL_SURFACE('',#46087,0.006);
#41971=CYLINDRICAL_SURFACE('',#46091,0.01201615316635);
#41972=CYLINDRICAL_SURFACE('',#46093,0.006);
#41973=CYLINDRICAL_SURFACE('',#46097,0.006);
#41974=CYLINDRICAL_SURFACE('',#46111,0.006);
#41975=CYLINDRICAL_SURFACE('',#46115,0.006);
#41976=CYLINDRICAL_SURFACE('',#46126,0.006);
#41977=CYLINDRICAL_SURFACE('',#46129,0.006);
#41978=CYLINDRICAL_SURFACE('',#46140,0.006);
#41979=CYLINDRICAL_SURFACE('',#46144,0.006);
#41980=CYLINDRICAL_SURFACE('',#46157,0.006);
#41981=CYLINDRICAL_SURFACE('',#46161,0.006);
#41982=CYLINDRICAL_SURFACE('',#46175,0.006);
#41983=CYLINDRICAL_SURFACE('',#46179,0.00672352098562279);
#41984=CYLINDRICAL_SURFACE('',#46186,0.0115242502778466);
#41985=CYLINDRICAL_SURFACE('',#46193,0.006);
#41986=CYLINDRICAL_SURFACE('',#46201,0.0120161531663839);
#41987=CYLINDRICAL_SURFACE('',#46209,0.006);
#41988=CYLINDRICAL_SURFACE('',#46213,0.006);
#41989=CYLINDRICAL_SURFACE('',#46219,0.006);
#41990=CYLINDRICAL_SURFACE('',#46227,0.006);
#41991=CYLINDRICAL_SURFACE('',#46236,0.006);
#41992=CYLINDRICAL_SURFACE('',#46245,0.0067235209855194);
#41993=CYLINDRICAL_SURFACE('',#46248,0.0115242502778774);
#41994=CYLINDRICAL_SURFACE('',#46254,0.006);
#41995=CYLINDRICAL_SURFACE('',#46262,0.0120161531664264);
#41996=CYLINDRICAL_SURFACE('',#46265,0.006);
#41997=CYLINDRICAL_SURFACE('',#46276,0.006);
#41998=CYLINDRICAL_SURFACE('',#46280,0.006);
#41999=CYLINDRICAL_SURFACE('',#46288,0.006);
#42000=CYLINDRICAL_SURFACE('',#46297,0.006);
#42001=CYLINDRICAL_SURFACE('',#46306,0.00672352092876986);
#42002=CYLINDRICAL_SURFACE('',#46309,0.011524250277822);
#42003=CYLINDRICAL_SURFACE('',#46315,0.006);
#42004=CYLINDRICAL_SURFACE('',#46323,0.012016153166251);
#42005=CYLINDRICAL_SURFACE('',#46326,0.006);
#42006=CYLINDRICAL_SURFACE('',#46335,0.006);
#42007=CYLINDRICAL_SURFACE('',#46346,0.006);
#42008=CYLINDRICAL_SURFACE('',#46349,0.006);
#42009=CYLINDRICAL_SURFACE('',#46358,0.006);
#42010=CYLINDRICAL_SURFACE('',#46367,0.00672352092876213);
#42011=CYLINDRICAL_SURFACE('',#46370,0.0115242502778217);
#42012=CYLINDRICAL_SURFACE('',#46376,0.006);
#42013=CYLINDRICAL_SURFACE('',#46384,0.0120161531662437);
#42014=CYLINDRICAL_SURFACE('',#46387,0.006);
#42015=CYLINDRICAL_SURFACE('',#46396,0.006);
#42016=CYLINDRICAL_SURFACE('',#46402,0.006);
#42017=CYLINDRICAL_SURFACE('',#46415,0.006);
#42018=CYLINDRICAL_SURFACE('',#46419,0.006);
#42019=CYLINDRICAL_SURFACE('',#46428,0.00672352092874661);
#42020=CYLINDRICAL_SURFACE('',#46431,0.0115242502777059);
#42021=CYLINDRICAL_SURFACE('',#46437,0.006);
#42022=CYLINDRICAL_SURFACE('',#46445,0.012016153166215);
#42023=CYLINDRICAL_SURFACE('',#46448,0.006);
#42024=CYLINDRICAL_SURFACE('',#46457,0.006);
#42025=CYLINDRICAL_SURFACE('',#46463,0.006);
#42026=CYLINDRICAL_SURFACE('',#46471,0.006);
#42027=CYLINDRICAL_SURFACE('',#46485,0.006);
#42028=CYLINDRICAL_SURFACE('',#46489,0.00672352098540828);
#42029=CYLINDRICAL_SURFACE('',#46492,0.011524250277971);
#42030=CYLINDRICAL_SURFACE('',#46498,0.006);
#42031=CYLINDRICAL_SURFACE('',#46506,0.0120161531662294);
#42032=CYLINDRICAL_SURFACE('',#46509,0.006);
#42033=CYLINDRICAL_SURFACE('',#46518,0.006);
#42034=CYLINDRICAL_SURFACE('',#46524,0.006);
#42035=CYLINDRICAL_SURFACE('',#46532,0.006);
#42036=CYLINDRICAL_SURFACE('',#46541,0.006);
#42037=CYLINDRICAL_SURFACE('',#46550,0.00672352092867469);
#42038=CYLINDRICAL_SURFACE('',#46553,0.0115242502779462);
#42039=CYLINDRICAL_SURFACE('',#46559,0.006);
#42040=CYLINDRICAL_SURFACE('',#46567,0.0120161531662171);
#42041=CYLINDRICAL_SURFACE('',#46570,0.006);
#42042=CYLINDRICAL_SURFACE('',#46579,0.006);
#42043=CYLINDRICAL_SURFACE('',#46585,0.006);
#42044=CYLINDRICAL_SURFACE('',#46593,0.006);
#42045=CYLINDRICAL_SURFACE('',#46602,0.006);
#42046=CYLINDRICAL_SURFACE('',#46611,0.00672352092871933);
#42047=CYLINDRICAL_SURFACE('',#46614,0.011524250277966);
#42048=CYLINDRICAL_SURFACE('',#46620,0.006);
#42049=CYLINDRICAL_SURFACE('',#46628,0.0120161531661977);
#42050=CYLINDRICAL_SURFACE('',#46631,0.006);
#42051=CYLINDRICAL_SURFACE('',#46640,0.006);
#42052=CYLINDRICAL_SURFACE('',#46646,0.006);
#42053=CYLINDRICAL_SURFACE('',#46654,0.006);
#42054=CYLINDRICAL_SURFACE('',#46663,0.006);
#42055=CYLINDRICAL_SURFACE('',#46672,0.0067235209286786);
#42056=CYLINDRICAL_SURFACE('',#46675,0.0115242502779575);
#42057=CYLINDRICAL_SURFACE('',#46681,0.006);
#42058=CYLINDRICAL_SURFACE('',#46689,0.0120161531661926);
#42059=CYLINDRICAL_SURFACE('',#46692,0.006);
#42060=CYLINDRICAL_SURFACE('',#46701,0.006);
#42061=CYLINDRICAL_SURFACE('',#46707,0.006);
#42062=CYLINDRICAL_SURFACE('',#46715,0.006);
#42063=CYLINDRICAL_SURFACE('',#46724,0.006);
#42064=CYLINDRICAL_SURFACE('',#46733,0.00672352092870445);
#42065=CYLINDRICAL_SURFACE('',#46736,0.0115242502780043);
#42066=CYLINDRICAL_SURFACE('',#46742,0.006);
#42067=CYLINDRICAL_SURFACE('',#46750,0.0120161531661802);
#42068=CYLINDRICAL_SURFACE('',#46753,0.006);
#42069=CYLINDRICAL_SURFACE('',#46762,0.006);
#42070=CYLINDRICAL_SURFACE('',#46768,0.006);
#42071=CYLINDRICAL_SURFACE('',#46776,0.006);
#42072=CYLINDRICAL_SURFACE('',#46785,0.006);
#42073=CYLINDRICAL_SURFACE('',#46794,0.00672352092873228);
#42074=CYLINDRICAL_SURFACE('',#46797,0.011524250277956);
#42075=CYLINDRICAL_SURFACE('',#46803,0.006);
#42076=CYLINDRICAL_SURFACE('',#46811,0.0120161531661636);
#42077=CYLINDRICAL_SURFACE('',#46814,0.006);
#42078=CYLINDRICAL_SURFACE('',#46823,0.006);
#42079=CYLINDRICAL_SURFACE('',#46829,0.006);
#42080=CYLINDRICAL_SURFACE('',#46837,0.006);
#42081=CYLINDRICAL_SURFACE('',#46846,0.006);
#42082=CYLINDRICAL_SURFACE('',#46855,0.00672352092873291);
#42083=CYLINDRICAL_SURFACE('',#46858,0.0115242502780166);
#42084=CYLINDRICAL_SURFACE('',#46864,0.006);
#42085=CYLINDRICAL_SURFACE('',#46872,0.0120161531661576);
#42086=CYLINDRICAL_SURFACE('',#46875,0.006);
#42087=CYLINDRICAL_SURFACE('',#46884,0.006);
#42088=CYLINDRICAL_SURFACE('',#46890,0.006);
#42089=CYLINDRICAL_SURFACE('',#46898,0.006);
#42090=CYLINDRICAL_SURFACE('',#46907,0.006);
#42091=CYLINDRICAL_SURFACE('',#46916,0.0067235209287966);
#42092=CYLINDRICAL_SURFACE('',#46919,0.0115242502780193);
#42093=CYLINDRICAL_SURFACE('',#46925,0.006);
#42094=CYLINDRICAL_SURFACE('',#46933,0.0120161531661516);
#42095=CYLINDRICAL_SURFACE('',#46936,0.006);
#42096=CYLINDRICAL_SURFACE('',#46945,0.006);
#42097=CYLINDRICAL_SURFACE('',#46951,0.006);
#42098=CYLINDRICAL_SURFACE('',#46959,0.006);
#42099=CYLINDRICAL_SURFACE('',#46968,0.006);
#42100=CYLINDRICAL_SURFACE('',#46977,0.00672352092871571);
#42101=CYLINDRICAL_SURFACE('',#46980,0.0115242502780358);
#42102=CYLINDRICAL_SURFACE('',#46986,0.006);
#42103=CYLINDRICAL_SURFACE('',#46994,0.0120161531661375);
#42104=CYLINDRICAL_SURFACE('',#46997,0.006);
#42105=CYLINDRICAL_SURFACE('',#47006,0.006);
#42106=CYLINDRICAL_SURFACE('',#47012,0.006);
#42107=CYLINDRICAL_SURFACE('',#47020,0.006);
#42108=CYLINDRICAL_SURFACE('',#47029,0.006);
#42109=CYLINDRICAL_SURFACE('',#47038,0.00672352092882081);
#42110=CYLINDRICAL_SURFACE('',#47041,0.0115242502780597);
#42111=CYLINDRICAL_SURFACE('',#47047,0.006);
#42112=CYLINDRICAL_SURFACE('',#47055,0.0120161531661259);
#42113=CYLINDRICAL_SURFACE('',#47058,0.006);
#42114=CYLINDRICAL_SURFACE('',#47067,0.006);
#42115=CYLINDRICAL_SURFACE('',#47073,0.006);
#42116=CYLINDRICAL_SURFACE('',#47081,0.006);
#42117=CYLINDRICAL_SURFACE('',#47090,0.006);
#42118=CYLINDRICAL_SURFACE('',#47099,0.00672352092887584);
#42119=CYLINDRICAL_SURFACE('',#47102,0.0115242502780683);
#42120=CYLINDRICAL_SURFACE('',#47108,0.006);
#42121=CYLINDRICAL_SURFACE('',#47116,0.0120161531661189);
#42122=CYLINDRICAL_SURFACE('',#47119,0.006);
#42123=CYLINDRICAL_SURFACE('',#47128,0.006);
#42124=CYLINDRICAL_SURFACE('',#47134,0.006);
#42125=CYLINDRICAL_SURFACE('',#47142,0.006);
#42126=CYLINDRICAL_SURFACE('',#47151,0.006);
#42127=CYLINDRICAL_SURFACE('',#47160,0.00672352092894656);
#42128=CYLINDRICAL_SURFACE('',#47163,0.0115242502780745);
#42129=CYLINDRICAL_SURFACE('',#47169,0.006);
#42130=CYLINDRICAL_SURFACE('',#47177,0.0120161531661058);
#42131=CYLINDRICAL_SURFACE('',#47180,0.006);
#42132=CYLINDRICAL_SURFACE('',#47189,0.006);
#42133=CYLINDRICAL_SURFACE('',#47195,0.006);
#42134=CYLINDRICAL_SURFACE('',#47203,0.006);
#42135=CYLINDRICAL_SURFACE('',#47212,0.006);
#42136=CYLINDRICAL_SURFACE('',#47221,0.0067235209289897);
#42137=CYLINDRICAL_SURFACE('',#47224,0.0115242502781104);
#42138=CYLINDRICAL_SURFACE('',#47230,0.006);
#42139=CYLINDRICAL_SURFACE('',#47238,0.0120161531661046);
#42140=CYLINDRICAL_SURFACE('',#47241,0.006);
#42141=CYLINDRICAL_SURFACE('',#47250,0.006);
#42142=CYLINDRICAL_SURFACE('',#47256,0.006);
#42143=CYLINDRICAL_SURFACE('',#47264,0.006);
#42144=CYLINDRICAL_SURFACE('',#47273,0.006);
#42145=CYLINDRICAL_SURFACE('',#47282,0.00672352092902962);
#42146=CYLINDRICAL_SURFACE('',#47285,0.0115242502780876);
#42147=CYLINDRICAL_SURFACE('',#47291,0.006);
#42148=CYLINDRICAL_SURFACE('',#47299,0.0120161531660918);
#42149=CYLINDRICAL_SURFACE('',#47302,0.006);
#42150=CYLINDRICAL_SURFACE('',#47311,0.006);
#42151=CYLINDRICAL_SURFACE('',#47317,0.006);
#42152=CYLINDRICAL_SURFACE('',#47325,0.006);
#42153=CYLINDRICAL_SURFACE('',#47334,0.006);
#42154=CYLINDRICAL_SURFACE('',#47343,0.00672352092909496);
#42155=CYLINDRICAL_SURFACE('',#47346,0.0115242502781071);
#42156=CYLINDRICAL_SURFACE('',#47352,0.006);
#42157=CYLINDRICAL_SURFACE('',#47360,0.0120161531660884);
#42158=CYLINDRICAL_SURFACE('',#47363,0.006);
#42159=CYLINDRICAL_SURFACE('',#47372,0.006);
#42160=CYLINDRICAL_SURFACE('',#47378,0.006);
#42161=CYLINDRICAL_SURFACE('',#47386,0.006);
#42162=CYLINDRICAL_SURFACE('',#47395,0.006);
#42163=CYLINDRICAL_SURFACE('',#47404,0.00672352092911924);
#42164=CYLINDRICAL_SURFACE('',#47407,0.0115242502781167);
#42165=CYLINDRICAL_SURFACE('',#47413,0.006);
#42166=CYLINDRICAL_SURFACE('',#47421,0.0120161531660803);
#42167=CYLINDRICAL_SURFACE('',#47424,0.006);
#42168=CYLINDRICAL_SURFACE('',#47433,0.006);
#42169=CYLINDRICAL_SURFACE('',#47439,0.006);
#42170=CYLINDRICAL_SURFACE('',#47447,0.006);
#42171=CYLINDRICAL_SURFACE('',#47456,0.006);
#42172=CYLINDRICAL_SURFACE('',#47465,0.00672352092921552);
#42173=CYLINDRICAL_SURFACE('',#47468,0.0115242502781272);
#42174=CYLINDRICAL_SURFACE('',#47474,0.006);
#42175=CYLINDRICAL_SURFACE('',#47482,0.0120161531660835);
#42176=CYLINDRICAL_SURFACE('',#47485,0.006);
#42177=CYLINDRICAL_SURFACE('',#47494,0.006);
#42178=CYLINDRICAL_SURFACE('',#47500,0.006);
#42179=CYLINDRICAL_SURFACE('',#47508,0.006);
#42180=CYLINDRICAL_SURFACE('',#47517,0.006);
#42181=CYLINDRICAL_SURFACE('',#47526,0.00672352092925948);
#42182=CYLINDRICAL_SURFACE('',#47529,0.0115242502781359);
#42183=CYLINDRICAL_SURFACE('',#47535,0.006);
#42184=CYLINDRICAL_SURFACE('',#47543,0.0120161531660829);
#42185=CYLINDRICAL_SURFACE('',#47546,0.006);
#42186=CYLINDRICAL_SURFACE('',#47555,0.006);
#42187=CYLINDRICAL_SURFACE('',#47561,0.006);
#42188=CYLINDRICAL_SURFACE('',#47569,0.006);
#42189=CYLINDRICAL_SURFACE('',#47578,0.006);
#42190=CYLINDRICAL_SURFACE('',#47587,0.00672352092931105);
#42191=CYLINDRICAL_SURFACE('',#47590,0.0115242502781424);
#42192=CYLINDRICAL_SURFACE('',#47596,0.006);
#42193=CYLINDRICAL_SURFACE('',#47604,0.0120161531662401);
#42194=CYLINDRICAL_SURFACE('',#47607,0.006);
#42195=CYLINDRICAL_SURFACE('',#47616,0.006);
#42196=CYLINDRICAL_SURFACE('',#47622,0.006);
#42197=CYLINDRICAL_SURFACE('',#47630,0.006);
#42198=CYLINDRICAL_SURFACE('',#47639,0.006);
#42199=CYLINDRICAL_SURFACE('',#47648,0.00672352092933407);
#42200=CYLINDRICAL_SURFACE('',#47651,0.0115242502781404);
#42201=CYLINDRICAL_SURFACE('',#47657,0.006);
#42202=CYLINDRICAL_SURFACE('',#47665,0.0120161531662008);
#42203=CYLINDRICAL_SURFACE('',#47668,0.006);
#42204=CYLINDRICAL_SURFACE('',#47677,0.006);
#42205=CYLINDRICAL_SURFACE('',#47683,0.006);
#42206=CYLINDRICAL_SURFACE('',#47691,0.006);
#42207=CYLINDRICAL_SURFACE('',#47700,0.006);
#42208=CYLINDRICAL_SURFACE('',#47709,0.00672352092934602);
#42209=CYLINDRICAL_SURFACE('',#47712,0.0115242502781491);
#42210=CYLINDRICAL_SURFACE('',#47718,0.006);
#42211=CYLINDRICAL_SURFACE('',#47726,0.0120161531661581);
#42212=CYLINDRICAL_SURFACE('',#47729,0.006);
#42213=CYLINDRICAL_SURFACE('',#47738,0.006);
#42214=CYLINDRICAL_SURFACE('',#47744,0.006);
#42215=CYLINDRICAL_SURFACE('',#47752,0.006);
#42216=CYLINDRICAL_SURFACE('',#47761,0.006);
#42217=CYLINDRICAL_SURFACE('',#47770,0.00672352092933986);
#42218=CYLINDRICAL_SURFACE('',#47773,0.0115242502781903);
#42219=CYLINDRICAL_SURFACE('',#47779,0.006);
#42220=CYLINDRICAL_SURFACE('',#47787,0.0120161531661162);
#42221=CYLINDRICAL_SURFACE('',#47790,0.006);
#42222=CYLINDRICAL_SURFACE('',#47799,0.006);
#42223=CYLINDRICAL_SURFACE('',#47805,0.006);
#42224=CYLINDRICAL_SURFACE('',#47813,0.006);
#42225=CYLINDRICAL_SURFACE('',#47822,0.006);
#42226=CYLINDRICAL_SURFACE('',#47831,0.00672352092930669);
#42227=CYLINDRICAL_SURFACE('',#47834,0.0115242502778983);
#42228=CYLINDRICAL_SURFACE('',#47840,0.006);
#42229=CYLINDRICAL_SURFACE('',#47848,0.0120161531661211);
#42230=CYLINDRICAL_SURFACE('',#47851,0.006);
#42231=CYLINDRICAL_SURFACE('',#47860,0.006);
#42232=CYLINDRICAL_SURFACE('',#47866,0.006);
#42233=CYLINDRICAL_SURFACE('',#47874,0.006);
#42234=CYLINDRICAL_SURFACE('',#47883,0.006);
#42235=CYLINDRICAL_SURFACE('',#47892,0.00672352092933276);
#42236=CYLINDRICAL_SURFACE('',#47895,0.0115242502779026);
#42237=CYLINDRICAL_SURFACE('',#47901,0.006);
#42238=CYLINDRICAL_SURFACE('',#47909,0.0120161531661695);
#42239=CYLINDRICAL_SURFACE('',#47912,0.006);
#42240=CYLINDRICAL_SURFACE('',#47921,0.006);
#42241=CYLINDRICAL_SURFACE('',#47927,0.006);
#42242=CYLINDRICAL_SURFACE('',#47935,0.006);
#42243=CYLINDRICAL_SURFACE('',#47944,0.006);
#42244=CYLINDRICAL_SURFACE('',#47953,0.00672352092937054);
#42245=CYLINDRICAL_SURFACE('',#47956,0.0115242502779253);
#42246=CYLINDRICAL_SURFACE('',#47962,0.006);
#42247=CYLINDRICAL_SURFACE('',#47970,0.0120161531662158);
#42248=CYLINDRICAL_SURFACE('',#47973,0.006);
#42249=CYLINDRICAL_SURFACE('',#47982,0.006);
#42250=CYLINDRICAL_SURFACE('',#47988,0.006);
#42251=CYLINDRICAL_SURFACE('',#47996,0.006);
#42252=CYLINDRICAL_SURFACE('',#48005,0.006);
#42253=CYLINDRICAL_SURFACE('',#48014,0.00672352092931684);
#42254=CYLINDRICAL_SURFACE('',#48017,0.0115242502779055);
#42255=CYLINDRICAL_SURFACE('',#48023,0.006);
#42256=CYLINDRICAL_SURFACE('',#48031,0.0120161531662664);
#42257=CYLINDRICAL_SURFACE('',#48034,0.006);
#42258=CYLINDRICAL_SURFACE('',#48043,0.006);
#42259=CYLINDRICAL_SURFACE('',#48049,0.006);
#42260=CYLINDRICAL_SURFACE('',#48057,0.006);
#42261=CYLINDRICAL_SURFACE('',#48066,0.006);
#42262=CYLINDRICAL_SURFACE('',#48075,0.00672352092935101);
#42263=CYLINDRICAL_SURFACE('',#48078,0.0115242502778479);
#42264=CYLINDRICAL_SURFACE('',#48084,0.006);
#42265=CYLINDRICAL_SURFACE('',#48092,0.0120161531662955);
#42266=CYLINDRICAL_SURFACE('',#48095,0.006);
#42267=CYLINDRICAL_SURFACE('',#48104,0.006);
#42268=CYLINDRICAL_SURFACE('',#48110,0.006);
#42269=CYLINDRICAL_SURFACE('',#48118,0.006);
#42270=CYLINDRICAL_SURFACE('',#48127,0.006);
#42271=CYLINDRICAL_SURFACE('',#48136,0.0067235209293286);
#42272=CYLINDRICAL_SURFACE('',#48139,0.0115242502777874);
#42273=CYLINDRICAL_SURFACE('',#48145,0.006);
#42274=CYLINDRICAL_SURFACE('',#48153,0.0120161531663449);
#42275=CYLINDRICAL_SURFACE('',#48156,0.006);
#42276=CYLINDRICAL_SURFACE('',#48165,0.006);
#42277=CYLINDRICAL_SURFACE('',#48171,0.006);
#42278=CYLINDRICAL_SURFACE('',#48179,0.006);
#42279=CYLINDRICAL_SURFACE('',#48188,0.006);
#42280=CYLINDRICAL_SURFACE('',#48197,0.00672352092931084);
#42281=CYLINDRICAL_SURFACE('',#48200,0.0115242502777255);
#42282=CYLINDRICAL_SURFACE('',#48206,0.006);
#42283=CYLINDRICAL_SURFACE('',#48214,0.0120161531663728);
#42284=CYLINDRICAL_SURFACE('',#48217,0.006);
#42285=CYLINDRICAL_SURFACE('',#48226,0.006);
#42286=CYLINDRICAL_SURFACE('',#48232,0.006);
#42287=CYLINDRICAL_SURFACE('',#48240,0.006);
#42288=CYLINDRICAL_SURFACE('',#48249,0.006);
#42289=CYLINDRICAL_SURFACE('',#48258,0.00672352092931385);
#42290=CYLINDRICAL_SURFACE('',#48261,0.0115242502777398);
#42291=CYLINDRICAL_SURFACE('',#48267,0.006);
#42292=CYLINDRICAL_SURFACE('',#48275,0.0120161531664183);
#42293=CYLINDRICAL_SURFACE('',#48278,0.006);
#42294=CYLINDRICAL_SURFACE('',#48287,0.006);
#42295=CYLINDRICAL_SURFACE('',#48293,0.006);
#42296=CYLINDRICAL_SURFACE('',#48301,0.006);
#42297=CYLINDRICAL_SURFACE('',#48310,0.006);
#42298=CYLINDRICAL_SURFACE('',#48319,0.00672352092933332);
#42299=CYLINDRICAL_SURFACE('',#48322,0.0115242502778913);
#42300=CYLINDRICAL_SURFACE('',#48328,0.006);
#42301=CYLINDRICAL_SURFACE('',#48336,0.0120161531664379);
#42302=CYLINDRICAL_SURFACE('',#48339,0.006);
#42303=CYLINDRICAL_SURFACE('',#48348,0.006);
#42304=CYLINDRICAL_SURFACE('',#48354,0.006);
#42305=CYLINDRICAL_SURFACE('',#48362,0.006);
#42306=CYLINDRICAL_SURFACE('',#48371,0.006);
#42307=CYLINDRICAL_SURFACE('',#48380,0.00672352092934512);
#42308=CYLINDRICAL_SURFACE('',#48383,0.0115242502779201);
#42309=CYLINDRICAL_SURFACE('',#48389,0.006);
#42310=CYLINDRICAL_SURFACE('',#48397,0.0120161531664445);
#42311=CYLINDRICAL_SURFACE('',#48400,0.006);
#42312=CYLINDRICAL_SURFACE('',#48409,0.006);
#42313=CYLINDRICAL_SURFACE('',#48415,0.006);
#42314=CYLINDRICAL_SURFACE('',#48423,0.006);
#42315=CYLINDRICAL_SURFACE('',#48432,0.006);
#42316=CYLINDRICAL_SURFACE('',#48441,0.00672352092933164);
#42317=CYLINDRICAL_SURFACE('',#48444,0.0115242502779111);
#42318=CYLINDRICAL_SURFACE('',#48450,0.006);
#42319=CYLINDRICAL_SURFACE('',#48458,0.0120161531664562);
#42320=CYLINDRICAL_SURFACE('',#48461,0.006);
#42321=CYLINDRICAL_SURFACE('',#48470,0.006);
#42322=CYLINDRICAL_SURFACE('',#48476,0.006);
#42323=CYLINDRICAL_SURFACE('',#48484,0.006);
#42324=CYLINDRICAL_SURFACE('',#48493,0.006);
#42325=CYLINDRICAL_SURFACE('',#48502,0.00672352092931991);
#42326=CYLINDRICAL_SURFACE('',#48505,0.0115242502778819);
#42327=CYLINDRICAL_SURFACE('',#48511,0.006);
#42328=CYLINDRICAL_SURFACE('',#48519,0.0120161531664664);
#42329=CYLINDRICAL_SURFACE('',#48522,0.006);
#42330=CYLINDRICAL_SURFACE('',#48531,0.006);
#42331=CYLINDRICAL_SURFACE('',#48537,0.006);
#42332=CYLINDRICAL_SURFACE('',#48545,0.006);
#42333=CYLINDRICAL_SURFACE('',#48554,0.006);
#42334=CYLINDRICAL_SURFACE('',#48563,0.00672352092931163);
#42335=CYLINDRICAL_SURFACE('',#48566,0.0115242502779297);
#42336=CYLINDRICAL_SURFACE('',#48572,0.006);
#42337=CYLINDRICAL_SURFACE('',#48580,0.0120161531664594);
#42338=CYLINDRICAL_SURFACE('',#48583,0.006);
#42339=CYLINDRICAL_SURFACE('',#48592,0.006);
#42340=CYLINDRICAL_SURFACE('',#48598,0.006);
#42341=CYLINDRICAL_SURFACE('',#48606,0.006);
#42342=CYLINDRICAL_SURFACE('',#48615,0.006);
#42343=CYLINDRICAL_SURFACE('',#48624,0.00672352092935956);
#42344=CYLINDRICAL_SURFACE('',#48627,0.0115242502779183);
#42345=CYLINDRICAL_SURFACE('',#48633,0.006);
#42346=CYLINDRICAL_SURFACE('',#48641,0.0120161531664567);
#42347=CYLINDRICAL_SURFACE('',#48644,0.006);
#42348=CYLINDRICAL_SURFACE('',#48653,0.006);
#42349=CYLINDRICAL_SURFACE('',#48659,0.006);
#42350=CYLINDRICAL_SURFACE('',#48667,0.006);
#42351=CYLINDRICAL_SURFACE('',#48676,0.006);
#42352=CYLINDRICAL_SURFACE('',#48685,0.0067235209293039);
#42353=CYLINDRICAL_SURFACE('',#48688,0.0115242502778913);
#42354=CYLINDRICAL_SURFACE('',#48694,0.006);
#42355=CYLINDRICAL_SURFACE('',#48702,0.0120161531664457);
#42356=CYLINDRICAL_SURFACE('',#48705,0.006);
#42357=CYLINDRICAL_SURFACE('',#48714,0.006);
#42358=CYLINDRICAL_SURFACE('',#48720,0.006);
#42359=CYLINDRICAL_SURFACE('',#48728,0.006);
#42360=CYLINDRICAL_SURFACE('',#48737,0.006);
#42361=CYLINDRICAL_SURFACE('',#48746,0.00672352092926038);
#42362=CYLINDRICAL_SURFACE('',#48749,0.0115242502779262);
#42363=CYLINDRICAL_SURFACE('',#48751,0.006);
#42364=CYLINDRICAL_SURFACE('',#48763,0.0120161531664297);
#42365=CYLINDRICAL_SURFACE('',#48766,0.006);
#42366=CYLINDRICAL_SURFACE('',#48775,0.006);
#42367=CYLINDRICAL_SURFACE('',#48781,0.006);
#42368=CYLINDRICAL_SURFACE('',#48789,0.006);
#42369=CYLINDRICAL_SURFACE('',#48798,0.006);
#42370=CYLINDRICAL_SURFACE('',#48807,0.00672352092922533);
#42371=CYLINDRICAL_SURFACE('',#48810,0.0115242502779126);
#42372=CYLINDRICAL_SURFACE('',#48812,0.006);
#42373=CYLINDRICAL_SURFACE('',#48817,0.006);
#42374=CYLINDRICAL_SURFACE('',#48829,0.0120161531664118);
#42375=CYLINDRICAL_SURFACE('',#48836,0.006);
#42376=CYLINDRICAL_SURFACE('',#48842,0.006);
#42377=CYLINDRICAL_SURFACE('',#48850,0.006);
#42378=CYLINDRICAL_SURFACE('',#48859,0.006);
#42379=CYLINDRICAL_SURFACE('',#48868,0.00672352092915246);
#42380=CYLINDRICAL_SURFACE('',#48871,0.0115242502779174);
#42381=CYLINDRICAL_SURFACE('',#48873,0.006);
#42382=CYLINDRICAL_SURFACE('',#48878,0.006);
#42383=CYLINDRICAL_SURFACE('',#48883,0.006);
#42384=CYLINDRICAL_SURFACE('',#48892,0.0120161531663761);
#42385=CYLINDRICAL_SURFACE('',#48903,0.006);
#42386=CYLINDRICAL_SURFACE('',#48911,0.006);
#42387=CYLINDRICAL_SURFACE('',#48920,0.006);
#42388=CYLINDRICAL_SURFACE('',#48929,0.0067235209291287);
#42389=CYLINDRICAL_SURFACE('',#48932,0.0115242502779053);
#42390=CYLINDRICAL_SURFACE('',#48934,0.006);
#42391=CYLINDRICAL_SURFACE('',#48939,0.006);
#42392=CYLINDRICAL_SURFACE('',#48944,0.006);
#42393=CYLINDRICAL_SURFACE('',#48947,0.006);
#42394=CYLINDRICAL_SURFACE('',#48970,0.0120161531663417);
#42395=CYLINDRICAL_SURFACE('',#48972,0.006);
#42396=CYLINDRICAL_SURFACE('',#48981,0.006);
#42397=CYLINDRICAL_SURFACE('',#48990,0.00672352092909558);
#42398=CYLINDRICAL_SURFACE('',#48993,0.0115242502776438);
#42399=CYLINDRICAL_SURFACE('',#48995,0.006);
#42400=CYLINDRICAL_SURFACE('',#49000,0.006);
#42401=CYLINDRICAL_SURFACE('',#49005,0.006);
#42402=CYLINDRICAL_SURFACE('',#49010,0.006);
#42403=CYLINDRICAL_SURFACE('',#49015,0.006);
#42404=CYLINDRICAL_SURFACE('',#49036,0.0120161531663077);
#42405=CYLINDRICAL_SURFACE('',#49042,0.006);
#42406=CYLINDRICAL_SURFACE('',#49051,0.00672352092901901);
#42407=CYLINDRICAL_SURFACE('',#49054,0.011524250277674);
#42408=CYLINDRICAL_SURFACE('',#49056,0.006);
#42409=CYLINDRICAL_SURFACE('',#49061,0.006);
#42410=CYLINDRICAL_SURFACE('',#49064,0.006);
#42411=CYLINDRICAL_SURFACE('',#49069,0.006);
#42412=CYLINDRICAL_SURFACE('',#49074,0.006);
#42413=CYLINDRICAL_SURFACE('',#49079,0.006);
#42414=CYLINDRICAL_SURFACE('',#49104,0.012016153166264);
#42415=CYLINDRICAL_SURFACE('',#49112,0.00672352092891286);
#42416=CYLINDRICAL_SURFACE('',#49115,0.0115242502777387);
#42417=CYLINDRICAL_SURFACE('',#49117,0.00672352092892855);
#42418=CYLINDRICAL_SURFACE('',#49120,0.011524250277794);
#42419=CYLINDRICAL_SURFACE('',#49122,0.0120161531662885);
#42420=CYLINDRICAL_SURFACE('',#49136,0.00830951479144525);
#42421=CYLINDRICAL_SURFACE('',#49137,0.00489777760244533);
#42422=CYLINDRICAL_SURFACE('',#49142,0.00830951479147278);
#42423=CYLINDRICAL_SURFACE('',#49143,0.0048977776024695);
#42424=CYLINDRICAL_SURFACE('',#49157,0.00830951479145815);
#42425=CYLINDRICAL_SURFACE('',#49158,0.00489777760247165);
#42426=CYLINDRICAL_SURFACE('',#49172,0.00830951479142899);
#42427=CYLINDRICAL_SURFACE('',#49173,0.00489777760244579);
#42428=CYLINDRICAL_SURFACE('',#49187,0.00830951479141785);
#42429=CYLINDRICAL_SURFACE('',#49188,0.00489777760247916);
#42430=CYLINDRICAL_SURFACE('',#49202,0.00830951479144501);
#42431=CYLINDRICAL_SURFACE('',#49203,0.00489777760244294);
#42432=CYLINDRICAL_SURFACE('',#49217,0.00830951479145066);
#42433=CYLINDRICAL_SURFACE('',#49218,0.00489777760242687);
#42434=CYLINDRICAL_SURFACE('',#49232,0.00830951479140252);
#42435=CYLINDRICAL_SURFACE('',#49233,0.00489777760240844);
#42436=CYLINDRICAL_SURFACE('',#49247,0.00830951479142787);
#42437=CYLINDRICAL_SURFACE('',#49248,0.00489777760239372);
#42438=CYLINDRICAL_SURFACE('',#49262,0.00830951479138556);
#42439=CYLINDRICAL_SURFACE('',#49263,0.00489777760235847);
#42440=CYLINDRICAL_SURFACE('',#49277,0.00830951479141585);
#42441=CYLINDRICAL_SURFACE('',#49278,0.00489777760236036);
#42442=CYLINDRICAL_SURFACE('',#49292,0.00830951479142129);
#42443=CYLINDRICAL_SURFACE('',#49293,0.00489777760234243);
#42444=CYLINDRICAL_SURFACE('',#49307,0.00830951479143295);
#42445=CYLINDRICAL_SURFACE('',#49308,0.00489777760232894);
#42446=CYLINDRICAL_SURFACE('',#49322,0.00830951479143844);
#42447=CYLINDRICAL_SURFACE('',#49323,0.00489777760230745);
#42448=CYLINDRICAL_SURFACE('',#49337,0.00830951479141942);
#42449=CYLINDRICAL_SURFACE('',#49338,0.00489777760230435);
#42450=CYLINDRICAL_SURFACE('',#49352,0.0083095147914072);
#42451=CYLINDRICAL_SURFACE('',#49353,0.00489777760230926);
#42452=CYLINDRICAL_SURFACE('',#49367,0.00830951479140723);
#42453=CYLINDRICAL_SURFACE('',#49368,0.00489777760229998);
#42454=CYLINDRICAL_SURFACE('',#49382,0.00830951479140655);
#42455=CYLINDRICAL_SURFACE('',#49383,0.00489777760231482);
#42456=CYLINDRICAL_SURFACE('',#49397,0.00830951479140061);
#42457=CYLINDRICAL_SURFACE('',#49398,0.00489777760230995);
#42458=CYLINDRICAL_SURFACE('',#49412,0.00830951479141865);
#42459=CYLINDRICAL_SURFACE('',#49413,0.00489777760231243);
#42460=CYLINDRICAL_SURFACE('',#49427,0.00830951479139597);
#42461=CYLINDRICAL_SURFACE('',#49428,0.00489777760228124);
#42462=CYLINDRICAL_SURFACE('',#49442,0.00830951479139311);
#42463=CYLINDRICAL_SURFACE('',#49443,0.0048977776023241);
#42464=CYLINDRICAL_SURFACE('',#49457,0.00830951479138788);
#42465=CYLINDRICAL_SURFACE('',#49458,0.00489777760231598);
#42466=CYLINDRICAL_SURFACE('',#49472,0.00830951479139345);
#42467=CYLINDRICAL_SURFACE('',#49473,0.00489777760238264);
#42468=CYLINDRICAL_SURFACE('',#49487,0.00830951479136789);
#42469=CYLINDRICAL_SURFACE('',#49488,0.00489777760236428);
#42470=CYLINDRICAL_SURFACE('',#49502,0.00830951479137509);
#42471=CYLINDRICAL_SURFACE('',#49503,0.00489777760239822);
#42472=CYLINDRICAL_SURFACE('',#49517,0.00830951479138404);
#42473=CYLINDRICAL_SURFACE('',#49518,0.004897777602424);
#42474=CYLINDRICAL_SURFACE('',#49532,0.00830951479139002);
#42475=CYLINDRICAL_SURFACE('',#49533,0.00489777760244448);
#42476=CYLINDRICAL_SURFACE('',#49547,0.0083095147913546);
#42477=CYLINDRICAL_SURFACE('',#49548,0.00489777760246637);
#42478=CYLINDRICAL_SURFACE('',#49562,0.00830951479138939);
#42479=CYLINDRICAL_SURFACE('',#49563,0.00489777760247895);
#42480=CYLINDRICAL_SURFACE('',#49577,0.00830951479137315);
#42481=CYLINDRICAL_SURFACE('',#49578,0.00489777760247943);
#42482=CYLINDRICAL_SURFACE('',#49592,0.00830951479133772);
#42483=CYLINDRICAL_SURFACE('',#49593,0.00489777760248803);
#42484=CYLINDRICAL_SURFACE('',#49607,0.00830951479137358);
#42485=CYLINDRICAL_SURFACE('',#49608,0.00489777760245939);
#42486=CYLINDRICAL_SURFACE('',#49622,0.00830951479136423);
#42487=CYLINDRICAL_SURFACE('',#49623,0.00489777760247564);
#42488=CYLINDRICAL_SURFACE('',#49637,0.00830951479136581);
#42489=CYLINDRICAL_SURFACE('',#49638,0.00489777760248512);
#42490=CYLINDRICAL_SURFACE('',#49652,0.00830951479137988);
#42491=CYLINDRICAL_SURFACE('',#49653,0.00489777760253342);
#42492=CYLINDRICAL_SURFACE('',#49667,0.00830951479136722);
#42493=CYLINDRICAL_SURFACE('',#49668,0.00489777760257392);
#42494=CYLINDRICAL_SURFACE('',#49682,0.00830951479136156);
#42495=CYLINDRICAL_SURFACE('',#49683,0.00489777760253943);
#42496=CYLINDRICAL_SURFACE('',#49697,0.00830951479135765);
#42497=CYLINDRICAL_SURFACE('',#49698,0.00489777760256031);
#42498=CYLINDRICAL_SURFACE('',#49712,0.00830951479137079);
#42499=CYLINDRICAL_SURFACE('',#49713,0.0048977776025707);
#42500=CYLINDRICAL_SURFACE('',#49727,0.00830951479137468);
#42501=CYLINDRICAL_SURFACE('',#49728,0.00489777760256102);
#42502=CYLINDRICAL_SURFACE('',#49742,0.00830951479138694);
#42503=CYLINDRICAL_SURFACE('',#49743,0.00489777760258809);
#42504=CYLINDRICAL_SURFACE('',#49757,0.00830951479138659);
#42505=CYLINDRICAL_SURFACE('',#49758,0.00489777760258593);
#42506=CYLINDRICAL_SURFACE('',#49774,0.00830951479140578);
#42507=CYLINDRICAL_SURFACE('',#49775,0.00489777760257164);
#42508=CYLINDRICAL_SURFACE('',#49787,0.00830951479141365);
#42509=CYLINDRICAL_SURFACE('',#49788,0.00489777760255856);
#42510=CYLINDRICAL_SURFACE('',#49802,0.0083095147914008);
#42511=CYLINDRICAL_SURFACE('',#49803,0.00489777760254268);
#42512=CYLINDRICAL_SURFACE('',#49817,0.0083095147914313);
#42513=CYLINDRICAL_SURFACE('',#49818,0.00489777760254623);
#42514=CYLINDRICAL_SURFACE('',#49832,0.00830951479143087);
#42515=CYLINDRICAL_SURFACE('',#49833,0.00489777760250727);
#42516=CYLINDRICAL_SURFACE('',#49847,0.00830951479143416);
#42517=CYLINDRICAL_SURFACE('',#49848,0.00489777760251401);
#42518=CYLINDRICAL_SURFACE('',#49862,0.0083095147914544);
#42519=CYLINDRICAL_SURFACE('',#49863,0.00489777760247736);
#42648=ADVANCED_FACE('',(#3793),#41969,.T.);
#42649=ADVANCED_FACE('',(#3794),#881,.T.);
#42650=ADVANCED_FACE('',(#3795),#882,.T.);
#42651=ADVANCED_FACE('',(#3796),#2199,.T.);
#42652=ADVANCED_FACE('',(#3797),#2200,.T.);
#42653=ADVANCED_FACE('',(#3798),#101,.T.);
#42654=ADVANCED_FACE('',(#3799),#102,.T.);
#42655=ADVANCED_FACE('',(#3800),#2201,.T.);
#42656=ADVANCED_FACE('',(#3801),#2202,.T.);
#42657=ADVANCED_FACE('',(#3802),#41970,.T.);
#42658=ADVANCED_FACE('',(#3803),#2203,.T.);
#42659=ADVANCED_FACE('',(#3804),#41971,.T.);
#42660=ADVANCED_FACE('',(#3805),#41972,.T.);
#42661=ADVANCED_FACE('',(#3806),#41973,.T.);
#42662=ADVANCED_FACE('',(#3807),#103,.T.);
#42663=ADVANCED_FACE('',(#3808),#104,.T.);
#42664=ADVANCED_FACE('',(#3809),#2204,.T.);
#42665=ADVANCED_FACE('',(#3810),#2205,.T.);
#42666=ADVANCED_FACE('',(#3811),#105,.T.);
#42667=ADVANCED_FACE('',(#3812),#106,.T.);
#42668=ADVANCED_FACE('',(#3813),#41974,.T.);
#42669=ADVANCED_FACE('',(#3814),#41975,.T.);
#42670=ADVANCED_FACE('',(#3815),#107,.T.);
#42671=ADVANCED_FACE('',(#3816),#108,.T.);
#42672=ADVANCED_FACE('',(#3817),#2206,.T.);
#42673=ADVANCED_FACE('',(#3818),#2207,.T.);
#42674=ADVANCED_FACE('',(#3819),#109,.T.);
#42675=ADVANCED_FACE('',(#3820),#110,.T.);
#42676=ADVANCED_FACE('',(#3821),#41976,.T.);
#42677=ADVANCED_FACE('',(#3822),#41977,.T.);
#42678=ADVANCED_FACE('',(#3823),#111,.T.);
#42679=ADVANCED_FACE('',(#3824),#112,.T.);
#42680=ADVANCED_FACE('',(#3825),#2208,.T.);
#42681=ADVANCED_FACE('',(#3826),#2209,.T.);
#42682=ADVANCED_FACE('',(#3827),#2210,.T.);
#42683=ADVANCED_FACE('',(#3828),#113,.T.);
#42684=ADVANCED_FACE('',(#3829),#41978,.T.);
#42685=ADVANCED_FACE('',(#3830),#41979,.T.);
#42686=ADVANCED_FACE('',(#3831),#2211,.T.);
#42687=ADVANCED_FACE('',(#3832),#114,.T.);
#42688=ADVANCED_FACE('',(#3833),#2212,.T.);
#42689=ADVANCED_FACE('',(#3834),#2213,.T.);
#42690=ADVANCED_FACE('',(#3835),#2214,.T.);
#42691=ADVANCED_FACE('',(#3836),#2215,.T.);
#42692=ADVANCED_FACE('',(#3837),#41980,.T.);
#42693=ADVANCED_FACE('',(#3838),#41981,.T.);
#42694=ADVANCED_FACE('',(#3839),#115,.T.);
#42695=ADVANCED_FACE('',(#3840),#2216,.T.);
#42696=ADVANCED_FACE('',(#3841),#2217,.T.);
#42697=ADVANCED_FACE('',(#3842),#2218,.T.);
#42698=ADVANCED_FACE('',(#3843),#2219,.T.);
#42699=ADVANCED_FACE('',(#3844),#2220,.T.);
#42700=ADVANCED_FACE('',(#3845),#41982,.T.);
#42701=ADVANCED_FACE('',(#3846),#41983,.T.);
#42702=ADVANCED_FACE('',(#3847),#116,.T.);
#42703=ADVANCED_FACE('',(#3848),#41984,.T.);
#42704=ADVANCED_FACE('',(#3849),#2221,.T.);
#42705=ADVANCED_FACE('',(#3850),#2222,.T.);
#42706=ADVANCED_FACE('',(#3851),#2223,.T.);
#42707=ADVANCED_FACE('',(#3852),#2224,.T.);
#42708=ADVANCED_FACE('',(#3853),#41985,.T.);
#42709=ADVANCED_FACE('',(#3854),#117,.T.);
#42710=ADVANCED_FACE('',(#3855),#2225,.T.);
#42711=ADVANCED_FACE('',(#3856),#41986,.T.);
#42712=ADVANCED_FACE('',(#3857),#2226,.T.);
#42713=ADVANCED_FACE('',(#3858),#118,.T.);
#42714=ADVANCED_FACE('',(#3859),#119,.T.);
#42715=ADVANCED_FACE('',(#3860),#41987,.T.);
#42716=ADVANCED_FACE('',(#3861),#2227,.T.);
#42717=ADVANCED_FACE('',(#3862),#41988,.T.);
#42718=ADVANCED_FACE('',(#3863),#120,.T.);
#42719=ADVANCED_FACE('',(#3864),#2228,.T.);
#42720=ADVANCED_FACE('',(#3865),#121,.T.);
#42721=ADVANCED_FACE('',(#3866),#41989,.T.);
#42722=ADVANCED_FACE('',(#3867),#122,.T.);
#42723=ADVANCED_FACE('',(#3868),#2229,.T.);
#42724=ADVANCED_FACE('',(#3869),#123,.T.);
#42725=ADVANCED_FACE('',(#3870),#41990,.T.);
#42726=ADVANCED_FACE('',(#3871),#2230,.T.);
#42727=ADVANCED_FACE('',(#3872),#2231,.T.);
#42728=ADVANCED_FACE('',(#3873),#2232,.T.);
#42729=ADVANCED_FACE('',(#3874),#41991,.T.);
#42730=ADVANCED_FACE('',(#3875),#124,.T.);
#42731=ADVANCED_FACE('',(#3876),#2233,.T.);
#42732=ADVANCED_FACE('',(#3877),#2234,.T.);
#42733=ADVANCED_FACE('',(#3878),#41992,.T.);
#42734=ADVANCED_FACE('',(#3879),#41993,.T.);
#42735=ADVANCED_FACE('',(#3880),#2235,.T.);
#42736=ADVANCED_FACE('',(#3881),#2236,.T.);
#42737=ADVANCED_FACE('',(#3882),#41994,.T.);
#42738=ADVANCED_FACE('',(#3883),#125,.T.);
#42739=ADVANCED_FACE('',(#3884),#2237,.T.);
#42740=ADVANCED_FACE('',(#3885),#41995,.T.);
#42741=ADVANCED_FACE('',(#3886),#2238,.T.);
#42742=ADVANCED_FACE('',(#3887),#41996,.T.);
#42743=ADVANCED_FACE('',(#3888),#126,.T.);
#42744=ADVANCED_FACE('',(#3889),#2239,.T.);
#42745=ADVANCED_FACE('',(#3890),#127,.T.);
#42746=ADVANCED_FACE('',(#3891),#128,.T.);
#42747=ADVANCED_FACE('',(#3892),#129,.T.);
#42748=ADVANCED_FACE('',(#3893),#41997,.T.);
#42749=ADVANCED_FACE('',(#3894),#2240,.T.);
#42750=ADVANCED_FACE('',(#3895),#41998,.T.);
#42751=ADVANCED_FACE('',(#3896),#130,.T.);
#42752=ADVANCED_FACE('',(#3897),#2241,.T.);
#42753=ADVANCED_FACE('',(#3898),#131,.T.);
#42754=ADVANCED_FACE('',(#3899),#41999,.T.);
#42755=ADVANCED_FACE('',(#3900),#2242,.T.);
#42756=ADVANCED_FACE('',(#3901),#2243,.T.);
#42757=ADVANCED_FACE('',(#3902),#132,.T.);
#42758=ADVANCED_FACE('',(#3903),#42000,.T.);
#42759=ADVANCED_FACE('',(#3904),#133,.T.);
#42760=ADVANCED_FACE('',(#3905),#2244,.T.);
#42761=ADVANCED_FACE('',(#3906),#2245,.T.);
#42762=ADVANCED_FACE('',(#3907),#42001,.T.);
#42763=ADVANCED_FACE('',(#3908),#42002,.T.);
#42764=ADVANCED_FACE('',(#3909),#2246,.T.);
#42765=ADVANCED_FACE('',(#3910),#2247,.T.);
#42766=ADVANCED_FACE('',(#3911),#42003,.T.);
#42767=ADVANCED_FACE('',(#3912),#134,.T.);
#42768=ADVANCED_FACE('',(#3913),#2248,.T.);
#42769=ADVANCED_FACE('',(#3914),#42004,.T.);
#42770=ADVANCED_FACE('',(#3915),#2249,.T.);
#42771=ADVANCED_FACE('',(#3916),#42005,.T.);
#42772=ADVANCED_FACE('',(#3917),#135,.T.);
#42773=ADVANCED_FACE('',(#3918),#2250,.T.);
#42774=ADVANCED_FACE('',(#3919),#136,.T.);
#42775=ADVANCED_FACE('',(#3920),#42006,.T.);
#42776=ADVANCED_FACE('',(#3921),#137,.T.);
#42777=ADVANCED_FACE('',(#3922),#2251,.T.);
#42778=ADVANCED_FACE('',(#3923),#138,.T.);
#42779=ADVANCED_FACE('',(#3924),#139,.T.);
#42780=ADVANCED_FACE('',(#3925),#140,.T.);
#42781=ADVANCED_FACE('',(#3926),#42007,.T.);
#42782=ADVANCED_FACE('',(#3927),#2252,.T.);
#42783=ADVANCED_FACE('',(#3928),#42008,.T.);
#42784=ADVANCED_FACE('',(#3929),#2253,.T.);
#42785=ADVANCED_FACE('',(#3930),#2254,.T.);
#42786=ADVANCED_FACE('',(#3931),#141,.T.);
#42787=ADVANCED_FACE('',(#3932),#42009,.T.);
#42788=ADVANCED_FACE('',(#3933),#142,.T.);
#42789=ADVANCED_FACE('',(#3934),#2255,.T.);
#42790=ADVANCED_FACE('',(#3935),#143,.T.);
#42791=ADVANCED_FACE('',(#3936),#42010,.T.);
#42792=ADVANCED_FACE('',(#3937),#42011,.T.);
#42793=ADVANCED_FACE('',(#3938),#2256,.T.);
#42794=ADVANCED_FACE('',(#3939),#2257,.T.);
#42795=ADVANCED_FACE('',(#3940),#42012,.T.);
#42796=ADVANCED_FACE('',(#3941),#144,.T.);
#42797=ADVANCED_FACE('',(#3942),#2258,.T.);
#42798=ADVANCED_FACE('',(#3943),#42013,.T.);
#42799=ADVANCED_FACE('',(#3944),#2259,.T.);
#42800=ADVANCED_FACE('',(#3945),#42014,.T.);
#42801=ADVANCED_FACE('',(#3946),#145,.T.);
#42802=ADVANCED_FACE('',(#3947),#2260,.T.);
#42803=ADVANCED_FACE('',(#3948),#146,.T.);
#42804=ADVANCED_FACE('',(#3949),#42015,.T.);
#42805=ADVANCED_FACE('',(#3950),#147,.T.);
#42806=ADVANCED_FACE('',(#3951),#2261,.T.);
#42807=ADVANCED_FACE('',(#3952),#148,.T.);
#42808=ADVANCED_FACE('',(#3953),#42016,.T.);
#42809=ADVANCED_FACE('',(#3954),#149,.T.);
#42810=ADVANCED_FACE('',(#3955),#2262,.T.);
#42811=ADVANCED_FACE('',(#3956),#150,.T.);
#42812=ADVANCED_FACE('',(#3957),#2263,.T.);
#42813=ADVANCED_FACE('',(#3958),#151,.T.);
#42814=ADVANCED_FACE('',(#3959),#42017,.T.);
#42815=ADVANCED_FACE('',(#3960),#2264,.T.);
#42816=ADVANCED_FACE('',(#3961),#42018,.T.);
#42817=ADVANCED_FACE('',(#3962),#152,.T.);
#42818=ADVANCED_FACE('',(#3963),#2265,.T.);
#42819=ADVANCED_FACE('',(#3964),#153,.T.);
#42820=ADVANCED_FACE('',(#3965),#42019,.T.);
#42821=ADVANCED_FACE('',(#3966),#42020,.T.);
#42822=ADVANCED_FACE('',(#3967),#2266,.T.);
#42823=ADVANCED_FACE('',(#3968),#2267,.T.);
#42824=ADVANCED_FACE('',(#3969),#42021,.T.);
#42825=ADVANCED_FACE('',(#3970),#154,.T.);
#42826=ADVANCED_FACE('',(#3971),#2268,.T.);
#42827=ADVANCED_FACE('',(#3972),#42022,.T.);
#42828=ADVANCED_FACE('',(#3973),#2269,.T.);
#42829=ADVANCED_FACE('',(#3974),#42023,.T.);
#42830=ADVANCED_FACE('',(#3975),#155,.T.);
#42831=ADVANCED_FACE('',(#3976),#2270,.T.);
#42832=ADVANCED_FACE('',(#3977),#156,.T.);
#42833=ADVANCED_FACE('',(#3978),#42024,.T.);
#42834=ADVANCED_FACE('',(#3979),#157,.T.);
#42835=ADVANCED_FACE('',(#3980),#2271,.T.);
#42836=ADVANCED_FACE('',(#3981),#158,.T.);
#42837=ADVANCED_FACE('',(#3982),#42025,.T.);
#42838=ADVANCED_FACE('',(#3983),#159,.T.);
#42839=ADVANCED_FACE('',(#3984),#2272,.T.);
#42840=ADVANCED_FACE('',(#3985),#160,.T.);
#42841=ADVANCED_FACE('',(#3986),#42026,.T.);
#42842=ADVANCED_FACE('',(#3987),#2273,.T.);
#42843=ADVANCED_FACE('',(#3988),#2274,.T.);
#42844=ADVANCED_FACE('',(#3989),#161,.T.);
#42845=ADVANCED_FACE('',(#3990),#162,.T.);
#42846=ADVANCED_FACE('',(#3991),#163,.T.);
#42847=ADVANCED_FACE('',(#3992),#42027,.T.);
#42848=ADVANCED_FACE('',(#3993),#2275,.T.);
#42849=ADVANCED_FACE('',(#3994),#42028,.T.);
#42850=ADVANCED_FACE('',(#3995),#42029,.T.);
#42851=ADVANCED_FACE('',(#3996),#2276,.T.);
#42852=ADVANCED_FACE('',(#3997),#2277,.T.);
#42853=ADVANCED_FACE('',(#3998),#42030,.T.);
#42854=ADVANCED_FACE('',(#3999),#164,.T.);
#42855=ADVANCED_FACE('',(#4000),#2278,.T.);
#42856=ADVANCED_FACE('',(#4001),#42031,.T.);
#42857=ADVANCED_FACE('',(#4002),#2279,.T.);
#42858=ADVANCED_FACE('',(#4003),#42032,.T.);
#42859=ADVANCED_FACE('',(#4004),#165,.T.);
#42860=ADVANCED_FACE('',(#4005),#2280,.T.);
#42861=ADVANCED_FACE('',(#4006),#166,.T.);
#42862=ADVANCED_FACE('',(#4007),#42033,.T.);
#42863=ADVANCED_FACE('',(#4008),#167,.T.);
#42864=ADVANCED_FACE('',(#4009),#2281,.T.);
#42865=ADVANCED_FACE('',(#4010),#168,.T.);
#42866=ADVANCED_FACE('',(#4011),#42034,.T.);
#42867=ADVANCED_FACE('',(#4012),#169,.T.);
#42868=ADVANCED_FACE('',(#4013),#2282,.T.);
#42869=ADVANCED_FACE('',(#4014),#170,.T.);
#42870=ADVANCED_FACE('',(#4015),#42035,.T.);
#42871=ADVANCED_FACE('',(#4016),#2283,.T.);
#42872=ADVANCED_FACE('',(#4017),#2284,.T.);
#42873=ADVANCED_FACE('',(#4018),#171,.T.);
#42874=ADVANCED_FACE('',(#4019),#42036,.T.);
#42875=ADVANCED_FACE('',(#4020),#172,.T.);
#42876=ADVANCED_FACE('',(#4021),#2285,.T.);
#42877=ADVANCED_FACE('',(#4022),#173,.T.);
#42878=ADVANCED_FACE('',(#4023),#42037,.T.);
#42879=ADVANCED_FACE('',(#4024),#42038,.T.);
#42880=ADVANCED_FACE('',(#4025),#2286,.T.);
#42881=ADVANCED_FACE('',(#4026),#2287,.T.);
#42882=ADVANCED_FACE('',(#4027),#42039,.T.);
#42883=ADVANCED_FACE('',(#4028),#174,.T.);
#42884=ADVANCED_FACE('',(#4029),#2288,.T.);
#42885=ADVANCED_FACE('',(#4030),#42040,.T.);
#42886=ADVANCED_FACE('',(#4031),#2289,.T.);
#42887=ADVANCED_FACE('',(#4032),#42041,.T.);
#42888=ADVANCED_FACE('',(#4033),#175,.T.);
#42889=ADVANCED_FACE('',(#4034),#2290,.T.);
#42890=ADVANCED_FACE('',(#4035),#176,.T.);
#42891=ADVANCED_FACE('',(#4036),#42042,.T.);
#42892=ADVANCED_FACE('',(#4037),#177,.T.);
#42893=ADVANCED_FACE('',(#4038),#2291,.T.);
#42894=ADVANCED_FACE('',(#4039),#178,.T.);
#42895=ADVANCED_FACE('',(#4040),#42043,.T.);
#42896=ADVANCED_FACE('',(#4041),#179,.T.);
#42897=ADVANCED_FACE('',(#4042),#2292,.T.);
#42898=ADVANCED_FACE('',(#4043),#180,.T.);
#42899=ADVANCED_FACE('',(#4044),#42044,.T.);
#42900=ADVANCED_FACE('',(#4045),#2293,.T.);
#42901=ADVANCED_FACE('',(#4046),#2294,.T.);
#42902=ADVANCED_FACE('',(#4047),#181,.T.);
#42903=ADVANCED_FACE('',(#4048),#42045,.T.);
#42904=ADVANCED_FACE('',(#4049),#182,.T.);
#42905=ADVANCED_FACE('',(#4050),#2295,.T.);
#42906=ADVANCED_FACE('',(#4051),#183,.T.);
#42907=ADVANCED_FACE('',(#4052),#42046,.T.);
#42908=ADVANCED_FACE('',(#4053),#42047,.T.);
#42909=ADVANCED_FACE('',(#4054),#2296,.T.);
#42910=ADVANCED_FACE('',(#4055),#2297,.T.);
#42911=ADVANCED_FACE('',(#4056),#42048,.T.);
#42912=ADVANCED_FACE('',(#4057),#184,.T.);
#42913=ADVANCED_FACE('',(#4058),#2298,.T.);
#42914=ADVANCED_FACE('',(#4059),#42049,.T.);
#42915=ADVANCED_FACE('',(#4060),#2299,.T.);
#42916=ADVANCED_FACE('',(#4061),#42050,.T.);
#42917=ADVANCED_FACE('',(#4062),#185,.T.);
#42918=ADVANCED_FACE('',(#4063),#2300,.T.);
#42919=ADVANCED_FACE('',(#4064),#186,.T.);
#42920=ADVANCED_FACE('',(#4065),#42051,.T.);
#42921=ADVANCED_FACE('',(#4066),#187,.T.);
#42922=ADVANCED_FACE('',(#4067),#2301,.T.);
#42923=ADVANCED_FACE('',(#4068),#188,.T.);
#42924=ADVANCED_FACE('',(#4069),#42052,.T.);
#42925=ADVANCED_FACE('',(#4070),#189,.T.);
#42926=ADVANCED_FACE('',(#4071),#2302,.T.);
#42927=ADVANCED_FACE('',(#4072),#190,.T.);
#42928=ADVANCED_FACE('',(#4073),#42053,.T.);
#42929=ADVANCED_FACE('',(#4074),#2303,.T.);
#42930=ADVANCED_FACE('',(#4075),#2304,.T.);
#42931=ADVANCED_FACE('',(#4076),#191,.T.);
#42932=ADVANCED_FACE('',(#4077),#42054,.T.);
#42933=ADVANCED_FACE('',(#4078),#192,.T.);
#42934=ADVANCED_FACE('',(#4079),#2305,.T.);
#42935=ADVANCED_FACE('',(#4080),#193,.T.);
#42936=ADVANCED_FACE('',(#4081),#42055,.T.);
#42937=ADVANCED_FACE('',(#4082),#42056,.T.);
#42938=ADVANCED_FACE('',(#4083),#2306,.T.);
#42939=ADVANCED_FACE('',(#4084),#2307,.T.);
#42940=ADVANCED_FACE('',(#4085),#42057,.T.);
#42941=ADVANCED_FACE('',(#4086),#194,.T.);
#42942=ADVANCED_FACE('',(#4087),#2308,.T.);
#42943=ADVANCED_FACE('',(#4088),#42058,.T.);
#42944=ADVANCED_FACE('',(#4089),#2309,.T.);
#42945=ADVANCED_FACE('',(#4090),#42059,.T.);
#42946=ADVANCED_FACE('',(#4091),#195,.T.);
#42947=ADVANCED_FACE('',(#4092),#2310,.T.);
#42948=ADVANCED_FACE('',(#4093),#196,.T.);
#42949=ADVANCED_FACE('',(#4094),#42060,.T.);
#42950=ADVANCED_FACE('',(#4095),#197,.T.);
#42951=ADVANCED_FACE('',(#4096),#2311,.T.);
#42952=ADVANCED_FACE('',(#4097),#198,.T.);
#42953=ADVANCED_FACE('',(#4098),#42061,.T.);
#42954=ADVANCED_FACE('',(#4099),#199,.T.);
#42955=ADVANCED_FACE('',(#4100),#2312,.T.);
#42956=ADVANCED_FACE('',(#4101),#200,.T.);
#42957=ADVANCED_FACE('',(#4102),#42062,.T.);
#42958=ADVANCED_FACE('',(#4103),#2313,.T.);
#42959=ADVANCED_FACE('',(#4104),#2314,.T.);
#42960=ADVANCED_FACE('',(#4105),#201,.T.);
#42961=ADVANCED_FACE('',(#4106),#42063,.T.);
#42962=ADVANCED_FACE('',(#4107),#202,.T.);
#42963=ADVANCED_FACE('',(#4108),#2315,.T.);
#42964=ADVANCED_FACE('',(#4109),#203,.T.);
#42965=ADVANCED_FACE('',(#4110),#42064,.T.);
#42966=ADVANCED_FACE('',(#4111),#42065,.T.);
#42967=ADVANCED_FACE('',(#4112),#2316,.T.);
#42968=ADVANCED_FACE('',(#4113),#2317,.T.);
#42969=ADVANCED_FACE('',(#4114),#42066,.T.);
#42970=ADVANCED_FACE('',(#4115),#204,.T.);
#42971=ADVANCED_FACE('',(#4116),#2318,.T.);
#42972=ADVANCED_FACE('',(#4117),#42067,.T.);
#42973=ADVANCED_FACE('',(#4118),#2319,.T.);
#42974=ADVANCED_FACE('',(#4119),#42068,.T.);
#42975=ADVANCED_FACE('',(#4120),#205,.T.);
#42976=ADVANCED_FACE('',(#4121),#2320,.T.);
#42977=ADVANCED_FACE('',(#4122),#206,.T.);
#42978=ADVANCED_FACE('',(#4123),#42069,.T.);
#42979=ADVANCED_FACE('',(#4124),#207,.T.);
#42980=ADVANCED_FACE('',(#4125),#2321,.T.);
#42981=ADVANCED_FACE('',(#4126),#208,.T.);
#42982=ADVANCED_FACE('',(#4127),#42070,.T.);
#42983=ADVANCED_FACE('',(#4128),#209,.T.);
#42984=ADVANCED_FACE('',(#4129),#2322,.T.);
#42985=ADVANCED_FACE('',(#4130),#210,.T.);
#42986=ADVANCED_FACE('',(#4131),#42071,.T.);
#42987=ADVANCED_FACE('',(#4132),#2323,.T.);
#42988=ADVANCED_FACE('',(#4133),#2324,.T.);
#42989=ADVANCED_FACE('',(#4134),#211,.T.);
#42990=ADVANCED_FACE('',(#4135),#42072,.T.);
#42991=ADVANCED_FACE('',(#4136),#212,.T.);
#42992=ADVANCED_FACE('',(#4137),#2325,.T.);
#42993=ADVANCED_FACE('',(#4138),#213,.T.);
#42994=ADVANCED_FACE('',(#4139),#42073,.T.);
#42995=ADVANCED_FACE('',(#4140),#42074,.T.);
#42996=ADVANCED_FACE('',(#4141),#2326,.T.);
#42997=ADVANCED_FACE('',(#4142),#2327,.T.);
#42998=ADVANCED_FACE('',(#4143),#42075,.T.);
#42999=ADVANCED_FACE('',(#4144),#214,.T.);
#43000=ADVANCED_FACE('',(#4145),#2328,.T.);
#43001=ADVANCED_FACE('',(#4146),#42076,.T.);
#43002=ADVANCED_FACE('',(#4147),#2329,.T.);
#43003=ADVANCED_FACE('',(#4148),#42077,.T.);
#43004=ADVANCED_FACE('',(#4149),#215,.T.);
#43005=ADVANCED_FACE('',(#4150),#2330,.T.);
#43006=ADVANCED_FACE('',(#4151),#216,.T.);
#43007=ADVANCED_FACE('',(#4152),#42078,.T.);
#43008=ADVANCED_FACE('',(#4153),#217,.T.);
#43009=ADVANCED_FACE('',(#4154),#2331,.T.);
#43010=ADVANCED_FACE('',(#4155),#218,.T.);
#43011=ADVANCED_FACE('',(#4156),#42079,.T.);
#43012=ADVANCED_FACE('',(#4157),#219,.T.);
#43013=ADVANCED_FACE('',(#4158),#2332,.T.);
#43014=ADVANCED_FACE('',(#4159),#220,.T.);
#43015=ADVANCED_FACE('',(#4160),#42080,.T.);
#43016=ADVANCED_FACE('',(#4161),#2333,.T.);
#43017=ADVANCED_FACE('',(#4162),#2334,.T.);
#43018=ADVANCED_FACE('',(#4163),#221,.T.);
#43019=ADVANCED_FACE('',(#4164),#42081,.T.);
#43020=ADVANCED_FACE('',(#4165),#222,.T.);
#43021=ADVANCED_FACE('',(#4166),#2335,.T.);
#43022=ADVANCED_FACE('',(#4167),#223,.T.);
#43023=ADVANCED_FACE('',(#4168),#42082,.T.);
#43024=ADVANCED_FACE('',(#4169),#42083,.T.);
#43025=ADVANCED_FACE('',(#4170),#2336,.T.);
#43026=ADVANCED_FACE('',(#4171),#2337,.T.);
#43027=ADVANCED_FACE('',(#4172),#42084,.T.);
#43028=ADVANCED_FACE('',(#4173),#224,.T.);
#43029=ADVANCED_FACE('',(#4174),#2338,.T.);
#43030=ADVANCED_FACE('',(#4175),#42085,.T.);
#43031=ADVANCED_FACE('',(#4176),#2339,.T.);
#43032=ADVANCED_FACE('',(#4177),#42086,.T.);
#43033=ADVANCED_FACE('',(#4178),#225,.T.);
#43034=ADVANCED_FACE('',(#4179),#2340,.T.);
#43035=ADVANCED_FACE('',(#4180),#226,.T.);
#43036=ADVANCED_FACE('',(#4181),#42087,.T.);
#43037=ADVANCED_FACE('',(#4182),#227,.T.);
#43038=ADVANCED_FACE('',(#4183),#2341,.T.);
#43039=ADVANCED_FACE('',(#4184),#228,.T.);
#43040=ADVANCED_FACE('',(#4185),#42088,.T.);
#43041=ADVANCED_FACE('',(#4186),#229,.T.);
#43042=ADVANCED_FACE('',(#4187),#2342,.T.);
#43043=ADVANCED_FACE('',(#4188),#230,.T.);
#43044=ADVANCED_FACE('',(#4189),#42089,.T.);
#43045=ADVANCED_FACE('',(#4190),#2343,.T.);
#43046=ADVANCED_FACE('',(#4191),#2344,.T.);
#43047=ADVANCED_FACE('',(#4192),#231,.T.);
#43048=ADVANCED_FACE('',(#4193),#42090,.T.);
#43049=ADVANCED_FACE('',(#4194),#232,.T.);
#43050=ADVANCED_FACE('',(#4195),#2345,.T.);
#43051=ADVANCED_FACE('',(#4196),#233,.T.);
#43052=ADVANCED_FACE('',(#4197),#42091,.T.);
#43053=ADVANCED_FACE('',(#4198),#42092,.T.);
#43054=ADVANCED_FACE('',(#4199),#2346,.T.);
#43055=ADVANCED_FACE('',(#4200),#2347,.T.);
#43056=ADVANCED_FACE('',(#4201),#42093,.T.);
#43057=ADVANCED_FACE('',(#4202),#234,.T.);
#43058=ADVANCED_FACE('',(#4203),#2348,.T.);
#43059=ADVANCED_FACE('',(#4204),#42094,.T.);
#43060=ADVANCED_FACE('',(#4205),#2349,.T.);
#43061=ADVANCED_FACE('',(#4206),#42095,.T.);
#43062=ADVANCED_FACE('',(#4207),#235,.T.);
#43063=ADVANCED_FACE('',(#4208),#2350,.T.);
#43064=ADVANCED_FACE('',(#4209),#236,.T.);
#43065=ADVANCED_FACE('',(#4210),#42096,.T.);
#43066=ADVANCED_FACE('',(#4211),#237,.T.);
#43067=ADVANCED_FACE('',(#4212),#2351,.T.);
#43068=ADVANCED_FACE('',(#4213),#238,.T.);
#43069=ADVANCED_FACE('',(#4214),#42097,.T.);
#43070=ADVANCED_FACE('',(#4215),#239,.T.);
#43071=ADVANCED_FACE('',(#4216),#2352,.T.);
#43072=ADVANCED_FACE('',(#4217),#240,.T.);
#43073=ADVANCED_FACE('',(#4218),#42098,.T.);
#43074=ADVANCED_FACE('',(#4219),#2353,.T.);
#43075=ADVANCED_FACE('',(#4220),#2354,.T.);
#43076=ADVANCED_FACE('',(#4221),#241,.T.);
#43077=ADVANCED_FACE('',(#4222),#42099,.T.);
#43078=ADVANCED_FACE('',(#4223),#242,.T.);
#43079=ADVANCED_FACE('',(#4224),#2355,.T.);
#43080=ADVANCED_FACE('',(#4225),#243,.T.);
#43081=ADVANCED_FACE('',(#4226),#42100,.T.);
#43082=ADVANCED_FACE('',(#4227),#42101,.T.);
#43083=ADVANCED_FACE('',(#4228),#2356,.T.);
#43084=ADVANCED_FACE('',(#4229),#2357,.T.);
#43085=ADVANCED_FACE('',(#4230),#42102,.T.);
#43086=ADVANCED_FACE('',(#4231),#244,.T.);
#43087=ADVANCED_FACE('',(#4232),#2358,.T.);
#43088=ADVANCED_FACE('',(#4233),#42103,.T.);
#43089=ADVANCED_FACE('',(#4234),#2359,.T.);
#43090=ADVANCED_FACE('',(#4235),#42104,.T.);
#43091=ADVANCED_FACE('',(#4236),#245,.T.);
#43092=ADVANCED_FACE('',(#4237),#2360,.T.);
#43093=ADVANCED_FACE('',(#4238),#2361,.T.);
#43094=ADVANCED_FACE('',(#4239),#42105,.T.);
#43095=ADVANCED_FACE('',(#4240),#246,.T.);
#43096=ADVANCED_FACE('',(#4241),#2362,.T.);
#43097=ADVANCED_FACE('',(#4242),#247,.T.);
#43098=ADVANCED_FACE('',(#4243),#42106,.T.);
#43099=ADVANCED_FACE('',(#4244),#248,.T.);
#43100=ADVANCED_FACE('',(#4245),#2363,.T.);
#43101=ADVANCED_FACE('',(#4246),#249,.T.);
#43102=ADVANCED_FACE('',(#4247),#42107,.T.);
#43103=ADVANCED_FACE('',(#4248),#2364,.T.);
#43104=ADVANCED_FACE('',(#4249),#2365,.T.);
#43105=ADVANCED_FACE('',(#4250),#250,.T.);
#43106=ADVANCED_FACE('',(#4251),#42108,.T.);
#43107=ADVANCED_FACE('',(#4252),#251,.T.);
#43108=ADVANCED_FACE('',(#4253),#2366,.T.);
#43109=ADVANCED_FACE('',(#4254),#252,.T.);
#43110=ADVANCED_FACE('',(#4255),#42109,.T.);
#43111=ADVANCED_FACE('',(#4256),#42110,.T.);
#43112=ADVANCED_FACE('',(#4257),#2367,.T.);
#43113=ADVANCED_FACE('',(#4258),#2368,.T.);
#43114=ADVANCED_FACE('',(#4259),#42111,.T.);
#43115=ADVANCED_FACE('',(#4260),#253,.T.);
#43116=ADVANCED_FACE('',(#4261),#2369,.T.);
#43117=ADVANCED_FACE('',(#4262),#42112,.T.);
#43118=ADVANCED_FACE('',(#4263),#2370,.T.);
#43119=ADVANCED_FACE('',(#4264),#42113,.T.);
#43120=ADVANCED_FACE('',(#4265),#254,.T.);
#43121=ADVANCED_FACE('',(#4266),#2371,.T.);
#43122=ADVANCED_FACE('',(#4267),#255,.T.);
#43123=ADVANCED_FACE('',(#4268),#42114,.T.);
#43124=ADVANCED_FACE('',(#4269),#256,.T.);
#43125=ADVANCED_FACE('',(#4270),#2372,.T.);
#43126=ADVANCED_FACE('',(#4271),#257,.T.);
#43127=ADVANCED_FACE('',(#4272),#42115,.T.);
#43128=ADVANCED_FACE('',(#4273),#258,.T.);
#43129=ADVANCED_FACE('',(#4274),#2373,.T.);
#43130=ADVANCED_FACE('',(#4275),#259,.T.);
#43131=ADVANCED_FACE('',(#4276),#42116,.T.);
#43132=ADVANCED_FACE('',(#4277),#2374,.T.);
#43133=ADVANCED_FACE('',(#4278),#2375,.T.);
#43134=ADVANCED_FACE('',(#4279),#260,.T.);
#43135=ADVANCED_FACE('',(#4280),#42117,.T.);
#43136=ADVANCED_FACE('',(#4281),#261,.T.);
#43137=ADVANCED_FACE('',(#4282),#2376,.T.);
#43138=ADVANCED_FACE('',(#4283),#262,.T.);
#43139=ADVANCED_FACE('',(#4284),#42118,.T.);
#43140=ADVANCED_FACE('',(#4285),#42119,.T.);
#43141=ADVANCED_FACE('',(#4286),#2377,.T.);
#43142=ADVANCED_FACE('',(#4287),#2378,.T.);
#43143=ADVANCED_FACE('',(#4288),#42120,.T.);
#43144=ADVANCED_FACE('',(#4289),#263,.T.);
#43145=ADVANCED_FACE('',(#4290),#2379,.T.);
#43146=ADVANCED_FACE('',(#4291),#42121,.T.);
#43147=ADVANCED_FACE('',(#4292),#2380,.T.);
#43148=ADVANCED_FACE('',(#4293),#42122,.T.);
#43149=ADVANCED_FACE('',(#4294),#264,.T.);
#43150=ADVANCED_FACE('',(#4295),#2381,.T.);
#43151=ADVANCED_FACE('',(#4296),#265,.T.);
#43152=ADVANCED_FACE('',(#4297),#42123,.T.);
#43153=ADVANCED_FACE('',(#4298),#266,.T.);
#43154=ADVANCED_FACE('',(#4299),#2382,.T.);
#43155=ADVANCED_FACE('',(#4300),#267,.T.);
#43156=ADVANCED_FACE('',(#4301),#42124,.T.);
#43157=ADVANCED_FACE('',(#4302),#268,.T.);
#43158=ADVANCED_FACE('',(#4303),#2383,.T.);
#43159=ADVANCED_FACE('',(#4304),#269,.T.);
#43160=ADVANCED_FACE('',(#4305),#42125,.T.);
#43161=ADVANCED_FACE('',(#4306),#2384,.T.);
#43162=ADVANCED_FACE('',(#4307),#2385,.T.);
#43163=ADVANCED_FACE('',(#4308),#270,.T.);
#43164=ADVANCED_FACE('',(#4309),#42126,.T.);
#43165=ADVANCED_FACE('',(#4310),#271,.T.);
#43166=ADVANCED_FACE('',(#4311),#2386,.T.);
#43167=ADVANCED_FACE('',(#4312),#272,.T.);
#43168=ADVANCED_FACE('',(#4313),#42127,.T.);
#43169=ADVANCED_FACE('',(#4314),#42128,.T.);
#43170=ADVANCED_FACE('',(#4315),#2387,.T.);
#43171=ADVANCED_FACE('',(#4316),#2388,.T.);
#43172=ADVANCED_FACE('',(#4317),#42129,.T.);
#43173=ADVANCED_FACE('',(#4318),#273,.T.);
#43174=ADVANCED_FACE('',(#4319),#2389,.T.);
#43175=ADVANCED_FACE('',(#4320),#42130,.T.);
#43176=ADVANCED_FACE('',(#4321),#2390,.T.);
#43177=ADVANCED_FACE('',(#4322),#42131,.T.);
#43178=ADVANCED_FACE('',(#4323),#274,.T.);
#43179=ADVANCED_FACE('',(#4324),#2391,.T.);
#43180=ADVANCED_FACE('',(#4325),#275,.T.);
#43181=ADVANCED_FACE('',(#4326),#42132,.T.);
#43182=ADVANCED_FACE('',(#4327),#276,.T.);
#43183=ADVANCED_FACE('',(#4328),#2392,.T.);
#43184=ADVANCED_FACE('',(#4329),#277,.T.);
#43185=ADVANCED_FACE('',(#4330),#42133,.T.);
#43186=ADVANCED_FACE('',(#4331),#278,.T.);
#43187=ADVANCED_FACE('',(#4332),#2393,.T.);
#43188=ADVANCED_FACE('',(#4333),#279,.T.);
#43189=ADVANCED_FACE('',(#4334),#42134,.T.);
#43190=ADVANCED_FACE('',(#4335),#2394,.T.);
#43191=ADVANCED_FACE('',(#4336),#2395,.T.);
#43192=ADVANCED_FACE('',(#4337),#280,.T.);
#43193=ADVANCED_FACE('',(#4338),#42135,.T.);
#43194=ADVANCED_FACE('',(#4339),#281,.T.);
#43195=ADVANCED_FACE('',(#4340),#2396,.T.);
#43196=ADVANCED_FACE('',(#4341),#282,.T.);
#43197=ADVANCED_FACE('',(#4342),#42136,.T.);
#43198=ADVANCED_FACE('',(#4343),#42137,.T.);
#43199=ADVANCED_FACE('',(#4344),#2397,.T.);
#43200=ADVANCED_FACE('',(#4345),#2398,.T.);
#43201=ADVANCED_FACE('',(#4346),#42138,.T.);
#43202=ADVANCED_FACE('',(#4347),#283,.T.);
#43203=ADVANCED_FACE('',(#4348),#2399,.T.);
#43204=ADVANCED_FACE('',(#4349),#42139,.T.);
#43205=ADVANCED_FACE('',(#4350),#2400,.T.);
#43206=ADVANCED_FACE('',(#4351),#42140,.T.);
#43207=ADVANCED_FACE('',(#4352),#284,.T.);
#43208=ADVANCED_FACE('',(#4353),#2401,.T.);
#43209=ADVANCED_FACE('',(#4354),#285,.T.);
#43210=ADVANCED_FACE('',(#4355),#42141,.T.);
#43211=ADVANCED_FACE('',(#4356),#286,.T.);
#43212=ADVANCED_FACE('',(#4357),#2402,.T.);
#43213=ADVANCED_FACE('',(#4358),#287,.T.);
#43214=ADVANCED_FACE('',(#4359),#42142,.T.);
#43215=ADVANCED_FACE('',(#4360),#288,.T.);
#43216=ADVANCED_FACE('',(#4361),#2403,.T.);
#43217=ADVANCED_FACE('',(#4362),#289,.T.);
#43218=ADVANCED_FACE('',(#4363),#42143,.T.);
#43219=ADVANCED_FACE('',(#4364),#2404,.T.);
#43220=ADVANCED_FACE('',(#4365),#2405,.T.);
#43221=ADVANCED_FACE('',(#4366),#290,.T.);
#43222=ADVANCED_FACE('',(#4367),#42144,.T.);
#43223=ADVANCED_FACE('',(#4368),#291,.T.);
#43224=ADVANCED_FACE('',(#4369),#2406,.T.);
#43225=ADVANCED_FACE('',(#4370),#292,.T.);
#43226=ADVANCED_FACE('',(#4371),#42145,.T.);
#43227=ADVANCED_FACE('',(#4372),#42146,.T.);
#43228=ADVANCED_FACE('',(#4373),#2407,.T.);
#43229=ADVANCED_FACE('',(#4374),#2408,.T.);
#43230=ADVANCED_FACE('',(#4375),#42147,.T.);
#43231=ADVANCED_FACE('',(#4376),#293,.T.);
#43232=ADVANCED_FACE('',(#4377),#2409,.T.);
#43233=ADVANCED_FACE('',(#4378),#42148,.T.);
#43234=ADVANCED_FACE('',(#4379),#2410,.T.);
#43235=ADVANCED_FACE('',(#4380),#42149,.T.);
#43236=ADVANCED_FACE('',(#4381),#294,.T.);
#43237=ADVANCED_FACE('',(#4382),#2411,.T.);
#43238=ADVANCED_FACE('',(#4383),#2412,.T.);
#43239=ADVANCED_FACE('',(#4384),#42150,.T.);
#43240=ADVANCED_FACE('',(#4385),#295,.T.);
#43241=ADVANCED_FACE('',(#4386),#2413,.T.);
#43242=ADVANCED_FACE('',(#4387),#296,.T.);
#43243=ADVANCED_FACE('',(#4388),#42151,.T.);
#43244=ADVANCED_FACE('',(#4389),#297,.T.);
#43245=ADVANCED_FACE('',(#4390),#2414,.T.);
#43246=ADVANCED_FACE('',(#4391),#298,.T.);
#43247=ADVANCED_FACE('',(#4392),#42152,.T.);
#43248=ADVANCED_FACE('',(#4393),#2415,.T.);
#43249=ADVANCED_FACE('',(#4394),#2416,.T.);
#43250=ADVANCED_FACE('',(#4395),#299,.T.);
#43251=ADVANCED_FACE('',(#4396),#42153,.T.);
#43252=ADVANCED_FACE('',(#4397),#300,.T.);
#43253=ADVANCED_FACE('',(#4398),#2417,.T.);
#43254=ADVANCED_FACE('',(#4399),#301,.T.);
#43255=ADVANCED_FACE('',(#4400),#42154,.T.);
#43256=ADVANCED_FACE('',(#4401),#42155,.T.);
#43257=ADVANCED_FACE('',(#4402),#2418,.T.);
#43258=ADVANCED_FACE('',(#4403),#2419,.T.);
#43259=ADVANCED_FACE('',(#4404),#42156,.T.);
#43260=ADVANCED_FACE('',(#4405),#302,.T.);
#43261=ADVANCED_FACE('',(#4406),#2420,.T.);
#43262=ADVANCED_FACE('',(#4407),#42157,.T.);
#43263=ADVANCED_FACE('',(#4408),#2421,.T.);
#43264=ADVANCED_FACE('',(#4409),#42158,.T.);
#43265=ADVANCED_FACE('',(#4410),#303,.T.);
#43266=ADVANCED_FACE('',(#4411),#2422,.T.);
#43267=ADVANCED_FACE('',(#4412),#304,.T.);
#43268=ADVANCED_FACE('',(#4413),#42159,.T.);
#43269=ADVANCED_FACE('',(#4414),#2423,.T.);
#43270=ADVANCED_FACE('',(#4415),#2424,.T.);
#43271=ADVANCED_FACE('',(#4416),#305,.T.);
#43272=ADVANCED_FACE('',(#4417),#42160,.T.);
#43273=ADVANCED_FACE('',(#4418),#306,.T.);
#43274=ADVANCED_FACE('',(#4419),#2425,.T.);
#43275=ADVANCED_FACE('',(#4420),#307,.T.);
#43276=ADVANCED_FACE('',(#4421),#42161,.T.);
#43277=ADVANCED_FACE('',(#4422),#2426,.T.);
#43278=ADVANCED_FACE('',(#4423),#2427,.T.);
#43279=ADVANCED_FACE('',(#4424),#308,.T.);
#43280=ADVANCED_FACE('',(#4425),#42162,.T.);
#43281=ADVANCED_FACE('',(#4426),#309,.T.);
#43282=ADVANCED_FACE('',(#4427),#2428,.T.);
#43283=ADVANCED_FACE('',(#4428),#310,.T.);
#43284=ADVANCED_FACE('',(#4429),#42163,.T.);
#43285=ADVANCED_FACE('',(#4430),#42164,.T.);
#43286=ADVANCED_FACE('',(#4431),#2429,.T.);
#43287=ADVANCED_FACE('',(#4432),#2430,.T.);
#43288=ADVANCED_FACE('',(#4433),#42165,.T.);
#43289=ADVANCED_FACE('',(#4434),#311,.T.);
#43290=ADVANCED_FACE('',(#4435),#2431,.T.);
#43291=ADVANCED_FACE('',(#4436),#42166,.T.);
#43292=ADVANCED_FACE('',(#4437),#2432,.T.);
#43293=ADVANCED_FACE('',(#4438),#42167,.T.);
#43294=ADVANCED_FACE('',(#4439),#312,.T.);
#43295=ADVANCED_FACE('',(#4440),#2433,.T.);
#43296=ADVANCED_FACE('',(#4441),#2434,.T.);
#43297=ADVANCED_FACE('',(#4442),#42168,.T.);
#43298=ADVANCED_FACE('',(#4443),#313,.T.);
#43299=ADVANCED_FACE('',(#4444),#2435,.T.);
#43300=ADVANCED_FACE('',(#4445),#314,.T.);
#43301=ADVANCED_FACE('',(#4446),#42169,.T.);
#43302=ADVANCED_FACE('',(#4447),#315,.T.);
#43303=ADVANCED_FACE('',(#4448),#2436,.T.);
#43304=ADVANCED_FACE('',(#4449),#2437,.T.);
#43305=ADVANCED_FACE('',(#4450),#42170,.T.);
#43306=ADVANCED_FACE('',(#4451),#2438,.T.);
#43307=ADVANCED_FACE('',(#4452),#2439,.T.);
#43308=ADVANCED_FACE('',(#4453),#316,.T.);
#43309=ADVANCED_FACE('',(#4454),#42171,.T.);
#43310=ADVANCED_FACE('',(#4455),#317,.T.);
#43311=ADVANCED_FACE('',(#4456),#2440,.T.);
#43312=ADVANCED_FACE('',(#4457),#318,.T.);
#43313=ADVANCED_FACE('',(#4458),#42172,.T.);
#43314=ADVANCED_FACE('',(#4459),#42173,.T.);
#43315=ADVANCED_FACE('',(#4460),#2441,.T.);
#43316=ADVANCED_FACE('',(#4461),#2442,.T.);
#43317=ADVANCED_FACE('',(#4462),#42174,.T.);
#43318=ADVANCED_FACE('',(#4463),#319,.T.);
#43319=ADVANCED_FACE('',(#4464),#2443,.T.);
#43320=ADVANCED_FACE('',(#4465),#42175,.T.);
#43321=ADVANCED_FACE('',(#4466),#2444,.T.);
#43322=ADVANCED_FACE('',(#4467),#42176,.T.);
#43323=ADVANCED_FACE('',(#4468),#320,.T.);
#43324=ADVANCED_FACE('',(#4469),#2445,.T.);
#43325=ADVANCED_FACE('',(#4470),#321,.T.);
#43326=ADVANCED_FACE('',(#4471),#42177,.T.);
#43327=ADVANCED_FACE('',(#4472),#322,.T.);
#43328=ADVANCED_FACE('',(#4473),#2446,.T.);
#43329=ADVANCED_FACE('',(#4474),#323,.T.);
#43330=ADVANCED_FACE('',(#4475),#42178,.T.);
#43331=ADVANCED_FACE('',(#4476),#324,.T.);
#43332=ADVANCED_FACE('',(#4477),#2447,.T.);
#43333=ADVANCED_FACE('',(#4478),#325,.T.);
#43334=ADVANCED_FACE('',(#4479),#42179,.T.);
#43335=ADVANCED_FACE('',(#4480),#2448,.T.);
#43336=ADVANCED_FACE('',(#4481),#2449,.T.);
#43337=ADVANCED_FACE('',(#4482),#2450,.T.);
#43338=ADVANCED_FACE('',(#4483),#42180,.T.);
#43339=ADVANCED_FACE('',(#4484),#326,.T.);
#43340=ADVANCED_FACE('',(#4485),#2451,.T.);
#43341=ADVANCED_FACE('',(#4486),#327,.T.);
#43342=ADVANCED_FACE('',(#4487),#42181,.T.);
#43343=ADVANCED_FACE('',(#4488),#42182,.T.);
#43344=ADVANCED_FACE('',(#4489),#2452,.T.);
#43345=ADVANCED_FACE('',(#4490),#2453,.T.);
#43346=ADVANCED_FACE('',(#4491),#42183,.T.);
#43347=ADVANCED_FACE('',(#4492),#328,.T.);
#43348=ADVANCED_FACE('',(#4493),#2454,.T.);
#43349=ADVANCED_FACE('',(#4494),#42184,.T.);
#43350=ADVANCED_FACE('',(#4495),#2455,.T.);
#43351=ADVANCED_FACE('',(#4496),#42185,.T.);
#43352=ADVANCED_FACE('',(#4497),#329,.T.);
#43353=ADVANCED_FACE('',(#4498),#2456,.T.);
#43354=ADVANCED_FACE('',(#4499),#330,.T.);
#43355=ADVANCED_FACE('',(#4500),#42186,.T.);
#43356=ADVANCED_FACE('',(#4501),#331,.T.);
#43357=ADVANCED_FACE('',(#4502),#2457,.T.);
#43358=ADVANCED_FACE('',(#4503),#332,.T.);
#43359=ADVANCED_FACE('',(#4504),#42187,.T.);
#43360=ADVANCED_FACE('',(#4505),#333,.T.);
#43361=ADVANCED_FACE('',(#4506),#2458,.T.);
#43362=ADVANCED_FACE('',(#4507),#334,.T.);
#43363=ADVANCED_FACE('',(#4508),#42188,.T.);
#43364=ADVANCED_FACE('',(#4509),#2459,.T.);
#43365=ADVANCED_FACE('',(#4510),#2460,.T.);
#43366=ADVANCED_FACE('',(#4511),#335,.T.);
#43367=ADVANCED_FACE('',(#4512),#42189,.T.);
#43368=ADVANCED_FACE('',(#4513),#336,.T.);
#43369=ADVANCED_FACE('',(#4514),#2461,.T.);
#43370=ADVANCED_FACE('',(#4515),#2462,.T.);
#43371=ADVANCED_FACE('',(#4516),#42190,.T.);
#43372=ADVANCED_FACE('',(#4517),#42191,.T.);
#43373=ADVANCED_FACE('',(#4518),#2463,.T.);
#43374=ADVANCED_FACE('',(#4519),#2464,.T.);
#43375=ADVANCED_FACE('',(#4520),#42192,.T.);
#43376=ADVANCED_FACE('',(#4521),#337,.T.);
#43377=ADVANCED_FACE('',(#4522),#2465,.T.);
#43378=ADVANCED_FACE('',(#4523),#42193,.T.);
#43379=ADVANCED_FACE('',(#4524),#2466,.T.);
#43380=ADVANCED_FACE('',(#4525),#42194,.T.);
#43381=ADVANCED_FACE('',(#4526),#338,.T.);
#43382=ADVANCED_FACE('',(#4527),#2467,.T.);
#43383=ADVANCED_FACE('',(#4528),#339,.T.);
#43384=ADVANCED_FACE('',(#4529),#42195,.T.);
#43385=ADVANCED_FACE('',(#4530),#340,.T.);
#43386=ADVANCED_FACE('',(#4531),#2468,.T.);
#43387=ADVANCED_FACE('',(#4532),#341,.T.);
#43388=ADVANCED_FACE('',(#4533),#42196,.T.);
#43389=ADVANCED_FACE('',(#4534),#342,.T.);
#43390=ADVANCED_FACE('',(#4535),#2469,.T.);
#43391=ADVANCED_FACE('',(#4536),#343,.T.);
#43392=ADVANCED_FACE('',(#4537),#42197,.T.);
#43393=ADVANCED_FACE('',(#4538),#2470,.T.);
#43394=ADVANCED_FACE('',(#4539),#2471,.T.);
#43395=ADVANCED_FACE('',(#4540),#344,.T.);
#43396=ADVANCED_FACE('',(#4541),#42198,.T.);
#43397=ADVANCED_FACE('',(#4542),#345,.T.);
#43398=ADVANCED_FACE('',(#4543),#2472,.T.);
#43399=ADVANCED_FACE('',(#4544),#346,.T.);
#43400=ADVANCED_FACE('',(#4545),#42199,.T.);
#43401=ADVANCED_FACE('',(#4546),#42200,.T.);
#43402=ADVANCED_FACE('',(#4547),#2473,.T.);
#43403=ADVANCED_FACE('',(#4548),#2474,.T.);
#43404=ADVANCED_FACE('',(#4549),#42201,.T.);
#43405=ADVANCED_FACE('',(#4550),#347,.T.);
#43406=ADVANCED_FACE('',(#4551),#2475,.T.);
#43407=ADVANCED_FACE('',(#4552),#42202,.T.);
#43408=ADVANCED_FACE('',(#4553),#2476,.T.);
#43409=ADVANCED_FACE('',(#4554),#42203,.T.);
#43410=ADVANCED_FACE('',(#4555),#348,.T.);
#43411=ADVANCED_FACE('',(#4556),#2477,.T.);
#43412=ADVANCED_FACE('',(#4557),#349,.T.);
#43413=ADVANCED_FACE('',(#4558),#42204,.T.);
#43414=ADVANCED_FACE('',(#4559),#350,.T.);
#43415=ADVANCED_FACE('',(#4560),#2478,.T.);
#43416=ADVANCED_FACE('',(#4561),#351,.T.);
#43417=ADVANCED_FACE('',(#4562),#42205,.T.);
#43418=ADVANCED_FACE('',(#4563),#352,.T.);
#43419=ADVANCED_FACE('',(#4564),#2479,.T.);
#43420=ADVANCED_FACE('',(#4565),#353,.T.);
#43421=ADVANCED_FACE('',(#4566),#42206,.T.);
#43422=ADVANCED_FACE('',(#4567),#2480,.T.);
#43423=ADVANCED_FACE('',(#4568),#2481,.T.);
#43424=ADVANCED_FACE('',(#4569),#354,.T.);
#43425=ADVANCED_FACE('',(#4570),#42207,.T.);
#43426=ADVANCED_FACE('',(#4571),#355,.T.);
#43427=ADVANCED_FACE('',(#4572),#2482,.T.);
#43428=ADVANCED_FACE('',(#4573),#356,.T.);
#43429=ADVANCED_FACE('',(#4574),#42208,.T.);
#43430=ADVANCED_FACE('',(#4575),#42209,.T.);
#43431=ADVANCED_FACE('',(#4576),#2483,.T.);
#43432=ADVANCED_FACE('',(#4577),#2484,.T.);
#43433=ADVANCED_FACE('',(#4578),#42210,.T.);
#43434=ADVANCED_FACE('',(#4579),#357,.T.);
#43435=ADVANCED_FACE('',(#4580),#2485,.T.);
#43436=ADVANCED_FACE('',(#4581),#42211,.T.);
#43437=ADVANCED_FACE('',(#4582),#2486,.T.);
#43438=ADVANCED_FACE('',(#4583),#42212,.T.);
#43439=ADVANCED_FACE('',(#4584),#358,.T.);
#43440=ADVANCED_FACE('',(#4585),#2487,.T.);
#43441=ADVANCED_FACE('',(#4586),#359,.T.);
#43442=ADVANCED_FACE('',(#4587),#42213,.T.);
#43443=ADVANCED_FACE('',(#4588),#360,.T.);
#43444=ADVANCED_FACE('',(#4589),#2488,.T.);
#43445=ADVANCED_FACE('',(#4590),#361,.T.);
#43446=ADVANCED_FACE('',(#4591),#42214,.T.);
#43447=ADVANCED_FACE('',(#4592),#362,.T.);
#43448=ADVANCED_FACE('',(#4593),#2489,.T.);
#43449=ADVANCED_FACE('',(#4594),#363,.T.);
#43450=ADVANCED_FACE('',(#4595),#42215,.T.);
#43451=ADVANCED_FACE('',(#4596),#2490,.T.);
#43452=ADVANCED_FACE('',(#4597),#2491,.T.);
#43453=ADVANCED_FACE('',(#4598),#364,.T.);
#43454=ADVANCED_FACE('',(#4599),#42216,.T.);
#43455=ADVANCED_FACE('',(#4600),#365,.T.);
#43456=ADVANCED_FACE('',(#4601),#2492,.T.);
#43457=ADVANCED_FACE('',(#4602),#366,.T.);
#43458=ADVANCED_FACE('',(#4603),#42217,.T.);
#43459=ADVANCED_FACE('',(#4604),#42218,.T.);
#43460=ADVANCED_FACE('',(#4605),#2493,.T.);
#43461=ADVANCED_FACE('',(#4606),#2494,.T.);
#43462=ADVANCED_FACE('',(#4607),#42219,.T.);
#43463=ADVANCED_FACE('',(#4608),#367,.T.);
#43464=ADVANCED_FACE('',(#4609),#2495,.T.);
#43465=ADVANCED_FACE('',(#4610),#42220,.T.);
#43466=ADVANCED_FACE('',(#4611),#2496,.T.);
#43467=ADVANCED_FACE('',(#4612),#42221,.T.);
#43468=ADVANCED_FACE('',(#4613),#368,.T.);
#43469=ADVANCED_FACE('',(#4614),#2497,.T.);
#43470=ADVANCED_FACE('',(#4615),#369,.T.);
#43471=ADVANCED_FACE('',(#4616),#42222,.T.);
#43472=ADVANCED_FACE('',(#4617),#370,.T.);
#43473=ADVANCED_FACE('',(#4618),#2498,.T.);
#43474=ADVANCED_FACE('',(#4619),#371,.T.);
#43475=ADVANCED_FACE('',(#4620),#42223,.T.);
#43476=ADVANCED_FACE('',(#4621),#372,.T.);
#43477=ADVANCED_FACE('',(#4622),#2499,.T.);
#43478=ADVANCED_FACE('',(#4623),#373,.T.);
#43479=ADVANCED_FACE('',(#4624),#42224,.T.);
#43480=ADVANCED_FACE('',(#4625),#2500,.T.);
#43481=ADVANCED_FACE('',(#4626),#2501,.T.);
#43482=ADVANCED_FACE('',(#4627),#374,.T.);
#43483=ADVANCED_FACE('',(#4628),#42225,.T.);
#43484=ADVANCED_FACE('',(#4629),#375,.T.);
#43485=ADVANCED_FACE('',(#4630),#2502,.T.);
#43486=ADVANCED_FACE('',(#4631),#376,.T.);
#43487=ADVANCED_FACE('',(#4632),#42226,.T.);
#43488=ADVANCED_FACE('',(#4633),#42227,.T.);
#43489=ADVANCED_FACE('',(#4634),#2503,.T.);
#43490=ADVANCED_FACE('',(#4635),#2504,.T.);
#43491=ADVANCED_FACE('',(#4636),#42228,.T.);
#43492=ADVANCED_FACE('',(#4637),#377,.T.);
#43493=ADVANCED_FACE('',(#4638),#2505,.T.);
#43494=ADVANCED_FACE('',(#4639),#42229,.T.);
#43495=ADVANCED_FACE('',(#4640),#2506,.T.);
#43496=ADVANCED_FACE('',(#4641),#42230,.T.);
#43497=ADVANCED_FACE('',(#4642),#378,.T.);
#43498=ADVANCED_FACE('',(#4643),#2507,.T.);
#43499=ADVANCED_FACE('',(#4644),#379,.T.);
#43500=ADVANCED_FACE('',(#4645),#42231,.T.);
#43501=ADVANCED_FACE('',(#4646),#380,.T.);
#43502=ADVANCED_FACE('',(#4647),#2508,.T.);
#43503=ADVANCED_FACE('',(#4648),#381,.T.);
#43504=ADVANCED_FACE('',(#4649),#42232,.T.);
#43505=ADVANCED_FACE('',(#4650),#382,.T.);
#43506=ADVANCED_FACE('',(#4651),#2509,.T.);
#43507=ADVANCED_FACE('',(#4652),#383,.T.);
#43508=ADVANCED_FACE('',(#4653),#42233,.T.);
#43509=ADVANCED_FACE('',(#4654),#2510,.T.);
#43510=ADVANCED_FACE('',(#4655),#2511,.T.);
#43511=ADVANCED_FACE('',(#4656),#384,.T.);
#43512=ADVANCED_FACE('',(#4657),#42234,.T.);
#43513=ADVANCED_FACE('',(#4658),#385,.T.);
#43514=ADVANCED_FACE('',(#4659),#2512,.T.);
#43515=ADVANCED_FACE('',(#4660),#386,.T.);
#43516=ADVANCED_FACE('',(#4661),#42235,.T.);
#43517=ADVANCED_FACE('',(#4662),#42236,.T.);
#43518=ADVANCED_FACE('',(#4663),#2513,.T.);
#43519=ADVANCED_FACE('',(#4664),#2514,.T.);
#43520=ADVANCED_FACE('',(#4665),#42237,.T.);
#43521=ADVANCED_FACE('',(#4666),#387,.T.);
#43522=ADVANCED_FACE('',(#4667),#2515,.T.);
#43523=ADVANCED_FACE('',(#4668),#42238,.T.);
#43524=ADVANCED_FACE('',(#4669),#2516,.T.);
#43525=ADVANCED_FACE('',(#4670),#42239,.T.);
#43526=ADVANCED_FACE('',(#4671),#388,.T.);
#43527=ADVANCED_FACE('',(#4672),#2517,.T.);
#43528=ADVANCED_FACE('',(#4673),#389,.T.);
#43529=ADVANCED_FACE('',(#4674),#42240,.T.);
#43530=ADVANCED_FACE('',(#4675),#390,.T.);
#43531=ADVANCED_FACE('',(#4676),#2518,.T.);
#43532=ADVANCED_FACE('',(#4677),#391,.T.);
#43533=ADVANCED_FACE('',(#4678),#42241,.T.);
#43534=ADVANCED_FACE('',(#4679),#392,.T.);
#43535=ADVANCED_FACE('',(#4680),#2519,.T.);
#43536=ADVANCED_FACE('',(#4681),#393,.T.);
#43537=ADVANCED_FACE('',(#4682),#42242,.T.);
#43538=ADVANCED_FACE('',(#4683),#2520,.T.);
#43539=ADVANCED_FACE('',(#4684),#2521,.T.);
#43540=ADVANCED_FACE('',(#4685),#394,.T.);
#43541=ADVANCED_FACE('',(#4686),#42243,.T.);
#43542=ADVANCED_FACE('',(#4687),#395,.T.);
#43543=ADVANCED_FACE('',(#4688),#2522,.T.);
#43544=ADVANCED_FACE('',(#4689),#396,.T.);
#43545=ADVANCED_FACE('',(#4690),#42244,.T.);
#43546=ADVANCED_FACE('',(#4691),#42245,.T.);
#43547=ADVANCED_FACE('',(#4692),#2523,.T.);
#43548=ADVANCED_FACE('',(#4693),#2524,.T.);
#43549=ADVANCED_FACE('',(#4694),#42246,.T.);
#43550=ADVANCED_FACE('',(#4695),#397,.T.);
#43551=ADVANCED_FACE('',(#4696),#2525,.T.);
#43552=ADVANCED_FACE('',(#4697),#42247,.T.);
#43553=ADVANCED_FACE('',(#4698),#2526,.T.);
#43554=ADVANCED_FACE('',(#4699),#42248,.T.);
#43555=ADVANCED_FACE('',(#4700),#398,.T.);
#43556=ADVANCED_FACE('',(#4701),#2527,.T.);
#43557=ADVANCED_FACE('',(#4702),#2528,.T.);
#43558=ADVANCED_FACE('',(#4703),#42249,.T.);
#43559=ADVANCED_FACE('',(#4704),#399,.T.);
#43560=ADVANCED_FACE('',(#4705),#2529,.T.);
#43561=ADVANCED_FACE('',(#4706),#400,.T.);
#43562=ADVANCED_FACE('',(#4707),#42250,.T.);
#43563=ADVANCED_FACE('',(#4708),#401,.T.);
#43564=ADVANCED_FACE('',(#4709),#2530,.T.);
#43565=ADVANCED_FACE('',(#4710),#402,.T.);
#43566=ADVANCED_FACE('',(#4711),#42251,.T.);
#43567=ADVANCED_FACE('',(#4712),#2531,.T.);
#43568=ADVANCED_FACE('',(#4713),#2532,.T.);
#43569=ADVANCED_FACE('',(#4714),#403,.T.);
#43570=ADVANCED_FACE('',(#4715),#42252,.T.);
#43571=ADVANCED_FACE('',(#4716),#404,.T.);
#43572=ADVANCED_FACE('',(#4717),#2533,.T.);
#43573=ADVANCED_FACE('',(#4718),#405,.T.);
#43574=ADVANCED_FACE('',(#4719),#42253,.T.);
#43575=ADVANCED_FACE('',(#4720),#42254,.T.);
#43576=ADVANCED_FACE('',(#4721),#2534,.T.);
#43577=ADVANCED_FACE('',(#4722),#2535,.T.);
#43578=ADVANCED_FACE('',(#4723),#42255,.T.);
#43579=ADVANCED_FACE('',(#4724),#406,.T.);
#43580=ADVANCED_FACE('',(#4725),#2536,.T.);
#43581=ADVANCED_FACE('',(#4726),#42256,.T.);
#43582=ADVANCED_FACE('',(#4727),#2537,.T.);
#43583=ADVANCED_FACE('',(#4728),#42257,.T.);
#43584=ADVANCED_FACE('',(#4729),#407,.T.);
#43585=ADVANCED_FACE('',(#4730),#2538,.T.);
#43586=ADVANCED_FACE('',(#4731),#408,.T.);
#43587=ADVANCED_FACE('',(#4732),#42258,.T.);
#43588=ADVANCED_FACE('',(#4733),#2539,.T.);
#43589=ADVANCED_FACE('',(#4734),#2540,.T.);
#43590=ADVANCED_FACE('',(#4735),#409,.T.);
#43591=ADVANCED_FACE('',(#4736),#42259,.T.);
#43592=ADVANCED_FACE('',(#4737),#410,.T.);
#43593=ADVANCED_FACE('',(#4738),#2541,.T.);
#43594=ADVANCED_FACE('',(#4739),#411,.T.);
#43595=ADVANCED_FACE('',(#4740),#42260,.T.);
#43596=ADVANCED_FACE('',(#4741),#2542,.T.);
#43597=ADVANCED_FACE('',(#4742),#2543,.T.);
#43598=ADVANCED_FACE('',(#4743),#412,.T.);
#43599=ADVANCED_FACE('',(#4744),#42261,.T.);
#43600=ADVANCED_FACE('',(#4745),#413,.T.);
#43601=ADVANCED_FACE('',(#4746),#2544,.T.);
#43602=ADVANCED_FACE('',(#4747),#414,.T.);
#43603=ADVANCED_FACE('',(#4748),#42262,.T.);
#43604=ADVANCED_FACE('',(#4749),#42263,.T.);
#43605=ADVANCED_FACE('',(#4750),#2545,.T.);
#43606=ADVANCED_FACE('',(#4751),#2546,.T.);
#43607=ADVANCED_FACE('',(#4752),#42264,.T.);
#43608=ADVANCED_FACE('',(#4753),#415,.T.);
#43609=ADVANCED_FACE('',(#4754),#2547,.T.);
#43610=ADVANCED_FACE('',(#4755),#42265,.T.);
#43611=ADVANCED_FACE('',(#4756),#2548,.T.);
#43612=ADVANCED_FACE('',(#4757),#42266,.T.);
#43613=ADVANCED_FACE('',(#4758),#416,.T.);
#43614=ADVANCED_FACE('',(#4759),#2549,.T.);
#43615=ADVANCED_FACE('',(#4760),#417,.T.);
#43616=ADVANCED_FACE('',(#4761),#42267,.T.);
#43617=ADVANCED_FACE('',(#4762),#418,.T.);
#43618=ADVANCED_FACE('',(#4763),#2550,.T.);
#43619=ADVANCED_FACE('',(#4764),#419,.T.);
#43620=ADVANCED_FACE('',(#4765),#42268,.T.);
#43621=ADVANCED_FACE('',(#4766),#420,.T.);
#43622=ADVANCED_FACE('',(#4767),#2551,.T.);
#43623=ADVANCED_FACE('',(#4768),#2552,.T.);
#43624=ADVANCED_FACE('',(#4769),#42269,.T.);
#43625=ADVANCED_FACE('',(#4770),#2553,.T.);
#43626=ADVANCED_FACE('',(#4771),#2554,.T.);
#43627=ADVANCED_FACE('',(#4772),#421,.T.);
#43628=ADVANCED_FACE('',(#4773),#42270,.T.);
#43629=ADVANCED_FACE('',(#4774),#422,.T.);
#43630=ADVANCED_FACE('',(#4775),#2555,.T.);
#43631=ADVANCED_FACE('',(#4776),#423,.T.);
#43632=ADVANCED_FACE('',(#4777),#42271,.T.);
#43633=ADVANCED_FACE('',(#4778),#42272,.T.);
#43634=ADVANCED_FACE('',(#4779),#2556,.T.);
#43635=ADVANCED_FACE('',(#4780),#2557,.T.);
#43636=ADVANCED_FACE('',(#4781),#42273,.T.);
#43637=ADVANCED_FACE('',(#4782),#424,.T.);
#43638=ADVANCED_FACE('',(#4783),#2558,.T.);
#43639=ADVANCED_FACE('',(#4784),#42274,.T.);
#43640=ADVANCED_FACE('',(#4785),#2559,.T.);
#43641=ADVANCED_FACE('',(#4786),#42275,.T.);
#43642=ADVANCED_FACE('',(#4787),#425,.T.);
#43643=ADVANCED_FACE('',(#4788),#2560,.T.);
#43644=ADVANCED_FACE('',(#4789),#426,.T.);
#43645=ADVANCED_FACE('',(#4790),#42276,.T.);
#43646=ADVANCED_FACE('',(#4791),#427,.T.);
#43647=ADVANCED_FACE('',(#4792),#2561,.T.);
#43648=ADVANCED_FACE('',(#4793),#428,.T.);
#43649=ADVANCED_FACE('',(#4794),#42277,.T.);
#43650=ADVANCED_FACE('',(#4795),#429,.T.);
#43651=ADVANCED_FACE('',(#4796),#2562,.T.);
#43652=ADVANCED_FACE('',(#4797),#430,.T.);
#43653=ADVANCED_FACE('',(#4798),#42278,.T.);
#43654=ADVANCED_FACE('',(#4799),#2563,.T.);
#43655=ADVANCED_FACE('',(#4800),#2564,.T.);
#43656=ADVANCED_FACE('',(#4801),#2565,.T.);
#43657=ADVANCED_FACE('',(#4802),#42279,.T.);
#43658=ADVANCED_FACE('',(#4803),#431,.T.);
#43659=ADVANCED_FACE('',(#4804),#2566,.T.);
#43660=ADVANCED_FACE('',(#4805),#432,.T.);
#43661=ADVANCED_FACE('',(#4806),#42280,.T.);
#43662=ADVANCED_FACE('',(#4807),#42281,.T.);
#43663=ADVANCED_FACE('',(#4808),#2567,.T.);
#43664=ADVANCED_FACE('',(#4809),#2568,.T.);
#43665=ADVANCED_FACE('',(#4810),#42282,.T.);
#43666=ADVANCED_FACE('',(#4811),#433,.T.);
#43667=ADVANCED_FACE('',(#4812),#2569,.T.);
#43668=ADVANCED_FACE('',(#4813),#42283,.T.);
#43669=ADVANCED_FACE('',(#4814),#2570,.T.);
#43670=ADVANCED_FACE('',(#4815),#42284,.T.);
#43671=ADVANCED_FACE('',(#4816),#434,.T.);
#43672=ADVANCED_FACE('',(#4817),#2571,.T.);
#43673=ADVANCED_FACE('',(#4818),#435,.T.);
#43674=ADVANCED_FACE('',(#4819),#42285,.T.);
#43675=ADVANCED_FACE('',(#4820),#436,.T.);
#43676=ADVANCED_FACE('',(#4821),#2572,.T.);
#43677=ADVANCED_FACE('',(#4822),#437,.T.);
#43678=ADVANCED_FACE('',(#4823),#42286,.T.);
#43679=ADVANCED_FACE('',(#4824),#438,.T.);
#43680=ADVANCED_FACE('',(#4825),#2573,.T.);
#43681=ADVANCED_FACE('',(#4826),#439,.T.);
#43682=ADVANCED_FACE('',(#4827),#42287,.T.);
#43683=ADVANCED_FACE('',(#4828),#2574,.T.);
#43684=ADVANCED_FACE('',(#4829),#2575,.T.);
#43685=ADVANCED_FACE('',(#4830),#440,.T.);
#43686=ADVANCED_FACE('',(#4831),#42288,.T.);
#43687=ADVANCED_FACE('',(#4832),#441,.T.);
#43688=ADVANCED_FACE('',(#4833),#2576,.T.);
#43689=ADVANCED_FACE('',(#4834),#2577,.T.);
#43690=ADVANCED_FACE('',(#4835),#42289,.T.);
#43691=ADVANCED_FACE('',(#4836),#42290,.T.);
#43692=ADVANCED_FACE('',(#4837),#2578,.T.);
#43693=ADVANCED_FACE('',(#4838),#2579,.T.);
#43694=ADVANCED_FACE('',(#4839),#42291,.T.);
#43695=ADVANCED_FACE('',(#4840),#442,.T.);
#43696=ADVANCED_FACE('',(#4841),#2580,.T.);
#43697=ADVANCED_FACE('',(#4842),#42292,.T.);
#43698=ADVANCED_FACE('',(#4843),#2581,.T.);
#43699=ADVANCED_FACE('',(#4844),#42293,.T.);
#43700=ADVANCED_FACE('',(#4845),#443,.T.);
#43701=ADVANCED_FACE('',(#4846),#2582,.T.);
#43702=ADVANCED_FACE('',(#4847),#444,.T.);
#43703=ADVANCED_FACE('',(#4848),#42294,.T.);
#43704=ADVANCED_FACE('',(#4849),#445,.T.);
#43705=ADVANCED_FACE('',(#4850),#2583,.T.);
#43706=ADVANCED_FACE('',(#4851),#446,.T.);
#43707=ADVANCED_FACE('',(#4852),#42295,.T.);
#43708=ADVANCED_FACE('',(#4853),#447,.T.);
#43709=ADVANCED_FACE('',(#4854),#2584,.T.);
#43710=ADVANCED_FACE('',(#4855),#448,.T.);
#43711=ADVANCED_FACE('',(#4856),#42296,.T.);
#43712=ADVANCED_FACE('',(#4857),#2585,.T.);
#43713=ADVANCED_FACE('',(#4858),#2586,.T.);
#43714=ADVANCED_FACE('',(#4859),#449,.T.);
#43715=ADVANCED_FACE('',(#4860),#42297,.T.);
#43716=ADVANCED_FACE('',(#4861),#450,.T.);
#43717=ADVANCED_FACE('',(#4862),#2587,.T.);
#43718=ADVANCED_FACE('',(#4863),#451,.T.);
#43719=ADVANCED_FACE('',(#4864),#42298,.T.);
#43720=ADVANCED_FACE('',(#4865),#42299,.T.);
#43721=ADVANCED_FACE('',(#4866),#2588,.T.);
#43722=ADVANCED_FACE('',(#4867),#2589,.T.);
#43723=ADVANCED_FACE('',(#4868),#42300,.T.);
#43724=ADVANCED_FACE('',(#4869),#452,.T.);
#43725=ADVANCED_FACE('',(#4870),#2590,.T.);
#43726=ADVANCED_FACE('',(#4871),#42301,.T.);
#43727=ADVANCED_FACE('',(#4872),#2591,.T.);
#43728=ADVANCED_FACE('',(#4873),#42302,.T.);
#43729=ADVANCED_FACE('',(#4874),#453,.T.);
#43730=ADVANCED_FACE('',(#4875),#2592,.T.);
#43731=ADVANCED_FACE('',(#4876),#454,.T.);
#43732=ADVANCED_FACE('',(#4877),#42303,.T.);
#43733=ADVANCED_FACE('',(#4878),#455,.T.);
#43734=ADVANCED_FACE('',(#4879),#2593,.T.);
#43735=ADVANCED_FACE('',(#4880),#456,.T.);
#43736=ADVANCED_FACE('',(#4881),#42304,.T.);
#43737=ADVANCED_FACE('',(#4882),#457,.T.);
#43738=ADVANCED_FACE('',(#4883),#2594,.T.);
#43739=ADVANCED_FACE('',(#4884),#458,.T.);
#43740=ADVANCED_FACE('',(#4885),#42305,.T.);
#43741=ADVANCED_FACE('',(#4886),#2595,.T.);
#43742=ADVANCED_FACE('',(#4887),#2596,.T.);
#43743=ADVANCED_FACE('',(#4888),#459,.T.);
#43744=ADVANCED_FACE('',(#4889),#42306,.T.);
#43745=ADVANCED_FACE('',(#4890),#460,.T.);
#43746=ADVANCED_FACE('',(#4891),#2597,.T.);
#43747=ADVANCED_FACE('',(#4892),#461,.T.);
#43748=ADVANCED_FACE('',(#4893),#42307,.T.);
#43749=ADVANCED_FACE('',(#4894),#42308,.T.);
#43750=ADVANCED_FACE('',(#4895),#2598,.T.);
#43751=ADVANCED_FACE('',(#4896),#2599,.T.);
#43752=ADVANCED_FACE('',(#4897),#42309,.T.);
#43753=ADVANCED_FACE('',(#4898),#462,.T.);
#43754=ADVANCED_FACE('',(#4899),#2600,.T.);
#43755=ADVANCED_FACE('',(#4900),#42310,.T.);
#43756=ADVANCED_FACE('',(#4901),#2601,.T.);
#43757=ADVANCED_FACE('',(#4902),#42311,.T.);
#43758=ADVANCED_FACE('',(#4903),#463,.T.);
#43759=ADVANCED_FACE('',(#4904),#2602,.T.);
#43760=ADVANCED_FACE('',(#4905),#464,.T.);
#43761=ADVANCED_FACE('',(#4906),#42312,.T.);
#43762=ADVANCED_FACE('',(#4907),#465,.T.);
#43763=ADVANCED_FACE('',(#4908),#2603,.T.);
#43764=ADVANCED_FACE('',(#4909),#466,.T.);
#43765=ADVANCED_FACE('',(#4910),#42313,.T.);
#43766=ADVANCED_FACE('',(#4911),#467,.T.);
#43767=ADVANCED_FACE('',(#4912),#2604,.T.);
#43768=ADVANCED_FACE('',(#4913),#468,.T.);
#43769=ADVANCED_FACE('',(#4914),#42314,.T.);
#43770=ADVANCED_FACE('',(#4915),#2605,.T.);
#43771=ADVANCED_FACE('',(#4916),#2606,.T.);
#43772=ADVANCED_FACE('',(#4917),#469,.T.);
#43773=ADVANCED_FACE('',(#4918),#42315,.T.);
#43774=ADVANCED_FACE('',(#4919),#470,.T.);
#43775=ADVANCED_FACE('',(#4920),#2607,.T.);
#43776=ADVANCED_FACE('',(#4921),#471,.T.);
#43777=ADVANCED_FACE('',(#4922),#42316,.T.);
#43778=ADVANCED_FACE('',(#4923),#42317,.T.);
#43779=ADVANCED_FACE('',(#4924),#2608,.T.);
#43780=ADVANCED_FACE('',(#4925),#2609,.T.);
#43781=ADVANCED_FACE('',(#4926),#42318,.T.);
#43782=ADVANCED_FACE('',(#4927),#472,.T.);
#43783=ADVANCED_FACE('',(#4928),#2610,.T.);
#43784=ADVANCED_FACE('',(#4929),#42319,.T.);
#43785=ADVANCED_FACE('',(#4930),#2611,.T.);
#43786=ADVANCED_FACE('',(#4931),#42320,.T.);
#43787=ADVANCED_FACE('',(#4932),#473,.T.);
#43788=ADVANCED_FACE('',(#4933),#2612,.T.);
#43789=ADVANCED_FACE('',(#4934),#474,.T.);
#43790=ADVANCED_FACE('',(#4935),#42321,.T.);
#43791=ADVANCED_FACE('',(#4936),#475,.T.);
#43792=ADVANCED_FACE('',(#4937),#2613,.T.);
#43793=ADVANCED_FACE('',(#4938),#476,.T.);
#43794=ADVANCED_FACE('',(#4939),#42322,.T.);
#43795=ADVANCED_FACE('',(#4940),#477,.T.);
#43796=ADVANCED_FACE('',(#4941),#2614,.T.);
#43797=ADVANCED_FACE('',(#4942),#478,.T.);
#43798=ADVANCED_FACE('',(#4943),#42323,.T.);
#43799=ADVANCED_FACE('',(#4944),#2615,.T.);
#43800=ADVANCED_FACE('',(#4945),#2616,.T.);
#43801=ADVANCED_FACE('',(#4946),#479,.T.);
#43802=ADVANCED_FACE('',(#4947),#42324,.T.);
#43803=ADVANCED_FACE('',(#4948),#480,.T.);
#43804=ADVANCED_FACE('',(#4949),#2617,.T.);
#43805=ADVANCED_FACE('',(#4950),#481,.T.);
#43806=ADVANCED_FACE('',(#4951),#42325,.T.);
#43807=ADVANCED_FACE('',(#4952),#42326,.T.);
#43808=ADVANCED_FACE('',(#4953),#2618,.T.);
#43809=ADVANCED_FACE('',(#4954),#2619,.T.);
#43810=ADVANCED_FACE('',(#4955),#42327,.T.);
#43811=ADVANCED_FACE('',(#4956),#482,.T.);
#43812=ADVANCED_FACE('',(#4957),#2620,.T.);
#43813=ADVANCED_FACE('',(#4958),#42328,.T.);
#43814=ADVANCED_FACE('',(#4959),#2621,.T.);
#43815=ADVANCED_FACE('',(#4960),#42329,.T.);
#43816=ADVANCED_FACE('',(#4961),#483,.T.);
#43817=ADVANCED_FACE('',(#4962),#2622,.T.);
#43818=ADVANCED_FACE('',(#4963),#484,.T.);
#43819=ADVANCED_FACE('',(#4964),#42330,.T.);
#43820=ADVANCED_FACE('',(#4965),#485,.T.);
#43821=ADVANCED_FACE('',(#4966),#2623,.T.);
#43822=ADVANCED_FACE('',(#4967),#486,.T.);
#43823=ADVANCED_FACE('',(#4968),#42331,.T.);
#43824=ADVANCED_FACE('',(#4969),#487,.T.);
#43825=ADVANCED_FACE('',(#4970),#2624,.T.);
#43826=ADVANCED_FACE('',(#4971),#488,.T.);
#43827=ADVANCED_FACE('',(#4972),#42332,.T.);
#43828=ADVANCED_FACE('',(#4973),#2625,.T.);
#43829=ADVANCED_FACE('',(#4974),#2626,.T.);
#43830=ADVANCED_FACE('',(#4975),#489,.T.);
#43831=ADVANCED_FACE('',(#4976),#42333,.T.);
#43832=ADVANCED_FACE('',(#4977),#490,.T.);
#43833=ADVANCED_FACE('',(#4978),#2627,.T.);
#43834=ADVANCED_FACE('',(#4979),#491,.T.);
#43835=ADVANCED_FACE('',(#4980),#42334,.T.);
#43836=ADVANCED_FACE('',(#4981),#42335,.T.);
#43837=ADVANCED_FACE('',(#4982),#2628,.T.);
#43838=ADVANCED_FACE('',(#4983),#2629,.T.);
#43839=ADVANCED_FACE('',(#4984),#42336,.T.);
#43840=ADVANCED_FACE('',(#4985),#492,.T.);
#43841=ADVANCED_FACE('',(#4986),#2630,.T.);
#43842=ADVANCED_FACE('',(#4987),#42337,.T.);
#43843=ADVANCED_FACE('',(#4988),#2631,.T.);
#43844=ADVANCED_FACE('',(#4989),#42338,.T.);
#43845=ADVANCED_FACE('',(#4990),#493,.T.);
#43846=ADVANCED_FACE('',(#4991),#2632,.T.);
#43847=ADVANCED_FACE('',(#4992),#494,.T.);
#43848=ADVANCED_FACE('',(#4993),#42339,.T.);
#43849=ADVANCED_FACE('',(#4994),#495,.T.);
#43850=ADVANCED_FACE('',(#4995),#2633,.T.);
#43851=ADVANCED_FACE('',(#4996),#496,.T.);
#43852=ADVANCED_FACE('',(#4997),#42340,.T.);
#43853=ADVANCED_FACE('',(#4998),#497,.T.);
#43854=ADVANCED_FACE('',(#4999),#2634,.T.);
#43855=ADVANCED_FACE('',(#5000),#498,.T.);
#43856=ADVANCED_FACE('',(#5001),#42341,.T.);
#43857=ADVANCED_FACE('',(#5002),#2635,.T.);
#43858=ADVANCED_FACE('',(#5003),#2636,.T.);
#43859=ADVANCED_FACE('',(#5004),#499,.T.);
#43860=ADVANCED_FACE('',(#5005),#42342,.T.);
#43861=ADVANCED_FACE('',(#5006),#500,.T.);
#43862=ADVANCED_FACE('',(#5007),#2637,.T.);
#43863=ADVANCED_FACE('',(#5008),#501,.T.);
#43864=ADVANCED_FACE('',(#5009),#42343,.T.);
#43865=ADVANCED_FACE('',(#5010),#42344,.T.);
#43866=ADVANCED_FACE('',(#5011),#2638,.T.);
#43867=ADVANCED_FACE('',(#5012),#2639,.T.);
#43868=ADVANCED_FACE('',(#5013),#42345,.T.);
#43869=ADVANCED_FACE('',(#5014),#502,.T.);
#43870=ADVANCED_FACE('',(#5015),#2640,.T.);
#43871=ADVANCED_FACE('',(#5016),#42346,.T.);
#43872=ADVANCED_FACE('',(#5017),#2641,.T.);
#43873=ADVANCED_FACE('',(#5018),#42347,.T.);
#43874=ADVANCED_FACE('',(#5019),#503,.T.);
#43875=ADVANCED_FACE('',(#5020),#2642,.T.);
#43876=ADVANCED_FACE('',(#5021),#504,.T.);
#43877=ADVANCED_FACE('',(#5022),#42348,.T.);
#43878=ADVANCED_FACE('',(#5023),#505,.T.);
#43879=ADVANCED_FACE('',(#5024),#2643,.T.);
#43880=ADVANCED_FACE('',(#5025),#506,.T.);
#43881=ADVANCED_FACE('',(#5026),#42349,.T.);
#43882=ADVANCED_FACE('',(#5027),#507,.T.);
#43883=ADVANCED_FACE('',(#5028),#2644,.T.);
#43884=ADVANCED_FACE('',(#5029),#508,.T.);
#43885=ADVANCED_FACE('',(#5030),#42350,.T.);
#43886=ADVANCED_FACE('',(#5031),#2645,.T.);
#43887=ADVANCED_FACE('',(#5032),#2646,.T.);
#43888=ADVANCED_FACE('',(#5033),#509,.T.);
#43889=ADVANCED_FACE('',(#5034),#42351,.T.);
#43890=ADVANCED_FACE('',(#5035),#510,.T.);
#43891=ADVANCED_FACE('',(#5036),#2647,.T.);
#43892=ADVANCED_FACE('',(#5037),#511,.T.);
#43893=ADVANCED_FACE('',(#5038),#42352,.T.);
#43894=ADVANCED_FACE('',(#5039),#42353,.T.);
#43895=ADVANCED_FACE('',(#5040),#2648,.T.);
#43896=ADVANCED_FACE('',(#5041),#2649,.T.);
#43897=ADVANCED_FACE('',(#5042),#42354,.T.);
#43898=ADVANCED_FACE('',(#5043),#512,.T.);
#43899=ADVANCED_FACE('',(#5044),#2650,.T.);
#43900=ADVANCED_FACE('',(#5045),#42355,.T.);
#43901=ADVANCED_FACE('',(#5046),#2651,.T.);
#43902=ADVANCED_FACE('',(#5047),#42356,.T.);
#43903=ADVANCED_FACE('',(#5048),#513,.T.);
#43904=ADVANCED_FACE('',(#5049),#2652,.T.);
#43905=ADVANCED_FACE('',(#5050),#514,.T.);
#43906=ADVANCED_FACE('',(#5051),#42357,.T.);
#43907=ADVANCED_FACE('',(#5052),#515,.T.);
#43908=ADVANCED_FACE('',(#5053),#2653,.T.);
#43909=ADVANCED_FACE('',(#5054),#516,.T.);
#43910=ADVANCED_FACE('',(#5055),#42358,.T.);
#43911=ADVANCED_FACE('',(#5056),#517,.T.);
#43912=ADVANCED_FACE('',(#5057),#2654,.T.);
#43913=ADVANCED_FACE('',(#5058),#518,.T.);
#43914=ADVANCED_FACE('',(#5059),#42359,.T.);
#43915=ADVANCED_FACE('',(#5060),#2655,.T.);
#43916=ADVANCED_FACE('',(#5061),#2656,.T.);
#43917=ADVANCED_FACE('',(#5062),#519,.T.);
#43918=ADVANCED_FACE('',(#5063),#42360,.T.);
#43919=ADVANCED_FACE('',(#5064),#520,.T.);
#43920=ADVANCED_FACE('',(#5065),#2657,.T.);
#43921=ADVANCED_FACE('',(#5066),#521,.T.);
#43922=ADVANCED_FACE('',(#5067),#42361,.T.);
#43923=ADVANCED_FACE('',(#5068),#42362,.T.);
#43924=ADVANCED_FACE('',(#5069),#42363,.T.);
#43925=ADVANCED_FACE('',(#5070),#2658,.T.);
#43926=ADVANCED_FACE('',(#5071),#2659,.T.);
#43927=ADVANCED_FACE('',(#5072),#522,.T.);
#43928=ADVANCED_FACE('',(#5073),#2660,.T.);
#43929=ADVANCED_FACE('',(#5074),#42364,.T.);
#43930=ADVANCED_FACE('',(#5075),#2661,.T.);
#43931=ADVANCED_FACE('',(#5076),#42365,.T.);
#43932=ADVANCED_FACE('',(#5077),#523,.T.);
#43933=ADVANCED_FACE('',(#5078),#2662,.T.);
#43934=ADVANCED_FACE('',(#5079),#524,.T.);
#43935=ADVANCED_FACE('',(#5080),#42366,.T.);
#43936=ADVANCED_FACE('',(#5081),#525,.T.);
#43937=ADVANCED_FACE('',(#5082),#2663,.T.);
#43938=ADVANCED_FACE('',(#5083),#526,.T.);
#43939=ADVANCED_FACE('',(#5084),#42367,.T.);
#43940=ADVANCED_FACE('',(#5085),#527,.T.);
#43941=ADVANCED_FACE('',(#5086),#2664,.T.);
#43942=ADVANCED_FACE('',(#5087),#528,.T.);
#43943=ADVANCED_FACE('',(#5088),#42368,.T.);
#43944=ADVANCED_FACE('',(#5089),#2665,.T.);
#43945=ADVANCED_FACE('',(#5090),#2666,.T.);
#43946=ADVANCED_FACE('',(#5091),#529,.T.);
#43947=ADVANCED_FACE('',(#5092),#42369,.T.);
#43948=ADVANCED_FACE('',(#5093),#530,.T.);
#43949=ADVANCED_FACE('',(#5094),#2667,.T.);
#43950=ADVANCED_FACE('',(#5095),#531,.T.);
#43951=ADVANCED_FACE('',(#5096),#42370,.T.);
#43952=ADVANCED_FACE('',(#5097),#42371,.T.);
#43953=ADVANCED_FACE('',(#5098),#42372,.T.);
#43954=ADVANCED_FACE('',(#5099),#42373,.T.);
#43955=ADVANCED_FACE('',(#5100),#2668,.T.);
#43956=ADVANCED_FACE('',(#5101),#2669,.T.);
#43957=ADVANCED_FACE('',(#5102),#532,.T.);
#43958=ADVANCED_FACE('',(#5103),#2670,.T.);
#43959=ADVANCED_FACE('',(#5104),#42374,.T.);
#43960=ADVANCED_FACE('',(#5105),#2671,.T.);
#43961=ADVANCED_FACE('',(#5106),#533,.T.);
#43962=ADVANCED_FACE('',(#5107),#2672,.T.);
#43963=ADVANCED_FACE('',(#5108),#2673,.T.);
#43964=ADVANCED_FACE('',(#5109),#42375,.T.);
#43965=ADVANCED_FACE('',(#5110),#534,.T.);
#43966=ADVANCED_FACE('',(#5111),#2674,.T.);
#43967=ADVANCED_FACE('',(#5112),#535,.T.);
#43968=ADVANCED_FACE('',(#5113),#42376,.T.);
#43969=ADVANCED_FACE('',(#5114),#536,.T.);
#43970=ADVANCED_FACE('',(#5115),#2675,.T.);
#43971=ADVANCED_FACE('',(#5116),#537,.T.);
#43972=ADVANCED_FACE('',(#5117),#42377,.T.);
#43973=ADVANCED_FACE('',(#5118),#2676,.T.);
#43974=ADVANCED_FACE('',(#5119),#2677,.T.);
#43975=ADVANCED_FACE('',(#5120),#538,.T.);
#43976=ADVANCED_FACE('',(#5121),#42378,.T.);
#43977=ADVANCED_FACE('',(#5122),#539,.T.);
#43978=ADVANCED_FACE('',(#5123),#2678,.T.);
#43979=ADVANCED_FACE('',(#5124),#540,.T.);
#43980=ADVANCED_FACE('',(#5125),#42379,.T.);
#43981=ADVANCED_FACE('',(#5126),#42380,.T.);
#43982=ADVANCED_FACE('',(#5127),#42381,.T.);
#43983=ADVANCED_FACE('',(#5128),#42382,.T.);
#43984=ADVANCED_FACE('',(#5129),#42383,.T.);
#43985=ADVANCED_FACE('',(#5130),#541,.T.);
#43986=ADVANCED_FACE('',(#5131),#2679,.T.);
#43987=ADVANCED_FACE('',(#5132),#42384,.T.);
#43988=ADVANCED_FACE('',(#5133),#2680,.T.);
#43989=ADVANCED_FACE('',(#5134),#542,.T.);
#43990=ADVANCED_FACE('',(#5135),#2681,.T.);
#43991=ADVANCED_FACE('',(#5136),#543,.T.);
#43992=ADVANCED_FACE('',(#5137),#2682,.T.);
#43993=ADVANCED_FACE('',(#5138),#2683,.T.);
#43994=ADVANCED_FACE('',(#5139),#544,.T.);
#43995=ADVANCED_FACE('',(#5140),#545,.T.);
#43996=ADVANCED_FACE('',(#5141),#2684,.T.);
#43997=ADVANCED_FACE('',(#5142),#42385,.T.);
#43998=ADVANCED_FACE('',(#5143),#546,.T.);
#43999=ADVANCED_FACE('',(#5144),#2685,.T.);
#44000=ADVANCED_FACE('',(#5145),#547,.T.);
#44001=ADVANCED_FACE('',(#5146),#42386,.T.);
#44002=ADVANCED_FACE('',(#5147),#2686,.T.);
#44003=ADVANCED_FACE('',(#5148),#2687,.T.);
#44004=ADVANCED_FACE('',(#5149),#548,.T.);
#44005=ADVANCED_FACE('',(#5150),#42387,.T.);
#44006=ADVANCED_FACE('',(#5151),#549,.T.);
#44007=ADVANCED_FACE('',(#5152),#2688,.T.);
#44008=ADVANCED_FACE('',(#5153),#550,.T.);
#44009=ADVANCED_FACE('',(#5154),#42388,.T.);
#44010=ADVANCED_FACE('',(#5155),#42389,.T.);
#44011=ADVANCED_FACE('',(#5156),#42390,.T.);
#44012=ADVANCED_FACE('',(#5157),#42391,.T.);
#44013=ADVANCED_FACE('',(#5158),#42392,.T.);
#44014=ADVANCED_FACE('',(#5159),#42393,.T.);
#44015=ADVANCED_FACE('',(#5160),#551,.T.);
#44016=ADVANCED_FACE('',(#5161),#2689,.T.);
#44017=ADVANCED_FACE('',(#5162),#2690,.T.);
#44018=ADVANCED_FACE('',(#5163),#552,.T.);
#44019=ADVANCED_FACE('',(#5164),#2691,.T.);
#44020=ADVANCED_FACE('',(#5165),#553,.T.);
#44021=ADVANCED_FACE('',(#5166),#554,.T.);
#44022=ADVANCED_FACE('',(#5167),#2692,.T.);
#44023=ADVANCED_FACE('',(#5168),#2693,.T.);
#44024=ADVANCED_FACE('',(#5169),#555,.T.);
#44025=ADVANCED_FACE('',(#5170),#2694,.T.);
#44026=ADVANCED_FACE('',(#5171),#556,.T.);
#44027=ADVANCED_FACE('',(#5172),#2695,.T.);
#44028=ADVANCED_FACE('',(#5173),#42394,.T.);
#44029=ADVANCED_FACE('',(#5174),#2696,.T.);
#44030=ADVANCED_FACE('',(#5175),#42395,.T.);
#44031=ADVANCED_FACE('',(#5176),#2697,.T.);
#44032=ADVANCED_FACE('',(#5177),#2698,.T.);
#44033=ADVANCED_FACE('',(#5178),#557,.T.);
#44034=ADVANCED_FACE('',(#5179),#42396,.T.);
#44035=ADVANCED_FACE('',(#5180),#558,.T.);
#44036=ADVANCED_FACE('',(#5181),#2699,.T.);
#44037=ADVANCED_FACE('',(#5182),#559,.T.);
#44038=ADVANCED_FACE('',(#5183),#42397,.T.);
#44039=ADVANCED_FACE('',(#5184),#42398,.T.);
#44040=ADVANCED_FACE('',(#5185),#42399,.T.);
#44041=ADVANCED_FACE('',(#5186),#42400,.T.);
#44042=ADVANCED_FACE('',(#5187),#42401,.T.);
#44043=ADVANCED_FACE('',(#5188),#42402,.T.);
#44044=ADVANCED_FACE('',(#5189),#42403,.T.);
#44045=ADVANCED_FACE('',(#5190),#2700,.T.);
#44046=ADVANCED_FACE('',(#5191),#2701,.T.);
#44047=ADVANCED_FACE('',(#5192),#560,.T.);
#44048=ADVANCED_FACE('',(#5193),#561,.T.);
#44049=ADVANCED_FACE('',(#5194),#2702,.T.);
#44050=ADVANCED_FACE('',(#5195),#562,.T.);
#44051=ADVANCED_FACE('',(#5196),#2703,.T.);
#44052=ADVANCED_FACE('',(#5197),#2704,.T.);
#44053=ADVANCED_FACE('',(#5198),#2705,.T.);
#44054=ADVANCED_FACE('',(#5199),#2706,.T.);
#44055=ADVANCED_FACE('',(#5200),#563,.T.);
#44056=ADVANCED_FACE('',(#5201),#564,.T.);
#44057=ADVANCED_FACE('',(#5202),#2707,.T.);
#44058=ADVANCED_FACE('',(#5203),#42404,.T.);
#44059=ADVANCED_FACE('',(#5204),#2708,.T.);
#44060=ADVANCED_FACE('',(#5205),#565,.T.);
#44061=ADVANCED_FACE('',(#5206),#2709,.T.);
#44062=ADVANCED_FACE('',(#5207),#566,.T.);
#44063=ADVANCED_FACE('',(#5208),#42405,.T.);
#44064=ADVANCED_FACE('',(#5209),#567,.T.);
#44065=ADVANCED_FACE('',(#5210),#2710,.T.);
#44066=ADVANCED_FACE('',(#5211),#568,.T.);
#44067=ADVANCED_FACE('',(#5212),#42406,.T.);
#44068=ADVANCED_FACE('',(#5213),#42407,.T.);
#44069=ADVANCED_FACE('',(#5214),#42408,.T.);
#44070=ADVANCED_FACE('',(#5215),#42409,.T.);
#44071=ADVANCED_FACE('',(#5216),#42410,.T.);
#44072=ADVANCED_FACE('',(#5217),#42411,.T.);
#44073=ADVANCED_FACE('',(#5218),#42412,.T.);
#44074=ADVANCED_FACE('',(#5219),#42413,.T.);
#44075=ADVANCED_FACE('',(#5220),#569,.T.);
#44076=ADVANCED_FACE('',(#5221),#2711,.T.);
#44077=ADVANCED_FACE('',(#5222),#2712,.T.);
#44078=ADVANCED_FACE('',(#5223),#570,.T.);
#44079=ADVANCED_FACE('',(#5224),#2713,.T.);
#44080=ADVANCED_FACE('',(#5225),#571,.T.);
#44081=ADVANCED_FACE('',(#5226),#572,.T.);
#44082=ADVANCED_FACE('',(#5227),#2714,.T.);
#44083=ADVANCED_FACE('',(#5228),#2715,.T.);
#44084=ADVANCED_FACE('',(#5229),#573,.T.);
#44085=ADVANCED_FACE('',(#5230),#574,.T.);
#44086=ADVANCED_FACE('',(#5231),#575,.T.);
#44087=ADVANCED_FACE('',(#5232),#2716,.T.);
#44088=ADVANCED_FACE('',(#5233),#42414,.T.);
#44089=ADVANCED_FACE('',(#5234),#576,.T.);
#44090=ADVANCED_FACE('',(#5235),#577,.T.);
#44091=ADVANCED_FACE('',(#5236),#2717,.T.);
#44092=ADVANCED_FACE('',(#5237),#578,.T.);
#44093=ADVANCED_FACE('',(#5238),#579,.T.);
#44094=ADVANCED_FACE('',(#5239),#2718,.T.);
#44095=ADVANCED_FACE('',(#5240),#580,.T.);
#44096=ADVANCED_FACE('',(#5241),#42415,.T.);
#44097=ADVANCED_FACE('',(#5242),#42416,.T.);
#44098=ADVANCED_FACE('',(#5243),#42417,.T.);
#44099=ADVANCED_FACE('',(#5244),#42418,.T.);
#44100=ADVANCED_FACE('',(#5245),#42419,.T.);
#44101=ADVANCED_FACE('',(#5246),#3566,.F.);
#44102=ADVANCED_FACE('',(#5247,#3513),#3567,.F.);
#44103=ADVANCED_FACE('',(#5248),#3568,.T.);
#44104=ADVANCED_FACE('',(#5249),#2719,.T.);
#44105=ADVANCED_FACE('',(#5250),#2720,.T.);
#44106=ADVANCED_FACE('',(#5251),#581,.T.);
#44107=ADVANCED_FACE('',(#5252),#2721,.T.);
#44108=ADVANCED_FACE('',(#5253),#582,.T.);
#44109=ADVANCED_FACE('',(#5254),#2722,.T.);
#44110=ADVANCED_FACE('',(#5255),#2723,.T.);
#44111=ADVANCED_FACE('',(#5256),#2724,.T.);
#44112=ADVANCED_FACE('',(#5257),#583,.T.);
#44113=ADVANCED_FACE('',(#5258),#2725,.T.);
#44114=ADVANCED_FACE('',(#5259),#2726,.T.);
#44115=ADVANCED_FACE('',(#5260),#584,.T.);
#44116=ADVANCED_FACE('',(#5261),#2727,.T.);
#44117=ADVANCED_FACE('',(#5262),#2728,.T.);
#44118=ADVANCED_FACE('',(#5263),#585,.T.);
#44119=ADVANCED_FACE('',(#5264),#42420,.F.);
#44120=ADVANCED_FACE('',(#5265),#42421,.F.);
#44121=ADVANCED_FACE('',(#5266),#2729,.T.);
#44122=ADVANCED_FACE('',(#5267),#2730,.T.);
#44123=ADVANCED_FACE('',(#5268),#586,.T.);
#44124=ADVANCED_FACE('',(#5269),#2731,.T.);
#44125=ADVANCED_FACE('',(#5270),#2732,.T.);
#44126=ADVANCED_FACE('',(#5271),#2733,.T.);
#44127=ADVANCED_FACE('',(#5272),#42422,.F.);
#44128=ADVANCED_FACE('',(#5273),#42423,.F.);
#44129=ADVANCED_FACE('',(#5274),#2734,.T.);
#44130=ADVANCED_FACE('',(#5275),#2735,.T.);
#44131=ADVANCED_FACE('',(#5276),#587,.T.);
#44132=ADVANCED_FACE('',(#5277),#588,.T.);
#44133=ADVANCED_FACE('',(#5278),#2736,.T.);
#44134=ADVANCED_FACE('',(#5279),#2737,.T.);
#44135=ADVANCED_FACE('',(#5280),#2738,.T.);
#44136=ADVANCED_FACE('',(#5281),#2739,.T.);
#44137=ADVANCED_FACE('',(#5282),#589,.T.);
#44138=ADVANCED_FACE('',(#5283),#2740,.T.);
#44139=ADVANCED_FACE('',(#5284),#2741,.T.);
#44140=ADVANCED_FACE('',(#5285),#590,.T.);
#44141=ADVANCED_FACE('',(#5286),#2742,.T.);
#44142=ADVANCED_FACE('',(#5287),#2743,.T.);
#44143=ADVANCED_FACE('',(#5288),#591,.T.);
#44144=ADVANCED_FACE('',(#5289),#2744,.T.);
#44145=ADVANCED_FACE('',(#5290),#2745,.T.);
#44146=ADVANCED_FACE('',(#5291),#2746,.T.);
#44147=ADVANCED_FACE('',(#5292),#592,.T.);
#44148=ADVANCED_FACE('',(#5293),#2747,.T.);
#44149=ADVANCED_FACE('',(#5294),#2748,.T.);
#44150=ADVANCED_FACE('',(#5295),#42424,.F.);
#44151=ADVANCED_FACE('',(#5296),#42425,.F.);
#44152=ADVANCED_FACE('',(#5297),#2749,.T.);
#44153=ADVANCED_FACE('',(#5298),#2750,.T.);
#44154=ADVANCED_FACE('',(#5299),#593,.T.);
#44155=ADVANCED_FACE('',(#5300),#2751,.T.);
#44156=ADVANCED_FACE('',(#5301),#2752,.T.);
#44157=ADVANCED_FACE('',(#5302),#2753,.T.);
#44158=ADVANCED_FACE('',(#5303),#2754,.T.);
#44159=ADVANCED_FACE('',(#5304),#2755,.T.);
#44160=ADVANCED_FACE('',(#5305),#594,.T.);
#44161=ADVANCED_FACE('',(#5306),#2756,.T.);
#44162=ADVANCED_FACE('',(#5307),#2757,.T.);
#44163=ADVANCED_FACE('',(#5308),#595,.T.);
#44164=ADVANCED_FACE('',(#5309),#2758,.T.);
#44165=ADVANCED_FACE('',(#5310),#2759,.T.);
#44166=ADVANCED_FACE('',(#5311),#596,.T.);
#44167=ADVANCED_FACE('',(#5312),#2760,.T.);
#44168=ADVANCED_FACE('',(#5313),#2761,.T.);
#44169=ADVANCED_FACE('',(#5314),#597,.T.);
#44170=ADVANCED_FACE('',(#5315),#2762,.T.);
#44171=ADVANCED_FACE('',(#5316),#598,.T.);
#44172=ADVANCED_FACE('',(#5317),#2763,.T.);
#44173=ADVANCED_FACE('',(#5318),#42426,.F.);
#44174=ADVANCED_FACE('',(#5319),#42427,.F.);
#44175=ADVANCED_FACE('',(#5320),#2764,.T.);
#44176=ADVANCED_FACE('',(#5321),#2765,.T.);
#44177=ADVANCED_FACE('',(#5322),#599,.T.);
#44178=ADVANCED_FACE('',(#5323),#2766,.T.);
#44179=ADVANCED_FACE('',(#5324),#2767,.T.);
#44180=ADVANCED_FACE('',(#5325),#2768,.T.);
#44181=ADVANCED_FACE('',(#5326),#2769,.T.);
#44182=ADVANCED_FACE('',(#5327),#2770,.T.);
#44183=ADVANCED_FACE('',(#5328),#600,.T.);
#44184=ADVANCED_FACE('',(#5329),#2771,.T.);
#44185=ADVANCED_FACE('',(#5330),#2772,.T.);
#44186=ADVANCED_FACE('',(#5331),#601,.T.);
#44187=ADVANCED_FACE('',(#5332),#2773,.T.);
#44188=ADVANCED_FACE('',(#5333),#2774,.T.);
#44189=ADVANCED_FACE('',(#5334),#602,.T.);
#44190=ADVANCED_FACE('',(#5335),#2775,.T.);
#44191=ADVANCED_FACE('',(#5336),#603,.T.);
#44192=ADVANCED_FACE('',(#5337),#2776,.T.);
#44193=ADVANCED_FACE('',(#5338),#604,.T.);
#44194=ADVANCED_FACE('',(#5339),#2777,.T.);
#44195=ADVANCED_FACE('',(#5340),#2778,.T.);
#44196=ADVANCED_FACE('',(#5341),#42428,.F.);
#44197=ADVANCED_FACE('',(#5342),#42429,.F.);
#44198=ADVANCED_FACE('',(#5343),#2779,.T.);
#44199=ADVANCED_FACE('',(#5344),#2780,.T.);
#44200=ADVANCED_FACE('',(#5345),#605,.T.);
#44201=ADVANCED_FACE('',(#5346),#2781,.T.);
#44202=ADVANCED_FACE('',(#5347),#2782,.T.);
#44203=ADVANCED_FACE('',(#5348),#2783,.T.);
#44204=ADVANCED_FACE('',(#5349),#2784,.T.);
#44205=ADVANCED_FACE('',(#5350),#2785,.T.);
#44206=ADVANCED_FACE('',(#5351),#606,.T.);
#44207=ADVANCED_FACE('',(#5352),#2786,.T.);
#44208=ADVANCED_FACE('',(#5353),#607,.T.);
#44209=ADVANCED_FACE('',(#5354),#2787,.T.);
#44210=ADVANCED_FACE('',(#5355),#2788,.T.);
#44211=ADVANCED_FACE('',(#5356),#608,.T.);
#44212=ADVANCED_FACE('',(#5357),#2789,.T.);
#44213=ADVANCED_FACE('',(#5358),#2790,.T.);
#44214=ADVANCED_FACE('',(#5359),#2791,.T.);
#44215=ADVANCED_FACE('',(#5360),#609,.T.);
#44216=ADVANCED_FACE('',(#5361),#610,.T.);
#44217=ADVANCED_FACE('',(#5362),#2792,.T.);
#44218=ADVANCED_FACE('',(#5363),#2793,.T.);
#44219=ADVANCED_FACE('',(#5364),#42430,.F.);
#44220=ADVANCED_FACE('',(#5365),#42431,.F.);
#44221=ADVANCED_FACE('',(#5366),#2794,.T.);
#44222=ADVANCED_FACE('',(#5367),#2795,.T.);
#44223=ADVANCED_FACE('',(#5368),#611,.T.);
#44224=ADVANCED_FACE('',(#5369),#2796,.T.);
#44225=ADVANCED_FACE('',(#5370),#2797,.T.);
#44226=ADVANCED_FACE('',(#5371),#2798,.T.);
#44227=ADVANCED_FACE('',(#5372),#2799,.T.);
#44228=ADVANCED_FACE('',(#5373),#2800,.T.);
#44229=ADVANCED_FACE('',(#5374),#612,.T.);
#44230=ADVANCED_FACE('',(#5375),#2801,.T.);
#44231=ADVANCED_FACE('',(#5376),#613,.T.);
#44232=ADVANCED_FACE('',(#5377),#2802,.T.);
#44233=ADVANCED_FACE('',(#5378),#2803,.T.);
#44234=ADVANCED_FACE('',(#5379),#2804,.T.);
#44235=ADVANCED_FACE('',(#5380),#614,.T.);
#44236=ADVANCED_FACE('',(#5381),#2805,.T.);
#44237=ADVANCED_FACE('',(#5382),#2806,.T.);
#44238=ADVANCED_FACE('',(#5383),#615,.T.);
#44239=ADVANCED_FACE('',(#5384),#616,.T.);
#44240=ADVANCED_FACE('',(#5385),#2807,.T.);
#44241=ADVANCED_FACE('',(#5386),#2808,.T.);
#44242=ADVANCED_FACE('',(#5387),#42432,.F.);
#44243=ADVANCED_FACE('',(#5388),#42433,.F.);
#44244=ADVANCED_FACE('',(#5389),#2809,.T.);
#44245=ADVANCED_FACE('',(#5390),#2810,.T.);
#44246=ADVANCED_FACE('',(#5391),#617,.T.);
#44247=ADVANCED_FACE('',(#5392),#2811,.T.);
#44248=ADVANCED_FACE('',(#5393),#2812,.T.);
#44249=ADVANCED_FACE('',(#5394),#2813,.T.);
#44250=ADVANCED_FACE('',(#5395),#2814,.T.);
#44251=ADVANCED_FACE('',(#5396),#2815,.T.);
#44252=ADVANCED_FACE('',(#5397),#618,.T.);
#44253=ADVANCED_FACE('',(#5398),#2816,.T.);
#44254=ADVANCED_FACE('',(#5399),#619,.T.);
#44255=ADVANCED_FACE('',(#5400),#2817,.T.);
#44256=ADVANCED_FACE('',(#5401),#2818,.T.);
#44257=ADVANCED_FACE('',(#5402),#2819,.T.);
#44258=ADVANCED_FACE('',(#5403),#620,.T.);
#44259=ADVANCED_FACE('',(#5404),#2820,.T.);
#44260=ADVANCED_FACE('',(#5405),#2821,.T.);
#44261=ADVANCED_FACE('',(#5406),#621,.T.);
#44262=ADVANCED_FACE('',(#5407),#622,.T.);
#44263=ADVANCED_FACE('',(#5408),#2822,.T.);
#44264=ADVANCED_FACE('',(#5409),#2823,.T.);
#44265=ADVANCED_FACE('',(#5410),#42434,.F.);
#44266=ADVANCED_FACE('',(#5411),#42435,.F.);
#44267=ADVANCED_FACE('',(#5412),#2824,.T.);
#44268=ADVANCED_FACE('',(#5413),#2825,.T.);
#44269=ADVANCED_FACE('',(#5414),#623,.T.);
#44270=ADVANCED_FACE('',(#5415),#2826,.T.);
#44271=ADVANCED_FACE('',(#5416),#2827,.T.);
#44272=ADVANCED_FACE('',(#5417),#2828,.T.);
#44273=ADVANCED_FACE('',(#5418),#2829,.T.);
#44274=ADVANCED_FACE('',(#5419),#2830,.T.);
#44275=ADVANCED_FACE('',(#5420),#624,.T.);
#44276=ADVANCED_FACE('',(#5421),#2831,.T.);
#44277=ADVANCED_FACE('',(#5422),#625,.T.);
#44278=ADVANCED_FACE('',(#5423),#2832,.T.);
#44279=ADVANCED_FACE('',(#5424),#2833,.T.);
#44280=ADVANCED_FACE('',(#5425),#2834,.T.);
#44281=ADVANCED_FACE('',(#5426),#626,.T.);
#44282=ADVANCED_FACE('',(#5427),#2835,.T.);
#44283=ADVANCED_FACE('',(#5428),#2836,.T.);
#44284=ADVANCED_FACE('',(#5429),#627,.T.);
#44285=ADVANCED_FACE('',(#5430),#628,.T.);
#44286=ADVANCED_FACE('',(#5431),#2837,.T.);
#44287=ADVANCED_FACE('',(#5432),#2838,.T.);
#44288=ADVANCED_FACE('',(#5433),#42436,.F.);
#44289=ADVANCED_FACE('',(#5434),#42437,.F.);
#44290=ADVANCED_FACE('',(#5435),#2839,.T.);
#44291=ADVANCED_FACE('',(#5436),#2840,.T.);
#44292=ADVANCED_FACE('',(#5437),#629,.T.);
#44293=ADVANCED_FACE('',(#5438),#2841,.T.);
#44294=ADVANCED_FACE('',(#5439),#2842,.T.);
#44295=ADVANCED_FACE('',(#5440),#2843,.T.);
#44296=ADVANCED_FACE('',(#5441),#2844,.T.);
#44297=ADVANCED_FACE('',(#5442),#2845,.T.);
#44298=ADVANCED_FACE('',(#5443),#630,.T.);
#44299=ADVANCED_FACE('',(#5444),#2846,.T.);
#44300=ADVANCED_FACE('',(#5445),#631,.T.);
#44301=ADVANCED_FACE('',(#5446),#2847,.T.);
#44302=ADVANCED_FACE('',(#5447),#2848,.T.);
#44303=ADVANCED_FACE('',(#5448),#2849,.T.);
#44304=ADVANCED_FACE('',(#5449),#632,.T.);
#44305=ADVANCED_FACE('',(#5450),#2850,.T.);
#44306=ADVANCED_FACE('',(#5451),#2851,.T.);
#44307=ADVANCED_FACE('',(#5452),#633,.T.);
#44308=ADVANCED_FACE('',(#5453),#634,.T.);
#44309=ADVANCED_FACE('',(#5454),#2852,.T.);
#44310=ADVANCED_FACE('',(#5455),#2853,.T.);
#44311=ADVANCED_FACE('',(#5456),#42438,.F.);
#44312=ADVANCED_FACE('',(#5457),#42439,.F.);
#44313=ADVANCED_FACE('',(#5458),#2854,.T.);
#44314=ADVANCED_FACE('',(#5459),#2855,.T.);
#44315=ADVANCED_FACE('',(#5460),#635,.T.);
#44316=ADVANCED_FACE('',(#5461),#2856,.T.);
#44317=ADVANCED_FACE('',(#5462),#2857,.T.);
#44318=ADVANCED_FACE('',(#5463),#2858,.T.);
#44319=ADVANCED_FACE('',(#5464),#2859,.T.);
#44320=ADVANCED_FACE('',(#5465),#2860,.T.);
#44321=ADVANCED_FACE('',(#5466),#636,.T.);
#44322=ADVANCED_FACE('',(#5467),#2861,.T.);
#44323=ADVANCED_FACE('',(#5468),#637,.T.);
#44324=ADVANCED_FACE('',(#5469),#2862,.T.);
#44325=ADVANCED_FACE('',(#5470),#2863,.T.);
#44326=ADVANCED_FACE('',(#5471),#2864,.T.);
#44327=ADVANCED_FACE('',(#5472),#638,.T.);
#44328=ADVANCED_FACE('',(#5473),#2865,.T.);
#44329=ADVANCED_FACE('',(#5474),#2866,.T.);
#44330=ADVANCED_FACE('',(#5475),#639,.T.);
#44331=ADVANCED_FACE('',(#5476),#640,.T.);
#44332=ADVANCED_FACE('',(#5477),#2867,.T.);
#44333=ADVANCED_FACE('',(#5478),#2868,.T.);
#44334=ADVANCED_FACE('',(#5479),#42440,.F.);
#44335=ADVANCED_FACE('',(#5480),#42441,.F.);
#44336=ADVANCED_FACE('',(#5481),#2869,.T.);
#44337=ADVANCED_FACE('',(#5482),#2870,.T.);
#44338=ADVANCED_FACE('',(#5483),#641,.T.);
#44339=ADVANCED_FACE('',(#5484),#2871,.T.);
#44340=ADVANCED_FACE('',(#5485),#2872,.T.);
#44341=ADVANCED_FACE('',(#5486),#2873,.T.);
#44342=ADVANCED_FACE('',(#5487),#2874,.T.);
#44343=ADVANCED_FACE('',(#5488),#2875,.T.);
#44344=ADVANCED_FACE('',(#5489),#642,.T.);
#44345=ADVANCED_FACE('',(#5490),#2876,.T.);
#44346=ADVANCED_FACE('',(#5491),#643,.T.);
#44347=ADVANCED_FACE('',(#5492),#2877,.T.);
#44348=ADVANCED_FACE('',(#5493),#2878,.T.);
#44349=ADVANCED_FACE('',(#5494),#2879,.T.);
#44350=ADVANCED_FACE('',(#5495),#644,.T.);
#44351=ADVANCED_FACE('',(#5496),#2880,.T.);
#44352=ADVANCED_FACE('',(#5497),#2881,.T.);
#44353=ADVANCED_FACE('',(#5498),#645,.T.);
#44354=ADVANCED_FACE('',(#5499),#646,.T.);
#44355=ADVANCED_FACE('',(#5500),#2882,.T.);
#44356=ADVANCED_FACE('',(#5501),#2883,.T.);
#44357=ADVANCED_FACE('',(#5502),#42442,.F.);
#44358=ADVANCED_FACE('',(#5503),#42443,.F.);
#44359=ADVANCED_FACE('',(#5504),#2884,.T.);
#44360=ADVANCED_FACE('',(#5505),#2885,.T.);
#44361=ADVANCED_FACE('',(#5506),#647,.T.);
#44362=ADVANCED_FACE('',(#5507),#2886,.T.);
#44363=ADVANCED_FACE('',(#5508),#2887,.T.);
#44364=ADVANCED_FACE('',(#5509),#2888,.T.);
#44365=ADVANCED_FACE('',(#5510),#2889,.T.);
#44366=ADVANCED_FACE('',(#5511),#2890,.T.);
#44367=ADVANCED_FACE('',(#5512),#648,.T.);
#44368=ADVANCED_FACE('',(#5513),#2891,.T.);
#44369=ADVANCED_FACE('',(#5514),#649,.T.);
#44370=ADVANCED_FACE('',(#5515),#2892,.T.);
#44371=ADVANCED_FACE('',(#5516),#2893,.T.);
#44372=ADVANCED_FACE('',(#5517),#2894,.T.);
#44373=ADVANCED_FACE('',(#5518),#650,.T.);
#44374=ADVANCED_FACE('',(#5519),#2895,.T.);
#44375=ADVANCED_FACE('',(#5520),#2896,.T.);
#44376=ADVANCED_FACE('',(#5521),#651,.T.);
#44377=ADVANCED_FACE('',(#5522),#652,.T.);
#44378=ADVANCED_FACE('',(#5523),#2897,.T.);
#44379=ADVANCED_FACE('',(#5524),#2898,.T.);
#44380=ADVANCED_FACE('',(#5525),#42444,.F.);
#44381=ADVANCED_FACE('',(#5526),#42445,.F.);
#44382=ADVANCED_FACE('',(#5527),#2899,.T.);
#44383=ADVANCED_FACE('',(#5528),#2900,.T.);
#44384=ADVANCED_FACE('',(#5529),#653,.T.);
#44385=ADVANCED_FACE('',(#5530),#2901,.T.);
#44386=ADVANCED_FACE('',(#5531),#2902,.T.);
#44387=ADVANCED_FACE('',(#5532),#2903,.T.);
#44388=ADVANCED_FACE('',(#5533),#2904,.T.);
#44389=ADVANCED_FACE('',(#5534),#2905,.T.);
#44390=ADVANCED_FACE('',(#5535),#654,.T.);
#44391=ADVANCED_FACE('',(#5536),#2906,.T.);
#44392=ADVANCED_FACE('',(#5537),#655,.T.);
#44393=ADVANCED_FACE('',(#5538),#2907,.T.);
#44394=ADVANCED_FACE('',(#5539),#2908,.T.);
#44395=ADVANCED_FACE('',(#5540),#2909,.T.);
#44396=ADVANCED_FACE('',(#5541),#656,.T.);
#44397=ADVANCED_FACE('',(#5542),#2910,.T.);
#44398=ADVANCED_FACE('',(#5543),#2911,.T.);
#44399=ADVANCED_FACE('',(#5544),#657,.T.);
#44400=ADVANCED_FACE('',(#5545),#658,.T.);
#44401=ADVANCED_FACE('',(#5546),#2912,.T.);
#44402=ADVANCED_FACE('',(#5547),#2913,.T.);
#44403=ADVANCED_FACE('',(#5548),#42446,.F.);
#44404=ADVANCED_FACE('',(#5549),#42447,.F.);
#44405=ADVANCED_FACE('',(#5550),#2914,.T.);
#44406=ADVANCED_FACE('',(#5551),#2915,.T.);
#44407=ADVANCED_FACE('',(#5552),#659,.T.);
#44408=ADVANCED_FACE('',(#5553),#2916,.T.);
#44409=ADVANCED_FACE('',(#5554),#2917,.T.);
#44410=ADVANCED_FACE('',(#5555),#2918,.T.);
#44411=ADVANCED_FACE('',(#5556),#2919,.T.);
#44412=ADVANCED_FACE('',(#5557),#2920,.T.);
#44413=ADVANCED_FACE('',(#5558),#660,.T.);
#44414=ADVANCED_FACE('',(#5559),#2921,.T.);
#44415=ADVANCED_FACE('',(#5560),#661,.T.);
#44416=ADVANCED_FACE('',(#5561),#2922,.T.);
#44417=ADVANCED_FACE('',(#5562),#2923,.T.);
#44418=ADVANCED_FACE('',(#5563),#2924,.T.);
#44419=ADVANCED_FACE('',(#5564),#662,.T.);
#44420=ADVANCED_FACE('',(#5565),#2925,.T.);
#44421=ADVANCED_FACE('',(#5566),#2926,.T.);
#44422=ADVANCED_FACE('',(#5567),#663,.T.);
#44423=ADVANCED_FACE('',(#5568),#664,.T.);
#44424=ADVANCED_FACE('',(#5569),#2927,.T.);
#44425=ADVANCED_FACE('',(#5570),#2928,.T.);
#44426=ADVANCED_FACE('',(#5571),#42448,.F.);
#44427=ADVANCED_FACE('',(#5572),#42449,.F.);
#44428=ADVANCED_FACE('',(#5573),#2929,.T.);
#44429=ADVANCED_FACE('',(#5574),#2930,.T.);
#44430=ADVANCED_FACE('',(#5575),#665,.T.);
#44431=ADVANCED_FACE('',(#5576),#2931,.T.);
#44432=ADVANCED_FACE('',(#5577),#2932,.T.);
#44433=ADVANCED_FACE('',(#5578),#2933,.T.);
#44434=ADVANCED_FACE('',(#5579),#2934,.T.);
#44435=ADVANCED_FACE('',(#5580),#2935,.T.);
#44436=ADVANCED_FACE('',(#5581),#666,.T.);
#44437=ADVANCED_FACE('',(#5582),#2936,.T.);
#44438=ADVANCED_FACE('',(#5583),#667,.T.);
#44439=ADVANCED_FACE('',(#5584),#2937,.T.);
#44440=ADVANCED_FACE('',(#5585),#2938,.T.);
#44441=ADVANCED_FACE('',(#5586),#2939,.T.);
#44442=ADVANCED_FACE('',(#5587),#668,.T.);
#44443=ADVANCED_FACE('',(#5588),#2940,.T.);
#44444=ADVANCED_FACE('',(#5589),#2941,.T.);
#44445=ADVANCED_FACE('',(#5590),#669,.T.);
#44446=ADVANCED_FACE('',(#5591),#670,.T.);
#44447=ADVANCED_FACE('',(#5592),#2942,.T.);
#44448=ADVANCED_FACE('',(#5593),#2943,.T.);
#44449=ADVANCED_FACE('',(#5594),#42450,.F.);
#44450=ADVANCED_FACE('',(#5595),#42451,.F.);
#44451=ADVANCED_FACE('',(#5596),#2944,.T.);
#44452=ADVANCED_FACE('',(#5597),#2945,.T.);
#44453=ADVANCED_FACE('',(#5598),#671,.T.);
#44454=ADVANCED_FACE('',(#5599),#2946,.T.);
#44455=ADVANCED_FACE('',(#5600),#2947,.T.);
#44456=ADVANCED_FACE('',(#5601),#2948,.T.);
#44457=ADVANCED_FACE('',(#5602),#2949,.T.);
#44458=ADVANCED_FACE('',(#5603),#2950,.T.);
#44459=ADVANCED_FACE('',(#5604),#672,.T.);
#44460=ADVANCED_FACE('',(#5605),#2951,.T.);
#44461=ADVANCED_FACE('',(#5606),#673,.T.);
#44462=ADVANCED_FACE('',(#5607),#2952,.T.);
#44463=ADVANCED_FACE('',(#5608),#2953,.T.);
#44464=ADVANCED_FACE('',(#5609),#2954,.T.);
#44465=ADVANCED_FACE('',(#5610),#674,.T.);
#44466=ADVANCED_FACE('',(#5611),#2955,.T.);
#44467=ADVANCED_FACE('',(#5612),#2956,.T.);
#44468=ADVANCED_FACE('',(#5613),#675,.T.);
#44469=ADVANCED_FACE('',(#5614),#676,.T.);
#44470=ADVANCED_FACE('',(#5615),#2957,.T.);
#44471=ADVANCED_FACE('',(#5616),#2958,.T.);
#44472=ADVANCED_FACE('',(#5617),#42452,.F.);
#44473=ADVANCED_FACE('',(#5618),#42453,.F.);
#44474=ADVANCED_FACE('',(#5619),#2959,.T.);
#44475=ADVANCED_FACE('',(#5620),#2960,.T.);
#44476=ADVANCED_FACE('',(#5621),#677,.T.);
#44477=ADVANCED_FACE('',(#5622),#2961,.T.);
#44478=ADVANCED_FACE('',(#5623),#2962,.T.);
#44479=ADVANCED_FACE('',(#5624),#2963,.T.);
#44480=ADVANCED_FACE('',(#5625),#2964,.T.);
#44481=ADVANCED_FACE('',(#5626),#2965,.T.);
#44482=ADVANCED_FACE('',(#5627),#678,.T.);
#44483=ADVANCED_FACE('',(#5628),#2966,.T.);
#44484=ADVANCED_FACE('',(#5629),#679,.T.);
#44485=ADVANCED_FACE('',(#5630),#2967,.T.);
#44486=ADVANCED_FACE('',(#5631),#2968,.T.);
#44487=ADVANCED_FACE('',(#5632),#2969,.T.);
#44488=ADVANCED_FACE('',(#5633),#680,.T.);
#44489=ADVANCED_FACE('',(#5634),#2970,.T.);
#44490=ADVANCED_FACE('',(#5635),#2971,.T.);
#44491=ADVANCED_FACE('',(#5636),#681,.T.);
#44492=ADVANCED_FACE('',(#5637),#682,.T.);
#44493=ADVANCED_FACE('',(#5638),#2972,.T.);
#44494=ADVANCED_FACE('',(#5639),#2973,.T.);
#44495=ADVANCED_FACE('',(#5640),#42454,.F.);
#44496=ADVANCED_FACE('',(#5641),#42455,.F.);
#44497=ADVANCED_FACE('',(#5642),#2974,.T.);
#44498=ADVANCED_FACE('',(#5643),#2975,.T.);
#44499=ADVANCED_FACE('',(#5644),#683,.T.);
#44500=ADVANCED_FACE('',(#5645),#2976,.T.);
#44501=ADVANCED_FACE('',(#5646),#2977,.T.);
#44502=ADVANCED_FACE('',(#5647),#2978,.T.);
#44503=ADVANCED_FACE('',(#5648),#2979,.T.);
#44504=ADVANCED_FACE('',(#5649),#2980,.T.);
#44505=ADVANCED_FACE('',(#5650),#684,.T.);
#44506=ADVANCED_FACE('',(#5651),#2981,.T.);
#44507=ADVANCED_FACE('',(#5652),#685,.T.);
#44508=ADVANCED_FACE('',(#5653),#2982,.T.);
#44509=ADVANCED_FACE('',(#5654),#2983,.T.);
#44510=ADVANCED_FACE('',(#5655),#2984,.T.);
#44511=ADVANCED_FACE('',(#5656),#686,.T.);
#44512=ADVANCED_FACE('',(#5657),#2985,.T.);
#44513=ADVANCED_FACE('',(#5658),#2986,.T.);
#44514=ADVANCED_FACE('',(#5659),#687,.T.);
#44515=ADVANCED_FACE('',(#5660),#688,.T.);
#44516=ADVANCED_FACE('',(#5661),#2987,.T.);
#44517=ADVANCED_FACE('',(#5662),#2988,.T.);
#44518=ADVANCED_FACE('',(#5663),#42456,.F.);
#44519=ADVANCED_FACE('',(#5664),#42457,.F.);
#44520=ADVANCED_FACE('',(#5665),#2989,.T.);
#44521=ADVANCED_FACE('',(#5666),#2990,.T.);
#44522=ADVANCED_FACE('',(#5667),#689,.T.);
#44523=ADVANCED_FACE('',(#5668),#2991,.T.);
#44524=ADVANCED_FACE('',(#5669),#2992,.T.);
#44525=ADVANCED_FACE('',(#5670),#2993,.T.);
#44526=ADVANCED_FACE('',(#5671),#2994,.T.);
#44527=ADVANCED_FACE('',(#5672),#2995,.T.);
#44528=ADVANCED_FACE('',(#5673),#690,.T.);
#44529=ADVANCED_FACE('',(#5674),#2996,.T.);
#44530=ADVANCED_FACE('',(#5675),#691,.T.);
#44531=ADVANCED_FACE('',(#5676),#2997,.T.);
#44532=ADVANCED_FACE('',(#5677),#2998,.T.);
#44533=ADVANCED_FACE('',(#5678),#2999,.T.);
#44534=ADVANCED_FACE('',(#5679),#692,.T.);
#44535=ADVANCED_FACE('',(#5680),#3000,.T.);
#44536=ADVANCED_FACE('',(#5681),#3001,.T.);
#44537=ADVANCED_FACE('',(#5682),#693,.T.);
#44538=ADVANCED_FACE('',(#5683),#694,.T.);
#44539=ADVANCED_FACE('',(#5684),#3002,.T.);
#44540=ADVANCED_FACE('',(#5685),#3003,.T.);
#44541=ADVANCED_FACE('',(#5686),#42458,.F.);
#44542=ADVANCED_FACE('',(#5687),#42459,.F.);
#44543=ADVANCED_FACE('',(#5688),#3004,.T.);
#44544=ADVANCED_FACE('',(#5689),#3005,.T.);
#44545=ADVANCED_FACE('',(#5690),#695,.T.);
#44546=ADVANCED_FACE('',(#5691),#3006,.T.);
#44547=ADVANCED_FACE('',(#5692),#3007,.T.);
#44548=ADVANCED_FACE('',(#5693),#3008,.T.);
#44549=ADVANCED_FACE('',(#5694),#3009,.T.);
#44550=ADVANCED_FACE('',(#5695),#3010,.T.);
#44551=ADVANCED_FACE('',(#5696),#696,.T.);
#44552=ADVANCED_FACE('',(#5697),#3011,.T.);
#44553=ADVANCED_FACE('',(#5698),#697,.T.);
#44554=ADVANCED_FACE('',(#5699),#3012,.T.);
#44555=ADVANCED_FACE('',(#5700),#3013,.T.);
#44556=ADVANCED_FACE('',(#5701),#3014,.T.);
#44557=ADVANCED_FACE('',(#5702),#698,.T.);
#44558=ADVANCED_FACE('',(#5703),#3015,.T.);
#44559=ADVANCED_FACE('',(#5704),#3016,.T.);
#44560=ADVANCED_FACE('',(#5705),#699,.T.);
#44561=ADVANCED_FACE('',(#5706),#700,.T.);
#44562=ADVANCED_FACE('',(#5707),#3017,.T.);
#44563=ADVANCED_FACE('',(#5708),#3018,.T.);
#44564=ADVANCED_FACE('',(#5709),#42460,.F.);
#44565=ADVANCED_FACE('',(#5710),#42461,.F.);
#44566=ADVANCED_FACE('',(#5711),#3019,.T.);
#44567=ADVANCED_FACE('',(#5712),#3020,.T.);
#44568=ADVANCED_FACE('',(#5713),#701,.T.);
#44569=ADVANCED_FACE('',(#5714),#3021,.T.);
#44570=ADVANCED_FACE('',(#5715),#3022,.T.);
#44571=ADVANCED_FACE('',(#5716),#3023,.T.);
#44572=ADVANCED_FACE('',(#5717),#3024,.T.);
#44573=ADVANCED_FACE('',(#5718),#3025,.T.);
#44574=ADVANCED_FACE('',(#5719),#702,.T.);
#44575=ADVANCED_FACE('',(#5720),#3026,.T.);
#44576=ADVANCED_FACE('',(#5721),#703,.T.);
#44577=ADVANCED_FACE('',(#5722),#3027,.T.);
#44578=ADVANCED_FACE('',(#5723),#3028,.T.);
#44579=ADVANCED_FACE('',(#5724),#3029,.T.);
#44580=ADVANCED_FACE('',(#5725),#704,.T.);
#44581=ADVANCED_FACE('',(#5726),#3030,.T.);
#44582=ADVANCED_FACE('',(#5727),#3031,.T.);
#44583=ADVANCED_FACE('',(#5728),#705,.T.);
#44584=ADVANCED_FACE('',(#5729),#706,.T.);
#44585=ADVANCED_FACE('',(#5730),#3032,.T.);
#44586=ADVANCED_FACE('',(#5731),#3033,.T.);
#44587=ADVANCED_FACE('',(#5732),#42462,.F.);
#44588=ADVANCED_FACE('',(#5733),#42463,.F.);
#44589=ADVANCED_FACE('',(#5734),#3034,.T.);
#44590=ADVANCED_FACE('',(#5735),#3035,.T.);
#44591=ADVANCED_FACE('',(#5736),#707,.T.);
#44592=ADVANCED_FACE('',(#5737),#3036,.T.);
#44593=ADVANCED_FACE('',(#5738),#3037,.T.);
#44594=ADVANCED_FACE('',(#5739),#3038,.T.);
#44595=ADVANCED_FACE('',(#5740),#3039,.T.);
#44596=ADVANCED_FACE('',(#5741),#3040,.T.);
#44597=ADVANCED_FACE('',(#5742),#708,.T.);
#44598=ADVANCED_FACE('',(#5743),#3041,.T.);
#44599=ADVANCED_FACE('',(#5744),#709,.T.);
#44600=ADVANCED_FACE('',(#5745),#3042,.T.);
#44601=ADVANCED_FACE('',(#5746),#3043,.T.);
#44602=ADVANCED_FACE('',(#5747),#3044,.T.);
#44603=ADVANCED_FACE('',(#5748),#710,.T.);
#44604=ADVANCED_FACE('',(#5749),#3045,.T.);
#44605=ADVANCED_FACE('',(#5750),#3046,.T.);
#44606=ADVANCED_FACE('',(#5751),#711,.T.);
#44607=ADVANCED_FACE('',(#5752),#712,.T.);
#44608=ADVANCED_FACE('',(#5753),#3047,.T.);
#44609=ADVANCED_FACE('',(#5754),#3048,.T.);
#44610=ADVANCED_FACE('',(#5755),#42464,.F.);
#44611=ADVANCED_FACE('',(#5756),#42465,.F.);
#44612=ADVANCED_FACE('',(#5757),#3049,.T.);
#44613=ADVANCED_FACE('',(#5758),#3050,.T.);
#44614=ADVANCED_FACE('',(#5759),#713,.T.);
#44615=ADVANCED_FACE('',(#5760),#3051,.T.);
#44616=ADVANCED_FACE('',(#5761),#3052,.T.);
#44617=ADVANCED_FACE('',(#5762),#3053,.T.);
#44618=ADVANCED_FACE('',(#5763),#3054,.T.);
#44619=ADVANCED_FACE('',(#5764),#3055,.T.);
#44620=ADVANCED_FACE('',(#5765),#714,.T.);
#44621=ADVANCED_FACE('',(#5766),#3056,.T.);
#44622=ADVANCED_FACE('',(#5767),#715,.T.);
#44623=ADVANCED_FACE('',(#5768),#3057,.T.);
#44624=ADVANCED_FACE('',(#5769),#3058,.T.);
#44625=ADVANCED_FACE('',(#5770),#3059,.T.);
#44626=ADVANCED_FACE('',(#5771),#716,.T.);
#44627=ADVANCED_FACE('',(#5772),#3060,.T.);
#44628=ADVANCED_FACE('',(#5773),#3061,.T.);
#44629=ADVANCED_FACE('',(#5774),#717,.T.);
#44630=ADVANCED_FACE('',(#5775),#718,.T.);
#44631=ADVANCED_FACE('',(#5776),#3062,.T.);
#44632=ADVANCED_FACE('',(#5777),#3063,.T.);
#44633=ADVANCED_FACE('',(#5778),#42466,.F.);
#44634=ADVANCED_FACE('',(#5779),#42467,.F.);
#44635=ADVANCED_FACE('',(#5780),#3064,.T.);
#44636=ADVANCED_FACE('',(#5781),#3065,.T.);
#44637=ADVANCED_FACE('',(#5782),#719,.T.);
#44638=ADVANCED_FACE('',(#5783),#3066,.T.);
#44639=ADVANCED_FACE('',(#5784),#3067,.T.);
#44640=ADVANCED_FACE('',(#5785),#3068,.T.);
#44641=ADVANCED_FACE('',(#5786),#3069,.T.);
#44642=ADVANCED_FACE('',(#5787),#3070,.T.);
#44643=ADVANCED_FACE('',(#5788),#720,.T.);
#44644=ADVANCED_FACE('',(#5789),#3071,.T.);
#44645=ADVANCED_FACE('',(#5790),#721,.T.);
#44646=ADVANCED_FACE('',(#5791),#3072,.T.);
#44647=ADVANCED_FACE('',(#5792),#3073,.T.);
#44648=ADVANCED_FACE('',(#5793),#3074,.T.);
#44649=ADVANCED_FACE('',(#5794),#722,.T.);
#44650=ADVANCED_FACE('',(#5795),#3075,.T.);
#44651=ADVANCED_FACE('',(#5796),#3076,.T.);
#44652=ADVANCED_FACE('',(#5797),#723,.T.);
#44653=ADVANCED_FACE('',(#5798),#724,.T.);
#44654=ADVANCED_FACE('',(#5799),#3077,.T.);
#44655=ADVANCED_FACE('',(#5800),#3078,.T.);
#44656=ADVANCED_FACE('',(#5801),#42468,.F.);
#44657=ADVANCED_FACE('',(#5802),#42469,.F.);
#44658=ADVANCED_FACE('',(#5803),#3079,.T.);
#44659=ADVANCED_FACE('',(#5804),#3080,.T.);
#44660=ADVANCED_FACE('',(#5805),#725,.T.);
#44661=ADVANCED_FACE('',(#5806),#3081,.T.);
#44662=ADVANCED_FACE('',(#5807),#3082,.T.);
#44663=ADVANCED_FACE('',(#5808),#3083,.T.);
#44664=ADVANCED_FACE('',(#5809),#3084,.T.);
#44665=ADVANCED_FACE('',(#5810),#3085,.T.);
#44666=ADVANCED_FACE('',(#5811),#726,.T.);
#44667=ADVANCED_FACE('',(#5812),#3086,.T.);
#44668=ADVANCED_FACE('',(#5813),#727,.T.);
#44669=ADVANCED_FACE('',(#5814),#3087,.T.);
#44670=ADVANCED_FACE('',(#5815),#3088,.T.);
#44671=ADVANCED_FACE('',(#5816),#3089,.T.);
#44672=ADVANCED_FACE('',(#5817),#728,.T.);
#44673=ADVANCED_FACE('',(#5818),#3090,.T.);
#44674=ADVANCED_FACE('',(#5819),#3091,.T.);
#44675=ADVANCED_FACE('',(#5820),#729,.T.);
#44676=ADVANCED_FACE('',(#5821),#730,.T.);
#44677=ADVANCED_FACE('',(#5822),#3092,.T.);
#44678=ADVANCED_FACE('',(#5823),#3093,.T.);
#44679=ADVANCED_FACE('',(#5824),#42470,.F.);
#44680=ADVANCED_FACE('',(#5825),#42471,.F.);
#44681=ADVANCED_FACE('',(#5826),#3094,.T.);
#44682=ADVANCED_FACE('',(#5827),#3095,.T.);
#44683=ADVANCED_FACE('',(#5828),#731,.T.);
#44684=ADVANCED_FACE('',(#5829),#3096,.T.);
#44685=ADVANCED_FACE('',(#5830),#3097,.T.);
#44686=ADVANCED_FACE('',(#5831),#3098,.T.);
#44687=ADVANCED_FACE('',(#5832),#3099,.T.);
#44688=ADVANCED_FACE('',(#5833),#3100,.T.);
#44689=ADVANCED_FACE('',(#5834),#732,.T.);
#44690=ADVANCED_FACE('',(#5835),#3101,.T.);
#44691=ADVANCED_FACE('',(#5836),#733,.T.);
#44692=ADVANCED_FACE('',(#5837),#3102,.T.);
#44693=ADVANCED_FACE('',(#5838),#3103,.T.);
#44694=ADVANCED_FACE('',(#5839),#3104,.T.);
#44695=ADVANCED_FACE('',(#5840),#734,.T.);
#44696=ADVANCED_FACE('',(#5841),#3105,.T.);
#44697=ADVANCED_FACE('',(#5842),#3106,.T.);
#44698=ADVANCED_FACE('',(#5843),#735,.T.);
#44699=ADVANCED_FACE('',(#5844),#736,.T.);
#44700=ADVANCED_FACE('',(#5845),#3107,.T.);
#44701=ADVANCED_FACE('',(#5846),#3108,.T.);
#44702=ADVANCED_FACE('',(#5847),#42472,.F.);
#44703=ADVANCED_FACE('',(#5848),#42473,.F.);
#44704=ADVANCED_FACE('',(#5849),#3109,.T.);
#44705=ADVANCED_FACE('',(#5850),#3110,.T.);
#44706=ADVANCED_FACE('',(#5851),#737,.T.);
#44707=ADVANCED_FACE('',(#5852),#3111,.T.);
#44708=ADVANCED_FACE('',(#5853),#3112,.T.);
#44709=ADVANCED_FACE('',(#5854),#3113,.T.);
#44710=ADVANCED_FACE('',(#5855),#3114,.T.);
#44711=ADVANCED_FACE('',(#5856),#3115,.T.);
#44712=ADVANCED_FACE('',(#5857),#738,.T.);
#44713=ADVANCED_FACE('',(#5858),#3116,.T.);
#44714=ADVANCED_FACE('',(#5859),#739,.T.);
#44715=ADVANCED_FACE('',(#5860),#3117,.T.);
#44716=ADVANCED_FACE('',(#5861),#3118,.T.);
#44717=ADVANCED_FACE('',(#5862),#3119,.T.);
#44718=ADVANCED_FACE('',(#5863),#740,.T.);
#44719=ADVANCED_FACE('',(#5864),#3120,.T.);
#44720=ADVANCED_FACE('',(#5865),#3121,.T.);
#44721=ADVANCED_FACE('',(#5866),#741,.T.);
#44722=ADVANCED_FACE('',(#5867),#742,.T.);
#44723=ADVANCED_FACE('',(#5868),#3122,.T.);
#44724=ADVANCED_FACE('',(#5869),#3123,.T.);
#44725=ADVANCED_FACE('',(#5870),#42474,.F.);
#44726=ADVANCED_FACE('',(#5871),#42475,.F.);
#44727=ADVANCED_FACE('',(#5872),#3124,.T.);
#44728=ADVANCED_FACE('',(#5873),#3125,.T.);
#44729=ADVANCED_FACE('',(#5874),#743,.T.);
#44730=ADVANCED_FACE('',(#5875),#3126,.T.);
#44731=ADVANCED_FACE('',(#5876),#3127,.T.);
#44732=ADVANCED_FACE('',(#5877),#3128,.T.);
#44733=ADVANCED_FACE('',(#5878),#3129,.T.);
#44734=ADVANCED_FACE('',(#5879),#3130,.T.);
#44735=ADVANCED_FACE('',(#5880),#744,.T.);
#44736=ADVANCED_FACE('',(#5881),#3131,.T.);
#44737=ADVANCED_FACE('',(#5882),#745,.T.);
#44738=ADVANCED_FACE('',(#5883),#3132,.T.);
#44739=ADVANCED_FACE('',(#5884),#3133,.T.);
#44740=ADVANCED_FACE('',(#5885),#3134,.T.);
#44741=ADVANCED_FACE('',(#5886),#746,.T.);
#44742=ADVANCED_FACE('',(#5887),#3135,.T.);
#44743=ADVANCED_FACE('',(#5888),#3136,.T.);
#44744=ADVANCED_FACE('',(#5889),#747,.T.);
#44745=ADVANCED_FACE('',(#5890),#748,.T.);
#44746=ADVANCED_FACE('',(#5891),#3137,.T.);
#44747=ADVANCED_FACE('',(#5892),#3138,.T.);
#44748=ADVANCED_FACE('',(#5893),#42476,.F.);
#44749=ADVANCED_FACE('',(#5894),#42477,.F.);
#44750=ADVANCED_FACE('',(#5895),#3139,.T.);
#44751=ADVANCED_FACE('',(#5896),#3140,.T.);
#44752=ADVANCED_FACE('',(#5897),#749,.T.);
#44753=ADVANCED_FACE('',(#5898),#3141,.T.);
#44754=ADVANCED_FACE('',(#5899),#3142,.T.);
#44755=ADVANCED_FACE('',(#5900),#3143,.T.);
#44756=ADVANCED_FACE('',(#5901),#3144,.T.);
#44757=ADVANCED_FACE('',(#5902),#3145,.T.);
#44758=ADVANCED_FACE('',(#5903),#750,.T.);
#44759=ADVANCED_FACE('',(#5904),#3146,.T.);
#44760=ADVANCED_FACE('',(#5905),#751,.T.);
#44761=ADVANCED_FACE('',(#5906),#3147,.T.);
#44762=ADVANCED_FACE('',(#5907),#3148,.T.);
#44763=ADVANCED_FACE('',(#5908),#3149,.T.);
#44764=ADVANCED_FACE('',(#5909),#752,.T.);
#44765=ADVANCED_FACE('',(#5910),#3150,.T.);
#44766=ADVANCED_FACE('',(#5911),#3151,.T.);
#44767=ADVANCED_FACE('',(#5912),#753,.T.);
#44768=ADVANCED_FACE('',(#5913),#754,.T.);
#44769=ADVANCED_FACE('',(#5914),#3152,.T.);
#44770=ADVANCED_FACE('',(#5915),#3153,.T.);
#44771=ADVANCED_FACE('',(#5916),#42478,.F.);
#44772=ADVANCED_FACE('',(#5917),#42479,.F.);
#44773=ADVANCED_FACE('',(#5918),#3154,.T.);
#44774=ADVANCED_FACE('',(#5919),#3155,.T.);
#44775=ADVANCED_FACE('',(#5920),#755,.T.);
#44776=ADVANCED_FACE('',(#5921),#3156,.T.);
#44777=ADVANCED_FACE('',(#5922),#3157,.T.);
#44778=ADVANCED_FACE('',(#5923),#3158,.T.);
#44779=ADVANCED_FACE('',(#5924),#3159,.T.);
#44780=ADVANCED_FACE('',(#5925),#3160,.T.);
#44781=ADVANCED_FACE('',(#5926),#756,.T.);
#44782=ADVANCED_FACE('',(#5927),#3161,.T.);
#44783=ADVANCED_FACE('',(#5928),#757,.T.);
#44784=ADVANCED_FACE('',(#5929),#3162,.T.);
#44785=ADVANCED_FACE('',(#5930),#3163,.T.);
#44786=ADVANCED_FACE('',(#5931),#3164,.T.);
#44787=ADVANCED_FACE('',(#5932),#758,.T.);
#44788=ADVANCED_FACE('',(#5933),#3165,.T.);
#44789=ADVANCED_FACE('',(#5934),#3166,.T.);
#44790=ADVANCED_FACE('',(#5935),#759,.T.);
#44791=ADVANCED_FACE('',(#5936),#760,.T.);
#44792=ADVANCED_FACE('',(#5937),#3167,.T.);
#44793=ADVANCED_FACE('',(#5938),#3168,.T.);
#44794=ADVANCED_FACE('',(#5939),#42480,.F.);
#44795=ADVANCED_FACE('',(#5940),#42481,.F.);
#44796=ADVANCED_FACE('',(#5941),#3169,.T.);
#44797=ADVANCED_FACE('',(#5942),#3170,.T.);
#44798=ADVANCED_FACE('',(#5943),#761,.T.);
#44799=ADVANCED_FACE('',(#5944),#3171,.T.);
#44800=ADVANCED_FACE('',(#5945),#3172,.T.);
#44801=ADVANCED_FACE('',(#5946),#3173,.T.);
#44802=ADVANCED_FACE('',(#5947),#3174,.T.);
#44803=ADVANCED_FACE('',(#5948),#3175,.T.);
#44804=ADVANCED_FACE('',(#5949),#762,.T.);
#44805=ADVANCED_FACE('',(#5950),#3176,.T.);
#44806=ADVANCED_FACE('',(#5951),#763,.T.);
#44807=ADVANCED_FACE('',(#5952),#3177,.T.);
#44808=ADVANCED_FACE('',(#5953),#3178,.T.);
#44809=ADVANCED_FACE('',(#5954),#3179,.T.);
#44810=ADVANCED_FACE('',(#5955),#764,.T.);
#44811=ADVANCED_FACE('',(#5956),#3180,.T.);
#44812=ADVANCED_FACE('',(#5957),#3181,.T.);
#44813=ADVANCED_FACE('',(#5958),#765,.T.);
#44814=ADVANCED_FACE('',(#5959),#766,.T.);
#44815=ADVANCED_FACE('',(#5960),#3182,.T.);
#44816=ADVANCED_FACE('',(#5961),#3183,.T.);
#44817=ADVANCED_FACE('',(#5962),#42482,.F.);
#44818=ADVANCED_FACE('',(#5963),#42483,.F.);
#44819=ADVANCED_FACE('',(#5964),#3184,.T.);
#44820=ADVANCED_FACE('',(#5965),#3185,.T.);
#44821=ADVANCED_FACE('',(#5966),#767,.T.);
#44822=ADVANCED_FACE('',(#5967),#3186,.T.);
#44823=ADVANCED_FACE('',(#5968),#3187,.T.);
#44824=ADVANCED_FACE('',(#5969),#3188,.T.);
#44825=ADVANCED_FACE('',(#5970),#3189,.T.);
#44826=ADVANCED_FACE('',(#5971),#3190,.T.);
#44827=ADVANCED_FACE('',(#5972),#768,.T.);
#44828=ADVANCED_FACE('',(#5973),#3191,.T.);
#44829=ADVANCED_FACE('',(#5974),#769,.T.);
#44830=ADVANCED_FACE('',(#5975),#3192,.T.);
#44831=ADVANCED_FACE('',(#5976),#3193,.T.);
#44832=ADVANCED_FACE('',(#5977),#3194,.T.);
#44833=ADVANCED_FACE('',(#5978),#770,.T.);
#44834=ADVANCED_FACE('',(#5979),#3195,.T.);
#44835=ADVANCED_FACE('',(#5980),#3196,.T.);
#44836=ADVANCED_FACE('',(#5981),#771,.T.);
#44837=ADVANCED_FACE('',(#5982),#772,.T.);
#44838=ADVANCED_FACE('',(#5983),#3197,.T.);
#44839=ADVANCED_FACE('',(#5984),#3198,.T.);
#44840=ADVANCED_FACE('',(#5985),#42484,.F.);
#44841=ADVANCED_FACE('',(#5986),#42485,.F.);
#44842=ADVANCED_FACE('',(#5987),#3199,.T.);
#44843=ADVANCED_FACE('',(#5988),#3200,.T.);
#44844=ADVANCED_FACE('',(#5989),#773,.T.);
#44845=ADVANCED_FACE('',(#5990),#3201,.T.);
#44846=ADVANCED_FACE('',(#5991),#3202,.T.);
#44847=ADVANCED_FACE('',(#5992),#3203,.T.);
#44848=ADVANCED_FACE('',(#5993),#3204,.T.);
#44849=ADVANCED_FACE('',(#5994),#3205,.T.);
#44850=ADVANCED_FACE('',(#5995),#774,.T.);
#44851=ADVANCED_FACE('',(#5996),#3206,.T.);
#44852=ADVANCED_FACE('',(#5997),#775,.T.);
#44853=ADVANCED_FACE('',(#5998),#3207,.T.);
#44854=ADVANCED_FACE('',(#5999),#3208,.T.);
#44855=ADVANCED_FACE('',(#6000),#3209,.T.);
#44856=ADVANCED_FACE('',(#6001),#776,.T.);
#44857=ADVANCED_FACE('',(#6002),#3210,.T.);
#44858=ADVANCED_FACE('',(#6003),#3211,.T.);
#44859=ADVANCED_FACE('',(#6004),#777,.T.);
#44860=ADVANCED_FACE('',(#6005),#778,.T.);
#44861=ADVANCED_FACE('',(#6006),#3212,.T.);
#44862=ADVANCED_FACE('',(#6007),#3213,.T.);
#44863=ADVANCED_FACE('',(#6008),#42486,.F.);
#44864=ADVANCED_FACE('',(#6009),#42487,.F.);
#44865=ADVANCED_FACE('',(#6010),#3214,.T.);
#44866=ADVANCED_FACE('',(#6011),#3215,.T.);
#44867=ADVANCED_FACE('',(#6012),#779,.T.);
#44868=ADVANCED_FACE('',(#6013),#3216,.T.);
#44869=ADVANCED_FACE('',(#6014),#3217,.T.);
#44870=ADVANCED_FACE('',(#6015),#3218,.T.);
#44871=ADVANCED_FACE('',(#6016),#3219,.T.);
#44872=ADVANCED_FACE('',(#6017),#3220,.T.);
#44873=ADVANCED_FACE('',(#6018),#780,.T.);
#44874=ADVANCED_FACE('',(#6019),#3221,.T.);
#44875=ADVANCED_FACE('',(#6020),#781,.T.);
#44876=ADVANCED_FACE('',(#6021),#3222,.T.);
#44877=ADVANCED_FACE('',(#6022),#3223,.T.);
#44878=ADVANCED_FACE('',(#6023),#3224,.T.);
#44879=ADVANCED_FACE('',(#6024),#782,.T.);
#44880=ADVANCED_FACE('',(#6025),#3225,.T.);
#44881=ADVANCED_FACE('',(#6026),#3226,.T.);
#44882=ADVANCED_FACE('',(#6027),#783,.T.);
#44883=ADVANCED_FACE('',(#6028),#784,.T.);
#44884=ADVANCED_FACE('',(#6029),#3227,.T.);
#44885=ADVANCED_FACE('',(#6030),#3228,.T.);
#44886=ADVANCED_FACE('',(#6031),#42488,.F.);
#44887=ADVANCED_FACE('',(#6032),#42489,.F.);
#44888=ADVANCED_FACE('',(#6033),#3229,.T.);
#44889=ADVANCED_FACE('',(#6034),#3230,.T.);
#44890=ADVANCED_FACE('',(#6035),#785,.T.);
#44891=ADVANCED_FACE('',(#6036),#3231,.T.);
#44892=ADVANCED_FACE('',(#6037),#3232,.T.);
#44893=ADVANCED_FACE('',(#6038),#3233,.T.);
#44894=ADVANCED_FACE('',(#6039),#3234,.T.);
#44895=ADVANCED_FACE('',(#6040),#3235,.T.);
#44896=ADVANCED_FACE('',(#6041),#786,.T.);
#44897=ADVANCED_FACE('',(#6042),#3236,.T.);
#44898=ADVANCED_FACE('',(#6043),#787,.T.);
#44899=ADVANCED_FACE('',(#6044),#3237,.T.);
#44900=ADVANCED_FACE('',(#6045),#3238,.T.);
#44901=ADVANCED_FACE('',(#6046),#3239,.T.);
#44902=ADVANCED_FACE('',(#6047),#788,.T.);
#44903=ADVANCED_FACE('',(#6048),#3240,.T.);
#44904=ADVANCED_FACE('',(#6049),#3241,.T.);
#44905=ADVANCED_FACE('',(#6050),#789,.T.);
#44906=ADVANCED_FACE('',(#6051),#790,.T.);
#44907=ADVANCED_FACE('',(#6052),#3242,.T.);
#44908=ADVANCED_FACE('',(#6053),#3243,.T.);
#44909=ADVANCED_FACE('',(#6054),#42490,.F.);
#44910=ADVANCED_FACE('',(#6055),#42491,.F.);
#44911=ADVANCED_FACE('',(#6056),#3244,.T.);
#44912=ADVANCED_FACE('',(#6057),#3245,.T.);
#44913=ADVANCED_FACE('',(#6058),#791,.T.);
#44914=ADVANCED_FACE('',(#6059),#3246,.T.);
#44915=ADVANCED_FACE('',(#6060),#3247,.T.);
#44916=ADVANCED_FACE('',(#6061),#3248,.T.);
#44917=ADVANCED_FACE('',(#6062),#3249,.T.);
#44918=ADVANCED_FACE('',(#6063),#3250,.T.);
#44919=ADVANCED_FACE('',(#6064),#792,.T.);
#44920=ADVANCED_FACE('',(#6065),#3251,.T.);
#44921=ADVANCED_FACE('',(#6066),#793,.T.);
#44922=ADVANCED_FACE('',(#6067),#3252,.T.);
#44923=ADVANCED_FACE('',(#6068),#3253,.T.);
#44924=ADVANCED_FACE('',(#6069),#3254,.T.);
#44925=ADVANCED_FACE('',(#6070),#794,.T.);
#44926=ADVANCED_FACE('',(#6071),#3255,.T.);
#44927=ADVANCED_FACE('',(#6072),#3256,.T.);
#44928=ADVANCED_FACE('',(#6073),#795,.T.);
#44929=ADVANCED_FACE('',(#6074),#796,.T.);
#44930=ADVANCED_FACE('',(#6075),#3257,.T.);
#44931=ADVANCED_FACE('',(#6076),#3258,.T.);
#44932=ADVANCED_FACE('',(#6077),#42492,.F.);
#44933=ADVANCED_FACE('',(#6078),#42493,.F.);
#44934=ADVANCED_FACE('',(#6079),#3259,.T.);
#44935=ADVANCED_FACE('',(#6080),#3260,.T.);
#44936=ADVANCED_FACE('',(#6081),#797,.T.);
#44937=ADVANCED_FACE('',(#6082),#3261,.T.);
#44938=ADVANCED_FACE('',(#6083),#3262,.T.);
#44939=ADVANCED_FACE('',(#6084),#3263,.T.);
#44940=ADVANCED_FACE('',(#6085),#3264,.T.);
#44941=ADVANCED_FACE('',(#6086),#3265,.T.);
#44942=ADVANCED_FACE('',(#6087),#798,.T.);
#44943=ADVANCED_FACE('',(#6088),#3266,.T.);
#44944=ADVANCED_FACE('',(#6089),#799,.T.);
#44945=ADVANCED_FACE('',(#6090),#3267,.T.);
#44946=ADVANCED_FACE('',(#6091),#3268,.T.);
#44947=ADVANCED_FACE('',(#6092),#3269,.T.);
#44948=ADVANCED_FACE('',(#6093),#800,.T.);
#44949=ADVANCED_FACE('',(#6094),#3270,.T.);
#44950=ADVANCED_FACE('',(#6095),#3271,.T.);
#44951=ADVANCED_FACE('',(#6096),#801,.T.);
#44952=ADVANCED_FACE('',(#6097),#802,.T.);
#44953=ADVANCED_FACE('',(#6098),#3272,.T.);
#44954=ADVANCED_FACE('',(#6099),#3273,.T.);
#44955=ADVANCED_FACE('',(#6100),#42494,.F.);
#44956=ADVANCED_FACE('',(#6101),#42495,.F.);
#44957=ADVANCED_FACE('',(#6102),#3274,.T.);
#44958=ADVANCED_FACE('',(#6103),#3275,.T.);
#44959=ADVANCED_FACE('',(#6104),#803,.T.);
#44960=ADVANCED_FACE('',(#6105),#3276,.T.);
#44961=ADVANCED_FACE('',(#6106),#3277,.T.);
#44962=ADVANCED_FACE('',(#6107),#3278,.T.);
#44963=ADVANCED_FACE('',(#6108),#3279,.T.);
#44964=ADVANCED_FACE('',(#6109),#3280,.T.);
#44965=ADVANCED_FACE('',(#6110),#804,.T.);
#44966=ADVANCED_FACE('',(#6111),#3281,.T.);
#44967=ADVANCED_FACE('',(#6112),#805,.T.);
#44968=ADVANCED_FACE('',(#6113),#3282,.T.);
#44969=ADVANCED_FACE('',(#6114),#3283,.T.);
#44970=ADVANCED_FACE('',(#6115),#3284,.T.);
#44971=ADVANCED_FACE('',(#6116),#806,.T.);
#44972=ADVANCED_FACE('',(#6117),#3285,.T.);
#44973=ADVANCED_FACE('',(#6118),#3286,.T.);
#44974=ADVANCED_FACE('',(#6119),#807,.T.);
#44975=ADVANCED_FACE('',(#6120),#808,.T.);
#44976=ADVANCED_FACE('',(#6121),#3287,.T.);
#44977=ADVANCED_FACE('',(#6122),#3288,.T.);
#44978=ADVANCED_FACE('',(#6123),#42496,.F.);
#44979=ADVANCED_FACE('',(#6124),#42497,.F.);
#44980=ADVANCED_FACE('',(#6125),#3289,.T.);
#44981=ADVANCED_FACE('',(#6126),#3290,.T.);
#44982=ADVANCED_FACE('',(#6127),#809,.T.);
#44983=ADVANCED_FACE('',(#6128),#3291,.T.);
#44984=ADVANCED_FACE('',(#6129),#3292,.T.);
#44985=ADVANCED_FACE('',(#6130),#3293,.T.);
#44986=ADVANCED_FACE('',(#6131),#3294,.T.);
#44987=ADVANCED_FACE('',(#6132),#3295,.T.);
#44988=ADVANCED_FACE('',(#6133),#810,.T.);
#44989=ADVANCED_FACE('',(#6134),#3296,.T.);
#44990=ADVANCED_FACE('',(#6135),#811,.T.);
#44991=ADVANCED_FACE('',(#6136),#3297,.T.);
#44992=ADVANCED_FACE('',(#6137),#3298,.T.);
#44993=ADVANCED_FACE('',(#6138),#3299,.T.);
#44994=ADVANCED_FACE('',(#6139),#812,.T.);
#44995=ADVANCED_FACE('',(#6140),#3300,.T.);
#44996=ADVANCED_FACE('',(#6141),#3301,.T.);
#44997=ADVANCED_FACE('',(#6142),#813,.T.);
#44998=ADVANCED_FACE('',(#6143),#814,.T.);
#44999=ADVANCED_FACE('',(#6144),#3302,.T.);
#45000=ADVANCED_FACE('',(#6145),#3303,.T.);
#45001=ADVANCED_FACE('',(#6146),#42498,.F.);
#45002=ADVANCED_FACE('',(#6147),#42499,.F.);
#45003=ADVANCED_FACE('',(#6148),#3304,.T.);
#45004=ADVANCED_FACE('',(#6149),#3305,.T.);
#45005=ADVANCED_FACE('',(#6150),#815,.T.);
#45006=ADVANCED_FACE('',(#6151),#3306,.T.);
#45007=ADVANCED_FACE('',(#6152),#3307,.T.);
#45008=ADVANCED_FACE('',(#6153),#3308,.T.);
#45009=ADVANCED_FACE('',(#6154),#3309,.T.);
#45010=ADVANCED_FACE('',(#6155),#3310,.T.);
#45011=ADVANCED_FACE('',(#6156),#816,.T.);
#45012=ADVANCED_FACE('',(#6157),#3311,.T.);
#45013=ADVANCED_FACE('',(#6158),#817,.T.);
#45014=ADVANCED_FACE('',(#6159),#3312,.T.);
#45015=ADVANCED_FACE('',(#6160),#3313,.T.);
#45016=ADVANCED_FACE('',(#6161),#3314,.T.);
#45017=ADVANCED_FACE('',(#6162),#818,.T.);
#45018=ADVANCED_FACE('',(#6163),#3315,.T.);
#45019=ADVANCED_FACE('',(#6164),#3316,.T.);
#45020=ADVANCED_FACE('',(#6165),#819,.T.);
#45021=ADVANCED_FACE('',(#6166),#820,.T.);
#45022=ADVANCED_FACE('',(#6167),#3317,.T.);
#45023=ADVANCED_FACE('',(#6168),#3318,.T.);
#45024=ADVANCED_FACE('',(#6169),#42500,.F.);
#45025=ADVANCED_FACE('',(#6170),#42501,.F.);
#45026=ADVANCED_FACE('',(#6171),#3319,.T.);
#45027=ADVANCED_FACE('',(#6172),#3320,.T.);
#45028=ADVANCED_FACE('',(#6173),#821,.T.);
#45029=ADVANCED_FACE('',(#6174),#3321,.T.);
#45030=ADVANCED_FACE('',(#6175),#3322,.T.);
#45031=ADVANCED_FACE('',(#6176),#3323,.T.);
#45032=ADVANCED_FACE('',(#6177),#3324,.T.);
#45033=ADVANCED_FACE('',(#6178),#3325,.T.);
#45034=ADVANCED_FACE('',(#6179),#822,.T.);
#45035=ADVANCED_FACE('',(#6180),#3326,.T.);
#45036=ADVANCED_FACE('',(#6181),#823,.T.);
#45037=ADVANCED_FACE('',(#6182),#3327,.T.);
#45038=ADVANCED_FACE('',(#6183),#3328,.T.);
#45039=ADVANCED_FACE('',(#6184),#3329,.T.);
#45040=ADVANCED_FACE('',(#6185),#824,.T.);
#45041=ADVANCED_FACE('',(#6186),#3330,.T.);
#45042=ADVANCED_FACE('',(#6187),#3331,.T.);
#45043=ADVANCED_FACE('',(#6188),#825,.T.);
#45044=ADVANCED_FACE('',(#6189),#826,.T.);
#45045=ADVANCED_FACE('',(#6190),#3332,.T.);
#45046=ADVANCED_FACE('',(#6191),#3333,.T.);
#45047=ADVANCED_FACE('',(#6192),#42502,.F.);
#45048=ADVANCED_FACE('',(#6193),#42503,.F.);
#45049=ADVANCED_FACE('',(#6194),#3334,.T.);
#45050=ADVANCED_FACE('',(#6195),#3335,.T.);
#45051=ADVANCED_FACE('',(#6196),#827,.T.);
#45052=ADVANCED_FACE('',(#6197),#3336,.T.);
#45053=ADVANCED_FACE('',(#6198),#3337,.T.);
#45054=ADVANCED_FACE('',(#6199),#3338,.T.);
#45055=ADVANCED_FACE('',(#6200),#3339,.T.);
#45056=ADVANCED_FACE('',(#6201),#3340,.T.);
#45057=ADVANCED_FACE('',(#6202),#828,.T.);
#45058=ADVANCED_FACE('',(#6203),#3341,.T.);
#45059=ADVANCED_FACE('',(#6204),#829,.T.);
#45060=ADVANCED_FACE('',(#6205),#3342,.T.);
#45061=ADVANCED_FACE('',(#6206),#3343,.T.);
#45062=ADVANCED_FACE('',(#6207),#3344,.T.);
#45063=ADVANCED_FACE('',(#6208),#830,.T.);
#45064=ADVANCED_FACE('',(#6209),#3345,.T.);
#45065=ADVANCED_FACE('',(#6210),#3346,.T.);
#45066=ADVANCED_FACE('',(#6211),#831,.T.);
#45067=ADVANCED_FACE('',(#6212),#832,.T.);
#45068=ADVANCED_FACE('',(#6213),#3347,.T.);
#45069=ADVANCED_FACE('',(#6214),#3348,.T.);
#45070=ADVANCED_FACE('',(#6215),#42504,.F.);
#45071=ADVANCED_FACE('',(#6216),#42505,.F.);
#45072=ADVANCED_FACE('',(#6217),#3349,.T.);
#45073=ADVANCED_FACE('',(#6218),#3350,.T.);
#45074=ADVANCED_FACE('',(#6219),#833,.T.);
#45075=ADVANCED_FACE('',(#6220),#3351,.T.);
#45076=ADVANCED_FACE('',(#6221),#3352,.T.);
#45077=ADVANCED_FACE('',(#6222),#3353,.T.);
#45078=ADVANCED_FACE('',(#6223),#3354,.T.);
#45079=ADVANCED_FACE('',(#6224),#3355,.T.);
#45080=ADVANCED_FACE('',(#6225),#834,.T.);
#45081=ADVANCED_FACE('',(#6226),#3356,.T.);
#45082=ADVANCED_FACE('',(#6227),#835,.T.);
#45083=ADVANCED_FACE('',(#6228),#3357,.T.);
#45084=ADVANCED_FACE('',(#6229),#3358,.T.);
#45085=ADVANCED_FACE('',(#6230),#3359,.T.);
#45086=ADVANCED_FACE('',(#6231),#836,.T.);
#45087=ADVANCED_FACE('',(#6232),#3360,.T.);
#45088=ADVANCED_FACE('',(#6233),#3361,.T.);
#45089=ADVANCED_FACE('',(#6234),#837,.T.);
#45090=ADVANCED_FACE('',(#6235),#838,.T.);
#45091=ADVANCED_FACE('',(#6236),#3362,.T.);
#45092=ADVANCED_FACE('',(#6237),#3363,.T.);
#45093=ADVANCED_FACE('',(#6238),#3364,.T.);
#45094=ADVANCED_FACE('',(#6239),#3365,.T.);
#45095=ADVANCED_FACE('',(#6240),#839,.T.);
#45096=ADVANCED_FACE('',(#6241),#42506,.F.);
#45097=ADVANCED_FACE('',(#6242),#42507,.F.);
#45098=ADVANCED_FACE('',(#6243),#3366,.T.);
#45099=ADVANCED_FACE('',(#6244),#3367,.T.);
#45100=ADVANCED_FACE('',(#6245),#3368,.T.);
#45101=ADVANCED_FACE('',(#6246),#3369,.T.);
#45102=ADVANCED_FACE('',(#6247),#3370,.T.);
#45103=ADVANCED_FACE('',(#6248),#840,.T.);
#45104=ADVANCED_FACE('',(#6249),#3371,.T.);
#45105=ADVANCED_FACE('',(#6250),#841,.T.);
#45106=ADVANCED_FACE('',(#6251),#3372,.T.);
#45107=ADVANCED_FACE('',(#6252),#3373,.T.);
#45108=ADVANCED_FACE('',(#6253),#3374,.T.);
#45109=ADVANCED_FACE('',(#6254),#842,.T.);
#45110=ADVANCED_FACE('',(#6255),#3375,.T.);
#45111=ADVANCED_FACE('',(#6256),#3376,.T.);
#45112=ADVANCED_FACE('',(#6257),#843,.T.);
#45113=ADVANCED_FACE('',(#6258),#844,.T.);
#45114=ADVANCED_FACE('',(#6259),#3377,.T.);
#45115=ADVANCED_FACE('',(#6260),#3378,.T.);
#45116=ADVANCED_FACE('',(#6261),#42508,.F.);
#45117=ADVANCED_FACE('',(#6262),#42509,.F.);
#45118=ADVANCED_FACE('',(#6263),#3379,.T.);
#45119=ADVANCED_FACE('',(#6264),#3380,.T.);
#45120=ADVANCED_FACE('',(#6265),#845,.T.);
#45121=ADVANCED_FACE('',(#6266),#3381,.T.);
#45122=ADVANCED_FACE('',(#6267),#3382,.T.);
#45123=ADVANCED_FACE('',(#6268),#3383,.T.);
#45124=ADVANCED_FACE('',(#6269),#3384,.T.);
#45125=ADVANCED_FACE('',(#6270),#3385,.T.);
#45126=ADVANCED_FACE('',(#6271),#846,.T.);
#45127=ADVANCED_FACE('',(#6272),#3386,.T.);
#45128=ADVANCED_FACE('',(#6273),#847,.T.);
#45129=ADVANCED_FACE('',(#6274),#3387,.T.);
#45130=ADVANCED_FACE('',(#6275),#3388,.T.);
#45131=ADVANCED_FACE('',(#6276),#3389,.T.);
#45132=ADVANCED_FACE('',(#6277),#848,.T.);
#45133=ADVANCED_FACE('',(#6278),#3390,.T.);
#45134=ADVANCED_FACE('',(#6279),#3391,.T.);
#45135=ADVANCED_FACE('',(#6280),#849,.T.);
#45136=ADVANCED_FACE('',(#6281),#850,.T.);
#45137=ADVANCED_FACE('',(#6282),#3392,.T.);
#45138=ADVANCED_FACE('',(#6283),#3393,.T.);
#45139=ADVANCED_FACE('',(#6284),#42510,.F.);
#45140=ADVANCED_FACE('',(#6285),#42511,.F.);
#45141=ADVANCED_FACE('',(#6286),#3394,.T.);
#45142=ADVANCED_FACE('',(#6287),#3395,.T.);
#45143=ADVANCED_FACE('',(#6288),#851,.T.);
#45144=ADVANCED_FACE('',(#6289),#3396,.T.);
#45145=ADVANCED_FACE('',(#6290),#3397,.T.);
#45146=ADVANCED_FACE('',(#6291),#3398,.T.);
#45147=ADVANCED_FACE('',(#6292),#3399,.T.);
#45148=ADVANCED_FACE('',(#6293),#3400,.T.);
#45149=ADVANCED_FACE('',(#6294),#852,.T.);
#45150=ADVANCED_FACE('',(#6295),#3401,.T.);
#45151=ADVANCED_FACE('',(#6296),#853,.T.);
#45152=ADVANCED_FACE('',(#6297),#3402,.T.);
#45153=ADVANCED_FACE('',(#6298),#3403,.T.);
#45154=ADVANCED_FACE('',(#6299),#3404,.T.);
#45155=ADVANCED_FACE('',(#6300),#854,.T.);
#45156=ADVANCED_FACE('',(#6301),#3405,.T.);
#45157=ADVANCED_FACE('',(#6302),#3406,.T.);
#45158=ADVANCED_FACE('',(#6303),#855,.T.);
#45159=ADVANCED_FACE('',(#6304),#856,.T.);
#45160=ADVANCED_FACE('',(#6305),#3407,.T.);
#45161=ADVANCED_FACE('',(#6306),#3408,.T.);
#45162=ADVANCED_FACE('',(#6307),#42512,.F.);
#45163=ADVANCED_FACE('',(#6308),#42513,.F.);
#45164=ADVANCED_FACE('',(#6309),#3409,.T.);
#45165=ADVANCED_FACE('',(#6310),#3410,.T.);
#45166=ADVANCED_FACE('',(#6311),#857,.T.);
#45167=ADVANCED_FACE('',(#6312),#3411,.T.);
#45168=ADVANCED_FACE('',(#6313),#3412,.T.);
#45169=ADVANCED_FACE('',(#6314),#3413,.T.);
#45170=ADVANCED_FACE('',(#6315),#3414,.T.);
#45171=ADVANCED_FACE('',(#6316),#3415,.T.);
#45172=ADVANCED_FACE('',(#6317),#858,.T.);
#45173=ADVANCED_FACE('',(#6318),#3416,.T.);
#45174=ADVANCED_FACE('',(#6319),#859,.T.);
#45175=ADVANCED_FACE('',(#6320),#3417,.T.);
#45176=ADVANCED_FACE('',(#6321),#3418,.T.);
#45177=ADVANCED_FACE('',(#6322),#3419,.T.);
#45178=ADVANCED_FACE('',(#6323),#860,.T.);
#45179=ADVANCED_FACE('',(#6324),#3420,.T.);
#45180=ADVANCED_FACE('',(#6325),#3421,.T.);
#45181=ADVANCED_FACE('',(#6326),#861,.T.);
#45182=ADVANCED_FACE('',(#6327),#862,.T.);
#45183=ADVANCED_FACE('',(#6328),#3422,.T.);
#45184=ADVANCED_FACE('',(#6329),#3423,.T.);
#45185=ADVANCED_FACE('',(#6330),#42514,.F.);
#45186=ADVANCED_FACE('',(#6331),#42515,.F.);
#45187=ADVANCED_FACE('',(#6332),#3424,.T.);
#45188=ADVANCED_FACE('',(#6333),#3425,.T.);
#45189=ADVANCED_FACE('',(#6334),#863,.T.);
#45190=ADVANCED_FACE('',(#6335),#3426,.T.);
#45191=ADVANCED_FACE('',(#6336),#3427,.T.);
#45192=ADVANCED_FACE('',(#6337),#3428,.T.);
#45193=ADVANCED_FACE('',(#6338),#3429,.T.);
#45194=ADVANCED_FACE('',(#6339),#3430,.T.);
#45195=ADVANCED_FACE('',(#6340),#864,.T.);
#45196=ADVANCED_FACE('',(#6341),#3431,.T.);
#45197=ADVANCED_FACE('',(#6342),#865,.T.);
#45198=ADVANCED_FACE('',(#6343),#3432,.T.);
#45199=ADVANCED_FACE('',(#6344),#3433,.T.);
#45200=ADVANCED_FACE('',(#6345),#3434,.T.);
#45201=ADVANCED_FACE('',(#6346),#866,.T.);
#45202=ADVANCED_FACE('',(#6347),#3435,.T.);
#45203=ADVANCED_FACE('',(#6348),#3436,.T.);
#45204=ADVANCED_FACE('',(#6349),#867,.T.);
#45205=ADVANCED_FACE('',(#6350),#868,.T.);
#45206=ADVANCED_FACE('',(#6351),#3437,.T.);
#45207=ADVANCED_FACE('',(#6352),#3438,.T.);
#45208=ADVANCED_FACE('',(#6353),#42516,.F.);
#45209=ADVANCED_FACE('',(#6354),#42517,.F.);
#45210=ADVANCED_FACE('',(#6355),#3439,.T.);
#45211=ADVANCED_FACE('',(#6356),#3440,.T.);
#45212=ADVANCED_FACE('',(#6357),#869,.T.);
#45213=ADVANCED_FACE('',(#6358),#3441,.T.);
#45214=ADVANCED_FACE('',(#6359),#3442,.T.);
#45215=ADVANCED_FACE('',(#6360),#3443,.T.);
#45216=ADVANCED_FACE('',(#6361),#3444,.T.);
#45217=ADVANCED_FACE('',(#6362),#3445,.T.);
#45218=ADVANCED_FACE('',(#6363),#870,.T.);
#45219=ADVANCED_FACE('',(#6364),#3446,.T.);
#45220=ADVANCED_FACE('',(#6365),#871,.T.);
#45221=ADVANCED_FACE('',(#6366),#3447,.T.);
#45222=ADVANCED_FACE('',(#6367),#3448,.T.);
#45223=ADVANCED_FACE('',(#6368),#3449,.T.);
#45224=ADVANCED_FACE('',(#6369),#872,.T.);
#45225=ADVANCED_FACE('',(#6370),#3450,.T.);
#45226=ADVANCED_FACE('',(#6371),#3451,.T.);
#45227=ADVANCED_FACE('',(#6372),#873,.T.);
#45228=ADVANCED_FACE('',(#6373),#874,.T.);
#45229=ADVANCED_FACE('',(#6374),#3452,.T.);
#45230=ADVANCED_FACE('',(#6375),#3453,.T.);
#45231=ADVANCED_FACE('',(#6376),#42518,.F.);
#45232=ADVANCED_FACE('',(#6377),#42519,.F.);
#45233=ADVANCED_FACE('',(#6378),#3454,.T.);
#45234=ADVANCED_FACE('',(#6379),#3455,.T.);
#45235=ADVANCED_FACE('',(#6380),#875,.T.);
#45236=ADVANCED_FACE('',(#6381),#3456,.T.);
#45237=ADVANCED_FACE('',(#6382),#3457,.T.);
#45238=ADVANCED_FACE('',(#6383),#3458,.T.);
#45239=ADVANCED_FACE('',(#6384),#3459,.T.);
#45240=ADVANCED_FACE('',(#6385),#3460,.T.);
#45241=ADVANCED_FACE('',(#6386),#876,.T.);
#45242=ADVANCED_FACE('',(#6387),#3461,.T.);
#45243=ADVANCED_FACE('',(#6388),#877,.T.);
#45244=ADVANCED_FACE('',(#6389),#3462,.T.);
#45245=ADVANCED_FACE('',(#6390),#3463,.T.);
#45246=ADVANCED_FACE('',(#6391),#3464,.T.);
#45247=ADVANCED_FACE('',(#6392),#878,.T.);
#45248=ADVANCED_FACE('',(#6393),#3465,.T.);
#45249=ADVANCED_FACE('',(#6394),#3466,.T.);
#45250=ADVANCED_FACE('',(#6395),#879,.T.);
#45251=ADVANCED_FACE('',(#6396),#880,.T.);
#45252=ADVANCED_FACE('',(#6397),#3467,.T.);
#45253=ADVANCED_FACE('',(#6398),#3468,.T.);
#45542=CLOSED_SHELL('',(#42648,#42649,#42650,#42651,#42652,#42653,#42654,
#42655,#42656,#42657,#42658,#42659,#42660,#42661,#42662,#42663,#42664,#42665,
#42666,#42667,#42668,#42669,#42670,#42671,#42672,#42673,#42674,#42675,#42676,
#42677,#42678,#42679,#42680,#42681,#42682,#42683,#42684,#42685,#42686,#42687,
#42688,#42689,#42690,#42691,#42692,#42693,#42694,#42695,#42696,#42697,#42698,
#42699,#42700,#42701,#42702,#42703,#42704,#42705,#42706,#42707,#42708,#42709,
#42710,#42711,#42712,#42713,#42714,#42715,#42716,#42717,#42718,#42719,#42720,
#42721,#42722,#42723,#42724,#42725,#42726,#42727,#42728,#42729,#42730,#42731,
#42732,#42733,#42734,#42735,#42736,#42737,#42738,#42739,#42740,#42741,#42742,
#42743,#42744,#42745,#42746,#42747,#42748,#42749,#42750,#42751,#42752,#42753,
#42754,#42755,#42756,#42757,#42758,#42759,#42760,#42761,#42762,#42763,#42764,
#42765,#42766,#42767,#42768,#42769,#42770,#42771,#42772,#42773,#42774,#42775,
#42776,#42777,#42778,#42779,#42780,#42781,#42782,#42783,#42784,#42785,#42786,
#42787,#42788,#42789,#42790,#42791,#42792,#42793,#42794,#42795,#42796,#42797,
#42798,#42799,#42800,#42801,#42802,#42803,#42804,#42805,#42806,#42807,#42808,
#42809,#42810,#42811,#42812,#42813,#42814,#42815,#42816,#42817,#42818,#42819,
#42820,#42821,#42822,#42823,#42824,#42825,#42826,#42827,#42828,#42829,#42830,
#42831,#42832,#42833,#42834,#42835,#42836,#42837,#42838,#42839,#42840,#42841,
#42842,#42843,#42844,#42845,#42846,#42847,#42848,#42849,#42850,#42851,#42852,
#42853,#42854,#42855,#42856,#42857,#42858,#42859,#42860,#42861,#42862,#42863,
#42864,#42865,#42866,#42867,#42868,#42869,#42870,#42871,#42872,#42873,#42874,
#42875,#42876,#42877,#42878,#42879,#42880,#42881,#42882,#42883,#42884,#42885,
#42886,#42887,#42888,#42889,#42890,#42891,#42892,#42893,#42894,#42895,#42896,
#42897,#42898,#42899,#42900,#42901,#42902,#42903,#42904,#42905,#42906,#42907,
#42908,#42909,#42910,#42911,#42912,#42913,#42914,#42915,#42916,#42917,#42918,
#42919,#42920,#42921,#42922,#42923,#42924,#42925,#42926,#42927,#42928,#42929,
#42930,#42931,#42932,#42933,#42934,#42935,#42936,#42937,#42938,#42939,#42940,
#42941,#42942,#42943,#42944,#42945,#42946,#42947,#42948,#42949,#42950,#42951,
#42952,#42953,#42954,#42955,#42956,#42957,#42958,#42959,#42960,#42961,#42962,
#42963,#42964,#42965,#42966,#42967,#42968,#42969,#42970,#42971,#42972,#42973,
#42974,#42975,#42976,#42977,#42978,#42979,#42980,#42981,#42982,#42983,#42984,
#42985,#42986,#42987,#42988,#42989,#42990,#42991,#42992,#42993,#42994,#42995,
#42996,#42997,#42998,#42999,#43000,#43001,#43002,#43003,#43004,#43005,#43006,
#43007,#43008,#43009,#43010,#43011,#43012,#43013,#43014,#43015,#43016,#43017,
#43018,#43019,#43020,#43021,#43022,#43023,#43024,#43025,#43026,#43027,#43028,
#43029,#43030,#43031,#43032,#43033,#43034,#43035,#43036,#43037,#43038,#43039,
#43040,#43041,#43042,#43043,#43044,#43045,#43046,#43047,#43048,#43049,#43050,
#43051,#43052,#43053,#43054,#43055,#43056,#43057,#43058,#43059,#43060,#43061,
#43062,#43063,#43064,#43065,#43066,#43067,#43068,#43069,#43070,#43071,#43072,
#43073,#43074,#43075,#43076,#43077,#43078,#43079,#43080,#43081,#43082,#43083,
#43084,#43085,#43086,#43087,#43088,#43089,#43090,#43091,#43092,#43093,#43094,
#43095,#43096,#43097,#43098,#43099,#43100,#43101,#43102,#43103,#43104,#43105,
#43106,#43107,#43108,#43109,#43110,#43111,#43112,#43113,#43114,#43115,#43116,
#43117,#43118,#43119,#43120,#43121,#43122,#43123,#43124,#43125,#43126,#43127,
#43128,#43129,#43130,#43131,#43132,#43133,#43134,#43135,#43136,#43137,#43138,
#43139,#43140,#43141,#43142,#43143,#43144,#43145,#43146,#43147,#43148,#43149,
#43150,#43151,#43152,#43153,#43154,#43155,#43156,#43157,#43158,#43159,#43160,
#43161,#43162,#43163,#43164,#43165,#43166,#43167,#43168,#43169,#43170,#43171,
#43172,#43173,#43174,#43175,#43176,#43177,#43178,#43179,#43180,#43181,#43182,
#43183,#43184,#43185,#43186,#43187,#43188,#43189,#43190,#43191,#43192,#43193,
#43194,#43195,#43196,#43197,#43198,#43199,#43200,#43201,#43202,#43203,#43204,
#43205,#43206,#43207,#43208,#43209,#43210,#43211,#43212,#43213,#43214,#43215,
#43216,#43217,#43218,#43219,#43220,#43221,#43222,#43223,#43224,#43225,#43226,
#43227,#43228,#43229,#43230,#43231,#43232,#43233,#43234,#43235,#43236,#43237,
#43238,#43239,#43240,#43241,#43242,#43243,#43244,#43245,#43246,#43247,#43248,
#43249,#43250,#43251,#43252,#43253,#43254,#43255,#43256,#43257,#43258,#43259,
#43260,#43261,#43262,#43263,#43264,#43265,#43266,#43267,#43268,#43269,#43270,
#43271,#43272,#43273,#43274,#43275,#43276,#43277,#43278,#43279,#43280,#43281,
#43282,#43283,#43284,#43285,#43286,#43287,#43288,#43289,#43290,#43291,#43292,
#43293,#43294,#43295,#43296,#43297,#43298,#43299,#43300,#43301,#43302,#43303,
#43304,#43305,#43306,#43307,#43308,#43309,#43310,#43311,#43312,#43313,#43314,
#43315,#43316,#43317,#43318,#43319,#43320,#43321,#43322,#43323,#43324,#43325,
#43326,#43327,#43328,#43329,#43330,#43331,#43332,#43333,#43334,#43335,#43336,
#43337,#43338,#43339,#43340,#43341,#43342,#43343,#43344,#43345,#43346,#43347,
#43348,#43349,#43350,#43351,#43352,#43353,#43354,#43355,#43356,#43357,#43358,
#43359,#43360,#43361,#43362,#43363,#43364,#43365,#43366,#43367,#43368,#43369,
#43370,#43371,#43372,#43373,#43374,#43375,#43376,#43377,#43378,#43379,#43380,
#43381,#43382,#43383,#43384,#43385,#43386,#43387,#43388,#43389,#43390,#43391,
#43392,#43393,#43394,#43395,#43396,#43397,#43398,#43399,#43400,#43401,#43402,
#43403,#43404,#43405,#43406,#43407,#43408,#43409,#43410,#43411,#43412,#43413,
#43414,#43415,#43416,#43417,#43418,#43419,#43420,#43421,#43422,#43423,#43424,
#43425,#43426,#43427,#43428,#43429,#43430,#43431,#43432,#43433,#43434,#43435,
#43436,#43437,#43438,#43439,#43440,#43441,#43442,#43443,#43444,#43445,#43446,
#43447,#43448,#43449,#43450,#43451,#43452,#43453,#43454,#43455,#43456,#43457,
#43458,#43459,#43460,#43461,#43462,#43463,#43464,#43465,#43466,#43467,#43468,
#43469,#43470,#43471,#43472,#43473,#43474,#43475,#43476,#43477,#43478,#43479,
#43480,#43481,#43482,#43483,#43484,#43485,#43486,#43487,#43488,#43489,#43490,
#43491,#43492,#43493,#43494,#43495,#43496,#43497,#43498,#43499,#43500,#43501,
#43502,#43503,#43504,#43505,#43506,#43507,#43508,#43509,#43510,#43511,#43512,
#43513,#43514,#43515,#43516,#43517,#43518,#43519,#43520,#43521,#43522,#43523,
#43524,#43525,#43526,#43527,#43528,#43529,#43530,#43531,#43532,#43533,#43534,
#43535,#43536,#43537,#43538,#43539,#43540,#43541,#43542,#43543,#43544,#43545,
#43546,#43547,#43548,#43549,#43550,#43551,#43552,#43553,#43554,#43555,#43556,
#43557,#43558,#43559,#43560,#43561,#43562,#43563,#43564,#43565,#43566,#43567,
#43568,#43569,#43570,#43571,#43572,#43573,#43574,#43575,#43576,#43577,#43578,
#43579,#43580,#43581,#43582,#43583,#43584,#43585,#43586,#43587,#43588,#43589,
#43590,#43591,#43592,#43593,#43594,#43595,#43596,#43597,#43598,#43599,#43600,
#43601,#43602,#43603,#43604,#43605,#43606,#43607,#43608,#43609,#43610,#43611,
#43612,#43613,#43614,#43615,#43616,#43617,#43618,#43619,#43620,#43621,#43622,
#43623,#43624,#43625,#43626,#43627,#43628,#43629,#43630,#43631,#43632,#43633,
#43634,#43635,#43636,#43637,#43638,#43639,#43640,#43641,#43642,#43643,#43644,
#43645,#43646,#43647,#43648,#43649,#43650,#43651,#43652,#43653,#43654,#43655,
#43656,#43657,#43658,#43659,#43660,#43661,#43662,#43663,#43664,#43665,#43666,
#43667,#43668,#43669,#43670,#43671,#43672,#43673,#43674,#43675,#43676,#43677,
#43678,#43679,#43680,#43681,#43682,#43683,#43684,#43685,#43686,#43687,#43688,
#43689,#43690,#43691,#43692,#43693,#43694,#43695,#43696,#43697,#43698,#43699,
#43700,#43701,#43702,#43703,#43704,#43705,#43706,#43707,#43708,#43709,#43710,
#43711,#43712,#43713,#43714,#43715,#43716,#43717,#43718,#43719,#43720,#43721,
#43722,#43723,#43724,#43725,#43726,#43727,#43728,#43729,#43730,#43731,#43732,
#43733,#43734,#43735,#43736,#43737,#43738,#43739,#43740,#43741,#43742,#43743,
#43744,#43745,#43746,#43747,#43748,#43749,#43750,#43751,#43752,#43753,#43754,
#43755,#43756,#43757,#43758,#43759,#43760,#43761,#43762,#43763,#43764,#43765,
#43766,#43767,#43768,#43769,#43770,#43771,#43772,#43773,#43774,#43775,#43776,
#43777,#43778,#43779,#43780,#43781,#43782,#43783,#43784,#43785,#43786,#43787,
#43788,#43789,#43790,#43791,#43792,#43793,#43794,#43795,#43796,#43797,#43798,
#43799,#43800,#43801,#43802,#43803,#43804,#43805,#43806,#43807,#43808,#43809,
#43810,#43811,#43812,#43813,#43814,#43815,#43816,#43817,#43818,#43819,#43820,
#43821,#43822,#43823,#43824,#43825,#43826,#43827,#43828,#43829,#43830,#43831,
#43832,#43833,#43834,#43835,#43836,#43837,#43838,#43839,#43840,#43841,#43842,
#43843,#43844,#43845,#43846,#43847,#43848,#43849,#43850,#43851,#43852,#43853,
#43854,#43855,#43856,#43857,#43858,#43859,#43860,#43861,#43862,#43863,#43864,
#43865,#43866,#43867,#43868,#43869,#43870,#43871,#43872,#43873,#43874,#43875,
#43876,#43877,#43878,#43879,#43880,#43881,#43882,#43883,#43884,#43885,#43886,
#43887,#43888,#43889,#43890,#43891,#43892,#43893,#43894,#43895,#43896,#43897,
#43898,#43899,#43900,#43901,#43902,#43903,#43904,#43905,#43906,#43907,#43908,
#43909,#43910,#43911,#43912,#43913,#43914,#43915,#43916,#43917,#43918,#43919,
#43920,#43921,#43922,#43923,#43924,#43925,#43926,#43927,#43928,#43929,#43930,
#43931,#43932,#43933,#43934,#43935,#43936,#43937,#43938,#43939,#43940,#43941,
#43942,#43943,#43944,#43945,#43946,#43947,#43948,#43949,#43950,#43951,#43952,
#43953,#43954,#43955,#43956,#43957,#43958,#43959,#43960,#43961,#43962,#43963,
#43964,#43965,#43966,#43967,#43968,#43969,#43970,#43971,#43972,#43973,#43974,
#43975,#43976,#43977,#43978,#43979,#43980,#43981,#43982,#43983,#43984,#43985,
#43986,#43987,#43988,#43989,#43990,#43991,#43992,#43993,#43994,#43995,#43996,
#43997,#43998,#43999,#44000,#44001,#44002,#44003,#44004,#44005,#44006,#44007,
#44008,#44009,#44010,#44011,#44012,#44013,#44014,#44015,#44016,#44017,#44018,
#44019,#44020,#44021,#44022,#44023,#44024,#44025,#44026,#44027,#44028,#44029,
#44030,#44031,#44032,#44033,#44034,#44035,#44036,#44037,#44038,#44039,#44040,
#44041,#44042,#44043,#44044,#44045,#44046,#44047,#44048,#44049,#44050,#44051,
#44052,#44053,#44054,#44055,#44056,#44057,#44058,#44059,#44060,#44061,#44062,
#44063,#44064,#44065,#44066,#44067,#44068,#44069,#44070,#44071,#44072,#44073,
#44074,#44075,#44076,#44077,#44078,#44079,#44080,#44081,#44082,#44083,#44084,
#44085,#44086,#44087,#44088,#44089,#44090,#44091,#44092,#44093,#44094,#44095,
#44096,#44097,#44098,#44099,#44100,#44101,#44102,#44103,#44104,#44105,#44106,
#44107,#44108,#44109,#44110,#44111,#44112,#44113,#44114,#44115,#44116,#44117,
#44118,#44119,#44120,#44121,#44122,#44123,#44124,#44125,#44126,#44127,#44128,
#44129,#44130,#44131,#44132,#44133,#44134,#44135,#44136,#44137,#44138,#44139,
#44140,#44141,#44142,#44143,#44144,#44145,#44146,#44147,#44148,#44149,#44150,
#44151,#44152,#44153,#44154,#44155,#44156,#44157,#44158,#44159,#44160,#44161,
#44162,#44163,#44164,#44165,#44166,#44167,#44168,#44169,#44170,#44171,#44172,
#44173,#44174,#44175,#44176,#44177,#44178,#44179,#44180,#44181,#44182,#44183,
#44184,#44185,#44186,#44187,#44188,#44189,#44190,#44191,#44192,#44193,#44194,
#44195,#44196,#44197,#44198,#44199,#44200,#44201,#44202,#44203,#44204,#44205,
#44206,#44207,#44208,#44209,#44210,#44211,#44212,#44213,#44214,#44215,#44216,
#44217,#44218,#44219,#44220,#44221,#44222,#44223,#44224,#44225,#44226,#44227,
#44228,#44229,#44230,#44231,#44232,#44233,#44234,#44235,#44236,#44237,#44238,
#44239,#44240,#44241,#44242,#44243,#44244,#44245,#44246,#44247,#44248,#44249,
#44250,#44251,#44252,#44253,#44254,#44255,#44256,#44257,#44258,#44259,#44260,
#44261,#44262,#44263,#44264,#44265,#44266,#44267,#44268,#44269,#44270,#44271,
#44272,#44273,#44274,#44275,#44276,#44277,#44278,#44279,#44280,#44281,#44282,
#44283,#44284,#44285,#44286,#44287,#44288,#44289,#44290,#44291,#44292,#44293,
#44294,#44295,#44296,#44297,#44298,#44299,#44300,#44301,#44302,#44303,#44304,
#44305,#44306,#44307,#44308,#44309,#44310,#44311,#44312,#44313,#44314,#44315,
#44316,#44317,#44318,#44319,#44320,#44321,#44322,#44323,#44324,#44325,#44326,
#44327,#44328,#44329,#44330,#44331,#44332,#44333,#44334,#44335,#44336,#44337,
#44338,#44339,#44340,#44341,#44342,#44343,#44344,#44345,#44346,#44347,#44348,
#44349,#44350,#44351,#44352,#44353,#44354,#44355,#44356,#44357,#44358,#44359,
#44360,#44361,#44362,#44363,#44364,#44365,#44366,#44367,#44368,#44369,#44370,
#44371,#44372,#44373,#44374,#44375,#44376,#44377,#44378,#44379,#44380,#44381,
#44382,#44383,#44384,#44385,#44386,#44387,#44388,#44389,#44390,#44391,#44392,
#44393,#44394,#44395,#44396,#44397,#44398,#44399,#44400,#44401,#44402,#44403,
#44404,#44405,#44406,#44407,#44408,#44409,#44410,#44411,#44412,#44413,#44414,
#44415,#44416,#44417,#44418,#44419,#44420,#44421,#44422,#44423,#44424,#44425,
#44426,#44427,#44428,#44429,#44430,#44431,#44432,#44433,#44434,#44435,#44436,
#44437,#44438,#44439,#44440,#44441,#44442,#44443,#44444,#44445,#44446,#44447,
#44448,#44449,#44450,#44451,#44452,#44453,#44454,#44455,#44456,#44457,#44458,
#44459,#44460,#44461,#44462,#44463,#44464,#44465,#44466,#44467,#44468,#44469,
#44470,#44471,#44472,#44473,#44474,#44475,#44476,#44477,#44478,#44479,#44480,
#44481,#44482,#44483,#44484,#44485,#44486,#44487,#44488,#44489,#44490,#44491,
#44492,#44493,#44494,#44495,#44496,#44497,#44498,#44499,#44500,#44501,#44502,
#44503,#44504,#44505,#44506,#44507,#44508,#44509,#44510,#44511,#44512,#44513,
#44514,#44515,#44516,#44517,#44518,#44519,#44520,#44521,#44522,#44523,#44524,
#44525,#44526,#44527,#44528,#44529,#44530,#44531,#44532,#44533,#44534,#44535,
#44536,#44537,#44538,#44539,#44540,#44541,#44542,#44543,#44544,#44545,#44546,
#44547,#44548,#44549,#44550,#44551,#44552,#44553,#44554,#44555,#44556,#44557,
#44558,#44559,#44560,#44561,#44562,#44563,#44564,#44565,#44566,#44567,#44568,
#44569,#44570,#44571,#44572,#44573,#44574,#44575,#44576,#44577,#44578,#44579,
#44580,#44581,#44582,#44583,#44584,#44585,#44586,#44587,#44588,#44589,#44590,
#44591,#44592,#44593,#44594,#44595,#44596,#44597,#44598,#44599,#44600,#44601,
#44602,#44603,#44604,#44605,#44606,#44607,#44608,#44609,#44610,#44611,#44612,
#44613,#44614,#44615,#44616,#44617,#44618,#44619,#44620,#44621,#44622,#44623,
#44624,#44625,#44626,#44627,#44628,#44629,#44630,#44631,#44632,#44633,#44634,
#44635,#44636,#44637,#44638,#44639,#44640,#44641,#44642,#44643,#44644,#44645,
#44646,#44647,#44648,#44649,#44650,#44651,#44652,#44653,#44654,#44655,#44656,
#44657,#44658,#44659,#44660,#44661,#44662,#44663,#44664,#44665,#44666,#44667,
#44668,#44669,#44670,#44671,#44672,#44673,#44674,#44675,#44676,#44677,#44678,
#44679,#44680,#44681,#44682,#44683,#44684,#44685,#44686,#44687,#44688,#44689,
#44690,#44691,#44692,#44693,#44694,#44695,#44696,#44697,#44698,#44699,#44700,
#44701,#44702,#44703,#44704,#44705,#44706,#44707,#44708,#44709,#44710,#44711,
#44712,#44713,#44714,#44715,#44716,#44717,#44718,#44719,#44720,#44721,#44722,
#44723,#44724,#44725,#44726,#44727,#44728,#44729,#44730,#44731,#44732,#44733,
#44734,#44735,#44736,#44737,#44738,#44739,#44740,#44741,#44742,#44743,#44744,
#44745,#44746,#44747,#44748,#44749,#44750,#44751,#44752,#44753,#44754,#44755,
#44756,#44757,#44758,#44759,#44760,#44761,#44762,#44763,#44764,#44765,#44766,
#44767,#44768,#44769,#44770,#44771,#44772,#44773,#44774,#44775,#44776,#44777,
#44778,#44779,#44780,#44781,#44782,#44783,#44784,#44785,#44786,#44787,#44788,
#44789,#44790,#44791,#44792,#44793,#44794,#44795,#44796,#44797,#44798,#44799,
#44800,#44801,#44802,#44803,#44804,#44805,#44806,#44807,#44808,#44809,#44810,
#44811,#44812,#44813,#44814,#44815,#44816,#44817,#44818,#44819,#44820,#44821,
#44822,#44823,#44824,#44825,#44826,#44827,#44828,#44829,#44830,#44831,#44832,
#44833,#44834,#44835,#44836,#44837,#44838,#44839,#44840,#44841,#44842,#44843,
#44844,#44845,#44846,#44847,#44848,#44849,#44850,#44851,#44852,#44853,#44854,
#44855,#44856,#44857,#44858,#44859,#44860,#44861,#44862,#44863,#44864,#44865,
#44866,#44867,#44868,#44869,#44870,#44871,#44872,#44873,#44874,#44875,#44876,
#44877,#44878,#44879,#44880,#44881,#44882,#44883,#44884,#44885,#44886,#44887,
#44888,#44889,#44890,#44891,#44892,#44893,#44894,#44895,#44896,#44897,#44898,
#44899,#44900,#44901,#44902,#44903,#44904,#44905,#44906,#44907,#44908,#44909,
#44910,#44911,#44912,#44913,#44914,#44915,#44916,#44917,#44918,#44919,#44920,
#44921,#44922,#44923,#44924,#44925,#44926,#44927,#44928,#44929,#44930,#44931,
#44932,#44933,#44934,#44935,#44936,#44937,#44938,#44939,#44940,#44941,#44942,
#44943,#44944,#44945,#44946,#44947,#44948,#44949,#44950,#44951,#44952,#44953,
#44954,#44955,#44956,#44957,#44958,#44959,#44960,#44961,#44962,#44963,#44964,
#44965,#44966,#44967,#44968,#44969,#44970,#44971,#44972,#44973,#44974,#44975,
#44976,#44977,#44978,#44979,#44980,#44981,#44982,#44983,#44984,#44985,#44986,
#44987,#44988,#44989,#44990,#44991,#44992,#44993,#44994,#44995,#44996,#44997,
#44998,#44999,#45000,#45001,#45002,#45003,#45004,#45005,#45006,#45007,#45008,
#45009,#45010,#45011,#45012,#45013,#45014,#45015,#45016,#45017,#45018,#45019,
#45020,#45021,#45022,#45023,#45024,#45025,#45026,#45027,#45028,#45029,#45030,
#45031,#45032,#45033,#45034,#45035,#45036,#45037,#45038,#45039,#45040,#45041,
#45042,#45043,#45044,#45045,#45046,#45047,#45048,#45049,#45050,#45051,#45052,
#45053,#45054,#45055,#45056,#45057,#45058,#45059,#45060,#45061,#45062,#45063,
#45064,#45065,#45066,#45067,#45068,#45069,#45070,#45071,#45072,#45073,#45074,
#45075,#45076,#45077,#45078,#45079,#45080,#45081,#45082,#45083,#45084,#45085,
#45086,#45087,#45088,#45089,#45090,#45091,#45092,#45093,#45094,#45095,#45096,
#45097,#45098,#45099,#45100,#45101,#45102,#45103,#45104,#45105,#45106,#45107,
#45108,#45109,#45110,#45111,#45112,#45113,#45114,#45115,#45116,#45117,#45118,
#45119,#45120,#45121,#45122,#45123,#45124,#45125,#45126,#45127,#45128,#45129,
#45130,#45131,#45132,#45133,#45134,#45135,#45136,#45137,#45138,#45139,#45140,
#45141,#45142,#45143,#45144,#45145,#45146,#45147,#45148,#45149,#45150,#45151,
#45152,#45153,#45154,#45155,#45156,#45157,#45158,#45159,#45160,#45161,#45162,
#45163,#45164,#45165,#45166,#45167,#45168,#45169,#45170,#45171,#45172,#45173,
#45174,#45175,#45176,#45177,#45178,#45179,#45180,#45181,#45182,#45183,#45184,
#45185,#45186,#45187,#45188,#45189,#45190,#45191,#45192,#45193,#45194,#45195,
#45196,#45197,#45198,#45199,#45200,#45201,#45202,#45203,#45204,#45205,#45206,
#45207,#45208,#45209,#45210,#45211,#45212,#45213,#45214,#45215,#45216,#45217,
#45218,#45219,#45220,#45221,#45222,#45223,#45224,#45225,#45226,#45227,#45228,
#45229,#45230,#45231,#45232,#45233,#45234,#45235,#45236,#45237,#45238,#45239,
#45240,#45241,#45242,#45243,#45244,#45245,#45246,#45247,#45248,#45249,#45250,
#45251,#45252,#45253));
#45717=AXIS2_PLACEMENT_3D('',#63522,#50541,#50542);
#45718=AXIS2_PLACEMENT_3D('',#63523,#50543,#50544);
#45719=AXIS2_PLACEMENT_3D('',#63525,#50545,#50546);
#45720=AXIS2_PLACEMENT_3D('',#63528,#50548,#50549);
#45721=AXIS2_PLACEMENT_3D('',#63529,#50550,#50551);
#45722=AXIS2_PLACEMENT_3D('',#63540,#50553,#50554);
#45723=AXIS2_PLACEMENT_3D('',#63547,#50555,#50556);
#45724=AXIS2_PLACEMENT_3D('',#63549,#50557,#50558);
#45725=AXIS2_PLACEMENT_3D('',#63565,#50559,#50560);
#45726=AXIS2_PLACEMENT_3D('',#63567,#50561,#50562);
#45727=AXIS2_PLACEMENT_3D('',#63583,#50563,#50564);
#45728=AXIS2_PLACEMENT_3D('',#63585,#50565,#50566);
#45729=AXIS2_PLACEMENT_3D('',#63601,#50567,#50568);
#45730=AXIS2_PLACEMENT_3D('',#63603,#50569,#50570);
#45731=AXIS2_PLACEMENT_3D('',#63619,#50571,#50572);
#45732=AXIS2_PLACEMENT_3D('',#63621,#50573,#50574);
#45733=AXIS2_PLACEMENT_3D('',#63637,#50575,#50576);
#45734=AXIS2_PLACEMENT_3D('',#63639,#50577,#50578);
#45735=AXIS2_PLACEMENT_3D('',#63655,#50579,#50580);
#45736=AXIS2_PLACEMENT_3D('',#63657,#50581,#50582);
#45737=AXIS2_PLACEMENT_3D('',#63673,#50583,#50584);
#45738=AXIS2_PLACEMENT_3D('',#63675,#50585,#50586);
#45739=AXIS2_PLACEMENT_3D('',#63691,#50587,#50588);
#45740=AXIS2_PLACEMENT_3D('',#63693,#50589,#50590);
#45741=AXIS2_PLACEMENT_3D('',#63709,#50591,#50592);
#45742=AXIS2_PLACEMENT_3D('',#63711,#50593,#50594);
#45743=AXIS2_PLACEMENT_3D('',#63727,#50595,#50596);
#45744=AXIS2_PLACEMENT_3D('',#63729,#50597,#50598);
#45745=AXIS2_PLACEMENT_3D('',#63745,#50599,#50600);
#45746=AXIS2_PLACEMENT_3D('',#63747,#50601,#50602);
#45747=AXIS2_PLACEMENT_3D('',#63763,#50603,#50604);
#45748=AXIS2_PLACEMENT_3D('',#63765,#50605,#50606);
#45749=AXIS2_PLACEMENT_3D('',#63781,#50607,#50608);
#45750=AXIS2_PLACEMENT_3D('',#63783,#50609,#50610);
#45751=AXIS2_PLACEMENT_3D('',#63799,#50611,#50612);
#45752=AXIS2_PLACEMENT_3D('',#63801,#50613,#50614);
#45753=AXIS2_PLACEMENT_3D('',#63817,#50615,#50616);
#45754=AXIS2_PLACEMENT_3D('',#63819,#50617,#50618);
#45755=AXIS2_PLACEMENT_3D('',#63835,#50619,#50620);
#45756=AXIS2_PLACEMENT_3D('',#63837,#50621,#50622);
#45757=AXIS2_PLACEMENT_3D('',#63853,#50623,#50624);
#45758=AXIS2_PLACEMENT_3D('',#63855,#50625,#50626);
#45759=AXIS2_PLACEMENT_3D('',#63871,#50627,#50628);
#45760=AXIS2_PLACEMENT_3D('',#63873,#50629,#50630);
#45761=AXIS2_PLACEMENT_3D('',#63889,#50631,#50632);
#45762=AXIS2_PLACEMENT_3D('',#63891,#50633,#50634);
#45763=AXIS2_PLACEMENT_3D('',#63907,#50635,#50636);
#45764=AXIS2_PLACEMENT_3D('',#63909,#50637,#50638);
#45765=AXIS2_PLACEMENT_3D('',#63925,#50639,#50640);
#45766=AXIS2_PLACEMENT_3D('',#63927,#50641,#50642);
#45767=AXIS2_PLACEMENT_3D('',#63943,#50643,#50644);
#45768=AXIS2_PLACEMENT_3D('',#63945,#50645,#50646);
#45769=AXIS2_PLACEMENT_3D('',#63961,#50647,#50648);
#45770=AXIS2_PLACEMENT_3D('',#63963,#50649,#50650);
#45771=AXIS2_PLACEMENT_3D('',#63979,#50651,#50652);
#45772=AXIS2_PLACEMENT_3D('',#63981,#50653,#50654);
#45773=AXIS2_PLACEMENT_3D('',#63997,#50655,#50656);
#45774=AXIS2_PLACEMENT_3D('',#63999,#50657,#50658);
#45775=AXIS2_PLACEMENT_3D('',#64015,#50659,#50660);
#45776=AXIS2_PLACEMENT_3D('',#64017,#50661,#50662);
#45777=AXIS2_PLACEMENT_3D('',#64033,#50663,#50664);
#45778=AXIS2_PLACEMENT_3D('',#64035,#50665,#50666);
#45779=AXIS2_PLACEMENT_3D('',#64051,#50667,#50668);
#45780=AXIS2_PLACEMENT_3D('',#64053,#50669,#50670);
#45781=AXIS2_PLACEMENT_3D('',#64069,#50671,#50672);
#45782=AXIS2_PLACEMENT_3D('',#64071,#50673,#50674);
#45783=AXIS2_PLACEMENT_3D('',#64087,#50675,#50676);
#45784=AXIS2_PLACEMENT_3D('',#64089,#50677,#50678);
#45785=AXIS2_PLACEMENT_3D('',#64105,#50679,#50680);
#45786=AXIS2_PLACEMENT_3D('',#64107,#50681,#50682);
#45787=AXIS2_PLACEMENT_3D('',#64123,#50683,#50684);
#45788=AXIS2_PLACEMENT_3D('',#64125,#50685,#50686);
#45789=AXIS2_PLACEMENT_3D('',#64141,#50687,#50688);
#45790=AXIS2_PLACEMENT_3D('',#64143,#50689,#50690);
#45791=AXIS2_PLACEMENT_3D('',#64159,#50691,#50692);
#45792=AXIS2_PLACEMENT_3D('',#64161,#50693,#50694);
#45793=AXIS2_PLACEMENT_3D('',#64177,#50695,#50696);
#45794=AXIS2_PLACEMENT_3D('',#64179,#50697,#50698);
#45795=AXIS2_PLACEMENT_3D('',#64195,#50699,#50700);
#45796=AXIS2_PLACEMENT_3D('',#64197,#50701,#50702);
#45797=AXIS2_PLACEMENT_3D('',#64213,#50703,#50704);
#45798=AXIS2_PLACEMENT_3D('',#64215,#50705,#50706);
#45799=AXIS2_PLACEMENT_3D('',#64231,#50707,#50708);
#45800=AXIS2_PLACEMENT_3D('',#64233,#50709,#50710);
#45801=AXIS2_PLACEMENT_3D('',#64249,#50711,#50712);
#45802=AXIS2_PLACEMENT_3D('',#64251,#50713,#50714);
#45803=AXIS2_PLACEMENT_3D('',#64267,#50715,#50716);
#45804=AXIS2_PLACEMENT_3D('',#64269,#50717,#50718);
#45805=AXIS2_PLACEMENT_3D('',#64285,#50719,#50720);
#45806=AXIS2_PLACEMENT_3D('',#64287,#50721,#50722);
#45807=AXIS2_PLACEMENT_3D('',#64303,#50723,#50724);
#45808=AXIS2_PLACEMENT_3D('',#64305,#50725,#50726);
#45809=AXIS2_PLACEMENT_3D('',#64321,#50727,#50728);
#45810=AXIS2_PLACEMENT_3D('',#64323,#50729,#50730);
#45811=AXIS2_PLACEMENT_3D('',#64339,#50731,#50732);
#45812=AXIS2_PLACEMENT_3D('',#64341,#50733,#50734);
#45813=AXIS2_PLACEMENT_3D('',#64357,#50735,#50736);
#45814=AXIS2_PLACEMENT_3D('',#64359,#50737,#50738);
#45815=AXIS2_PLACEMENT_3D('',#64375,#50739,#50740);
#45816=AXIS2_PLACEMENT_3D('',#64377,#50741,#50742);
#45817=AXIS2_PLACEMENT_3D('',#64393,#50743,#50744);
#45818=AXIS2_PLACEMENT_3D('',#64395,#50745,#50746);
#45819=AXIS2_PLACEMENT_3D('',#64411,#50747,#50748);
#45820=AXIS2_PLACEMENT_3D('',#64413,#50749,#50750);
#45821=AXIS2_PLACEMENT_3D('',#64429,#50751,#50752);
#45822=AXIS2_PLACEMENT_3D('',#64431,#50753,#50754);
#45823=AXIS2_PLACEMENT_3D('',#64438,#50755,#50756);
#45824=AXIS2_PLACEMENT_3D('',#64447,#50758,#50759);
#45825=AXIS2_PLACEMENT_3D('',#64456,#50760,#50761);
#45826=AXIS2_PLACEMENT_3D('',#64458,#50762,#50763);
#45827=AXIS2_PLACEMENT_3D('',#64460,#50764,#50765);
#45828=AXIS2_PLACEMENT_3D('',#64462,#50766,#50767);
#45829=AXIS2_PLACEMENT_3D('',#64469,#50768,#50769);
#45830=AXIS2_PLACEMENT_3D('',#64471,#50770,#50771);
#45831=AXIS2_PLACEMENT_3D('',#64473,#50772,#50773);
#45832=AXIS2_PLACEMENT_3D('',#64475,#50774,#50775);
#45833=AXIS2_PLACEMENT_3D('',#64477,#50776,#50777);
#45834=AXIS2_PLACEMENT_3D('',#64484,#50778,#50779);
#45835=AXIS2_PLACEMENT_3D('',#64486,#50780,#50781);
#45836=AXIS2_PLACEMENT_3D('',#64488,#50782,#50783);
#45837=AXIS2_PLACEMENT_3D('',#64490,#50784,#50785);
#45838=AXIS2_PLACEMENT_3D('',#64492,#50786,#50787);
#45839=AXIS2_PLACEMENT_3D('',#64499,#50788,#50789);
#45840=AXIS2_PLACEMENT_3D('',#64501,#50790,#50791);
#45841=AXIS2_PLACEMENT_3D('',#64503,#50792,#50793);
#45842=AXIS2_PLACEMENT_3D('',#64505,#50794,#50795);
#45843=AXIS2_PLACEMENT_3D('',#64507,#50796,#50797);
#45844=AXIS2_PLACEMENT_3D('',#64514,#50798,#50799);
#45845=AXIS2_PLACEMENT_3D('',#64516,#50800,#50801);
#45846=AXIS2_PLACEMENT_3D('',#64518,#50802,#50803);
#45847=AXIS2_PLACEMENT_3D('',#64520,#50804,#50805);
#45848=AXIS2_PLACEMENT_3D('',#64522,#50806,#50807);
#45849=AXIS2_PLACEMENT_3D('',#64529,#50808,#50809);
#45850=AXIS2_PLACEMENT_3D('',#64531,#50810,#50811);
#45851=AXIS2_PLACEMENT_3D('',#64533,#50812,#50813);
#45852=AXIS2_PLACEMENT_3D('',#64535,#50814,#50815);
#45853=AXIS2_PLACEMENT_3D('',#64537,#50816,#50817);
#45854=AXIS2_PLACEMENT_3D('',#64544,#50818,#50819);
#45855=AXIS2_PLACEMENT_3D('',#64546,#50820,#50821);
#45856=AXIS2_PLACEMENT_3D('',#64548,#50822,#50823);
#45857=AXIS2_PLACEMENT_3D('',#64550,#50824,#50825);
#45858=AXIS2_PLACEMENT_3D('',#64552,#50826,#50827);
#45859=AXIS2_PLACEMENT_3D('',#64559,#50828,#50829);
#45860=AXIS2_PLACEMENT_3D('',#64561,#50830,#50831);
#45861=AXIS2_PLACEMENT_3D('',#64563,#50832,#50833);
#45862=AXIS2_PLACEMENT_3D('',#64565,#50834,#50835);
#45863=AXIS2_PLACEMENT_3D('',#64567,#50836,#50837);
#45864=AXIS2_PLACEMENT_3D('',#64574,#50838,#50839);
#45865=AXIS2_PLACEMENT_3D('',#64576,#50840,#50841);
#45866=AXIS2_PLACEMENT_3D('',#64578,#50842,#50843);
#45867=AXIS2_PLACEMENT_3D('',#64580,#50844,#50845);
#45868=AXIS2_PLACEMENT_3D('',#64582,#50846,#50847);
#45869=AXIS2_PLACEMENT_3D('',#64589,#50848,#50849);
#45870=AXIS2_PLACEMENT_3D('',#64591,#50850,#50851);
#45871=AXIS2_PLACEMENT_3D('',#64593,#50852,#50853);
#45872=AXIS2_PLACEMENT_3D('',#64595,#50854,#50855);
#45873=AXIS2_PLACEMENT_3D('',#64597,#50856,#50857);
#45874=AXIS2_PLACEMENT_3D('',#64604,#50858,#50859);
#45875=AXIS2_PLACEMENT_3D('',#64606,#50860,#50861);
#45876=AXIS2_PLACEMENT_3D('',#64608,#50862,#50863);
#45877=AXIS2_PLACEMENT_3D('',#64610,#50864,#50865);
#45878=AXIS2_PLACEMENT_3D('',#64612,#50866,#50867);
#45879=AXIS2_PLACEMENT_3D('',#64619,#50868,#50869);
#45880=AXIS2_PLACEMENT_3D('',#64621,#50870,#50871);
#45881=AXIS2_PLACEMENT_3D('',#64623,#50872,#50873);
#45882=AXIS2_PLACEMENT_3D('',#64625,#50874,#50875);
#45883=AXIS2_PLACEMENT_3D('',#64627,#50876,#50877);
#45884=AXIS2_PLACEMENT_3D('',#64634,#50878,#50879);
#45885=AXIS2_PLACEMENT_3D('',#64636,#50880,#50881);
#45886=AXIS2_PLACEMENT_3D('',#64638,#50882,#50883);
#45887=AXIS2_PLACEMENT_3D('',#64640,#50884,#50885);
#45888=AXIS2_PLACEMENT_3D('',#64642,#50886,#50887);
#45889=AXIS2_PLACEMENT_3D('',#64649,#50888,#50889);
#45890=AXIS2_PLACEMENT_3D('',#64651,#50890,#50891);
#45891=AXIS2_PLACEMENT_3D('',#64653,#50892,#50893);
#45892=AXIS2_PLACEMENT_3D('',#64655,#50894,#50895);
#45893=AXIS2_PLACEMENT_3D('',#64657,#50896,#50897);
#45894=AXIS2_PLACEMENT_3D('',#64664,#50898,#50899);
#45895=AXIS2_PLACEMENT_3D('',#64666,#50900,#50901);
#45896=AXIS2_PLACEMENT_3D('',#64668,#50902,#50903);
#45897=AXIS2_PLACEMENT_3D('',#64670,#50904,#50905);
#45898=AXIS2_PLACEMENT_3D('',#64672,#50906,#50907);
#45899=AXIS2_PLACEMENT_3D('',#64679,#50908,#50909);
#45900=AXIS2_PLACEMENT_3D('',#64681,#50910,#50911);
#45901=AXIS2_PLACEMENT_3D('',#64683,#50912,#50913);
#45902=AXIS2_PLACEMENT_3D('',#64685,#50914,#50915);
#45903=AXIS2_PLACEMENT_3D('',#64687,#50916,#50917);
#45904=AXIS2_PLACEMENT_3D('',#64694,#50918,#50919);
#45905=AXIS2_PLACEMENT_3D('',#64696,#50920,#50921);
#45906=AXIS2_PLACEMENT_3D('',#64698,#50922,#50923);
#45907=AXIS2_PLACEMENT_3D('',#64700,#50924,#50925);
#45908=AXIS2_PLACEMENT_3D('',#64702,#50926,#50927);
#45909=AXIS2_PLACEMENT_3D('',#64709,#50928,#50929);
#45910=AXIS2_PLACEMENT_3D('',#64711,#50930,#50931);
#45911=AXIS2_PLACEMENT_3D('',#64713,#50932,#50933);
#45912=AXIS2_PLACEMENT_3D('',#64715,#50934,#50935);
#45913=AXIS2_PLACEMENT_3D('',#64717,#50936,#50937);
#45914=AXIS2_PLACEMENT_3D('',#64724,#50938,#50939);
#45915=AXIS2_PLACEMENT_3D('',#64726,#50940,#50941);
#45916=AXIS2_PLACEMENT_3D('',#64728,#50942,#50943);
#45917=AXIS2_PLACEMENT_3D('',#64730,#50944,#50945);
#45918=AXIS2_PLACEMENT_3D('',#64732,#50946,#50947);
#45919=AXIS2_PLACEMENT_3D('',#64739,#50948,#50949);
#45920=AXIS2_PLACEMENT_3D('',#64741,#50950,#50951);
#45921=AXIS2_PLACEMENT_3D('',#64743,#50952,#50953);
#45922=AXIS2_PLACEMENT_3D('',#64745,#50954,#50955);
#45923=AXIS2_PLACEMENT_3D('',#64747,#50956,#50957);
#45924=AXIS2_PLACEMENT_3D('',#64754,#50958,#50959);
#45925=AXIS2_PLACEMENT_3D('',#64756,#50960,#50961);
#45926=AXIS2_PLACEMENT_3D('',#64758,#50962,#50963);
#45927=AXIS2_PLACEMENT_3D('',#64760,#50964,#50965);
#45928=AXIS2_PLACEMENT_3D('',#64762,#50966,#50967);
#45929=AXIS2_PLACEMENT_3D('',#64769,#50968,#50969);
#45930=AXIS2_PLACEMENT_3D('',#64771,#50970,#50971);
#45931=AXIS2_PLACEMENT_3D('',#64773,#50972,#50973);
#45932=AXIS2_PLACEMENT_3D('',#64775,#50974,#50975);
#45933=AXIS2_PLACEMENT_3D('',#64777,#50976,#50977);
#45934=AXIS2_PLACEMENT_3D('',#64784,#50978,#50979);
#45935=AXIS2_PLACEMENT_3D('',#64786,#50980,#50981);
#45936=AXIS2_PLACEMENT_3D('',#64788,#50982,#50983);
#45937=AXIS2_PLACEMENT_3D('',#64790,#50984,#50985);
#45938=AXIS2_PLACEMENT_3D('',#64792,#50986,#50987);
#45939=AXIS2_PLACEMENT_3D('',#64799,#50988,#50989);
#45940=AXIS2_PLACEMENT_3D('',#64801,#50990,#50991);
#45941=AXIS2_PLACEMENT_3D('',#64803,#50992,#50993);
#45942=AXIS2_PLACEMENT_3D('',#64805,#50994,#50995);
#45943=AXIS2_PLACEMENT_3D('',#64807,#50996,#50997);
#45944=AXIS2_PLACEMENT_3D('',#64814,#50998,#50999);
#45945=AXIS2_PLACEMENT_3D('',#64816,#51000,#51001);
#45946=AXIS2_PLACEMENT_3D('',#64818,#51002,#51003);
#45947=AXIS2_PLACEMENT_3D('',#64820,#51004,#51005);
#45948=AXIS2_PLACEMENT_3D('',#64822,#51006,#51007);
#45949=AXIS2_PLACEMENT_3D('',#64829,#51008,#51009);
#45950=AXIS2_PLACEMENT_3D('',#64831,#51010,#51011);
#45951=AXIS2_PLACEMENT_3D('',#64833,#51012,#51013);
#45952=AXIS2_PLACEMENT_3D('',#64835,#51014,#51015);
#45953=AXIS2_PLACEMENT_3D('',#64837,#51016,#51017);
#45954=AXIS2_PLACEMENT_3D('',#64844,#51018,#51019);
#45955=AXIS2_PLACEMENT_3D('',#64846,#51020,#51021);
#45956=AXIS2_PLACEMENT_3D('',#64848,#51022,#51023);
#45957=AXIS2_PLACEMENT_3D('',#64850,#51024,#51025);
#45958=AXIS2_PLACEMENT_3D('',#64852,#51026,#51027);
#45959=AXIS2_PLACEMENT_3D('',#64859,#51028,#51029);
#45960=AXIS2_PLACEMENT_3D('',#64861,#51030,#51031);
#45961=AXIS2_PLACEMENT_3D('',#64863,#51032,#51033);
#45962=AXIS2_PLACEMENT_3D('',#64865,#51034,#51035);
#45963=AXIS2_PLACEMENT_3D('',#64867,#51036,#51037);
#45964=AXIS2_PLACEMENT_3D('',#64874,#51038,#51039);
#45965=AXIS2_PLACEMENT_3D('',#64876,#51040,#51041);
#45966=AXIS2_PLACEMENT_3D('',#64878,#51042,#51043);
#45967=AXIS2_PLACEMENT_3D('',#64880,#51044,#51045);
#45968=AXIS2_PLACEMENT_3D('',#64882,#51046,#51047);
#45969=AXIS2_PLACEMENT_3D('',#64889,#51048,#51049);
#45970=AXIS2_PLACEMENT_3D('',#64891,#51050,#51051);
#45971=AXIS2_PLACEMENT_3D('',#64893,#51052,#51053);
#45972=AXIS2_PLACEMENT_3D('',#64895,#51054,#51055);
#45973=AXIS2_PLACEMENT_3D('',#64897,#51056,#51057);
#45974=AXIS2_PLACEMENT_3D('',#64904,#51058,#51059);
#45975=AXIS2_PLACEMENT_3D('',#64906,#51060,#51061);
#45976=AXIS2_PLACEMENT_3D('',#64908,#51062,#51063);
#45977=AXIS2_PLACEMENT_3D('',#64910,#51064,#51065);
#45978=AXIS2_PLACEMENT_3D('',#64912,#51066,#51067);
#45979=AXIS2_PLACEMENT_3D('',#64919,#51068,#51069);
#45980=AXIS2_PLACEMENT_3D('',#64921,#51070,#51071);
#45981=AXIS2_PLACEMENT_3D('',#64923,#51072,#51073);
#45982=AXIS2_PLACEMENT_3D('',#64925,#51074,#51075);
#45983=AXIS2_PLACEMENT_3D('',#64927,#51076,#51077);
#45984=AXIS2_PLACEMENT_3D('',#64934,#51078,#51079);
#45985=AXIS2_PLACEMENT_3D('',#64936,#51080,#51081);
#45986=AXIS2_PLACEMENT_3D('',#64938,#51082,#51083);
#45987=AXIS2_PLACEMENT_3D('',#64940,#51084,#51085);
#45988=AXIS2_PLACEMENT_3D('',#64942,#51086,#51087);
#45989=AXIS2_PLACEMENT_3D('',#64949,#51088,#51089);
#45990=AXIS2_PLACEMENT_3D('',#64951,#51090,#51091);
#45991=AXIS2_PLACEMENT_3D('',#64953,#51092,#51093);
#45992=AXIS2_PLACEMENT_3D('',#64955,#51094,#51095);
#45993=AXIS2_PLACEMENT_3D('',#64957,#51096,#51097);
#45994=AXIS2_PLACEMENT_3D('',#64964,#51098,#51099);
#45995=AXIS2_PLACEMENT_3D('',#64966,#51100,#51101);
#45996=AXIS2_PLACEMENT_3D('',#64968,#51102,#51103);
#45997=AXIS2_PLACEMENT_3D('',#64970,#51104,#51105);
#45998=AXIS2_PLACEMENT_3D('',#64972,#51106,#51107);
#45999=AXIS2_PLACEMENT_3D('',#64979,#51108,#51109);
#46000=AXIS2_PLACEMENT_3D('',#64981,#51110,#51111);
#46001=AXIS2_PLACEMENT_3D('',#64983,#51112,#51113);
#46002=AXIS2_PLACEMENT_3D('',#64985,#51114,#51115);
#46003=AXIS2_PLACEMENT_3D('',#64987,#51116,#51117);
#46004=AXIS2_PLACEMENT_3D('',#64994,#51118,#51119);
#46005=AXIS2_PLACEMENT_3D('',#64996,#51120,#51121);
#46006=AXIS2_PLACEMENT_3D('',#64998,#51122,#51123);
#46007=AXIS2_PLACEMENT_3D('',#65000,#51124,#51125);
#46008=AXIS2_PLACEMENT_3D('',#65002,#51126,#51127);
#46009=AXIS2_PLACEMENT_3D('',#65009,#51128,#51129);
#46010=AXIS2_PLACEMENT_3D('',#65011,#51130,#51131);
#46011=AXIS2_PLACEMENT_3D('',#65013,#51132,#51133);
#46012=AXIS2_PLACEMENT_3D('',#65015,#51134,#51135);
#46013=AXIS2_PLACEMENT_3D('',#65017,#51136,#51137);
#46014=AXIS2_PLACEMENT_3D('',#65024,#51138,#51139);
#46015=AXIS2_PLACEMENT_3D('',#65026,#51140,#51141);
#46016=AXIS2_PLACEMENT_3D('',#65028,#51142,#51143);
#46017=AXIS2_PLACEMENT_3D('',#65030,#51144,#51145);
#46018=AXIS2_PLACEMENT_3D('',#65032,#51146,#51147);
#46019=AXIS2_PLACEMENT_3D('',#65039,#51148,#51149);
#46020=AXIS2_PLACEMENT_3D('',#65041,#51150,#51151);
#46021=AXIS2_PLACEMENT_3D('',#65043,#51152,#51153);
#46022=AXIS2_PLACEMENT_3D('',#65045,#51154,#51155);
#46023=AXIS2_PLACEMENT_3D('',#65047,#51156,#51157);
#46024=AXIS2_PLACEMENT_3D('',#65054,#51158,#51159);
#46025=AXIS2_PLACEMENT_3D('',#65056,#51160,#51161);
#46026=AXIS2_PLACEMENT_3D('',#65058,#51162,#51163);
#46027=AXIS2_PLACEMENT_3D('',#65060,#51164,#51165);
#46028=AXIS2_PLACEMENT_3D('',#65062,#51166,#51167);
#46029=AXIS2_PLACEMENT_3D('',#65069,#51168,#51169);
#46030=AXIS2_PLACEMENT_3D('',#65071,#51170,#51171);
#46031=AXIS2_PLACEMENT_3D('',#65073,#51172,#51173);
#46032=AXIS2_PLACEMENT_3D('',#65075,#51174,#51175);
#46033=AXIS2_PLACEMENT_3D('',#65077,#51176,#51177);
#46034=AXIS2_PLACEMENT_3D('',#65084,#51178,#51179);
#46035=AXIS2_PLACEMENT_3D('',#65086,#51180,#51181);
#46036=AXIS2_PLACEMENT_3D('',#65088,#51182,#51183);
#46037=AXIS2_PLACEMENT_3D('',#65090,#51184,#51185);
#46038=AXIS2_PLACEMENT_3D('',#65092,#51186,#51187);
#46039=AXIS2_PLACEMENT_3D('',#65099,#51188,#51189);
#46040=AXIS2_PLACEMENT_3D('',#65101,#51190,#51191);
#46041=AXIS2_PLACEMENT_3D('',#65103,#51192,#51193);
#46042=AXIS2_PLACEMENT_3D('',#65105,#51194,#51195);
#46043=AXIS2_PLACEMENT_3D('',#65107,#51196,#51197);
#46044=AXIS2_PLACEMENT_3D('',#65114,#51198,#51199);
#46045=AXIS2_PLACEMENT_3D('',#65116,#51200,#51201);
#46046=AXIS2_PLACEMENT_3D('',#65118,#51202,#51203);
#46047=AXIS2_PLACEMENT_3D('',#65120,#51204,#51205);
#46048=AXIS2_PLACEMENT_3D('',#65122,#51206,#51207);
#46049=AXIS2_PLACEMENT_3D('',#65129,#51208,#51209);
#46050=AXIS2_PLACEMENT_3D('',#65131,#51210,#51211);
#46051=AXIS2_PLACEMENT_3D('',#65133,#51212,#51213);
#46052=AXIS2_PLACEMENT_3D('',#65135,#51214,#51215);
#46053=AXIS2_PLACEMENT_3D('',#65137,#51216,#51217);
#46054=AXIS2_PLACEMENT_3D('',#65144,#51218,#51219);
#46055=AXIS2_PLACEMENT_3D('',#65146,#51220,#51221);
#46056=AXIS2_PLACEMENT_3D('',#65148,#51222,#51223);
#46057=AXIS2_PLACEMENT_3D('',#65150,#51224,#51225);
#46058=AXIS2_PLACEMENT_3D('',#65152,#51226,#51227);
#46059=AXIS2_PLACEMENT_3D('',#65159,#51228,#51229);
#46060=AXIS2_PLACEMENT_3D('',#65161,#51230,#51231);
#46061=AXIS2_PLACEMENT_3D('',#65163,#51232,#51233);
#46062=AXIS2_PLACEMENT_3D('',#65165,#51234,#51235);
#46063=AXIS2_PLACEMENT_3D('',#65167,#51236,#51237);
#46064=AXIS2_PLACEMENT_3D('',#65174,#51238,#51239);
#46065=AXIS2_PLACEMENT_3D('',#65176,#51240,#51241);
#46066=AXIS2_PLACEMENT_3D('',#65178,#51242,#51243);
#46067=AXIS2_PLACEMENT_3D('',#65180,#51244,#51245);
#46068=AXIS2_PLACEMENT_3D('',#65182,#51246,#51247);
#46069=AXIS2_PLACEMENT_3D('',#65189,#51248,#51249);
#46070=AXIS2_PLACEMENT_3D('',#65191,#51250,#51251);
#46071=AXIS2_PLACEMENT_3D('',#65193,#51252,#51253);
#46072=AXIS2_PLACEMENT_3D('',#65195,#51254,#51255);
#46073=AXIS2_PLACEMENT_3D('',#65197,#51256,#51257);
#46074=AXIS2_PLACEMENT_3D('',#65220,#51258,#51259);
#46075=AXIS2_PLACEMENT_3D('',#65221,#51260,#51261);
#46076=AXIS2_PLACEMENT_3D('',#65231,#51262,#51263);
#46077=AXIS2_PLACEMENT_3D('',#65251,#51265,#51266);
#46078=AXIS2_PLACEMENT_3D('',#65267,#51268,#51269);
#46079=AXIS2_PLACEMENT_3D('',#65269,#51270,#51271);
#46080=AXIS2_PLACEMENT_3D('',#65273,#51273,#51274);
#46081=AXIS2_PLACEMENT_3D('',#65275,#51275,#51276);
#46082=AXIS2_PLACEMENT_3D('',#65294,#51278,#51279);
#46083=AXIS2_PLACEMENT_3D('',#65298,#51281,#51282);
#46084=AXIS2_PLACEMENT_3D('',#65299,#51283,#51284);
#46085=AXIS2_PLACEMENT_3D('',#65318,#51285,#51286);
#46086=AXIS2_PLACEMENT_3D('',#65345,#51289,#51290);
#46087=AXIS2_PLACEMENT_3D('',#65352,#51291,#51292);
#46088=AXIS2_PLACEMENT_3D('',#65355,#51293,#51294);
#46089=AXIS2_PLACEMENT_3D('',#65356,#51295,#51296);
#46090=AXIS2_PLACEMENT_3D('',#65357,#51297,#51298);
#46091=AXIS2_PLACEMENT_3D('',#65381,#51300,#51301);
#46092=AXIS2_PLACEMENT_3D('',#65382,#51302,#51303);
#46093=AXIS2_PLACEMENT_3D('',#65383,#51304,#51305);
#46094=AXIS2_PLACEMENT_3D('',#65386,#51306,#51307);
#46095=AXIS2_PLACEMENT_3D('',#65387,#51308,#51309);
#46096=AXIS2_PLACEMENT_3D('',#65388,#51310,#51311);
#46097=AXIS2_PLACEMENT_3D('',#65389,#51312,#51313);
#46098=AXIS2_PLACEMENT_3D('',#65391,#51314,#51315);
#46099=AXIS2_PLACEMENT_3D('',#65393,#51316,#51317);
#46100=AXIS2_PLACEMENT_3D('',#65394,#51318,#51319);
#46101=AXIS2_PLACEMENT_3D('',#65406,#51320,#51321);
#46102=AXIS2_PLACEMENT_3D('',#65408,#51322,#51323);
#46103=AXIS2_PLACEMENT_3D('',#65412,#51325,#51326);
#46104=AXIS2_PLACEMENT_3D('',#65414,#51327,#51328);
#46105=AXIS2_PLACEMENT_3D('',#65427,#51330,#51331);
#46106=AXIS2_PLACEMENT_3D('',#65428,#51332,#51333);
#46107=AXIS2_PLACEMENT_3D('',#65432,#51335,#51336);
#46108=AXIS2_PLACEMENT_3D('',#65434,#51337,#51338);
#46109=AXIS2_PLACEMENT_3D('',#65493,#51342,#51343);
#46110=AXIS2_PLACEMENT_3D('',#65513,#51346,#51347);
#46111=AXIS2_PLACEMENT_3D('',#65520,#51348,#51349);
#46112=AXIS2_PLACEMENT_3D('',#65523,#51350,#51351);
#46113=AXIS2_PLACEMENT_3D('',#65524,#51352,#51353);
#46114=AXIS2_PLACEMENT_3D('',#65525,#51354,#51355);
#46115=AXIS2_PLACEMENT_3D('',#65526,#51356,#51357);
#46116=AXIS2_PLACEMENT_3D('',#65528,#51358,#51359);
#46117=AXIS2_PLACEMENT_3D('',#65530,#51360,#51361);
#46118=AXIS2_PLACEMENT_3D('',#65531,#51362,#51363);
#46119=AXIS2_PLACEMENT_3D('',#65568,#51365,#51366);
#46120=AXIS2_PLACEMENT_3D('',#65570,#51367,#51368);
#46121=AXIS2_PLACEMENT_3D('',#65580,#51370,#51371);
#46122=AXIS2_PLACEMENT_3D('',#65581,#51372,#51373);
#46123=AXIS2_PLACEMENT_3D('',#65585,#51375,#51376);
#46124=AXIS2_PLACEMENT_3D('',#65587,#51377,#51378);
#46125=AXIS2_PLACEMENT_3D('',#65677,#51384,#51385);
#46126=AXIS2_PLACEMENT_3D('',#65684,#51386,#51387);
#46127=AXIS2_PLACEMENT_3D('',#65687,#51388,#51389);
#46128=AXIS2_PLACEMENT_3D('',#65694,#51390,#51391);
#46129=AXIS2_PLACEMENT_3D('',#65695,#51392,#51393);
#46130=AXIS2_PLACEMENT_3D('',#65697,#51394,#51395);
#46131=AXIS2_PLACEMENT_3D('',#65699,#51396,#51397);
#46132=AXIS2_PLACEMENT_3D('',#65700,#51398,#51399);
#46133=AXIS2_PLACEMENT_3D('',#65709,#51400,#51401);
#46134=AXIS2_PLACEMENT_3D('',#65711,#51402,#51403);
#46135=AXIS2_PLACEMENT_3D('',#65715,#51405,#51406);
#46136=AXIS2_PLACEMENT_3D('',#65717,#51407,#51408);
#46137=AXIS2_PLACEMENT_3D('',#65736,#51410,#51411);
#46138=AXIS2_PLACEMENT_3D('',#65737,#51412,#51413);
#46139=AXIS2_PLACEMENT_3D('',#65822,#51418,#51419);
#46140=AXIS2_PLACEMENT_3D('',#65855,#51422,#51423);
#46141=AXIS2_PLACEMENT_3D('',#65858,#51424,#51425);
#46142=AXIS2_PLACEMENT_3D('',#65859,#51426,#51427);
#46143=AXIS2_PLACEMENT_3D('',#65860,#51428,#51429);
#46144=AXIS2_PLACEMENT_3D('',#65861,#51430,#51431);
#46145=AXIS2_PLACEMENT_3D('',#65863,#51432,#51433);
#46146=AXIS2_PLACEMENT_3D('',#65865,#51434,#51435);
#46147=AXIS2_PLACEMENT_3D('',#65890,#51436,#51437);
#46148=AXIS2_PLACEMENT_3D('',#65892,#51438,#51439);
#46149=AXIS2_PLACEMENT_3D('',#65896,#51441,#51442);
#46150=AXIS2_PLACEMENT_3D('',#65898,#51443,#51444);
#46151=AXIS2_PLACEMENT_3D('',#65911,#51446,#51447);
#46152=AXIS2_PLACEMENT_3D('',#65912,#51448,#51449);
#46153=AXIS2_PLACEMENT_3D('',#65916,#51451,#51452);
#46154=AXIS2_PLACEMENT_3D('',#65918,#51453,#51454);
#46155=AXIS2_PLACEMENT_3D('',#65984,#51458,#51459);
#46156=AXIS2_PLACEMENT_3D('',#66011,#51462,#51463);
#46157=AXIS2_PLACEMENT_3D('',#66018,#51464,#51465);
#46158=AXIS2_PLACEMENT_3D('',#66021,#51466,#51467);
#46159=AXIS2_PLACEMENT_3D('',#66022,#51468,#51469);
#46160=AXIS2_PLACEMENT_3D('',#66023,#51470,#51471);
#46161=AXIS2_PLACEMENT_3D('',#66024,#51472,#51473);
#46162=AXIS2_PLACEMENT_3D('',#66026,#51474,#51475);
#46163=AXIS2_PLACEMENT_3D('',#66028,#51476,#51477);
#46164=AXIS2_PLACEMENT_3D('',#66029,#51478,#51479);
#46165=AXIS2_PLACEMENT_3D('',#66041,#51480,#51481);
#46166=AXIS2_PLACEMENT_3D('',#66043,#51482,#51483);
#46167=AXIS2_PLACEMENT_3D('',#66047,#51485,#51486);
#46168=AXIS2_PLACEMENT_3D('',#66049,#51487,#51488);
#46169=AXIS2_PLACEMENT_3D('',#66069,#51490,#51491);
#46170=AXIS2_PLACEMENT_3D('',#66070,#51492,#51493);
#46171=AXIS2_PLACEMENT_3D('',#66074,#51495,#51496);
#46172=AXIS2_PLACEMENT_3D('',#66076,#51497,#51498);
#46173=AXIS2_PLACEMENT_3D('',#66140,#51502,#51503);
#46174=AXIS2_PLACEMENT_3D('',#66161,#51506,#51507);
#46175=AXIS2_PLACEMENT_3D('',#66168,#51508,#51509);
#46176=AXIS2_PLACEMENT_3D('',#66170,#51510,#51511);
#46177=AXIS2_PLACEMENT_3D('',#66172,#51512,#51513);
#46178=AXIS2_PLACEMENT_3D('',#66173,#51514,#51515);
#46179=AXIS2_PLACEMENT_3D('',#66174,#51516,#51517);
#46180=AXIS2_PLACEMENT_3D('',#66176,#51518,#51519);
#46181=AXIS2_PLACEMENT_3D('',#66179,#51521,#51522);
#46182=AXIS2_PLACEMENT_3D('',#66191,#51523,#51524);
#46183=AXIS2_PLACEMENT_3D('',#66192,#51525,#51526);
#46184=AXIS2_PLACEMENT_3D('',#66196,#51528,#51529);
#46185=AXIS2_PLACEMENT_3D('',#66198,#51530,#51531);
#46186=AXIS2_PLACEMENT_3D('',#66200,#51533,#51534);
#46187=AXIS2_PLACEMENT_3D('',#66201,#51535,#51536);
#46188=AXIS2_PLACEMENT_3D('',#66242,#51539,#51540);
#46189=AXIS2_PLACEMENT_3D('',#66261,#51541,#51542);
#46190=AXIS2_PLACEMENT_3D('',#66262,#51543,#51544);
#46191=AXIS2_PLACEMENT_3D('',#66272,#51545,#51546);
#46192=AXIS2_PLACEMENT_3D('',#66292,#51548,#51549);
#46193=AXIS2_PLACEMENT_3D('',#66300,#51551,#51552);
#46194=AXIS2_PLACEMENT_3D('',#66303,#51553,#51554);
#46195=AXIS2_PLACEMENT_3D('',#66304,#51555,#51556);
#46196=AXIS2_PLACEMENT_3D('',#66305,#51557,#51558);
#46197=AXIS2_PLACEMENT_3D('',#66314,#51559,#51560);
#46198=AXIS2_PLACEMENT_3D('',#66315,#51561,#51562);
#46199=AXIS2_PLACEMENT_3D('',#66319,#51564,#51565);
#46200=AXIS2_PLACEMENT_3D('',#66321,#51566,#51567);
#46201=AXIS2_PLACEMENT_3D('',#66346,#51570,#51571);
#46202=AXIS2_PLACEMENT_3D('',#66347,#51572,#51573);
#46203=AXIS2_PLACEMENT_3D('',#66366,#51574,#51575);
#46204=AXIS2_PLACEMENT_3D('',#66385,#51577,#51578);
#46205=AXIS2_PLACEMENT_3D('',#66386,#51579,#51580);
#46206=AXIS2_PLACEMENT_3D('',#66390,#51582,#51583);
#46207=AXIS2_PLACEMENT_3D('',#66392,#51584,#51585);
#46208=AXIS2_PLACEMENT_3D('',#66405,#51587,#51588);
#46209=AXIS2_PLACEMENT_3D('',#66413,#51590,#51591);
#46210=AXIS2_PLACEMENT_3D('',#66416,#51592,#51593);
#46211=AXIS2_PLACEMENT_3D('',#66417,#51594,#51595);
#46212=AXIS2_PLACEMENT_3D('',#66418,#51596,#51597);
#46213=AXIS2_PLACEMENT_3D('',#66442,#51599,#51600);
#46214=AXIS2_PLACEMENT_3D('',#66445,#51601,#51602);
#46215=AXIS2_PLACEMENT_3D('',#66446,#51603,#51604);
#46216=AXIS2_PLACEMENT_3D('',#66447,#51605,#51606);
#46217=AXIS2_PLACEMENT_3D('',#66483,#51608,#51609);
#46218=AXIS2_PLACEMENT_3D('',#66485,#51610,#51611);
#46219=AXIS2_PLACEMENT_3D('',#66540,#51615,#51616);
#46220=AXIS2_PLACEMENT_3D('',#66543,#51617,#51618);
#46221=AXIS2_PLACEMENT_3D('',#66550,#51619,#51620);
#46222=AXIS2_PLACEMENT_3D('',#66559,#51621,#51622);
#46223=AXIS2_PLACEMENT_3D('',#66560,#51623,#51624);
#46224=AXIS2_PLACEMENT_3D('',#66564,#51626,#51627);
#46225=AXIS2_PLACEMENT_3D('',#66566,#51628,#51629);
#46226=AXIS2_PLACEMENT_3D('',#66602,#51632,#51633);
#46227=AXIS2_PLACEMENT_3D('',#66610,#51635,#51636);
#46228=AXIS2_PLACEMENT_3D('',#66613,#51637,#51638);
#46229=AXIS2_PLACEMENT_3D('',#66614,#51639,#51640);
#46230=AXIS2_PLACEMENT_3D('',#66615,#51641,#51642);
#46231=AXIS2_PLACEMENT_3D('',#66634,#51643,#51644);
#46232=AXIS2_PLACEMENT_3D('',#66635,#51645,#51646);
#46233=AXIS2_PLACEMENT_3D('',#66639,#51648,#51649);
#46234=AXIS2_PLACEMENT_3D('',#66641,#51650,#51651);
#46235=AXIS2_PLACEMENT_3D('',#66684,#51654,#51655);
#46236=AXIS2_PLACEMENT_3D('',#66692,#51657,#51658);
#46237=AXIS2_PLACEMENT_3D('',#66695,#51659,#51660);
#46238=AXIS2_PLACEMENT_3D('',#66696,#51661,#51662);
#46239=AXIS2_PLACEMENT_3D('',#66697,#51663,#51664);
#46240=AXIS2_PLACEMENT_3D('',#66712,#51665,#51666);
#46241=AXIS2_PLACEMENT_3D('',#66713,#51667,#51668);
#46242=AXIS2_PLACEMENT_3D('',#66717,#51670,#51671);
#46243=AXIS2_PLACEMENT_3D('',#66719,#51672,#51673);
#46244=AXIS2_PLACEMENT_3D('',#66760,#51676,#51677);
#46245=AXIS2_PLACEMENT_3D('',#66762,#51679,#51680);
#46246=AXIS2_PLACEMENT_3D('',#66763,#51681,#51682);
#46247=AXIS2_PLACEMENT_3D('',#66766,#51684,#51685);
#46248=AXIS2_PLACEMENT_3D('',#66767,#51686,#51687);
#46249=AXIS2_PLACEMENT_3D('',#66768,#51688,#51689);
#46250=AXIS2_PLACEMENT_3D('',#66787,#51690,#51691);
#46251=AXIS2_PLACEMENT_3D('',#66788,#51692,#51693);
#46252=AXIS2_PLACEMENT_3D('',#66798,#51694,#51695);
#46253=AXIS2_PLACEMENT_3D('',#66818,#51697,#51698);
#46254=AXIS2_PLACEMENT_3D('',#66826,#51700,#51701);
#46255=AXIS2_PLACEMENT_3D('',#66829,#51702,#51703);
#46256=AXIS2_PLACEMENT_3D('',#66830,#51704,#51705);
#46257=AXIS2_PLACEMENT_3D('',#66831,#51706,#51707);
#46258=AXIS2_PLACEMENT_3D('',#66840,#51708,#51709);
#46259=AXIS2_PLACEMENT_3D('',#66841,#51710,#51711);
#46260=AXIS2_PLACEMENT_3D('',#66845,#51713,#51714);
#46261=AXIS2_PLACEMENT_3D('',#66847,#51715,#51716);
#46262=AXIS2_PLACEMENT_3D('',#66872,#51719,#51720);
#46263=AXIS2_PLACEMENT_3D('',#66873,#51721,#51722);
#46264=AXIS2_PLACEMENT_3D('',#66892,#51723,#51724);
#46265=AXIS2_PLACEMENT_3D('',#66900,#51726,#51727);
#46266=AXIS2_PLACEMENT_3D('',#66903,#51728,#51729);
#46267=AXIS2_PLACEMENT_3D('',#66904,#51730,#51731);
#46268=AXIS2_PLACEMENT_3D('',#66905,#51732,#51733);
#46269=AXIS2_PLACEMENT_3D('',#66917,#51734,#51735);
#46270=AXIS2_PLACEMENT_3D('',#66918,#51736,#51737);
#46271=AXIS2_PLACEMENT_3D('',#66922,#51739,#51740);
#46272=AXIS2_PLACEMENT_3D('',#66924,#51741,#51742);
#46273=AXIS2_PLACEMENT_3D('',#66960,#51745,#51746);
#46274=AXIS2_PLACEMENT_3D('',#67003,#51749,#51750);
#46275=AXIS2_PLACEMENT_3D('',#67005,#51751,#51752);
#46276=AXIS2_PLACEMENT_3D('',#67037,#51755,#51756);
#46277=AXIS2_PLACEMENT_3D('',#67040,#51757,#51758);
#46278=AXIS2_PLACEMENT_3D('',#67041,#51759,#51760);
#46279=AXIS2_PLACEMENT_3D('',#67042,#51761,#51762);
#46280=AXIS2_PLACEMENT_3D('',#67066,#51764,#51765);
#46281=AXIS2_PLACEMENT_3D('',#67069,#51766,#51767);
#46282=AXIS2_PLACEMENT_3D('',#67076,#51768,#51769);
#46283=AXIS2_PLACEMENT_3D('',#67088,#51770,#51771);
#46284=AXIS2_PLACEMENT_3D('',#67089,#51772,#51773);
#46285=AXIS2_PLACEMENT_3D('',#67093,#51775,#51776);
#46286=AXIS2_PLACEMENT_3D('',#67095,#51777,#51778);
#46287=AXIS2_PLACEMENT_3D('',#67131,#51781,#51782);
#46288=AXIS2_PLACEMENT_3D('',#67139,#51784,#51785);
#46289=AXIS2_PLACEMENT_3D('',#67142,#51786,#51787);
#46290=AXIS2_PLACEMENT_3D('',#67143,#51788,#51789);
#46291=AXIS2_PLACEMENT_3D('',#67144,#51790,#51791);
#46292=AXIS2_PLACEMENT_3D('',#67163,#51792,#51793);
#46293=AXIS2_PLACEMENT_3D('',#67164,#51794,#51795);
#46294=AXIS2_PLACEMENT_3D('',#67168,#51797,#51798);
#46295=AXIS2_PLACEMENT_3D('',#67170,#51799,#51800);
#46296=AXIS2_PLACEMENT_3D('',#67206,#51803,#51804);
#46297=AXIS2_PLACEMENT_3D('',#67214,#51806,#51807);
#46298=AXIS2_PLACEMENT_3D('',#67217,#51808,#51809);
#46299=AXIS2_PLACEMENT_3D('',#67218,#51810,#51811);
#46300=AXIS2_PLACEMENT_3D('',#67219,#51812,#51813);
#46301=AXIS2_PLACEMENT_3D('',#67234,#51814,#51815);
#46302=AXIS2_PLACEMENT_3D('',#67235,#51816,#51817);
#46303=AXIS2_PLACEMENT_3D('',#67239,#51819,#51820);
#46304=AXIS2_PLACEMENT_3D('',#67241,#51821,#51822);
#46305=AXIS2_PLACEMENT_3D('',#67282,#51825,#51826);
#46306=AXIS2_PLACEMENT_3D('',#67284,#51828,#51829);
#46307=AXIS2_PLACEMENT_3D('',#67285,#51830,#51831);
#46308=AXIS2_PLACEMENT_3D('',#67288,#51833,#51834);
#46309=AXIS2_PLACEMENT_3D('',#67289,#51835,#51836);
#46310=AXIS2_PLACEMENT_3D('',#67290,#51837,#51838);
#46311=AXIS2_PLACEMENT_3D('',#67309,#51839,#51840);
#46312=AXIS2_PLACEMENT_3D('',#67310,#51841,#51842);
#46313=AXIS2_PLACEMENT_3D('',#67320,#51843,#51844);
#46314=AXIS2_PLACEMENT_3D('',#67340,#51846,#51847);
#46315=AXIS2_PLACEMENT_3D('',#67348,#51849,#51850);
#46316=AXIS2_PLACEMENT_3D('',#67351,#51851,#51852);
#46317=AXIS2_PLACEMENT_3D('',#67352,#51853,#51854);
#46318=AXIS2_PLACEMENT_3D('',#67353,#51855,#51856);
#46319=AXIS2_PLACEMENT_3D('',#67362,#51857,#51858);
#46320=AXIS2_PLACEMENT_3D('',#67363,#51859,#51860);
#46321=AXIS2_PLACEMENT_3D('',#67367,#51862,#51863);
#46322=AXIS2_PLACEMENT_3D('',#67369,#51864,#51865);
#46323=AXIS2_PLACEMENT_3D('',#67394,#51868,#51869);
#46324=AXIS2_PLACEMENT_3D('',#67395,#51870,#51871);
#46325=AXIS2_PLACEMENT_3D('',#67414,#51872,#51873);
#46326=AXIS2_PLACEMENT_3D('',#67422,#51875,#51876);
#46327=AXIS2_PLACEMENT_3D('',#67425,#51877,#51878);
#46328=AXIS2_PLACEMENT_3D('',#67426,#51879,#51880);
#46329=AXIS2_PLACEMENT_3D('',#67427,#51881,#51882);
#46330=AXIS2_PLACEMENT_3D('',#67439,#51883,#51884);
#46331=AXIS2_PLACEMENT_3D('',#67440,#51885,#51886);
#46332=AXIS2_PLACEMENT_3D('',#67444,#51888,#51889);
#46333=AXIS2_PLACEMENT_3D('',#67446,#51890,#51891);
#46334=AXIS2_PLACEMENT_3D('',#67482,#51894,#51895);
#46335=AXIS2_PLACEMENT_3D('',#67490,#51897,#51898);
#46336=AXIS2_PLACEMENT_3D('',#67493,#51899,#51900);
#46337=AXIS2_PLACEMENT_3D('',#67494,#51901,#51902);
#46338=AXIS2_PLACEMENT_3D('',#67495,#51903,#51904);
#46339=AXIS2_PLACEMENT_3D('',#67531,#51906,#51907);
#46340=AXIS2_PLACEMENT_3D('',#67533,#51908,#51909);
#46341=AXIS2_PLACEMENT_3D('',#67599,#51913,#51914);
#46342=AXIS2_PLACEMENT_3D('',#67600,#51915,#51916);
#46343=AXIS2_PLACEMENT_3D('',#67604,#51918,#51919);
#46344=AXIS2_PLACEMENT_3D('',#67606,#51920,#51921);
#46345=AXIS2_PLACEMENT_3D('',#67619,#51923,#51924);
#46346=AXIS2_PLACEMENT_3D('',#67627,#51926,#51927);
#46347=AXIS2_PLACEMENT_3D('',#67630,#51928,#51929);
#46348=AXIS2_PLACEMENT_3D('',#67637,#51930,#51931);
#46349=AXIS2_PLACEMENT_3D('',#67661,#51933,#51934);
#46350=AXIS2_PLACEMENT_3D('',#67664,#51935,#51936);
#46351=AXIS2_PLACEMENT_3D('',#67665,#51937,#51938);
#46352=AXIS2_PLACEMENT_3D('',#67666,#51939,#51940);
#46353=AXIS2_PLACEMENT_3D('',#67685,#51941,#51942);
#46354=AXIS2_PLACEMENT_3D('',#67686,#51943,#51944);
#46355=AXIS2_PLACEMENT_3D('',#67690,#51946,#51947);
#46356=AXIS2_PLACEMENT_3D('',#67692,#51948,#51949);
#46357=AXIS2_PLACEMENT_3D('',#67728,#51952,#51953);
#46358=AXIS2_PLACEMENT_3D('',#67736,#51955,#51956);
#46359=AXIS2_PLACEMENT_3D('',#67739,#51957,#51958);
#46360=AXIS2_PLACEMENT_3D('',#67740,#51959,#51960);
#46361=AXIS2_PLACEMENT_3D('',#67741,#51961,#51962);
#46362=AXIS2_PLACEMENT_3D('',#67753,#51963,#51964);
#46363=AXIS2_PLACEMENT_3D('',#67754,#51965,#51966);
#46364=AXIS2_PLACEMENT_3D('',#67758,#51968,#51969);
#46365=AXIS2_PLACEMENT_3D('',#67760,#51970,#51971);
#46366=AXIS2_PLACEMENT_3D('',#67794,#51974,#51975);
#46367=AXIS2_PLACEMENT_3D('',#67796,#51977,#51978);
#46368=AXIS2_PLACEMENT_3D('',#67797,#51979,#51980);
#46369=AXIS2_PLACEMENT_3D('',#67800,#51982,#51983);
#46370=AXIS2_PLACEMENT_3D('',#67801,#51984,#51985);
#46371=AXIS2_PLACEMENT_3D('',#67802,#51986,#51987);
#46372=AXIS2_PLACEMENT_3D('',#67821,#51988,#51989);
#46373=AXIS2_PLACEMENT_3D('',#67822,#51990,#51991);
#46374=AXIS2_PLACEMENT_3D('',#67832,#51992,#51993);
#46375=AXIS2_PLACEMENT_3D('',#67852,#51995,#51996);
#46376=AXIS2_PLACEMENT_3D('',#67860,#51998,#51999);
#46377=AXIS2_PLACEMENT_3D('',#67863,#52000,#52001);
#46378=AXIS2_PLACEMENT_3D('',#67864,#52002,#52003);
#46379=AXIS2_PLACEMENT_3D('',#67865,#52004,#52005);
#46380=AXIS2_PLACEMENT_3D('',#67874,#52006,#52007);
#46381=AXIS2_PLACEMENT_3D('',#67875,#52008,#52009);
#46382=AXIS2_PLACEMENT_3D('',#67879,#52011,#52012);
#46383=AXIS2_PLACEMENT_3D('',#67881,#52013,#52014);
#46384=AXIS2_PLACEMENT_3D('',#67906,#52017,#52018);
#46385=AXIS2_PLACEMENT_3D('',#67907,#52019,#52020);
#46386=AXIS2_PLACEMENT_3D('',#67926,#52021,#52022);
#46387=AXIS2_PLACEMENT_3D('',#67934,#52024,#52025);
#46388=AXIS2_PLACEMENT_3D('',#67937,#52026,#52027);
#46389=AXIS2_PLACEMENT_3D('',#67938,#52028,#52029);
#46390=AXIS2_PLACEMENT_3D('',#67939,#52030,#52031);
#46391=AXIS2_PLACEMENT_3D('',#67951,#52032,#52033);
#46392=AXIS2_PLACEMENT_3D('',#67952,#52034,#52035);
#46393=AXIS2_PLACEMENT_3D('',#67956,#52037,#52038);
#46394=AXIS2_PLACEMENT_3D('',#67958,#52039,#52040);
#46395=AXIS2_PLACEMENT_3D('',#67994,#52043,#52044);
#46396=AXIS2_PLACEMENT_3D('',#68002,#52046,#52047);
#46397=AXIS2_PLACEMENT_3D('',#68005,#52048,#52049);
#46398=AXIS2_PLACEMENT_3D('',#68006,#52050,#52051);
#46399=AXIS2_PLACEMENT_3D('',#68007,#52052,#52053);
#46400=AXIS2_PLACEMENT_3D('',#68043,#52055,#52056);
#46401=AXIS2_PLACEMENT_3D('',#68045,#52057,#52058);
#46402=AXIS2_PLACEMENT_3D('',#68100,#52062,#52063);
#46403=AXIS2_PLACEMENT_3D('',#68103,#52064,#52065);
#46404=AXIS2_PLACEMENT_3D('',#68110,#52066,#52067);
#46405=AXIS2_PLACEMENT_3D('',#68122,#52068,#52069);
#46406=AXIS2_PLACEMENT_3D('',#68123,#52070,#52071);
#46407=AXIS2_PLACEMENT_3D('',#68127,#52073,#52074);
#46408=AXIS2_PLACEMENT_3D('',#68129,#52075,#52076);
#46409=AXIS2_PLACEMENT_3D('',#68165,#52079,#52080);
#46410=AXIS2_PLACEMENT_3D('',#68191,#52082,#52083);
#46411=AXIS2_PLACEMENT_3D('',#68192,#52084,#52085);
#46412=AXIS2_PLACEMENT_3D('',#68196,#52087,#52088);
#46413=AXIS2_PLACEMENT_3D('',#68198,#52089,#52090);
#46414=AXIS2_PLACEMENT_3D('',#68211,#52092,#52093);
#46415=AXIS2_PLACEMENT_3D('',#68219,#52095,#52096);
#46416=AXIS2_PLACEMENT_3D('',#68222,#52097,#52098);
#46417=AXIS2_PLACEMENT_3D('',#68223,#52099,#52100);
#46418=AXIS2_PLACEMENT_3D('',#68224,#52101,#52102);
#46419=AXIS2_PLACEMENT_3D('',#68248,#52104,#52105);
#46420=AXIS2_PLACEMENT_3D('',#68251,#52106,#52107);
#46421=AXIS2_PLACEMENT_3D('',#68252,#52108,#52109);
#46422=AXIS2_PLACEMENT_3D('',#68253,#52110,#52111);
#46423=AXIS2_PLACEMENT_3D('',#68265,#52112,#52113);
#46424=AXIS2_PLACEMENT_3D('',#68266,#52114,#52115);
#46425=AXIS2_PLACEMENT_3D('',#68270,#52117,#52118);
#46426=AXIS2_PLACEMENT_3D('',#68272,#52119,#52120);
#46427=AXIS2_PLACEMENT_3D('',#68306,#52123,#52124);
#46428=AXIS2_PLACEMENT_3D('',#68308,#52126,#52127);
#46429=AXIS2_PLACEMENT_3D('',#68309,#52128,#52129);
#46430=AXIS2_PLACEMENT_3D('',#68312,#52131,#52132);
#46431=AXIS2_PLACEMENT_3D('',#68313,#52133,#52134);
#46432=AXIS2_PLACEMENT_3D('',#68314,#52135,#52136);
#46433=AXIS2_PLACEMENT_3D('',#68333,#52137,#52138);
#46434=AXIS2_PLACEMENT_3D('',#68334,#52139,#52140);
#46435=AXIS2_PLACEMENT_3D('',#68344,#52141,#52142);
#46436=AXIS2_PLACEMENT_3D('',#68364,#52144,#52145);
#46437=AXIS2_PLACEMENT_3D('',#68372,#52147,#52148);
#46438=AXIS2_PLACEMENT_3D('',#68375,#52149,#52150);
#46439=AXIS2_PLACEMENT_3D('',#68376,#52151,#52152);
#46440=AXIS2_PLACEMENT_3D('',#68377,#52153,#52154);
#46441=AXIS2_PLACEMENT_3D('',#68386,#52155,#52156);
#46442=AXIS2_PLACEMENT_3D('',#68387,#52157,#52158);
#46443=AXIS2_PLACEMENT_3D('',#68391,#52160,#52161);
#46444=AXIS2_PLACEMENT_3D('',#68393,#52162,#52163);
#46445=AXIS2_PLACEMENT_3D('',#68418,#52166,#52167);
#46446=AXIS2_PLACEMENT_3D('',#68419,#52168,#52169);
#46447=AXIS2_PLACEMENT_3D('',#68438,#52170,#52171);
#46448=AXIS2_PLACEMENT_3D('',#68446,#52173,#52174);
#46449=AXIS2_PLACEMENT_3D('',#68449,#52175,#52176);
#46450=AXIS2_PLACEMENT_3D('',#68450,#52177,#52178);
#46451=AXIS2_PLACEMENT_3D('',#68451,#52179,#52180);
#46452=AXIS2_PLACEMENT_3D('',#68463,#52181,#52182);
#46453=AXIS2_PLACEMENT_3D('',#68464,#52183,#52184);
#46454=AXIS2_PLACEMENT_3D('',#68468,#52186,#52187);
#46455=AXIS2_PLACEMENT_3D('',#68470,#52188,#52189);
#46456=AXIS2_PLACEMENT_3D('',#68506,#52192,#52193);
#46457=AXIS2_PLACEMENT_3D('',#68514,#52195,#52196);
#46458=AXIS2_PLACEMENT_3D('',#68517,#52197,#52198);
#46459=AXIS2_PLACEMENT_3D('',#68518,#52199,#52200);
#46460=AXIS2_PLACEMENT_3D('',#68519,#52201,#52202);
#46461=AXIS2_PLACEMENT_3D('',#68555,#52204,#52205);
#46462=AXIS2_PLACEMENT_3D('',#68557,#52206,#52207);
#46463=AXIS2_PLACEMENT_3D('',#68612,#52211,#52212);
#46464=AXIS2_PLACEMENT_3D('',#68615,#52213,#52214);
#46465=AXIS2_PLACEMENT_3D('',#68622,#52215,#52216);
#46466=AXIS2_PLACEMENT_3D('',#68634,#52217,#52218);
#46467=AXIS2_PLACEMENT_3D('',#68635,#52219,#52220);
#46468=AXIS2_PLACEMENT_3D('',#68639,#52222,#52223);
#46469=AXIS2_PLACEMENT_3D('',#68641,#52224,#52225);
#46470=AXIS2_PLACEMENT_3D('',#68677,#52228,#52229);
#46471=AXIS2_PLACEMENT_3D('',#68685,#52231,#52232);
#46472=AXIS2_PLACEMENT_3D('',#68688,#52233,#52234);
#46473=AXIS2_PLACEMENT_3D('',#68689,#52235,#52236);
#46474=AXIS2_PLACEMENT_3D('',#68690,#52237,#52238);
#46475=AXIS2_PLACEMENT_3D('',#68709,#52239,#52240);
#46476=AXIS2_PLACEMENT_3D('',#68710,#52241,#52242);
#46477=AXIS2_PLACEMENT_3D('',#68714,#52244,#52245);
#46478=AXIS2_PLACEMENT_3D('',#68716,#52246,#52247);
#46479=AXIS2_PLACEMENT_3D('',#68752,#52250,#52251);
#46480=AXIS2_PLACEMENT_3D('',#68774,#52253,#52254);
#46481=AXIS2_PLACEMENT_3D('',#68775,#52255,#52256);
#46482=AXIS2_PLACEMENT_3D('',#68779,#52258,#52259);
#46483=AXIS2_PLACEMENT_3D('',#68781,#52260,#52261);
#46484=AXIS2_PLACEMENT_3D('',#68792,#52263,#52264);
#46485=AXIS2_PLACEMENT_3D('',#68794,#52266,#52267);
#46486=AXIS2_PLACEMENT_3D('',#68797,#52268,#52269);
#46487=AXIS2_PLACEMENT_3D('',#68798,#52270,#52271);
#46488=AXIS2_PLACEMENT_3D('',#68799,#52272,#52273);
#46489=AXIS2_PLACEMENT_3D('',#68823,#52275,#52276);
#46490=AXIS2_PLACEMENT_3D('',#68824,#52277,#52278);
#46491=AXIS2_PLACEMENT_3D('',#68827,#52280,#52281);
#46492=AXIS2_PLACEMENT_3D('',#68828,#52282,#52283);
#46493=AXIS2_PLACEMENT_3D('',#68829,#52284,#52285);
#46494=AXIS2_PLACEMENT_3D('',#68848,#52286,#52287);
#46495=AXIS2_PLACEMENT_3D('',#68849,#52288,#52289);
#46496=AXIS2_PLACEMENT_3D('',#68859,#52290,#52291);
#46497=AXIS2_PLACEMENT_3D('',#68879,#52293,#52294);
#46498=AXIS2_PLACEMENT_3D('',#68887,#52296,#52297);
#46499=AXIS2_PLACEMENT_3D('',#68890,#52298,#52299);
#46500=AXIS2_PLACEMENT_3D('',#68891,#52300,#52301);
#46501=AXIS2_PLACEMENT_3D('',#68892,#52302,#52303);
#46502=AXIS2_PLACEMENT_3D('',#68901,#52304,#52305);
#46503=AXIS2_PLACEMENT_3D('',#68902,#52306,#52307);
#46504=AXIS2_PLACEMENT_3D('',#68906,#52309,#52310);
#46505=AXIS2_PLACEMENT_3D('',#68908,#52311,#52312);
#46506=AXIS2_PLACEMENT_3D('',#68933,#52315,#52316);
#46507=AXIS2_PLACEMENT_3D('',#68934,#52317,#52318);
#46508=AXIS2_PLACEMENT_3D('',#68953,#52319,#52320);
#46509=AXIS2_PLACEMENT_3D('',#68961,#52322,#52323);
#46510=AXIS2_PLACEMENT_3D('',#68964,#52324,#52325);
#46511=AXIS2_PLACEMENT_3D('',#68965,#52326,#52327);
#46512=AXIS2_PLACEMENT_3D('',#68966,#52328,#52329);
#46513=AXIS2_PLACEMENT_3D('',#68978,#52330,#52331);
#46514=AXIS2_PLACEMENT_3D('',#68979,#52332,#52333);
#46515=AXIS2_PLACEMENT_3D('',#68983,#52335,#52336);
#46516=AXIS2_PLACEMENT_3D('',#68985,#52337,#52338);
#46517=AXIS2_PLACEMENT_3D('',#69021,#52341,#52342);
#46518=AXIS2_PLACEMENT_3D('',#69029,#52344,#52345);
#46519=AXIS2_PLACEMENT_3D('',#69032,#52346,#52347);
#46520=AXIS2_PLACEMENT_3D('',#69033,#52348,#52349);
#46521=AXIS2_PLACEMENT_3D('',#69034,#52350,#52351);
#46522=AXIS2_PLACEMENT_3D('',#69070,#52353,#52354);
#46523=AXIS2_PLACEMENT_3D('',#69072,#52355,#52356);
#46524=AXIS2_PLACEMENT_3D('',#69127,#52360,#52361);
#46525=AXIS2_PLACEMENT_3D('',#69130,#52362,#52363);
#46526=AXIS2_PLACEMENT_3D('',#69137,#52364,#52365);
#46527=AXIS2_PLACEMENT_3D('',#69149,#52366,#52367);
#46528=AXIS2_PLACEMENT_3D('',#69150,#52368,#52369);
#46529=AXIS2_PLACEMENT_3D('',#69154,#52371,#52372);
#46530=AXIS2_PLACEMENT_3D('',#69156,#52373,#52374);
#46531=AXIS2_PLACEMENT_3D('',#69192,#52377,#52378);
#46532=AXIS2_PLACEMENT_3D('',#69200,#52380,#52381);
#46533=AXIS2_PLACEMENT_3D('',#69203,#52382,#52383);
#46534=AXIS2_PLACEMENT_3D('',#69204,#52384,#52385);
#46535=AXIS2_PLACEMENT_3D('',#69205,#52386,#52387);
#46536=AXIS2_PLACEMENT_3D('',#69224,#52388,#52389);
#46537=AXIS2_PLACEMENT_3D('',#69225,#52390,#52391);
#46538=AXIS2_PLACEMENT_3D('',#69229,#52393,#52394);
#46539=AXIS2_PLACEMENT_3D('',#69231,#52395,#52396);
#46540=AXIS2_PLACEMENT_3D('',#69267,#52399,#52400);
#46541=AXIS2_PLACEMENT_3D('',#69275,#52402,#52403);
#46542=AXIS2_PLACEMENT_3D('',#69278,#52404,#52405);
#46543=AXIS2_PLACEMENT_3D('',#69279,#52406,#52407);
#46544=AXIS2_PLACEMENT_3D('',#69280,#52408,#52409);
#46545=AXIS2_PLACEMENT_3D('',#69295,#52410,#52411);
#46546=AXIS2_PLACEMENT_3D('',#69296,#52412,#52413);
#46547=AXIS2_PLACEMENT_3D('',#69300,#52415,#52416);
#46548=AXIS2_PLACEMENT_3D('',#69302,#52417,#52418);
#46549=AXIS2_PLACEMENT_3D('',#69336,#52421,#52422);
#46550=AXIS2_PLACEMENT_3D('',#69338,#52424,#52425);
#46551=AXIS2_PLACEMENT_3D('',#69339,#52426,#52427);
#46552=AXIS2_PLACEMENT_3D('',#69342,#52429,#52430);
#46553=AXIS2_PLACEMENT_3D('',#69343,#52431,#52432);
#46554=AXIS2_PLACEMENT_3D('',#69344,#52433,#52434);
#46555=AXIS2_PLACEMENT_3D('',#69363,#52435,#52436);
#46556=AXIS2_PLACEMENT_3D('',#69364,#52437,#52438);
#46557=AXIS2_PLACEMENT_3D('',#69374,#52439,#52440);
#46558=AXIS2_PLACEMENT_3D('',#69394,#52442,#52443);
#46559=AXIS2_PLACEMENT_3D('',#69402,#52445,#52446);
#46560=AXIS2_PLACEMENT_3D('',#69405,#52447,#52448);
#46561=AXIS2_PLACEMENT_3D('',#69406,#52449,#52450);
#46562=AXIS2_PLACEMENT_3D('',#69407,#52451,#52452);
#46563=AXIS2_PLACEMENT_3D('',#69416,#52453,#52454);
#46564=AXIS2_PLACEMENT_3D('',#69417,#52455,#52456);
#46565=AXIS2_PLACEMENT_3D('',#69421,#52458,#52459);
#46566=AXIS2_PLACEMENT_3D('',#69423,#52460,#52461);
#46567=AXIS2_PLACEMENT_3D('',#69448,#52464,#52465);
#46568=AXIS2_PLACEMENT_3D('',#69449,#52466,#52467);
#46569=AXIS2_PLACEMENT_3D('',#69468,#52468,#52469);
#46570=AXIS2_PLACEMENT_3D('',#69476,#52471,#52472);
#46571=AXIS2_PLACEMENT_3D('',#69479,#52473,#52474);
#46572=AXIS2_PLACEMENT_3D('',#69480,#52475,#52476);
#46573=AXIS2_PLACEMENT_3D('',#69481,#52477,#52478);
#46574=AXIS2_PLACEMENT_3D('',#69493,#52479,#52480);
#46575=AXIS2_PLACEMENT_3D('',#69494,#52481,#52482);
#46576=AXIS2_PLACEMENT_3D('',#69498,#52484,#52485);
#46577=AXIS2_PLACEMENT_3D('',#69500,#52486,#52487);
#46578=AXIS2_PLACEMENT_3D('',#69536,#52490,#52491);
#46579=AXIS2_PLACEMENT_3D('',#69544,#52493,#52494);
#46580=AXIS2_PLACEMENT_3D('',#69547,#52495,#52496);
#46581=AXIS2_PLACEMENT_3D('',#69548,#52497,#52498);
#46582=AXIS2_PLACEMENT_3D('',#69549,#52499,#52500);
#46583=AXIS2_PLACEMENT_3D('',#69585,#52502,#52503);
#46584=AXIS2_PLACEMENT_3D('',#69587,#52504,#52505);
#46585=AXIS2_PLACEMENT_3D('',#69642,#52509,#52510);
#46586=AXIS2_PLACEMENT_3D('',#69645,#52511,#52512);
#46587=AXIS2_PLACEMENT_3D('',#69652,#52513,#52514);
#46588=AXIS2_PLACEMENT_3D('',#69664,#52515,#52516);
#46589=AXIS2_PLACEMENT_3D('',#69665,#52517,#52518);
#46590=AXIS2_PLACEMENT_3D('',#69669,#52520,#52521);
#46591=AXIS2_PLACEMENT_3D('',#69671,#52522,#52523);
#46592=AXIS2_PLACEMENT_3D('',#69707,#52526,#52527);
#46593=AXIS2_PLACEMENT_3D('',#69715,#52529,#52530);
#46594=AXIS2_PLACEMENT_3D('',#69718,#52531,#52532);
#46595=AXIS2_PLACEMENT_3D('',#69719,#52533,#52534);
#46596=AXIS2_PLACEMENT_3D('',#69720,#52535,#52536);
#46597=AXIS2_PLACEMENT_3D('',#69739,#52537,#52538);
#46598=AXIS2_PLACEMENT_3D('',#69740,#52539,#52540);
#46599=AXIS2_PLACEMENT_3D('',#69744,#52542,#52543);
#46600=AXIS2_PLACEMENT_3D('',#69746,#52544,#52545);
#46601=AXIS2_PLACEMENT_3D('',#69782,#52548,#52549);
#46602=AXIS2_PLACEMENT_3D('',#69790,#52551,#52552);
#46603=AXIS2_PLACEMENT_3D('',#69793,#52553,#52554);
#46604=AXIS2_PLACEMENT_3D('',#69794,#52555,#52556);
#46605=AXIS2_PLACEMENT_3D('',#69795,#52557,#52558);
#46606=AXIS2_PLACEMENT_3D('',#69810,#52559,#52560);
#46607=AXIS2_PLACEMENT_3D('',#69811,#52561,#52562);
#46608=AXIS2_PLACEMENT_3D('',#69815,#52564,#52565);
#46609=AXIS2_PLACEMENT_3D('',#69817,#52566,#52567);
#46610=AXIS2_PLACEMENT_3D('',#69851,#52570,#52571);
#46611=AXIS2_PLACEMENT_3D('',#69853,#52573,#52574);
#46612=AXIS2_PLACEMENT_3D('',#69854,#52575,#52576);
#46613=AXIS2_PLACEMENT_3D('',#69857,#52578,#52579);
#46614=AXIS2_PLACEMENT_3D('',#69858,#52580,#52581);
#46615=AXIS2_PLACEMENT_3D('',#69859,#52582,#52583);
#46616=AXIS2_PLACEMENT_3D('',#69878,#52584,#52585);
#46617=AXIS2_PLACEMENT_3D('',#69879,#52586,#52587);
#46618=AXIS2_PLACEMENT_3D('',#69889,#52588,#52589);
#46619=AXIS2_PLACEMENT_3D('',#69909,#52591,#52592);
#46620=AXIS2_PLACEMENT_3D('',#69917,#52594,#52595);
#46621=AXIS2_PLACEMENT_3D('',#69920,#52596,#52597);
#46622=AXIS2_PLACEMENT_3D('',#69921,#52598,#52599);
#46623=AXIS2_PLACEMENT_3D('',#69922,#52600,#52601);
#46624=AXIS2_PLACEMENT_3D('',#69931,#52602,#52603);
#46625=AXIS2_PLACEMENT_3D('',#69932,#52604,#52605);
#46626=AXIS2_PLACEMENT_3D('',#69936,#52607,#52608);
#46627=AXIS2_PLACEMENT_3D('',#69938,#52609,#52610);
#46628=AXIS2_PLACEMENT_3D('',#69963,#52613,#52614);
#46629=AXIS2_PLACEMENT_3D('',#69964,#52615,#52616);
#46630=AXIS2_PLACEMENT_3D('',#69983,#52617,#52618);
#46631=AXIS2_PLACEMENT_3D('',#69991,#52620,#52621);
#46632=AXIS2_PLACEMENT_3D('',#69994,#52622,#52623);
#46633=AXIS2_PLACEMENT_3D('',#69995,#52624,#52625);
#46634=AXIS2_PLACEMENT_3D('',#69996,#52626,#52627);
#46635=AXIS2_PLACEMENT_3D('',#70008,#52628,#52629);
#46636=AXIS2_PLACEMENT_3D('',#70009,#52630,#52631);
#46637=AXIS2_PLACEMENT_3D('',#70013,#52633,#52634);
#46638=AXIS2_PLACEMENT_3D('',#70015,#52635,#52636);
#46639=AXIS2_PLACEMENT_3D('',#70051,#52639,#52640);
#46640=AXIS2_PLACEMENT_3D('',#70059,#52642,#52643);
#46641=AXIS2_PLACEMENT_3D('',#70062,#52644,#52645);
#46642=AXIS2_PLACEMENT_3D('',#70063,#52646,#52647);
#46643=AXIS2_PLACEMENT_3D('',#70064,#52648,#52649);
#46644=AXIS2_PLACEMENT_3D('',#70100,#52651,#52652);
#46645=AXIS2_PLACEMENT_3D('',#70102,#52653,#52654);
#46646=AXIS2_PLACEMENT_3D('',#70157,#52658,#52659);
#46647=AXIS2_PLACEMENT_3D('',#70160,#52660,#52661);
#46648=AXIS2_PLACEMENT_3D('',#70167,#52662,#52663);
#46649=AXIS2_PLACEMENT_3D('',#70179,#52664,#52665);
#46650=AXIS2_PLACEMENT_3D('',#70180,#52666,#52667);
#46651=AXIS2_PLACEMENT_3D('',#70184,#52669,#52670);
#46652=AXIS2_PLACEMENT_3D('',#70186,#52671,#52672);
#46653=AXIS2_PLACEMENT_3D('',#70222,#52675,#52676);
#46654=AXIS2_PLACEMENT_3D('',#70230,#52678,#52679);
#46655=AXIS2_PLACEMENT_3D('',#70233,#52680,#52681);
#46656=AXIS2_PLACEMENT_3D('',#70234,#52682,#52683);
#46657=AXIS2_PLACEMENT_3D('',#70235,#52684,#52685);
#46658=AXIS2_PLACEMENT_3D('',#70254,#52686,#52687);
#46659=AXIS2_PLACEMENT_3D('',#70255,#52688,#52689);
#46660=AXIS2_PLACEMENT_3D('',#70259,#52691,#52692);
#46661=AXIS2_PLACEMENT_3D('',#70261,#52693,#52694);
#46662=AXIS2_PLACEMENT_3D('',#70297,#52697,#52698);
#46663=AXIS2_PLACEMENT_3D('',#70305,#52700,#52701);
#46664=AXIS2_PLACEMENT_3D('',#70308,#52702,#52703);
#46665=AXIS2_PLACEMENT_3D('',#70309,#52704,#52705);
#46666=AXIS2_PLACEMENT_3D('',#70310,#52706,#52707);
#46667=AXIS2_PLACEMENT_3D('',#70325,#52708,#52709);
#46668=AXIS2_PLACEMENT_3D('',#70326,#52710,#52711);
#46669=AXIS2_PLACEMENT_3D('',#70330,#52713,#52714);
#46670=AXIS2_PLACEMENT_3D('',#70332,#52715,#52716);
#46671=AXIS2_PLACEMENT_3D('',#70366,#52719,#52720);
#46672=AXIS2_PLACEMENT_3D('',#70368,#52722,#52723);
#46673=AXIS2_PLACEMENT_3D('',#70369,#52724,#52725);
#46674=AXIS2_PLACEMENT_3D('',#70372,#52727,#52728);
#46675=AXIS2_PLACEMENT_3D('',#70373,#52729,#52730);
#46676=AXIS2_PLACEMENT_3D('',#70374,#52731,#52732);
#46677=AXIS2_PLACEMENT_3D('',#70393,#52733,#52734);
#46678=AXIS2_PLACEMENT_3D('',#70394,#52735,#52736);
#46679=AXIS2_PLACEMENT_3D('',#70404,#52737,#52738);
#46680=AXIS2_PLACEMENT_3D('',#70424,#52740,#52741);
#46681=AXIS2_PLACEMENT_3D('',#70432,#52743,#52744);
#46682=AXIS2_PLACEMENT_3D('',#70435,#52745,#52746);
#46683=AXIS2_PLACEMENT_3D('',#70436,#52747,#52748);
#46684=AXIS2_PLACEMENT_3D('',#70437,#52749,#52750);
#46685=AXIS2_PLACEMENT_3D('',#70446,#52751,#52752);
#46686=AXIS2_PLACEMENT_3D('',#70447,#52753,#52754);
#46687=AXIS2_PLACEMENT_3D('',#70451,#52756,#52757);
#46688=AXIS2_PLACEMENT_3D('',#70453,#52758,#52759);
#46689=AXIS2_PLACEMENT_3D('',#70478,#52762,#52763);
#46690=AXIS2_PLACEMENT_3D('',#70479,#52764,#52765);
#46691=AXIS2_PLACEMENT_3D('',#70498,#52766,#52767);
#46692=AXIS2_PLACEMENT_3D('',#70506,#52769,#52770);
#46693=AXIS2_PLACEMENT_3D('',#70509,#52771,#52772);
#46694=AXIS2_PLACEMENT_3D('',#70510,#52773,#52774);
#46695=AXIS2_PLACEMENT_3D('',#70511,#52775,#52776);
#46696=AXIS2_PLACEMENT_3D('',#70523,#52777,#52778);
#46697=AXIS2_PLACEMENT_3D('',#70524,#52779,#52780);
#46698=AXIS2_PLACEMENT_3D('',#70528,#52782,#52783);
#46699=AXIS2_PLACEMENT_3D('',#70530,#52784,#52785);
#46700=AXIS2_PLACEMENT_3D('',#70566,#52788,#52789);
#46701=AXIS2_PLACEMENT_3D('',#70574,#52791,#52792);
#46702=AXIS2_PLACEMENT_3D('',#70577,#52793,#52794);
#46703=AXIS2_PLACEMENT_3D('',#70578,#52795,#52796);
#46704=AXIS2_PLACEMENT_3D('',#70579,#52797,#52798);
#46705=AXIS2_PLACEMENT_3D('',#70615,#52800,#52801);
#46706=AXIS2_PLACEMENT_3D('',#70617,#52802,#52803);
#46707=AXIS2_PLACEMENT_3D('',#70672,#52807,#52808);
#46708=AXIS2_PLACEMENT_3D('',#70675,#52809,#52810);
#46709=AXIS2_PLACEMENT_3D('',#70682,#52811,#52812);
#46710=AXIS2_PLACEMENT_3D('',#70694,#52813,#52814);
#46711=AXIS2_PLACEMENT_3D('',#70695,#52815,#52816);
#46712=AXIS2_PLACEMENT_3D('',#70699,#52818,#52819);
#46713=AXIS2_PLACEMENT_3D('',#70701,#52820,#52821);
#46714=AXIS2_PLACEMENT_3D('',#70737,#52824,#52825);
#46715=AXIS2_PLACEMENT_3D('',#70745,#52827,#52828);
#46716=AXIS2_PLACEMENT_3D('',#70748,#52829,#52830);
#46717=AXIS2_PLACEMENT_3D('',#70749,#52831,#52832);
#46718=AXIS2_PLACEMENT_3D('',#70750,#52833,#52834);
#46719=AXIS2_PLACEMENT_3D('',#70769,#52835,#52836);
#46720=AXIS2_PLACEMENT_3D('',#70770,#52837,#52838);
#46721=AXIS2_PLACEMENT_3D('',#70774,#52840,#52841);
#46722=AXIS2_PLACEMENT_3D('',#70776,#52842,#52843);
#46723=AXIS2_PLACEMENT_3D('',#70812,#52846,#52847);
#46724=AXIS2_PLACEMENT_3D('',#70820,#52849,#52850);
#46725=AXIS2_PLACEMENT_3D('',#70823,#52851,#52852);
#46726=AXIS2_PLACEMENT_3D('',#70824,#52853,#52854);
#46727=AXIS2_PLACEMENT_3D('',#70825,#52855,#52856);
#46728=AXIS2_PLACEMENT_3D('',#70840,#52857,#52858);
#46729=AXIS2_PLACEMENT_3D('',#70841,#52859,#52860);
#46730=AXIS2_PLACEMENT_3D('',#70845,#52862,#52863);
#46731=AXIS2_PLACEMENT_3D('',#70847,#52864,#52865);
#46732=AXIS2_PLACEMENT_3D('',#70881,#52868,#52869);
#46733=AXIS2_PLACEMENT_3D('',#70883,#52871,#52872);
#46734=AXIS2_PLACEMENT_3D('',#70884,#52873,#52874);
#46735=AXIS2_PLACEMENT_3D('',#70887,#52876,#52877);
#46736=AXIS2_PLACEMENT_3D('',#70888,#52878,#52879);
#46737=AXIS2_PLACEMENT_3D('',#70889,#52880,#52881);
#46738=AXIS2_PLACEMENT_3D('',#70908,#52882,#52883);
#46739=AXIS2_PLACEMENT_3D('',#70909,#52884,#52885);
#46740=AXIS2_PLACEMENT_3D('',#70919,#52886,#52887);
#46741=AXIS2_PLACEMENT_3D('',#70939,#52889,#52890);
#46742=AXIS2_PLACEMENT_3D('',#70947,#52892,#52893);
#46743=AXIS2_PLACEMENT_3D('',#70950,#52894,#52895);
#46744=AXIS2_PLACEMENT_3D('',#70951,#52896,#52897);
#46745=AXIS2_PLACEMENT_3D('',#70952,#52898,#52899);
#46746=AXIS2_PLACEMENT_3D('',#70961,#52900,#52901);
#46747=AXIS2_PLACEMENT_3D('',#70962,#52902,#52903);
#46748=AXIS2_PLACEMENT_3D('',#70966,#52905,#52906);
#46749=AXIS2_PLACEMENT_3D('',#70968,#52907,#52908);
#46750=AXIS2_PLACEMENT_3D('',#70993,#52911,#52912);
#46751=AXIS2_PLACEMENT_3D('',#70994,#52913,#52914);
#46752=AXIS2_PLACEMENT_3D('',#71013,#52915,#52916);
#46753=AXIS2_PLACEMENT_3D('',#71021,#52918,#52919);
#46754=AXIS2_PLACEMENT_3D('',#71024,#52920,#52921);
#46755=AXIS2_PLACEMENT_3D('',#71025,#52922,#52923);
#46756=AXIS2_PLACEMENT_3D('',#71026,#52924,#52925);
#46757=AXIS2_PLACEMENT_3D('',#71038,#52926,#52927);
#46758=AXIS2_PLACEMENT_3D('',#71039,#52928,#52929);
#46759=AXIS2_PLACEMENT_3D('',#71043,#52931,#52932);
#46760=AXIS2_PLACEMENT_3D('',#71045,#52933,#52934);
#46761=AXIS2_PLACEMENT_3D('',#71081,#52937,#52938);
#46762=AXIS2_PLACEMENT_3D('',#71089,#52940,#52941);
#46763=AXIS2_PLACEMENT_3D('',#71092,#52942,#52943);
#46764=AXIS2_PLACEMENT_3D('',#71093,#52944,#52945);
#46765=AXIS2_PLACEMENT_3D('',#71094,#52946,#52947);
#46766=AXIS2_PLACEMENT_3D('',#71130,#52949,#52950);
#46767=AXIS2_PLACEMENT_3D('',#71132,#52951,#52952);
#46768=AXIS2_PLACEMENT_3D('',#71187,#52956,#52957);
#46769=AXIS2_PLACEMENT_3D('',#71190,#52958,#52959);
#46770=AXIS2_PLACEMENT_3D('',#71197,#52960,#52961);
#46771=AXIS2_PLACEMENT_3D('',#71209,#52962,#52963);
#46772=AXIS2_PLACEMENT_3D('',#71210,#52964,#52965);
#46773=AXIS2_PLACEMENT_3D('',#71214,#52967,#52968);
#46774=AXIS2_PLACEMENT_3D('',#71216,#52969,#52970);
#46775=AXIS2_PLACEMENT_3D('',#71252,#52973,#52974);
#46776=AXIS2_PLACEMENT_3D('',#71260,#52976,#52977);
#46777=AXIS2_PLACEMENT_3D('',#71263,#52978,#52979);
#46778=AXIS2_PLACEMENT_3D('',#71264,#52980,#52981);
#46779=AXIS2_PLACEMENT_3D('',#71265,#52982,#52983);
#46780=AXIS2_PLACEMENT_3D('',#71284,#52984,#52985);
#46781=AXIS2_PLACEMENT_3D('',#71285,#52986,#52987);
#46782=AXIS2_PLACEMENT_3D('',#71289,#52989,#52990);
#46783=AXIS2_PLACEMENT_3D('',#71291,#52991,#52992);
#46784=AXIS2_PLACEMENT_3D('',#71327,#52995,#52996);
#46785=AXIS2_PLACEMENT_3D('',#71335,#52998,#52999);
#46786=AXIS2_PLACEMENT_3D('',#71338,#53000,#53001);
#46787=AXIS2_PLACEMENT_3D('',#71339,#53002,#53003);
#46788=AXIS2_PLACEMENT_3D('',#71340,#53004,#53005);
#46789=AXIS2_PLACEMENT_3D('',#71355,#53006,#53007);
#46790=AXIS2_PLACEMENT_3D('',#71356,#53008,#53009);
#46791=AXIS2_PLACEMENT_3D('',#71360,#53011,#53012);
#46792=AXIS2_PLACEMENT_3D('',#71362,#53013,#53014);
#46793=AXIS2_PLACEMENT_3D('',#71396,#53017,#53018);
#46794=AXIS2_PLACEMENT_3D('',#71398,#53020,#53021);
#46795=AXIS2_PLACEMENT_3D('',#71399,#53022,#53023);
#46796=AXIS2_PLACEMENT_3D('',#71402,#53025,#53026);
#46797=AXIS2_PLACEMENT_3D('',#71403,#53027,#53028);
#46798=AXIS2_PLACEMENT_3D('',#71404,#53029,#53030);
#46799=AXIS2_PLACEMENT_3D('',#71423,#53031,#53032);
#46800=AXIS2_PLACEMENT_3D('',#71424,#53033,#53034);
#46801=AXIS2_PLACEMENT_3D('',#71434,#53035,#53036);
#46802=AXIS2_PLACEMENT_3D('',#71454,#53038,#53039);
#46803=AXIS2_PLACEMENT_3D('',#71462,#53041,#53042);
#46804=AXIS2_PLACEMENT_3D('',#71465,#53043,#53044);
#46805=AXIS2_PLACEMENT_3D('',#71466,#53045,#53046);
#46806=AXIS2_PLACEMENT_3D('',#71467,#53047,#53048);
#46807=AXIS2_PLACEMENT_3D('',#71476,#53049,#53050);
#46808=AXIS2_PLACEMENT_3D('',#71477,#53051,#53052);
#46809=AXIS2_PLACEMENT_3D('',#71481,#53054,#53055);
#46810=AXIS2_PLACEMENT_3D('',#71483,#53056,#53057);
#46811=AXIS2_PLACEMENT_3D('',#71508,#53060,#53061);
#46812=AXIS2_PLACEMENT_3D('',#71509,#53062,#53063);
#46813=AXIS2_PLACEMENT_3D('',#71528,#53064,#53065);
#46814=AXIS2_PLACEMENT_3D('',#71536,#53067,#53068);
#46815=AXIS2_PLACEMENT_3D('',#71539,#53069,#53070);
#46816=AXIS2_PLACEMENT_3D('',#71540,#53071,#53072);
#46817=AXIS2_PLACEMENT_3D('',#71541,#53073,#53074);
#46818=AXIS2_PLACEMENT_3D('',#71553,#53075,#53076);
#46819=AXIS2_PLACEMENT_3D('',#71554,#53077,#53078);
#46820=AXIS2_PLACEMENT_3D('',#71558,#53080,#53081);
#46821=AXIS2_PLACEMENT_3D('',#71560,#53082,#53083);
#46822=AXIS2_PLACEMENT_3D('',#71596,#53086,#53087);
#46823=AXIS2_PLACEMENT_3D('',#71604,#53089,#53090);
#46824=AXIS2_PLACEMENT_3D('',#71607,#53091,#53092);
#46825=AXIS2_PLACEMENT_3D('',#71608,#53093,#53094);
#46826=AXIS2_PLACEMENT_3D('',#71609,#53095,#53096);
#46827=AXIS2_PLACEMENT_3D('',#71645,#53098,#53099);
#46828=AXIS2_PLACEMENT_3D('',#71647,#53100,#53101);
#46829=AXIS2_PLACEMENT_3D('',#71702,#53105,#53106);
#46830=AXIS2_PLACEMENT_3D('',#71705,#53107,#53108);
#46831=AXIS2_PLACEMENT_3D('',#71712,#53109,#53110);
#46832=AXIS2_PLACEMENT_3D('',#71724,#53111,#53112);
#46833=AXIS2_PLACEMENT_3D('',#71725,#53113,#53114);
#46834=AXIS2_PLACEMENT_3D('',#71729,#53116,#53117);
#46835=AXIS2_PLACEMENT_3D('',#71731,#53118,#53119);
#46836=AXIS2_PLACEMENT_3D('',#71767,#53122,#53123);
#46837=AXIS2_PLACEMENT_3D('',#71775,#53125,#53126);
#46838=AXIS2_PLACEMENT_3D('',#71778,#53127,#53128);
#46839=AXIS2_PLACEMENT_3D('',#71779,#53129,#53130);
#46840=AXIS2_PLACEMENT_3D('',#71780,#53131,#53132);
#46841=AXIS2_PLACEMENT_3D('',#71799,#53133,#53134);
#46842=AXIS2_PLACEMENT_3D('',#71800,#53135,#53136);
#46843=AXIS2_PLACEMENT_3D('',#71804,#53138,#53139);
#46844=AXIS2_PLACEMENT_3D('',#71806,#53140,#53141);
#46845=AXIS2_PLACEMENT_3D('',#71842,#53144,#53145);
#46846=AXIS2_PLACEMENT_3D('',#71850,#53147,#53148);
#46847=AXIS2_PLACEMENT_3D('',#71853,#53149,#53150);
#46848=AXIS2_PLACEMENT_3D('',#71854,#53151,#53152);
#46849=AXIS2_PLACEMENT_3D('',#71855,#53153,#53154);
#46850=AXIS2_PLACEMENT_3D('',#71870,#53155,#53156);
#46851=AXIS2_PLACEMENT_3D('',#71871,#53157,#53158);
#46852=AXIS2_PLACEMENT_3D('',#71875,#53160,#53161);
#46853=AXIS2_PLACEMENT_3D('',#71877,#53162,#53163);
#46854=AXIS2_PLACEMENT_3D('',#71911,#53166,#53167);
#46855=AXIS2_PLACEMENT_3D('',#71913,#53169,#53170);
#46856=AXIS2_PLACEMENT_3D('',#71914,#53171,#53172);
#46857=AXIS2_PLACEMENT_3D('',#71917,#53174,#53175);
#46858=AXIS2_PLACEMENT_3D('',#71918,#53176,#53177);
#46859=AXIS2_PLACEMENT_3D('',#71919,#53178,#53179);
#46860=AXIS2_PLACEMENT_3D('',#71938,#53180,#53181);
#46861=AXIS2_PLACEMENT_3D('',#71939,#53182,#53183);
#46862=AXIS2_PLACEMENT_3D('',#71949,#53184,#53185);
#46863=AXIS2_PLACEMENT_3D('',#71969,#53187,#53188);
#46864=AXIS2_PLACEMENT_3D('',#71977,#53190,#53191);
#46865=AXIS2_PLACEMENT_3D('',#71980,#53192,#53193);
#46866=AXIS2_PLACEMENT_3D('',#71981,#53194,#53195);
#46867=AXIS2_PLACEMENT_3D('',#71982,#53196,#53197);
#46868=AXIS2_PLACEMENT_3D('',#71991,#53198,#53199);
#46869=AXIS2_PLACEMENT_3D('',#71992,#53200,#53201);
#46870=AXIS2_PLACEMENT_3D('',#71996,#53203,#53204);
#46871=AXIS2_PLACEMENT_3D('',#71998,#53205,#53206);
#46872=AXIS2_PLACEMENT_3D('',#72023,#53209,#53210);
#46873=AXIS2_PLACEMENT_3D('',#72024,#53211,#53212);
#46874=AXIS2_PLACEMENT_3D('',#72043,#53213,#53214);
#46875=AXIS2_PLACEMENT_3D('',#72051,#53216,#53217);
#46876=AXIS2_PLACEMENT_3D('',#72054,#53218,#53219);
#46877=AXIS2_PLACEMENT_3D('',#72055,#53220,#53221);
#46878=AXIS2_PLACEMENT_3D('',#72056,#53222,#53223);
#46879=AXIS2_PLACEMENT_3D('',#72068,#53224,#53225);
#46880=AXIS2_PLACEMENT_3D('',#72069,#53226,#53227);
#46881=AXIS2_PLACEMENT_3D('',#72073,#53229,#53230);
#46882=AXIS2_PLACEMENT_3D('',#72075,#53231,#53232);
#46883=AXIS2_PLACEMENT_3D('',#72111,#53235,#53236);
#46884=AXIS2_PLACEMENT_3D('',#72119,#53238,#53239);
#46885=AXIS2_PLACEMENT_3D('',#72122,#53240,#53241);
#46886=AXIS2_PLACEMENT_3D('',#72123,#53242,#53243);
#46887=AXIS2_PLACEMENT_3D('',#72124,#53244,#53245);
#46888=AXIS2_PLACEMENT_3D('',#72160,#53247,#53248);
#46889=AXIS2_PLACEMENT_3D('',#72162,#53249,#53250);
#46890=AXIS2_PLACEMENT_3D('',#72217,#53254,#53255);
#46891=AXIS2_PLACEMENT_3D('',#72220,#53256,#53257);
#46892=AXIS2_PLACEMENT_3D('',#72227,#53258,#53259);
#46893=AXIS2_PLACEMENT_3D('',#72239,#53260,#53261);
#46894=AXIS2_PLACEMENT_3D('',#72240,#53262,#53263);
#46895=AXIS2_PLACEMENT_3D('',#72244,#53265,#53266);
#46896=AXIS2_PLACEMENT_3D('',#72246,#53267,#53268);
#46897=AXIS2_PLACEMENT_3D('',#72282,#53271,#53272);
#46898=AXIS2_PLACEMENT_3D('',#72290,#53274,#53275);
#46899=AXIS2_PLACEMENT_3D('',#72293,#53276,#53277);
#46900=AXIS2_PLACEMENT_3D('',#72294,#53278,#53279);
#46901=AXIS2_PLACEMENT_3D('',#72295,#53280,#53281);
#46902=AXIS2_PLACEMENT_3D('',#72314,#53282,#53283);
#46903=AXIS2_PLACEMENT_3D('',#72315,#53284,#53285);
#46904=AXIS2_PLACEMENT_3D('',#72319,#53287,#53288);
#46905=AXIS2_PLACEMENT_3D('',#72321,#53289,#53290);
#46906=AXIS2_PLACEMENT_3D('',#72357,#53293,#53294);
#46907=AXIS2_PLACEMENT_3D('',#72365,#53296,#53297);
#46908=AXIS2_PLACEMENT_3D('',#72368,#53298,#53299);
#46909=AXIS2_PLACEMENT_3D('',#72369,#53300,#53301);
#46910=AXIS2_PLACEMENT_3D('',#72370,#53302,#53303);
#46911=AXIS2_PLACEMENT_3D('',#72385,#53304,#53305);
#46912=AXIS2_PLACEMENT_3D('',#72386,#53306,#53307);
#46913=AXIS2_PLACEMENT_3D('',#72390,#53309,#53310);
#46914=AXIS2_PLACEMENT_3D('',#72392,#53311,#53312);
#46915=AXIS2_PLACEMENT_3D('',#72426,#53315,#53316);
#46916=AXIS2_PLACEMENT_3D('',#72428,#53318,#53319);
#46917=AXIS2_PLACEMENT_3D('',#72429,#53320,#53321);
#46918=AXIS2_PLACEMENT_3D('',#72432,#53323,#53324);
#46919=AXIS2_PLACEMENT_3D('',#72433,#53325,#53326);
#46920=AXIS2_PLACEMENT_3D('',#72434,#53327,#53328);
#46921=AXIS2_PLACEMENT_3D('',#72453,#53329,#53330);
#46922=AXIS2_PLACEMENT_3D('',#72454,#53331,#53332);
#46923=AXIS2_PLACEMENT_3D('',#72464,#53333,#53334);
#46924=AXIS2_PLACEMENT_3D('',#72484,#53336,#53337);
#46925=AXIS2_PLACEMENT_3D('',#72492,#53339,#53340);
#46926=AXIS2_PLACEMENT_3D('',#72495,#53341,#53342);
#46927=AXIS2_PLACEMENT_3D('',#72496,#53343,#53344);
#46928=AXIS2_PLACEMENT_3D('',#72497,#53345,#53346);
#46929=AXIS2_PLACEMENT_3D('',#72506,#53347,#53348);
#46930=AXIS2_PLACEMENT_3D('',#72507,#53349,#53350);
#46931=AXIS2_PLACEMENT_3D('',#72511,#53352,#53353);
#46932=AXIS2_PLACEMENT_3D('',#72513,#53354,#53355);
#46933=AXIS2_PLACEMENT_3D('',#72538,#53358,#53359);
#46934=AXIS2_PLACEMENT_3D('',#72539,#53360,#53361);
#46935=AXIS2_PLACEMENT_3D('',#72558,#53362,#53363);
#46936=AXIS2_PLACEMENT_3D('',#72566,#53365,#53366);
#46937=AXIS2_PLACEMENT_3D('',#72569,#53367,#53368);
#46938=AXIS2_PLACEMENT_3D('',#72570,#53369,#53370);
#46939=AXIS2_PLACEMENT_3D('',#72571,#53371,#53372);
#46940=AXIS2_PLACEMENT_3D('',#72583,#53373,#53374);
#46941=AXIS2_PLACEMENT_3D('',#72584,#53375,#53376);
#46942=AXIS2_PLACEMENT_3D('',#72588,#53378,#53379);
#46943=AXIS2_PLACEMENT_3D('',#72590,#53380,#53381);
#46944=AXIS2_PLACEMENT_3D('',#72626,#53384,#53385);
#46945=AXIS2_PLACEMENT_3D('',#72634,#53387,#53388);
#46946=AXIS2_PLACEMENT_3D('',#72637,#53389,#53390);
#46947=AXIS2_PLACEMENT_3D('',#72638,#53391,#53392);
#46948=AXIS2_PLACEMENT_3D('',#72639,#53393,#53394);
#46949=AXIS2_PLACEMENT_3D('',#72675,#53396,#53397);
#46950=AXIS2_PLACEMENT_3D('',#72677,#53398,#53399);
#46951=AXIS2_PLACEMENT_3D('',#72732,#53403,#53404);
#46952=AXIS2_PLACEMENT_3D('',#72735,#53405,#53406);
#46953=AXIS2_PLACEMENT_3D('',#72742,#53407,#53408);
#46954=AXIS2_PLACEMENT_3D('',#72754,#53409,#53410);
#46955=AXIS2_PLACEMENT_3D('',#72755,#53411,#53412);
#46956=AXIS2_PLACEMENT_3D('',#72759,#53414,#53415);
#46957=AXIS2_PLACEMENT_3D('',#72761,#53416,#53417);
#46958=AXIS2_PLACEMENT_3D('',#72797,#53420,#53421);
#46959=AXIS2_PLACEMENT_3D('',#72805,#53423,#53424);
#46960=AXIS2_PLACEMENT_3D('',#72808,#53425,#53426);
#46961=AXIS2_PLACEMENT_3D('',#72809,#53427,#53428);
#46962=AXIS2_PLACEMENT_3D('',#72810,#53429,#53430);
#46963=AXIS2_PLACEMENT_3D('',#72829,#53431,#53432);
#46964=AXIS2_PLACEMENT_3D('',#72830,#53433,#53434);
#46965=AXIS2_PLACEMENT_3D('',#72834,#53436,#53437);
#46966=AXIS2_PLACEMENT_3D('',#72836,#53438,#53439);
#46967=AXIS2_PLACEMENT_3D('',#72872,#53442,#53443);
#46968=AXIS2_PLACEMENT_3D('',#72880,#53445,#53446);
#46969=AXIS2_PLACEMENT_3D('',#72883,#53447,#53448);
#46970=AXIS2_PLACEMENT_3D('',#72884,#53449,#53450);
#46971=AXIS2_PLACEMENT_3D('',#72885,#53451,#53452);
#46972=AXIS2_PLACEMENT_3D('',#72900,#53453,#53454);
#46973=AXIS2_PLACEMENT_3D('',#72901,#53455,#53456);
#46974=AXIS2_PLACEMENT_3D('',#72905,#53458,#53459);
#46975=AXIS2_PLACEMENT_3D('',#72907,#53460,#53461);
#46976=AXIS2_PLACEMENT_3D('',#72941,#53464,#53465);
#46977=AXIS2_PLACEMENT_3D('',#72943,#53467,#53468);
#46978=AXIS2_PLACEMENT_3D('',#72944,#53469,#53470);
#46979=AXIS2_PLACEMENT_3D('',#72947,#53472,#53473);
#46980=AXIS2_PLACEMENT_3D('',#72948,#53474,#53475);
#46981=AXIS2_PLACEMENT_3D('',#72949,#53476,#53477);
#46982=AXIS2_PLACEMENT_3D('',#72968,#53478,#53479);
#46983=AXIS2_PLACEMENT_3D('',#72969,#53480,#53481);
#46984=AXIS2_PLACEMENT_3D('',#72979,#53482,#53483);
#46985=AXIS2_PLACEMENT_3D('',#72999,#53485,#53486);
#46986=AXIS2_PLACEMENT_3D('',#73007,#53488,#53489);
#46987=AXIS2_PLACEMENT_3D('',#73010,#53490,#53491);
#46988=AXIS2_PLACEMENT_3D('',#73011,#53492,#53493);
#46989=AXIS2_PLACEMENT_3D('',#73012,#53494,#53495);
#46990=AXIS2_PLACEMENT_3D('',#73021,#53496,#53497);
#46991=AXIS2_PLACEMENT_3D('',#73022,#53498,#53499);
#46992=AXIS2_PLACEMENT_3D('',#73026,#53501,#53502);
#46993=AXIS2_PLACEMENT_3D('',#73028,#53503,#53504);
#46994=AXIS2_PLACEMENT_3D('',#73053,#53507,#53508);
#46995=AXIS2_PLACEMENT_3D('',#73054,#53509,#53510);
#46996=AXIS2_PLACEMENT_3D('',#73073,#53511,#53512);
#46997=AXIS2_PLACEMENT_3D('',#73081,#53514,#53515);
#46998=AXIS2_PLACEMENT_3D('',#73084,#53516,#53517);
#46999=AXIS2_PLACEMENT_3D('',#73085,#53518,#53519);
#47000=AXIS2_PLACEMENT_3D('',#73086,#53520,#53521);
#47001=AXIS2_PLACEMENT_3D('',#73095,#53522,#53523);
#47002=AXIS2_PLACEMENT_3D('',#73096,#53524,#53525);
#47003=AXIS2_PLACEMENT_3D('',#73100,#53527,#53528);
#47004=AXIS2_PLACEMENT_3D('',#73102,#53529,#53530);
#47005=AXIS2_PLACEMENT_3D('',#73145,#53533,#53534);
#47006=AXIS2_PLACEMENT_3D('',#73153,#53536,#53537);
#47007=AXIS2_PLACEMENT_3D('',#73156,#53538,#53539);
#47008=AXIS2_PLACEMENT_3D('',#73157,#53540,#53541);
#47009=AXIS2_PLACEMENT_3D('',#73158,#53542,#53543);
#47010=AXIS2_PLACEMENT_3D('',#73194,#53545,#53546);
#47011=AXIS2_PLACEMENT_3D('',#73196,#53547,#53548);
#47012=AXIS2_PLACEMENT_3D('',#73251,#53552,#53553);
#47013=AXIS2_PLACEMENT_3D('',#73254,#53554,#53555);
#47014=AXIS2_PLACEMENT_3D('',#73261,#53556,#53557);
#47015=AXIS2_PLACEMENT_3D('',#73273,#53558,#53559);
#47016=AXIS2_PLACEMENT_3D('',#73274,#53560,#53561);
#47017=AXIS2_PLACEMENT_3D('',#73278,#53563,#53564);
#47018=AXIS2_PLACEMENT_3D('',#73280,#53565,#53566);
#47019=AXIS2_PLACEMENT_3D('',#73316,#53569,#53570);
#47020=AXIS2_PLACEMENT_3D('',#73324,#53572,#53573);
#47021=AXIS2_PLACEMENT_3D('',#73327,#53574,#53575);
#47022=AXIS2_PLACEMENT_3D('',#73328,#53576,#53577);
#47023=AXIS2_PLACEMENT_3D('',#73329,#53578,#53579);
#47024=AXIS2_PLACEMENT_3D('',#73348,#53580,#53581);
#47025=AXIS2_PLACEMENT_3D('',#73349,#53582,#53583);
#47026=AXIS2_PLACEMENT_3D('',#73353,#53585,#53586);
#47027=AXIS2_PLACEMENT_3D('',#73355,#53587,#53588);
#47028=AXIS2_PLACEMENT_3D('',#73391,#53591,#53592);
#47029=AXIS2_PLACEMENT_3D('',#73399,#53594,#53595);
#47030=AXIS2_PLACEMENT_3D('',#73402,#53596,#53597);
#47031=AXIS2_PLACEMENT_3D('',#73403,#53598,#53599);
#47032=AXIS2_PLACEMENT_3D('',#73404,#53600,#53601);
#47033=AXIS2_PLACEMENT_3D('',#73419,#53602,#53603);
#47034=AXIS2_PLACEMENT_3D('',#73420,#53604,#53605);
#47035=AXIS2_PLACEMENT_3D('',#73424,#53607,#53608);
#47036=AXIS2_PLACEMENT_3D('',#73426,#53609,#53610);
#47037=AXIS2_PLACEMENT_3D('',#73460,#53613,#53614);
#47038=AXIS2_PLACEMENT_3D('',#73462,#53616,#53617);
#47039=AXIS2_PLACEMENT_3D('',#73463,#53618,#53619);
#47040=AXIS2_PLACEMENT_3D('',#73466,#53621,#53622);
#47041=AXIS2_PLACEMENT_3D('',#73467,#53623,#53624);
#47042=AXIS2_PLACEMENT_3D('',#73468,#53625,#53626);
#47043=AXIS2_PLACEMENT_3D('',#73487,#53627,#53628);
#47044=AXIS2_PLACEMENT_3D('',#73488,#53629,#53630);
#47045=AXIS2_PLACEMENT_3D('',#73498,#53631,#53632);
#47046=AXIS2_PLACEMENT_3D('',#73518,#53634,#53635);
#47047=AXIS2_PLACEMENT_3D('',#73526,#53637,#53638);
#47048=AXIS2_PLACEMENT_3D('',#73529,#53639,#53640);
#47049=AXIS2_PLACEMENT_3D('',#73530,#53641,#53642);
#47050=AXIS2_PLACEMENT_3D('',#73531,#53643,#53644);
#47051=AXIS2_PLACEMENT_3D('',#73540,#53645,#53646);
#47052=AXIS2_PLACEMENT_3D('',#73541,#53647,#53648);
#47053=AXIS2_PLACEMENT_3D('',#73545,#53650,#53651);
#47054=AXIS2_PLACEMENT_3D('',#73547,#53652,#53653);
#47055=AXIS2_PLACEMENT_3D('',#73572,#53656,#53657);
#47056=AXIS2_PLACEMENT_3D('',#73573,#53658,#53659);
#47057=AXIS2_PLACEMENT_3D('',#73592,#53660,#53661);
#47058=AXIS2_PLACEMENT_3D('',#73600,#53663,#53664);
#47059=AXIS2_PLACEMENT_3D('',#73603,#53665,#53666);
#47060=AXIS2_PLACEMENT_3D('',#73604,#53667,#53668);
#47061=AXIS2_PLACEMENT_3D('',#73605,#53669,#53670);
#47062=AXIS2_PLACEMENT_3D('',#73617,#53671,#53672);
#47063=AXIS2_PLACEMENT_3D('',#73618,#53673,#53674);
#47064=AXIS2_PLACEMENT_3D('',#73622,#53676,#53677);
#47065=AXIS2_PLACEMENT_3D('',#73624,#53678,#53679);
#47066=AXIS2_PLACEMENT_3D('',#73660,#53682,#53683);
#47067=AXIS2_PLACEMENT_3D('',#73668,#53685,#53686);
#47068=AXIS2_PLACEMENT_3D('',#73671,#53687,#53688);
#47069=AXIS2_PLACEMENT_3D('',#73672,#53689,#53690);
#47070=AXIS2_PLACEMENT_3D('',#73673,#53691,#53692);
#47071=AXIS2_PLACEMENT_3D('',#73709,#53694,#53695);
#47072=AXIS2_PLACEMENT_3D('',#73711,#53696,#53697);
#47073=AXIS2_PLACEMENT_3D('',#73766,#53701,#53702);
#47074=AXIS2_PLACEMENT_3D('',#73769,#53703,#53704);
#47075=AXIS2_PLACEMENT_3D('',#73776,#53705,#53706);
#47076=AXIS2_PLACEMENT_3D('',#73788,#53707,#53708);
#47077=AXIS2_PLACEMENT_3D('',#73789,#53709,#53710);
#47078=AXIS2_PLACEMENT_3D('',#73793,#53712,#53713);
#47079=AXIS2_PLACEMENT_3D('',#73795,#53714,#53715);
#47080=AXIS2_PLACEMENT_3D('',#73831,#53718,#53719);
#47081=AXIS2_PLACEMENT_3D('',#73839,#53721,#53722);
#47082=AXIS2_PLACEMENT_3D('',#73842,#53723,#53724);
#47083=AXIS2_PLACEMENT_3D('',#73843,#53725,#53726);
#47084=AXIS2_PLACEMENT_3D('',#73844,#53727,#53728);
#47085=AXIS2_PLACEMENT_3D('',#73863,#53729,#53730);
#47086=AXIS2_PLACEMENT_3D('',#73864,#53731,#53732);
#47087=AXIS2_PLACEMENT_3D('',#73868,#53734,#53735);
#47088=AXIS2_PLACEMENT_3D('',#73870,#53736,#53737);
#47089=AXIS2_PLACEMENT_3D('',#73906,#53740,#53741);
#47090=AXIS2_PLACEMENT_3D('',#73914,#53743,#53744);
#47091=AXIS2_PLACEMENT_3D('',#73917,#53745,#53746);
#47092=AXIS2_PLACEMENT_3D('',#73918,#53747,#53748);
#47093=AXIS2_PLACEMENT_3D('',#73919,#53749,#53750);
#47094=AXIS2_PLACEMENT_3D('',#73934,#53751,#53752);
#47095=AXIS2_PLACEMENT_3D('',#73935,#53753,#53754);
#47096=AXIS2_PLACEMENT_3D('',#73939,#53756,#53757);
#47097=AXIS2_PLACEMENT_3D('',#73941,#53758,#53759);
#47098=AXIS2_PLACEMENT_3D('',#73975,#53762,#53763);
#47099=AXIS2_PLACEMENT_3D('',#73977,#53765,#53766);
#47100=AXIS2_PLACEMENT_3D('',#73978,#53767,#53768);
#47101=AXIS2_PLACEMENT_3D('',#73981,#53770,#53771);
#47102=AXIS2_PLACEMENT_3D('',#73982,#53772,#53773);
#47103=AXIS2_PLACEMENT_3D('',#73983,#53774,#53775);
#47104=AXIS2_PLACEMENT_3D('',#74002,#53776,#53777);
#47105=AXIS2_PLACEMENT_3D('',#74003,#53778,#53779);
#47106=AXIS2_PLACEMENT_3D('',#74013,#53780,#53781);
#47107=AXIS2_PLACEMENT_3D('',#74033,#53783,#53784);
#47108=AXIS2_PLACEMENT_3D('',#74041,#53786,#53787);
#47109=AXIS2_PLACEMENT_3D('',#74044,#53788,#53789);
#47110=AXIS2_PLACEMENT_3D('',#74045,#53790,#53791);
#47111=AXIS2_PLACEMENT_3D('',#74046,#53792,#53793);
#47112=AXIS2_PLACEMENT_3D('',#74055,#53794,#53795);
#47113=AXIS2_PLACEMENT_3D('',#74056,#53796,#53797);
#47114=AXIS2_PLACEMENT_3D('',#74060,#53799,#53800);
#47115=AXIS2_PLACEMENT_3D('',#74062,#53801,#53802);
#47116=AXIS2_PLACEMENT_3D('',#74087,#53805,#53806);
#47117=AXIS2_PLACEMENT_3D('',#74088,#53807,#53808);
#47118=AXIS2_PLACEMENT_3D('',#74107,#53809,#53810);
#47119=AXIS2_PLACEMENT_3D('',#74115,#53812,#53813);
#47120=AXIS2_PLACEMENT_3D('',#74118,#53814,#53815);
#47121=AXIS2_PLACEMENT_3D('',#74119,#53816,#53817);
#47122=AXIS2_PLACEMENT_3D('',#74120,#53818,#53819);
#47123=AXIS2_PLACEMENT_3D('',#74132,#53820,#53821);
#47124=AXIS2_PLACEMENT_3D('',#74133,#53822,#53823);
#47125=AXIS2_PLACEMENT_3D('',#74137,#53825,#53826);
#47126=AXIS2_PLACEMENT_3D('',#74139,#53827,#53828);
#47127=AXIS2_PLACEMENT_3D('',#74175,#53831,#53832);
#47128=AXIS2_PLACEMENT_3D('',#74183,#53834,#53835);
#47129=AXIS2_PLACEMENT_3D('',#74186,#53836,#53837);
#47130=AXIS2_PLACEMENT_3D('',#74187,#53838,#53839);
#47131=AXIS2_PLACEMENT_3D('',#74188,#53840,#53841);
#47132=AXIS2_PLACEMENT_3D('',#74224,#53843,#53844);
#47133=AXIS2_PLACEMENT_3D('',#74226,#53845,#53846);
#47134=AXIS2_PLACEMENT_3D('',#74281,#53850,#53851);
#47135=AXIS2_PLACEMENT_3D('',#74284,#53852,#53853);
#47136=AXIS2_PLACEMENT_3D('',#74291,#53854,#53855);
#47137=AXIS2_PLACEMENT_3D('',#74303,#53856,#53857);
#47138=AXIS2_PLACEMENT_3D('',#74304,#53858,#53859);
#47139=AXIS2_PLACEMENT_3D('',#74308,#53861,#53862);
#47140=AXIS2_PLACEMENT_3D('',#74310,#53863,#53864);
#47141=AXIS2_PLACEMENT_3D('',#74346,#53867,#53868);
#47142=AXIS2_PLACEMENT_3D('',#74354,#53870,#53871);
#47143=AXIS2_PLACEMENT_3D('',#74357,#53872,#53873);
#47144=AXIS2_PLACEMENT_3D('',#74358,#53874,#53875);
#47145=AXIS2_PLACEMENT_3D('',#74359,#53876,#53877);
#47146=AXIS2_PLACEMENT_3D('',#74378,#53878,#53879);
#47147=AXIS2_PLACEMENT_3D('',#74379,#53880,#53881);
#47148=AXIS2_PLACEMENT_3D('',#74383,#53883,#53884);
#47149=AXIS2_PLACEMENT_3D('',#74385,#53885,#53886);
#47150=AXIS2_PLACEMENT_3D('',#74421,#53889,#53890);
#47151=AXIS2_PLACEMENT_3D('',#74429,#53892,#53893);
#47152=AXIS2_PLACEMENT_3D('',#74432,#53894,#53895);
#47153=AXIS2_PLACEMENT_3D('',#74433,#53896,#53897);
#47154=AXIS2_PLACEMENT_3D('',#74434,#53898,#53899);
#47155=AXIS2_PLACEMENT_3D('',#74449,#53900,#53901);
#47156=AXIS2_PLACEMENT_3D('',#74450,#53902,#53903);
#47157=AXIS2_PLACEMENT_3D('',#74454,#53905,#53906);
#47158=AXIS2_PLACEMENT_3D('',#74456,#53907,#53908);
#47159=AXIS2_PLACEMENT_3D('',#74490,#53911,#53912);
#47160=AXIS2_PLACEMENT_3D('',#74492,#53914,#53915);
#47161=AXIS2_PLACEMENT_3D('',#74493,#53916,#53917);
#47162=AXIS2_PLACEMENT_3D('',#74496,#53919,#53920);
#47163=AXIS2_PLACEMENT_3D('',#74497,#53921,#53922);
#47164=AXIS2_PLACEMENT_3D('',#74498,#53923,#53924);
#47165=AXIS2_PLACEMENT_3D('',#74517,#53925,#53926);
#47166=AXIS2_PLACEMENT_3D('',#74518,#53927,#53928);
#47167=AXIS2_PLACEMENT_3D('',#74528,#53929,#53930);
#47168=AXIS2_PLACEMENT_3D('',#74548,#53932,#53933);
#47169=AXIS2_PLACEMENT_3D('',#74556,#53935,#53936);
#47170=AXIS2_PLACEMENT_3D('',#74559,#53937,#53938);
#47171=AXIS2_PLACEMENT_3D('',#74560,#53939,#53940);
#47172=AXIS2_PLACEMENT_3D('',#74561,#53941,#53942);
#47173=AXIS2_PLACEMENT_3D('',#74570,#53943,#53944);
#47174=AXIS2_PLACEMENT_3D('',#74571,#53945,#53946);
#47175=AXIS2_PLACEMENT_3D('',#74575,#53948,#53949);
#47176=AXIS2_PLACEMENT_3D('',#74577,#53950,#53951);
#47177=AXIS2_PLACEMENT_3D('',#74602,#53954,#53955);
#47178=AXIS2_PLACEMENT_3D('',#74603,#53956,#53957);
#47179=AXIS2_PLACEMENT_3D('',#74622,#53958,#53959);
#47180=AXIS2_PLACEMENT_3D('',#74630,#53961,#53962);
#47181=AXIS2_PLACEMENT_3D('',#74633,#53963,#53964);
#47182=AXIS2_PLACEMENT_3D('',#74634,#53965,#53966);
#47183=AXIS2_PLACEMENT_3D('',#74635,#53967,#53968);
#47184=AXIS2_PLACEMENT_3D('',#74647,#53969,#53970);
#47185=AXIS2_PLACEMENT_3D('',#74648,#53971,#53972);
#47186=AXIS2_PLACEMENT_3D('',#74652,#53974,#53975);
#47187=AXIS2_PLACEMENT_3D('',#74654,#53976,#53977);
#47188=AXIS2_PLACEMENT_3D('',#74690,#53980,#53981);
#47189=AXIS2_PLACEMENT_3D('',#74698,#53983,#53984);
#47190=AXIS2_PLACEMENT_3D('',#74701,#53985,#53986);
#47191=AXIS2_PLACEMENT_3D('',#74702,#53987,#53988);
#47192=AXIS2_PLACEMENT_3D('',#74703,#53989,#53990);
#47193=AXIS2_PLACEMENT_3D('',#74739,#53992,#53993);
#47194=AXIS2_PLACEMENT_3D('',#74741,#53994,#53995);
#47195=AXIS2_PLACEMENT_3D('',#74796,#53999,#54000);
#47196=AXIS2_PLACEMENT_3D('',#74799,#54001,#54002);
#47197=AXIS2_PLACEMENT_3D('',#74806,#54003,#54004);
#47198=AXIS2_PLACEMENT_3D('',#74818,#54005,#54006);
#47199=AXIS2_PLACEMENT_3D('',#74819,#54007,#54008);
#47200=AXIS2_PLACEMENT_3D('',#74823,#54010,#54011);
#47201=AXIS2_PLACEMENT_3D('',#74825,#54012,#54013);
#47202=AXIS2_PLACEMENT_3D('',#74861,#54016,#54017);
#47203=AXIS2_PLACEMENT_3D('',#74869,#54019,#54020);
#47204=AXIS2_PLACEMENT_3D('',#74872,#54021,#54022);
#47205=AXIS2_PLACEMENT_3D('',#74873,#54023,#54024);
#47206=AXIS2_PLACEMENT_3D('',#74874,#54025,#54026);
#47207=AXIS2_PLACEMENT_3D('',#74893,#54027,#54028);
#47208=AXIS2_PLACEMENT_3D('',#74894,#54029,#54030);
#47209=AXIS2_PLACEMENT_3D('',#74898,#54032,#54033);
#47210=AXIS2_PLACEMENT_3D('',#74900,#54034,#54035);
#47211=AXIS2_PLACEMENT_3D('',#74936,#54038,#54039);
#47212=AXIS2_PLACEMENT_3D('',#74944,#54041,#54042);
#47213=AXIS2_PLACEMENT_3D('',#74947,#54043,#54044);
#47214=AXIS2_PLACEMENT_3D('',#74948,#54045,#54046);
#47215=AXIS2_PLACEMENT_3D('',#74949,#54047,#54048);
#47216=AXIS2_PLACEMENT_3D('',#74964,#54049,#54050);
#47217=AXIS2_PLACEMENT_3D('',#74965,#54051,#54052);
#47218=AXIS2_PLACEMENT_3D('',#74969,#54054,#54055);
#47219=AXIS2_PLACEMENT_3D('',#74971,#54056,#54057);
#47220=AXIS2_PLACEMENT_3D('',#75005,#54060,#54061);
#47221=AXIS2_PLACEMENT_3D('',#75007,#54063,#54064);
#47222=AXIS2_PLACEMENT_3D('',#75008,#54065,#54066);
#47223=AXIS2_PLACEMENT_3D('',#75011,#54068,#54069);
#47224=AXIS2_PLACEMENT_3D('',#75012,#54070,#54071);
#47225=AXIS2_PLACEMENT_3D('',#75013,#54072,#54073);
#47226=AXIS2_PLACEMENT_3D('',#75032,#54074,#54075);
#47227=AXIS2_PLACEMENT_3D('',#75033,#54076,#54077);
#47228=AXIS2_PLACEMENT_3D('',#75043,#54078,#54079);
#47229=AXIS2_PLACEMENT_3D('',#75063,#54081,#54082);
#47230=AXIS2_PLACEMENT_3D('',#75071,#54084,#54085);
#47231=AXIS2_PLACEMENT_3D('',#75074,#54086,#54087);
#47232=AXIS2_PLACEMENT_3D('',#75075,#54088,#54089);
#47233=AXIS2_PLACEMENT_3D('',#75076,#54090,#54091);
#47234=AXIS2_PLACEMENT_3D('',#75085,#54092,#54093);
#47235=AXIS2_PLACEMENT_3D('',#75086,#54094,#54095);
#47236=AXIS2_PLACEMENT_3D('',#75090,#54097,#54098);
#47237=AXIS2_PLACEMENT_3D('',#75092,#54099,#54100);
#47238=AXIS2_PLACEMENT_3D('',#75117,#54103,#54104);
#47239=AXIS2_PLACEMENT_3D('',#75118,#54105,#54106);
#47240=AXIS2_PLACEMENT_3D('',#75137,#54107,#54108);
#47241=AXIS2_PLACEMENT_3D('',#75145,#54110,#54111);
#47242=AXIS2_PLACEMENT_3D('',#75148,#54112,#54113);
#47243=AXIS2_PLACEMENT_3D('',#75149,#54114,#54115);
#47244=AXIS2_PLACEMENT_3D('',#75150,#54116,#54117);
#47245=AXIS2_PLACEMENT_3D('',#75162,#54118,#54119);
#47246=AXIS2_PLACEMENT_3D('',#75163,#54120,#54121);
#47247=AXIS2_PLACEMENT_3D('',#75167,#54123,#54124);
#47248=AXIS2_PLACEMENT_3D('',#75169,#54125,#54126);
#47249=AXIS2_PLACEMENT_3D('',#75205,#54129,#54130);
#47250=AXIS2_PLACEMENT_3D('',#75213,#54132,#54133);
#47251=AXIS2_PLACEMENT_3D('',#75216,#54134,#54135);
#47252=AXIS2_PLACEMENT_3D('',#75217,#54136,#54137);
#47253=AXIS2_PLACEMENT_3D('',#75218,#54138,#54139);
#47254=AXIS2_PLACEMENT_3D('',#75254,#54141,#54142);
#47255=AXIS2_PLACEMENT_3D('',#75256,#54143,#54144);
#47256=AXIS2_PLACEMENT_3D('',#75311,#54148,#54149);
#47257=AXIS2_PLACEMENT_3D('',#75314,#54150,#54151);
#47258=AXIS2_PLACEMENT_3D('',#75321,#54152,#54153);
#47259=AXIS2_PLACEMENT_3D('',#75333,#54154,#54155);
#47260=AXIS2_PLACEMENT_3D('',#75334,#54156,#54157);
#47261=AXIS2_PLACEMENT_3D('',#75338,#54159,#54160);
#47262=AXIS2_PLACEMENT_3D('',#75340,#54161,#54162);
#47263=AXIS2_PLACEMENT_3D('',#75376,#54165,#54166);
#47264=AXIS2_PLACEMENT_3D('',#75384,#54168,#54169);
#47265=AXIS2_PLACEMENT_3D('',#75387,#54170,#54171);
#47266=AXIS2_PLACEMENT_3D('',#75388,#54172,#54173);
#47267=AXIS2_PLACEMENT_3D('',#75389,#54174,#54175);
#47268=AXIS2_PLACEMENT_3D('',#75408,#54176,#54177);
#47269=AXIS2_PLACEMENT_3D('',#75409,#54178,#54179);
#47270=AXIS2_PLACEMENT_3D('',#75413,#54181,#54182);
#47271=AXIS2_PLACEMENT_3D('',#75415,#54183,#54184);
#47272=AXIS2_PLACEMENT_3D('',#75451,#54187,#54188);
#47273=AXIS2_PLACEMENT_3D('',#75459,#54190,#54191);
#47274=AXIS2_PLACEMENT_3D('',#75462,#54192,#54193);
#47275=AXIS2_PLACEMENT_3D('',#75463,#54194,#54195);
#47276=AXIS2_PLACEMENT_3D('',#75464,#54196,#54197);
#47277=AXIS2_PLACEMENT_3D('',#75479,#54198,#54199);
#47278=AXIS2_PLACEMENT_3D('',#75480,#54200,#54201);
#47279=AXIS2_PLACEMENT_3D('',#75484,#54203,#54204);
#47280=AXIS2_PLACEMENT_3D('',#75486,#54205,#54206);
#47281=AXIS2_PLACEMENT_3D('',#75520,#54209,#54210);
#47282=AXIS2_PLACEMENT_3D('',#75522,#54212,#54213);
#47283=AXIS2_PLACEMENT_3D('',#75523,#54214,#54215);
#47284=AXIS2_PLACEMENT_3D('',#75526,#54217,#54218);
#47285=AXIS2_PLACEMENT_3D('',#75527,#54219,#54220);
#47286=AXIS2_PLACEMENT_3D('',#75528,#54221,#54222);
#47287=AXIS2_PLACEMENT_3D('',#75547,#54223,#54224);
#47288=AXIS2_PLACEMENT_3D('',#75548,#54225,#54226);
#47289=AXIS2_PLACEMENT_3D('',#75558,#54227,#54228);
#47290=AXIS2_PLACEMENT_3D('',#75578,#54230,#54231);
#47291=AXIS2_PLACEMENT_3D('',#75586,#54233,#54234);
#47292=AXIS2_PLACEMENT_3D('',#75589,#54235,#54236);
#47293=AXIS2_PLACEMENT_3D('',#75590,#54237,#54238);
#47294=AXIS2_PLACEMENT_3D('',#75591,#54239,#54240);
#47295=AXIS2_PLACEMENT_3D('',#75600,#54241,#54242);
#47296=AXIS2_PLACEMENT_3D('',#75601,#54243,#54244);
#47297=AXIS2_PLACEMENT_3D('',#75605,#54246,#54247);
#47298=AXIS2_PLACEMENT_3D('',#75607,#54248,#54249);
#47299=AXIS2_PLACEMENT_3D('',#75632,#54252,#54253);
#47300=AXIS2_PLACEMENT_3D('',#75633,#54254,#54255);
#47301=AXIS2_PLACEMENT_3D('',#75652,#54256,#54257);
#47302=AXIS2_PLACEMENT_3D('',#75660,#54259,#54260);
#47303=AXIS2_PLACEMENT_3D('',#75663,#54261,#54262);
#47304=AXIS2_PLACEMENT_3D('',#75664,#54263,#54264);
#47305=AXIS2_PLACEMENT_3D('',#75665,#54265,#54266);
#47306=AXIS2_PLACEMENT_3D('',#75674,#54267,#54268);
#47307=AXIS2_PLACEMENT_3D('',#75675,#54269,#54270);
#47308=AXIS2_PLACEMENT_3D('',#75679,#54272,#54273);
#47309=AXIS2_PLACEMENT_3D('',#75681,#54274,#54275);
#47310=AXIS2_PLACEMENT_3D('',#75724,#54278,#54279);
#47311=AXIS2_PLACEMENT_3D('',#75732,#54281,#54282);
#47312=AXIS2_PLACEMENT_3D('',#75735,#54283,#54284);
#47313=AXIS2_PLACEMENT_3D('',#75736,#54285,#54286);
#47314=AXIS2_PLACEMENT_3D('',#75737,#54287,#54288);
#47315=AXIS2_PLACEMENT_3D('',#75773,#54290,#54291);
#47316=AXIS2_PLACEMENT_3D('',#75775,#54292,#54293);
#47317=AXIS2_PLACEMENT_3D('',#75830,#54297,#54298);
#47318=AXIS2_PLACEMENT_3D('',#75833,#54299,#54300);
#47319=AXIS2_PLACEMENT_3D('',#75840,#54301,#54302);
#47320=AXIS2_PLACEMENT_3D('',#75852,#54303,#54304);
#47321=AXIS2_PLACEMENT_3D('',#75853,#54305,#54306);
#47322=AXIS2_PLACEMENT_3D('',#75857,#54308,#54309);
#47323=AXIS2_PLACEMENT_3D('',#75859,#54310,#54311);
#47324=AXIS2_PLACEMENT_3D('',#75895,#54314,#54315);
#47325=AXIS2_PLACEMENT_3D('',#75903,#54317,#54318);
#47326=AXIS2_PLACEMENT_3D('',#75906,#54319,#54320);
#47327=AXIS2_PLACEMENT_3D('',#75907,#54321,#54322);
#47328=AXIS2_PLACEMENT_3D('',#75908,#54323,#54324);
#47329=AXIS2_PLACEMENT_3D('',#75927,#54325,#54326);
#47330=AXIS2_PLACEMENT_3D('',#75928,#54327,#54328);
#47331=AXIS2_PLACEMENT_3D('',#75932,#54330,#54331);
#47332=AXIS2_PLACEMENT_3D('',#75934,#54332,#54333);
#47333=AXIS2_PLACEMENT_3D('',#75970,#54336,#54337);
#47334=AXIS2_PLACEMENT_3D('',#75978,#54339,#54340);
#47335=AXIS2_PLACEMENT_3D('',#75981,#54341,#54342);
#47336=AXIS2_PLACEMENT_3D('',#75982,#54343,#54344);
#47337=AXIS2_PLACEMENT_3D('',#75983,#54345,#54346);
#47338=AXIS2_PLACEMENT_3D('',#75998,#54347,#54348);
#47339=AXIS2_PLACEMENT_3D('',#75999,#54349,#54350);
#47340=AXIS2_PLACEMENT_3D('',#76003,#54352,#54353);
#47341=AXIS2_PLACEMENT_3D('',#76005,#54354,#54355);
#47342=AXIS2_PLACEMENT_3D('',#76039,#54358,#54359);
#47343=AXIS2_PLACEMENT_3D('',#76041,#54361,#54362);
#47344=AXIS2_PLACEMENT_3D('',#76042,#54363,#54364);
#47345=AXIS2_PLACEMENT_3D('',#76045,#54366,#54367);
#47346=AXIS2_PLACEMENT_3D('',#76046,#54368,#54369);
#47347=AXIS2_PLACEMENT_3D('',#76047,#54370,#54371);
#47348=AXIS2_PLACEMENT_3D('',#76066,#54372,#54373);
#47349=AXIS2_PLACEMENT_3D('',#76067,#54374,#54375);
#47350=AXIS2_PLACEMENT_3D('',#76077,#54376,#54377);
#47351=AXIS2_PLACEMENT_3D('',#76097,#54379,#54380);
#47352=AXIS2_PLACEMENT_3D('',#76105,#54382,#54383);
#47353=AXIS2_PLACEMENT_3D('',#76108,#54384,#54385);
#47354=AXIS2_PLACEMENT_3D('',#76109,#54386,#54387);
#47355=AXIS2_PLACEMENT_3D('',#76110,#54388,#54389);
#47356=AXIS2_PLACEMENT_3D('',#76119,#54390,#54391);
#47357=AXIS2_PLACEMENT_3D('',#76120,#54392,#54393);
#47358=AXIS2_PLACEMENT_3D('',#76124,#54395,#54396);
#47359=AXIS2_PLACEMENT_3D('',#76126,#54397,#54398);
#47360=AXIS2_PLACEMENT_3D('',#76151,#54401,#54402);
#47361=AXIS2_PLACEMENT_3D('',#76152,#54403,#54404);
#47362=AXIS2_PLACEMENT_3D('',#76171,#54405,#54406);
#47363=AXIS2_PLACEMENT_3D('',#76179,#54408,#54409);
#47364=AXIS2_PLACEMENT_3D('',#76182,#54410,#54411);
#47365=AXIS2_PLACEMENT_3D('',#76183,#54412,#54413);
#47366=AXIS2_PLACEMENT_3D('',#76184,#54414,#54415);
#47367=AXIS2_PLACEMENT_3D('',#76196,#54416,#54417);
#47368=AXIS2_PLACEMENT_3D('',#76197,#54418,#54419);
#47369=AXIS2_PLACEMENT_3D('',#76201,#54421,#54422);
#47370=AXIS2_PLACEMENT_3D('',#76203,#54423,#54424);
#47371=AXIS2_PLACEMENT_3D('',#76239,#54427,#54428);
#47372=AXIS2_PLACEMENT_3D('',#76247,#54430,#54431);
#47373=AXIS2_PLACEMENT_3D('',#76250,#54432,#54433);
#47374=AXIS2_PLACEMENT_3D('',#76251,#54434,#54435);
#47375=AXIS2_PLACEMENT_3D('',#76252,#54436,#54437);
#47376=AXIS2_PLACEMENT_3D('',#76287,#54439,#54440);
#47377=AXIS2_PLACEMENT_3D('',#76289,#54441,#54442);
#47378=AXIS2_PLACEMENT_3D('',#76339,#54446,#54447);
#47379=AXIS2_PLACEMENT_3D('',#76342,#54448,#54449);
#47380=AXIS2_PLACEMENT_3D('',#76349,#54450,#54451);
#47381=AXIS2_PLACEMENT_3D('',#76361,#54452,#54453);
#47382=AXIS2_PLACEMENT_3D('',#76362,#54454,#54455);
#47383=AXIS2_PLACEMENT_3D('',#76366,#54457,#54458);
#47384=AXIS2_PLACEMENT_3D('',#76368,#54459,#54460);
#47385=AXIS2_PLACEMENT_3D('',#76404,#54463,#54464);
#47386=AXIS2_PLACEMENT_3D('',#76412,#54466,#54467);
#47387=AXIS2_PLACEMENT_3D('',#76415,#54468,#54469);
#47388=AXIS2_PLACEMENT_3D('',#76416,#54470,#54471);
#47389=AXIS2_PLACEMENT_3D('',#76417,#54472,#54473);
#47390=AXIS2_PLACEMENT_3D('',#76436,#54474,#54475);
#47391=AXIS2_PLACEMENT_3D('',#76437,#54476,#54477);
#47392=AXIS2_PLACEMENT_3D('',#76441,#54479,#54480);
#47393=AXIS2_PLACEMENT_3D('',#76443,#54481,#54482);
#47394=AXIS2_PLACEMENT_3D('',#76479,#54485,#54486);
#47395=AXIS2_PLACEMENT_3D('',#76487,#54488,#54489);
#47396=AXIS2_PLACEMENT_3D('',#76490,#54490,#54491);
#47397=AXIS2_PLACEMENT_3D('',#76491,#54492,#54493);
#47398=AXIS2_PLACEMENT_3D('',#76492,#54494,#54495);
#47399=AXIS2_PLACEMENT_3D('',#76507,#54496,#54497);
#47400=AXIS2_PLACEMENT_3D('',#76508,#54498,#54499);
#47401=AXIS2_PLACEMENT_3D('',#76512,#54501,#54502);
#47402=AXIS2_PLACEMENT_3D('',#76514,#54503,#54504);
#47403=AXIS2_PLACEMENT_3D('',#76548,#54507,#54508);
#47404=AXIS2_PLACEMENT_3D('',#76550,#54510,#54511);
#47405=AXIS2_PLACEMENT_3D('',#76551,#54512,#54513);
#47406=AXIS2_PLACEMENT_3D('',#76554,#54515,#54516);
#47407=AXIS2_PLACEMENT_3D('',#76555,#54517,#54518);
#47408=AXIS2_PLACEMENT_3D('',#76556,#54519,#54520);
#47409=AXIS2_PLACEMENT_3D('',#76575,#54521,#54522);
#47410=AXIS2_PLACEMENT_3D('',#76576,#54523,#54524);
#47411=AXIS2_PLACEMENT_3D('',#76586,#54525,#54526);
#47412=AXIS2_PLACEMENT_3D('',#76606,#54528,#54529);
#47413=AXIS2_PLACEMENT_3D('',#76614,#54531,#54532);
#47414=AXIS2_PLACEMENT_3D('',#76617,#54533,#54534);
#47415=AXIS2_PLACEMENT_3D('',#76618,#54535,#54536);
#47416=AXIS2_PLACEMENT_3D('',#76619,#54537,#54538);
#47417=AXIS2_PLACEMENT_3D('',#76628,#54539,#54540);
#47418=AXIS2_PLACEMENT_3D('',#76629,#54541,#54542);
#47419=AXIS2_PLACEMENT_3D('',#76633,#54544,#54545);
#47420=AXIS2_PLACEMENT_3D('',#76635,#54546,#54547);
#47421=AXIS2_PLACEMENT_3D('',#76660,#54550,#54551);
#47422=AXIS2_PLACEMENT_3D('',#76661,#54552,#54553);
#47423=AXIS2_PLACEMENT_3D('',#76680,#54554,#54555);
#47424=AXIS2_PLACEMENT_3D('',#76688,#54557,#54558);
#47425=AXIS2_PLACEMENT_3D('',#76691,#54559,#54560);
#47426=AXIS2_PLACEMENT_3D('',#76692,#54561,#54562);
#47427=AXIS2_PLACEMENT_3D('',#76693,#54563,#54564);
#47428=AXIS2_PLACEMENT_3D('',#76702,#54565,#54566);
#47429=AXIS2_PLACEMENT_3D('',#76703,#54567,#54568);
#47430=AXIS2_PLACEMENT_3D('',#76707,#54570,#54571);
#47431=AXIS2_PLACEMENT_3D('',#76709,#54572,#54573);
#47432=AXIS2_PLACEMENT_3D('',#76752,#54576,#54577);
#47433=AXIS2_PLACEMENT_3D('',#76760,#54579,#54580);
#47434=AXIS2_PLACEMENT_3D('',#76763,#54581,#54582);
#47435=AXIS2_PLACEMENT_3D('',#76764,#54583,#54584);
#47436=AXIS2_PLACEMENT_3D('',#76765,#54585,#54586);
#47437=AXIS2_PLACEMENT_3D('',#76801,#54588,#54589);
#47438=AXIS2_PLACEMENT_3D('',#76803,#54590,#54591);
#47439=AXIS2_PLACEMENT_3D('',#76858,#54595,#54596);
#47440=AXIS2_PLACEMENT_3D('',#76861,#54597,#54598);
#47441=AXIS2_PLACEMENT_3D('',#76868,#54599,#54600);
#47442=AXIS2_PLACEMENT_3D('',#76877,#54601,#54602);
#47443=AXIS2_PLACEMENT_3D('',#76878,#54603,#54604);
#47444=AXIS2_PLACEMENT_3D('',#76882,#54606,#54607);
#47445=AXIS2_PLACEMENT_3D('',#76884,#54608,#54609);
#47446=AXIS2_PLACEMENT_3D('',#76927,#54612,#54613);
#47447=AXIS2_PLACEMENT_3D('',#76935,#54615,#54616);
#47448=AXIS2_PLACEMENT_3D('',#76938,#54617,#54618);
#47449=AXIS2_PLACEMENT_3D('',#76939,#54619,#54620);
#47450=AXIS2_PLACEMENT_3D('',#76940,#54621,#54622);
#47451=AXIS2_PLACEMENT_3D('',#76959,#54623,#54624);
#47452=AXIS2_PLACEMENT_3D('',#76960,#54625,#54626);
#47453=AXIS2_PLACEMENT_3D('',#76964,#54628,#54629);
#47454=AXIS2_PLACEMENT_3D('',#76966,#54630,#54631);
#47455=AXIS2_PLACEMENT_3D('',#77002,#54634,#54635);
#47456=AXIS2_PLACEMENT_3D('',#77010,#54637,#54638);
#47457=AXIS2_PLACEMENT_3D('',#77013,#54639,#54640);
#47458=AXIS2_PLACEMENT_3D('',#77014,#54641,#54642);
#47459=AXIS2_PLACEMENT_3D('',#77015,#54643,#54644);
#47460=AXIS2_PLACEMENT_3D('',#77030,#54645,#54646);
#47461=AXIS2_PLACEMENT_3D('',#77031,#54647,#54648);
#47462=AXIS2_PLACEMENT_3D('',#77035,#54650,#54651);
#47463=AXIS2_PLACEMENT_3D('',#77037,#54652,#54653);
#47464=AXIS2_PLACEMENT_3D('',#77071,#54656,#54657);
#47465=AXIS2_PLACEMENT_3D('',#77073,#54659,#54660);
#47466=AXIS2_PLACEMENT_3D('',#77074,#54661,#54662);
#47467=AXIS2_PLACEMENT_3D('',#77077,#54664,#54665);
#47468=AXIS2_PLACEMENT_3D('',#77078,#54666,#54667);
#47469=AXIS2_PLACEMENT_3D('',#77079,#54668,#54669);
#47470=AXIS2_PLACEMENT_3D('',#77098,#54670,#54671);
#47471=AXIS2_PLACEMENT_3D('',#77099,#54672,#54673);
#47472=AXIS2_PLACEMENT_3D('',#77109,#54674,#54675);
#47473=AXIS2_PLACEMENT_3D('',#77129,#54677,#54678);
#47474=AXIS2_PLACEMENT_3D('',#77137,#54680,#54681);
#47475=AXIS2_PLACEMENT_3D('',#77140,#54682,#54683);
#47476=AXIS2_PLACEMENT_3D('',#77141,#54684,#54685);
#47477=AXIS2_PLACEMENT_3D('',#77142,#54686,#54687);
#47478=AXIS2_PLACEMENT_3D('',#77151,#54688,#54689);
#47479=AXIS2_PLACEMENT_3D('',#77152,#54690,#54691);
#47480=AXIS2_PLACEMENT_3D('',#77156,#54693,#54694);
#47481=AXIS2_PLACEMENT_3D('',#77158,#54695,#54696);
#47482=AXIS2_PLACEMENT_3D('',#77183,#54699,#54700);
#47483=AXIS2_PLACEMENT_3D('',#77184,#54701,#54702);
#47484=AXIS2_PLACEMENT_3D('',#77203,#54703,#54704);
#47485=AXIS2_PLACEMENT_3D('',#77211,#54706,#54707);
#47486=AXIS2_PLACEMENT_3D('',#77214,#54708,#54709);
#47487=AXIS2_PLACEMENT_3D('',#77215,#54710,#54711);
#47488=AXIS2_PLACEMENT_3D('',#77216,#54712,#54713);
#47489=AXIS2_PLACEMENT_3D('',#77228,#54714,#54715);
#47490=AXIS2_PLACEMENT_3D('',#77229,#54716,#54717);
#47491=AXIS2_PLACEMENT_3D('',#77233,#54719,#54720);
#47492=AXIS2_PLACEMENT_3D('',#77235,#54721,#54722);
#47493=AXIS2_PLACEMENT_3D('',#77271,#54725,#54726);
#47494=AXIS2_PLACEMENT_3D('',#77279,#54728,#54729);
#47495=AXIS2_PLACEMENT_3D('',#77282,#54730,#54731);
#47496=AXIS2_PLACEMENT_3D('',#77283,#54732,#54733);
#47497=AXIS2_PLACEMENT_3D('',#77284,#54734,#54735);
#47498=AXIS2_PLACEMENT_3D('',#77320,#54737,#54738);
#47499=AXIS2_PLACEMENT_3D('',#77322,#54739,#54740);
#47500=AXIS2_PLACEMENT_3D('',#77377,#54744,#54745);
#47501=AXIS2_PLACEMENT_3D('',#77380,#54746,#54747);
#47502=AXIS2_PLACEMENT_3D('',#77387,#54748,#54749);
#47503=AXIS2_PLACEMENT_3D('',#77399,#54750,#54751);
#47504=AXIS2_PLACEMENT_3D('',#77400,#54752,#54753);
#47505=AXIS2_PLACEMENT_3D('',#77404,#54755,#54756);
#47506=AXIS2_PLACEMENT_3D('',#77406,#54757,#54758);
#47507=AXIS2_PLACEMENT_3D('',#77442,#54761,#54762);
#47508=AXIS2_PLACEMENT_3D('',#77450,#54764,#54765);
#47509=AXIS2_PLACEMENT_3D('',#77453,#54766,#54767);
#47510=AXIS2_PLACEMENT_3D('',#77454,#54768,#54769);
#47511=AXIS2_PLACEMENT_3D('',#77455,#54770,#54771);
#47512=AXIS2_PLACEMENT_3D('',#77474,#54772,#54773);
#47513=AXIS2_PLACEMENT_3D('',#77475,#54774,#54775);
#47514=AXIS2_PLACEMENT_3D('',#77479,#54777,#54778);
#47515=AXIS2_PLACEMENT_3D('',#77481,#54779,#54780);
#47516=AXIS2_PLACEMENT_3D('',#77524,#54783,#54784);
#47517=AXIS2_PLACEMENT_3D('',#77532,#54786,#54787);
#47518=AXIS2_PLACEMENT_3D('',#77535,#54788,#54789);
#47519=AXIS2_PLACEMENT_3D('',#77536,#54790,#54791);
#47520=AXIS2_PLACEMENT_3D('',#77537,#54792,#54793);
#47521=AXIS2_PLACEMENT_3D('',#77552,#54794,#54795);
#47522=AXIS2_PLACEMENT_3D('',#77553,#54796,#54797);
#47523=AXIS2_PLACEMENT_3D('',#77557,#54799,#54800);
#47524=AXIS2_PLACEMENT_3D('',#77559,#54801,#54802);
#47525=AXIS2_PLACEMENT_3D('',#77593,#54805,#54806);
#47526=AXIS2_PLACEMENT_3D('',#77595,#54808,#54809);
#47527=AXIS2_PLACEMENT_3D('',#77596,#54810,#54811);
#47528=AXIS2_PLACEMENT_3D('',#77599,#54813,#54814);
#47529=AXIS2_PLACEMENT_3D('',#77600,#54815,#54816);
#47530=AXIS2_PLACEMENT_3D('',#77601,#54817,#54818);
#47531=AXIS2_PLACEMENT_3D('',#77620,#54819,#54820);
#47532=AXIS2_PLACEMENT_3D('',#77621,#54821,#54822);
#47533=AXIS2_PLACEMENT_3D('',#77631,#54823,#54824);
#47534=AXIS2_PLACEMENT_3D('',#77651,#54826,#54827);
#47535=AXIS2_PLACEMENT_3D('',#77659,#54829,#54830);
#47536=AXIS2_PLACEMENT_3D('',#77662,#54831,#54832);
#47537=AXIS2_PLACEMENT_3D('',#77663,#54833,#54834);
#47538=AXIS2_PLACEMENT_3D('',#77664,#54835,#54836);
#47539=AXIS2_PLACEMENT_3D('',#77673,#54837,#54838);
#47540=AXIS2_PLACEMENT_3D('',#77674,#54839,#54840);
#47541=AXIS2_PLACEMENT_3D('',#77678,#54842,#54843);
#47542=AXIS2_PLACEMENT_3D('',#77680,#54844,#54845);
#47543=AXIS2_PLACEMENT_3D('',#77705,#54848,#54849);
#47544=AXIS2_PLACEMENT_3D('',#77706,#54850,#54851);
#47545=AXIS2_PLACEMENT_3D('',#77725,#54852,#54853);
#47546=AXIS2_PLACEMENT_3D('',#77733,#54855,#54856);
#47547=AXIS2_PLACEMENT_3D('',#77736,#54857,#54858);
#47548=AXIS2_PLACEMENT_3D('',#77737,#54859,#54860);
#47549=AXIS2_PLACEMENT_3D('',#77738,#54861,#54862);
#47550=AXIS2_PLACEMENT_3D('',#77750,#54863,#54864);
#47551=AXIS2_PLACEMENT_3D('',#77751,#54865,#54866);
#47552=AXIS2_PLACEMENT_3D('',#77755,#54868,#54869);
#47553=AXIS2_PLACEMENT_3D('',#77757,#54870,#54871);
#47554=AXIS2_PLACEMENT_3D('',#77793,#54874,#54875);
#47555=AXIS2_PLACEMENT_3D('',#77801,#54877,#54878);
#47556=AXIS2_PLACEMENT_3D('',#77804,#54879,#54880);
#47557=AXIS2_PLACEMENT_3D('',#77805,#54881,#54882);
#47558=AXIS2_PLACEMENT_3D('',#77806,#54883,#54884);
#47559=AXIS2_PLACEMENT_3D('',#77842,#54886,#54887);
#47560=AXIS2_PLACEMENT_3D('',#77844,#54888,#54889);
#47561=AXIS2_PLACEMENT_3D('',#77899,#54893,#54894);
#47562=AXIS2_PLACEMENT_3D('',#77902,#54895,#54896);
#47563=AXIS2_PLACEMENT_3D('',#77909,#54897,#54898);
#47564=AXIS2_PLACEMENT_3D('',#77921,#54899,#54900);
#47565=AXIS2_PLACEMENT_3D('',#77922,#54901,#54902);
#47566=AXIS2_PLACEMENT_3D('',#77926,#54904,#54905);
#47567=AXIS2_PLACEMENT_3D('',#77928,#54906,#54907);
#47568=AXIS2_PLACEMENT_3D('',#77964,#54910,#54911);
#47569=AXIS2_PLACEMENT_3D('',#77972,#54913,#54914);
#47570=AXIS2_PLACEMENT_3D('',#77975,#54915,#54916);
#47571=AXIS2_PLACEMENT_3D('',#77976,#54917,#54918);
#47572=AXIS2_PLACEMENT_3D('',#77977,#54919,#54920);
#47573=AXIS2_PLACEMENT_3D('',#77996,#54921,#54922);
#47574=AXIS2_PLACEMENT_3D('',#77997,#54923,#54924);
#47575=AXIS2_PLACEMENT_3D('',#78001,#54926,#54927);
#47576=AXIS2_PLACEMENT_3D('',#78003,#54928,#54929);
#47577=AXIS2_PLACEMENT_3D('',#78039,#54932,#54933);
#47578=AXIS2_PLACEMENT_3D('',#78047,#54935,#54936);
#47579=AXIS2_PLACEMENT_3D('',#78050,#54937,#54938);
#47580=AXIS2_PLACEMENT_3D('',#78051,#54939,#54940);
#47581=AXIS2_PLACEMENT_3D('',#78052,#54941,#54942);
#47582=AXIS2_PLACEMENT_3D('',#78064,#54943,#54944);
#47583=AXIS2_PLACEMENT_3D('',#78065,#54945,#54946);
#47584=AXIS2_PLACEMENT_3D('',#78069,#54948,#54949);
#47585=AXIS2_PLACEMENT_3D('',#78071,#54950,#54951);
#47586=AXIS2_PLACEMENT_3D('',#78112,#54954,#54955);
#47587=AXIS2_PLACEMENT_3D('',#78114,#54957,#54958);
#47588=AXIS2_PLACEMENT_3D('',#78115,#54959,#54960);
#47589=AXIS2_PLACEMENT_3D('',#78118,#54962,#54963);
#47590=AXIS2_PLACEMENT_3D('',#78119,#54964,#54965);
#47591=AXIS2_PLACEMENT_3D('',#78120,#54966,#54967);
#47592=AXIS2_PLACEMENT_3D('',#78139,#54968,#54969);
#47593=AXIS2_PLACEMENT_3D('',#78140,#54970,#54971);
#47594=AXIS2_PLACEMENT_3D('',#78150,#54972,#54973);
#47595=AXIS2_PLACEMENT_3D('',#78170,#54975,#54976);
#47596=AXIS2_PLACEMENT_3D('',#78178,#54978,#54979);
#47597=AXIS2_PLACEMENT_3D('',#78181,#54980,#54981);
#47598=AXIS2_PLACEMENT_3D('',#78182,#54982,#54983);
#47599=AXIS2_PLACEMENT_3D('',#78183,#54984,#54985);
#47600=AXIS2_PLACEMENT_3D('',#78192,#54986,#54987);
#47601=AXIS2_PLACEMENT_3D('',#78193,#54988,#54989);
#47602=AXIS2_PLACEMENT_3D('',#78197,#54991,#54992);
#47603=AXIS2_PLACEMENT_3D('',#78199,#54993,#54994);
#47604=AXIS2_PLACEMENT_3D('',#78224,#54997,#54998);
#47605=AXIS2_PLACEMENT_3D('',#78225,#54999,#55000);
#47606=AXIS2_PLACEMENT_3D('',#78244,#55001,#55002);
#47607=AXIS2_PLACEMENT_3D('',#78252,#55004,#55005);
#47608=AXIS2_PLACEMENT_3D('',#78255,#55006,#55007);
#47609=AXIS2_PLACEMENT_3D('',#78256,#55008,#55009);
#47610=AXIS2_PLACEMENT_3D('',#78257,#55010,#55011);
#47611=AXIS2_PLACEMENT_3D('',#78269,#55012,#55013);
#47612=AXIS2_PLACEMENT_3D('',#78270,#55014,#55015);
#47613=AXIS2_PLACEMENT_3D('',#78274,#55017,#55018);
#47614=AXIS2_PLACEMENT_3D('',#78276,#55019,#55020);
#47615=AXIS2_PLACEMENT_3D('',#78312,#55023,#55024);
#47616=AXIS2_PLACEMENT_3D('',#78320,#55026,#55027);
#47617=AXIS2_PLACEMENT_3D('',#78323,#55028,#55029);
#47618=AXIS2_PLACEMENT_3D('',#78324,#55030,#55031);
#47619=AXIS2_PLACEMENT_3D('',#78325,#55032,#55033);
#47620=AXIS2_PLACEMENT_3D('',#78361,#55035,#55036);
#47621=AXIS2_PLACEMENT_3D('',#78363,#55037,#55038);
#47622=AXIS2_PLACEMENT_3D('',#78418,#55042,#55043);
#47623=AXIS2_PLACEMENT_3D('',#78421,#55044,#55045);
#47624=AXIS2_PLACEMENT_3D('',#78428,#55046,#55047);
#47625=AXIS2_PLACEMENT_3D('',#78440,#55048,#55049);
#47626=AXIS2_PLACEMENT_3D('',#78441,#55050,#55051);
#47627=AXIS2_PLACEMENT_3D('',#78445,#55053,#55054);
#47628=AXIS2_PLACEMENT_3D('',#78447,#55055,#55056);
#47629=AXIS2_PLACEMENT_3D('',#78483,#55059,#55060);
#47630=AXIS2_PLACEMENT_3D('',#78491,#55062,#55063);
#47631=AXIS2_PLACEMENT_3D('',#78494,#55064,#55065);
#47632=AXIS2_PLACEMENT_3D('',#78495,#55066,#55067);
#47633=AXIS2_PLACEMENT_3D('',#78496,#55068,#55069);
#47634=AXIS2_PLACEMENT_3D('',#78515,#55070,#55071);
#47635=AXIS2_PLACEMENT_3D('',#78516,#55072,#55073);
#47636=AXIS2_PLACEMENT_3D('',#78520,#55075,#55076);
#47637=AXIS2_PLACEMENT_3D('',#78522,#55077,#55078);
#47638=AXIS2_PLACEMENT_3D('',#78558,#55081,#55082);
#47639=AXIS2_PLACEMENT_3D('',#78566,#55084,#55085);
#47640=AXIS2_PLACEMENT_3D('',#78569,#55086,#55087);
#47641=AXIS2_PLACEMENT_3D('',#78570,#55088,#55089);
#47642=AXIS2_PLACEMENT_3D('',#78571,#55090,#55091);
#47643=AXIS2_PLACEMENT_3D('',#78586,#55092,#55093);
#47644=AXIS2_PLACEMENT_3D('',#78587,#55094,#55095);
#47645=AXIS2_PLACEMENT_3D('',#78591,#55097,#55098);
#47646=AXIS2_PLACEMENT_3D('',#78593,#55099,#55100);
#47647=AXIS2_PLACEMENT_3D('',#78627,#55103,#55104);
#47648=AXIS2_PLACEMENT_3D('',#78629,#55106,#55107);
#47649=AXIS2_PLACEMENT_3D('',#78630,#55108,#55109);
#47650=AXIS2_PLACEMENT_3D('',#78633,#55111,#55112);
#47651=AXIS2_PLACEMENT_3D('',#78634,#55113,#55114);
#47652=AXIS2_PLACEMENT_3D('',#78635,#55115,#55116);
#47653=AXIS2_PLACEMENT_3D('',#78654,#55117,#55118);
#47654=AXIS2_PLACEMENT_3D('',#78655,#55119,#55120);
#47655=AXIS2_PLACEMENT_3D('',#78665,#55121,#55122);
#47656=AXIS2_PLACEMENT_3D('',#78685,#55124,#55125);
#47657=AXIS2_PLACEMENT_3D('',#78693,#55127,#55128);
#47658=AXIS2_PLACEMENT_3D('',#78696,#55129,#55130);
#47659=AXIS2_PLACEMENT_3D('',#78697,#55131,#55132);
#47660=AXIS2_PLACEMENT_3D('',#78698,#55133,#55134);
#47661=AXIS2_PLACEMENT_3D('',#78707,#55135,#55136);
#47662=AXIS2_PLACEMENT_3D('',#78708,#55137,#55138);
#47663=AXIS2_PLACEMENT_3D('',#78712,#55140,#55141);
#47664=AXIS2_PLACEMENT_3D('',#78714,#55142,#55143);
#47665=AXIS2_PLACEMENT_3D('',#78739,#55146,#55147);
#47666=AXIS2_PLACEMENT_3D('',#78740,#55148,#55149);
#47667=AXIS2_PLACEMENT_3D('',#78759,#55150,#55151);
#47668=AXIS2_PLACEMENT_3D('',#78767,#55153,#55154);
#47669=AXIS2_PLACEMENT_3D('',#78770,#55155,#55156);
#47670=AXIS2_PLACEMENT_3D('',#78771,#55157,#55158);
#47671=AXIS2_PLACEMENT_3D('',#78772,#55159,#55160);
#47672=AXIS2_PLACEMENT_3D('',#78784,#55161,#55162);
#47673=AXIS2_PLACEMENT_3D('',#78785,#55163,#55164);
#47674=AXIS2_PLACEMENT_3D('',#78789,#55166,#55167);
#47675=AXIS2_PLACEMENT_3D('',#78791,#55168,#55169);
#47676=AXIS2_PLACEMENT_3D('',#78827,#55172,#55173);
#47677=AXIS2_PLACEMENT_3D('',#78835,#55175,#55176);
#47678=AXIS2_PLACEMENT_3D('',#78838,#55177,#55178);
#47679=AXIS2_PLACEMENT_3D('',#78839,#55179,#55180);
#47680=AXIS2_PLACEMENT_3D('',#78840,#55181,#55182);
#47681=AXIS2_PLACEMENT_3D('',#78876,#55184,#55185);
#47682=AXIS2_PLACEMENT_3D('',#78878,#55186,#55187);
#47683=AXIS2_PLACEMENT_3D('',#78933,#55191,#55192);
#47684=AXIS2_PLACEMENT_3D('',#78936,#55193,#55194);
#47685=AXIS2_PLACEMENT_3D('',#78943,#55195,#55196);
#47686=AXIS2_PLACEMENT_3D('',#78955,#55197,#55198);
#47687=AXIS2_PLACEMENT_3D('',#78956,#55199,#55200);
#47688=AXIS2_PLACEMENT_3D('',#78960,#55202,#55203);
#47689=AXIS2_PLACEMENT_3D('',#78962,#55204,#55205);
#47690=AXIS2_PLACEMENT_3D('',#78998,#55208,#55209);
#47691=AXIS2_PLACEMENT_3D('',#79006,#55211,#55212);
#47692=AXIS2_PLACEMENT_3D('',#79009,#55213,#55214);
#47693=AXIS2_PLACEMENT_3D('',#79010,#55215,#55216);
#47694=AXIS2_PLACEMENT_3D('',#79011,#55217,#55218);
#47695=AXIS2_PLACEMENT_3D('',#79030,#55219,#55220);
#47696=AXIS2_PLACEMENT_3D('',#79031,#55221,#55222);
#47697=AXIS2_PLACEMENT_3D('',#79035,#55224,#55225);
#47698=AXIS2_PLACEMENT_3D('',#79037,#55226,#55227);
#47699=AXIS2_PLACEMENT_3D('',#79073,#55230,#55231);
#47700=AXIS2_PLACEMENT_3D('',#79081,#55233,#55234);
#47701=AXIS2_PLACEMENT_3D('',#79084,#55235,#55236);
#47702=AXIS2_PLACEMENT_3D('',#79085,#55237,#55238);
#47703=AXIS2_PLACEMENT_3D('',#79086,#55239,#55240);
#47704=AXIS2_PLACEMENT_3D('',#79101,#55241,#55242);
#47705=AXIS2_PLACEMENT_3D('',#79102,#55243,#55244);
#47706=AXIS2_PLACEMENT_3D('',#79106,#55246,#55247);
#47707=AXIS2_PLACEMENT_3D('',#79108,#55248,#55249);
#47708=AXIS2_PLACEMENT_3D('',#79142,#55252,#55253);
#47709=AXIS2_PLACEMENT_3D('',#79144,#55255,#55256);
#47710=AXIS2_PLACEMENT_3D('',#79145,#55257,#55258);
#47711=AXIS2_PLACEMENT_3D('',#79148,#55260,#55261);
#47712=AXIS2_PLACEMENT_3D('',#79149,#55262,#55263);
#47713=AXIS2_PLACEMENT_3D('',#79150,#55264,#55265);
#47714=AXIS2_PLACEMENT_3D('',#79169,#55266,#55267);
#47715=AXIS2_PLACEMENT_3D('',#79170,#55268,#55269);
#47716=AXIS2_PLACEMENT_3D('',#79180,#55270,#55271);
#47717=AXIS2_PLACEMENT_3D('',#79200,#55273,#55274);
#47718=AXIS2_PLACEMENT_3D('',#79208,#55276,#55277);
#47719=AXIS2_PLACEMENT_3D('',#79211,#55278,#55279);
#47720=AXIS2_PLACEMENT_3D('',#79212,#55280,#55281);
#47721=AXIS2_PLACEMENT_3D('',#79213,#55282,#55283);
#47722=AXIS2_PLACEMENT_3D('',#79222,#55284,#55285);
#47723=AXIS2_PLACEMENT_3D('',#79223,#55286,#55287);
#47724=AXIS2_PLACEMENT_3D('',#79227,#55289,#55290);
#47725=AXIS2_PLACEMENT_3D('',#79229,#55291,#55292);
#47726=AXIS2_PLACEMENT_3D('',#79254,#55295,#55296);
#47727=AXIS2_PLACEMENT_3D('',#79255,#55297,#55298);
#47728=AXIS2_PLACEMENT_3D('',#79274,#55299,#55300);
#47729=AXIS2_PLACEMENT_3D('',#79282,#55302,#55303);
#47730=AXIS2_PLACEMENT_3D('',#79285,#55304,#55305);
#47731=AXIS2_PLACEMENT_3D('',#79286,#55306,#55307);
#47732=AXIS2_PLACEMENT_3D('',#79287,#55308,#55309);
#47733=AXIS2_PLACEMENT_3D('',#79299,#55310,#55311);
#47734=AXIS2_PLACEMENT_3D('',#79300,#55312,#55313);
#47735=AXIS2_PLACEMENT_3D('',#79304,#55315,#55316);
#47736=AXIS2_PLACEMENT_3D('',#79306,#55317,#55318);
#47737=AXIS2_PLACEMENT_3D('',#79342,#55321,#55322);
#47738=AXIS2_PLACEMENT_3D('',#79350,#55324,#55325);
#47739=AXIS2_PLACEMENT_3D('',#79353,#55326,#55327);
#47740=AXIS2_PLACEMENT_3D('',#79354,#55328,#55329);
#47741=AXIS2_PLACEMENT_3D('',#79355,#55330,#55331);
#47742=AXIS2_PLACEMENT_3D('',#79391,#55333,#55334);
#47743=AXIS2_PLACEMENT_3D('',#79393,#55335,#55336);
#47744=AXIS2_PLACEMENT_3D('',#79448,#55340,#55341);
#47745=AXIS2_PLACEMENT_3D('',#79451,#55342,#55343);
#47746=AXIS2_PLACEMENT_3D('',#79458,#55344,#55345);
#47747=AXIS2_PLACEMENT_3D('',#79470,#55346,#55347);
#47748=AXIS2_PLACEMENT_3D('',#79471,#55348,#55349);
#47749=AXIS2_PLACEMENT_3D('',#79475,#55351,#55352);
#47750=AXIS2_PLACEMENT_3D('',#79477,#55353,#55354);
#47751=AXIS2_PLACEMENT_3D('',#79513,#55357,#55358);
#47752=AXIS2_PLACEMENT_3D('',#79521,#55360,#55361);
#47753=AXIS2_PLACEMENT_3D('',#79524,#55362,#55363);
#47754=AXIS2_PLACEMENT_3D('',#79525,#55364,#55365);
#47755=AXIS2_PLACEMENT_3D('',#79526,#55366,#55367);
#47756=AXIS2_PLACEMENT_3D('',#79545,#55368,#55369);
#47757=AXIS2_PLACEMENT_3D('',#79546,#55370,#55371);
#47758=AXIS2_PLACEMENT_3D('',#79550,#55373,#55374);
#47759=AXIS2_PLACEMENT_3D('',#79552,#55375,#55376);
#47760=AXIS2_PLACEMENT_3D('',#79588,#55379,#55380);
#47761=AXIS2_PLACEMENT_3D('',#79596,#55382,#55383);
#47762=AXIS2_PLACEMENT_3D('',#79599,#55384,#55385);
#47763=AXIS2_PLACEMENT_3D('',#79600,#55386,#55387);
#47764=AXIS2_PLACEMENT_3D('',#79601,#55388,#55389);
#47765=AXIS2_PLACEMENT_3D('',#79616,#55390,#55391);
#47766=AXIS2_PLACEMENT_3D('',#79617,#55392,#55393);
#47767=AXIS2_PLACEMENT_3D('',#79621,#55395,#55396);
#47768=AXIS2_PLACEMENT_3D('',#79623,#55397,#55398);
#47769=AXIS2_PLACEMENT_3D('',#79657,#55401,#55402);
#47770=AXIS2_PLACEMENT_3D('',#79659,#55404,#55405);
#47771=AXIS2_PLACEMENT_3D('',#79660,#55406,#55407);
#47772=AXIS2_PLACEMENT_3D('',#79663,#55409,#55410);
#47773=AXIS2_PLACEMENT_3D('',#79664,#55411,#55412);
#47774=AXIS2_PLACEMENT_3D('',#79665,#55413,#55414);
#47775=AXIS2_PLACEMENT_3D('',#79684,#55415,#55416);
#47776=AXIS2_PLACEMENT_3D('',#79685,#55417,#55418);
#47777=AXIS2_PLACEMENT_3D('',#79695,#55419,#55420);
#47778=AXIS2_PLACEMENT_3D('',#79715,#55422,#55423);
#47779=AXIS2_PLACEMENT_3D('',#79723,#55425,#55426);
#47780=AXIS2_PLACEMENT_3D('',#79726,#55427,#55428);
#47781=AXIS2_PLACEMENT_3D('',#79727,#55429,#55430);
#47782=AXIS2_PLACEMENT_3D('',#79728,#55431,#55432);
#47783=AXIS2_PLACEMENT_3D('',#79737,#55433,#55434);
#47784=AXIS2_PLACEMENT_3D('',#79738,#55435,#55436);
#47785=AXIS2_PLACEMENT_3D('',#79742,#55438,#55439);
#47786=AXIS2_PLACEMENT_3D('',#79744,#55440,#55441);
#47787=AXIS2_PLACEMENT_3D('',#79769,#55444,#55445);
#47788=AXIS2_PLACEMENT_3D('',#79770,#55446,#55447);
#47789=AXIS2_PLACEMENT_3D('',#79789,#55448,#55449);
#47790=AXIS2_PLACEMENT_3D('',#79797,#55451,#55452);
#47791=AXIS2_PLACEMENT_3D('',#79800,#55453,#55454);
#47792=AXIS2_PLACEMENT_3D('',#79801,#55455,#55456);
#47793=AXIS2_PLACEMENT_3D('',#79802,#55457,#55458);
#47794=AXIS2_PLACEMENT_3D('',#79814,#55459,#55460);
#47795=AXIS2_PLACEMENT_3D('',#79815,#55461,#55462);
#47796=AXIS2_PLACEMENT_3D('',#79819,#55464,#55465);
#47797=AXIS2_PLACEMENT_3D('',#79821,#55466,#55467);
#47798=AXIS2_PLACEMENT_3D('',#79857,#55470,#55471);
#47799=AXIS2_PLACEMENT_3D('',#79865,#55473,#55474);
#47800=AXIS2_PLACEMENT_3D('',#79868,#55475,#55476);
#47801=AXIS2_PLACEMENT_3D('',#79869,#55477,#55478);
#47802=AXIS2_PLACEMENT_3D('',#79870,#55479,#55480);
#47803=AXIS2_PLACEMENT_3D('',#79906,#55482,#55483);
#47804=AXIS2_PLACEMENT_3D('',#79908,#55484,#55485);
#47805=AXIS2_PLACEMENT_3D('',#79963,#55489,#55490);
#47806=AXIS2_PLACEMENT_3D('',#79966,#55491,#55492);
#47807=AXIS2_PLACEMENT_3D('',#79973,#55493,#55494);
#47808=AXIS2_PLACEMENT_3D('',#79985,#55495,#55496);
#47809=AXIS2_PLACEMENT_3D('',#79986,#55497,#55498);
#47810=AXIS2_PLACEMENT_3D('',#79990,#55500,#55501);
#47811=AXIS2_PLACEMENT_3D('',#79992,#55502,#55503);
#47812=AXIS2_PLACEMENT_3D('',#80028,#55506,#55507);
#47813=AXIS2_PLACEMENT_3D('',#80036,#55509,#55510);
#47814=AXIS2_PLACEMENT_3D('',#80039,#55511,#55512);
#47815=AXIS2_PLACEMENT_3D('',#80040,#55513,#55514);
#47816=AXIS2_PLACEMENT_3D('',#80041,#55515,#55516);
#47817=AXIS2_PLACEMENT_3D('',#80060,#55517,#55518);
#47818=AXIS2_PLACEMENT_3D('',#80061,#55519,#55520);
#47819=AXIS2_PLACEMENT_3D('',#80065,#55522,#55523);
#47820=AXIS2_PLACEMENT_3D('',#80067,#55524,#55525);
#47821=AXIS2_PLACEMENT_3D('',#80103,#55528,#55529);
#47822=AXIS2_PLACEMENT_3D('',#80111,#55531,#55532);
#47823=AXIS2_PLACEMENT_3D('',#80114,#55533,#55534);
#47824=AXIS2_PLACEMENT_3D('',#80115,#55535,#55536);
#47825=AXIS2_PLACEMENT_3D('',#80116,#55537,#55538);
#47826=AXIS2_PLACEMENT_3D('',#80131,#55539,#55540);
#47827=AXIS2_PLACEMENT_3D('',#80132,#55541,#55542);
#47828=AXIS2_PLACEMENT_3D('',#80136,#55544,#55545);
#47829=AXIS2_PLACEMENT_3D('',#80138,#55546,#55547);
#47830=AXIS2_PLACEMENT_3D('',#80172,#55550,#55551);
#47831=AXIS2_PLACEMENT_3D('',#80174,#55553,#55554);
#47832=AXIS2_PLACEMENT_3D('',#80175,#55555,#55556);
#47833=AXIS2_PLACEMENT_3D('',#80178,#55558,#55559);
#47834=AXIS2_PLACEMENT_3D('',#80179,#55560,#55561);
#47835=AXIS2_PLACEMENT_3D('',#80180,#55562,#55563);
#47836=AXIS2_PLACEMENT_3D('',#80199,#55564,#55565);
#47837=AXIS2_PLACEMENT_3D('',#80200,#55566,#55567);
#47838=AXIS2_PLACEMENT_3D('',#80210,#55568,#55569);
#47839=AXIS2_PLACEMENT_3D('',#80230,#55571,#55572);
#47840=AXIS2_PLACEMENT_3D('',#80238,#55574,#55575);
#47841=AXIS2_PLACEMENT_3D('',#80241,#55576,#55577);
#47842=AXIS2_PLACEMENT_3D('',#80242,#55578,#55579);
#47843=AXIS2_PLACEMENT_3D('',#80243,#55580,#55581);
#47844=AXIS2_PLACEMENT_3D('',#80252,#55582,#55583);
#47845=AXIS2_PLACEMENT_3D('',#80253,#55584,#55585);
#47846=AXIS2_PLACEMENT_3D('',#80257,#55587,#55588);
#47847=AXIS2_PLACEMENT_3D('',#80259,#55589,#55590);
#47848=AXIS2_PLACEMENT_3D('',#80284,#55593,#55594);
#47849=AXIS2_PLACEMENT_3D('',#80285,#55595,#55596);
#47850=AXIS2_PLACEMENT_3D('',#80304,#55597,#55598);
#47851=AXIS2_PLACEMENT_3D('',#80312,#55600,#55601);
#47852=AXIS2_PLACEMENT_3D('',#80315,#55602,#55603);
#47853=AXIS2_PLACEMENT_3D('',#80316,#55604,#55605);
#47854=AXIS2_PLACEMENT_3D('',#80317,#55606,#55607);
#47855=AXIS2_PLACEMENT_3D('',#80329,#55608,#55609);
#47856=AXIS2_PLACEMENT_3D('',#80330,#55610,#55611);
#47857=AXIS2_PLACEMENT_3D('',#80334,#55613,#55614);
#47858=AXIS2_PLACEMENT_3D('',#80336,#55615,#55616);
#47859=AXIS2_PLACEMENT_3D('',#80372,#55619,#55620);
#47860=AXIS2_PLACEMENT_3D('',#80380,#55622,#55623);
#47861=AXIS2_PLACEMENT_3D('',#80383,#55624,#55625);
#47862=AXIS2_PLACEMENT_3D('',#80384,#55626,#55627);
#47863=AXIS2_PLACEMENT_3D('',#80385,#55628,#55629);
#47864=AXIS2_PLACEMENT_3D('',#80421,#55631,#55632);
#47865=AXIS2_PLACEMENT_3D('',#80423,#55633,#55634);
#47866=AXIS2_PLACEMENT_3D('',#80478,#55638,#55639);
#47867=AXIS2_PLACEMENT_3D('',#80481,#55640,#55641);
#47868=AXIS2_PLACEMENT_3D('',#80488,#55642,#55643);
#47869=AXIS2_PLACEMENT_3D('',#80500,#55644,#55645);
#47870=AXIS2_PLACEMENT_3D('',#80501,#55646,#55647);
#47871=AXIS2_PLACEMENT_3D('',#80505,#55649,#55650);
#47872=AXIS2_PLACEMENT_3D('',#80507,#55651,#55652);
#47873=AXIS2_PLACEMENT_3D('',#80543,#55655,#55656);
#47874=AXIS2_PLACEMENT_3D('',#80551,#55658,#55659);
#47875=AXIS2_PLACEMENT_3D('',#80554,#55660,#55661);
#47876=AXIS2_PLACEMENT_3D('',#80555,#55662,#55663);
#47877=AXIS2_PLACEMENT_3D('',#80556,#55664,#55665);
#47878=AXIS2_PLACEMENT_3D('',#80575,#55666,#55667);
#47879=AXIS2_PLACEMENT_3D('',#80576,#55668,#55669);
#47880=AXIS2_PLACEMENT_3D('',#80580,#55671,#55672);
#47881=AXIS2_PLACEMENT_3D('',#80582,#55673,#55674);
#47882=AXIS2_PLACEMENT_3D('',#80618,#55677,#55678);
#47883=AXIS2_PLACEMENT_3D('',#80626,#55680,#55681);
#47884=AXIS2_PLACEMENT_3D('',#80629,#55682,#55683);
#47885=AXIS2_PLACEMENT_3D('',#80630,#55684,#55685);
#47886=AXIS2_PLACEMENT_3D('',#80631,#55686,#55687);
#47887=AXIS2_PLACEMENT_3D('',#80646,#55688,#55689);
#47888=AXIS2_PLACEMENT_3D('',#80647,#55690,#55691);
#47889=AXIS2_PLACEMENT_3D('',#80651,#55693,#55694);
#47890=AXIS2_PLACEMENT_3D('',#80653,#55695,#55696);
#47891=AXIS2_PLACEMENT_3D('',#80687,#55699,#55700);
#47892=AXIS2_PLACEMENT_3D('',#80689,#55702,#55703);
#47893=AXIS2_PLACEMENT_3D('',#80690,#55704,#55705);
#47894=AXIS2_PLACEMENT_3D('',#80693,#55707,#55708);
#47895=AXIS2_PLACEMENT_3D('',#80694,#55709,#55710);
#47896=AXIS2_PLACEMENT_3D('',#80695,#55711,#55712);
#47897=AXIS2_PLACEMENT_3D('',#80714,#55713,#55714);
#47898=AXIS2_PLACEMENT_3D('',#80715,#55715,#55716);
#47899=AXIS2_PLACEMENT_3D('',#80725,#55717,#55718);
#47900=AXIS2_PLACEMENT_3D('',#80745,#55720,#55721);
#47901=AXIS2_PLACEMENT_3D('',#80753,#55723,#55724);
#47902=AXIS2_PLACEMENT_3D('',#80756,#55725,#55726);
#47903=AXIS2_PLACEMENT_3D('',#80757,#55727,#55728);
#47904=AXIS2_PLACEMENT_3D('',#80758,#55729,#55730);
#47905=AXIS2_PLACEMENT_3D('',#80767,#55731,#55732);
#47906=AXIS2_PLACEMENT_3D('',#80768,#55733,#55734);
#47907=AXIS2_PLACEMENT_3D('',#80772,#55736,#55737);
#47908=AXIS2_PLACEMENT_3D('',#80774,#55738,#55739);
#47909=AXIS2_PLACEMENT_3D('',#80799,#55742,#55743);
#47910=AXIS2_PLACEMENT_3D('',#80800,#55744,#55745);
#47911=AXIS2_PLACEMENT_3D('',#80819,#55746,#55747);
#47912=AXIS2_PLACEMENT_3D('',#80827,#55749,#55750);
#47913=AXIS2_PLACEMENT_3D('',#80830,#55751,#55752);
#47914=AXIS2_PLACEMENT_3D('',#80831,#55753,#55754);
#47915=AXIS2_PLACEMENT_3D('',#80832,#55755,#55756);
#47916=AXIS2_PLACEMENT_3D('',#80844,#55757,#55758);
#47917=AXIS2_PLACEMENT_3D('',#80845,#55759,#55760);
#47918=AXIS2_PLACEMENT_3D('',#80849,#55762,#55763);
#47919=AXIS2_PLACEMENT_3D('',#80851,#55764,#55765);
#47920=AXIS2_PLACEMENT_3D('',#80887,#55768,#55769);
#47921=AXIS2_PLACEMENT_3D('',#80895,#55771,#55772);
#47922=AXIS2_PLACEMENT_3D('',#80898,#55773,#55774);
#47923=AXIS2_PLACEMENT_3D('',#80899,#55775,#55776);
#47924=AXIS2_PLACEMENT_3D('',#80900,#55777,#55778);
#47925=AXIS2_PLACEMENT_3D('',#80936,#55780,#55781);
#47926=AXIS2_PLACEMENT_3D('',#80938,#55782,#55783);
#47927=AXIS2_PLACEMENT_3D('',#80993,#55787,#55788);
#47928=AXIS2_PLACEMENT_3D('',#80996,#55789,#55790);
#47929=AXIS2_PLACEMENT_3D('',#81003,#55791,#55792);
#47930=AXIS2_PLACEMENT_3D('',#81015,#55793,#55794);
#47931=AXIS2_PLACEMENT_3D('',#81016,#55795,#55796);
#47932=AXIS2_PLACEMENT_3D('',#81020,#55798,#55799);
#47933=AXIS2_PLACEMENT_3D('',#81022,#55800,#55801);
#47934=AXIS2_PLACEMENT_3D('',#81058,#55804,#55805);
#47935=AXIS2_PLACEMENT_3D('',#81066,#55807,#55808);
#47936=AXIS2_PLACEMENT_3D('',#81069,#55809,#55810);
#47937=AXIS2_PLACEMENT_3D('',#81070,#55811,#55812);
#47938=AXIS2_PLACEMENT_3D('',#81071,#55813,#55814);
#47939=AXIS2_PLACEMENT_3D('',#81090,#55815,#55816);
#47940=AXIS2_PLACEMENT_3D('',#81091,#55817,#55818);
#47941=AXIS2_PLACEMENT_3D('',#81095,#55820,#55821);
#47942=AXIS2_PLACEMENT_3D('',#81097,#55822,#55823);
#47943=AXIS2_PLACEMENT_3D('',#81133,#55826,#55827);
#47944=AXIS2_PLACEMENT_3D('',#81141,#55829,#55830);
#47945=AXIS2_PLACEMENT_3D('',#81144,#55831,#55832);
#47946=AXIS2_PLACEMENT_3D('',#81145,#55833,#55834);
#47947=AXIS2_PLACEMENT_3D('',#81146,#55835,#55836);
#47948=AXIS2_PLACEMENT_3D('',#81161,#55837,#55838);
#47949=AXIS2_PLACEMENT_3D('',#81162,#55839,#55840);
#47950=AXIS2_PLACEMENT_3D('',#81166,#55842,#55843);
#47951=AXIS2_PLACEMENT_3D('',#81168,#55844,#55845);
#47952=AXIS2_PLACEMENT_3D('',#81202,#55848,#55849);
#47953=AXIS2_PLACEMENT_3D('',#81204,#55851,#55852);
#47954=AXIS2_PLACEMENT_3D('',#81205,#55853,#55854);
#47955=AXIS2_PLACEMENT_3D('',#81208,#55856,#55857);
#47956=AXIS2_PLACEMENT_3D('',#81209,#55858,#55859);
#47957=AXIS2_PLACEMENT_3D('',#81210,#55860,#55861);
#47958=AXIS2_PLACEMENT_3D('',#81229,#55862,#55863);
#47959=AXIS2_PLACEMENT_3D('',#81230,#55864,#55865);
#47960=AXIS2_PLACEMENT_3D('',#81240,#55866,#55867);
#47961=AXIS2_PLACEMENT_3D('',#81260,#55869,#55870);
#47962=AXIS2_PLACEMENT_3D('',#81268,#55872,#55873);
#47963=AXIS2_PLACEMENT_3D('',#81271,#55874,#55875);
#47964=AXIS2_PLACEMENT_3D('',#81272,#55876,#55877);
#47965=AXIS2_PLACEMENT_3D('',#81273,#55878,#55879);
#47966=AXIS2_PLACEMENT_3D('',#81282,#55880,#55881);
#47967=AXIS2_PLACEMENT_3D('',#81283,#55882,#55883);
#47968=AXIS2_PLACEMENT_3D('',#81287,#55885,#55886);
#47969=AXIS2_PLACEMENT_3D('',#81289,#55887,#55888);
#47970=AXIS2_PLACEMENT_3D('',#81314,#55891,#55892);
#47971=AXIS2_PLACEMENT_3D('',#81315,#55893,#55894);
#47972=AXIS2_PLACEMENT_3D('',#81334,#55895,#55896);
#47973=AXIS2_PLACEMENT_3D('',#81342,#55898,#55899);
#47974=AXIS2_PLACEMENT_3D('',#81345,#55900,#55901);
#47975=AXIS2_PLACEMENT_3D('',#81346,#55902,#55903);
#47976=AXIS2_PLACEMENT_3D('',#81347,#55904,#55905);
#47977=AXIS2_PLACEMENT_3D('',#81356,#55906,#55907);
#47978=AXIS2_PLACEMENT_3D('',#81357,#55908,#55909);
#47979=AXIS2_PLACEMENT_3D('',#81361,#55911,#55912);
#47980=AXIS2_PLACEMENT_3D('',#81363,#55913,#55914);
#47981=AXIS2_PLACEMENT_3D('',#81406,#55917,#55918);
#47982=AXIS2_PLACEMENT_3D('',#81414,#55920,#55921);
#47983=AXIS2_PLACEMENT_3D('',#81417,#55922,#55923);
#47984=AXIS2_PLACEMENT_3D('',#81418,#55924,#55925);
#47985=AXIS2_PLACEMENT_3D('',#81419,#55926,#55927);
#47986=AXIS2_PLACEMENT_3D('',#81455,#55929,#55930);
#47987=AXIS2_PLACEMENT_3D('',#81457,#55931,#55932);
#47988=AXIS2_PLACEMENT_3D('',#81512,#55936,#55937);
#47989=AXIS2_PLACEMENT_3D('',#81515,#55938,#55939);
#47990=AXIS2_PLACEMENT_3D('',#81522,#55940,#55941);
#47991=AXIS2_PLACEMENT_3D('',#81534,#55942,#55943);
#47992=AXIS2_PLACEMENT_3D('',#81535,#55944,#55945);
#47993=AXIS2_PLACEMENT_3D('',#81539,#55947,#55948);
#47994=AXIS2_PLACEMENT_3D('',#81541,#55949,#55950);
#47995=AXIS2_PLACEMENT_3D('',#81577,#55953,#55954);
#47996=AXIS2_PLACEMENT_3D('',#81585,#55956,#55957);
#47997=AXIS2_PLACEMENT_3D('',#81588,#55958,#55959);
#47998=AXIS2_PLACEMENT_3D('',#81589,#55960,#55961);
#47999=AXIS2_PLACEMENT_3D('',#81590,#55962,#55963);
#48000=AXIS2_PLACEMENT_3D('',#81609,#55964,#55965);
#48001=AXIS2_PLACEMENT_3D('',#81610,#55966,#55967);
#48002=AXIS2_PLACEMENT_3D('',#81614,#55969,#55970);
#48003=AXIS2_PLACEMENT_3D('',#81616,#55971,#55972);
#48004=AXIS2_PLACEMENT_3D('',#81652,#55975,#55976);
#48005=AXIS2_PLACEMENT_3D('',#81660,#55978,#55979);
#48006=AXIS2_PLACEMENT_3D('',#81663,#55980,#55981);
#48007=AXIS2_PLACEMENT_3D('',#81664,#55982,#55983);
#48008=AXIS2_PLACEMENT_3D('',#81665,#55984,#55985);
#48009=AXIS2_PLACEMENT_3D('',#81680,#55986,#55987);
#48010=AXIS2_PLACEMENT_3D('',#81681,#55988,#55989);
#48011=AXIS2_PLACEMENT_3D('',#81685,#55991,#55992);
#48012=AXIS2_PLACEMENT_3D('',#81687,#55993,#55994);
#48013=AXIS2_PLACEMENT_3D('',#81721,#55997,#55998);
#48014=AXIS2_PLACEMENT_3D('',#81723,#56000,#56001);
#48015=AXIS2_PLACEMENT_3D('',#81724,#56002,#56003);
#48016=AXIS2_PLACEMENT_3D('',#81727,#56005,#56006);
#48017=AXIS2_PLACEMENT_3D('',#81728,#56007,#56008);
#48018=AXIS2_PLACEMENT_3D('',#81729,#56009,#56010);
#48019=AXIS2_PLACEMENT_3D('',#81748,#56011,#56012);
#48020=AXIS2_PLACEMENT_3D('',#81749,#56013,#56014);
#48021=AXIS2_PLACEMENT_3D('',#81759,#56015,#56016);
#48022=AXIS2_PLACEMENT_3D('',#81779,#56018,#56019);
#48023=AXIS2_PLACEMENT_3D('',#81787,#56021,#56022);
#48024=AXIS2_PLACEMENT_3D('',#81790,#56023,#56024);
#48025=AXIS2_PLACEMENT_3D('',#81791,#56025,#56026);
#48026=AXIS2_PLACEMENT_3D('',#81792,#56027,#56028);
#48027=AXIS2_PLACEMENT_3D('',#81801,#56029,#56030);
#48028=AXIS2_PLACEMENT_3D('',#81802,#56031,#56032);
#48029=AXIS2_PLACEMENT_3D('',#81806,#56034,#56035);
#48030=AXIS2_PLACEMENT_3D('',#81808,#56036,#56037);
#48031=AXIS2_PLACEMENT_3D('',#81833,#56040,#56041);
#48032=AXIS2_PLACEMENT_3D('',#81834,#56042,#56043);
#48033=AXIS2_PLACEMENT_3D('',#81853,#56044,#56045);
#48034=AXIS2_PLACEMENT_3D('',#81861,#56047,#56048);
#48035=AXIS2_PLACEMENT_3D('',#81864,#56049,#56050);
#48036=AXIS2_PLACEMENT_3D('',#81865,#56051,#56052);
#48037=AXIS2_PLACEMENT_3D('',#81866,#56053,#56054);
#48038=AXIS2_PLACEMENT_3D('',#81878,#56055,#56056);
#48039=AXIS2_PLACEMENT_3D('',#81879,#56057,#56058);
#48040=AXIS2_PLACEMENT_3D('',#81883,#56060,#56061);
#48041=AXIS2_PLACEMENT_3D('',#81885,#56062,#56063);
#48042=AXIS2_PLACEMENT_3D('',#81921,#56066,#56067);
#48043=AXIS2_PLACEMENT_3D('',#81929,#56069,#56070);
#48044=AXIS2_PLACEMENT_3D('',#81932,#56071,#56072);
#48045=AXIS2_PLACEMENT_3D('',#81933,#56073,#56074);
#48046=AXIS2_PLACEMENT_3D('',#81934,#56075,#56076);
#48047=AXIS2_PLACEMENT_3D('',#81969,#56078,#56079);
#48048=AXIS2_PLACEMENT_3D('',#81971,#56080,#56081);
#48049=AXIS2_PLACEMENT_3D('',#82021,#56085,#56086);
#48050=AXIS2_PLACEMENT_3D('',#82024,#56087,#56088);
#48051=AXIS2_PLACEMENT_3D('',#82031,#56089,#56090);
#48052=AXIS2_PLACEMENT_3D('',#82043,#56091,#56092);
#48053=AXIS2_PLACEMENT_3D('',#82044,#56093,#56094);
#48054=AXIS2_PLACEMENT_3D('',#82048,#56096,#56097);
#48055=AXIS2_PLACEMENT_3D('',#82050,#56098,#56099);
#48056=AXIS2_PLACEMENT_3D('',#82086,#56102,#56103);
#48057=AXIS2_PLACEMENT_3D('',#82094,#56105,#56106);
#48058=AXIS2_PLACEMENT_3D('',#82097,#56107,#56108);
#48059=AXIS2_PLACEMENT_3D('',#82098,#56109,#56110);
#48060=AXIS2_PLACEMENT_3D('',#82099,#56111,#56112);
#48061=AXIS2_PLACEMENT_3D('',#82118,#56113,#56114);
#48062=AXIS2_PLACEMENT_3D('',#82119,#56115,#56116);
#48063=AXIS2_PLACEMENT_3D('',#82123,#56118,#56119);
#48064=AXIS2_PLACEMENT_3D('',#82125,#56120,#56121);
#48065=AXIS2_PLACEMENT_3D('',#82161,#56124,#56125);
#48066=AXIS2_PLACEMENT_3D('',#82169,#56127,#56128);
#48067=AXIS2_PLACEMENT_3D('',#82172,#56129,#56130);
#48068=AXIS2_PLACEMENT_3D('',#82173,#56131,#56132);
#48069=AXIS2_PLACEMENT_3D('',#82174,#56133,#56134);
#48070=AXIS2_PLACEMENT_3D('',#82189,#56135,#56136);
#48071=AXIS2_PLACEMENT_3D('',#82190,#56137,#56138);
#48072=AXIS2_PLACEMENT_3D('',#82194,#56140,#56141);
#48073=AXIS2_PLACEMENT_3D('',#82196,#56142,#56143);
#48074=AXIS2_PLACEMENT_3D('',#82230,#56146,#56147);
#48075=AXIS2_PLACEMENT_3D('',#82232,#56149,#56150);
#48076=AXIS2_PLACEMENT_3D('',#82233,#56151,#56152);
#48077=AXIS2_PLACEMENT_3D('',#82236,#56154,#56155);
#48078=AXIS2_PLACEMENT_3D('',#82237,#56156,#56157);
#48079=AXIS2_PLACEMENT_3D('',#82238,#56158,#56159);
#48080=AXIS2_PLACEMENT_3D('',#82257,#56160,#56161);
#48081=AXIS2_PLACEMENT_3D('',#82258,#56162,#56163);
#48082=AXIS2_PLACEMENT_3D('',#82268,#56164,#56165);
#48083=AXIS2_PLACEMENT_3D('',#82288,#56167,#56168);
#48084=AXIS2_PLACEMENT_3D('',#82296,#56170,#56171);
#48085=AXIS2_PLACEMENT_3D('',#82299,#56172,#56173);
#48086=AXIS2_PLACEMENT_3D('',#82300,#56174,#56175);
#48087=AXIS2_PLACEMENT_3D('',#82301,#56176,#56177);
#48088=AXIS2_PLACEMENT_3D('',#82310,#56178,#56179);
#48089=AXIS2_PLACEMENT_3D('',#82311,#56180,#56181);
#48090=AXIS2_PLACEMENT_3D('',#82315,#56183,#56184);
#48091=AXIS2_PLACEMENT_3D('',#82317,#56185,#56186);
#48092=AXIS2_PLACEMENT_3D('',#82342,#56189,#56190);
#48093=AXIS2_PLACEMENT_3D('',#82343,#56191,#56192);
#48094=AXIS2_PLACEMENT_3D('',#82362,#56193,#56194);
#48095=AXIS2_PLACEMENT_3D('',#82370,#56196,#56197);
#48096=AXIS2_PLACEMENT_3D('',#82373,#56198,#56199);
#48097=AXIS2_PLACEMENT_3D('',#82374,#56200,#56201);
#48098=AXIS2_PLACEMENT_3D('',#82375,#56202,#56203);
#48099=AXIS2_PLACEMENT_3D('',#82387,#56204,#56205);
#48100=AXIS2_PLACEMENT_3D('',#82388,#56206,#56207);
#48101=AXIS2_PLACEMENT_3D('',#82392,#56209,#56210);
#48102=AXIS2_PLACEMENT_3D('',#82394,#56211,#56212);
#48103=AXIS2_PLACEMENT_3D('',#82430,#56215,#56216);
#48104=AXIS2_PLACEMENT_3D('',#82438,#56218,#56219);
#48105=AXIS2_PLACEMENT_3D('',#82441,#56220,#56221);
#48106=AXIS2_PLACEMENT_3D('',#82442,#56222,#56223);
#48107=AXIS2_PLACEMENT_3D('',#82443,#56224,#56225);
#48108=AXIS2_PLACEMENT_3D('',#82479,#56227,#56228);
#48109=AXIS2_PLACEMENT_3D('',#82481,#56229,#56230);
#48110=AXIS2_PLACEMENT_3D('',#82536,#56234,#56235);
#48111=AXIS2_PLACEMENT_3D('',#82539,#56236,#56237);
#48112=AXIS2_PLACEMENT_3D('',#82546,#56238,#56239);
#48113=AXIS2_PLACEMENT_3D('',#82555,#56240,#56241);
#48114=AXIS2_PLACEMENT_3D('',#82556,#56242,#56243);
#48115=AXIS2_PLACEMENT_3D('',#82560,#56245,#56246);
#48116=AXIS2_PLACEMENT_3D('',#82562,#56247,#56248);
#48117=AXIS2_PLACEMENT_3D('',#82605,#56251,#56252);
#48118=AXIS2_PLACEMENT_3D('',#82613,#56254,#56255);
#48119=AXIS2_PLACEMENT_3D('',#82616,#56256,#56257);
#48120=AXIS2_PLACEMENT_3D('',#82617,#56258,#56259);
#48121=AXIS2_PLACEMENT_3D('',#82618,#56260,#56261);
#48122=AXIS2_PLACEMENT_3D('',#82637,#56262,#56263);
#48123=AXIS2_PLACEMENT_3D('',#82638,#56264,#56265);
#48124=AXIS2_PLACEMENT_3D('',#82642,#56267,#56268);
#48125=AXIS2_PLACEMENT_3D('',#82644,#56269,#56270);
#48126=AXIS2_PLACEMENT_3D('',#82680,#56273,#56274);
#48127=AXIS2_PLACEMENT_3D('',#82688,#56276,#56277);
#48128=AXIS2_PLACEMENT_3D('',#82691,#56278,#56279);
#48129=AXIS2_PLACEMENT_3D('',#82692,#56280,#56281);
#48130=AXIS2_PLACEMENT_3D('',#82693,#56282,#56283);
#48131=AXIS2_PLACEMENT_3D('',#82708,#56284,#56285);
#48132=AXIS2_PLACEMENT_3D('',#82709,#56286,#56287);
#48133=AXIS2_PLACEMENT_3D('',#82713,#56289,#56290);
#48134=AXIS2_PLACEMENT_3D('',#82715,#56291,#56292);
#48135=AXIS2_PLACEMENT_3D('',#82749,#56295,#56296);
#48136=AXIS2_PLACEMENT_3D('',#82751,#56298,#56299);
#48137=AXIS2_PLACEMENT_3D('',#82752,#56300,#56301);
#48138=AXIS2_PLACEMENT_3D('',#82755,#56303,#56304);
#48139=AXIS2_PLACEMENT_3D('',#82756,#56305,#56306);
#48140=AXIS2_PLACEMENT_3D('',#82757,#56307,#56308);
#48141=AXIS2_PLACEMENT_3D('',#82776,#56309,#56310);
#48142=AXIS2_PLACEMENT_3D('',#82777,#56311,#56312);
#48143=AXIS2_PLACEMENT_3D('',#82787,#56313,#56314);
#48144=AXIS2_PLACEMENT_3D('',#82807,#56316,#56317);
#48145=AXIS2_PLACEMENT_3D('',#82815,#56319,#56320);
#48146=AXIS2_PLACEMENT_3D('',#82818,#56321,#56322);
#48147=AXIS2_PLACEMENT_3D('',#82819,#56323,#56324);
#48148=AXIS2_PLACEMENT_3D('',#82820,#56325,#56326);
#48149=AXIS2_PLACEMENT_3D('',#82829,#56327,#56328);
#48150=AXIS2_PLACEMENT_3D('',#82830,#56329,#56330);
#48151=AXIS2_PLACEMENT_3D('',#82834,#56332,#56333);
#48152=AXIS2_PLACEMENT_3D('',#82836,#56334,#56335);
#48153=AXIS2_PLACEMENT_3D('',#82861,#56338,#56339);
#48154=AXIS2_PLACEMENT_3D('',#82862,#56340,#56341);
#48155=AXIS2_PLACEMENT_3D('',#82881,#56342,#56343);
#48156=AXIS2_PLACEMENT_3D('',#82889,#56345,#56346);
#48157=AXIS2_PLACEMENT_3D('',#82892,#56347,#56348);
#48158=AXIS2_PLACEMENT_3D('',#82893,#56349,#56350);
#48159=AXIS2_PLACEMENT_3D('',#82894,#56351,#56352);
#48160=AXIS2_PLACEMENT_3D('',#82906,#56353,#56354);
#48161=AXIS2_PLACEMENT_3D('',#82907,#56355,#56356);
#48162=AXIS2_PLACEMENT_3D('',#82911,#56358,#56359);
#48163=AXIS2_PLACEMENT_3D('',#82913,#56360,#56361);
#48164=AXIS2_PLACEMENT_3D('',#82949,#56364,#56365);
#48165=AXIS2_PLACEMENT_3D('',#82957,#56367,#56368);
#48166=AXIS2_PLACEMENT_3D('',#82960,#56369,#56370);
#48167=AXIS2_PLACEMENT_3D('',#82961,#56371,#56372);
#48168=AXIS2_PLACEMENT_3D('',#82962,#56373,#56374);
#48169=AXIS2_PLACEMENT_3D('',#82998,#56376,#56377);
#48170=AXIS2_PLACEMENT_3D('',#83000,#56378,#56379);
#48171=AXIS2_PLACEMENT_3D('',#83055,#56383,#56384);
#48172=AXIS2_PLACEMENT_3D('',#83058,#56385,#56386);
#48173=AXIS2_PLACEMENT_3D('',#83065,#56387,#56388);
#48174=AXIS2_PLACEMENT_3D('',#83077,#56389,#56390);
#48175=AXIS2_PLACEMENT_3D('',#83078,#56391,#56392);
#48176=AXIS2_PLACEMENT_3D('',#83082,#56394,#56395);
#48177=AXIS2_PLACEMENT_3D('',#83084,#56396,#56397);
#48178=AXIS2_PLACEMENT_3D('',#83120,#56400,#56401);
#48179=AXIS2_PLACEMENT_3D('',#83128,#56403,#56404);
#48180=AXIS2_PLACEMENT_3D('',#83131,#56405,#56406);
#48181=AXIS2_PLACEMENT_3D('',#83132,#56407,#56408);
#48182=AXIS2_PLACEMENT_3D('',#83133,#56409,#56410);
#48183=AXIS2_PLACEMENT_3D('',#83152,#56411,#56412);
#48184=AXIS2_PLACEMENT_3D('',#83153,#56413,#56414);
#48185=AXIS2_PLACEMENT_3D('',#83157,#56416,#56417);
#48186=AXIS2_PLACEMENT_3D('',#83159,#56418,#56419);
#48187=AXIS2_PLACEMENT_3D('',#83202,#56422,#56423);
#48188=AXIS2_PLACEMENT_3D('',#83210,#56425,#56426);
#48189=AXIS2_PLACEMENT_3D('',#83213,#56427,#56428);
#48190=AXIS2_PLACEMENT_3D('',#83214,#56429,#56430);
#48191=AXIS2_PLACEMENT_3D('',#83215,#56431,#56432);
#48192=AXIS2_PLACEMENT_3D('',#83230,#56433,#56434);
#48193=AXIS2_PLACEMENT_3D('',#83231,#56435,#56436);
#48194=AXIS2_PLACEMENT_3D('',#83235,#56438,#56439);
#48195=AXIS2_PLACEMENT_3D('',#83237,#56440,#56441);
#48196=AXIS2_PLACEMENT_3D('',#83271,#56444,#56445);
#48197=AXIS2_PLACEMENT_3D('',#83273,#56447,#56448);
#48198=AXIS2_PLACEMENT_3D('',#83274,#56449,#56450);
#48199=AXIS2_PLACEMENT_3D('',#83277,#56452,#56453);
#48200=AXIS2_PLACEMENT_3D('',#83278,#56454,#56455);
#48201=AXIS2_PLACEMENT_3D('',#83279,#56456,#56457);
#48202=AXIS2_PLACEMENT_3D('',#83298,#56458,#56459);
#48203=AXIS2_PLACEMENT_3D('',#83299,#56460,#56461);
#48204=AXIS2_PLACEMENT_3D('',#83309,#56462,#56463);
#48205=AXIS2_PLACEMENT_3D('',#83329,#56465,#56466);
#48206=AXIS2_PLACEMENT_3D('',#83337,#56468,#56469);
#48207=AXIS2_PLACEMENT_3D('',#83340,#56470,#56471);
#48208=AXIS2_PLACEMENT_3D('',#83341,#56472,#56473);
#48209=AXIS2_PLACEMENT_3D('',#83342,#56474,#56475);
#48210=AXIS2_PLACEMENT_3D('',#83351,#56476,#56477);
#48211=AXIS2_PLACEMENT_3D('',#83352,#56478,#56479);
#48212=AXIS2_PLACEMENT_3D('',#83356,#56481,#56482);
#48213=AXIS2_PLACEMENT_3D('',#83358,#56483,#56484);
#48214=AXIS2_PLACEMENT_3D('',#83383,#56487,#56488);
#48215=AXIS2_PLACEMENT_3D('',#83384,#56489,#56490);
#48216=AXIS2_PLACEMENT_3D('',#83403,#56491,#56492);
#48217=AXIS2_PLACEMENT_3D('',#83411,#56494,#56495);
#48218=AXIS2_PLACEMENT_3D('',#83414,#56496,#56497);
#48219=AXIS2_PLACEMENT_3D('',#83415,#56498,#56499);
#48220=AXIS2_PLACEMENT_3D('',#83416,#56500,#56501);
#48221=AXIS2_PLACEMENT_3D('',#83428,#56502,#56503);
#48222=AXIS2_PLACEMENT_3D('',#83429,#56504,#56505);
#48223=AXIS2_PLACEMENT_3D('',#83433,#56507,#56508);
#48224=AXIS2_PLACEMENT_3D('',#83435,#56509,#56510);
#48225=AXIS2_PLACEMENT_3D('',#83471,#56513,#56514);
#48226=AXIS2_PLACEMENT_3D('',#83479,#56516,#56517);
#48227=AXIS2_PLACEMENT_3D('',#83482,#56518,#56519);
#48228=AXIS2_PLACEMENT_3D('',#83483,#56520,#56521);
#48229=AXIS2_PLACEMENT_3D('',#83484,#56522,#56523);
#48230=AXIS2_PLACEMENT_3D('',#83520,#56525,#56526);
#48231=AXIS2_PLACEMENT_3D('',#83522,#56527,#56528);
#48232=AXIS2_PLACEMENT_3D('',#83577,#56532,#56533);
#48233=AXIS2_PLACEMENT_3D('',#83580,#56534,#56535);
#48234=AXIS2_PLACEMENT_3D('',#83587,#56536,#56537);
#48235=AXIS2_PLACEMENT_3D('',#83599,#56538,#56539);
#48236=AXIS2_PLACEMENT_3D('',#83600,#56540,#56541);
#48237=AXIS2_PLACEMENT_3D('',#83604,#56543,#56544);
#48238=AXIS2_PLACEMENT_3D('',#83606,#56545,#56546);
#48239=AXIS2_PLACEMENT_3D('',#83642,#56549,#56550);
#48240=AXIS2_PLACEMENT_3D('',#83650,#56552,#56553);
#48241=AXIS2_PLACEMENT_3D('',#83653,#56554,#56555);
#48242=AXIS2_PLACEMENT_3D('',#83654,#56556,#56557);
#48243=AXIS2_PLACEMENT_3D('',#83655,#56558,#56559);
#48244=AXIS2_PLACEMENT_3D('',#83674,#56560,#56561);
#48245=AXIS2_PLACEMENT_3D('',#83675,#56562,#56563);
#48246=AXIS2_PLACEMENT_3D('',#83679,#56565,#56566);
#48247=AXIS2_PLACEMENT_3D('',#83681,#56567,#56568);
#48248=AXIS2_PLACEMENT_3D('',#83717,#56571,#56572);
#48249=AXIS2_PLACEMENT_3D('',#83725,#56574,#56575);
#48250=AXIS2_PLACEMENT_3D('',#83728,#56576,#56577);
#48251=AXIS2_PLACEMENT_3D('',#83729,#56578,#56579);
#48252=AXIS2_PLACEMENT_3D('',#83730,#56580,#56581);
#48253=AXIS2_PLACEMENT_3D('',#83742,#56582,#56583);
#48254=AXIS2_PLACEMENT_3D('',#83743,#56584,#56585);
#48255=AXIS2_PLACEMENT_3D('',#83747,#56587,#56588);
#48256=AXIS2_PLACEMENT_3D('',#83749,#56589,#56590);
#48257=AXIS2_PLACEMENT_3D('',#83790,#56593,#56594);
#48258=AXIS2_PLACEMENT_3D('',#83792,#56596,#56597);
#48259=AXIS2_PLACEMENT_3D('',#83793,#56598,#56599);
#48260=AXIS2_PLACEMENT_3D('',#83796,#56601,#56602);
#48261=AXIS2_PLACEMENT_3D('',#83797,#56603,#56604);
#48262=AXIS2_PLACEMENT_3D('',#83798,#56605,#56606);
#48263=AXIS2_PLACEMENT_3D('',#83817,#56607,#56608);
#48264=AXIS2_PLACEMENT_3D('',#83818,#56609,#56610);
#48265=AXIS2_PLACEMENT_3D('',#83828,#56611,#56612);
#48266=AXIS2_PLACEMENT_3D('',#83848,#56614,#56615);
#48267=AXIS2_PLACEMENT_3D('',#83856,#56617,#56618);
#48268=AXIS2_PLACEMENT_3D('',#83859,#56619,#56620);
#48269=AXIS2_PLACEMENT_3D('',#83860,#56621,#56622);
#48270=AXIS2_PLACEMENT_3D('',#83861,#56623,#56624);
#48271=AXIS2_PLACEMENT_3D('',#83870,#56625,#56626);
#48272=AXIS2_PLACEMENT_3D('',#83871,#56627,#56628);
#48273=AXIS2_PLACEMENT_3D('',#83875,#56630,#56631);
#48274=AXIS2_PLACEMENT_3D('',#83877,#56632,#56633);
#48275=AXIS2_PLACEMENT_3D('',#83902,#56636,#56637);
#48276=AXIS2_PLACEMENT_3D('',#83903,#56638,#56639);
#48277=AXIS2_PLACEMENT_3D('',#83922,#56640,#56641);
#48278=AXIS2_PLACEMENT_3D('',#83930,#56643,#56644);
#48279=AXIS2_PLACEMENT_3D('',#83933,#56645,#56646);
#48280=AXIS2_PLACEMENT_3D('',#83934,#56647,#56648);
#48281=AXIS2_PLACEMENT_3D('',#83935,#56649,#56650);
#48282=AXIS2_PLACEMENT_3D('',#83947,#56651,#56652);
#48283=AXIS2_PLACEMENT_3D('',#83948,#56653,#56654);
#48284=AXIS2_PLACEMENT_3D('',#83952,#56656,#56657);
#48285=AXIS2_PLACEMENT_3D('',#83954,#56658,#56659);
#48286=AXIS2_PLACEMENT_3D('',#83990,#56662,#56663);
#48287=AXIS2_PLACEMENT_3D('',#83998,#56665,#56666);
#48288=AXIS2_PLACEMENT_3D('',#84001,#56667,#56668);
#48289=AXIS2_PLACEMENT_3D('',#84002,#56669,#56670);
#48290=AXIS2_PLACEMENT_3D('',#84003,#56671,#56672);
#48291=AXIS2_PLACEMENT_3D('',#84039,#56674,#56675);
#48292=AXIS2_PLACEMENT_3D('',#84041,#56676,#56677);
#48293=AXIS2_PLACEMENT_3D('',#84096,#56681,#56682);
#48294=AXIS2_PLACEMENT_3D('',#84099,#56683,#56684);
#48295=AXIS2_PLACEMENT_3D('',#84106,#56685,#56686);
#48296=AXIS2_PLACEMENT_3D('',#84118,#56687,#56688);
#48297=AXIS2_PLACEMENT_3D('',#84119,#56689,#56690);
#48298=AXIS2_PLACEMENT_3D('',#84123,#56692,#56693);
#48299=AXIS2_PLACEMENT_3D('',#84125,#56694,#56695);
#48300=AXIS2_PLACEMENT_3D('',#84161,#56698,#56699);
#48301=AXIS2_PLACEMENT_3D('',#84169,#56701,#56702);
#48302=AXIS2_PLACEMENT_3D('',#84172,#56703,#56704);
#48303=AXIS2_PLACEMENT_3D('',#84173,#56705,#56706);
#48304=AXIS2_PLACEMENT_3D('',#84174,#56707,#56708);
#48305=AXIS2_PLACEMENT_3D('',#84193,#56709,#56710);
#48306=AXIS2_PLACEMENT_3D('',#84194,#56711,#56712);
#48307=AXIS2_PLACEMENT_3D('',#84198,#56714,#56715);
#48308=AXIS2_PLACEMENT_3D('',#84200,#56716,#56717);
#48309=AXIS2_PLACEMENT_3D('',#84236,#56720,#56721);
#48310=AXIS2_PLACEMENT_3D('',#84244,#56723,#56724);
#48311=AXIS2_PLACEMENT_3D('',#84247,#56725,#56726);
#48312=AXIS2_PLACEMENT_3D('',#84248,#56727,#56728);
#48313=AXIS2_PLACEMENT_3D('',#84249,#56729,#56730);
#48314=AXIS2_PLACEMENT_3D('',#84264,#56731,#56732);
#48315=AXIS2_PLACEMENT_3D('',#84265,#56733,#56734);
#48316=AXIS2_PLACEMENT_3D('',#84269,#56736,#56737);
#48317=AXIS2_PLACEMENT_3D('',#84271,#56738,#56739);
#48318=AXIS2_PLACEMENT_3D('',#84305,#56742,#56743);
#48319=AXIS2_PLACEMENT_3D('',#84307,#56745,#56746);
#48320=AXIS2_PLACEMENT_3D('',#84308,#56747,#56748);
#48321=AXIS2_PLACEMENT_3D('',#84311,#56750,#56751);
#48322=AXIS2_PLACEMENT_3D('',#84312,#56752,#56753);
#48323=AXIS2_PLACEMENT_3D('',#84313,#56754,#56755);
#48324=AXIS2_PLACEMENT_3D('',#84332,#56756,#56757);
#48325=AXIS2_PLACEMENT_3D('',#84333,#56758,#56759);
#48326=AXIS2_PLACEMENT_3D('',#84343,#56760,#56761);
#48327=AXIS2_PLACEMENT_3D('',#84363,#56763,#56764);
#48328=AXIS2_PLACEMENT_3D('',#84371,#56766,#56767);
#48329=AXIS2_PLACEMENT_3D('',#84374,#56768,#56769);
#48330=AXIS2_PLACEMENT_3D('',#84375,#56770,#56771);
#48331=AXIS2_PLACEMENT_3D('',#84376,#56772,#56773);
#48332=AXIS2_PLACEMENT_3D('',#84385,#56774,#56775);
#48333=AXIS2_PLACEMENT_3D('',#84386,#56776,#56777);
#48334=AXIS2_PLACEMENT_3D('',#84390,#56779,#56780);
#48335=AXIS2_PLACEMENT_3D('',#84392,#56781,#56782);
#48336=AXIS2_PLACEMENT_3D('',#84417,#56785,#56786);
#48337=AXIS2_PLACEMENT_3D('',#84418,#56787,#56788);
#48338=AXIS2_PLACEMENT_3D('',#84437,#56789,#56790);
#48339=AXIS2_PLACEMENT_3D('',#84445,#56792,#56793);
#48340=AXIS2_PLACEMENT_3D('',#84448,#56794,#56795);
#48341=AXIS2_PLACEMENT_3D('',#84449,#56796,#56797);
#48342=AXIS2_PLACEMENT_3D('',#84450,#56798,#56799);
#48343=AXIS2_PLACEMENT_3D('',#84462,#56800,#56801);
#48344=AXIS2_PLACEMENT_3D('',#84463,#56802,#56803);
#48345=AXIS2_PLACEMENT_3D('',#84467,#56805,#56806);
#48346=AXIS2_PLACEMENT_3D('',#84469,#56807,#56808);
#48347=AXIS2_PLACEMENT_3D('',#84505,#56811,#56812);
#48348=AXIS2_PLACEMENT_3D('',#84513,#56814,#56815);
#48349=AXIS2_PLACEMENT_3D('',#84516,#56816,#56817);
#48350=AXIS2_PLACEMENT_3D('',#84517,#56818,#56819);
#48351=AXIS2_PLACEMENT_3D('',#84518,#56820,#56821);
#48352=AXIS2_PLACEMENT_3D('',#84554,#56823,#56824);
#48353=AXIS2_PLACEMENT_3D('',#84556,#56825,#56826);
#48354=AXIS2_PLACEMENT_3D('',#84611,#56830,#56831);
#48355=AXIS2_PLACEMENT_3D('',#84614,#56832,#56833);
#48356=AXIS2_PLACEMENT_3D('',#84621,#56834,#56835);
#48357=AXIS2_PLACEMENT_3D('',#84633,#56836,#56837);
#48358=AXIS2_PLACEMENT_3D('',#84634,#56838,#56839);
#48359=AXIS2_PLACEMENT_3D('',#84638,#56841,#56842);
#48360=AXIS2_PLACEMENT_3D('',#84640,#56843,#56844);
#48361=AXIS2_PLACEMENT_3D('',#84676,#56847,#56848);
#48362=AXIS2_PLACEMENT_3D('',#84684,#56850,#56851);
#48363=AXIS2_PLACEMENT_3D('',#84687,#56852,#56853);
#48364=AXIS2_PLACEMENT_3D('',#84688,#56854,#56855);
#48365=AXIS2_PLACEMENT_3D('',#84689,#56856,#56857);
#48366=AXIS2_PLACEMENT_3D('',#84708,#56858,#56859);
#48367=AXIS2_PLACEMENT_3D('',#84709,#56860,#56861);
#48368=AXIS2_PLACEMENT_3D('',#84713,#56863,#56864);
#48369=AXIS2_PLACEMENT_3D('',#84715,#56865,#56866);
#48370=AXIS2_PLACEMENT_3D('',#84751,#56869,#56870);
#48371=AXIS2_PLACEMENT_3D('',#84759,#56872,#56873);
#48372=AXIS2_PLACEMENT_3D('',#84762,#56874,#56875);
#48373=AXIS2_PLACEMENT_3D('',#84763,#56876,#56877);
#48374=AXIS2_PLACEMENT_3D('',#84764,#56878,#56879);
#48375=AXIS2_PLACEMENT_3D('',#84779,#56880,#56881);
#48376=AXIS2_PLACEMENT_3D('',#84780,#56882,#56883);
#48377=AXIS2_PLACEMENT_3D('',#84784,#56885,#56886);
#48378=AXIS2_PLACEMENT_3D('',#84786,#56887,#56888);
#48379=AXIS2_PLACEMENT_3D('',#84820,#56891,#56892);
#48380=AXIS2_PLACEMENT_3D('',#84822,#56894,#56895);
#48381=AXIS2_PLACEMENT_3D('',#84823,#56896,#56897);
#48382=AXIS2_PLACEMENT_3D('',#84826,#56899,#56900);
#48383=AXIS2_PLACEMENT_3D('',#84827,#56901,#56902);
#48384=AXIS2_PLACEMENT_3D('',#84828,#56903,#56904);
#48385=AXIS2_PLACEMENT_3D('',#84847,#56905,#56906);
#48386=AXIS2_PLACEMENT_3D('',#84848,#56907,#56908);
#48387=AXIS2_PLACEMENT_3D('',#84858,#56909,#56910);
#48388=AXIS2_PLACEMENT_3D('',#84878,#56912,#56913);
#48389=AXIS2_PLACEMENT_3D('',#84886,#56915,#56916);
#48390=AXIS2_PLACEMENT_3D('',#84889,#56917,#56918);
#48391=AXIS2_PLACEMENT_3D('',#84890,#56919,#56920);
#48392=AXIS2_PLACEMENT_3D('',#84891,#56921,#56922);
#48393=AXIS2_PLACEMENT_3D('',#84900,#56923,#56924);
#48394=AXIS2_PLACEMENT_3D('',#84901,#56925,#56926);
#48395=AXIS2_PLACEMENT_3D('',#84905,#56928,#56929);
#48396=AXIS2_PLACEMENT_3D('',#84907,#56930,#56931);
#48397=AXIS2_PLACEMENT_3D('',#84932,#56934,#56935);
#48398=AXIS2_PLACEMENT_3D('',#84933,#56936,#56937);
#48399=AXIS2_PLACEMENT_3D('',#84952,#56938,#56939);
#48400=AXIS2_PLACEMENT_3D('',#84960,#56941,#56942);
#48401=AXIS2_PLACEMENT_3D('',#84963,#56943,#56944);
#48402=AXIS2_PLACEMENT_3D('',#84964,#56945,#56946);
#48403=AXIS2_PLACEMENT_3D('',#84965,#56947,#56948);
#48404=AXIS2_PLACEMENT_3D('',#84977,#56949,#56950);
#48405=AXIS2_PLACEMENT_3D('',#84978,#56951,#56952);
#48406=AXIS2_PLACEMENT_3D('',#84982,#56954,#56955);
#48407=AXIS2_PLACEMENT_3D('',#84984,#56956,#56957);
#48408=AXIS2_PLACEMENT_3D('',#85020,#56960,#56961);
#48409=AXIS2_PLACEMENT_3D('',#85028,#56963,#56964);
#48410=AXIS2_PLACEMENT_3D('',#85031,#56965,#56966);
#48411=AXIS2_PLACEMENT_3D('',#85032,#56967,#56968);
#48412=AXIS2_PLACEMENT_3D('',#85033,#56969,#56970);
#48413=AXIS2_PLACEMENT_3D('',#85069,#56972,#56973);
#48414=AXIS2_PLACEMENT_3D('',#85071,#56974,#56975);
#48415=AXIS2_PLACEMENT_3D('',#85126,#56979,#56980);
#48416=AXIS2_PLACEMENT_3D('',#85129,#56981,#56982);
#48417=AXIS2_PLACEMENT_3D('',#85136,#56983,#56984);
#48418=AXIS2_PLACEMENT_3D('',#85148,#56985,#56986);
#48419=AXIS2_PLACEMENT_3D('',#85149,#56987,#56988);
#48420=AXIS2_PLACEMENT_3D('',#85153,#56990,#56991);
#48421=AXIS2_PLACEMENT_3D('',#85155,#56992,#56993);
#48422=AXIS2_PLACEMENT_3D('',#85191,#56996,#56997);
#48423=AXIS2_PLACEMENT_3D('',#85199,#56999,#57000);
#48424=AXIS2_PLACEMENT_3D('',#85202,#57001,#57002);
#48425=AXIS2_PLACEMENT_3D('',#85203,#57003,#57004);
#48426=AXIS2_PLACEMENT_3D('',#85204,#57005,#57006);
#48427=AXIS2_PLACEMENT_3D('',#85223,#57007,#57008);
#48428=AXIS2_PLACEMENT_3D('',#85224,#57009,#57010);
#48429=AXIS2_PLACEMENT_3D('',#85228,#57012,#57013);
#48430=AXIS2_PLACEMENT_3D('',#85230,#57014,#57015);
#48431=AXIS2_PLACEMENT_3D('',#85266,#57018,#57019);
#48432=AXIS2_PLACEMENT_3D('',#85274,#57021,#57022);
#48433=AXIS2_PLACEMENT_3D('',#85277,#57023,#57024);
#48434=AXIS2_PLACEMENT_3D('',#85278,#57025,#57026);
#48435=AXIS2_PLACEMENT_3D('',#85279,#57027,#57028);
#48436=AXIS2_PLACEMENT_3D('',#85294,#57029,#57030);
#48437=AXIS2_PLACEMENT_3D('',#85295,#57031,#57032);
#48438=AXIS2_PLACEMENT_3D('',#85299,#57034,#57035);
#48439=AXIS2_PLACEMENT_3D('',#85301,#57036,#57037);
#48440=AXIS2_PLACEMENT_3D('',#85335,#57040,#57041);
#48441=AXIS2_PLACEMENT_3D('',#85337,#57043,#57044);
#48442=AXIS2_PLACEMENT_3D('',#85338,#57045,#57046);
#48443=AXIS2_PLACEMENT_3D('',#85341,#57048,#57049);
#48444=AXIS2_PLACEMENT_3D('',#85342,#57050,#57051);
#48445=AXIS2_PLACEMENT_3D('',#85343,#57052,#57053);
#48446=AXIS2_PLACEMENT_3D('',#85362,#57054,#57055);
#48447=AXIS2_PLACEMENT_3D('',#85363,#57056,#57057);
#48448=AXIS2_PLACEMENT_3D('',#85373,#57058,#57059);
#48449=AXIS2_PLACEMENT_3D('',#85393,#57061,#57062);
#48450=AXIS2_PLACEMENT_3D('',#85401,#57064,#57065);
#48451=AXIS2_PLACEMENT_3D('',#85404,#57066,#57067);
#48452=AXIS2_PLACEMENT_3D('',#85405,#57068,#57069);
#48453=AXIS2_PLACEMENT_3D('',#85406,#57070,#57071);
#48454=AXIS2_PLACEMENT_3D('',#85415,#57072,#57073);
#48455=AXIS2_PLACEMENT_3D('',#85416,#57074,#57075);
#48456=AXIS2_PLACEMENT_3D('',#85420,#57077,#57078);
#48457=AXIS2_PLACEMENT_3D('',#85422,#57079,#57080);
#48458=AXIS2_PLACEMENT_3D('',#85447,#57083,#57084);
#48459=AXIS2_PLACEMENT_3D('',#85448,#57085,#57086);
#48460=AXIS2_PLACEMENT_3D('',#85467,#57087,#57088);
#48461=AXIS2_PLACEMENT_3D('',#85475,#57090,#57091);
#48462=AXIS2_PLACEMENT_3D('',#85478,#57092,#57093);
#48463=AXIS2_PLACEMENT_3D('',#85479,#57094,#57095);
#48464=AXIS2_PLACEMENT_3D('',#85480,#57096,#57097);
#48465=AXIS2_PLACEMENT_3D('',#85492,#57098,#57099);
#48466=AXIS2_PLACEMENT_3D('',#85493,#57100,#57101);
#48467=AXIS2_PLACEMENT_3D('',#85497,#57103,#57104);
#48468=AXIS2_PLACEMENT_3D('',#85499,#57105,#57106);
#48469=AXIS2_PLACEMENT_3D('',#85535,#57109,#57110);
#48470=AXIS2_PLACEMENT_3D('',#85543,#57112,#57113);
#48471=AXIS2_PLACEMENT_3D('',#85546,#57114,#57115);
#48472=AXIS2_PLACEMENT_3D('',#85547,#57116,#57117);
#48473=AXIS2_PLACEMENT_3D('',#85548,#57118,#57119);
#48474=AXIS2_PLACEMENT_3D('',#85584,#57121,#57122);
#48475=AXIS2_PLACEMENT_3D('',#85586,#57123,#57124);
#48476=AXIS2_PLACEMENT_3D('',#85641,#57128,#57129);
#48477=AXIS2_PLACEMENT_3D('',#85644,#57130,#57131);
#48478=AXIS2_PLACEMENT_3D('',#85651,#57132,#57133);
#48479=AXIS2_PLACEMENT_3D('',#85663,#57134,#57135);
#48480=AXIS2_PLACEMENT_3D('',#85664,#57136,#57137);
#48481=AXIS2_PLACEMENT_3D('',#85668,#57139,#57140);
#48482=AXIS2_PLACEMENT_3D('',#85670,#57141,#57142);
#48483=AXIS2_PLACEMENT_3D('',#85706,#57145,#57146);
#48484=AXIS2_PLACEMENT_3D('',#85714,#57148,#57149);
#48485=AXIS2_PLACEMENT_3D('',#85717,#57150,#57151);
#48486=AXIS2_PLACEMENT_3D('',#85718,#57152,#57153);
#48487=AXIS2_PLACEMENT_3D('',#85719,#57154,#57155);
#48488=AXIS2_PLACEMENT_3D('',#85738,#57156,#57157);
#48489=AXIS2_PLACEMENT_3D('',#85739,#57158,#57159);
#48490=AXIS2_PLACEMENT_3D('',#85743,#57161,#57162);
#48491=AXIS2_PLACEMENT_3D('',#85745,#57163,#57164);
#48492=AXIS2_PLACEMENT_3D('',#85781,#57167,#57168);
#48493=AXIS2_PLACEMENT_3D('',#85789,#57170,#57171);
#48494=AXIS2_PLACEMENT_3D('',#85792,#57172,#57173);
#48495=AXIS2_PLACEMENT_3D('',#85793,#57174,#57175);
#48496=AXIS2_PLACEMENT_3D('',#85794,#57176,#57177);
#48497=AXIS2_PLACEMENT_3D('',#85809,#57178,#57179);
#48498=AXIS2_PLACEMENT_3D('',#85810,#57180,#57181);
#48499=AXIS2_PLACEMENT_3D('',#85814,#57183,#57184);
#48500=AXIS2_PLACEMENT_3D('',#85816,#57185,#57186);
#48501=AXIS2_PLACEMENT_3D('',#85850,#57189,#57190);
#48502=AXIS2_PLACEMENT_3D('',#85852,#57192,#57193);
#48503=AXIS2_PLACEMENT_3D('',#85853,#57194,#57195);
#48504=AXIS2_PLACEMENT_3D('',#85856,#57197,#57198);
#48505=AXIS2_PLACEMENT_3D('',#85857,#57199,#57200);
#48506=AXIS2_PLACEMENT_3D('',#85858,#57201,#57202);
#48507=AXIS2_PLACEMENT_3D('',#85877,#57203,#57204);
#48508=AXIS2_PLACEMENT_3D('',#85878,#57205,#57206);
#48509=AXIS2_PLACEMENT_3D('',#85888,#57207,#57208);
#48510=AXIS2_PLACEMENT_3D('',#85908,#57210,#57211);
#48511=AXIS2_PLACEMENT_3D('',#85916,#57213,#57214);
#48512=AXIS2_PLACEMENT_3D('',#85919,#57215,#57216);
#48513=AXIS2_PLACEMENT_3D('',#85920,#57217,#57218);
#48514=AXIS2_PLACEMENT_3D('',#85921,#57219,#57220);
#48515=AXIS2_PLACEMENT_3D('',#85930,#57221,#57222);
#48516=AXIS2_PLACEMENT_3D('',#85931,#57223,#57224);
#48517=AXIS2_PLACEMENT_3D('',#85935,#57226,#57227);
#48518=AXIS2_PLACEMENT_3D('',#85937,#57228,#57229);
#48519=AXIS2_PLACEMENT_3D('',#85962,#57232,#57233);
#48520=AXIS2_PLACEMENT_3D('',#85963,#57234,#57235);
#48521=AXIS2_PLACEMENT_3D('',#85982,#57236,#57237);
#48522=AXIS2_PLACEMENT_3D('',#85990,#57239,#57240);
#48523=AXIS2_PLACEMENT_3D('',#85993,#57241,#57242);
#48524=AXIS2_PLACEMENT_3D('',#85994,#57243,#57244);
#48525=AXIS2_PLACEMENT_3D('',#85995,#57245,#57246);
#48526=AXIS2_PLACEMENT_3D('',#86007,#57247,#57248);
#48527=AXIS2_PLACEMENT_3D('',#86008,#57249,#57250);
#48528=AXIS2_PLACEMENT_3D('',#86012,#57252,#57253);
#48529=AXIS2_PLACEMENT_3D('',#86014,#57254,#57255);
#48530=AXIS2_PLACEMENT_3D('',#86050,#57258,#57259);
#48531=AXIS2_PLACEMENT_3D('',#86058,#57261,#57262);
#48532=AXIS2_PLACEMENT_3D('',#86061,#57263,#57264);
#48533=AXIS2_PLACEMENT_3D('',#86062,#57265,#57266);
#48534=AXIS2_PLACEMENT_3D('',#86063,#57267,#57268);
#48535=AXIS2_PLACEMENT_3D('',#86099,#57270,#57271);
#48536=AXIS2_PLACEMENT_3D('',#86101,#57272,#57273);
#48537=AXIS2_PLACEMENT_3D('',#86156,#57277,#57278);
#48538=AXIS2_PLACEMENT_3D('',#86159,#57279,#57280);
#48539=AXIS2_PLACEMENT_3D('',#86166,#57281,#57282);
#48540=AXIS2_PLACEMENT_3D('',#86178,#57283,#57284);
#48541=AXIS2_PLACEMENT_3D('',#86179,#57285,#57286);
#48542=AXIS2_PLACEMENT_3D('',#86183,#57288,#57289);
#48543=AXIS2_PLACEMENT_3D('',#86185,#57290,#57291);
#48544=AXIS2_PLACEMENT_3D('',#86221,#57294,#57295);
#48545=AXIS2_PLACEMENT_3D('',#86229,#57297,#57298);
#48546=AXIS2_PLACEMENT_3D('',#86232,#57299,#57300);
#48547=AXIS2_PLACEMENT_3D('',#86233,#57301,#57302);
#48548=AXIS2_PLACEMENT_3D('',#86234,#57303,#57304);
#48549=AXIS2_PLACEMENT_3D('',#86253,#57305,#57306);
#48550=AXIS2_PLACEMENT_3D('',#86254,#57307,#57308);
#48551=AXIS2_PLACEMENT_3D('',#86258,#57310,#57311);
#48552=AXIS2_PLACEMENT_3D('',#86260,#57312,#57313);
#48553=AXIS2_PLACEMENT_3D('',#86296,#57316,#57317);
#48554=AXIS2_PLACEMENT_3D('',#86304,#57319,#57320);
#48555=AXIS2_PLACEMENT_3D('',#86307,#57321,#57322);
#48556=AXIS2_PLACEMENT_3D('',#86308,#57323,#57324);
#48557=AXIS2_PLACEMENT_3D('',#86309,#57325,#57326);
#48558=AXIS2_PLACEMENT_3D('',#86324,#57327,#57328);
#48559=AXIS2_PLACEMENT_3D('',#86325,#57329,#57330);
#48560=AXIS2_PLACEMENT_3D('',#86329,#57332,#57333);
#48561=AXIS2_PLACEMENT_3D('',#86331,#57334,#57335);
#48562=AXIS2_PLACEMENT_3D('',#86365,#57338,#57339);
#48563=AXIS2_PLACEMENT_3D('',#86367,#57341,#57342);
#48564=AXIS2_PLACEMENT_3D('',#86368,#57343,#57344);
#48565=AXIS2_PLACEMENT_3D('',#86371,#57346,#57347);
#48566=AXIS2_PLACEMENT_3D('',#86372,#57348,#57349);
#48567=AXIS2_PLACEMENT_3D('',#86373,#57350,#57351);
#48568=AXIS2_PLACEMENT_3D('',#86392,#57352,#57353);
#48569=AXIS2_PLACEMENT_3D('',#86393,#57354,#57355);
#48570=AXIS2_PLACEMENT_3D('',#86403,#57356,#57357);
#48571=AXIS2_PLACEMENT_3D('',#86423,#57359,#57360);
#48572=AXIS2_PLACEMENT_3D('',#86431,#57362,#57363);
#48573=AXIS2_PLACEMENT_3D('',#86434,#57364,#57365);
#48574=AXIS2_PLACEMENT_3D('',#86435,#57366,#57367);
#48575=AXIS2_PLACEMENT_3D('',#86436,#57368,#57369);
#48576=AXIS2_PLACEMENT_3D('',#86445,#57370,#57371);
#48577=AXIS2_PLACEMENT_3D('',#86446,#57372,#57373);
#48578=AXIS2_PLACEMENT_3D('',#86450,#57375,#57376);
#48579=AXIS2_PLACEMENT_3D('',#86452,#57377,#57378);
#48580=AXIS2_PLACEMENT_3D('',#86477,#57381,#57382);
#48581=AXIS2_PLACEMENT_3D('',#86478,#57383,#57384);
#48582=AXIS2_PLACEMENT_3D('',#86497,#57385,#57386);
#48583=AXIS2_PLACEMENT_3D('',#86505,#57388,#57389);
#48584=AXIS2_PLACEMENT_3D('',#86508,#57390,#57391);
#48585=AXIS2_PLACEMENT_3D('',#86509,#57392,#57393);
#48586=AXIS2_PLACEMENT_3D('',#86510,#57394,#57395);
#48587=AXIS2_PLACEMENT_3D('',#86522,#57396,#57397);
#48588=AXIS2_PLACEMENT_3D('',#86523,#57398,#57399);
#48589=AXIS2_PLACEMENT_3D('',#86527,#57401,#57402);
#48590=AXIS2_PLACEMENT_3D('',#86529,#57403,#57404);
#48591=AXIS2_PLACEMENT_3D('',#86565,#57407,#57408);
#48592=AXIS2_PLACEMENT_3D('',#86573,#57410,#57411);
#48593=AXIS2_PLACEMENT_3D('',#86576,#57412,#57413);
#48594=AXIS2_PLACEMENT_3D('',#86577,#57414,#57415);
#48595=AXIS2_PLACEMENT_3D('',#86578,#57416,#57417);
#48596=AXIS2_PLACEMENT_3D('',#86614,#57419,#57420);
#48597=AXIS2_PLACEMENT_3D('',#86616,#57421,#57422);
#48598=AXIS2_PLACEMENT_3D('',#86671,#57426,#57427);
#48599=AXIS2_PLACEMENT_3D('',#86674,#57428,#57429);
#48600=AXIS2_PLACEMENT_3D('',#86681,#57430,#57431);
#48601=AXIS2_PLACEMENT_3D('',#86693,#57432,#57433);
#48602=AXIS2_PLACEMENT_3D('',#86694,#57434,#57435);
#48603=AXIS2_PLACEMENT_3D('',#86698,#57437,#57438);
#48604=AXIS2_PLACEMENT_3D('',#86700,#57439,#57440);
#48605=AXIS2_PLACEMENT_3D('',#86736,#57443,#57444);
#48606=AXIS2_PLACEMENT_3D('',#86744,#57446,#57447);
#48607=AXIS2_PLACEMENT_3D('',#86747,#57448,#57449);
#48608=AXIS2_PLACEMENT_3D('',#86748,#57450,#57451);
#48609=AXIS2_PLACEMENT_3D('',#86749,#57452,#57453);
#48610=AXIS2_PLACEMENT_3D('',#86768,#57454,#57455);
#48611=AXIS2_PLACEMENT_3D('',#86769,#57456,#57457);
#48612=AXIS2_PLACEMENT_3D('',#86773,#57459,#57460);
#48613=AXIS2_PLACEMENT_3D('',#86775,#57461,#57462);
#48614=AXIS2_PLACEMENT_3D('',#86811,#57465,#57466);
#48615=AXIS2_PLACEMENT_3D('',#86819,#57468,#57469);
#48616=AXIS2_PLACEMENT_3D('',#86822,#57470,#57471);
#48617=AXIS2_PLACEMENT_3D('',#86823,#57472,#57473);
#48618=AXIS2_PLACEMENT_3D('',#86824,#57474,#57475);
#48619=AXIS2_PLACEMENT_3D('',#86839,#57476,#57477);
#48620=AXIS2_PLACEMENT_3D('',#86840,#57478,#57479);
#48621=AXIS2_PLACEMENT_3D('',#86844,#57481,#57482);
#48622=AXIS2_PLACEMENT_3D('',#86846,#57483,#57484);
#48623=AXIS2_PLACEMENT_3D('',#86880,#57487,#57488);
#48624=AXIS2_PLACEMENT_3D('',#86882,#57490,#57491);
#48625=AXIS2_PLACEMENT_3D('',#86883,#57492,#57493);
#48626=AXIS2_PLACEMENT_3D('',#86886,#57495,#57496);
#48627=AXIS2_PLACEMENT_3D('',#86887,#57497,#57498);
#48628=AXIS2_PLACEMENT_3D('',#86888,#57499,#57500);
#48629=AXIS2_PLACEMENT_3D('',#86907,#57501,#57502);
#48630=AXIS2_PLACEMENT_3D('',#86908,#57503,#57504);
#48631=AXIS2_PLACEMENT_3D('',#86918,#57505,#57506);
#48632=AXIS2_PLACEMENT_3D('',#86938,#57508,#57509);
#48633=AXIS2_PLACEMENT_3D('',#86946,#57511,#57512);
#48634=AXIS2_PLACEMENT_3D('',#86949,#57513,#57514);
#48635=AXIS2_PLACEMENT_3D('',#86950,#57515,#57516);
#48636=AXIS2_PLACEMENT_3D('',#86951,#57517,#57518);
#48637=AXIS2_PLACEMENT_3D('',#86960,#57519,#57520);
#48638=AXIS2_PLACEMENT_3D('',#86961,#57521,#57522);
#48639=AXIS2_PLACEMENT_3D('',#86965,#57524,#57525);
#48640=AXIS2_PLACEMENT_3D('',#86967,#57526,#57527);
#48641=AXIS2_PLACEMENT_3D('',#86992,#57530,#57531);
#48642=AXIS2_PLACEMENT_3D('',#86993,#57532,#57533);
#48643=AXIS2_PLACEMENT_3D('',#87012,#57534,#57535);
#48644=AXIS2_PLACEMENT_3D('',#87020,#57537,#57538);
#48645=AXIS2_PLACEMENT_3D('',#87023,#57539,#57540);
#48646=AXIS2_PLACEMENT_3D('',#87024,#57541,#57542);
#48647=AXIS2_PLACEMENT_3D('',#87025,#57543,#57544);
#48648=AXIS2_PLACEMENT_3D('',#87037,#57545,#57546);
#48649=AXIS2_PLACEMENT_3D('',#87038,#57547,#57548);
#48650=AXIS2_PLACEMENT_3D('',#87042,#57550,#57551);
#48651=AXIS2_PLACEMENT_3D('',#87044,#57552,#57553);
#48652=AXIS2_PLACEMENT_3D('',#87080,#57556,#57557);
#48653=AXIS2_PLACEMENT_3D('',#87088,#57559,#57560);
#48654=AXIS2_PLACEMENT_3D('',#87091,#57561,#57562);
#48655=AXIS2_PLACEMENT_3D('',#87092,#57563,#57564);
#48656=AXIS2_PLACEMENT_3D('',#87093,#57565,#57566);
#48657=AXIS2_PLACEMENT_3D('',#87129,#57568,#57569);
#48658=AXIS2_PLACEMENT_3D('',#87131,#57570,#57571);
#48659=AXIS2_PLACEMENT_3D('',#87186,#57575,#57576);
#48660=AXIS2_PLACEMENT_3D('',#87189,#57577,#57578);
#48661=AXIS2_PLACEMENT_3D('',#87196,#57579,#57580);
#48662=AXIS2_PLACEMENT_3D('',#87208,#57581,#57582);
#48663=AXIS2_PLACEMENT_3D('',#87209,#57583,#57584);
#48664=AXIS2_PLACEMENT_3D('',#87213,#57586,#57587);
#48665=AXIS2_PLACEMENT_3D('',#87215,#57588,#57589);
#48666=AXIS2_PLACEMENT_3D('',#87251,#57592,#57593);
#48667=AXIS2_PLACEMENT_3D('',#87259,#57595,#57596);
#48668=AXIS2_PLACEMENT_3D('',#87262,#57597,#57598);
#48669=AXIS2_PLACEMENT_3D('',#87263,#57599,#57600);
#48670=AXIS2_PLACEMENT_3D('',#87264,#57601,#57602);
#48671=AXIS2_PLACEMENT_3D('',#87283,#57603,#57604);
#48672=AXIS2_PLACEMENT_3D('',#87284,#57605,#57606);
#48673=AXIS2_PLACEMENT_3D('',#87288,#57608,#57609);
#48674=AXIS2_PLACEMENT_3D('',#87290,#57610,#57611);
#48675=AXIS2_PLACEMENT_3D('',#87326,#57614,#57615);
#48676=AXIS2_PLACEMENT_3D('',#87334,#57617,#57618);
#48677=AXIS2_PLACEMENT_3D('',#87337,#57619,#57620);
#48678=AXIS2_PLACEMENT_3D('',#87338,#57621,#57622);
#48679=AXIS2_PLACEMENT_3D('',#87339,#57623,#57624);
#48680=AXIS2_PLACEMENT_3D('',#87354,#57625,#57626);
#48681=AXIS2_PLACEMENT_3D('',#87355,#57627,#57628);
#48682=AXIS2_PLACEMENT_3D('',#87359,#57630,#57631);
#48683=AXIS2_PLACEMENT_3D('',#87361,#57632,#57633);
#48684=AXIS2_PLACEMENT_3D('',#87395,#57636,#57637);
#48685=AXIS2_PLACEMENT_3D('',#87397,#57639,#57640);
#48686=AXIS2_PLACEMENT_3D('',#87398,#57641,#57642);
#48687=AXIS2_PLACEMENT_3D('',#87401,#57644,#57645);
#48688=AXIS2_PLACEMENT_3D('',#87402,#57646,#57647);
#48689=AXIS2_PLACEMENT_3D('',#87403,#57648,#57649);
#48690=AXIS2_PLACEMENT_3D('',#87422,#57650,#57651);
#48691=AXIS2_PLACEMENT_3D('',#87423,#57652,#57653);
#48692=AXIS2_PLACEMENT_3D('',#87433,#57654,#57655);
#48693=AXIS2_PLACEMENT_3D('',#87453,#57657,#57658);
#48694=AXIS2_PLACEMENT_3D('',#87461,#57660,#57661);
#48695=AXIS2_PLACEMENT_3D('',#87464,#57662,#57663);
#48696=AXIS2_PLACEMENT_3D('',#87465,#57664,#57665);
#48697=AXIS2_PLACEMENT_3D('',#87466,#57666,#57667);
#48698=AXIS2_PLACEMENT_3D('',#87475,#57668,#57669);
#48699=AXIS2_PLACEMENT_3D('',#87476,#57670,#57671);
#48700=AXIS2_PLACEMENT_3D('',#87480,#57673,#57674);
#48701=AXIS2_PLACEMENT_3D('',#87482,#57675,#57676);
#48702=AXIS2_PLACEMENT_3D('',#87507,#57679,#57680);
#48703=AXIS2_PLACEMENT_3D('',#87508,#57681,#57682);
#48704=AXIS2_PLACEMENT_3D('',#87527,#57683,#57684);
#48705=AXIS2_PLACEMENT_3D('',#87535,#57686,#57687);
#48706=AXIS2_PLACEMENT_3D('',#87538,#57688,#57689);
#48707=AXIS2_PLACEMENT_3D('',#87539,#57690,#57691);
#48708=AXIS2_PLACEMENT_3D('',#87540,#57692,#57693);
#48709=AXIS2_PLACEMENT_3D('',#87552,#57694,#57695);
#48710=AXIS2_PLACEMENT_3D('',#87553,#57696,#57697);
#48711=AXIS2_PLACEMENT_3D('',#87557,#57699,#57700);
#48712=AXIS2_PLACEMENT_3D('',#87559,#57701,#57702);
#48713=AXIS2_PLACEMENT_3D('',#87595,#57705,#57706);
#48714=AXIS2_PLACEMENT_3D('',#87603,#57708,#57709);
#48715=AXIS2_PLACEMENT_3D('',#87606,#57710,#57711);
#48716=AXIS2_PLACEMENT_3D('',#87607,#57712,#57713);
#48717=AXIS2_PLACEMENT_3D('',#87608,#57714,#57715);
#48718=AXIS2_PLACEMENT_3D('',#87644,#57717,#57718);
#48719=AXIS2_PLACEMENT_3D('',#87646,#57719,#57720);
#48720=AXIS2_PLACEMENT_3D('',#87701,#57724,#57725);
#48721=AXIS2_PLACEMENT_3D('',#87704,#57726,#57727);
#48722=AXIS2_PLACEMENT_3D('',#87711,#57728,#57729);
#48723=AXIS2_PLACEMENT_3D('',#87723,#57730,#57731);
#48724=AXIS2_PLACEMENT_3D('',#87724,#57732,#57733);
#48725=AXIS2_PLACEMENT_3D('',#87728,#57735,#57736);
#48726=AXIS2_PLACEMENT_3D('',#87730,#57737,#57738);
#48727=AXIS2_PLACEMENT_3D('',#87766,#57741,#57742);
#48728=AXIS2_PLACEMENT_3D('',#87774,#57744,#57745);
#48729=AXIS2_PLACEMENT_3D('',#87777,#57746,#57747);
#48730=AXIS2_PLACEMENT_3D('',#87778,#57748,#57749);
#48731=AXIS2_PLACEMENT_3D('',#87779,#57750,#57751);
#48732=AXIS2_PLACEMENT_3D('',#87798,#57752,#57753);
#48733=AXIS2_PLACEMENT_3D('',#87799,#57754,#57755);
#48734=AXIS2_PLACEMENT_3D('',#87803,#57757,#57758);
#48735=AXIS2_PLACEMENT_3D('',#87805,#57759,#57760);
#48736=AXIS2_PLACEMENT_3D('',#87841,#57763,#57764);
#48737=AXIS2_PLACEMENT_3D('',#87849,#57766,#57767);
#48738=AXIS2_PLACEMENT_3D('',#87852,#57768,#57769);
#48739=AXIS2_PLACEMENT_3D('',#87853,#57770,#57771);
#48740=AXIS2_PLACEMENT_3D('',#87854,#57772,#57773);
#48741=AXIS2_PLACEMENT_3D('',#87869,#57774,#57775);
#48742=AXIS2_PLACEMENT_3D('',#87870,#57776,#57777);
#48743=AXIS2_PLACEMENT_3D('',#87874,#57779,#57780);
#48744=AXIS2_PLACEMENT_3D('',#87876,#57781,#57782);
#48745=AXIS2_PLACEMENT_3D('',#87910,#57785,#57786);
#48746=AXIS2_PLACEMENT_3D('',#87912,#57788,#57789);
#48747=AXIS2_PLACEMENT_3D('',#87913,#57790,#57791);
#48748=AXIS2_PLACEMENT_3D('',#87916,#57793,#57794);
#48749=AXIS2_PLACEMENT_3D('',#87917,#57795,#57796);
#48750=AXIS2_PLACEMENT_3D('',#87918,#57797,#57798);
#48751=AXIS2_PLACEMENT_3D('',#87919,#57799,#57800);
#48752=AXIS2_PLACEMENT_3D('',#87922,#57801,#57802);
#48753=AXIS2_PLACEMENT_3D('',#87924,#57803,#57804);
#48754=AXIS2_PLACEMENT_3D('',#87926,#57805,#57806);
#48755=AXIS2_PLACEMENT_3D('',#87927,#57807,#57808);
#48756=AXIS2_PLACEMENT_3D('',#87946,#57809,#57810);
#48757=AXIS2_PLACEMENT_3D('',#87947,#57811,#57812);
#48758=AXIS2_PLACEMENT_3D('',#87957,#57813,#57814);
#48759=AXIS2_PLACEMENT_3D('',#87990,#57817,#57818);
#48760=AXIS2_PLACEMENT_3D('',#87991,#57819,#57820);
#48761=AXIS2_PLACEMENT_3D('',#87995,#57822,#57823);
#48762=AXIS2_PLACEMENT_3D('',#87997,#57824,#57825);
#48763=AXIS2_PLACEMENT_3D('',#88022,#57828,#57829);
#48764=AXIS2_PLACEMENT_3D('',#88023,#57830,#57831);
#48765=AXIS2_PLACEMENT_3D('',#88042,#57832,#57833);
#48766=AXIS2_PLACEMENT_3D('',#88050,#57835,#57836);
#48767=AXIS2_PLACEMENT_3D('',#88053,#57837,#57838);
#48768=AXIS2_PLACEMENT_3D('',#88054,#57839,#57840);
#48769=AXIS2_PLACEMENT_3D('',#88055,#57841,#57842);
#48770=AXIS2_PLACEMENT_3D('',#88067,#57843,#57844);
#48771=AXIS2_PLACEMENT_3D('',#88068,#57845,#57846);
#48772=AXIS2_PLACEMENT_3D('',#88072,#57848,#57849);
#48773=AXIS2_PLACEMENT_3D('',#88074,#57850,#57851);
#48774=AXIS2_PLACEMENT_3D('',#88110,#57854,#57855);
#48775=AXIS2_PLACEMENT_3D('',#88118,#57857,#57858);
#48776=AXIS2_PLACEMENT_3D('',#88121,#57859,#57860);
#48777=AXIS2_PLACEMENT_3D('',#88122,#57861,#57862);
#48778=AXIS2_PLACEMENT_3D('',#88123,#57863,#57864);
#48779=AXIS2_PLACEMENT_3D('',#88159,#57866,#57867);
#48780=AXIS2_PLACEMENT_3D('',#88161,#57868,#57869);
#48781=AXIS2_PLACEMENT_3D('',#88216,#57873,#57874);
#48782=AXIS2_PLACEMENT_3D('',#88219,#57875,#57876);
#48783=AXIS2_PLACEMENT_3D('',#88226,#57877,#57878);
#48784=AXIS2_PLACEMENT_3D('',#88238,#57879,#57880);
#48785=AXIS2_PLACEMENT_3D('',#88239,#57881,#57882);
#48786=AXIS2_PLACEMENT_3D('',#88243,#57884,#57885);
#48787=AXIS2_PLACEMENT_3D('',#88245,#57886,#57887);
#48788=AXIS2_PLACEMENT_3D('',#88281,#57890,#57891);
#48789=AXIS2_PLACEMENT_3D('',#88289,#57893,#57894);
#48790=AXIS2_PLACEMENT_3D('',#88292,#57895,#57896);
#48791=AXIS2_PLACEMENT_3D('',#88293,#57897,#57898);
#48792=AXIS2_PLACEMENT_3D('',#88294,#57899,#57900);
#48793=AXIS2_PLACEMENT_3D('',#88313,#57901,#57902);
#48794=AXIS2_PLACEMENT_3D('',#88314,#57903,#57904);
#48795=AXIS2_PLACEMENT_3D('',#88318,#57906,#57907);
#48796=AXIS2_PLACEMENT_3D('',#88320,#57908,#57909);
#48797=AXIS2_PLACEMENT_3D('',#88356,#57912,#57913);
#48798=AXIS2_PLACEMENT_3D('',#88364,#57915,#57916);
#48799=AXIS2_PLACEMENT_3D('',#88367,#57917,#57918);
#48800=AXIS2_PLACEMENT_3D('',#88368,#57919,#57920);
#48801=AXIS2_PLACEMENT_3D('',#88369,#57921,#57922);
#48802=AXIS2_PLACEMENT_3D('',#88384,#57923,#57924);
#48803=AXIS2_PLACEMENT_3D('',#88385,#57925,#57926);
#48804=AXIS2_PLACEMENT_3D('',#88389,#57928,#57929);
#48805=AXIS2_PLACEMENT_3D('',#88391,#57930,#57931);
#48806=AXIS2_PLACEMENT_3D('',#88425,#57934,#57935);
#48807=AXIS2_PLACEMENT_3D('',#88427,#57937,#57938);
#48808=AXIS2_PLACEMENT_3D('',#88428,#57939,#57940);
#48809=AXIS2_PLACEMENT_3D('',#88431,#57942,#57943);
#48810=AXIS2_PLACEMENT_3D('',#88432,#57944,#57945);
#48811=AXIS2_PLACEMENT_3D('',#88433,#57946,#57947);
#48812=AXIS2_PLACEMENT_3D('',#88434,#57948,#57949);
#48813=AXIS2_PLACEMENT_3D('',#88437,#57950,#57951);
#48814=AXIS2_PLACEMENT_3D('',#88439,#57952,#57953);
#48815=AXIS2_PLACEMENT_3D('',#88441,#57954,#57955);
#48816=AXIS2_PLACEMENT_3D('',#88442,#57956,#57957);
#48817=AXIS2_PLACEMENT_3D('',#88443,#57958,#57959);
#48818=AXIS2_PLACEMENT_3D('',#88446,#57960,#57961);
#48819=AXIS2_PLACEMENT_3D('',#88448,#57962,#57963);
#48820=AXIS2_PLACEMENT_3D('',#88450,#57964,#57965);
#48821=AXIS2_PLACEMENT_3D('',#88451,#57966,#57967);
#48822=AXIS2_PLACEMENT_3D('',#88470,#57968,#57969);
#48823=AXIS2_PLACEMENT_3D('',#88471,#57970,#57971);
#48824=AXIS2_PLACEMENT_3D('',#88481,#57972,#57973);
#48825=AXIS2_PLACEMENT_3D('',#88517,#57976,#57977);
#48826=AXIS2_PLACEMENT_3D('',#88518,#57978,#57979);
#48827=AXIS2_PLACEMENT_3D('',#88522,#57981,#57982);
#48828=AXIS2_PLACEMENT_3D('',#88524,#57983,#57984);
#48829=AXIS2_PLACEMENT_3D('',#88549,#57987,#57988);
#48830=AXIS2_PLACEMENT_3D('',#88550,#57989,#57990);
#48831=AXIS2_PLACEMENT_3D('',#88582,#57992,#57993);
#48832=AXIS2_PLACEMENT_3D('',#88583,#57994,#57995);
#48833=AXIS2_PLACEMENT_3D('',#88587,#57997,#57998);
#48834=AXIS2_PLACEMENT_3D('',#88589,#57999,#58000);
#48835=AXIS2_PLACEMENT_3D('',#88632,#58003,#58004);
#48836=AXIS2_PLACEMENT_3D('',#88640,#58006,#58007);
#48837=AXIS2_PLACEMENT_3D('',#88643,#58008,#58009);
#48838=AXIS2_PLACEMENT_3D('',#88644,#58010,#58011);
#48839=AXIS2_PLACEMENT_3D('',#88645,#58012,#58013);
#48840=AXIS2_PLACEMENT_3D('',#88681,#58015,#58016);
#48841=AXIS2_PLACEMENT_3D('',#88683,#58017,#58018);
#48842=AXIS2_PLACEMENT_3D('',#88738,#58022,#58023);
#48843=AXIS2_PLACEMENT_3D('',#88741,#58024,#58025);
#48844=AXIS2_PLACEMENT_3D('',#88748,#58026,#58027);
#48845=AXIS2_PLACEMENT_3D('',#88760,#58028,#58029);
#48846=AXIS2_PLACEMENT_3D('',#88761,#58030,#58031);
#48847=AXIS2_PLACEMENT_3D('',#88765,#58033,#58034);
#48848=AXIS2_PLACEMENT_3D('',#88767,#58035,#58036);
#48849=AXIS2_PLACEMENT_3D('',#88803,#58039,#58040);
#48850=AXIS2_PLACEMENT_3D('',#88811,#58042,#58043);
#48851=AXIS2_PLACEMENT_3D('',#88814,#58044,#58045);
#48852=AXIS2_PLACEMENT_3D('',#88815,#58046,#58047);
#48853=AXIS2_PLACEMENT_3D('',#88816,#58048,#58049);
#48854=AXIS2_PLACEMENT_3D('',#88835,#58050,#58051);
#48855=AXIS2_PLACEMENT_3D('',#88836,#58052,#58053);
#48856=AXIS2_PLACEMENT_3D('',#88840,#58055,#58056);
#48857=AXIS2_PLACEMENT_3D('',#88842,#58057,#58058);
#48858=AXIS2_PLACEMENT_3D('',#88878,#58061,#58062);
#48859=AXIS2_PLACEMENT_3D('',#88886,#58064,#58065);
#48860=AXIS2_PLACEMENT_3D('',#88889,#58066,#58067);
#48861=AXIS2_PLACEMENT_3D('',#88890,#58068,#58069);
#48862=AXIS2_PLACEMENT_3D('',#88891,#58070,#58071);
#48863=AXIS2_PLACEMENT_3D('',#88906,#58072,#58073);
#48864=AXIS2_PLACEMENT_3D('',#88907,#58074,#58075);
#48865=AXIS2_PLACEMENT_3D('',#88911,#58077,#58078);
#48866=AXIS2_PLACEMENT_3D('',#88913,#58079,#58080);
#48867=AXIS2_PLACEMENT_3D('',#88947,#58083,#58084);
#48868=AXIS2_PLACEMENT_3D('',#88949,#58086,#58087);
#48869=AXIS2_PLACEMENT_3D('',#88950,#58088,#58089);
#48870=AXIS2_PLACEMENT_3D('',#88953,#58091,#58092);
#48871=AXIS2_PLACEMENT_3D('',#88954,#58093,#58094);
#48872=AXIS2_PLACEMENT_3D('',#88955,#58095,#58096);
#48873=AXIS2_PLACEMENT_3D('',#88956,#58097,#58098);
#48874=AXIS2_PLACEMENT_3D('',#88959,#58099,#58100);
#48875=AXIS2_PLACEMENT_3D('',#88961,#58101,#58102);
#48876=AXIS2_PLACEMENT_3D('',#88963,#58103,#58104);
#48877=AXIS2_PLACEMENT_3D('',#88964,#58105,#58106);
#48878=AXIS2_PLACEMENT_3D('',#88965,#58107,#58108);
#48879=AXIS2_PLACEMENT_3D('',#88968,#58109,#58110);
#48880=AXIS2_PLACEMENT_3D('',#88970,#58111,#58112);
#48881=AXIS2_PLACEMENT_3D('',#88972,#58113,#58114);
#48882=AXIS2_PLACEMENT_3D('',#88973,#58115,#58116);
#48883=AXIS2_PLACEMENT_3D('',#88974,#58117,#58118);
#48884=AXIS2_PLACEMENT_3D('',#88977,#58119,#58120);
#48885=AXIS2_PLACEMENT_3D('',#88979,#58121,#58122);
#48886=AXIS2_PLACEMENT_3D('',#88981,#58123,#58124);
#48887=AXIS2_PLACEMENT_3D('',#88982,#58125,#58126);
#48888=AXIS2_PLACEMENT_3D('',#88991,#58127,#58128);
#48889=AXIS2_PLACEMENT_3D('',#88992,#58129,#58130);
#48890=AXIS2_PLACEMENT_3D('',#88996,#58132,#58133);
#48891=AXIS2_PLACEMENT_3D('',#88998,#58134,#58135);
#48892=AXIS2_PLACEMENT_3D('',#89023,#58138,#58139);
#48893=AXIS2_PLACEMENT_3D('',#89024,#58140,#58141);
#48894=AXIS2_PLACEMENT_3D('',#89062,#58143,#58144);
#48895=AXIS2_PLACEMENT_3D('',#89063,#58145,#58146);
#48896=AXIS2_PLACEMENT_3D('',#89067,#58148,#58149);
#48897=AXIS2_PLACEMENT_3D('',#89069,#58150,#58151);
#48898=AXIS2_PLACEMENT_3D('',#89144,#58156,#58157);
#48899=AXIS2_PLACEMENT_3D('',#89146,#58158,#58159);
#48900=AXIS2_PLACEMENT_3D('',#89207,#58163,#58164);
#48901=AXIS2_PLACEMENT_3D('',#89208,#58165,#58166);
#48902=AXIS2_PLACEMENT_3D('',#89218,#58167,#58168);
#48903=AXIS2_PLACEMENT_3D('',#89243,#58171,#58172);
#48904=AXIS2_PLACEMENT_3D('',#89246,#58173,#58174);
#48905=AXIS2_PLACEMENT_3D('',#89253,#58175,#58176);
#48906=AXIS2_PLACEMENT_3D('',#89265,#58177,#58178);
#48907=AXIS2_PLACEMENT_3D('',#89266,#58179,#58180);
#48908=AXIS2_PLACEMENT_3D('',#89270,#58182,#58183);
#48909=AXIS2_PLACEMENT_3D('',#89272,#58184,#58185);
#48910=AXIS2_PLACEMENT_3D('',#89308,#58188,#58189);
#48911=AXIS2_PLACEMENT_3D('',#89316,#58191,#58192);
#48912=AXIS2_PLACEMENT_3D('',#89319,#58193,#58194);
#48913=AXIS2_PLACEMENT_3D('',#89320,#58195,#58196);
#48914=AXIS2_PLACEMENT_3D('',#89321,#58197,#58198);
#48915=AXIS2_PLACEMENT_3D('',#89340,#58199,#58200);
#48916=AXIS2_PLACEMENT_3D('',#89341,#58201,#58202);
#48917=AXIS2_PLACEMENT_3D('',#89345,#58204,#58205);
#48918=AXIS2_PLACEMENT_3D('',#89347,#58206,#58207);
#48919=AXIS2_PLACEMENT_3D('',#89383,#58210,#58211);
#48920=AXIS2_PLACEMENT_3D('',#89391,#58213,#58214);
#48921=AXIS2_PLACEMENT_3D('',#89394,#58215,#58216);
#48922=AXIS2_PLACEMENT_3D('',#89395,#58217,#58218);
#48923=AXIS2_PLACEMENT_3D('',#89396,#58219,#58220);
#48924=AXIS2_PLACEMENT_3D('',#89411,#58221,#58222);
#48925=AXIS2_PLACEMENT_3D('',#89412,#58223,#58224);
#48926=AXIS2_PLACEMENT_3D('',#89416,#58226,#58227);
#48927=AXIS2_PLACEMENT_3D('',#89418,#58228,#58229);
#48928=AXIS2_PLACEMENT_3D('',#89452,#58232,#58233);
#48929=AXIS2_PLACEMENT_3D('',#89454,#58235,#58236);
#48930=AXIS2_PLACEMENT_3D('',#89455,#58237,#58238);
#48931=AXIS2_PLACEMENT_3D('',#89458,#58240,#58241);
#48932=AXIS2_PLACEMENT_3D('',#89459,#58242,#58243);
#48933=AXIS2_PLACEMENT_3D('',#89460,#58244,#58245);
#48934=AXIS2_PLACEMENT_3D('',#89461,#58246,#58247);
#48935=AXIS2_PLACEMENT_3D('',#89464,#58248,#58249);
#48936=AXIS2_PLACEMENT_3D('',#89466,#58250,#58251);
#48937=AXIS2_PLACEMENT_3D('',#89468,#58252,#58253);
#48938=AXIS2_PLACEMENT_3D('',#89469,#58254,#58255);
#48939=AXIS2_PLACEMENT_3D('',#89470,#58256,#58257);
#48940=AXIS2_PLACEMENT_3D('',#89473,#58258,#58259);
#48941=AXIS2_PLACEMENT_3D('',#89475,#58260,#58261);
#48942=AXIS2_PLACEMENT_3D('',#89477,#58262,#58263);
#48943=AXIS2_PLACEMENT_3D('',#89478,#58264,#58265);
#48944=AXIS2_PLACEMENT_3D('',#89479,#58266,#58267);
#48945=AXIS2_PLACEMENT_3D('',#89482,#58268,#58269);
#48946=AXIS2_PLACEMENT_3D('',#89497,#58270,#58271);
#48947=AXIS2_PLACEMENT_3D('',#89498,#58272,#58273);
#48948=AXIS2_PLACEMENT_3D('',#89501,#58274,#58275);
#48949=AXIS2_PLACEMENT_3D('',#89503,#58276,#58277);
#48950=AXIS2_PLACEMENT_3D('',#89505,#58278,#58279);
#48951=AXIS2_PLACEMENT_3D('',#89506,#58280,#58281);
#48952=AXIS2_PLACEMENT_3D('',#89515,#58282,#58283);
#48953=AXIS2_PLACEMENT_3D('',#89516,#58284,#58285);
#48954=AXIS2_PLACEMENT_3D('',#89520,#58287,#58288);
#48955=AXIS2_PLACEMENT_3D('',#89522,#58289,#58290);
#48956=AXIS2_PLACEMENT_3D('',#89610,#58295,#58296);
#48957=AXIS2_PLACEMENT_3D('',#89612,#58297,#58298);
#48958=AXIS2_PLACEMENT_3D('',#89667,#58302,#58303);
#48959=AXIS2_PLACEMENT_3D('',#89668,#58304,#58305);
#48960=AXIS2_PLACEMENT_3D('',#89672,#58307,#58308);
#48961=AXIS2_PLACEMENT_3D('',#89674,#58309,#58310);
#48962=AXIS2_PLACEMENT_3D('',#89717,#58313,#58314);
#48963=AXIS2_PLACEMENT_3D('',#89736,#58316,#58317);
#48964=AXIS2_PLACEMENT_3D('',#89737,#58318,#58319);
#48965=AXIS2_PLACEMENT_3D('',#89747,#58320,#58321);
#48966=AXIS2_PLACEMENT_3D('',#89786,#58324,#58325);
#48967=AXIS2_PLACEMENT_3D('',#89787,#58326,#58327);
#48968=AXIS2_PLACEMENT_3D('',#89791,#58329,#58330);
#48969=AXIS2_PLACEMENT_3D('',#89793,#58331,#58332);
#48970=AXIS2_PLACEMENT_3D('',#89818,#58335,#58336);
#48971=AXIS2_PLACEMENT_3D('',#89819,#58337,#58338);
#48972=AXIS2_PLACEMENT_3D('',#89843,#58340,#58341);
#48973=AXIS2_PLACEMENT_3D('',#89846,#58342,#58343);
#48974=AXIS2_PLACEMENT_3D('',#89847,#58344,#58345);
#48975=AXIS2_PLACEMENT_3D('',#89848,#58346,#58347);
#48976=AXIS2_PLACEMENT_3D('',#89867,#58348,#58349);
#48977=AXIS2_PLACEMENT_3D('',#89868,#58350,#58351);
#48978=AXIS2_PLACEMENT_3D('',#89872,#58353,#58354);
#48979=AXIS2_PLACEMENT_3D('',#89874,#58355,#58356);
#48980=AXIS2_PLACEMENT_3D('',#89910,#58359,#58360);
#48981=AXIS2_PLACEMENT_3D('',#89918,#58362,#58363);
#48982=AXIS2_PLACEMENT_3D('',#89921,#58364,#58365);
#48983=AXIS2_PLACEMENT_3D('',#89922,#58366,#58367);
#48984=AXIS2_PLACEMENT_3D('',#89923,#58368,#58369);
#48985=AXIS2_PLACEMENT_3D('',#89938,#58370,#58371);
#48986=AXIS2_PLACEMENT_3D('',#89939,#58372,#58373);
#48987=AXIS2_PLACEMENT_3D('',#89943,#58375,#58376);
#48988=AXIS2_PLACEMENT_3D('',#89945,#58377,#58378);
#48989=AXIS2_PLACEMENT_3D('',#89979,#58381,#58382);
#48990=AXIS2_PLACEMENT_3D('',#89981,#58384,#58385);
#48991=AXIS2_PLACEMENT_3D('',#89982,#58386,#58387);
#48992=AXIS2_PLACEMENT_3D('',#89985,#58389,#58390);
#48993=AXIS2_PLACEMENT_3D('',#89986,#58391,#58392);
#48994=AXIS2_PLACEMENT_3D('',#89987,#58393,#58394);
#48995=AXIS2_PLACEMENT_3D('',#89988,#58395,#58396);
#48996=AXIS2_PLACEMENT_3D('',#89991,#58397,#58398);
#48997=AXIS2_PLACEMENT_3D('',#89993,#58399,#58400);
#48998=AXIS2_PLACEMENT_3D('',#89995,#58401,#58402);
#48999=AXIS2_PLACEMENT_3D('',#89996,#58403,#58404);
#49000=AXIS2_PLACEMENT_3D('',#89997,#58405,#58406);
#49001=AXIS2_PLACEMENT_3D('',#90000,#58407,#58408);
#49002=AXIS2_PLACEMENT_3D('',#90002,#58409,#58410);
#49003=AXIS2_PLACEMENT_3D('',#90004,#58411,#58412);
#49004=AXIS2_PLACEMENT_3D('',#90005,#58413,#58414);
#49005=AXIS2_PLACEMENT_3D('',#90006,#58415,#58416);
#49006=AXIS2_PLACEMENT_3D('',#90009,#58417,#58418);
#49007=AXIS2_PLACEMENT_3D('',#90011,#58419,#58420);
#49008=AXIS2_PLACEMENT_3D('',#90013,#58421,#58422);
#49009=AXIS2_PLACEMENT_3D('',#90014,#58423,#58424);
#49010=AXIS2_PLACEMENT_3D('',#90015,#58425,#58426);
#49011=AXIS2_PLACEMENT_3D('',#90018,#58427,#58428);
#49012=AXIS2_PLACEMENT_3D('',#90020,#58429,#58430);
#49013=AXIS2_PLACEMENT_3D('',#90022,#58431,#58432);
#49014=AXIS2_PLACEMENT_3D('',#90023,#58433,#58434);
#49015=AXIS2_PLACEMENT_3D('',#90024,#58435,#58436);
#49016=AXIS2_PLACEMENT_3D('',#90027,#58437,#58438);
#49017=AXIS2_PLACEMENT_3D('',#90042,#58439,#58440);
#49018=AXIS2_PLACEMENT_3D('',#90077,#58442,#58443);
#49019=AXIS2_PLACEMENT_3D('',#90079,#58444,#58445);
#49020=AXIS2_PLACEMENT_3D('',#90135,#58449,#58450);
#49021=AXIS2_PLACEMENT_3D('',#90136,#58451,#58452);
#49022=AXIS2_PLACEMENT_3D('',#90140,#58454,#58455);
#49023=AXIS2_PLACEMENT_3D('',#90142,#58456,#58457);
#49024=AXIS2_PLACEMENT_3D('',#90201,#58461,#58462);
#49025=AXIS2_PLACEMENT_3D('',#90202,#58463,#58464);
#49026=AXIS2_PLACEMENT_3D('',#90206,#58466,#58467);
#49027=AXIS2_PLACEMENT_3D('',#90208,#58468,#58469);
#49028=AXIS2_PLACEMENT_3D('',#90251,#58472,#58473);
#49029=AXIS2_PLACEMENT_3D('',#90277,#58475,#58476);
#49030=AXIS2_PLACEMENT_3D('',#90278,#58477,#58478);
#49031=AXIS2_PLACEMENT_3D('',#90288,#58479,#58480);
#49032=AXIS2_PLACEMENT_3D('',#90320,#58483,#58484);
#49033=AXIS2_PLACEMENT_3D('',#90321,#58485,#58486);
#49034=AXIS2_PLACEMENT_3D('',#90325,#58488,#58489);
#49035=AXIS2_PLACEMENT_3D('',#90327,#58490,#58491);
#49036=AXIS2_PLACEMENT_3D('',#90352,#58494,#58495);
#49037=AXIS2_PLACEMENT_3D('',#90353,#58496,#58497);
#49038=AXIS2_PLACEMENT_3D('',#90391,#58499,#58500);
#49039=AXIS2_PLACEMENT_3D('',#90392,#58501,#58502);
#49040=AXIS2_PLACEMENT_3D('',#90396,#58504,#58505);
#49041=AXIS2_PLACEMENT_3D('',#90398,#58506,#58507);
#49042=AXIS2_PLACEMENT_3D('',#90439,#58511,#58512);
#49043=AXIS2_PLACEMENT_3D('',#90442,#58513,#58514);
#49044=AXIS2_PLACEMENT_3D('',#90443,#58515,#58516);
#49045=AXIS2_PLACEMENT_3D('',#90444,#58517,#58518);
#49046=AXIS2_PLACEMENT_3D('',#90459,#58519,#58520);
#49047=AXIS2_PLACEMENT_3D('',#90460,#58521,#58522);
#49048=AXIS2_PLACEMENT_3D('',#90464,#58524,#58525);
#49049=AXIS2_PLACEMENT_3D('',#90466,#58526,#58527);
#49050=AXIS2_PLACEMENT_3D('',#90500,#58530,#58531);
#49051=AXIS2_PLACEMENT_3D('',#90502,#58533,#58534);
#49052=AXIS2_PLACEMENT_3D('',#90503,#58535,#58536);
#49053=AXIS2_PLACEMENT_3D('',#90506,#58538,#58539);
#49054=AXIS2_PLACEMENT_3D('',#90507,#58540,#58541);
#49055=AXIS2_PLACEMENT_3D('',#90508,#58542,#58543);
#49056=AXIS2_PLACEMENT_3D('',#90509,#58544,#58545);
#49057=AXIS2_PLACEMENT_3D('',#90512,#58546,#58547);
#49058=AXIS2_PLACEMENT_3D('',#90514,#58548,#58549);
#49059=AXIS2_PLACEMENT_3D('',#90516,#58550,#58551);
#49060=AXIS2_PLACEMENT_3D('',#90517,#58552,#58553);
#49061=AXIS2_PLACEMENT_3D('',#90518,#58554,#58555);
#49062=AXIS2_PLACEMENT_3D('',#90521,#58556,#58557);
#49063=AXIS2_PLACEMENT_3D('',#90536,#58558,#58559);
#49064=AXIS2_PLACEMENT_3D('',#90537,#58560,#58561);
#49065=AXIS2_PLACEMENT_3D('',#90540,#58562,#58563);
#49066=AXIS2_PLACEMENT_3D('',#90542,#58564,#58565);
#49067=AXIS2_PLACEMENT_3D('',#90544,#58566,#58567);
#49068=AXIS2_PLACEMENT_3D('',#90545,#58568,#58569);
#49069=AXIS2_PLACEMENT_3D('',#90546,#58570,#58571);
#49070=AXIS2_PLACEMENT_3D('',#90549,#58572,#58573);
#49071=AXIS2_PLACEMENT_3D('',#90551,#58574,#58575);
#49072=AXIS2_PLACEMENT_3D('',#90553,#58576,#58577);
#49073=AXIS2_PLACEMENT_3D('',#90554,#58578,#58579);
#49074=AXIS2_PLACEMENT_3D('',#90555,#58580,#58581);
#49075=AXIS2_PLACEMENT_3D('',#90558,#58582,#58583);
#49076=AXIS2_PLACEMENT_3D('',#90560,#58584,#58585);
#49077=AXIS2_PLACEMENT_3D('',#90562,#58586,#58587);
#49078=AXIS2_PLACEMENT_3D('',#90563,#58588,#58589);
#49079=AXIS2_PLACEMENT_3D('',#90564,#58590,#58591);
#49080=AXIS2_PLACEMENT_3D('',#90567,#58592,#58593);
#49081=AXIS2_PLACEMENT_3D('',#90569,#58594,#58595);
#49082=AXIS2_PLACEMENT_3D('',#90571,#58596,#58597);
#49083=AXIS2_PLACEMENT_3D('',#90572,#58598,#58599);
#49084=AXIS2_PLACEMENT_3D('',#90581,#58600,#58601);
#49085=AXIS2_PLACEMENT_3D('',#90582,#58602,#58603);
#49086=AXIS2_PLACEMENT_3D('',#90586,#58605,#58606);
#49087=AXIS2_PLACEMENT_3D('',#90587,#58607,#58608);
#49088=AXIS2_PLACEMENT_3D('',#90649,#58612,#58613);
#49089=AXIS2_PLACEMENT_3D('',#90650,#58614,#58615);
#49090=AXIS2_PLACEMENT_3D('',#90654,#58617,#58618);
#49091=AXIS2_PLACEMENT_3D('',#90655,#58619,#58620);
#49092=AXIS2_PLACEMENT_3D('',#90707,#58624,#58625);
#49093=AXIS2_PLACEMENT_3D('',#90708,#58626,#58627);
#49094=AXIS2_PLACEMENT_3D('',#90712,#58629,#58630);
#49095=AXIS2_PLACEMENT_3D('',#90714,#58631,#58632);
#49096=AXIS2_PLACEMENT_3D('',#90755,#58635,#58636);
#49097=AXIS2_PLACEMENT_3D('',#90768,#58638,#58639);
#49098=AXIS2_PLACEMENT_3D('',#90769,#58640,#58641);
#49099=AXIS2_PLACEMENT_3D('',#90778,#58642,#58643);
#49100=AXIS2_PLACEMENT_3D('',#90807,#58646,#58647);
#49101=AXIS2_PLACEMENT_3D('',#90808,#58648,#58649);
#49102=AXIS2_PLACEMENT_3D('',#90812,#58651,#58652);
#49103=AXIS2_PLACEMENT_3D('',#90813,#58653,#58654);
#49104=AXIS2_PLACEMENT_3D('',#90838,#58657,#58658);
#49105=AXIS2_PLACEMENT_3D('',#90839,#58659,#58660);
#49106=AXIS2_PLACEMENT_3D('',#90870,#58662,#58663);
#49107=AXIS2_PLACEMENT_3D('',#90871,#58664,#58665);
#49108=AXIS2_PLACEMENT_3D('',#90875,#58667,#58668);
#49109=AXIS2_PLACEMENT_3D('',#90876,#58669,#58670);
#49110=AXIS2_PLACEMENT_3D('',#90957,#58675,#58676);
#49111=AXIS2_PLACEMENT_3D('',#90958,#58677,#58678);
#49112=AXIS2_PLACEMENT_3D('',#91005,#58682,#58683);
#49113=AXIS2_PLACEMENT_3D('',#91006,#58684,#58685);
#49114=AXIS2_PLACEMENT_3D('',#91009,#58687,#58688);
#49115=AXIS2_PLACEMENT_3D('',#91010,#58689,#58690);
#49116=AXIS2_PLACEMENT_3D('',#91011,#58691,#58692);
#49117=AXIS2_PLACEMENT_3D('',#91012,#58693,#58694);
#49118=AXIS2_PLACEMENT_3D('',#91013,#58695,#58696);
#49119=AXIS2_PLACEMENT_3D('',#91016,#58698,#58699);
#49120=AXIS2_PLACEMENT_3D('',#91017,#58700,#58701);
#49121=AXIS2_PLACEMENT_3D('',#91018,#58702,#58703);
#49122=AXIS2_PLACEMENT_3D('',#91019,#58704,#58705);
#49123=AXIS2_PLACEMENT_3D('',#91020,#58706,#58707);
#49124=AXIS2_PLACEMENT_3D('',#91021,#58708,#58709);
#49125=AXIS2_PLACEMENT_3D('',#91022,#58710,#58711);
#49126=AXIS2_PLACEMENT_3D('',#91023,#58712,#58713);
#49127=AXIS2_PLACEMENT_3D('',#91040,#58714,#58715);
#49128=AXIS2_PLACEMENT_3D('',#91057,#58716,#58717);
#49129=AXIS2_PLACEMENT_3D('',#91080,#58718,#58719);
#49130=AXIS2_PLACEMENT_3D('',#91128,#58720,#58721);
#49131=AXIS2_PLACEMENT_3D('',#91145,#58722,#58723);
#49132=AXIS2_PLACEMENT_3D('',#91168,#58724,#58725);
#49133=AXIS2_PLACEMENT_3D('',#91185,#58726,#58727);
#49134=AXIS2_PLACEMENT_3D('',#91208,#58728,#58729);
#49135=AXIS2_PLACEMENT_3D('',#91225,#58730,#58731);
#49136=AXIS2_PLACEMENT_3D('',#91232,#58732,#58733);
#49137=AXIS2_PLACEMENT_3D('',#91237,#58734,#58735);
#49138=AXIS2_PLACEMENT_3D('',#91254,#58736,#58737);
#49139=AXIS2_PLACEMENT_3D('',#91271,#58738,#58739);
#49140=AXIS2_PLACEMENT_3D('',#91294,#58740,#58741);
#49141=AXIS2_PLACEMENT_3D('',#91295,#58742,#58743);
#49142=AXIS2_PLACEMENT_3D('',#91328,#58744,#58745);
#49143=AXIS2_PLACEMENT_3D('',#91333,#58746,#58747);
#49144=AXIS2_PLACEMENT_3D('',#91350,#58748,#58749);
#49145=AXIS2_PLACEMENT_3D('',#91367,#58750,#58751);
#49146=AXIS2_PLACEMENT_3D('',#91405,#58752,#58753);
#49147=AXIS2_PLACEMENT_3D('',#91438,#58754,#58755);
#49148=AXIS2_PLACEMENT_3D('',#91455,#58756,#58757);
#49149=AXIS2_PLACEMENT_3D('',#91478,#58758,#58759);
#49150=AXIS2_PLACEMENT_3D('',#91495,#58760,#58761);
#49151=AXIS2_PLACEMENT_3D('',#91518,#58762,#58763);
#49152=AXIS2_PLACEMENT_3D('',#91535,#58764,#58765);
#49153=AXIS2_PLACEMENT_3D('',#91558,#58766,#58767);
#49154=AXIS2_PLACEMENT_3D('',#91575,#58768,#58769);
#49155=AXIS2_PLACEMENT_3D('',#91598,#58770,#58771);
#49156=AXIS2_PLACEMENT_3D('',#91599,#58772,#58773);
#49157=AXIS2_PLACEMENT_3D('',#91632,#58774,#58775);
#49158=AXIS2_PLACEMENT_3D('',#91637,#58776,#58777);
#49159=AXIS2_PLACEMENT_3D('',#91654,#58778,#58779);
#49160=AXIS2_PLACEMENT_3D('',#91671,#58780,#58781);
#49161=AXIS2_PLACEMENT_3D('',#91694,#58782,#58783);
#49162=AXIS2_PLACEMENT_3D('',#91711,#58784,#58785);
#49163=AXIS2_PLACEMENT_3D('',#91744,#58786,#58787);
#49164=AXIS2_PLACEMENT_3D('',#91761,#58788,#58789);
#49165=AXIS2_PLACEMENT_3D('',#91784,#58790,#58791);
#49166=AXIS2_PLACEMENT_3D('',#91801,#58792,#58793);
#49167=AXIS2_PLACEMENT_3D('',#91824,#58794,#58795);
#49168=AXIS2_PLACEMENT_3D('',#91841,#58796,#58797);
#49169=AXIS2_PLACEMENT_3D('',#91864,#58798,#58799);
#49170=AXIS2_PLACEMENT_3D('',#91881,#58800,#58801);
#49171=AXIS2_PLACEMENT_3D('',#91909,#58802,#58803);
#49172=AXIS2_PLACEMENT_3D('',#91936,#58804,#58805);
#49173=AXIS2_PLACEMENT_3D('',#91941,#58806,#58807);
#49174=AXIS2_PLACEMENT_3D('',#91958,#58808,#58809);
#49175=AXIS2_PLACEMENT_3D('',#91975,#58810,#58811);
#49176=AXIS2_PLACEMENT_3D('',#91998,#58812,#58813);
#49177=AXIS2_PLACEMENT_3D('',#92015,#58814,#58815);
#49178=AXIS2_PLACEMENT_3D('',#92048,#58816,#58817);
#49179=AXIS2_PLACEMENT_3D('',#92065,#58818,#58819);
#49180=AXIS2_PLACEMENT_3D('',#92088,#58820,#58821);
#49181=AXIS2_PLACEMENT_3D('',#92105,#58822,#58823);
#49182=AXIS2_PLACEMENT_3D('',#92128,#58824,#58825);
#49183=AXIS2_PLACEMENT_3D('',#92145,#58826,#58827);
#49184=AXIS2_PLACEMENT_3D('',#92168,#58828,#58829);
#49185=AXIS2_PLACEMENT_3D('',#92206,#58830,#58831);
#49186=AXIS2_PLACEMENT_3D('',#92207,#58832,#58833);
#49187=AXIS2_PLACEMENT_3D('',#92240,#58834,#58835);
#49188=AXIS2_PLACEMENT_3D('',#92245,#58836,#58837);
#49189=AXIS2_PLACEMENT_3D('',#92262,#58838,#58839);
#49190=AXIS2_PLACEMENT_3D('',#92279,#58840,#58841);
#49191=AXIS2_PLACEMENT_3D('',#92302,#58842,#58843);
#49192=AXIS2_PLACEMENT_3D('',#92319,#58844,#58845);
#49193=AXIS2_PLACEMENT_3D('',#92352,#58846,#58847);
#49194=AXIS2_PLACEMENT_3D('',#92369,#58848,#58849);
#49195=AXIS2_PLACEMENT_3D('',#92392,#58850,#58851);
#49196=AXIS2_PLACEMENT_3D('',#92440,#58852,#58853);
#49197=AXIS2_PLACEMENT_3D('',#92447,#58854,#58855);
#49198=AXIS2_PLACEMENT_3D('',#92480,#58856,#58857);
#49199=AXIS2_PLACEMENT_3D('',#92497,#58858,#58859);
#49200=AXIS2_PLACEMENT_3D('',#92510,#58860,#58861);
#49201=AXIS2_PLACEMENT_3D('',#92511,#58862,#58863);
#49202=AXIS2_PLACEMENT_3D('',#92544,#58864,#58865);
#49203=AXIS2_PLACEMENT_3D('',#92549,#58866,#58867);
#49204=AXIS2_PLACEMENT_3D('',#92566,#58868,#58869);
#49205=AXIS2_PLACEMENT_3D('',#92583,#58870,#58871);
#49206=AXIS2_PLACEMENT_3D('',#92606,#58872,#58873);
#49207=AXIS2_PLACEMENT_3D('',#92623,#58874,#58875);
#49208=AXIS2_PLACEMENT_3D('',#92656,#58876,#58877);
#49209=AXIS2_PLACEMENT_3D('',#92673,#58878,#58879);
#49210=AXIS2_PLACEMENT_3D('',#92696,#58880,#58881);
#49211=AXIS2_PLACEMENT_3D('',#92744,#58882,#58883);
#49212=AXIS2_PLACEMENT_3D('',#92761,#58884,#58885);
#49213=AXIS2_PLACEMENT_3D('',#92784,#58886,#58887);
#49214=AXIS2_PLACEMENT_3D('',#92801,#58888,#58889);
#49215=AXIS2_PLACEMENT_3D('',#92814,#58890,#58891);
#49216=AXIS2_PLACEMENT_3D('',#92815,#58892,#58893);
#49217=AXIS2_PLACEMENT_3D('',#92848,#58894,#58895);
#49218=AXIS2_PLACEMENT_3D('',#92853,#58896,#58897);
#49219=AXIS2_PLACEMENT_3D('',#92870,#58898,#58899);
#49220=AXIS2_PLACEMENT_3D('',#92887,#58900,#58901);
#49221=AXIS2_PLACEMENT_3D('',#92910,#58902,#58903);
#49222=AXIS2_PLACEMENT_3D('',#92927,#58904,#58905);
#49223=AXIS2_PLACEMENT_3D('',#92960,#58906,#58907);
#49224=AXIS2_PLACEMENT_3D('',#92977,#58908,#58909);
#49225=AXIS2_PLACEMENT_3D('',#93000,#58910,#58911);
#49226=AXIS2_PLACEMENT_3D('',#93048,#58912,#58913);
#49227=AXIS2_PLACEMENT_3D('',#93065,#58914,#58915);
#49228=AXIS2_PLACEMENT_3D('',#93088,#58916,#58917);
#49229=AXIS2_PLACEMENT_3D('',#93105,#58918,#58919);
#49230=AXIS2_PLACEMENT_3D('',#93118,#58920,#58921);
#49231=AXIS2_PLACEMENT_3D('',#93119,#58922,#58923);
#49232=AXIS2_PLACEMENT_3D('',#93152,#58924,#58925);
#49233=AXIS2_PLACEMENT_3D('',#93157,#58926,#58927);
#49234=AXIS2_PLACEMENT_3D('',#93174,#58928,#58929);
#49235=AXIS2_PLACEMENT_3D('',#93191,#58930,#58931);
#49236=AXIS2_PLACEMENT_3D('',#93214,#58932,#58933);
#49237=AXIS2_PLACEMENT_3D('',#93231,#58934,#58935);
#49238=AXIS2_PLACEMENT_3D('',#93264,#58936,#58937);
#49239=AXIS2_PLACEMENT_3D('',#93281,#58938,#58939);
#49240=AXIS2_PLACEMENT_3D('',#93304,#58940,#58941);
#49241=AXIS2_PLACEMENT_3D('',#93352,#58942,#58943);
#49242=AXIS2_PLACEMENT_3D('',#93369,#58944,#58945);
#49243=AXIS2_PLACEMENT_3D('',#93392,#58946,#58947);
#49244=AXIS2_PLACEMENT_3D('',#93409,#58948,#58949);
#49245=AXIS2_PLACEMENT_3D('',#93422,#58950,#58951);
#49246=AXIS2_PLACEMENT_3D('',#93423,#58952,#58953);
#49247=AXIS2_PLACEMENT_3D('',#93456,#58954,#58955);
#49248=AXIS2_PLACEMENT_3D('',#93461,#58956,#58957);
#49249=AXIS2_PLACEMENT_3D('',#93478,#58958,#58959);
#49250=AXIS2_PLACEMENT_3D('',#93495,#58960,#58961);
#49251=AXIS2_PLACEMENT_3D('',#93518,#58962,#58963);
#49252=AXIS2_PLACEMENT_3D('',#93535,#58964,#58965);
#49253=AXIS2_PLACEMENT_3D('',#93568,#58966,#58967);
#49254=AXIS2_PLACEMENT_3D('',#93585,#58968,#58969);
#49255=AXIS2_PLACEMENT_3D('',#93608,#58970,#58971);
#49256=AXIS2_PLACEMENT_3D('',#93656,#58972,#58973);
#49257=AXIS2_PLACEMENT_3D('',#93673,#58974,#58975);
#49258=AXIS2_PLACEMENT_3D('',#93696,#58976,#58977);
#49259=AXIS2_PLACEMENT_3D('',#93713,#58978,#58979);
#49260=AXIS2_PLACEMENT_3D('',#93726,#58980,#58981);
#49261=AXIS2_PLACEMENT_3D('',#93727,#58982,#58983);
#49262=AXIS2_PLACEMENT_3D('',#93760,#58984,#58985);
#49263=AXIS2_PLACEMENT_3D('',#93765,#58986,#58987);
#49264=AXIS2_PLACEMENT_3D('',#93782,#58988,#58989);
#49265=AXIS2_PLACEMENT_3D('',#93799,#58990,#58991);
#49266=AXIS2_PLACEMENT_3D('',#93822,#58992,#58993);
#49267=AXIS2_PLACEMENT_3D('',#93839,#58994,#58995);
#49268=AXIS2_PLACEMENT_3D('',#93872,#58996,#58997);
#49269=AXIS2_PLACEMENT_3D('',#93889,#58998,#58999);
#49270=AXIS2_PLACEMENT_3D('',#93912,#59000,#59001);
#49271=AXIS2_PLACEMENT_3D('',#93960,#59002,#59003);
#49272=AXIS2_PLACEMENT_3D('',#93977,#59004,#59005);
#49273=AXIS2_PLACEMENT_3D('',#94000,#59006,#59007);
#49274=AXIS2_PLACEMENT_3D('',#94017,#59008,#59009);
#49275=AXIS2_PLACEMENT_3D('',#94030,#59010,#59011);
#49276=AXIS2_PLACEMENT_3D('',#94031,#59012,#59013);
#49277=AXIS2_PLACEMENT_3D('',#94064,#59014,#59015);
#49278=AXIS2_PLACEMENT_3D('',#94069,#59016,#59017);
#49279=AXIS2_PLACEMENT_3D('',#94086,#59018,#59019);
#49280=AXIS2_PLACEMENT_3D('',#94103,#59020,#59021);
#49281=AXIS2_PLACEMENT_3D('',#94126,#59022,#59023);
#49282=AXIS2_PLACEMENT_3D('',#94143,#59024,#59025);
#49283=AXIS2_PLACEMENT_3D('',#94176,#59026,#59027);
#49284=AXIS2_PLACEMENT_3D('',#94193,#59028,#59029);
#49285=AXIS2_PLACEMENT_3D('',#94216,#59030,#59031);
#49286=AXIS2_PLACEMENT_3D('',#94264,#59032,#59033);
#49287=AXIS2_PLACEMENT_3D('',#94281,#59034,#59035);
#49288=AXIS2_PLACEMENT_3D('',#94304,#59036,#59037);
#49289=AXIS2_PLACEMENT_3D('',#94321,#59038,#59039);
#49290=AXIS2_PLACEMENT_3D('',#94334,#59040,#59041);
#49291=AXIS2_PLACEMENT_3D('',#94335,#59042,#59043);
#49292=AXIS2_PLACEMENT_3D('',#94368,#59044,#59045);
#49293=AXIS2_PLACEMENT_3D('',#94373,#59046,#59047);
#49294=AXIS2_PLACEMENT_3D('',#94390,#59048,#59049);
#49295=AXIS2_PLACEMENT_3D('',#94407,#59050,#59051);
#49296=AXIS2_PLACEMENT_3D('',#94430,#59052,#59053);
#49297=AXIS2_PLACEMENT_3D('',#94447,#59054,#59055);
#49298=AXIS2_PLACEMENT_3D('',#94480,#59056,#59057);
#49299=AXIS2_PLACEMENT_3D('',#94497,#59058,#59059);
#49300=AXIS2_PLACEMENT_3D('',#94520,#59060,#59061);
#49301=AXIS2_PLACEMENT_3D('',#94568,#59062,#59063);
#49302=AXIS2_PLACEMENT_3D('',#94585,#59064,#59065);
#49303=AXIS2_PLACEMENT_3D('',#94608,#59066,#59067);
#49304=AXIS2_PLACEMENT_3D('',#94625,#59068,#59069);
#49305=AXIS2_PLACEMENT_3D('',#94638,#59070,#59071);
#49306=AXIS2_PLACEMENT_3D('',#94639,#59072,#59073);
#49307=AXIS2_PLACEMENT_3D('',#94672,#59074,#59075);
#49308=AXIS2_PLACEMENT_3D('',#94677,#59076,#59077);
#49309=AXIS2_PLACEMENT_3D('',#94694,#59078,#59079);
#49310=AXIS2_PLACEMENT_3D('',#94711,#59080,#59081);
#49311=AXIS2_PLACEMENT_3D('',#94734,#59082,#59083);
#49312=AXIS2_PLACEMENT_3D('',#94751,#59084,#59085);
#49313=AXIS2_PLACEMENT_3D('',#94784,#59086,#59087);
#49314=AXIS2_PLACEMENT_3D('',#94801,#59088,#59089);
#49315=AXIS2_PLACEMENT_3D('',#94824,#59090,#59091);
#49316=AXIS2_PLACEMENT_3D('',#94872,#59092,#59093);
#49317=AXIS2_PLACEMENT_3D('',#94889,#59094,#59095);
#49318=AXIS2_PLACEMENT_3D('',#94912,#59096,#59097);
#49319=AXIS2_PLACEMENT_3D('',#94929,#59098,#59099);
#49320=AXIS2_PLACEMENT_3D('',#94942,#59100,#59101);
#49321=AXIS2_PLACEMENT_3D('',#94943,#59102,#59103);
#49322=AXIS2_PLACEMENT_3D('',#94976,#59104,#59105);
#49323=AXIS2_PLACEMENT_3D('',#94981,#59106,#59107);
#49324=AXIS2_PLACEMENT_3D('',#94998,#59108,#59109);
#49325=AXIS2_PLACEMENT_3D('',#95015,#59110,#59111);
#49326=AXIS2_PLACEMENT_3D('',#95038,#59112,#59113);
#49327=AXIS2_PLACEMENT_3D('',#95055,#59114,#59115);
#49328=AXIS2_PLACEMENT_3D('',#95088,#59116,#59117);
#49329=AXIS2_PLACEMENT_3D('',#95105,#59118,#59119);
#49330=AXIS2_PLACEMENT_3D('',#95128,#59120,#59121);
#49331=AXIS2_PLACEMENT_3D('',#95176,#59122,#59123);
#49332=AXIS2_PLACEMENT_3D('',#95193,#59124,#59125);
#49333=AXIS2_PLACEMENT_3D('',#95216,#59126,#59127);
#49334=AXIS2_PLACEMENT_3D('',#95233,#59128,#59129);
#49335=AXIS2_PLACEMENT_3D('',#95246,#59130,#59131);
#49336=AXIS2_PLACEMENT_3D('',#95247,#59132,#59133);
#49337=AXIS2_PLACEMENT_3D('',#95280,#59134,#59135);
#49338=AXIS2_PLACEMENT_3D('',#95285,#59136,#59137);
#49339=AXIS2_PLACEMENT_3D('',#95302,#59138,#59139);
#49340=AXIS2_PLACEMENT_3D('',#95319,#59140,#59141);
#49341=AXIS2_PLACEMENT_3D('',#95342,#59142,#59143);
#49342=AXIS2_PLACEMENT_3D('',#95359,#59144,#59145);
#49343=AXIS2_PLACEMENT_3D('',#95392,#59146,#59147);
#49344=AXIS2_PLACEMENT_3D('',#95409,#59148,#59149);
#49345=AXIS2_PLACEMENT_3D('',#95432,#59150,#59151);
#49346=AXIS2_PLACEMENT_3D('',#95480,#59152,#59153);
#49347=AXIS2_PLACEMENT_3D('',#95497,#59154,#59155);
#49348=AXIS2_PLACEMENT_3D('',#95520,#59156,#59157);
#49349=AXIS2_PLACEMENT_3D('',#95537,#59158,#59159);
#49350=AXIS2_PLACEMENT_3D('',#95550,#59160,#59161);
#49351=AXIS2_PLACEMENT_3D('',#95551,#59162,#59163);
#49352=AXIS2_PLACEMENT_3D('',#95584,#59164,#59165);
#49353=AXIS2_PLACEMENT_3D('',#95589,#59166,#59167);
#49354=AXIS2_PLACEMENT_3D('',#95606,#59168,#59169);
#49355=AXIS2_PLACEMENT_3D('',#95623,#59170,#59171);
#49356=AXIS2_PLACEMENT_3D('',#95646,#59172,#59173);
#49357=AXIS2_PLACEMENT_3D('',#95663,#59174,#59175);
#49358=AXIS2_PLACEMENT_3D('',#95696,#59176,#59177);
#49359=AXIS2_PLACEMENT_3D('',#95713,#59178,#59179);
#49360=AXIS2_PLACEMENT_3D('',#95736,#59180,#59181);
#49361=AXIS2_PLACEMENT_3D('',#95784,#59182,#59183);
#49362=AXIS2_PLACEMENT_3D('',#95801,#59184,#59185);
#49363=AXIS2_PLACEMENT_3D('',#95824,#59186,#59187);
#49364=AXIS2_PLACEMENT_3D('',#95841,#59188,#59189);
#49365=AXIS2_PLACEMENT_3D('',#95854,#59190,#59191);
#49366=AXIS2_PLACEMENT_3D('',#95855,#59192,#59193);
#49367=AXIS2_PLACEMENT_3D('',#95888,#59194,#59195);
#49368=AXIS2_PLACEMENT_3D('',#95893,#59196,#59197);
#49369=AXIS2_PLACEMENT_3D('',#95910,#59198,#59199);
#49370=AXIS2_PLACEMENT_3D('',#95927,#59200,#59201);
#49371=AXIS2_PLACEMENT_3D('',#95950,#59202,#59203);
#49372=AXIS2_PLACEMENT_3D('',#95967,#59204,#59205);
#49373=AXIS2_PLACEMENT_3D('',#96000,#59206,#59207);
#49374=AXIS2_PLACEMENT_3D('',#96017,#59208,#59209);
#49375=AXIS2_PLACEMENT_3D('',#96040,#59210,#59211);
#49376=AXIS2_PLACEMENT_3D('',#96088,#59212,#59213);
#49377=AXIS2_PLACEMENT_3D('',#96105,#59214,#59215);
#49378=AXIS2_PLACEMENT_3D('',#96128,#59216,#59217);
#49379=AXIS2_PLACEMENT_3D('',#96145,#59218,#59219);
#49380=AXIS2_PLACEMENT_3D('',#96158,#59220,#59221);
#49381=AXIS2_PLACEMENT_3D('',#96159,#59222,#59223);
#49382=AXIS2_PLACEMENT_3D('',#96192,#59224,#59225);
#49383=AXIS2_PLACEMENT_3D('',#96197,#59226,#59227);
#49384=AXIS2_PLACEMENT_3D('',#96214,#59228,#59229);
#49385=AXIS2_PLACEMENT_3D('',#96231,#59230,#59231);
#49386=AXIS2_PLACEMENT_3D('',#96254,#59232,#59233);
#49387=AXIS2_PLACEMENT_3D('',#96271,#59234,#59235);
#49388=AXIS2_PLACEMENT_3D('',#96304,#59236,#59237);
#49389=AXIS2_PLACEMENT_3D('',#96321,#59238,#59239);
#49390=AXIS2_PLACEMENT_3D('',#96344,#59240,#59241);
#49391=AXIS2_PLACEMENT_3D('',#96392,#59242,#59243);
#49392=AXIS2_PLACEMENT_3D('',#96409,#59244,#59245);
#49393=AXIS2_PLACEMENT_3D('',#96432,#59246,#59247);
#49394=AXIS2_PLACEMENT_3D('',#96449,#59248,#59249);
#49395=AXIS2_PLACEMENT_3D('',#96462,#59250,#59251);
#49396=AXIS2_PLACEMENT_3D('',#96463,#59252,#59253);
#49397=AXIS2_PLACEMENT_3D('',#96496,#59254,#59255);
#49398=AXIS2_PLACEMENT_3D('',#96501,#59256,#59257);
#49399=AXIS2_PLACEMENT_3D('',#96518,#59258,#59259);
#49400=AXIS2_PLACEMENT_3D('',#96535,#59260,#59261);
#49401=AXIS2_PLACEMENT_3D('',#96558,#59262,#59263);
#49402=AXIS2_PLACEMENT_3D('',#96575,#59264,#59265);
#49403=AXIS2_PLACEMENT_3D('',#96608,#59266,#59267);
#49404=AXIS2_PLACEMENT_3D('',#96625,#59268,#59269);
#49405=AXIS2_PLACEMENT_3D('',#96648,#59270,#59271);
#49406=AXIS2_PLACEMENT_3D('',#96696,#59272,#59273);
#49407=AXIS2_PLACEMENT_3D('',#96713,#59274,#59275);
#49408=AXIS2_PLACEMENT_3D('',#96736,#59276,#59277);
#49409=AXIS2_PLACEMENT_3D('',#96753,#59278,#59279);
#49410=AXIS2_PLACEMENT_3D('',#96766,#59280,#59281);
#49411=AXIS2_PLACEMENT_3D('',#96767,#59282,#59283);
#49412=AXIS2_PLACEMENT_3D('',#96800,#59284,#59285);
#49413=AXIS2_PLACEMENT_3D('',#96805,#59286,#59287);
#49414=AXIS2_PLACEMENT_3D('',#96822,#59288,#59289);
#49415=AXIS2_PLACEMENT_3D('',#96839,#59290,#59291);
#49416=AXIS2_PLACEMENT_3D('',#96862,#59292,#59293);
#49417=AXIS2_PLACEMENT_3D('',#96879,#59294,#59295);
#49418=AXIS2_PLACEMENT_3D('',#96912,#59296,#59297);
#49419=AXIS2_PLACEMENT_3D('',#96929,#59298,#59299);
#49420=AXIS2_PLACEMENT_3D('',#96952,#59300,#59301);
#49421=AXIS2_PLACEMENT_3D('',#97000,#59302,#59303);
#49422=AXIS2_PLACEMENT_3D('',#97017,#59304,#59305);
#49423=AXIS2_PLACEMENT_3D('',#97040,#59306,#59307);
#49424=AXIS2_PLACEMENT_3D('',#97057,#59308,#59309);
#49425=AXIS2_PLACEMENT_3D('',#97070,#59310,#59311);
#49426=AXIS2_PLACEMENT_3D('',#97071,#59312,#59313);
#49427=AXIS2_PLACEMENT_3D('',#97104,#59314,#59315);
#49428=AXIS2_PLACEMENT_3D('',#97109,#59316,#59317);
#49429=AXIS2_PLACEMENT_3D('',#97126,#59318,#59319);
#49430=AXIS2_PLACEMENT_3D('',#97143,#59320,#59321);
#49431=AXIS2_PLACEMENT_3D('',#97166,#59322,#59323);
#49432=AXIS2_PLACEMENT_3D('',#97183,#59324,#59325);
#49433=AXIS2_PLACEMENT_3D('',#97216,#59326,#59327);
#49434=AXIS2_PLACEMENT_3D('',#97233,#59328,#59329);
#49435=AXIS2_PLACEMENT_3D('',#97256,#59330,#59331);
#49436=AXIS2_PLACEMENT_3D('',#97304,#59332,#59333);
#49437=AXIS2_PLACEMENT_3D('',#97321,#59334,#59335);
#49438=AXIS2_PLACEMENT_3D('',#97344,#59336,#59337);
#49439=AXIS2_PLACEMENT_3D('',#97361,#59338,#59339);
#49440=AXIS2_PLACEMENT_3D('',#97374,#59340,#59341);
#49441=AXIS2_PLACEMENT_3D('',#97375,#59342,#59343);
#49442=AXIS2_PLACEMENT_3D('',#97408,#59344,#59345);
#49443=AXIS2_PLACEMENT_3D('',#97413,#59346,#59347);
#49444=AXIS2_PLACEMENT_3D('',#97430,#59348,#59349);
#49445=AXIS2_PLACEMENT_3D('',#97447,#59350,#59351);
#49446=AXIS2_PLACEMENT_3D('',#97470,#59352,#59353);
#49447=AXIS2_PLACEMENT_3D('',#97487,#59354,#59355);
#49448=AXIS2_PLACEMENT_3D('',#97520,#59356,#59357);
#49449=AXIS2_PLACEMENT_3D('',#97537,#59358,#59359);
#49450=AXIS2_PLACEMENT_3D('',#97560,#59360,#59361);
#49451=AXIS2_PLACEMENT_3D('',#97608,#59362,#59363);
#49452=AXIS2_PLACEMENT_3D('',#97625,#59364,#59365);
#49453=AXIS2_PLACEMENT_3D('',#97648,#59366,#59367);
#49454=AXIS2_PLACEMENT_3D('',#97665,#59368,#59369);
#49455=AXIS2_PLACEMENT_3D('',#97678,#59370,#59371);
#49456=AXIS2_PLACEMENT_3D('',#97679,#59372,#59373);
#49457=AXIS2_PLACEMENT_3D('',#97712,#59374,#59375);
#49458=AXIS2_PLACEMENT_3D('',#97717,#59376,#59377);
#49459=AXIS2_PLACEMENT_3D('',#97734,#59378,#59379);
#49460=AXIS2_PLACEMENT_3D('',#97751,#59380,#59381);
#49461=AXIS2_PLACEMENT_3D('',#97774,#59382,#59383);
#49462=AXIS2_PLACEMENT_3D('',#97791,#59384,#59385);
#49463=AXIS2_PLACEMENT_3D('',#97824,#59386,#59387);
#49464=AXIS2_PLACEMENT_3D('',#97841,#59388,#59389);
#49465=AXIS2_PLACEMENT_3D('',#97864,#59390,#59391);
#49466=AXIS2_PLACEMENT_3D('',#97912,#59392,#59393);
#49467=AXIS2_PLACEMENT_3D('',#97929,#59394,#59395);
#49468=AXIS2_PLACEMENT_3D('',#97952,#59396,#59397);
#49469=AXIS2_PLACEMENT_3D('',#97969,#59398,#59399);
#49470=AXIS2_PLACEMENT_3D('',#97982,#59400,#59401);
#49471=AXIS2_PLACEMENT_3D('',#97983,#59402,#59403);
#49472=AXIS2_PLACEMENT_3D('',#98016,#59404,#59405);
#49473=AXIS2_PLACEMENT_3D('',#98021,#59406,#59407);
#49474=AXIS2_PLACEMENT_3D('',#98038,#59408,#59409);
#49475=AXIS2_PLACEMENT_3D('',#98055,#59410,#59411);
#49476=AXIS2_PLACEMENT_3D('',#98078,#59412,#59413);
#49477=AXIS2_PLACEMENT_3D('',#98095,#59414,#59415);
#49478=AXIS2_PLACEMENT_3D('',#98128,#59416,#59417);
#49479=AXIS2_PLACEMENT_3D('',#98145,#59418,#59419);
#49480=AXIS2_PLACEMENT_3D('',#98168,#59420,#59421);
#49481=AXIS2_PLACEMENT_3D('',#98216,#59422,#59423);
#49482=AXIS2_PLACEMENT_3D('',#98233,#59424,#59425);
#49483=AXIS2_PLACEMENT_3D('',#98256,#59426,#59427);
#49484=AXIS2_PLACEMENT_3D('',#98273,#59428,#59429);
#49485=AXIS2_PLACEMENT_3D('',#98286,#59430,#59431);
#49486=AXIS2_PLACEMENT_3D('',#98287,#59432,#59433);
#49487=AXIS2_PLACEMENT_3D('',#98320,#59434,#59435);
#49488=AXIS2_PLACEMENT_3D('',#98325,#59436,#59437);
#49489=AXIS2_PLACEMENT_3D('',#98342,#59438,#59439);
#49490=AXIS2_PLACEMENT_3D('',#98359,#59440,#59441);
#49491=AXIS2_PLACEMENT_3D('',#98382,#59442,#59443);
#49492=AXIS2_PLACEMENT_3D('',#98399,#59444,#59445);
#49493=AXIS2_PLACEMENT_3D('',#98432,#59446,#59447);
#49494=AXIS2_PLACEMENT_3D('',#98449,#59448,#59449);
#49495=AXIS2_PLACEMENT_3D('',#98472,#59450,#59451);
#49496=AXIS2_PLACEMENT_3D('',#98520,#59452,#59453);
#49497=AXIS2_PLACEMENT_3D('',#98537,#59454,#59455);
#49498=AXIS2_PLACEMENT_3D('',#98560,#59456,#59457);
#49499=AXIS2_PLACEMENT_3D('',#98577,#59458,#59459);
#49500=AXIS2_PLACEMENT_3D('',#98590,#59460,#59461);
#49501=AXIS2_PLACEMENT_3D('',#98591,#59462,#59463);
#49502=AXIS2_PLACEMENT_3D('',#98624,#59464,#59465);
#49503=AXIS2_PLACEMENT_3D('',#98629,#59466,#59467);
#49504=AXIS2_PLACEMENT_3D('',#98646,#59468,#59469);
#49505=AXIS2_PLACEMENT_3D('',#98663,#59470,#59471);
#49506=AXIS2_PLACEMENT_3D('',#98686,#59472,#59473);
#49507=AXIS2_PLACEMENT_3D('',#98703,#59474,#59475);
#49508=AXIS2_PLACEMENT_3D('',#98736,#59476,#59477);
#49509=AXIS2_PLACEMENT_3D('',#98753,#59478,#59479);
#49510=AXIS2_PLACEMENT_3D('',#98776,#59480,#59481);
#49511=AXIS2_PLACEMENT_3D('',#98824,#59482,#59483);
#49512=AXIS2_PLACEMENT_3D('',#98841,#59484,#59485);
#49513=AXIS2_PLACEMENT_3D('',#98864,#59486,#59487);
#49514=AXIS2_PLACEMENT_3D('',#98881,#59488,#59489);
#49515=AXIS2_PLACEMENT_3D('',#98894,#59490,#59491);
#49516=AXIS2_PLACEMENT_3D('',#98895,#59492,#59493);
#49517=AXIS2_PLACEMENT_3D('',#98928,#59494,#59495);
#49518=AXIS2_PLACEMENT_3D('',#98933,#59496,#59497);
#49519=AXIS2_PLACEMENT_3D('',#98950,#59498,#59499);
#49520=AXIS2_PLACEMENT_3D('',#98967,#59500,#59501);
#49521=AXIS2_PLACEMENT_3D('',#98990,#59502,#59503);
#49522=AXIS2_PLACEMENT_3D('',#99007,#59504,#59505);
#49523=AXIS2_PLACEMENT_3D('',#99040,#59506,#59507);
#49524=AXIS2_PLACEMENT_3D('',#99057,#59508,#59509);
#49525=AXIS2_PLACEMENT_3D('',#99080,#59510,#59511);
#49526=AXIS2_PLACEMENT_3D('',#99128,#59512,#59513);
#49527=AXIS2_PLACEMENT_3D('',#99145,#59514,#59515);
#49528=AXIS2_PLACEMENT_3D('',#99168,#59516,#59517);
#49529=AXIS2_PLACEMENT_3D('',#99185,#59518,#59519);
#49530=AXIS2_PLACEMENT_3D('',#99198,#59520,#59521);
#49531=AXIS2_PLACEMENT_3D('',#99199,#59522,#59523);
#49532=AXIS2_PLACEMENT_3D('',#99232,#59524,#59525);
#49533=AXIS2_PLACEMENT_3D('',#99237,#59526,#59527);
#49534=AXIS2_PLACEMENT_3D('',#99254,#59528,#59529);
#49535=AXIS2_PLACEMENT_3D('',#99271,#59530,#59531);
#49536=AXIS2_PLACEMENT_3D('',#99294,#59532,#59533);
#49537=AXIS2_PLACEMENT_3D('',#99311,#59534,#59535);
#49538=AXIS2_PLACEMENT_3D('',#99344,#59536,#59537);
#49539=AXIS2_PLACEMENT_3D('',#99361,#59538,#59539);
#49540=AXIS2_PLACEMENT_3D('',#99384,#59540,#59541);
#49541=AXIS2_PLACEMENT_3D('',#99432,#59542,#59543);
#49542=AXIS2_PLACEMENT_3D('',#99449,#59544,#59545);
#49543=AXIS2_PLACEMENT_3D('',#99472,#59546,#59547);
#49544=AXIS2_PLACEMENT_3D('',#99489,#59548,#59549);
#49545=AXIS2_PLACEMENT_3D('',#99502,#59550,#59551);
#49546=AXIS2_PLACEMENT_3D('',#99503,#59552,#59553);
#49547=AXIS2_PLACEMENT_3D('',#99536,#59554,#59555);
#49548=AXIS2_PLACEMENT_3D('',#99541,#59556,#59557);
#49549=AXIS2_PLACEMENT_3D('',#99558,#59558,#59559);
#49550=AXIS2_PLACEMENT_3D('',#99575,#59560,#59561);
#49551=AXIS2_PLACEMENT_3D('',#99598,#59562,#59563);
#49552=AXIS2_PLACEMENT_3D('',#99615,#59564,#59565);
#49553=AXIS2_PLACEMENT_3D('',#99648,#59566,#59567);
#49554=AXIS2_PLACEMENT_3D('',#99665,#59568,#59569);
#49555=AXIS2_PLACEMENT_3D('',#99688,#59570,#59571);
#49556=AXIS2_PLACEMENT_3D('',#99736,#59572,#59573);
#49557=AXIS2_PLACEMENT_3D('',#99753,#59574,#59575);
#49558=AXIS2_PLACEMENT_3D('',#99776,#59576,#59577);
#49559=AXIS2_PLACEMENT_3D('',#99793,#59578,#59579);
#49560=AXIS2_PLACEMENT_3D('',#99806,#59580,#59581);
#49561=AXIS2_PLACEMENT_3D('',#99807,#59582,#59583);
#49562=AXIS2_PLACEMENT_3D('',#99840,#59584,#59585);
#49563=AXIS2_PLACEMENT_3D('',#99845,#59586,#59587);
#49564=AXIS2_PLACEMENT_3D('',#99862,#59588,#59589);
#49565=AXIS2_PLACEMENT_3D('',#99879,#59590,#59591);
#49566=AXIS2_PLACEMENT_3D('',#99902,#59592,#59593);
#49567=AXIS2_PLACEMENT_3D('',#99919,#59594,#59595);
#49568=AXIS2_PLACEMENT_3D('',#99952,#59596,#59597);
#49569=AXIS2_PLACEMENT_3D('',#99969,#59598,#59599);
#49570=AXIS2_PLACEMENT_3D('',#99992,#59600,#59601);
#49571=AXIS2_PLACEMENT_3D('',#100040,#59602,#59603);
#49572=AXIS2_PLACEMENT_3D('',#100057,#59604,#59605);
#49573=AXIS2_PLACEMENT_3D('',#100080,#59606,#59607);
#49574=AXIS2_PLACEMENT_3D('',#100097,#59608,#59609);
#49575=AXIS2_PLACEMENT_3D('',#100110,#59610,#59611);
#49576=AXIS2_PLACEMENT_3D('',#100111,#59612,#59613);
#49577=AXIS2_PLACEMENT_3D('',#100144,#59614,#59615);
#49578=AXIS2_PLACEMENT_3D('',#100149,#59616,#59617);
#49579=AXIS2_PLACEMENT_3D('',#100166,#59618,#59619);
#49580=AXIS2_PLACEMENT_3D('',#100183,#59620,#59621);
#49581=AXIS2_PLACEMENT_3D('',#100206,#59622,#59623);
#49582=AXIS2_PLACEMENT_3D('',#100223,#59624,#59625);
#49583=AXIS2_PLACEMENT_3D('',#100256,#59626,#59627);
#49584=AXIS2_PLACEMENT_3D('',#100273,#59628,#59629);
#49585=AXIS2_PLACEMENT_3D('',#100296,#59630,#59631);
#49586=AXIS2_PLACEMENT_3D('',#100344,#59632,#59633);
#49587=AXIS2_PLACEMENT_3D('',#100361,#59634,#59635);
#49588=AXIS2_PLACEMENT_3D('',#100384,#59636,#59637);
#49589=AXIS2_PLACEMENT_3D('',#100401,#59638,#59639);
#49590=AXIS2_PLACEMENT_3D('',#100414,#59640,#59641);
#49591=AXIS2_PLACEMENT_3D('',#100415,#59642,#59643);
#49592=AXIS2_PLACEMENT_3D('',#100448,#59644,#59645);
#49593=AXIS2_PLACEMENT_3D('',#100453,#59646,#59647);
#49594=AXIS2_PLACEMENT_3D('',#100470,#59648,#59649);
#49595=AXIS2_PLACEMENT_3D('',#100487,#59650,#59651);
#49596=AXIS2_PLACEMENT_3D('',#100510,#59652,#59653);
#49597=AXIS2_PLACEMENT_3D('',#100527,#59654,#59655);
#49598=AXIS2_PLACEMENT_3D('',#100560,#59656,#59657);
#49599=AXIS2_PLACEMENT_3D('',#100577,#59658,#59659);
#49600=AXIS2_PLACEMENT_3D('',#100600,#59660,#59661);
#49601=AXIS2_PLACEMENT_3D('',#100648,#59662,#59663);
#49602=AXIS2_PLACEMENT_3D('',#100665,#59664,#59665);
#49603=AXIS2_PLACEMENT_3D('',#100688,#59666,#59667);
#49604=AXIS2_PLACEMENT_3D('',#100705,#59668,#59669);
#49605=AXIS2_PLACEMENT_3D('',#100718,#59670,#59671);
#49606=AXIS2_PLACEMENT_3D('',#100719,#59672,#59673);
#49607=AXIS2_PLACEMENT_3D('',#100752,#59674,#59675);
#49608=AXIS2_PLACEMENT_3D('',#100757,#59676,#59677);
#49609=AXIS2_PLACEMENT_3D('',#100774,#59678,#59679);
#49610=AXIS2_PLACEMENT_3D('',#100791,#59680,#59681);
#49611=AXIS2_PLACEMENT_3D('',#100814,#59682,#59683);
#49612=AXIS2_PLACEMENT_3D('',#100831,#59684,#59685);
#49613=AXIS2_PLACEMENT_3D('',#100864,#59686,#59687);
#49614=AXIS2_PLACEMENT_3D('',#100881,#59688,#59689);
#49615=AXIS2_PLACEMENT_3D('',#100904,#59690,#59691);
#49616=AXIS2_PLACEMENT_3D('',#100952,#59692,#59693);
#49617=AXIS2_PLACEMENT_3D('',#100969,#59694,#59695);
#49618=AXIS2_PLACEMENT_3D('',#100992,#59696,#59697);
#49619=AXIS2_PLACEMENT_3D('',#101009,#59698,#59699);
#49620=AXIS2_PLACEMENT_3D('',#101022,#59700,#59701);
#49621=AXIS2_PLACEMENT_3D('',#101023,#59702,#59703);
#49622=AXIS2_PLACEMENT_3D('',#101056,#59704,#59705);
#49623=AXIS2_PLACEMENT_3D('',#101061,#59706,#59707);
#49624=AXIS2_PLACEMENT_3D('',#101078,#59708,#59709);
#49625=AXIS2_PLACEMENT_3D('',#101095,#59710,#59711);
#49626=AXIS2_PLACEMENT_3D('',#101118,#59712,#59713);
#49627=AXIS2_PLACEMENT_3D('',#101135,#59714,#59715);
#49628=AXIS2_PLACEMENT_3D('',#101168,#59716,#59717);
#49629=AXIS2_PLACEMENT_3D('',#101185,#59718,#59719);
#49630=AXIS2_PLACEMENT_3D('',#101208,#59720,#59721);
#49631=AXIS2_PLACEMENT_3D('',#101256,#59722,#59723);
#49632=AXIS2_PLACEMENT_3D('',#101273,#59724,#59725);
#49633=AXIS2_PLACEMENT_3D('',#101296,#59726,#59727);
#49634=AXIS2_PLACEMENT_3D('',#101313,#59728,#59729);
#49635=AXIS2_PLACEMENT_3D('',#101326,#59730,#59731);
#49636=AXIS2_PLACEMENT_3D('',#101327,#59732,#59733);
#49637=AXIS2_PLACEMENT_3D('',#101360,#59734,#59735);
#49638=AXIS2_PLACEMENT_3D('',#101365,#59736,#59737);
#49639=AXIS2_PLACEMENT_3D('',#101382,#59738,#59739);
#49640=AXIS2_PLACEMENT_3D('',#101399,#59740,#59741);
#49641=AXIS2_PLACEMENT_3D('',#101422,#59742,#59743);
#49642=AXIS2_PLACEMENT_3D('',#101439,#59744,#59745);
#49643=AXIS2_PLACEMENT_3D('',#101472,#59746,#59747);
#49644=AXIS2_PLACEMENT_3D('',#101489,#59748,#59749);
#49645=AXIS2_PLACEMENT_3D('',#101512,#59750,#59751);
#49646=AXIS2_PLACEMENT_3D('',#101560,#59752,#59753);
#49647=AXIS2_PLACEMENT_3D('',#101577,#59754,#59755);
#49648=AXIS2_PLACEMENT_3D('',#101600,#59756,#59757);
#49649=AXIS2_PLACEMENT_3D('',#101617,#59758,#59759);
#49650=AXIS2_PLACEMENT_3D('',#101630,#59760,#59761);
#49651=AXIS2_PLACEMENT_3D('',#101631,#59762,#59763);
#49652=AXIS2_PLACEMENT_3D('',#101664,#59764,#59765);
#49653=AXIS2_PLACEMENT_3D('',#101669,#59766,#59767);
#49654=AXIS2_PLACEMENT_3D('',#101686,#59768,#59769);
#49655=AXIS2_PLACEMENT_3D('',#101703,#59770,#59771);
#49656=AXIS2_PLACEMENT_3D('',#101726,#59772,#59773);
#49657=AXIS2_PLACEMENT_3D('',#101743,#59774,#59775);
#49658=AXIS2_PLACEMENT_3D('',#101776,#59776,#59777);
#49659=AXIS2_PLACEMENT_3D('',#101793,#59778,#59779);
#49660=AXIS2_PLACEMENT_3D('',#101816,#59780,#59781);
#49661=AXIS2_PLACEMENT_3D('',#101864,#59782,#59783);
#49662=AXIS2_PLACEMENT_3D('',#101881,#59784,#59785);
#49663=AXIS2_PLACEMENT_3D('',#101904,#59786,#59787);
#49664=AXIS2_PLACEMENT_3D('',#101921,#59788,#59789);
#49665=AXIS2_PLACEMENT_3D('',#101934,#59790,#59791);
#49666=AXIS2_PLACEMENT_3D('',#101935,#59792,#59793);
#49667=AXIS2_PLACEMENT_3D('',#101968,#59794,#59795);
#49668=AXIS2_PLACEMENT_3D('',#101973,#59796,#59797);
#49669=AXIS2_PLACEMENT_3D('',#101990,#59798,#59799);
#49670=AXIS2_PLACEMENT_3D('',#102007,#59800,#59801);
#49671=AXIS2_PLACEMENT_3D('',#102030,#59802,#59803);
#49672=AXIS2_PLACEMENT_3D('',#102047,#59804,#59805);
#49673=AXIS2_PLACEMENT_3D('',#102080,#59806,#59807);
#49674=AXIS2_PLACEMENT_3D('',#102097,#59808,#59809);
#49675=AXIS2_PLACEMENT_3D('',#102120,#59810,#59811);
#49676=AXIS2_PLACEMENT_3D('',#102168,#59812,#59813);
#49677=AXIS2_PLACEMENT_3D('',#102185,#59814,#59815);
#49678=AXIS2_PLACEMENT_3D('',#102208,#59816,#59817);
#49679=AXIS2_PLACEMENT_3D('',#102225,#59818,#59819);
#49680=AXIS2_PLACEMENT_3D('',#102238,#59820,#59821);
#49681=AXIS2_PLACEMENT_3D('',#102239,#59822,#59823);
#49682=AXIS2_PLACEMENT_3D('',#102272,#59824,#59825);
#49683=AXIS2_PLACEMENT_3D('',#102277,#59826,#59827);
#49684=AXIS2_PLACEMENT_3D('',#102294,#59828,#59829);
#49685=AXIS2_PLACEMENT_3D('',#102311,#59830,#59831);
#49686=AXIS2_PLACEMENT_3D('',#102334,#59832,#59833);
#49687=AXIS2_PLACEMENT_3D('',#102351,#59834,#59835);
#49688=AXIS2_PLACEMENT_3D('',#102384,#59836,#59837);
#49689=AXIS2_PLACEMENT_3D('',#102401,#59838,#59839);
#49690=AXIS2_PLACEMENT_3D('',#102424,#59840,#59841);
#49691=AXIS2_PLACEMENT_3D('',#102472,#59842,#59843);
#49692=AXIS2_PLACEMENT_3D('',#102489,#59844,#59845);
#49693=AXIS2_PLACEMENT_3D('',#102512,#59846,#59847);
#49694=AXIS2_PLACEMENT_3D('',#102529,#59848,#59849);
#49695=AXIS2_PLACEMENT_3D('',#102542,#59850,#59851);
#49696=AXIS2_PLACEMENT_3D('',#102543,#59852,#59853);
#49697=AXIS2_PLACEMENT_3D('',#102576,#59854,#59855);
#49698=AXIS2_PLACEMENT_3D('',#102581,#59856,#59857);
#49699=AXIS2_PLACEMENT_3D('',#102598,#59858,#59859);
#49700=AXIS2_PLACEMENT_3D('',#102615,#59860,#59861);
#49701=AXIS2_PLACEMENT_3D('',#102638,#59862,#59863);
#49702=AXIS2_PLACEMENT_3D('',#102655,#59864,#59865);
#49703=AXIS2_PLACEMENT_3D('',#102688,#59866,#59867);
#49704=AXIS2_PLACEMENT_3D('',#102705,#59868,#59869);
#49705=AXIS2_PLACEMENT_3D('',#102728,#59870,#59871);
#49706=AXIS2_PLACEMENT_3D('',#102776,#59872,#59873);
#49707=AXIS2_PLACEMENT_3D('',#102793,#59874,#59875);
#49708=AXIS2_PLACEMENT_3D('',#102816,#59876,#59877);
#49709=AXIS2_PLACEMENT_3D('',#102833,#59878,#59879);
#49710=AXIS2_PLACEMENT_3D('',#102846,#59880,#59881);
#49711=AXIS2_PLACEMENT_3D('',#102847,#59882,#59883);
#49712=AXIS2_PLACEMENT_3D('',#102880,#59884,#59885);
#49713=AXIS2_PLACEMENT_3D('',#102885,#59886,#59887);
#49714=AXIS2_PLACEMENT_3D('',#102902,#59888,#59889);
#49715=AXIS2_PLACEMENT_3D('',#102919,#59890,#59891);
#49716=AXIS2_PLACEMENT_3D('',#102942,#59892,#59893);
#49717=AXIS2_PLACEMENT_3D('',#102959,#59894,#59895);
#49718=AXIS2_PLACEMENT_3D('',#102992,#59896,#59897);
#49719=AXIS2_PLACEMENT_3D('',#103009,#59898,#59899);
#49720=AXIS2_PLACEMENT_3D('',#103032,#59900,#59901);
#49721=AXIS2_PLACEMENT_3D('',#103080,#59902,#59903);
#49722=AXIS2_PLACEMENT_3D('',#103097,#59904,#59905);
#49723=AXIS2_PLACEMENT_3D('',#103120,#59906,#59907);
#49724=AXIS2_PLACEMENT_3D('',#103137,#59908,#59909);
#49725=AXIS2_PLACEMENT_3D('',#103150,#59910,#59911);
#49726=AXIS2_PLACEMENT_3D('',#103151,#59912,#59913);
#49727=AXIS2_PLACEMENT_3D('',#103184,#59914,#59915);
#49728=AXIS2_PLACEMENT_3D('',#103189,#59916,#59917);
#49729=AXIS2_PLACEMENT_3D('',#103206,#59918,#59919);
#49730=AXIS2_PLACEMENT_3D('',#103223,#59920,#59921);
#49731=AXIS2_PLACEMENT_3D('',#103246,#59922,#59923);
#49732=AXIS2_PLACEMENT_3D('',#103263,#59924,#59925);
#49733=AXIS2_PLACEMENT_3D('',#103296,#59926,#59927);
#49734=AXIS2_PLACEMENT_3D('',#103313,#59928,#59929);
#49735=AXIS2_PLACEMENT_3D('',#103336,#59930,#59931);
#49736=AXIS2_PLACEMENT_3D('',#103384,#59932,#59933);
#49737=AXIS2_PLACEMENT_3D('',#103401,#59934,#59935);
#49738=AXIS2_PLACEMENT_3D('',#103424,#59936,#59937);
#49739=AXIS2_PLACEMENT_3D('',#103441,#59938,#59939);
#49740=AXIS2_PLACEMENT_3D('',#103454,#59940,#59941);
#49741=AXIS2_PLACEMENT_3D('',#103455,#59942,#59943);
#49742=AXIS2_PLACEMENT_3D('',#103488,#59944,#59945);
#49743=AXIS2_PLACEMENT_3D('',#103493,#59946,#59947);
#49744=AXIS2_PLACEMENT_3D('',#103510,#59948,#59949);
#49745=AXIS2_PLACEMENT_3D('',#103527,#59950,#59951);
#49746=AXIS2_PLACEMENT_3D('',#103550,#59952,#59953);
#49747=AXIS2_PLACEMENT_3D('',#103567,#59954,#59955);
#49748=AXIS2_PLACEMENT_3D('',#103600,#59956,#59957);
#49749=AXIS2_PLACEMENT_3D('',#103617,#59958,#59959);
#49750=AXIS2_PLACEMENT_3D('',#103640,#59960,#59961);
#49751=AXIS2_PLACEMENT_3D('',#103688,#59962,#59963);
#49752=AXIS2_PLACEMENT_3D('',#103705,#59964,#59965);
#49753=AXIS2_PLACEMENT_3D('',#103728,#59966,#59967);
#49754=AXIS2_PLACEMENT_3D('',#103745,#59968,#59969);
#49755=AXIS2_PLACEMENT_3D('',#103758,#59970,#59971);
#49756=AXIS2_PLACEMENT_3D('',#103759,#59972,#59973);
#49757=AXIS2_PLACEMENT_3D('',#103792,#59974,#59975);
#49758=AXIS2_PLACEMENT_3D('',#103797,#59976,#59977);
#49759=AXIS2_PLACEMENT_3D('',#103814,#59978,#59979);
#49760=AXIS2_PLACEMENT_3D('',#103831,#59980,#59981);
#49761=AXIS2_PLACEMENT_3D('',#103854,#59982,#59983);
#49762=AXIS2_PLACEMENT_3D('',#103871,#59984,#59985);
#49763=AXIS2_PLACEMENT_3D('',#103904,#59986,#59987);
#49764=AXIS2_PLACEMENT_3D('',#103921,#59988,#59989);
#49765=AXIS2_PLACEMENT_3D('',#103944,#59990,#59991);
#49766=AXIS2_PLACEMENT_3D('',#103992,#59992,#59993);
#49767=AXIS2_PLACEMENT_3D('',#104009,#59994,#59995);
#49768=AXIS2_PLACEMENT_3D('',#104032,#59996,#59997);
#49769=AXIS2_PLACEMENT_3D('',#104049,#59998,#59999);
#49770=AXIS2_PLACEMENT_3D('',#104062,#60000,#60001);
#49771=AXIS2_PLACEMENT_3D('',#104063,#60002,#60003);
#49772=AXIS2_PLACEMENT_3D('',#104112,#60004,#60005);
#49773=AXIS2_PLACEMENT_3D('',#104129,#60006,#60007);
#49774=AXIS2_PLACEMENT_3D('',#104136,#60008,#60009);
#49775=AXIS2_PLACEMENT_3D('',#104141,#60010,#60011);
#49776=AXIS2_PLACEMENT_3D('',#104158,#60012,#60013);
#49777=AXIS2_PLACEMENT_3D('',#104175,#60014,#60015);
#49778=AXIS2_PLACEMENT_3D('',#104208,#60016,#60017);
#49779=AXIS2_PLACEMENT_3D('',#104225,#60018,#60019);
#49780=AXIS2_PLACEMENT_3D('',#104248,#60020,#60021);
#49781=AXIS2_PLACEMENT_3D('',#104296,#60022,#60023);
#49782=AXIS2_PLACEMENT_3D('',#104313,#60024,#60025);
#49783=AXIS2_PLACEMENT_3D('',#104336,#60026,#60027);
#49784=AXIS2_PLACEMENT_3D('',#104353,#60028,#60029);
#49785=AXIS2_PLACEMENT_3D('',#104366,#60030,#60031);
#49786=AXIS2_PLACEMENT_3D('',#104367,#60032,#60033);
#49787=AXIS2_PLACEMENT_3D('',#104400,#60034,#60035);
#49788=AXIS2_PLACEMENT_3D('',#104405,#60036,#60037);
#49789=AXIS2_PLACEMENT_3D('',#104422,#60038,#60039);
#49790=AXIS2_PLACEMENT_3D('',#104439,#60040,#60041);
#49791=AXIS2_PLACEMENT_3D('',#104462,#60042,#60043);
#49792=AXIS2_PLACEMENT_3D('',#104479,#60044,#60045);
#49793=AXIS2_PLACEMENT_3D('',#104512,#60046,#60047);
#49794=AXIS2_PLACEMENT_3D('',#104529,#60048,#60049);
#49795=AXIS2_PLACEMENT_3D('',#104552,#60050,#60051);
#49796=AXIS2_PLACEMENT_3D('',#104600,#60052,#60053);
#49797=AXIS2_PLACEMENT_3D('',#104617,#60054,#60055);
#49798=AXIS2_PLACEMENT_3D('',#104640,#60056,#60057);
#49799=AXIS2_PLACEMENT_3D('',#104657,#60058,#60059);
#49800=AXIS2_PLACEMENT_3D('',#104670,#60060,#60061);
#49801=AXIS2_PLACEMENT_3D('',#104671,#60062,#60063);
#49802=AXIS2_PLACEMENT_3D('',#104704,#60064,#60065);
#49803=AXIS2_PLACEMENT_3D('',#104709,#60066,#60067);
#49804=AXIS2_PLACEMENT_3D('',#104726,#60068,#60069);
#49805=AXIS2_PLACEMENT_3D('',#104743,#60070,#60071);
#49806=AXIS2_PLACEMENT_3D('',#104766,#60072,#60073);
#49807=AXIS2_PLACEMENT_3D('',#104783,#60074,#60075);
#49808=AXIS2_PLACEMENT_3D('',#104816,#60076,#60077);
#49809=AXIS2_PLACEMENT_3D('',#104833,#60078,#60079);
#49810=AXIS2_PLACEMENT_3D('',#104856,#60080,#60081);
#49811=AXIS2_PLACEMENT_3D('',#104904,#60082,#60083);
#49812=AXIS2_PLACEMENT_3D('',#104921,#60084,#60085);
#49813=AXIS2_PLACEMENT_3D('',#104944,#60086,#60087);
#49814=AXIS2_PLACEMENT_3D('',#104961,#60088,#60089);
#49815=AXIS2_PLACEMENT_3D('',#104974,#60090,#60091);
#49816=AXIS2_PLACEMENT_3D('',#104975,#60092,#60093);
#49817=AXIS2_PLACEMENT_3D('',#105008,#60094,#60095);
#49818=AXIS2_PLACEMENT_3D('',#105013,#60096,#60097);
#49819=AXIS2_PLACEMENT_3D('',#105030,#60098,#60099);
#49820=AXIS2_PLACEMENT_3D('',#105047,#60100,#60101);
#49821=AXIS2_PLACEMENT_3D('',#105070,#60102,#60103);
#49822=AXIS2_PLACEMENT_3D('',#105087,#60104,#60105);
#49823=AXIS2_PLACEMENT_3D('',#105120,#60106,#60107);
#49824=AXIS2_PLACEMENT_3D('',#105137,#60108,#60109);
#49825=AXIS2_PLACEMENT_3D('',#105160,#60110,#60111);
#49826=AXIS2_PLACEMENT_3D('',#105208,#60112,#60113);
#49827=AXIS2_PLACEMENT_3D('',#105225,#60114,#60115);
#49828=AXIS2_PLACEMENT_3D('',#105248,#60116,#60117);
#49829=AXIS2_PLACEMENT_3D('',#105265,#60118,#60119);
#49830=AXIS2_PLACEMENT_3D('',#105278,#60120,#60121);
#49831=AXIS2_PLACEMENT_3D('',#105279,#60122,#60123);
#49832=AXIS2_PLACEMENT_3D('',#105312,#60124,#60125);
#49833=AXIS2_PLACEMENT_3D('',#105317,#60126,#60127);
#49834=AXIS2_PLACEMENT_3D('',#105334,#60128,#60129);
#49835=AXIS2_PLACEMENT_3D('',#105351,#60130,#60131);
#49836=AXIS2_PLACEMENT_3D('',#105374,#60132,#60133);
#49837=AXIS2_PLACEMENT_3D('',#105391,#60134,#60135);
#49838=AXIS2_PLACEMENT_3D('',#105424,#60136,#60137);
#49839=AXIS2_PLACEMENT_3D('',#105441,#60138,#60139);
#49840=AXIS2_PLACEMENT_3D('',#105464,#60140,#60141);
#49841=AXIS2_PLACEMENT_3D('',#105512,#60142,#60143);
#49842=AXIS2_PLACEMENT_3D('',#105529,#60144,#60145);
#49843=AXIS2_PLACEMENT_3D('',#105552,#60146,#60147);
#49844=AXIS2_PLACEMENT_3D('',#105569,#60148,#60149);
#49845=AXIS2_PLACEMENT_3D('',#105582,#60150,#60151);
#49846=AXIS2_PLACEMENT_3D('',#105583,#60152,#60153);
#49847=AXIS2_PLACEMENT_3D('',#105616,#60154,#60155);
#49848=AXIS2_PLACEMENT_3D('',#105621,#60156,#60157);
#49849=AXIS2_PLACEMENT_3D('',#105638,#60158,#60159);
#49850=AXIS2_PLACEMENT_3D('',#105655,#60160,#60161);
#49851=AXIS2_PLACEMENT_3D('',#105678,#60162,#60163);
#49852=AXIS2_PLACEMENT_3D('',#105695,#60164,#60165);
#49853=AXIS2_PLACEMENT_3D('',#105728,#60166,#60167);
#49854=AXIS2_PLACEMENT_3D('',#105745,#60168,#60169);
#49855=AXIS2_PLACEMENT_3D('',#105768,#60170,#60171);
#49856=AXIS2_PLACEMENT_3D('',#105816,#60172,#60173);
#49857=AXIS2_PLACEMENT_3D('',#105833,#60174,#60175);
#49858=AXIS2_PLACEMENT_3D('',#105856,#60176,#60177);
#49859=AXIS2_PLACEMENT_3D('',#105873,#60178,#60179);
#49860=AXIS2_PLACEMENT_3D('',#105886,#60180,#60181);
#49861=AXIS2_PLACEMENT_3D('',#105887,#60182,#60183);
#49862=AXIS2_PLACEMENT_3D('',#105920,#60184,#60185);
#49863=AXIS2_PLACEMENT_3D('',#105925,#60186,#60187);
#49864=AXIS2_PLACEMENT_3D('',#105942,#60188,#60189);
#49865=AXIS2_PLACEMENT_3D('',#105959,#60190,#60191);
#49866=AXIS2_PLACEMENT_3D('',#105982,#60192,#60193);
#49867=AXIS2_PLACEMENT_3D('',#105999,#60194,#60195);
#49868=AXIS2_PLACEMENT_3D('',#106032,#60196,#60197);
#49869=AXIS2_PLACEMENT_3D('',#106049,#60198,#60199);
#49870=AXIS2_PLACEMENT_3D('',#106072,#60200,#60201);
#49871=AXIS2_PLACEMENT_3D('',#106120,#60202,#60203);
#49872=AXIS2_PLACEMENT_3D('',#106137,#60204,#60205);
#49873=AXIS2_PLACEMENT_3D('',#106160,#60206,#60207);
#49874=AXIS2_PLACEMENT_3D('',#106177,#60208,#60209);
#49875=AXIS2_PLACEMENT_3D('',#106190,#60210,#60211);
#49876=AXIS2_PLACEMENT_3D('',#106191,#60212,#60213);
#50541=DIRECTION('axis',(0.,0.,1.));
#50542=DIRECTION('refdir',(1.,0.,0.));
#50543=DIRECTION('center_axis',(0.,1.,-1.45983193964168E-32));
#50544=DIRECTION('ref_axis',(-1.,0.,0.));
#50545=DIRECTION('center_axis',(0.,-1.,6.6666666666222E-12));
#50546=DIRECTION('ref_axis',(1.,0.,0.));
#50547=DIRECTION('',(0.,-1.,1.45983193964168E-32));
#50548=DIRECTION('center_axis',(0.,-1.,6.6666666666222E-12));
#50549=DIRECTION('ref_axis',(1.,0.,0.));
#50550=DIRECTION('center_axis',(0.,-1.,0.));
#50551=DIRECTION('ref_axis',(0.,0.,-1.));
#50552=DIRECTION('',(8.65956056235495E-17,0.707106781186546,-0.707106781186549));
#50553=DIRECTION('center_axis',(0.,1.,-1.81818181817851E-12));
#50554=DIRECTION('ref_axis',(1.,0.,0.));
#50555=DIRECTION('center_axis',(0.470181317528933,0.878565373676135,0.0839786450478365));
#50556=DIRECTION('ref_axis',(-0.430724319865323,0.14537209543693,0.890698329483575));
#50557=DIRECTION('center_axis',(-0.431958871988205,0.885461953092126,0.171372875732875));
#50558=DIRECTION('ref_axis',(0.528713288045884,0.0946722161324461,0.843504256383026));
#50559=DIRECTION('center_axis',(0.476999112541715,0.878565373674465,0.0243871034496678));
#50560=DIRECTION('ref_axis',(-0.315693828177029,0.145372095444832,0.937658978902731));
#50561=DIRECTION('center_axis',(-0.407074030600313,0.885461953092291,0.224160351616429));
#50562=DIRECTION('ref_axis',(0.630263341829312,0.0946722161298985,0.770587627359278));
#50563=DIRECTION('center_axis',(0.47629434659331,0.878565373678942,-0.0355890372956794));
#50564=DIRECTION('ref_axis',(-0.195684656275447,0.145372095425782,0.969832186086788));
#50565=DIRECTION('center_axis',(-0.375769388577795,0.885461953092213,0.273412684844712));
#50566=DIRECTION('ref_axis',(0.721873766209692,0.0946722161311678,0.685518371125857));
#50567=DIRECTION('center_axis',(0.468078134286444,0.878565373674476,-0.0950039177252697));
#50568=DIRECTION('ref_axis',(-0.0725894203991882,0.145372095453218,0.986710560351743));
#50569=DIRECTION('center_axis',(-0.338538638842928,0.885461953090034,0.318353136689997));
#50570=DIRECTION('ref_axis',(0.802099810062447,0.0946722161536946,0.589638080678593));
#50571=DIRECTION('center_axis',(0.452480050181005,0.878565373677713,-0.152920529565967));
#50572=DIRECTION('ref_axis',(0.0516505940339392,0.145372095401793,0.988027919653303));
#50573=DIRECTION('center_axis',(-0.295968932481847,0.885461953094103,0.358272969435782));
#50574=DIRECTION('ref_axis',(0.869676260782141,0.0946722161116901,0.484458845443548));
#50575=DIRECTION('center_axis',(0.429746085383579,0.87856537367488,-0.208425493347162));
#50576=DIRECTION('ref_axis',(0.175076047702811,0.145372095419575,0.97376348842729));
#50577=DIRECTION('center_axis',(-0.248731619302135,0.885461953092945,0.392542623397975));
#50578=DIRECTION('ref_axis',(0.923537397331102,0.0946722161240135,0.371639404833586));
#50579=DIRECTION('center_axis',(0.400234768100223,0.878565373673598,-0.260643462579693));
#50580=DIRECTION('ref_axis',(0.295740447509778,0.145372095427147,0.94414222529121));
#50581=DIRECTION('center_axis',(-0.197571659886334,0.885461953093207,0.420621645703265));
#50582=DIRECTION('ref_axis',(0.962833797434217,0.0946722161215446,0.252958988796685));
#50583=DIRECTION('center_axis',(0.364411509455074,0.878565373679554,-0.3087509286593));
#50584=DIRECTION('ref_axis',(0.411740843713011,0.145372095421878,0.899631275296246));
#50585=DIRECTION('center_axis',(-0.143295877392587,0.885461953091437,0.442067213384781));
#50586=DIRECTION('ref_axis',(0.986945733379162,0.0946722161389514,0.130289258406083));
#50587=DIRECTION('center_axis',(0.322841263593088,0.878565373676854,-0.35198920821194));
#50588=DIRECTION('ref_axis',(0.521247840989627,0.145372095407339,0.840932602614819));
#50589=DIRECTION('center_axis',(-0.0867602332807392,0.885461953092501,0.456541117038417));
#50590=DIRECTION('ref_axis',(0.995492945540836,0.0946722161283294,0.0055647885656998));
#50591=DIRECTION('center_axis',(0.276179618172625,0.878565373680365,-0.389676407646017));
#50592=DIRECTION('ref_axis',(0.622534448311122,0.145372095417224,0.768971920514639));
#50593=DIRECTION('center_axis',(-0.0288563284685773,0.88546195309315,0.463815094549301));
#50594=DIRECTION('ref_axis',(0.988340639271075,0.0946722161237086,-0.11924744131204));
#50595=DIRECTION('center_axis',(0.225162455177494,0.878565373680138,-0.421218177372158));
#50596=DIRECTION('ref_axis',(0.714003315567455,0.145372095415238,0.684884091823766));
#50597=DIRECTION('center_axis',(0.0295026578968582,0.885461953094759,0.463774430945299));
#50598=DIRECTION('ref_axis',(0.965601610712996,0.09467221610468,-0.242179067812014));
#50599=DIRECTION('center_axis',(0.170594345751946,0.878565373678822,-0.446117084821976));
#50600=DIRECTION('ref_axis',(0.794211924045204,0.145372095394835,0.589995231832369));
#50601=DIRECTION('center_axis',(0.0873963697059013,0.885461953095116,0.45641976752022));
#50602=DIRECTION('ref_axis',(0.927634467930516,0.0946722161010694,-0.361291385734258));
#50603=DIRECTION('center_axis',(0.113335861610607,0.878565373681749,-0.463980459330379));
#50604=DIRECTION('ref_axis',(0.861895335995359,0.145372095376466,0.485801794639854));
#50605=DIRECTION('center_axis',(0.143911788527641,0.885461953092717,0.441867091723299));
#50606=DIRECTION('ref_axis',(0.875037975450806,0.0946722161263171,-0.474705922664428));
#50607=DIRECTION('center_axis',(0.0542900032060115,0.878565373680826,-0.474526584841104));
#50608=DIRECTION('ref_axis',(0.915986143629403,0.145372095381604,0.373946972929714));
#50609=DIRECTION('center_axis',(0.198157632482187,0.885461953090638,0.420345907935318));
#50610=DIRECTION('ref_axis',(0.808641611378265,0.0946722161478671,-0.580634063621154));
#50611=DIRECTION('center_axis',(-0.00561204098253765,0.878565373679935,
-0.47758914263899));
#50612=DIRECTION('ref_axis',(0.955631302573077,0.145372095420351,0.256194784130318));
#50613=DIRECTION('center_axis',(0.2492784122292,0.88546195309152,0.392195618057929));
#50614=DIRECTION('ref_axis',(0.729492486028889,0.0946722161374401,-0.677405258555775));
#50615=DIRECTION('center_axis',(-0.0654255799087193,0.878565373682163,-0.473119834355239));
#50616=DIRECTION('ref_axis',(0.980205585037586,0.145372095405399,0.134402250496665));
#50617=DIRECTION('center_axis',(0.296467922535388,0.885461953097206,0.357860168955463));
#50618=DIRECTION('ref_axis',(0.638838828380997,0.094672216080367,-0.763493367918299));
#50619=DIRECTION('center_axis',(-0.124207318411051,0.878565373676778,-0.461189143659432));
#50620=DIRECTION('ref_axis',(0.989321439874569,0.14537209543964,0.0104901130593315));
#50621=DIRECTION('center_axis',(0.338981956513975,0.885461953090639,0.317881051317736));
#50622=DIRECTION('ref_axis',(0.538110300825814,0.0946722161462289,-0.837540730732013));
#50623=DIRECTION('center_axis',(-0.181030233209146,0.878565373684908,-0.441985224669491));
#50624=DIRECTION('ref_axis',(0.982835104623311,0.145372095356493,-0.113587459746872));
#50625=DIRECTION('center_axis',(0.376150042589092,0.885461953090726,0.272888759550445));
#50626=DIRECTION('ref_axis',(0.428895452353032,0.0946722161448653,-0.898379575926072));
#50627=DIRECTION('center_axis',(-0.234998193211149,0.878565373675165,-0.415810934640389));
#50628=DIRECTION('ref_axis',(0.960848872626057,0.145372095417506,-0.23587369045139));
#50629=DIRECTION('center_axis',(0.407386017797145,0.885461953092542,0.223592849011155));
#50630=DIRECTION('ref_axis',(0.312916666379303,0.0946722161266354,-0.945050438545867));
#50631=DIRECTION('center_axis',(-0.285260091217153,0.878565373681205,-0.383079057802938));
#50632=DIRECTION('ref_axis',(0.923709479949017,0.145372095379356,-0.354440052106603));
#50633=DIRECTION('center_axis',(0.432197272136797,0.885461953093454,0.170770745683908));
#50634=DIRECTION('ref_axis',(0.192002997652503,0.0946722161181877,-0.976817291200214));
#50635=DIRECTION('center_axis',(-0.331023267233894,0.878565373679115,-0.344305795364926));
#50636=DIRECTION('ref_axis',(0.872002636966723,0.14537209540145,-0.467416682416955));
#50637=DIRECTION('center_axis',(0.450192517310335,0.885461953094449,0.115255485682668));
#50638=DIRECTION('ref_axis',(0.0680613269555309,0.0946722161089431,-0.993179151648923));
#50639=DIRECTION('center_axis',(-0.371566008536628,0.87856537368448,-0.300102624884903));
#50640=DIRECTION('ref_axis',(0.806543791497076,0.145372095359132,-0.573021872434566));
#50641=DIRECTION('center_axis',(0.46108795755193,0.885461953094479,0.057922577831964));
#50642=DIRECTION('ref_axis',(-0.0569537115214824,0.0946722161090591,-0.993877983577928));
#50643=DIRECTION('center_axis',(-0.406248931959853,0.87856537368365,-0.251166656715393));
#50644=DIRECTION('ref_axis',(0.728365268655383,0.145372095392437,-0.669590165174029));
#50645=DIRECTION('center_axis',(0.464711765269602,0.885461953090712,-0.000323803632485891));
#50646=DIRECTION('ref_axis',(-0.181070555926217,0.0946722161451853,-0.97890276599197));
#50647=DIRECTION('center_axis',(-0.434525067050534,0.878565373681443,-0.198269640320233));
#50648=DIRECTION('ref_axis',(0.638699990373455,0.145372095395856,-0.75559862107945));
#50649=DIRECTION('center_axis',(0.46100679083195,0.885461953093654,-0.0585650785912394));
#50650=DIRECTION('ref_axis',(-0.302331809531034,0.094672216116691,-0.9484896670187));
#50651=DIRECTION('center_axis',(-0.455948482255112,0.878565373679943,-0.142245793259001));
#50652=DIRECTION('ref_axis',(0.538962031740231,0.145372095419794,-0.829690835321025));
#50653=DIRECTION('center_axis',(0.450031463915207,0.885461953093974,-0.115882747246262));
#50654=DIRECTION('ref_axis',(-0.418825109881704,0.0946722161145024,-0.90311831939594));
#50655=DIRECTION('center_axis',(-0.470181317508262,0.878565373682988,-0.0839786450918718));
#50656=DIRECTION('ref_axis',(0.430724319845604,0.145372095368486,-0.890698329504281));
#50657=DIRECTION('center_axis',(0.431958824442153,0.885461961244214,-0.171372953455624));
#50658=DIRECTION('ref_axis',(-0.528713326932488,0.0946721347508802,-0.843504241142682));
#50659=DIRECTION('center_axis',(-0.476999112532178,0.878565373678833,-0.0243871034788126));
#50660=DIRECTION('ref_axis',(0.315693828207894,0.145372095426544,-0.937658978895174));
#50661=DIRECTION('center_axis',(0.407073973687001,0.885461961244578,-0.224160422768117));
#50662=DIRECTION('ref_axis',(-0.630263378499859,0.0946721347472922,-0.770587607364882));
#50663=DIRECTION('center_axis',(-0.476294346599364,0.878565373674358,0.0355890373278207));
#50664=DIRECTION('ref_axis',(0.195684656259467,0.145372095454662,-0.969832186085683));
#50665=DIRECTION('center_axis',(0.375769388575765,0.885461953092483,-0.273412684846627));
#50666=DIRECTION('ref_axis',(-0.721873766210669,0.0946722161286249,-0.68551837112518));
#50667=DIRECTION('center_axis',(-0.468078134283175,0.878565373681661,0.0950039176749343));
#50668=DIRECTION('ref_axis',(0.0725894203633281,0.145372095377612,-0.98671056036552));
#50669=DIRECTION('center_axis',(0.338538638809758,0.885461953093661,-0.318353136715184));
#50670=DIRECTION('ref_axis',(-0.802099810076275,0.0946722161163834,-0.589638080665773));
#50671=DIRECTION('center_axis',(-0.45248005018208,0.878565373679752,0.152920529551074));
#50672=DIRECTION('ref_axis',(-0.0516505939966993,0.145372095404103,-0.98802791965491));
#50673=DIRECTION('center_axis',(0.295968932486342,0.885461953093587,-0.358272969433345));
#50674=DIRECTION('ref_axis',(-0.869676260780677,0.0946722161163057,-0.484458845445274));
#50675=DIRECTION('center_axis',(-0.429746085391914,0.878565373681383,0.208425493302567));
#50676=DIRECTION('ref_axis',(-0.17507604768326,0.145372095379237,-0.973763488436827));
#50677=DIRECTION('center_axis',(0.248731619323381,0.885461953090817,-0.392542623389315));
#50678=DIRECTION('ref_axis',(-0.923537397325435,0.0946722161445156,-0.371639404842446));
#50679=DIRECTION('center_axis',(-0.400234768116551,0.878565373680973,0.260643462529762));
#50680=DIRECTION('ref_axis',(-0.295740447488144,0.145372095380758,-0.944142225305129));
#50681=DIRECTION('center_axis',(0.197571659905606,0.885461953091393,-0.420621645698031));
#50682=DIRECTION('ref_axis',(-0.962833797430249,0.0946722161392853,-0.252958988805146));
#50683=DIRECTION('center_axis',(-0.364411509442283,0.878565373675362,0.308750928686326));
#50684=DIRECTION('ref_axis',(-0.411740843782727,0.14537209541642,-0.89963127526522));
#50685=DIRECTION('center_axis',(0.143295877377764,0.885461953092811,-0.442067213386835));
#50686=DIRECTION('ref_axis',(-0.986945733381312,0.0946722161256203,-0.130289258399489));
#50687=DIRECTION('center_axis',(-0.32284126361482,0.878565373682674,0.35198920817748));
#50688=DIRECTION('ref_axis',(-0.521247840921593,0.145372095402714,-0.840932602657789));
#50689=DIRECTION('center_axis',(0.0867602333015312,0.885461953090746,-0.456541117037869));
#50690=DIRECTION('ref_axis',(-0.995492945539012,0.0946722161469667,-0.00556478857491395));
#50691=DIRECTION('center_axis',(-0.276179618153645,0.878565373676274,0.389676407668691));
#50692=DIRECTION('ref_axis',(-0.622534448319981,0.145372095443063,-0.768971920502582));
#50693=DIRECTION('center_axis',(0.0288563284973618,0.885461953090383,-0.463815094552793));
#50694=DIRECTION('ref_axis',(-0.988340639270242,0.0946722161494783,0.119247441298489));
#50695=DIRECTION('center_axis',(-0.225162455131814,0.878565373671252,0.42121817741511));
#50696=DIRECTION('ref_axis',(-0.714003315623988,0.145372095441861,-0.684884091759178));
#50697=DIRECTION('center_axis',(-0.0295026578689006,0.885461953092215,-0.463774430951935));
#50698=DIRECTION('ref_axis',(-0.965601610713841,0.0946722161302304,0.242179067798656));
#50699=DIRECTION('center_axis',(-0.170594345743913,0.878565373677633,0.446117084827388));
#50700=DIRECTION('ref_axis',(-0.794211924010337,0.145372095431894,-0.589995231870173));
#50701=DIRECTION('center_axis',(-0.0873963696730955,0.885461953092048,-0.456419767532454));
#50702=DIRECTION('ref_axis',(-0.927634467933496,0.0946722161323006,0.361291385718422));
#50703=DIRECTION('center_axis',(-0.113335861582412,0.878565373677204,0.463980459345873));
#50704=DIRECTION('ref_axis',(-0.861895335999343,0.145372095404732,-0.485801794624327));
#50705=DIRECTION('center_axis',(-0.143911788525932,0.885461953092382,-0.441867091724528));
#50706=DIRECTION('ref_axis',(-0.875037975451224,0.0946722161280739,0.474705922663308));
#50707=DIRECTION('center_axis',(-0.0542900031638738,0.878565373674397,0.474526584857829));
#50708=DIRECTION('ref_axis',(-0.915986143631796,0.145372095421936,-0.373946972908173));
#50709=DIRECTION('center_axis',(-0.198157632504344,0.885461953092994,-0.42034590791991));
#50710=DIRECTION('ref_axis',(-0.808641611372961,0.094672216123831,0.58063406363246));
#50711=DIRECTION('center_axis',(0.005612041014381,0.878565373675177,0.477589142647369));
#50712=DIRECTION('ref_axis',(-0.955631302593608,0.145372095417575,-0.25619478405531));
#50713=DIRECTION('center_axis',(-0.249278412244268,0.885461953093368,-0.392195618044179));
#50714=DIRECTION('ref_axis',(-0.729492486023782,0.0946722161193055,0.677405258563809));
#50715=DIRECTION('center_axis',(0.0654255799497689,0.8785653736764,0.473119834360264));
#50716=DIRECTION('ref_axis',(-0.980205585048038,0.145372095409979,-0.134402250415481));
#50717=DIRECTION('center_axis',(-0.296467922503249,0.88546195309275,-0.357860168993115));
#50718=DIRECTION('ref_axis',(-0.638838828395272,0.0946722161246698,0.763493367900862));
#50719=DIRECTION('center_axis',(0.124207318409077,0.878565373677123,0.461189143659306));
#50720=DIRECTION('ref_axis',(-0.989321439880191,0.145372095405823,-0.0104901129977411));
#50721=DIRECTION('center_axis',(-0.338981956504719,0.885461953089255,-0.31788105133146));
#50722=DIRECTION('ref_axis',(-0.538110300831041,0.0946722161611699,0.837540730726965));
#50723=DIRECTION('center_axis',(0.181030233273647,0.87856537367578,0.441985224661216));
#50724=DIRECTION('ref_axis',(-0.982835104611445,0.145372095414437,0.113587459775392));
#50725=DIRECTION('center_axis',(-0.376150042596336,0.885461953092368,-0.272888759535135));
#50726=DIRECTION('ref_axis',(-0.428895452346745,0.0946722161297347,0.898379575930667));
#50727=DIRECTION('center_axis',(0.234998193217866,0.878565373674249,0.415810934638528));
#50728=DIRECTION('ref_axis',(-0.960848872633557,0.145372095452043,0.235873690399552));
#50729=DIRECTION('center_axis',(-0.407386017798389,0.885461953092885,-0.22359284900753));
#50730=DIRECTION('ref_axis',(-0.312916666377336,0.0946722161234403,0.945050438546838));
#50731=DIRECTION('center_axis',(0.28526009123465,0.878565373678539,0.383079057796023));
#50732=DIRECTION('ref_axis',(-0.923709479959308,0.145372095424003,0.354440052061472));
#50733=DIRECTION('center_axis',(-0.432197272133671,0.885461953092218,-0.170770745698229));
#50734=DIRECTION('ref_axis',(-0.192002997658825,0.0946722161312271,0.976817291197708));
#50735=DIRECTION('center_axis',(0.331023267286328,0.878565373670557,0.344305795336355));
#50736=DIRECTION('ref_axis',(-0.87200263694079,0.14537209544692,0.467416682451193));
#50737=DIRECTION('center_axis',(-0.450192517308106,0.885461953091926,-0.115255485710757));
#50738=DIRECTION('ref_axis',(-0.0680613269678815,0.0946722161341875,0.99317915164567));
#50739=DIRECTION('center_axis',(0.371566008567699,0.878565373679051,0.300102624862328));
#50740=DIRECTION('ref_axis',(-0.806543791482632,0.145372095393174,0.573021872446261));
#50741=DIRECTION('center_axis',(-0.46108795755314,0.885461953092287,-0.0579225778558486));
#50742=DIRECTION('ref_axis',(0.056953711510405,0.0946722161303211,0.993877983576537));
#50743=DIRECTION('center_axis',(0.406248931974331,0.878565373680964,0.251166656701371));
#50744=DIRECTION('ref_axis',(-0.728365268650857,0.14537209541337,0.669590165174408));
#50745=DIRECTION('center_axis',(-0.464711749675408,0.885461961242092,0.000323893391809522));
#50746=DIRECTION('ref_axis',(0.181070597688607,0.0946721347711845,0.978902766136942));
#50747=DIRECTION('center_axis',(0.434525067034736,0.878565373684967,0.19826964033924));
#50748=DIRECTION('ref_axis',(-0.638699990404053,0.145372095388073,0.755598621055083));
#50749=DIRECTION('center_axis',(-0.461006790844013,0.885461953090007,0.0585650785514288));
#50750=DIRECTION('ref_axis',(0.302331809512097,0.0946722161538305,0.94848966702103));
#50751=DIRECTION('center_axis',(0.455948482273978,0.878565373675013,0.142245793228975));
#50752=DIRECTION('ref_axis',(-0.538962031724008,0.145372095451307,0.829690835326042));
#50753=DIRECTION('center_axis',(-0.450031463932584,0.885461953090173,0.115882747207818));
#50754=DIRECTION('ref_axis',(0.418825109863107,0.0946722161522763,0.903118319400605));
#50755=DIRECTION('center_axis',(0.,1.,0.));
#50756=DIRECTION('ref_axis',(0.,0.,1.));
#50757=DIRECTION('',(8.65956056235503E-17,-0.707106781186539,0.707106781186556));
#50758=DIRECTION('center_axis',(0.,-1.,1.81818181817852E-12));
#50759=DIRECTION('ref_axis',(1.,0.,0.));
#50760=DIRECTION('center_axis',(-0.458818968797312,-0.87926072867782,-0.12800673762236));
#50761=DIRECTION('ref_axis',(0.477771165970434,-0.122671608382798,-0.869877226661343));
#50762=DIRECTION('center_axis',(-0.0510528487249554,0.705424652954679,0.70694389143753));
#50763=DIRECTION('ref_axis',(-0.993134147532106,-0.110462470651433,0.0385046436583641));
#50764=DIRECTION('center_axis',(-0.0747813385372569,0.160364694830346,0.984220969121541));
#50765=DIRECTION('ref_axis',(-0.00205849356672293,-0.987007291747137,0.160662281330179));
#50766=DIRECTION('center_axis',(-0.0897986376521124,-0.137109889430621,
0.986477107132318));
#50767=DIRECTION('ref_axis',(0.0344440051966361,-0.99031373067732,-0.134507714789833));
#50768=DIRECTION('center_axis',(0.473783675120008,-0.879260729005327,-0.0492909689375137));
#50769=DIRECTION('ref_axis',(-0.342664178411406,-0.132503133709511,-0.930066761254694));
#50770=DIRECTION('center_axis',(-0.43915754583858,-0.879260728678471,-0.184502631246384));
#50771=DIRECTION('ref_axis',(0.583028323247161,-0.122671608378535,-0.80313737977349));
#50772=DIRECTION('center_axis',(-0.139253845558219,0.705424652962835,0.694970809091656));
#50773=DIRECTION('ref_axis',(-0.990128899650558,-0.110462470602953,-0.0862716909830027));
#50774=DIRECTION('center_axis',(-0.197547261949399,0.160364694810999,0.967087505841364));
#50775=DIRECTION('ref_axis',(-0.0221785849573792,-0.987007291750282,0.159137413580408));
#50776=DIRECTION('center_axis',(-0.212728914248208,-0.137109889396287,0.967443686874082));
#50777=DIRECTION('ref_axis',(0.0510306907533597,-0.990313730682094,-0.129130102701686));
#50778=DIRECTION('center_axis',(0.476225545845609,-0.879260729009032,0.0104785450591571));
#50779=DIRECTION('ref_axis',(-0.22339389441128,-0.132503133683585,-0.965680116551952));
#50780=DIRECTION('center_axis',(-0.412570346035416,-0.879260728680131,-0.238088808164313));
#50781=DIRECTION('ref_axis',(0.679090775560755,-0.122671608348556,-0.723731576659102));
#50782=DIRECTION('center_axis',(-0.225258726217264,0.705424652951847,0.672037621916171));
#50783=DIRECTION('ref_axis',(-0.971508727523255,-0.110462470666646,-0.209687469631274));
#50784=DIRECTION('center_axis',(-0.317197747029055,0.160364694845115,0.934702494875736));
#50785=DIRECTION('ref_axis',(-0.0419489068256087,-0.987007291744729,0.15510285380634));
#50786=DIRECTION('center_axis',(-0.332304328785672,-0.137109889416642,0.933153101744007));
#50787=DIRECTION('ref_axis',(0.0668125918448412,-0.990313730679244,-0.121716031808188));
#50788=DIRECTION('center_axis',(0.471157055240052,-0.879260729008505,0.0700828061720898));
#50789=DIRECTION('ref_axis',(-0.100600555230665,-0.132503133686602,-0.986064119543203));
#50790=DIRECTION('center_axis',(-0.379476665467412,-0.879260728673145,-0.287920182305626));
#50791=DIRECTION('ref_axis',(0.764443560670196,-0.122671608391771,-0.632912094247257));
#50792=DIRECTION('center_axis',(-0.307711142019788,0.705424652963427,0.638506000025298));
#50793=DIRECTION('ref_axis',(-0.937567282419065,-0.110462470446083,-0.329796351647918));
#50794=DIRECTION('center_axis',(-0.431845834156375,0.160364694827406,0.887576667209486));
#50795=DIRECTION('ref_axis',(-0.0610576693612533,-0.987007291747613,0.148622229323928));
#50796=DIRECTION('center_axis',(-0.446639105538544,-0.137109889604953,0.88414613474032));
#50797=DIRECTION('ref_axis',(0.0815408184091089,-0.99031373065616,-0.112382426593533));
#50798=DIRECTION('center_axis',(0.458658136415686,-0.879260729004838,0.128581819591928));
#50799=DIRECTION('ref_axis',(0.0237793148120579,-0.132503133713074,-0.990897302319107));
#50800=DIRECTION('center_axis',(-0.34039841113939,-0.879260728676267,-0.333210883227814));
#50801=DIRECTION('ref_axis',(0.837740614229303,-0.12267160839414,-0.532111209959632));
#50802=DIRECTION('center_axis',(-0.385310769468071,0.705424652953116,0.594904757030819));
#50803=DIRECTION('ref_axis',(-0.888839841209568,-0.110462470660403,-0.444704148006457));
#50804=DIRECTION('center_axis',(-0.539683454506372,0.160364694818675,0.826453225287301));
#50805=DIRECTION('ref_axis',(-0.0792035159775513,-0.987007291749035,0.139797743511935));
#50806=DIRECTION('center_axis',(-0.553930116811,-0.137109889434077,0.821195655071998));
#50807=DIRECTION('ref_axis',(0.0949830976385117,-0.990313730676833,-0.101276482936196));
#50808=DIRECTION('center_axis',(0.43892590479466,-0.879260729009627,0.185053020839027));
#50809=DIRECTION('ref_axis',(0.147784170781883,-0.132503133701823,-0.980103442716894));
#50810=DIRECTION('center_axis',(-0.295951870544099,-0.879260728675819,-0.373246649455714));
#50811=DIRECTION('ref_axis',(0.897825997808071,-0.122671608373307,-0.42291861410802));
#50812=DIRECTION('center_axis',(-0.456833815793938,0.705424652957863,0.541921510688059));
#50813=DIRECTION('ref_axis',(-0.826094864746202,-0.110462470633544,-0.552598694371863));
#50814=DIRECTION('center_axis',(-0.639009944386313,0.160364694822305,0.752296122301551));
#50815=DIRECTION('ref_axis',(-0.0961002758384732,-0.987007291748441,0.128768563784709));
#50816=DIRECTION('center_axis',(-0.652485319215739,-0.137109889569417,0.745294429329911));
#50817=DIRECTION('ref_axis',(0.106927436622317,-0.990313730661046,-0.0885733490480162));
#50818=DIRECTION('center_axis',(0.412271549450918,-0.879260729009111,0.238605825443777));
#50819=DIRECTION('ref_axis',(0.269458382201844,-0.132503133682721,-0.953852766324774));
#50820=DIRECTION('center_axis',(-0.246837992119163,-0.879260728680677,-0.407396093067306));
#50821=DIRECTION('ref_axis',(0.943752129107433,-0.12267160836025,-0.307056338979503));
#50822=DIRECTION('center_axis',(-0.521152320027383,0.705424652950378,0.480391838336077));
#50823=DIRECTION('ref_axis',(-0.750321878732873,-0.11046247067845,-0.651778429273618));
#50824=DIRECTION('center_axis',(-0.728258865719209,0.160364694810991,0.666274860068687));
#50825=DIRECTION('ref_axis',(-0.11148147693236,-0.987007291750285,0.115708626872619));
#50826=DIRECTION('center_axis',(-0.740750438384919,-0.137109889435947,0.6576394652478));
#50827=DIRECTION('ref_axis',(0.117185466079654,-0.990313730676577,-0.0744733601574021));
#50828=DIRECTION('center_axis',(0.379115425475678,-0.879260729003382,0.288395673682593));
#50829=DIRECTION('ref_axis',(0.386883073940472,-0.132503133722346,-0.9125592619946));
#50830=DIRECTION('center_axis',(-0.193831331191601,-0.87926072867378,-0.435120656899377));
#50831=DIRECTION('ref_axis',(0.974794725525188,-0.122671608410494,-0.186351602027606));
#50832=DIRECTION('center_axis',(-0.577251940727125,0.705424652962881,0.411286099836799));
#50833=DIRECTION('ref_axis',(-0.662715868563518,-0.110462470601243,-0.74067922891274));
#50834=DIRECTION('center_axis',(-0.806022709697782,0.160364694810026,0.56974604527801));
#50835=DIRECTION('ref_axis',(-0.12510454854524,-0.987007291750441,0.100823895802292));
#50836=DIRECTION('center_axis',(-0.817333480602069,-0.137109889640004,0.559613133914683));
#50837=DIRECTION('ref_axis',(0.125595410813388,-0.990313730651293,-0.0591988823047837));
#50838=DIRECTION('center_axis',(0.339980424795607,-0.87926072900711,0.333637349800174));
#50839=DIRECTION('ref_axis',(0.498206388459968,-0.132503133697411,-0.856874152987498));
#50840=DIRECTION('center_axis',(-0.137767834283508,-0.879260728679782,-0.455983108062493));
#50841=DIRECTION('ref_axis',(0.990464226825965,-0.122671608346041,-0.062707988995335));
#50842=DIRECTION('center_axis',(-0.624247953590279,0.70542465295917,0.335694133752414));
#50843=DIRECTION('ref_axis',(-0.564658433181154,-0.110462470627397,-0.817899074715393));
#50844=DIRECTION('center_axis',(-0.87107509404991,0.160364694808483,0.464231995003493));
#50845=DIRECTION('ref_axis',(-0.136754646693211,-0.987007291750693,0.0843491116656059));
#50846=DIRECTION('center_axis',(-0.881026685627242,-0.137109889424586,0.452761369194254));
#50847=DIRECTION('ref_axis',(0.132024640697849,-0.990313730678156,-0.0429908022595161));
#50848=DIRECTION('center_axis',(0.295483729709509,-0.87926072900682,0.373617365634084));
#50849=DIRECTION('ref_axis',(0.601672690632676,-0.132503133698707,-0.787675626706107));
#50850=DIRECTION('center_axis',(-0.0795316564451785,-0.879260728670998,
-0.469654433216628));
#50851=DIRECTION('ref_axis',(0.990513515580251,-0.122671608429301,0.0619245665162102));
#50852=DIRECTION('center_axis',(-0.661399203311531,0.705424652954368,0.254808070639612));
#50853=DIRECTION('ref_axis',(-0.457695996992253,-0.110462470652642,-0.882220163516218));
#50854=DIRECTION('center_axis',(-0.922390103810698,0.160364694827014,0.351396728848077));
#50855=DIRECTION('ref_axis',(-0.146248042387767,-0.987007291747676,0.0665440916585738));
#50856=DIRECTION('center_axis',(-0.930825573503264,-0.137109889365752,0.338769287200641));
#50857=DIRECTION('ref_axis',(0.136371763177505,-0.990313730686301,-0.0261047317940428));
#50858=DIRECTION('center_axis',(0.246327079714757,-0.879260729010737,0.407705212400709));
#50859=DIRECTION('ref_axis',(0.695650255042948,-0.132503133672225,-0.70605498527078));
#50860=DIRECTION('center_axis',(-0.0200412167434643,-0.879260728679161,
-0.4759190273923));
#50861=DIRECTION('ref_axis',(0.974941814511513,-0.12267160834986,0.185580534598479));
#50862=DIRECTION('center_axis',(-0.688119792457086,0.705424652960527,0.169903532112602));
#50863=DIRECTION('ref_axis',(-0.343515421574124,-0.110462470618877,-0.932628113304293));
#50864=DIRECTION('center_axis',(-0.95915847062965,0.160364694817076,0.233019726365851));
#50865=DIRECTION('ref_axis',(-0.153435019064046,-0.987007291749297,0.0476896315621617));
#50866=DIRECTION('center_axis',(-0.965944786020493,-0.137109889429341,0.219434611172664));
#50867=DIRECTION('ref_axis',(0.138568221601756,-0.99031373067749,-0.00880697415449896));
#50868=DIRECTION('center_axis',(0.193285704483541,-0.8792607290072,0.435363304457355));
#50869=DIRECTION('ref_axis',(0.778656999385461,-0.132503133696502,-0.613299434916287));
#50870=DIRECTION('center_axis',(0.0397652848177643,-0.879260728674355,-0.474678094222183));
#50871=DIRECTION('ref_axis',(0.943994698616188,-0.122671608384915,0.306309786785845));
#50872=DIRECTION('center_axis',(-0.703988321455513,0.705424652950248,0.0823195132655206));
#50873=DIRECTION('ref_axis',(-0.223917402658416,-0.110462470676263,-0.968327960640817));
#50874=DIRECTION('center_axis',(-0.980800335390021,0.160364694827208,0.110967863599328));
#50875=DIRECTION('ref_axis',(-0.158202233851104,-0.987007291747647,0.0280830774933107));
#50876=DIRECTION('center_axis',(-0.985830472241187,-0.137109889443731,0.0966393202451538));
#50877=DIRECTION('ref_axis',(0.138579376349179,-0.990313730675486,0.00862967474895586));
#50878=DIRECTION('center_axis',(0.13719609829506,-0.879260729013987,0.456155457082784));
#50879=DIRECTION('ref_axis',(0.84938385766004,-0.132503133672304,-0.51087178617885));
#50880=DIRECTION('center_axis',(0.0989446641324139,-0.879260728675946,-0.465951203934456));
#50881=DIRECTION('ref_axis',(0.89816022240913,-0.122671608372746,0.422208350676802));
#50882=DIRECTION('center_axis',(-0.708754534050761,0.705424652952351,-0.00656273338962056));
#50883=DIRECTION('ref_axis',(-0.100788072609723,-0.110462470665894,-0.988756697572261));
#50884=DIRECTION('center_axis',(-0.986974392960287,0.160364694833053,-0.012834028665036));
#50885=DIRECTION('ref_axis',(-0.160474504900988,-0.987007291746699,0.00803363651342823));
#50886=DIRECTION('center_axis',(-0.990169023015502,-0.137109889404239,-0.0276800304928161));
#50887=DIRECTION('ref_axis',(0.136405051494663,-0.990313730680973,0.0259302285271826));
#50888=DIRECTION('center_axis',(0.0789428275537311,-0.879260729002341,0.469753765724228));
#50889=DIRECTION('ref_axis',(0.906715425170266,-0.132503133730031,-0.400387384054525));
#50890=DIRECTION('center_axis',(0.156563626958717,-0.879260728673591,-0.449875984829061));
#50891=DIRECTION('ref_axis',(0.838161222937335,-0.122671608411932,0.531448436683957));
#50892=DIRECTION('center_axis',(-0.702343264258627,0.70542465295162,-0.0953414818356713));
#50893=DIRECTION('ref_axis',(0.0239307455634354,-0.110462470668693,-0.993592150729134));
#50894=DIRECTION('center_axis',(-0.977583274769392,0.160364694802967,-0.136433520631487));
#50895=DIRECTION('ref_axis',(-0.160215997110056,-0.987007291751593,-0.0121424997103922));
#50896=DIRECTION('center_axis',(-0.978892016790465,-0.137109889424122,-0.151562850613205));
#50897=DIRECTION('ref_axis',(0.132079537552637,-0.990313730678209,0.0428218471120587));
#50898=DIRECTION('center_axis',(0.0194445813316385,-0.879260729000878,0.475943776819996));
#50899=DIRECTION('ref_axis',(0.949747548726854,-0.132503133762174,-0.283588633817605));
#50900=DIRECTION('center_axis',(0.211713487886367,-0.879260728674883,-0.426705952685338));
#50901=DIRECTION('ref_axis',(0.764943920330387,-0.122671608382308,0.632307263319406));
#50902=DIRECTION('center_axis',(-0.684855621636837,0.705424652958876,-0.182616638098152));
#50903=DIRECTION('ref_axis',(0.14827216179308,-0.110462470380521,-0.982758062126503));
#50904=DIRECTION('center_axis',(-0.952775084346285,0.160364694830759,-0.257881374474325));
#50905=DIRECTION('ref_axis',(-0.15743078739333,-0.987007291747074,-0.0321271414667282));
#50906=DIRECTION('center_axis',(-0.952177298702754,-0.137109889415165,-0.273055434041677));
#50907=DIRECTION('ref_axis',(0.125671050374487,-0.990313730679455,0.059038139583782));
#50908=DIRECTION('center_axis',(-0.0403603174395375,-0.879260729014459,
0.474627870219545));
#50909=DIRECTION('ref_axis',(0.977801586111893,-0.132503133669077,-0.162317521435431));
#50910=DIRECTION('center_axis',(0.263524500644688,-0.879260728677615,-0.396806512755622));
#50911=DIRECTION('ref_axis',(0.679662995120437,-0.12267160836076,0.723194226723431));
#50912=DIRECTION('center_axis',(-0.65656739675031,0.705424652959475,-0.267011820939683));
#50913=DIRECTION('ref_axis',(0.270275237180936,-0.110462470438146,-0.956425291798314));
#50914=DIRECTION('center_axis',(-0.912941061687989,0.160364694825961,-0.375262284991956));
#50915=DIRECTION('ref_axis',(-0.152162800082905,-0.98700729174785,-0.0516051190048394));
#50916=DIRECTION('center_axis',(-0.910446175781508,-0.137109889642671,-0.390241770146408));
#50917=DIRECTION('ref_axis',(0.117280655931353,-0.990313730650938,0.0743233652933744));
#50918=DIRECTION('center_axis',(-0.099528710080768,-0.879260729003441,0.465826798608664));
#50919=DIRECTION('ref_axis',(0.990435108372055,-0.132503133721845,-0.038486564641797));
#50920=DIRECTION('center_axis',(0.311179574584837,-0.879260728676818,-0.360649197098664));
#50921=DIRECTION('ref_axis',(0.583663378466932,-0.122671608369214,0.802675985150096));
#50922=DIRECTION('center_axis',(-0.61792471178816,0.705424652955238,-0.347196067898963));
#50923=DIRECTION('ref_axis',(0.388015910533207,-0.110462470648107,-0.915009123315939));
#50924=DIRECTION('center_axis',(-0.858709413119038,0.160364694843852,-0.48672508510287));
#50925=DIRECTION('ref_axis',(-0.144495114537597,-0.987007291744945,-0.0702692529992742));
#50926=DIRECTION('center_axis',(-0.85435677284678,-0.137109889450976,-0.501273760439918));
#50927=DIRECTION('ref_axis',(0.107040674993316,-0.990313730674492,0.0884364672210806));
#50928=DIRECTION('center_axis',(-0.157127475408515,-0.879260729005603,0.449679360100375));
#50929=DIRECTION('ref_axis',(0.98744887731259,-0.132503133730221,0.0859513481323921));
#50930=DIRECTION('center_axis',(0.353927160734071,-0.879260728672657,-0.318804228185179));
#50931=DIRECTION('ref_axis',(0.478459041683958,-0.122671608397634,0.869499063785583));
#50932=DIRECTION('center_axis',(-0.569536984911877,0.705424652934478,-0.421904825582453));
#50933=DIRECTION('ref_axis',(0.499637341450765,-0.110462470774635,-0.859162714262191));
#50934=DIRECTION('center_axis',(-0.790935404138116,0.160364694856304,-0.590511939866181));
#50935=DIRECTION('ref_axis',(-0.134548654712423,-0.98700729174292,-0.0878251988974902));
#50936=DIRECTION('center_axis',(-0.784793653210681,-0.137109889462256,-0.604400364073253));
#50937=DIRECTION('ref_axis',(0.0951125989073771,-0.990313730672959,0.10115487318805));
#50938=DIRECTION('center_axis',(-0.212248246590896,-0.879260729007012,0.426440209461007));
#50939=DIRECTION('ref_axis',(0.96888998759003,-0.132503133720377,0.209033756848198));
#50940=DIRECTION('center_axis',(0.39109310415168,-0.879260728672932,-0.271931526121096));
#50941=DIRECTION('ref_axis',(0.365709119989659,-0.122671608393851,0.922609622782277));
#50942=DIRECTION('center_axis',(-0.512167319731713,0.705424652954773,-0.489959891830414));
#50943=DIRECTION('ref_axis',(0.60337919282722,-0.110462470649097,-0.789766796112162));
#50944=DIRECTION('center_axis',(-0.710687871354221,0.160364694851882,-0.684986068584661));
#50945=DIRECTION('ref_axis',(-0.122480282212692,-0.98700729174364,-0.103996088935997));
#50946=DIRECTION('center_axis',(-0.702853868861137,-0.137109889358614,-0.697995212925562));
#50947=DIRECTION('ref_axis',(0.0816845402343855,-0.990313730687279,0.112278006301063));
#50948=DIRECTION('center_axis',(-0.264021736139023,-0.879260729007782,0.396475841976331));
#50949=DIRECTION('ref_axis',(0.935051123976042,-0.132503133714817,0.328819578350948));
#50950=DIRECTION('center_axis',(0.422091275700155,-0.879260728678951,-0.220770301401197));
#50951=DIRECTION('ref_axis',(0.247191746984302,-0.122671608351982,0.961170076899602));
#50952=DIRECTION('center_axis',(-0.44672046979781,0.7054246529415,-0.550287998130059));
#50953=DIRECTION('ref_axis',(0.697605394040524,-0.110462470732661,-0.707915783667239));
#50954=DIRECTION('center_axis',(-0.619232366294704,0.160364694847693,-0.768657557810673));
#50955=DIRECTION('ref_axis',(-0.108480322497183,-0.987007291744323,-0.118526898527059));
#50956=DIRECTION('center_axis',(-0.609829659120054,-0.13710988941858,-0.780582260291088));
#50957=DIRECTION('ref_axis',(0.0669682676856494,-0.990313730678976,0.121630448292651));
#50958=DIRECTION('center_axis',(-0.311631445195416,-0.879260729007769,0.360258813618964));
#50959=DIRECTION('ref_axis',(0.886465945546352,-0.132503133692648,0.443419718718327));
#50960=DIRECTION('center_axis',(0.446432815664272,-0.879260728674888,-0.16612739722326));
#50961=DIRECTION('ref_axis',(0.124776012454926,-0.122671608403339,0.984572304712857));
#50962=DIRECTION('center_axis',(-0.374228571398007,0.70542465296098,-0.601937733776748));
#50963=DIRECTION('ref_axis',(0.780829941339811,-0.110462470613005,-0.614900516582429));
#50964=DIRECTION('center_axis',(-0.518011196904828,0.160364694872858,-0.840206858172178));
#50965=DIRECTION('ref_axis',(-0.0927695633096054,-0.987007291740231,-0.131188468147773));
#50966=DIRECTION('center_axis',(-0.50718807135462,-0.137109889581385,-0.850859059101189));
#50967=DIRECTION('ref_axis',(0.0511958657084904,-0.990313730659423,0.129064705484394));
#50968=DIRECTION('center_axis',(-0.354326540197732,-0.879260729008234,0.318360288565352));
#50969=DIRECTION('ref_axis',(0.82390066964127,-0.132503133711363,0.551026865153901));
#50970=DIRECTION('center_axis',(0.463733843447336,-0.87926072867611,-0.10886456471009));
#50971=DIRECTION('ref_axis',(0.000392485695471339,-0.122671608394846,0.99244723912599));
#50972=DIRECTION('center_axis',(-0.295834864707477,0.705424652953782,-0.644094551932048));
#50973=DIRECTION('ref_axis',(0.851740334110555,-0.110462470655033,-0.512187900897733));
#50974=DIRECTION('center_axis',(-0.408620681497454,0.160364694865246,-0.898505594469691));
#50975=DIRECTION('ref_axis',(-0.0755957726710143,-0.987007291741473,-0.14178111723158));
#50976=DIRECTION('center_axis',(-0.396547824745071,-0.137109889425071,-0.907717302309369));
#50977=DIRECTION('ref_axis',(0.034616073952146,-0.990313730678103,0.134463535036669));
#50978=DIRECTION('center_axis',(-0.391433693969208,-0.879260729013596,0.271441031607419));
#50979=DIRECTION('ref_axis',(0.748341987973332,-0.132503133651729,0.649943988824109));
#50980=DIRECTION('center_axis',(0.473721511152887,-0.879260729012473,-0.0498848703263812));
#50981=DIRECTION('ref_axis',(-0.123997232081177,-0.122671606019574,0.98467068785091));
#50982=DIRECTION('center_axis',(-0.21277567187849,0.705424653817806,-0.676093611301486));
#50983=DIRECTION('ref_axis',(0.909218271556588,-0.110462465555327,-0.401397780725167));
#50984=DIRECTION('center_axis',(-0.292785973845394,0.160364694840491,-0.94263436080387));
#50985=DIRECTION('ref_axis',(-0.0572297915357268,-0.987007291745495,-0.150137793383277));
#50986=DIRECTION('center_axis',(-0.279653782043359,-0.137109889431314,-0.950260301395875));
#50987=DIRECTION('ref_axis',(0.0174903662277315,-0.990313730677212,0.137741794388638));
#50988=DIRECTION('center_axis',(-0.422367704644081,-0.879260729003134,0.220240987344697));
#50989=DIRECTION('ref_axis',(0.660981506120526,-0.132503133747519,0.738611107494145));
#50990=DIRECTION('center_axis',(0.476238308330351,-0.879260728672218,0.00988153295016984));
#50991=DIRECTION('ref_axis',(-0.246431436826979,-0.122671608401111,0.961365291362069));
#50992=DIRECTION('center_axis',(-0.126360866737994,0.705424652922653,-0.697430276376197));
#50993=DIRECTION('ref_axis',(0.95235729655815,-0.110462470915775,-0.284277368447847));
#50994=DIRECTION('center_axis',(-0.172333856482792,0.160364694839762,-0.971897220162049));
#50995=DIRECTION('ref_axis',(-0.0379612624110037,-0.987007291745612,-0.156126706867071));
#50996=DIRECTION('center_axis',(-0.158349432088054,-0.137109891155577,-0.977817127639262));
#50997=DIRECTION('ref_axis',(8.88252939813159E-5,-0.990313730439543,0.138847785048893));
#50998=DIRECTION('center_axis',(-0.446640724223604,-0.879260729008031,0.165567611232637));
#50999=DIRECTION('ref_axis',(0.563196951084305,-0.13250313371093,0.815629887783746));
#51000=DIRECTION('center_axis',(0.471244542523149,-0.879260728680165,0.0694921012991661));
#51001=DIRECTION('ref_axis',(-0.364979272010298,-0.122671608366607,0.922898590043122));
#51002=DIRECTION('center_axis',(-0.0379532822265761,0.705424652970262,-0.707768046290602));
#51003=DIRECTION('ref_axis',(0.9804770766421,-0.110462470559006,-0.162673737208444));
#51004=DIRECTION('center_axis',(-0.0491639312551466,0.160364694821936,-0.985832679777967));
#51005=DIRECTION('ref_axis',(-0.0180940614984255,-0.987007291748523,-0.159653408901083));
#51006=DIRECTION('center_axis',(-0.0345478170780039,-0.137109891131492,
-0.989953193888002));
#51007=DIRECTION('ref_axis',(-0.0173141169948037,-0.990313730442863,0.137764061529232));
#51008=DIRECTION('center_axis',(-0.463852070615388,-0.879265855918343,0.10831810191284));
#51009=DIRECTION('ref_axis',(0.440180830784498,-0.122636854730908,0.889494821835169));
#51010=DIRECTION('center_axis',(0.458818968799936,-0.879260728677175,0.128006737617385));
#51011=DIRECTION('ref_axis',(-0.477771165967333,-0.122671608387466,0.869877226662388));
#51012=DIRECTION('center_axis',(0.0510528487577276,0.705424652951044,-0.70694389143879));
#51013=DIRECTION('ref_axis',(0.993134147530435,-0.110462470674624,-0.0385046436349503));
#51014=DIRECTION('center_axis',(0.0747813385357381,0.16036469488283,-0.984220969113105));
#51015=DIRECTION('ref_axis',(0.0020584935708628,-0.987007291738614,-0.160662281382488));
#51016=DIRECTION('center_axis',(0.0897986376532112,-0.137109889370473,-0.986477107140578));
#51017=DIRECTION('ref_axis',(-0.0344440051901882,-0.990313730685666,0.134507714730033));
#51018=DIRECTION('center_axis',(-0.473783675110741,-0.879260729008865,0.0492909689634806));
#51019=DIRECTION('ref_axis',(0.342664178424753,-0.132503133685172,0.930066761253244));
#51020=DIRECTION('center_axis',(0.439157545850119,-0.879260728675988,0.184502631230756));
#51021=DIRECTION('ref_axis',(-0.583028323238382,-0.122671608395633,0.803137379777252));
#51022=DIRECTION('center_axis',(0.139253845616515,0.705424652955838,-0.694970809087078));
#51023=DIRECTION('ref_axis',(0.990128899642354,-0.110462470644664,0.0862716910237555));
#51024=DIRECTION('center_axis',(0.197547261947256,0.16036469485379,-0.967087505834706));
#51025=DIRECTION('ref_axis',(0.0221785849666862,-0.987007291743339,-0.159137413622173));
#51026=DIRECTION('center_axis',(0.212728914246855,-0.137109889420509,-0.967443686870947));
#51027=DIRECTION('ref_axis',(-0.0510306907593974,-0.990313730678721,0.129130102725165));
#51028=DIRECTION('center_axis',(-0.47622554584437,-0.87926072900977,-0.0104785450535443));
#51029=DIRECTION('ref_axis',(0.223393894456238,-0.132503133701192,0.965680116539136));
#51030=DIRECTION('center_axis',(0.412570346078638,-0.879260728672076,0.23808880811916));
#51031=DIRECTION('ref_axis',(-0.679090775549037,-0.122671608414792,0.723731576658871));
#51032=DIRECTION('center_axis',(0.225258726238494,0.705424652949409,-0.672037621911614));
#51033=DIRECTION('ref_axis',(0.971508727518402,-0.110462470682718,0.209687469645291));
#51034=DIRECTION('center_axis',(0.317197747027847,0.160364694860719,-0.934702494873469));
#51035=DIRECTION('ref_axis',(0.0419489068324215,-0.987007291742214,-0.155102853820504));
#51036=DIRECTION('center_axis',(0.332304328786436,-0.137109889415776,-0.933153101743862));
#51037=DIRECTION('ref_axis',(-0.0668125918447864,-0.990313730679361,0.121716031807269));
#51038=DIRECTION('center_axis',(-0.471157055239204,-0.879260729009568,-0.0700828061644564));
#51039=DIRECTION('ref_axis',(0.10060055527342,-0.132503133700201,0.986064119537014));
#51040=DIRECTION('center_axis',(0.379476665444939,-0.879260728676914,0.287920182323735));
#51041=DIRECTION('ref_axis',(-0.764443560681583,-0.122671608366485,0.632912094238404));
#51042=DIRECTION('center_axis',(0.307711142173716,0.705424652944235,-0.63850599997232));
#51043=DIRECTION('ref_axis',(0.93756728240383,-0.110462470713733,0.329796351601583));
#51044=DIRECTION('center_axis',(0.431845834156531,0.160364694815792,-0.887576667211508));
#51045=DIRECTION('ref_axis',(0.0610576693579444,-0.987007291749521,-0.148622229312618));
#51046=DIRECTION('center_axis',(0.446639105450297,-0.137109891249355,-0.884146134529891));
#51047=DIRECTION('ref_axis',(-0.0815408191148127,-0.990313730429522,0.112382428078637));
#51048=DIRECTION('center_axis',(-0.458658136415822,-0.879260729004999,-0.128581819590344));
#51049=DIRECTION('ref_axis',(-0.0237793147674236,-0.132503133734286,0.990897302317342));
#51050=DIRECTION('center_axis',(0.340398408902727,-0.879260729007449,0.333210884638814));
#51051=DIRECTION('ref_axis',(-0.83774061513981,-0.122671606054293,0.53211120906558));
#51052=DIRECTION('center_axis',(0.385310763021079,0.705424653838188,-0.59490476015694));
#51053=DIRECTION('ref_axis',(0.888839843993657,-0.110462465576322,0.444704143704701));
#51054=DIRECTION('center_axis',(0.539683454502762,0.160364694851086,-0.826453225283369));
#51055=DIRECTION('ref_axis',(0.0792035159962911,-0.987007291743783,-0.139797743538397));
#51056=DIRECTION('center_axis',(0.553930116811889,-0.137109889420056,-0.821195655073739));
#51057=DIRECTION('ref_axis',(-0.0949830976305822,-0.990313730678775,0.101276482924643));
#51058=DIRECTION('center_axis',(-0.43892590478839,-0.879260729004544,-0.185053020878046));
#51059=DIRECTION('ref_axis',(-0.147784170842995,-0.132503133714334,0.980103442705988));
#51060=DIRECTION('center_axis',(0.2959518705077,-0.879260728681021,0.373246649472321));
#51061=DIRECTION('ref_axis',(-0.897825997836381,-0.122671608360944,0.422918614051506));
#51062=DIRECTION('center_axis',(0.45683381573245,0.70542465296641,-0.541921510728767));
#51063=DIRECTION('ref_axis',(0.826094864780288,-0.110462470581545,0.552598694331301));
#51064=DIRECTION('center_axis',(0.639009944383963,0.160364694842497,-0.752296122299243));
#51065=DIRECTION('ref_axis',(0.0961002758532159,-0.987007291745183,-0.128768563798679));
#51066=DIRECTION('center_axis',(0.652485319230149,-0.137109889417251,-0.745294429345289));
#51067=DIRECTION('ref_axis',(-0.106927436623215,-0.990313730679154,0.088573348844475));
#51068=DIRECTION('center_axis',(-0.412271549460581,-0.879260729013579,-0.238605825410616));
#51069=DIRECTION('ref_axis',(-0.269458382143699,-0.132503133675119,0.953852766342256));
#51070=DIRECTION('center_axis',(0.246837992152326,-0.87926072867621,0.407396093056855));
#51071=DIRECTION('ref_axis',(-0.943752129089521,-0.122671608371701,0.307056339029983));
#51072=DIRECTION('center_axis',(0.521152319951747,0.705424652961949,-0.480391838401139));
#51073=DIRECTION('ref_axis',(0.750321878785262,-0.110462470607681,0.651778429225302));
#51074=DIRECTION('center_axis',(0.728258865710466,0.160364694878353,-0.66627486006203));
#51075=DIRECTION('ref_axis',(0.111481476982423,-0.987007291739349,-0.115708626917674));
#51076=DIRECTION('center_axis',(0.740750438389486,-0.137109889397372,-0.657639465250699));
#51077=DIRECTION('ref_axis',(-0.117185466050305,-0.990313730681934,0.074473360132347));
#51078=DIRECTION('center_axis',(-0.379115425491949,-0.879260729008477,-0.288395673645669));
#51079=DIRECTION('ref_axis',(-0.386883073924451,-0.132503133686919,0.912559262006536));
#51080=DIRECTION('center_axis',(0.19383133116877,-0.879260728676786,0.435120656903474));
#51081=DIRECTION('ref_axis',(-0.974794725529707,-0.12267160838987,0.186351602017545));
#51082=DIRECTION('center_axis',(0.57725194078524,0.705424652952856,-0.41128609977243));
#51083=DIRECTION('ref_axis',(0.66271586851335,-0.110462470663156,0.740679228948394));
#51084=DIRECTION('center_axis',(0.806022709691879,0.160364694850647,-0.569746045274927));
#51085=DIRECTION('ref_axis',(0.125104548578956,-0.987007291743853,-0.100823895824952));
#51086=DIRECTION('center_axis',(0.817333480632928,-0.137109889377541,-0.559613133933918));
#51087=DIRECTION('ref_axis',(-0.125595410672812,-0.990313730684659,0.0591988820448487));
#51088=DIRECTION('center_axis',(-0.339980424780122,-0.879260729003266,-0.333637349826085));
#51089=DIRECTION('ref_axis',(-0.498206388471336,-0.132503133723577,0.856874152976842));
#51090=DIRECTION('center_axis',(0.137767834334762,-0.87926072867318,0.455983108059737));
#51091=DIRECTION('ref_axis',(-0.990464226818836,-0.122671608391281,0.0627079890194332));
#51092=DIRECTION('center_axis',(0.624247953561087,0.705424652964862,-0.335694133794737));
#51093=DIRECTION('ref_axis',(0.564658433212921,-0.110462470590227,0.817899074698481));
#51094=DIRECTION('center_axis',(0.871075094041514,0.160364694862904,-0.464231995000448));
#51095=DIRECTION('ref_axis',(0.136754646741252,-0.987007291741855,-0.0843491116911401));
#51096=DIRECTION('center_axis',(0.881026685614934,-0.137109889525777,-0.452761369187559));
#51097=DIRECTION('ref_axis',(-0.132024640726991,-0.990313730667086,0.0429908024250133));
#51098=DIRECTION('center_axis',(-0.295483729705123,-0.879260729005976,-0.37361736563954));
#51099=DIRECTION('ref_axis',(-0.601672690597617,-0.132503133727805,0.787675626727992));
#51100=DIRECTION('center_axis',(0.0795316564089272,-0.879260728675799,0.469654433213779));
#51101=DIRECTION('ref_axis',(-0.990513515588166,-0.122671608376523,-0.0619245664941464));
#51102=DIRECTION('center_axis',(0.661399203298246,0.70542465295776,-0.254808070664704));
#51103=DIRECTION('ref_axis',(0.457695997011179,-0.110462470632492,0.882220163508922));
#51104=DIRECTION('center_axis',(0.922390103807476,0.160364694846821,-0.351396728847495));
#51105=DIRECTION('ref_axis',(0.146248042406897,-0.987007291744476,-0.066544091663986));
#51106=DIRECTION('center_axis',(0.930825573497249,-0.137109889410855,-0.338769287198916));
#51107=DIRECTION('ref_axis',(-0.13637176322006,-0.990313730680047,0.0261047318089868));
#51108=DIRECTION('center_axis',(-0.246327079694008,-0.87926072900698,-0.407705212421348));
#51109=DIRECTION('ref_axis',(-0.695650255050645,-0.132503133697876,0.706054985258383));
#51110=DIRECTION('center_axis',(0.020041216796702,-0.879260728672416,0.475919027402519));
#51111=DIRECTION('ref_axis',(-0.974941814499448,-0.122671608420682,-0.185580534615046));
#51112=DIRECTION('center_axis',(0.68811979247493,0.705424652954293,-0.169903532066213));
#51113=DIRECTION('ref_axis',(0.343515421538055,-0.110462470652446,0.932628113313603));
#51114=DIRECTION('center_axis',(0.959158470620454,0.160364694873863,-0.233019726364624));
#51115=DIRECTION('ref_axis',(0.153435019119225,-0.987007291740073,-0.0476896315755246));
#51116=DIRECTION('center_axis',(0.965944786002725,-0.137109889560608,-0.219434611168856));
#51117=DIRECTION('ref_axis',(-0.138568221700355,-0.990313730662269,0.00880697431474339));
#51118=DIRECTION('center_axis',(-0.193285704507149,-0.879260729010939,-0.435363304439324));
#51119=DIRECTION('ref_axis',(-0.778656999349661,-0.132503133693184,0.613299434962456));
#51120=DIRECTION('center_axis',(-0.039765284845021,-0.879260728678037,0.47467809421308));
#51121=DIRECTION('ref_axis',(-0.943994698599503,-0.12267160838127,-0.306309786838725));
#51122=DIRECTION('center_axis',(0.703988321442307,0.705424652957028,-0.0823195133203546));
#51123=DIRECTION('ref_axis',(0.223917402698939,-0.110462470636748,0.968327960635954));
#51124=DIRECTION('center_axis',(0.980800335382066,0.160364694875923,-0.110967863599237));
#51125=DIRECTION('ref_axis',(0.1582022338996,-0.987007291739743,-0.0280830774979129));
#51126=DIRECTION('center_axis',(0.985830472224448,-0.137109889565211,-0.0966393202435602));
#51127=DIRECTION('ref_axis',(-0.138579376457204,-0.990313730661652,-0.0086296746018274));
#51128=DIRECTION('center_axis',(-0.137196098265259,-0.879260729009514,-0.45615545710037));
#51129=DIRECTION('ref_axis',(-0.849383857664955,-0.132503133702865,0.510871786162751));
#51130=DIRECTION('center_axis',(-0.0989446641002374,-0.879260728671348,
0.465951203949965));
#51131=DIRECTION('ref_axis',(-0.898160222391755,-0.122671608426907,-0.422208350698027));
#51132=DIRECTION('center_axis',(0.708754534051182,0.705424652951909,0.00656273339169857));
#51133=DIRECTION('ref_axis',(0.10078807260931,-0.110462470668518,0.98875669757201));
#51134=DIRECTION('center_axis',(0.986974392953023,0.160364694877827,0.0128340286641733));
#51135=DIRECTION('ref_axis',(0.160474504945745,-0.987007291739428,-0.00803363651259044));
#51136=DIRECTION('center_axis',(0.990169023015283,-0.137109889405871,0.027680030492564));
#51137=DIRECTION('ref_axis',(-0.136405051496291,-0.99031373068074,-0.0259302285275058));
#51138=DIRECTION('center_axis',(-0.0789428275667312,-0.87926072900407,-0.469753765718808));
#51139=DIRECTION('ref_axis',(-0.906715425169113,-0.132503133717594,0.400387384061252));
#51140=DIRECTION('center_axis',(-0.156563626986478,-0.879260728677805,0.449875984811163));
#51141=DIRECTION('ref_axis',(-0.838161222932035,-0.122671608382732,-0.531448436699056));
#51142=DIRECTION('center_axis',(0.70234326425919,0.705424652958555,0.0953414817802181));
#51143=DIRECTION('ref_axis',(-0.0239307455239352,-0.110462470629527,0.99359215073444));
#51144=DIRECTION('center_axis',(0.977583274764738,0.160364694832406,0.136433520630231));
#51145=DIRECTION('ref_axis',(0.160215997139136,-0.987007291746816,0.0121424997149576));
#51146=DIRECTION('center_axis',(0.978892016791562,-0.137109889415534,0.151562850613888));
#51147=DIRECTION('ref_axis',(-0.132079537544142,-0.9903137306794,-0.0428218471107381));
#51148=DIRECTION('center_axis',(-0.0194445814035528,-0.87926072901053,-0.475943776799227));
#51149=DIRECTION('ref_axis',(-0.949747548733399,-0.132503133684082,0.283588633832173));
#51150=DIRECTION('center_axis',(-0.211713487892645,-0.879260728675838,0.426705952680256));
#51151=DIRECTION('ref_axis',(-0.764943920330541,-0.122671608373738,-0.632307263320882));
#51152=DIRECTION('center_axis',(0.68485562163539,0.705424652957529,0.182616638108781));
#51153=DIRECTION('ref_axis',(-0.148272161548486,-0.110462470635442,0.982758062134752));
#51154=DIRECTION('center_axis',(0.952775084340861,0.160364694866168,0.257881374472347));
#51155=DIRECTION('ref_axis',(0.157430787427507,-0.987007291741322,0.0321271414759624));
#51156=DIRECTION('center_axis',(0.952177298703104,-0.137109889411569,0.27305543404226));
#51157=DIRECTION('ref_axis',(-0.125671050370933,-0.990313730679946,-0.0590381395830944));
#51158=DIRECTION('center_axis',(0.0403603174543297,-0.879260729012547,-0.47462787022183));
#51159=DIRECTION('ref_axis',(-0.977801586111239,-0.132503133682443,0.162317521428458));
#51160=DIRECTION('center_axis',(-0.263524500637211,-0.879260728676324,0.396806512763449));
#51161=DIRECTION('ref_axis',(-0.679662995110619,-0.122671608378878,-0.723194226729585));
#51162=DIRECTION('center_axis',(0.656567396744409,0.705424652956745,0.267011820961406));
#51163=DIRECTION('ref_axis',(-0.270275237259081,-0.110462470391246,0.956425291781648));
#51164=DIRECTION('center_axis',(0.912941061682396,0.160364694864044,0.375262284989289));
#51165=DIRECTION('ref_axis',(0.152162800118094,-0.987007291741665,0.0516051190193879));
#51166=DIRECTION('center_axis',(0.910446175811195,-0.137109889406173,0.390241770160241));
#51167=DIRECTION('ref_axis',(-0.117280655660036,-0.990313730680689,-0.0743233653251029));
#51168=DIRECTION('center_axis',(0.0995287100521309,-0.879260729007236,-0.465826798607619));
#51169=DIRECTION('ref_axis',(-0.990435108370254,-0.132503133718826,0.0384865646985363));
#51170=DIRECTION('center_axis',(-0.311179574561562,-0.87926072867168,0.360649197131272));
#51171=DIRECTION('ref_axis',(-0.583663378483035,-0.122671608402557,-0.802675985133291));
#51172=DIRECTION('center_axis',(0.617924711791022,0.705424652956328,0.347196067891656));
#51173=DIRECTION('ref_axis',(-0.38801591053027,-0.110462470640521,0.9150091233181));
#51174=DIRECTION('center_axis',(0.858709413117082,0.160364694858558,0.486725085101475));
#51175=DIRECTION('ref_axis',(0.144495114550315,-0.987007291742558,0.0702692530066537));
#51176=DIRECTION('center_axis',(0.854356772853503,-0.137109889390124,0.501273760445104));
#51177=DIRECTION('ref_axis',(-0.107040674940543,-0.990313730682904,-0.0884364671907566));
#51178=DIRECTION('center_axis',(0.157127475379704,-0.87926072900933,-0.449679360103155));
#51179=DIRECTION('ref_axis',(-0.987448877316381,-0.13250313368182,-0.0859513481634601));
#51180=DIRECTION('center_axis',(-0.353927160753815,-0.87926072867792,0.318804228148744));
#51181=DIRECTION('ref_axis',(-0.478459041636315,-0.122671608379725,-0.869499063814327));
#51182=DIRECTION('center_axis',(0.569536985000032,0.705424652955541,0.421904825428232));
#51183=DIRECTION('ref_axis',(-0.499637341350622,-0.110462470646596,0.85916271433689));
#51184=DIRECTION('center_axis',(0.790935404140268,0.160364694840428,0.59051193986761));
#51185=DIRECTION('ref_axis',(0.134548654699449,-0.987007291745503,0.0878251988883308));
#51186=DIRECTION('center_axis',(0.784793653213853,-0.13710988942998,0.604400364076457));
#51187=DIRECTION('ref_axis',(-0.095112598881028,-0.9903137306774,-0.101154873169351));
#51188=DIRECTION('center_axis',(0.212248246609885,-0.879260729004504,-0.426440209456727));
#51189=DIRECTION('ref_axis',(-0.968889987585865,-0.132503133737634,-0.209033756856564));
#51190=DIRECTION('center_axis',(-0.391093104159856,-0.879260728675769,0.271931526100164));
#51191=DIRECTION('ref_axis',(-0.365709119951303,-0.122671608390012,-0.922609622797991));
#51192=DIRECTION('center_axis',(0.512167319772571,0.705424652962821,0.489959891776117));
#51193=DIRECTION('ref_axis',(-0.603379192791661,-0.110462470601419,0.789766796145998));
#51194=DIRECTION('center_axis',(0.710687871353904,0.160364694855864,0.684986068584057));
#51195=DIRECTION('ref_axis',(0.122480282215561,-0.987007291742994,0.103996088938754));
#51196=DIRECTION('center_axis',(0.70285386885858,-0.137109889388095,0.697995212922345));
#51197=DIRECTION('ref_axis',(-0.0816845402554354,-0.990313730683201,-0.11227800632171));
#51198=DIRECTION('center_axis',(0.264021736112348,-0.879260729011344,-0.396475841986194));
#51199=DIRECTION('ref_axis',(-0.93505112398369,-0.132503133689779,-0.328819578339287));
#51200=DIRECTION('center_axis',(-0.422091275691081,-0.879260728674362,0.220770301436824));
#51201=DIRECTION('ref_axis',(-0.247191747000703,-0.122671608384156,-0.961170076891278));
#51202=DIRECTION('center_axis',(0.446720469914802,0.705424652961171,0.55028799800987));
#51203=DIRECTION('ref_axis',(-0.697605393966077,-0.110462470612296,0.707915783759383));
#51204=DIRECTION('center_axis',(0.619232366294981,0.160364694844356,0.768657557811146));
#51205=DIRECTION('ref_axis',(0.108480322495231,-0.987007291744863,0.118526898524347));
#51206=DIRECTION('center_axis',(0.609829659124712,-0.137109889358621,0.780582260297981));
#51207=DIRECTION('ref_axis',(-0.0669682676488701,-0.990313730687279,-0.1216304482453));
#51208=DIRECTION('center_axis',(0.31163144517232,-0.879260729011096,-0.360258813630823));
#51209=DIRECTION('ref_axis',(-0.88646594556642,-0.132503133685564,-0.443419718680325));
#51210=DIRECTION('center_axis',(-0.446432815665649,-0.879260728676026,0.166127397213536));
#51211=DIRECTION('ref_axis',(-0.124776012493544,-0.122671608372295,-0.98457230471183));
#51212=DIRECTION('center_axis',(0.374228571297439,0.705424652945905,0.601937733856939));
#51213=DIRECTION('ref_axis',(-0.780829941387608,-0.110462470705292,0.614900516505156));
#51214=DIRECTION('center_axis',(0.518011196907874,0.160364694830562,0.840206858178373));
#51215=DIRECTION('ref_axis',(0.0927695632868828,-0.987007291747108,0.131188468112105));
#51216=DIRECTION('center_axis',(0.507188071362947,-0.137109889457119,0.85085905911625));
#51217=DIRECTION('ref_axis',(-0.0511958655288825,-0.990313730673669,-0.129064705446333));
#51218=DIRECTION('center_axis',(0.354326540219259,-0.879260729004894,-0.318360288550618));
#51219=DIRECTION('ref_axis',(-0.823900669610395,-0.132503133712186,-0.551026865199868));
#51220=DIRECTION('center_axis',(-0.463733843447264,-0.879260728676205,0.10886456470963));
#51221=DIRECTION('ref_axis',(-0.000392485740395515,-0.122671608370983,-0.992447239128922));
#51222=DIRECTION('center_axis',(0.295834864657644,0.705424652947218,0.644094551962125));
#51223=DIRECTION('ref_axis',(-0.851740334128267,-0.110462470695732,0.512187900859501));
#51224=DIRECTION('center_axis',(0.408620681499501,0.160364694829131,0.898505594475206));
#51225=DIRECTION('ref_axis',(0.0755957726563047,-0.987007291747337,0.141781117198601));
#51226=DIRECTION('center_axis',(0.396547824746198,-0.137109889419203,0.907717302309762));
#51227=DIRECTION('ref_axis',(-0.0346160739492184,-0.990313730678898,-0.134463535031565));
#51228=DIRECTION('center_axis',(0.391433693991048,-0.879260729009837,-0.271441031588101));
#51229=DIRECTION('ref_axis',(-0.748341987988513,-0.132503133700379,-0.649943988796711));
#51230=DIRECTION('center_axis',(-0.473721511495587,-0.879260728677342,0.0498848729789476));
#51231=DIRECTION('ref_axis',(0.123997230797718,-0.122671608386178,-0.984670687717699));
#51232=DIRECTION('center_axis',(0.212775665524956,0.705424652954647,0.676093614201634));
#51233=DIRECTION('ref_axis',(-0.909218272985087,-0.110462470653129,0.401397776086544));
#51234=DIRECTION('center_axis',(0.292785973844741,0.160364694852788,0.942634360801981));
#51235=DIRECTION('ref_axis',(0.0572297915402712,-0.987007291743488,0.150137793394741));
#51236=DIRECTION('center_axis',(0.279653782042791,-0.137109889440163,0.950260301394765));
#51237=DIRECTION('ref_axis',(-0.0174903662316186,-0.99031373067602,-0.137741794396716));
#51238=DIRECTION('center_axis',(0.422367704615302,-0.879260729008736,-0.220240987377524));
#51239=DIRECTION('ref_axis',(-0.660981506108124,-0.132503133685961,-0.738611107516287));
#51240=DIRECTION('center_axis',(-0.476238308321661,-0.879260728676558,-0.00988153298285341));
#51241=DIRECTION('ref_axis',(0.246431436838738,-0.122671608368691,-0.961365291363191));
#51242=DIRECTION('center_axis',(0.126360866964444,0.705424652951288,0.697430276306204));
#51243=DIRECTION('ref_axis',(-0.952357296558165,-0.110462470671254,0.284277368542813));
#51244=DIRECTION('center_axis',(0.172333856482175,0.160364694835558,0.971897220162852));
#51245=DIRECTION('ref_axis',(0.0379612624105628,-0.98700729174629,0.156126706862887));
#51246=DIRECTION('center_axis',(0.158349432142159,-0.137109889429416,0.977817127872543));
#51247=DIRECTION('ref_axis',(-8.88249781092152E-5,-0.990313730677477,-0.138847783352057));
#51248=DIRECTION('center_axis',(0.446640724211219,-0.879260729010886,-0.165567611250882));
#51249=DIRECTION('ref_axis',(-0.563196951097272,-0.132503133693378,-0.815629887777644));
#51250=DIRECTION('center_axis',(-0.471244542531502,-0.879260728677323,-0.0694921012784819));
#51251=DIRECTION('ref_axis',(0.364979272000188,-0.122671608386658,-0.922898590044455));
#51252=DIRECTION('center_axis',(0.0379532820704627,0.705424652950965,0.707768046318206));
#51253=DIRECTION('ref_axis',(-0.980477076648027,-0.110462470672139,0.162673737095898));
#51254=DIRECTION('center_axis',(0.0491639312547749,0.160364694836564,0.985832679775606));
#51255=DIRECTION('ref_axis',(0.0180940615012009,-0.987007291746126,0.15965340891559));
#51256=DIRECTION('center_axis',(0.0345478171019963,-0.137109889427261,0.989953194123203));
#51257=DIRECTION('ref_axis',(0.017314117093875,-0.990313730677783,-0.137764059828063));
#51258=DIRECTION('center_axis',(-0.75633600629039,0.584827951390054,-0.293141796510861));
#51259=DIRECTION('ref_axis',(-0.343345849080795,0.0265489689972696,0.938833734036102));
#51260=DIRECTION('center_axis',(0.963047106314052,-1.31484110737795E-11,
0.269333011382066));
#51261=DIRECTION('ref_axis',(0.269299613072503,-0.0157477670567345,-0.96292768484021));
#51262=DIRECTION('center_axis',(-0.947192631974055,-0.000115441176542844,
-0.32066509727034));
#51263=DIRECTION('ref_axis',(0.00786439770681546,0.999690782633873,-0.0235900480199696));
#51264=DIRECTION('',(0.944235193661784,-6.06181771180169E-10,0.329271770807176));
#51265=DIRECTION('center_axis',(0.755847214530432,-0.601098527978643,0.259568002551347));
#51266=DIRECTION('ref_axis',(-0.304733775776946,0.0279220144013082,0.95202819654278));
#51267=DIRECTION('',(0.434844806368806,2.24206636476412E-10,0.900505410519046));
#51268=DIRECTION('center_axis',(-0.787112483927548,0.584827952222553,-0.19603623120378));
#51269=DIRECTION('ref_axis',(-0.243954870275565,-0.00326197145111748,0.969781099429703));
#51270=DIRECTION('center_axis',(0.978058326780646,-5.2326700288553E-10,
0.208331249252345));
#51271=DIRECTION('ref_axis',(0.208305626739765,-0.0156832196319802,-0.977938036120146));
#51272=DIRECTION('',(-0.978058312613197,8.32144303432302E-8,-0.208331315764625));
#51273=DIRECTION('center_axis',(-0.777850283233954,0.584827969931555,-0.230054737961631));
#51274=DIRECTION('ref_axis',(-0.278731662566012,0.0070448013555362,0.960343184000932));
#51275=DIRECTION('center_axis',(-0.96304708547139,5.92586886094829E-10,
-0.269333085908621));
#51276=DIRECTION('ref_axis',(0.269300010215738,0.0156715280545403,-0.96292881756973));
#51277=DIRECTION('',(0.963047106749921,-1.36557432027528E-11,0.26933300982354));
#51278=DIRECTION('center_axis',(-0.978058312798117,-2.50584992505245E-13,
-0.208331314896489));
#51279=DIRECTION('ref_axis',(0.00340963653580824,0.999866061277598,-0.0160073072037918));
#51280=DIRECTION('',(0.978058312887135,-6.06514838087569E-10,0.208331314478577));
#51281=DIRECTION('center_axis',(-0.787112480221453,0.584827951389699,-0.196036248568883));
#51282=DIRECTION('ref_axis',(-0.222971396850376,0.0265489690037058,0.974463395121352));
#51283=DIRECTION('center_axis',(0.989209569349546,-1.2561123777913E-11,
0.146507432942106));
#51284=DIRECTION('ref_axis',(0.146489265467591,-0.0157477670536161,-0.989086903631623));
#51285=DIRECTION('center_axis',(0.782419632888726,-0.601098528018349,0.162788444566697));
#51286=DIRECTION('ref_axis',(-0.205370608821025,-0.00227572672788967,0.978681630613522));
#51287=DIRECTION('',(0.490529942139282,5.19500677922187E-12,0.871424337429723));
#51288=DIRECTION('',(0.544279180131203,2.24062901110918E-10,0.838904150708355));
#51289=DIRECTION('center_axis',(0.78241963073013,-0.601098528002463,0.162788455000345));
#51290=DIRECTION('ref_axis',(-0.183010085949976,0.0279220138800812,0.982714439489653));
#51291=DIRECTION('center_axis',(0.,-1.,1.45983193964168E-32));
#51292=DIRECTION('ref_axis',(1.,0.,0.));
#51293=DIRECTION('center_axis',(-0.756949290928045,0.60109853604161,-0.256336343369729));
#51294=DIRECTION('ref_axis',(-0.302155559728147,0.0258666713804852,0.952907620410848));
#51295=DIRECTION('center_axis',(-0.780842226674104,-0.601098522914074,-0.170193956394304));
#51296=DIRECTION('ref_axis',(-0.232606079276408,0.0268944878410888,0.972199104302932));
#51297=DIRECTION('center_axis',(0.78010795135025,0.601098531832816,0.173528496992713));
#51298=DIRECTION('ref_axis',(-0.236757469743944,0.0268942924313918,0.971196477318086));
#51299=DIRECTION('',(-0.838904141906341,-3.07807852447804E-8,0.544279193697853));
#51300=DIRECTION('center_axis',(-0.115217253588766,0.793626260376509,0.59739630340023));
#51301=DIRECTION('ref_axis',(-2.69955750324411E-17,-0.601401446663863,0.798946994456211));
#51302=DIRECTION('center_axis',(-0.503978321595855,0.471546674544287,-0.723636362469196));
#51303=DIRECTION('ref_axis',(0.614174030924001,-0.393423319529449,-0.684111358909494));
#51304=DIRECTION('center_axis',(0.,-1.,1.45983193964168E-32));
#51305=DIRECTION('ref_axis',(1.,0.,0.));
#51306=DIRECTION('center_axis',(-0.783107990018738,0.601098526871089,-0.159444149978034));
#51307=DIRECTION('ref_axis',(-0.202698002714123,-0.00432816599900778,0.979231732877765));
#51308=DIRECTION('center_axis',(-0.780842215871236,-0.601098528389853,-0.170193986617777));
#51309=DIRECTION('ref_axis',(-0.210533861636455,-0.00330175297127346,0.977580989755713));
#51310=DIRECTION('center_axis',(0.78010795247552,0.601098527550831,0.173528506766684));
#51311=DIRECTION('ref_axis',(-0.214708427362672,-0.003301934692242,0.976672610677056));
#51312=DIRECTION('center_axis',(0.,-1.,1.45983193964168E-32));
#51313=DIRECTION('ref_axis',(1.,0.,0.));
#51314=DIRECTION('center_axis',(0.795705453891954,0.601098532045573,0.0743867287844844));
#51315=DIRECTION('ref_axis',(-0.113167377776585,0.0268942876583815,0.993211881674056));
#51316=DIRECTION('center_axis',(-0.783107979656637,0.601098535644099,-0.159444167797447));
#51317=DIRECTION('ref_axis',(-0.180341991740008,0.0258666807695524,0.983263790059012));
#51318=DIRECTION('center_axis',(-0.796016009810675,-0.601098523313665,-0.0709864592385278));
#51319=DIRECTION('ref_axis',(-0.10892306480896,0.0268944792246232,0.993686295034735));
#51320=DIRECTION('center_axis',(-0.805474420453926,0.584828255987311,-0.0958481559199371));
#51321=DIRECTION('ref_axis',(-0.141747987849753,-0.0330815410845231,0.989349846909585));
#51322=DIRECTION('center_axis',(0.989214559142771,-1.08101365926502E-7,
0.146473738192076));
#51323=DIRECTION('ref_axis',(0.146455740324152,-0.0156751635321152,-0.989093021598245));
#51324=DIRECTION('',(-0.989209569691844,-4.44089209849706E-13,-0.146507430630931));
#51325=DIRECTION('center_axis',(-0.80054981432474,0.584827952226173,-0.13075267140508));
#51326=DIRECTION('ref_axis',(-0.1773246910663,-0.0227607295940804,0.983889172176718));
#51327=DIRECTION('center_axis',(-0.978058297134577,5.77132968639425E-10,
-0.208331388432495));
#51328=DIRECTION('ref_axis',(0.208305732673441,0.0156933905082622,-0.97793785039221));
#51329=DIRECTION('',(0.978058312885186,-2.20379270384577E-11,0.208331314487726));
#51330=DIRECTION('center_axis',(-0.80055020562547,0.584827969931532,-0.130750196400547));
#51331=DIRECTION('ref_axis',(-0.156170863562451,0.00704480134783312,0.987704931722085));
#51332=DIRECTION('center_axis',(-0.989209560482432,4.66318822968212E-10,
-0.146507492812327));
#51333=DIRECTION('ref_axis',(0.146489500829708,0.0156715280542981,-0.989088079674963));
#51334=DIRECTION('',(0.989209569691789,-1.4432899319988E-11,0.146507430631303));
#51335=DIRECTION('center_axis',(-0.80547572164662,0.584827952222745,-0.0958390741650192));
#51336=DIRECTION('ref_axis',(-0.120485412206387,-0.00326197145934098,0.992709738537734));
#51337=DIRECTION('center_axis',(0.996456866177649,1.93578415386087E-10,
0.0841053734752966));
#51338=DIRECTION('ref_axis',(0.084095029421336,-0.0156832196296146,-0.996334312692619));
#51339=DIRECTION('',(-0.996456868143889,8.32140417651974E-8,-0.0841053501797939));
#51340=DIRECTION('',(-0.803073192437107,-1.43735365430951E-13,0.595880397050342));
#51341=DIRECTION('',(-0.764072860871016,-3.07812369845586E-8,0.645129958442778));
#51342=DIRECTION('center_axis',(0.796652822001855,-0.601098527974287,0.0634416335195257));
#51343=DIRECTION('ref_axis',(-0.103672281525895,-0.0324816871225219,0.994080981633232));
#51344=DIRECTION('',(0.544279180225795,8.00811321699502E-12,0.838904150646984));
#51345=DIRECTION('',(0.595880397048087,5.05127141378972E-12,0.80307319243878));
#51346=DIRECTION('center_axis',(0.796652822107589,-0.601098528033706,0.0634416316288104));
#51347=DIRECTION('ref_axis',(-0.0810898709684607,-0.00227572362146215,0.996704195791468));
#51348=DIRECTION('center_axis',(0.,-1.,1.45983193964168E-32));
#51349=DIRECTION('ref_axis',(1.,0.,0.));
#51350=DIRECTION('center_axis',(-0.796916614506406,0.601098515216612,-0.0600373594358867));
#51351=DIRECTION('ref_axis',(-0.100958817490252,-0.0345386959223724,0.994290900921331));
#51352=DIRECTION('center_axis',(-0.780842210528445,-0.601098532642785,-0.170193996109563));
#51353=DIRECTION('ref_axis',(-0.188148565998907,-0.033509922223831,0.981568745542108));
#51354=DIRECTION('center_axis',(0.780107924867447,0.601098517625842,0.173528665260302));
#51355=DIRECTION('ref_axis',(-0.19234048933514,-0.0335101945242414,0.980755934483838));
#51356=DIRECTION('center_axis',(0.,-1.,1.45983193964168E-32));
#51357=DIRECTION('ref_axis',(1.,0.,0.));
#51358=DIRECTION('center_axis',(0.795705456777408,0.601098527536453,0.0743867343560998));
#51359=DIRECTION('ref_axis',(-0.0906058539709184,-0.00330193705786042,0.995881356607235));
#51360=DIRECTION('center_axis',(-0.796916600686538,0.6010985268631,-0.0600374262708134));
#51361=DIRECTION('ref_axis',(-0.0783693870587833,-0.00432816741275879,0.996914994439785));
#51362=DIRECTION('center_axis',(-0.796016004324672,-0.601098528386779,-0.0709864777984713));
#51363=DIRECTION('ref_axis',(-0.0863503538729397,-0.00330175382353104,0.996259361214592));
#51364=DIRECTION('',(-0.996456868253698,-7.77156117236895E-13,-0.0841053488788494));
#51365=DIRECTION('center_axis',(-0.810624895144558,0.584827952146236,-0.0293861491236025));
#51366=DIRECTION('ref_axis',(-0.0740902026680098,-0.052656272846004,0.995860411301996));
#51367=DIRECTION('center_axis',(-0.989209555778179,7.0544820002307E-10,
-0.146507524575151));
#51368=DIRECTION('ref_axis',(0.146489298830423,0.01577299981401,-0.989086496624556));
#51369=DIRECTION('',(0.989209569692257,-1.77302617009905E-10,0.146507430628141));
#51370=DIRECTION('center_axis',(-0.810624895029856,0.58482795222639,-0.0293861506925126));
#51371=DIRECTION('ref_axis',(-0.0526124215066951,-0.0227607295861682,0.998355589102354));
#51372=DIRECTION('center_axis',(-0.996456861480342,6.15511979164734E-10,
-0.0841054291276525));
#51373=DIRECTION('ref_axis',(0.0840950716516077,0.0156933905097029,-0.99633414897725));
#51374=DIRECTION('',(0.996456868253725,-2.32591723655397E-11,0.0841053488785229));
#51375=DIRECTION('center_axis',(-0.81113612605453,0.584827952238869,0.00586952207091835));
#51376=DIRECTION('ref_axis',(-0.0166244013107426,-0.0330869090662063,0.999314207709219));
#51377=DIRECTION('center_axis',(0.999771608389312,-5.84500981991017E-10,
0.0213712671278065));
#51378=DIRECTION('ref_axis',(0.0213686413800553,-0.0156751701950672,-0.999648773422409));
#51379=DIRECTION('',(-0.999771606794424,-3.88578058618759E-13,-0.021371341738294));
#51380=DIRECTION('',(-0.764072871228432,0.,0.645129946175761));
#51381=DIRECTION('',(-0.72205710346861,0.,0.691833462135593));
#51382=DIRECTION('',(0.59588039702185,6.70833484120459E-11,0.803073192458248));
#51383=DIRECTION('',(0.645129946172589,8.00811321699427E-12,0.76407287123111));
#51384=DIRECTION('center_axis',(0.798322321538695,-0.601098527845071,-0.0369057008544292));
#51385=DIRECTION('ref_axis',(0.0217365923777059,-0.0324816894873403,0.99923593830479));
#51386=DIRECTION('center_axis',(0.,-1.,1.45983193964168E-32));
#51387=DIRECTION('ref_axis',(1.,0.,0.));
#51388=DIRECTION('center_axis',(-0.784612619000654,0.60109854236896,-0.151866982806818));
#51389=DIRECTION('ref_axis',(-0.151616329939511,0.0514848335721866,0.987097665080673));
#51390=DIRECTION('center_axis',(0.798967517066683,0.601098534860787,-0.0182059896878827));
#51391=DIRECTION('ref_axis',(-0.0167582471047594,0.0525165168369252,0.998479432243495));
#51392=DIRECTION('center_axis',(0.,-1.,1.45983193964168E-32));
#51393=DIRECTION('ref_axis',(1.,0.,0.));
#51394=DIRECTION('center_axis',(0.795705459175127,0.601098522337475,0.074386750719496));
#51395=DIRECTION('ref_axis',(-0.0679024024563864,-0.0335101098683029,0.997129046952933));
#51396=DIRECTION('center_axis',(-0.798157366407851,0.601098516594213,0.0403161480937846));
#51397=DIRECTION('ref_axis',(0.0244549337192487,-0.0345386712358531,0.99910411689976));
#51398=DIRECTION('center_axis',(-0.79601600041738,-0.601098532679962,-0.0709864852596231));
#51399=DIRECTION('ref_axis',(-0.0636417725517395,-0.0335099214952075,0.997410051056163));
#51400=DIRECTION('center_axis',(-0.806364311797864,0.584827908068084,-0.0880506365875126));
#51401=DIRECTION('ref_axis',(-0.0927703937601591,0.0219600677301591,0.995445332234208));
#51402=DIRECTION('center_axis',(0.999771754696857,-1.94678874097512E-8,
0.0213644216014981));
#51403=DIRECTION('ref_axis',(0.0213617749287953,-0.0157391387090833,-0.999647915060392));
#51404=DIRECTION('',(-0.999771606794415,-3.88578058618275E-13,-0.0213713417387115));
#51405=DIRECTION('center_axis',(-0.801776305997045,0.584827952320353,-0.123008216500021));
#51406=DIRECTION('ref_axis',(-0.128518655158662,0.032283433062828,0.991181484505177));
#51407=DIRECTION('center_axis',(-0.99645686226659,5.28005960808625E-10,
-0.0841054198124182));
#51408=DIRECTION('ref_axis',(0.0840950508622084,0.0157020800817931,-0.996334013823471));
#51409=DIRECTION('',(0.996456868253682,-7.77156117237624E-13,0.0841053488790393));
#51410=DIRECTION('center_axis',(-0.807915936815818,0.584827952145957,0.0724438087608944));
#51411=DIRECTION('ref_axis',(0.0513084262408636,-0.0526562728494161,0.997293719185223));
#51412=DIRECTION('center_axis',(-0.999771605207897,5.41160526128575E-10,
-0.0213714159574124));
#51413=DIRECTION('ref_axis',(0.0213687573297561,0.0157729998140531,-0.999647232120936));
#51414=DIRECTION('',(0.999771606794473,-1.77302617010133E-10,0.021371341736028));
#51415=DIRECTION('',(-0.999140703555321,7.77156117237103E-13,0.0414470083236203));
#51416=DIRECTION('',(-0.72205710346864,0.,0.691833462135562));
#51417=DIRECTION('',(-0.677191706198013,0.,0.735806627488924));
#51418=DIRECTION('center_axis',(0.797228847766677,-0.60109852812305,0.0557379922218206));
#51419=DIRECTION('ref_axis',(-0.0522531812709769,0.0232723689287435,0.998362660505443));
#51420=DIRECTION('',(0.64512994617573,0.,0.764072871228458));
#51421=DIRECTION('',(0.691833462110807,6.51326541667403E-11,0.722057103492359));
#51422=DIRECTION('center_axis',(0.,-1.,1.45983193964168E-32));
#51423=DIRECTION('ref_axis',(1.,0.,0.));
#51424=DIRECTION('center_axis',(-0.797459701698008,0.601098534578107,-0.052331404488862));
#51425=DIRECTION('ref_axis',(-0.0495338937900471,0.0212179603895841,0.998547040215383));
#51426=DIRECTION('center_axis',(-0.798882449897006,-0.601098524060562,0.0216193343739451));
#51427=DIRECTION('ref_axis',(0.0103159222699735,0.0222453126288138,0.999699318702262));
#51428=DIRECTION('center_axis',(0.798967520085859,0.601098531169166,-0.0182059790762032));
#51429=DIRECTION('ref_axis',(0.00604483790312725,0.0222451252052261,0.999734271863943));
#51430=DIRECTION('center_axis',(0.,-1.,1.45983193964168E-32));
#51431=DIRECTION('ref_axis',(1.,0.,0.));
#51432=DIRECTION('center_axis',(0.790385605091053,0.60109853538485,-0.118199602465651));
#51433=DIRECTION('ref_axis',(0.108516544623323,0.0525165107899705,0.992706490175954));
#51434=DIRECTION('center_axis',(-0.797459694190177,0.601098542402019,-0.0523314290295791));
#51435=DIRECTION('ref_axis',(-0.0267046471782287,0.0514848332083756,0.998316670084494));
#51436=DIRECTION('center_axis',(-0.811041494763648,0.584827953016302,0.0137098191932171));
#51437=DIRECTION('ref_axis',(0.0112444354981666,-0.00784645566785257,0.999905993483277));
#51438=DIRECTION('center_axis',(0.999140686056023,-1.52846821713024E-9,
-0.0414474301676266));
#51439=DIRECTION('ref_axis',(-0.0414423360944754,-0.0156778483090111,-0.999017886652402));
#51440=DIRECTION('',(-0.999140703563491,1.2575884663851E-8,0.0414470081266709));
#51441=DIRECTION('center_axis',(-0.810871087291932,0.584827953187666,-0.0215486650242196));
#51442=DIRECTION('ref_axis',(-0.0247910851729539,0.00246158313914707,0.999689623185315));
#51443=DIRECTION('center_axis',(-0.999771605317616,5.21632347592839E-10,
-0.0213714108246876));
#51444=DIRECTION('ref_axis',(0.0213687865604974,0.0156707406169895,-0.999648839767969));
#51445=DIRECTION('',(0.999771606794421,-6.46149800302255E-11,0.0213713417384283));
#51446=DIRECTION('center_axis',(-0.810871077874132,0.584827952320916,-0.0215490429339312));
#51447=DIRECTION('ref_axis',(-0.00327726666415344,0.0322834330552977,0.999473381072941));
#51448=DIRECTION('center_axis',(-0.999140706103433,4.51516519363189E-10,
0.0414469468976114));
#51449=DIRECTION('ref_axis',(-0.0414418370929418,0.0157020800815274,-0.999017526782927));
#51450=DIRECTION('',(0.999140703555301,-7.77156117237896E-13,-0.0414470083241067));
#51451=DIRECTION('center_axis',(-0.811041537039199,0.58482792304389,0.0137085967649634));
#51452=DIRECTION('ref_axis',(0.0327240637255072,0.0219596690916775,0.999223152547354));
#51453=DIRECTION('center_axis',(0.994566169398982,-1.3078163819384E-8,-0.104106362375384));
#51454=DIRECTION('ref_axis',(-0.104093467141315,-0.0157391391449197,-0.994442974532716));
#51455=DIRECTION('',(-0.994566648423267,7.77156117236963E-13,0.10410178597944));
#51456=DIRECTION('',(-0.677191704413373,-4.65201564659664E-9,0.735806629131398));
#51457=DIRECTION('',(-0.629653742642429,-1.43735365430928E-13,0.776875900241719));
#51458=DIRECTION('center_axis',(0.797928283300872,-0.601098528053661,-0.04462078305281));
#51459=DIRECTION('ref_axis',(0.0506350763003886,-0.0069195234725463,0.99869325082478));
#51460=DIRECTION('',(0.691833462126601,2.34493981894284E-11,0.722057103477226));
#51461=DIRECTION('',(0.735806627488914,0.,0.677191706198024));
#51462=DIRECTION('center_axis',(0.797928295444368,-0.601098524297468,-0.0446206164978998));
#51463=DIRECTION('ref_axis',(0.0732867338760961,0.023272472024472,0.997039340589751));
#51464=DIRECTION('center_axis',(0.,-1.,1.45983193964168E-32));
#51465=DIRECTION('ref_axis',(1.,0.,0.));
#51466=DIRECTION('center_axis',(-0.797730380563259,0.601098527999986,0.048029153257653));
#51467=DIRECTION('ref_axis',(0.053358553918965,-0.0089720006035093,0.998535111014554));
#51468=DIRECTION('center_axis',(-0.798882451489998,-0.601098528053305,0.0216191644954361));
#51469=DIRECTION('ref_axis',(0.0330247131478521,-0.00794574335897238,0.99942295024878));
#51470=DIRECTION('center_axis',(0.798967518742967,0.601098528198664,-0.0182061360839188));
#51471=DIRECTION('ref_axis',(0.0287548632853352,-0.00794573399547077,0.999554912522926));
#51472=DIRECTION('center_axis',(0.,-1.,1.45983193964168E-32));
#51473=DIRECTION('ref_axis',(1.,0.,0.));
#51474=DIRECTION('center_axis',(0.79038559015766,0.601098528086115,-0.118199739440638));
#51475=DIRECTION('ref_axis',(0.131297210925068,0.0222452083715773,0.991093433086812));
#51476=DIRECTION('center_axis',(-0.797730380655153,0.601098528105586,0.0480291504097525));
#51477=DIRECTION('ref_axis',(0.0760075873921403,0.0212181391866325,0.996881455955663));
#51478=DIRECTION('center_axis',(-0.789873402538101,-0.601098524330917,0.121575375837698));
#51479=DIRECTION('ref_axis',(0.135530123087635,0.0222453097977533,0.990523463592788));
#51480=DIRECTION('center_axis',(-0.80292169045898,0.584826536164717,0.115302565401089));
#51481=DIRECTION('ref_axis',(0.129132272514604,-0.0181846250656886,0.991460627360681));
#51482=DIRECTION('center_axis',(0.994566501061888,-4.70791329828775E-9,
-0.104103193829549));
#51483=DIRECTION('ref_axis',(-0.104090396391608,-0.0156795063510537,-0.994444237984023));
#51484=DIRECTION('',(-0.994566648759581,2.06170772008968E-7,0.104101782766161));
#51485=DIRECTION('center_axis',(-0.807177436659008,0.584827782536509,0.0802561556643659));
#51486=DIRECTION('ref_axis',(0.0792583150449474,-0.0273551074277302,0.996478709051956));
#51487=DIRECTION('center_axis',(-0.999140707616432,6.53531644443777E-10,
0.0414469104244949));
#51488=DIRECTION('ref_axis',(-0.0414418004598346,0.0157023279240177,-0.999017524407062));
#51489=DIRECTION('',(-0.999140703510251,-1.29267417449312E-5,0.0414470073942642));
#51490=DIRECTION('center_axis',(-0.807177928572345,0.584827952254024,0.0802499712649406));
#51491=DIRECTION('ref_axis',(0.100698427306123,0.00246180457994313,0.994913949171627));
#51492=DIRECTION('center_axis',(-0.994566654136008,4.10157440230847E-10,
0.1041017314011));
#51493=DIRECTION('ref_axis',(-0.104088948368872,0.0156707406194045,-0.994444527721834));
#51494=DIRECTION('',(0.994566648423206,-6.42264019716518E-11,-0.104101785980022));
#51495=DIRECTION('center_axis',(-0.802927900605498,0.58482795337543,0.115252120934729));
#51496=DIRECTION('ref_axis',(0.136477184444299,-0.00784642890627583,0.990612139880981));
#51497=DIRECTION('center_axis',(0.986067412984717,-1.20307368323152E-9,
-0.1663461963786));
#51498=DIRECTION('ref_axis',(-0.166325751615243,-0.0156778482801143,-0.985946220350243));
#51499=DIRECTION('',(-0.986067493104144,0.,0.166345721445757));
#51500=DIRECTION('',(-0.629653711784272,-7.62628872217157E-8,0.776875925252085));
#51501=DIRECTION('',(-0.579630823425917,0.,0.814879198737207));
#51502=DIRECTION('center_axis',(0.994566627728983,-1.61526260366513E-7,
-0.10410198368798));
#51503=DIRECTION('ref_axis',(-0.0803539506773033,-0.635772804014541,-0.767682345951786));
#51504=DIRECTION('',(-0.735806627488086,0.,-0.677191706198924));
#51505=DIRECTION('',(0.776875900233977,2.35931335548636E-11,0.629653742651982));
#51506=DIRECTION('center_axis',(0.786043912908388,-0.601098528034509,-0.144275869688652));
#51507=DIRECTION('ref_axis',(0.175405260409767,-0.00691952526967788,0.984471997971818));
#51508=DIRECTION('center_axis',(0.,-1.,1.45983193964168E-32));
#51509=DIRECTION('ref_axis',(1.,0.,0.));
#51510=DIRECTION('center_axis',(0.790385590374402,0.601098528024184,-0.118199738306259));
#51511=DIRECTION('ref_axis',(0.15380555625738,-0.00794574594539266,0.988069185829479));
#51512=DIRECTION('center_axis',(-0.78542038860029,0.601098527972214,0.147632560231834));
#51513=DIRECTION('ref_axis',(0.178087442540051,-0.00897200248407754,0.983973762851922));
#51514=DIRECTION('center_axis',(-0.789873424064263,-0.601098528093318,0.121575217380206));
#51515=DIRECTION('ref_axis',(0.158025217926938,-0.00794573996386805,0.987403107001173));
#51516=DIRECTION('center_axis',(-0.904842557875188,0.398564395022499,0.149687569551504));
#51517=DIRECTION('ref_axis',(-0.40310605101085,-0.915153272210966,2.27467263527814E-16));
#51518=DIRECTION('center_axis',(0.984879681053578,5.74456348530311E-5,-0.173239748752421));
#51519=DIRECTION('ref_axis',(0.1732397170712,0.000363132139149149,0.984879621356915));
#51520=DIRECTION('',(-0.986067643452147,5.94973695487231E-5,0.166344819567047));
#51521=DIRECTION('center_axis',(-0.804293392145717,0.590180063977743,0.069279372355438));
#51522=DIRECTION('ref_axis',(0.565263839752734,0.795824505360262,-0.217117820862523));
#51523=DIRECTION('center_axis',(-0.790753837980066,0.584827782536617,0.180789470083574));
#51524=DIRECTION('ref_axis',(0.203525238326007,-0.02735510741636,0.978687475889306));
#51525=DIRECTION('center_axis',(-0.986067496545839,4.69894213309026E-11,
0.166345701044009));
#51526=DIRECTION('ref_axis',(-0.16632519242299,0.0157023279237646,-0.985945925121266));
#51527=DIRECTION('',(-0.986067493175983,-1.29267417804204E-5,0.16634572051764));
#51528=DIRECTION('center_axis',(-0.78213916976026,0.584826536166289,0.215026141951326));
#51529=DIRECTION('ref_axis',(0.252376992392512,-0.018184624930405,0.967458098899922));
#51530=DIRECTION('center_axis',(0.973676800738548,7.17798744206148E-10,
-0.227933077247569));
#51531=DIRECTION('ref_axis',(-0.227905057190963,-0.0156795066151571,-0.973557105658979));
#51532=DIRECTION('',(-0.973676780617697,2.06170660986877E-7,0.227933163199029));
#51533=DIRECTION('center_axis',(-0.220379505183991,0.550037558020212,0.805538055253767));
#51534=DIRECTION('ref_axis',(2.93242547267914E-16,-0.825842037277522,0.563901524616942));
#51535=DIRECTION('center_axis',(-0.716151223202446,-0.477126089861736,-0.509389948741523));
#51536=DIRECTION('ref_axis',(0.61922185901425,-0.0976233195081025,-0.779123852033267));
#51537=DIRECTION('',(-0.52732033240823,-7.62630514906775E-8,0.849666562263614));
#51538=DIRECTION('',(-0.81487919873641,0.,-0.579630823427038));
#51539=DIRECTION('center_axis',(0.973676779882379,4.07347797860785E-12,
-0.227933166340226));
#51540=DIRECTION('ref_axis',(-0.175936196944572,-0.635772805085134,-0.751557978414747));
#51541=DIRECTION('center_axis',(-0.713631661728486,0.584827951390276,-0.385624323210159));
#51542=DIRECTION('ref_axis',(-0.458305532168383,0.0265489689922669,0.888398104134235));
#51543=DIRECTION('center_axis',(0.921696813429137,2.97646228428206E-11,
0.387911051807723));
#51544=DIRECTION('ref_axis',(0.387862949374495,-0.0157477670559207,-0.921582519547365));
#51545=DIRECTION('center_axis',(-0.899533742181365,-0.000115441197578976,
-0.436851271430586));
#51546=DIRECTION('ref_axis',(0.0107693567476671,0.99969019274119,-0.0224396856556493));
#51547=DIRECTION('',(0.895520921373541,-6.06958927296726E-10,0.445019414612761));
#51548=DIRECTION('center_axis',(0.717354636765597,-0.601098528005662,0.352254005996133));
#51549=DIRECTION('ref_axis',(-0.421651630621408,0.027922013862445,0.906327900671812));
#51550=DIRECTION('',(0.318552670246311,2.24206636476423E-10,0.947905162069996));
#51551=DIRECTION('center_axis',(0.,-1.,1.45983193964168E-32));
#51552=DIRECTION('ref_axis',(1.,0.,0.));
#51553=DIRECTION('center_axis',(-0.718853053469519,0.601098535825989,-0.349185964416385));
#51554=DIRECTION('ref_axis',(-0.419203972104053,0.0258666762854648,0.907523523017518));
#51555=DIRECTION('center_axis',(-0.753354093398353,-0.601098522929298,-0.266717407928618));
#51556=DIRECTION('ref_axis',(-0.352620768704926,0.0268944874816471,0.935379751769861));
#51557=DIRECTION('center_axis',(0.752207681322588,0.601098531694907,0.269933620272695));
#51558=DIRECTION('ref_axis',(-0.356613757471971,0.0268942954984485,0.933864725134944));
#51559=DIRECTION('center_axis',(-0.756336012135367,0.584827952222443,-0.293141779769575));
#51560=DIRECTION('ref_axis',(-0.363577014308828,-0.00326197144318428,0.931558433061814));
#51561=DIRECTION('center_axis',(0.944235222537388,-6.87901178487106E-10,
0.329271688002125));
#51562=DIRECTION('ref_axis',(0.329231191113268,-0.0156832196311381,-0.944119091757041));
#51563=DIRECTION('',(-0.944235193228753,8.32144303432336E-8,-0.329271772048945));
#51564=DIRECTION('center_axis',(-0.742883197204518,0.584827969931003,-0.325731178884637));
#51565=DIRECTION('ref_axis',(-0.396896696751271,0.00704480136778811,0.917836250581561));
#51566=DIRECTION('center_axis',(-0.921696788164321,5.28962013185638E-10,
-0.387911111838235));
#51567=DIRECTION('ref_axis',(0.387863474058534,0.0156715280546057,-0.921583598323928));
#51568=DIRECTION('',(0.921696815638088,-1.44328993199795E-11,0.387911046559141));
#51569=DIRECTION('',(-0.900505403486899,-3.07809289801569E-8,0.434844820931441));
#51570=DIRECTION('center_axis',(-0.189182341558766,0.793626260374901,0.57824510416059));
#51571=DIRECTION('ref_axis',(1.24306842251369E-16,-0.588879097818246,0.808221138150178));
#51572=DIRECTION('center_axis',(-0.409308616753587,0.4715466745495,-0.781095506306734));
#51573=DIRECTION('ref_axis',(0.695078489039964,-0.393415955336541,-0.601738963472167));
#51574=DIRECTION('center_axis',(0.75584721514625,-0.601098528044197,0.259568000606312));
#51575=DIRECTION('ref_axis',(-0.326412540790778,-0.00227572104232137,0.945224668694298));
#51576=DIRECTION('',(0.377443537014619,5.19500677922227E-12,0.926032600055686));
#51577=DIRECTION('center_axis',(-0.787110054750406,0.584828255987491,-0.196045078258655));
#51578=DIRECTION('ref_axis',(-0.264628678073429,-0.0330815410799287,0.96378279419218));
#51579=DIRECTION('center_axis',(0.96305628431587,-1.08237348364162E-7,0.269300191681512));
#51580=DIRECTION('ref_axis',(0.269267103038703,-0.0156751635310825,-0.962937960862183));
#51581=DIRECTION('',(-0.963047106749948,7.77156117236919E-13,-0.269333009823441));
#51582=DIRECTION('center_axis',(-0.777849584821009,0.584827952226153,-0.230057144398405));
#51583=DIRECTION('ref_axis',(-0.299240444333017,-0.0227607295926439,0.953906235257842));
#51584=DIRECTION('center_axis',(-0.944235167903987,5.97413398597196E-10,
-0.329271844671434));
#51585=DIRECTION('ref_axis',(0.329231295236,0.0156933905095839,-0.944118886439383));
#51586=DIRECTION('',(0.944235193658857,-2.20379270384694E-11,0.329271770815569));
#51587=DIRECTION('center_axis',(0.782419631380168,-0.601098527991307,0.162788451917224));
#51588=DIRECTION('ref_axis',(-0.227446178817791,-0.032481686875515,0.973248773828617));
#51589=DIRECTION('',(0.434844806470272,8.00811321699437E-12,0.900505410470049));
#51590=DIRECTION('center_axis',(0.,-1.,1.45983193964168E-32));
#51591=DIRECTION('ref_axis',(1.,0.,0.));
#51592=DIRECTION('center_axis',(-0.756949293860049,0.601098526927086,-0.256336356084852));
#51593=DIRECTION('ref_axis',(-0.323829959303373,-0.00432815696677943,0.946105398206165));
#51594=DIRECTION('center_axis',(-0.753354077033342,-0.601098528375901,-0.266717441877294));
#51595=DIRECTION('ref_axis',(-0.331397130446077,-0.00330175671303345,0.943485580353359));
#51596=DIRECTION('center_axis',(0.752207682272757,0.60109852758074,0.269933626786501));
#51597=DIRECTION('ref_axis',(-0.335424917255577,-0.00330192953264533,0.942061156266116));
#51598=DIRECTION('',(-0.871424337428488,0.,0.490529942141476));
#51599=DIRECTION('center_axis',(0.,-1.,1.45983193964168E-32));
#51600=DIRECTION('ref_axis',(1.,0.,0.));
#51601=DIRECTION('center_axis',(-0.783108000754804,0.601098516989598,-0.159444134500836));
#51602=DIRECTION('ref_axis',(-0.224780462152304,-0.0345386642712182,0.973797116706019));
#51603=DIRECTION('center_axis',(-0.753354077630504,-0.601098533169073,-0.26671742938826));
#51604=DIRECTION('ref_axis',(-0.309688131015092,-0.0335099124882587,0.950247518951462));
#51605=DIRECTION('center_axis',(0.752207680104345,0.60109852274501,0.269933643597471));
#51606=DIRECTION('ref_axis',(-0.313745024739697,-0.0335101026406503,0.948915766794977));
#51607=DIRECTION('',(-0.978058312885208,3.88578058618623E-13,-0.208331314487622));
#51608=DIRECTION('center_axis',(-0.800549814629415,0.584827952146848,-0.130752669894475));
#51609=DIRECTION('ref_axis',(-0.198320384831937,-0.05265627283548,0.978721789831609));
#51610=DIRECTION('center_axis',(-0.963047086493937,5.49753720943777E-10,
-0.269333082252329));
#51611=DIRECTION('ref_axis',(0.269299576821397,0.0157729998148347,-0.962927281990005));
#51612=DIRECTION('',(0.963047106750697,-1.76580972044047E-10,0.269333009820765));
#51613=DIRECTION('',(-0.838904150644731,-6.16008708989698E-13,0.544279180229266));
#51614=DIRECTION('',(0.490529942110868,6.72270837774838E-11,0.871424337445718));
#51615=DIRECTION('center_axis',(0.,-1.,1.45983193964168E-32));
#51616=DIRECTION('ref_axis',(1.,0.,0.));
#51617=DIRECTION('center_axis',(-0.759391731897356,0.601098541947915,-0.249007510718101));
#51618=DIRECTION('ref_axis',(-0.274136938268848,0.0514848384475658,0.960311538245069));
#51619=DIRECTION('center_axis',(0.794949235440494,0.601098534738984,0.0820747501197568));
#51620=DIRECTION('ref_axis',(-0.141768757368629,0.052516518220691,0.988505758581168));
#51621=DIRECTION('center_axis',(-0.788970434280454,0.584827930050748,-0.188419601060691));
#51622=DIRECTION('ref_axis',(-0.216800464321758,0.0219594825770514,0.975968923580468));
#51623=DIRECTION('center_axis',(0.989210085096209,-1.01053617270023E-8,
0.146503950608683));
#51624=DIRECTION('ref_axis',(0.146485803310934,-0.015739139347894,-0.989087553718546));
#51625=DIRECTION('',(-0.98920956969183,0.,-0.146507430631025));
#51626=DIRECTION('center_axis',(-0.780037042816505,0.584827952320453,-0.222527476997218));
#51627=DIRECTION('ref_axis',(-0.251733227677601,0.0322834330622996,0.967258063824091));
#51628=DIRECTION('center_axis',(-0.978058295676359,6.17736426195848E-10,
-0.208331395278425));
#51629=DIRECTION('ref_axis',(0.208305711097874,0.0157020800811686,-0.977937715503975));
#51630=DIRECTION('',(0.978058312885197,-7.77156117237441E-13,0.208331314487675));
#51631=DIRECTION('',(-0.803073192437192,-1.64268989063981E-13,0.595880397050227));
#51632=DIRECTION('center_axis',(0.783956636563995,-0.601098528016923,0.155217755437825));
#51633=DIRECTION('ref_axis',(-0.176969173465271,0.0232723717115823,0.983941211840391));
#51634=DIRECTION('',(0.544279180229423,0.,0.838904150644629));
#51635=DIRECTION('center_axis',(0.,-1.,1.45983193964168E-32));
#51636=DIRECTION('ref_axis',(1.,0.,0.));
#51637=DIRECTION('center_axis',(-0.784612628717512,0.601098534467104,-0.151866963881205));
#51638=DIRECTION('ref_axis',(-0.174294437728632,0.0212179634901381,0.98446495468462));
#51639=DIRECTION('center_axis',(-0.795292643209686,-0.601098524266774,-0.0786776701539809));
#51640=DIRECTION('ref_axis',(-0.115060977215054,0.0222453072138315,0.993109318166575));
#51641=DIRECTION('center_axis',(0.794949236451677,0.601098531229447,0.0820747660288937));
#51642=DIRECTION('ref_axis',(-0.119302758621563,0.0222451235580996,0.992608687380465));
#51643=DIRECTION('center_axis',(-0.806364486303598,0.584827953016318,-0.0880487399062475));
#51644=DIRECTION('ref_axis',(-0.114165681646991,-0.00784645567563293,0.993430737528998));
#51645=DIRECTION('center_axis',(0.996456902738626,-1.43266585541422E-9,
0.0841049403099755));
#51646=DIRECTION('ref_axis',(0.0840946033685045,-0.0156778483110181,-0.99633443318829));
#51647=DIRECTION('',(-0.996456868253666,0.,-0.0841053488792232));
#51648=DIRECTION('center_axis',(-0.801776305949045,0.584827952254045,-0.123008217128146));
#51649=DIRECTION('ref_axis',(-0.149890236715455,0.00246180457886108,0.988699578464359));
#51650=DIRECTION('center_axis',(-0.989209559600953,5.20282766649608E-10,
-0.14650749876402));
#51651=DIRECTION('ref_axis',(0.146489508589636,0.0156707406169381,-0.98908809100185));
#51652=DIRECTION('',(0.989209569691921,-6.41708908203814E-11,0.146507430630414));
#51653=DIRECTION('',(-0.76407287122841,0.,0.645129946175786));
#51654=DIRECTION('center_axis',(0.79722884753577,-0.601098528049182,0.0557379963211305));
#51655=DIRECTION('ref_axis',(-0.0749336502850237,-0.00691952391171873,0.997164514131844));
#51656=DIRECTION('',(0.595880397040365,2.35931335548661E-11,0.80307319244451));
#51657=DIRECTION('center_axis',(0.,-1.,1.45983193964168E-32));
#51658=DIRECTION('ref_axis',(1.,0.,0.));
#51659=DIRECTION('center_axis',(-0.797459710617155,0.601098525255623,-0.0523313756547448));
#51660=DIRECTION('ref_axis',(-0.0722115697536528,-0.00897219529730149,0.997348980500437));
#51661=DIRECTION('center_axis',(-0.795292639168737,-0.601098529139514,-0.0786776737730471));
#51662=DIRECTION('ref_axis',(-0.0924964820476553,-0.00794564883199728,0.995681308187236));
#51663=DIRECTION('center_axis',(0.794949237650369,0.601098526741823,0.0820747872851781));
#51664=DIRECTION('ref_axis',(-0.0967494703898303,-0.00794584267896273,0.995277048646963));
#51665=DIRECTION('center_axis',(-0.811041749443006,0.584825719451611,0.0137897979801614));
#51666=DIRECTION('ref_axis',(0.00387504240444698,-0.0182013008699368,0.999826833353159));
#51667=DIRECTION('center_axis',(0.999771637473267,-4.86463518547559E-9,
0.0213699065047608));
#51668=DIRECTION('ref_axis',(0.0213672794041909,-0.015679506350074,-0.999648734532026));
#51669=DIRECTION('',(-0.999771606725344,2.06171160587013E-7,-0.0213713449689478));
#51670=DIRECTION('center_axis',(-0.810871364980857,0.584827782536638,-0.0215428463151879));
#51671=DIRECTION('ref_axis',(-0.0462585592451372,-0.027355107413009,0.998554877708274));
#51672=DIRECTION('center_axis',(-0.996456860583546,6.00919128441484E-10,
-0.0841054397526283));
#51673=DIRECTION('ref_axis',(0.0840950704737484,0.0157023279254457,-0.996334008262157));
#51674=DIRECTION('',(-0.996456868092506,-1.29267420448973E-5,-0.0841053497952053));
#51675=DIRECTION('',(-0.722057075988495,-7.62629077544141E-8,0.691833490816208));
#51676=DIRECTION('center_axis',(0.999771611042803,-1.6152775507127E-7,0.0213711429936039));
#51677=DIRECTION('ref_axis',(0.0164957749902458,-0.635772804014574,-0.771699961826432));
#51678=DIRECTION('',(-0.645129946174611,0.,-0.764072871229403));
#51679=DIRECTION('center_axis',(-0.916468431161503,0.398564395017297,0.0351003947110158));
#51680=DIRECTION('ref_axis',(-0.398810145302877,-0.91703351520187,-1.87163520774561E-17));
#51681=DIRECTION('center_axis',(0.998826308492376,5.74456517323226E-5,-0.0484355464869609));
#51682=DIRECTION('ref_axis',(0.0484355225308032,0.000363221802276343,0.998826245263454));
#51683=DIRECTION('',(-0.999140739682403,5.94973695487116E-5,0.0414460947130521));
#51684=DIRECTION('center_axis',(-0.806634306274172,0.590180063977203,-0.0320716077777504));
#51685=DIRECTION('ref_axis',(0.588016977321403,0.795820729355314,-0.144587001871456));
#51686=DIRECTION('center_axis',(-0.319602436182492,0.550037558023316,0.771565271088561));
#51687=DIRECTION('ref_axis',(-8.09024547853229E-17,-0.814272451734368,0.580482880321634));
#51688=DIRECTION('center_axis',(-0.646660667342669,-0.477126090214631,-0.595130805242372));
#51689=DIRECTION('ref_axis',(0.711992768894656,-0.0976346405864383,-0.695365928126536));
#51690=DIRECTION('center_axis',(-0.659672919556613,0.584827951390368,-0.472025323977644));
#51691=DIRECTION('ref_axis',(-0.566037463239915,0.0265489689911301,0.823951905425572));
#51692=DIRECTION('center_axis',(0.865810812945574,1.21936651804102E-11,
0.50037149817563));
#51693=DIRECTION('ref_axis',(0.500309450222573,-0.0157477670562345,-0.865703449138751));
#51694=DIRECTION('center_axis',(-0.837688665629566,-0.000115441167396227,
-0.546148044168515));
#51695=DIRECTION('ref_axis',(0.0134844972654758,0.999690756780727,-0.0208939977188291));
#51696=DIRECTION('',(0.832683749197156,-6.06126260028676E-10,0.553748836407778));
#51697=DIRECTION('center_axis',(0.667548951037651,-0.601098528184639,0.439384748691613));
#51698=DIRECTION('ref_axis',(-0.531919783696298,0.0279220099678944,0.846334275018941));
#51699=DIRECTION('',(0.197236768219723,2.24206636476402E-10,0.980355882964059));
#51700=DIRECTION('center_axis',(0.,-1.,1.45983193964168E-32));
#51701=DIRECTION('ref_axis',(1.,0.,0.));
#51702=DIRECTION('center_axis',(-0.669420073431964,0.601098535677805,-0.436528711189015));
#51703=DIRECTION('ref_axis',(-0.52964128500097,0.0258666796488071,0.847827237181295));
#51704=DIRECTION('center_axis',(-0.71398511283608,-0.601098523128875,-0.359034572347476));
#51705=DIRECTION('ref_axis',(-0.46707442261457,0.0268944831968703,0.883808899317516));
#51706=DIRECTION('center_axis',(0.712444648251792,0.601098531545889,0.362081729103742));
#51707=DIRECTION('ref_axis',(-0.470846033187989,0.0268942988832825,0.8818053695225));
#51708=DIRECTION('center_axis',(-0.713631669633069,0.584827952222616,-0.385624307319729));
#51709=DIRECTION('ref_axis',(-0.477465331608741,-0.00326197145780636,0.878644533730202));
#51710=DIRECTION('center_axis',(0.895520951623367,-5.33044822369668E-10,
0.445019353740464));
#51711=DIRECTION('ref_axis',(0.44496462113546,-0.0156832196306143,-0.895410812174945));
#51712=DIRECTION('',(-0.895520920788556,8.32136531871802E-8,-0.445019415789929));
#51713=DIRECTION('center_axis',(-0.696200399396224,0.584827969931464,-0.416270644492716));
#51714=DIRECTION('ref_axis',(-0.508802432901024,0.00704480135282949,0.860854491216662));
#51715=DIRECTION('center_axis',(-0.86581078309822,4.76354188381577E-10,
-0.500371549821578));
#51716=DIRECTION('ref_axis',(0.500310101231311,0.0156715280534181,-0.865704456390509));
#51717=DIRECTION('',(0.865810815148979,-1.44328993199734E-11,0.500371494362999));
#51718=DIRECTION('',(-0.94790515691845,-3.07809289801676E-8,0.31855268557557));
#51719=DIRECTION('center_axis',(-0.260163910989382,0.79362626037384,0.54997463420029));
#51720=DIRECTION('ref_axis',(2.06655110892397E-16,-0.569588725712686,0.821929853175439));
#51721=DIRECTION('center_axis',(-0.308183870524933,0.471546674550742,-0.826236307401465));
#51722=DIRECTION('ref_axis',(0.765017150085957,-0.393413621124861,-0.509876929060126));
#51723=DIRECTION('center_axis',(0.717354637754989,-0.601098528042064,0.352254003919151));
#51724=DIRECTION('ref_axis',(-0.442306743760686,-0.00227572172927009,0.896860951047836));
#51725=DIRECTION('',(0.258404621837449,5.19500677922238E-12,0.966036775393693));
#51726=DIRECTION('center_axis',(0.,-1.,1.45983193964168E-32));
#51727=DIRECTION('ref_axis',(1.,0.,0.));
#51728=DIRECTION('center_axis',(-0.718853055774957,0.601098526949856,-0.349185974949911));
#51729=DIRECTION('ref_axis',(-0.43985491616893,-0.00432815365740093,0.898058416701242));
#51730=DIRECTION('center_axis',(-0.713985095789305,-0.60109852837797,-0.359034597459042));
#51731=DIRECTION('ref_axis',(-0.447034063521164,-0.00330175656877996,0.89451084088194));
#51732=DIRECTION('center_axis',(0.712444648108363,0.60109852759936,0.362081735937665));
#51733=DIRECTION('ref_axis',(-0.450851558771531,-0.00330192635974614,0.892592835079688));
#51734=DIRECTION('center_axis',(-0.756332493285849,0.584828255987547,-0.293150252598519));
#51735=DIRECTION('ref_axis',(-0.383336015959487,-0.033081541076345,0.92301631107382));
#51736=DIRECTION('center_axis',(0.921710028648617,-1.08128393816517E-7,
0.387879650263524));
#51737=DIRECTION('ref_axis',(0.387831992673483,-0.0156751635321966,-0.921596785317285));
#51738=DIRECTION('',(-0.921696815638291,3.88578058618578E-13,-0.38791104655866));
#51739=DIRECTION('center_axis',(-0.742882202695379,0.584827952226373,-0.3257334788031));
#51740=DIRECTION('ref_axis',(-0.416436997041045,-0.0227607295851117,0.908879627169732));
#51741=DIRECTION('center_axis',(-0.895520885907555,6.09172716946589E-10,
-0.445019485981622));
#51742=DIRECTION('ref_axis',(0.444964682358649,0.0156933905080377,-0.895410603548913));
#51743=DIRECTION('',(0.89552092136948,-2.16493489798338E-11,0.445019414620934));
#51744=DIRECTION('',(-0.926032600054708,0.,0.377443537017017));
#51745=DIRECTION('center_axis',(0.755847217242881,-0.601098527856549,0.259567994935592));
#51746=DIRECTION('ref_axis',(-0.347633110564671,-0.0324816893235681,0.937067852558084));
#51747=DIRECTION('',(0.318552670353073,8.15184858242943E-12,0.947905162034117));
#51748=DIRECTION('',(-0.944235193658598,7.77156117236542E-13,-0.329271770816312));
#51749=DIRECTION('center_axis',(-0.777849585318546,0.584827952146123,-0.230057142919619));
#51750=DIRECTION('ref_axis',(-0.319422936029011,-0.052656272845511,0.946148141079728));
#51751=DIRECTION('center_axis',(-0.921696780470485,6.71476112526404E-10,
-0.387911130119185));
#51752=DIRECTION('ref_axis',(0.387862873402704,0.0157729998154662,-0.921582120004842));
#51753=DIRECTION('',(0.921696815639179,-1.75748304775626E-10,0.38791104655655));
#51754=DIRECTION('',(0.377443536984304,6.72270837774768E-11,0.926032600068042));
#51755=DIRECTION('center_axis',(0.,-1.,1.45983193964168E-32));
#51756=DIRECTION('ref_axis',(1.,0.,0.));
#51757=DIRECTION('center_axis',(-0.756949309663079,0.601098517154981,-0.256336332334437));
#51758=DIRECTION('ref_axis',(-0.345057146162678,-0.0345386613841079,0.937945972192355));
#51759=DIRECTION('center_axis',(-0.713985090105492,-0.601098532579805,-0.359034601727267));
#51760=DIRECTION('ref_axis',(-0.42634375475666,-0.0335099233942814,0.903940312085982));
#51761=DIRECTION('center_axis',(0.712444636107614,0.601098522329735,0.362081768298954));
#51762=DIRECTION('ref_axis',(-0.430201741828989,-0.0335101101284208,0.902110599564424));
#51763=DIRECTION('',(-0.900505410468168,-1.43735365431037E-13,0.434844806474168));
#51764=DIRECTION('center_axis',(0.,-1.,1.45983193964168E-32));
#51765=DIRECTION('ref_axis',(1.,0.,0.));
#51766=DIRECTION('center_axis',(-0.722194785664401,0.601098542066865,-0.342221031329518));
#51767=DIRECTION('ref_axis',(-0.392334235304463,0.0514848370752,0.918380726800929));
#51768=DIRECTION('center_axis',(0.778394129727655,0.601098534684237,0.18106112339757));
#51769=DIRECTION('ref_axis',(-0.264543490688213,0.0525165188511361,0.962942758829544));
#51770=DIRECTION('center_axis',(-0.759133928885502,0.584827930050941,-0.285818071939465));
#51771=DIRECTION('ref_axis',(-0.337412268953248,0.0219594825745819,0.941100813879617));
#51772=DIRECTION('center_axis',(0.963048054265193,-1.01060003967696E-8,
0.269329621794607));
#51773=DIRECTION('ref_axis',(0.269296260339939,-0.0157391393484892,-0.962928763543541));
#51774=DIRECTION('',(-0.963047106750002,0.,-0.269333009823247));
#51775=DIRECTION('center_axis',(-0.745996129502959,0.584827952320933,-0.318537346241708));
#51776=DIRECTION('ref_axis',(-0.370977816810699,0.0322834330561264,0.928080405667784));
#51777=DIRECTION('center_axis',(-0.944235167368485,5.9634126920769E-10,
-0.329271846207066));
#51778=DIRECTION('ref_axis',(0.329231251851031,0.015702080083906,-0.944118757088133));
#51779=DIRECTION('',(0.944235193658916,-3.88578058618636E-13,0.3292717708154));
#51780=DIRECTION('',(-0.871424337428328,-1.64268989063966E-13,0.490529942141761));
#51781=DIRECTION('center_axis',(0.758320962041116,-0.601098528084844,0.252249634416525));
#51782=DIRECTION('ref_axis',(-0.298894250086174,0.0232723698954888,0.954002423511005));
#51783=DIRECTION('',(0.434844806474003,0.,0.900505410468248));
#51784=DIRECTION('center_axis',(0.,-1.,1.45983193964168E-32));
#51785=DIRECTION('ref_axis',(1.,0.,0.));
#51786=DIRECTION('center_axis',(-0.759391743085759,0.601098534241087,-0.249007495201229));
#51787=DIRECTION('ref_axis',(-0.296306257953441,0.021217969680861,0.954857266433183));
#51788=DIRECTION('center_axis',(-0.779160595905135,-0.601098524313,-0.177733873691787));
#51789=DIRECTION('ref_axis',(-0.238623290661855,0.0222453060519611,0.970857389894294));
#51790=DIRECTION('center_axis',(0.778394129827603,0.601098531103878,0.181061134854196));
#51791=DIRECTION('ref_axis',(-0.242768872812476,0.0222451269395338,0.96982907190948));
#51792=DIRECTION('center_axis',(-0.788970628195854,0.584827953016308,-0.188418717793627));
#51793=DIRECTION('ref_axis',(-0.237775337804514,-0.00784645567500136,0.971288485397253));
#51794=DIRECTION('center_axis',(0.978058403447699,-1.62597700528713E-9,
0.208330889321143));
#51795=DIRECTION('ref_axis',(0.208305284384794,-0.0156778483096643,-0.977938195168667));
#51796=DIRECTION('',(-0.978058312885179,0.,-0.208331314487758));
#51797=DIRECTION('center_axis',(-0.780037042689349,0.584827952253964,-0.222527477617686));
#51798=DIRECTION('ref_axis',(-0.272625222623443,0.00246180458055105,0.962117158930099));
#51799=DIRECTION('center_axis',(-0.9630470847767,6.1993888346627E-10,-0.269333088392605));
#51800=DIRECTION('ref_axis',(0.269300016023813,0.0156707406182653,-0.96292882876049));
#51801=DIRECTION('',(0.963047106750167,-6.41708908203662E-11,0.269333009822659));
#51802=DIRECTION('',(-0.838904150644707,0.,0.544279180229304));
#51803=DIRECTION('center_axis',(0.783956637020661,-0.601098528036003,0.155217753057459));
#51804=DIRECTION('ref_axis',(-0.199320627528099,-0.00691952505566824,0.979909897702237));
#51805=DIRECTION('',(0.490529942130914,2.35931335548666E-11,0.871424337434434));
#51806=DIRECTION('center_axis',(0.,-1.,1.45983193964168E-32));
#51807=DIRECTION('ref_axis',(1.,0.,0.));
#51808=DIRECTION('center_axis',(-0.784612638143514,0.60109852542789,-0.151866950960011));
#51809=DIRECTION('ref_axis',(-0.196643148413631,-0.00897218324522628,0.980434073311301));
#51810=DIRECTION('center_axis',(-0.779160598291669,-0.601098529343444,-0.177733846216521));
#51811=DIRECTION('ref_axis',(-0.216559054708591,-0.00794563115865621,0.976237185713192));
#51812=DIRECTION('center_axis',(0.778394127547434,0.601098526761477,0.181061159072981));
#51813=DIRECTION('ref_axis',(-0.220727860741832,-0.00794584115531741,0.975303068333464));
#51814=DIRECTION('center_axis',(-0.806374762979318,0.584825719450409,-0.0879694236616418));
#51815=DIRECTION('ref_axis',(-0.121467043420276,-0.0182013008530597,0.992428571742064));
#51816=DIRECTION('center_axis',(0.989209578813874,-4.87840080647454E-10,
0.146507369039505));
#51817=DIRECTION('ref_axis',(0.146489358731641,-0.01567950661673,-0.989087974272586));
#51818=DIRECTION('',(-0.989209569218337,2.06171160587046E-7,-0.146507433827873));
#51819=DIRECTION('center_axis',(-0.801777367483258,0.584827782536624,-0.123002104717406));
#51820=DIRECTION('ref_axis',(-0.171045908405215,-0.0273551074118827,0.984883239433142));
#51821=DIRECTION('center_axis',(-0.978058291785313,6.8004977939135E-10,
-0.20833141354581));
#51822=DIRECTION('ref_axis',(0.208305728553097,0.0157023279262274,-0.977937707806413));
#51823=DIRECTION('',(-0.97805831261045,-1.29267420804535E-5,-0.20833131537649));
#51824=DIRECTION('',(-0.803073168768253,-7.62642219063171E-8,0.595880428949056));
#51825=DIRECTION('center_axis',(0.989209569691421,2.03930294082373E-12,
0.146507430633788));
#51826=DIRECTION('ref_axis',(0.113085605681508,-0.635772805085229,-0.763547369913423));
#51827=DIRECTION('',(-0.544279180228737,0.,-0.838904150645075));
#51828=DIRECTION('center_axis',(-0.913641051314188,0.398564391558955,-0.0800403344242509));
#51829=DIRECTION('ref_axis',(-0.399847251243964,-0.916581788861554,-6.67217341138553E-17));
#51830=DIRECTION('center_axis',(0.997020848376458,5.74456518849634E-5,0.077132513265712));
#51831=DIRECTION('ref_axis',(0.077132529104784,-0.000363102228566342,-0.997020782687438));
#51832=DIRECTION('',(-0.996456789590132,5.94973691223711E-5,-0.0841062598133456));
#51833=DIRECTION('center_axis',(-0.796254114841391,0.590180063812382,-0.132916804342285));
#51834=DIRECTION('ref_axis',(0.601501199445676,0.795822082110392,-0.0697389467291665));
#51835=DIRECTION('center_axis',(-0.413785045848131,0.550037558019381,0.72542444168951));
#51836=DIRECTION('ref_axis',(3.87855366211629E-16,-0.796841686270309,0.604188155314129));
#51837=DIRECTION('center_axis',(-0.566971886742689,-0.477126089856525,-0.671486093691938));
#51838=DIRECTION('ref_axis',(0.793527238897196,-0.0976199624324114,-0.600653697285622));
#51839=DIRECTION('center_axis',(-0.595310741375292,0.584827951390672,-0.550982203410772));
#51840=DIRECTION('ref_axis',(-0.664842645381441,0.0265489689884084,0.746511492964348));
#51841=DIRECTION('center_axis',(0.796270460755438,-3.00458614992124E-11,
0.60494078497678));
#51842=DIRECTION('ref_axis',(0.604865770037167,-0.0157477670566697,-0.796171720214976));
#51843=DIRECTION('center_axis',(-0.762632744771221,-0.000115441241507041,
-0.646831727171784));
#51844=DIRECTION('ref_axis',(0.0160163222934664,0.99969000865124,-0.0190621096176581));
#51845=DIRECTION('',(0.756714656875199,-6.07736083413749E-10,0.653745308258691));
#51846=DIRECTION('center_axis',(0.607215616380602,-0.601098528161896,0.519586137868524));
#51847=DIRECTION('ref_axis',(-0.633799249129408,0.0279220104056515,0.772993449608666));
#51848=DIRECTION('',(0.0728103245348834,2.24206636476344E-10,0.997345805947528));
#51849=DIRECTION('center_axis',(0.,-1.,1.45983193964168E-32));
#51850=DIRECTION('ref_axis',(1.,0.,0.));
#51851=DIRECTION('center_axis',(-0.609429936565619,0.601098535479941,-0.516987140131643));
#51852=DIRECTION('ref_axis',(-0.631725838972641,0.0258666841461149,0.774760207435564));
#51853=DIRECTION('center_axis',(-0.66335616311592,-0.601098523127959,-0.44568954031872));
#51854=DIRECTION('ref_axis',(-0.574162028410077,0.0268944832644721,0.818299854516645));
#51855=DIRECTION('center_axis',(0.661445936087663,0.601098531516931,0.44851959716528));
#51856=DIRECTION('ref_axis',(-0.577652789222863,0.0268942995145629,0.815839415422341));
#51857=DIRECTION('center_axis',(-0.659672929381783,0.584827952222579,-0.472025309215514));
#51858=DIRECTION('ref_axis',(-0.583823735431116,-0.00326197144977297,0.81187388521218));
#51859=DIRECTION('center_axis',(0.832683801792781,-7.44626053212263E-10,
0.553748757318625));
#51860=DIRECTION('ref_axis',(0.553680652163339,-0.015683219631694,-0.832581390641157));
#51861=DIRECTION('',(-0.832683748468971,8.32144303432563E-8,-0.553748837502758));
#51862=DIRECTION('center_axis',(-0.638538105377738,0.584827969931015,-0.500245273407933));
#51863=DIRECTION('ref_axis',(-0.61268405077085,0.00704480136482595,0.790296542257875));
#51864=DIRECTION('center_axis',(-0.796270418241213,5.26330196580228E-10,
-0.60494084093733));
#51865=DIRECTION('ref_axis',(0.604866550617452,0.0156715280534126,-0.796172631501873));
#51866=DIRECTION('',(0.796270460894481,-1.40443212613737E-11,0.604940784793761));
#51867=DIRECTION('',(-0.980355879774395,-3.07807852448036E-8,0.19723678407379));
#51868=DIRECTION('center_axis',(-0.327042540108679,0.793626260381241,0.513030735719167));
#51869=DIRECTION('ref_axis',(-9.03584097610045E-18,-0.542884142424063,0.839807601718685));
#51870=DIRECTION('center_axis',(-0.202198880525624,0.471546674565983,-0.858346868357978));
#51871=DIRECTION('ref_axis',(0.822883322106636,-0.393422484402515,-0.409977788380418));
#51872=DIRECTION('center_axis',(0.667548955300865,-0.601098528008301,0.439384742455831));
#51873=DIRECTION('ref_axis',(-0.551225498185787,-0.00227572877616902,0.83435320530838));
#51874=DIRECTION('',(0.135290511410413,5.05127141378944E-12,0.990805973701365));
#51875=DIRECTION('center_axis',(0.,-1.,1.45983193964168E-32));
#51876=DIRECTION('ref_axis',(1.,0.,0.));
#51877=DIRECTION('center_axis',(-0.669420074346758,0.601098526972795,-0.436528721772939));
#51878=DIRECTION('ref_axis',(-0.54894309775187,-0.00432815035528203,0.835848516505882));
#51879=DIRECTION('center_axis',(-0.663356142061132,-0.601098528374394,-0.445689564580449));
#51880=DIRECTION('ref_axis',(-0.555621003655155,-0.00330175758509039,0.83142913028958));
#51881=DIRECTION('center_axis',(0.661445935961308,0.601098527608529,0.448519602589595));
#51882=DIRECTION('ref_axis',(-0.559168004095893,-0.00330192476536948,0.82904779143802));
#51883=DIRECTION('center_axis',(-0.713627116581051,0.584828255988157,-0.385632272350314));
#51884=DIRECTION('ref_axis',(-0.495997915892786,-0.0330815410631934,0.867693309338557));
#51885=DIRECTION('center_axis',(0.865827858828577,-1.0812546324535E-7,0.500342001911003));
#51886=DIRECTION('ref_axis',(0.500280526962411,-0.0156751635318979,-0.865721481534599));
#51887=DIRECTION('',(-0.865810815149254,3.88578058618869E-13,-0.500371494362523));
#51888=DIRECTION('center_axis',(-0.696199124466262,0.584827952226206,-0.416272801642521));
#51889=DIRECTION('ref_axis',(-0.527066089522084,-0.0227607295921243,0.84951944442981));
#51890=DIRECTION('center_axis',(-0.832683715238848,4.65217159593631E-10,
-0.553748887471596));
#51891=DIRECTION('ref_axis',(0.553680693946936,0.0156933905093404,-0.832581171204802));
#51892=DIRECTION('',(0.832683749192512,-2.28705943069147E-11,0.553748836414761));
#51893=DIRECTION('',(-0.966036775393065,0.,0.258404621839796));
#51894=DIRECTION('center_axis',(0.717354638086269,-0.601098527996424,0.35225400332239));
#51895=DIRECTION('ref_axis',(-0.462337666708267,-0.0324816867803975,0.886108809326855));
#51896=DIRECTION('',(0.197236768330282,8.15184858243042E-12,0.980355882941816));
#51897=DIRECTION('center_axis',(0.,-1.,1.45983193964168E-32));
#51898=DIRECTION('ref_axis',(1.,0.,0.));
#51899=DIRECTION('center_axis',(-0.718853072762017,0.601098517458356,-0.349185956318367));
#51900=DIRECTION('ref_axis',(-0.459892075508836,-0.0345386560330738,0.887302857046907));
#51901=DIRECTION('center_axis',(-0.663356131866617,-0.601098532278994,-0.445689574487668));
#51902=DIRECTION('ref_axis',(-0.536275675289761,-0.0335099289335965,0.84337742722661));
#51903=DIRECTION('center_axis',(0.661445920052673,0.601098522425337,0.448519632996985));
#51904=DIRECTION('ref_axis',(-0.539873909196622,-0.0335101084212974,0.841078613925209));
#51905=DIRECTION('',(-0.895520921369859,8.32667268468674E-13,-0.44501941462017));
#51906=DIRECTION('center_axis',(-0.742882203369472,0.584827952147132,-0.325733477408004));
#51907=DIRECTION('ref_axis',(-0.435487996740383,-0.0526562728318949,0.898653170932202));
#51908=DIRECTION('center_axis',(-0.865810776031052,5.73356427121151E-10,
-0.50037156205015));
#51909=DIRECTION('ref_axis',(0.500309315085384,0.015772999814506,-0.865703067867757));
#51910=DIRECTION('',(0.865810815150186,-1.7652546089277E-10,0.50037149436091));
#51911=DIRECTION('',(-0.947905162032818,-1.43735365431086E-13,0.31855267035694));
#51912=DIRECTION('',(0.258404621807034,6.51326541667456E-11,0.966036775401829));
#51913=DIRECTION('center_axis',(-0.717325427945312,0.584827930050931,-0.378709021090623));
#51914=DIRECTION('ref_axis',(-0.452702880547943,0.0219594825762896,0.891390982155741));
#51915=DIRECTION('center_axis',(0.921698179088528,-1.00810072301223E-8,
0.38790780691408));
#51916=DIRECTION('ref_axis',(0.387859757432562,-0.0157391393497043,-0.921584010308819));
#51917=DIRECTION('',(-0.921696815638489,1.60982338570588E-12,-0.387911046558189));
#51918=DIRECTION('center_axis',(-0.700190411576892,0.584827952319919,-0.409523691281803));
#51919=DIRECTION('ref_axis',(-0.484371864185748,0.0322834330701548,0.874266365093858));
#51920=DIRECTION('center_axis',(-0.895520892717308,4.74561357526579E-10,
-0.445019472278231));
#51921=DIRECTION('ref_axis',(0.444964607943966,0.0157020800824926,-0.895410488188716));
#51922=DIRECTION('',(0.895520921369544,0.,0.445019414620803));
#51923=DIRECTION('center_axis',(0.720726111367983,-0.601098528029885,0.345303391226748));
#51924=DIRECTION('ref_axis',(-0.416105590020171,0.0232723713891031,0.90901844573358));
#51925=DIRECTION('',(0.318552670357153,0.,0.947905162032746));
#51926=DIRECTION('center_axis',(0.,-1.,1.45983193964168E-32));
#51927=DIRECTION('ref_axis',(1.,0.,0.));
#51928=DIRECTION('center_axis',(-0.673608395900761,0.601098542100637,-0.430037523544739));
#51929=DIRECTION('ref_axis',(-0.504344188395324,0.0514848367856261,0.861966502372928));
#51930=DIRECTION('center_axis',(0.749563254147552,0.601098538699542,0.277192126159831));
#51931=DIRECTION('ref_axis',(-0.3831462732819,0.0525164728782138,0.922193555251078));
#51932=DIRECTION('',(-0.926032600054682,-1.64268989064055E-13,0.377443537017083));
#51933=DIRECTION('center_axis',(0.,-1.,1.45983193964168E-32));
#51934=DIRECTION('ref_axis',(1.,0.,0.));
#51935=DIRECTION('center_axis',(-0.722194799748368,0.601098534343069,-0.342221015174447));
#51936=DIRECTION('ref_axis',(-0.413645140020028,0.0212179668797318,0.910190911852729));
#51937=DIRECTION('center_axis',(-0.750740720407566,-0.601098524335125,-0.27398710693035));
#51938=DIRECTION('ref_axis',(-0.358422371524481,0.0222453054265748,0.933294460487817));
#51939=DIRECTION('center_axis',(0.749563276968541,0.601098531420702,0.277192080233288));
#51940=DIRECTION('ref_axis',(-0.362406391970458,0.0222451184080069,0.931754668228697));
#51941=DIRECTION('center_axis',(-0.759134231971544,0.584827953016391,-0.285817219949449));
#51942=DIRECTION('ref_axis',(-0.35763513484838,-0.00784645567247245,0.933828433629733));
#51943=DIRECTION('center_axis',(0.94423530926095,-9.70178035548998E-10,
0.329271439309392));
#51944=DIRECTION('ref_axis',(0.32923097018331,-0.0156778483086887,-0.944119258009583));
#51945=DIRECTION('',(-0.944235193658824,3.88578058618818E-13,-0.329271770815664));
#51946=DIRECTION('center_axis',(-0.74599612929426,0.58482795225407,-0.318537346853226));
#51947=DIRECTION('ref_axis',(-0.391060745912263,0.00246180458148873,0.920361577058032));
#51948=DIRECTION('center_axis',(-0.921696791818101,4.61753290138909E-10,
-0.387911103156664));
#51949=DIRECTION('ref_axis',(0.387863470164475,0.015670740618503,-0.921583613352819));
#51950=DIRECTION('',(0.92169681563878,-6.42264019716333E-11,0.387911046557498));
#51951=DIRECTION('',(-0.90050541046819,0.,0.434844806474122));
#51952=DIRECTION('center_axis',(0.758320961992543,-0.601098528033327,0.252249634685309));
#51953=DIRECTION('ref_axis',(-0.320564200670215,-0.00691952525868305,0.947201516795059));
#51954=DIRECTION('',(0.3774435370056,2.35931335548606E-11,0.926032600059362));
#51955=DIRECTION('center_axis',(0.,-1.,1.45983193964168E-32));
#51956=DIRECTION('ref_axis',(1.,0.,0.));
#51957=DIRECTION('center_axis',(-0.759391757226185,0.601098525421464,-0.249007473367908));
#51958=DIRECTION('ref_axis',(-0.317973530880616,-0.00897218348452268,0.94805713624382));
#51959=DIRECTION('center_axis',(-0.750740714555744,-0.601098529097443,-0.273987112516669));
#51960=DIRECTION('ref_axis',(-0.337206411814674,-0.00794565257757915,0.941397207578283));
#51961=DIRECTION('center_axis',(0.749563277928319,0.601098526787934,0.277192087684207));
#51962=DIRECTION('ref_axis',(-0.341225240450696,-0.00794583919521706,0.939947976708737));
#51963=DIRECTION('center_axis',(-0.788970653144117,0.584827952229847,-0.18841861576816));
#51964=DIRECTION('ref_axis',(-0.244956601238545,-0.0181546317064356,0.969364055892967));
#51965=DIRECTION('center_axis',(0.963047096323551,3.03853506791505E-10,
0.269333047104838));
#51966=DIRECTION('ref_axis',(0.26929993772326,-0.0156795066156373,-0.962928707960531));
#51967=DIRECTION('',(-0.963047105879734,2.06171549165051E-7,-0.269333012934965));
#51968=DIRECTION('center_axis',(-0.780038861941738,0.584827782536567,-0.222521546448878));
#51969=DIRECTION('ref_axis',(-0.293135761410684,-0.0273551074116156,0.955679404131259));
#51970=DIRECTION('center_axis',(-0.944235164423757,5.82024366209817E-10,
-0.329271854651504));
#51971=DIRECTION('ref_axis',(0.329231259012644,0.0157023279254938,-0.944118750468748));
#51972=DIRECTION('',(-0.944235193274803,-1.29267418160562E-5,-0.329271771663157));
#51973=DIRECTION('',(-0.871424317944096,-7.62629077544537E-8,0.490529976755408));
#51974=DIRECTION('center_axis',(0.963047106749398,1.61336649447084E-12,
0.269333009825408));
#51975=DIRECTION('ref_axis',(0.20789175275403,-0.635772805084664,-0.74335318621207));
#51976=DIRECTION('',(-0.434844806473195,0.,-0.900505410468638));
#51977=DIRECTION('center_axis',(-0.896405004805104,0.39856439155694,-0.193918779758972));
#51978=DIRECTION('ref_axis',(-0.40627649968951,-0.91375018785226,2.11715934575633E-16));
#51979=DIRECTION('center_axis',(0.979491773889296,5.74456562550402E-5,0.201484147225525));
#51980=DIRECTION('ref_axis',(0.201484154709456,-0.00036293807059144,-0.979491706793362));
#51981=DIRECTION('',(-0.978058120671607,5.94973691578955E-5,-0.20833220837976));
#51982=DIRECTION('center_axis',(-0.773316520430496,0.590180063812117,-0.231665818600838));
#51983=DIRECTION('ref_axis',(0.605499692316029,0.795821432315522,0.00619439040305992));
#51984=DIRECTION('center_axis',(-0.501442018156305,0.550037558016864,0.667843235496308));
#51985=DIRECTION('ref_axis',(-5.60351980611002E-16,-0.771902436601816,0.635741007304216));
#51986=DIRECTION('center_axis',(-0.478341620775355,-0.477126089438627,-0.737251645376943));
#51987=DIRECTION('ref_axis',(0.862552725675641,-0.0976242841602588,-0.496459761281536));
#51988=DIRECTION('center_axis',(-0.521560157177763,0.58482795139038,-0.621249764359906));
#51989=DIRECTION('ref_axis',(-0.753162861850607,0.0265489689898624,0.657298148312148));
#51990=DIRECTION('center_axis',(0.714172443316223,9.09561476418819E-12,
0.699969800211221));
#51991=DIRECTION('ref_axis',(0.699883001315757,-0.0157477670549617,-0.714083883239238));
#51992=DIRECTION('center_axis',(-0.675549637427138,-0.000115441124074375,
-0.73731450144793));
#51993=DIRECTION('ref_axis',(0.0187140380375274,0.999675144775611,-0.0173028812106884));
#51994=DIRECTION('',(0.668811722374505,-6.06625860390613E-10,0.743431826070453));
#51995=DIRECTION('center_axis',(0.53730612122198,-0.601098527862433,0.591593350113916));
#51996=DIRECTION('ref_axis',(-0.725683327143529,0.0279220169301707,0.687462049626341));
#51997=DIRECTION('',(-0.0527643814626423,2.24206636476439E-10,0.998606989785704));
#51998=DIRECTION('center_axis',(0.,-1.,1.45983193964168E-32));
#51999=DIRECTION('ref_axis',(1.,0.,0.));
#52000=DIRECTION('center_axis',(-0.53982872696825,0.60109853538561,-0.589292369114953));
#52001=DIRECTION('ref_axis',(-0.723847695975665,0.0258666862474939,0.689474747596527));
#52002=DIRECTION('center_axis',(-0.602265686714187,-0.601098523280458,-0.525315722129789));
#52003=DIRECTION('ref_axis',(-0.672194759395683,0.0268944799871021,0.739885729276625));
#52004=DIRECTION('center_axis',(0.600015829518251,0.601098531375124,0.52788404020788));
#52005=DIRECTION('ref_axis',(-0.675349613221344,0.0268943027491544,0.737007188839714));
#52006=DIRECTION('center_axis',(-0.595310752991289,0.584827952222906,-0.550982189976869));
#52007=DIRECTION('ref_axis',(-0.68097489015979,-0.00326197146842053,0.732299500555613));
#52008=DIRECTION('center_axis',(0.756714686154918,-3.50932338498322E-10,
0.653745274367214));
#52009=DIRECTION('ref_axis',(0.653664870720632,-0.0156832196319518,-0.756621618385145));
#52010=DIRECTION('',(-0.756714656015473,8.32132090980655E-8,-0.653745309253824));
#52011=DIRECTION('center_axis',(-0.570805683990802,0.584827969930714,-0.576330735524762));
#52012=DIRECTION('ref_axis',(-0.706903275156747,0.00704480137507825,0.707275144725339));
#52013=DIRECTION('center_axis',(-0.714172407611761,4.01813307213759E-10,
-0.699969836640137));
#52014=DIRECTION('ref_axis',(0.699883876193368,0.0156715280549141,-0.714084702996059));
#52015=DIRECTION('',(0.714172445802828,-1.60427227056679E-11,0.699969797674162));
#52016=DIRECTION('',(-0.997345804770054,-3.07807852448081E-8,0.0728103406637648));
#52017=DIRECTION('center_axis',(-0.38876351302317,0.793626260381023,0.467996036068166));
#52018=DIRECTION('ref_axis',(5.14608281189496E-16,-0.507952836951219,0.861384882287359));
#52019=DIRECTION('center_axis',(-0.0930250935211342,0.471546674525771,-0.876920786456263));
#52020=DIRECTION('ref_axis',(0.867779998855256,-0.393420034062469,-0.303609206686916));
#52021=DIRECTION('center_axis',(0.607215617952052,-0.601098528024132,0.51958613619142));
#52022=DIRECTION('ref_axis',(-0.651451109280604,-0.0022757251850946,0.7586872038541));
#52023=DIRECTION('',(0.0100427887997458,5.05127141378811E-12,0.999949569924966));
#52024=DIRECTION('center_axis',(0.,-1.,1.45983193964168E-32));
#52025=DIRECTION('ref_axis',(1.,0.,0.));
#52026=DIRECTION('center_axis',(-0.609429937620773,0.601098526993246,-0.516987148755257));
#52027=DIRECTION('ref_axis',(-0.64937411786308,-0.00432814735280087,0.760456785221908));
#52028=DIRECTION('center_axis',(-0.602265662641906,-0.601098528361773,-0.525315743913902));
#52029=DIRECTION('ref_axis',(-0.655445470963613,-0.00330176107082695,0.75523528318473));
#52030=DIRECTION('center_axis',(0.600015828005484,0.601098527623849,0.527884046198912));
#52031=DIRECTION('ref_axis',(-0.658666035184986,-0.00330192209803078,0.752428170262218));
#52032=DIRECTION('center_axis',(-0.659667413965905,0.584828255987831,-0.472032640767318));
#52033=DIRECTION('ref_axis',(-0.600837632369412,-0.0330815410726327,0.798686265794635));
#52034=DIRECTION('center_axis',(0.796291065774804,-1.08116165302368E-7,
0.604913662076842));
#52035=DIRECTION('ref_axis',(0.604839339266343,-0.0156751635312651,-0.796193232151669));
#52036=DIRECTION('',(-0.796270460894816,0.,-0.604940784793319));
#52037=DIRECTION('center_axis',(-0.638536570136217,0.584827952226412,-0.500247253758917));
#52038=DIRECTION('ref_axis',(-0.629383034939896,-0.0227607295784563,0.776761832558026));
#52039=DIRECTION('center_axis',(-0.756714605335634,6.02210338294383E-10,
-0.653745367916084));
#52040=DIRECTION('ref_axis',(0.653664859942376,0.0156933905078516,-0.756621416806901));
#52041=DIRECTION('',(0.756714656868826,-2.2482016248314E-11,0.653745308266067));
#52042=DIRECTION('',(-0.990805973701014,0.,0.13529051141298));
#52043=DIRECTION('center_axis',(0.667548949926352,-0.601098527953579,0.439384750696091));
#52044=DIRECTION('ref_axis',(-0.569750877659947,-0.0324816875124569,0.82117530246718));
#52045=DIRECTION('',(0.0728103246472944,8.15184858242776E-12,0.997345805939322));
#52046=DIRECTION('center_axis',(0.,-1.,1.45983193964168E-32));
#52047=DIRECTION('ref_axis',(1.,0.,0.));
#52048=DIRECTION('center_axis',(-0.669420094475072,0.601098517583778,-0.436528703834663));
#52049=DIRECTION('ref_axis',(-0.567474227812613,-0.0345386538450982,0.822666446476971));
#52050=DIRECTION('center_axis',(-0.602265649429205,-0.601098531988501,-0.525315754912117));
#52051=DIRECTION('ref_axis',(-0.637750206829724,-0.0335099342688502,0.769513975177801));
#52052=DIRECTION('center_axis',(0.600015812540529,0.60109852279929,0.527884069270744));
#52053=DIRECTION('ref_axis',(-0.641031937936639,-0.0335101017961318,0.766782320885667));
#52054=DIRECTION('',(-0.832683749192486,0.,-0.5537488364148));
#52055=DIRECTION('center_axis',(-0.696199125313164,0.58482795214638,-0.416272800338259));
#52056=DIRECTION('ref_axis',(-0.544685151566205,-0.0526562728418925,0.836985903461761));
#52057=DIRECTION('center_axis',(-0.796270413842743,5.69899567997189E-10,
-0.60494084672694));
#52058=DIRECTION('ref_axis',(0.604865591185688,0.0157729998149048,-0.796171356603858));
#52059=DIRECTION('',(0.796270460896058,-1.76914038951424E-10,0.604940784791685));
#52060=DIRECTION('',(-0.980355882940996,0.,0.197236768334354));
#52061=DIRECTION('',(0.135290511377995,6.7370819142914E-11,0.990805973705791));
#52062=DIRECTION('center_axis',(0.,-1.,1.45983193964168E-32));
#52063=DIRECTION('ref_axis',(1.,0.,0.));
#52064=DIRECTION('center_axis',(-0.614398793752247,0.601098541642861,-0.511072074633911));
#52065=DIRECTION('ref_axis',(-0.608400338225441,0.051484842085893,0.791958546568291));
#52066=DIRECTION('center_axis',(0.708911344827112,0.601098538035799,0.368951558807712));
#52067=DIRECTION('ref_axis',(-0.495706541700321,0.0525164805429546,0.866900826961706));
#52068=DIRECTION('center_axis',(-0.664203715286355,0.584827908067513,-0.465628330909084));
#52069=DIRECTION('ref_axis',(-0.56085476194302,0.0219600677391468,0.82762291620685));
#52070=DIRECTION('center_axis',(0.865814280566785,-1.94983737445407E-8,
0.500365497977848));
#52071=DIRECTION('ref_axis',(0.500303518481015,-0.0157391387106383,-0.865707034110365));
#52072=DIRECTION('',(-0.865810815149096,3.88578058618736E-13,-0.500371494362796));
#52073=DIRECTION('center_axis',(-0.643342272598766,0.584827952320221,-0.494051603046071));
#52074=DIRECTION('ref_axis',(-0.590127077891625,0.032283433066789,0.806664621691391));
#52075=DIRECTION('center_axis',(-0.832683710697438,5.14805201568008E-10,
-0.553748894300607));
#52076=DIRECTION('ref_axis',(0.553680625231442,0.0157020800817568,-0.832581053065961));
#52077=DIRECTION('',(0.832683749192297,-7.77156117237866E-13,0.553748836415085));
#52078=DIRECTION('',(-0.966036775393088,0.,0.258404621839711));
#52079=DIRECTION('center_axis',(0.671764979831684,-0.601098528016402,0.432911505377545));
#52080=DIRECTION('ref_axis',(-0.526754694709403,0.0232723717226879,0.849698704433521));
#52081=DIRECTION('',(0.197236768334356,1.43735365432692E-13,0.980355882940996));
#52082=DIRECTION('center_axis',(-0.717325835416885,0.584827953016236,-0.378708213819436));
#52083=DIRECTION('ref_axis',(-0.471854812183757,-0.00784645566122617,0.881641349615924));
#52084=DIRECTION('center_axis',(0.895521109945517,-1.54028260138715E-9,
0.445019035145632));
#52085=DIRECTION('ref_axis',(0.444964340052093,-0.0156778483093563,-0.895411045919356));
#52086=DIRECTION('',(-0.895520921369635,3.88578058618527E-13,-0.445019414620621));
#52087=DIRECTION('center_axis',(-0.7001904113086,0.584827952254159,-0.40952369183443));
#52088=DIRECTION('ref_axis',(-0.503329007621636,0.00246180457671532,0.864091343322478));
#52089=DIRECTION('center_axis',(-0.865810778099468,5.60508848932578E-10,
-0.500371558471097));
#52090=DIRECTION('ref_axis',(0.500310116056249,0.0156707406188733,-0.865704462077122));
#52091=DIRECTION('',(0.865810815149366,-6.46149800302453E-11,0.50037149436233));
#52092=DIRECTION('center_axis',(0.720726110244692,-0.60109852806954,0.345303393502279));
#52093=DIRECTION('ref_axis',(-0.436752288568508,-0.00691952239342252,0.899555200440761));
#52094=DIRECTION('',(0.258404621828094,2.35931335548689E-11,0.966036775396196));
#52095=DIRECTION('center_axis',(0.,-1.,1.45983193964168E-32));
#52096=DIRECTION('ref_axis',(1.,0.,0.));
#52097=DIRECTION('center_axis',(-0.673608405718115,0.601098534097765,-0.430037519353157));
#52098=DIRECTION('ref_axis',(-0.524460602283865,0.0212179736208634,0.851170296854554));
#52099=DIRECTION('center_axis',(-0.710481210982187,-0.601098524559535,-0.365919407265637));
#52100=DIRECTION('ref_axis',(-0.472568923490101,0.0222452996576803,0.881012916587803));
#52101=DIRECTION('center_axis',(0.708911378994718,0.601098530857045,0.368951504853022));
#52102=DIRECTION('ref_axis',(-0.476328516796978,0.0222451336537348,0.878985948758408));
#52103=DIRECTION('',(-0.947905162032792,1.64268989064054E-13,0.318552670357018));
#52104=DIRECTION('center_axis',(0.,-1.,1.45983193964168E-32));
#52105=DIRECTION('ref_axis',(1.,0.,0.));
#52106=DIRECTION('center_axis',(-0.722194816033392,0.601098525392591,-0.342220996529068));
#52107=DIRECTION('ref_axis',(-0.434289278687137,-0.00897218548941485,0.900728772886128));
#52108=DIRECTION('center_axis',(-0.710481209891288,-0.601098529111296,-0.365919401906551));
#52109=DIRECTION('ref_axis',(-0.452535793264877,-0.00794565142206212,0.891710840148087));
#52110=DIRECTION('center_axis',(0.708911366633865,0.601098526781341,0.368951535243596));
#52111=DIRECTION('ref_axis',(-0.456341297275093,-0.0079458395878439,0.889769343164019));
#52112=DIRECTION('center_axis',(-0.759134269503231,0.584827952230624,-0.285817121872591));
#52113=DIRECTION('ref_axis',(-0.364518576916482,-0.018154631692394,0.931019127854469));
#52114=DIRECTION('center_axis',(0.92169678288755,6.8097117849751E-10,0.387911124376114));
#52115=DIRECTION('ref_axis',(0.387863438075824,-0.0156795066142625,-0.921583477757894));
#52116=DIRECTION('',(-0.921696815638345,1.99840144432174E-12,-0.387911046558531));
#52117=DIRECTION('center_axis',(-0.745996131539549,0.58482795217557,-0.318537341739014));
#52118=DIRECTION('ref_axis',(-0.410607314150629,-0.0273514813181276,0.911401958542832));
#52119=DIRECTION('center_axis',(-0.895520883366674,5.55358532199175E-10,
-0.445019491094685));
#52120=DIRECTION('ref_axis',(0.444964625027153,0.0157023279249333,-0.895410475353166));
#52121=DIRECTION('',(-0.895520920882602,-1.29267412633629E-5,-0.445019415412942));
#52122=DIRECTION('',(-0.926032600054565,-7.39210450788166E-13,0.37744353701737));
#52123=DIRECTION('center_axis',(0.921696815868328,-4.81892124678041E-10,
0.38791104601208));
#52124=DIRECTION('ref_axis',(0.299419321991596,-0.635772805082133,-0.711435879005332));
#52125=DIRECTION('',(-0.318552670356402,0.,-0.947905162032999));
#52126=DIRECTION('center_axis',(-0.865032115883027,0.398564391556874,-0.304739010095249));
#52127=DIRECTION('ref_axis',(-0.418468469414644,-0.908231325217186,1.44167877428543E-16));
#52128=DIRECTION('center_axis',(0.946515529011113,5.74456512495677E-5,0.322658255807611));
#52129=DIRECTION('ref_axis',(0.322658254835461,-0.000362742142822936,-0.946515461577185));
#52130=DIRECTION('',(-0.944234890926654,5.94973683762808E-5,-0.329272633567979));
#52131=DIRECTION('center_axis',(-0.73818326258567,0.590180063815931,-0.326761324383104));
#52132=DIRECTION('ref_axis',(0.599952266514969,0.795819902379834,0.0820241481498212));
#52133=DIRECTION('center_axis',(-0.581190950296166,0.550037558009473,0.599729742528095));
#52134=DIRECTION('ref_axis',(0.718118878862159,-2.4451179902057E-16,0.695920452222634));
#52135=DIRECTION('center_axis',(-0.382167621418612,-0.477126090026257,-0.791390297739047));
#52136=DIRECTION('ref_axis',(0.917972909631245,-0.0976141048661876,-0.384444044971853));
#52137=DIRECTION('center_axis',(-0.439584257727902,0.584827951390055,-0.681719845413584));
#52138=DIRECTION('ref_axis',(-0.829605250075042,0.0265489689967324,0.557718819202955));
#52139=DIRECTION('center_axis',(0.62081150436806,-2.72556222406521E-11,
0.783959868899082));
#52140=DIRECTION('ref_axis',(0.783862654917877,-0.0157477670581149,-0.620734521400076));
#52141=DIRECTION('center_axis',(-0.577812718057188,-0.000115441154269082,
-0.816169375512647));
#52142=DIRECTION('ref_axis',(0.0202289007957235,0.999690764743852,-0.0144625882347842));
#52143=DIRECTION('',(0.570361227482597,-6.06126260028481E-10,0.821393979880876));
#52144=DIRECTION('center_axis',(0.458923006270181,-0.601098528268336,0.6542707647676));
#52145=DIRECTION('ref_axis',(-0.806122932258831,0.0279220081159775,0.591088977692188));
#52146=DIRECTION('',(-0.177506961644612,2.24206636476395E-10,0.98411954485606));
#52147=DIRECTION('center_axis',(0.,-1.,1.45983193964168E-32));
#52148=DIRECTION('ref_axis',(1.,0.,0.));
#52149=DIRECTION('center_axis',(-0.461714093721715,0.601098535245096,-0.652304105908383));
#52150=DIRECTION('ref_axis',(-0.804554042774789,0.0258666894925332,0.593315857389165));
#52151=DIRECTION('center_axis',(-0.531677123659475,-0.60109852328464,-0.596657356849148));
#52152=DIRECTION('ref_axis',(-0.759626573944644,0.0268944798668635,0.649803166435663));
#52153=DIRECTION('center_axis',(0.529123109915892,0.601098531435083,0.598923442569684));
#52154=DIRECTION('ref_axis',(-0.76239577523424,0.0268943012708223,0.646551914747869));
#52155=DIRECTION('center_axis',(-0.521560170386556,0.584827952222643,-0.621249752487208));
#52156=DIRECTION('ref_axis',(-0.767386664096021,-0.00326197146761128,0.641176315306269));
#52157=DIRECTION('center_axis',(0.668811781409396,-6.23322798646924E-10,
0.743431772961037));
#52158=DIRECTION('ref_axis',(0.743340338836695,-0.0156832196313301,-0.668729524755818));
#52159=DIRECTION('',(-0.668811721396591,8.32139862539898E-8,-0.743431826950207));
#52160=DIRECTION('center_axis',(-0.494071316001355,0.584827969930883,-0.643327117640172));
#52161=DIRECTION('ref_axis',(-0.789974212594529,0.00704480137084633,0.613099595668843));
#52162=DIRECTION('center_axis',(-0.620811426879039,7.50881692280034E-10,
-0.783959930262008));
#52163=DIRECTION('ref_axis',(0.78386365533596,0.0156715280539164,-0.620735187541195));
#52164=DIRECTION('',(0.620811504614624,-1.36557432027502E-11,0.78395986870383));
#52165=DIRECTION('',(-0.998606990638996,-3.07807852448225E-8,-0.0527643653134219));
#52166=DIRECTION('center_axis',(-0.444353453098131,0.793626260382086,0.415580759361779));
#52167=DIRECTION('ref_axis',(-0.872542221931499,-0.488538709773179,-1.44217452160079E-16));
#52168=DIRECTION('center_axis',(0.0176157549639931,0.471546674566232,-0.881665139881677));
#52169=DIRECTION('ref_axis',(0.898990386289206,-0.393418648488291,-0.192452727653393));
#52170=DIRECTION('center_axis',(0.537306130849713,-0.601098528023407,0.591593341206106));
#52171=DIRECTION('ref_axis',(-0.741402943245098,-0.00227572516403292,0.671056254588603));
#52172=DIRECTION('',(-0.115363314589492,5.19500677922248E-12,0.993323364089925));
#52173=DIRECTION('center_axis',(0.,-1.,1.45983193964168E-32));
#52174=DIRECTION('ref_axis',(1.,0.,0.));
#52175=DIRECTION('center_axis',(-0.539828728548569,0.601098526995621,-0.589292376225359));
#52176=DIRECTION('ref_axis',(-0.739564117538253,-0.00432814660592568,0.673072197610942));
#52177=DIRECTION('center_axis',(-0.531677101688084,-0.601098528380341,-0.596657371294068));
#52178=DIRECTION('ref_axis',(-0.744933164574353,-0.00330175743698294,0.667130930713805));
#52179=DIRECTION('center_axis',(0.529123113241154,0.601098527640399,0.598923443440423));
#52180=DIRECTION('ref_axis',(-0.747776509741548,-0.00330191911101335,0.66394230834383));
#52181=DIRECTION('center_axis',(-0.595304362154782,0.584828255987947,-0.5509887724787));
#52182=DIRECTION('ref_axis',(-0.696201780475317,-0.0330815410697006,0.717083462717871));
#52183=DIRECTION('center_axis',(0.714196283526239,-1.08070422970347E-7,
0.699945475445978));
#52184=DIRECTION('ref_axis',(0.699859476888709,-0.015675163530811,-0.714108536468614));
#52185=DIRECTION('',(-0.714172445803004,-1.60982338570655E-12,-0.699969797673982));
#52186=DIRECTION('center_axis',(-0.570803912671749,0.584827952226411,-0.576332507822772));
#52187=DIRECTION('ref_axis',(-0.721774233899328,-0.0227607295851833,0.691754222587609));
#52188=DIRECTION('center_axis',(-0.668811664780684,5.92864469603341E-10,
-0.743431877883435));
#52189=DIRECTION('ref_axis',(0.743340325119513,0.0156933905087102,-0.668729301395982));
#52190=DIRECTION('',(0.668811722367516,-2.32591723654911E-11,0.743431826076741));
#52191=DIRECTION('',(-0.999949569924939,0.,0.010042788802444));
#52192=DIRECTION('center_axis',(0.607215618103716,-0.601098527827829,0.519586136241278));
#52193=DIRECTION('ref_axis',(-0.668178775416595,-0.0324816898727424,0.7432913721454));
#52194=DIRECTION('',(-0.0527643813501558,8.17238220606145E-12,0.998606989791647));
#52195=DIRECTION('center_axis',(0.,-1.,1.45983193964168E-32));
#52196=DIRECTION('ref_axis',(1.,0.,0.));
#52197=DIRECTION('center_axis',(-0.609429958764808,0.601098517802545,-0.516987134516428));
#52198=DIRECTION('ref_axis',(-0.666106973868854,-0.0345386499370693,0.745056092535188));
#52199=DIRECTION('center_axis',(-0.531677091111748,-0.601098532367363,-0.596657376701866));
#52200=DIRECTION('ref_axis',(-0.729167024598296,-0.0335099273449384,0.683514838908275));
#52201=DIRECTION('center_axis',(0.529123081475363,0.601098522341261,0.598923476822515));
#52202=DIRECTION('ref_axis',(-0.732080524449355,-0.0335101098726774,0.680393399628684));
#52203=DIRECTION('',(-0.756714656869205,4.44089209849579E-13,-0.653745308265628));
#52204=DIRECTION('center_axis',(-0.638536571159005,0.584827952146087,-0.500247252547293));
#52205=DIRECTION('ref_axis',(-0.645292296180387,-0.0526562728463764,0.762118868300852));
#52206=DIRECTION('center_axis',(-0.714172381807117,6.7742520729511E-10,
-0.699969862968364));
#52207=DIRECTION('ref_axis',(0.699882785675474,0.0157729998148926,-0.714083537684477));
#52208=DIRECTION('',(0.714172445804168,-1.75692793624375E-10,0.699969797672794));
#52209=DIRECTION('',(-0.997345805939016,0.,0.0728103246514788));
#52210=DIRECTION('',(0.0100427887670809,6.72270837774816E-11,0.999949569925294));
#52211=DIRECTION('center_axis',(0.,-1.,1.45983193964168E-32));
#52212=DIRECTION('ref_axis',(1.,0.,0.));
#52213=DIRECTION('center_axis',(-0.545499755366481,0.601098541294413,-0.584046710930588));
#52214=DIRECTION('ref_axis',(-0.7028616489713,0.051484846090818,0.70946093129104));
#52215=DIRECTION('center_axis',(0.657079473241136,0.60109853820579,0.454892419382884));
#52216=DIRECTION('ref_axis',(-0.60044923356296,0.0525164785306523,0.797936549730862));
#52217=DIRECTION('center_axis',(-0.600608226829493,0.584827930050726,-0.545202760537138));
#52218=DIRECTION('ref_axis',(-0.660160309869158,0.0219594825803943,0.750803667011729));
#52219=DIRECTION('center_axis',(0.796272582239159,-1.00169709512767E-8,
0.604937992503515));
#52220=DIRECTION('ref_axis',(0.604863059963878,-0.0157391393487521,-0.796173949701756));
#52221=DIRECTION('',(-0.796270460894404,-3.88578058618498E-13,-0.604940784793862));
#52222=DIRECTION('center_axis',(-0.576348241677965,0.584827952320902,-0.570788025889523));
#52223=DIRECTION('ref_axis',(-0.686575635047655,0.0322834330554533,0.726341295335095));
#52224=DIRECTION('center_axis',(-0.756714608220924,5.53608283030036E-10,
-0.653745364576342));
#52225=DIRECTION('ref_axis',(0.653664767416266,0.0157020800830109,-0.756621316458706));
#52226=DIRECTION('',(0.75671465686865,-8.32667268468213E-13,0.653745308266271));
#52227=DIRECTION('',(-0.990805973700979,0.,0.135290511413238));
#52228=DIRECTION('center_axis',(0.612209714621429,-0.601098528058252,0.513692344589007));
#52229=DIRECTION('ref_axis',(-0.629096561700259,0.0232723706551922,0.776978708087294));
#52230=DIRECTION('',(0.0728103246514612,1.43735365432664E-13,0.997345805939018));
#52231=DIRECTION('center_axis',(0.,-1.,1.45983193964168E-32));
#52232=DIRECTION('ref_axis',(1.,0.,0.));
#52233=DIRECTION('center_axis',(-0.614398801971386,0.601098533841799,-0.511072073928291));
#52234=DIRECTION('ref_axis',(-0.627005006672677,0.0212179807364959,0.778726215624504));
#52235=DIRECTION('center_axis',(-0.659016991795236,-0.601098524564669,-0.452080931129964));
#52236=DIRECTION('ref_axis',(-0.579262774122748,0.0222452995525509,0.814837275266317));
#52237=DIRECTION('center_axis',(0.657079518485687,0.60109853076028,0.454892363866938));
#52238=DIRECTION('ref_axis',(-0.582738672468509,0.0222451363282048,0.812355090781968));
#52239=DIRECTION('center_axis',(-0.664204781937783,0.584827953016243,-0.465626752906031));
#52240=DIRECTION('ref_axis',(-0.578633057240995,-0.00784645566470083,0.815550254859528));
#52241=DIRECTION('center_axis',(0.832683926477417,-7.28256137447449E-10,
0.553748569827636));
#52242=DIRECTION('ref_axis',(0.553680511340963,-0.0156778483074527,-0.832581585451935));
#52243=DIRECTION('',(-0.8326837491923,0.,-0.55374883641508));
#52244=DIRECTION('center_axis',(-0.6433422722591,0.58482795225408,-0.49405160356667));
#52245=DIRECTION('ref_axis',(-0.607659470213678,0.00246180457784726,0.794193872916338));
#52246=DIRECTION('center_axis',(-0.796270419146702,5.21210358149189E-10,
-0.604940839745454));
#52247=DIRECTION('ref_axis',(0.604866556891538,0.0156707406191342,-0.796172642234474));
#52248=DIRECTION('',(0.796270460894934,-6.33937347031928E-11,0.604940784793165));
#52249=DIRECTION('',(-0.980355882941021,1.64268989064092E-13,0.197236768334231));
#52250=DIRECTION('center_axis',(0.671764979565829,-0.601098528057821,0.432911505732573));
#52251=DIRECTION('ref_axis',(-0.546052527331169,-0.00691952331713121,0.837722363072818));
#52252=DIRECTION('',(0.13529051140086,2.3613667178499E-11,0.990805973702669));
#52253=DIRECTION('center_axis',(-0.717325884960116,0.584827952229979,-0.378708121191871));
#52254=DIRECTION('ref_axis',(-0.478331876855593,-0.0181546317001112,0.877991472015326));
#52255=DIRECTION('center_axis',(0.865810846544381,-4.91898929192996E-10,
0.500371440038401));
#52256=DIRECTION('ref_axis',(0.500309928860263,-0.0156795066183271,-0.865704411537821));
#52257=DIRECTION('',(-0.865810813532527,2.06171160586968E-7,-0.500371497159962));
#52258=DIRECTION('center_axis',(-0.700193645032136,0.584827782588847,-0.409518405164925));
#52259=DIRECTION('ref_axis',(-0.521594170261362,-0.0273551035144114,0.852755076127417));
#52260=DIRECTION('center_axis',(-0.832683698962267,7.12366036531364E-10,
-0.553748911947027));
#52261=DIRECTION('ref_axis',(0.553680640722956,0.0157023279285975,-0.83258103808953));
#52262=DIRECTION('',(-0.83268374860965,-1.29267411567854E-5,-0.553748837140342));
#52263=DIRECTION('center_axis',(0.865810815155372,-1.00468440339018E-11,
0.500371494351937));
#52264=DIRECTION('ref_axis',(0.386224871041075,-0.635772805085301,-0.668298802410474));
#52265=DIRECTION('',(-0.197236768333327,0.,-0.980355882941203));
#52266=DIRECTION('center_axis',(0.,-1.,1.45983193964168E-32));
#52267=DIRECTION('ref_axis',(1.,0.,0.));
#52268=DIRECTION('center_axis',(-0.673608428738637,0.601098525416304,-0.430037495428723));
#52269=DIRECTION('ref_axis',(-0.543756029387751,-0.00897218398747796,0.83919537678598));
#52270=DIRECTION('center_axis',(-0.659016985594954,-0.601098529035859,-0.452080934223361));
#52271=DIRECTION('ref_axis',(-0.56072842327227,-0.00794565772609306,0.827961654823394));
#52272=DIRECTION('center_axis',(0.657079502595968,0.601098526821226,0.454892392024299));
#52273=DIRECTION('ref_axis',(-0.564260575522972,-0.00794583663500264,0.825558517968687));
#52274=DIRECTION('',(-0.966036765128978,-7.62629077544845E-8,0.258404660211721));
#52275=DIRECTION('center_axis',(-0.820017152393108,0.398564395010779,-0.410753323554162));
#52276=DIRECTION('ref_axis',(-0.447863103182219,-5.76011272065838E-16,0.894102142267869));
#52277=DIRECTION('center_axis',(0.898612168814772,5.74456501979234E-5,0.438743850963189));
#52278=DIRECTION('ref_axis',(0.438743841499205,-0.000363186155216258,-0.898612101878412));
#52279=DIRECTION('',(-0.895520512893129,5.94973688026089E-5,-0.445020232627338));
#52280=DIRECTION('center_axis',(-0.6914084161041,0.590180063979457,-0.416703604761975));
#52281=DIRECTION('ref_axis',(0.584945575469874,0.795818476300859,0.156561893564165));
#52282=DIRECTION('center_axis',(-0.651774153934771,0.550037558029746,0.52215815326325));
#52283=DIRECTION('ref_axis',(-0.644941563435971,-0.764231888730616,1.41890158173865E-16));
#52284=DIRECTION('center_axis',(-0.279966610619734,-0.477126089615033,-0.833048252832191));
#52285=DIRECTION('ref_axis',(0.95891877528538,-0.0976282465771925,-0.266352225212124));
#52286=DIRECTION('center_axis',(-0.350675851952374,0.584827951390166,-0.731438797255285));
#52287=DIRECTION('ref_axis',(-0.89296426791565,0.0265489689935778,0.449343931161027));
#52288=DIRECTION('center_axis',(0.517659993435585,-2.35082575115718E-11,
0.85558642532258));
#52289=DIRECTION('ref_axis',(0.855480329378303,-0.0157477670555638,-0.517595801644058));
#52290=DIRECTION('center_axis',(-0.470963348342342,-0.000115441184994627,
-0.882152770891473));
#52291=DIRECTION('ref_axis',(0.0218910266942953,0.99969051108519,-0.0118179946057292));
#52292=DIRECTION('',(0.462915795316803,-6.06958927296742E-10,0.886402259950984));
#52293=DIRECTION('center_axis',(0.37330239356122,-0.601098528356447,0.706629947121673));
#52294=DIRECTION('ref_axis',(-0.873849503844342,0.0279220061610186,0.485394073102404));
#52295=DIRECTION('',(-0.299450151004041,2.24350371841882E-10,0.954111946819479));
#52296=DIRECTION('center_axis',(0.,-1.,1.45983193964168E-32));
#52297=DIRECTION('ref_axis',(1.,0.,0.));
#52298=DIRECTION('center_axis',(-0.376317949464262,0.601098535010339,-0.705028617943582));
#52299=DIRECTION('ref_axis',(-0.872572092162209,0.0258666949039728,0.487800018526456));
#52300=DIRECTION('center_axis',(-0.452703687647038,-0.601098523524197,-0.658589353245103));
#52301=DIRECTION('ref_axis',(-0.835078627465076,0.0268944746709312,0.549472813870913));
#52302=DIRECTION('center_axis',(0.449885809662912,0.601098531270677,0.660517459245539));
#52303=DIRECTION('ref_axis',(-0.837418496166001,0.0268943050251962,0.545900136138731));
#52304=DIRECTION('center_axis',(-0.439584272333921,0.584827952222756,-0.68171983528103));
#52305=DIRECTION('ref_axis',(-0.841696291922646,-0.00326197147019357,0.539941396547621));
#52306=DIRECTION('center_axis',(0.570361301697443,-7.08808782319137E-10,
0.821393928347415));
#52307=DIRECTION('ref_axis',(0.821292905716089,-0.0156832196307858,-0.570291153396611));
#52308=DIRECTION('',(-0.570361226402818,8.3214818921328E-8,-0.821393980630651));
#52309=DIRECTION('center_axis',(-0.40954514820993,0.58482796993091,-0.700177846810506));
#52310=DIRECTION('ref_axis',(-0.860586784796277,0.00704480137018753,0.509255099736528));
#52311=DIRECTION('center_axis',(-0.517659939546137,4.83271880986753E-10,
-0.855586457927596));
#52312=DIRECTION('ref_axis',(0.855481386835343,0.0156715280552529,-0.517596367826022));
#52313=DIRECTION('',(0.517659995144269,-1.48214773786002E-11,0.855586424288766));
#52314=DIRECTION('',(-0.984119547726674,-3.07809289801987E-8,-0.177506945729585));
#52315=DIRECTION('center_axis',(-0.492935673776194,0.79362626038218,0.356611525824118));
#52316=DIRECTION('ref_axis',(-0.849477030546853,-0.527625600756161,-4.09521487904968E-16));
#52317=DIRECTION('center_axis',(0.127978792334609,0.47154667454649,-0.872505107398646));
#52318=DIRECTION('ref_axis',(0.916024775580547,-0.393413511721289,-0.078258669281638));
#52319=DIRECTION('center_axis',(0.458922996999573,-0.601098528053855,0.654270771467302));
#52320=DIRECTION('ref_axis',(-0.819662414427714,-0.00227571922525397,0.572842340855264));
#52321=DIRECTION('',(-0.238950069592984,5.051271413789E-12,0.971031855420567));
#52322=DIRECTION('center_axis',(0.,-1.,1.45983193964168E-32));
#52323=DIRECTION('ref_axis',(1.,0.,0.));
#52324=DIRECTION('center_axis',(-0.461714089613293,0.601098527038454,-0.652304116378833));
#52325=DIRECTION('ref_axis',(-0.818090753690027,-0.00432813989567482,0.575072852716877));
#52326=DIRECTION('center_axis',(-0.452703668569484,-0.601098528371206,-0.658589361934811));
#52327=DIRECTION('ref_axis',(-0.822672822304874,-0.00330175941561732,0.56850551960882));
#52328=DIRECTION('center_axis',(0.449885812549619,0.601098527660819,0.660517460564492));
#52329=DIRECTION('ref_axis',(-0.825094102333532,-0.00330191552492792,0.564985680923233));
#52330=DIRECTION('center_axis',(-0.521553004948764,0.584828255987703,-0.621255482090336));
#52331=DIRECTION('ref_axis',(-0.780586410601624,-0.0330815410779919,0.624171825080224));
#52332=DIRECTION('center_axis',(0.620838225739205,-1.08300056263464E-7,
0.783938707719541));
#52333=DIRECTION('ref_axis',(0.783842389664105,-0.0156751635317241,-0.620761949070591));
#52334=DIRECTION('',(-0.620811504614934,1.16573417585605E-12,-0.783959868703585));
#52335=DIRECTION('center_axis',(-0.49406933650575,0.584827952226459,-0.643328653970406));
#52336=DIRECTION('ref_axis',(-0.802782622036335,-0.0227607295775255,0.595837235279539));
#52337=DIRECTION('center_axis',(-0.570361157887498,6.48541563533731E-10,
-0.821394028206459));
#52338=DIRECTION('ref_axis',(0.821292874494091,0.0156933905080219,-0.570290918566652));
#52339=DIRECTION('',(0.570361227475292,-2.28150831556906E-11,0.821393979885949));
#52340=DIRECTION('',(-0.993323364090245,0.,-0.115363314586734));
#52341=DIRECTION('center_axis',(0.537306131419502,-0.601098527806004,0.5915933409095));
#52342=DIRECTION('ref_axis',(-0.756069097064001,-0.0324816901882255,0.653685291457092));
#52343=DIRECTION('',(-0.177506961533698,8.00811321699377E-12,0.984119544876065));
#52344=DIRECTION('center_axis',(0.,-1.,1.45983193964168E-32));
#52345=DIRECTION('ref_axis',(1.,0.,0.));
#52346=DIRECTION('center_axis',(-0.53982874725037,0.601098518028139,-0.589292368240478));
#52347=DIRECTION('ref_axis',(-0.754234814257284,-0.0345386459730884,0.655695757876034));
#52348=DIRECTION('center_axis',(-0.45270365302585,-0.601098532080463,-0.658589369233792));
#52349=DIRECTION('ref_axis',(-0.809084453718785,-0.0335099325942185,0.58673625349735));
#52350=DIRECTION('center_axis',(0.449885781508012,0.601098522737911,0.660517486187328));
#52351=DIRECTION('ref_axis',(-0.811583750412878,-0.0335101027780247,0.583274282887196));
#52352=DIRECTION('',(-0.668811722367349,-3.8857805861924E-13,-0.743431826076891));
#52353=DIRECTION('center_axis',(-0.570803913814109,0.58482795214713,-0.57633250677182));
#52354=DIRECTION('ref_axis',(-0.735722795822873,-0.0526562728337489,0.67523276330302));
#52355=DIRECTION('center_axis',(-0.620811448742737,5.19037977403783E-10,
-0.783959912948324));
#52356=DIRECTION('ref_axis',(0.783862387164722,0.0157729998154696,-0.620734218861216));
#52357=DIRECTION('',(0.620811504616689,-1.78523862336725E-10,0.783959868702195));
#52358=DIRECTION('',(-0.99860698979188,0.,-0.0527643813457488));
#52359=DIRECTION('',(-0.115363314620757,6.51326541667565E-11,0.993323364086294));
#52360=DIRECTION('center_axis',(0.,-1.,1.45983193964168E-32));
#52361=DIRECTION('ref_axis',(1.,0.,0.));
#52362=DIRECTION('center_axis',(-0.467997860236714,0.60109854104577,-0.647810579387605));
#52363=DIRECTION('ref_axis',(-0.786238409799018,0.0514848489886549,0.61577469360256));
#52364=DIRECTION('center_axis',(0.594885072803049,0.601098537808415,0.533659346400581));
#52365=DIRECTION('ref_axis',(-0.69572247542785,0.0525164831338593,0.716388341741961));
#52366=DIRECTION('center_axis',(-0.52754022664394,0.584827930050739,-0.616179845098027));
#52367=DIRECTION('ref_axis',(-0.749055400002377,0.0219594825787594,0.662143329538366));
#52368=DIRECTION('center_axis',(0.714174875099444,-9.73286011102838E-9,
0.699967319077608));
#52369=DIRECTION('ref_axis',(0.699880615468601,-0.0157391393466766,-0.714086411846577));
#52370=DIRECTION('',(-0.714172445802862,1.16573417585578E-12,-0.699969797674127));
#52371=DIRECTION('center_axis',(-0.500264854685563,0.584827952321108,-0.638522780604054));
#52372=DIRECTION('ref_axis',(-0.772196484307766,0.032283433051883,0.634563132850554));
#52373=DIRECTION('center_axis',(-0.668811663975281,5.85773660908862E-10,
-0.743431878607998));
#52374=DIRECTION('ref_axis',(0.743340224422381,0.0157020800826207,-0.668729209349168));
#52375=DIRECTION('',(0.668811722367304,-3.88578058619029E-13,0.743431826076931));
#52376=DIRECTION('',(-0.999949569924938,0.,0.0100427888025238));
#52377=DIRECTION('center_axis',(0.542999531328701,-0.601098527924313,0.586371954227037));
#52378=DIRECTION('ref_axis',(-0.721517204487967,0.0232723741764296,0.692005289161912));
#52379=DIRECTION('',(-0.0527643813459068,0.,0.998606989791872));
#52380=DIRECTION('center_axis',(0.,-1.,1.45983193964168E-32));
#52381=DIRECTION('ref_axis',(1.,0.,0.));
#52382=DIRECTION('center_axis',(-0.545499761809049,0.601098533647117,-0.584046712783795));
#52383=DIRECTION('ref_axis',(-0.719661164504588,0.0212179861508259,0.694001156603938));
#52384=DIRECTION('center_axis',(-0.597159676907081,-0.601098524704973,-0.531112873006986));
#52385=DIRECTION('ref_axis',(-0.676821308316238,0.0222452958767956,0.73581116016302));
#52386=DIRECTION('center_axis',(0.594885119307456,0.601098530760866,0.533659302498965));
#52387=DIRECTION('ref_axis',(-0.67995869433305,0.0222451362999726,0.732912906089046));
#52388=DIRECTION('center_axis',(-0.600608822257759,0.584827953016275,-0.545202079963881));
#52389=DIRECTION('ref_axis',(-0.676285913340346,-0.00784645565583719,0.736597445387272));
#52390=DIRECTION('center_axis',(0.756714871630385,-7.93392647660612E-10,
0.653745059678014));
#52391=DIRECTION('ref_axis',(0.65366471112118,-0.0156778483085135,-0.756621867584647));
#52392=DIRECTION('',(-0.756714656868892,3.88578058618794E-13,-0.65374530826599));
#52393=DIRECTION('center_axis',(-0.576348241270836,0.58482795225427,-0.57078802636889));
#52394=DIRECTION('ref_axis',(-0.702406779954916,0.00246180457067037,0.711771490712871));
#52395=DIRECTION('center_axis',(-0.714172408549139,3.97521702241774E-10,
-0.699969835683739));
#52396=DIRECTION('ref_axis',(0.699883883875737,0.0156707406191022,-0.714084712747348));
#52397=DIRECTION('',(0.714172445802881,-6.46149800301959E-11,0.699969797674108));
#52398=DIRECTION('',(-0.997345805939002,1.64268989064134E-13,0.0728103246516758));
#52399=DIRECTION('center_axis',(0.612209720657188,-0.601098527971134,0.513692337497635));
#52400=DIRECTION('ref_axis',(-0.646741185585192,-0.00691953024425702,0.762678149004584));
#52401=DIRECTION('',(0.0100427887901276,2.35931335548657E-11,0.999949569925062));
#52402=DIRECTION('center_axis',(0.,-1.,1.45983193964168E-32));
#52403=DIRECTION('ref_axis',(1.,0.,0.));
#52404=DIRECTION('center_axis',(-0.614398828791068,0.601098525500061,-0.511072051497454));
#52405=DIRECTION('ref_axis',(-0.644647426983502,-0.00897217798432998,0.764427364048258));
#52406=DIRECTION('center_axis',(-0.597159673304864,-0.601098529024544,-0.531112872168391));
#52407=DIRECTION('ref_axis',(-0.660078024723387,-0.00794565881973064,0.751155022470856));
#52408=DIRECTION('center_axis',(0.594885098139866,0.601098526797091,0.533659330559758));
#52409=DIRECTION('ref_axis',(-0.663281132608099,-0.00794583835980365,0.748328138438531));
#52410=DIRECTION('center_axis',(-0.664204842698312,0.584827952230054,-0.465626667220115));
#52411=DIRECTION('ref_axis',(-0.584601597363002,-0.0181546317022303,0.811117366173591));
#52412=DIRECTION('center_axis',(0.796270423924654,4.79391517388211E-10,
0.60494083345634));
#52413=DIRECTION('ref_axis',(0.604866467468704,-0.0156795066158151,-0.796172537584797));
#52414=DIRECTION('',(-0.796270458940246,2.06171937743057E-7,-0.604940787366042));
#52415=DIRECTION('center_axis',(-0.643346147146909,0.584827782537135,-0.494046758641251));
#52416=DIRECTION('ref_axis',(-0.624359791305129,-0.0273551073958671,0.780657766950907));
#52417=DIRECTION('center_axis',(-0.756714597939265,5.92328891388393E-10,
-0.65374537647743));
#52418=DIRECTION('ref_axis',(0.65366477677188,0.0157023279245459,-0.756621303232679));
#52419=DIRECTION('',(-0.756714656199794,-1.29267412633769E-5,-0.653745308912674));
#52420=DIRECTION('',(-0.990805968327174,-7.6263051489871E-8,0.135290550768501));
#52421=DIRECTION('center_axis',(0.796270460902336,-1.03532362406177E-11,
0.604940784783422));
#52422=DIRECTION('ref_axis',(0.466939422466012,-0.635772805085451,-0.614622254771892));
#52423=DIRECTION('',(-0.0728103246508497,0.,-0.997345805939062));
#52424=DIRECTION('center_axis',(-0.762070031246047,0.398564391552654,-0.510289813011108));
#52425=DIRECTION('ref_axis',(-0.556392281443859,9.44692024466823E-17,0.830919748922661));
#52426=DIRECTION('center_axis',(0.83653715793225,5.74456598775067E-5,0.547910193461146));
#52427=DIRECTION('ref_axis',(0.547910175655507,-0.0003633645381878,-0.836537092650029));
#52428=DIRECTION('',(-0.832683241412774,5.94973691934172E-5,-0.553749596776718));
#52429=DIRECTION('center_axis',(-0.633729640882618,0.59018006380588,-0.500074229042925));
#52430=DIRECTION('ref_axis',(0.560699752632307,0.795821258487725,0.228657630393309));
#52431=DIRECTION('center_axis',(-0.712078489837049,0.550037558028519,0.436351817997143));
#52432=DIRECTION('ref_axis',(-0.611304898379798,-0.791395173865032,-8.76719162497403E-17));
#52433=DIRECTION('center_axis',(-0.173350358948395,-0.477126090400623,-0.861568538719631));
#52434=DIRECTION('ref_axis',(0.984740390653664,-0.0976174117503724,-0.144073605974262));
#52435=DIRECTION('center_axis',(-0.256237078487173,0.58482795138957,-0.769622522332758));
#52436=DIRECTION('ref_axis',(-0.94224070582697,0.0265489690038872,0.333882620882736));
#52437=DIRECTION('center_axis',(0.406344677055198,-1.12068438201966E-11,
0.913719871420616));
#52438=DIRECTION('ref_axis',(0.913606566709862,-0.0157477670552894,-0.406294288782639));
#52439=DIRECTION('center_axis',(-0.356686602128754,-0.00011544118293406,
-0.934224092247239));
#52440=DIRECTION('ref_axis',(0.0231987777512836,0.999690532904092,-0.00898082027316364));
#52441=DIRECTION('',(0.348169904526055,-6.07736083413689E-10,0.937431446870819));
#52442=DIRECTION('center_axis',(0.281794559405976,-0.601098527852825,0.747845161849937));
#52443=DIRECTION('ref_axis',(-0.927794953421368,0.0279220172196599,0.372044198127354));
#52444=DIRECTION('',(-0.416670832598985,2.2420663647639E-10,0.909057433422811));
#52445=DIRECTION('center_axis',(0.,-1.,1.45983193964168E-32));
#52446=DIRECTION('ref_axis',(1.,0.,0.));
#52447=DIRECTION('center_axis',(-0.284987050396032,0.601098534917648,-0.746634403457561));
#52448=DIRECTION('ref_axis',(-0.926829155228736,0.0258666969731542,0.374591285277283));
#52449=DIRECTION('center_axis',(-0.366590846799548,-0.601098523644121,-0.710134998374005));
#52450=DIRECTION('ref_axis',(-0.897360989139196,0.0268944721096581,0.440476948932707));
#52451=DIRECTION('center_axis',(0.36355353887101,0.601098531205687,0.711694723991074));
#52452=DIRECTION('ref_axis',(-0.899234629581645,0.0268943064871736,0.43663918426973));
#52453=DIRECTION('center_axis',(-0.350675867677086,0.584827952222683,-0.731438789050694));
#52454=DIRECTION('ref_axis',(-0.902731866435013,-0.00326197144967307,0.430191279392108));
#52455=DIRECTION('center_axis',(0.462915873277324,-6.89120218774699E-10,
0.886402219236782));
#52456=DIRECTION('ref_axis',(0.886293201285704,-0.0156832196313558,-0.462858939609827));
#52457=DIRECTION('',(-0.462915794151209,8.32139862540845E-8,-0.886402260559701));
#52458=DIRECTION('center_axis',(-0.318560208793917,0.584827969931273,-0.745986353065016));
#52459=DIRECTION('ref_axis',(-0.917627389307625,0.0070448013615417,0.397379346678018));
#52460=DIRECTION('center_axis',(-0.406344585065271,7.73278930637216E-10,
-0.913719912329885));
#52461=DIRECTION('ref_axis',(0.913607702105341,0.0156715280544491,-0.406294683526916));
#52462=DIRECTION('',(0.406344678314967,-1.565414464706E-11,0.913719870860378));
#52463=DIRECTION('',(-0.954111951662124,-3.07809289802008E-8,-0.299450135574341));
#52464=DIRECTION('center_axis',(-0.533744004413321,0.793626260382327,0.292018315494759));
#52465=DIRECTION('ref_axis',(-0.829794751147533,-0.558068697355446,-2.23533872199617E-16));
#52466=DIRECTION('center_axis',(0.23632352768933,0.471546674520354,-0.849585148180726));
#52467=DIRECTION('ref_axis',(0.918610213450041,-0.393413126094722,0.0371670278829099));
#52468=DIRECTION('center_axis',(0.373302383932541,-0.601098528045228,0.706629952473105));
#52469=DIRECTION('ref_axis',(-0.884995312998488,-0.00227572143390278,0.465594369663835));
#52470=DIRECTION('',(-0.358768439257086,5.19500677922277E-12,0.933426594324928));
#52471=DIRECTION('center_axis',(0.,-1.,1.45983193964168E-32));
#52472=DIRECTION('ref_axis',(1.,0.,0.));
#52473=DIRECTION('center_axis',(-0.376317948744125,0.601098527048046,-0.705028625116515));
#52474=DIRECTION('ref_axis',(-0.883715605272235,-0.00432813772470444,0.468004269448648));
#52475=DIRECTION('center_axis',(-0.366590819735879,-0.601098528339074,-0.710135008370927));
#52476=DIRECTION('ref_axis',(-0.887438440940119,-0.00330176677718059,0.460914430103811));
#52477=DIRECTION('center_axis',(0.363553538492343,0.601098527658307,0.71169472718063));
#52478=DIRECTION('ref_axis',(-0.889399471565693,-0.00330191612723909,0.457118887521128));
#52479=DIRECTION('center_axis',(-0.439576445278285,0.584828255987864,-0.6817246216433));
#52480=DIRECTION('ref_axis',(-0.852660726744351,-0.0330815410735374,0.521416624886467));
#52481=DIRECTION('center_axis',(0.517689131149895,-1.08056920685984E-7,
0.855568795298926));
#52482=DIRECTION('ref_axis',(0.855463676738608,-0.0156751635310533,-0.517625527798946));
#52483=DIRECTION('',(-0.517659995144338,0.,-0.855586424288724));
#52484=DIRECTION('center_axis',(-0.409542991772211,0.584827952226587,-0.700179122928358));
#52485=DIRECTION('ref_axis',(-0.871130648656311,-0.0227607295796337,0.490523538844608));
#52486=DIRECTION('center_axis',(-0.462915703310323,7.97913436906672E-10,
-0.886402308000554));
#52487=DIRECTION('ref_axis',(0.886293148594207,0.0156933905085995,-0.462858695769359));
#52488=DIRECTION('',(0.4629157953087,-2.3259172365528E-11,0.886402259955216));
#52489=DIRECTION('',(-0.971031855421177,0.,-0.238950069590505));
#52490=DIRECTION('center_axis',(0.458923001955571,-0.601098527953781,0.654270768082974));
#52491=DIRECTION('ref_axis',(-0.83203575979251,-0.0324816874711891,0.553770199997729));
#52492=DIRECTION('',(-0.299450150896404,8.00811321699499E-12,0.954111946853262));
#52493=DIRECTION('center_axis',(0.,-1.,1.45983193964168E-32));
#52494=DIRECTION('ref_axis',(1.,0.,0.));
#52495=DIRECTION('center_axis',(-0.461714116117164,0.601098518117668,-0.652304105839362));
#52496=DIRECTION('ref_axis',(-0.830467918261611,-0.0345386443924794,0.555994711109518));
#52497=DIRECTION('center_axis',(-0.366590812751239,-0.601098532026415,-0.710135008855412));
#52498=DIRECTION('ref_axis',(-0.876242133670582,-0.0335099336422242,0.480704490854536));
#52499=DIRECTION('center_axis',(0.363553507319193,0.601098522813485,0.711694747196689));
#52500=DIRECTION('ref_axis',(-0.878287821258083,-0.033510101446702,0.476956576776924));
#52501=DIRECTION('',(-0.570361227475679,-3.88578058618649E-13,-0.82139397988568));
#52502=DIRECTION('center_axis',(-0.494069337794621,0.584827952146325,-0.643328653053415));
#52503=DIRECTION('ref_axis',(-0.814550507452863,-0.0526562728431611,0.57769783428584));
#52504=DIRECTION('center_axis',(-0.517659889573965,9.29479950426669E-10,
-0.855586488162518));
#52505=DIRECTION('ref_axis',(0.855480051928071,0.015772999815068,-0.517595491894953));
#52506=DIRECTION('',(0.517659995146304,-1.77302617009957E-10,0.855586424287534));
#52507=DIRECTION('',(-0.98411954487684,0.,-0.177506961529406));
#52508=DIRECTION('',(-0.238950069624714,6.73708191429337E-11,0.971031855412758));
#52509=DIRECTION('center_axis',(0.,-1.,1.45983193964168E-32));
#52510=DIRECTION('ref_axis',(1.,0.,0.));
#52511=DIRECTION('center_axis',(-0.383115352763055,0.601098540442394,-0.701358090532407));
#52512=DIRECTION('ref_axis',(-0.857215723028873,0.0514848559344195,0.512377315853756));
#52513=DIRECTION('center_axis',(0.523308968761393,0.601098538211298,0.604010157674628));
#52514=DIRECTION('ref_axis',(-0.780023767323197,0.0525164784582637,0.623542253501132));
#52515=DIRECTION('center_axis',(-0.446152601960881,0.584827930051338,-0.677439405404943));
#52516=DIRECTION('ref_axis',(-0.826137439006878,0.0219594825671946,0.563040596224232));
#52517=DIRECTION('center_axis',(0.620814204536648,-9.52273684387182E-9,
0.783957730649765));
#52518=DIRECTION('ref_axis',(0.783860623339077,-0.0157391393472892,-0.620737305686617));
#52519=DIRECTION('',(-0.620811504615104,-1.60982338570751E-12,-0.78395986870345));
#52520=DIRECTION('center_axis',(-0.416291992083781,0.584827952321421,-0.696187649639414));
#52521=DIRECTION('ref_axis',(-0.8456393337275,0.0322834330537012,0.532777530685349));
#52522=DIRECTION('center_axis',(-0.570361157976486,6.33614257171157E-10,
-0.821394028144667));
#52523=DIRECTION('ref_axis',(0.821292762374769,0.0157020800825937,-0.570290840845179));
#52524=DIRECTION('',(0.570361227475211,-1.99840144432419E-12,0.821393979886005));
#52525=DIRECTION('',(-0.99332336409025,0.,-0.115363314586692));
#52526=DIRECTION('center_axis',(0.46522593544058,-0.601098528225849,0.649804115374899));
#52527=DIRECTION('ref_axis',(-0.802559080156761,0.0232723661732835,0.596118545115508));
#52528=DIRECTION('',(-0.177506961529595,0.,0.984119544876806));
#52529=DIRECTION('center_axis',(0.,-1.,1.45983193964168E-32));
#52530=DIRECTION('ref_axis',(1.,0.,0.));
#52531=DIRECTION('center_axis',(-0.4679978757003,0.601098533795021,-0.64781057494416));
#52532=DIRECTION('ref_axis',(-0.800967827107389,0.0212179820057374,0.59833129383183));
#52533=DIRECTION('center_axis',(-0.525884798108242,-0.60109852478409,-0.601768844840812));
#52534=DIRECTION('ref_axis',(-0.763705963940892,0.022245293807787,0.64518086421136));
#52535=DIRECTION('center_axis',(0.523309032241945,0.601098530594663,0.604010110255562));
#52536=DIRECTION('ref_axis',(-0.76645535742454,0.0222451408421469,0.641912251623331));
#52537=DIRECTION('center_axis',(-0.527540902698841,0.584827953016229,-0.616179244498335));
#52538=DIRECTION('ref_axis',(-0.763273336564778,-0.00784645567575521,0.646028054207091));
#52539=DIRECTION('center_axis',(0.668811959513174,-7.18937375996525E-10,
0.743431612733914));
#52540=DIRECTION('ref_axis',(0.743340241251659,-0.0156778483086904,-0.668729759176556));
#52541=DIRECTION('',(-0.668811722367591,3.88578058618546E-13,-0.743431826076673));
#52542=DIRECTION('center_axis',(-0.500264854224869,0.584827952254413,-0.638522781026082));
#52543=DIRECTION('ref_axis',(-0.786076715181059,0.00246180456478883,0.618124046910036));
#52544=DIRECTION('center_axis',(-0.620811426908302,7.56581079087839E-10,
-0.783959930238834));
#52545=DIRECTION('ref_axis',(0.783863664988098,0.0156707406189149,-0.620735195232138));
#52546=DIRECTION('',(0.620811504615392,-6.42264019716503E-11,0.783959868703222));
#52547=DIRECTION('',(-0.998606989791874,1.64268989064165E-13,-0.0527643813458644));
#52548=DIRECTION('center_axis',(0.542999531338148,-0.601098528084606,0.586371954053971));
#52549=DIRECTION('ref_axis',(-0.737230364923761,-0.00691952120981509,0.675606031101414));
#52550=DIRECTION('',(-0.115363314599122,2.37574025439407E-11,0.993323364088807));
#52551=DIRECTION('center_axis',(0.,-1.,1.45983193964168E-32));
#52552=DIRECTION('ref_axis',(1.,0.,0.));
#52553=DIRECTION('center_axis',(-0.545499785857832,0.601098525638433,-0.584046698564731));
#52554=DIRECTION('ref_axis',(-0.735372351633788,-0.00897216828780553,0.677603870007254));
#52555=DIRECTION('center_axis',(-0.525884793701434,-0.601098528988418,-0.601768844492269));
#52556=DIRECTION('ref_axis',(-0.749017802714225,-0.00794566167936899,0.662502224658628));
#52557=DIRECTION('center_axis',(0.523309006927691,0.601098526850466,0.604010135913755));
#52558=DIRECTION('ref_axis',(-0.751841344649372,-0.00794583436748203,0.659296182449155));
#52559=DIRECTION('center_axis',(-0.600608893317819,0.584827952228866,-0.545202002526895));
#52560=DIRECTION('ref_axis',(-0.6816518014331,-0.0181546317269892,0.731451454950954));
#52561=DIRECTION('center_axis',(0.714172486918624,-4.60209657606995E-10,
0.699969755724109));
#52562=DIRECTION('ref_axis',(0.699883707722976,-0.0156795066181786,-0.714084692971464));
#52563=DIRECTION('',(-0.714172443541281,2.06170660986742E-7,-0.699969799981566));
#52564=DIRECTION('center_axis',(-0.576352692830911,0.584827782537096,-0.570783705302894));
#52565=DIRECTION('ref_axis',(-0.717278890098503,-0.0273551073999281,0.696249015739483));
#52566=DIRECTION('center_axis',(-0.668811641026249,7.44449369156047E-10,
-0.743431899253574));
#52567=DIRECTION('ref_axis',(0.743340242173521,0.0157023279256583,-0.66872918379799));
#52568=DIRECTION('',(-0.668811721622572,-1.29267404107118E-5,-0.743431826634528));
#52569=DIRECTION('',(-0.999949569526027,-7.62629077545172E-8,0.0100428285212935));
#52570=DIRECTION('center_axis',(0.714172445812284,-1.09814043632675E-11,
0.699969797664514));
#52571=DIRECTION('ref_axis',(0.540290060262428,-0.635772805085269,-0.551252747018671));
#52572=DIRECTION('',(0.0527643813464523,0.,-0.998606989791843));
#52573=DIRECTION('center_axis',(-0.692104609109857,0.398564391554928,-0.60177872663741));
#52574=DIRECTION('ref_axis',(-0.656146821083495,2.49882806495788E-16,0.754633254754933));
#52575=DIRECTION('center_axis',(0.76126945630972,5.74456474002762E-5,0.648435664958292));
#52576=DIRECTION('ref_axis',(0.648435639152938,-0.000363146004023474,-0.761269393842482));
#52577=DIRECTION('',(-0.756714057795,5.94973699394661E-5,-0.653745998990042));
#52578=DIRECTION('center_axis',(-0.566056573296636,0.590180063808837,-0.575558379411044));
#52579=DIRECTION('ref_axis',(0.527623534722438,0.795820516823244,0.297124739141971));
#52580=DIRECTION('center_axis',(-0.761152922577171,0.550037558029868,0.343663953897947));
#52581=DIRECTION('ref_axis',(-0.585711678833674,-0.81051948112173,-3.01370648851509E-16));
#52582=DIRECTION('center_axis',(-0.0640002687006948,-0.477126090261306,
-0.876501374555796));
#52583=DIRECTION('ref_axis',(0.995031847779778,-0.0976263647563779,-0.0195119145245918));
#52584=DIRECTION('center_axis',(-0.157757293237268,0.584827951389508,-0.795668840475736));
#52585=DIRECTION('ref_axis',(-0.97665744493467,0.0265489690060458,0.213155782230737));
#52586=DIRECTION('center_axis',(0.288621060453656,-9.51818097282618E-12,
0.957443410057538));
#52587=DIRECTION('ref_axis',(0.957324683463083,-0.015747767055969,-0.288585270353598));
#52588=DIRECTION('center_axis',(-0.236784693339787,-0.00011544116316845,
-0.971562141951466));
#52589=DIRECTION('ref_axis',(0.0241339308308979,0.999690725296098,-0.00600059493807027));
#52590=DIRECTION('',(0.227933166354572,-6.0612626002843E-10,0.973676779879021));
#52591=DIRECTION('center_axis',(0.185842683821483,-0.601098528165775,0.777266399831465));
#52592=DIRECTION('ref_axis',(-0.967108513356064,0.0279220103706326,0.252826985765141));
#52593=DIRECTION('',(-0.527320366256967,2.24206636476404E-10,0.849666541256403));
#52594=DIRECTION('center_axis',(0.,-1.,1.45983193964168E-32));
#52595=DIRECTION('ref_axis',(1.,0.,0.));
#52596=DIRECTION('center_axis',(-0.189161725627372,0.601098534572865,-0.776465320083279));
#52597=DIRECTION('ref_axis',(-0.966469570041807,0.025866704851165,0.255475015927873));
#52598=DIRECTION('center_axis',(-0.274696652837102,-0.601098523645616,-0.750481388037807));
#52599=DIRECTION('ref_axis',(-0.94549143003686,0.0268944720827181,0.324534502169254));
#52600=DIRECTION('center_axis',(0.271487805717504,0.601098531311225,0.751648140423551));
#52601=DIRECTION('ref_axis',(-0.946869297906245,0.0268943040459628,0.320492166975135));
#52602=DIRECTION('center_axis',(-0.256237095134423,0.584827952222713,-0.769622516157149));
#52603=DIRECTION('ref_axis',(-0.949530820132141,-0.00326197145096664,0.313656788801768));
#52604=DIRECTION('center_axis',(0.348169990616235,-7.19927070234003E-10,
0.9374314148962));
#52605=DIRECTION('ref_axis',(0.937316120903577,-0.0156832196315479,-0.348127169460041));
#52606=DIRECTION('',(-0.348169903293503,8.32132090980276E-8,-0.937431447328596));
#52607=DIRECTION('center_axis',(-0.222551384603853,0.584827969931453,-0.780030208900119));
#52608=DIRECTION('ref_axis',(-0.960196461724811,0.00704480134305794,0.279236683953222));
#52609=DIRECTION('center_axis',(-0.288620999812851,4.93139200386861E-10,
-0.957443428337691));
#52610=DIRECTION('ref_axis',(0.957325848603127,0.015671528054376,-0.288585555433297));
#52611=DIRECTION('',(0.288621063170277,-1.40443212613482E-11,0.957443409238613));
#52612=DIRECTION('',(-0.909057440161158,-3.07809289802204E-8,-0.416670817897825));
#52613=DIRECTION('center_axis',(-0.566134873256367,0.793626260383097,0.222819801887843));
#52614=DIRECTION('ref_axis',(-0.814092839857193,-0.580734748480966,-1.58476235549859E-16));
#52615=DIRECTION('center_axis',(0.340941299925238,0.471546674535792,-0.813266723615029));
#52616=DIRECTION('ref_axis',(0.90670649220367,-0.393419297900025,0.152001950762374));
#52617=DIRECTION('center_axis',(0.281794570900451,-0.601098528027835,0.747845157378051));
#52618=DIRECTION('ref_axis',(-0.936371307102128,-0.00227572440954448,0.351003698433882));
#52619=DIRECTION('',(-0.472928816316283,5.19500677922167E-12,0.881100638234748));
#52620=DIRECTION('center_axis',(0.,-1.,1.45983193964168E-32));
#52621=DIRECTION('ref_axis',(1.,0.,0.));
#52622=DIRECTION('center_axis',(-0.284987038209989,0.60109852710865,-0.746634414395767));
#52623=DIRECTION('ref_axis',(-0.93540373637898,-0.00432812888194756,0.353554970646186));
#52624=DIRECTION('center_axis',(-0.274696621413743,-0.601098528330619,-0.750481395787156));
#52625=DIRECTION('ref_axis',(-0.938208620668851,-0.00330176892258368,0.346054450086448));
#52626=DIRECTION('center_axis',(0.271487805197435,0.601098527639148,0.751648143547982));
#52627=DIRECTION('ref_axis',(-0.939678480413728,-0.00330191842797677,0.342043053988882));
#52628=DIRECTION('center_axis',(-0.350667502455631,0.58482825598845,-0.731442556677582));
#52629=DIRECTION('ref_axis',(-0.911288073877589,-0.0330815410569061,0.410438373023008));
#52630=DIRECTION('center_axis',(0.406375835800862,-1.08414464411254E-7,
0.913706014031395));
#52631=DIRECTION('ref_axis',(0.913593752748676,-0.0156751635316695,-0.406325908830394));
#52632=DIRECTION('',(-0.40634467831564,-4.44089209849844E-13,-0.913719870860079));
#52633=DIRECTION('center_axis',(-0.318557909437256,0.584827952226086,-0.745987348840453));
#52634=DIRECTION('ref_axis',(-0.925740424549813,-0.0227607295990099,0.377473993200132));
#52635=DIRECTION('center_axis',(-0.348169818716519,7.02758491966354E-10,
-0.937431478741196));
#52636=DIRECTION('ref_axis',(0.937316035149934,0.0156933905084249,-0.348126941998399));
#52637=DIRECTION('',(0.348169904517226,-2.20379270384261E-11,0.937431446874098));
#52638=DIRECTION('',(-0.933426594325903,-1.43735365431306E-13,-0.358768439254552));
#52639=DIRECTION('center_axis',(0.373302387671571,-0.601098527899086,0.706629950622146));
#52640=DIRECTION('ref_axis',(-0.894880718438291,-0.032481688583243,0.445121825654673));
#52641=DIRECTION('',(-0.416670832496686,8.17238220606245E-12,0.9090574334697));
#52642=DIRECTION('center_axis',(0.,-1.,1.45983193964168E-32));
#52643=DIRECTION('ref_axis',(1.,0.,0.));
#52644=DIRECTION('center_axis',(-0.376317985627075,0.601098517887626,-0.705028613239832));
#52645=DIRECTION('ref_axis',(-0.893604043109341,-0.0345386484892894,0.447525301965344));
#52646=DIRECTION('center_axis',(-0.27469661328818,-0.601098531871184,-0.750481395925516));
#52647=DIRECTION('ref_axis',(-0.92958095227624,-0.0335099365428258,0.367091728751949));
#52648=DIRECTION('center_axis',(0.27148778682652,0.601098523227746,0.751648153711203));
#52649=DIRECTION('ref_axis',(-0.931140766145985,-0.0335100940379686,0.363116988336589));
#52650=DIRECTION('',(-0.46291579530913,-3.8857805861882E-13,-0.886402259954991));
#52651=DIRECTION('center_axis',(-0.409542993149134,0.584827952146895,-0.700179122189542));
#52652=DIRECTION('ref_axis',(-0.880532271007807,-0.0526562728339964,0.471052265300854));
#52653=DIRECTION('center_axis',(-0.406344618832969,4.69796662330587E-10,
-0.913719897312896));
#52654=DIRECTION('ref_axis',(0.913606229190611,0.0157729998145959,-0.406294068946325));
#52655=DIRECTION('',(0.406344678317545,-1.76525460892821E-10,0.913719870859232));
#52656=DIRECTION('',(-0.954111946854531,0.,-0.299450150892358));
#52657=DIRECTION('',(-0.358768439286625,6.5132654166774E-11,0.933426594313575));
#52658=DIRECTION('center_axis',(0.,-1.,1.45983193964168E-32));
#52659=DIRECTION('ref_axis',(1.,0.,0.));
#52660=DIRECTION('center_axis',(-0.292190888656869,0.601098540001039,-0.743844761892243));
#52661=DIRECTION('ref_axis',(-0.914674229293506,0.0514848610180654,0.40089944294334));
#52662=DIRECTION('center_axis',(0.443479987208326,0.601098537465326,0.664835354958466));
#52663=DIRECTION('ref_axis',(-0.852023607513652,0.0525164870226359,0.520862545044489));
#52664=DIRECTION('center_axis',(-0.357728884201083,0.58482793005104,-0.728015341624381));
#52665=DIRECTION('ref_axis',(-0.890190797102062,0.0219594825743353,0.455058376342929));
#52666=DIRECTION('center_axis',(0.51766303052389,-1.03400239175962E-8,0.855584587769568));
#52667=DIRECTION('ref_axis',(0.855478608197473,-0.0157391393486956,-0.517598908817509));
#52668=DIRECTION('',(-0.517659995144606,0.,-0.855586424288562));
#52669=DIRECTION('center_axis',(-0.325753956097604,0.58482795232135,-0.74287322355189));
#52670=DIRECTION('ref_axis',(-0.90574594568893,0.0322834330483309,0.422589708604789));
#52671=DIRECTION('center_axis',(-0.462915741151528,4.48487702201447E-10,
-0.886402288238321));
#52672=DIRECTION('ref_axis',(0.88629300790583,0.0157020800818683,-0.462858670458207));
#52673=DIRECTION('',(0.462915795308233,-8.32667268468716E-13,0.88640225995546));
#52674=DIRECTION('',(-0.971031855421231,0.,-0.238950069590282));
#52675=DIRECTION('center_axis',(0.380115437938402,-0.601098528198227,0.702988487273314));
#52676=DIRECTION('ref_axis',(-0.870944127416965,0.0232723669164295,0.490830646818236));
#52677=DIRECTION('',(-0.299450150892453,1.43735365432663E-13,0.954111946854502));
#52678=DIRECTION('center_axis',(0.,-1.,1.45983193964168E-32));
#52679=DIRECTION('ref_axis',(1.,0.,0.));
#52680=DIRECTION('center_axis',(-0.38311537327739,0.601098533661765,-0.701358085137829));
#52681=DIRECTION('ref_axis',(-0.869642754686168,0.0212179856622501,0.493225380841547));
#52682=DIRECTION('center_axis',(-0.446316399920546,-0.601098524901484,-0.662934562776164));
#52683=DIRECTION('ref_axis',(-0.838546520538259,0.0222452907237038,0.544375679043248));
#52684=DIRECTION('center_axis',(0.443480040215139,0.601098530690299,0.664835325725659));
#52685=DIRECTION('ref_axis',(-0.840864568154533,0.0222451381343953,0.540788250474871));
#52686=DIRECTION('center_axis',(-0.446153347918924,0.584827953016325,-0.677438894300786));
#52687=DIRECTION('ref_axis',(-0.838223483347709,-0.00784645565821609,0.545270414655001));
#52688=DIRECTION('center_axis',(0.57036150323578,-8.49799438812077E-10,
0.82139378840275));
#52689=DIRECTION('ref_axis',(0.821292834977943,-0.0156778483083717,-0.570291402956694));
#52690=DIRECTION('',(-0.570361227475616,-7.7715611723776E-13,-0.821393979885724));
#52691=DIRECTION('center_axis',(-0.416291991565607,0.584827952254239,-0.696187650005697));
#52692=DIRECTION('ref_axis',(-0.857349751040828,0.00246180457236924,0.514728417622806));
#52693=DIRECTION('center_axis',(-0.517659944790757,4.41968251467754E-10,
-0.855586454754416));
#52694=DIRECTION('ref_axis',(0.855481394221478,0.0156707406182415,-0.517596379459277));
#52695=DIRECTION('',(0.517659995144688,-6.50590692400118E-11,0.855586424288512));
#52696=DIRECTION('',(-0.984119544876815,1.64268989064223E-13,-0.177506961529541));
#52697=DIRECTION('center_axis',(0.465225925216188,-0.601098528074967,0.649804122834605));
#52698=DIRECTION('ref_axis',(-0.816092971536365,-0.00691952152621577,0.577879210588851));
#52699=DIRECTION('',(-0.238950069602231,2.34493981894294E-11,0.971031855418291));
#52700=DIRECTION('center_axis',(0.,-1.,1.45983193964168E-32));
#52701=DIRECTION('ref_axis',(1.,0.,0.));
#52702=DIRECTION('center_axis',(-0.467997902155121,0.601098525572697,-0.647810563461832));
#52703=DIRECTION('ref_axis',(-0.814500001467842,-0.00897217296524106,0.580094171424922));
#52704=DIRECTION('center_axis',(-0.446316403197408,-0.601098529023294,-0.662934556832694));
#52705=DIRECTION('ref_axis',(-0.826145117889556,-0.00794565927750685,0.563401376183887));
#52706=DIRECTION('center_axis',(0.443480015076013,0.601098526843241,0.664835345973019));
#52707=DIRECTION('ref_axis',(-0.828544573820292,-0.00794583479468556,0.559866727804365));
#52708=DIRECTION('center_axis',(-0.527540982838747,0.5848279522305,-0.616179176632422));
#52709=DIRECTION('ref_axis',(-0.767951949450662,-0.0181546316971145,0.640250117284542));
#52710=DIRECTION('center_axis',(0.620811582090657,-7.74860921390325E-10,
0.783959807351178));
#52711=DIRECTION('ref_axis',(0.783863434364948,-0.0156795066180816,-0.620735265099223));
#52712=DIRECTION('',(-0.620811502082354,2.06171549165036E-7,-0.783959870709088));
#52713=DIRECTION('center_axis',(-0.50026981225926,0.584827782536682,-0.638519051959542));
#52714=DIRECTION('ref_axis',(-0.798886072311127,-0.0273551074082388,0.600860001635976));
#52715=DIRECTION('center_axis',(-0.570361141665806,7.05271550366232E-10,
-0.821394039470508));
#52716=DIRECTION('ref_axis',(0.821292770502868,0.0157023279247815,-0.570290822315655));
#52717=DIRECTION('',(-0.570361226666628,-1.29267412278592E-5,-0.821393980345753));
#52718=DIRECTION('',(-0.993323368672574,-7.62630514899115E-8,-0.115363275131056));
#52719=DIRECTION('center_axis',(0.620811504614919,1.410173336424E-14,0.783959868703597));
#52720=DIRECTION('ref_axis',(0.605120001066379,-0.635772805085093,-0.47918965412836));
#52721=DIRECTION('',(0.17750696153003,0.,-0.984119544876727));
#52722=DIRECTION('center_axis',(-0.61122428384635,0.398564391552574,-0.68377723026059));
#52723=DIRECTION('ref_axis',(-0.745553533391341,-2.17675110791388E-16,0.666445743363769));
#52724=DIRECTION('center_axis',(0.673996080582493,5.74456607852808E-5,0.738734918668012));
#52725=DIRECTION('ref_axis',(0.73873488531722,-0.000362796013170164,-0.673996021942568));
#52726=DIRECTION('',(-0.668811041446666,5.94973683763053E-5,-0.743432436270499));
#52727=DIRECTION('center_axis',(-0.489456455415781,0.590180063811213,-0.641965630335154));
#52728=DIRECTION('ref_axis',(0.486222843277527,0.795820632489076,0.360911163002481));
#52729=DIRECTION('center_axis',(-0.798223519039003,0.550037558029662,0.24555630395035));
#52730=DIRECTION('ref_axis',(-0.567410340630547,-0.82343518588018,3.06798539265314E-16));
#52731=DIRECTION('center_axis',(0.0463591440219179,-0.477126090531288,-0.877611259898074));
#52732=DIRECTION('ref_axis',(0.989629241963715,-0.0976390452529731,0.105359291438438));
#52733=DIRECTION('center_axis',(-0.0567895812488869,0.584827951389893,-0.809166985692494));
#52734=DIRECTION('ref_axis',(-0.995671712707148,0.0265489689991942,0.0890673495726409));
#52735=DIRECTION('center_axis',(0.16634571851791,2.36699141555689E-12,0.98606749359806));
#52736=DIRECTION('ref_axis',(0.985945217509321,-0.015747767056103,-0.166325091021305));
#52737=DIRECTION('center_axis',(-0.113148552631875,-0.00011544118542266,
-0.993578075296876));
#52738=DIRECTION('ref_axis',(0.024707162564102,0.999690438280507,-0.00292980008858347));
#52739=DIRECTION('',(0.104101785988569,-6.06903416145004E-10,0.994566648422312));
#52740=DIRECTION('center_axis',(0.0869599339253347,-0.601098527785029,0.794429688384298));
#52741=DIRECTION('ref_axis',(-0.991170198717985,0.0279220186133635,0.129622521383846));
#52742=DIRECTION('',(-0.629653742733209,2.24350371841873E-10,0.776875900168143));
#52743=DIRECTION('center_axis',(0.,-1.,1.45983193964168E-32));
#52744=DIRECTION('ref_axis',(1.,0.,0.));
#52745=DIRECTION('center_axis',(-0.0903532208711649,0.601098534606634,-0.794050909685244));
#52746=DIRECTION('ref_axis',(-0.990868178537547,0.0258667040795945,0.132329763778762));
#52747=DIRECTION('center_axis',(-0.178470325633292,-0.601098523730062,-0.778992238496564));
#52748=DIRECTION('ref_axis',(-0.97871090680517,0.0268944702660908,0.20347395010101));
#52749=DIRECTION('center_axis',(0.175140560780707,0.601098531055857,0.779747612969678));
#52750=DIRECTION('ref_axis',(-0.979571268606861,0.0268943098413773,0.199290807159039));
#52751=DIRECTION('center_axis',(-0.15775731054866,0.584827952222719,-0.795668836430984));
#52752=DIRECTION('ref_axis',(-0.981355105571386,-0.00326197146141438,0.19217574329545));
#52753=DIRECTION('center_axis',(0.227933218521286,-4.1940118515531E-10,
0.973676767667036));
#52754=DIRECTION('ref_axis',(0.973557015888024,-0.015683219630834,-0.227905185191599));
#52755=DIRECTION('',(-0.22793316507402,8.32144303433845E-8,-0.973676780178788));
#52756=DIRECTION('center_axis',(-0.123032792071934,0.584827969931186,-0.801772522390954));
#52757=DIRECTION('ref_axis',(-0.98762266236098,0.00704480136197383,0.15669029186513));
#52758=DIRECTION('center_axis',(-0.166345664255104,4.29216190013688E-10,
-0.986067502751981));
#52759=DIRECTION('ref_axis',(0.985946407810043,0.0156715280543889,-0.166325236013402));
#52760=DIRECTION('',(0.166345721445477,-1.44328993199749E-11,0.986067493104191));
#52761=DIRECTION('',(-0.849666549784077,-3.07807852448522E-8,-0.527320352516401));
#52762=DIRECTION('center_axis',(-0.58959745695761,0.793626260382879,0.150107286897758));
#52763=DIRECTION('ref_axis',(-0.802721322940073,-0.59635432227606,1.12566621593397E-16));
#52764=DIRECTION('center_axis',(0.440182224109369,0.47154667450417,-0.764122597062924));
#52765=DIRECTION('ref_axis',(0.88050646203643,-0.39341697707929,0.264445556699071));
#52766=DIRECTION('center_axis',(0.185842684630873,-0.601098528028628,0.777266399744004));
#52767=DIRECTION('ref_axis',(-0.972980168207799,-0.00227572432940167,0.230877485591603));
#52768=DIRECTION('',(-0.579630823428198,5.19500677922228E-12,0.814879198735585));
#52769=DIRECTION('center_axis',(0.,-1.,1.45983193964168E-32));
#52770=DIRECTION('ref_axis',(1.,0.,0.));
#52771=DIRECTION('center_axis',(-0.189161721372458,0.601098527118791,-0.776465326890408));
#52772=DIRECTION('ref_axis',(-0.972339986917059,-0.00432812674195253,0.233529906352568));
#52773=DIRECTION('center_axis',(-0.17847030044431,-0.601098528344443,-0.778992240706839));
#52774=DIRECTION('ref_axis',(-0.974182687949423,-0.00330176646215566,0.22573699040668));
#52775=DIRECTION('center_axis',(0.175140559098384,0.601098527670136,0.779747615957561));
#52776=DIRECTION('ref_axis',(-0.975138195345261,-0.00330191308371978,0.2215730068144));
#52777=DIRECTION('center_axis',(-0.256228323701883,0.584828255987388,-0.769625205623928));
#52778=DIRECTION('ref_axis',(-0.955543863686363,-0.0330815410800097,0.292987262882038));
#52779=DIRECTION('center_axis',(0.288653685344861,-1.08198123761921E-7,
0.957433574686421));
#52780=DIRECTION('ref_axis',(0.9573159411088,-0.0156751635316667,-0.288618222133026));
#52781=DIRECTION('',(-0.288621063170684,3.88578058619192E-13,-0.957443409238491));
#52782=DIRECTION('center_axis',(-0.22254897853054,0.584827952226241,-0.78003090865034));
#52783=DIRECTION('ref_axis',(-0.965750720954388,-0.0227607295905163,0.258471457156465));
#52784=DIRECTION('center_axis',(-0.227933086768831,6.25622020348082E-10,
-0.973676798509666));
#52785=DIRECTION('ref_axis',(0.973556891347874,0.0156933905084927,-0.227905017065031));
#52786=DIRECTION('',(0.227933166345219,-2.28705943068783E-11,0.97367677988121));
#52787=DIRECTION('',(-0.881100638236051,0.,-0.472928816313854));
#52788=DIRECTION('center_axis',(0.281794569239125,-0.601098527928147,0.747845158084179));
#52789=DIRECTION('ref_axis',(-0.943612874711639,-0.0324816879688959,0.329453612250841));
#52790=DIRECTION('',(-0.52732036616135,8.17238220606277E-12,0.849666541315745));
#52791=DIRECTION('center_axis',(0.,-1.,1.45983193964168E-32));
#52792=DIRECTION('ref_axis',(1.,0.,0.));
#52793=DIRECTION('center_axis',(-0.284987069308705,0.601098518635038,-0.746634409347439));
#52794=DIRECTION('ref_axis',(-0.942647507793442,-0.0345386352562879,0.331998130605347));
#52795=DIRECTION('center_axis',(-0.178470279873277,-0.601098531582791,-0.77899224292092));
#52796=DIRECTION('ref_axis',(-0.968259723758394,-0.0335099418156356,0.247689707389773));
#52797=DIRECTION('center_axis',(0.175140532367362,0.601098523279556,0.779747625346313));
#52798=DIRECTION('ref_axis',(-0.969309069137841,-0.033510093144419,0.243550820455579));
#52799=DIRECTION('',(-0.348169904517746,7.77156117238016E-13,-0.937431446873905));
#52800=DIRECTION('center_axis',(-0.31855791089476,0.584827952145615,-0.745987348281143));
#52801=DIRECTION('ref_axis',(-0.932627514626529,-0.0526562728524064,0.356977920732972));
#52802=DIRECTION('center_axis',(-0.288620975689055,6.76985696212227E-10,
-0.9574434356098));
#52803=DIRECTION('ref_axis',(0.957324328213855,0.0157729998150228,-0.288585070796683));
#52804=DIRECTION('',(0.288621063172828,-1.76914038951305E-10,0.957443409237844));
#52805=DIRECTION('',(-0.909057433471482,0.,-0.416670832492798));
#52806=DIRECTION('',(-0.472928816344037,6.51531877903919E-11,0.881100638219851));
#52807=DIRECTION('center_axis',(0.,-1.,1.45983193964168E-32));
#52808=DIRECTION('ref_axis',(1.,0.,0.));
#52809=DIRECTION('center_axis',(-0.196658414391181,0.601098540407601,-0.774600550457459));
#52810=DIRECTION('ref_axis',(-0.957707771787014,0.0514848563389987,0.283099158293531));
#52811=DIRECTION('center_axis',(0.356657049198021,0.601098537525625,0.715175710886434));
#52812=DIRECTION('ref_axis',(-0.910586534296204,0.0525164863478813,0.409968513693552));
#52813=DIRECTION('center_axis',(-0.263663568245725,0.584827930050699,-0.767110041006209));
#52814=DIRECTION('ref_axis',(-0.940205314548717,0.0219594825774785,0.339899614032258));
#52815=DIRECTION('center_axis',(0.406347874870001,-9.95120379307527E-9,
0.913718449298598));
#52816=DIRECTION('ref_axis',(0.913605268826287,-0.0157391393485702,-0.406297541544881));
#52817=DIRECTION('',(-0.406344678315089,4.44089209849855E-13,-0.913719870860324));
#52818=DIRECTION('center_axis',(-0.230078585608708,0.584827952321108,-0.777843242966214));
#52819=DIRECTION('ref_axis',(-0.951568403027054,0.0322834330550571,0.30573739436111));
#52820=DIRECTION('center_axis',(-0.348169832796153,5.70023818185921E-10,
-0.937431473511904));
#52821=DIRECTION('ref_axis',(0.93731590203293,0.0157020800826772,-0.348126908579719));
#52822=DIRECTION('',(0.348169904517199,-8.32667268468792E-13,0.937431446874109));
#52823=DIRECTION('',(-0.933426594325893,0.,-0.358768439254578));
#52824=DIRECTION('center_axis',(0.289010303054396,-0.601098528424121,0.74508630631274));
#52825=DIRECTION('ref_axis',(-0.925593862075092,0.0232723609802456,0.377802064186156));
#52826=DIRECTION('',(-0.416670832492792,0.,0.909057433471485));
#52827=DIRECTION('center_axis',(0.,-1.,1.45983193964168E-32));
#52828=DIRECTION('ref_axis',(1.,0.,0.));
#52829=DIRECTION('center_axis',(-0.292190908012313,0.60109853343636,-0.743844759594095));
#52830=DIRECTION('ref_axis',(-0.924602896651822,0.0212179917817949,0.380341005319974));
#52831=DIRECTION('center_axis',(-0.359709332547123,-0.601098524824285,-0.713645401815616));
#52832=DIRECTION('ref_axis',(-0.900162693631838,0.0222452928133851,0.434985369801238));
#52833=DIRECTION('center_axis',(0.356657114723764,0.601098530486833,0.71517568412488));
#52834=DIRECTION('ref_axis',(-0.902012836724754,0.0222451436298874,0.431135704817691));
#52835=DIRECTION('center_axis',(-0.357729647164783,0.584827953375185,-0.728014947985515));
#52836=DIRECTION('ref_axis',(-0.899954361421966,-0.0078464288985307,0.435913501638939));
#52837=DIRECTION('center_axis',(0.46291631123801,-1.99076621249946E-9,0.886401990515474));
#52838=DIRECTION('ref_axis',(0.886293047250042,-0.0156778482806867,-0.462859416528954));
#52839=DIRECTION('',(-0.462915795308943,0.,-0.886402259955089));
#52840=DIRECTION('center_axis',(-0.325753955539869,0.584827952254261,-0.742873223849276));
#52841=DIRECTION('ref_axis',(-0.915101869160062,0.00246180456567018,0.403215213723443));
#52842=DIRECTION('center_axis',(-0.406344585355985,7.77170922148946E-10,
-0.9137199122006));
#52843=DIRECTION('ref_axis',(0.913607713252797,0.0156707406185981,-0.406294688832453));
#52844=DIRECTION('',(0.406344678315861,-6.37823127618327E-11,0.913719870859981));
#52845=DIRECTION('',(-0.954111946854573,1.64268989064276E-13,-0.299450150892225));
#52846=DIRECTION('center_axis',(0.380115435494561,-0.6010985280191,0.702988488747897));
#52847=DIRECTION('ref_axis',(-0.882085301519085,-0.00691952667751051,0.471038895415808));
#52848=DIRECTION('',(-0.358768439266198,2.35931335548739E-11,0.933426594321426));
#52849=DIRECTION('center_axis',(0.,-1.,1.45983193964168E-32));
#52850=DIRECTION('ref_axis',(1.,0.,0.));
#52851=DIRECTION('center_axis',(-0.38311538656434,0.601098525760556,-0.701358084651587));
#52852=DIRECTION('ref_axis',(-0.880782512520894,-0.00897215952289311,0.473436021011157));
#52853=DIRECTION('center_axis',(-0.35970932549862,-0.601098528958347,-0.713645401886286));
#52854=DIRECTION('ref_axis',(-0.890243636339669,-0.00794566461597056,0.455415342704365));
#52855=DIRECTION('center_axis',(0.356657089597931,0.601098526944953,0.715175699632014));
#52856=DIRECTION('ref_axis',(-0.892181155505171,-0.0079458276464437,0.451607849338861));
#52857=DIRECTION('center_axis',(-0.446153435948076,0.584827952230776,-0.677438837003964));
#52858=DIRECTION('ref_axis',(-0.842141036447412,-0.0181546316901292,0.538951652821915));
#52859=DIRECTION('center_axis',(0.517659926830274,6.26752252576661E-10,
0.855586465621141));
#52860=DIRECTION('ref_axis',(0.855481287509428,-0.0156795066150229,-0.517596290359118));
#52861=DIRECTION('',(-0.517659992379576,2.06170327919809E-7,-0.855586425961478));
#52862=DIRECTION('center_axis',(-0.416297377895457,0.584827782536603,-0.69618457174135));
#52863=DIRECTION('ref_axis',(-0.867894343937951,-0.0273551074107471,0.495995066365645));
#52864=DIRECTION('center_axis',(-0.462915705502022,6.80458439970798E-10,
-0.886402306855959));
#52865=DIRECTION('ref_axis',(0.886293023072826,0.0157023279257069,-0.462858633008119));
#52866=DIRECTION('',(-0.46291579444854,-1.29267404107022E-5,-0.886402260310169));
#52867=DIRECTION('',(-0.971031864912521,-7.62630514899288E-8,-0.238950031020097));
#52868=DIRECTION('center_axis',(0.517659995141469,1.97424267101112E-12,
0.85558642429046));
#52869=DIRECTION('ref_axis',(0.660406837962033,-0.635772805084829,-0.399569454147282));
#52870=DIRECTION('',(0.299450150892762,0.,-0.954111946854405));
#52871=DIRECTION('center_axis',(-0.520704586498207,0.398564391553765,-0.754992158492463));
#52872=DIRECTION('ref_axis',(-0.823202421105205,4.20107565333048E-17,0.567747984484779));
#52873=DIRECTION('center_axis',(0.576093384093487,5.7445652595911E-5,0.817383881357903));
#52874=DIRECTION('ref_axis',(0.817383840831677,-0.000363133212873767,-0.576093330009579));
#52875=DIRECTION('',(-0.570360475446356,5.94973691578862E-5,-0.821394499925991));
#52876=DIRECTION('center_axis',(-0.405137316619699,0.590180063805294,-0.698248699940766));
#52877=DIRECTION('ref_axis',(0.437157251884037,0.795820196456205,0.41900328404155));
#52878=DIRECTION('center_axis',(-0.822705653767276,0.550037558032886,0.143576084403282));
#52879=DIRECTION('ref_axis',(-0.555796003831724,-0.831318712723758,1.13199349268201E-16));
#52880=DIRECTION('center_axis',(0.155987445281772,-0.477126091130184,-0.864880691238565));
#52881=DIRECTION('ref_axis',(0.968621986494132,-0.0976332342635064,0.228558961424418));
#52882=DIRECTION('center_axis',(0.0450737363500213,0.584827951390675,-0.809904084175179));
#52883=DIRECTION('ref_axis',(-0.998983642787651,0.0265489689862998,-0.0364257283864013));
#52884=DIRECTION('center_axis',(0.0414470066457046,-1.35743970630672E-11,
0.999140703624925));
#52885=DIRECTION('ref_axis',(0.999016806408817,-0.0157477670559316,-0.0414418670607522));
#52886=DIRECTION('center_axis',(0.0122720119993164,-0.000115441169559691,
-0.999924689361567));
#52887=DIRECTION('ref_axis',(0.0248707036530095,0.99969065818745,0.000189822410529044));
#52888=DIRECTION('',(-0.0213713417294297,-6.06514838087198E-10,0.999771606794614));
#52889=DIRECTION('center_axis',(-0.0132941993870834,-0.601098528157791,
0.799064342659084));
#52890=DIRECTION('ref_axis',(-0.999600535579284,0.0279220105392125,0.00437385379914484));
#52891=DIRECTION('',(-0.722057103549597,2.24206636476414E-10,0.691833462051068));
#52892=DIRECTION('center_axis',(0.,-1.,1.45983193964168E-32));
#52893=DIRECTION('ref_axis',(1.,0.,0.));
#52894=DIRECTION('center_axis',(0.00988022332258178,0.601098534236258,-0.799113842531912));
#52895=DIRECTION('ref_axis',(-0.999640204045365,0.0258667124555254,0.0070975800723927));
#52896=DIRECTION('center_axis',(-0.079429416547992,-0.60109852376284,-0.795217915113197));
#52897=DIRECTION('ref_axis',(-0.996495527177138,0.0268944696049595,0.0792044936895975));
#52898=DIRECTION('center_axis',(0.0760312438730437,0.601098530830715,0.795550002318065));
#52899=DIRECTION('ref_axis',(-0.996824817208516,0.0268943149207247,0.0749465117410669));
#52900=DIRECTION('center_axis',(-0.0567895989104308,0.58482795222283,-0.80916698385095));
#52901=DIRECTION('ref_axis',(-0.997702834767716,-0.00326197145638583,0.0676639714965141));
#52902=DIRECTION('center_axis',(0.104101880233295,-7.42459677259694E-10,
0.994566638557665));
#52903=DIRECTION('ref_axis',(0.994444317549335,-0.0156832196312127,-0.104089076832476));
#52904=DIRECTION('',(-0.104101784680852,8.32143748321909E-8,-0.994566648559188));
#52905=DIRECTION('center_axis',(-0.0215738989994039,0.584827969932201,-0.810870404236672));
#52906=DIRECTION('ref_axis',(-0.999473463626067,0.00704480132966553,0.031672800342533));
#52907=DIRECTION('center_axis',(-0.0414469282271476,6.03116713776065E-10,
-0.999140706877932));
#52908=DIRECTION('ref_axis',(0.999018006468192,0.0156715280543576,-0.0414418382888709));
#52909=DIRECTION('',(0.0414470083234698,-1.48214773785843E-11,0.999140703555327));
#52910=DIRECTION('',(-0.776875910350776,-3.07809289802272E-8,-0.629653730169728));
#52911=DIRECTION('center_axis',(-0.603761736552382,0.793626260383761,0.075027490325471));
#52912=DIRECTION('ref_axis',(-0.795869445650856,-0.605468269589249,3.41264943846719E-17));
#52913=DIRECTION('center_axis',(0.532481211718397,0.471546674499199,-0.702927800656408));
#52914=DIRECTION('ref_axis',(0.840419115869136,-0.393420680742697,0.372714203708004));
#52915=DIRECTION('center_axis',(0.086959942795448,-0.601098528044268,0.794429687217205));
#52916=DIRECTION('ref_axis',(-0.994244551277268,-0.00227572098346056,0.107110192556405));
#52917=DIRECTION('',(-0.677191706199959,5.05127141378919E-12,0.735806627487133));
#52918=DIRECTION('center_axis',(0.,-1.,1.45983193964168E-32));
#52919=DIRECTION('ref_axis',(1.,0.,0.));
#52920=DIRECTION('center_axis',(-0.0903532064474036,0.601098527152084,-0.794050916969603));
#52921=DIRECTION('ref_axis',(-0.993941854728559,-0.00432812185830315,0.109821932144412));
#52922=DIRECTION('center_axis',(-0.0794293726861269,-0.601098528292757,
-0.795217916070161));
#52923=DIRECTION('ref_axis',(-0.994793314994779,-0.00330177835730735,0.101859504717909));
#52924=DIRECTION('center_axis',(0.0760312337800567,0.601098527673595,0.795550005668103));
#52925=DIRECTION('ref_axis',(-0.995219400801409,-0.00330191285651983,0.0976086145787));
#52926=DIRECTION('center_axis',(-0.157748271170264,0.584828255987902,-0.795670405344413));
#52927=DIRECTION('ref_axis',(-0.984730155966502,-0.033081541071693,0.17091556854339));
#52928=DIRECTION('center_axis',(0.166379301644552,-1.08060781329185E-7,
0.986061827668154));
#52929=DIRECTION('ref_axis',(0.985940676947419,-0.0156751635313546,-0.166358861467401));
#52930=DIRECTION('',(-0.166345721445974,0.,-0.986067493104107));
#52931=DIRECTION('center_axis',(-0.123030317275551,0.584827952226511,-0.801772915061131));
#52932=DIRECTION('ref_axis',(-0.990530551576628,-0.0227607295753553,0.135392671819783));
#52933=DIRECTION('center_axis',(-0.104101721443439,4.93313746308513E-10,
-0.994566655178281));
#52934=DIRECTION('ref_axis',(0.994444175453534,0.0156933905082854,-0.104088901429955));
#52935=DIRECTION('',(0.104101785979735,-2.28705943069056E-11,0.994566648423236));
#52936=DIRECTION('',(-0.814879198737184,1.43735365431383E-13,-0.579630823425951));
#52937=DIRECTION('center_axis',(0.185842686022657,-0.601098527830234,0.77726639956466));
#52938=DIRECTION('ref_axis',(-0.977463691313877,-0.0324816898131399,0.208589721678543));
#52939=DIRECTION('',(-0.629653742645588,8.00811321699454E-12,0.776875900239159));
#52940=DIRECTION('center_axis',(0.,-1.,1.45983193964168E-32));
#52941=DIRECTION('ref_axis',(1.,0.,0.));
#52942=DIRECTION('center_axis',(-0.189161734660047,0.6010985193897,-0.776465329636754));
#52943=DIRECTION('ref_axis',(-0.9768248540831,-0.0345386219249532,0.211235148687562));
#52944=DIRECTION('center_axis',(-0.0794293717565466,-0.601098531586404,
-0.795217913673371));
#52945=DIRECTION('ref_axis',(-0.991668458571965,-0.0335099417813519,0.124381478023516));
#52946=DIRECTION('center_axis',(0.076031206768239,0.601098523311899,0.795550011545233));
#52947=DIRECTION('ref_axis',(-0.992190789392835,-0.0335100925034672,0.120143710382328));
#52948=DIRECTION('',(-0.227933166345721,0.,-0.973676779881093));
#52949=DIRECTION('center_axis',(-0.222548980029614,0.584827952147113,-0.780030908281969));
#52950=DIRECTION('ref_axis',(-0.970014665235007,-0.0526562728337964,0.237273821059698));
#52951=DIRECTION('center_axis',(-0.166345655494771,4.83957742611337E-10,
-0.986067504229814));
#52952=DIRECTION('ref_axis',(0.985944835955002,0.015772999814884,-0.166324961838274));
#52953=DIRECTION('',(0.166345721448234,-1.76914038951275E-10,0.986067493103726));
#52954=DIRECTION('',(-0.849666541317971,0.,-0.527320366157762));
#52955=DIRECTION('',(-0.579630823453725,6.51326541667441E-11,0.814879198717428));
#52956=DIRECTION('center_axis',(0.,-1.,1.45983193964168E-32));
#52957=DIRECTION('ref_axis',(1.,0.,0.));
#52958=DIRECTION('center_axis',(-0.098024518104039,0.601098540713194,-0.793140427795065));
#52959=DIRECTION('ref_axis',(-0.985637692309511,0.051484852820372,0.160834229655403));
#52960=DIRECTION('center_axis',(0.264209415125226,0.601098537645921,0.754237318752606));
#52961=DIRECTION('ref_axis',(-0.954788967611246,0.0525164848971561,0.292609032912346));
#52962=DIRECTION('center_axis',(-0.165440120329679,0.584827930051102,-0.794106956786959));
#52963=DIRECTION('ref_axis',(-0.975392232529833,0.0219594825708578,0.219380431774778));
#52964=DIRECTION('center_axis',(0.288624384642661,-9.72083670309824E-9,
0.957442407975355));
#52965=DIRECTION('ref_axis',(0.957323811526494,-0.015739139347579,-0.288588633485421));
#52966=DIRECTION('',(-0.288621063170532,3.88578058618535E-13,-0.957443409238537));
#52967=DIRECTION('center_axis',(-0.130774738400328,0.584827952321201,-0.800546209771876));
#52968=DIRECTION('ref_axis',(-0.982384058205275,0.0322834330508441,0.184063418784358));
#52969=DIRECTION('center_axis',(-0.227933087277152,6.06662003836226E-10,
-0.973676798390671));
#52970=DIRECTION('ref_axis',(0.973556758396492,0.0157020800821283,-0.227904986478159));
#52971=DIRECTION('',(0.227933166345052,-3.88578058618627E-13,0.973676779881249));
#52972=DIRECTION('',(-0.881100638236031,-1.64268989064337E-13,-0.472928816313892));
#52973=DIRECTION('center_axis',(0.193347282237507,-0.601098528136115,0.775433677321256));
#52974=DIRECTION('ref_axis',(-0.965646434806065,0.0232723685696349,0.258815300566825));
#52975=DIRECTION('',(-0.527320366157789,0.,0.849666541317955));
#52976=DIRECTION('center_axis',(0.,-1.,1.45983193964168E-32));
#52977=DIRECTION('ref_axis',(1.,0.,0.));
#52978=DIRECTION('center_axis',(-0.196658433615245,0.601098533602547,-0.77460055085758));
#52979=DIRECTION('ref_axis',(-0.964981493238737,0.0212179873045292,0.26145843784717));
#52980=DIRECTION('center_axis',(-0.267429420305788,-0.601098525088523,-0.753101632113032));
#52981=DIRECTION('ref_axis',(-0.947582767948786,0.0222452859069907,0.318735070460458));
#52982=DIRECTION('center_axis',(0.264209492842463,0.601098530326073,0.754237297361887));
#52983=DIRECTION('ref_axis',(-0.948935826115031,0.0222451481022262,0.314683891073716));
#52984=DIRECTION('center_axis',(-0.263664252983005,0.584827954381707,-0.767109787105224));
#52985=DIRECTION('ref_axis',(-0.947492435019574,-0.00784635387838365,0.319681904885925));
#52986=DIRECTION('center_axis',(0.348170767516168,-2.42832855999574E-9,
0.937431126348599));
#52987=DIRECTION('ref_axis',(0.937315911348809,-0.0156778481980674,-0.348127975618494));
#52988=DIRECTION('',(-0.348169904517986,0.,-0.937431446873816));
#52989=DIRECTION('center_axis',(-0.230078585026532,0.584827952254463,-0.777843243188524));
#52990=DIRECTION('ref_axis',(-0.958422284152977,0.00246180456700299,0.285343065023952));
#52991=DIRECTION('center_axis',(-0.288621003383784,4.69944830746473E-10,
-0.957443427261234));
#52992=DIRECTION('ref_axis',(0.957325859343011,0.0156707406186114,-0.288585562566163));
#52993=DIRECTION('',(0.288621063170873,-6.42264019715572E-11,0.957443409238434));
#52994=DIRECTION('',(-0.90905743347151,1.64268989064311E-13,-0.416670832492738));
#52995=DIRECTION('center_axis',(0.28901028694578,-0.601098528046295,0.745086312865895));
#52996=DIRECTION('ref_axis',(-0.934166624693501,-0.00691952387371952,0.356770006444086));
#52997=DIRECTION('',(-0.472928816324628,2.3449398189427E-11,0.881100638230269));
#52998=DIRECTION('center_axis',(0.,-1.,1.45983193964168E-32));
#52999=DIRECTION('ref_axis',(1.,0.,0.));
#53000=DIRECTION('center_axis',(-0.292190927015802,0.601098525790784,-0.743844758307668));
#53001=DIRECTION('ref_axis',(-0.933174547879557,-0.00897215717209348,0.359311513293776));
#53002=DIRECTION('center_axis',(-0.26742942804773,-0.60109852898886,-0.753101626250729));
#53003=DIRECTION('ref_axis',(-0.940302475780628,-0.00794566216052988,0.340247146194722));
#53004=DIRECTION('center_axis',(0.264209457521186,0.601098526927667,0.754237312443338));
#53005=DIRECTION('ref_axis',(-0.941747513064489,-0.00794582853994121,0.336226836296069));
#53006=DIRECTION('center_axis',(-0.357729782847908,0.58482795223096,-0.728014882233139));
#53007=DIRECTION('ref_axis',(-0.903049056228438,-0.0181546316809015,0.429153598835497));
#53008=DIRECTION('center_axis',(0.406344760815415,-7.08143957842295E-10,
0.91371983417121));
#53009=DIRECTION('ref_axis',(0.913607509655577,-0.0156795066176049,-0.406294808449681));
#53010=DIRECTION('',(-0.406344675363295,2.06171937743088E-7,-0.913719872173007));
#53011=DIRECTION('center_axis',(-0.325759685202577,0.584827782536742,-0.742870844945389));
#53012=DIRECTION('ref_axis',(-0.923215403305287,-0.0273551074156397,0.383307992609254));
#53013=DIRECTION('center_axis',(-0.34816980557852,7.1282886651966E-10,-0.937431483620758));
#53014=DIRECTION('ref_axis',(0.937315908492689,0.0157023279253457,-0.348126880008208));
#53015=DIRECTION('',(-0.348169903619823,-1.29267404106986E-5,-0.937431447118275));
#53016=DIRECTION('',(-0.933426608576392,-7.6262907754578E-8,-0.358768402178298));
#53017=DIRECTION('center_axis',(0.406344678308733,5.73812350350916E-12,
0.91371987086315));
#53018=DIRECTION('ref_axis',(0.70527866451459,-0.635772805084979,-0.313647805181057));
#53019=DIRECTION('',(0.416670832493319,0.,-0.909057433471244));
#53020=DIRECTION('center_axis',(-0.421973066766652,0.398564391555568,-0.814300409374505));
#53021=DIRECTION('ref_axis',(-0.887868914881341,-7.97986771087996E-17,0.460096500733737));
#53022=DIRECTION('center_axis',(0.469105350796176,5.74456488072083E-5,0.883142211964978));
#53023=DIRECTION('ref_axis',(0.883142165012923,-0.000363020440370894,-0.469105302242948));
#53024=DIRECTION('',(-0.462914984031325,5.94973683763289E-5,-0.886402681640428));
#53025=DIRECTION('center_axis',(-0.314428920608558,0.590180063809988,-0.743519970253775));
#53026=DIRECTION('ref_axis',(0.381196510278465,0.795819976664742,0.470488879032066));
#53027=DIRECTION('center_axis',(-0.834213228879005,0.550037558031181,0.0393315842340603));
#53028=DIRECTION('ref_axis',(-0.550463499052738,-0.834859231374138,7.73147444792113E-19));
#53029=DIRECTION('center_axis',(0.26315573158457,-0.477126089798436,-0.838510438437021));
#53030=DIRECTION('ref_axis',(0.932339990205128,-0.0976265035258249,0.348154001088059));
#53031=DIRECTION('center_axis',(0.14622621420636,0.584827951391204,-0.797868511441856));
#53032=DIRECTION('ref_axis',(-0.986541004061149,0.0265489689768779,-0.16134435085334));
#53033=DIRECTION('center_axis',(-0.0841053527532984,9.82782766916969E-12,
0.996456867926677));
#53034=DIRECTION('ref_axis',(0.996333303516304,-0.0157477670566241,0.0840949233724572));
#53035=DIRECTION('center_axis',(0.137499035826066,-0.000115441193923135,
-0.990501893900377));
#53036=DIRECTION('ref_axis',(0.0246629893145987,0.999690351939331,0.00330714340248807));
#53037=DIRECTION('',(-0.14650743062218,-6.06126260029117E-10,0.98920956969314));
#53038=DIRECTION('center_axis',(-0.113338700331315,-0.601098527834891,0.791097275208261));
#53039=DIRECTION('ref_axis',(-0.992266574683714,0.0279220176816331,-0.120943812136201));
#53040=DIRECTION('',(-0.803073192506799,2.24206636476386E-10,0.595880396956418));
#53041=DIRECTION('center_axis',(0.,-1.,1.45983193964168E-32));
#53042=DIRECTION('ref_axis',(1.,0.,0.));
#53043=DIRECTION('center_axis',(0.109957851633899,0.601098533843261,-0.791574269083792));
#53044=DIRECTION('ref_axis',(-0.992647303462575,0.0258667215027917,-0.118246537569502));
#53045=DIRECTION('center_axis',(0.0208641544658999,-0.601098524137728,-0.79890252930997));
#53046=DIRECTION('ref_axis',(-0.998564817328578,0.0268944613826216,-0.0463140749716835));
#53047=DIRECTION('center_axis',(-0.0242771357386957,0.601098530732607,0.79880609476357));
#53048=DIRECTION('ref_axis',(-0.998357844538717,0.0268943171535404,-0.0505797385605408));
#53049=DIRECTION('center_axis',(0.0450737186086209,0.584827952222913,-0.809904084561589));
#53050=DIRECTION('ref_axis',(-0.998316194260093,-0.00326197146239322,-0.0579149015385696));
#53051=DIRECTION('center_axis',(-0.0213712893727949,-4.10500129431464E-10,
0.9997716079138));
#53052=DIRECTION('ref_axis',(0.999648646751534,-0.0156832196310207,0.0213686609274604));
#53053=DIRECTION('',(0.0213713430443167,8.32140417652696E-8,-0.999771606766503));
#53054=DIRECTION('center_axis',(0.080225227444987,0.584827969931439,-0.807180375422539));
#53055=DIRECTION('ref_axis',(-0.995561971316665,0.00704480135439165,-0.0938441902408085));
#53056=DIRECTION('center_axis',(0.0841054060144577,4.23273412101713E-10,
-0.996456863431199));
#53057=DIRECTION('ref_axis',(0.996334492612421,0.0156715280540825,0.0840950773779236));
#53058=DIRECTION('',(-0.0841053488789075,-1.40443212613677E-11,0.996456868253693));
#53059=DIRECTION('',(-0.69183347372805,-3.07809289802329E-8,-0.722057092361385));
#53060=DIRECTION('center_axis',(-0.608404332892848,0.79362626038425,-0.00123553458889862));
#53061=DIRECTION('ref_axis',(-0.793626866138329,-0.608404797271895,-2.90994740798271E-19));
#53062=DIRECTION('center_axis',(0.616382652636135,0.471546674578011,-0.630647412762204));
#53063=DIRECTION('ref_axis',(0.78707911312239,-0.393406599041741,0.475118635202708));
#53064=DIRECTION('center_axis',(-0.0132942036922927,-0.601098528044386,
0.799064342672766));
#53065=DIRECTION('ref_axis',(-0.999829102807158,-0.00227572108321212,-0.0183462877276236));
#53066=DIRECTION('',(-0.764072871230124,5.05127141378843E-12,0.645129946173757));
#53067=DIRECTION('center_axis',(0.,-1.,1.45983193964168E-32));
#53068=DIRECTION('ref_axis',(1.,0.,0.));
#53069=DIRECTION('center_axis',(0.00988022742892383,0.601098527162617,-0.79911384780198));
#53070=DIRECTION('ref_axis',(-0.999868664172006,-0.00432812016876069,-0.015617995476148));
#53071=DIRECTION('center_axis',(0.0208641859867265,-0.601098528288371,-0.798902525363805));
#53072=DIRECTION('ref_axis',(-0.999715453639247,-0.00330177928429916,-0.0236243520214359));
#53073=DIRECTION('center_axis',(-0.0242771432463745,0.60109852769626,0.798806096820238));
#53074=DIRECTION('ref_axis',(-0.999605402018444,-0.00330190886658757,-0.0278951188092559));
#53075=DIRECTION('center_axis',(-0.0567768155313816,0.584828375911606,-0.809167574700512));
#53076=DIRECTION('ref_axis',(-0.998386871228108,-0.0330794214893115,0.0461455006829729));
#53077=DIRECTION('center_axis',(0.0414944557150844,-1.50624413674013E-7,
0.999138734183039));
#53078=DIRECTION('ref_axis',(0.999015977020359,-0.0156751609036203,-0.0414893599456838));
#53079=DIRECTION('',(-0.041447008323888,-4.4408920985015E-13,-0.99914070355531));
#53080=DIRECTION('center_axis',(-0.0215713945108209,0.584827952225678,-0.810870483637417));
#53081=DIRECTION('ref_axis',(-0.999689123679031,-0.0227607296123229,0.0101786632406399));
#53082=DIRECTION('center_axis',(0.0213714187153477,5.88437628125681E-10,
-0.999771605148943));
#53083=DIRECTION('ref_axis',(0.999648484439658,0.0156933905086753,0.0213687868592492));
#53084=DIRECTION('',(-0.0213713417386148,-2.36477504241347E-11,0.999771606794418));
#53085=DIRECTION('',(-0.735806627489112,0.,-0.677191706197809));
#53086=DIRECTION('center_axis',(0.0869599425730912,-0.601098528069535,0.794429687222427));
#53087=DIRECTION('ref_axis',(-0.995899323085398,-0.0324816854912687,0.0844362385809061));
#53088=DIRECTION('',(-0.722057103471557,8.1518485824276E-12,0.691833462132518));
#53089=DIRECTION('center_axis',(0.,-1.,1.45983193964168E-32));
#53090=DIRECTION('ref_axis',(1.,0.,0.));
#53091=DIRECTION('center_axis',(-0.090353228593366,0.601098519348321,-0.794050920357134));
#53092=DIRECTION('ref_axis',(-0.99559708246167,-0.0345386226702202,0.0871408798317705));
#53093=DIRECTION('center_axis',(0.0208641849024253,-0.601098531590183,-0.798902522907822));
#53094=DIRECTION('ref_axis',(-0.999437989418741,-0.033509941682649,-0.000888321478876713));
#53095=DIRECTION('center_axis',(-0.0242771705949099,0.601098523543119,0.79880609911429));
#53096=DIRECTION('ref_axis',(-0.999425068545745,-0.0335100884017672,-0.00515813315444326));
#53097=DIRECTION('',(-0.104101785979609,-4.44089209850367E-13,-0.99456664842325));
#53098=DIRECTION('center_axis',(-0.123030318860491,0.584827952146009,-0.801772914876645));
#53099=DIRECTION('ref_axis',(-0.992104105100685,-0.0526562728490771,0.113827771532309));
#53100=DIRECTION('center_axis',(-0.0414469425911784,4.75766052612418E-10,
-0.999140706282075));
#53101=DIRECTION('ref_axis',(0.99901641168037,0.0157729998146264,-0.0414417865218749));
#53102=DIRECTION('',(0.0414470083264018,-1.77746706219692E-10,0.999140703555206));
#53103=DIRECTION('',(-0.776875900241758,0.,-0.629653742642381));
#53104=DIRECTION('',(-0.677191706222999,6.51326541667412E-11,0.735806627465928));
#53105=DIRECTION('center_axis',(0.,-1.,1.45983193964168E-32));
#53106=DIRECTION('ref_axis',(1.,0.,0.));
#53107=DIRECTION('center_axis',(0.00215530640688391,0.601098539803382,-0.799172009082234));
#53108=DIRECTION('ref_axis',(-0.998023518743271,0.0514848633080921,0.0360328306610393));
#53109=DIRECTION('center_axis',(0.167595042660841,0.601098537659878,0.781404152598812));
#53110=DIRECTION('ref_axis',(-0.98393380773214,0.0525164847285,0.170634934387698));
#53111=DIRECTION('center_axis',(-0.0646072654724011,0.584827923044615,-0.808580361915562));
#53112=DIRECTION('ref_axis',(-0.995196652942778,0.021959669079551,0.0954012311524769));
#53113=DIRECTION('center_axis',(0.166350249831606,-1.30064135257624E-8,
0.986066729172505));
#53114=DIRECTION('ref_axis',(0.985944587101618,-0.0157391391447165,-0.166329644573669));
#53115=DIRECTION('',(-0.166345721445869,3.88578058619102E-13,-0.986067493104125));
#53116=DIRECTION('center_axis',(-0.0294084954082734,0.584827952319998,-0.81062408463049));
#53117=DIRECTION('ref_axis',(-0.997706929940489,0.0322834330689216,0.0594866531081364));
#53118=DIRECTION('center_axis',(-0.104101714517271,5.33328897972409E-10,
-0.994566655903245));
#53119=DIRECTION('ref_axis',(0.994444040496267,0.0157020800824344,-0.104088880302097));
#53120=DIRECTION('',(0.104101785979298,-1.22124532708759E-12,0.994566648423282));
#53121=DIRECTION('',(-0.814879198737126,0.,-0.579630823426032));
#53122=DIRECTION('center_axis',(0.0946350700368982,-0.601098528112436,0.793551991378116));
#53123=DIRECTION('ref_axis',(-0.990470182848417,0.023272369138899,0.135746873713121));
#53124=DIRECTION('',(-0.629653742642369,0.,0.776875900241768));
#53125=DIRECTION('center_axis',(0.,-1.,1.45983193964168E-32));
#53126=DIRECTION('ref_axis',(1.,0.,0.));
#53127=DIRECTION('center_axis',(-0.0980245238225754,0.601098533435455,-0.7931404326039));
#53128=DIRECTION('ref_axis',(-0.990141758144127,0.0212179918813064,0.138452503046286));
#53129=DIRECTION('center_axis',(-0.170932004530704,-0.60109852490719,-0.780680993224195));
#53130=DIRECTION('ref_axis',(-0.980058890457948,0.0222452907071548,0.197458143097949));
#53131=DIRECTION('center_axis',(0.167595116543381,0.601098530461403,0.781404142289988));
#53132=DIRECTION('ref_axis',(-0.980893534367322,0.0222451443138458,0.193269314146968));
#53133=DIRECTION('center_axis',(-0.165440957226946,0.584827953375188,-0.794106765254409));
#53134=DIRECTION('ref_axis',(-0.980087919791214,-0.0078464289079487,0.198408928813002));
#53135=DIRECTION('center_axis',(0.227933641184126,-1.25033758461367E-9,
0.973676668723528));
#53136=DIRECTION('ref_axis',(0.973556998972359,-0.0156778482793224,-0.22790562701536));
#53137=DIRECTION('',(-0.227933166345836,3.88578058618775E-13,-0.973676779881066));
#53138=DIRECTION('center_axis',(-0.130774737773183,0.584827952254203,-0.800546209923269));
#53139=DIRECTION('ref_axis',(-0.986627807192036,0.00246180457580221,0.162970885723999));
#53140=DIRECTION('center_axis',(-0.166345641911318,6.12618273329711E-10,
-0.986067506521289));
#53141=DIRECTION('ref_axis',(0.985946423748941,0.0156707406188289,-0.166325215722484));
#53142=DIRECTION('',(0.16634572144638,-6.41708908203574E-11,0.986067493104039));
#53143=DIRECTION('',(-0.849666541318022,1.64268989064345E-13,-0.527320366157681));
#53144=DIRECTION('center_axis',(0.193347264597227,-0.60109852814683,0.775433681711392));
#53145=DIRECTION('ref_axis',(-0.971515582976909,-0.00691951581125515,0.23687463421391));
#53146=DIRECTION('',(-0.579630823436063,2.36136671785042E-11,0.814879198729991));
#53147=DIRECTION('center_axis',(0.,-1.,1.45983193964168E-32));
#53148=DIRECTION('ref_axis',(1.,0.,0.));
#53149=DIRECTION('center_axis',(-0.196658430624571,0.60109852592005,-0.774600557578565));
#53150=DIRECTION('ref_axis',(-0.970849864666905,-0.00897214799424333,0.239520439287802));
#53151=DIRECTION('center_axis',(-0.17093200004291,-0.60109852895254,-0.780680991092023));
#53152=DIRECTION('ref_axis',(-0.975532185834689,-0.00794566528748167,0.219713041951845));
#53153=DIRECTION('center_axis',(0.167595094659997,0.601098527004474,0.781404149642781));
#53154=DIRECTION('ref_axis',(-0.976461947719334,-0.00794582307778729,0.215543333350353));
#53155=DIRECTION('center_axis',(-0.263664517425136,0.584827952230139,-0.767109697853751));
#53156=DIRECTION('ref_axis',(-0.949715452919976,-0.0181546317036599,0.312587536272178));
#53157=DIRECTION('center_axis',(0.288621117749965,-4.46288586079944E-10,
0.957443392785579));
#53158=DIRECTION('ref_axis',(0.957325693290781,-0.0156795066178608,-0.288585637268293));
#53159=DIRECTION('',(-0.288621060077174,2.06171493654015E-7,-0.957443410171006));
#53160=DIRECTION('center_axis',(-0.230084567678364,0.58482778253655,-0.777841601156458));
#53161=DIRECTION('ref_axis',(-0.96397680426132,-0.0273551074224977,0.264575922835083));
#53162=DIRECTION('center_axis',(-0.227933076190557,6.11666218383047E-10,
-0.973676800985989));
#53163=DIRECTION('ref_axis',(0.9735567572018,0.0157023279251935,-0.227904974505702));
#53164=DIRECTION('',(-0.227933165424191,-1.29267396645822E-5,-0.973676780011009));
#53165=DIRECTION('',(-0.881100657021103,-7.62629077545992E-8,-0.472928781315934));
#53166=DIRECTION('center_axis',(0.288621063162946,6.19194292263073E-12,
0.957443409240823));
#53167=DIRECTION('ref_axis',(0.739027825212226,-0.635772805085107,-0.222779742966684));
#53168=DIRECTION('',(0.527320366158135,0.,-0.84966654131774));
#53169=DIRECTION('center_axis',(-0.316586779698294,0.398564391555877,-0.860766656361617));
#53170=DIRECTION('ref_axis',(2.94490590170337E-16,0.907442263779439,0.420176793631974));
#53171=DIRECTION('center_axis',(0.35471924586863,5.74456547725441E-5,0.934972862339002));
#53172=DIRECTION('ref_axis',(0.93497280964334,-0.000363109780049791,-0.354719203566606));
#53173=DIRECTION('',(-0.348169046786133,5.94973699394781E-5,-0.937431763554073));
#53174=DIRECTION('center_axis',(-0.218761792525728,0.590180063808641,-0.777065486567097));
#53175=DIRECTION('ref_axis',(0.319217807250868,0.795820705788151,0.514557475674775));
#53176=DIRECTION('center_axis',(-0.832564763033601,0.550037558033772,-0.0655331985107512));
#53177=DIRECTION('ref_axis',(-0.551222471627934,-0.834358308385787,-6.13931407995218E-17));
#53178=DIRECTION('center_axis',(0.366173894521264,-0.477126090432259,-0.798916374096788));
#53179=DIRECTION('ref_axis',(0.881350386866143,-0.0976339845307942,0.462265184321229));
#53180=DIRECTION('center_axis',(0.245072617384947,0.584827951389285,-0.773250075642999));
#53181=DIRECTION('ref_axis',(-0.95854002435476,0.026548969010481,-0.283718476582785));
#53182=DIRECTION('center_axis',(-0.208331315235233,-3.25592671745016E-11,
0.978058312725963));
#53183=DIRECTION('ref_axis',(0.977937029805949,-0.015747767057039,0.208305481365794));
#53184=DIRECTION('center_axis',(0.260557615828758,-0.00011544123373398,
-0.965458292991963));
#53185=DIRECTION('ref_axis',(0.0240700430029388,0.999689938683564,0.00637648215625154));
#53186=DIRECTION('',(-0.269333009814431,-6.06514838087046E-10,0.963047106752468));
#53187=DIRECTION('center_axis',(-0.211595760985938,-0.601098528097979,0.770654133480918));
#53188=DIRECTION('ref_axis',(-0.969283979365573,0.0279220118464045,-0.244354104937259));
#53189=DIRECTION('',(-0.871424337485721,2.24206636476429E-10,0.490529942039803));
#53190=DIRECTION('center_axis',(0.,-1.,1.45983193964168E-32));
#53191=DIRECTION('ref_axis',(1.,0.,0.));
#53192=DIRECTION('center_axis',(0.208301364394399,0.601098533826222,-0.771551096314041));
#53193=DIRECTION('ref_axis',(-0.969999761963384,0.0258667218163505,-0.241725825044521));
#53194=DIRECTION('center_axis',(0.120828674064531,-0.60109852420491,-0.789987971884691));
#53195=DIRECTION('ref_axis',(-0.984886142419322,0.026894459919668,-0.171102234047416));
#53196=DIRECTION('center_axis',(-0.124202644056001,0.601098530459505,0.789464539981957));
#53197=DIRECTION('ref_axis',(-0.984146173822937,0.0268943232999321,-0.175308311052021));
#53198=DIRECTION('center_axis',(0.146226196685621,0.58482795222256,-0.797868514043527));
#53199=DIRECTION('ref_axis',(-0.983185511002024,-0.00326197145263899,-0.182580422000639));
#53200=DIRECTION('center_axis',(-0.146507360718647,-5.54529865880287E-10,
0.989209580046239));
#53201=DIRECTION('ref_axis',(0.989087917901018,-0.015683219631045,0.146489341879311));
#53202=DIRECTION('',(0.146507431922858,8.32148189213204E-8,-0.989209569500499));
#53203=DIRECTION('center_axis',(0.180759154061358,0.584827969932013,-0.790760629905298));
#53204=DIRECTION('ref_axis',(-0.975949872003341,0.00704480134002263,-0.217881201829672));
#53205=DIRECTION('center_axis',(0.208331415279698,7.80545475967607E-10,
-0.978058291415986));
#53206=DIRECTION('ref_axis',(0.977938180049076,0.0156715280545262,0.208305830957121));
#53207=DIRECTION('',(-0.208331314487837,-1.44328993199869E-11,0.978058312885162));
#53208=DIRECTION('',(-0.595880409943332,-3.07809289802393E-8,-0.803073182870507));
#53209=DIRECTION('center_axis',(-0.603452029460871,0.793626260384574,-0.0774790743849719));
#53210=DIRECTION('ref_axis',(-0.796019110999669,-0.605271488609282,-3.39050861409775E-17));
#53211=DIRECTION('center_axis',(0.690563370785492,0.4715466745671,-0.548421338602072));
#53212=DIRECTION('ref_axis',(0.721326027536678,-0.393427780058085,0.570002933217648));
#53213=DIRECTION('center_axis',(-0.113338608937478,-0.601098527844478,0.791097288294758));
#53214=DIRECTION('ref_axis',(-0.989645761738707,-0.00227577203245932,-0.143513369183052));
#53215=DIRECTION('',(-0.838904150647018,7.57690712069459E-12,0.544279180225742));
#53216=DIRECTION('center_axis',(0.,-1.,1.45983193964168E-32));
#53217=DIRECTION('ref_axis',(1.,0.,0.));
#53218=DIRECTION('center_axis',(0.109957852882409,0.601098527208925,-0.791574273948284));
#53219=DIRECTION('ref_axis',(-0.990026945959674,-0.00432811321328217,-0.140811624909925));
#53220=DIRECTION('center_axis',(0.120828705633355,-0.60109852827952,-0.789987963955884));
#53221=DIRECTION('ref_axis',(-0.988871481869316,-0.00330178122241446,-0.148735639933211));
#53222=DIRECTION('center_axis',(-0.124202642833808,0.601098527766976,0.78946454222433));
#53223=DIRECTION('ref_axis',(-0.988227031801981,-0.00330189731720042,-0.152958919615538));
#53224=DIRECTION('center_axis',(0.0450828641671435,0.584828255987828,-0.809903356183145));
#53225=DIRECTION('ref_axis',(-0.996298020780763,-0.0330815410749405,-0.0793464897045918));
#53226=DIRECTION('center_axis',(-0.0840714188105122,-1.08029305018116E-7,
0.99645973151913));
#53227=DIRECTION('ref_axis',(0.99633730370572,-0.0156751635313067,0.0840610878628315));
#53228=DIRECTION('',(0.0841053488787466,4.44089209849881E-13,-0.996456868253706));
#53229=DIRECTION('center_axis',(0.0802277221187175,0.584827952226099,-0.807180140302442));
#53230=DIRECTION('ref_axis',(-0.993082001121473,-0.0227607295978636,-0.115195869009022));
#53231=DIRECTION('center_axis',(0.146507493237112,4.80800404034445E-10,
-0.989209560419519));
#53232=DIRECTION('ref_axis',(0.989087740412835,0.0156933905088255,0.14648945101737));
#53233=DIRECTION('',(-0.146507430631075,-2.24820162482982E-11,0.989209569691823));
#53234=DIRECTION('',(-0.645129946175771,0.,-0.764072871228423));
#53235=DIRECTION('center_axis',(-0.0132941449757976,-0.601098526145228,
0.799064345078291));
#53236=DIRECTION('ref_axis',(-0.998629027060397,-0.0324817210721147,-0.0410488015488608));
#53237=DIRECTION('',(-0.803073192440483,1.02462781930395E-11,0.595880397045793));
#53238=DIRECTION('center_axis',(0.,-1.,1.45983193964168E-32));
#53239=DIRECTION('ref_axis',(1.,0.,0.));
#53240=DIRECTION('center_axis',(0.00988020448522983,0.601098519395469,-0.799113853928153));
#53241=DIRECTION('ref_axis',(-0.998668150326737,-0.0345386218180123,-0.0383276548445816));
#53242=DIRECTION('center_axis',(0.120828713187755,-0.601098531192363,-0.789987960584068));
#53243=DIRECTION('ref_axis',(-0.991445784674722,-0.0335099490343529,-0.126144121410551));
#53244=DIRECTION('center_axis',(-0.124202696628462,0.601098523288246,0.789464537171182));
#53245=DIRECTION('ref_axis',(-0.990897816933698,-0.0335100928779197,-0.130378641162362));
#53246=DIRECTION('',(0.021371341738508,-7.77156117237601E-13,-0.99977160679442));
#53247=DIRECTION('center_axis',(-0.0215713960520066,0.58482795214548,-0.810870483654259));
#53248=DIRECTION('ref_axis',(-0.99854747058022,-0.0526562728540313,-0.0114134099622345));
#53249=DIRECTION('center_axis',(0.0841054675363998,8.95626188632988E-10,
-0.996456858238471));
#53250=DIRECTION('ref_axis',(0.996332897509981,0.0157729998150688,0.084095004704203));
#53251=DIRECTION('',(-0.0841053488765219,-1.77302617009861E-10,0.996456868253894));
#53252=DIRECTION('',(-0.691833462135605,0.,-0.722057103468599));
#53253=DIRECTION('',(-0.764072871250423,6.51326541667476E-11,0.645129946149715));
#53254=DIRECTION('center_axis',(0.,-1.,1.45983193964168E-32));
#53255=DIRECTION('ref_axis',(1.,0.,0.));
#53256=DIRECTION('center_axis',(0.102301128745808,0.601098539514464,-0.792600167077267));
#53257=DIRECTION('ref_axis',(-0.994669915818139,0.0514848666272864,-0.0893368181362392));
#53258=DIRECTION('center_axis',(0.0683376233553293,0.601098536259686,0.796247774841857));
#53259=DIRECTION('ref_axis',(-0.997561422019287,0.0525165008945674,0.0459698426432973));
#53260=DIRECTION('center_axis',(0.0372448546931241,0.584827908068242,-0.810301881241437));
#53261=DIRECTION('ref_axis',(-0.999306149480362,0.021960067725517,-0.0300828029981178));
#53262=DIRECTION('center_axis',(0.0414539038352585,-1.93069262314765E-8,
0.99914041748736));
#53263=DIRECTION('ref_axis',(0.999016656034164,-0.0157391387097842,-0.0414487693302229));
#53264=DIRECTION('',(-0.0414470083237126,-1.60982338570645E-12,-0.999140703555317));
#53265=DIRECTION('center_axis',(0.0724215370721092,0.584827952320769,-0.807917933426663));
#53266=DIRECTION('ref_axis',(-0.997295367386826,0.0322834330562048,-0.0660282525808609));
#53267=DIRECTION('center_axis',(0.0213714252574956,6.25304076798456E-10,
-0.999771605009096));
#53268=DIRECTION('ref_axis',(0.999648347907534,0.0157020800826177,0.021368790485612));
#53269=DIRECTION('',(-0.0213713417391225,-1.60982338570518E-12,0.999771606794407));
#53270=DIRECTION('',(-0.735806627488928,0.,-0.677191706198008));
#53271=DIRECTION('center_axis',(-0.00556959565550501,-0.601098528052763,
0.799155516265161));
#53272=DIRECTION('ref_axis',(-0.9996736242306,0.0232723708321993,0.0105376360491782));
#53273=DIRECTION('',(-0.722057103468721,0.,0.691833462135478));
#53274=DIRECTION('center_axis',(0.,-1.,1.45983193964168E-32));
#53275=DIRECTION('ref_axis',(1.,0.,0.));
#53276=DIRECTION('center_axis',(0.00215530436841184,0.601098532989542,-0.799172014212772));
#53277=DIRECTION('ref_axis',(-0.999686894498085,0.0212180041744757,0.0132630791156127));
#53278=DIRECTION('center_axis',(-0.0717388699212962,-0.601098525174619,
-0.79594855209072));
#53279=DIRECTION('ref_axis',(-0.997078901768021,0.0222452838102306,0.0730671677108043));
#53280=DIRECTION('center_axis',(0.0683376830885089,0.601098530194654,0.796247774293857));
#53281=DIRECTION('ref_axis',(-0.997381963140672,0.0222451515272063,0.0688067789915375));
#53282=DIRECTION('center_axis',(-0.0646084828443836,0.584827953016101,-0.808580242966364));
#53283=DIRECTION('ref_axis',(-0.997226863463135,-0.0078464556861505,0.0740068640103327));
#53284=DIRECTION('center_axis',(0.104102207062556,-1.53723582553726E-9,
0.994566604348198));
#53285=DIRECTION('ref_axis',(0.994444367120634,-0.0156778483100078,-0.104089412403035));
#53286=DIRECTION('',(-0.104101785979623,0.,-0.994566648423248));
#53287=DIRECTION('center_axis',(-0.0294084948096632,0.584827952254358,-0.810624084699563));
#53288=DIRECTION('ref_axis',(-0.999273620325167,0.00246180456904867,0.038028558222716));
#53289=DIRECTION('center_axis',(-0.0414469199711997,6.73631675134276E-10,
-0.99914070722041));
#53290=DIRECTION('ref_axis',(0.999018019141589,0.0156707406190299,-0.0414418305443513));
#53291=DIRECTION('',(0.0414470083242613,-6.4614980030209E-11,0.999140703555294));
#53292=DIRECTION('',(-0.776875900241837,1.64268989064397E-13,-0.629653742642284));
#53293=DIRECTION('center_axis',(0.0946350652757326,-0.601098528055325,0.79355199198917));
#53294=DIRECTION('ref_axis',(-0.993543155106225,-0.00691952328441555,0.113243627366327));
#53295=DIRECTION('',(-0.677191706207015,2.34699318130683E-11,0.735806627480639));
#53296=DIRECTION('center_axis',(0.,-1.,1.45983193964168E-32));
#53297=DIRECTION('ref_axis',(1.,0.,0.));
#53298=DIRECTION('center_axis',(-0.09802452438425,0.601098525946293,-0.793140438210305));
#53299=DIRECTION('ref_axis',(-0.993214294979514,-0.00897214607806965,0.115951993700411));
#53300=DIRECTION('center_axis',(-0.0717388784411376,-0.601098528963249,
-0.795948548461662));
#53301=DIRECTION('ref_axis',(-0.995377169084396,-0.00794566452399397,0.0957139367114593));
#53302=DIRECTION('center_axis',(0.0683376456977897,0.601098526979802,0.796247779929838));
#53303=DIRECTION('ref_axis',(-0.995776996739739,-0.00794582476184027,0.0914605741991623));
#53304=DIRECTION('center_axis',(-0.165441105016554,0.58482795223037,-0.794106735307625));
#53305=DIRECTION('ref_axis',(-0.981404269601245,-0.0181546317005234,0.191091781498484));
#53306=DIRECTION('center_axis',(0.166345793588914,-5.72962025682916E-10,
0.986067480933873));
#53307=DIRECTION('ref_axis',(0.985946262651246,-0.0156795066181454,-0.166325344539709));
#53308=DIRECTION('',(-0.166345718259955,2.06171882231989E-7,-0.986067493641555));
#53309=DIRECTION('center_axis',(-0.130780879077022,0.584827782536271,-0.800545330660013));
#53310=DIRECTION('ref_axis',(-0.989535715164436,-0.0273551074289179,0.14167133270906));
#53311=DIRECTION('center_axis',(-0.104101642227122,1.01911928448842E-9,
-0.994566663469883));
#53312=DIRECTION('ref_axis',(0.99444404419175,0.0157023279255542,-0.104088807608093));
#53313=DIRECTION('',(-0.104101785049298,-1.29267396645623E-5,-0.994566648436619));
#53314=DIRECTION('',(-0.814879221760667,-7.6262887221002E-8,-0.579630791058173));
#53315=DIRECTION('center_axis',(0.166345721445505,1.76912654930784E-13,
0.986067493104186));
#53316=DIRECTION('ref_axis',(0.761122075630443,-0.635772805085226,-0.128398311134019));
#53317=DIRECTION('',(0.6296537426427,0.,-0.7768759002415));
#53318=DIRECTION('center_axis',(-0.206207729994026,0.398564391559433,-0.893658098979453));
#53319=DIRECTION('ref_axis',(1.81224450895921E-16,0.913286229134016,0.407318381213235));
#53320=DIRECTION('center_axis',(0.234739006587026,5.74456419399389E-5,0.972058432135916));
#53321=DIRECTION('ref_axis',(0.972058374626882,-0.000362894799268911,-0.234738971253411));
#53322=DIRECTION('',(-0.227932275687093,5.94973683762914E-5,-0.973676986561851));
#53323=DIRECTION('center_axis',(-0.1196446603478,0.590180063809313,-0.798356215941414));
#53324=DIRECTION('ref_axis',(0.252206560643778,0.795821124358454,0.550509390286017));
#53325=DIRECTION('center_axis',(-0.817786253526483,0.550037558034545,-0.169364483568763));
#53326=DIRECTION('ref_axis',(-0.558100160398776,-0.829773590181599,6.40047726430736E-17));
#53327=DIRECTION('center_axis',(0.463417276847617,-0.477126089246125,-0.746722922160447));
#53328=DIRECTION('ref_axis',(0.816468152271752,-0.0976221507206682,0.569077913834848));
#53329=DIRECTION('center_axis',(0.340054078907099,0.584827951390133,-0.736437024253577));
#53330=DIRECTION('ref_axis',(-0.915422295877618,0.026548968994854,-0.401618192386079));
#53331=DIRECTION('center_axis',(-0.329271771466537,-4.74095418533005E-11,
0.944235193431853));
#53332=DIRECTION('ref_axis',(0.944118104706356,-0.0157477670569709,0.329230940524122));
#53333=DIRECTION('center_axis',(0.379507057814437,-0.000115441161244248,
-0.925188834639917));
#53334=DIRECTION('ref_axis',(0.0230516160204343,0.99969073081804,0.00933090110008984));
#53335=DIRECTION('',(-0.387911046549999,-6.0690341614628E-10,0.921696815641936));
#53336=DIRECTION('center_axis',(-0.306515843341055,-0.601098527987144,0.738057313108278));
#53337=DIRECTION('ref_axis',(-0.931015194377809,0.0279220141825818,-0.36391079808332));
#53338=DIRECTION('',(-0.926032600098767,2.24062901110949E-10,0.377443536908922));
#53339=DIRECTION('center_axis',(0.,-1.,1.45983193964168E-32));
#53340=DIRECTION('ref_axis',(1.,0.,0.));
#53341=DIRECTION('center_axis',(0.30335983449366,0.601098533973444,-0.739360103921598));
#53342=DIRECTION('ref_axis',(-0.932054746514114,0.0258667184698823,-0.361392947324807));
#53343=DIRECTION('center_axis',(0.218887642670481,-0.601098523971291,-0.768614834859239));
#53344=DIRECTION('ref_axis',(-0.95567522663093,0.0268944650784618,-0.293192000150183));
#53345=DIRECTION('center_axis',(-0.222169422774876,0.601098530737144,0.767672654149883));
#53346=DIRECTION('ref_axis',(-0.954413927449797,0.0268943169511852,-0.297272183033635));
#53347=DIRECTION('center_axis',(0.245072600276168,0.58482795222252,-0.773250080435231));
#53348=DIRECTION('ref_axis',(-0.952549404908864,-0.00326197145103078,-0.304366540128876));
#53349=DIRECTION('center_axis',(-0.269332908043605,-8.28266897459133E-10,
0.963047135214458));
#53350=DIRECTION('ref_axis',(0.962928690770987,-0.0156832196310515,0.269299782978149));
#53351=DIRECTION('',(0.269333011080688,8.3214818921303E-8,-0.963047106398334));
#53352=DIRECTION('center_axis',(0.278442400844468,0.584827969932124,-0.761870116881506));
#53353=DIRECTION('ref_axis',(-0.940946460207726,0.00704480132855519,-0.338482096715308));
#53354=DIRECTION('center_axis',(0.329271851494279,6.43150047631334E-10,
-0.944235165524738));
#53355=DIRECTION('ref_axis',(0.944119207837706,0.0156715280545467,0.329231414965733));
#53356=DIRECTION('',(-0.329271770815784,-1.48214773786022E-11,0.944235193658782));
#53357=DIRECTION('',(-0.490529956132129,-3.07809289802454E-8,-0.871424329553066));
#53358=DIRECTION('center_axis',(-0.588982927039396,0.793626260385285,-0.152500722893282));
#53359=DIRECTION('ref_axis',(-0.803018883943793,-0.595953582109937,3.751356198321E-17));
#53360=DIRECTION('center_axis',(0.753853492055292,0.47154667454953,-0.457546332339493));
#53361=DIRECTION('ref_axis',(0.644196855355331,-0.393421735031793,0.655919011734586));
#53362=DIRECTION('center_axis',(-0.211595771064685,-0.601098528069342,0.770654130735969));
#53363=DIRECTION('ref_axis',(-0.96385509500095,-0.0022757160895087,-0.266417298531812));
#53364=DIRECTION('',(-0.900505410469423,5.19500677922231E-12,0.43484480647157));
#53365=DIRECTION('center_axis',(0.,-1.,1.45983193964168E-32));
#53366=DIRECTION('ref_axis',(1.,0.,0.));
#53367=DIRECTION('center_axis',(0.208301378683891,0.601098527259043,-0.771551097572546));
#53368=DIRECTION('ref_axis',(-0.964571908712687,-0.00432810514597244,-0.26378457200566));
#53369=DIRECTION('center_axis',(0.21888768672917,-0.601098528263956,-0.76861481895502));
#53370=DIRECTION('ref_axis',(-0.962432414917285,-0.00330178468193749,-0.271501279802502));
#53371=DIRECTION('center_axis',(-0.222169419447295,0.601098527734523,0.767672657464001));
#53372=DIRECTION('ref_axis',(-0.961263728712235,-0.00330190212277808,-0.275610488379203));
#53373=DIRECTION('center_axis',(0.146235178796552,0.584828255987166,-0.797866645174086));
#53374=DIRECTION('ref_axis',(-0.978497161184359,-0.0330815410904191,-0.203590071450535));
#53375=DIRECTION('center_axis',(-0.208297965837032,-1.08390100212757E-7,
0.97806541572031));
#53376=DIRECTION('ref_axis',(0.977945248097851,-0.0156751635316394,0.208272372078222));
#53377=DIRECTION('',(0.208331314487311,3.88578058618561E-13,-0.978058312885274));
#53378=DIRECTION('center_axis',(0.180761599638725,0.584827952226355,-0.790760083964016));
#53379=DIRECTION('ref_axis',(-0.970813382163765,-0.0227607295866176,-0.23875369358491));
#53380=DIRECTION('center_axis',(0.269333103715099,7.48422893903147E-10,
-0.963047080491495));
#53381=DIRECTION('ref_axis',(0.9629284823617,0.0156933905083944,0.269299935668288));
#53382=DIRECTION('',(-0.269333009823168,-2.20934381896949E-11,0.963047106750025));
#53383=DIRECTION('',(-0.544279180229307,0.,-0.838904150644705));
#53384=DIRECTION('center_axis',(-0.113338678411945,-0.601098527569091,0.791097278550561));
#53385=DIRECTION('ref_axis',(-0.98560975486667,-0.0324816945160823,-0.165886559530982));
#53386=DIRECTION('',(-0.871424337430412,8.00811321699429E-12,0.490529942138059));
#53387=DIRECTION('center_axis',(0.,-1.,1.45983193964168E-32));
#53388=DIRECTION('ref_axis',(1.,0.,0.));
#53389=DIRECTION('center_axis',(0.10995783127813,0.601098519808573,-0.791574282568953));
#53390=DIRECTION('ref_axis',(-0.985989623433843,-0.0345386145953561,-0.163191747899895));
#53391=DIRECTION('center_axis',(0.218887680548057,-0.601098531456249,-0.768614818218744));
#53392=DIRECTION('ref_axis',(-0.967817889648016,-0.0335099442410043,-0.249410537295892));
#53393=DIRECTION('center_axis',(-0.222169453489029,0.601098523668802,0.767672650795619));
#53394=DIRECTION('ref_axis',(-0.966743517525389,-0.0335100860343741,-0.253542985421816));
#53395=DIRECTION('',(0.146507430630888,0.,-0.98920956969185));
#53396=DIRECTION('center_axis',(0.080227720602025,0.58482795214713,-0.807180140510406));
#53397=DIRECTION('ref_axis',(-0.989243145943592,-0.0526562728337357,-0.136474595199564));
#53398=DIRECTION('center_axis',(0.208331373152654,4.29367531478973E-10,
-0.978058300389261));
#53399=DIRECTION('ref_axis',(0.977936628468742,0.0157729998144705,0.208305456424077));
#53400=DIRECTION('',(-0.208331314485257,-1.76081371683112E-10,0.978058312885712));
#53401=DIRECTION('',(-0.595880397050137,0.,-0.803073192437259));
#53402=DIRECTION('',(-0.83890415066404,6.73708191429374E-11,0.544279180199506));
#53403=DIRECTION('center_axis',(0.,-1.,1.45983193964168E-32));
#53404=DIRECTION('ref_axis',(1.,0.,0.));
#53405=DIRECTION('center_axis',(0.200833593520141,0.601098539633411,-0.773528547220054));
#53406=DIRECTION('ref_axis',(-0.97562977458375,0.051484865311369,-0.21329756583124));
#53407=DIRECTION('center_axis',(-0.0319975640352948,0.601098537119618,0.798534097311106));
#53408=DIRECTION('ref_axis',(-0.995456900744133,0.0525164909496035,-0.0794202552200983));
#53409=DIRECTION('center_axis',(0.138507934572584,0.584827930050219,-0.799244545989282));
#53410=DIRECTION('ref_axis',(-0.987656085635407,0.0219594825865639,-0.155091062385544));
#53411=DIRECTION('center_axis',(-0.0841018096930555,-1.0371211046821E-8,
0.996457166970238));
#53412=DIRECTION('ref_axis',(0.996333737901996,-0.0157391393485509,0.0840913920137152));
#53413=DIRECTION('',(0.08410534887882,-3.88578058619033E-13,-0.9964568682537));
#53414=DIRECTION('center_axis',(0.173109438633622,0.584827952322477,-0.792470433794379));
#53415=DIRECTION('ref_axis',(-0.981155861141504,0.0322834330334646,-0.190501853269852));
#53416=DIRECTION('center_axis',(0.146507522183494,6.95832293934272E-10,
-0.989209556132397));
#53417=DIRECTION('ref_axis',(0.989087601174383,0.0157020800821761,0.146489459976472));
#53418=DIRECTION('',(-0.146507430631413,-1.16573417585542E-12,0.989209569691773));
#53419=DIRECTION('',(-0.645129946175793,-1.64268989064484E-13,-0.764072871228405));
#53420=DIRECTION('center_axis',(-0.105686420127036,-0.601098528110706,0.792155881189981));
#53421=DIRECTION('ref_axis',(-0.993111615389959,0.0232723692717861,-0.114837782136476));
#53422=DIRECTION('',(-0.803073192437354,1.43735365432664E-13,0.595880397050009));
#53423=DIRECTION('center_axis',(0.,-1.,1.45983193964168E-32));
#53424=DIRECTION('ref_axis',(1.,0.,0.));
#53425=DIRECTION('center_axis',(0.102301118167672,0.601098533074067,-0.792600173326911));
#53426=DIRECTION('ref_axis',(-0.993466369715916,0.0212180019323403,-0.112135492318351));
#53427=DIRECTION('center_axis',(0.0285856187492689,-0.601098525185125,-0.798663524533949));
#53428=DIRECTION('ref_axis',(-0.998374381198037,0.0222452835218335,-0.052476111979347));
#53429=DIRECTION('center_axis',(-0.0319974908985116,0.601098530253856,0.79853410540994));
#53430=DIRECTION('ref_axis',(-0.998141084474372,0.0222451499143489,-0.0567408916885656));
#53431=DIRECTION('center_axis',(0.0372429508152893,0.584827953016182,-0.810301936308604));
#53432=DIRECTION('ref_axis',(-0.998638951358832,-0.00784645567012263,-0.0515623696347268));
#53433=DIRECTION('center_axis',(-0.0213710049213545,-8.58526880578322E-10,
0.999771613994242));
#53434=DIRECTION('ref_axis',(0.999648737047707,-0.0156778483081366,0.0213683783041829));
#53435=DIRECTION('',(0.0213713417385381,-3.88578058618843E-13,-0.999771606794419));
#53436=DIRECTION('center_axis',(0.0724215377014447,0.584827952254335,-0.807917933418339));
#53437=DIRECTION('ref_axis',(-0.996160291529796,0.00246180457187916,-0.087513502372616));
#53438=DIRECTION('center_axis',(0.0841054050042859,4.22320839248603E-10,
-0.996456863516462));
#53439=DIRECTION('ref_axis',(0.99633450499547,0.0156707406185972,0.0840950774058495));
#53440=DIRECTION('',(-0.0841053488781393,-6.50035580887595E-11,0.996456868253758));
#53441=DIRECTION('',(-0.691833462135694,1.64268989064481E-13,-0.722057103468513));
#53442=DIRECTION('center_axis',(-0.00556958958256345,-0.601098527996718,
0.799155516349641));
#53443=DIRECTION('ref_axis',(-0.999901960614497,-0.00691952812673157,-0.012173302337035));
#53444=DIRECTION('',(-0.764072871236518,2.36136671785041E-11,0.645129946166184));
#53445=DIRECTION('center_axis',(0.,-1.,1.45983193964168E-32));
#53446=DIRECTION('ref_axis',(1.,0.,0.));
#53447=DIRECTION('center_axis',(0.00215529775560142,0.601098526063912,-0.79917201943973));
#53448=DIRECTION('ref_axis',(-0.999915141883942,-0.00897213785214235,-0.00944509256586728));
#53449=DIRECTION('center_axis',(0.028585614071655,-0.601098528930697,-0.798663521882337));
#53450=DIRECTION('ref_axis',(-0.999524459852295,-0.0079456673545495,-0.029794639237111));
#53451=DIRECTION('center_axis',(-0.0319975271426687,0.601098526968027,0.798534106431042));
#53452=DIRECTION('ref_axis',(-0.999388047168573,-0.00794582543224992,-0.0340645715485336));
#53453=DIRECTION('center_axis',(-0.0646085875882672,0.584827952229195,-0.808580235166094));
#53454=DIRECTION('ref_axis',(-0.997615754686242,-0.0181546317615242,0.066582395176232));
#53455=DIRECTION('center_axis',(0.0414484569980076,-4.97663449248963E-9,
0.99914064345941));
#53456=DIRECTION('ref_axis',(0.999017818082041,-0.0156795063500311,-0.0414433617750534));
#53457=DIRECTION('',(-0.0414470050956686,2.06171493653918E-7,-0.999140703689204));
#53458=DIRECTION('center_axis',(-0.0294146978379073,0.584827782536786,-0.810623982080601));
#53459=DIRECTION('ref_axis',(-0.999489056723302,-0.0273551074064042,0.0165325009949378));
#53460=DIRECTION('center_axis',(0.0213714460906926,7.0386369386079E-10,
-0.999771604563759));
#53461=DIRECTION('ref_axis',(0.999648343570961,0.0157023279251134,0.021368811234293));
#53462=DIRECTION('',(0.0213713426633156,-1.29267396290012E-5,-0.999771606691082));
#53463=DIRECTION('',(-0.735806654387649,-7.62629077546487E-8,-0.677191676971039));
#53464=DIRECTION('center_axis',(0.041447206939856,-1.61525101140892E-7,
0.99914069531616));
#53465=DIRECTION('ref_axis',(0.771212966511889,-0.635772804014362,-0.0319922171730482));
#53466=DIRECTION('',(0.722057103468862,0.,-0.69183346213533));
#53467=DIRECTION('center_axis',(-0.0925766612059187,0.398564391554733,-0.912456019534405));
#53468=DIRECTION('ref_axis',(-6.9062910639093E-17,0.916391407641987,0.400283384616372));
#53469=DIRECTION('center_axis',(0.111056792872745,5.7445687582888E-5,0.99381405980033));
#53470=DIRECTION('ref_axis',(0.993813998268466,-0.000363029792981438,-0.111056765012375));
#53471=DIRECTION('',(-0.10410087644023,5.9497368305179E-5,-0.994566741845131));
#53472=DIRECTION('center_axis',(-0.0186406604881565,0.590180063812162,-0.807056390876894));
#53473=DIRECTION('ref_axis',(0.181223283205387,0.795820770431835,0.577778004923639));
#53474=DIRECTION('center_axis',(-0.790110766279426,0.550037558035771,-0.270524789546882));
#53475=DIRECTION('ref_axis',(-0.571341150200151,-0.820712672064936,-1.98680099173155E-16));
#53476=DIRECTION('center_axis',(0.553352291168644,-0.477126090543816,-0.682753202541582));
#53477=DIRECTION('ref_axis',(0.738701542742593,-0.0976315438263697,0.666924367825762));
#53478=DIRECTION('center_axis',(0.429672684498432,0.584827951389853,-0.688009921054238));
#53479=DIRECTION('ref_axis',(-0.857867810937999,0.0265489689994253,-0.513184149405954));
#53480=DIRECTION('center_axis',(-0.44501941753188,-2.58199235088207E-13,
0.895520919922916));
#53481=DIRECTION('ref_axis',(0.895409871950847,-0.0157477670569058,0.444964233445442));
#53482=DIRECTION('center_axis',(0.492471434687182,-0.000115441210406181,
-0.870328600409337));
#53483=DIRECTION('ref_axis',(0.0217249806890136,0.999690027137922,0.0121603805467594));
#53484=DIRECTION('',(-0.50037149435502,-6.06903416145897E-10,0.86581081515359));
#53485=DIRECTION('center_axis',(-0.396601982854688,-0.601098528025573,0.693820889568208));
#53486=DIRECTION('ref_axis',(-0.878063744941495,0.0279220134200669,-0.477728396671044));
#53487=DIRECTION('',(-0.966036775423284,2.24206636476442E-10,0.258404621726826));
#53488=DIRECTION('center_axis',(0.,-1.,1.45983193964168E-32));
#53489=DIRECTION('ref_axis',(1.,0.,0.));
#53490=DIRECTION('center_axis',(0.393634151697023,0.60109853374655,-0.695508955618483));
#53491=DIRECTION('ref_axis',(-0.879410666406445,0.0258667235993845,-0.475360697177213));
#53492=DIRECTION('center_axis',(0.313494643752222,-0.601098524363107,-0.735120175445595));
#53493=DIRECTION('ref_axis',(-0.911392736151507,0.0268944565563492,-0.410657970453282));
#53494=DIRECTION('center_axis',(-0.316632441871935,0.601098530599997,0.733774115968082));
#53495=DIRECTION('ref_axis',(-0.909630006253576,0.0268943200603761,-0.41454788296602));
#53496=DIRECTION('center_axis',(0.340054062537767,0.584827952222704,-0.736437031151041));
#53497=DIRECTION('ref_axis',(-0.906891025682966,-0.00326197146399792,-0.421352616080481));
#53498=DIRECTION('center_axis',(-0.387910988888561,-4.91125118611069E-10,
0.921696839909685));
#53499=DIRECTION('ref_axis',(0.921583481107603,-0.015683219630754,0.387863279999029));
#53500=DIRECTION('',(0.387911047762143,8.3213597675953E-8,-0.921696815131782));
#53501=DIRECTION('center_axis',(0.371734444692853,0.584827969931374,-0.720964456970553));
#53502=DIRECTION('ref_axis',(-0.891103760619904,0.0070448013553493,-0.453744926784783));
#53503=DIRECTION('center_axis',(0.445019483355182,5.75499300180527E-10,
-0.895520887212737));
#53504=DIRECTION('ref_axis',(0.89541091192758,0.0156715280541854,0.444964832328877));
#53505=DIRECTION('',(-0.445019414620638,-1.44328993199847E-11,0.895520921369626));
#53506=DIRECTION('',(-0.377443551884409,-3.07809289802548E-8,-0.926032593994877));
#53507=DIRECTION('center_axis',(-0.565225212017908,0.793626260385261,-0.225117343903613));
#53508=DIRECTION('ref_axis',(-0.814533996880245,-0.58011582285462,-1.01709000961919E-17));
#53509=DIRECTION('center_axis',(0.805254893431975,0.471546674524301,-0.359455547111087));
#53510=DIRECTION('ref_axis',(0.556909986835466,-0.39342664753178,0.731482562727797));
#53511=DIRECTION('center_axis',(-0.306515839351534,-0.601098528038064,0.738057314723659));
#53512=DIRECTION('ref_axis',(-0.922863871513281,-0.00227572262241581,-0.385119586287253));
#53513=DIRECTION('',(-0.947905162033643,5.19500677922257E-12,0.318552670354485));
#53514=DIRECTION('center_axis',(0.,-1.,1.45983193964168E-32));
#53515=DIRECTION('ref_axis',(1.,0.,0.));
#53516=DIRECTION('center_axis',(0.303359854367542,0.601098527259698,-0.739360101225597));
#53517=DIRECTION('ref_axis',(-0.923904997618405,-0.00432810492030727,-0.382597468475071));
#53518=DIRECTION('center_axis',(0.313494662811144,-0.601098528298344,-0.735120164100055));
#53519=DIRECTION('ref_axis',(-0.920815217868027,-0.0033017783155422,-0.389985169977799));
#53520=DIRECTION('center_axis',(-0.316632443585747,0.601098527734296,0.733774117576097));
#53521=DIRECTION('ref_axis',(-0.919140723420251,-0.00330190204970445,-0.393915508698696));
#53522=DIRECTION('center_axis',(0.24507260052094,0.584827952239687,-0.77325008034467));
#53523=DIRECTION('ref_axis',(-0.945267066533668,-0.0330869090465625,-0.324615818124407));
#53524=DIRECTION('center_axis',(-0.329271704502654,-5.5048012952267E-10,
0.944235216783359));
#53525=DIRECTION('ref_axis',(0.944119205188345,-0.0156751701945281,0.329231249175864));
#53526=DIRECTION('',(0.329271770815259,3.88578058618359E-13,-0.944235193658965));
#53527=DIRECTION('center_axis',(0.278444758722175,0.584827952226138,-0.761869268729965));
#53528=DIRECTION('ref_axis',(-0.933234456237909,-0.0227607295922861,-0.358546229765089));
#53529=DIRECTION('center_axis',(0.387911135664321,7.42148139023014E-10,
-0.921696778136724));
#53530=DIRECTION('ref_axis',(0.921583272247153,0.0156933905090626,0.387863364870362));
#53531=DIRECTION('',(-0.387911046558538,-2.20379270384585E-11,0.921696815638342));
#53532=DIRECTION('',(-0.434844806474186,0.,-0.900505410468159));
#53533=DIRECTION('center_axis',(-0.211595749425156,-0.601098527583133,0.770654137056693));
#53534=DIRECTION('ref_axis',(-0.957046828571228,-0.0324816942905735,-0.28810815236256));
#53535=DIRECTION('',(-0.926032600056252,8.17238220606226E-12,0.37744353701323));
#53536=DIRECTION('center_axis',(0.,-1.,1.45983193964168E-32));
#53537=DIRECTION('ref_axis',(1.,0.,0.));
#53538=DIRECTION('center_axis',(0.208301341754461,0.601098519678007,-0.771551113448876));
#53539=DIRECTION('ref_axis',(-0.957761452083959,-0.0345386168713349,-0.285482197074776));
#53540=DIRECTION('center_axis',(0.313494679133752,-0.601098531002521,-0.735120154928048));
#53541=DIRECTION('ref_axis',(-0.928926923074171,-0.0335099525260047,-0.368743616445977));
#53542=DIRECTION('center_axis',(-0.31663247868647,0.601098523595813,0.733774105819901));
#53543=DIRECTION('ref_axis',(-0.927343093225053,-0.0335100873639033,-0.372708815957785));
#53544=DIRECTION('',(0.269333009822791,8.32667268467739E-13,-0.96304710675013));
#53545=DIRECTION('center_axis',(0.180761598115075,0.584827952145732,-0.790760084371937));
#53546=DIRECTION('ref_axis',(-0.96433786595444,-0.0526562728494128,-0.259383494494242));
#53547=DIRECTION('center_axis',(0.329271876752694,8.41810918162305E-10,
-0.944235156716672));
#53548=DIRECTION('ref_axis',(0.944117692442974,0.0157729998149326,0.329230914850038));
#53549=DIRECTION('',(-0.329271770813475,-1.76136882834204E-10,0.944235193659588));
#53550=DIRECTION('',(-0.490529942141654,0.,-0.871424337428388));
#53551=DIRECTION('',(-0.900505410483609,6.73708191429276E-11,0.434844806442192));
#53552=DIRECTION('center_axis',(0.,-1.,1.45983193964168E-32));
#53553=DIRECTION('ref_axis',(1.,0.,0.));
#53554=DIRECTION('center_axis',(0.296198809704822,0.601098538800504,-0.742257914596635));
#53555=DIRECTION('ref_axis',(-0.941203364053214,0.0514848748675469,-0.333894497041784));
#53556=DIRECTION('center_axis',(-0.131828106546344,0.601098536710114,0.788227060871019));
#53557=DIRECTION('ref_axis',(-0.977653429390555,0.0525164956588446,-0.203557828846257));
#53558=DIRECTION('center_axis',(0.237588622522883,0.584827908067953,-0.775582338886427));
#53559=DIRECTION('ref_axis',(-0.960429820312543,0.0219600677334787,-0.277655029991458));
#53560=DIRECTION('center_axis',(-0.208324618392494,-1.88734789164305E-8,
0.978059739163013));
#53561=DIRECTION('ref_axis',(0.977938589004,-0.0157391387081356,0.20829881336578));
#53562=DIRECTION('',(0.20833131448726,8.32667268468638E-13,-0.978058312885285));
#53563=DIRECTION('center_axis',(0.271067301054217,0.584827952319284,-0.764525201994817));
#53564=DIRECTION('ref_axis',(-0.949542940826784,0.032283433081186,-0.311971126026936));
#53565=DIRECTION('center_axis',(0.269333078423088,5.28470611559298E-10,
-0.963047087564852));
#53566=DIRECTION('ref_axis',(0.962928358052914,0.0157020800824718,0.269299873632726));
#53567=DIRECTION('',(-0.26933300982351,0.,0.963047106749929));
#53568=DIRECTION('',(-0.544279180229341,0.,-0.838904150644683));
#53569=DIRECTION('center_axis',(-0.204136505045659,-0.601098528206328,0.772663475709788));
#53570=DIRECTION('ref_axis',(-0.970887643980288,0.0232723666889749,-0.238402138654625));
#53571=DIRECTION('',(-0.871424337428441,0.,0.49052994214156));
#53572=DIRECTION('center_axis',(0.,-1.,1.45983193964168E-32));
#53573=DIRECTION('ref_axis',(1.,0.,0.));
#53574=DIRECTION('center_axis',(0.200833592354618,0.601098532928243,-0.773528552733158));
#53575=DIRECTION('ref_axis',(-0.971578285480988,0.0212180058948169,-0.235765628130294));
#53576=DIRECTION('center_axis',(0.128459301139359,-0.601098525336866,-0.78878309489278));
#53577=DIRECTION('ref_axis',(-0.983924899358624,0.0222452795628364,-0.177191816851943));
#53578=DIRECTION('center_axis',(-0.131828036158469,0.601098530106885,0.788227077678726));
#53579=DIRECTION('ref_axis',(-0.983158925334848,0.0222451538963128,-0.181393717263182));
#53580=DIRECTION('center_axis',(0.138507040834489,0.58482795301623,-0.799244684067476));
#53581=DIRECTION('ref_axis',(-0.984301906436154,-0.00784645568808815,-0.17631843386126));
#53582=DIRECTION('center_axis',(-0.146507111242795,-7.49259406551241E-10,
0.989209616994948));
#53583=DIRECTION('ref_axis',(0.989088038172257,-0.0156778483085329,0.146489104772234));
#53584=DIRECTION('',(0.146507430631052,-4.44089209850505E-13,-0.989209569691826));
#53585=DIRECTION('center_axis',(0.173109439256193,0.584827952254779,-0.792470433708342));
#53586=DIRECTION('ref_axis',(-0.977336919866491,0.0024618045487747,-0.211675422721308));
#53587=DIRECTION('center_axis',(0.208331416101965,7.95303813231119E-10,
-0.978058291240839));
#53588=DIRECTION('ref_axis',(0.977938191944633,0.0156707406189369,0.208305834350639));
#53589=DIRECTION('',(-0.208331314486965,-6.3837823912962E-11,0.978058312885348));
#53590=DIRECTION('',(-0.595880397050185,1.64268989064468E-13,-0.803073192437223));
#53591=DIRECTION('center_axis',(-0.105686432079547,-0.60109852811121,0.792155879594939));
#53592=DIRECTION('ref_axis',(-0.990491714011746,-0.00691951878544824,-0.137398270490755));
#53593=DIRECTION('',(-0.838904150651509,2.34493981894382E-11,0.54427918021882));
#53594=DIRECTION('center_axis',(0.,-1.,1.45983193964168E-32));
#53595=DIRECTION('ref_axis',(1.,0.,0.));
#53596=DIRECTION('center_axis',(0.102301118391204,0.601098526083832,-0.79260017859937));
#53597=DIRECTION('ref_axis',(-0.990846728085701,-0.00897213638327582,-0.134693215161644));
#53598=DIRECTION('center_axis',(0.128459309556313,-0.601098528782676,-0.788783090896108));
#53599=DIRECTION('ref_axis',(-0.987908649882266,-0.00794567944767794,-0.154833348042058));
#53600=DIRECTION('center_axis',(-0.131828062205383,0.601098527104583,0.788227075612019));
#53601=DIRECTION('ref_axis',(-0.987238153221425,-0.00794581535552585,-0.159052484552382));
#53602=DIRECTION('center_axis',(0.037242845866466,0.584827952228643,-0.810301941700634));
#53603=DIRECTION('ref_axis',(-0.998094243374912,-0.0181546317616234,-0.0589770352549358));
#53604=DIRECTION('center_axis',(-0.084103933977164,-4.74152240553405E-9,
0.996456987676621));
#53605=DIRECTION('ref_axis',(0.996334492213274,-0.0156795063497496,0.0840935949210542));
#53606=DIRECTION('',(0.0841053520983884,2.06170327919954E-7,-0.996456867981933));
#53607=DIRECTION('center_axis',(0.0724153707322235,0.584827782537017,-0.807918609053257));
#53608=DIRECTION('ref_axis',(-0.993679858785782,-0.0273551073987626,-0.108867058115254));
#53609=DIRECTION('center_axis',(0.146507538530465,7.41923804238371E-10,
-0.989209553711318));
#53610=DIRECTION('ref_axis',(0.989087594903337,0.0157023279249282,0.146489475751914));
#53611=DIRECTION('',(0.146507431535495,-1.29267395934322E-5,-0.989209569473411));
#53612=DIRECTION('',(-0.645129976525437,-7.62630514900407E-8,-0.764072845603273));
#53613=DIRECTION('center_axis',(-0.0841051507916142,-1.61528648367539E-7,
0.9964568849731));
#53614=DIRECTION('ref_axis',(0.769141409948316,-0.635772804014554,0.0649186658688223));
#53615=DIRECTION('',(0.803073192437323,0.,-0.59588039705005));
#53616=DIRECTION('center_axis',(0.0225143968323005,0.398564391561196,-0.916863963581693));
#53617=DIRECTION('ref_axis',(3.39181432986796E-17,0.917096430247481,0.39866544574032));
#53618=DIRECTION('center_axis',(-0.0143768528108244,5.7445659478889E-5,
0.999896646060608));
#53619=DIRECTION('ref_axis',(0.999896581537589,-0.000362987245248623,0.0143768727372876));
#53620=DIRECTION('',(0.0213722558148867,5.94973683407431E-5,-0.999771585484128));
#53621=DIRECTION('center_axis',(0.0826573141490685,0.590180063802952,-0.803028804406919));
#53622=DIRECTION('ref_axis',(0.107376602486449,0.795821166339074,0.595935345859921));
#53623=DIRECTION('center_axis',(-0.749974760259059,0.550037558037291,-0.367418757989764));
#53624=DIRECTION('ref_axis',(-0.591402864747467,-0.806376246902455,1.34536393528168E-16));
#53625=DIRECTION('center_axis',(0.634560609589244,-0.477126090761952,-0.608016057577384));
#53626=DIRECTION('ref_axis',(0.64929247946224,-0.0976240300752894,0.754247190823828));
#53627=DIRECTION('center_axis',(0.512515095169429,0.584827951389991,-0.628732490409441));
#53628=DIRECTION('ref_axis',(-0.786784238160081,0.0265489689956428,-0.616656885819115));
#53629=DIRECTION('center_axis',(-0.553748840165996,1.08058537688362E-11,
0.832683746697877));
#53630=DIRECTION('ref_axis',(0.832580490772235,-0.0157477670557757,0.553680173221167));
#53631=DIRECTION('center_axis',(0.597669253808723,-0.000115441150256891,
-0.801742757825143));
#53632=DIRECTION('ref_axis',(0.0190168739071945,0.999720685825276,0.0140324210255403));
#53633=DIRECTION('',(-0.604940784786227,-6.06181771179997E-10,0.796270460900204));
#53634=DIRECTION('center_axis',(-0.480433469444791,-0.601098528159146,0.638642498493601));
#53635=DIRECTION('ref_axis',(-0.811264707648814,0.0279220105145261,-0.584011930916065));
#53636=DIRECTION('',(-0.990805973716841,2.24350371841859E-10,0.135290511297072));
#53637=DIRECTION('center_axis',(0.,-1.,1.45983193964168E-32));
#53638=DIRECTION('ref_axis',(1.,0.,0.));
#53639=DIRECTION('center_axis',(0.477700620491674,0.601098533573279,-0.640689214922433));
#53640=DIRECTION('ref_axis',(-0.812897754247503,0.0258667274892258,-0.581831722707145));
#53641=DIRECTION('center_axis',(0.403157636441818,-0.601098524456693,-0.690032234083766));
#53642=DIRECTION('ref_axis',(-0.852737039489665,0.0268944544782255,-0.521647610749557));
#53643=DIRECTION('center_axis',(-0.406101978505186,0.60109853045139,0.688303522977584));
#53644=DIRECTION('ref_axis',(-0.850500677540323,0.0268943233501674,-0.525285915359424));
#53645=DIRECTION('center_axis',(0.429672669126836,0.584827952222689,-0.6880099299461));
#53646=DIRECTION('ref_axis',(-0.84693043322058,-0.00326197145677045,-0.531693709598878));
#53647=DIRECTION('center_axis',(-0.500371404828997,-8.11024626575273E-10,
0.865810866892681));
#53648=DIRECTION('ref_axis',(0.865704381467998,-0.0156832196312531,0.500309864513093));
#53649=DIRECTION('',(0.50037149549337,8.32135976759965E-8,-0.865810814495708));
#53650=DIRECTION('center_axis',(0.459164014243506,0.584827969931117,-0.668688756904166));
#53651=DIRECTION('ref_axis',(-0.827207822419288,0.00704480135620463,-0.561851928271312));
#53652=DIRECTION('center_axis',(0.55374888242709,4.06970665576237E-10,-0.83268371859353));
#53653=DIRECTION('ref_axis',(0.832581460086186,0.0156715280544909,0.553680878782347));
#53654=DIRECTION('',(-0.55374883641498,-1.32116539928992E-11,0.832683749192366));
#53655=DIRECTION('',(-0.258404637349593,-3.0780928980269E-8,-0.966036771244358));
#53656=DIRECTION('center_axis',(-0.532553557753611,0.793626260385853,-0.2941837299205));
#53657=DIRECTION('ref_axis',(-0.830371106917834,-0.557210754379392,1.99771634101076E-17));
#53658=DIRECTION('center_axis',(0.843956944123754,0.471546674539063,-0.255695933085463));
#53659=DIRECTION('ref_axis',(0.460837498610183,-0.39342086414382,0.795517959276244));
#53660=DIRECTION('center_axis',(-0.396601983388789,-0.601098528044585,0.693820889246434));
#53661=DIRECTION('ref_axis',(-0.867318529731536,-0.00227572042476273,-0.497748319013611));
#53662=DIRECTION('',(-0.980355882941529,5.05127141378872E-12,0.197236768331708));
#53663=DIRECTION('center_axis',(0.,-1.,1.45983193964168E-32));
#53664=DIRECTION('ref_axis',(1.,0.,0.));
#53665=DIRECTION('center_axis',(0.393634171246799,0.601098527296137,-0.695508950128797));
#53666=DIRECTION('ref_axis',(-0.868667549393486,-0.00432809960814291,-0.495376580173606));
#53667=DIRECTION('center_axis',(0.40315766119088,-0.601098528266436,-0.69003221630517));
#53668=DIRECTION('ref_axis',(-0.864676207687786,-0.00330178542044302,-0.502318777343339));
#53669=DIRECTION('center_axis',(-0.406101983502883,0.601098527737377,0.688303522399081));
#53670=DIRECTION('ref_axis',(-0.862522320557366,-0.00330190096595632,-0.506008244982577));
#53671=DIRECTION('center_axis',(0.340062297717029,0.584828255987335,-0.736432987223025));
#53672=DIRECTION('ref_axis',(-0.897125081634952,-0.0330815410846242,-0.44053626359353));
#53673=DIRECTION('center_axis',(-0.444988893932816,-1.08268168110917E-7,
0.895536087646075));
#53674=DIRECTION('ref_axis',(0.895426060219439,-0.0156751635312524,0.444934219776545));
#53675=DIRECTION('',(0.445019414620048,3.8857805861828E-13,-0.89552092136992));
#53676=DIRECTION('center_axis',(0.371736677655948,0.584827952226369,-0.72096331999626));
#53677=DIRECTION('ref_axis',(-0.88093786543938,-0.0227607295790456,-0.472684277741643));
#53678=DIRECTION('center_axis',(0.500371546002264,4.5264802562808E-10,-0.865810785305487));
#53679=DIRECTION('ref_axis',(0.865704161711832,0.015693390508689,0.500309925835133));
#53680=DIRECTION('',(-0.50037149436294,-2.12607709212252E-11,0.865810815149013));
#53681=DIRECTION('',(-0.318552670357103,0.,-0.947905162032763));
#53682=DIRECTION('center_axis',(-0.306515838597793,-0.601098527943026,0.73805731511409));
#53683=DIRECTION('ref_axis',(-0.91339069879748,-0.0324816877714825,-0.405786115225456));
#53684=DIRECTION('',(-0.966036775394095,8.00811321699466E-12,0.258404621835947));
#53685=DIRECTION('center_axis',(0.,-1.,1.45983193964168E-32));
#53686=DIRECTION('ref_axis',(1.,0.,0.));
#53687=DIRECTION('center_axis',(0.303359823568943,0.601098519834244,-0.73936011989916));
#53688=DIRECTION('ref_axis',(-0.914428808686088,-0.0345386141111437,-0.403270427852358));
#53689=DIRECTION('center_axis',(0.40315766702957,-0.601098530966851,-0.690032210541485));
#53690=DIRECTION('ref_axis',(-0.875386226563281,-0.0335099532194896,-0.482261378692642));
#53691=DIRECTION('center_axis',(-0.406102014405697,0.60109852375045,0.68830350764809));
#53692=DIRECTION('ref_axis',(-0.873317916729201,-0.0335100846096989,-0.485996800966035));
#53693=DIRECTION('',(0.387911046558289,7.77156117236932E-13,-0.921696815638447));
#53694=DIRECTION('center_axis',(0.278444757278483,0.584827952146073,-0.76186926931906));
#53695=DIRECTION('ref_axis',(-0.924224401747177,-0.0526562728447773,-0.378201761160852));
#53696=DIRECTION('center_axis',(0.44501947109597,4.54565369276803E-10,-0.89552089330482));
#53697=DIRECTION('ref_axis',(0.895409489159723,0.0157729998144009,0.444964110012907));
#53698=DIRECTION('',(-0.445019414618126,-1.75304215565769E-10,0.895520921370875));
#53699=DIRECTION('',(-0.37744353701714,-1.43735365431523E-13,-0.926032600054658));
#53700=DIRECTION('',(-0.947905162043636,6.51326541667543E-11,0.31855267032475));
#53701=DIRECTION('center_axis',(0.,-1.,1.45983193964168E-32));
#53702=DIRECTION('ref_axis',(1.,0.,0.));
#53703=DIRECTION('center_axis',(0.386892778599255,0.601098538778694,-0.699281434435283));
#53704=DIRECTION('ref_axis',(-0.891933617243813,0.0514848751370183,-0.449225700581002));
#53705=DIRECTION('center_axis',(-0.229579642912527,0.601098536382064,0.765489214241127));
#53706=DIRECTION('ref_axis',(-0.944431780630213,0.0525164994541969,-0.324485175348155));
#53707=DIRECTION('center_axis',(0.332920489062412,0.584827930050483,-0.73968928625154));
#53708=DIRECTION('ref_axis',(-0.918057474730095,0.0219594825824973,-0.395838671957289));
#53709=DIRECTION('center_axis',(-0.329268426587499,-1.02921683725058E-8,
0.944236359844606));
#53710=DIRECTION('ref_axis',(0.944119399299011,-0.0157391393486129,0.329227640637658));
#53711=DIRECTION('',(0.32927177081541,1.16573417585652E-12,-0.944235193658913));
#53712=DIRECTION('center_axis',(0.364750270111432,0.584827952319838,-0.724522951078172));
#53713=DIRECTION('ref_axis',(-0.902955161127037,0.0322834330697393,-0.428520427684933));
#53714=DIRECTION('center_axis',(0.387911115801846,5.59178227092144E-10,
-0.92169678649617));
#53715=DIRECTION('ref_axis',(0.92158315486564,0.0157020800826605,0.387863292087524));
#53716=DIRECTION('',(-0.387911046558911,0.,0.921696815638185));
#53717=DIRECTION('',(-0.434844806474091,-1.64268989064544E-13,-0.900505410468205));
#53718=DIRECTION('center_axis',(-0.299367242653868,-0.601098528133014,0.740985703979601));
#53719=DIRECTION('ref_axis',(-0.933352193011291,0.0232723686584569,-0.35820675685704));
#53720=DIRECTION('',(-0.926032600054671,0.,0.377443537017109));
#53721=DIRECTION('center_axis',(0.,-1.,1.45983193964168E-32));
#53722=DIRECTION('ref_axis',(1.,0.,0.));
#53723=DIRECTION('center_axis',(0.296198799055564,0.601098532815511,-0.742257923693026));
#53724=DIRECTION('ref_axis',(-0.934367830445983,0.0212180089737124,-0.3556775977242));
#53725=DIRECTION('center_axis',(0.226307099698326,-0.60109852540265,-0.766463084163153));
#53726=DIRECTION('ref_axis',(-0.95395833364752,0.0222452778845224,-0.299113097801297));
#53727=DIRECTION('center_axis',(-0.22957958291146,0.601098530145375,0.765489237133527));
#53728=DIRECTION('ref_axis',(-0.952671761995156,0.0222451527836799,-0.303185862260555));
#53729=DIRECTION('center_axis',(0.237586792125608,0.584827953016327,-0.775582865706945));
#53730=DIRECTION('ref_axis',(-0.954441832450582,-0.0078464556792525,-0.298293851095942));
#53731=DIRECTION('center_axis',(-0.269332588157193,-1.65064812737033E-9,
0.963047224676209));
#53732=DIRECTION('ref_axis',(0.962928861348009,-0.0156778483098861,0.269299485806043));
#53733=DIRECTION('',(0.269333009823076,7.77156117237388E-13,-0.96304710675005));
#53734=DIRECTION('center_axis',(0.271067301623241,0.584827952254122,-0.764525201842912));
#53735=DIRECTION('ref_axis',(-0.943100361129656,0.00246180457329884,-0.332499095269981));
#53736=DIRECTION('center_axis',(0.329271815799476,3.54739971595345E-10,
-0.94423517797216));
#53737=DIRECTION('ref_axis',(0.944119231938393,0.0156707406186497,0.329231383334763));
#53738=DIRECTION('',(-0.329271770814866,-6.33937347031782E-11,0.944235193659102));
#53739=DIRECTION('',(-0.49052994214159,1.64268989064518E-13,-0.871424337428425));
#53740=DIRECTION('center_axis',(-0.204136514467861,-0.60109852806508,0.772663473330341));
#53741=DIRECTION('ref_axis',(-0.965460822828727,-0.00691952277231014,-0.260456368298956));
#53742=DIRECTION('',(-0.900505410473572,2.35931335548655E-11,0.434844806462977));
#53743=DIRECTION('center_axis',(0.,-1.,1.45983193964168E-32));
#53744=DIRECTION('ref_axis',(1.,0.,0.));
#53745=DIRECTION('center_axis',(0.200833585503954,0.601098526072395,-0.773528559839402));
#53746=DIRECTION('ref_axis',(-0.966152069761189,-0.00897213720975653,-0.257817142273473));
#53747=DIRECTION('center_axis',(0.226307095413984,-0.601098528854831,-0.766463082720782));
#53748=DIRECTION('ref_axis',(-0.960712933164148,-0.00794567351718236,-0.277430218836191));
#53749=DIRECTION('center_axis',(-0.229579616820753,0.601098527017376,0.765489229419969));
#53750=DIRECTION('ref_axis',(-0.95951892089988,-0.0079458216776583,-0.281532066296179));
#53751=DIRECTION('center_axis',(0.138506937414431,0.584827952228472,-0.799244702566321));
#53752=DIRECTION('ref_axis',(-0.982832189620029,-0.0181546317366621,-0.183606362616349));
#53753=DIRECTION('center_axis',(-0.208331222268825,-7.38316845110491E-10,
0.978058332528269));
#53754=DIRECTION('ref_axis',(0.977938098822323,-0.015679506618582,0.208305611887868));
#53755=DIRECTION('',(0.208331317647447,2.06171549165144E-7,-0.978058312212128));
#53756=DIRECTION('center_axis',(0.173103405619857,0.584827782536667,-0.792471876937));
#53757=DIRECTION('ref_axis',(-0.972199735881759,-0.0273551074073029,-0.232549718662854));
#53758=DIRECTION('center_axis',(0.269333098110424,6.04766748526227E-10,
-0.963047082058941));
#53759=DIRECTION('ref_axis',(0.96292834879903,0.0157023279251934,0.269299892270502));
#53760=DIRECTION('',(0.269333010693047,-1.2926740481586E-5,-0.963047106419991));
#53761=DIRECTION('',(-0.544279213551348,-7.6263051490058E-8,-0.838904129025433));
#53762=DIRECTION('center_axis',(-0.208331314516526,2.31191508624251E-11,
0.978058312879051));
#53763=DIRECTION('ref_axis',(0.754939979655494,-0.635772805085298,0.160805993146194));
#53764=DIRECTION('',(0.871424337428539,0.,-0.490529942141387));
#53765=DIRECTION('center_axis',(0.137250389382567,0.398564391564464,-0.906812415216721));
#53766=DIRECTION('ref_axis',(-4.29084615902504E-17,0.915476128559304,0.402372287860469));
#53767=DIRECTION('center_axis',(-0.139583766916631,5.7445652467052E-5,0.990210264900017));
#53768=DIRECTION('ref_axis',(0.990210198381314,-0.000363006345283363,0.139583778599206));
#53769=DIRECTION('',(0.146508334828672,5.9497368376234E-5,-0.989209433985439));
#53770=DIRECTION('center_axis',(0.182651732966148,0.590180063810584,-0.786336974028945));
#53771=DIRECTION('ref_axis',(0.0318357966482478,0.795821663447861,0.604693610052935));
#53772=DIRECTION('center_axis',(-0.698011204256667,0.550037558037817,-0.458518313134768));
#53773=DIRECTION('ref_axis',(-0.618934249318816,-0.785442801876849,1.08964565723535E-17));
#53774=DIRECTION('center_axis',(0.70576152845033,-0.477126090197719,-0.523690136447205));
#53775=DIRECTION('ref_axis',(0.54964196122163,-0.0976209307608887,0.829676966259651));
#53776=DIRECTION('center_axis',(0.587274836641366,0.584827951389706,-0.559539572792825));
#53777=DIRECTION('ref_axis',(-0.703292607934828,0.0265489690024795,-0.71040457478055));
#53778=DIRECTION('center_axis',(-0.653745311499404,2.14805049941619E-11,
0.756714654075463));
#53779=DIRECTION('ref_axis',(0.756620818603737,-0.0157477670561346,0.653664244615045));
#53780=DIRECTION('center_axis',(0.693441464837208,-0.000115441142812938,
-0.720512957217127));
#53781=DIRECTION('ref_axis',(0.017310355292461,0.999714013427519,0.016499786552871));
#53782=DIRECTION('',(-0.699969797667544,-6.06958927296982E-10,0.714172445809314));
#53783=DIRECTION('center_axis',(-0.556688241105297,-0.601098528020006,0.573392328015707));
#53784=DIRECTION('ref_axis',(-0.731671536606546,0.0279220135032058,-0.681085254341733));
#53785=DIRECTION('',(-0.999949569926115,2.24206636476405E-10,0.0100427886853574));
#53786=DIRECTION('center_axis',(0.,-1.,1.45983193964168E-32));
#53787=DIRECTION('ref_axis',(1.,0.,0.));
#53788=DIRECTION('center_axis',(0.554233466834936,0.60109853330817,-0.575765418807777));
#53789=DIRECTION('ref_axis',(-0.733564955864417,0.0258667335491262,-0.679126915696275));
#53790=DIRECTION('center_axis',(0.486462590005111,-0.601098524487545,-0.63406207297426));
#53791=DIRECTION('ref_axis',(-0.780633170909662,0.0268944538704173,-0.624410554704626));
#53792=DIRECTION('center_axis',(-0.489167050999535,0.601098530508858,0.631977968632222));
#53793=DIRECTION('ref_axis',(-0.777958442290685,0.0268943220480753,-0.627739880452265));
#53794=DIRECTION('center_axis',(0.512515081052865,0.584827952222668,-0.628732501142112));
#53795=DIRECTION('ref_axis',(-0.77361324188928,-0.0032619714457999,-0.633649675700892));
#53796=DIRECTION('center_axis',(-0.604940734512417,-4.95210567798345E-10,
0.796270499094106));
#53797=DIRECTION('ref_axis',(0.796172566385581,-0.015683219631898,0.604866333297676));
#53798=DIRECTION('',(0.604940785833409,8.32148189212586E-8,-0.796270460104637));
#53799=DIRECTION('center_axis',(0.539352292991265,0.584827969931393,-0.605867435691167));
#53800=DIRECTION('ref_axis',(-0.750266322713667,0.00704480135244388,-0.661098189209149));
#53801=DIRECTION('center_axis',(0.653745360770694,5.17440208614981E-10,
-0.756714611508721));
#53802=DIRECTION('ref_axis',(0.756621682456946,0.0156715280541952,0.653665076965617));
#53803=DIRECTION('',(-0.653745308265973,-1.48214773786071E-11,0.756714656868907));
#53804=DIRECTION('',(-0.135290527320362,-3.07809289802733E-8,-0.990805971528925));
#53805=DIRECTION('center_axis',(-0.491483215751795,0.793626260386506,-0.358610662779573));
#53806=DIRECTION('ref_axis',(-0.850173673706501,-0.526502349981832,-3.01975261095387E-16));
#53807=DIRECTION('center_axis',(0.869349289640561,0.471546674565597,-0.147903841422661));
#53808=DIRECTION('ref_axis',(0.3574942912207,-0.393410391429238,0.84701009182896));
#53809=DIRECTION('center_axis',(-0.480433476380654,-0.601098528055858,0.638642493373155));
#53810=DIRECTION('ref_axis',(-0.798095056225195,-0.00227571851785752,-0.602527262731015));
#53811=DIRECTION('',(-0.997345805939199,5.19500677922194E-12,0.0728103246489838));
#53812=DIRECTION('center_axis',(0.,-1.,1.45983193964168E-32));
#53813=DIRECTION('ref_axis',(1.,0.,0.));
#53814=DIRECTION('center_axis',(0.477700635629862,0.60109852730126,-0.640689209519782));
#53815=DIRECTION('ref_axis',(-0.799730696663546,-0.00432809833535144,-0.600343302102089));
#53816=DIRECTION('center_axis',(0.486462610921983,-0.601098528267777,-0.634062053342794));
#53817=DIRECTION('ref_axis',(-0.794900741263355,-0.0033017849475055,-0.606730508343803));
#53818=DIRECTION('center_axis',(-0.489167051144032,0.601098527750881,0.631977971143595));
#53819=DIRECTION('ref_axis',(-0.792301426769745,-0.00330189864368045,-0.61012092785281));
#53820=DIRECTION('center_axis',(0.429680332517662,0.584828255987283,-0.688004885772176));
#53821=DIRECTION('ref_axis',(-0.834837147990686,-0.0330815410860676,-0.549502090964309));
#53822=DIRECTION('center_axis',(-0.553720478367964,-1.08069513787359E-7,
0.832702607078867));
#53823=DIRECTION('ref_axis',(0.832600299740156,-0.0156751635310958,0.553652445240582));
#53824=DIRECTION('',(0.553748836414939,1.16573417585621E-12,-0.832683749192394));
#53825=DIRECTION('center_axis',(0.459166087091293,0.584827952226198,-0.668687349035544));
#53826=DIRECTION('ref_axis',(-0.814748358265621,-0.0227607295829982,-0.579367812268101));
#53827=DIRECTION('center_axis',(0.604940842662418,5.5376368860139E-10,-0.796270416930633));
#53828=DIRECTION('ref_axis',(0.796172357150687,0.0156933905073754,0.604866344908941));
#53829=DIRECTION('',(-0.604940784793415,-2.24265050970792E-11,0.796270460894743));
#53830=DIRECTION('',(-0.197236768334464,0.,-0.980355882940974));
#53831=DIRECTION('center_axis',(-0.39660197790353,-0.601098527876615,0.69382089252744));
#53832=DIRECTION('ref_axis',(-0.855329855112446,-0.0324816889100509,-0.517064578983005));
#53833=DIRECTION('',(-0.99080597370157,8.1518485824271E-12,0.135290511408906));
#53834=DIRECTION('center_axis',(0.,-1.,1.45983193964168E-32));
#53835=DIRECTION('ref_axis',(1.,0.,0.));
#53836=DIRECTION('center_axis',(0.393634150632677,0.601098520441866,-0.695508967719533));
#53837=DIRECTION('ref_axis',(-0.856675070654286,-0.0345386033944676,-0.514698851946489));
#53838=DIRECTION('center_axis',(0.486462608228835,-0.601098531310315,-0.634062052524657));
#53839=DIRECTION('ref_axis',(-0.808040171738806,-0.0335099469771996,-0.588173583485272));
#53840=DIRECTION('center_axis',(-0.489167083046666,0.601098523747394,0.631977950258014));
#53841=DIRECTION('ref_axis',(-0.805519993522239,-0.0335100846374624,-0.591620329488027));
#53842=DIRECTION('',(0.500371494362523,1.60982338570607E-12,-0.865810815149254));
#53843=DIRECTION('center_axis',(0.371736676294122,0.584827952147084,-0.720963320762747));
#53844=DIRECTION('ref_axis',(-0.869535366613621,-0.0526562728332215,-0.491055560134929));
#53845=DIRECTION('center_axis',(0.553748893832433,4.99550230227221E-10,
-0.832683711008782));
#53846=DIRECTION('ref_axis',(0.832580123902208,0.0157729998146186,0.553680006646287));
#53847=DIRECTION('',(-0.553748836412657,-1.76525460892907E-10,0.832683749193911));
#53848=DIRECTION('',(-0.258404621839997,0.,-0.966036775393012));
#53849=DIRECTION('',(-0.98035588294767,6.51326541667506E-11,0.197236768301184));
#53850=DIRECTION('center_axis',(0.,-1.,1.45983193964168E-32));
#53851=DIRECTION('ref_axis',(1.,0.,0.));
#53852=DIRECTION('center_axis',(0.47148522438417,0.601098538304408,-0.645276863397188));
#53853=DIRECTION('ref_axis',(-0.828597540311574,0.0514848806124787,-0.557472352012123));
#53854=DIRECTION('center_axis',(-0.323710583623996,0.60109853674469,0.730679141055228));
#53855=DIRECTION('ref_axis',(-0.896315875410475,0.0525164952408666,-0.440295206895068));
#53856=DIRECTION('center_axis',(0.423002961639728,0.584827930050679,-0.692130613884878));
#53857=DIRECTION('ref_axis',(-0.861206576608442,0.0219594825779789,-0.507780477698066));
#53858=DIRECTION('center_axis',(-0.445016265398051,-1.00945786707435E-8,
0.89552248633475));
#53859=DIRECTION('ref_axis',(0.89541155989297,-0.015739139348497,0.44496114201423));
#53860=DIRECTION('',(0.445019414620412,1.60982338570637E-12,-0.895520921369739));
#53861=DIRECTION('center_axis',(0.452680909523334,0.584827952320435,-0.673094540415991));
#53862=DIRECTION('ref_axis',(-0.842127239138703,0.0322834330609294,-0.538311706217157));
#53863=DIRECTION('center_axis',(0.500371556578268,5.32646000511302E-10,
-0.865810779193376));
#53864=DIRECTION('ref_axis',(0.865704037482965,0.0157020800820386,0.500309868148521));
#53865=DIRECTION('',(-0.500371494363197,-4.44089209850264E-13,0.865810815148864));
#53866=DIRECTION('',(-0.318552670357111,-1.64268989064552E-13,-0.94790516203276));
#53867=DIRECTION('center_axis',(-0.389876779295978,-0.601098528066563,0.697622144518082));
#53868=DIRECTION('ref_axis',(-0.88109721997925,0.0232723703365245,-0.472362239942777));
#53869=DIRECTION('',(-0.966036775392989,0.,0.258404621840081));
#53870=DIRECTION('center_axis',(0.,-1.,1.45983193964168E-32));
#53871=DIRECTION('ref_axis',(1.,0.,0.));
#53872=DIRECTION('center_axis',(0.386892787612457,0.60109853235182,-0.699281434973037));
#53873=DIRECTION('ref_axis',(-0.882421829328887,0.0212180217980572,-0.469980330093545));
#53874=DIRECTION('center_axis',(0.320585907961959,-0.601098525668862,-0.732055488371562));
#53875=DIRECTION('ref_axis',(-0.908947271769225,0.0222452708710491,-0.416317192855587));
#53876=DIRECTION('center_axis',(-0.323710520662284,0.60109853014702,0.730679174376584));
#53877=DIRECTION('ref_axis',(-0.907160396119142,0.022245152793508,-0.420196583625039));
#53878=DIRECTION('center_axis',(0.332919657819598,0.584827953016086,-0.739689642220504));
#53879=DIRECTION('ref_axis',(-0.909529640592536,-0.00784645564255627,-0.41556499614075));
#53880=DIRECTION('center_axis',(-0.387910658915138,-1.51457921573024E-9,
0.921696978784255));
#53881=DIRECTION('ref_axis',(0.921583697610959,-0.0156778483096378,0.387862982727266));
#53882=DIRECTION('',(0.387911046558196,1.22124532708725E-12,-0.921696815638486));
#53883=DIRECTION('center_axis',(0.364750270664268,0.584827952254338,-0.724522950852725));
#53884=DIRECTION('ref_axis',(-0.893990546328477,0.00246180456674765,-0.448079058418921));
#53885=DIRECTION('center_axis',(0.445019479869039,5.51522626024051E-10,
-0.895520888945138));
#53886=DIRECTION('ref_axis',(0.895410924712026,0.0156707406188141,0.444964834335043));
#53887=DIRECTION('',(-0.445019414619707,-6.38378239129916E-11,0.895520921370089));
#53888=DIRECTION('',(-0.377443537017128,1.64268989064547E-13,-0.926032600054663));
#53889=DIRECTION('center_axis',(-0.299367251286446,-0.601098528085944,0.740985700530117));
#53890=DIRECTION('ref_axis',(-0.925204036176552,-0.00691952105771956,-0.379406920958157));
#53891=DIRECTION('',(-0.947905162036754,2.35931335548688E-11,0.318552670345227));
#53892=DIRECTION('center_axis',(0.,-1.,1.45983193964168E-32));
#53893=DIRECTION('ref_axis',(1.,0.,0.));
#53894=DIRECTION('center_axis',(0.296198808422639,0.601098526255464,-0.74225792526757));
#53895=DIRECTION('ref_axis',(-0.926220609588028,-0.0089721241941348,-0.376875156201396));
#53896=DIRECTION('center_axis',(0.320585901750229,-0.601098528786845,-0.73205548853163));
#53897=DIRECTION('ref_axis',(-0.918366195244468,-0.00794567929387724,-0.395651864159336));
#53898=DIRECTION('center_axis',(-0.323710545522671,0.601098527087631,0.730679165879592));
#53899=DIRECTION('ref_axis',(-0.91666750615744,-0.00794581654303214,-0.399571704647068));
#53900=DIRECTION('center_axis',(0.237586691867558,0.584827952229731,-0.775582897012441));
#53901=DIRECTION('ref_axis',(-0.952070285106708,-0.0181546317102868,-0.305340108017759));
#53902=DIRECTION('center_axis',(-0.329271743027232,-2.29656697345778E-10,
0.944235203349149));
#53903=DIRECTION('ref_axis',(0.944119127553756,-0.0156795066177309,0.329231265312635));
#53904=DIRECTION('',(0.329271773866349,2.06172326321069E-7,-0.944235192594973));
#53905=DIRECTION('center_axis',(0.271061496426085,0.584827782537064,-0.764527389913555));
#53906=DIRECTION('ref_axis',(-0.935387442372695,-0.0273551073963662,-0.35256493125494));
#53907=DIRECTION('center_axis',(0.387911113057852,4.51452499428076E-10,
-0.921696787651025));
#53908=DIRECTION('ref_axis',(0.921583152433633,0.0157023279244598,0.387863287832504));
#53909=DIRECTION('',(0.387911047380125,-1.29267404815429E-5,-0.921696815201915));
#53910=DIRECTION('',(-0.434844842242925,-7.62630514900653E-8,-0.900505393195799));
#53911=DIRECTION('center_axis',(-0.329271770804114,-1.01359413495107E-11,
0.944235193662852));
#53912=DIRECTION('ref_axis',(0.728832717346511,-0.635772805085059,0.254157058606634));
#53913=DIRECTION('',(0.92603260005471,0.,-0.377443537017014));
#53914=DIRECTION('center_axis',(0.249821861302329,0.398564391568801,-0.882459893359937));
#53915=DIRECTION('ref_axis',(-4.0408704040895E-16,0.91135738249489,0.411615987750794));
#53916=DIRECTION('center_axis',(-0.262589361671171,5.74456459349265E-5,
0.96490767632822));
#53917=DIRECTION('ref_axis',(0.964907608885033,-0.000362964710733412,0.262589364926279));
#53918=DIRECTION('',(0.269333889882249,5.94973682696981E-5,-0.963046858787754));
#53919=DIRECTION('center_axis',(0.279765625248216,0.590180063806943,-0.757244139768877));
#53920=DIRECTION('ref_axis',(-0.0441970528704828,0.79582076062354,0.603917161105837));
#53921=DIRECTION('center_axis',(-0.635039594591643,0.550037558039011,-0.542386760575297));
#53922=DIRECTION('ref_axis',(-0.654706135033812,-0.755883507393228,-4.32073907844199E-16));
#53923=DIRECTION('center_axis',(0.76583216617711,-0.477126090214006,-0.431105308811632));
#53924=DIRECTION('ref_axis',(-0.441323162917497,0.0976183354969225,-0.89202271632919));
#53925=DIRECTION('center_axis',(0.652772903104731,0.584827951389971,-0.481522381873607));
#53926=DIRECTION('ref_axis',(-0.608709633166722,0.0265489689982835,-0.792948759211567));
#53927=DIRECTION('center_axis',(-0.743431828170876,-3.27000309038643E-12,
0.668811720039735));
#53928=DIRECTION('ref_axis',(0.668728784863672,-0.01574776705564,0.743339639819859));
#53929=DIRECTION('center_axis',(0.778277686855452,-0.000115441219111835,
-0.627920240807901));
#53930=DIRECTION('ref_axis',(0.0157248311762356,0.999689948221239,0.0193064007493675));
#53931=DIRECTION('',(-0.783959868697913,-6.06570349238166E-10,0.620811504622097));
#53932=DIRECTION('center_axis',(-0.624163700784653,-0.601098528100592,0.499099423099355));
#53933=DIRECTION('ref_axis',(-0.640539472529953,0.0279220117807904,-0.767417451840368));
#53934=DIRECTION('',(-0.99332336407675,2.24206636476409E-10,-0.115363314702931));
#53935=DIRECTION('center_axis',(0.,-1.,1.45983193964168E-32));
#53936=DIRECTION('ref_axis',(1.,0.,0.));
#53937=DIRECTION('center_axis',(0.622025706030483,0.601098533560836,-0.501761471207477));
#53938=DIRECTION('ref_axis',(-0.642663410630348,0.0258667278601001,-0.765711860314818));
#53939=DIRECTION('center_axis',(0.562095733968384,-0.601098524369219,-0.568092377924304));
#53940=DIRECTION('ref_axis',(-0.696218253805938,0.0268944565437029,-0.717326167984014));
#53941=DIRECTION('center_axis',(-0.564517655764164,0.601098530153958,0.565685754971154));
#53942=DIRECTION('ref_axis',(-0.693147346115239,0.0268943300857719,-0.720294003572596));
#53943=DIRECTION('center_axis',(0.587274823952193,0.584827952222734,-0.559539585240297));
#53944=DIRECTION('ref_axis',(-0.688095707625187,-0.0032619714632092,-0.725612607863153));
#53945=DIRECTION('center_axis',(-0.699969746350645,-5.63643803412786E-10,
0.714172496105677));
#53946=DIRECTION('ref_axis',(0.714084660570638,-0.0156832196315775,0.699883657588677));
#53947=DIRECTION('',(0.699969798606842,8.32135976760244E-8,-0.714172444888691));
#53948=DIRECTION('center_axis',(0.611034663886251,0.58482796993141,-0.533491223091179));
#53949=DIRECTION('ref_axis',(-0.661492674912475,0.00704480134835528,-0.74991853678323));
#53950=DIRECTION('center_axis',(0.743431876282904,5.62385146219574E-10,
-0.668811666559787));
#53951=DIRECTION('ref_axis',(0.668729532510225,0.0156715280548055,0.743340578441056));
#53952=DIRECTION('',(-0.743431826076989,-1.44328993199839E-11,0.66881172236724));
#53953=DIRECTION('',(-0.0100428048565106,-3.07809289802904E-8,-0.999949569763702));
#53954=DIRECTION('center_axis',(-0.442661889839964,0.793626260386774,-0.417382091263887));
#53955=DIRECTION('ref_axis',(-0.873334555251418,-0.487120882947763,4.49831660585486E-16));
#53956=DIRECTION('center_axis',(0.881031477541083,0.471546674544276,-0.0377792179380582));
#53957=DIRECTION('ref_axis',(0.248517210562371,-0.393411140887218,0.885136639327576));
#53958=DIRECTION('center_axis',(-0.556688238442204,-0.601098528035278,0.573392330585209));
#53959=DIRECTION('ref_axis',(-0.716285152269076,-0.0022757229430359,-0.697803985173453));
#53960=DIRECTION('',(-0.998606989791731,5.05127141378911E-12,-0.0527643813485665));
#53961=DIRECTION('center_axis',(0.,-1.,1.45983193964168E-32));
#53962=DIRECTION('ref_axis',(1.,0.,0.));
#53963=DIRECTION('center_axis',(0.554233477834988,0.601098527323786,-0.575765414466786));
#53964=DIRECTION('ref_axis',(-0.718181610818199,-0.00432809493829295,-0.695842253299397));
#53965=DIRECTION('center_axis',(0.562095757374046,-0.601098528262797,-0.568092350645912));
#53966=DIRECTION('ref_axis',(-0.712589213394155,-0.00330178665336215,-0.70157373893212));
#53967=DIRECTION('center_axis',(-0.564517663858828,0.601098527757849,0.565685749439314));
#53968=DIRECTION('ref_axis',(-0.70958546592687,-0.00330189725113067,-0.704611640565134));
#53969=DIRECTION('center_axis',(0.512522051794119,0.584828255986954,-0.62872653628108));
#53970=DIRECTION('ref_axis',(-0.759383333816913,-0.0330815410895385,-0.649801942102555));
#53971=DIRECTION('center_axis',(-0.653719533738691,-1.0810677741567E-7,
0.756736923381209));
#53972=DIRECTION('ref_axis',(0.756643949578265,-0.0156751635310768,0.653639214563263));
#53973=DIRECTION('',(0.65374530826584,0.,-0.756714656869022));
#53974=DIRECTION('center_axis',(0.539354173045247,0.58482795222633,-0.605865779123921));
#53975=DIRECTION('ref_axis',(-0.735709782773397,-0.0227607295838477,-0.676914370301246));
#53976=DIRECTION('center_axis',(0.699969849654639,5.54772316281761E-10,
-0.714172394856075));
#53977=DIRECTION('ref_axis',(0.7140844453511,0.0156933905089797,0.699883649188881));
#53978=DIRECTION('',(-0.699969797674486,-2.28150831557062E-11,0.71417244580251));
#53979=DIRECTION('',(-0.0728103246514917,-1.4373536543164E-13,-0.997345805939016));
#53980=DIRECTION('center_axis',(-0.480433477524117,-0.601098528245212,0.638642492334737));
#53981=DIRECTION('ref_axis',(-0.783779942752042,-0.0324816822283564,-0.62018863393263));
#53982=DIRECTION('',(-0.999949569924982,8.00811321699498E-12,0.0100427887981127));
#53983=DIRECTION('center_axis',(0.,-1.,1.45983193964168E-32));
#53984=DIRECTION('ref_axis',(1.,0.,0.));
#53985=DIRECTION('center_axis',(0.477700614898206,0.601098520407419,-0.640689231445236));
#53986=DIRECTION('ref_axis',(-0.785411060893115,-0.0345386039953625,-0.618010153849274));
#53987=DIRECTION('center_axis',(0.562095763024861,-0.601098530840434,-0.568092342327346));
#53988=DIRECTION('ref_axis',(-0.727950828462085,-0.0335099556139018,-0.684809954816749));
#53989=DIRECTION('center_axis',(-0.564517689922951,0.601098523962191,0.565685727462282));
#53990=DIRECTION('ref_axis',(-0.725018542428448,-0.0335100808076772,-0.687913648373974));
#53991=DIRECTION('',(0.604940784793647,0.,-0.796270460894567));
#53992=DIRECTION('center_axis',(0.459166085830651,0.584827952146512,-0.668687349970878));
#53993=DIRECTION('ref_axis',(-0.801133239325096,-0.0526562728411134,-0.596165119559137));
#53994=DIRECTION('center_axis',(0.653745376981871,6.72256483690371E-10,
-0.756714597503465));
#53995=DIRECTION('ref_axis',(0.756620461065956,0.0157729998144629,0.653664050084746));
#53996=DIRECTION('',(-0.653745308264173,-1.77302617010168E-10,0.756714656870463));
#53997=DIRECTION('',(-0.135290511413073,-1.43735365431586E-13,-0.990805973701001));
#53998=DIRECTION('',(-0.9973458059415,6.51326541667556E-11,0.0728103246174644));
#53999=DIRECTION('center_axis',(0.,-1.,1.45983193964168E-32));
#54000=DIRECTION('ref_axis',(1.,0.,0.));
#54001=DIRECTION('center_axis',(0.548642066116338,0.601098537770836,-0.581095888109148));
#54002=DIRECTION('ref_axis',(-0.752193983083953,0.0514848867700612,-0.656927331024195));
#54003=DIRECTION('center_axis',(-0.412736402430169,0.601098536370573,0.684345827547854));
#54004=DIRECTION('ref_axis',(-0.834064537983385,0.0525164995610771,-0.549161509714959));
#54005=DIRECTION('center_axis',(0.506414424843185,0.58482793005016,-0.63365662826486));
#54006=DIRECTION('ref_axis',(-0.79077393630234,0.0219594825879678,-0.611714281989044));
#54007=DIRECTION('center_axis',(-0.55374598213335,-9.39659742892925E-9,
0.832685647331075));
#54008=DIRECTION('ref_axis',(0.832582504369383,-0.0157391393474978,0.553677390644233));
#54009=DIRECTION('',(0.553748836414868,3.88578058618135E-13,-0.832683749192441));
#54010=DIRECTION('center_axis',(0.533472500561931,0.58482795232209,-0.611051026778412));
#54011=DIRECTION('ref_axis',(-0.768018467538781,0.0322834330421544,-0.639613487561352));
#54012=DIRECTION('center_axis',(0.604940834163369,4.55365815109069E-10,
-0.796270423387512));
#54013=DIRECTION('ref_axis',(0.796172254977744,0.0157020800819334,0.604866253881596));
#54014=DIRECTION('',(-0.604940784794057,-1.16573417585723E-12,0.796270460894256));
#54015=DIRECTION('',(-0.197236768334425,0.,-0.980355882940982));
#54016=DIRECTION('center_axis',(-0.47423772019324,-0.601098528163163,0.64325667053362));
#54017=DIRECTION('ref_axis',(-0.814946820275726,0.0232723678061855,-0.579068283554865));
#54018=DIRECTION('',(-0.990805973700986,0.,0.135290511413188));
#54019=DIRECTION('center_axis',(0.,-1.,1.45983193964168E-32));
#54020=DIRECTION('ref_axis',(1.,0.,0.));
#54021=DIRECTION('center_axis',(0.471485217112986,0.601098532584745,-0.645276874038104));
#54022=DIRECTION('ref_axis',(-0.816559520194112,0.021218015378734,-0.576871169156293));
#54023=DIRECTION('center_axis',(0.409808866426316,-0.601098525471459,-0.686102948306168));
#54024=DIRECTION('ref_axis',(-0.849601574644904,0.0222452761089785,-0.526955702172142));
#54025=DIRECTION('center_axis',(-0.412736344185965,0.601098529989856,0.684345868280096));
#54026=DIRECTION('ref_axis',(-0.847342571781816,0.0222451570215671,-0.530580549054772));
#54027=DIRECTION('center_axis',(0.423002181533233,0.584827953016183,-0.692131071249533));
#54028=DIRECTION('ref_axis',(-0.85027362301044,-0.00784645566944904,-0.526282432868634));
#54029=DIRECTION('center_axis',(-0.500371129583691,-1.52148457841835E-9,
0.865811025963022));
#54030=DIRECTION('ref_axis',(0.865704613456417,-0.0156778483093056,0.500309631441038));
#54031=DIRECTION('',(0.50037149436275,3.88578058618399E-13,-0.865810815149123));
#54032=DIRECTION('center_axis',(0.452680910063766,0.584827952254225,-0.673094540110058));
#54033=DIRECTION('ref_axis',(-0.830781966560561,0.0024618045719596,-0.55659254716176));
#54034=DIRECTION('center_axis',(0.553748900359298,5.82366288656275E-10,
-0.832683706668305));
#54035=DIRECTION('ref_axis',(0.832581458437494,0.0156707406186236,0.553680903548749));
#54036=DIRECTION('',(-0.55374883641417,-6.4170890820376E-11,0.832683749192905));
#54037=DIRECTION('',(-0.258404621839981,1.64268989064578E-13,-0.966036775393016));
#54038=DIRECTION('center_axis',(-0.38987678399407,-0.601098528077048,0.697622141883447));
#54039=DIRECTION('ref_axis',(-0.870356230200551,-0.00691952173119867,-0.492373996845991));
#54040=DIRECTION('',(-0.980355882943439,2.3449398189433E-11,0.197236768322213));
#54041=DIRECTION('center_axis',(0.,-1.,1.45983193964168E-32));
#54042=DIRECTION('ref_axis',(1.,0.,0.));
#54043=DIRECTION('center_axis',(0.386892766875141,0.601098526142014,-0.699281451784327));
#54044=DIRECTION('ref_axis',(-0.871682106507819,-0.00897213204655847,-0.489989597890231));
#54045=DIRECTION('center_axis',(0.409808864115314,-0.601098528821877,-0.686102946751208));
#54046=DIRECTION('ref_axis',(-0.861536277690818,-0.00794567680510276,-0.507633833035939));
#54047=DIRECTION('center_axis',(-0.412736369131606,0.60109852713163,0.684345855745649));
#54048=DIRECTION('ref_axis',(-0.859359697506052,-0.00794581332026708,-0.511309861388362));
#54049=DIRECTION('center_axis',(0.332919562152049,0.584827952227919,-0.739689685901721));
#54050=DIRECTION('ref_axis',(-0.90629366348865,-0.0181546317530755,-0.42225845742416));
#54051=DIRECTION('center_axis',(-0.445019481897012,6.08170420604607E-10,
0.895520887937359));
#54052=DIRECTION('ref_axis',(0.895410800637064,-0.0156795066141847,0.444964775206789));
#54053=DIRECTION('',(0.445019417513644,2.06171882231856E-7,-0.895520919931955));
#54054=DIRECTION('center_axis',(0.364744785491104,0.584827782537139,-0.724525849248833));
#54055=DIRECTION('ref_axis',(-0.883823530127309,-0.0273551073961588,-0.467019984254042));
#54056=DIRECTION('center_axis',(0.500371579043315,6.52716079657588E-10,
-0.865810766210319));
#54057=DIRECTION('ref_axis',(0.865704021130687,0.0157023279252462,0.500309888664902));
#54058=DIRECTION('',(0.500371495123498,-1.29267395933215E-5,-0.86581081461297));
#54059=DIRECTION('',(-0.318552708008709,-7.62629077547213E-8,-0.947905149379574));
#54060=DIRECTION('center_axis',(-0.445019414093066,-4.78825638661493E-10,
0.895520921631798));
#54061=DIRECTION('ref_axis',(0.691231328023145,-0.635772805081915,0.343499914814592));
#54062=DIRECTION('',(0.966036775393033,0.,-0.258404621839916));
#54063=DIRECTION('center_axis',(0.35845349323297,0.398564391571384,-0.844190451829689));
#54064=DIRECTION('ref_axis',(-3.77661288183636E-16,0.904282187137336,0.426935271471116));
#54065=DIRECTION('center_axis',(-0.38145376525024,5.74456466242848E-5,0.924387917314161));
#54066=DIRECTION('ref_axis',(0.924387849993085,-0.000362969539878445,0.381453760026396));
#54067=DIRECTION('',(0.387911888600281,5.94973684118082E-5,-0.921696459330634));
#54068=DIRECTION('center_axis',(0.37246744627126,0.590180063809394,-0.716209113143714));
#54069=DIRECTION('ref_axis',(-0.119540363498291,0.795820897101943,0.59361536471907));
#54070=DIRECTION('center_axis',(-0.562053031166013,0.550037558040921,-0.617701444794714));
#54071=DIRECTION('ref_axis',(-0.73963826964566,-4.1371342815621E-16,0.673004628569205));
#54072=DIRECTION('center_axis',(0.813825173309153,-0.477126089925489,-0.33172169299089));
#54073=DIRECTION('ref_axis',(-0.326037099188356,0.0976292430140872,-0.940302260372343));
#54074=DIRECTION('center_axis',(0.70797635094518,0.584827951389921,-0.395911295336993));
#54075=DIRECTION('ref_axis',(-0.504526943851804,0.026548969000283,-0.862987668030419));
#54076=DIRECTION('center_axis',(-0.821393980625655,-2.78574751580884E-11,
0.570361226410019));
#54077=DIRECTION('ref_axis',(0.57029049946684,-0.0157477670569905,0.82129212467342));
#54078=DIRECTION('center_axis',(0.85084000898608,-0.000115441208927885,
-0.52542484313353));
#54079=DIRECTION('ref_axis',(0.0131765282484206,0.999690165025676,0.0211176005799707));
#54080=DIRECTION('',(-0.855586424283945,-6.07347505355654E-10,0.517659995152236));
#54081=DIRECTION('center_axis',(-0.681795727521764,-0.601098528130143,0.416935421153978));
#54082=DIRECTION('ref_axis',(-0.539305717521858,0.0279220110851815,-0.841647018853624));
#54083=DIRECTION('',(-0.971031855393334,2.24206636476412E-10,-0.23895006970365));
#54084=DIRECTION('center_axis',(0.,-1.,1.45983193964168E-32));
#54085=DIRECTION('ref_axis',(1.,0.,0.));
#54086=DIRECTION('center_axis',(0.680008247647369,0.601098532952695,-0.419844419771982));
#54087=DIRECTION('ref_axis',(-0.54162665863951,0.0258667416307407,-0.840221086576865));
#54088=DIRECTION('center_axis',(0.628864298647871,-0.601098524492875,-0.493163520283698));
#54089=DIRECTION('ref_axis',(-0.600823553899494,0.0268944537977208,-0.798929124162152));
#54090=DIRECTION('center_axis',(-0.630965493733841,0.60109853030328,0.490472326012841));
#54091=DIRECTION('ref_axis',(-0.597404892030046,0.0268943266317125,-0.801488671269654));
#54092=DIRECTION('center_axis',(0.652772892098893,0.584827952222548,-0.481522395782406));
#54093=DIRECTION('ref_axis',(-0.591726492967278,-0.00326197144519419,-0.806132195773706));
#54094=DIRECTION('center_axis',(-0.783959817463517,-6.47203937932624E-10,
0.620811569320812));
#54095=DIRECTION('ref_axis',(0.620735216178117,-0.0156832196310024,0.78386339882553));
#54096=DIRECTION('',(0.783959869514184,8.32140417652251E-8,-0.620811503591305));
#54097=DIRECTION('center_axis',(0.673080653132819,0.584827969931241,-0.452701535191125));
#54098=DIRECTION('ref_axis',(-0.562286892455316,0.00704480135906427,-0.826912221065063));
#54099=DIRECTION('center_axis',(0.821394025877762,6.05711839516913E-10,
-0.570361161241124));
#54100=DIRECTION('ref_axis',(0.57029111749682,0.0156715280541059,0.821293153820654));
#54101=DIRECTION('',(-0.821393979885835,-1.5210055437211E-11,0.570361227475456));
#54102=DIRECTION('',(0.11536329863905,-3.07809289802874E-8,-0.993323365942389));
#54103=DIRECTION('center_axis',(-0.386859521492136,0.793626260387047,-0.469571154836993));
#54104=DIRECTION('ref_axis',(-2.69928171055445E-16,0.509219680892889,0.860636576373178));
#54105=DIRECTION('center_axis',(0.878819272722778,0.471546674561253,0.0729412064695383));
#54106=DIRECTION('ref_axis',(0.135633310371155,-0.393433170232164,0.909293102183686));
#54107=DIRECTION('center_axis',(-0.624163700568947,-0.601098528038163,0.4990994234443));
#54108=DIRECTION('ref_axis',(-0.623178999774232,-0.0022757226821621,-0.782075926829781));
#54109=DIRECTION('',(-0.984119544876305,5.19500677922197E-12,-0.177506961532368));
#54110=DIRECTION('center_axis',(0.,-1.,1.45983193964168E-32));
#54111=DIRECTION('ref_axis',(1.,0.,0.));
#54112=DIRECTION('center_axis',(0.622025724926714,0.601098527339717,-0.501761455234875));
#54113=DIRECTION('ref_axis',(-0.625306372224195,-0.00432809260108738,-0.780367354820954));
#54114=DIRECTION('center_axis',(0.628864322227214,-0.601098528236074,-0.493163485653725));
#54115=DIRECTION('ref_axis',(-0.619039722698785,-0.00330179299804888,-0.785352735962643));
#54116=DIRECTION('center_axis',(-0.630965496664613,0.601098527762398,0.490472325356545));
#54117=DIRECTION('ref_axis',(-0.615678918250599,-0.00330189631434547,-0.787990207491503));
#54118=DIRECTION('center_axis',(0.587280992156649,0.584828255987147,-0.559532793722169));
#54119=DIRECTION('ref_axis',(-0.671953590829443,-0.0330815410858397,-0.739854028448047));
#54120=DIRECTION('center_axis',(-0.743409036258055,-1.0821547404186E-7,
0.668837054004829));
#54121=DIRECTION('ref_axis',(0.668754879990046,-0.0156751635329546,0.743317697715932));
#54122=DIRECTION('',(0.743431826076993,0.,-0.668811722367235));
#54123=DIRECTION('center_axis',(0.611036321497906,0.584827952226251,-0.533489343947148));
#54124=DIRECTION('ref_axis',(-0.645068624513626,-0.0227607295831316,-0.763785584347428));
#54125=DIRECTION('center_axis',(0.783959924147141,6.84547634730646E-10,
-0.620811434600886));
#54126=DIRECTION('ref_axis',(0.620734982387142,0.0156933905081134,0.783863380401964));
#54127=DIRECTION('',(-0.783959868704082,-2.28705943069331E-11,0.620811504614306));
#54128=DIRECTION('',(0.0527643813458746,0.,-0.998606989791874));
#54129=DIRECTION('center_axis',(-0.556688234994435,-0.601098527787945,0.573392334191822));
#54130=DIRECTION('ref_axis',(-0.699869364617338,-0.0324816905828272,-0.713531927980105));
#54131=DIRECTION('',(-0.993323364089748,8.17238220606141E-12,-0.115363314591021));
#54132=DIRECTION('center_axis',(0.,-1.,1.45983193964168E-32));
#54133=DIRECTION('ref_axis',(1.,0.,0.));
#54134=DIRECTION('center_axis',(0.55423346574626,0.601098520880261,-0.575765432830464));
#54135=DIRECTION('ref_axis',(-0.701760641393952,-0.0345385956231396,-0.711575075169677));
#54136=DIRECTION('center_axis',(0.628864320118186,-0.601098530849351,-0.493163485157857));
#54137=DIRECTION('ref_axis',(-0.636381272887134,-0.0335099554704704,-0.770646454869493));
#54138=DIRECTION('center_axis',(-0.630965517497451,0.601098524134483,0.490472303002444));
#54139=DIRECTION('ref_axis',(-0.633083115930161,-0.0335100777499132,-0.773358159595768));
#54140=DIRECTION('',(0.699969797674222,0.,-0.714172445802769));
#54141=DIRECTION('center_axis',(0.539354171899053,0.584827952145603,-0.60586578022221));
#54142=DIRECTION('ref_axis',(-0.720096762283953,-0.0526562728523631,-0.69187279891427));
#54143=DIRECTION('center_axis',(0.743431873707654,5.17806860950093E-10,
-0.668811669422363));
#54144=DIRECTION('ref_axis',(0.668728468241762,0.0157729998153311,0.743339389673285));
#54145=DIRECTION('',(-0.743431826075324,-1.7769119506863E-10,0.668811722369091));
#54146=DIRECTION('',(-0.0100427888024932,-1.43735365431651E-13,-0.999949569924938));
#54147=DIRECTION('',(-0.998606989790074,6.51326541667587E-11,-0.0527643813799327));
#54148=DIRECTION('center_axis',(0.,-1.,1.45983193964168E-32));
#54149=DIRECTION('ref_axis',(1.,0.,0.));
#54150=DIRECTION('center_axis',(0.617146485119927,0.601098537856876,-0.507750690487413));
#54151=DIRECTION('ref_axis',(-0.663927883266848,0.0514848857726378,-0.746022166130324));
#54152=DIRECTION('center_axis',(-0.495253123111622,0.601098536029601,0.627219972602321));
#54153=DIRECTION('ref_axis',(-0.758659505446537,0.0525165034839058,-0.649367208640413));
#54154=DIRECTION('center_axis',(0.581839430013544,0.584827930051117,-0.56518949911834));
#54155=DIRECTION('ref_axis',(-0.70787031866,0.0219594825710829,-0.706000986603702));
#54156=DIRECTION('center_axis',(-0.653742635283663,-1.02194371156788E-8,
0.756716966119018));
#54157=DIRECTION('ref_axis',(0.756623233263496,-0.0157391393489811,0.653661657418));
#54158=DIRECTION('',(0.653745308265769,0.,-0.756714656869083));
#54159=DIRECTION('center_axis',(0.605850911637909,0.584827952320374,-0.539370873381454));
#54160=DIRECTION('ref_axis',(-0.681797585877112,0.032283433062499,-0.730828182161745));
#54161=DIRECTION('center_axis',(0.699969850606534,5.5076297820919E-10,-0.714172393923111));
#54162=DIRECTION('ref_axis',(0.71408434698844,0.0157020800825275,0.699883554648325));
#54163=DIRECTION('',(-0.699969797674564,-1.22124532708828E-12,0.714172445802433));
#54164=DIRECTION('',(-0.0728103246515018,-1.6426898906465E-13,-0.997345805939015));
#54165=DIRECTION('center_axis',(-0.551119654299467,-0.601098528114907,0.578746651085713));
#54166=DIRECTION('ref_axis',(-0.73594421951875,0.0232723691575943,-0.676642078643304));
#54167=DIRECTION('',(-0.99994956992494,0.,0.0100427888023022));
#54168=DIRECTION('center_axis',(0.,-1.,1.45983193964168E-32));
#54169=DIRECTION('ref_axis',(1.,0.,0.));
#54170=DIRECTION('center_axis',(0.548642063374605,0.601098532266458,-0.581095896391607));
#54171=DIRECTION('ref_axis',(-0.73781956742827,0.0212180242146453,-0.674664421300239));
#54172=DIRECTION('center_axis',(0.492568906019118,-0.601098525584716,-0.629330148144049));
#54173=DIRECTION('ref_axis',(-0.776857147932723,0.0222452731343194,-0.629283814768039));
#54174=DIRECTION('center_axis',(-0.495253075494428,0.601098529992903,0.627220015986163));
#54175=DIRECTION('ref_axis',(-0.774161646564126,0.0222451569315223,-0.632596947496756));
#54176=DIRECTION('center_axis',(0.506413708192182,0.58482795301627,-0.633657179810853));
#54177=DIRECTION('ref_axis',(-0.777608282452322,-0.00784645567321364,-0.628700081274782));
#54178=DIRECTION('center_axis',(-0.604940525637679,-7.70162739777139E-10,
0.796270657779884));
#54179=DIRECTION('ref_axis',(0.796172792128776,-0.0156778483076014,0.604866175402719));
#54180=DIRECTION('',(0.604940784793799,0.,-0.796270460894452));
#54181=DIRECTION('center_axis',(0.533472501095234,0.584827952254122,-0.611051026377869));
#54182=DIRECTION('ref_axis',(-0.754471458890974,0.0024618045796853,-0.656328238945375));
#54183=DIRECTION('center_axis',(0.653745370650952,6.26092348591291E-10,
-0.75671460297291));
#54184=DIRECTION('ref_axis',(0.756621683260073,0.015670740619388,0.653665094914156));
#54185=DIRECTION('',(-0.653745308265284,-6.46149800302507E-11,0.756714656869502));
#54186=DIRECTION('',(-0.13529051141302,1.64268989064603E-13,-0.990805973701009));
#54187=DIRECTION('center_axis',(-0.474237728369273,-0.601098528079538,0.643256664584025));
#54188=DIRECTION('ref_axis',(-0.801782385968023,-0.00691952141559517,-0.59757604183468));
#54189=DIRECTION('',(-0.997345805939891,2.36136671784977E-11,0.0728103246395067));
#54190=DIRECTION('center_axis',(0.,-1.,1.45983193964168E-32));
#54191=DIRECTION('ref_axis',(1.,0.,0.));
#54192=DIRECTION('center_axis',(0.471485217296396,0.601098526249266,-0.645276879805818));
#54193=DIRECTION('ref_axis',(-0.80339664619811,-0.00897212462668922,-0.595376628578341));
#54194=DIRECTION('center_axis',(0.492568909358048,-0.601098528730169,-0.62933014252636));
#54195=DIRECTION('ref_axis',(-0.791119411035074,-0.00794568415793535,-0.611610123842616));
#54196=DIRECTION('center_axis',(-0.495253100626083,0.601098527106587,0.627219998908312));
#54197=DIRECTION('ref_axis',(-0.788499270034972,-0.00794581489403096,-0.614984361736122));
#54198=DIRECTION('center_axis',(0.423002092228966,0.584827952231097,-0.69213112649201));
#54199=DIRECTION('ref_axis',(-0.846224249338951,-0.0181546316873852,-0.532517538846397));
#54200=DIRECTION('center_axis',(-0.553748779401505,-5.17795029430526E-10,
0.832683787107293));
#54201=DIRECTION('ref_axis',(0.83258142444458,-0.0156795066178101,0.553680706492521));
#54202=DIRECTION('',(0.553748839105272,2.06171493653695E-7,-0.832683747403251));
#54203=DIRECTION('center_axis',(0.452675831374959,0.584827782536344,-0.673098103148875));
#54204=DIRECTION('ref_axis',(-0.81832119285553,-0.0273551074146088,-0.574109853095937));
#54205=DIRECTION('center_axis',(0.604940866149408,6.8645898744654E-10,-0.796270399087147));
#54206=DIRECTION('ref_axis',(0.79617222757896,0.0157023279254072,0.604866283512049));
#54207=DIRECTION('',(0.604940785481077,-1.29267396288052E-5,-0.796270460267387));
#54208=DIRECTION('',(-0.197236807274973,-7.62630514901014E-8,-0.98035587510657));
#54209=DIRECTION('center_axis',(-0.553748835937082,-4.67000694238083E-10,
0.832683749510177));
#54210=DIRECTION('ref_axis',(0.642728807477492,-0.635772805082059,0.42742557288568));
#54211=DIRECTION('',(0.990805973701098,0.,-0.135290511412364));
#54212=DIRECTION('center_axis',(0.461432099445187,0.398564391573976,-0.79260762257934));
#54213=DIRECTION('ref_axis',(-0.864216279017837,1.03620976188408E-16,-0.503120485649872));
#54214=DIRECTION('center_axis',(-0.494302415132049,5.74456528004925E-5,
0.869290008624637));
#54215=DIRECTION('ref_axis',(0.869289942541571,-0.000362817023473896,0.494302401531572));
#54216=DIRECTION('',(0.500372285107575,5.9497368376275E-5,-0.865810356115175));
#54217=DIRECTION('center_axis',(0.459295233292948,0.590180063808867,-0.663879040908009));
#54218=DIRECTION('ref_axis',(-0.192989148209777,0.79581959433691,0.573956759645446));
#54219=DIRECTION('center_axis',(-0.480202555684534,0.550037558040659,-0.683274608235013));
#54220=DIRECTION('ref_axis',(-4.07701821964641E-16,0.778964448248472,0.627068089097949));
#54221=DIRECTION('center_axis',(0.848983671137801,-0.477126089978748,-0.22710662782705));
#54222=DIRECTION('ref_axis',(-0.205617355534998,0.0976251537602208,-0.973750908834537));
#54223=DIRECTION('center_axis',(0.752014588807973,0.584827951389544,-0.304056451162418));
#54224=DIRECTION('ref_axis',(-0.392387563238403,0.02654896900435,-0.919416745801725));
#54225=DIRECTION('center_axis',(-0.886402263734747,5.45006096916998E-11,
0.462915788071564));
#54226=DIRECTION('ref_axis',(0.462858384766917,-0.0157477670565849,0.886292346510841));
#54227=DIRECTION('center_axis',(0.909984076723602,-0.000115441199351685,
-0.414643180075138));
#54228=DIRECTION('ref_axis',(0.0104254267660666,0.999690192852031,0.0226015219004144));
#54229=DIRECTION('',(-0.913719870856715,-6.06958927297027E-10,0.406344678323204));
#54230=DIRECTION('center_axis',(-0.728675430621122,-0.601098528034678,0.328196094436946));
#54231=DIRECTION('ref_axis',(-0.429566785864648,0.0279220132424748,-0.902603311349124));
#54232=DIRECTION('',(-0.933426594283892,2.24206636476396E-10,-0.358768439363852));
#54233=DIRECTION('center_axis',(0.,-1.,1.45983193964168E-32));
#54234=DIRECTION('ref_axis',(1.,0.,0.));
#54235=DIRECTION('center_axis',(0.727266639106194,0.601098532901112,-0.331306186762807));
#54236=DIRECTION('ref_axis',(-0.432048143497244,0.0258667428545896,-0.901479513530219));
#54237=DIRECTION('center_axis',(0.685715297905327,-0.601098524686556,-0.410457176619259));
#54238=DIRECTION('ref_axis',(-0.495953505479251,0.0268944496490568,-0.867932491027336));
#54239=DIRECTION('center_axis',(-0.687462619750625,0.601098530023253,0.407523868809536));
#54240=DIRECTION('ref_axis',(-0.492241016448715,0.0268943329637461,-0.870043376263489));
#54241=DIRECTION('center_axis',(0.707976341754609,0.584827952222725,-0.39591131054156));
#54242=DIRECTION('ref_axis',(-0.48602539807284,-0.00326197146067777,-0.873938597368446));
#54243=DIRECTION('center_axis',(-0.855586379305734,-6.81865596053655E-10,
0.517660069492041));
#54244=DIRECTION('ref_axis',(0.517596402876359,-0.0156832196314315,0.85548115137123));
#54245=DIRECTION('',(0.855586424964706,8.32132090979335E-8,-0.517659994027071));
#54246=DIRECTION('center_axis',(0.724511758384335,0.584827969931324,-0.364772473672077));
#54247=DIRECTION('ref_axis',(-0.454213509827986,0.00704480135380958,-0.890865005634202));
#54248=DIRECTION('center_axis',(0.886402299924587,6.50267358417405E-10,
-0.462915718774382));
#54249=DIRECTION('ref_axis',(0.462858869967012,0.0156715280551234,0.886293444464799));
#54250=DIRECTION('',(-0.886402259955359,-1.44328993199847E-11,0.462915795308425));
#54251=DIRECTION('',(0.238950054000536,-3.0781093249293E-8,-0.971031859257532));
#54252=DIRECTION('center_axis',(-0.324956147391805,0.793626260387304,-0.514354800790212));
#54253=DIRECTION('ref_axis',(-1.18555920776032E-18,0.543871187776492,0.839168714327809));
#54254=DIRECTION('center_axis',(0.8627475630211,0.471546674539849,0.1825113043939));
#54255=DIRECTION('ref_axis',(0.0205917296021878,-0.393421568437244,0.919127548363321));
#54256=DIRECTION('center_axis',(-0.681795727685446,-0.601098528036579,0.416935421021206));
#54257=DIRECTION('ref_axis',(-0.520244942803458,-0.00227572300687119,-0.854014063451078));
#54258=DIRECTION('',(-0.954111946853705,5.05127141378909E-12,-0.299450150894991));
#54259=DIRECTION('center_axis',(0.,-1.,1.45983193964168E-32));
#54260=DIRECTION('ref_axis',(1.,0.,0.));
#54261=DIRECTION('center_axis',(0.680008254497479,0.601098527358381,-0.419844416686559));
#54262=DIRECTION('ref_axis',(-0.522569677456327,-0.00432808968609659,-0.852585596783607));
#54263=DIRECTION('center_axis',(0.685715309048858,-0.601098528261091,-0.410457152767959));
#54264=DIRECTION('ref_axis',(-0.515727617683695,-0.0033017877527314,-0.856746241635139));
#54265=DIRECTION('center_axis',(-0.687462624690007,0.601098527784663,0.40752386377909));
#54266=DIRECTION('ref_axis',(-0.512062749502158,-0.00330189269620656,-0.858941696552748));
#54267=DIRECTION('center_axis',(0.652772892221425,0.584827952239017,-0.481522395596295));
#54268=DIRECTION('ref_axis',(-0.573932730512764,-0.0330869090627003,-0.818233754678234));
#54269=DIRECTION('center_axis',(-0.82139394258747,-5.1287838017996E-10,
0.570361281189925));
#54270=DIRECTION('ref_axis',(0.570291204882479,-0.0156751701947647,0.821293023635934));
#54271=DIRECTION('',(0.821393979885559,-8.32667268468003E-13,-0.570361227475854));
#54272=DIRECTION('center_axis',(0.673082062143511,0.584827952226365,-0.452699463126869));
#54273=DIRECTION('ref_axis',(-0.544254348701349,-0.0227607295837561,-0.838611443463828));
#54274=DIRECTION('center_axis',(0.855586476863532,7.80700868016979E-10,
-0.517659908248889));
#54275=DIRECTION('ref_axis',(0.517596159023445,0.0156933905086436,0.855481112391454));
#54276=DIRECTION('',(-0.855586424288594,-2.28705943069067E-11,0.517659995144553));
#54277=DIRECTION('',(0.177506961529544,0.,-0.984119544876815));
#54278=DIRECTION('center_axis',(-0.624163698886024,-0.601098527870402,0.499099425750974));
#54279=DIRECTION('ref_axis',(-0.60492142024746,-0.0324816890410056,-0.795622407428825));
#54280=DIRECTION('',(-0.971031855420269,8.00811321699544E-12,-0.238950069594192));
#54281=DIRECTION('center_axis',(0.,-1.,1.45983193964168E-32));
#54282=DIRECTION('ref_axis',(1.,0.,0.));
#54283=DIRECTION('center_axis',(0.622025719321274,0.601098521249722,-0.501761469479523));
#54284=DIRECTION('ref_axis',(-0.607043037353427,-0.0345385891650894,-0.793918028929442));
#54285=DIRECTION('center_axis',(0.685715312759475,-0.601098530765051,-0.410457142901999));
#54286=DIRECTION('ref_axis',(-0.534775602600504,-0.0335099570183753,-0.844329401148565));
#54287=DIRECTION('center_axis',(-0.687462640971433,0.601098524430712,0.407523841260609));
#54288=DIRECTION('ref_axis',(-0.531163593663202,-0.0335100724645697,-0.846606349970405));
#54289=DIRECTION('',(0.783959868703576,-3.88578058618413E-13,-0.620811504614945));
#54290=DIRECTION('center_axis',(0.611036320517163,0.584827952146974,-0.533489345157354));
#54291=DIRECTION('ref_axis',(-0.627703929108623,-0.0526562728345706,-0.776669230955346));
#54292=DIRECTION('center_axis',(0.821394034568631,7.121806854496E-10,-0.570361148725144));
#54293=DIRECTION('ref_axis',(0.570290194933799,0.0157729998139083,0.821291851925514));
#54294=DIRECTION('',(-0.821393979884609,-1.76914038951462E-10,0.570361227477222));
#54295=DIRECTION('',(0.115363314586777,-1.43735365431646E-13,-0.99332336409024));
#54296=DIRECTION('',(-0.984119544870761,6.51326541667581E-11,-0.177506961563108));
#54297=DIRECTION('center_axis',(0.,-1.,1.45983193964168E-32));
#54298=DIRECTION('ref_axis',(1.,0.,0.));
#54299=DIRECTION('center_axis',(0.675918141245002,0.60109853743272,-0.426397953362991));
#54300=DIRECTION('ref_axis',(-0.565191237695565,0.051484890664322,-0.823351790467136));
#54301=DIRECTION('center_axis',(-0.569959409941816,0.601098535897603,0.560202482287017));
#54302=DIRECTION('ref_axis',(-0.671289958056372,0.0525165049909385,-0.739332001820705));
#54303=DIRECTION('center_axis',(0.648089094031815,0.584827908067798,-0.487808204258665));
#54304=DIRECTION('ref_axis',(-0.613802514678574,0.0219600677380753,-0.789154122082118));
#54305=DIRECTION('center_axis',(-0.743427237289871,-1.89899202024935E-8,
0.668816823095495));
#54306=DIRECTION('ref_axis',(0.668733978372119,-0.0157391387083452,0.743335150307933));
#54307=DIRECTION('',(0.743431826076532,-7.77156117236683E-13,-0.668811722367748));
#54308=DIRECTION('center_axis',(0.668674691879153,0.584827952321432,-0.459184519146543));
#54309=DIRECTION('ref_axis',(-0.584824349033833,0.0322834330501032,-0.810517279721817));
#54310=DIRECTION('center_axis',(0.783959913257619,5.32263755173338E-10,
-0.62081144835216));
#54311=DIRECTION('ref_axis',(0.620734911445354,0.0157020800825522,0.783863262561788));
#54312=DIRECTION('',(-0.783959868704053,-8.32667268469007E-13,0.620811504614342));
#54313=DIRECTION('',(0.0527643813458762,0.,-0.998606989791874));
#54314=DIRECTION('center_axis',(-0.619310106536488,-0.601098527900125,0.50510944526713));
#54315=DIRECTION('ref_axis',(-0.645335333969567,0.0232723748746104,-0.76354482730098));
#54316=DIRECTION('',(-0.993323364090226,0.,-0.115363314586904));
#54317=DIRECTION('center_axis',(0.,-1.,1.45983193964168E-32));
#54318=DIRECTION('ref_axis',(1.,0.,0.));
#54319=DIRECTION('center_axis',(0.617146491191372,0.601098532042902,-0.507750689990714));
#54320=DIRECTION('ref_axis',(-0.647443759929067,0.0212180303810229,-0.761817808216415));
#54321=DIRECTION('center_axis',(0.567560843501483,-0.60109852584814,-0.562632429875027));
#54322=DIRECTION('ref_axis',(-0.691861215403394,0.0222452661870624,-0.721687748789464));
#54323=DIRECTION('center_axis',(-0.569959361942305,0.601098529742556,0.5602025377269));
#54324=DIRECTION('ref_axis',(-0.688771736305674,0.022245163805164,-0.724636907667384));
#54325=DIRECTION('center_axis',(0.581838788174164,0.584827953016256,-0.565190136101858));
#54326=DIRECTION('ref_axis',(-0.692679594745998,-0.00784645566272457,-0.721202753846692));
#54327=DIRECTION('center_axis',(-0.699969556481948,-8.6612246402921E-10,
0.714172682198406));
#54328=DIRECTION('ref_axis',(0.714084906802545,-0.0156778483080594,0.699883526702286));
#54329=DIRECTION('',(0.69996979767401,-3.88578058618449E-13,-0.714172445802976));
#54330=DIRECTION('center_axis',(0.605850912066346,0.584827952254572,-0.539370872971558));
#54331=DIRECTION('ref_axis',(-0.666262485644979,0.00246180455746111,-0.745713242299274));
#54332=DIRECTION('center_axis',(0.743431873636875,5.37764966112024E-10,
-0.668811669501039));
#54333=DIRECTION('ref_axis',(0.668729543705554,0.0156707406195515,0.743340584970171));
#54334=DIRECTION('',(-0.743431826076294,-6.42264019716035E-11,0.668811722368012));
#54335=DIRECTION('',(-0.0100427888024313,1.64268989064697E-13,-0.999949569924939));
#54336=DIRECTION('center_axis',(-0.551119660015009,-0.601098528080819,0.578746645678412));
#54337=DIRECTION('ref_axis',(-0.720563954751441,-0.00691952141674007,-0.693353955304451));
#54338=DIRECTION('',(-0.998606989791231,2.34493981894322E-11,-0.0527643813580464));
#54339=DIRECTION('center_axis',(0.,-1.,1.45983193964168E-32));
#54340=DIRECTION('ref_axis',(1.,0.,0.));
#54341=DIRECTION('center_axis',(0.548642054612441,0.601098526265418,-0.58109591087202));
#54342=DIRECTION('ref_axis',(-0.722441144725833,-0.00897212363898524,-0.691374206493585));
#54343=DIRECTION('center_axis',(0.567560837458516,-0.601098528740018,-0.562632432881339));
#54344=DIRECTION('ref_axis',(-0.708226124218215,-0.00794568359613293,-0.7059409487252));
#54345=DIRECTION('center_axis',(-0.569959387553192,0.601098527165284,0.560202514435375));
#54346=DIRECTION('ref_axis',(-0.705203743225232,-0.00794581057331358,-0.708960185507941));
#54347=DIRECTION('center_axis',(0.506413626493858,0.584827952229861,-0.633657245829295));
#54348=DIRECTION('ref_axis',(-0.772809373322586,-0.018154631707971,-0.634378500465061));
#54349=DIRECTION('center_axis',(-0.653745273667852,-3.58579868904279E-10,
0.756714686759115));
#54350=DIRECTION('ref_axis',(0.756621663054565,-0.0156795066181202,0.653664908090343));
#54351=DIRECTION('',(0.653745310710866,2.06170660986647E-7,-0.756714654756673));
#54352=DIRECTION('center_axis',(0.533467909010792,0.584827782536611,-0.611055197857742));
#54353=DIRECTION('ref_axis',(-0.739913441519287,-0.0273551074141563,-0.672145666621042));
#54354=DIRECTION('center_axis',(0.699969873412294,7.17574584943481E-10,
-0.714172371570882));
#54355=DIRECTION('ref_axis',(0.714084321857467,0.0157023279247992,0.699883574728757));
#54356=DIRECTION('',(0.699969798277374,-1.29267396287503E-5,-0.714172445094622));
#54357=DIRECTION('',(-0.0728103642668903,-7.62630514901185E-8,-0.997345803046926));
#54358=DIRECTION('center_axis',(-0.653745308271402,5.55864689695122E-12,
0.756714656864217));
#54359=DIRECTION('ref_axis',(0.584090069207158,-0.635772805085269,0.504610474888885));
#54360=DIRECTION('',(0.999949569924943,0.,-0.0100427888020118));
#54361=DIRECTION('center_axis',(0.557133645802655,0.39856439157781,-0.728524897639642));
#54362=DIRECTION('ref_axis',(-0.794343958189859,8.99985877814131E-17,-0.607468251094053));
#54363=DIRECTION('center_axis',(-0.599355620645822,5.74456453289826E-5,
0.800482877206165));
#54364=DIRECTION('ref_axis',(0.800482813270424,-0.000363058141650564,0.59935559882882));
#54365=DIRECTION('',(0.604941511770917,5.94973675946086E-5,-0.7962699063737));
#54366=DIRECTION('center_axis',(0.538879660101934,0.590180063808305,-0.601079199616531));
#54367=DIRECTION('ref_axis',(-0.263407883652486,0.795820382742406,0.545239585174673));
#54368=DIRECTION('center_axis',(-0.390778999041342,0.550037558041802,-0.738072122933564));
#54369=DIRECTION('ref_axis',(1.23414151848966E-16,0.801830011437534,0.597552200864563));
#54370=DIRECTION('center_axis',(0.870753189285527,-0.47712609008213,-0.118909955479017));
#54371=DIRECTION('ref_axis',(-0.0819527892227191,0.0976249050665862,-0.9918432931917));
#54372=DIRECTION('center_axis',(0.784193107367589,0.584827951389862,-0.207406455131711));
#54373=DIRECTION('ref_axis',(-0.274059996363077,0.0265489690005161,-0.961346072254149));
#54374=DIRECTION('center_axis',(-0.937431447214792,-3.39662097952973E-11,
0.348169903599926));
#54375=DIRECTION('ref_axis',(0.348126729219042,-0.0157477670578398,0.937315202179045));
#54376=DIRECTION('center_axis',(0.954777148801951,-0.000115441274343246,
-0.297322355027215));
#54377=DIRECTION('ref_axis',(0.00751840455574443,0.999689530367805,0.0237553460495545));
#54378=DIRECTION('',(-0.957443409235868,-6.06958927296624E-10,0.288621063179385));
#54379=DIRECTION('center_axis',(-0.764063486277657,-0.601098527918401,0.234280918283082));
#54380=DIRECTION('ref_axis',(-0.31305332861039,0.027922015765269,-0.949325009931561));
#54381=DIRECTION('',(-0.881100638180729,2.24206636476402E-10,-0.472928816416923));
#54382=DIRECTION('center_axis',(0.,-1.,1.45983193964168E-32));
#54383=DIRECTION('ref_axis',(1.,0.,0.));
#54384=DIRECTION('center_axis',(0.763055601588081,0.601098532777718,-0.237543054576486));
#54385=DIRECTION('ref_axis',(-0.315655968867838,0.0258667456400521,-0.948521070292115));
#54386=DIRECTION('center_axis',(0.731752155373931,-0.601098524847347,-0.32127767823481));
#54387=DIRECTION('ref_axis',(-0.383261974100595,0.0268944461499746,-0.92324804249714));
#54388=DIRECTION('center_axis',(-0.733118057082605,0.601098530103798,0.318148505397211));
#54389=DIRECTION('ref_axis',(-0.379314197018005,0.0268943310871904,-0.924876983655642));
#54390=DIRECTION('center_axis',(0.752014581597193,0.584827952222676,-0.304056467394184));
#54391=DIRECTION('ref_axis',(-0.372659392285939,-0.00326197145339533,-0.92796246523408));
#54392=DIRECTION('center_axis',(-0.913719837201684,-6.49433504233456E-10,
0.406344754000995));
#54393=DIRECTION('ref_axis',(0.406294777972886,-0.0156832196303141,0.91360745947808));
#54394=DIRECTION('',(0.913719871390962,8.3214485854382E-8,-0.40634467712187));
#54395=DIRECTION('center_axis',(0.764516880406742,0.584827969931339,-0.271090732337225));
#54396=DIRECTION('ref_axis',(-0.338976908815281,0.00704480134988046,-0.940768316889965));
#54397=DIRECTION('center_axis',(0.937431473544162,5.74387473960981E-10,
-0.348169832709298));
#54398=DIRECTION('ref_axis',(0.348127075378515,0.0156715280548011,0.937316351397344));
#54399=DIRECTION('',(-0.937431446874083,-1.40443212613657E-11,0.348169904517268));
#54400=DIRECTION('',(0.358768424268607,-3.07809289803191E-8,-0.933426600085845));
#54401=DIRECTION('center_axis',(-0.257928020727969,0.793626260387635,-0.551026764274196));
#54402=DIRECTION('ref_axis',(-2.1533635937977E-16,0.570324175992147,0.821419706531854));
#54403=DIRECTION('center_axis',(0.833069808817712,0.471546674569471,0.289203090126806));
#54404=DIRECTION('ref_axis',(-0.0947771047399993,-0.39340819536142,0.914465577394564));
#54405=DIRECTION('center_axis',(-0.728675431885439,-0.601098528055605,0.328196091591526));
#54406=DIRECTION('ref_axis',(-0.409106307232236,-0.00227571910488544,-0.912483890534709));
#54407=DIRECTION('',(-0.909057433470373,5.21554040285535E-12,-0.416670832495219));
#54408=DIRECTION('center_axis',(0.,-1.,1.45983193964168E-32));
#54409=DIRECTION('ref_axis',(1.,0.,0.));
#54410=DIRECTION('center_axis',(0.727266651289212,0.601098527417744,-0.331306169967894));
#54411=DIRECTION('ref_axis',(-0.411591737982606,-0.00432808000034288,-0.911358057487818));
#54412=DIRECTION('center_axis',(0.731752164393736,-0.601098528240813,-0.321277651341967));
#54413=DIRECTION('ref_axis',(-0.404282168821871,-0.00330179248364486,-0.914628354108421));
#54414=DIRECTION('center_axis',(-0.733118059057979,0.60109852779211,0.318148505212928));
#54415=DIRECTION('ref_axis',(-0.400371043525822,-0.00330189103679421,-0.916347164027709));
#54416=DIRECTION('center_axis',(0.707980627187698,0.58482825598716,-0.395903198428518));
#54417=DIRECTION('ref_axis',(-0.466848718286939,-0.0330815410881358,-0.883718216329773));
#54418=DIRECTION('center_axis',(-0.886386486654161,-1.08201782972538E-7,
0.462945997149647));
#54419=DIRECTION('ref_axis',(0.462889119754394,-0.015675163531169,0.88627758183386));
#54420=DIRECTION('',(0.886402259955066,0.,-0.462915795308987));
#54421=DIRECTION('center_axis',(0.724512896584358,0.584827952226229,-0.364770241354499));
#54422=DIRECTION('ref_axis',(-0.434856856697224,-0.022760729591192,-0.900211899150354));
#54423=DIRECTION('center_axis',(0.913719906847962,6.78823475718525E-10,
-0.406344597392105));
#54424=DIRECTION('ref_axis',(0.406294556518327,0.0156933905092881,0.913607383309646));
#54425=DIRECTION('',(-0.91371987086029,-2.24820162483051E-11,0.406344678315164));
#54426=DIRECTION('',(0.299450150892431,-1.43735365431748E-13,-0.954111946854509));
#54427=DIRECTION('center_axis',(-0.68179572955443,-0.601098528064928,0.416935417924071));
#54428=DIRECTION('ref_axis',(-0.500433501112916,-0.032481685474193,-0.865165447225341));
#54429=DIRECTION('',(-0.933426594324375,8.00811321699499E-12,-0.358768439258525));
#54430=DIRECTION('center_axis',(0.,-1.,1.45983193964168E-32));
#54431=DIRECTION('ref_axis',(1.,0.,0.));
#54432=DIRECTION('center_axis',(0.680008250771264,0.601098521421985,-0.419844431221028));
#54433=DIRECTION('ref_axis',(-0.502752004436133,-0.034538586081331,-0.863740417085453));
#54434=DIRECTION('center_axis',(0.731752165467864,-0.6010985306281,-0.321277644428976));
#54435=DIRECTION('ref_axis',(-0.424736200095745,-0.0335099595817295,-0.904696768501501));
#54436=DIRECTION('center_axis',(-0.733118072971343,0.601098524471746,0.31814847942537));
#54437=DIRECTION('ref_axis',(-0.420867299587536,-0.0335100717230877,-0.906503056382607));
#54438=DIRECTION('',(0.855586424288569,0.,-0.517659995144593));
#54439=DIRECTION('center_axis',(0.673082061319651,0.584827952146743,-0.452699464454661));
#54440=DIRECTION('ref_axis',(-0.525411830020171,-0.0526562728378581,-0.84921712524282));
#54441=DIRECTION('center_axis',(0.886402301749942,6.68497750786553E-10,
-0.462915715279147));
#54442=DIRECTION('ref_axis',(0.46285812786071,0.0157729998138629,0.886292031979387));
#54443=DIRECTION('',(-0.886402259954249,-1.7691403895149E-10,0.46291579531055));
#54444=DIRECTION('',(0.238950069590302,0.,-0.971031855421227));
#54445=DIRECTION('',(-0.954111946844362,6.51326541667565E-11,-0.299450150924759));
#54446=DIRECTION('center_axis',(0.,-1.,1.45983193964168E-32));
#54447=DIRECTION('ref_axis',(1.,0.,0.));
#54448=DIRECTION('center_axis',(0.724030162875529,0.60109853700323,-0.338320664546244));
#54449=DIRECTION('ref_axis',(-0.457541187731248,0.0514848956254042,-0.887696663873375));
#54450=DIRECTION('center_axis',(-0.635677097276993,0.601098535801653,0.484350264018309));
#54451=DIRECTION('ref_axis',(-0.573333766911368,0.052516506081434,-0.817637088388375));
#54452=DIRECTION('center_axis',(0.704117297543295,0.58482790806807,-0.40273458908449));
#54453=DIRECTION('ref_axis',(-0.510055260623721,0.0219600677308701,-0.85986126005032));
#54454=DIRECTION('center_axis',(-0.821390062079794,-1.90520203153216E-8,
0.570366869581809));
#54455=DIRECTION('ref_axis',(0.57029621967304,-0.0157391387082167,0.82128831803415));
#54456=DIRECTION('',(0.821393979885973,3.88578058618525E-13,-0.570361227475258));
#54457=DIRECTION('center_axis',(0.720953072804471,0.584827952320772,-0.371756550713075));
#54458=DIRECTION('ref_axis',(-0.478628082825391,0.0322834330580714,-0.877424035618398));
#54459=DIRECTION('center_axis',(0.855586464117781,5.7300538042428E-10,-0.517659929315022));
#54460=DIRECTION('ref_axis',(0.51759610946881,0.0157020800836657,0.855480982923523));
#54461=DIRECTION('',(-0.855586424289036,-7.77156117237386E-13,0.517659995143822));
#54462=DIRECTION('',(0.177506961529499,0.,-0.984119544876823));
#54463=DIRECTION('center_axis',(-0.677733658023607,-0.60109852804148,0.423506373468341));
#54464=DIRECTION('ref_axis',(-0.544549134192793,0.0232723710871578,-0.838406009755334));
#54465=DIRECTION('',(-0.971031855421207,0.,-0.238950069590381));
#54466=DIRECTION('center_axis',(0.,-1.,1.45983193964168E-32));
#54467=DIRECTION('ref_axis',(1.,0.,0.));
#54468=DIRECTION('center_axis',(0.675918145787789,0.601098531915386,-0.426397953939702));
#54469=DIRECTION('ref_axis',(-0.546857379262444,0.0212180338772051,-0.836956869727824));
#54470=DIRECTION('center_axis',(0.633601998742522,-0.60109852586306,-0.48706166898529));
#54471=DIRECTION('ref_axis',(-0.595954223605553,0.0222452659052586,-0.802710228856906));
#54472=DIRECTION('center_axis',(-0.63567705631572,0.601098529692435,0.484350325359005));
#54473=DIRECTION('ref_axis',(-0.59251948005633,0.022245165155015,-0.805248917031872));
#54474=DIRECTION('center_axis',(0.648087922879121,0.584827953016226,-0.4878097063293));
#54475=DIRECTION('ref_axis',(-0.596826936052606,-0.00784645566273247,-0.80233162815359));
#54476=DIRECTION('center_axis',(-0.783959669330724,-7.36093815513976E-10,
0.620811756382611));
#54477=DIRECTION('ref_axis',(0.620735455512434,-0.0156778483077018,0.783863316747386));
#54478=DIRECTION('',(0.783959868703302,0.,-0.620811504615291));
#54479=DIRECTION('center_axis',(0.668674692288739,0.584827952254013,-0.45918451863596));
#54480=DIRECTION('ref_axis',(-0.567546154946495,0.0024618045803074,-0.823337902397101));
#54481=DIRECTION('center_axis',(0.821394021188847,5.47809383740317E-10,
-0.570361167993768));
#54482=DIRECTION('ref_axis',(0.570291131288506,0.0156707406187205,0.82129315926905));
#54483=DIRECTION('',(-0.821393979885388,-6.42264019716009E-11,0.5703612274761));
#54484=DIRECTION('',(0.115363314586857,1.64268989064744E-13,-0.993323364090231));
#54485=DIRECTION('center_axis',(-0.619310103632507,-0.601098528057576,0.505109448640301));
#54486=DIRECTION('ref_axis',(-0.62798180126612,-0.0069195231192547,-0.778197261289425));
#54487=DIRECTION('',(-0.984119544874669,2.3449398189432E-11,-0.17750696154144));
#54488=DIRECTION('center_axis',(0.,-1.,1.45983193964168E-32));
#54489=DIRECTION('ref_axis',(1.,0.,0.));
#54490=DIRECTION('center_axis',(0.617146484443659,0.601098526356143,-0.507750704924479));
#54491=DIRECTION('ref_axis',(-0.630092308969899,-0.00897211717893297,-0.77646840456667));
#54492=DIRECTION('center_axis',(0.633601991244654,-0.601098528762654,-0.487061675160531));
#54493=DIRECTION('ref_axis',(-0.614163689544919,-0.00794568202695358,-0.789138662455274));
#54494=DIRECTION('center_axis',(-0.635677075874747,0.601098527221414,0.484350302755741));
#54495=DIRECTION('ref_axis',(-0.610786732984478,-0.00794580638708497,-0.791755284776178));
#54496=DIRECTION('center_axis',(0.581838715418155,0.584827952231152,-0.565190211813394));
#54497=DIRECTION('ref_axis',(-0.687206831789029,-0.0181546316769224,-0.726234934226632));
#54498=DIRECTION('center_axis',(-0.74343177523546,-5.95613149885961E-10,
0.668811778881214));
#54499=DIRECTION('ref_axis',(0.668729561174049,-0.015679506618148,0.743340384402849));
#54500=DIRECTION('',(0.743431828237445,2.06171493653824E-7,-0.668811719965707));
#54501=DIRECTION('center_axis',(0.605846879048239,0.584827782536647,-0.539375587064132));
#54502=DIRECTION('ref_axis',(-0.649836813202612,-0.0273551074096476,-0.759581341467311));
#54503=DIRECTION('center_axis',(0.783959932758504,6.94783626924064E-10,
-0.620811423726467));
#54504=DIRECTION('ref_axis',(0.620734884404402,0.0157023279250529,0.78386327901056));
#54505=DIRECTION('',(0.783959869213733,-1.29267396286675E-5,-0.620811503836137));
#54506=DIRECTION('',(0.0527643416803934,-7.62629077547763E-8,-0.998606991887714));
#54507=DIRECTION('center_axis',(-0.743431826069816,-8.3225866364936E-12,
0.668811722375213));
#54508=DIRECTION('ref_axis',(0.516239882061012,-0.63577280508478,0.573837367626284));
#54509=DIRECTION('',(0.993323364090158,0.,0.115363314587482));
#54510=DIRECTION('center_axis',(0.644048861750526,0.398564391578944,-0.652952899865801));
#54511=DIRECTION('ref_axis',(-0.711944358623389,-3.14655782804113E-17,-0.702235879334239));
#54512=DIRECTION('center_axis',(-0.694956629961929,5.74456601172877E-5,
0.719051652645312));
#54513=DIRECTION('ref_axis',(0.719051591920785,-0.000363148938065183,0.694956600284531));
#54514=DIRECTION('',(0.699970449419168,5.94973683762338E-5,-0.71417180454005));
#54515=DIRECTION('center_axis',(0.609965632634555,0.590180063812721,-0.528799980411062));
#54516=DIRECTION('ref_axis',(-0.329667854669152,0.795820454315329,0.507926087232368));
#54517=DIRECTION('center_axis',(-0.295192624143355,0.550037558042699,-0.78122979935086));
#54518=DIRECTION('ref_axis',(1.61303840242307E-17,0.817666865860829,0.575691667885969));
#54519=DIRECTION('center_axis',(0.878790409519382,-0.477126090101351,-0.0088380021133009));
#54520=DIRECTION('ref_axis',(0.0430060492887833,0.097628009236126,-0.994293342800384));
#54521=DIRECTION('center_axis',(0.804004432172478,0.584827951389866,-0.107485535399622));
#54522=DIRECTION('ref_axis',(-0.151410339624816,0.0265489689996098,-0.988114396868984));
#54523=DIRECTION('center_axis',(-0.973676780225177,-1.7969074443091E-11,
0.227933164875875));
#54524=DIRECTION('ref_axis',(0.227904900303916,-0.0157477670572438,0.973556040631546));
#54525=DIRECTION('center_axis',(0.984512820719522,-0.000115441120459348,
-0.175312556630262));
#54526=DIRECTION('ref_axis',(0.00445422974340059,0.999693435572462,0.024355588901113));
#54527=DIRECTION('',(-0.986067493102614,-6.06126260028834E-10,0.166345721454827));
#54528=DIRECTION('center_axis',(-0.787401801638329,-0.601098528045545,0.136671000428739));
#54529=DIRECTION('ref_axis',(-0.191602840052081,0.02792201296917,-0.981075284000023));
#54530=DIRECTION('',(-0.814879198669324,2.24206636476394E-10,-0.579630823521352));
#54531=DIRECTION('center_axis',(0.,-1.,1.45983193964168E-32));
#54532=DIRECTION('ref_axis',(1.,0.,0.));
#54533=DIRECTION('center_axis',(0.786810721571387,0.601098532483053,-0.140033719750047));
#54534=DIRECTION('ref_axis',(-0.194285705633603,0.0258667523495679,-0.980603883180838));
#54535=DIRECTION('center_axis',(0.766248842216283,-0.601098524937294,-0.227031440819144));
#54536=DIRECTION('ref_axis',(-0.264526173897541,0.0268944441817508,-0.964003419182361));
#54537=DIRECTION('center_axis',(-0.767211782381243,0.601098530024342,0.223755755630937));
#54538=DIRECTION('ref_axis',(-0.260405370577914,0.0268943328939305,-0.965124726567696));
#54539=DIRECTION('center_axis',(0.784193102256011,0.584827952222485,-0.207406472110561));
#54540=DIRECTION('ref_axis',(-0.253416325257633,-0.00326197144058285,-0.96735181068484));
#54541=DIRECTION('center_axis',(-0.957443383072194,-7.10515928356689E-10,
0.288621149972196));
#54542=DIRECTION('ref_axis',(0.288585652683465,-0.0156832196316195,0.957325627823284));
#54543=DIRECTION('',(0.957443409615542,8.32140417652626E-8,-0.28862106191988));
#54544=DIRECTION('center_axis',(0.792465114525967,0.584827969931577,-0.173133728213359));
#54545=DIRECTION('ref_axis',(-0.218394439457572,0.0070448013461047,-0.975835149801444));
#54546=DIRECTION('center_axis',(0.973676798398358,6.10870585646325E-10,
-0.227933087244314));
#54547=DIRECTION('ref_axis',(0.227905095698771,0.0156715280541824,0.973557225109537));
#54548=DIRECTION('',(-0.973676779881279,-1.44328993199777E-11,0.227933166344924));
#54549=DIRECTION('',(0.472928802167947,-3.07809289803151E-8,-0.881100645828835));
#54550=DIRECTION('center_axis',(-0.186832215098181,0.793626260387618,-0.579008706518885));
#54551=DIRECTION('ref_axis',(-2.13507208284854E-16,0.589386723415692,0.807851032221483));
#54552=DIRECTION('center_axis',(0.790254046116485,0.471546674563101,0.391333970292646));
#54553=DIRECTION('ref_axis',(-0.208633832128906,-0.393420324212994,0.895372756223546));
#54554=DIRECTION('center_axis',(-0.764063484811556,-0.601098528043994,0.234280922742262));
#54555=DIRECTION('ref_axis',(-0.291515827985554,-0.00227572128403759,-0.956563298023991));
#54556=DIRECTION('',(-0.849666541316623,5.19500677922216E-12,-0.527320366159934));
#54557=DIRECTION('center_axis',(0.,-1.,1.45983193964168E-32));
#54558=DIRECTION('ref_axis',(1.,0.,0.));
#54559=DIRECTION('center_axis',(0.763055610642251,0.601098527425935,-0.237543039034519));
#54560=DIRECTION('ref_axis',(-0.294122760511087,-0.00432807889280782,-0.955757850860999));
#54561=DIRECTION('center_axis',(0.766248848566382,-0.601098528229855,-0.227031410669529));
#54562=DIRECTION('ref_axis',(-0.286460949644773,-0.00330179593875977,-0.958086229142343));
#54563=DIRECTION('center_axis',(-0.767211782659897,0.601098527823099,0.22375576058892));
#54564=DIRECTION('ref_axis',(-0.28236525175776,-0.00330188583807953,-0.959301288516642));
#54565=DIRECTION('center_axis',(0.752014581679907,0.584827952239308,-0.304056467157619));
#54566=DIRECTION('ref_axis',(-0.352415118259546,-0.0330869090552597,-0.935258702643969));
#54567=DIRECTION('center_axis',(-0.937431425362165,-4.83895775299484E-10,
0.348169962437112));
#54568=DIRECTION('ref_axis',(0.348127185228387,-0.0156751701945908,0.937316249696084));
#54569=DIRECTION('',(0.937431446874013,8.32667268468572E-13,-0.348169904517457));
#54570=DIRECTION('center_axis',(0.764517729849789,0.58482795222609,-0.271088374963522));
#54571=DIRECTION('ref_axis',(-0.318601412284451,-0.022760729592207,-0.9476154754323));
#54572=DIRECTION('center_axis',(0.957443431034098,5.76612977251272E-10,
-0.288620990868051));
#54573=DIRECTION('ref_axis',(0.288585447520421,0.0156933905081676,0.957325522992987));
#54574=DIRECTION('',(-0.957443409238604,-2.20934381896848E-11,0.288621063170307));
#54575=DIRECTION('',(0.416670832492647,-1.43735365431753E-13,-0.909057433471552));
#54576=DIRECTION('center_axis',(-0.728675429110272,-0.601098527932451,0.328196097978636));
#54577=DIRECTION('ref_axis',(-0.388053453397706,-0.0324816879404024,-0.921064306796576));
#54578=DIRECTION('',(-0.881100638234071,8.00811321699558E-12,-0.472928816317543));
#54579=DIRECTION('center_axis',(0.,-1.,1.45983193964168E-32));
#54580=DIRECTION('ref_axis',(1.,0.,0.));
#54581=DIRECTION('center_axis',(0.727266646009034,0.601098521703302,-0.331306191926556));
#54582=DIRECTION('ref_axis',(-0.390532269241283,-0.0345385811012187,-0.919941103058652));
#54583=DIRECTION('center_axis',(0.766248846196635,-0.601098530728883,-0.227031412051072));
#54584=DIRECTION('ref_axis',(-0.30799845922305,-0.0335099577670905,-0.950796524944572));
#54585=DIRECTION('center_axis',(-0.767211793970439,0.601098524659991,0.223755730304821));
#54586=DIRECTION('ref_axis',(-0.303933680231947,-0.0335100683557745,-0.952103667328015));
#54587=DIRECTION('',(0.913719870860091,3.88578058618523E-13,-0.406344678315612));
#54588=DIRECTION('center_axis',(0.724512895936988,0.584827952146467,-0.364770242768198));
#54589=DIRECTION('ref_axis',(-0.414833672506597,-0.0526562728409388,-0.908372358168824));
#54590=DIRECTION('center_axis',(0.937431473538846,5.60668931630099E-10,
-0.348169832723611));
#54591=DIRECTION('ref_axis',(0.348126519866068,0.0157729998148864,0.937314855660988));
#54592=DIRECTION('',(-0.937431446873068,-1.76136882834246E-10,0.34816990452));
#54593=DIRECTION('',(0.358768439254553,0.,-0.933426594325902));
#54594=DIRECTION('',(-0.909057433457263,6.5132654166753E-11,-0.416670832523821));
#54595=DIRECTION('center_axis',(0.,-1.,1.45983193964168E-32));
#54596=DIRECTION('ref_axis',(1.,0.,0.));
#54597=DIRECTION('center_axis',(0.760723794998593,0.601098536495491,-0.244907854398175));
#54598=DIRECTION('ref_axis',(-0.342675438066658,0.0514849014682537,-0.938042029477693));
#54599=DIRECTION('center_axis',(-0.691369775202577,0.601098535458906,0.400859557208627));
#54600=DIRECTION('ref_axis',(-0.466335763285318,0.0525165100196524,-0.883047548015653));
#54601=DIRECTION('center_axis',(0.749041150657826,0.584827908068299,-0.311309608855329));
#54602=DIRECTION('ref_axis',(-0.398264130414358,0.0219600677272139,-0.917007872294841));
#54603=DIRECTION('center_axis',(-0.886399045287157,-1.96457150103562E-8,
0.462921950780061));
#54604=DIRECTION('ref_axis',(0.462864609877147,-0.0157391387108218,0.886289248742146));
#54605=DIRECTION('',(0.886402259955037,0.,-0.462915795309042));
#54606=DIRECTION('center_axis',(0.761861593086633,0.584827952320782,-0.278465759409983));
#54607=DIRECTION('ref_axis',(-0.364883565842199,0.0322834330579322,-0.930493290318783));
#54608=DIRECTION('center_axis',(0.913719904256589,6.14490181019606E-10,
-0.406344603219152));
#54609=DIRECTION('ref_axis',(0.406294506910647,0.0157020800829072,0.913607256065375));
#54610=DIRECTION('',(-0.91371987086035,-3.88578058618498E-13,0.406344678315031));
#54611=DIRECTION('',(0.299450150892393,0.,-0.95411194685452));
#54612=DIRECTION('center_axis',(-0.725468945452924,-0.601098528222859,0.335224355546754));
#54613=DIRECTION('ref_axis',(-0.435175071162971,0.0232723662834079,-0.90004502909903));
#54614=DIRECTION('',(-0.933426594325924,1.43735365432682E-13,-0.358768439254497));
#54615=DIRECTION('center_axis',(0.,-1.,1.45983193964168E-32));
#54616=DIRECTION('ref_axis',(1.,0.,0.));
#54617=DIRECTION('center_axis',(0.724030164751593,0.601098531862174,-0.338320669665511));
#54618=DIRECTION('ref_axis',(-0.43764673286923,0.0212180353560184,-0.898896619297525));
#54619=DIRECTION('center_axis',(0.689650872581711,-0.601098525907596,-0.403809653300909));
#54620=DIRECTION('ref_axis',(-0.490648676648319,0.0222452647620465,-0.871073489608609));
#54621=DIRECTION('center_axis',(-0.691369747346035,0.601098529780441,0.400859613768302));
#54622=DIRECTION('ref_axis',(-0.486922833503873,0.0222451626493677,-0.873161672859765));
#54623=DIRECTION('center_axis',(0.704116346373504,0.584827953375381,-0.402736186256451));
#54624=DIRECTION('ref_axis',(-0.491561927845562,-0.00784642891601187,-0.870807271815079));
#54625=DIRECTION('center_axis',(-0.85558611995522,-2.03617710913708E-9,
0.517660498145235));
#54626=DIRECTION('ref_axis',(0.517596875100651,-0.0156778482803438,0.855480964112785));
#54627=DIRECTION('',(0.855586424288614,3.88578058618633E-13,-0.51765999514452));
#54628=DIRECTION('center_axis',(0.720953073132771,0.584827952254103,-0.37175655018128));
#54629=DIRECTION('ref_axis',(-0.459879282384634,0.00246180457136728,-0.887978031908248));
#54630=DIRECTION('center_axis',(0.886402295876551,5.88964994383866E-10,
-0.462915726525661));
#54631=DIRECTION('ref_axis',(0.462858883431285,0.0156707406183786,0.886293451356387));
#54632=DIRECTION('',(-0.886402259954842,-6.37823127617598E-11,0.462915795309415));
#54633=DIRECTION('',(0.23895006959035,1.64268989064786E-13,-0.971031855421215));
#54634=DIRECTION('center_axis',(-0.677733660142661,-0.601098528074642,0.42350637003017));
#54635=DIRECTION('ref_axis',(-0.525495996600591,-0.00691952178971143,-0.850767934148292));
#54636=DIRECTION('',(-0.954111946850841,2.34493981894321E-11,-0.299450150904116));
#54637=DIRECTION('center_axis',(0.,-1.,1.45983193964168E-32));
#54638=DIRECTION('ref_axis',(1.,0.,0.));
#54639=DIRECTION('center_axis',(0.675918144140183,0.601098526458222,-0.426397964244489));
#54640=DIRECTION('ref_axis',(-0.52780653885738,-0.00897210993944167,-0.849317230946498));
#54641=DIRECTION('center_axis',(0.689650870426024,-0.601098528684547,-0.403809652848841));
#54642=DIRECTION('ref_axis',(-0.510415517766898,-0.00794568844090066,-0.859891193848355));
#54643=DIRECTION('center_axis',(-0.691369757445448,0.601098527295095,0.400859600076498));
#54644=DIRECTION('ref_axis',(-0.506737253187209,-0.00794580112719611,-0.862063930620421));
#54645=DIRECTION('center_axis',(0.648087860131304,0.584827952228637,-0.487809790638203));
#54646=DIRECTION('ref_axis',(-0.590766628087855,-0.0181546317314174,-0.806638209164681));
#54647=DIRECTION('center_axis',(-0.821393943279879,-5.02776464207159E-10,
0.570361280192766));
#54648=DIRECTION('ref_axis',(0.570291165105354,-0.015679506617579,0.821292968480193));
#54649=DIRECTION('',(0.821393981728486,2.06171105075815E-7,-0.570361224821762));
#54650=DIRECTION('center_axis',(0.66867128189068,0.584827782537022,-0.45918970104686));
#54651=DIRECTION('ref_axis',(-0.549511870141489,-0.0273551074001155,-0.835037964809224));
#54652=DIRECTION('center_axis',(0.855586473862625,6.3690949927931E-10,-0.517659913208778));
#54653=DIRECTION('ref_axis',(0.517596091348888,0.0157023279254066,0.855480989337622));
#54654=DIRECTION('',(0.855586424697114,-1.2926739628574E-5,-0.517659994307953));
#54655=DIRECTION('',(0.1775069224395,-7.62629077547996E-8,-0.984119551927535));
#54656=DIRECTION('center_axis',(-0.821393979889483,4.55998777965875E-12,
0.570361227470202));
#54657=DIRECTION('ref_axis',(0.440248283555354,-0.635772805085312,0.634014502310885));
#54658=DIRECTION('',(0.971031855420999,0.,0.238950069591228));
#54659=DIRECTION('center_axis',(0.720807042410979,0.39856439158468,-0.567083444804617));
#54660=DIRECTION('ref_axis',(-0.618316971226317,2.54116158780968E-16,-0.785928828262149));
#54661=DIRECTION('center_axis',(-0.779597758073224,5.74456515223888E-5,
0.626280553990941));
#54662=DIRECTION('ref_axis',(0.626280497544892,-0.00036285465843142,0.77959772109173));
#54663=DIRECTION('',(0.783960434937778,5.94973676301789E-5,-0.620810786723486));
#54664=DIRECTION('center_axis',(0.6714320830097,0.590180063806611,-0.448181269343644));
#54665=DIRECTION('ref_axis',(-0.390731048633041,0.795821036217624,0.462599314685649));
#54666=DIRECTION('center_axis',(-0.194950885223199,0.550037558043462,-0.812067015148551));
#54667=DIRECTION('ref_axis',(1.05327946492612E-16,0.827952943471004,0.560797577917114));
#54668=DIRECTION('center_axis',(0.872968580073513,-0.477126090041954,0.101373331827024));
#54669=DIRECTION('ref_axis',(0.16728754861143,0.097632994085021,-0.981062013608504));
#54670=DIRECTION('center_axis',(0.811136126793024,0.584827951390207,-0.0058695045741029));
#54671=DIRECTION('ref_axis',(-0.026372851389724,0.0265489689940623,-0.999299567174392));
#54672=DIRECTION('center_axis',(-0.994566648465754,-2.99637009883098E-11,
0.104101785573529));
#54673=DIRECTION('ref_axis',(0.104088876559904,-0.0157477670567439,0.994443318449686));
#54674=DIRECTION('center_axis',(0.998722132125226,-0.000115441216901894,
-0.0505380003222111));
#54675=DIRECTION('ref_axis',(0.00137352177937294,0.999690005520608,0.0248597325031408));
#54676=DIRECTION('',(-0.999140703554944,-6.06958927296906E-10,0.0414470083327064));
#54677=DIRECTION('center_axis',(-0.798322321672281,-0.60109852804191,0.0369056947587686));
#54678=DIRECTION('ref_axis',(-0.067130656640417,0.0279220130298706,-0.997353415859888));
#54679=DIRECTION('',(-0.735806627409701,2.24062901110931E-10,-0.677191706284094));
#54680=DIRECTION('center_axis',(0.,-1.,1.45983193964168E-32));
#54681=DIRECTION('ref_axis',(1.,0.,0.));
#54682=DIRECTION('center_axis',(0.798157363031323,0.601098532444239,-0.0403159786222247));
#54683=DIRECTION('ref_axis',(-0.0698514481007516,0.0258667532426018,-0.997221984452266));
#54684=DIRECTION('center_axis',(0.78866132617452,-0.601098525006615,-0.129204782541199));
#54685=DIRECTION('ref_axis',(-0.14161863837021,0.0268944426871824,-0.989555885343882));
#54686=DIRECTION('center_axis',(-0.789206120912546,0.601098530062168,0.125834239661842));
#54687=DIRECTION('ref_axis',(-0.137389792491866,0.0268943319889687,-0.990151877151131));
#54688=DIRECTION('center_axis',(0.804004429227664,0.584827952222659,-0.107485552895957));
#54689=DIRECTION('ref_axis',(-0.130176731423392,-0.00326197144762294,-0.991485440204846));
#54690=DIRECTION('center_axis',(-0.986067481533857,-5.45168758924053E-10,
0.166345790032317));
#54691=DIRECTION('ref_axis',(0.16632533129643,-0.0156832196306599,0.985946205830292));
#54692=DIRECTION('',(0.986067493321353,8.32139862540711E-8,-0.166345720158157));
#54693=DIRECTION('center_axis',(0.807915700397312,0.584827969931308,-0.0724463017520282));
#54694=DIRECTION('ref_axis',(-0.0943677593111905,0.00704480135220278,-0.995512479467984));
#54695=DIRECTION('center_axis',(0.994566654888419,4.60698908371065E-10,
-0.104101724212714));
#54696=DIRECTION('ref_axis',(0.104088939895806,0.0156715280552417,0.994444516199763));
#54697=DIRECTION('',(-0.99456664842325,-1.40443212613684E-11,0.104101785979601));
#54698=DIRECTION('',(0.579630810343267,-3.07809289803229E-8,-0.814879208043012));
#54699=DIRECTION('center_axis',(-0.112789953828636,0.793626260387895,-0.597859335578244));
#54700=DIRECTION('ref_axis',(-7.60995088010986E-17,0.601698864092707,0.798723028934026));
#54701=DIRECTION('center_axis',(0.734975505022815,0.471546674564434,0.487293279990277));
#54702=DIRECTION('ref_axis',(-0.319217348238282,-0.393408855917977,0.86216573619521));
#54703=DIRECTION('center_axis',(-0.787401802043575,-0.601098528049665,0.13667099807588));
#54704=DIRECTION('ref_axis',(-0.169327965428505,-0.00227571981498317,-0.985557132399318));
#54705=DIRECTION('',(-0.776875900240117,5.05127141378907E-12,-0.629653742644406));
#54706=DIRECTION('center_axis',(0.,-1.,1.45983193964168E-32));
#54707=DIRECTION('ref_axis',(1.,0.,0.));
#54708=DIRECTION('center_axis',(0.786810727775904,0.601098527454823,-0.140033706472389));
#54709=DIRECTION('ref_axis',(-0.172015286604093,-0.00432807421381841,-0.985084772467888));
#54710=DIRECTION('center_axis',(0.788661328976348,-0.601098528218721,-0.129204750495282));
#54711=DIRECTION('ref_axis',(-0.164122071343041,-0.00330179825181832,-0.986434510662707));
#54712=DIRECTION('center_axis',(-0.789206121376638,0.601098527829134,0.125834247418145));
#54713=DIRECTION('ref_axis',(-0.159906386064952,-0.00330188499779538,-0.987126661199619));
#54714=DIRECTION('center_axis',(0.784195235648826,0.584828255987593,-0.207397549127737));
#54715=DIRECTION('ref_axis',(-0.232410023808953,-0.033081541078036,-0.972055138597098));
#54716=DIRECTION('center_axis',(-0.973669012885895,-1.08205910182348E-7,
0.227966342572307));
#54717=DIRECTION('ref_axis',(0.227938335612477,-0.015675163532481,0.973549384677759));
#54718=DIRECTION('',(0.973676779881262,3.88578058618882E-13,-0.227933166344996));
#54719=DIRECTION('center_axis',(0.792465661815022,0.584827952226149,-0.173131282959057));
#54720=DIRECTION('ref_axis',(-0.197321433276741,-0.0227607295932086,-0.980074589588975));
#54721=DIRECTION('center_axis',(0.986067506826153,6.31299538322982E-10,
-0.166345640104134));
#54722=DIRECTION('ref_axis',(0.16632515482247,0.0156933905090719,0.98594607376246));
#54723=DIRECTION('',(-0.98606749310408,-2.28705943069118E-11,0.166345721446137));
#54724=DIRECTION('',(0.527320366157672,0.,-0.849666541318027));
#54725=DIRECTION('center_axis',(-0.764063484700029,-0.601098528029406,0.234280923143411));
#54726=DIRECTION('ref_axis',(-0.269553565881082,-0.0324816861699376,-0.962437434425922));
#54727=DIRECTION('',(-0.814879198734831,8.1518485824293E-12,-0.579630823429258));
#54728=DIRECTION('center_axis',(0.,-1.,1.45983193964168E-32));
#54729=DIRECTION('ref_axis',(1.,0.,0.));
#54730=DIRECTION('center_axis',(0.763055608651005,0.601098521833866,-0.237543059581597));
#54731=DIRECTION('ref_axis',(-0.272153609616772,-0.0345385788119736,-0.96163376570616));
#54732=DIRECTION('center_axis',(0.788661328100161,-0.601098530387989,-0.129204745751426));
#54733=DIRECTION('ref_axis',(-0.186403388257063,-0.0335099640094169,-0.981901654524716));
#54734=DIRECTION('center_axis',(-0.789206129626374,0.601098524547363,0.125834211354237));
#54735=DIRECTION('ref_axis',(-0.18220683847475,-0.0335100703121061,-0.982689036878256));
#54736=DIRECTION('',(0.957443409238448,3.88578058618626E-13,-0.288621063170825));
#54737=DIRECTION('center_axis',(0.764517729385345,0.584827952146375,-0.271088376445309));
#54738=DIRECTION('ref_axis',(-0.297713340163934,-0.0526562728410443,-0.953202016373719));
#54739=DIRECTION('center_axis',(0.973676797912358,5.80360093127206E-10,
-0.227933089320392));
#54740=DIRECTION('ref_axis',(0.227904734093392,0.0157729998154154,0.973555671060799));
#54741=DIRECTION('',(-0.973676779880651,-1.76914038951436E-10,0.227933166347607));
#54742=DIRECTION('',(0.472928816313919,0.,-0.881100638236016));
#54743=DIRECTION('',(-0.84966654129999,6.52763895321867E-11,-0.527320366186736));
#54744=DIRECTION('center_axis',(0.,-1.,1.45983193964168E-32));
#54745=DIRECTION('ref_axis',(1.,0.,0.));
#54746=DIRECTION('center_axis',(0.785420354371214,0.601098536404089,-0.147632708002865));
#54747=DIRECTION('ref_axis',(-0.222405497715741,0.0514849025470141,-0.973593908873478));
#54748=DIRECTION('center_axis',(-0.736159142124515,0.601098535395105,0.311047051444564));
#54749=DIRECTION('ref_axis',(-0.351983362770681,0.0525165107314909,-0.934531823124945));
#54750=DIRECTION('center_axis',(0.782151897001614,0.584827930050724,-0.21497605040879));
#54751=DIRECTION('ref_axis',(-0.280192919620054,0.0219594825788432,-0.959692507483339));
#54752=DIRECTION('center_axis',(-0.937430242585242,-9.64037678221773E-9,
0.348173146992377));
#54753=DIRECTION('ref_axis',(0.348130019649239,-0.0157391393477757,0.937314124993117));
#54754=DIRECTION('',(0.937431446873851,3.88578058618657E-13,-0.348169904517893));
#54755=DIRECTION('center_axis',(0.790755100932567,0.584827952320671,-0.180783396730828));
#54756=DIRECTION('ref_axis',(-0.245384617052312,0.0322834330591902,-0.968888109981748));
#54757=DIRECTION('center_axis',(0.957443430073302,5.35836324334506E-10,
-0.2886209940553));
#54758=DIRECTION('ref_axis',(0.288585411333215,0.0157020800824498,0.957325391414394));
#54759=DIRECTION('',(-0.957443409238708,-8.32667268468881E-13,0.288621063169962));
#54760=DIRECTION('',(0.416670832492843,0.,-0.909057433471462));
#54761=DIRECTION('center_axis',(-0.761763160213927,-0.601098528106845,0.2416556377341));
#54762=DIRECTION('ref_axis',(-0.318938027994497,0.0232723693707062,-0.947489805287031));
#54763=DIRECTION('',(-0.881100638235951,1.43735365432651E-13,-0.472928816314041));
#54764=DIRECTION('center_axis',(0.,-1.,1.45983193964168E-32));
#54765=DIRECTION('ref_axis',(1.,0.,0.));
#54766=DIRECTION('center_axis',(0.760723795872547,0.601098531745845,-0.244907863340997));
#54767=DIRECTION('ref_axis',(-0.321534133665856,0.0212180385557474,-0.946660232463366));
#54768=DIRECTION('center_axis',(0.734823540351965,-0.601098525986883,-0.314189316497238));
#54769=DIRECTION('ref_axis',(-0.377605305630028,0.0222452626969263,-0.925699401235411));
#54770=DIRECTION('center_axis',(-0.736159118843831,0.601098529596128,0.311047117749781));
#54771=DIRECTION('ref_axis',(-0.373647131821486,0.0222451677062268,-0.927304142876165));
#54772=DIRECTION('center_axis',(0.749040407179186,0.584827953375494,-0.311311312617244));
#54773=DIRECTION('ref_axis',(-0.378544724015712,-0.00784642890189125,-0.925549742300951));
#54774=DIRECTION('center_axis',(-0.913719631733798,-2.04042747348083E-9,
0.406345216022352));
#54775=DIRECTION('ref_axis',(0.406295274186236,-0.0156778482801616,0.913607330994687));
#54776=DIRECTION('',(0.91371987086025,3.88578058618712E-13,-0.406344678315255));
#54777=DIRECTION('center_axis',(0.761861593344965,0.584827952254111,-0.278465758843226));
#54778=DIRECTION('ref_axis',(-0.344959838812461,0.0024618045699357,-0.938614217410295));
#54779=DIRECTION('center_axis',(0.937431472565835,5.58909274130683E-10,
-0.3481698353434));
#54780=DIRECTION('ref_axis',(0.348127082309473,0.0156707406182684,0.937316361988399));
#54781=DIRECTION('',(-0.937431446873651,-6.41708908203805E-11,0.348169904518431));
#54782=DIRECTION('',(0.358768439254525,1.642689890648E-13,-0.933426594325913));
#54783=DIRECTION('center_axis',(-0.725468949669201,-0.601098528058629,0.335224346716666));
#54784=DIRECTION('ref_axis',(-0.414722809127897,-0.00691952313171273,-0.909921486606782));
#54785=DIRECTION('',(-0.909057433466375,2.34493981894292E-11,-0.416670832503941));
#54786=DIRECTION('center_axis',(0.,-1.,1.45983193964168E-32));
#54787=DIRECTION('ref_axis',(1.,0.,0.));
#54788=DIRECTION('center_axis',(0.724030164855667,0.601098526489808,-0.338320678987934));
#54789=DIRECTION('ref_axis',(-0.417196949127517,-0.008972107745217,-0.908771812349668));
#54790=DIRECTION('center_axis',(0.734823539271242,-0.60109852864006,-0.314189313948835));
#54791=DIRECTION('ref_axis',(-0.398617790674048,-0.0079456920901308,-0.917082724150526));
#54792=DIRECTION('center_axis',(-0.736159130438184,0.601098527290318,0.311047094765258));
#54793=DIRECTION('ref_axis',(-0.394696218349555,-0.00794580135155318,-0.918777317668129));
#54794=DIRECTION('center_axis',(0.704116272234799,0.584827952230113,-0.40273631753854));
#54795=DIRECTION('ref_axis',(-0.485009681656924,-0.0181546316947643,-0.874320317759502));
#54796=DIRECTION('center_axis',(-0.886402227433596,-5.50280066249969E-10,
0.462915857581872));
#54797=DIRECTION('ref_axis',(0.462858950871009,-0.0156795066187817,0.886293261099722));
#54798=DIRECTION('',(0.886402261451109,2.06171493653986E-7,-0.462915792444281));
#54799=DIRECTION('center_axis',(0.720950339158042,0.584827782536829,-0.371762119158151));
#54800=DIRECTION('ref_axis',(-0.440520796642366,-0.0273551074055604,-0.89732554060631));
#54801=DIRECTION('center_axis',(0.91371990856544,6.13568318143281E-10,-0.406344593530127));
#54802=DIRECTION('ref_axis',(0.406294495641273,0.0157023279256281,0.913607256817348));
#54803=DIRECTION('',(0.91371987116043,-1.29267404456195E-5,-0.406344677434645));
#54804=DIRECTION('',(0.299450112994266,-7.62629077548155E-8,-0.954111958748928));
#54805=DIRECTION('center_axis',(-0.886402259959937,8.07131938721877E-12,
0.462915795299659));
#54806=DIRECTION('ref_axis',(0.357313706637834,-0.635772805085138,0.684192849540908));
#54807=DIRECTION('',(0.933426594325498,0.,0.358768439255605));
#54808=DIRECTION('center_axis',(0.78619766542402,0.398564391587654,-0.472270745060694));
#54809=DIRECTION('ref_axis',(-0.514938355828296,-1.84676138194459E-16,-0.857227210077265));
#54810=DIRECTION('center_axis',(-0.85194416385074,5.74456496553722E-5,0.523632636855898));
#54811=DIRECTION('ref_axis',(0.523632585551374,-0.000362597540125659,0.851944120158011));
#54812=DIRECTION('',(0.855586896082549,5.94973692289276E-5,-0.517659211945361));
#54813=DIRECTION('center_axis',(0.722309648105342,0.590180063812333,-0.360494472263318));
#54814=DIRECTION('ref_axis',(-0.445629721318181,0.795821199110888,0.409978987904977));
#54815=DIRECTION('center_axis',(-0.0916346543850253,0.5500375580439,-0.830097449012368));
#54816=DIRECTION('ref_axis',(-4.21286816843194E-17,0.833604678689015,0.552361511754561));
#54817=DIRECTION('center_axis',(0.853379514663138,-0.477126089924881,0.209985947782943));
#54818=DIRECTION('ref_axis',(0.288924638246151,0.0976260041170478,-0.952361127269729));
#54819=DIRECTION('center_axis',(0.805475720145869,0.584827951390078,0.0958390918591059));
#54820=DIRECTION('ref_axis',(0.0990805524777462,0.0265489689969947,-0.994725186353448));
#54821=DIRECTION('center_axis',(-0.999771606733593,7.98851526112104E-15,
-0.0213713445840403));
#54822=DIRECTION('ref_axis',(-0.0213686944566971,-0.015747767056506,0.999647631283119));
#54823=DIRECTION('center_axis',(0.997181000919987,-0.000115441232581829,
0.0750335796662666));
#54824=DIRECTION('ref_axis',(0.001753101083015,-0.99968999170467,-0.0248364071900295));
#54825=DIRECTION('',(-0.996456868254473,-6.06514838087359E-10,-0.0841053488696623));
#54826=DIRECTION('center_axis',(-0.79665282157886,-0.601098527948266,-0.0634416390777339));
#54827=DIRECTION('ref_axis',(0.0584002199716004,0.0279220150878775,-0.997902688332234));
#54828=DIRECTION('',(-0.645129946086362,2.24206636476389E-10,-0.764072871303914));
#54829=DIRECTION('center_axis',(0.,-1.,1.45983193964168E-32));
#54830=DIRECTION('ref_axis',(1.,0.,0.));
#54831=DIRECTION('center_axis',(0.79691658507517,0.601098532103177,0.0600375810266817));
#54832=DIRECTION('ref_axis',(0.0556844176437354,0.0258667610074719,-0.998113298331738));
#54833=DIRECTION('center_axis',(0.798636149364674,-0.601098525218913,-0.0293404824025407));
#54834=DIRECTION('ref_axis',(-0.0164776880985398,0.0268944380938454,-0.9995024637261));
#54835=DIRECTION('center_axis',(-0.798754206951309,0.601098529797617,0.0259282539467715));
#54836=DIRECTION('ref_axis',(-0.0122075043862703,0.0268943379739908,-0.999563740549646));
#54837=DIRECTION('center_axis',(0.811136126064599,0.584827952222597,-0.00586952230073281));
#54838=DIRECTION('ref_axis',(-0.00488417276898191,-0.00326197145228212,
-0.999982752050558));
#54839=DIRECTION('center_axis',(-0.999140700839568,-5.13744792983439E-10,
0.0414470737907721));
#54840=DIRECTION('ref_axis',(0.0414419762542119,-0.0156832196311383,0.999017817271618));
#54841=DIRECTION('',(0.999140703609452,8.32140417652197E-8,-0.0414470070186271));
#54842=DIRECTION('center_axis',(0.810624973045492,0.584827969931702,0.0293836461413375));
#54843=DIRECTION('ref_axis',(0.0311471567522389,0.00704480134473847,-0.999489982641279));
#54844=DIRECTION('center_axis',(0.999771605383917,4.91098306320819E-10,
0.0213714077230609));
#54845=DIRECTION('ref_axis',(-0.0213687831950173,0.0156715280538888,0.999648827495546));
#54846=DIRECTION('',(-0.99977160679441,-1.44884104712086E-11,-0.0213713417389639));
#54847=DIRECTION('',(0.677191694384778,-3.07809289803371E-8,-0.735806638361106));
#54848=DIRECTION('center_axis',(-0.0369689276092246,0.793626260387842,-0.60728136577227));
#54849=DIRECTION('ref_axis',(-6.40118045451157E-18,0.607696777838784,0.794169142062546));
#54850=DIRECTION('center_axis',(0.668105961119928,0.471546674587854,0.575567683596947));
#54851=DIRECTION('ref_axis',(-0.424747386385162,-0.393422882089557,0.815357647665931));
#54852=DIRECTION('center_axis',(-0.79832232140634,-0.601098528027703,0.0369057007428594));
#54853=DIRECTION('ref_axis',(-0.0444697081985339,-0.00227572478171658,-0.999008141172761));
#54854=DIRECTION('',(-0.691833462133681,5.19500677922273E-12,-0.722057103470442));
#54855=DIRECTION('center_axis',(0.,-1.,1.45983193964168E-32));
#54856=DIRECTION('ref_axis',(1.,0.,0.));
#54857=DIRECTION('center_axis',(0.79815736744895,0.601098527458077,-0.0403159655061622));
#54858=DIRECTION('ref_axis',(-0.0471950343009395,-0.00432807382640624,-0.998876316925317));
#54859=DIRECTION('center_axis',(0.798636148022719,-0.601098528218913,-0.0293404574690105));
#54860=DIRECTION('ref_axis',(-0.0391948925249827,-0.00330179850900792,-0.999226129825757));
#54861=DIRECTION('center_axis',(-0.798754208373615,0.601098527841249,0.025928255485519));
#54862=DIRECTION('ref_axis',(-0.0349257031272392,-0.00330188269111536,-0.99938445696927));
#54863=DIRECTION('center_axis',(0.804005427453076,0.584828255987368,-0.107476432880749));
#54864=DIRECTION('ref_axis',(-0.1087465876337,-0.03308154108069,-0.993518893286762));
#54865=DIRECTION('center_axis',(-0.994563102620099,-1.08065969665897E-7,
0.104135656269459));
#54866=DIRECTION('ref_axis',(0.104122863543029,-0.0156751635318716,0.994440907513286));
#54867=DIRECTION('',(0.994566648423216,0.,-0.10410178597993));
#54868=DIRECTION('center_axis',(0.807915936897985,0.584827952226251,-0.0724438071963501));
#54869=DIRECTION('ref_axis',(-0.0729295773905037,-0.0227607295923756,-0.997077342000141));
#54870=DIRECTION('center_axis',(0.999140706524478,5.45925022813738E-10,
-0.0414469367476885));
#54871=DIRECTION('ref_axis',(0.0414418325971275,0.0156933905076496,0.999017663510193));
#54872=DIRECTION('',(-0.99914070355531,-2.24820162482996E-11,0.0414470083238722));
#54873=DIRECTION('',(0.629653742642299,0.,-0.776875900241824));
#54874=DIRECTION('center_axis',(-0.787401800997156,-0.601098527900108,0.136671004762377));
#54875=DIRECTION('ref_axis',(-0.146802662815299,-0.0324816885186914,-0.988632347286549));
#54876=DIRECTION('',(-0.735806627485984,8.17238220606064E-12,-0.677191706201208));
#54877=DIRECTION('center_axis',(0.,-1.,1.45983193964168E-32));
#54878=DIRECTION('ref_axis',(1.,0.,0.));
#54879=DIRECTION('center_axis',(0.786810728237449,0.601098522108102,-0.140033726830044));
#54880=DIRECTION('ref_axis',(-0.14948292141722,-0.0345385739796511,-0.988160889284749));
#54881=DIRECTION('center_axis',(0.798636146090112,-0.601098530631398,-0.0293404606492082));
#54882=DIRECTION('ref_axis',(-0.0618686383501138,-0.0335099595911008,-0.997521605879745));
#54883=DIRECTION('center_axis',(-0.798754211564724,0.601098524902521,0.0259282253081593));
#54884=DIRECTION('ref_axis',(-0.0576064969356273,-0.0335100640083441,-0.997776812278659));
#54885=DIRECTION('',(0.986067493104221,0.,-0.166345721445301));
#54886=DIRECTION('center_axis',(0.792465661535211,0.584827952145566,-0.173131284512027));
#54887=DIRECTION('ref_axis',(-0.175897890623464,-0.0526562728562727,-0.982999109360279));
#54888=DIRECTION('center_axis',(0.994566658297495,7.04166480481068E-10,
-0.10410169164309));
#54889=DIRECTION('ref_axis',(0.104088741225509,0.015772999814322,0.994442932715069));
#54890=DIRECTION('',(-0.994566648422976,-1.76969550102655E-10,0.104101785982223));
#54891=DIRECTION('',(0.579630823425986,0.,-0.814879198737159));
#54892=DIRECTION('',(-0.776875900220307,6.49889188013141E-11,-0.629653742668848));
#54893=DIRECTION('center_axis',(0.,-1.,1.45983193964168E-32));
#54894=DIRECTION('ref_axis',(1.,0.,0.));
#54895=DIRECTION('center_axis',(0.797730365318786,0.601098536214713,-0.0480293036477394));
#54896=DIRECTION('ref_axis',(-0.0986280882349215,0.0514849047391242,-0.993791630471463));
#54897=DIRECTION('center_axis',(-0.769338840674988,0.601098535510728,0.216329144674784));
#54898=DIRECTION('ref_axis',(-0.232079971852678,0.0525165093863018,-0.971277974066507));
#54899=DIRECTION('center_axis',(0.802928089510673,0.58482792304435,-0.115250958791558));
#54900=DIRECTION('ref_axis',(-0.157701893482256,0.0219596690837393,-0.987242566812151));
#54901=DIRECTION('center_axis',(-0.973675747383018,-1.25141579433899E-8,
0.227937576889204));
#54902=DIRECTION('ref_axis',(0.227909342926954,-0.0157391391449199,0.973555140146454));
#54903=DIRECTION('',(0.973676779881215,0.,-0.227933166345199));
#54904=DIRECTION('center_axis',(0.807177928460976,0.584827952320853,-0.0802499718981004));
#54905=DIRECTION('ref_axis',(-0.122015806272558,0.0322834330565352,-0.992002985363321));
#54906=DIRECTION('center_axis',(0.986067504831869,5.22694560534451E-10,
-0.1663456519259));
#54907=DIRECTION('ref_axis',(0.166325143951013,0.015702080081768,0.985945937245436));
#54908=DIRECTION('',(-0.986067493104268,-8.32667268468834E-13,0.16634572144502));
#54909=DIRECTION('',(0.527320366157604,0.,-0.849666541318069));
#54910=DIRECTION('center_axis',(-0.786043912893678,-0.601098528080546,0.144275869576991));
#54911=DIRECTION('ref_axis',(-0.197671144361105,0.0232723701079249,-0.97999209970108));
#54912=DIRECTION('',(-0.814879198737222,0.,-0.579630823425897));
#54913=DIRECTION('center_axis',(0.,-1.,1.45983193964168E-32));
#54914=DIRECTION('ref_axis',(1.,0.,0.));
#54915=DIRECTION('center_axis',(0.785420358017335,0.601098531523994,-0.147632708474847));
#54916=DIRECTION('ref_axis',(-0.200350744918924,0.0212180447058338,-0.979494447962465));
#54917=DIRECTION('center_axis',(0.768407600938775,-0.601098526051774,-0.219614026869643));
#54918=DIRECTION('ref_axis',(-0.258606873673701,0.0222452610627766,-0.965726479521486));
#54919=DIRECTION('center_axis',(-0.769338824807468,0.60109852954767,0.216329217674113));
#54920=DIRECTION('ref_axis',(-0.254478787566266,0.0222451690245878,-0.966822475500994));
#54921=DIRECTION('center_axis',(0.782151653292242,0.584827953375421,-0.214976873646746));
#54922=DIRECTION('ref_axis',(-0.259557643786552,-0.00784642891152066,-0.965695740440699));
#54923=DIRECTION('center_axis',(-0.957443242555532,-1.95480487174851E-9,
0.288621616107921));
#54924=DIRECTION('ref_axis',(0.288586143092863,-0.0156778482815104,0.957325567969459));
#54925=DIRECTION('',(0.957443409238456,0.,-0.2886210631708));
#54926=DIRECTION('center_axis',(0.790755101116753,0.584827952254255,-0.180783396140045));
#54927=DIRECTION('ref_axis',(-0.224600172512662,0.00246180456921715,-0.974447896003448));
#54928=DIRECTION('center_axis',(0.973676796191129,5.41348134919956E-10,
-0.22793309667308));
#54929=DIRECTION('ref_axis',(0.227905107940483,0.0156707406184557,0.973557234918988));
#54930=DIRECTION('',(-0.973676779881,-6.42264019716094E-11,0.227933166346118));
#54931=DIRECTION('',(0.472928816313867,1.64268989064855E-13,-0.881100638236044));
#54932=DIRECTION('center_axis',(-0.761763162109401,-0.601098528069507,0.241655631851939));
#54933=DIRECTION('ref_axis',(-0.297409192544541,-0.00691952221419285,-0.954725034972023));
#54934=DIRECTION('',(-0.849666541311454,2.36136671784956E-11,-0.527320366168264));
#54935=DIRECTION('center_axis',(0.,-1.,1.45983193964168E-32));
#54936=DIRECTION('ref_axis',(1.,0.,0.));
#54937=DIRECTION('center_axis',(0.760723795752158,0.601098526498427,-0.244907876594135));
#54938=DIRECTION('ref_axis',(-0.300007915937367,-0.00897210709785068,-0.953894518104147));
#54939=DIRECTION('center_axis',(0.768407598352854,-0.601098528653796,-0.219614028795614));
#54940=DIRECTION('ref_axis',(-0.280533628432852,-0.00794569101660869,-0.959811309223103));
#54941=DIRECTION('center_axis',(-0.769338832903073,0.601098527321917,0.21632919506798));
#54942=DIRECTION('ref_axis',(-0.276430591656974,-0.00794579897947787,-0.961001036562788));
#54943=DIRECTION('center_axis',(0.749021847101764,0.584826536164618,-0.311358627890662));
#54944=DIRECTION('ref_axis',(-0.371641576340283,-0.018184624961436,-0.928198178273542));
#54945=DIRECTION('center_axis',(-0.937431424039985,-5.13910947046991E-10,
0.348169965997019));
#54946=DIRECTION('ref_axis',(0.348127165115549,-0.0156795066182876,0.937316184636123));
#54947=DIRECTION('',(0.937431447998912,2.06171160587093E-7,-0.348169901488658));
#54948=DIRECTION('center_axis',(0.761859578895022,0.584827782536468,-0.278471626596639));
#54949=DIRECTION('ref_axis',(-0.324582447047109,-0.0273551074266564,-0.945461756585948));
#54950=DIRECTION('center_axis',(0.957443440341857,7.30692533559346E-10,
-0.288620959991386));
#54951=DIRECTION('ref_axis',(0.288585376147215,0.0157023279247365,0.957325397956053));
#54952=DIRECTION('',(0.957443409426106,-1.29267410337996E-5,-0.288621062258828));
#54953=DIRECTION('',(0.416670796384349,-7.62630514902167E-8,-0.909057450021959));
#54954=DIRECTION('center_axis',(-0.937431446875436,3.17801790996086E-12,
0.348169904513626));
#54955=DIRECTION('ref_axis',(0.268744079129297,-0.635772805085123,0.723581066810858));
#54956=DIRECTION('',(0.8811006382356,0.,0.472928816314695));
#54957=DIRECTION('center_axis',(0.839189481601217,0.398564391590654,-0.370010053547));
#54958=DIRECTION('ref_axis',(-0.42901236436663,0.903298616859648,2.02564385446472E-16));
#54959=DIRECTION('center_axis',(-0.910854901243392,5.744564612845E-5,0.412726720216767));
#54960=DIRECTION('ref_axis',(0.412726674767955,-0.00036272125224494,0.910854851427097));
#54961=DIRECTION('',(0.91372024077296,5.94973683052012E-5,-0.406343842160635));
#54962=DIRECTION('center_axis',(0.761795958734543,0.59018006380744,-0.267122461691196));
#54963=DIRECTION('ref_axis',(0.493508984532234,-0.795824167217403,-0.350874303787966));
#54964=DIRECTION('center_axis',(0.0131267096924739,0.550037558044511,-0.835036750229043));
#54965=DIRECTION('ref_axis',(-1.16798815570368E-17,0.835108702330798,0.550084952794903));
#54966=DIRECTION('center_axis',(0.820332144110193,-0.477126090614814,0.315286959759198));
#54967=DIRECTION('ref_axis',(0.40600907759125,0.0976264307245231,-0.908639482378733));
#54968=DIRECTION('center_axis',(0.787112480220966,0.58482795138957,0.196036248571223));
#54969=DIRECTION('ref_axis',(0.22297139685242,0.0265489690048779,-0.974463395120852));
#54970=DIRECTION('center_axis',(-0.989209569180196,-1.7727863172603E-12,
-0.146507434085546));
#54971=DIRECTION('ref_axis',(-0.146489266611052,-0.0157477670559463,0.989086903462232));
#54972=DIRECTION('center_axis',(0.97991372776366,-0.00011544114226027,0.199421846380157));
#54973=DIRECTION('ref_axis',(0.00484665943939179,-0.999690671402767,-0.0243940854012324));
#54974=DIRECTION('',(-0.978058312887152,-6.06514838087335E-10,-0.208331314478496));
#54975=DIRECTION('center_axis',(-0.782419630478694,-0.601098527966524,-0.162788456341543));
#54976=DIRECTION('ref_axis',(0.183010087021585,0.0279220146957969,-0.982714439266911));
#54977=DIRECTION('',(-0.5442791801312,2.24206636476379E-10,-0.838904150708357));
#54978=DIRECTION('center_axis',(0.,-1.,1.45983193964168E-32));
#54979=DIRECTION('ref_axis',(1.,0.,0.));
#54980=DIRECTION('center_axis',(0.783107954819573,0.601098531987497,0.159444303569561));
#54981=DIRECTION('ref_axis',(0.180342099955132,0.0258667636464215,-0.983263768030854));
#54982=DIRECTION('center_axis',(0.796016001373979,-0.601098525456467,0.0709865356996868));
#54983=DIRECTION('ref_axis',(0.108923126008378,0.0268944328893104,-0.993686289580432));
#54984=DIRECTION('center_axis',(-0.795705463599409,0.601098529740564,-0.0743866435711483));
#54985=DIRECTION('ref_axis',(0.113167309509515,0.0268943392310359,-0.99321188805597));
#54986=DIRECTION('center_axis',(0.805475721645465,0.584827952222615,0.0958390741755142));
#54987=DIRECTION('ref_axis',(0.120485412214686,-0.00326197145288064,-0.992709738536748));
#54988=DIRECTION('center_axis',(-0.996456874308969,-5.64487442434603E-10,
-0.0841052771376477));
#54989=DIRECTION('ref_axis',(-0.0840949330836856,-0.0156832196320191,0.996334320823901));
#54990=DIRECTION('',(0.996456868143877,8.32144303432584E-8,0.0841053501799309));
#54991=DIRECTION('center_axis',(0.80055020562484,0.584827969931446,0.130750196404785));
#54992=DIRECTION('ref_axis',(0.156170863565598,0.00704480135073622,-0.987704931721566));
#54993=DIRECTION('center_axis',(0.989209560314072,4.75626585929023E-10,
0.146507493949079));
#54994=DIRECTION('ref_axis',(-0.146489501966464,0.0156715280545244,0.9890880795066));
#54995=DIRECTION('',(-0.989209569691783,-1.4432899319981E-11,-0.146507430631343));
#54996=DIRECTION('',(0.764072860870889,-3.07809495139578E-8,-0.645129958442928));
#54997=DIRECTION('center_axis',(0.0394351206968075,0.793626260381199,-0.607126206063436));
#54998=DIRECTION('ref_axis',(1.38549959453206E-18,0.607598837093761,0.794244076567341));
#54999=DIRECTION('center_axis',(0.590699987184514,0.471546674567145,0.654765040945897));
#55000=DIRECTION('ref_axis',(-0.523586731929217,-0.393426487751019,0.755693411962536));
#55001=DIRECTION('center_axis',(-0.796652821640193,-0.601098528049027,-0.0634416373528684));
#55002=DIRECTION('ref_axis',(0.0810898755505838,-0.00227572017840687,-0.996704195426537));
#55003=DIRECTION('',(-0.595880397048102,5.19500677922242E-12,-0.803073192438769));
#55004=DIRECTION('center_axis',(0.,-1.,1.45983193964168E-32));
#55005=DIRECTION('ref_axis',(1.,0.,0.));
#55006=DIRECTION('center_axis',(0.796916587647907,0.601098527501541,0.0600375929488731));
#55007=DIRECTION('ref_axis',(0.0783695203868449,-0.00432806703985685,-0.996914984394374));
#55008=DIRECTION('center_axis',(0.796015997482586,-0.601098528209201,0.0709865560267364));
#55009=DIRECTION('ref_axis',(0.0863504162892312,-0.00330180114940477,-0.996259355647838));
#55010=DIRECTION('center_axis',(-0.795705465563001,0.601098527863717,-0.074386637733132));
#55011=DIRECTION('ref_axis',(0.0906057767860851,-0.00330187871639367,-0.995881363822987));
#55012=DIRECTION('center_axis',(0.811135913073174,0.584828375911389,-0.00585672705487716));
#55013=DIRECTION('ref_axis',(0.0166347872562848,-0.0330794214899682,-0.999314282759347));
#55014=DIRECTION('center_axis',(-0.999772620560389,-1.50627415268376E-7,
-0.0213238640445531));
#55015=DIRECTION('ref_axis',(-0.0213212417725825,-0.0156751609036356,0.99964978566492));
#55016=DIRECTION('',(0.99977160679441,3.88578058618689E-13,0.0213713417389563));
#55017=DIRECTION('center_axis',(0.810624895030398,0.584827952226214,0.029386150681072));
#55018=DIRECTION('ref_axis',(0.0526124214975072,-0.0227607295930021,-0.998355589102682));
#55019=DIRECTION('center_axis',(0.996456862410338,5.28963084084849E-10,
0.0841054181093271));
#55020=DIRECTION('ref_axis',(-0.0840950606332875,0.0156933905084143,0.996334149907266));
#55021=DIRECTION('',(-0.996456868253738,-2.24820162483037E-11,-0.0841053488783731));
#55022=DIRECTION('',(0.722057103468553,0.,-0.691833462135653));
#55023=DIRECTION('center_axis',(-0.798322321646307,-0.601098528011999,0.0369056958078118));
#55024=DIRECTION('ref_axis',(-0.0217365883386131,-0.0324816864609622,-0.99923593849103));
#55025=DIRECTION('',(-0.645129946172534,8.00811321699476E-12,-0.764072871231157));
#55026=DIRECTION('center_axis',(0.,-1.,1.45983193964168E-32));
#55027=DIRECTION('ref_axis',(1.,0.,0.));
#55028=DIRECTION('center_axis',(0.798157370548727,0.601098522271916,-0.0403159814622186));
#55029=DIRECTION('ref_axis',(-0.0244548005322686,-0.034538571078463,-0.99910412362215));
#55030=DIRECTION('center_axis',(0.796015995627959,-0.601098530265478,0.0709865594117118));
#55031=DIRECTION('ref_axis',(0.0636418316459174,-0.0335099662987225,-0.997410045780275));
#55032=DIRECTION('center_axis',(-0.795705464507517,0.601098524981808,-0.0743866723114541));
#55033=DIRECTION('ref_axis',(0.0679023398853725,-0.0335100626041385,-0.997129052802273));
#55034=DIRECTION('',(0.999140703555293,3.88578058618659E-13,-0.0414470083242979));
#55035=DIRECTION('center_axis',(0.807915936815926,0.584827952146018,-0.0724438087592005));
#55036=DIRECTION('ref_axis',(-0.051308426239449,-0.0526562728484819,-0.997293719185345));
#55037=DIRECTION('center_axis',(0.999771605233908,5.32086166830061E-10,
0.0213714147406051));
#55038=DIRECTION('ref_axis',(-0.0213687561129565,0.0157729998156971,0.99964723214692));
#55039=DIRECTION('',(-0.999771606794473,-1.76525460892867E-10,-0.0213713417360126));
#55040=DIRECTION('',(0.677191706197975,-1.43735365431834E-13,-0.735806627488959));
#55041=DIRECTION('',(-0.691833462110934,6.51326541667552E-11,-0.722057103492237));
#55042=DIRECTION('center_axis',(0.,-1.,1.45983193964168E-32));
#55043=DIRECTION('ref_axis',(1.,0.,0.));
#55044=DIRECTION('center_axis',(0.797459690717028,0.60109853555185,0.0523315606390982));
#55045=DIRECTION('ref_axis',(0.0267047523711035,0.0514849123724737,-0.998316663187987));
#55046=DIRECTION('center_axis',(-0.79038560520097,0.60109853544184,0.118199601440836));
#55047=DIRECTION('ref_axis',(-0.108516543809086,0.0525165101673011,-0.992706490297902));
#55048=DIRECTION('center_axis',(0.811041537039342,0.584827923043801,-0.0137085967602897));
#55049=DIRECTION('ref_axis',(-0.032724063722221,0.0219596690951161,-0.999223152547386));
#55050=DIRECTION('center_axis',(-0.994566168142843,-1.31729277523896E-8,
0.104106374375744));
#55051=DIRECTION('ref_axis',(0.104093479141674,-0.0157391391440287,0.994442973276591));
#55052=DIRECTION('',(0.994566648423253,0.,-0.104101785979579));
#55053=DIRECTION('center_axis',(0.810871077874088,0.584827952321184,0.0215490429283152));
#55054=DIRECTION('ref_axis',(0.00327726665943345,0.0322834330522339,-0.999473381073055));
#55055=DIRECTION('center_axis',(0.999140706846209,5.92341332246755E-10,
-0.0414469289918896));
#55056=DIRECTION('ref_axis',(0.0414418191872178,0.0157020800820226,0.999017527525695));
#55057=DIRECTION('',(-0.999140703555343,-1.16573417585624E-12,0.0414470083230859));
#55058=DIRECTION('',(0.629653742642216,0.,-0.776875900241892));
#55059=DIRECTION('center_axis',(-0.797928283125533,-0.601098528079163,0.0446207858447481));
#55060=DIRECTION('ref_axis',(-0.0732868695549994,0.0232723701520699,-0.997039332994608));
#55061=DIRECTION('',(-0.735806627488915,1.43735365432665E-13,-0.677191706198023));
#55062=DIRECTION('center_axis',(0.,-1.,1.45983193964168E-32));
#55063=DIRECTION('ref_axis',(1.,0.,0.));
#55064=DIRECTION('center_axis',(0.797730369155652,0.60109853137464,-0.0480293004949925));
#55065=DIRECTION('ref_axis',(-0.0760077075841752,0.0212180487987468,-0.996881448715429));
#55066=DIRECTION('center_axis',(0.789873413751279,-0.601098526075908,-0.121575294358155));
#55067=DIRECTION('ref_axis',(-0.135530058031665,0.0222452604497166,-0.990523473602447));
#55068=DIRECTION('center_axis',(-0.79038559828228,0.601098529468463,0.118199678082531));
#55069=DIRECTION('ref_axis',(-0.131297161989445,0.022245171162852,-0.991093440404815));
#55070=DIRECTION('center_axis',(0.80292790060668,0.584827953375448,-0.1152521209264));
#55071=DIRECTION('ref_axis',(-0.136477184437087,-0.0078464289019961,-0.990612139882008));
#55072=DIRECTION('center_axis',(-0.98606739651783,-1.97928475987955E-9,
0.166346293991028));
#55073=DIRECTION('ref_axis',(0.166325849227674,-0.0156778482801063,0.985946203883355));
#55074=DIRECTION('',(0.986067493104167,3.88578058618637E-13,-0.166345721445622));
#55075=DIRECTION('center_axis',(0.807177928571927,0.584827952254115,-0.0802499712684867));
#55076=DIRECTION('ref_axis',(-0.100698427309043,0.00246180457790776,-0.994913949171337));
#55077=DIRECTION('center_axis',(0.994566655474391,5.112341101984E-10,-0.104101718614458));
#55078=DIRECTION('ref_axis',(0.104088935582225,0.0156707406191776,0.994444529060222));
#55079=DIRECTION('',(-0.994566648423222,-6.41708908203981E-11,0.104101785979871));
#55080=DIRECTION('',(0.579630823425857,1.64268989064856E-13,-0.81487919873725));
#55081=DIRECTION('center_axis',(-0.786043913859459,-0.601098528073676,0.144275864343844));
#55082=DIRECTION('ref_axis',(-0.175405256149202,-0.00691952199720874,-0.984471998753932));
#55083=DIRECTION('',(-0.776875900234022,2.3593133554863E-11,-0.629653742651926));
#55084=DIRECTION('center_axis',(0.,-1.,1.45983193964168E-32));
#55085=DIRECTION('ref_axis',(1.,0.,0.));
#55086=DIRECTION('center_axis',(0.785420358955231,0.60109852656773,-0.147632723664982));
#55087=DIRECTION('ref_axis',(-0.178087573082603,-0.00897210222286303,-0.983973738315841));
#55088=DIRECTION('center_axis',(0.789873411738925,-0.601098528636561,-0.121575294771892));
#55089=DIRECTION('ref_axis',(-0.158025279743992,-0.00794569274266845,-0.987403097487886));
#55090=DIRECTION('center_axis',(-0.790385604202826,0.601098527305987,0.118199649489781));
#55091=DIRECTION('ref_axis',(-0.153805485205631,-0.00794579997179938,-0.988069196455121));
#55092=DIRECTION('center_axis',(0.782151614114705,0.584827952228535,-0.214977019306578));
#55093=DIRECTION('ref_axis',(-0.252337589513471,-0.0181546317291736,-0.967468940207028));
#55094=DIRECTION('center_axis',(-0.973676763012146,-5.60776949172076E-10,
0.227933238405875));
#55095=DIRECTION('ref_axis',(0.22790521834897,-0.0156795066172466,0.973557067932614));
#55096=DIRECTION('',(0.973676780617487,2.06171160587071E-7,-0.227933163199926));
#55097=DIRECTION('center_axis',(0.790753837977295,0.584827782536514,-0.180789470096029));
#55098=DIRECTION('ref_axis',(-0.20352523833637,-0.0273551074234324,-0.978687475886953));
#55099=DIRECTION('center_axis',(0.986067510177297,6.90490385794096E-10,
-0.166345620239144));
#55100=DIRECTION('ref_axis',(0.166325111618119,0.0157023279257334,0.985945938752695));
#55101=DIRECTION('',(0.986067493175933,-1.2926740480983E-5,-0.166345720517936));
#55102=DIRECTION('',(0.527320332408238,-7.62629077548565E-8,-0.849666562263609));
#55103=DIRECTION('center_axis',(-0.973676779746441,-4.80402468853765E-10,
0.227933166920922));
#55104=DIRECTION('ref_axis',(0.175936197693315,-0.635772805081887,0.751557978242216));
#55105=DIRECTION('',(0.814879198736464,0.,0.579630823426963));
#55106=DIRECTION('center_axis',(0.878946778346926,0.398564391591961,-0.261914082455468));
#55107=DIRECTION('ref_axis',(-0.412981067411442,0.910739610404481,-3.93877995988757E-17));
#55108=DIRECTION('center_axis',(-0.955400912706611,5.74456610291878E-5,
0.295311856686064));
#55109=DIRECTION('ref_axis',(0.295311817849053,-0.000362660813026997,0.955400857606807));
#55110=DIRECTION('',(0.957443671436224,5.94973684118189E-5,-0.288620187247509));
#55111=DIRECTION('center_axis',(0.789268291915765,0.590180063811103,-0.169537770589014));
#55112=DIRECTION('ref_axis',(0.533587214447737,-0.795821262434452,-0.286274698209849));
#55113=DIRECTION('center_axis',(0.117681057716851,0.550037558044731,-0.82680702306816));
#55114=DIRECTION('ref_axis',(1.5271491548741E-16,0.83259233830046,0.553886268292843));
#55115=DIRECTION('center_axis',(0.774347646173993,-0.477126090177126,0.415615708241503));
#55116=DIRECTION('ref_axis',(0.51669272472535,0.0976322306155627,-0.850586019025074));
#55117=DIRECTION('center_axis',(0.756336006288325,0.584827951389734,0.293141796516828));
#55118=DIRECTION('ref_axis',(0.343345849085406,0.0265489690012112,-0.938833734034304));
#55119=DIRECTION('center_axis',(-0.9630471056442,7.61707667613043E-12,-0.269333013777237));
#55120=DIRECTION('ref_axis',(-0.269299615467692,-0.0157477670567472,0.962927684170353));
#55121=DIRECTION('center_axis',(0.947192633567712,-0.000115441243345257,
0.320665092562912));
#55122=DIRECTION('ref_axis',(0.00787578078550292,-0.999689899016347,-0.023623672062273));
#55123=DIRECTION('',(-0.944235193661842,-6.06570349238513E-10,-0.329271770807008));
#55124=DIRECTION('center_axis',(-0.755847216535123,-0.601098528159584,-0.259567996294784));
#55125=DIRECTION('ref_axis',(0.304733770807828,0.027922010452604,-0.952028198249152));
#55126=DIRECTION('',(-0.434844806368847,2.24350371841866E-10,-0.900505410519026));
#55127=DIRECTION('center_axis',(0.,-1.,1.45983193964168E-32));
#55128=DIRECTION('ref_axis',(1.,0.,0.));
#55129=DIRECTION('center_axis',(0.756949243714246,0.601098531914126,0.256336492468616));
#55130=DIRECTION('ref_axis',(0.302155678236854,0.0258667653067949,-0.952907580283518));
#55131=DIRECTION('center_axis',(0.780842206360819,-0.601098525344159,0.170194041008038));
#55132=DIRECTION('ref_axis',(0.232606147173315,0.0268944354086559,-0.972199089508541));
#55133=DIRECTION('center_axis',(-0.780107969953459,0.601098529720276,-0.173528420678617));
#55134=DIRECTION('ref_axis',(0.236757408448613,0.026894339668752,-0.971196490952515));
#55135=DIRECTION('center_axis',(0.787112483925137,0.58482795222257,0.196036231213407));
#55136=DIRECTION('ref_axis',(0.243954870283373,-0.00326197144530851,-0.969781099427759));
#55137=DIRECTION('center_axis',(-0.978058329448275,-6.23278424207892E-10,
-0.208331236728554));
#55138=DIRECTION('ref_axis',(-0.208305614215986,-0.0156832196301943,0.977938038787802));
#55139=DIRECTION('',(0.978058312613238,8.3214430343242E-8,0.208331315764432));
#55140=DIRECTION('center_axis',(0.777850283241406,0.584827969931775,0.230054737935873));
#55141=DIRECTION('ref_axis',(0.278731662545331,0.00704480133959886,-0.960343184007051));
#55142=DIRECTION('center_axis',(0.963047084611284,6.17958183329108E-10,
0.269333088984082));
#55143=DIRECTION('ref_axis',(-0.2693000132912,0.015671528055328,0.96292881670961));
#55144=DIRECTION('',(-0.963047106749995,-1.40443212613654E-11,-0.269333009823273));
#55145=DIRECTION('',(0.838904141906417,-3.07810727157134E-8,-0.544279193697736));
#55146=DIRECTION('center_axis',(0.115217253574516,0.793626260383203,-0.597396303394086));
#55147=DIRECTION('ref_axis',(2.53029610822811E-17,0.601401446656677,0.79894699446162));
#55148=DIRECTION('center_axis',(0.503978321585131,0.471546674548375,0.723636362474001));
#55149=DIRECTION('ref_axis',(0.614178693886623,0.39341725961525,-0.684110657578544));
#55150=DIRECTION('center_axis',(-0.782419630395453,-0.601098528053825,-0.162788456419267));
#55151=DIRECTION('ref_axis',(0.205370618307549,-0.002275719460754,-0.978681628639728));
#55152=DIRECTION('',(-0.4905299421393,5.05127141378903E-12,-0.871424337429714));
#55153=DIRECTION('center_axis',(0.,-1.,1.45983193964168E-32));
#55154=DIRECTION('ref_axis',(1.,0.,0.));
#55155=DIRECTION('center_axis',(0.783107955385302,0.601098527525842,0.159444317611245));
#55156=DIRECTION('ref_axis',(0.202698136851968,-0.00432806322786716,-0.979231705565867));
#55157=DIRECTION('center_axis',(0.780842198431431,-0.601098528204078,0.17019406728691));
#55158=DIRECTION('ref_axis',(0.210533925993421,-0.00330180270151346,-0.977580975727698));
#55159=DIRECTION('center_axis',(-0.780107972007283,0.60109852785516,-0.173528417906242));
#55160=DIRECTION('ref_axis',(0.214708356390796,-0.00330187999745221,-0.976672626464183));
#55161=DIRECTION('center_axis',(0.805474420452859,0.584828255987408,0.0958481559283075));
#55162=DIRECTION('ref_axis',(0.141747987856584,-0.0330815410796403,-0.98934984690877));
#55163=DIRECTION('center_axis',(-0.989214558882193,-1.08087088037379E-7,
-0.146473739951897));
#55164=DIRECTION('ref_axis',(-0.146455742083979,-0.0156751635316721,0.989093021337673));
#55165=DIRECTION('',(0.989209569691817,3.88578058618681E-13,0.146507430631113));
#55166=DIRECTION('center_axis',(0.800549814323794,0.58482795222629,0.130752671410353));
#55167=DIRECTION('ref_axis',(0.177324691070629,-0.0227607295910026,-0.983889172176008));
#55168=DIRECTION('center_axis',(0.978058296034405,6.18594720556444E-10,
0.208331393597502));
#55169=DIRECTION('ref_axis',(-0.208305737838454,0.015693390506422,0.977937849292065));
#55170=DIRECTION('',(-0.978058312885219,-2.24265050970653E-11,-0.208331314487569));
#55171=DIRECTION('',(0.803073192437117,-1.43735365431889E-13,-0.595880397050329));
#55172=DIRECTION('center_axis',(-0.796652821848156,-0.601098528024524,-0.0634416349735795));
#55173=DIRECTION('ref_axis',(0.103672282694559,-0.0324816862473311,-0.99408098153995));
#55174=DIRECTION('',(-0.544279180225778,8.17238220606129E-12,-0.838904150646995));
#55175=DIRECTION('center_axis',(0.,-1.,1.45983193964168E-32));
#55176=DIRECTION('ref_axis',(1.,0.,0.));
#55177=DIRECTION('center_axis',(0.796916592183571,0.601098522752696,0.0600375802897754));
#55178=DIRECTION('ref_axis',(0.100958994621709,-0.0345385625894204,-0.99429088756723));
#55179=DIRECTION('center_axis',(0.780842196599987,-0.601098530248933,0.17019406846738));
#55180=DIRECTION('ref_axis',(0.188148623470608,-0.0335099666683606,-0.981568733008545));
#55181=DIRECTION('center_axis',(-0.780107967744112,0.601098525096341,-0.173528446628081));
#55182=DIRECTION('ref_axis',(0.192340315430215,-0.0335100605282662,-0.980755973167432));
#55183=DIRECTION('',(0.996456868253704,3.88578058618601E-13,0.0841053488787717));
#55184=DIRECTION('center_axis',(0.810624895144929,0.584827952145969,0.0293861491186781));
#55185=DIRECTION('ref_axis',(0.0740902026644828,-0.0526562728495679,-0.99586041130207));
#55186=DIRECTION('center_axis',(0.989209556839538,6.48209010908156E-10,
0.146507517408919));
#55187=DIRECTION('ref_axis',(-0.146489291664188,0.0157729998144143,0.98908649768591));
#55188=DIRECTION('',(-0.989209569692122,-1.76969550102591E-10,-0.146507430629054));
#55189=DIRECTION('',(0.764072871228435,0.,-0.645129946175758));
#55190=DIRECTION('',(-0.595880397021771,6.72270837774884E-11,-0.803073192458307));
#55191=DIRECTION('center_axis',(0.,-1.,1.45983193964168E-32));
#55192=DIRECTION('ref_axis',(1.,0.,0.));
#55193=DIRECTION('center_axis',(0.784612598448139,0.601098535311237,0.151867116925111));
#55194=DIRECTION('ref_axis',(0.151616436599874,0.0514849151660113,-0.987097644442081));
#55195=DIRECTION('center_axis',(-0.798967517010862,0.601098535033961,0.0182059864199733));
#55196=DIRECTION('ref_axis',(0.0167582497254366,0.0525165148770827,-0.998479432302591));
#55197=DIRECTION('center_axis',(0.806364404619297,0.58482793005053,0.0880496405204397));
#55198=DIRECTION('ref_axis',(0.0927695868605033,0.0219594825816756,-0.995445420341305));
#55199=DIRECTION('center_axis',(-0.999771680335281,-9.50272957164279E-9,
-0.0213679011502948));
#55200=DIRECTION('ref_axis',(-0.0213652542031799,-0.0157391393478712,0.999647840694623));
#55201=DIRECTION('',(0.999771606794418,3.88578058618524E-13,0.0213713417386143));
#55202=DIRECTION('center_axis',(0.801776305997875,0.584827952320729,0.123008216492823));
#55203=DIRECTION('ref_axis',(0.128518655152663,0.0322834330588407,-0.991181484506085));
#55204=DIRECTION('center_axis',(0.996456862274223,5.27118926555364E-10,
0.084105419721982));
#55205=DIRECTION('ref_axis',(-0.0840950507717687,0.0157020800823933,0.996334013831095));
#55206=DIRECTION('',(-0.996456868253673,-4.44089209850033E-13,-0.0841053488791432));
#55207=DIRECTION('',(0.722057103468734,-1.64268989064969E-13,-0.691833462135463));
#55208=DIRECTION('center_axis',(-0.797228847712849,-0.601098528101694,-0.0557379932220375));
#55209=DIRECTION('ref_axis',(0.0522531820751103,0.0232723695238065,-0.998362660449484));
#55210=DIRECTION('',(-0.645129946175722,1.43735365432679E-13,-0.764072871228465));
#55211=DIRECTION('center_axis',(0.,-1.,1.45983193964168E-32));
#55212=DIRECTION('ref_axis',(1.,0.,0.));
#55213=DIRECTION('center_axis',(0.79745969424158,0.601098531278079,0.0523315560198833));
#55214=DIRECTION('ref_axis',(0.0495340149003826,0.0212180514793412,-0.998547032272025));
#55215=DIRECTION('center_axis',(0.798882450803113,-0.601098526263612,-0.0216192396380311));
#55216=DIRECTION('ref_axis',(-0.0103158466528301,0.0222452555462506,-0.999699320752754));
#55217=DIRECTION('center_axis',(-0.798967519598811,0.60109852937561,0.0182060596671171));
#55218=DIRECTION('ref_axis',(-0.00604490231352095,0.0222451736562014,-0.999734270396402));
#55219=DIRECTION('center_axis',(0.811041496720708,0.584827954381744,-0.0137096451704552));
#55220=DIRECTION('ref_axis',(-0.0112442943397282,-0.00784635389251968,-0.999905995869309));
#55221=DIRECTION('center_axis',(-0.999140665572378,-2.39543322650626E-9,
0.0414479239478296));
#55222=DIRECTION('ref_axis',(0.0414428298276432,-0.0156778481977069,0.999017866172456));
#55223=DIRECTION('',(0.999140703555307,0.,-0.0414470083239631));
#55224=DIRECTION('center_axis',(0.810871077905441,0.584827952254198,0.0215490435664711));
#55225=DIRECTION('ref_axis',(0.0247913922286098,0.00246180457413497,-0.999689615025387));
#55226=DIRECTION('center_axis',(0.999771605140397,5.87028746314927E-10,
0.021371419115121));
#55227=DIRECTION('ref_axis',(-0.0213687948509366,0.0156707406192051,0.999648839590716));
#55228=DIRECTION('',(-0.999771606794419,-6.41708908203814E-11,-0.0213713417385345));
#55229=DIRECTION('',(0.677191706198009,1.64268989064928E-13,-0.735806627488928));
#55230=DIRECTION('center_axis',(-0.797928283093221,-0.601098528023317,0.0446207871748926));
#55231=DIRECTION('ref_axis',(-0.0506350795953401,-0.00691952595144905,-0.998693250640546));
#55232=DIRECTION('',(-0.691833462126744,2.36136671785025E-11,-0.722057103477089));
#55233=DIRECTION('center_axis',(0.,-1.,1.45983193964168E-32));
#55234=DIRECTION('ref_axis',(1.,0.,0.));
#55235=DIRECTION('center_axis',(0.797730371835312,0.601098526624151,-0.0480293154414078));
#55236=DIRECTION('ref_axis',(-0.0533586835760229,-0.00897209812163425,-0.998535103209862));
#55237=DIRECTION('center_axis',(0.798882448921765,-0.601098528604706,-0.0216192440668271));
#55238=DIRECTION('ref_axis',(-0.0330247766656794,-0.00794569538969458,-0.999422948531279));
#55239=DIRECTION('center_axis',(-0.798967521824576,0.601098527331365,0.0182060294836761));
#55240=DIRECTION('ref_axis',(-0.0287547780917037,-0.00794579812142253,-0.999554914463988));
#55241=DIRECTION('center_axis',(0.802927879994109,0.58482795222914,-0.115252270344828));
#55242=DIRECTION('ref_axis',(-0.129091821551966,-0.0181546317646192,-0.991466444693862));
#55243=DIRECTION('center_axis',(-0.994566499546172,-4.82169677984236E-9,
0.104103208310188));
#55244=DIRECTION('ref_axis',(0.104090410872243,-0.0156795063499374,0.994444236468325));
#55245=DIRECTION('',(0.994566648759578,2.06171493653893E-7,-0.104101782766194));
#55246=DIRECTION('center_axis',(0.80717743665864,0.584827782536333,-0.0802561556693508));
#55247=DIRECTION('ref_axis',(-0.0792583150492463,-0.0273551074302921,-0.996478709051544));
#55248=DIRECTION('center_axis',(0.999140707823812,6.92958397042268E-10,
-0.041446905425273));
#55249=DIRECTION('ref_axis',(0.0414417954606099,0.0157023279249861,0.999017524614427));
#55250=DIRECTION('',(0.999140703510251,-1.29267396282542E-5,-0.0414470073942771));
#55251=DIRECTION('',(0.629653711784213,-7.62630514902441E-8,-0.776875925252133));
#55252=DIRECTION('center_axis',(-0.994566627728716,-1.61528326269501E-7,
0.104101983690535));
#55253=DIRECTION('ref_axis',(0.0803539506805691,-0.635772804014687,0.767682345951323));
#55254=DIRECTION('',(0.735806627488049,0.,0.677191706198964));
#55255=DIRECTION('center_axis',(0.904842559340681,0.39856439159295,-0.149687569824443));
#55256=DIRECTION('ref_axis',(-0.403106047559068,0.915153273731404,-2.21620707676059E-17));
#55257=DIRECTION('center_axis',(-0.984879681052153,5.74456494182127E-5,
0.173239748760516));
#55258=DIRECTION('ref_axis',(0.173239717104257,-0.000362923152739352,0.984879621428133));
#55259=DIRECTION('',(0.986067643452047,5.94973683762695E-5,-0.166344819567638));
#55260=DIRECTION('center_axis',(0.80429339270289,0.590180063807686,-0.0692793673356712));
#55261=DIRECTION('ref_axis',(0.565257933865613,-0.795820139095679,-0.217149198505803));
#55262=DIRECTION('center_axis',(0.220379505161487,0.550037558045268,-0.805538055242815));
#55263=DIRECTION('ref_axis',(-1.78365250524718E-16,0.82584203726199,0.56390152463969));
#55264=DIRECTION('center_axis',(0.716151222799951,-0.477126090775243,0.509389948451743));
#55265=DIRECTION('ref_axis',(0.619221586313834,0.0976225795884288,-0.779124161477155));
#55266=DIRECTION('center_axis',(0.713631661727888,0.584827951390377,0.385624323211112));
#55267=DIRECTION('ref_axis',(0.458305532169128,0.0265489689930021,-0.888398104133829));
#55268=DIRECTION('center_axis',(-0.921696814299896,-7.64602880816405E-12,
-0.387911049738756));
#55269=DIRECTION('ref_axis',(-0.387862947305241,-0.0157477670559312,0.921582520418244));
#55270=DIRECTION('center_axis',(0.899533739617671,-0.000115441140596853,
0.43685127670958));
#55271=DIRECTION('ref_axis',(0.0107128862560727,-0.99969340280687,-0.0223234059338097));
#55272=DIRECTION('',(-0.895520921373816,-6.06903416145823E-10,-0.445019414612207));
#55273=DIRECTION('center_axis',(-0.717354638076182,-0.601098528089715,-0.352254003183738));
#55274=DIRECTION('ref_axis',(0.421651628388622,0.0279220120055917,-0.906327901767778));
#55275=DIRECTION('',(-0.318552670246172,2.24206636476366E-10,-0.947905162070043));
#55276=DIRECTION('center_axis',(0.,-1.,1.45983193964168E-32));
#55277=DIRECTION('ref_axis',(1.,0.,0.));
#55278=DIRECTION('center_axis',(0.718852989379429,0.601098531789471,0.349186103304242));
#55279=DIRECTION('ref_axis',(0.419204082182475,0.0258667681431969,-0.907523469551821));
#55280=DIRECTION('center_axis',(0.753354059151887,-0.601098525631524,0.26671749856915));
#55281=DIRECTION('ref_axis',(0.352620841655527,0.0268944291101661,-0.935379725947161));
#55282=DIRECTION('center_axis',(-0.752207708651457,0.601098529635836,-0.269933548702196));
#55283=DIRECTION('ref_axis',(0.356613699824013,0.0268943415657175,-0.933864745822207));
#55284=DIRECTION('center_axis',(0.756336012141187,0.58482795222267,0.293141779754106));
#55285=DIRECTION('ref_axis',(0.363577014296436,-0.00326197145300851,-0.931558433066616));
#55286=DIRECTION('center_axis',(-0.94423522144996,-6.61920013744243E-10,
-0.329271691120486));
#55287=DIRECTION('ref_axis',(-0.32923119423163,-0.0156832196310547,0.944119090669614));
#55288=DIRECTION('',(0.94423519322909,8.32144303432419E-8,0.329271772047978));
#55289=DIRECTION('center_axis',(0.742883197217908,0.584827969931451,0.325731178853293));
#55290=DIRECTION('ref_axis',(0.396896696726391,0.00704480134718826,-0.917836250592478));
#55291=DIRECTION('center_axis',(0.921696784377478,6.05482782476995E-10,
0.387911120835967));
#55292=DIRECTION('ref_axis',(-0.387863483056267,0.0156715280544747,0.921583594537087));
#55293=DIRECTION('',(-0.921696815638182,-1.44328993199795E-11,-0.387911046558918));
#55294=DIRECTION('',(0.900505403486833,-3.07809289803555E-8,-0.434844820931577));
#55295=DIRECTION('center_axis',(0.189182341537265,0.793626260384412,-0.578245104154571));
#55296=DIRECTION('ref_axis',(7.61514585110326E-17,0.588879097809632,0.808221138156454));
#55297=DIRECTION('center_axis',(0.409308616765261,0.471546674544237,0.781095506303794));
#55298=DIRECTION('ref_axis',(0.695084368764266,0.393408104074107,-0.601737304767121));
#55299=DIRECTION('center_axis',(-0.75584721418306,-0.601098528053673,-0.259568003389123));
#55300=DIRECTION('ref_axis',(0.326412543019652,-0.00227571927650737,-0.945224667928857));
#55301=DIRECTION('',(-0.377443537014696,5.05127141378908E-12,-0.926032600055655));
#55302=DIRECTION('center_axis',(0.,-1.,1.45983193964168E-32));
#55303=DIRECTION('ref_axis',(1.,0.,0.));
#55304=DIRECTION('center_axis',(0.756949242071626,0.60109852753972,0.256336507576995));
#55305=DIRECTION('ref_axis',(0.323830080576638,-0.00432806085017039,-0.946105357136828));
#55306=DIRECTION('center_axis',(0.753354050301488,-0.601098528194456,0.266717517791394));
#55307=DIRECTION('ref_axis',(0.331397190998648,-0.00330180520380201,-0.94348555891471));
#55308=DIRECTION('center_axis',(-0.752207710703613,0.601098527861535,-0.269933546934659));
#55309=DIRECTION('ref_axis',(0.335424853501877,-0.0033018785742854,-0.9420611791445));
#55310=DIRECTION('center_axis',(0.787110054748738,0.584828255987617,0.196045078264979));
#55311=DIRECTION('ref_axis',(0.264628678078428,-0.0330815410758865,-0.963782794190946));
#55312=DIRECTION('center_axis',(-0.963056284291006,-1.0823643437071E-7,
-0.269300191770429));
#55313=DIRECTION('ref_axis',(-0.269267103127621,-0.0156751635316013,0.96293796083731));
#55314=DIRECTION('',(0.963047106749919,3.88578058618612E-13,0.269333009823547));
#55315=DIRECTION('center_axis',(0.77784958482566,0.584827952226003,0.230057144383061));
#55316=DIRECTION('ref_axis',(0.29924044432063,-0.0227607296021428,-0.953906235261501));
#55317=DIRECTION('center_axis',(0.944235165175771,6.62804140859967E-10,
0.329271852494993));
#55318=DIRECTION('ref_axis',(-0.329231303059565,0.0156933905093517,0.944118883711168));
#55319=DIRECTION('',(-0.944235193658685,-2.28705943069057E-11,-0.329271770816064));
#55320=DIRECTION('',(0.87142433742843,0.,-0.49052994214158));
#55321=DIRECTION('center_axis',(-0.782419630834816,-0.601098528069948,-0.162788454247995));
#55322=DIRECTION('ref_axis',(0.227446180684351,-0.0324816854257597,-0.973248773440791));
#55323=DIRECTION('',(-0.43484480647018,8.1518485824254E-12,-0.900505410470094));
#55324=DIRECTION('center_axis',(0.,-1.,1.45983193964168E-32));
#55325=DIRECTION('ref_axis',(1.,0.,0.));
#55326=DIRECTION('center_axis',(0.78310796246243,0.601098522796805,0.159444300680334));
#55327=DIRECTION('ref_axis',(0.224780595854182,-0.0345385618110103,-0.973797089477816));
#55328=DIRECTION('center_axis',(0.7533540488904,-0.601098530160528,0.266717517346152));
#55329=DIRECTION('ref_axis',(0.309688200669007,-0.0335099682690439,-0.950247494283989));
#55330=DIRECTION('center_axis',(-0.752207704481693,0.601098525353629,-0.269933569857612));
#55331=DIRECTION('ref_axis',(0.31374496629142,-0.033510055923605,-0.948915787769806));
#55332=DIRECTION('',(0.978058312885182,0.,0.208331314487746));
#55333=DIRECTION('center_axis',(0.800549814629832,0.584827952146791,0.130752669892176));
#55334=DIRECTION('ref_axis',(0.198320384830501,-0.0526562728374665,-0.978721789831793));
#55335=DIRECTION('center_axis',(0.963047084639028,6.04071551872731E-10,
0.269333088884878));
#55336=DIRECTION('ref_axis',(-0.269299583453945,0.0157729998151177,0.962927280135091));
#55337=DIRECTION('',(-0.963047106750702,-1.7691403895138E-10,-0.269333009820746));
#55338=DIRECTION('',(0.838904150644647,0.,-0.544279180229396));
#55339=DIRECTION('',(-0.490529942111875,6.5132654166756E-11,-0.871424337445151));
#55340=DIRECTION('center_axis',(0.,-1.,1.45983193964168E-32));
#55341=DIRECTION('ref_axis',(1.,0.,0.));
#55342=DIRECTION('center_axis',(0.759391695701333,0.601098535079257,0.249007637684921));
#55343=DIRECTION('ref_axis',(0.274137038722192,0.0514849178358315,-0.960311505312763));
#55344=DIRECTION('center_axis',(-0.794949234662874,0.601098535026273,-0.0820747555474917));
#55345=DIRECTION('ref_axis',(0.141768761737848,0.0525165149262143,-0.988505758129573));
#55346=DIRECTION('center_axis',(0.788970434278718,0.584827930050502,0.188419601068719));
#55347=DIRECTION('ref_axis',(0.216800464328143,0.0219594825819946,-0.975968923578939));
#55348=DIRECTION('center_axis',(-0.989210085707457,-1.01383751197917E-8,
-0.146503946481472));
#55349=DIRECTION('ref_axis',(-0.146485799183718,-0.0157391393489173,0.989087554329779));
#55350=DIRECTION('',(0.989209569691852,0.,0.146507430630876));
#55351=DIRECTION('center_axis',(0.780037042821315,0.584827952321357,0.222527476977982));
#55352=DIRECTION('ref_axis',(0.251733227661971,0.0322834330509041,-0.967258063828539));
#55353=DIRECTION('center_axis',(0.978058297637846,5.43689378628934E-10,
0.208331386069788));
#55354=DIRECTION('ref_axis',(-0.20830570188923,0.0157020800826578,0.977937717465439));
#55355=DIRECTION('',(-0.978058312885196,-7.77156117237457E-13,-0.208331314487679));
#55356=DIRECTION('',(0.803073192437116,0.,-0.59588039705033));
#55357=DIRECTION('center_axis',(-0.783956636806604,-0.601098528048292,-0.155217754091001));
#55358=DIRECTION('ref_axis',(0.176969172392052,0.0232723708888864,-0.983941212052876));
#55359=DIRECTION('',(-0.54427918022921,0.,-0.838904150644768));
#55360=DIRECTION('center_axis',(0.,-1.,1.45983193964168E-32));
#55361=DIRECTION('ref_axis',(1.,0.,0.));
#55362=DIRECTION('center_axis',(0.784612601745812,0.601098531093903,0.151867116580321));
#55363=DIRECTION('ref_axis',(0.174294559514057,0.0212180565961819,-0.984464931116432));
#55364=DIRECTION('center_axis',(0.795292633422098,-0.601098526236438,0.0786777540409415));
#55365=DIRECTION('ref_axis',(0.115061044311964,0.0222452563148451,-0.993109311532888));
#55366=DIRECTION('center_axis',(-0.794949246499047,0.601098529356507,-0.0820746824303406));
#55367=DIRECTION('ref_axis',(0.119302691667852,0.0222451741801302,-0.992608694293225));
#55368=DIRECTION('center_axis',(0.806364486303306,0.584827953016348,0.0880487399087191));
#55369=DIRECTION('ref_axis',(0.114165681649204,-0.00784645567446514,-0.993430737528753));
#55370=DIRECTION('center_axis',(-0.996456903954996,-1.54610479594417E-9,
-0.0841049258986923));
#55371=DIRECTION('ref_axis',(-0.0840945889572224,-0.0156778483095254,0.996334434404683));
#55372=DIRECTION('',(0.996456868253732,3.88578058618602E-13,0.0841053488784387));
#55373=DIRECTION('center_axis',(0.801776305949548,0.584827952254047,0.123008217124855));
#55374=DIRECTION('ref_axis',(0.149890236712957,0.00246180457667358,-0.988699578464743));
#55375=DIRECTION('center_axis',(0.98920956001149,4.98288762736695E-10,0.146507495992097));
#55376=DIRECTION('ref_axis',(-0.146489505817707,0.0156707406191989,0.989088091412352));
#55377=DIRECTION('',(-0.989209569691896,-6.37823127618053E-11,-0.146507430630582));
#55378=DIRECTION('',(0.76407287122843,1.64268989064961E-13,-0.645129946175764));
#55379=DIRECTION('center_axis',(-0.797228847335996,-0.601098528067765,-0.0557379989781326));
#55380=DIRECTION('ref_axis',(0.0749336524077195,-0.00691952230795232,-0.99716451398346));
#55381=DIRECTION('',(-0.595880397040262,2.34493981894256E-11,-0.803073192444586));
#55382=DIRECTION('center_axis',(0.,-1.,1.45983193964168E-32));
#55383=DIRECTION('ref_axis',(1.,0.,0.));
#55384=DIRECTION('center_axis',(0.797459698279166,0.60109852670928,0.0523315469715389));
#55385=DIRECTION('ref_axis',(0.0722117068174117,-0.00897209216443674,-0.997348971504312));
#55386=DIRECTION('center_axis',(0.795292631668755,-0.601098528582469,0.0786777538404375));
#55387=DIRECTION('ref_axis',(0.0924965459119079,-0.00794569729621685,-0.995681301867642));
#55388=DIRECTION('center_axis',(-0.794949245543195,0.601098527392003,-0.0820747060760524));
#55389=DIRECTION('ref_axis',(0.0967494055274045,-0.00794579363142727,-0.995277055343717));
#55390=DIRECTION('center_axis',(0.811041493555078,0.584827952230365,-0.0137099242151991));
#55391=DIRECTION('ref_axis',(-0.00381019848136195,-0.018154631726411,-0.999827931063346));
#55392=DIRECTION('center_axis',(-0.999771634704107,-3.84875494615878E-9,
-0.0213700360570086));
#55393=DIRECTION('ref_axis',(-0.0213674089564386,-0.0156795063471331,0.999648731762912));
#55394=DIRECTION('',(0.999771606725356,2.06171160587047E-7,0.0213713449683962));
#55395=DIRECTION('center_axis',(0.810871364980605,0.584827782536739,0.0215428463219416));
#55396=DIRECTION('ref_axis',(0.0462585592507087,-0.0273551074091835,-0.998554877708121));
#55397=DIRECTION('center_axis',(0.996456858641484,7.82376094411192E-10,
0.0841054627616138));
#55398=DIRECTION('ref_axis',(-0.0840950934827374,0.015702327924652,0.996334006320108));
#55399=DIRECTION('',(0.996456868092494,-1.29267395926603E-5,0.0841053497953458));
#55400=DIRECTION('',(0.722057075988427,-7.62630514902547E-8,-0.691833490816278));
#55401=DIRECTION('center_axis',(-0.999771611042796,-1.61527610287435E-7,
-0.0213711429938946));
#55402=DIRECTION('ref_axis',(-0.016495774990561,-0.635772804014641,0.771699961826371));
#55403=DIRECTION('',(0.645129946174821,0.,0.764072871229226));
#55404=DIRECTION('center_axis',(0.916468432647469,0.398564391592776,-0.0351003947979456));
#55405=DIRECTION('ref_axis',(-0.398810141877463,0.917033516691554,5.53686176681803E-17));
#55406=DIRECTION('center_axis',(-0.998826308491894,5.74456525261277E-5,
0.048435546496896));
#55407=DIRECTION('ref_axis',(0.0484355225642264,-0.000362908471667172,0.998826245375727));
#55408=DIRECTION('',(0.999140739682401,5.94973683407417E-5,-0.0414460947131014));
#55409=DIRECTION('center_axis',(0.806634306200451,0.590180063810972,0.0320716126908823));
#55410=DIRECTION('ref_axis',(0.588016972727278,-0.795820717445797,-0.144587086106277));
#55411=DIRECTION('center_axis',(0.31960243616028,0.550037558046786,-0.77156527108103));
#55412=DIRECTION('ref_axis',(-1.40687696057311E-16,0.814272451719983,0.580482880341814));
#55413=DIRECTION('center_axis',(0.64666066718635,-0.477126090607359,0.595130805097369));
#55414=DIRECTION('ref_axis',(0.711989593230198,0.0976245058129954,-0.695370602626158));
#55415=DIRECTION('center_axis',(0.659672919556294,0.584827951390327,0.472025323978142));
#55416=DIRECTION('ref_axis',(0.566037463240398,0.0265489689913246,-0.823951905425234));
#55417=DIRECTION('center_axis',(-0.865810814540078,-2.02897135812954E-11,
-0.500371495416602));
#55418=DIRECTION('ref_axis',(-0.500309447463457,-0.0157477670546732,0.865703450733334));
#55419=DIRECTION('center_axis',(0.837688665200949,-0.000115441160790834,
0.546148044825934));
#55420=DIRECTION('ref_axis',(0.0127915959477522,-0.999721510045263,-0.0198312235106537));
#55421=DIRECTION('',(-0.832683749197209,-6.07014438448021E-10,-0.553748836407698));
#55422=DIRECTION('center_axis',(-0.667548946793382,-0.601098527962809,-0.439384755443325));
#55423=DIRECTION('ref_axis',(0.531919789020974,0.0279220147650522,-0.846334271514124));
#55424=DIRECTION('',(-0.197236768219774,2.24206636476456E-10,-0.980355882964049));
#55425=DIRECTION('center_axis',(0.,-1.,1.45983193964168E-32));
#55426=DIRECTION('ref_axis',(1.,0.,0.));
#55427=DIRECTION('center_axis',(0.669419990798359,0.601098531560112,0.436528843578293));
#55428=DIRECTION('ref_axis',(0.529641389590394,0.0258667733636549,-0.84782716898464));
#55429=DIRECTION('center_axis',(0.713985067372484,-0.601098525837634,0.359034658222479));
#55430=DIRECTION('ref_axis',(0.467074491946653,0.0268944246589108,-0.883808864458284));
#55431=DIRECTION('center_axis',(-0.712444686287866,0.601098529375266,-0.362081657866117));
#55432=DIRECTION('ref_axis',(0.470845975634754,0.0268943474458885,-0.881805398772324));
#55433=DIRECTION('center_axis',(0.713631669624092,0.584827952222598,0.385624307336369));
#55434=DIRECTION('ref_axis',(0.477465331622029,-0.00326197144642527,-0.878644533723023));
#55435=DIRECTION('center_axis',(-0.895520966472167,-7.947455469195E-10,
-0.445019323859937));
#55436=DIRECTION('ref_axis',(-0.444964591254928,-0.0156832196312974,0.895410827023736));
#55437=DIRECTION('',(0.895520920788632,8.32139862540598E-8,0.445019415789777));
#55438=DIRECTION('center_axis',(0.69620039940266,0.58482796993151,0.416270644481887));
#55439=DIRECTION('ref_axis',(0.50880243289223,0.00704480134550057,-0.86085449122192));
#55440=DIRECTION('center_axis',(0.865810765649482,7.49484263326867E-10,
0.500371580013751));
#55441=DIRECTION('ref_axis',(-0.50031013142348,0.0156715280536838,0.865704438941769));
#55442=DIRECTION('',(-0.865810815148925,-1.48214773785942E-11,-0.500371494363093));
#55443=DIRECTION('',(0.947905156918536,-3.07810316484846E-8,-0.318552685575313));
#55444=DIRECTION('center_axis',(0.260163910959887,0.793626260386302,-0.54997463419626));
#55445=DIRECTION('ref_axis',(-1.5872085081592E-17,0.569588725703824,0.82192985318158));
#55446=DIRECTION('center_axis',(0.308183870415267,0.471546674597968,0.826236307415417));
#55447=DIRECTION('ref_axis',(0.765014665445126,0.393417088882177,-0.509877981314505));
#55448=DIRECTION('center_axis',(-0.717354637119605,-0.6010985280463,-0.352254005205861));
#55449=DIRECTION('ref_axis',(0.442306744791282,-0.00227572086838956,-0.89686095054176));
#55450=DIRECTION('',(-0.258404621837415,5.05127141378918E-12,-0.966036775393702));
#55451=DIRECTION('center_axis',(0.,-1.,1.45983193964168E-32));
#55452=DIRECTION('ref_axis',(1.,0.,0.));
#55453=DIRECTION('center_axis',(0.71885298669406,0.601098527551182,0.349186116128391));
#55454=DIRECTION('ref_axis',(0.439855029239441,-0.0043280593061185,-0.898058361775789));
#55455=DIRECTION('center_axis',(0.713985057703359,-0.601098528184557,0.3590346735215));
#55456=DIRECTION('ref_axis',(0.447034124176754,-0.00330180781928047,-0.894510810379979));
#55457=DIRECTION('center_axis',(-0.712444684573304,0.601098527865069,-0.362081663746858));
#55458=DIRECTION('ref_axis',(0.450851501151844,-0.00330187774175132,-0.892592864363427));
#55459=DIRECTION('center_axis',(0.756332493291777,0.584828255987081,0.293150252584156));
#55460=DIRECTION('ref_axis',(0.383336015948029,-0.0330815410858942,-0.923016311078236));
#55461=DIRECTION('center_axis',(-0.921710034200493,-1.08240530837605E-7,
-0.387879637070721));
#55462=DIRECTION('ref_axis',(-0.387831979480682,-0.0156751635319584,0.921596790869164));
#55463=DIRECTION('',(0.921696815638239,0.,0.387911046558782));
#55464=DIRECTION('center_axis',(0.742882202703939,0.584827952226054,0.325733478784151));
#55465=DIRECTION('ref_axis',(0.416436997026077,-0.0227607295980158,-0.908879627176266));
#55466=DIRECTION('center_axis',(0.895520879251373,7.26913384781663E-10,
0.44501949937598));
#55467=DIRECTION('ref_axis',(-0.444964695753017,0.0156933905072713,0.895410596892739));
#55468=DIRECTION('',(-0.895520921369782,-2.24820162482919E-11,-0.445019414620325));
#55469=DIRECTION('',(0.926032600054683,-1.43735365431985E-13,-0.377443537017079));
#55470=DIRECTION('center_axis',(-0.755847215917792,-0.601098527981938,-0.259567998503803));
#55471=DIRECTION('ref_axis',(0.347633113441175,-0.0324816870314175,-0.937067851570413));
#55472=DIRECTION('',(-0.318552670353025,8.15184858242886E-12,-0.947905162034134));
#55473=DIRECTION('center_axis',(0.,-1.,1.45983193964168E-32));
#55474=DIRECTION('ref_axis',(1.,0.,0.));
#55475=DIRECTION('center_axis',(0.756949252602283,0.601098522786963,0.256336487625497));
#55476=DIRECTION('ref_axis',(0.345057271550156,-0.0345385619991088,-0.937945929723774));
#55477=DIRECTION('center_axis',(0.713985059025465,-0.601098530219434,0.359034667485523));
#55478=DIRECTION('ref_axis',(0.426343806632472,-0.0335099672547986,-0.903940285992784));
#55479=DIRECTION('center_axis',(-0.712444668004794,0.601098524805671,-0.362081701426605));
#55480=DIRECTION('ref_axis',(0.430201689006238,-0.0335100655799265,-0.902110626409538));
#55481=DIRECTION('',(0.944235193658814,-3.88578058618719E-13,0.329271770815693));
#55482=DIRECTION('center_axis',(0.777849585313836,0.584827952146828,0.230057142933752));
#55483=DIRECTION('ref_axis',(0.319422936040306,-0.0526562728363321,-0.946148141076426));
#55484=DIRECTION('center_axis',(0.921696777606893,7.30033026013869E-10,
0.387911136923225));
#55485=DIRECTION('ref_axis',(-0.38786288020675,0.0157729998153751,0.92158211714125));
#55486=DIRECTION('',(-0.921696815639174,-1.76914038951287E-10,-0.387911046556562));
#55487=DIRECTION('',(0.90050541046818,0.,-0.434844806474143));
#55488=DIRECTION('',(-0.377443536985532,6.51326541667579E-11,-0.926032600067542));
#55489=DIRECTION('center_axis',(0.,-1.,1.45983193964168E-32));
#55490=DIRECTION('ref_axis',(1.,0.,0.));
#55491=DIRECTION('center_axis',(0.722194730403783,0.601098534741279,0.342221160814019));
#55492=DIRECTION('ref_axis',(0.392334337172448,0.0514849217340168,-0.918380678536683));
#55493=DIRECTION('center_axis',(-0.778394128429977,0.601098534940886,-0.181061128124333));
#55494=DIRECTION('ref_axis',(0.264543494507129,0.0525165158982934,-0.962942757941437));
#55495=DIRECTION('center_axis',(0.759133928885952,0.58482793005096,0.285818071938233));
#55496=DIRECTION('ref_axis',(0.337412268951842,0.0219594825744128,-0.941100813880125));
#55497=DIRECTION('center_axis',(-0.963048054619894,-1.01164058154922E-8,
-0.269329620526294));
#55498=DIRECTION('ref_axis',(-0.269296259071625,-0.0157391393485634,0.962928763898241));
#55499=DIRECTION('',(0.963047106750035,0.,0.269333009823132));
#55500=DIRECTION('center_axis',(0.745996129500833,0.584827952320648,0.318537346247209));
#55501=DIRECTION('ref_axis',(0.370977816814879,0.0322834330599069,-0.928080405665981));
#55502=DIRECTION('center_axis',(0.944235168505604,5.6877892465971E-10,0.329271842946209));
#55503=DIRECTION('ref_axis',(-0.329231248590178,0.0157020800818962,0.944118758225285));
#55504=DIRECTION('',(-0.944235193658622,-3.88578058618715E-13,-0.329271770816244));
#55505=DIRECTION('',(0.87142433742845,-1.43735365431918E-13,-0.490529942141545));
#55506=DIRECTION('center_axis',(-0.758320962878211,-0.601098528151806,-0.252249631740454));
#55507=DIRECTION('ref_axis',(0.298894247961264,0.0232723682068303,-0.954002424217945));
#55508=DIRECTION('',(-0.434844806473994,1.43735365432644E-13,-0.900505410468252));
#55509=DIRECTION('center_axis',(0.,-1.,1.45983193964168E-32));
#55510=DIRECTION('ref_axis',(1.,0.,0.));
#55511=DIRECTION('center_axis',(0.759391699445769,0.60109853103519,0.249007636027903));
#55512=DIRECTION('ref_axis',(0.296306370032838,0.0212180581951432,-0.954857229686402));
#55513=DIRECTION('center_axis',(0.779160575653599,-0.601098526282654,0.177733955810289));
#55514=DIRECTION('ref_axis',(0.23862335649232,0.0222452550770015,-0.970857374882067));
#55515=DIRECTION('center_axis',(-0.778394148784845,0.601098529365771,-0.181061059125989));
#55516=DIRECTION('ref_axis',(0.242768812035222,0.0222451738801953,-0.969829086046633));
#55517=DIRECTION('center_axis',(0.788970628196199,0.584827953016268,0.188418717792304));
#55518=DIRECTION('ref_axis',(0.237775337803774,-0.00784645567628602,-0.971288485397424));
#55519=DIRECTION('center_axis',(-0.97805838109112,-7.84599393169719E-10,
-0.208330994279336));
#55520=DIRECTION('ref_axis',(-0.208305389342993,-0.015677848308091,0.977938172812112));
#55521=DIRECTION('',(0.978058312885159,3.88578058618636E-13,0.208331314487851));
#55522=DIRECTION('center_axis',(0.780037042689973,0.58482795225398,0.222527477615458));
#55523=DIRECTION('ref_axis',(0.2726252226216,0.00246180457925343,-0.962117158930625));
#55524=DIRECTION('center_axis',(0.963047086738829,5.62745578224248E-10,
0.269333081376674));
#55525=DIRECTION('ref_axis',(-0.269300009007876,0.0156707406191654,0.962928830722606));
#55526=DIRECTION('',(-0.963047106750114,-6.41708908203849E-11,-0.269333009822849));
#55527=DIRECTION('',(0.838904150644651,1.6426898906501E-13,-0.544279180229389));
#55528=DIRECTION('center_axis',(-0.783956636830115,-0.601098528045093,-0.155217753984645));
#55529=DIRECTION('ref_axis',(0.199320628268647,-0.00691952448456596,-0.979909897555637));
#55530=DIRECTION('',(-0.490529942130889,2.35931335548681E-11,-0.871424337434448));
#55531=DIRECTION('center_axis',(0.,-1.,1.45983193964168E-32));
#55532=DIRECTION('ref_axis',(1.,0.,0.));
#55533=DIRECTION('center_axis',(0.784612606923713,0.601098526770815,0.151867106940017));
#55534=DIRECTION('ref_axis',(0.196643273319265,-0.00897208774518776,-0.980434049133228));
#55535=DIRECTION('center_axis',(0.779160573919315,-0.601098528567099,0.177733955687123));
#55536=DIRECTION('ref_axis',(0.216559142005727,-0.00794569869411633,-0.976237165798356));
#55537=DIRECTION('center_axis',(-0.778394144807355,0.601098527383943,-0.181061082804895));
#55538=DIRECTION('ref_axis',(0.220727799876673,-0.00794579414360136,-0.9753030824913));
#55539=DIRECTION('center_axis',(0.806364498274801,0.584827952228293,0.0880486355061219));
#55540=DIRECTION('ref_axis',(0.121531513603223,-0.0181546317370622,-0.992421533698157));
#55541=DIRECTION('center_axis',(-0.989209558181874,6.15894848857748E-10,
-0.14650750834555));
#55542=DIRECTION('ref_axis',(-0.146489498037684,-0.0156795066150825,0.989087953640613));
#55543=DIRECTION('',(0.989209569218361,2.06171493653842E-7,0.146507433827718));
#55544=DIRECTION('center_axis',(0.801777367482884,0.584827782536652,0.123002104719708));
#55545=DIRECTION('ref_axis',(0.171045908407409,-0.0273551074109777,-0.984883239432786));
#55546=DIRECTION('center_axis',(0.978058291383363,6.95105897126313E-10,
0.208331415432856));
#55547=DIRECTION('ref_axis',(-0.208305730440146,0.0157023279250068,0.977937707404481));
#55548=DIRECTION('',(0.978058312610443,-1.29267404452746E-5,0.208331315376523));
#55549=DIRECTION('',(0.80307316876836,-7.6262907754909E-8,-0.595880428948912));
#55550=DIRECTION('center_axis',(-0.989209569691202,3.16135222513024E-12,
-0.146507430635265));
#55551=DIRECTION('ref_axis',(-0.113085605683379,-0.635772805085027,0.763547369913315));
#55552=DIRECTION('',(0.544279180228156,0.,0.838904150645451));
#55553=DIRECTION('center_axis',(0.913641051300077,0.398564391591664,0.0800403344224422));
#55554=DIRECTION('ref_axis',(-0.39984725127672,0.916581788847264,-1.13151217873397E-16));
#55555=DIRECTION('center_axis',(-0.997020848376335,5.7445662141833E-5,-0.0771325132672888));
#55556=DIRECTION('ref_axis',(0.077132529100234,0.000362892818154704,-0.997020782764032));
#55557=DIRECTION('',(0.996456789590153,5.94973683407411E-5,0.0841062598131004));
#55558=DIRECTION('center_axis',(0.796254114848551,0.590180063812527,0.13291680429875));
#55559=DIRECTION('ref_axis',(0.601502357066498,-0.795819654738625,-0.0697566597189352));
#55560=DIRECTION('center_axis',(0.413785045843809,0.550037558024795,-0.72542444168787));
#55561=DIRECTION('ref_axis',(-2.3512701952177E-16,0.796841686266789,0.604188155318772));
#55562=DIRECTION('center_axis',(0.56697188662127,-0.477126090203707,0.671486093547768));
#55563=DIRECTION('ref_axis',(0.793529116258299,0.0976273805452995,-0.60065001141945));
#55564=DIRECTION('center_axis',(0.595310741352729,0.584827951389405,0.550982203436496));
#55565=DIRECTION('ref_axis',(0.664842645401608,0.0265489690088179,-0.746511492945661));
#55566=DIRECTION('center_axis',(-0.796270459217244,-1.33926730831543E-11,
-0.604940787001471));
#55567=DIRECTION('ref_axis',(-0.604865772061812,-0.0157477670570415,0.796171718676809));
#55568=DIRECTION('center_axis',(0.762632738812627,-0.000115441153842097,
0.64683173419715));
#55569=DIRECTION('ref_axis',(0.0152930708773917,-0.999717230246732,-0.0182093803008533));
#55570=DIRECTION('',(-0.756714656874731,-6.07014438447633E-10,-0.653745308259232));
#55571=DIRECTION('center_axis',(-0.607215615508909,-0.601098528125524,-0.519586138929307));
#55572=DIRECTION('ref_axis',(0.633799249965789,0.0279220112272639,-0.772993448893215));
#55573=DIRECTION('',(-0.0728103245348818,2.24206636476418E-10,-0.997345805947529));
#55574=DIRECTION('center_axis',(0.,-1.,1.45983193964168E-32));
#55575=DIRECTION('ref_axis',(1.,0.,0.));
#55576=DIRECTION('center_axis',(0.609429838331448,0.601098531375975,0.516987260702768));
#55577=DIRECTION('ref_axis',(0.631725933862725,0.0258667775350435,-0.774760126945896));
#55578=DIRECTION('center_axis',(0.66335610523484,-0.601098525931305,0.445689622686996));
#55579=DIRECTION('ref_axis',(0.574162095150205,0.0268944226164245,-0.818299809681547));
#55580=DIRECTION('center_axis',(-0.661445984060744,0.601098529285794,-0.448519529407996));
#55581=DIRECTION('ref_axis',(0.577652734288884,0.0268943494357593,-0.815839452672524));
#55582=DIRECTION('center_axis',(0.659672929384356,0.584827952222519,0.472025309211994));
#55583=DIRECTION('ref_axis',(0.583823735428411,-0.00326197145261643,-0.811873885214114));
#55584=DIRECTION('center_axis',(-0.832683791162331,-5.94454085157781E-10,
-0.553748773303858));
#55585=DIRECTION('ref_axis',(-0.553680668148574,-0.0156832196308938,0.832581380010721));
#55586=DIRECTION('',(0.832683748469071,8.32136531871631E-8,0.553748837502608));
#55587=DIRECTION('center_axis',(0.638538105402631,0.584827969931605,0.500245273375468));
#55588=DIRECTION('ref_axis',(0.612684050745061,0.00704480134031414,-0.790296542278086));
#55589=DIRECTION('center_axis',(0.79627042978386,3.77540322483168E-10,0.604940825743995));
#55590=DIRECTION('ref_axis',(-0.604866535424114,0.0156715280546595,0.796172643044497));
#55591=DIRECTION('',(-0.796270460894472,-1.48769885298212E-11,-0.604940784793772));
#55592=DIRECTION('',(0.980355879774379,-3.07809289803698E-8,-0.197236784073871));
#55593=DIRECTION('center_axis',(0.327042540097583,0.793626260386024,-0.513030735718841));
#55594=DIRECTION('ref_axis',(1.25736257823514E-16,0.542884142421512,0.839807601720334));
#55595=DIRECTION('center_axis',(0.202198880588061,0.471546674539153,0.858346868358009));
#55596=DIRECTION('ref_axis',(0.82289066041759,0.393411577749833,-0.409973525352419));
#55597=DIRECTION('center_axis',(-0.667548947904293,-0.601098528046553,-0.439384753640974));
#55598=DIRECTION('ref_axis',(0.551225507145412,-0.00227572072850447,-0.834353199411046));
#55599=DIRECTION('',(-0.135290511410435,5.19500677922224E-12,-0.990805973701361));
#55600=DIRECTION('center_axis',(0.,-1.,1.45983193964168E-32));
#55601=DIRECTION('ref_axis',(1.,0.,0.));
#55602=DIRECTION('center_axis',(0.669419981668909,0.601098527615754,0.436528863009733));
#55603=DIRECTION('ref_axis',(0.548943210914805,-0.00432804893558317,-0.83584844271133));
#55604=DIRECTION('center_axis',(0.663356092189077,-0.601098528168137,0.445689639087264));
#55605=DIRECTION('ref_axis',(0.555621063060828,-0.00330181158883881,-0.831429090375954));
#55606=DIRECTION('center_axis',(-0.661445983008431,0.60109852788511,-0.448519532837048));
#55607=DIRECTION('ref_axis',(0.559167948443955,-0.00330187419158931,-0.829047829175013));
#55608=DIRECTION('center_axis',(0.713627116595045,0.58482825598741,0.385632272325549));
#55609=DIRECTION('ref_axis',(0.495997915872523,-0.0330815410799037,-0.867693309349503));
#55610=DIRECTION('center_axis',(-0.86582787538343,-1.08385228015312E-7,
-0.500341973263291));
#55611=DIRECTION('ref_axis',(-0.5002804983147,-0.0156751635309624,0.865721498089468));
#55612=DIRECTION('',(0.865810815149328,0.,0.500371494362396));
#55613=DIRECTION('center_axis',(0.696199124465904,0.584827952226065,0.416272801643317));
#55614=DIRECTION('ref_axis',(0.527066089522502,-0.0227607295913177,-0.849519444429572));
#55615=DIRECTION('center_axis',(0.832683703923129,6.25710847379276E-10,
0.553748904487276));
#55616=DIRECTION('ref_axis',(-0.553680710962633,0.0156933905077011,0.832581159889104));
#55617=DIRECTION('',(-0.832683749191998,-2.24820162482884E-11,-0.553748836415534));
#55618=DIRECTION('',(0.966036775392944,0.,-0.258404621840249));
#55619=DIRECTION('center_axis',(-0.71735463898416,-0.601098527931815,-0.352254001604114));
#55620=DIRECTION('ref_axis',(0.462337665315646,-0.0324816879447406,-0.88610881001079));
#55621=DIRECTION('',(-0.197236768330209,8.17238220606182E-12,-0.98035588294183));
#55622=DIRECTION('center_axis',(0.,-1.,1.45983193964168E-32));
#55623=DIRECTION('ref_axis',(1.,0.,0.));
#55624=DIRECTION('center_axis',(0.718852993768966,0.601098523304961,0.349186108873178));
#55625=DIRECTION('ref_axis',(0.459892199152257,-0.034538552828122,-0.887302796979385));
#55626=DIRECTION('center_axis',(0.663356092770367,-0.60109852991426,0.445689635867099));
#55627=DIRECTION('ref_axis',(0.53627572350735,-0.0335099728267182,-0.843377394822639));
#55628=DIRECTION('center_axis',(-0.661445962688288,0.601098525066399,-0.448519566581396));
#55629=DIRECTION('ref_axis',(0.539873856959319,-0.0335100609617226,-0.841078649346309));
#55630=DIRECTION('',(0.895520921369855,3.88578058618721E-13,0.445019414620179));
#55631=DIRECTION('center_axis',(0.742882203366681,0.584827952147364,0.325733477413953));
#55632=DIRECTION('ref_axis',(0.435487996745506,-0.0526562728284316,-0.898653170929922));
#55633=DIRECTION('center_axis',(0.865810771633002,6.42926458855253E-10,
0.500371569660253));
#55634=DIRECTION('ref_axis',(-0.500309322695488,0.0157729998147222,0.865703063469702));
#55635=DIRECTION('',(-0.865810815150161,-1.76914038951315E-10,-0.500371494360954));
#55636=DIRECTION('',(0.947905162032747,-1.43735365431978E-13,-0.318552670357151));
#55637=DIRECTION('',(-0.258404621806973,6.51326541667439E-11,-0.966036775401845));
#55638=DIRECTION('center_axis',(0.,-1.,1.45983193964168E-32));
#55639=DIRECTION('ref_axis',(1.,0.,0.));
#55640=DIRECTION('center_axis',(0.67360832250785,0.601098534529477,0.430037649089794));
#55641=DIRECTION('ref_axis',(0.504344286576578,0.0514849241852926,-0.86196643970586));
#55642=DIRECTION('center_axis',(-0.749563283555236,0.601098534670828,-0.277192055374023));
#55643=DIRECTION('ref_axis',(0.383146215747937,0.0525165190175251,-0.922193576527357));
#55644=DIRECTION('center_axis',(0.717324974950354,0.584827908067301,0.378709913070808));
#55645=DIRECTION('ref_axis',(0.452703598373547,0.0219600677454818,-0.891390603183731));
#55646=DIRECTION('center_axis',(-0.921699486410975,-1.91782754834668E-8,
-0.387904700602795));
#55647=DIRECTION('ref_axis',(-0.387856651377982,-0.0157391387101182,0.921585317534151));
#55648=DIRECTION('',(0.92169681563843,4.44089209850062E-13,0.38791104655833));
#55649=DIRECTION('center_axis',(0.700190411583638,0.584827952320447,0.409523691269515));
#55650=DIRECTION('ref_axis',(0.484371864175863,0.0322834330620492,-0.874266365099635));
#55651=DIRECTION('center_axis',(0.895520891779626,4.91459824244294E-10,
0.445019474165146));
#55652=DIRECTION('ref_axis',(-0.444964609830889,0.0157020800820199,0.895410487251039));
#55653=DIRECTION('',(-0.895520921369562,-8.32667268468546E-13,-0.445019414620768));
#55654=DIRECTION('',(0.926032600054668,0.,-0.377443537017117));
#55655=DIRECTION('center_axis',(-0.720726113507914,-0.601098528148682,-0.345303386553429));
#55656=DIRECTION('ref_axis',(0.416105586312613,0.0232723683016273,-0.909018447509769));
#55657=DIRECTION('',(-0.318552670356925,0.,-0.947905162032823));
#55658=DIRECTION('center_axis',(0.,-1.,1.45983193964168E-32));
#55659=DIRECTION('ref_axis',(1.,0.,0.));
#55660=DIRECTION('center_axis',(0.722194735685976,0.601098530972697,0.342221156286295));
#55661=DIRECTION('ref_axis',(0.413645252066319,0.0212180599124248,-0.910190858763449));
#55662=DIRECTION('center_axis',(0.750740685581025,-0.601098526591847,0.273987197406091));
#55663=DIRECTION('ref_axis',(0.358422444249889,0.0222452470260503,-0.93329443395034));
#55664=DIRECTION('center_axis',(-0.749563311433282,0.601098529303308,-0.277191991627778));
#55665=DIRECTION('ref_axis',(0.362406320684363,0.0222451755618634,-0.931754694590934));
#55666=DIRECTION('center_axis',(0.759134231974123,0.58482795301644,0.2858172199425));
#55667=DIRECTION('ref_axis',(0.357635134842662,-0.00784645567666929,-0.933828433631888));
#55668=DIRECTION('center_axis',(-0.944235336028488,-1.60783837117334E-9,
-0.329271362549446));
#55669=DIRECTION('ref_axis',(-0.329230893423353,-0.0156778483097205,0.944119284777108));
#55670=DIRECTION('',(0.944235193658949,3.88578058618655E-13,0.329271770815305));
#55671=DIRECTION('center_axis',(0.745996129292408,0.584827952253851,0.318537346857968));
#55672=DIRECTION('ref_axis',(0.391060745915754,0.00246180458492519,-0.920361577056539));
#55673=DIRECTION('center_axis',(0.921696792401348,4.50063191212345E-10,
0.387911101770839));
#55674=DIRECTION('ref_axis',(-0.387863468778648,0.0156707406191547,0.921583613936056));
#55675=DIRECTION('',(-0.921696815638753,-6.4226401971644E-11,-0.387911046557562));
#55676=DIRECTION('',(0.900505410468141,0.,-0.434844806474224));
#55677=DIRECTION('center_axis',(-0.758320961486058,-0.601098528044341,-0.252249636181676));
#55678=DIRECTION('ref_axis',(0.320564201865843,-0.00691952430573698,-0.947201516397381));
#55679=DIRECTION('',(-0.377443537005826,2.34493981894312E-11,-0.92603260005927));
#55680=DIRECTION('center_axis',(0.,-1.,1.45983193964168E-32));
#55681=DIRECTION('ref_axis',(1.,0.,0.));
#55682=DIRECTION('center_axis',(0.75939170473741,0.601098526820475,0.249007630064353));
#55683=DIRECTION('ref_axis',(0.31797365645609,-0.00897208425772004,-0.948057095065491));
#55684=DIRECTION('center_axis',(0.750740687421923,-0.601098528539803,0.273987188088317));
#55685=DIRECTION('ref_axis',(0.337206472014744,-0.00794570095967736,-0.941397185606388));
#55686=DIRECTION('center_axis',(-0.749563305959255,0.601098527443124,-0.277192010464118));
#55687=DIRECTION('ref_axis',(0.341225178879087,-0.00794578980304227,-0.939947999478344));
#55688=DIRECTION('center_axis',(0.788970653153501,0.584827952228961,0.188418615731616));
#55689=DIRECTION('ref_axis',(0.244956601208456,-0.0181546317280604,-0.969364055900166));
#55690=DIRECTION('center_axis',(-0.963047127164173,-5.9401172880047E-10,
-0.269332936828812));
#55691=DIRECTION('ref_axis',(-0.269299827447224,-0.0156795066176967,0.962928738801123));
#55692=DIRECTION('',(0.963047105879958,2.0617149365389E-7,0.269333012934164));
#55693=DIRECTION('center_axis',(0.780038861938788,0.584827782536756,0.222521546458721));
#55694=DIRECTION('ref_axis',(0.293135761418687,-0.0273551074055863,-0.955679404128976));
#55695=DIRECTION('center_axis',(0.94423516594774,5.45508720203076E-10,0.329271850281259));
#55696=DIRECTION('ref_axis',(-0.329231254642399,0.0157023279249513,0.94411875199274));
#55697=DIRECTION('',(0.944235193275004,-1.29267404097053E-5,0.329271771662581));
#55698=DIRECTION('',(0.871424317944201,-7.62629077549355E-8,-0.490529976755221));
#55699=DIRECTION('center_axis',(-0.963047106747145,8.30207502439632E-12,
-0.269333009833466));
#55700=DIRECTION('ref_axis',(-0.207891752764345,-0.635772805084664,0.743353186209185));
#55701=DIRECTION('',(0.434844806472752,0.,0.900505410468851));
#55702=DIRECTION('center_axis',(0.896405004789995,0.398564391592692,0.19391877975533));
#55703=DIRECTION('ref_axis',(-0.406276499725655,0.913750187836188,-3.10333992776203E-16));
#55704=DIRECTION('center_axis',(-0.979491773889536,5.74456556182148E-5,
-0.201484147224359));
#55705=DIRECTION('ref_axis',(0.201484154706541,0.000363041689850167,-0.979491706755561));
#55706=DIRECTION('',(0.978058120671662,5.94973683762348E-5,0.208332208379502));
#55707=DIRECTION('center_axis',(0.773316520448395,0.59018006381252,0.231665818540062));
#55708=DIRECTION('ref_axis',(0.60549942861941,-0.795821622328588,0.00619575466446112));
#55709=DIRECTION('center_axis',(0.501442018148417,0.550037558025294,-0.667843235495288));
#55710=DIRECTION('ref_axis',(-4.66273618249888E-16,0.771902436596558,0.6357410073106));
#55711=DIRECTION('center_axis',(0.478341620466137,-0.477126090494331,0.73725164489435));
#55712=DIRECTION('ref_axis',(0.862552891155475,0.0976251602361496,-0.496459301502346));
#55713=DIRECTION('center_axis',(0.521560157167445,0.584827951390025,0.621249764368902));
#55714=DIRECTION('ref_axis',(0.753162861857848,0.0265489689976712,-0.657298148303536));
#55715=DIRECTION('center_axis',(-0.714172445357471,-3.3520060503145E-11,
-0.699969798128555));
#55716=DIRECTION('ref_axis',(-0.699882999232859,-0.0157477670559804,0.714083885280692));
#55717=DIRECTION('center_axis',(0.675549640303332,-0.000115441165281704,
0.737314498812668));
#55718=DIRECTION('ref_axis',(0.0182582712999792,-0.999690713313198,-0.0168852966952043));
#55719=DIRECTION('',(-0.668811722373935,-6.06903416145164E-10,-0.743431826070966));
#55720=DIRECTION('center_axis',(-0.537306126172887,-0.601098528049546,-0.591593345427207));
#55721=DIRECTION('ref_axis',(0.725683323477494,0.0279220128337455,-0.687462053662579));
#55722=DIRECTION('',(0.0527643814626838,2.24062901110916E-10,-0.998606989785702));
#55723=DIRECTION('center_axis',(0.,-1.,1.45983193964168E-32));
#55724=DIRECTION('ref_axis',(1.,0.,0.));
#55725=DIRECTION('center_axis',(0.539828613186025,0.601098531243132,0.589292477572048));
#55726=DIRECTION('ref_axis',(0.723847780931745,0.0258667806383051,-0.68947465486383));
#55727=DIRECTION('center_axis',(0.602265620307525,-0.601098526029287,0.525315795118528));
#55728=DIRECTION('ref_axis',(0.672194818786008,0.0268944205332519,-0.739885677480938));
#55729=DIRECTION('center_axis',(-0.600015879953058,0.601098529364232,-0.527883985171283));
#55730=DIRECTION('ref_axis',(0.67534956841233,0.0268943476353437,-0.737007228262077));
#55731=DIRECTION('center_axis',(0.595310752969356,0.584827952222556,0.550982190000939));
#55732=DIRECTION('ref_axis',(0.680974890179038,-0.00326197144911916,-0.7322995005378));
#55733=DIRECTION('center_axis',(-0.756714706390063,-5.93515005629862E-10,
-0.653745250944893));
#55734=DIRECTION('ref_axis',(-0.653664847298321,-0.0156832196311885,0.756621638620297));
#55735=DIRECTION('',(0.75671465601544,8.32135976761057E-8,0.653745309253861));
#55736=DIRECTION('center_axis',(0.570805684013776,0.584827969931209,0.576330735501505));
#55737=DIRECTION('ref_axis',(0.706903275138169,0.00704480135579719,-0.7072751447441));
#55738=DIRECTION('center_axis',(0.714172389847507,6.00847554702783E-10,
0.699969854764832));
#55739=DIRECTION('ref_axis',(-0.699883894318067,0.0156715280547506,0.714084685231805));
#55740=DIRECTION('',(-0.714172445802532,-1.48214773785851E-11,-0.699969797674464));
#55741=DIRECTION('',(0.997345804770064,-3.07809289803779E-8,-0.0728103406636272));
#55742=DIRECTION('center_axis',(0.388763513015119,0.793626260384467,-0.467996036069014));
#55743=DIRECTION('ref_axis',(-5.74087223566324E-17,0.507952836950267,0.861384882287921));
#55744=DIRECTION('center_axis',(0.0930250935242046,0.471546674524122,0.876920786456824));
#55745=DIRECTION('ref_axis',(0.867787458195339,0.393407974295759,-0.303603513088007));
#55746=DIRECTION('center_axis',(-0.607215611590486,-0.601098528053039,-0.519586143592438));
#55747=DIRECTION('ref_axis',(0.651451115212137,-0.00227571932839452,-0.758687198778523));
#55748=DIRECTION('',(-0.0100427887997432,5.1950067792211E-12,-0.999949569924966));
#55749=DIRECTION('center_axis',(0.,-1.,1.45983193964168E-32));
#55750=DIRECTION('ref_axis',(1.,0.,0.));
#55751=DIRECTION('center_axis',(0.609429829516059,0.60109852762544,0.516987275455166));
#55752=DIRECTION('ref_axis',(0.649374219434502,-0.00432804735943733,-0.760456699056485));
#55753=DIRECTION('center_axis',(0.602265607328405,-0.601098528165844,0.525315807554088));
#55754=DIRECTION('ref_axis',(0.655445521675757,-0.00330181187803222,-0.755235238951094));
#55755=DIRECTION('center_axis',(-0.600015883320388,0.601098527900785,-0.527883983010249));
#55756=DIRECTION('ref_axis',(0.65866598479739,-0.00330187161489854,-0.752428214592411));
#55757=DIRECTION('center_axis',(0.659667413981856,0.584828255987001,0.472032640746055));
#55758=DIRECTION('ref_axis',(0.600837632351962,-0.0330815410883527,-0.798686265807112));
#55759=DIRECTION('center_axis',(-0.796291055960073,-1.07988306620361E-7,
-0.604913674996673));
#55760=DIRECTION('ref_axis',(-0.604839352186181,-0.0156751635314749,0.796193222336929));
#55761=DIRECTION('',(0.796270460894843,0.,0.604940784793284));
#55762=DIRECTION('center_axis',(0.63853657013902,0.584827952226448,0.500247253755297));
#55763=DIRECTION('ref_axis',(0.629383034937091,-0.0227607295813455,-0.776761832560214));
#55764=DIRECTION('center_axis',(0.756714603597912,6.23929002742358E-10,
0.653745369927508));
#55765=DIRECTION('ref_axis',(-0.653664861953803,0.0156933905085894,0.756621415069162));
#55766=DIRECTION('',(-0.756714656868878,-2.20379270384426E-11,-0.653745308266007));
#55767=DIRECTION('',(0.99080597370102,0.,-0.135290511412935));
#55768=DIRECTION('center_axis',(-0.667548948507381,-0.601098528036872,-0.439384752737956));
#55769=DIRECTION('ref_axis',(0.569750879323193,-0.0324816860210763,-0.821175301372172));
#55770=DIRECTION('',(-0.0728103246472255,8.1518485824278E-12,-0.997345805939327));
#55771=DIRECTION('center_axis',(0.,-1.,1.45983193964168E-32));
#55772=DIRECTION('ref_axis',(1.,0.,0.));
#55773=DIRECTION('center_axis',(0.669419994709514,0.601098523566272,0.436528848587996));
#55774=DIRECTION('ref_axis',(0.567474345638155,-0.0345385482279327,-0.822666369635258));
#55775=DIRECTION('center_axis',(0.602265611301596,-0.601098530053937,0.525315800838421));
#55776=DIRECTION('ref_axis',(0.637750242713869,-0.0335099703073872,-0.769513943868725));
#55777=DIRECTION('center_axis',(-0.600015867092371,0.601098525646047,-0.527884004023175));
#55778=DIRECTION('ref_axis',(0.64103188687302,-0.0335100506535652,-0.76678236581002));
#55779=DIRECTION('',(0.832683749192558,0.,0.553748836414691));
#55780=DIRECTION('center_axis',(0.696199125316928,0.584827952146109,0.416272800332345));
#55781=DIRECTION('ref_axis',(0.544685151561283,-0.0526562728459283,-0.83698590346471));
#55782=DIRECTION('center_axis',(0.796270393925419,8.30266888503259E-10,
0.604940872943678));
#55783=DIRECTION('ref_axis',(-0.604865617402429,0.0157729998155413,0.796171336686519));
#55784=DIRECTION('',(-0.796270460895877,-1.756927936244E-10,-0.604940784791923));
#55785=DIRECTION('',(0.980355882941038,0.,-0.197236768334149));
#55786=DIRECTION('',(-0.135290511379306,6.51326541667664E-11,-0.990805973705612));
#55787=DIRECTION('center_axis',(0.,-1.,1.45983193964168E-32));
#55788=DIRECTION('ref_axis',(1.,0.,0.));
#55789=DIRECTION('center_axis',(0.614398707753774,0.601098534286894,0.511072186670964));
#55790=DIRECTION('ref_axis',(0.608400425199828,0.0514849269706017,-0.791958474234287));
#55791=DIRECTION('center_axis',(-0.708911379310895,0.601098534382717,-0.368951498501462));
#55792=DIRECTION('ref_axis',(0.495706492384409,0.0525165223579738,-0.866900852628125));
#55793=DIRECTION('center_axis',(0.664204276505397,0.584827930051153,0.465627502735853));
#55794=DIRECTION('ref_axis',(0.560854097273766,0.0219594825688793,-0.827623382159141));
#55795=DIRECTION('center_axis',(-0.865812541374247,-9.56935734198916E-9,
-0.500368507401363));
#55796=DIRECTION('ref_axis',(-0.500306527662049,-0.0157391393472365,0.865705295046387));
#55797=DIRECTION('',(0.86581081514902,0.,0.500371494362928));
#55798=DIRECTION('center_axis',(0.643342272591299,0.584827952319625,0.494051603056501));
#55799=DIRECTION('ref_axis',(0.590127077899819,0.032283433074407,-0.806664621685091));
#55800=DIRECTION('center_axis',(0.832683701355471,6.47954253504361E-10,
0.553748908348317));
#55801=DIRECTION('ref_axis',(-0.553680639279151,0.0157020800829031,0.832581043723973));
#55802=DIRECTION('',(-0.832683749192111,-3.88578058618584E-13,-0.553748836415365));
#55803=DIRECTION('',(0.966036775392978,0.,-0.258404621840121));
#55804=DIRECTION('center_axis',(-0.671764981849494,-0.601098528105988,-0.432911502122043));
#55805=DIRECTION('ref_axis',(0.526754692134173,0.0232723694222049,-0.849698706092995));
#55806=DIRECTION('',(-0.197236768334325,0.,-0.980355882941002));
#55807=DIRECTION('center_axis',(0.,-1.,1.45983193964168E-32));
#55808=DIRECTION('ref_axis',(1.,0.,0.));
#55809=DIRECTION('center_axis',(0.67360832555935,0.601098530772093,0.430037649561942));
#55810=DIRECTION('ref_axis',(0.524460705381175,0.0212180654376879,-0.851170231040867));
#55811=DIRECTION('center_axis',(0.710481175414537,-0.601098526313104,0.365919473444354));
#55812=DIRECTION('ref_axis',(0.472568976800901,0.0222452543572108,-0.881012889136097));
#55813=DIRECTION('center_axis',(-0.708911410112214,0.601098529398319,-0.368951447439755));
#55814=DIRECTION('ref_axis',(0.476328470483819,0.0222451729067309,-0.87898597286242));
#55815=DIRECTION('center_axis',(0.717325835414934,0.584827953016227,0.378708213823145));
#55816=DIRECTION('ref_axis',(0.471854812187027,-0.00784645565919282,-0.881641349614192));
#55817=DIRECTION('center_axis',(-0.895521107072002,-1.4892603257905E-9,
-0.445019040928066));
#55818=DIRECTION('ref_axis',(-0.444964345834529,-0.0156778483098858,0.895411043045831));
#55819=DIRECTION('',(0.895520921369927,0.,0.445019414620034));
#55820=DIRECTION('center_axis',(0.700190411309518,0.584827952254178,0.409523691832833));
#55821=DIRECTION('ref_axis',(0.503329007620302,0.00246180457570976,-0.864091343323259));
#55822=DIRECTION('center_axis',(0.865810773374916,6.35123262430197E-10,
0.500371566646158));
#55823=DIRECTION('ref_axis',(-0.500310124231316,0.0156707406190989,0.865704457352562));
#55824=DIRECTION('',(-0.865810815149511,-6.37823127617821E-11,-0.500371494362078));
#55825=DIRECTION('',(0.947905162032825,1.64268989065083E-13,-0.31855267035692));
#55826=DIRECTION('center_axis',(-0.720726111162175,-0.601098528053417,-0.345303391615352));
#55827=DIRECTION('ref_axis',(0.436752287053821,-0.00691952365102899,-0.899555201166498));
#55828=DIRECTION('',(-0.25840462182816,2.3449398189435E-11,-0.966036775396178));
#55829=DIRECTION('center_axis',(0.,-1.,1.45983193964168E-32));
#55830=DIRECTION('ref_axis',(1.,0.,0.));
#55831=DIRECTION('center_axis',(0.722194739844622,0.601098526879159,0.342221154700384));
#55832=DIRECTION('ref_axis',(0.434289405563679,-0.00897208007322183,-0.900728712762231));
#55833=DIRECTION('center_axis',(0.710481170796042,-0.601098528513992,0.365919478796359));
#55834=DIRECTION('ref_axis',(0.452535854473705,-0.00794570338777936,-0.891710808622071));
#55835=DIRECTION('center_axis',(-0.708911406887304,0.601098527487534,-0.368951456749235));
#55836=DIRECTION('ref_axis',(0.456341234740237,-0.00794578655635072,-0.889769375710221));
#55837=DIRECTION('center_axis',(0.759134269518841,0.5848279522295,0.285817121833429));
#55838=DIRECTION('ref_axis',(0.364518576884325,-0.0181546317168159,-0.931019127866583));
#55839=DIRECTION('center_axis',(-0.921696778591536,7.48645501603821E-10,
-0.387911134583663));
#55840=DIRECTION('ref_axis',(-0.387863448283094,-0.015679506614589,0.921583473461992));
#55841=DIRECTION('',(0.921696814384977,2.06171049564735E-7,0.387911049536543));
#55842=DIRECTION('center_axis',(0.745998677573766,0.584827782536733,0.318531690466364));
#55843=DIRECTION('ref_axis',(0.410602688348994,-0.0273551074101987,-0.91140393373035));
#55844=DIRECTION('center_axis',(0.895520876536056,6.75843163070039E-10,
0.445019504840063));
#55845=DIRECTION('ref_axis',(-0.444964638772521,0.0157023279262793,0.89541046852253));
#55846=DIRECTION('',(0.895520920882366,-1.29267412267966E-5,0.445019415413417));
#55847=DIRECTION('',(0.926032585062198,-7.62629077549361E-8,-0.377443573800134));
#55848=DIRECTION('center_axis',(-0.921696815639292,-2.06910887724944E-12,
-0.387911046556281));
#55849=DIRECTION('ref_axis',(-0.29941932269188,-0.635772805085085,0.711435878707968));
#55850=DIRECTION('',(0.318552670355559,0.,0.947905162033282));
#55851=DIRECTION('center_axis',(0.865032115867938,0.398564391594533,0.304739010088827));
#55852=DIRECTION('ref_axis',(-0.41846846945328,0.908231325199384,-2.63657958565185E-16));
#55853=DIRECTION('center_axis',(-0.94651552901007,5.74456447744061E-5,-0.322658255810672));
#55854=DIRECTION('ref_axis',(0.32265825482549,0.00036294994602284,-0.946515461500923));
#55855=DIRECTION('',(0.94423489092648,5.94973683407405E-5,0.329272633568477));
#55856=DIRECTION('center_axis',(0.73818326248297,0.590180063806695,0.326761324631792));
#55857=DIRECTION('ref_axis',(0.599945994337841,-0.79582265730166,0.082043293469382));
#55858=DIRECTION('center_axis',(0.581190950280199,0.550037558025492,-0.599729742528877));
#55859=DIRECTION('ref_axis',(-0.718118878872167,-8.71609914090751E-16,-0.695920452212307));
#55860=DIRECTION('center_axis',(0.382167621345336,-0.47712609034057,0.791390297584934));
#55861=DIRECTION('ref_axis',(0.917974674576926,0.0976286238898018,-0.384436143764828));
#55862=DIRECTION('center_axis',(0.439584257719342,0.584827951389649,0.681719845419452));
#55863=DIRECTION('ref_axis',(0.829605250079619,0.0265489690027765,-0.557718819195858));
#55864=DIRECTION('center_axis',(-0.620811502736929,-1.44144189845694E-11,
-0.783959870190762));
#55865=DIRECTION('ref_axis',(-0.783862656209556,-0.0157477670553342,0.620734519769016));
#55866=DIRECTION('center_axis',(0.577812722908943,-0.000115441210598508,
0.816169372077806));
#55867=DIRECTION('ref_axis',(0.0202499730413635,-0.999690122184594,-0.0144775066353077));
#55868=DIRECTION('',(-0.570361227482914,-6.06570349238548E-10,-0.821393979880656));
#55869=DIRECTION('center_axis',(-0.458922997514026,-0.601098527969961,-0.654270771183528));
#55870=DIRECTION('ref_axis',(0.806122937243544,0.0279220146409949,-0.591088970585841));
#55871=DIRECTION('',(0.177506961644642,2.24206636476394E-10,-0.984119544856054));
#55872=DIRECTION('center_axis',(0.,-1.,1.45983193964168E-32));
#55873=DIRECTION('ref_axis',(1.,0.,0.));
#55874=DIRECTION('center_axis',(0.461713971852301,0.601098531247332,0.652304195853954));
#55875=DIRECTION('ref_axis',(0.804554112791792,0.0258667804468661,-0.593315758478675));
#55876=DIRECTION('center_axis',(0.531677054547471,-0.601098525820599,0.596657415879521));
#55877=DIRECTION('ref_axis',(0.759626622235968,0.0268944251012258,-0.649803112249278));
#55878=DIRECTION('center_axis',(-0.529123173962527,0.601098529180198,-0.598923388250304));
#55879=DIRECTION('ref_axis',(0.762395730785078,0.0268943517741113,-0.646551965060301));
#55880=DIRECTION('center_axis',(0.521560170384467,0.584827952222769,0.621249752488843));
#55881=DIRECTION('ref_axis',(0.767386664097426,-0.0032619714661072,-0.641176315304596));
#55882=DIRECTION('center_axis',(-0.668811782515035,-6.34029621191083E-10,
-0.743431771966373));
#55883=DIRECTION('ref_axis',(-0.743340337842035,-0.015683219631839,0.668729525861441));
#55884=DIRECTION('',(0.668811721396846,8.32135976761153E-8,0.743431826949977));
#55885=DIRECTION('center_axis',(0.494071316040898,0.584827969931514,0.64332711760923));
#55886=DIRECTION('ref_axis',(0.789974212569877,0.00704480134113012,-0.613099595700948));
#55887=DIRECTION('center_axis',(0.620811451437247,5.06106120414513E-10,
0.783959910814564));
#55888=DIRECTION('ref_axis',(-0.783863635888522,0.0156715280540463,0.620735212099393));
#55889=DIRECTION('',(-0.620811504614948,-1.44328993199751E-11,-0.783959868703574));
#55890=DIRECTION('',(0.998606990639008,-3.07809289803829E-8,0.0527643653131774));
#55891=DIRECTION('center_axis',(0.444353453097782,0.793626260382252,-0.415580759361835));
#55892=DIRECTION('ref_axis',(-0.872542221931706,0.488538709772809,-1.67697309061468E-16));
#55893=DIRECTION('center_axis',(-0.0176157550387083,0.471546674599121,0.881665139862594));
#55894=DIRECTION('ref_axis',(0.898991141509732,0.393417286499192,-0.192451984065224));
#55895=DIRECTION('center_axis',(-0.537306120944992,-0.601098528063561,-0.591593350161127));
#55896=DIRECTION('ref_axis',(0.741402950424546,-0.00227571714743173,-0.671056246683722));
#55897=DIRECTION('',(0.115363314589441,5.0512714137876E-12,-0.993323364089931));
#55898=DIRECTION('center_axis',(0.,-1.,1.45983193964168E-32));
#55899=DIRECTION('ref_axis',(1.,0.,0.));
#55900=DIRECTION('center_axis',(0.539828601331174,0.601098527651807,0.589292492095104));
#55901=DIRECTION('ref_axis',(0.739564210493411,-0.00432804329610699,-0.673072096137171));
#55902=DIRECTION('center_axis',(0.531677029917933,-0.601098528156719,0.596657435473213));
#55903=DIRECTION('ref_axis',(0.744933215704376,-0.00330181543041807,-0.667130873333862));
#55904=DIRECTION('center_axis',(-0.529123179217502,0.601098527932195,-0.598923384860293));
#55905=DIRECTION('ref_axis',(0.747776463056216,-0.00330186607709241,-0.663942361187735));
#55906=DIRECTION('center_axis',(0.595310752812087,0.584827952238646,0.550982190153782));
#55907=DIRECTION('ref_axis',(0.696196315803167,-0.0330869090691157,-0.717088520554017));
#55908=DIRECTION('center_axis',(-0.714172494850206,-5.48807989469595E-10,
-0.69996974763159));
#55909=DIRECTION('ref_axis',(-0.699883747222762,-0.0156751701944172,0.714084749461015));
#55910=DIRECTION('',(0.714172445802503,3.88578058618675E-13,0.699969797674493));
#55911=DIRECTION('center_axis',(0.570803912686522,0.584827952226004,0.576332507808553));
#55912=DIRECTION('ref_axis',(0.721774233887805,-0.022760729597555,-0.691754222599226));
#55913=DIRECTION('center_axis',(0.668811671170596,5.24710583738528E-10,
0.743431872134895));
#55914=DIRECTION('ref_axis',(-0.743340319370965,0.0156933905087981,0.668729307785901));
#55915=DIRECTION('',(-0.668811722367453,-2.20379270384528E-11,-0.743431826076797));
#55916=DIRECTION('',(0.999949569924938,0.,-0.0100427888024681));
#55917=DIRECTION('center_axis',(-0.607215610045583,-0.601098528222621,-0.519586145201708));
#55918=DIRECTION('ref_axis',(0.668178782739805,-0.032481682628503,-0.743291365878801));
#55919=DIRECTION('',(0.0527643813501149,8.17238220606147E-12,-0.99860698979165));
#55920=DIRECTION('center_axis',(0.,-1.,1.45983193964168E-32));
#55921=DIRECTION('ref_axis',(1.,0.,0.));
#55922=DIRECTION('center_axis',(0.609429841859766,0.601098523778736,0.516987265376823));
#55923=DIRECTION('ref_axis',(0.666107080935483,-0.034538544519953,-0.745056001700579));
#55924=DIRECTION('center_axis',(0.531677035164203,-0.601098529878237,0.596657429063969));
#55925=DIRECTION('ref_axis',(0.729167065292789,-0.0335099735574638,-0.683514793230169));
#55926=DIRECTION('center_axis',(-0.529123151656913,0.601098525557496,-0.598923411592216));
#55927=DIRECTION('ref_axis',(0.732080473725266,-0.0335100522421239,-0.680393457044467));
#55928=DIRECTION('',(0.756714656868998,7.7715611723784E-13,0.653745308265868));
#55929=DIRECTION('center_axis',(0.638536571144397,0.584827952147131,0.500247252564718));
#55930=DIRECTION('ref_axis',(0.645292296194971,-0.0526562728331614,-0.762118868289417));
#55931=DIRECTION('center_axis',(0.714172398215871,4.92767641735136E-10,
0.699969846226673));
#55932=DIRECTION('ref_axis',(-0.699882768933784,0.0157729998150548,0.714083554093227));
#55933=DIRECTION('',(-0.714172445804273,-1.76525460892683E-10,-0.699969797672688));
#55934=DIRECTION('',(0.997345805939024,-1.43735365432053E-13,-0.0728103246513699));
#55935=DIRECTION('',(-0.0100427887682085,6.51326541667426E-11,-0.999949569925282));
#55936=DIRECTION('center_axis',(0.,-1.,1.45983193964168E-32));
#55937=DIRECTION('ref_axis',(1.,0.,0.));
#55938=DIRECTION('center_axis',(0.545499654375564,0.601098533820789,0.584046812947933));
#55939=DIRECTION('ref_axis',(0.70286172745956,0.0514849323635992,-0.709460847272123));
#55940=DIRECTION('center_axis',(-0.657079521879776,0.601098533955509,-0.454892354742068));
#55941=DIRECTION('ref_axis',(0.60044918033672,0.0525165272278878,-0.79793658657871));
#55942=DIRECTION('center_axis',(0.600608226843436,0.584827930051093,0.545202760521384));
#55943=DIRECTION('ref_axis',(0.660160309856493,0.0219594825681387,-0.750803667023223));
#55944=DIRECTION('center_axis',(-0.796272568887257,-9.84282189124006E-9,
-0.604938010078462));
#55945=DIRECTION('ref_axis',(-0.604863077538847,-0.0157391393470823,0.796173936349871));
#55946=DIRECTION('',(0.796270460894685,1.22124532708776E-12,0.604940784793492));
#55947=DIRECTION('center_axis',(0.576348241675388,0.584827952320947,0.570788025892079));
#55948=DIRECTION('ref_axis',(0.686575635049832,0.0322834330574119,-0.72634129533295));
#55949=DIRECTION('center_axis',(0.756714599701,6.55778036687605E-10,0.653745374438211));
#55950=DIRECTION('ref_axis',(-0.653664777278155,0.015702080080864,0.756621307938809));
#55951=DIRECTION('',(-0.756714656868477,-3.88578058618553E-13,-0.653745308266471));
#55952=DIRECTION('',(0.990805973700973,0.,-0.135290511413283));
#55953=DIRECTION('center_axis',(-0.612209713153376,-0.601098528006665,-0.513692346398972));
#55954=DIRECTION('ref_axis',(0.629096563127882,0.0232723720554988,-0.776978706889447));
#55955=DIRECTION('',(-0.0728103246514208,0.,-0.997345805939021));
#55956=DIRECTION('center_axis',(0.,-1.,1.45983193964168E-32));
#55957=DIRECTION('ref_axis',(1.,0.,0.));
#55958=DIRECTION('center_axis',(0.614398710488254,0.601098530667225,0.511072187640919));
#55959=DIRECTION('ref_axis',(0.627005096438769,0.0212180683557757,-0.778726140960389));
#55960=DIRECTION('center_axis',(0.659016935312657,-0.601098526825138,0.452081010461357));
#55961=DIRECTION('ref_axis',(0.579262838249883,0.0222452408855797,-0.814837231280354));
#55962=DIRECTION('center_axis',(-0.657079561225306,0.601098529124045,-0.454892304292861));
#55963=DIRECTION('ref_axis',(0.582738624272725,0.0222451803996117,-0.812355124148128));
#55964=DIRECTION('center_axis',(0.664204681256843,0.584827954381872,0.465626894809578));
#55965=DIRECTION('ref_axis',(0.578633172815619,-0.00784635391407085,-0.815550173838241));
#55966=DIRECTION('center_axis',(-0.832684316109069,-3.23656056986375E-9,
-0.553747983929488));
#55967=DIRECTION('ref_axis',(-0.553679925483015,-0.0156778481997066,0.832581975058882));
#55968=DIRECTION('',(0.832683749192755,3.88578058619072E-13,0.553748836414396));
#55969=DIRECTION('center_axis',(0.643342272241462,0.584827952253614,0.49405160359019));
#55970=DIRECTION('ref_axis',(0.60765947023258,0.00246180459506116,-0.794193872901823));
#55971=DIRECTION('center_axis',(0.796270420373333,5.05988671369472E-10,
0.604940838130867));
#55972=DIRECTION('ref_axis',(-0.604866555276953,0.0156707406197974,0.79617264346109));
#55973=DIRECTION('',(-0.796270460895025,-6.37823127617811E-11,-0.604940784793044));
#55974=DIRECTION('',(0.980355882941001,1.6426898906513E-13,-0.197236768334329));
#55975=DIRECTION('center_axis',(-0.671764980350506,-0.601098528045241,-0.432911504532425));
#55976=DIRECTION('ref_axis',(0.54605252636692,-0.00691952417752918,-0.837722363694238));
#55977=DIRECTION('',(-0.135290511400882,2.34493981894302E-11,-0.990805973702666));
#55978=DIRECTION('center_axis',(0.,-1.,1.45983193964168E-32));
#55979=DIRECTION('ref_axis',(1.,0.,0.));
#55980=DIRECTION('center_axis',(0.673608335974524,0.601098526858151,0.430037638718511));
#55981=DIRECTION('ref_axis',(0.543756144444565,-0.00897208149114492,-0.839195303330814));
#55982=DIRECTION('center_axis',(0.659016940608251,-0.601098528480747,0.452081000540414));
#55983=DIRECTION('ref_axis',(0.56072847601211,-0.0079457060119668,-0.827961618642499));
#55984=DIRECTION('center_axis',(-0.657079549965281,0.601098527488736,-0.454892322718572));
#55985=DIRECTION('ref_axis',(0.564260520362422,-0.00794578617095023,-0.825558556156045));
#55986=DIRECTION('center_axis',(0.717325884976863,0.58482795222916,0.378708121161413));
#55987=DIRECTION('ref_axis',(0.478331876830556,-0.018154631720293,-0.877991472028549));
#55988=DIRECTION('center_axis',(-0.865810784279634,4.83825714184073E-10,
-0.500371547777334));
#55989=DIRECTION('ref_axis',(-0.500310036599232,-0.015679506613961,0.865704349273133));
#55990=DIRECTION('',(0.865810813532333,2.06171882231919E-7,0.500371497160298));
#55991=DIRECTION('center_axis',(0.700193648426392,0.584827782536454,0.409518399436254));
#55992=DIRECTION('ref_axis',(0.521594165603633,-0.0273551074133822,-0.85275507885128));
#55993=DIRECTION('center_axis',(0.832683694838208,6.55764680054239E-10,
0.55374891814846));
#55994=DIRECTION('ref_axis',(-0.55368064692291,0.0157023279256327,0.83258103396651));
#55995=DIRECTION('',(0.832683748609624,-1.29267411912356E-5,0.55374883714038));
#55996=DIRECTION('',(0.966036765128944,-7.62629077549575E-8,-0.258404660211845));
#55997=DIRECTION('center_axis',(-0.8658108151466,3.96258707532583E-12,-0.500371494367116));
#55998=DIRECTION('ref_axis',(-0.386224871060518,-0.635772805085263,0.668298802399273));
#55999=DIRECTION('',(0.197236768332891,0.,0.980355882941291));
#56000=DIRECTION('center_axis',(0.820017153734806,0.398564391592048,0.410753324192914));
#56001=DIRECTION('ref_axis',(0.447863103153179,1.17847903490295E-17,-0.894102142282415));
#56002=DIRECTION('center_axis',(-0.898612168819394,5.74456518964492E-5,
-0.438743850953722));
#56003=DIRECTION('ref_axis',(0.438743841501099,0.000363080670879633,-0.898612101920114));
#56004=DIRECTION('',(0.895520512892924,5.94973684117939E-5,0.445020232627751));
#56005=DIRECTION('center_axis',(0.691408413580748,0.590180063808505,0.416703609190925));
#56006=DIRECTION('ref_axis',(0.584935624845923,-0.795821655632749,0.156582908428919));
#56007=DIRECTION('center_axis',(0.651774153940385,0.550037558024768,-0.522158153261486));
#56008=DIRECTION('ref_axis',(-0.644941563429318,0.764231888736231,-6.88734724809203E-18));
#56009=DIRECTION('center_axis',(0.279966610551229,-0.477126090010582,0.833048252628664));
#56010=DIRECTION('ref_axis',(0.958919043818676,0.0976333725527449,-0.266349379510922));
#56011=DIRECTION('center_axis',(0.350675851921805,0.584827951388939,0.731438797270922));
#56012=DIRECTION('ref_axis',(0.892964267927599,0.0265489690139539,-0.449343931136078));
#56013=DIRECTION('center_axis',(-0.517659995335373,-4.43418987557268E-11,
-0.855586424173141));
#56014=DIRECTION('ref_axis',(-0.855480328228814,-0.0157477670572569,0.517595803543877));
#56015=DIRECTION('center_axis',(0.470963347117226,-0.00011544117072539,
0.882152771545539));
#56016=DIRECTION('ref_axis',(0.0218840739070157,-0.999690707186623,-0.0118142826249362));
#56017=DIRECTION('',(-0.46291579531665,-6.06514838086686E-10,-0.886402259951064));
#56018=DIRECTION('center_axis',(-0.373302379157644,-0.601098527901457,-0.706629955117914));
#56019=DIRECTION('ref_axis',(0.873849509997278,0.0279220160657003,-0.48539406145558));
#56020=DIRECTION('',(0.299450151003895,2.24350371841883E-10,-0.954111946819525));
#56021=DIRECTION('center_axis',(0.,-1.,1.45983193964168E-32));
#56022=DIRECTION('ref_axis',(1.,0.,0.));
#56023=DIRECTION('center_axis',(0.376317811527839,0.601098530834626,0.705028695129037));
#56024=DIRECTION('ref_axis',(0.872572151713197,0.0258667898253148,-0.487799906968763));
#56025=DIRECTION('center_axis',(0.452703617578686,-0.601098525867147,0.658589399270528));
#56026=DIRECTION('ref_axis',(0.835078665382949,0.02689442413629,-0.549472758717491));
#56027=DIRECTION('center_axis',(-0.449885876190126,0.601098529134951,-0.660517415876706));
#56028=DIRECTION('ref_axis',(0.837418460426783,0.0268943527820764,-0.545900188610399));
#56029=DIRECTION('center_axis',(0.439584272309975,0.584827952222484,0.681719835296705));
#56030=DIRECTION('ref_axis',(0.841696291935165,-0.00326197145329843,-0.539941396528208));
#56031=DIRECTION('center_axis',(-0.570361291815053,-6.14013338689065E-10,
-0.82139393520957));
#56032=DIRECTION('ref_axis',(-0.821292912578248,-0.0156832196307606,0.570291143514215));
#56033=DIRECTION('',(0.570361226402489,8.32143748320893E-8,0.82139398063088));
#56034=DIRECTION('center_axis',(0.409545148242126,0.584827969931487,0.700177846791193));
#56035=DIRECTION('ref_axis',(0.860586784780955,0.00704480134808137,-0.509255099762726));
#56036=DIRECTION('center_axis',(0.517659921081644,6.52385431013528E-10,
0.855586469099264));
#56037=DIRECTION('ref_axis',(-0.855481398007026,0.015671528054159,0.517596349361538));
#56038=DIRECTION('',(-0.517659995144111,-1.36557432027408E-11,-0.855586424288861));
#56039=DIRECTION('',(0.984119547726679,-3.07809289803933E-8,0.177506945729556));
#56040=DIRECTION('center_axis',(0.49293567378062,0.793626260380211,-0.356611525822383));
#56041=DIRECTION('ref_axis',(-0.849477030544143,0.527625600760525,2.24172534152986E-16));
#56042=DIRECTION('center_axis',(-0.127978792423019,0.471546674587275,0.872505107363635));
#56043=DIRECTION('ref_axis',(0.91601707681542,0.393429494163488,-0.078268436197456));
#56044=DIRECTION('center_axis',(-0.458923008330418,-0.6010985280139,-0.654270763556253));
#56045=DIRECTION('ref_axis',(0.819662408082402,-0.00227572752435393,-0.572842349901604));
#56046=DIRECTION('',(0.238950069593058,5.19500677922368E-12,-0.971031855420548));
#56047=DIRECTION('center_axis',(0.,-1.,1.45983193964168E-32));
#56048=DIRECTION('ref_axis',(1.,0.,0.));
#56049=DIRECTION('center_axis',(0.461713950440732,0.601098527686159,0.652304214291112));
#56050=DIRECTION('ref_axis',(0.818090832306808,-0.00432803772398581,-0.575072741646667));
#56051=DIRECTION('center_axis',(0.452703595008796,-0.601098528162513,0.658589412689706));
#56052=DIRECTION('ref_axis',(0.822672862713188,-0.00330181325403135,-0.568505460822079));
#56053=DIRECTION('center_axis',(-0.449885881652066,0.60109852793641,-0.660517413247239));
#56054=DIRECTION('ref_axis',(0.825094064654831,-0.00330186518387631,-0.564985736242674));
#56055=DIRECTION('center_axis',(0.521553004954773,0.584828255987234,0.621255482085734));
#56056=DIRECTION('ref_axis',(0.780586410597556,-0.0330815410821509,-0.624171825085092));
#56057=DIRECTION('center_axis',(-0.620838200118697,-1.08043366079622E-7,
-0.783938728009636));
#56058=DIRECTION('ref_axis',(-0.783842409954205,-0.015675163531732,0.620761923450076));
#56059=DIRECTION('',(0.620811504614969,0.,0.783959868703557));
#56060=DIRECTION('center_axis',(0.494069336524158,0.584827952226326,0.643328653956391));
#56061=DIRECTION('ref_axis',(0.802782622024964,-0.022760729591192,-0.595837235294338));
#56062=DIRECTION('center_axis',(0.57036116034183,6.26445488212079E-10,0.821394026502215));
#56063=DIRECTION('ref_axis',(-0.821292872789849,0.0156933905088762,0.570290921020959));
#56064=DIRECTION('',(-0.570361227475226,-2.2482016248264E-11,-0.821393979885994));
#56065=DIRECTION('',(0.993323364090225,0.,0.115363314586913));
#56066=DIRECTION('center_axis',(-0.537306125094688,-0.601098528082298,-0.591593346373188));
#56067=DIRECTION('ref_axis',(0.756069101559276,-0.0324816851659188,-0.653685286507301));
#56068=DIRECTION('',(0.177506961533666,8.17238220606035E-12,-0.984119544876071));
#56069=DIRECTION('center_axis',(0.,-1.,1.45983193964168E-32));
#56070=DIRECTION('ref_axis',(1.,0.,0.));
#56071=DIRECTION('center_axis',(0.539828616369953,0.60109852393486,0.589292482110059));
#56072=DIRECTION('ref_axis',(0.754234908019797,-0.0345385417563714,-0.655695655512305));
#56073=DIRECTION('center_axis',(0.452703592957575,-0.601098529677169,0.658589412717247));
#56074=DIRECTION('ref_axis',(0.809084487247631,-0.0335099773181815,-0.586736204708191));
#56075=DIRECTION('center_axis',(-0.449885864064448,0.601098526155993,-0.660517426846618));
#56076=DIRECTION('ref_axis',(0.811583704649522,-0.0335100416239802,-0.583274350076974));
#56077=DIRECTION('',(0.668811722367532,4.44089209849998E-13,0.743431826076726));
#56078=DIRECTION('center_axis',(0.570803913820623,0.584827952146655,0.576332506765851));
#56079=DIRECTION('ref_axis',(0.735722795817769,-0.0526562728388038,-0.675232763308188));
#56080=DIRECTION('center_axis',(0.620811434513497,6.62050482000029E-10,
0.783959924216343));
#56081=DIRECTION('ref_axis',(-0.783862398432757,0.0157729998141104,0.620734204631991));
#56082=DIRECTION('',(-0.620811504616735,-1.75748304775537E-10,-0.783959868702159));
#56083=DIRECTION('',(0.998606989791864,-1.43735365432102E-13,0.0527643813460516));
#56084=DIRECTION('',(0.11536331462071,6.51326541667568E-11,-0.9933233640863));
#56085=DIRECTION('center_axis',(0.,-1.,1.45983193964168E-32));
#56086=DIRECTION('ref_axis',(1.,0.,0.));
#56087=DIRECTION('center_axis',(0.467997749689556,0.601098533729295,0.647810666039086));
#56088=DIRECTION('ref_axis',(0.786238475690617,0.0514849334007102,-0.61577460241262));
#56089=DIRECTION('center_axis',(-0.594885124104481,0.601098533936693,-0.533659293574426));
#56090=DIRECTION('ref_axis',(0.695722431559084,0.0525165274531211,-0.716388381096303));
#56091=DIRECTION('center_axis',(0.527540226646797,0.584827930050718,0.616179845095601));
#56092=DIRECTION('ref_axis',(0.749055400000351,0.0219594825766691,-0.662143329540727));
#56093=DIRECTION('center_axis',(-0.714174894398227,-9.94930068197513E-9,
-0.699967299387108));
#56094=DIRECTION('ref_axis',(-0.699880595778083,-0.0157391393488182,0.714086431145329));
#56095=DIRECTION('',(0.714172445802415,0.,0.699969797674583));
#56096=DIRECTION('center_axis',(0.500264854672132,0.584827952320526,0.638522780615109));
#56097=DIRECTION('ref_axis',(0.772196484316485,0.0322834330620383,-0.634563132839428));
#56098=DIRECTION('center_axis',(0.668811663491213,5.91155253666298E-10,
0.743431879043478));
#56099=DIRECTION('ref_axis',(-0.743340224857858,0.0157020800830934,0.668729208865093));
#56100=DIRECTION('',(-0.668811722367217,0.,-0.743431826077009));
#56101=DIRECTION('',(0.999949569924937,0.,-0.010042788802629));
#56102=DIRECTION('center_axis',(-0.542999537080384,-0.601098528106974,-0.586371948713543));
#56103=DIRECTION('ref_axis',(0.721517200158609,0.0232723693894611,-0.692005293836892));
#56104=DIRECTION('',(0.0527643813459379,1.43735365432659E-13,-0.99860698979187));
#56105=DIRECTION('center_axis',(0.,-1.,1.45983193964168E-32));
#56106=DIRECTION('ref_axis',(1.,0.,0.));
#56107=DIRECTION('center_axis',(0.545499660483158,0.601098530583077,0.584046810575681));
#56108=DIRECTION('ref_axis',(0.719661241409237,0.0212180706883322,-0.694001074271201));
#56109=DIRECTION('center_axis',(0.597159614763651,-0.601098526838636,0.531112940463467));
#56110=DIRECTION('ref_axis',(0.67682136303877,0.0222452406144092,-0.73581111149829));
#56111=DIRECTION('center_axis',(-0.594885168938924,0.601098529130676,-0.533659249009558));
#56112=DIRECTION('ref_axis',(0.679958650910506,0.0222451801649955,-0.732912945042855));
#56113=DIRECTION('center_axis',(0.600608822281924,0.584827953016299,0.545202079937235));
#56114=DIRECTION('ref_axis',(0.676285913318753,-0.00784645567689399,-0.736597445406872));
#56115=DIRECTION('center_axis',(-0.756714879539488,-8.8798175969817E-10,
-0.653745050523167));
#56116=DIRECTION('ref_axis',(-0.653664701966337,-0.0156778483084326,0.756621875493748));
#56117=DIRECTION('',(0.756714656869119,8.32667268468655E-13,0.653745308265727));
#56118=DIRECTION('center_axis',(0.576348241262515,0.584827952254101,0.570788026377464));
#56119=DIRECTION('ref_axis',(0.702406779961722,0.00246180457781366,-0.71177149070613));
#56120=DIRECTION('center_axis',(0.714172377412268,7.46039727085603E-10,
0.699969867452385));
#56121=DIRECTION('ref_axis',(-0.699883915644385,0.0156707406188272,0.71408468161048));
#56122=DIRECTION('',(-0.714172445803038,-6.33937347031602E-11,-0.699969797673947));
#56123=DIRECTION('',(0.99734580593901,1.64268989065177E-13,-0.0728103246515634));
#56124=DIRECTION('center_axis',(-0.612209711118165,-0.60109852808043,-0.513692348738184));
#56125=DIRECTION('ref_axis',(0.646741194614692,-0.00691952138882007,-0.762678141428028));
#56126=DIRECTION('',(-0.0100427887902123,2.36136671784991E-11,-0.999949569925061));
#56127=DIRECTION('center_axis',(0.,-1.,1.45983193964168E-32));
#56128=DIRECTION('ref_axis',(1.,0.,0.));
#56129=DIRECTION('center_axis',(0.614398716792201,0.601098526967397,0.511072184414025));
#56130=DIRECTION('ref_axis',(0.644647533842544,-0.0089720736175879,-0.764427275158158));
#56131=DIRECTION('center_axis',(0.597159621283849,-0.601098528479525,0.531112931275336));
#56132=DIRECTION('ref_axis',(0.660078071675325,-0.00794570627140616,-0.751154980709862));
#56133=DIRECTION('center_axis',(-0.594885156756865,0.601098527501109,-0.533659264424743));
#56134=DIRECTION('ref_axis',(0.663281080036902,-0.00794578523321746,-0.748328185599145));
#56135=DIRECTION('center_axis',(0.66420484270576,0.584827952229765,0.465626667209855));
#56136=DIRECTION('ref_axis',(0.584601597354615,-0.0181546317097263,-0.811117366179467));
#56137=DIRECTION('center_axis',(-0.796270496767386,-4.64388117108289E-10,
-0.60494073757503));
#56138=DIRECTION('ref_axis',(-0.604866371587384,-0.0156795066172821,0.796172610427508));
#56139=DIRECTION('',(0.796270458939758,2.0617116058701E-7,0.604940787366685));
#56140=DIRECTION('center_axis',(0.64334614715523,0.584827782537056,0.494046758630508));
#56141=DIRECTION('ref_axis',(0.624359791296606,-0.0273551074042075,-0.780657766957431));
#56142=DIRECTION('center_axis',(0.756714577676916,8.3606101144566E-10,0.653745399931233));
#56143=DIRECTION('ref_axis',(-0.653664800225672,0.0157023279260372,0.756621282970308));
#56144=DIRECTION('',(0.756714656200049,-1.29267412622836E-5,0.653745308912378));
#56145=DIRECTION('',(0.990805968327137,-7.62630514903484E-8,-0.135290550768773));
#56146=DIRECTION('center_axis',(-0.796270460895142,-8.75589444335316E-13,
-0.604940784792891));
#56147=DIRECTION('ref_axis',(-0.466939422478211,-0.635772805085266,0.614622254762815));
#56148=DIRECTION('',(0.0728103246501242,-3.74249790574711E-13,0.997345805939115));
#56149=DIRECTION('center_axis',(0.762070031231707,0.398564391593391,0.510289813000706));
#56150=DIRECTION('ref_axis',(0.556392281443257,2.67730606825651E-16,-0.830919748923064));
#56151=DIRECTION('center_axis',(-0.836537157930299,5.74456560985943E-5,
-0.547910193464124));
#56152=DIRECTION('ref_axis',(0.547910175674295,0.000363259836001831,-0.836537092683196));
#56153=DIRECTION('',(0.832683241412888,5.94973691578637E-5,0.553749596776548));
#56154=DIRECTION('center_axis',(0.63372964100381,0.59018006381091,0.500074228883405));
#56155=DIRECTION('ref_axis',(0.560701812787564,-0.795820734737636,0.228654401441101));
#56156=DIRECTION('center_axis',(0.712078489846112,0.550037558019866,-0.43635181799326));
#56157=DIRECTION('ref_axis',(-0.611304898368902,0.791395173873449,5.31197026603917E-16));
#56158=DIRECTION('center_axis',(0.173350359018707,-0.477126089715379,0.861568539084963));
#56159=DIRECTION('ref_axis',(0.984740254929913,0.0976251248572319,-0.144069307339142));
#56160=DIRECTION('center_axis',(0.256237078464303,0.584827951388878,0.769622522340898));
#56161=DIRECTION('ref_axis',(0.942240705833203,0.0265489690180492,-0.333882620864018));
#56162=DIRECTION('center_axis',(-0.406344674439861,1.212629090089E-11,-0.913719872583695));
#56163=DIRECTION('ref_axis',(-0.913606567872938,-0.0157477670558653,0.406294286167287));
#56164=DIRECTION('center_axis',(0.356686603111286,-0.000115441196879581,
0.934224091872107));
#56165=DIRECTION('ref_axis',(0.023208648645243,-0.999690269928019,-0.0089845889892695));
#56166=DIRECTION('',(-0.348169904526061,-6.0695892729679E-10,-0.937431446870817));
#56167=DIRECTION('center_axis',(-0.281794560966275,-0.601098527898774,-0.74784516122507));
#56168=DIRECTION('ref_axis',(0.927794952947662,0.0279220162086369,-0.372044199384548));
#56169=DIRECTION('',(0.416670832599042,2.24206636476383E-10,-0.909057433422785));
#56170=DIRECTION('center_axis',(0.,-1.,1.45983193964168E-32));
#56171=DIRECTION('ref_axis',(1.,0.,0.));
#56172=DIRECTION('center_axis',(0.284986911706633,0.60109853096743,0.746634459574907));
#56173=DIRECTION('ref_axis',(0.926829197919476,0.0258667868113062,-0.374591173446464));
#56174=DIRECTION('center_axis',(0.366590771873736,-0.601098525971635,0.710135035082587));
#56175=DIRECTION('ref_axis',(0.89736101970089,0.0268944218182806,-0.440476889741606));
#56176=DIRECTION('center_axis',(-0.363553605776339,0.601098529201857,-0.711694691506397));
#56177=DIRECTION('ref_axis',(0.899234602532466,0.0268943512091051,-0.436639237221438));
#56178=DIRECTION('center_axis',(0.350675867701933,0.58482795222295,0.731438789038568));
#56179=DIRECTION('ref_axis',(0.90273186642539,-0.00326197146607218,-0.430191279412179));
#56180=DIRECTION('center_axis',(-0.462915866366431,-6.27932174290943E-10,
-0.886402222845936));
#56181=DIRECTION('ref_axis',(-0.886293204894859,-0.0156832196313113,0.462858932698934));
#56182=DIRECTION('',(0.462915794151349,8.32143748321858E-8,0.886402260559628));
#56183=DIRECTION('center_axis',(0.318560208828588,0.584827969931739,0.745986353049844));
#56184=DIRECTION('ref_axis',(0.917627389295675,0.00704480133904469,-0.397379346706013));
#56185=DIRECTION('center_axis',(0.406344605395894,5.99603447787589E-10,
0.91371990328856));
#56186=DIRECTION('ref_axis',(-0.913607693064028,0.015671528053928,0.406294703857532));
#56187=DIRECTION('',(-0.406344678315143,-1.44328993199831E-11,-0.9137198708603));
#56188=DIRECTION('',(0.954111951662165,-3.07809289804025E-8,0.29945013557421));
#56189=DIRECTION('center_axis',(0.533744004419719,0.793626260379228,-0.292018315491485));
#56190=DIRECTION('ref_axis',(-0.829794751143426,0.558068697361553,1.37353446782025E-17));
#56191=DIRECTION('center_axis',(-0.236323527865057,0.471546674606097,0.849585148084255));
#56192=DIRECTION('ref_axis',(0.918611650451755,0.393409545157626,0.0371694152923138));
#56193=DIRECTION('center_axis',(-0.373302383231254,-0.601098528046985,-0.70662995284209));
#56194=DIRECTION('ref_axis',(0.884995313294357,-0.00227572095771443,-0.465594369103779));
#56195=DIRECTION('',(0.358768439256913,5.19500677922131E-12,-0.933426594324995));
#56196=DIRECTION('center_axis',(0.,-1.,1.45983193964168E-32));
#56197=DIRECTION('ref_axis',(1.,0.,0.));
#56198=DIRECTION('center_axis',(0.376317791083764,0.60109852773164,0.705028708686882));
#56199=DIRECTION('ref_axis',(0.883715672465122,-0.00432803058542384,-0.468004143561539));
#56200=DIRECTION('center_axis',(0.366590750308916,-0.601098528165542,0.710135044357878));
#56201=DIRECTION('ref_axis',(0.887438469564525,-0.00330181390545426,-0.460914374653153));
#56202=DIRECTION('center_axis',(-0.363553611789512,0.601098527926897,-0.711694689511534));
#56203=DIRECTION('ref_axis',(0.889399441604279,-0.0033018665924906,-0.457118946173752));
#56204=DIRECTION('center_axis',(0.439576445276083,0.584828255987649,0.681724621644904));
#56205=DIRECTION('ref_axis',(0.852660726745465,-0.033081541071735,-0.521416624884761));
#56206=DIRECTION('center_axis',(-0.517689160600361,-1.08326166762735E-7,
-0.855568777478984));
#56207=DIRECTION('ref_axis',(-0.855463658918661,-0.0156751635317574,0.517625557249398));
#56208=DIRECTION('',(0.517659995144627,1.16573417585677E-12,0.855586424288549));
#56209=DIRECTION('center_axis',(0.409542991805253,0.584827952225948,0.700179122909564));
#56210=DIRECTION('ref_axis',(0.871130648640799,-0.0227607296020412,-0.490523538871116));
#56211=DIRECTION('center_axis',(0.462915725331666,6.03583660258034E-10,
0.886402296500104));
#56212=DIRECTION('ref_axis',(-0.886293137093757,0.0156933905088725,0.462858717790691));
#56213=DIRECTION('',(-0.462915795308633,-2.16493489798453E-11,-0.886402259955251));
#56214=DIRECTION('',(0.971031855421239,0.,0.238950069590253));
#56215=DIRECTION('center_axis',(-0.458923003741332,-0.601098527885463,-0.65427076689316));
#56216=DIRECTION('ref_axis',(0.832035758807123,-0.0324816887614031,-0.553770201402587));
#56217=DIRECTION('',(0.299450150896321,8.17238220605966E-12,-0.954111946853288));
#56218=DIRECTION('center_axis',(0.,-1.,1.45983193964168E-32));
#56219=DIRECTION('ref_axis',(1.,0.,0.));
#56220=DIRECTION('center_axis',(0.461713957455863,0.601098524618822,0.652304212152214));
#56221=DIRECTION('ref_axis',(0.830468006537055,-0.0345385296351385,-0.555994586384627));
#56222=DIRECTION('center_axis',(0.366590743436293,-0.601098529457339,0.71013504681226));
#56223=DIRECTION('ref_axis',(0.876242162608083,-0.0335099812939027,-0.48070443478461));
#56224=DIRECTION('center_axis',(-0.363553589130721,0.601098525939916,-0.711694702764487));
#56225=DIRECTION('ref_axis',(0.878287787393539,-0.0335100454515292,-0.476956643070623));
#56226=DIRECTION('',(0.570361227475854,8.32667268470211E-13,0.821393979885559));
#56227=DIRECTION('center_axis',(0.494069337780756,0.584827952146981,0.643328653063466));
#56228=DIRECTION('ref_axis',(0.814550507461375,-0.0526562728332638,-0.57769783427474));
#56229=DIRECTION('center_axis',(0.517659905315428,7.85228749101234E-10,
0.855586478638379));
#56230=DIRECTION('ref_axis',(-0.855480042403958,0.0157729998136923,0.517595507636417));
#56231=DIRECTION('',(-0.51765999514652,-1.76914038951223E-10,-0.855586424287404));
#56232=DIRECTION('',(0.984119544876793,-1.43735365432129E-13,0.177506961529667));
#56233=DIRECTION('',(0.23895006962348,6.51326541667397E-11,-0.971031855413062));
#56234=DIRECTION('center_axis',(0.,-1.,1.45983193964168E-32));
#56235=DIRECTION('ref_axis',(1.,0.,0.));
#56236=DIRECTION('center_axis',(0.383115227651307,0.601098532850742,0.701358165380836));
#56237=DIRECTION('ref_axis',(0.857215779016419,0.0514849435566238,-0.512377213381163));
#56238=DIRECTION('center_axis',(-0.523309027811023,0.601098534236298,-0.604010110470393));
#56239=DIRECTION('ref_axis',(0.780023727708288,0.0525165239653635,-0.62354229922489));
#56240=DIRECTION('center_axis',(0.446152601933338,0.584827930050342,0.677439405423942));
#56241=DIRECTION('ref_axis',(0.826137439021757,0.0219594825869006,-0.563040596201631));
#56242=DIRECTION('center_axis',(-0.620814224972045,-9.72756495102324E-9,
-0.783957714467023));
#56243=DIRECTION('ref_axis',(-0.783860607156331,-0.0157391393478925,0.620737326122004));
#56244=DIRECTION('',(0.620811504615245,1.165734175857E-12,0.783959868703339));
#56245=DIRECTION('center_axis',(0.416291992044271,0.584827952319077,0.696187649665008));
#56246=DIRECTION('ref_axis',(0.845639333746944,0.0322834330816786,-0.532777530652791));
#56247=DIRECTION('center_axis',(0.570361160563746,6.0878364447281E-10,0.82139402634812));
#56248=DIRECTION('ref_axis',(-0.82129276057823,0.0157020800819259,0.570290843432447));
#56249=DIRECTION('',(-0.57036122747518,-8.3266726846866E-13,-0.821393979886027));
#56250=DIRECTION('',(0.993323364090257,-1.64268989065282E-13,0.115363314586632));
#56251=DIRECTION('center_axis',(-0.465225930454903,-0.601098528085867,-0.649804119073874));
#56252=DIRECTION('ref_axis',(0.802559083046984,0.0232723699029421,-0.596118541078773));
#56253=DIRECTION('',(0.177506961529538,0.,-0.984119544876816));
#56254=DIRECTION('center_axis',(0.,-1.,1.45983193964168E-32));
#56255=DIRECTION('ref_axis',(1.,0.,0.));
#56256=DIRECTION('center_axis',(0.467997751365031,0.601098530417989,0.647810667901207));
#56257=DIRECTION('ref_axis',(0.800967899836253,0.0212180752187776,-0.598331193166387));
#56258=DIRECTION('center_axis',(0.52588472722959,-0.601098526940685,0.601768904627348));
#56259=DIRECTION('ref_axis',(0.763706012663099,0.0222452379388547,-0.645180808464786));
#56260=DIRECTION('center_axis',(-0.523309087003531,0.60109852899713,-0.604010064400435));
#56261=DIRECTION('ref_axis',(0.766455320034414,0.0222451837789128,-0.641912294779891));
#56262=DIRECTION('center_axis',(0.527540769866512,0.584827954381971,0.616179356926251));
#56263=DIRECTION('ref_axis',(0.763273428376044,-0.00784635390595337,-0.646027946969373));
#56264=DIRECTION('center_axis',(-0.66881247587959,-3.15689300772054E-9,
-0.743431148195859));
#56265=DIRECTION('ref_axis',(-0.743339776746405,-0.0156778481997067,0.668730275509066));
#56266=DIRECTION('',(0.668811722367582,4.44089209850169E-13,0.743431826076681));
#56267=DIRECTION('center_axis',(0.500264854202378,0.584827952253931,0.638522781044144));
#56268=DIRECTION('ref_axis',(0.786076715195562,0.00246180458149666,-0.618124046891526));
#56269=DIRECTION('center_axis',(0.620811458452108,4.4207282963584E-10,0.783959905259552));
#56270=DIRECTION('ref_axis',(-0.783863640008822,0.0156707406190849,0.620735226775933));
#56271=DIRECTION('',(-0.62081150461559,-6.42264019716283E-11,-0.783959868703066));
#56272=DIRECTION('',(0.998606989791871,1.64268989065234E-13,0.0527643813459203));
#56273=DIRECTION('center_axis',(-0.542999538349175,-0.601098528013067,-0.586371947634867));
#56274=DIRECTION('ref_axis',(0.737230359758982,-0.00691952691788106,-0.675606036678829));
#56275=DIRECTION('',(0.11536331459892,2.34493981894245E-11,-0.99332336408883));
#56276=DIRECTION('center_axis',(0.,-1.,1.45983193964168E-32));
#56277=DIRECTION('ref_axis',(1.,0.,0.));
#56278=DIRECTION('center_axis',(0.545499656932936,0.601098527119734,0.584046817456046));
#56279=DIRECTION('ref_axis',(0.735372447364012,-0.00897206298346596,-0.677603767509954));
#56280=DIRECTION('center_axis',(0.525884739928065,-0.601098528496697,0.601768891975896));
#56281=DIRECTION('ref_axis',(0.749017840375685,-0.00794570493064833,-0.662502181560257));
#56282=DIRECTION('center_axis',(-0.523309064580667,0.601098527455218,-0.604010085361889));
#56283=DIRECTION('ref_axis',(0.751841304520338,-0.00794578827969788,-0.659296228766531));
#56284=DIRECTION('center_axis',(0.600608893325141,0.584827952228797,0.545202002518902));
#56285=DIRECTION('ref_axis',(0.681651801426565,-0.0181546317332704,-0.731451454956888));
#56286=DIRECTION('center_axis',(-0.714172423332152,2.70738924708545E-10,
-0.699969820600775));
#56287=DIRECTION('ref_axis',(-0.699883772599899,-0.0156795066139273,0.714084629384835));
#56288=DIRECTION('',(0.714172443541394,2.06172326321031E-7,0.699969799981451));
#56289=DIRECTION('center_axis',(0.576352692844794,0.584827782536587,0.570783705289397));
#56290=DIRECTION('ref_axis',(0.71727889008742,-0.0273551074114228,-0.696249015750449));
#56291=DIRECTION('center_axis',(0.668811635346391,8.0403432168573E-10,0.743431904363329));
#56292=DIRECTION('ref_axis',(-0.743340247283272,0.0157023279256694,0.668729178118137));
#56293=DIRECTION('',(0.668811721622696,-1.29267412267558E-5,0.743431826634416));
#56294=DIRECTION('',(0.999949569526026,-7.62630514903833E-8,-0.0100428285213587));
#56295=DIRECTION('center_axis',(-0.714172446213903,-4.77179581778534E-10,
-0.699969797254746));
#56296=DIRECTION('ref_axis',(-0.540290059736212,-0.635772805082231,0.551252747537926));
#56297=DIRECTION('',(-0.0527643813476595,0.,0.998606989791779));
#56298=DIRECTION('center_axis',(0.692104609098264,0.398564391591702,0.601778726626387));
#56299=DIRECTION('ref_axis',(0.65614682108291,-1.14922775163484E-16,-0.754633254755442));
#56300=DIRECTION('center_axis',(-0.761269456311017,5.7445664986067E-5,-0.648435664956766));
#56301=DIRECTION('ref_axis',(0.648435639191338,0.000362937741181404,-0.761269393909093));
#56302=DIRECTION('',(0.75671405779511,5.94973691933618E-5,0.653745998989915));
#56303=DIRECTION('center_axis',(0.566056573281352,0.590180063806646,0.575558379428322));
#56304=DIRECTION('ref_axis',(0.527619938303713,-0.795821286109522,0.297129065019519));
#56305=DIRECTION('center_axis',(0.761152922591209,0.550037558015138,-0.343663953890433));
#56306=DIRECTION('ref_axis',(-0.585711678816273,0.810519481134305,-4.28907078704251E-17));
#56307=DIRECTION('center_axis',(0.0640002686815192,-0.477126090766273,0.876501374282316));
#56308=DIRECTION('ref_axis',(0.995031674671247,0.0976283473316997,-0.0195108225919653));
#56309=DIRECTION('center_axis',(0.157757293231697,0.584827951389322,0.795668840476977));
#56310=DIRECTION('ref_axis',(0.976657444935551,0.026548969009499,-0.213155782226273));
#56311=DIRECTION('center_axis',(-0.288621061342871,-1.43925814653302E-11,
-0.957443409789485));
#56312=DIRECTION('ref_axis',(-0.95732468319503,-0.0157477670566732,0.288585271242773));
#56313=DIRECTION('center_axis',(0.236784694176708,-0.000115441177377208,
0.971562141747494));
#56314=DIRECTION('ref_axis',(0.0241396323370541,-0.999690579295746,-0.00600198450246929));
#56315=DIRECTION('',(-0.227933166354412,-6.07014438448248E-10,-0.973676779879058));
#56316=DIRECTION('center_axis',(-0.185842674628182,-0.601098527904035,-0.77726640223198));
#56317=DIRECTION('ref_axis',(0.967108515123235,0.0279220160808943,-0.252826978374757));
#56318=DIRECTION('',(0.527320366257025,2.24206636476405E-10,-0.849666541256367));
#56319=DIRECTION('center_axis',(0.,-1.,1.45983193964168E-32));
#56320=DIRECTION('ref_axis',(1.,0.,0.));
#56321=DIRECTION('center_axis',(0.189161578622374,0.601098530555737,0.776465359006327));
#56322=DIRECTION('ref_axis',(0.966469598843853,0.0258667961724589,-0.255474897722603));
#56323=DIRECTION('center_axis',(0.274696560809731,-0.601098526354879,0.750481419552342));
#56324=DIRECTION('ref_axis',(0.945491456743476,0.0268944134769082,-0.32453442921951));
#56325=DIRECTION('center_axis',(-0.271487881944521,0.601098529144406,-0.751648114623931));
#56326=DIRECTION('ref_axis',(0.946869276050077,0.0268943524351229,-0.320492227486875));
#56327=DIRECTION('center_axis',(0.256237095127745,0.584827952222611,0.76962251615945));
#56328=DIRECTION('ref_axis',(0.949530820133915,-0.0032619714466773,-0.313656788796442));
#56329=DIRECTION('center_axis',(-0.348169975729648,-5.95365837681765E-10,
-0.937431420425205));
#56330=DIRECTION('ref_axis',(-0.937316126432585,-0.0156832196313476,0.348127154573454));
#56331=DIRECTION('',(0.34816990329345,8.32135976760844E-8,0.937431447328615));
#56332=DIRECTION('center_axis',(0.22255138460994,0.584827969931679,0.780030208898213));
#56333=DIRECTION('ref_axis',(0.96019646172339,0.00704480133933188,-0.2792366839582));
#56334=DIRECTION('center_axis',(0.288620987568787,5.92193446020471E-10,
0.957443432028659));
#56335=DIRECTION('ref_axis',(-0.957325852294089,0.0156715280544834,0.28858554318925));
#56336=DIRECTION('',(-0.288621063170319,-1.48214773785991E-11,-0.957443409238601));
#56337=DIRECTION('',(0.909057440161087,-3.07809289804079E-8,0.41667081789798));
#56338=DIRECTION('center_axis',(0.566134873267341,0.793626260377381,-0.222819801880318));
#56339=DIRECTION('ref_axis',(-0.814092839849893,0.580734748491199,1.14572618823004E-16));
#56340=DIRECTION('center_axis',(-0.340941299947114,0.471546674547623,0.813266723598999));
#56341=DIRECTION('ref_axis',(0.906703761223004,0.393427978814542,0.151995772539772));
#56342=DIRECTION('center_axis',(-0.2817945677677,-0.601098528040889,-0.747845158548006));
#56343=DIRECTION('ref_axis',(0.936371308045141,-0.00227572240193344,-0.351003695931227));
#56344=DIRECTION('',(0.472928816316381,5.05127141379E-12,-0.881100638234695));
#56345=DIRECTION('center_axis',(0.,-1.,1.45983193964168E-32));
#56346=DIRECTION('ref_axis',(1.,0.,0.));
#56347=DIRECTION('center_axis',(0.284986893316741,0.601098527699123,0.746634469225483));
#56348=DIRECTION('ref_axis',(0.935403780561703,-0.00432803588139098,-0.353554854889991));
#56349=DIRECTION('center_axis',(0.274696550152684,-0.601098528163608,0.750481422004408));
#56350=DIRECTION('ref_axis',(0.938208641494535,-0.00330181468705492,-0.346054393188053));
#56351=DIRECTION('center_axis',(-0.27148789264536,0.60109852795299,-0.751648111711677));
#56352=DIRECTION('ref_axis',(0.939678455149161,-0.0033018624838774,-0.342043123937061));
#56353=DIRECTION('center_axis',(0.350667502483558,0.584828255987638,0.731442556664843));
#56354=DIRECTION('ref_axis',(0.911288073866872,-0.0330815410750519,-0.41043837304534));
#56355=DIRECTION('center_axis',(-0.406375812556749,-1.08214501188567E-7,
-0.913706024369343));
#56356=DIRECTION('ref_axis',(-0.913593763086638,-0.0156751635309797,0.406325885586278));
#56357=DIRECTION('',(0.406344678315595,3.88578058618905E-13,0.913719870860099));
#56358=DIRECTION('center_axis',(0.318557909444986,0.584827952226065,0.745987348837169));
#56359=DIRECTION('ref_axis',(0.925740424547197,-0.0227607296041559,-0.377473993206236));
#56360=DIRECTION('center_axis',(0.348169826705523,6.35249530183533E-10,
0.937431475774014));
#56361=DIRECTION('ref_axis',(-0.93731603218275,0.0156933905083093,0.348126949987413));
#56362=DIRECTION('',(-0.348169904517709,-2.28705943069384E-11,-0.937431446873919));
#56363=DIRECTION('',(0.933426594325848,0.,0.358768439254693));
#56364=DIRECTION('center_axis',(-0.373302380556704,-0.601098528158341,-0.70662995416029));
#56365=DIRECTION('ref_axis',(0.894880721407181,-0.0324816838077035,-0.445121820034447));
#56366=DIRECTION('',(0.416670832496624,8.17238220605976E-12,-0.909057433469729));
#56367=DIRECTION('center_axis',(0.,-1.,1.45983193964168E-32));
#56368=DIRECTION('ref_axis',(1.,0.,0.));
#56369=DIRECTION('center_axis',(0.376317810921175,0.601098524538565,0.705028700820793));
#56370=DIRECTION('ref_axis',(0.89360411672998,-0.034538531061908,-0.447525164024682));
#56371=DIRECTION('center_axis',(0.274696540277618,-0.601098529320043,0.750481424692703));
#56372=DIRECTION('ref_axis',(0.929580973804702,-0.0335099838657365,-0.367091669915867));
#56373=DIRECTION('center_axis',(-0.271487875923072,0.601098526440157,-0.751648118961426));
#56374=DIRECTION('ref_axis',(0.931140740168084,-0.0335100365203316,-0.363117060259688));
#56375=DIRECTION('',(0.462915795308873,1.22124532708699E-12,0.886402259955125));
#56376=DIRECTION('center_axis',(0.409542993165234,0.58482795214625,0.700179122180664));
#56377=DIRECTION('ref_axis',(0.880532271000263,-0.0526562728447166,-0.471052265313756));
#56378=DIRECTION('center_axis',(0.406344580513227,8.00067216176833E-10,
0.913719914354246));
#56379=DIRECTION('ref_axis',(-0.913606246231954,0.0157729998148722,0.406294030626588));
#56380=DIRECTION('',(-0.406344678317571,-1.75692793624627E-10,-0.91371987085922));
#56381=DIRECTION('',(0.954111946854583,0.,0.299450150892195));
#56382=DIRECTION('',(0.3587684392876,6.73708191429265E-11,-0.9334265943132));
#56383=DIRECTION('center_axis',(0.,-1.,1.45983193964168E-32));
#56384=DIRECTION('ref_axis',(1.,0.,0.));
#56385=DIRECTION('center_axis',(0.292190758314825,0.601098532593968,0.743844819077733));
#56386=DIRECTION('ref_axis',(0.914674270984079,0.051484946561636,-0.400899336838176));
#56387=DIRECTION('center_axis',(-0.443480041513362,0.601098534115099,-0.664835321763206));
#56388=DIRECTION('ref_axis',(0.852023579248202,0.052516525333457,-0.520862587418202));
#56389=DIRECTION('center_axis',(0.357728884211842,0.584827930051393,0.728015341618811));
#56390=DIRECTION('ref_axis',(0.890190797097705,0.0219594825673074,-0.455058376351791));
#56391=DIRECTION('center_axis',(-0.517662994394784,-1.00068004579382E-8,
-0.855584609629127));
#56392=DIRECTION('ref_axis',(-0.855478630057052,-0.0157391393477768,0.517598872688398));
#56393=DIRECTION('',(0.517659995144392,0.,0.855586424288691));
#56394=DIRECTION('center_axis',(0.325753956081705,0.584827952320803,0.742873223559293));
#56395=DIRECTION('ref_axis',(0.905745945694596,0.0322834330587411,-0.422589708591849));
#56396=DIRECTION('center_axis',(0.462915721400744,6.23428967396594E-10,
0.886402298552993));
#56397=DIRECTION('ref_axis',(-0.886293018220489,0.0157020800827689,0.462858650707417));
#56398=DIRECTION('',(-0.462915795308241,-1.60982338570617E-12,-0.886402259955456));
#56399=DIRECTION('',(0.971031855421229,0.,0.238950069590293));
#56400=DIRECTION('center_axis',(-0.380115429407096,-0.601098527976857,-0.702988492075592));
#56401=DIRECTION('ref_axis',(0.870944131140459,0.0232723727996506,-0.490830639932213));
#56402=DIRECTION('',(0.299450150892508,0.,-0.954111946854484));
#56403=DIRECTION('center_axis',(0.,-1.,1.45983193964168E-32));
#56404=DIRECTION('ref_axis',(1.,0.,0.));
#56405=DIRECTION('center_axis',(0.38311523762894,0.601098530269338,0.701358162142969));
#56406=DIRECTION('ref_axis',(0.869642814507809,0.0212180793202286,-0.493225271336432));
#56407=DIRECTION('center_axis',(0.446316331932025,-0.601098526794362,0.662934606832672));
#56408=DIRECTION('ref_axis',(0.83854655666011,0.022245241894255,-0.54437562539715));
#56409=DIRECTION('center_axis',(-0.443480105976362,0.601098528947103,-0.664835283435547));
#56410=DIRECTION('ref_axis',(0.840864533470763,0.0222451851397701,-0.540788302470655));
#56411=DIRECTION('center_axis',(0.446153347929533,0.584827953016334,0.677438894293791));
#56412=DIRECTION('ref_axis',(0.838223483341985,-0.00784645566550682,-0.545270414663695));
#56413=DIRECTION('center_axis',(-0.570361573111646,-1.51695271097795E-9,
-0.821393739882164));
#56414=DIRECTION('ref_axis',(-0.821292786457333,-0.0156778483100648,0.570291472832548));
#56415=DIRECTION('',(0.570361227475778,0.,0.821393979885611));
#56416=DIRECTION('center_axis',(0.416291991554971,0.584827952254014,0.696187650012245));
#56417=DIRECTION('ref_axis',(0.85734975104592,0.00246180457996112,-0.514728417614288));
#56418=DIRECTION('center_axis',(0.517659917881015,6.88305756872033E-10,
0.855586471035758));
#56419=DIRECTION('ref_axis',(-0.855481410502806,0.0156707406191949,0.517596352549529));
#56420=DIRECTION('',(-0.517659995144781,-6.46149800302453E-11,-0.855586424288456));
#56421=DIRECTION('',(0.984119544876784,1.64268989065259E-13,0.177506961529715));
#56422=DIRECTION('center_axis',(-0.465225922666287,-0.601098528102663,-0.649804124634581));
#56423=DIRECTION('ref_axis',(0.816092972990407,-0.00691951965448234,-0.577879208557835));
#56424=DIRECTION('',(0.238950069602214,2.34493981894305E-11,-0.971031855418295));
#56425=DIRECTION('center_axis',(0.,-1.,1.45983193964168E-32));
#56426=DIRECTION('ref_axis',(1.,0.,0.));
#56427=DIRECTION('center_axis',(0.467997750909437,0.601098527138387,0.64781067127346));
#56428=DIRECTION('ref_axis',(0.814500088444679,-0.00897206142817162,-0.580094051027365));
#56429=DIRECTION('center_axis',(0.446316335307023,-0.601098528453655,0.662934603055958));
#56430=DIRECTION('ref_axis',(0.826145154494294,-0.00794570877144874,-0.563401321810411));
#56431=DIRECTION('center_axis',(-0.44348009084144,0.601098527573114,-0.664835294773602));
#56432=DIRECTION('ref_axis',(0.828544533267035,-0.00794577982429505,-0.559866788599122));
#56433=DIRECTION('center_axis',(0.527540982864664,0.584827952229474,0.616179176611206));
#56434=DIRECTION('ref_axis',(0.767951949432859,-0.018154631716425,-0.640250117305349));
#56435=DIRECTION('center_axis',(-0.620811438041664,6.65490569819036E-10,
-0.783959921422417));
#56436=DIRECTION('ref_axis',(-0.783863548436222,-0.0156795066150567,0.620735121050262));
#56437=DIRECTION('',(0.620811502081951,2.06171105075976E-7,0.783959870709407));
#56438=DIRECTION('center_axis',(0.500269812260683,0.584827782536768,0.638519051958349));
#56439=DIRECTION('ref_axis',(0.798886072310224,-0.0273551074093783,-0.600860001637124));
#56440=DIRECTION('center_axis',(0.570361134901209,7.69554369147915E-10,
0.821394044167722));
#56441=DIRECTION('ref_axis',(-0.821292775200073,0.0157023279251403,0.57029081555106));
#56442=DIRECTION('',(0.570361226666348,-1.29267404451664E-5,0.821393980345947));
#56443=DIRECTION('',(0.993323368672551,-7.62630514903932E-8,0.115363275131251));
#56444=DIRECTION('center_axis',(-0.620811504599348,1.56670257677117E-11,
-0.783959868715927));
#56445=DIRECTION('ref_axis',(-0.605120001082122,-0.63577280508502,0.479189654108577));
#56446=DIRECTION('',(-0.177506961531102,0.,0.984119544876534));
#56447=DIRECTION('center_axis',(0.611224283835664,0.398564391591621,0.683777230247381));
#56448=DIRECTION('ref_axis',(0.745553533390733,2.85036533746566E-16,-0.666445743364449));
#56449=DIRECTION('center_axis',(-0.673996080620018,5.7445664793789E-5,-0.738734918633775));
#56450=DIRECTION('ref_axis',(0.738734885246909,0.000362953305560281,-0.673996021934948));
#56451=DIRECTION('',(0.668811041446531,5.94973700105111E-5,0.74343243627062));
#56452=DIRECTION('center_axis',(0.489456455373912,0.590180063808601,0.641965630369478));
#56453=DIRECTION('ref_axis',(0.486218742096034,-0.795821400074055,0.360914995558124));
#56454=DIRECTION('center_axis',(0.798223519056493,0.550037558009713,-0.245556303938181));
#56455=DIRECTION('ref_axis',(-0.567410340608164,0.823435185895604,7.65040472392408E-17));
#56456=DIRECTION('center_axis',(-0.046359144049487,-0.477126089681845,0.87761126035843));
#56457=DIRECTION('ref_axis',(0.989631716015808,0.0976231510478723,0.105350780894548));
#56458=DIRECTION('center_axis',(0.0567895812678342,0.584827951390709,0.809166985690575));
#56459=DIRECTION('ref_axis',(0.995671712706078,0.0265489689879054,-0.0890673495879593));
#56460=DIRECTION('center_axis',(-0.166345718370956,-5.79615458256036E-12,
-0.986067493622851));
#56461=DIRECTION('ref_axis',(-0.985945217534087,-0.0157477670560628,0.166325090874496));
#56462=DIRECTION('center_axis',(0.113148551236963,-0.000115441160388845,
0.993578075455731));
#56463=DIRECTION('ref_axis',(0.0247034058069071,-0.999690532374862,-0.00292937222011708));
#56464=DIRECTION('',(-0.10410178598878,-6.0812466147161E-10,-0.99456664842229));
#56465=DIRECTION('center_axis',(-0.0869599381853343,-0.601098527906027,
-0.794429687826437));
#56466=DIRECTION('ref_axis',(0.991170198344495,0.0279220160276409,-0.129622524796762));
#56467=DIRECTION('',(0.629653742733083,2.24062901110922E-10,-0.776875900168245));
#56468=DIRECTION('center_axis',(0.,-1.,1.45983193964168E-32));
#56469=DIRECTION('ref_axis',(1.,0.,0.));
#56470=DIRECTION('center_axis',(0.0903530626196487,0.601098530391009,0.794050930883542));
#56471=DIRECTION('ref_axis',(0.990868192983961,0.0258667999664512,-0.132329636862627));
#56472=DIRECTION('center_axis',(0.178470234888878,-0.601098526314079,0.778992257292556));
#56473=DIRECTION('ref_axis',(0.978710923336046,0.0268944144261749,-0.203473877968101));
#56474=DIRECTION('center_axis',(-0.175140634157931,0.60109852903841,-0.779747598043506));
#56475=DIRECTION('ref_axis',(0.979571255487549,0.02689435486768,-0.199290865567886));
#56476=DIRECTION('center_axis',(0.157757310542433,0.584827952222822,0.795668836432142));
#56477=DIRECTION('ref_axis',(0.981355105572388,-0.00326197145772807,-0.192175743290398));
#56478=DIRECTION('center_axis',(-0.227933249196464,-6.67224254800419E-10,
-0.973676760486119));
#56479=DIRECTION('ref_axis',(-0.973557008707097,-0.0156832196312757,0.227905215866787));
#56480=DIRECTION('',(0.227933165074045,8.32139862540016E-8,0.973676780178783));
#56481=DIRECTION('center_axis',(0.12303279206818,0.58482796993107,0.801772522391615));
#56482=DIRECTION('ref_axis',(0.987622662361441,0.00704480136426823,-0.15669029186212));
#56483=DIRECTION('center_axis',(0.166345636865383,6.46213028799582E-10,
0.986067507372518));
#56484=DIRECTION('ref_axis',(-0.985946412430586,0.0156715280538572,0.166325208623692));
#56485=DIRECTION('',(-0.16634572144554,-1.52655665884468E-11,-0.98606749310418));
#56486=DIRECTION('',(0.849666549784065,-3.07809289804128E-8,0.527320352516421));
#56487=DIRECTION('center_axis',(0.589597456970291,0.793626260375601,-0.150107286886432));
#56488=DIRECTION('ref_axis',(-0.802721322931315,0.596354322287849,8.06103090759229E-17));
#56489=DIRECTION('center_axis',(-0.440182224162468,0.47154667453567,0.764122597012897));
#56490=DIRECTION('ref_axis',(0.880508648889467,0.393407165948483,0.264452871058772));
#56491=DIRECTION('center_axis',(-0.185842683725629,-0.601098528037002,-0.777266399953971));
#56492=DIRECTION('ref_axis',(0.972980168381012,-0.00227572377380966,-0.23087748486711));
#56493=DIRECTION('',(0.579630823428158,5.19500677922247E-12,-0.814879198735614));
#56494=DIRECTION('center_axis',(0.,-1.,1.45983193964168E-32));
#56495=DIRECTION('ref_axis',(1.,0.,0.));
#56496=DIRECTION('center_axis',(0.189161557158541,0.601098527764655,0.776465366396029));
#56497=DIRECTION('ref_axis',(0.972340018886731,-0.00432802533413876,-0.233529775120988));
#56498=DIRECTION('center_axis',(0.178470202136203,-0.601098528104808,0.778992263414532));
#56499=DIRECTION('ref_axis',(0.974182705936134,-0.00330182722881675,-0.225736911895026));
#56500=DIRECTION('center_axis',(-0.175140642259538,0.60109852795263,-0.779747597060804));
#56501=DIRECTION('ref_axis',(0.97513818040934,-0.00330186181908194,-0.221573073311016));
#56502=DIRECTION('center_axis',(0.256228323716209,0.584828255987086,0.769625205619388));
#56503=DIRECTION('ref_axis',(0.955543863682515,-0.0330815410888132,-0.292987262893595));
#56504=DIRECTION('center_axis',(-0.288653681746295,-1.08169872562643E-7,
-0.957433575771341));
#56505=DIRECTION('ref_axis',(-0.957315942193711,-0.0156751635319026,0.288618218534477));
#56506=DIRECTION('',(0.288621063170579,0.,0.957443409238522));
#56507=DIRECTION('center_axis',(0.222548978555872,0.58482795222586,0.780030908643398));
#56508=DIRECTION('ref_axis',(0.96575072094856,-0.0227607296059838,-0.25847145717688));
#56509=DIRECTION('center_axis',(0.227933079194689,6.8622169776503E-10,0.973676800282736));
#56510=DIRECTION('ref_axis',(-0.973556893120938,0.0156933905088043,0.227905009490895));
#56511=DIRECTION('',(-0.227933166345564,-2.28705943069234E-11,-0.97367677988113));
#56512=DIRECTION('',(0.881100638236175,0.,0.472928816313623));
#56513=DIRECTION('center_axis',(-0.281794563711666,-0.601098528121939,-0.747845160011209));
#56514=DIRECTION('ref_axis',(0.943612876362721,-0.0324816844511772,-0.329453607868675));
#56515=DIRECTION('',(0.527320366161225,8.00811321699381E-12,-0.849666541315822));
#56516=DIRECTION('center_axis',(0.,-1.,1.45983193964168E-32));
#56517=DIRECTION('ref_axis',(1.,0.,0.));
#56518=DIRECTION('center_axis',(0.284986892580716,0.601098525015561,0.746634471666896));
#56519=DIRECTION('ref_axis',(0.942647561254193,-0.034538522663551,-0.331997990526662));
#56520=DIRECTION('center_axis',(0.178470203895147,-0.601098529032738,0.778992262295527));
#56521=DIRECTION('ref_axis',(0.96825973773138,-0.0335099891008813,-0.247689646369844));
#56522=DIRECTION('center_axis',(-0.175140622244973,0.601098526387723,-0.779747602762684));
#56523=DIRECTION('ref_axis',(0.969309052898517,-0.0335100374068191,-0.243550892755443));
#56524=DIRECTION('',(0.348169904517632,0.,0.937431446873948));
#56525=DIRECTION('center_axis',(0.318557910873374,0.584827952146795,0.745987348289352));
#56526=DIRECTION('ref_axis',(0.932627514633883,-0.0526562728392143,-0.356977920715706));
#56527=DIRECTION('center_axis',(0.288620968373058,7.36716723334152E-10,
0.957443437815205));
#56528=DIRECTION('ref_axis',(-0.957324330419263,0.0157729998146348,0.288585063480696));
#56529=DIRECTION('',(-0.288621063172965,-1.76525460893015E-10,-0.957443409237803));
#56530=DIRECTION('',(0.909057433471482,0.,0.4166708324928));
#56531=DIRECTION('',(0.472928816344016,6.51326541667589E-11,-0.881100638219862));
#56532=DIRECTION('center_axis',(0.,-1.,1.45983193964168E-32));
#56533=DIRECTION('ref_axis',(1.,0.,0.));
#56534=DIRECTION('center_axis',(0.196658269195918,0.601098532523592,0.774600593438225));
#56535=DIRECTION('ref_axis',(0.957707801639643,0.0514849473548277,-0.283099040751522));
#56536=DIRECTION('center_axis',(-0.356657108101514,0.601098534122288,-0.71517568437182));
#56537=DIRECTION('ref_axis',(0.910586511224675,0.0525165252266949,-0.409968559957699));
#56538=DIRECTION('center_axis',(0.263662627420127,0.584827908067115,0.767110381136742));
#56539=DIRECTION('ref_axis',(0.940205578398073,0.0219600677488413,-0.339898846384644));
#56540=DIRECTION('center_axis',(-0.406351027183781,-1.96778055995898E-8,
-0.913717047398529));
#56541=DIRECTION('ref_axis',(-0.913603867046846,-0.0157391387099202,0.406300693612155));
#56542=DIRECTION('',(0.406344678315241,1.1657341758555E-12,0.913719870860256));
#56543=DIRECTION('center_axis',(0.230078585587962,0.584827952320172,0.777843242973054));
#56544=DIRECTION('ref_axis',(0.951568403032065,0.0322834330679206,-0.305737394344157));
#56545=DIRECTION('center_axis',(0.348169842990746,4.83512735164658E-10,
0.937431469725547));
#56546=DIRECTION('ref_axis',(-0.937315898246574,0.0157020800822315,0.348126918774331));
#56547=DIRECTION('',(-0.3481699045172,-7.77156117238184E-13,-0.937431446874108));
#56548=DIRECTION('',(0.933426594325828,-1.64268989065341E-13,0.358768439254745));
#56549=DIRECTION('center_axis',(-0.289010284359285,-0.601098527964732,-0.745086313934968));
#56550=DIRECTION('ref_axis',(0.925593867913443,0.0232723731127603,-0.377802049135169));
#56551=DIRECTION('',(0.41667083249282,0.,-0.909057433471472));
#56552=DIRECTION('center_axis',(0.,-1.,1.45983193964168E-32));
#56553=DIRECTION('ref_axis',(1.,0.,0.));
#56554=DIRECTION('center_axis',(0.292190763392168,0.601098530037678,0.743844819149025));
#56555=DIRECTION('ref_axis',(0.924602942398734,0.0212180856973082,-0.380340888870688));
#56556=DIRECTION('center_axis',(0.359709254122371,-0.601098526854637,0.713645439635056));
#56557=DIRECTION('ref_axis',(0.900162724924359,0.0222452403493355,-0.43498530772723));
#56558=DIRECTION('center_axis',(-0.356657179733677,0.601098528884004,-0.715175653051686));
#56559=DIRECTION('ref_axis',(0.90201281102059,0.0222451869553289,-0.431135756359939));
#56560=DIRECTION('center_axis',(0.357729647163817,0.58482795337547,0.728014947985761));
#56561=DIRECTION('ref_axis',(0.899954361422345,-0.00784642889805246,-0.435913501638165));
#56562=DIRECTION('center_axis',(-0.462916327110225,-2.13103238692194E-9,
-0.886401982226337));
#56563=DIRECTION('ref_axis',(-0.886293038960898,-0.0156778482812414,0.462859432401163));
#56564=DIRECTION('',(0.462915795308865,-8.3266726846851E-13,0.88640225995513));
#56565=DIRECTION('center_axis',(0.325753955500558,0.584827952253567,0.742873223867061));
#56566=DIRECTION('ref_axis',(0.915101869174067,0.00246180459107409,-0.403215213691503));
#56567=DIRECTION('center_axis',(0.406344609651634,5.69456944890493E-10,
0.91371990139597));
#56568=DIRECTION('ref_axis',(-0.913607702448164,0.0156707406190495,0.40629471312809));
#56569=DIRECTION('',(-0.406344678315647,-6.46149800302078E-11,-0.913719870860076));
#56570=DIRECTION('',(0.954111946854455,1.64268989065293E-13,0.2994501508926));
#56571=DIRECTION('center_axis',(-0.380115429527852,-0.601098528065762,-0.702988491934279));
#56572=DIRECTION('ref_axis',(0.882085304090706,-0.00691952261253271,-0.471038890659807));
#56573=DIRECTION('',(0.358768439266062,2.34493981894336E-11,-0.933426594321478));
#56574=DIRECTION('center_axis',(0.,-1.,1.45983193964168E-32));
#56575=DIRECTION('ref_axis',(1.,0.,0.));
#56576=DIRECTION('center_axis',(0.383115245013786,0.601098527119973,0.701358160808175));
#56577=DIRECTION('ref_axis',(0.880782574146974,-0.00897206302439092,-0.47343590819045));
#56578=DIRECTION('center_axis',(0.359709246947306,-0.601098528345563,0.713645441995814));
#56579=DIRECTION('ref_axis',(0.890243668023657,-0.0079457177559491,-0.455415279841518));
#56580=DIRECTION('center_axis',(-0.356657173644811,0.60109852769709,-0.715175657085786));
#56581=DIRECTION('ref_axis',(0.892181121906817,-0.00794577101805003,-0.451607916710969));
#56582=DIRECTION('center_axis',(0.446196308910663,0.584826536165555,0.677411821945188));
#56583=DIRECTION('ref_axis',(0.84211854955642,-0.018184624938029,-0.538985777093287));
#56584=DIRECTION('center_axis',(-0.517660059578906,-5.71097183739979E-10,
-0.855586385303532));
#56585=DIRECTION('ref_axis',(-0.85548120719194,-0.0156795066172793,0.517596423107483));
#56586=DIRECTION('',(0.517659992380242,2.06171049564757E-7,0.855586425961074));
#56587=DIRECTION('center_axis',(0.416297377870238,0.584827782537028,0.696184571756073));
#56588=DIRECTION('ref_axis',(0.867894343950115,-0.0273551073936917,-0.495995066345301));
#56589=DIRECTION('center_axis',(0.462915689858085,8.19138286898656E-10,
0.886402315025865));
#56590=DIRECTION('ref_axis',(-0.88629303124274,0.0157023279251941,0.462858617364184));
#56591=DIRECTION('',(0.462915794448414,-1.2926741850564E-5,0.886402260310235));
#56592=DIRECTION('',(0.971031864912497,-7.62629077550481E-8,0.238950031020196));
#56593=DIRECTION('center_axis',(-0.517659995654058,-4.84222756609793E-10,
-0.855586423980325));
#56594=DIRECTION('ref_axis',(-0.66040683756443,-0.635772805082279,0.399569454808496));
#56595=DIRECTION('',(-0.299450150894097,0.,0.954111946853985));
#56596=DIRECTION('center_axis',(0.520704586489422,0.398564391591113,0.754992158478806));
#56597=DIRECTION('ref_axis',(0.823202421104882,-3.43454409686757E-16,-0.567747984485247));
#56598=DIRECTION('center_axis',(-0.576093384133844,5.74456620606364E-5,
-0.817383881329459));
#56599=DIRECTION('ref_axis',(0.817383840858432,0.000362923848892853,-0.57609333010355));
#56600=DIRECTION('',(0.57036047544634,5.94973683763054E-5,0.821394499926003));
#56601=DIRECTION('center_axis',(0.405137316878508,0.590180063814461,0.698248699782851));
#56602=DIRECTION('ref_axis',(0.43716135183174,-0.795819504651481,0.419000320382833));
#56603=DIRECTION('center_axis',(0.82270565378683,0.550037558008124,-0.143576084386098));
#56604=DIRECTION('ref_axis',(-0.555796003805303,0.831318712741422,-1.57794878871776E-16));
#56605=DIRECTION('center_axis',(-0.155987445342299,-0.477126090515431,0.864880691566787));
#56606=DIRECTION('ref_axis',(0.96862208907624,0.0976327713137033,0.228558724443385));
#56607=DIRECTION('center_axis',(-0.0450737364009293,0.584827951389048,0.80990408417352));
#56608=DIRECTION('ref_axis',(0.998983642785354,0.0265489690160679,0.036425728427699));
#56609=DIRECTION('center_axis',(-0.0414470086426727,-3.87595059013494E-11,
-0.999140703542086));
#56610=DIRECTION('ref_axis',(-0.999016806325967,-0.0157477670562018,0.0414418690578688));
#56611=DIRECTION('center_axis',(-0.0122720118683925,-0.000115441168890837,
0.999924689363173));
#56612=DIRECTION('ref_axis',(0.0248716549244404,-0.999690634518669,0.000189834085567114));
#56613=DIRECTION('',(0.0213713417293984,-6.05404615063059E-10,-0.999771606794615));
#56614=DIRECTION('center_axis',(0.0132941942386101,-0.601098528297747,-0.799064342639458));
#56615=DIRECTION('ref_axis',(0.999600535647751,0.027922007443411,-0.00437385791473135));
#56616=DIRECTION('',(0.72205710354946,2.24206636476366E-10,-0.691833462051211));
#56617=DIRECTION('center_axis',(0.,-1.,1.45983193964168E-32));
#56618=DIRECTION('ref_axis',(1.,0.,0.));
#56619=DIRECTION('center_axis',(-0.00988037512737149,0.601098530231419,
0.799113843667453));
#56620=DIRECTION('ref_axis',(0.999640202548808,0.0258668036150491,-0.00709745862388935));
#56621=DIRECTION('center_axis',(0.0794293293740866,-0.601098526204097,0.795217921975131));
#56622=DIRECTION('ref_axis',(0.996495534121554,0.02689441690441,-0.0792044242146213));
#56623=DIRECTION('center_axis',(-0.0760313169023642,0.60109852885632,-0.795549996830407));
#56624=DIRECTION('ref_axis',(0.996824811638328,0.0268943589583594,-0.0749465700244607));
#56625=DIRECTION('center_axis',(0.0567895988978252,0.584827952222578,0.809166983852017));
#56626=DIRECTION('ref_axis',(0.99770283476844,-0.00326197144910447,-0.0676639714861966));
#56627=DIRECTION('center_axis',(-0.104101854023608,-5.35833916009832E-10,
-0.994566641301048));
#56628=DIRECTION('ref_axis',(-0.994444320292724,-0.0156832196308266,0.10408905062279));
#56629=DIRECTION('',(0.104101784680632,8.32123764308129E-8,0.994566648559211));
#56630=DIRECTION('center_axis',(0.021573898985439,0.584827969931933,0.810870404237237));
#56631=DIRECTION('ref_axis',(0.999473463626372,0.00704480133771679,-0.0316728003311105));
#56632=DIRECTION('center_axis',(0.0414469425202581,4.90387004565544E-10,
0.999140706285017));
#56633=DIRECTION('ref_axis',(-0.999018005875278,0.0156715280542373,0.0414418525819914));
#56634=DIRECTION('',(-0.0414470083234317,-1.52100554371989E-11,-0.999140703555329));
#56635=DIRECTION('',(0.776875910350839,-3.07809289804261E-8,0.62965373016965));
#56636=DIRECTION('center_axis',(0.603761736567746,0.793626260373733,-0.0750274903079059));
#56637=DIRECTION('ref_axis',(-0.795869445639745,0.605468269603854,1.93408423312097E-18));
#56638=DIRECTION('center_axis',(-0.532481211769311,0.471546674534408,0.70292780059422));
#56639=DIRECTION('ref_axis',(0.840418742351967,0.393423605136949,0.37271195905764));
#56640=DIRECTION('center_axis',(-0.0869599531970929,-0.601098528018402,
-0.79442968609819));
#56641=DIRECTION('ref_axis',(0.994244550367405,-0.00227572727050743,-0.107110200868581));
#56642=DIRECTION('',(0.677191706199972,5.19500677922242E-12,-0.735806627487121));
#56643=DIRECTION('center_axis',(0.,-1.,1.45983193964168E-32));
#56644=DIRECTION('ref_axis',(1.,0.,0.));
#56645=DIRECTION('center_axis',(0.0903530431260819,0.601098527779805,0.794050935078354));
#56646=DIRECTION('ref_axis',(0.993941869584976,-0.00432802320240801,-0.109821801574556));
#56647=DIRECTION('center_axis',(0.0794293017766313,-0.601098528134647,0.795217923272381));
#56648=DIRECTION('ref_axis',(0.994793320646601,-0.00330182131864235,-0.101859448127744));
#56649=DIRECTION('center_axis',(-0.0760313175229954,0.601098527951306,-0.795549997454899));
#56650=DIRECTION('ref_axis',(0.995219394403722,-0.0033018622772266,-0.0976086815206026));
#56651=DIRECTION('center_axis',(0.157748271217537,0.584828255986589,0.795670405336005));
#56652=DIRECTION('ref_axis',(0.984730155958913,-0.0330815410996522,-0.170915568581701));
#56653=DIRECTION('center_axis',(-0.166379306364509,-1.08098869174227E-7,
-0.98606182687175));
#56654=DIRECTION('ref_axis',(-0.985940676151014,-0.0156751635313622,0.166358866187367));
#56655=DIRECTION('',(0.166345721446008,-4.44089209849642E-13,0.986067493104101));
#56656=DIRECTION('center_axis',(0.123030317359083,0.584827952225381,0.801772915049137));
#56657=DIRECTION('ref_axis',(0.990530551566245,-0.0227607296247098,-0.135392671887445));
#56658=DIRECTION('center_axis',(0.104101719042027,5.12252965996456E-10,
0.994566655429637));
#56659=DIRECTION('ref_axis',(-0.994444175704888,0.0156933905084582,0.104088899028543));
#56660=DIRECTION('',(-0.104101785979457,-2.24265050970633E-11,-0.994566648423266));
#56661=DIRECTION('',(0.814879198737199,0.,0.579630823425929));
#56662=DIRECTION('center_axis',(-0.185842672560432,-0.601098528282589,-0.77726640243362));
#56663=DIRECTION('ref_axis',(0.977463693873356,-0.0324816815353087,-0.208589710973703));
#56664=DIRECTION('',(0.62965374264558,8.0081132169946E-12,-0.776875900239165));
#56665=DIRECTION('center_axis',(0.,-1.,1.45983193964168E-32));
#56666=DIRECTION('ref_axis',(1.,0.,0.));
#56667=DIRECTION('center_axis',(0.189161568512983,0.601098525178652,0.776465365631821));
#56668=DIRECTION('ref_axis',(0.976824886273939,-0.0345385197933366,-0.211235016525178));
#56669=DIRECTION('center_axis',(0.0794293062798579,-0.601098529449489,0.795217921828704));
#56670=DIRECTION('ref_axis',(0.99166846380021,-0.0335099815858313,-0.124381425615923));
#56671=DIRECTION('center_axis',(-0.076031303748593,0.601098526592688,-0.795549999797868));
#56672=DIRECTION('ref_axis',(0.992190781961022,-0.0335100337510252,-0.120143788143963));
#56673=DIRECTION('',(0.227933166345836,0.,0.973676779881066));
#56674=DIRECTION('center_axis',(0.222548980042715,0.584827952146603,0.780030908278613));
#56675=DIRECTION('ref_axis',(0.970014665232009,-0.0526562728418158,-0.237273821070177));
#56676=DIRECTION('center_axis',(0.166345654650758,4.90609543879989E-10,
0.986067504372196));
#56677=DIRECTION('ref_axis',(-0.985944836097383,0.015772999814921,0.166324960994262));
#56678=DIRECTION('',(-0.166345721448132,-1.76525460892848E-10,-0.986067493103743));
#56679=DIRECTION('',(0.849666541318092,0.,0.527320366157567));
#56680=DIRECTION('',(0.579630823453911,6.52763895321938E-11,-0.814879198717295));
#56681=DIRECTION('center_axis',(0.,-1.,1.45983193964168E-32));
#56682=DIRECTION('ref_axis',(1.,0.,0.));
#56683=DIRECTION('center_axis',(0.0980243614840752,0.601098532447537,0.793140453416075));
#56684=DIRECTION('ref_axis',(0.985637707909252,0.0514849482174098,-0.160834103518025));
#56685=DIRECTION('center_axis',(-0.264209488022563,0.601098533639632,-0.754237296409519));
#56686=DIRECTION('ref_axis',(0.954788947439151,0.0525165307922483,-0.292609090497177));
#56687=DIRECTION('center_axis',(0.165440120299829,0.584827930050204,0.794106956793839));
#56688=DIRECTION('ref_axis',(0.975392232534895,0.0219594825888217,-0.219380431750472));
#56689=DIRECTION('center_axis',(-0.288624441049067,-1.01852615899359E-8,
-0.957442390971443));
#56690=DIRECTION('ref_axis',(-0.95732379452256,-0.0157391393488549,0.288588689891833));
#56691=DIRECTION('',(0.288621063170527,0.,0.957443409238538));
#56692=DIRECTION('center_axis',(0.130774738411927,0.58482795232171,0.80054620976961));
#56693=DIRECTION('ref_axis',(0.982384058203747,0.0322834330438129,-0.184063418793747));
#56694=DIRECTION('center_axis',(0.227933095961805,5.36713694051927E-10,
0.973676796357635));
#56695=DIRECTION('ref_axis',(-0.973556756363443,0.0157020800829616,0.227904995162808));
#56696=DIRECTION('',(-0.227933166345239,0.,-0.973676779881206));
#56697=DIRECTION('',(0.881100638235996,0.,0.472928816313958));
#56698=DIRECTION('center_axis',(-0.193347279669351,-0.601098528077531,-0.775433678007015));
#56699=DIRECTION('ref_axis',(0.965646435319799,0.0232723701693565,-0.258815298506224));
#56700=DIRECTION('',(0.527320366157741,1.43735365432636E-13,-0.849666541317984));
#56701=DIRECTION('center_axis',(0.,-1.,1.45983193964168E-32));
#56702=DIRECTION('ref_axis',(1.,0.,0.));
#56703=DIRECTION('center_axis',(0.196658274352736,0.601098530012063,0.774600594077968));
#56704=DIRECTION('ref_axis',(0.964981525726815,0.0212180863974566,-0.261458309899644));
#56705=DIRECTION('center_axis',(0.267429327870916,-0.601098527355575,0.753101663127542));
#56706=DIRECTION('ref_axis',(0.947582794004111,0.022245227166339,-0.318734997098971));
#56707=DIRECTION('center_axis',(-0.26420956622361,0.601098528605351,-0.754237273027802));
#56708=DIRECTION('ref_axis',(0.948935805683094,0.0222451945820041,-0.314683949400961));
#56709=DIRECTION('center_axis',(0.263664374551296,0.584827953375635,0.767109746087833));
#56710=DIRECTION('ref_axis',(0.947492401188789,-0.00784642890954199,-0.319682003314027));
#56711=DIRECTION('center_axis',(-0.348170453906574,-2.02285230155265E-9,
-0.937431242826102));
#56712=DIRECTION('ref_axis',(-0.937316027812998,-0.0156778482804679,0.348127662041035));
#56713=DIRECTION('',(0.348169904517851,0.,0.937431446873866));
#56714=DIRECTION('center_axis',(0.230078585025473,0.584827952254169,0.777843243189058));
#56715=DIRECTION('ref_axis',(0.958422284153197,0.00246180456792404,-0.285343065023208));
#56716=DIRECTION('center_axis',(0.288620995923767,5.31164864483657E-10,
0.957443429510054));
#56717=DIRECTION('ref_axis',(-0.957325861591825,0.0156707406190328,0.288585555106142));
#56718=DIRECTION('',(-0.288621063171154,-6.3837823913025E-11,-0.957443409238349));
#56719=DIRECTION('',(0.909057433471483,1.64268989065371E-13,0.416670832492798));
#56720=DIRECTION('center_axis',(-0.289010286880025,-0.601098528051554,-0.745086312887158));
#56721=DIRECTION('ref_axis',(0.934166624713937,-0.00691952383404778,-0.356770006391346));
#56722=DIRECTION('',(0.472928816324657,2.3593133554862E-11,-0.881100638230253));
#56723=DIRECTION('center_axis',(0.,-1.,1.45983193964168E-32));
#56724=DIRECTION('ref_axis',(1.,0.,0.));
#56725=DIRECTION('center_axis',(0.292190763391757,0.601098527273705,0.743844821382743));
#56726=DIRECTION('ref_axis',(0.933174599151579,-0.00897205187960923,-0.359311382763417));
#56727=DIRECTION('center_axis',(0.267429334256417,-0.601098528288515,0.753101660115387));
#56728=DIRECTION('ref_axis',(0.940302502417433,-0.00794572222091479,-0.34024707117902));
#56729=DIRECTION('center_axis',(-0.264209542754952,0.601098527650592,-0.754237282009787));
#56730=DIRECTION('ref_axis',(0.941747489151797,-0.00794577413585423,-0.336226904559507));
#56731=DIRECTION('center_axis',(0.357729782879291,0.584827952230029,0.728014882218466));
#56732=DIRECTION('ref_axis',(0.903049056216021,-0.0181546317010865,-0.429153598860771));
#56733=DIRECTION('center_axis',(-0.406344608639772,5.97918690298626E-10,
-0.91371990184596));
#56734=DIRECTION('ref_axis',(-0.91360757733036,-0.015679506615491,0.406294656274047));
#56735=DIRECTION('',(0.406344675363134,2.06170716497958E-7,0.913719872173079));
#56736=DIRECTION('center_axis',(0.325759685235944,0.584827782535944,0.742870844931385));
#56737=DIRECTION('ref_axis',(0.923215403293511,-0.0273551074368675,-0.383307992636101));
#56738=DIRECTION('center_axis',(0.348169814866188,6.35675375795079E-10,
0.937431480171241));
#56739=DIRECTION('ref_axis',(-0.937315905043182,0.0157023279249446,0.348126889295869));
#56740=DIRECTION('',(0.348169903620024,-1.29267404452099E-5,0.9374314471182));
#56741=DIRECTION('',(0.933426608576421,-7.62630514904304E-8,0.358768402178222));
#56742=DIRECTION('center_axis',(-0.406344678303629,9.72635009398676E-12,
-0.91371987086542));
#56743=DIRECTION('ref_axis',(-0.705278664517349,-0.63577280508501,0.31364780517479));
#56744=DIRECTION('',(-0.416670832494401,0.,0.909057433470748));
#56745=DIRECTION('center_axis',(0.42197306675971,0.398564391592602,0.814300409359976));
#56746=DIRECTION('ref_axis',(0.88786891488108,-3.68203022609066E-16,-0.460096500734241));
#56747=DIRECTION('center_axis',(-0.469105350786784,5.74456587699608E-5,
-0.883142211969966));
#56748=DIRECTION('ref_axis',(0.883142165048644,0.000362915771362469,-0.469105302256685));
#56749=DIRECTION('',(0.462914984031396,5.94973683407511E-5,0.88640268164039));
#56750=DIRECTION('center_axis',(0.31442892067083,0.59018006381212,0.743519970225749));
#56751=DIRECTION('ref_axis',(0.381193945724401,-0.795820376348163,0.470490280805172));
#56752=DIRECTION('center_axis',(0.834213228884336,0.550037558023509,-0.039331584228274));
#56753=DIRECTION('ref_axis',(-0.550463499044935,0.834859231379283,-4.10782205454431E-17));
#56754=DIRECTION('center_axis',(-0.263155731641066,-0.477126089454373,0.838510438615068));
#56755=DIRECTION('ref_axis',(0.932338856151779,0.0976304978256445,0.348155917950433));
#56756=DIRECTION('center_axis',(-0.146226214258538,0.584827951389492,0.797868511433548));
#56757=DIRECTION('ref_axis',(0.98654100405341,0.0265489690076915,0.161344350895589));
#56758=DIRECTION('center_axis',(0.0841053503384132,-1.04564632314426E-11,
-0.996456868130504));
#56759=DIRECTION('ref_axis',(-0.996333303720138,-0.015747767056287,-0.0840949209575536));
#56760=DIRECTION('center_axis',(-0.137499037186064,-0.000115441183750491,
0.990501893711586));
#56761=DIRECTION('ref_axis',(0.0246541028855363,-0.999690575213707,0.00330590982899623));
#56762=DIRECTION('',(0.14650743062224,-6.06570349238291E-10,-0.989209569693131));
#56763=DIRECTION('center_axis',(0.113338698242169,-0.601098527890642,-0.791097275465207));
#56764=DIRECTION('ref_axis',(0.992266574922364,0.0279220164159767,0.120943810470426));
#56765=DIRECTION('',(0.803073192506942,2.24206636476422E-10,-0.595880396956225));
#56766=DIRECTION('center_axis',(0.,-1.,1.45983193964168E-32));
#56767=DIRECTION('ref_axis',(1.,0.,0.));
#56768=DIRECTION('center_axis',(-0.109958002712627,0.601098529822913,0.791574251150316));
#56769=DIRECTION('ref_axis',(0.992647286720043,0.0258668128628887,0.118246658133127));
#56770=DIRECTION('center_axis',(-0.020864243568711,-0.601098526625939,0.798902525110812));
#56771=DIRECTION('ref_axis',(0.998564815473844,0.0268944076276533,0.0463141461763672));
#56772=DIRECTION('center_axis',(0.024277065154547,0.601098528826007,-0.798806098343454));
#56773=DIRECTION('ref_axis',(0.998357846255219,0.0268943596500547,0.0505796820833543));
#56774=DIRECTION('center_axis',(-0.0450737186594267,0.584827952222493,0.809904084559065));
#56775=DIRECTION('ref_axis',(0.998316194257801,-0.00326197143264825,0.0579149015797671));
#56776=DIRECTION('center_axis',(0.0213712886453174,-4.16287320721315E-10,
-0.99977160792935));
#56777=DIRECTION('ref_axis',(-0.999648646767079,-0.01568321963139,-0.0213686601999815));
#56778=DIRECTION('',(-0.0213713430443371,8.32155960773552E-8,0.999771606766503));
#56779=DIRECTION('center_axis',(-0.0802252274000674,0.584827969932243,0.807180375426422));
#56780=DIRECTION('ref_axis',(0.99556197132029,0.0070448013281525,0.0938441902043184));
#56781=DIRECTION('center_axis',(-0.0841054090067981,4.46159887102019E-10,
0.996456863178632));
#56782=DIRECTION('ref_axis',(-0.99633449235985,0.0156715280544274,-0.0840950803702535));
#56783=DIRECTION('',(0.0841053488789417,-1.28230759343022E-11,-0.99645686825369));
#56784=DIRECTION('',(0.691833473728012,-3.07809289804253E-8,0.722057092361422));
#56785=DIRECTION('center_axis',(0.608404332907485,0.793626260372994,0.0012355346107901));
#56786=DIRECTION('ref_axis',(-0.793626866127095,0.608404797286549,2.59767481348948E-19));
#56787=DIRECTION('center_axis',(-0.616382652520224,0.471546674485576,0.630647412944608));
#56788=DIRECTION('ref_axis',(0.787078545591813,0.393425210691968,0.475104164011491));
#56789=DIRECTION('center_axis',(0.0132942125182302,-0.601098528073487,-0.799064342504036));
#56790=DIRECTION('ref_axis',(0.999829102689717,-0.00227571578226521,0.0183462947854261));
#56791=DIRECTION('',(0.764072871230274,5.0512714137896E-12,-0.645129946173579));
#56792=DIRECTION('center_axis',(0.,-1.,1.45983193964168E-32));
#56793=DIRECTION('ref_axis',(1.,0.,0.));
#56794=DIRECTION('center_axis',(-0.00988040017072651,0.601098527820397,
0.799113845171399));
#56795=DIRECTION('ref_axis',(0.999868662463102,-0.00432801644249017,0.0156181336247414));
#56796=DIRECTION('center_axis',(-0.0208642534513744,-0.601098528142146,
0.798902523711912));
#56797=DIRECTION('ref_axis',(0.999715452232994,-0.00330181997161638,0.0236244058434362));
#56798=DIRECTION('center_axis',(0.024277053557954,0.601098527995585,-0.798806099320784));
#56799=DIRECTION('ref_axis',(0.999605404196658,-0.00330185493271657,0.0278950471381458));
#56800=DIRECTION('center_axis',(0.0567768155390874,0.584828375911211,0.809167574700257));
#56801=DIRECTION('ref_axis',(0.99838687122767,-0.0330794214939016,-0.0461455006891631));
#56802=DIRECTION('center_axis',(-0.0414944532586696,-1.506057891401E-7,
-0.999138734285055));
#56803=DIRECTION('ref_axis',(-0.999015977122379,-0.0156751609033304,0.0414893574892793));
#56804=DIRECTION('',(0.0414470083239282,-8.32667268469771E-13,0.999140703555308));
#56805=DIRECTION('center_axis',(0.0215713944646267,0.584827952226312,0.810870483638189));
#56806=DIRECTION('ref_axis',(0.999689123680026,-0.0227607295853948,-0.0101786632031094));
#56807=DIRECTION('center_axis',(-0.0213714117579914,5.34377304442964E-10,
0.999771605297665));
#56808=DIRECTION('ref_axis',(-0.999648484588385,0.0156933905084443,-0.0213687799019016));
#56809=DIRECTION('',(0.0213713417387848,-2.40918396339775E-11,-0.999771606794414));
#56810=DIRECTION('',(0.735806627489012,0.,0.677191706197917));
#56811=DIRECTION('center_axis',(-0.0869599395448373,-0.601098528164396,
-0.79442968748213));
#56812=DIRECTION('ref_axis',(0.995899323349845,-0.0324816836639048,-0.0844362361648036));
#56813=DIRECTION('',(0.722057103471606,8.00811321699473E-12,-0.691833462132467));
#56814=DIRECTION('center_axis',(0.,-1.,1.45983193964168E-32));
#56815=DIRECTION('ref_axis',(1.,0.,0.));
#56816=DIRECTION('center_axis',(0.0903530450352583,0.601098525620875,0.794050936495428));
#56817=DIRECTION('ref_axis',(0.995597099123901,-0.034538511957999,-0.0871407333444038));
#56818=DIRECTION('center_axis',(-0.0208642636661934,-0.601098529032989,
0.798902522774866));
#56819=DIRECTION('ref_axis',(0.999437987770463,-0.0335099891761658,0.000888384343415163));
#56820=DIRECTION('center_axis',(0.024277072871618,0.601098526825379,-0.798806099614384));
#56821=DIRECTION('ref_axis',(0.999425070919505,-0.0335100296281867,0.00515805504620711));
#56822=DIRECTION('',(0.104101785979659,3.88578058618678E-13,0.994566648423244));
#56823=DIRECTION('center_axis',(0.123030318886438,0.584827952145045,0.801772914873366));
#56824=DIRECTION('ref_axis',(0.992104105097463,-0.0526562728642782,-0.113827771553362));
#56825=DIRECTION('center_axis',(0.0414469144126123,6.97494215856958E-10,
0.999140707450994));
#56826=DIRECTION('ref_axis',(-0.999016412849288,0.0157729998147174,0.0414417583433199));
#56827=DIRECTION('',(-0.0414470083263993,-1.77358128161261E-10,-0.999140703555206));
#56828=DIRECTION('',(0.776875900241836,0.,0.629653742642285));
#56829=DIRECTION('',(0.677191706223117,6.51326541667497E-11,-0.735806627465819));
#56830=DIRECTION('center_axis',(0.,-1.,1.45983193964168E-32));
#56831=DIRECTION('ref_axis',(1.,0.,0.));
#56832=DIRECTION('center_axis',(-0.00215546144630236,0.601098531722126,
0.799172014742419));
#56833=DIRECTION('ref_axis',(0.99802351841858,0.0514849565616084,-0.0360327064102555));
#56834=DIRECTION('center_axis',(-0.167595112513565,0.601098533934261,-0.78140414048279));
#56835=DIRECTION('ref_axis',(0.983933795834039,0.052516527403456,-0.170634989861697));
#56836=DIRECTION('center_axis',(0.0646072654303257,0.584827923043277,0.808580361919891));
#56837=DIRECTION('ref_axis',(0.995196652945506,0.0219596691043631,-0.0954012311183076));
#56838=DIRECTION('center_axis',(-0.166350265005554,-1.31282301405503E-8,
-0.986066726612648));
#56839=DIRECTION('ref_axis',(-0.98594458454176,-0.0157391391446185,0.166329659747629));
#56840=DIRECTION('',(0.166345721446039,8.32667268468167E-13,0.986067493104096));
#56841=DIRECTION('center_axis',(0.0294084954526384,0.584827952321989,0.810624084627444));
#56842=DIRECTION('ref_axis',(0.997706929939182,0.0322834330428721,-0.0594866531442022));
#56843=DIRECTION('center_axis',(0.104101705406296,6.05294299319807E-10,
0.994566656856895));
#56844=DIRECTION('ref_axis',(-0.994444041449916,0.0157020800824323,0.104088871191121));
#56845=DIRECTION('',(-0.104101785979012,-8.32667268468189E-13,-0.994566648423312));
#56846=DIRECTION('',(0.814879198737093,0.,0.579630823426078));
#56847=DIRECTION('center_axis',(-0.0946350612128965,-0.601098527914393,
-0.793551992580436));
#56848=DIRECTION('ref_axis',(0.990470183691813,0.023272374490036,-0.135746866641933));
#56849=DIRECTION('',(0.629653742642401,1.43735365432657E-13,-0.776875900241742));
#56850=DIRECTION('center_axis',(0.,-1.,1.45983193964168E-32));
#56851=DIRECTION('ref_axis',(1.,0.,0.));
#56852=DIRECTION('center_axis',(0.0980243639847826,0.601098529928312,0.793140455016261));
#56853=DIRECTION('ref_axis',(0.990141773984808,0.0212180887973301,-0.13845237490923));
#56854=DIRECTION('center_axis',(0.170931915613415,-0.601098527019728,0.780681011066263));
#56855=DIRECTION('ref_axis',(0.980058905949232,0.0222452360632367,-0.19745807236496));
#56856=DIRECTION('center_axis',(-0.167595193935718,0.601098528699735,-0.78140412704609));
#56857=DIRECTION('ref_axis',(0.980893521143664,0.0222451917353439,-0.193269375802382));
#56858=DIRECTION('center_axis',(0.165440957208147,0.584827953375401,0.794106765258168));
#56859=DIRECTION('ref_axis',(0.980087919794378,-0.00784642889667977,-0.198408928797817));
#56860=DIRECTION('center_axis',(-0.22793372461516,-1.92270791500281E-9,
-0.973676649192667));
#56861=DIRECTION('ref_axis',(-0.973556979441473,-0.0156778482808568,0.227905710446399));
#56862=DIRECTION('',(0.227933166345677,7.77156117236961E-13,0.973676779881103));
#56863=DIRECTION('center_axis',(0.13077473776379,0.584827952253972,0.800546209924973));
#56864=DIRECTION('ref_axis',(0.986627807193293,0.00246180458131422,-0.162970885716307));
#56865=DIRECTION('center_axis',(0.16634562963675,7.10084872101303E-10,0.986067508591959));
#56866=DIRECTION('ref_axis',(-0.985946425819607,0.0156707406190697,0.166325203447917));
#56867=DIRECTION('',(-0.166345721446248,-6.37823127617725E-11,-0.986067493104061));
#56868=DIRECTION('',(0.849666541317975,1.64268989065366E-13,0.527320366157756));
#56869=DIRECTION('center_axis',(-0.19334727172034,-0.601098528097524,-0.77543367997353));
#56870=DIRECTION('ref_axis',(0.971515581559539,-0.00691952022034624,-0.236874639898302));
#56871=DIRECTION('',(0.579630823435965,2.34493981894383E-11,-0.814879198730061));
#56872=DIRECTION('center_axis',(0.,-1.,1.45983193964168E-32));
#56873=DIRECTION('ref_axis',(1.,0.,0.));
#56874=DIRECTION('center_axis',(0.196658270544328,0.601098527316492,0.774600597136652));
#56875=DIRECTION('ref_axis',(0.970849897117024,-0.008972048994066,-0.239520311465881));
#56876=DIRECTION('center_axis',(0.17093190968256,-0.601098528304482,0.780681011375619));
#56877=DIRECTION('ref_axis',(0.975532201644004,-0.00794572107663697,-0.219712969740464));
#56878=DIRECTION('center_axis',(-0.167595173693706,0.601098527646255,-0.781404132197982));
#56879=DIRECTION('ref_axis',(0.976461934154753,-0.0079457744237133,-0.215543396594667));
#56880=DIRECTION('center_axis',(0.263664517464618,0.584827952228799,0.767109697841202));
#56881=DIRECTION('ref_axis',(0.949715452909033,-0.0181546317278219,-0.312587536304022));
#56882=DIRECTION('center_axis',(-0.28862099104446,6.09872333951937E-10,
-0.957443430980919));
#56883=DIRECTION('ref_axis',(-0.957325731486259,-0.0156795066142757,0.288585510562525));
#56884=DIRECTION('',(0.28862106007695,2.06171937743006E-7,0.957443410171074));
#56885=DIRECTION('center_axis',(0.230084567703631,0.584827782535973,0.777841601149418));
#56886=DIRECTION('ref_axis',(0.963976804255236,-0.0273551074375476,-0.264575922855696));
#56887=DIRECTION('center_axis',(0.22793305193534,8.06705954572667E-10,0.973676806664019));
#56888=DIRECTION('ref_axis',(-0.97355676287983,0.0157023279251005,0.227904950250493));
#56889=DIRECTION('',(0.227933165424189,-1.29267412268658E-5,0.97367678001101));
#56890=DIRECTION('',(0.881100657021104,-7.62629077550825E-8,0.472928781315933));
#56891=DIRECTION('center_axis',(-0.288621063731909,-4.7686293377351E-10,
-0.95744340906931));
#56892=DIRECTION('ref_axis',(-0.739027824993722,-0.635772805081909,0.222779743700656));
#56893=DIRECTION('',(-0.527320366159318,0.,0.849666541317005));
#56894=DIRECTION('center_axis',(0.316586779693368,0.398564391592836,0.860766656346315));
#56895=DIRECTION('ref_axis',(4.1601212236768E-16,-0.907442263761735,0.420176793670209));
#56896=DIRECTION('center_axis',(-0.354719245873589,5.74456553038096E-5,
-0.934972862337121));
#56897=DIRECTION('ref_axis',(0.934972809691412,0.000362953207812999,-0.354719203600136));
#56898=DIRECTION('',(0.348169046786044,5.94973691579315E-5,0.937431763554106));
#56899=DIRECTION('center_axis',(0.218761792620593,0.590180063812006,0.777065486537834));
#56900=DIRECTION('ref_axis',(0.319216405899052,-0.795820911703122,0.51455802656348));
#56901=DIRECTION('center_axis',(0.83256476303904,0.550037558024637,0.065533198518315));
#56902=DIRECTION('ref_axis',(-0.551222471619054,0.834358308391653,-2.53035028927643E-17));
#56903=DIRECTION('center_axis',(-0.36617389431988,-0.477126091316635,0.798916373660925));
#56904=DIRECTION('ref_axis',(0.881353683148659,0.0976243413979602,0.462260936232889));
#56905=DIRECTION('center_axis',(-0.245072617360243,0.58482795139018,0.773250075650152));
#56906=DIRECTION('ref_axis',(0.958540024361042,0.0265489689952938,0.283718476562983));
#56907=DIRECTION('center_axis',(0.208331313444156,-5.80606616147636E-11,
-0.978058313107472));
#56908=DIRECTION('ref_axis',(-0.977937030187507,-0.0157477670561977,-0.208305479574549));
#56909=DIRECTION('center_axis',(-0.260557623648053,-0.000115441151282437,
0.965458290881704));
#56910=DIRECTION('ref_axis',(0.0229724391951117,-0.999717608876927,0.00608025812175752));
#56911=DIRECTION('',(0.269333009814414,-6.06958927297125E-10,-0.963047106752473));
#56912=DIRECTION('center_axis',(0.211595763952694,-0.60109852801139,-0.770654132733885));
#56913=DIRECTION('ref_axis',(0.969283978718163,0.0279220136873786,0.244354107294985));
#56914=DIRECTION('',(0.871424337485884,2.24206636476427E-10,-0.490529942039513));
#56915=DIRECTION('center_axis',(0.,-1.,1.45983193964168E-32));
#56916=DIRECTION('ref_axis',(1.,0.,0.));
#56917=DIRECTION('center_axis',(-0.208301504811785,0.601098530007901,0.771551061379275));
#56918=DIRECTION('ref_axis',(0.969999731793433,0.0258668087052201,0.241725936812905));
#56919=DIRECTION('center_axis',(-0.120828758075573,-0.601098526589866,0.789987957220493));
#56920=DIRECTION('ref_axis',(0.984886132128416,0.026894408524338,0.171102301361652));
#56921=DIRECTION('center_axis',(0.124202588650017,0.601098528934584,-0.789464549859785));
#56922=DIRECTION('ref_axis',(0.9841461808156,0.0268943571417947,0.175308266604853));
#56923=DIRECTION('center_axis',(-0.146226196689905,0.584827952222654,0.797868514042673));
#56924=DIRECTION('ref_axis',(0.983185511001358,-0.00326197145028403,0.182580422004266));
#56925=DIRECTION('center_axis',(0.146507367971168,-4.95981624200213E-10,
-0.989209578972101));
#56926=DIRECTION('ref_axis',(-0.989087916826879,-0.0156832196309275,-0.146489349131849));
#56927=DIRECTION('',(-0.146507431922664,8.32140417652522E-8,0.989209569500528));
#56928=DIRECTION('center_axis',(-0.180759154061673,0.584827969931817,0.790760629905371));
#56929=DIRECTION('ref_axis',(0.975949872003266,0.0070448013400457,0.217881201830008));
#56930=DIRECTION('center_axis',(-0.208331363027332,3.62541623983424E-10,
0.978058302546006));
#56931=DIRECTION('ref_axis',(-0.977938191179099,0.0156715280542195,-0.208305778704765));
#56932=DIRECTION('',(0.20833131448783,-1.48214773786036E-11,-0.978058312885164));
#56933=DIRECTION('',(0.595880409943404,-3.07809289804292E-8,0.803073182870453));
#56934=DIRECTION('center_axis',(0.603452029474063,0.793626260371976,0.077479074411271));
#56935=DIRECTION('ref_axis',(-0.796019110988665,0.605271488623754,1.14284199043117E-17));
#56936=DIRECTION('center_axis',(-0.690563370774189,0.471546674556346,0.548421338625551));
#56937=DIRECTION('ref_axis',(0.721325537428693,0.393420484789212,0.570008588708476));
#56938=DIRECTION('center_axis',(0.113338614706024,-0.60109852786219,-0.791097287454854));
#56939=DIRECTION('ref_axis',(0.989645761078243,-0.0022757685263134,0.143513373793104));
#56940=DIRECTION('',(0.838904150646891,7.72064248612649E-12,-0.544279180225937));
#56941=DIRECTION('center_axis',(0.,-1.,1.45983193964168E-32));
#56942=DIRECTION('ref_axis',(1.,0.,0.));
#56943=DIRECTION('center_axis',(-0.109958008733103,0.601098527808738,0.791574251843514));
#56944=DIRECTION('ref_axis',(0.990026928638139,-0.00432801871030212,0.140811749599867));
#56945=DIRECTION('center_axis',(-0.120828788033283,-0.601098528090992,0.789987951496256));
#56946=DIRECTION('ref_axis',(0.988871471812975,-0.0033018314369469,0.148735705678233));
#56947=DIRECTION('center_axis',(0.124202574739973,0.601098527983157,-0.789464552772601));
#56948=DIRECTION('ref_axis',(0.988227040359869,-0.00330185589360348,0.15295886521948));
#56949=DIRECTION('center_axis',(-0.0450828641579298,0.584828255987395,0.809903356183971));
#56950=DIRECTION('ref_axis',(0.996298020781173,-0.0330815410804403,0.0793464896971532));
#56951=DIRECTION('center_axis',(0.0840714036549145,-1.08148586559602E-7,
-0.996459732797809));
#56952=DIRECTION('ref_axis',(-0.9963373049844,-0.0156751635312903,-0.0840610727072327));
#56953=DIRECTION('',(-0.0841053488787986,1.16573417585502E-12,0.996456868253702));
#56954=DIRECTION('center_axis',(-0.0802277221050548,0.58482795222607,0.807180140303821));
#56955=DIRECTION('ref_axis',(0.993082001122573,-0.0227607296058987,0.115195868997946));
#56956=DIRECTION('center_axis',(-0.146507507156355,5.90512572813898E-10,
0.989209558358001));
#56957=DIRECTION('ref_axis',(-0.989087738351328,0.0156933905081884,-0.146489464936603));
#56958=DIRECTION('',(0.146507430631042,-2.16493489798574E-11,-0.989209569691827));
#56959=DIRECTION('',(0.64512994617575,0.,0.764072871228441));
#56960=DIRECTION('center_axis',(0.0132942055902067,-0.601098528115421,-0.799064342587754));
#56961=DIRECTION('ref_axis',(0.998629026253513,-0.0324816845862958,0.0410488500496337));
#56962=DIRECTION('',(0.803073192439769,8.15184858242782E-12,-0.595880397046754));
#56963=DIRECTION('center_axis',(0.,-1.,1.45983193964168E-32));
#56964=DIRECTION('ref_axis',(1.,0.,0.));
#56965=DIRECTION('center_axis',(-0.00988039429928425,0.601098525863136,
0.799113846716259));
#56966=DIRECTION('ref_axis',(0.998668148441378,-0.0345385076908348,0.0383278068138463));
#56967=DIRECTION('center_axis',(-0.12082876902967,-0.601098529374135,0.789987953426523));
#56968=DIRECTION('ref_axis',(0.991445777876212,-0.033509983014987,0.126144165817402));
#56969=DIRECTION('center_axis',(0.124202600035381,0.601098526561387,-0.789464549875535));
#56970=DIRECTION('ref_axis',(0.990897829041076,-0.033510034284593,0.130378564204122));
#56971=DIRECTION('',(-0.0213713417384466,-1.22124532708752E-12,0.999771606794421));
#56972=DIRECTION('center_axis',(0.0215713960453859,0.584827952145866,0.810870483654157));
#56973=DIRECTION('ref_axis',(0.998547470580346,-0.052656272850442,0.011413409967822));
#56974=DIRECTION('center_axis',(-0.0841054139654099,4.72602757267682E-10,
0.996456862760103));
#56975=DIRECTION('ref_axis',(-0.996332902031619,0.015772999814619,-0.0840949511332293));
#56976=DIRECTION('',(0.0841053488763018,-1.77691195068295E-10,-0.996456868253913));
#56977=DIRECTION('',(0.691833462135556,-1.43735365432298E-13,0.722057103468645));
#56978=DIRECTION('',(0.764072871250519,6.52763895321776E-11,-0.645129946149602));
#56979=DIRECTION('center_axis',(0.,-1.,1.45983193964168E-32));
#56980=DIRECTION('ref_axis',(1.,0.,0.));
#56981=DIRECTION('center_axis',(-0.102301277609593,0.601098531733207,0.792600153764575));
#56982=DIRECTION('ref_axis',(0.994669900505696,0.051484956462993,0.0893369368514132));
#56983=DIRECTION('center_axis',(-0.0683376730294128,0.601098533636227,-0.796247772559084));
#56984=DIRECTION('ref_axis',(0.997561418616392,0.0525165308253309,-0.0459698822939941));
#56985=DIRECTION('center_axis',(-0.037243854755886,0.584827930051135,0.810301911336156));
#56986=DIRECTION('ref_axis',(0.999306186748226,0.0219594825721155,0.030081992152864));
#56987=DIRECTION('center_axis',(-0.041450461752033,-9.62093338242311E-9,
-0.999140560291966));
#56988=DIRECTION('ref_axis',(-0.999016798817377,-0.0157391393471299,0.0414453275206271));
#56989=DIRECTION('',(0.0414470083237992,-3.88578058618537E-13,0.999140703555314));
#56990=DIRECTION('center_axis',(-0.0724215370767206,0.584827952320712,0.807917933426291));
#56991=DIRECTION('ref_axis',(0.997295367386491,0.0322834330589318,0.0660282525845819));
#56992=DIRECTION('center_axis',(-0.0213713965116663,3.99570979461207E-10,
0.999771605623575));
#56993=DIRECTION('ref_axis',(-0.999648348522012,0.0157020800826844,-0.0213687617397829));
#56994=DIRECTION('',(0.0213713417389734,-8.32667268468203E-13,-0.99977160679441));
#56995=DIRECTION('',(0.735806627488868,0.,0.677191706198074));
#56996=DIRECTION('center_axis',(0.0055695912840324,-0.601098528152127,-0.799155516220889));
#56997=DIRECTION('ref_axis',(0.999673624254888,0.023272368205861,-0.0105376395453706));
#56998=DIRECTION('',(0.722057103468578,1.43735365432649E-13,-0.691833462135626));
#56999=DIRECTION('center_axis',(0.,-1.,1.45983193964168E-32));
#57000=DIRECTION('ref_axis',(1.,0.,0.));
#57001=DIRECTION('center_axis',(-0.0021554625750434,0.601098529555253,0.799172016369192));
#57002=DIRECTION('ref_axis',(0.99968689416083,0.0212180991799879,-0.0132629525469103));
#57003=DIRECTION('center_axis',(0.0717387755805213,-0.601098527369297,0.795948558936236));
#57004=DIRECTION('ref_axis',(0.997078908551603,0.0222452268180101,-0.0730670924928601));
#57005=DIRECTION('center_axis',(-0.0683377528351415,0.601098528633598,-0.796247769486337));
#57006=DIRECTION('ref_axis',(0.997381958361871,0.0222451935625928,-0.0688068346721553));
#57007=DIRECTION('center_axis',(0.0646084828042011,0.584827953016284,0.808580242969443));
#57008=DIRECTION('ref_axis',(0.997226863465737,-0.00784645566254045,-0.0740068639777763));
#57009=DIRECTION('center_axis',(-0.104102226223653,-1.68828436960849E-9,
-0.994566602342588));
#57010=DIRECTION('ref_axis',(-0.994444365115028,-0.0156778483097638,0.104089431564132));
#57011=DIRECTION('',(0.1041017859799,0.,0.994566648423219));
#57012=DIRECTION('center_axis',(0.0294084947975279,0.584827952254149,0.810624084700154));
#57013=DIRECTION('ref_axis',(0.999273620325529,0.00246180457596316,-0.0380285582127298));
#57014=DIRECTION('center_axis',(0.0414469484098936,4.50535560692295E-10,
0.9991407060407));
#57015=DIRECTION('ref_axis',(-0.999018017961886,0.0156707406185484,0.0414418589830465));
#57016=DIRECTION('',(-0.0414470083243479,-6.41708908203792E-11,-0.999140703555291));
#57017=DIRECTION('',(0.776875900241734,1.64268989065426E-13,0.629653742642411));
#57018=DIRECTION('center_axis',(-0.0946350669774392,-0.601098528044088,
-0.793551991794744));
#57019=DIRECTION('ref_axis',(0.993543154944051,-0.00691952431293544,-0.11324362872632));
#57020=DIRECTION('',(0.677191706207041,2.34493981894341E-11,-0.735806627480616));
#57021=DIRECTION('center_axis',(0.,-1.,1.45983193964168E-32));
#57022=DIRECTION('ref_axis',(1.,0.,0.));
#57023=DIRECTION('center_axis',(0.0980243639266851,0.601098527314582,0.793140457004313));
#57024=DIRECTION('ref_axis',(0.993214310825923,-0.00897204908649078,-0.115951865469155));
#57025=DIRECTION('center_axis',(0.0717387832098065,-0.601098528296013,0.795948557548755));
#57026=DIRECTION('ref_axis',(0.995377175937633,-0.00794572215068903,-0.0957138606573088));
#57027=DIRECTION('center_axis',(-0.0683377344053666,0.601098527687643,-0.796247771782182));
#57028=DIRECTION('ref_axis',(0.995776990652027,-0.00794577121283169,-0.0914606451312635));
#57029=DIRECTION('center_axis',(0.165441105021194,0.584827952230366,0.794106735306661));
#57030=DIRECTION('ref_axis',(0.981404269600449,-0.0181546317031915,-0.191091781502323));
#57031=DIRECTION('center_axis',(-0.166345660993045,4.80436704184032E-10,
-0.986067503302277));
#57032=DIRECTION('ref_axis',(-0.98594628501969,-0.0156795066154144,0.16632521194386));
#57033=DIRECTION('',(0.166345718259841,2.06171493653946E-7,0.986067493641574));
#57034=DIRECTION('center_axis',(0.130780879082784,0.58482778253619,0.800545330659131));
#57035=DIRECTION('ref_axis',(0.989535715163695,-0.0273551074326196,-0.141671332713516));
#57036=DIRECTION('center_axis',(0.104101686357031,6.71216382327904E-10,
0.994566658850789));
#57037=DIRECTION('ref_axis',(-0.994444039572659,0.0157023279254252,0.104088851737994));
#57038=DIRECTION('',(0.104101785049356,-1.29267411913885E-5,0.994566648436613));
#57039=DIRECTION('',(0.814879221760606,-7.62629077551079E-8,0.57963079105826));
#57040=DIRECTION('center_axis',(-0.166345721435314,8.38219850921266E-12,
-0.986067493105906));
#57041=DIRECTION('ref_axis',(-0.761122075632713,-0.635772805085135,0.128398311121022));
#57042=DIRECTION('',(-0.629653742643417,0.,0.776875900240919));
#57043=DIRECTION('center_axis',(0.206207729991539,0.398564391592221,0.893658098965404));
#57044=DIRECTION('ref_axis',(7.977868849158E-17,-0.913286229119169,0.407318381246525));
#57045=DIRECTION('center_axis',(-0.234739006541716,5.74456595838224E-5,
-0.972058432146856));
#57046=DIRECTION('ref_axis',(0.972058374620108,0.000362947015312071,-0.234738971200731));
#57047=DIRECTION('',(0.227932275687214,5.94973691934203E-5,0.973676986561822));
#57048=DIRECTION('center_axis',(0.119644660393128,0.590180063811167,0.798356215933251));
#57049=DIRECTION('ref_axis',(0.252209298373921,-0.795820738081259,0.550508694439547));
#57050=DIRECTION('center_axis',(0.817786253531608,0.550037558024095,0.169364483577954));
#57051=DIRECTION('ref_axis',(-0.558100160389067,0.829773590188129,8.72788992253708E-17));
#57052=DIRECTION('center_axis',(-0.463417276442099,-0.477126090650508,0.746722921514768));
#57053=DIRECTION('ref_axis',(0.816467047629943,0.097624951635498,0.569079018197482));
#57054=DIRECTION('center_axis',(-0.340054078922432,0.584827951389632,0.736437024246896));
#57055=DIRECTION('ref_axis',(0.915422295871966,0.0265489690047848,0.401618192398304));
#57056=DIRECTION('center_axis',(0.329271775058143,2.52786593772104E-11,
-0.944235192179396));
#57057=DIRECTION('ref_axis',(-0.944118103453684,-0.0157477670564997,-0.329230944116365));
#57058=DIRECTION('center_axis',(-0.379507052682398,-0.000115441210108468,
0.925188836745043));
#57059=DIRECTION('ref_axis',(0.0230779722542089,-0.999690021762026,0.00934171215969518));
#57060=DIRECTION('',(0.387911046550329,-6.06126260028195E-10,-0.921696815641797));
#57061=DIRECTION('center_axis',(0.306515840649688,-0.601098528069313,-0.738057314159084));
#57062=DIRECTION('ref_axis',(0.931015195264333,0.0279220124474747,0.3639107959484));
#57063=DIRECTION('',(0.926032600098742,2.24206636476434E-10,-0.377443536908983));
#57064=DIRECTION('center_axis',(0.,-1.,1.45983193964168E-32));
#57065=DIRECTION('ref_axis',(1.,0.,0.));
#57066=DIRECTION('center_axis',(-0.30335997485622,0.60109852999791,0.739360049562854));
#57067=DIRECTION('ref_axis',(0.932054700806224,0.0258668088583444,0.361393058738691));
#57068=DIRECTION('center_axis',(-0.218887725620292,-0.601098526393931,0.768614809341988));
#57069=DIRECTION('ref_axis',(0.955675207654525,0.0268944127803095,0.293192066802092));
#57070=DIRECTION('center_axis',(0.222169359871822,0.60109852895906,-0.767672673746694));
#57071=DIRECTION('ref_axis',(0.954413942092609,0.0268943565695278,0.297272132437531));
#57072=DIRECTION('center_axis',(-0.245072600278341,0.584827952222495,0.773250080434561));
#57073=DIRECTION('ref_axis',(0.952549404908284,-0.00326197144980148,0.304366540130703));
#57074=DIRECTION('center_axis',(0.269332938029609,-5.8483345689954E-10,
-0.963047126828349));
#57075=DIRECTION('ref_axis',(-0.962928682384874,-0.0156832196315011,-0.269299812964139));
#57076=DIRECTION('',(-0.269333011080849,8.32135976759878E-8,0.963047106398288));
#57077=DIRECTION('center_axis',(-0.278442400876454,0.584827969931489,0.761870116870303));
#57078=DIRECTION('ref_axis',(0.940946460198289,0.00704480134837665,0.338482096741131));
#57079=DIRECTION('center_axis',(-0.329271851742164,6.46313079915493E-10,
0.944235165438296));
#57080=DIRECTION('ref_axis',(-0.944119207751262,0.015671528054241,-0.329231415213636));
#57081=DIRECTION('',(0.329271770815587,-1.32671651441181E-11,-0.944235193658851));
#57082=DIRECTION('',(0.490529956132169,-3.07809289804332E-8,0.871424329553044));
#57083=DIRECTION('center_axis',(0.588982927050323,0.793626260371225,0.15250072292425));
#57084=DIRECTION('ref_axis',(-0.803018883933449,0.595953582123875,-1.43142346962412E-16));
#57085=DIRECTION('center_axis',(-0.753853492062759,0.471546674560884,0.457546332315489));
#57086=DIRECTION('ref_axis',(0.64419412264145,0.39340505448244,0.655931700302616));
#57087=DIRECTION('center_axis',(0.211595757716834,-0.601098528031622,-0.770654134430262));
#57088=DIRECTION('ref_axis',(0.963855097930843,-0.00227572441773332,0.26641728786079));
#57089=DIRECTION('',(0.900505410469431,5.19500677922309E-12,-0.434844806471553));
#57090=DIRECTION('center_axis',(0.,-1.,1.45983193964168E-32));
#57091=DIRECTION('ref_axis',(1.,0.,0.));
#57092=DIRECTION('center_axis',(-0.208301530005171,0.601098527857505,0.771551056252952));
#57093=DIRECTION('ref_axis',(0.96457187601466,-0.0043280109716603,0.263784693116541));
#57094=DIRECTION('center_axis',(-0.218887748539973,-0.601098528126118,0.768614801460209));
#57095=DIRECTION('ref_axis',(0.962432400878757,-0.00330182340838835,0.271501329096068));
#57096=DIRECTION('center_axis',(0.222169344354683,0.601098527988436,-0.767672678997465));
#57097=DIRECTION('ref_axis',(0.961263746067348,-0.00330185516210308,0.275610428411295));
#57098=DIRECTION('center_axis',(-0.146235178803069,0.584828255987149,0.797866645172904));
#57099=DIRECTION('ref_axis',(0.978497161183396,-0.0330815410865203,0.203590071455794));
#57100=DIRECTION('center_axis',(0.208297997691912,-1.08134170125211E-7,
-0.978065408936196));
#57101=DIRECTION('ref_axis',(-0.977945241313742,-0.0156751635311632,-0.208272403933114));
#57102=DIRECTION('',(-0.20833131448759,0.,0.978058312885215));
#57103=DIRECTION('center_axis',(-0.180761599633245,0.584827952226279,0.790760083965325));
#57104=DIRECTION('ref_axis',(0.970813382164798,-0.0227607295898355,0.238753693580401));
#57105=DIRECTION('center_axis',(-0.269333108956724,7.92216648094451E-10,
0.963047079025582));
#57106=DIRECTION('ref_axis',(-0.962928480895791,0.0156933905078548,-0.269299940909932));
#57107=DIRECTION('',(0.269333009823161,-2.16493489798119E-11,-0.963047106750027));
#57108=DIRECTION('',(0.544279180229334,0.,0.838904150644687));
#57109=DIRECTION('center_axis',(0.113338686509647,-0.601098527841723,-0.791097277183269));
#57110=DIRECTION('ref_axis',(0.985609753935629,-0.0324816895753882,0.165886566030155));
#57111=DIRECTION('',(0.871424337430542,8.17238220606246E-12,-0.490529942137829));
#57112=DIRECTION('center_axis',(0.,-1.,1.45983193964168E-32));
#57113=DIRECTION('ref_axis',(1.,0.,0.));
#57114=DIRECTION('center_axis',(-0.109958010163819,0.60109852597944,0.791574253033889));
#57115=DIRECTION('ref_axis',(0.985989603468124,-0.034538505663073,0.163191891585745));
#57116=DIRECTION('center_axis',(-0.218887753379354,-0.601098529013112,0.768614799388362));
#57117=DIRECTION('ref_axis',(0.967817873192568,-0.0335099896073441,0.249410595054682));
#57118=DIRECTION('center_axis',(0.222169363956345,0.601098526776724,-0.767672674273408));
#57119=DIRECTION('ref_axis',(0.966743538100934,-0.0335100303655534,0.25354291432613));
#57120=DIRECTION('',(-0.146507430631127,1.1657341758556E-12,0.989209569691815));
#57121=DIRECTION('center_axis',(-0.0802277205987724,0.584827952146903,0.807180140510893));
#57122=DIRECTION('ref_axis',(0.989243145943866,-0.0526562728355991,0.136474595196858));
#57123=DIRECTION('center_axis',(-0.208331408096651,7.10677786846695E-10,
0.978058292946012));
#57124=DIRECTION('ref_axis',(-0.977936621025492,0.0157729998146215,-0.208305491368066));
#57125=DIRECTION('',(0.208331314485092,-1.75748304775633E-10,-0.978058312885747));
#57126=DIRECTION('',(0.59588039705036,0.,0.803073192437093));
#57127=DIRECTION('',(0.838904150663342,6.51326541667559E-11,-0.544279180200581));
#57128=DIRECTION('center_axis',(0.,-1.,1.45983193964168E-32));
#57129=DIRECTION('ref_axis',(1.,0.,0.));
#57130=DIRECTION('center_axis',(-0.200833745921226,0.60109853150529,0.773528513967929));
#57131=DIRECTION('ref_axis',(0.975629743199405,0.0514849590709439,0.213297686752872));
#57132=DIRECTION('center_axis',(0.0319974973800043,0.601098533599825,-0.798534102631539));
#57133=DIRECTION('ref_axis',(0.995456902887003,0.0525165311962358,0.0794202017482328));
#57134=DIRECTION('center_axis',(-0.138507934550866,0.584827930050956,0.799244545992506));
#57135=DIRECTION('ref_axis',(0.987656085638451,0.0219594825737406,0.155091062367971));
#57136=DIRECTION('center_axis',(0.08410187096805,-9.88649956170652E-9,-0.996457161798576));
#57137=DIRECTION('ref_axis',(-0.996333732730334,-0.0157391393484628,-0.0840914532887217));
#57138=DIRECTION('',(-0.0841053488788927,-7.77156117238321E-13,0.996456868253694));
#57139=DIRECTION('center_axis',(-0.17310943869208,0.584827952319961,0.792470433783466));
#57140=DIRECTION('ref_axis',(0.981155861131183,0.0322834330681012,0.190501853317139));
#57141=DIRECTION('center_axis',(-0.146507509371627,5.94611736450723E-10,
0.989209558029906));
#57142=DIRECTION('ref_axis',(-0.989087603071883,0.0157020800827092,-0.146489447164611));
#57143=DIRECTION('',(0.146507430631453,-1.22124532708676E-12,-0.989209569691767));
#57144=DIRECTION('',(0.645129946175734,0.,0.764072871228454));
#57145=DIRECTION('center_axis',(0.105686425993003,-0.601098527976467,-0.792155880509228));
#57146=DIRECTION('ref_axis',(0.993111614765757,0.0232723728235476,0.114837786814762));
#57147=DIRECTION('',(0.803073192437276,0.,-0.595880397050114));
#57148=DIRECTION('center_axis',(0.,-1.,1.45983193964168E-32));
#57149=DIRECTION('ref_axis',(1.,0.,0.));
#57150=DIRECTION('center_axis',(-0.10230128097518,0.601098529510368,0.792600155015952));
#57151=DIRECTION('ref_axis',(0.993466352943827,0.0212181003141552,0.112135622295283));
#57152=DIRECTION('center_axis',(-0.0285857038531819,-0.601098527168134,
0.798663519995448));
#57153=DIRECTION('ref_axis',(0.998374378768266,0.0222452321645403,0.0524761799774345));
#57154=DIRECTION('center_axis',(0.0319974136827314,0.601098528532173,-0.798534109799996));
#57155=DIRECTION('ref_axis',(0.998141086949402,0.0222451964194356,0.056740829917499));
#57156=DIRECTION('center_axis',(-0.0372429508028461,0.584827953016271,0.810301936309112));
#57157=DIRECTION('ref_axis',(0.9986389513593,-0.00784645567732753,0.0515623696245816));
#57158=DIRECTION('center_axis',(0.0213710252196031,-6.99985568850361E-10,
-0.999771613560349));
#57159=DIRECTION('ref_axis',(-0.999648736613809,-0.0156778483084573,-0.0213683986024217));
#57160=DIRECTION('',(-0.0213713417383099,-4.44089209849764E-13,0.999771606794424));
#57161=DIRECTION('center_axis',(-0.0724215376820377,0.584827952254425,0.807917933420013));
#57162=DIRECTION('ref_axis',(0.99616029153121,0.00246180456054646,0.0875135023568358));
#57163=DIRECTION('center_axis',(-0.084105442047678,7.13530268223119E-10,
0.996456860389834));
#57164=DIRECTION('ref_axis',(-0.996334501868839,0.0156707406187732,-0.0840951144492399));
#57165=DIRECTION('',(0.0841053488781944,-6.4226401971558E-11,-0.996456868253753));
#57166=DIRECTION('',(0.691833462135674,1.64268989065485E-13,0.722057103468532));
#57167=DIRECTION('center_axis',(0.00556959465845934,-0.601098528032363,
-0.799155516287454));
#57168=DIRECTION('ref_axis',(0.999901960586244,-0.0069195250739992,0.0121733063928809));
#57169=DIRECTION('',(0.764072871236398,2.34493981894309E-11,-0.645129946166326));
#57170=DIRECTION('center_axis',(0.,-1.,1.45983193964168E-32));
#57171=DIRECTION('ref_axis',(1.,0.,0.));
#57172=DIRECTION('center_axis',(-0.00215545266561574,0.601098527372563,
0.799172018037633));
#57173=DIRECTION('ref_axis',(0.999915141548093,-0.00897204484915501,0.00944521646556398));
#57174=DIRECTION('center_axis',(-0.0285856996086749,-0.601098528338824,
0.798663519266269));
#57175=DIRECTION('ref_axis',(0.999524457407752,-0.00794571891958214,0.0297947074929481));
#57176=DIRECTION('center_axis',(0.0319974503381975,0.6010985275747,-0.798534109051944));
#57177=DIRECTION('ref_axis',(0.99938804962766,-0.00794577923852444,0.0340645101786992));
#57178=DIRECTION('center_axis',(0.0646085875664995,0.584827952230155,0.808580235167139));
#57179=DIRECTION('ref_axis',(0.997615754687303,-0.0181546317371957,-0.0665823951669649));
#57180=DIRECTION('center_axis',(-0.0414482896573108,-3.66455749607626E-9,
-0.999140650401376));
#57181=DIRECTION('ref_axis',(-0.999017825024053,-0.0156795063469686,0.0414431944343749));
#57182=DIRECTION('',(0.0414470050956375,2.06171105075987E-7,0.999140703689205));
#57183=DIRECTION('center_axis',(0.0294146978912214,0.584827782535925,0.810623982079288));
#57184=DIRECTION('ref_axis',(0.999489056721735,-0.0273551074375189,-0.0165325010382245));
#57185=DIRECTION('center_axis',(-0.0213714686382134,8.82110719332692E-10,
0.999771604081775));
#57186=DIRECTION('ref_axis',(-0.999648343088967,0.0157023279257171,-0.021368833781832));
#57187=DIRECTION('',(-0.0213713426633531,-1.29267419730502E-5,0.999771606691081));
#57188=DIRECTION('',(0.735806654387714,-7.62629077551357E-8,0.677191676970969));
#57189=DIRECTION('center_axis',(-0.0414472069397243,-1.61525008678803E-7,
-0.999140695316165));
#57190=DIRECTION('ref_axis',(-0.771212966511826,-0.635772804014447,0.0319922171728849));
#57191=DIRECTION('',(-0.722057103469967,0.,0.691833462134176));
#57192=DIRECTION('center_axis',(0.0925766612049255,0.39856439159139,0.912456019518494));
#57193=DIRECTION('ref_axis',(-1.04051723405416E-16,-0.916391407625922,0.40028338465315));
#57194=DIRECTION('center_axis',(-0.111056792829436,5.74456674606717E-5,
-0.993814059805171));
#57195=DIRECTION('ref_axis',(0.993813998287295,0.000362990317359139,-0.111056764972918));
#57196=DIRECTION('',(0.104100876440593,5.94973699395232E-5,0.994566741845093));
#57197=DIRECTION('center_axis',(0.0186406606636707,0.590180063817314,0.807056390869072));
#57198=DIRECTION('ref_axis',(0.181219010772305,-0.795821359149822,0.577778534090387));
#57199=DIRECTION('center_axis',(0.790110766284182,0.550037558023235,0.270524789558478));
#57200=DIRECTION('ref_axis',(-0.571341150189064,0.820712672072655,1.13123986132218E-16));
#57201=DIRECTION('center_axis',(-0.553352291407227,-0.477126089849265,0.682753202833588));
#57202=DIRECTION('ref_axis',(0.73870537475839,0.0976228476931799,0.666921396351429));
#57203=DIRECTION('center_axis',(-0.429672684490192,0.584827951390324,0.688009921058984));
#57204=DIRECTION('ref_axis',(0.857867810942039,0.0265489689937178,0.513184149399496));
#57205=DIRECTION('center_axis',(0.44501941704254,-1.263031542495E-11,-0.895520920166088));
#57206=DIRECTION('ref_axis',(-0.895409872194088,-0.0157477670560035,-0.444964232955994));
#57207=DIRECTION('center_axis',(-0.492471439238968,-0.000115441170765423,
0.870328597833736));
#57208=DIRECTION('ref_axis',(0.0217041865571253,-0.999690621869625,0.0121486143990027));
#57209=DIRECTION('',(0.500371494355022,-6.08124661472372E-10,-0.865810815153589));
#57210=DIRECTION('center_axis',(0.396601983992574,-0.601098527988962,-0.693820888949488));
#57211=DIRECTION('ref_axis',(0.878063744427938,0.0279220141999334,0.47772839756938));
#57212=DIRECTION('',(0.966036775423212,2.24062901110976E-10,-0.258404621727094));
#57213=DIRECTION('center_axis',(0.,-1.,1.45983193964168E-32));
#57214=DIRECTION('ref_axis',(1.,0.,0.));
#57215=DIRECTION('center_axis',(-0.393634287432195,0.601098529677143,0.69550888231404));
#57216=DIRECTION('ref_axis',(0.879410605621152,0.0258668162395267,0.475360804588124));
#57217=DIRECTION('center_axis',(-0.313494723667525,-0.601098526808639,0.735120139365741));
#57218=DIRECTION('ref_axis',(0.911392708689532,0.0268944037202345,0.410658034861234));
#57219=DIRECTION('center_axis',(0.316632373895327,0.601098528588605,-0.733774146948517));
#57220=DIRECTION('ref_axis',(0.909630029913998,0.0268943649857957,0.414547828134064));
#57221=DIRECTION('center_axis',(-0.340054062561776,0.584827952222567,0.736437031140063));
#57222=DIRECTION('ref_axis',(0.906891025673923,-0.00326197144877692,0.421352616100064));
#57223=DIRECTION('center_axis',(0.387910953050161,-7.94897451911712E-10,
-0.921696854992853));
#57224=DIRECTION('ref_axis',(-0.921583496190756,-0.0156832196313773,-0.387863244160642));
#57225=DIRECTION('',(-0.387911047762012,8.32148189213521E-8,0.921696815131837));
#57226=DIRECTION('center_axis',(-0.371734444666745,0.584827969931767,0.720964456983695));
#57227=DIRECTION('ref_axis',(0.891103760630804,0.00704480133835922,0.453744926763641));
#57228=DIRECTION('center_axis',(-0.445019486730157,6.04376373905928E-10,
0.895520885535579));
#57229=DIRECTION('ref_axis',(-0.895410910250426,0.0156715280542697,-0.444964835703843));
#57230=DIRECTION('',(0.44501941462051,-1.52100554372157E-11,-0.89552092136969));
#57231=DIRECTION('',(0.377443551884433,-3.07807852450739E-8,0.926032593994867));
#57232=DIRECTION('center_axis',(0.565225212024928,0.793626260371114,0.22511734393586));
#57233=DIRECTION('ref_axis',(-0.814533996871954,0.580115822866261,8.98799277858797E-17));
#57234=DIRECTION('center_axis',(-0.805254893437658,0.471546674537444,0.359455547081114));
#57235=DIRECTION('ref_axis',(0.556903411321164,0.393401148446506,0.731501282883237));
#57236=DIRECTION('center_axis',(0.306515838186029,-0.601098528034889,-0.738057315210279));
#57237=DIRECTION('ref_axis',(0.922863871900687,-0.00227572338068341,0.38511958535443));
#57238=DIRECTION('',(0.947905162033646,5.19500677922244E-12,-0.318552670354477));
#57239=DIRECTION('center_axis',(0.,-1.,1.45983193964168E-32));
#57240=DIRECTION('ref_axis',(1.,0.,0.));
#57241=DIRECTION('center_axis',(-0.303359993099232,0.601098527830073,0.73936004384018));
#57242=DIRECTION('ref_axis',(0.92390495204079,-0.0043280147898287,0.38259757955649));
#57243=DIRECTION('center_axis',(-0.31349473879885,-0.601098528107193,0.735120131851119));
#57244=DIRECTION('ref_axis',(0.920815192023725,-0.00330182805213655,0.389985230579088));
#57245=DIRECTION('center_axis',(0.316632370525574,0.601098527993511,-0.733774148890099));
#57246=DIRECTION('ref_axis',(0.919140748588481,-0.00330185426789301,0.393915450373046));
#57247=DIRECTION('center_axis',(-0.245081277370425,0.584828255988135,0.773247100531491));
#57248=DIRECTION('ref_axis',(0.945264816817517,-0.0330815410633406,0.32462291620867));
#57249=DIRECTION('center_axis',(0.329239579421866,-1.08354798316671E-7,
-0.944246418760538));
#57250=DIRECTION('ref_axis',(-0.944130406444208,-0.0156751635322327,-0.329199126480815));
#57251=DIRECTION('',(-0.329271770815384,1.22124532708837E-12,0.944235193658922));
#57252=DIRECTION('center_axis',(-0.278444758713474,0.584827952226039,0.761869268733222));
#57253=DIRECTION('ref_axis',(0.933234456240481,-0.0227607295977756,0.358546229758049));
#57254=DIRECTION('center_axis',(-0.387911125646508,6.56837119634826E-10,
0.921696782352884));
#57255=DIRECTION('ref_axis',(-0.921583276463325,0.0156933905082965,-0.387863354852553));
#57256=DIRECTION('',(0.387911046558472,-2.28705943069176E-11,-0.92169681563837));
#57257=DIRECTION('',(0.434844806474066,0.,0.900505410468217));
#57258=DIRECTION('center_axis',(0.211595754170762,-0.601098527745205,-0.770654135627296));
#57259=DIRECTION('ref_axis',(0.957046827522298,-0.0324816913084358,0.288108156183139));
#57260=DIRECTION('',(0.926032600056353,8.00811321699569E-12,-0.377443537012983));
#57261=DIRECTION('center_axis',(0.,-1.,1.45983193964168E-32));
#57262=DIRECTION('ref_axis',(1.,0.,0.));
#57263=DIRECTION('center_axis',(-0.208301522446814,0.601098526095677,0.771551059666141));
#57264=DIRECTION('ref_axis',(0.957761412761915,-0.0345385035991132,0.28548234269992));
#57265=DIRECTION('center_axis',(-0.313494748360086,-0.601098528584498,0.735120127383408));
#57266=DIRECTION('ref_axis',(0.928926899735521,-0.0335099974581725,0.36874367115668));
#57267=DIRECTION('center_axis',(0.316632396784893,0.601098526555786,-0.733774138736653));
#57268=DIRECTION('ref_axis',(0.927343121189809,-0.0335100342769605,0.372708751151217));
#57269=DIRECTION('',(-0.269333009823004,1.16573417585691E-12,0.96304710675007));
#57270=DIRECTION('center_axis',(-0.180761598123538,0.5848279521463,0.790760084369583));
#57271=DIRECTION('ref_axis',(0.964337865952839,-0.0526562728443061,0.25938349450123));
#57272=DIRECTION('center_axis',(-0.329271845805718,5.83638447949411E-10,
0.944235167508442));
#57273=DIRECTION('ref_axis',(-0.944117703234743,0.0157729998148134,-0.329230883903067));
#57274=DIRECTION('',(0.329271770813222,-1.76914038951379E-10,-0.944235193659676));
#57275=DIRECTION('',(0.490529942141599,0.,0.871424337428419));
#57276=DIRECTION('',(0.900505410483596,6.72270837774942E-11,-0.434844806442219));
#57277=DIRECTION('center_axis',(0.,-1.,1.45983193964168E-32));
#57278=DIRECTION('ref_axis',(1.,0.,0.));
#57279=DIRECTION('center_axis',(-0.296198939617034,0.601098531624116,0.74225786856663));
#57280=DIRECTION('ref_axis',(0.941203323148457,0.0514849577008644,0.333894599574238));
#57281=DIRECTION('center_axis',(0.13182805295787,0.601098533827196,-0.788227072031995));
#57282=DIRECTION('ref_axis',(0.977653436616125,0.0525165286099951,0.203557785641906));
#57283=DIRECTION('center_axis',(-0.237587661479048,0.584827930050785,0.775582616711741));
#57284=DIRECTION('ref_axis',(0.960430058059983,0.0219594825764484,0.277654253883985));
#57285=DIRECTION('center_axis',(0.208327868813298,-1.01451858201418E-8,
-0.978059046824735));
#57286=DIRECTION('ref_axis',(-0.977937896713006,-0.0157391393483165,-0.208302063516224));
#57287=DIRECTION('',(-0.208331314487397,1.22124532708716E-12,0.978058312885256));
#57288=DIRECTION('center_axis',(-0.271067301023581,0.584827952320365,0.764525202004853));
#57289=DIRECTION('ref_axis',(0.94954294083552,0.0322834330622836,0.311971126002302));
#57290=DIRECTION('center_axis',(-0.269333079626839,5.38133350324857E-10,
0.963047087228201));
#57291=DIRECTION('ref_axis',(-0.962928357716265,0.0157020800824384,-0.269299874836475));
#57292=DIRECTION('',(0.269333009823372,0.,-0.963047106749968));
#57293=DIRECTION('',(0.544279180229277,0.,0.838904150644725));
#57294=DIRECTION('center_axis',(0.204136518769429,-0.601098527889654,-0.772663472330347));
#57295=DIRECTION('ref_axis',(0.970887641095373,0.0232723751933657,0.238402149573196));
#57296=DIRECTION('',(0.871424337428443,0.,-0.490529942141556));
#57297=DIRECTION('center_axis',(0.,-1.,1.45983193964168E-32));
#57298=DIRECTION('ref_axis',(1.,0.,0.));
#57299=DIRECTION('center_axis',(-0.200833748756779,0.601098529431724,0.773528514843065));
#57300=DIRECTION('ref_axis',(0.971578253134806,0.0212181025282827,0.235765752730581));
#57301=DIRECTION('center_axis',(-0.128459387649655,-0.601098527378134,0.788783079248353));
#57302=DIRECTION('ref_axis',(0.983924888080242,0.0222452265883128,0.177191886130033));
#57303=DIRECTION('center_axis',(0.131827962105105,0.6010985284313,-0.788227091341664));
#57304=DIRECTION('ref_axis',(0.983158935264301,0.0222451991726764,0.18139365789281));
#57305=DIRECTION('center_axis',(-0.13850704083771,0.584827953016387,0.799244684066803));
#57306=DIRECTION('ref_axis',(0.98430190643568,-0.00784645568629959,0.176318433863986));
#57307=DIRECTION('center_axis',(0.146507087593992,-9.36218342805786E-10,
-0.989209620497459));
#57308=DIRECTION('ref_axis',(-0.989088041674773,-0.015677848308132,-0.146489081123439));
#57309=DIRECTION('',(-0.14650743063097,-3.88578058618891E-13,0.989209569691838));
#57310=DIRECTION('center_axis',(-0.173109439351868,0.584827952253358,0.792470433688492));
#57311=DIRECTION('ref_axis',(0.977336919849494,0.00246180460537174,0.211675422799128));
#57312=DIRECTION('center_axis',(-0.208331386153898,5.54965824874705E-10,
0.97805829761993));
#57313=DIRECTION('ref_axis',(-0.977938198323729,0.0156707406186644,-0.208305804402567));
#57314=DIRECTION('',(0.208331314486879,-6.46149800301645E-11,-0.978058312885366));
#57315=DIRECTION('',(0.595880397050194,1.64268989065517E-13,0.803073192437217));
#57316=DIRECTION('center_axis',(0.105686416211157,-0.601098527992137,-0.792155881802394));
#57317=DIRECTION('ref_axis',(0.990491715704822,-0.00691952841778068,0.137398257800428));
#57318=DIRECTION('',(0.838904150651368,2.34493981894334E-11,-0.544279180219037));
#57319=DIRECTION('center_axis',(0.,-1.,1.45983193964168E-32));
#57320=DIRECTION('ref_axis',(1.,0.,0.));
#57321=DIRECTION('center_axis',(-0.102301275627061,0.601098527426145,0.792600157286886));
#57322=DIRECTION('ref_axis',(0.99084671183987,-0.00897204111701711,0.134693341016966));
#57323=DIRECTION('center_axis',(-0.128459379962898,-0.601098528294563,0.788783079801829));
#57324=DIRECTION('ref_axis',(0.987908640739109,-0.00794572241207701,0.154833404174798));
#57325=DIRECTION('center_axis',(0.131827982572337,0.601098527746006,-0.7882270884412));
#57326=DIRECTION('ref_axis',(0.987238163854929,-0.00794576686894387,0.159052420972501));
#57327=DIRECTION('center_axis',(-0.0372428459221002,0.584827952230008,0.810301941697092));
#57328=DIRECTION('ref_axis',(0.99809424337453,-0.0181546317010637,0.0589770352800358));
#57329=DIRECTION('center_axis',(0.0841052618395418,-6.64941428738438E-10,
-0.996456875600195));
#57330=DIRECTION('ref_axis',(-0.996334380141064,-0.0156795066176087,-0.0840949226835356));
#57331=DIRECTION('',(-0.0841053520982985,2.0617116058726E-7,0.996456867981941));
#57332=DIRECTION('center_axis',(-0.0724153706974204,0.584827782536221,0.807918609056953));
#57333=DIRECTION('ref_axis',(0.993679858788329,-0.0273551074191281,0.108867058086894));
#57334=DIRECTION('center_axis',(-0.146507522166042,6.11855090107436E-10,
0.989209556134981));
#57335=DIRECTION('ref_axis',(-0.989087597326991,0.0157023279255864,-0.146489459387487));
#57336=DIRECTION('',(-0.146507431535708,-1.29267420441721E-5,0.98920956947338));
#57337=DIRECTION('',(0.645129976525409,-7.62630514905186E-8,0.764072845603297));
#57338=DIRECTION('center_axis',(0.0841053482901251,-4.80180366554845E-10,
-0.996456868303389));
#57339=DIRECTION('ref_axis',(-0.769141387593958,-0.635772805081689,-0.0649189202667612));
#57340=DIRECTION('',(-0.803073192438327,0.,0.595880397048698));
#57341=DIRECTION('center_axis',(-0.0225143968314784,0.398564391590973,0.916863963568769));
#57342=DIRECTION('ref_axis',(1.32509733837405E-17,-0.917096430234536,0.398665445770097));
#57343=DIRECTION('center_axis',(0.0143768528772085,5.74456683306679E-5,
-0.999896646059653));
#57344=DIRECTION('ref_axis',(0.99989658156764,0.000362902000896798,0.0143768727992233));
#57345=DIRECTION('',(-0.0213722558148664,5.94973699395278E-5,0.999771585484128));
#57346=DIRECTION('center_axis',(-0.0826573138804223,0.590180063811489,0.803028804428297));
#57347=DIRECTION('ref_axis',(0.107377222157672,-0.795821081622156,0.595935347338487));
#57348=DIRECTION('center_axis',(0.749974760262434,0.550037558024859,0.367418758001486));
#57349=DIRECTION('ref_axis',(-0.591402864737045,0.806376246910099,3.44718433429239E-16));
#57350=DIRECTION('center_axis',(-0.634560609802729,-0.477126090219829,0.608016057779997));
#57351=DIRECTION('ref_axis',(0.649293907906614,0.097621054247684,0.754246346310626));
#57352=DIRECTION('center_axis',(-0.512515095180752,0.584827951389499,0.628732490400669));
#57353=DIRECTION('ref_axis',(0.786784238152812,0.0265489690042029,0.616656885828021));
#57354=DIRECTION('center_axis',(0.55374883837593,-1.94416449583736E-11,
-0.832683747888301));
#57355=DIRECTION('ref_axis',(-0.832580491962753,-0.0157477670575025,-0.553680171430911));
#57356=DIRECTION('center_axis',(-0.597669249882254,-0.000115441202897984,
0.801742760752171));
#57357=DIRECTION('ref_axis',(0.0200236790427926,-0.999690210189126,0.0147829607864248));
#57358=DIRECTION('',(0.604940784786562,-6.06070748877474E-10,-0.79627046089995));
#57359=DIRECTION('center_axis',(0.480433465069761,-0.601098528305781,-0.638642501646804));
#57360=DIRECTION('ref_axis',(0.811264710240501,0.0279220072711538,0.58401192747096));
#57361=DIRECTION('',(0.990805973716838,2.24350371841898E-10,-0.135290511297095));
#57362=DIRECTION('center_axis',(0.,-1.,1.45983193964168E-32));
#57363=DIRECTION('ref_axis',(1.,0.,0.));
#57364=DIRECTION('center_axis',(-0.477700744076694,0.601098529565722,0.640689126536809));
#57365=DIRECTION('ref_axis',(0.812897681593187,0.0258668187358074,0.581831820158464));
#57366=DIRECTION('center_axis',(-0.403157705739844,-0.601098526727984,0.690032191617197));
#57367=DIRECTION('ref_axis',(0.852737006755842,0.0268944054952872,0.521647666784911));
#57368=DIRECTION('center_axis',(0.406101919085641,0.601098528571327,-0.688303559677229));
#57369=DIRECTION('ref_axis',(0.850500705913757,0.0268943653428166,0.52528586726944));
#57370=DIRECTION('center_axis',(-0.429672669136689,0.584827952222573,0.688009929940045));
#57371=DIRECTION('ref_axis',(0.846930433215634,-0.00326197144994845,0.531693709606798));
#57372=DIRECTION('center_axis',(0.500371425977371,-6.18913571759043E-10,
-0.865810854670564));
#57373=DIRECTION('ref_axis',(-0.86570436924588,-0.015683219630985,-0.500309885661476));
#57374=DIRECTION('',(-0.500371495493563,8.32124319419546E-8,0.865810814495596));
#57375=DIRECTION('center_axis',(-0.459164014240661,0.584827969931258,0.668688756905995));
#57376=DIRECTION('ref_axis',(0.827207822420984,0.00704480135458538,0.561851928268835));
#57377=DIRECTION('center_axis',(-0.553748923309602,7.92180262186616E-10,
0.832683691405961));
#57378=DIRECTION('ref_axis',(-0.83258143289862,0.0156715280539033,-0.55368091966487));
#57379=DIRECTION('',(0.553748836415073,-1.48214773785855E-11,-0.832683749192304));
#57380=DIRECTION('',(0.258404637349547,-3.07809289804395E-8,0.96603677124437));
#57381=DIRECTION('center_axis',(0.532553557756658,0.793626260371024,0.294183729954989));
#57382=DIRECTION('ref_axis',(-0.830371106911542,0.557210754388769,8.10631680189143E-17));
#57383=DIRECTION('center_axis',(-0.843956944130239,0.471546674587893,0.25569593297401));
#57384=DIRECTION('ref_axis',(0.460838052815712,0.393422457595482,0.795516850190211));
#57385=DIRECTION('center_axis',(0.396601985414726,-0.601098528055261,-0.693820888079118));
#57386=DIRECTION('ref_axis',(0.867318528806137,-0.00227571901415262,0.497748320632553));
#57387=DIRECTION('',(0.980355882941517,5.19500677922323E-12,-0.197236768331765));
#57388=DIRECTION('center_axis',(0.,-1.,1.45983193964168E-32));
#57389=DIRECTION('ref_axis',(1.,0.,0.));
#57390=DIRECTION('center_axis',(-0.393634297367351,0.601098527846508,0.695508878273221));
#57391=DIRECTION('ref_axis',(0.868667492214279,-0.00432801246559104,0.495376681201541));
#57392=DIRECTION('center_axis',(-0.403157732486128,-0.601098528075926,0.690032174816218));
#57393=DIRECTION('ref_axis',(0.864676174475855,-0.00330183512154052,0.502318834186645));
#57394=DIRECTION('center_axis',(0.406101923931813,0.601098527962152,-0.688303557349963));
#57395=DIRECTION('ref_axis',(0.862522348605138,-0.00330185944770726,0.506008197444334));
#57396=DIRECTION('center_axis',(-0.340062297712719,0.584828255986933,0.736432987225334));
#57397=DIRECTION('ref_axis',(0.897125081636666,-0.0330815410873473,0.440536263589834));
#57398=DIRECTION('center_axis',(0.444988920947186,-1.08032394082146E-7,
-0.895536074222724));
#57399=DIRECTION('ref_axis',(-0.895426046796085,-0.0156751635317822,-0.444934246790902));
#57400=DIRECTION('',(-0.445019414620402,-4.44089209849761E-13,0.895520921369744));
#57401=DIRECTION('center_axis',(-0.371736677613563,0.584827952225974,0.720963320018434));
#57402=DIRECTION('ref_axis',(0.880937865457384,-0.0227607296063951,0.472684277706771));
#57403=DIRECTION('center_axis',(-0.500371604875772,9.85772978998244E-10,
0.865810751281158));
#57404=DIRECTION('ref_axis',(-0.86570412768751,0.0156933905084823,-0.500309984708637));
#57405=DIRECTION('',(0.500371494362832,-2.20379270384489E-11,-0.865810815149076));
#57406=DIRECTION('',(0.318552670357025,0.,0.947905162032789));
#57407=DIRECTION('center_axis',(0.306515842391656,-0.601098528076755,-0.738057313429582));
#57408=DIRECTION('ref_axis',(0.913390697523814,-0.0324816852769616,0.405786118292049));
#57409=DIRECTION('',(0.966036775394096,8.17238220606244E-12,-0.258404621835945));
#57410=DIRECTION('center_axis',(0.,-1.,1.45983193964168E-32));
#57411=DIRECTION('ref_axis',(1.,0.,0.));
#57412=DIRECTION('center_axis',(-0.303359997774148,0.601098526315498,0.739360043153406));
#57413=DIRECTION('ref_axis',(0.91442875086526,-0.0345384997365875,0.403270568758676));
#57414=DIRECTION('center_axis',(-0.403157730677928,-0.601098528603427,0.69003217541316));
#57415=DIRECTION('ref_axis',(0.875386197278205,-0.0335099970597739,0.482261428803774));
#57416=DIRECTION('center_axis',(0.406101946483679,0.601098526349531,-0.688303545452578));
#57417=DIRECTION('ref_axis',(0.873317948314018,-0.0335100378554978,0.485996747433064));
#57418=DIRECTION('',(-0.387911046558245,0.,0.921696815638465));
#57419=DIRECTION('center_axis',(-0.278444757256321,0.584827952145246,0.761869269327794));
#57420=DIRECTION('ref_axis',(0.924224401753873,-0.0526562728585254,0.378201761142575));
#57421=DIRECTION('center_axis',(-0.445019520156076,8.85968837443965E-10,
0.895520868924927));
#57422=DIRECTION('ref_axis',(-0.895409464779819,0.015772999815539,-0.444964159072995));
#57423=DIRECTION('',(0.445019414618192,-1.76525460892714E-10,-0.895520921370842));
#57424=DIRECTION('',(0.377443537017177,0.,0.926032600054643));
#57425=DIRECTION('',(0.947905162043632,6.51326541667647E-11,-0.31855267032476));
#57426=DIRECTION('center_axis',(0.,-1.,1.45983193964168E-32));
#57427=DIRECTION('ref_axis',(1.,0.,0.));
#57428=DIRECTION('center_axis',(-0.386892908655361,0.601098531195128,0.699281368997669));
#57429=DIRECTION('ref_axis',(0.891933560802797,0.0514849626451757,0.449225802614975));
#57430=DIRECTION('center_axis',(0.229579573086911,0.601098532501136,-0.765489238230174));
#57431=DIRECTION('ref_axis',(0.944431797604197,0.0525165438942013,0.32448511875202));
#57432=DIRECTION('center_axis',(-0.332920489065193,0.584827930050222,0.739689286250494));
#57433=DIRECTION('ref_axis',(0.918057474729132,0.0219594825843356,0.395838671959421));
#57434=DIRECTION('center_axis',(0.329268495354959,-9.71829046692891E-9,
-0.944236335864428));
#57435=DIRECTION('ref_axis',(-0.94411937531885,-0.0157391393472326,-0.329227709405136));
#57436=DIRECTION('',(-0.32927177081575,0.,0.944235193658794));
#57437=DIRECTION('center_axis',(-0.364750270081651,0.584827952321338,0.724522951091954));
#57438=DIRECTION('ref_axis',(0.902955161139128,0.0322834330509239,0.428520427660874));
#57439=DIRECTION('center_axis',(-0.387911153478514,8.80631342479224E-10,
0.92169677063933));
#57440=DIRECTION('ref_axis',(-0.9215831390088,0.0157020800823732,-0.387863329764201));
#57441=DIRECTION('',(0.387911046558865,-7.7715611723626E-13,-0.921696815638204));
#57442=DIRECTION('',(0.434844806474141,0.,0.900505410468181));
#57443=DIRECTION('center_axis',(0.299367248971426,-0.601098527980864,-0.740985701550657));
#57444=DIRECTION('ref_axis',(0.933352190985876,0.0232723727333417,0.35820676186977));
#57445=DIRECTION('',(0.926032600054566,2.46403483598868E-13,-0.377443537017367));
#57446=DIRECTION('center_axis',(0.,-1.,1.45983193964168E-32));
#57447=DIRECTION('ref_axis',(1.,0.,0.));
#57448=DIRECTION('center_axis',(-0.296198957591961,0.601098529132487,0.742257863411494));
#57449=DIRECTION('ref_axis',(0.934367780165617,0.0212181108285934,0.355677723734903));
#57450=DIRECTION('center_axis',(-0.22630718595971,-0.601098527503902,0.766463057045569));
#57451=DIRECTION('ref_axis',(0.953958313206604,0.022245223402675,0.299113167045142));
#57452=DIRECTION('center_axis',(0.229579503858799,0.601098528301044,-0.765489262290639));
#57453=DIRECTION('ref_axis',(0.952671781045117,0.0222452026643455,0.303185798741871));
#57454=DIRECTION('center_axis',(-0.237586792098395,0.584827953016338,0.775582865715273));
#57455=DIRECTION('ref_axis',(0.954441832457449,-0.00784645569542236,0.298293851073547));
#57456=DIRECTION('center_axis',(0.269332611586817,-1.45997421325207E-9,
-0.963047218123714));
#57457=DIRECTION('ref_axis',(-0.96292885479551,-0.0156778483101916,-0.269299509235665));
#57458=DIRECTION('',(-0.269333009823076,7.77156117237388E-13,0.96304710675005));
#57459=DIRECTION('center_axis',(-0.27106730162798,0.584827952254156,0.764525201841206));
#57460=DIRECTION('ref_axis',(0.943100361128264,0.00246180457613212,0.332499095273908));
#57461=DIRECTION('center_axis',(-0.329271852152496,6.5516650383206E-10,
0.944235165295206));
#57462=DIRECTION('ref_axis',(-0.944119219261441,0.0156707406189448,-0.329231419687763));
#57463=DIRECTION('',(0.329271770814934,-6.33937347031766E-11,-0.944235193659079));
#57464=DIRECTION('',(0.490529942141632,1.64268989065528E-13,0.871424337428401));
#57465=DIRECTION('center_axis',(0.204136512687545,-0.601098528048857,-0.772663473813319));
#57466=DIRECTION('ref_axis',(0.965460823204787,-0.00691952388372738,0.260456366875447));
#57467=DIRECTION('',(0.900505410473539,2.34493981894349E-11,-0.434844806463045));
#57468=DIRECTION('center_axis',(0.,-1.,1.45983193964168E-32));
#57469=DIRECTION('ref_axis',(1.,0.,0.));
#57470=DIRECTION('center_axis',(-0.200833749216353,0.601098527505302,0.773528516220741));
#57471=DIRECTION('ref_axis',(0.966152035710377,-0.00897203548261672,0.257817273416643));
#57472=DIRECTION('center_axis',(-0.226307184425563,-0.601098528211325,0.766463056943747));
#57473=DIRECTION('ref_axis',(0.960712912217245,-0.00794572934697725,0.277430289774215));
#57474=DIRECTION('center_axis',(0.229579534945688,0.60109852769211,-0.765489253445468));
#57475=DIRECTION('ref_axis',(0.959518940489111,-0.00794577038205849,0.281532000979798));
#57476=DIRECTION('center_axis',(-0.138506937461519,0.584827952229457,0.79924470255744));
#57477=DIRECTION('ref_axis',(0.982832189613404,-0.0181546317085302,0.183606362654589));
#57478=DIRECTION('center_axis',(0.208331388704263,5.95656447432217E-10,
-0.978058297076689));
#57479=DIRECTION('ref_axis',(-0.977938063370797,-0.0156795066151041,-0.208305778323314));
#57480=DIRECTION('',(-0.208331317647729,2.06170772009129E-7,0.978058312212068));
#57481=DIRECTION('center_axis',(-0.173103405649599,0.584827782537418,0.79247187692995));
#57482=DIRECTION('ref_axis',(0.972199735876484,-0.0273551073893314,0.232549718687021));
#57483=DIRECTION('center_axis',(-0.269333131312943,8.75931129577168E-10,
0.963047072773271));
#57484=DIRECTION('ref_axis',(-0.962928339513347,0.0157023279258724,-0.269299925473025));
#57485=DIRECTION('',(-0.269333010693124,-1.29267411915878E-5,0.96304710641997));
#57486=DIRECTION('',(0.544279213551341,-7.62630514905437E-8,0.838904129025437));
#57487=DIRECTION('center_axis',(0.208331314469237,-1.49811687359948E-11,
-0.978058312889124));
#57488=DIRECTION('ref_axis',(-0.754939979668634,-0.635772805084903,-0.160805993086069));
#57489=DIRECTION('',(-0.871424337429238,0.,0.490529942140145));
#57490=DIRECTION('center_axis',(-0.137250389380106,0.398564391593955,0.906812415204131));
#57491=DIRECTION('ref_axis',(-4.38221259861562E-17,-0.915476128546279,0.402372287890104));
#57492=DIRECTION('center_axis',(0.13958376690986,5.74456497710768E-5,-0.990210264900971));
#57493=DIRECTION('ref_axis',(0.990210198391864,0.000362980231419196,0.139583778592271));
#57494=DIRECTION('',(-0.146508334828668,5.94973691934673E-5,0.98920943398544));
#57495=DIRECTION('center_axis',(-0.18265173307186,0.590180063808731,0.786336974005781));
#57496=DIRECTION('ref_axis',(0.0318446813635314,-0.795820438448205,0.604694754414954));
#57497=DIRECTION('center_axis',(0.698011204258703,0.550037558024481,0.458518313147666));
#57498=DIRECTION('ref_axis',(-0.618934249308444,0.785442801885021,1.77536854630035E-16));
#57499=DIRECTION('center_axis',(-0.705761528390122,-0.477126090336105,0.523690136402264));
#57500=DIRECTION('ref_axis',(0.549640180293908,0.0976244106121075,0.829677736629782));
#57501=DIRECTION('center_axis',(-0.58727483662782,0.584827951390493,0.55953957280622));
#57502=DIRECTION('ref_axis',(0.703292607946138,0.0265489689915622,0.710404574769761));
#57503=DIRECTION('center_axis',(0.653745308372474,-5.67375835137551E-11,
-0.756714656776898));
#57504=DIRECTION('ref_axis',(-0.756620821305633,-0.015747767056935,-0.653664241487562));
#57505=DIRECTION('center_axis',(-0.693441462764553,-0.000115441186732093,
0.720512959211901));
#57506=DIRECTION('ref_axis',(0.0180067889625396,-0.999690424427228,0.0171700570694068));
#57507=DIRECTION('',(0.699969797667289,-6.06570349238745E-10,-0.714172445809564));
#57508=DIRECTION('center_axis',(0.556688242552792,-0.601098527968652,-0.573392326664217));
#57509=DIRECTION('ref_axis',(0.731671535505592,0.0279220146977377,0.681085255475486));
#57510=DIRECTION('',(0.999949569926111,2.24062901110943E-10,-0.0100427886856853));
#57511=DIRECTION('center_axis',(0.,-1.,1.45983193964168E-32));
#57512=DIRECTION('ref_axis',(1.,0.,0.));
#57513=DIRECTION('center_axis',(-0.554233567212543,0.601098529702217,0.575765325948595));
#57514=DIRECTION('ref_axis',(0.733564879997119,0.0258668156642469,0.679126994517377));
#57515=DIRECTION('center_axis',(-0.486462658812862,-0.601098526942828,0.634062017856206));
#57516=DIRECTION('ref_axis',(0.780633128058457,0.0268944007484411,0.624410610564916));
#57517=DIRECTION('center_axis',(0.489166992764132,0.601098528495421,-0.631978015622961));
#57518=DIRECTION('ref_axis',(0.777958478909273,0.0268943670421948,0.627739833143134));
#57519=DIRECTION('center_axis',(-0.512515081039449,0.58482795222263,0.628732501153084));
#57520=DIRECTION('ref_axis',(0.773613241898176,-0.00326197145590633,0.633649675689979));
#57521=DIRECTION('center_axis',(0.604940694421974,-8.90032992022572E-10,
-0.796270529551522));
#57522=DIRECTION('ref_axis',(-0.796172596843005,-0.015683219631179,-0.60486629320724));
#57523=DIRECTION('',(-0.604940785833219,8.32148189212505E-8,0.796270460104782));
#57524=DIRECTION('center_axis',(-0.539352292982029,0.584827969931407,0.605867435699376));
#57525=DIRECTION('ref_axis',(0.750266322720323,0.00704480134519892,0.661098189201673));
#57526=DIRECTION('center_axis',(-0.653745384148104,7.59107307410203E-10,
0.756714591312371));
#57527=DIRECTION('ref_axis',(-0.756621662260592,0.0156715280548858,-0.653665100343015));
#57528=DIRECTION('',(0.653745308266017,-1.44328993199912E-11,-0.756714656868869));
#57529=DIRECTION('',(0.135290527320277,-3.07809289804497E-8,0.990805971528937));
#57530=DIRECTION('center_axis',(0.491483215750491,0.793626260371511,0.358610662814545));
#57531=DIRECTION('ref_axis',(-0.850173673702674,0.526502349988012,1.8687162403211E-16));
#57532=DIRECTION('center_axis',(-0.869349289638193,0.471546674578613,0.147903841395081));
#57533=DIRECTION('ref_axis',(0.357497665685219,0.393418196486003,0.847005042312807));
#57534=DIRECTION('center_axis',(0.480433470466423,-0.601098528037282,-0.638642497839756));
#57535=DIRECTION('ref_axis',(0.798095059786291,-0.00227572297195063,0.602527257997238));
#57536=DIRECTION('',(0.997345805939219,5.19500677922227E-12,-0.0728103246487009));
#57537=DIRECTION('center_axis',(0.,-1.,1.45983193964168E-32));
#57538=DIRECTION('ref_axis',(1.,0.,0.));
#57539=DIRECTION('center_axis',(-0.477700756092285,0.60109852787616,0.640689119163087));
#57540=DIRECTION('ref_axis',(0.799730624680367,-0.00432800792574344,0.600343398644264));
#57541=DIRECTION('center_axis',(-0.48646267173064,-0.601098528094992,0.634062006853211));
#57542=DIRECTION('ref_axis',(0.794900704079075,-0.00330183107163924,0.606730556809335));
#57543=DIRECTION('center_axis',(0.489166986034203,0.601098528025653,-0.63197802127891));
#57544=DIRECTION('ref_axis',(0.792301466969707,-0.00330184925236548,0.610120875916539));
#57545=DIRECTION('center_axis',(-0.429680332528739,0.584828255987421,0.68800488576514));
#57546=DIRECTION('ref_axis',(0.834837147984965,-0.0330815410785944,0.549502090973451));
#57547=DIRECTION('center_axis',(0.553720447696691,-1.0835760102034E-7,-0.832702627474277));
#57548=DIRECTION('ref_axis',(-0.832600320135553,-0.0156751635316961,-0.553652414569312));
#57549=DIRECTION('',(-0.553748836414874,-3.88578058618755E-13,0.832683749192437));
#57550=DIRECTION('center_axis',(-0.459166087066968,0.584827952226069,0.668687349052359));
#57551=DIRECTION('ref_axis',(0.814748358279444,-0.0227607295997188,0.579367812248005));
#57552=DIRECTION('center_axis',(-0.604940859635535,7.21040668407962E-10,
0.796270404035853));
#57553=DIRECTION('ref_axis',(-0.79617234425589,0.0156933905087076,-0.604866361882046));
#57554=DIRECTION('',(0.604940784793816,-2.32591723655392E-11,-0.796270460894439));
#57555=DIRECTION('',(0.197236768334392,0.,0.980355882940989));
#57556=DIRECTION('center_axis',(0.396601986956849,-0.601098528226986,-0.693820887048835));
#57557=DIRECTION('ref_axis',(0.855329850916094,-0.0324816825391389,0.517064586324842));
#57558=DIRECTION('',(0.990805973701574,8.1723822060613E-12,-0.135290511408879));
#57559=DIRECTION('center_axis',(0.,-1.,1.45983193964168E-32));
#57560=DIRECTION('ref_axis',(1.,0.,0.));
#57561=DIRECTION('center_axis',(-0.393634294321039,0.601098526148187,0.695508881465115));
#57562=DIRECTION('ref_axis',(0.85667500460091,-0.0345385027092639,0.514698968643452));
#57563=DIRECTION('center_axis',(-0.486462676856388,-0.601098528542966,0.634062002495969));
#57564=DIRECTION('ref_axis',(0.80804013045387,-0.0335099981759193,0.588173637286084));
#57565=DIRECTION('center_axis',(0.489167013021502,0.601098526659551,-0.631978001689409));
#57566=DIRECTION('ref_axis',(0.805520036045076,-0.0335100323791407,0.591620274551074));
#57567=DIRECTION('',(-0.500371494362924,1.2212453270872E-12,0.865810815149022));
#57568=DIRECTION('center_axis',(-0.37173667630522,0.584827952147585,0.720963320756618));
#57569=DIRECTION('ref_axis',(0.869535366608895,-0.0526562728258266,0.49105556014409));
#57570=DIRECTION('center_axis',(-0.553748908457271,6.38498716108382E-10,
0.832683701283015));
#57571=DIRECTION('ref_axis',(-0.832580114176435,0.0157729998147555,-0.553680021271129));
#57572=DIRECTION('',(0.55374883641321,-1.7652546089297E-10,-0.832683749193544));
#57573=DIRECTION('',(0.258404621839954,0.,0.966036775393023));
#57574=DIRECTION('',(0.980355882947729,6.51326541667623E-11,-0.197236768300891));
#57575=DIRECTION('center_axis',(0.,-1.,1.45983193964168E-32));
#57576=DIRECTION('ref_axis',(1.,0.,0.));
#57577=DIRECTION('center_axis',(-0.471485344333914,0.601098530776743,0.645276782765638));
#57578=DIRECTION('ref_axis',(0.828597472026194,0.051484967479824,0.557472445485336));
#57579=DIRECTION('center_axis',(0.323710518197072,0.601098532913274,-0.730679173193059));
#57580=DIRECTION('ref_axis',(0.896315899040263,0.0525165391159678,0.440295153558299));
#57581=DIRECTION('center_axis',(-0.423002961639147,0.584827930050675,0.692130613885236));
#57582=DIRECTION('ref_axis',(0.861206576608726,0.0219594825775692,0.5077804776976));
#57583=DIRECTION('center_axis',(0.44501630379855,-9.7571629034851E-9,-0.895522467252205));
#57584=DIRECTION('ref_axis',(-0.895411540810433,-0.0157391393480044,-0.444961180414731));
#57585=DIRECTION('',(-0.445019414620135,8.32667268468322E-13,0.895520921369877));
#57586=DIRECTION('center_axis',(-0.452680909511843,0.58482795232107,0.673094540423167));
#57587=DIRECTION('ref_axis',(0.842127239144872,0.0322834330530846,0.538311706207976));
#57588=DIRECTION('center_axis',(-0.50037154967943,4.71272382541235E-10,
0.86581078318037));
#57589=DIRECTION('ref_axis',(-0.865704041469944,0.0157020800824796,-0.500309861249696));
#57590=DIRECTION('',(0.500371494363191,-1.60982338570577E-12,-0.865810815148868));
#57591=DIRECTION('',(0.318552670357066,0.,0.947905162032776));
#57592=DIRECTION('center_axis',(0.389876781786075,-0.601098528007569,-0.697622143177284));
#57593=DIRECTION('ref_axis',(0.881097218878822,0.0232723720441225,0.472362241911274));
#57594=DIRECTION('',(0.966036775393002,0.,-0.258404621840034));
#57595=DIRECTION('center_axis',(0.,-1.,1.45983193964168E-32));
#57596=DIRECTION('ref_axis',(1.,0.,0.));
#57597=DIRECTION('center_axis',(-0.386892919518056,0.601098529104829,0.699281364784452));
#57598=DIRECTION('ref_axis',(0.882421771467431,0.0212181115163354,0.469980434682084));
#57599=DIRECTION('center_axis',(-0.320585978010544,-0.601098527464425,0.732055456221127));
#57600=DIRECTION('ref_axis',(0.908947247090312,0.0222452244191775,0.41631724921925));
#57601=DIRECTION('center_axis',(0.323710438814069,0.601098528144864,-0.730679212284625));
#57602=DIRECTION('ref_axis',(0.907160425325583,0.0222452070252269,0.420196517700363));
#57603=DIRECTION('center_axis',(-0.332919816036326,0.58482795438189,0.739689569930409));
#57604=DIRECTION('ref_axis',(0.909529582677385,-0.00784635391606152,0.415565124817912));
#57605=DIRECTION('center_axis',(0.387910088892421,-3.35595830138579E-9,
-0.921697218687067));
#57606=DIRECTION('ref_axis',(-0.921583937497068,-0.0156778482000772,-0.387862412748666));
#57607=DIRECTION('',(-0.387911046558218,3.885780586189E-13,0.921696815638477));
#57608=DIRECTION('center_axis',(-0.36475027068107,0.58482795225389,0.724522950844629));
#57609=DIRECTION('ref_axis',(0.893990546321623,0.00246180457749375,0.448079058432537));
#57610=DIRECTION('center_axis',(-0.445019470826524,4.72904638593461E-10,
0.895520893438718));
#57611=DIRECTION('ref_axis',(-0.89541092920561,0.0156707406183176,-0.444964825292539));
#57612=DIRECTION('',(0.445019414619957,-6.46149800302003E-11,-0.895520921369965));
#57613=DIRECTION('',(0.37744353701708,1.642689890656E-13,0.926032600054683));
#57614=DIRECTION('center_axis',(0.299367244840995,-0.60109852803596,-0.740985703174706));
#57615=DIRECTION('ref_axis',(0.925204038262238,-0.00691952524571913,0.37940691579572));
#57616=DIRECTION('',(0.94790516203665,2.37574025439352E-11,-0.318552670345537));
#57617=DIRECTION('center_axis',(0.,-1.,1.45983193964168E-32));
#57618=DIRECTION('ref_axis',(1.,0.,0.));
#57619=DIRECTION('center_axis',(-0.296198948099129,0.601098527530323,0.742257868497093));
#57620=DIRECTION('ref_axis',(0.926220564894495,-0.00897203367556791,0.376875268196584));
#57621=DIRECTION('center_axis',(-0.320585971320242,-0.601098528265885,0.732055458492896));
#57622=DIRECTION('ref_axis',(0.918366170984935,-0.0079457249634534,0.395651919552117));
#57623=DIRECTION('center_axis',(0.323710475898501,0.60109852768299,-0.730679196235193));
#57624=DIRECTION('ref_axis',(0.916667530744144,-0.00794577088209146,0.399571649150091));
#57625=DIRECTION('center_axis',(-0.23758669196574,0.584827952232603,0.775582896980199));
#57626=DIRECTION('ref_axis',(0.952070285082109,-0.0181546316499588,0.305340108098044));
#57627=DIRECTION('center_axis',(0.329271828552448,4.79123238521358E-10,
-0.944235173524968));
#57628=DIRECTION('ref_axis',(-0.944119097729614,-0.0156795066156232,-0.329231350837842));
#57629=DIRECTION('',(-0.329271773866148,2.06172326320939E-7,0.944235192595043));
#57630=DIRECTION('center_axis',(-0.271061496415139,0.584827782536856,0.764527389917595));
#57631=DIRECTION('ref_axis',(0.935387442375913,-0.027355107402994,0.352564931245888));
#57632=DIRECTION('center_axis',(-0.387911138367906,6.66509159556812E-10,
0.921696776998876));
#57633=DIRECTION('ref_axis',(-0.92158314178148,0.0157023279249487,-0.387863313142547));
#57634=DIRECTION('',(-0.387911047380046,-1.29267419732928E-5,0.921696815201949));
#57635=DIRECTION('',(0.434844842242892,-7.62630514905467E-8,0.900505393195815));
#57636=DIRECTION('center_axis',(0.329271770822495,5.67466570329746E-12,
-0.944235193656442));
#57637=DIRECTION('ref_axis',(-0.728832717338233,-0.635772805085086,-0.254157058630306));
#57638=DIRECTION('',(-0.926032600055416,0.,0.377443537015281));
#57639=DIRECTION('center_axis',(-0.249821861299389,0.398564391590108,0.882459893351146));
#57640=DIRECTION('ref_axis',(-4.2359305722015E-16,-0.911357382485098,0.411615987772476));
#57641=DIRECTION('center_axis',(0.262589361637465,5.74456695676028E-5,-0.964907676337391));
#57642=DIRECTION('ref_axis',(0.96490760891343,0.000362912078006155,0.262589364894681));
#57643=DIRECTION('',(-0.269333889882224,5.94973691579809E-5,0.963046858787761));
#57644=DIRECTION('center_axis',(-0.279765625258245,0.590180063806458,0.75724413976555));
#57645=DIRECTION('ref_axis',(-0.0441943955513831,-0.795820385214085,0.603917850273987));
#57646=DIRECTION('center_axis',(0.635039594592039,0.550037558023176,0.54238676059089));
#57647=DIRECTION('ref_axis',(-0.65470613502281,0.755883507402757,2.94999188131179E-16));
#57648=DIRECTION('center_axis',(-0.765832166685461,-0.477126089142097,0.431105309094913));
#57649=DIRECTION('ref_axis',(-0.441318377353577,-0.0976272725723773,-0.892024105873874));
#57650=DIRECTION('center_axis',(-0.652772903110501,0.584827951389779,0.481522381866018));
#57651=DIRECTION('ref_axis',(0.608709633160469,0.0265489690038084,0.792948759216182));
#57652=DIRECTION('center_axis',(0.743431825330591,-5.08120091142919E-11,
-0.668811723196914));
#57653=DIRECTION('ref_axis',(-0.668728788021033,-0.0157477670540756,-0.743339636979444));
#57654=DIRECTION('center_axis',(-0.778277689636587,-0.00011544118093089,
0.627920237360821));
#57655=DIRECTION('ref_axis',(0.015710992834112,-0.999690496894265,0.0192892489087636));
#57656=DIRECTION('',(0.783959868698026,-6.07291994204368E-10,-0.620811504621954));
#57657=DIRECTION('center_axis',(0.624163700015786,-0.60109852813265,-0.499099424022274));
#57658=DIRECTION('ref_axis',(0.640539473279341,0.0279220110573426,0.767417451241199));
#57659=DIRECTION('',(0.993323364076756,2.24206636476405E-10,0.115363314702887));
#57660=DIRECTION('center_axis',(0.,-1.,1.45983193964168E-32));
#57661=DIRECTION('ref_axis',(1.,0.,0.));
#57662=DIRECTION('center_axis',(-0.622025798805131,0.601098529751936,0.501761360759175));
#57663=DIRECTION('ref_axis',(0.64266332081354,0.0258668144821308,0.765711932772018));
#57664=DIRECTION('center_axis',(-0.562095789923428,-0.601098526612776,0.568092320185995));
#57665=DIRECTION('ref_axis',(0.696218208653023,0.0268944080891951,0.71732621362495));
#57666=DIRECTION('center_axis',(0.564517616921446,0.60109852864008,-0.565685795342311));
#57667=DIRECTION('ref_axis',(0.693147377749455,0.0268943637794391,0.720293971872564));
#57668=DIRECTION('center_axis',(-0.587274823972098,0.584827952222541,0.559539585219608));
#57669=DIRECTION('ref_axis',(0.688095707608259,-0.0032619714465507,0.725612607879281));
#57670=DIRECTION('center_axis',(0.699969721790153,-8.33585723815394E-10,
-0.714172520177735));
#57671=DIRECTION('ref_axis',(-0.714084684642701,-0.0156832196312858,-0.699883633028184));
#57672=DIRECTION('',(-0.699969798606644,8.32140417651395E-8,0.714172444888885));
#57673=DIRECTION('center_axis',(-0.611034663879005,0.584827969931641,0.533491223099225));
#57674=DIRECTION('ref_axis',(0.661492674919247,0.00704480134231119,0.749918536777314));
#57675=DIRECTION('center_axis',(-0.743431879511351,5.99257470412741E-10,
0.668811662971139));
#57676=DIRECTION('ref_axis',(-0.66872952892159,0.0156715280544964,-0.743340581669496));
#57677=DIRECTION('',(0.743431826076751,-1.48214773786022E-11,-0.668811722367505));
#57678=DIRECTION('',(0.0100428048565612,-3.07809289804534E-8,0.999949569763702));
#57679=DIRECTION('center_axis',(0.442661889834435,0.793626260372119,0.417382091297616));
#57680=DIRECTION('ref_axis',(-0.873334555250179,0.487120882949984,-5.16666451419685E-16));
#57681=DIRECTION('center_axis',(-0.881031477526049,0.471546674578495,0.0377792178615387));
#57682=DIRECTION('ref_axis',(0.248516531292135,0.393409809153091,0.885137421950204));
#57683=DIRECTION('center_axis',(0.556688232289915,-0.601098528013371,-0.573392336581236));
#57684=DIRECTION('ref_axis',(0.716285157056349,-0.00227572809784918,0.697803980242579));
#57685=DIRECTION('',(0.998606989791734,5.19500677922203E-12,0.0527643813485244));
#57686=DIRECTION('center_axis',(0.,-1.,1.45983193964168E-32));
#57687=DIRECTION('ref_axis',(1.,0.,0.));
#57688=DIRECTION('center_axis',(-0.554233581699321,0.601098527875221,0.575765313910958));
#57689=DIRECTION('ref_axis',(0.718181530636935,-0.0043280081485485,0.695842336594616));
#57690=DIRECTION('center_axis',(-0.56209581458741,-0.601098528076768,0.568092294233303));
#57691=DIRECTION('ref_axis',(0.712589168289662,-0.00330183506205464,0.701573784516975));
#57692=DIRECTION('center_axis',(0.564517607904078,0.601098528021518,-0.565685804998342));
#57693=DIRECTION('ref_axis',(0.709585510442279,-0.00330184985540807,0.70461159595759));
#57694=DIRECTION('center_axis',(-0.512522051817965,0.584828255987753,0.628726536260899));
#57695=DIRECTION('ref_axis',(0.759383333800813,-0.0330815410714352,0.649801942122292));
#57696=DIRECTION('center_axis',(0.653719519633801,-1.08253155343526E-7,
-0.756736935565948));
#57697=DIRECTION('ref_axis',(-0.75664396176299,-0.01567516353247,-0.653639200458355));
#57698=DIRECTION('',(-0.6537453082656,0.,0.75671465686923));
#57699=DIRECTION('center_axis',(-0.539354173031852,0.584827952226096,0.605865779136071));
#57700=DIRECTION('ref_axis',(0.735709782783262,-0.0227607295942035,0.676914370290175));
#57701=DIRECTION('center_axis',(-0.699969862671832,6.97646258222362E-10,
0.714172382097752));
#57702=DIRECTION('ref_axis',(-0.714084432592782,0.0156933905086662,-0.699883662206075));
#57703=DIRECTION('',(0.699969797674119,-2.3259172365536E-11,-0.71417244580287));
#57704=DIRECTION('',(0.0728103246514921,0.,0.997345805939015));
#57705=DIRECTION('center_axis',(0.480433476314609,-0.601098528193226,-0.638642493293547));
#57706=DIRECTION('ref_axis',(0.783779943492905,-0.0324816831588366,0.620188632947612));
#57707=DIRECTION('',(0.999949569924982,8.00811321699464E-12,-0.0100427887981123));
#57708=DIRECTION('center_axis',(0.,-1.,1.45983193964168E-32));
#57709=DIRECTION('ref_axis',(1.,0.,0.));
#57710=DIRECTION('center_axis',(-0.477700756802861,0.601098526553358,0.64068911987434));
#57711=DIRECTION('ref_axis',(0.785410974555097,-0.0345384955415771,0.618010269634848));
#57712=DIRECTION('center_axis',(-0.562095813790538,-0.601098528572725,0.568092294496993));
#57713=DIRECTION('ref_axis',(0.727950789289693,-0.0335099976713577,0.684809994398868));
#57714=DIRECTION('center_axis',(0.564517632497287,0.601098526611315,-0.565685781954402));
#57715=DIRECTION('ref_axis',(0.725018587143443,-0.0335100331949467,0.687913603566464));
#57716=DIRECTION('',(-0.604940784793116,-3.88578058618287E-13,0.79627046089497));
#57717=DIRECTION('center_axis',(-0.459166085817877,0.584827952145803,0.66868734998027));
#57718=DIRECTION('ref_axis',(0.801133239332449,-0.0526562728502562,0.596165119548449));
#57719=DIRECTION('center_axis',(-0.653745378516728,6.88166267249251E-10,
0.756714596177463));
#57720=DIRECTION('ref_axis',(-0.756620459739955,0.0157729998143454,-0.653664051619603));
#57721=DIRECTION('',(0.653745308264166,-1.76914038951625E-10,-0.756714656870468));
#57722=DIRECTION('',(0.135290511413065,0.,0.990805973701002));
#57723=DIRECTION('',(0.997345805941503,6.5132654166752E-11,-0.0728103246174193));
#57724=DIRECTION('center_axis',(0.,-1.,1.45983193964168E-32));
#57725=DIRECTION('ref_axis',(1.,0.,0.));
#57726=DIRECTION('center_axis',(-0.548642170750967,0.601098530535707,0.581095796802455));
#57727=DIRECTION('ref_axis',(0.752193906731871,0.0514849702321019,0.65692741190762));
#57728=DIRECTION('center_axis',(0.412736343893058,0.601098532682348,-0.684345866091788));
#57729=DIRECTION('ref_axis',(0.834064566950636,0.052516541749496,0.549161461685105));
#57730=DIRECTION('center_axis',(-0.506414424847036,0.584827930049987,0.633656628261943));
#57731=DIRECTION('ref_axis',(0.790773936299874,0.0219594825907513,0.611714281992132));
#57732=DIRECTION('center_axis',(0.553745940067887,-9.79389565979201E-9,
-0.832685675305113));
#57733=DIRECTION('ref_axis',(-0.832582532343421,-0.0157391393472531,-0.553677348578776));
#57734=DIRECTION('',(-0.553748836414763,3.8857805861822E-13,0.832683749192511));
#57735=DIRECTION('center_axis',(-0.533472500586727,0.584827952320527,0.61105102675826));
#57736=DIRECTION('ref_axis',(0.768018467521465,0.0322834330602798,0.639613487581229));
#57737=DIRECTION('center_axis',(-0.604940838723149,5.00351481251069E-10,
0.796270419923365));
#57738=DIRECTION('ref_axis',(-0.796172251513586,0.0157020800827631,-0.604866258441369));
#57739=DIRECTION('',(0.604940784793812,-1.16573417585636E-12,-0.796270460894442));
#57740=DIRECTION('',(0.197236768334319,-1.64268989065584E-13,0.980355882941003));
#57741=DIRECTION('center_axis',(0.474237720943464,-0.601098528144826,-0.643256669997655));
#57742=DIRECTION('ref_axis',(0.814946819839827,0.0232723683639434,0.579068284145908));
#57743=DIRECTION('',(0.990805973701026,0.,-0.135290511412896));
#57744=DIRECTION('center_axis',(0.,-1.,1.45983193964168E-32));
#57745=DIRECTION('ref_axis',(1.,0.,0.));
#57746=DIRECTION('center_axis',(-0.471485348678522,0.601098529086282,0.645276781165882));
#57747=DIRECTION('ref_axis',(0.816559444195094,0.0212181120796413,0.576871273175892));
#57748=DIRECTION('center_axis',(-0.409808942054769,-0.601098527542422,0.686102901318951));
#57749=DIRECTION('ref_axis',(0.849601538195442,0.0222452224588818,0.526955763203795));
#57750=DIRECTION('center_axis',(0.412736271713158,0.601098528090446,-0.684345913657575));
#57751=DIRECTION('ref_axis',(0.847342607083042,0.0222452084305431,0.530580490522971));
#57752=DIRECTION('center_axis',(-0.423002181530047,0.584827953016395,0.692131071251301));
#57753=DIRECTION('ref_axis',(0.850273623012057,-0.00784645567137288,0.526282432865992));
#57754=DIRECTION('center_axis',(0.500371211619023,-7.78002359410976E-10,
-0.865810978553004));
#57755=DIRECTION('ref_axis',(-0.865704566046401,-0.0156778483087253,-0.500309713476384));
#57756=DIRECTION('',(-0.500371494362507,-3.88578058618512E-13,0.865810815149263));
#57757=DIRECTION('center_axis',(-0.452680910074828,0.584827952254067,0.673094540102756));
#57758=DIRECTION('ref_axis',(0.830781966554501,0.0024618045795608,0.556592547170772));
#57759=DIRECTION('center_axis',(-0.553748911662773,6.88113040807786E-10,
0.832683699151301));
#57760=DIRECTION('ref_axis',(-0.832581450920485,0.0156707406193936,-0.55368091485221));
#57761=DIRECTION('',(0.553748836414603,-6.50035580888534E-11,-0.832683749192617));
#57762=DIRECTION('',(0.258404621840001,1.64268989065638E-13,0.966036775393011));
#57763=DIRECTION('center_axis',(0.389876788530882,-0.601098528116778,-0.697622139313747));
#57764=DIRECTION('ref_axis',(0.870356228170294,-0.00691951858998903,0.492374000478967));
#57765=DIRECTION('',(0.980355882943393,2.34493981894308E-11,-0.197236768322441));
#57766=DIRECTION('center_axis',(0.,-1.,1.45983193964168E-32));
#57767=DIRECTION('ref_axis',(1.,0.,0.));
#57768=DIRECTION('center_axis',(-0.386892915864324,0.601098527591087,0.699281368107165));
#57769=DIRECTION('ref_axis',(0.87168204034931,-0.00897202944535721,0.489989717463638));
#57770=DIRECTION('center_axis',(-0.409808933300045,-0.601098528262936,0.686102905916898));
#57771=DIRECTION('ref_axis',(0.861536244811326,-0.00794572521358364,0.507633888080011));
#57772=DIRECTION('center_axis',(0.412736294851897,0.601098527818209,-0.684345899941477));
#57773=DIRECTION('ref_axis',(0.859359733181087,-0.00794576136272164,0.511309802236666));
#57774=DIRECTION('center_axis',(-0.332919562188109,0.584827952228835,0.739689685884767));
#57775=DIRECTION('ref_axis',(0.906293663475364,-0.0181546317298205,0.422258457453677));
#57776=DIRECTION('center_axis',(0.445019476003258,5.37775435232845E-10,
-0.895520890866196));
#57777=DIRECTION('ref_axis',(-0.89541080356602,-0.0156795066150552,-0.444964769312765));
#57778=DIRECTION('',(-0.445019417513705,2.06170716497847E-7,0.895520919931924));
#57779=DIRECTION('center_axis',(-0.364744785454799,0.584827782536393,0.724525849267711));
#57780=DIRECTION('ref_axis',(0.883823530142337,-0.0273551074198127,0.467019984224217));
#57781=DIRECTION('center_axis',(-0.500371575167866,6.17478624361332E-10,
0.865810768450029));
#57782=DIRECTION('ref_axis',(-0.865704023370405,0.0157023279246887,-0.500309884789456));
#57783=DIRECTION('',(-0.500371495123144,-1.29267411917713E-5,0.865810814613174));
#57784=DIRECTION('',(0.318552708008686,-7.62630514905686E-8,0.947905149379582));
#57785=DIRECTION('center_axis',(0.445019414614705,-5.06252227775145E-12,
-0.895520921372575));
#57786=DIRECTION('ref_axis',(-0.691231327686734,-0.635772805085008,-0.343499915485835));
#57787=DIRECTION('',(-0.96603677539344,0.,0.258404621838397));
#57788=DIRECTION('center_axis',(-0.358453493229671,0.398564391588364,0.844190451823073));
#57789=DIRECTION('ref_axis',(1.45643262671735E-16,-0.904282187129022,0.426935271488726));
#57790=DIRECTION('center_axis',(0.3814537653021,5.74456535097432E-5,-0.924387917292761));
#57791=DIRECTION('ref_axis',(0.924387849953043,0.000363021687504849,0.381453760073807));
#57792=DIRECTION('',(-0.387911888599863,5.94973691934224E-5,0.921696459330809));
#57793=DIRECTION('center_axis',(-0.372467446133925,0.59018006381471,0.716209113210755));
#57794=DIRECTION('ref_axis',(-0.119533762394807,-0.79581992529521,0.593617996821919));
#57795=DIRECTION('center_axis',(0.562053031164479,0.550037558024463,0.617701444810766));
#57796=DIRECTION('ref_axis',(0.73963826965528,1.66905152560888E-16,-0.673004628558633));
#57797=DIRECTION('center_axis',(-0.813825173144071,-0.47712609025277,0.331721692925152));
#57798=DIRECTION('ref_axis',(-0.326038799174341,-0.0976261562960603,-0.940301991404789));
#57799=DIRECTION('center_axis',(0.,-1.,1.45983193964168E-32));
#57800=DIRECTION('ref_axis',(1.,0.,0.));
#57801=DIRECTION('center_axis',(-0.680008321123557,0.601098529378286,0.41984430588253));
#57802=DIRECTION('ref_axis',(0.541626566377255,0.02586682302227,0.840221143545626));
#57803=DIRECTION('center_axis',(-0.62886435068494,-0.601098526908652,0.493163450983402));
#57804=DIRECTION('ref_axis',(0.600823499447581,0.0268944015745013,0.79892916686995));
#57805=DIRECTION('center_axis',(0.681795728548397,-0.601098528078482,-0.41693541954965));
#57806=DIRECTION('ref_axis',(0.539305716225786,0.0279220122353789,0.841647019645956));
#57807=DIRECTION('center_axis',(0.630965454817298,0.601098528548254,-0.490472378227687));
#57808=DIRECTION('ref_axis',(0.597404933134226,0.0268943657915818,0.801488639317838));
#57809=DIRECTION('center_axis',(-0.70797635094031,0.584827951390237,0.395911295345234));
#57810=DIRECTION('ref_axis',(0.504526943858353,0.0265489689943019,0.862987668026774));
#57811=DIRECTION('center_axis',(0.821393979803529,-3.34035840811973E-11,
-0.570361227593987));
#57812=DIRECTION('ref_axis',(-0.570290500650736,-0.0157477670566653,-0.82129212385135));
#57813=DIRECTION('center_axis',(-0.850840010906561,-0.000115441176905437,
0.525424840023631));
#57814=DIRECTION('ref_axis',(0.0131676303921038,-0.999690586528358,0.0211031920913415));
#57815=DIRECTION('',(0.855586424284002,-6.06570349238516E-10,-0.517659995152141));
#57816=DIRECTION('',(0.971031855393319,2.2406290111098E-10,0.238950069703709));
#57817=DIRECTION('center_axis',(-0.652772892093047,0.58482795222276,0.481522395790074));
#57818=DIRECTION('ref_axis',(0.59172649297372,-0.00326197145057506,0.806132195768955));
#57819=DIRECTION('center_axis',(0.783959821523761,-5.96131969645808E-10,
-0.620811564193543));
#57820=DIRECTION('ref_axis',(-0.620735211050847,-0.0156832196313396,-0.783863402885768));
#57821=DIRECTION('',(-0.783959869513934,8.321320909793E-8,0.620811503591621));
#57822=DIRECTION('center_axis',(-0.673080653115289,0.584827969931677,0.452701535216626));
#57823=DIRECTION('ref_axis',(0.562286892476256,0.00704480134115208,0.826912221050976));
#57824=DIRECTION('center_axis',(-0.821394020464315,5.31114300248357E-10,
0.570361169037189));
#57825=DIRECTION('ref_axis',(-0.570291125292885,0.0156715280545383,-0.8212931484072));
#57826=DIRECTION('',(0.821393979886223,-1.44328993199867E-11,-0.570361227474896));
#57827=DIRECTION('',(-0.115363298639103,-3.07809289804514E-8,0.993323365942382));
#57828=DIRECTION('center_axis',(0.386859521482828,0.793626260373017,0.469571154868373));
#57829=DIRECTION('ref_axis',(-2.13687929229864E-16,-0.509219680924762,0.860636576354319));
#57830=DIRECTION('center_axis',(-0.878819272724478,0.471546674559146,-0.0729412064626718));
#57831=DIRECTION('ref_axis',(0.135626041762887,0.393420630700766,0.909299611863297));
#57832=DIRECTION('center_axis',(0.624163699479745,-0.601098528034406,-0.499099424810959));
#57833=DIRECTION('ref_axis',(0.623179000875404,-0.00227572371504448,0.782075925949332));
#57834=DIRECTION('',(0.984119544876364,5.19500677922209E-12,0.177506961532043));
#57835=DIRECTION('center_axis',(0.,-1.,1.45983193964168E-32));
#57836=DIRECTION('ref_axis',(1.,0.,0.));
#57837=DIRECTION('center_axis',(-0.622025817027204,0.60109852790029,0.501761340387782));
#57838=DIRECTION('ref_axis',(0.625306280590028,-0.00432800421432909,0.780367428737378));
#57839=DIRECTION('center_axis',(-0.628864362189718,-0.601098528093964,0.493163434868188));
#57840=DIRECTION('ref_axis',(0.619039682119636,-0.00330183194536081,0.785352767784659));
#57841=DIRECTION('center_axis',(0.630965447315775,0.601098528031762,-0.490472388510966));
#57842=DIRECTION('ref_axis',(0.615678968825533,-0.00330184814314328,0.787990168177731));
#57843=DIRECTION('center_axis',(-0.587280992141335,0.584828255986637,0.559532793738774));
#57844=DIRECTION('ref_axis',(0.671953590842899,-0.0330815410987143,0.73985402843525));
#57845=DIRECTION('center_axis',(0.743409038173406,-1.08193554509994E-7,
-0.668837051875925));
#57846=DIRECTION('ref_axis',(-0.668754877861165,-0.0156751635313557,-0.743317699631297));
#57847=DIRECTION('',(-0.743431826102458,2.44243513872084E-9,0.668811722338929));
#57848=DIRECTION('center_axis',(-0.611036274076432,0.58482795055301,0.53348940009597));
#57849=DIRECTION('ref_axis',(0.645068669434817,-0.0227607725733292,0.763785545127335));
#57850=DIRECTION('center_axis',(-0.783959920609502,6.39561847536878E-10,
0.620811439068211));
#57851=DIRECTION('ref_axis',(-0.620734986854462,0.0156933905089844,-0.783863376864313));
#57852=DIRECTION('',(0.783959868703813,-2.2870594306917E-11,-0.620811504614646));
#57853=DIRECTION('',(-0.0527643808758776,-9.0376691099926E-10,0.998606989816707));
#57854=DIRECTION('center_axis',(0.556688242465508,-0.601098528137483,-0.573392326571969));
#57855=DIRECTION('ref_axis',(0.699869358675761,-0.0324816841607832,0.71353193410026));
#57856=DIRECTION('',(0.993323364089752,8.00811321699503E-12,0.115363314590982));
#57857=DIRECTION('center_axis',(0.,-1.,1.45983193964168E-32));
#57858=DIRECTION('ref_axis',(1.,0.,0.));
#57859=DIRECTION('center_axis',(-0.55423357818793,0.601098526332382,0.575765318901758));
#57860=DIRECTION('ref_axis',(0.701760552571379,-0.0345384994452432,0.711575167435447));
#57861=DIRECTION('center_axis',(-0.628864360507214,-0.601098528788258,0.493163436167407));
#57862=DIRECTION('ref_axis',(0.636381232999916,-0.0335099937670627,0.770646486142147));
#57863=DIRECTION('center_axis',(0.630965472559523,0.601098526509254,-0.490472357902198));
#57864=DIRECTION('ref_axis',(0.63308316071494,-0.0335100350712062,0.773358124783536));
#57865=DIRECTION('',(-0.69996979767421,-3.88578058618464E-13,0.714172445802781));
#57866=DIRECTION('center_axis',(-0.539354171922836,0.584827952147118,0.605865780199576));
#57867=DIRECTION('ref_axis',(0.720096762266244,-0.0526562728331108,0.691872798934167));
#57868=DIRECTION('center_axis',(-0.743431897726421,8.01204384872099E-10,
0.668811642723789));
#57869=DIRECTION('ref_axis',(-0.668728441543193,0.0157729998147021,-0.743339413692061));
#57870=DIRECTION('',(0.743431826075426,-1.76525460892892E-10,-0.668811722368977));
#57871=DIRECTION('',(0.010042788802475,0.,0.999949569924938));
#57872=DIRECTION('',(0.998606989790074,6.51326541667596E-11,0.0527643813799335));
#57873=DIRECTION('center_axis',(0.,-1.,1.45983193964168E-32));
#57874=DIRECTION('ref_axis',(1.,0.,0.));
#57875=DIRECTION('center_axis',(-0.617146580610682,0.601098530377361,0.507750583277577));
#57876=DIRECTION('ref_axis',(0.663927794474839,0.0514849720612138,0.746022239196414));
#57877=DIRECTION('center_axis',(0.495253069852363,0.601098532340813,-0.62722001819101));
#57878=DIRECTION('ref_axis',(0.758659540214554,0.0525165456835235,0.649367164607906));
#57879=DIRECTION('center_axis',(-0.581839430006672,0.584827930051382,0.565189499125141));
#57880=DIRECTION('ref_axis',(0.707870318665559,0.0219594825652875,0.706000986598309));
#57881=DIRECTION('center_axis',(0.653742689345644,-9.65698928568759E-9,
-0.756716919413809));
#57882=DIRECTION('ref_axis',(-0.756623186558303,-0.0157391393474532,-0.653661711479999));
#57883=DIRECTION('',(-0.653745308266206,0.,0.756714656868706));
#57884=DIRECTION('center_axis',(-0.605850911623636,0.584827952321254,0.539370873396533));
#57885=DIRECTION('ref_axis',(0.681797585889768,0.0322834330504779,0.730828182150469));
#57886=DIRECTION('center_axis',(-0.699969848687725,5.29825396220384E-10,
0.714172395803761));
#57887=DIRECTION('ref_axis',(-0.714084348869081,0.0157020800831493,-0.699883552729511));
#57888=DIRECTION('',(0.699969797674381,-3.88578058618674E-13,-0.714172445802613));
#57889=DIRECTION('',(0.0728103246515104,0.,0.997345805939014));
#57890=DIRECTION('center_axis',(0.551119652024366,-0.601098528185188,-0.578746653179215));
#57891=DIRECTION('ref_axis',(0.735944221221984,0.0232723672963963,0.676642076854809));
#57892=DIRECTION('',(0.99994956992494,0.,-0.0100427888023433));
#57893=DIRECTION('center_axis',(0.,-1.,1.45983193964168E-32));
#57894=DIRECTION('ref_axis',(1.,0.,0.));
#57895=DIRECTION('center_axis',(-0.548642181723866,0.601098528779788,0.581095788258743));
#57896=DIRECTION('ref_axis',(0.73781947939277,0.0212181204735827,0.674664514549379));
#57897=DIRECTION('center_axis',(-0.492568970194462,-0.601098527513249,0.629330096072778));
#57898=DIRECTION('ref_axis',(0.776857107271133,0.0222452233282606,0.629283866725823));
#57899=DIRECTION('center_axis',(0.495253018968578,0.601098528368869,-0.627220062175382));
#57900=DIRECTION('ref_axis',(0.774161682723275,0.0222452008249728,0.632596901702279));
#57901=DIRECTION('center_axis',(-0.506413843524673,0.584827954381722,0.633657070393962));
#57902=DIRECTION('ref_axis',(0.777608194314138,-0.00784635389937767,0.628700191558736));
#57903=DIRECTION('center_axis',(0.604939965639439,-3.27650173372792E-9,
-0.796271083219876));
#57904=DIRECTION('ref_axis',(-0.796173217541591,-0.0156778482002054,-0.604865615443036));
#57905=DIRECTION('',(-0.604940784793658,0.,0.796270460894559));
#57906=DIRECTION('center_axis',(-0.533472501099667,0.584827952254068,0.61105102637405));
#57907=DIRECTION('ref_axis',(0.75447145888779,0.00246180458297537,0.656328238949022));
#57908=DIRECTION('center_axis',(-0.653745361478494,5.31761636790432E-10,
0.756714610897235));
#57909=DIRECTION('ref_axis',(-0.7566216911844,0.0156707406186724,-0.653665085741713));
#57910=DIRECTION('',(0.653745308265349,-6.38378239129687E-11,-0.756714656869446));
#57911=DIRECTION('',(0.135290511412992,1.64268989065632E-13,0.990805973701012));
#57912=DIRECTION('center_axis',(0.474237725950656,-0.601098528057081,-0.643256666388123));
#57913=DIRECTION('ref_axis',(0.801782387397817,-0.00691952323199839,0.597576039895258));
#57914=DIRECTION('',(0.997345805939914,2.3449398189431E-11,-0.0728103246391816));
#57915=DIRECTION('center_axis',(0.,-1.,1.45983193964168E-32));
#57916=DIRECTION('ref_axis',(1.,0.,0.));
#57917=DIRECTION('center_axis',(-0.471485353517794,0.601098527683139,0.645276778937042));
#57918=DIRECTION('ref_axis',(0.803396566223726,-0.00897202285469235,0.595376738028805));
#57919=DIRECTION('center_axis',(-0.492568963228535,-0.601098528265706,0.629330100806221));
#57920=DIRECTION('ref_axis',(0.791119377524039,-0.00794572522958855,0.611610166655651));
#57921=DIRECTION('center_axis',(0.495253024655371,0.601098527880305,-0.627220058153306));
#57922=DIRECTION('ref_axis',(0.788499317751901,-0.00794575698719568,0.614984301304259));
#57923=DIRECTION('center_axis',(-0.423002092231914,0.584827952231039,0.692131126490257));
#57924=DIRECTION('ref_axis',(0.846224249337463,-0.0181546316854976,0.532517538848826));
#57925=DIRECTION('center_axis',(0.553748791295796,-4.24684809762998E-10,
-0.832683779197389));
#57926=DIRECTION('ref_axis',(-0.832581416534835,-0.0156795066181781,-0.553680718386562));
#57927=DIRECTION('',(-0.553748839105298,2.06170327919852E-7,0.832683747403234));
#57928=DIRECTION('center_axis',(-0.452675831355118,0.584827782536082,0.673098103162446));
#57929=DIRECTION('ref_axis',(0.818321192866598,-0.0273551074282337,0.574109853079511));
#57930=DIRECTION('center_axis',(-0.604940865737854,6.83049984403924E-10,
0.796270399399812));
#57931=DIRECTION('ref_axis',(-0.796172227891624,0.0157023279250567,-0.604866283100507));
#57932=DIRECTION('',(-0.604940785481047,-1.29267420445158E-5,0.79627046026741));
#57933=DIRECTION('',(0.197236807274931,-7.62630514905909E-8,0.980355875106579));
#57934=DIRECTION('center_axis',(0.553748836409908,-5.14328675068677E-12,
-0.832683749195739));
#57935=DIRECTION('ref_axis',(-0.642728807070213,-0.635772805084933,-0.427425573493839));
#57936=DIRECTION('',(-0.990805973701214,0.,0.135290511411514));
#57937=DIRECTION('center_axis',(-0.46143209944248,0.398564391585333,0.792607622575205));
#57938=DIRECTION('ref_axis',(0.864216279017979,-2.46944013809118E-16,0.503120485649628));
#57939=DIRECTION('center_axis',(0.49430241515009,5.74456554432761E-5,-0.869290008614378));
#57940=DIRECTION('ref_axis',(0.869289942423636,0.000363130101863143,0.494302401509076));
#57941=DIRECTION('',(-0.500372285107574,5.94973691578971E-5,0.865810356115176));
#57942=DIRECTION('center_axis',(-0.459295233458345,0.590180063803156,0.663879040798658));
#57943=DIRECTION('ref_axis',(-0.193006876961119,-0.795822364586091,0.573946957018084));
#57944=DIRECTION('center_axis',(0.480202555681032,0.550037558023931,0.68327460825094));
#57945=DIRECTION('ref_axis',(-2.67200776655505E-16,-0.778964448264928,0.627068089077508));
#57946=DIRECTION('center_axis',(-0.848983670875502,-0.477126090478573,0.227106627757515));
#57947=DIRECTION('ref_axis',(-0.205617745019631,-0.0976244547999203,-0.973750896666114));
#57948=DIRECTION('center_axis',(0.,-1.,1.45983193964168E-32));
#57949=DIRECTION('ref_axis',(1.,0.,0.));
#57950=DIRECTION('center_axis',(-0.680008328143395,0.601098527896,0.419844296634939));
#57951=DIRECTION('ref_axis',(0.522569581621024,-0.00432800512230333,0.852585655952579));
#57952=DIRECTION('center_axis',(-0.685715352438027,-0.601098528063218,0.410457080571191));
#57953=DIRECTION('ref_axis',(0.515727559994683,-0.00330183849355368,0.856746276166108));
#57954=DIRECTION('center_axis',(0.681795728152809,-0.601098528038952,-0.416935420253529));
#57955=DIRECTION('ref_axis',(0.520244942189748,-0.00227572246809452,0.854014063826371));
#57956=DIRECTION('center_axis',(0.687462588098602,0.601098528021724,-0.407523925156412));
#57957=DIRECTION('ref_axis',(0.512062798628297,-0.00330184974610516,0.858941667431037));
#57958=DIRECTION('center_axis',(0.,-1.,1.45983193964168E-32));
#57959=DIRECTION('ref_axis',(1.,0.,0.));
#57960=DIRECTION('center_axis',(-0.727266694147858,0.601098529543099,0.331306072030638));
#57961=DIRECTION('ref_axis',(0.432048050851811,0.0258668192715915,0.901479555739298));
#57962=DIRECTION('center_axis',(-0.685715334700198,-0.601098526757656,0.4104571121162));
#57963=DIRECTION('ref_axis',(0.495953454603779,0.0268944048963865,0.867932521485309));
#57964=DIRECTION('center_axis',(0.728675431061478,-0.601098528004021,-0.3281960935154));
#57965=DIRECTION('ref_axis',(0.429566785113303,0.0279220138465334,0.902603311688017));
#57966=DIRECTION('center_axis',(0.68746259021791,0.601098528408167,-0.407523921011294));
#57967=DIRECTION('ref_axis',(0.492241057688875,0.0268943690384856,0.87004335181608));
#57968=DIRECTION('center_axis',(-0.752014588816605,0.584827951388868,0.304056451142372));
#57969=DIRECTION('ref_axis',(0.392387563221727,0.0265489690167294,0.919416745808485));
#57970=DIRECTION('center_axis',(0.886402261674847,6.96815599083177E-12,
-0.46291579201591));
#57971=DIRECTION('ref_axis',(-0.462858388711434,-0.0157477670569393,-0.886292344450845));
#57972=DIRECTION('center_axis',(-0.909984078160621,-0.000115441171811356,
0.414643176921436));
#57973=DIRECTION('ref_axis',(0.010417872471279,-0.999690646286046,0.0225849432445623));
#57974=DIRECTION('',(0.913719870856373,-6.06514838087195E-10,-0.406344678323974));
#57975=DIRECTION('',(0.933426594283893,2.24206636476395E-10,0.358768439363851));
#57976=DIRECTION('center_axis',(-0.707976341755816,0.584827952222755,0.395911310539358));
#57977=DIRECTION('ref_axis',(0.486025398070987,-0.00326197145932844,0.873938597369482));
#57978=DIRECTION('center_axis',(0.855586388865124,-5.36828188002314E-10,
-0.517660053692322));
#57979=DIRECTION('ref_axis',(-0.517596387076646,-0.0156832196303758,-0.855481160930636));
#57980=DIRECTION('',(-0.85558642496489,8.32136531871927E-8,0.517659994026766));
#57981=DIRECTION('center_axis',(-0.724511758384697,0.584827969931394,0.364772473671245));
#57982=DIRECTION('ref_axis',(0.45421350982732,0.00704480135432238,0.890865005634538));
#57983=DIRECTION('center_axis',(-0.886402280378725,3.19828384669413E-10,
0.462915756201273));
#57984=DIRECTION('ref_axis',(-0.462858907393903,0.0156715280543384,-0.886293424918951));
#57985=DIRECTION('',(0.886402259955283,-1.40443212613674E-11,-0.462915795308571));
#57986=DIRECTION('',(-0.238950054000525,-3.07809289804526E-8,0.971031859257535));
#57987=DIRECTION('center_axis',(0.324956147379585,0.793626260374256,0.514354800818064));
#57988=DIRECTION('ref_axis',(1.18768397098885E-16,-0.543871187803528,0.839168714310287));
#57989=DIRECTION('center_axis',(-0.862747562988294,0.471546674573188,-0.182511304462839));
#57990=DIRECTION('ref_axis',(0.0205860831513606,0.393412747962545,0.919131450294812));
#57991=DIRECTION('',(0.954111946853708,5.05127141378893E-12,0.299450150894981));
#57992=DIRECTION('center_axis',(-0.652772892223738,0.584827952239051,0.481522395593117));
#57993=DIRECTION('ref_axis',(0.573932730509739,-0.033086909061157,0.818233754680418));
#57994=DIRECTION('center_axis',(0.821393938657068,-5.66605482047647E-10,
-0.570361286850211));
#57995=DIRECTION('ref_axis',(-0.570291210542767,-0.0156751701942392,-0.821293019705542));
#57996=DIRECTION('',(-0.821393979885579,0.,0.570361227475824));
#57997=DIRECTION('center_axis',(-0.673082062129668,0.584827952225996,0.452699463147927));
#57998=DIRECTION('ref_axis',(0.544254348718667,-0.0227607295979204,0.838611443452205));
#57999=DIRECTION('center_axis',(-0.85558645437424,4.39716529147059E-10,
0.517659945419111));
#58000=DIRECTION('ref_axis',(-0.517596196193671,0.0156933905082907,-0.855481089902166));
#58001=DIRECTION('',(0.855586424288824,-2.20934381896938E-11,-0.517659995144173));
#58002=DIRECTION('',(-0.177506961529562,0.,0.984119544876812));
#58003=DIRECTION('center_axis',(0.624163703184407,-0.601098528102421,-0.499099420096067));
#58004=DIRECTION('ref_axis',(0.6049214158146,-0.0324816847642132,0.795622410973785));
#58005=DIRECTION('',(0.971031855420263,8.00811321699492E-12,0.238950069594217));
#58006=DIRECTION('center_axis',(0.,-1.,1.45983193964168E-32));
#58007=DIRECTION('ref_axis',(1.,0.,0.));
#58008=DIRECTION('center_axis',(-0.622025811482655,0.60109852640924,0.501761349047517));
#58009=DIRECTION('ref_axis',(0.607042942905174,-0.0345384980589837,0.793918105109624));
#58010=DIRECTION('center_axis',(-0.685715346712145,-0.60109852870395,0.410457089198603));
#58011=DIRECTION('ref_axis',(0.534775559073474,-0.0335099953326465,0.84432942719679));
#58012=DIRECTION('center_axis',(0.687462605265226,0.601098526679091,-0.407523898177978));
#58013=DIRECTION('ref_axis',(0.53116363987613,-0.0335100320481414,0.846606322576009));
#58014=DIRECTION('',(-0.783959868703477,3.88578058618491E-13,0.62081150461507));
#58015=DIRECTION('center_axis',(-0.611036320506081,0.584827952146277,0.533489345170812));
#58016=DIRECTION('ref_axis',(0.627703929119516,-0.0526562728443811,0.776669230945877));
#58017=DIRECTION('center_axis',(-0.821394029079472,6.36178315555462E-10,
0.570361156630246));
#58018=DIRECTION('ref_axis',(-0.570290202838897,0.0157729998144146,-0.821291846436347));
#58019=DIRECTION('',(0.821393979884557,-1.76525460892916E-10,-0.570361227477296));
#58020=DIRECTION('',(-0.115363314586811,-1.4373536543246E-13,0.993323364090236));
#58021=DIRECTION('',(0.98411954487057,6.73708191429274E-11,0.177506961564164));
#58022=DIRECTION('center_axis',(0.,-1.,1.45983193964168E-32));
#58023=DIRECTION('ref_axis',(1.,0.,0.));
#58024=DIRECTION('center_axis',(-0.675918217257937,0.601098530441075,0.426397842724881));
#58025=DIRECTION('ref_axis',(0.565191146769487,0.0514849713402289,0.823351847838752));
#58026=DIRECTION('center_axis',(0.569959358794219,0.601098531899161,-0.560202538615773));
#58027=DIRECTION('ref_axis',(0.671290001483131,0.0525165507868081,0.739331959137595));
#58028=DIRECTION('center_axis',(-0.648088479825358,0.584827930050975,0.487808993920723));
#58029=DIRECTION('ref_axis',(0.613803163212554,0.0219594825743171,0.789153633936593));
#58030=DIRECTION('center_axis',(0.743429504550853,-9.7370770992602E-9,-0.668814302899746));
#58031=DIRECTION('ref_axis',(-0.668731458373539,-0.0157391393482095,-0.743337417377988));
#58032=DIRECTION('',(-0.743431826076801,3.88578058618555E-13,0.668811722367449));
#58033=DIRECTION('center_axis',(-0.668674691896985,0.58482795232003,0.459184519122361));
#58034=DIRECTION('ref_axis',(0.584824349013597,0.0322834330674684,0.810517279735726));
#58035=DIRECTION('center_axis',(-0.783959911974966,5.16098504643952E-10,
0.620811449971893));
#58036=DIRECTION('ref_axis',(-0.620734913065085,0.0157020800826335,-0.783863261279134));
#58037=DIRECTION('',(0.783959868703571,-3.88578058618765E-13,-0.620811504614952));
#58038=DIRECTION('',(-0.0527643813458578,0.,0.998606989791875));
#58039=DIRECTION('center_axis',(0.619310100008391,-0.601098528130847,-0.505109452996602));
#58040=DIRECTION('ref_axis',(0.645335340235233,0.0232723687883982,0.763544822190848));
#58041=DIRECTION('',(0.993323364090227,1.43735365432655E-13,0.115363314586895));
#58042=DIRECTION('center_axis',(0.,-1.,1.45983193964168E-32));
#58043=DIRECTION('ref_axis',(1.,0.,0.));
#58044=DIRECTION('center_axis',(-0.617146593637132,0.601098528605606,0.507750569542034));
#58045=DIRECTION('ref_axis',(0.647443662249848,0.0212181253246192,0.761817888586382));
#58046=DIRECTION('center_axis',(-0.567560897639404,-0.60109852767921,0.56263237330662));
#58047=DIRECTION('ref_axis',(0.691861171014227,0.0222452189954519,0.721687792798705));
#58048=DIRECTION('center_axis',(0.569959306223684,0.601098527946005,-0.560202596343646));
#58049=DIRECTION('ref_axis',(0.688771782411489,0.0222452124300358,0.724636862350821));
#58050=DIRECTION('center_axis',(-0.581838788167143,0.584827953016251,0.565190136109091));
#58051=DIRECTION('ref_axis',(0.692679594751913,-0.0078464556685245,0.721202753840948));
#58052=DIRECTION('center_axis',(0.699969489842962,-1.59750556575904E-9,
-0.714172747512102));
#58053=DIRECTION('ref_axis',(-0.714084972116213,-0.0156778483104737,-0.699883460063275));
#58054=DIRECTION('',(-0.69996979767378,4.44089209849797E-13,0.714172445803202));
#58055=DIRECTION('center_axis',(-0.605850912090104,0.584827952254016,0.539370872945475));
#58056=DIRECTION('ref_axis',(0.66626248562324,0.00246180457741594,0.74571324231863));
#58057=DIRECTION('center_axis',(-0.743431866551407,4.54777387042457E-10,
0.668811677377041));
#58058=DIRECTION('ref_axis',(-0.668729551581567,0.0156707406185188,-0.743340577884716));
#58059=DIRECTION('',(0.743431826076476,-6.42264019716054E-11,-0.66881172236781));
#58060=DIRECTION('',(0.0100427888024243,1.64268989065715E-13,0.999949569924939));
#58061=DIRECTION('center_axis',(0.551119657779422,-0.601098528057545,-0.578746647831454));
#58062=DIRECTION('ref_axis',(0.720563956462457,-0.00691952328167995,0.693353953507676));
#58063=DIRECTION('',(0.998606989791215,2.33056628239968E-11,0.0527643813583316));
#58064=DIRECTION('center_axis',(0.,-1.,1.45983193964168E-32));
#58065=DIRECTION('ref_axis',(1.,0.,0.));
#58066=DIRECTION('center_axis',(-0.548642174934512,0.601098527672761,0.581095795814053));
#58067=DIRECTION('ref_axis',(0.722441053324715,-0.00897202367764671,0.691374303299019));
#58068=DIRECTION('center_axis',(-0.567560894235305,-0.601098528183147,0.562632376202148));
#58069=DIRECTION('ref_axis',(0.708226078745709,-0.00794573193760378,0.705940993800794));
#58070=DIRECTION('center_axis',(0.569959316685545,0.601098527973058,-0.560202585670549));
#58071=DIRECTION('ref_axis',(0.705203800501899,-0.00794575017932217,0.708960129211626));
#58072=DIRECTION('center_axis',(-0.506413626476593,0.584827952229078,0.633657245843815));
#58073=DIRECTION('ref_axis',(0.772809373333965,-0.0181546317213056,0.634378500450818));
#58074=DIRECTION('center_axis',(0.653745352984885,4.63890099005459E-10,
-0.756714618235084));
#58075=DIRECTION('ref_axis',(-0.756621594530565,-0.0156795066149336,-0.653664987407417));
#58076=DIRECTION('',(-0.653745310710569,2.06171937743035E-7,0.75671465475693));
#58077=DIRECTION('center_axis',(-0.53346790901253,0.584827782536522,0.61105519785631));
#58078=DIRECTION('ref_axis',(0.739913441518089,-0.027355107412841,0.672145666622414));
#58079=DIRECTION('center_axis',(-0.699969862169507,5.94033433643584E-10,
0.714172382590087));
#58080=DIRECTION('ref_axis',(-0.714084332876665,0.0157023279254008,-0.699883563485964));
#58081=DIRECTION('',(-0.699969798277329,-1.29267419735568E-5,0.714172445094667));
#58082=DIRECTION('',(0.0728103642669414,-7.62629077552247E-8,0.997345803046922));
#58083=DIRECTION('center_axis',(0.653745308269215,3.24852657677469E-12,
-0.756714656866107));
#58084=DIRECTION('ref_axis',(-0.584090069209569,-0.635772805085282,-0.504610474886078));
#58085=DIRECTION('',(-0.999949569924953,0.,0.0100427888010589));
#58086=DIRECTION('center_axis',(-0.557133645801549,0.398564391581777,0.728524897638319));
#58087=DIRECTION('ref_axis',(0.794343958189908,-3.09877856731042E-16,0.607468251093989));
#58088=DIRECTION('center_axis',(0.599355620640818,5.74456531717371E-5,-0.80048287720991));
#58089=DIRECTION('ref_axis',(0.800482813240499,0.000363161708211434,0.599355598806042));
#58090=DIRECTION('',(-0.604941511771255,5.94973699394858E-5,0.796269906373443));
#58091=DIRECTION('center_axis',(-0.538879660020742,0.590180063812166,0.60107919968553));
#58092=DIRECTION('ref_axis',(-0.263409456277491,-0.795820649045882,0.545238436737349));
#58093=DIRECTION('center_axis',(0.390778999035457,0.550037558023876,0.738072122950039));
#58094=DIRECTION('ref_axis',(7.53656174059586E-17,-0.801830011453256,0.597552200843467));
#58095=DIRECTION('center_axis',(-0.870753189088995,-0.47712609044742,0.118909955452456));
#58096=DIRECTION('ref_axis',(-0.0819536582661743,-0.0976233394778846,-0.991843375481218));
#58097=DIRECTION('center_axis',(0.,-1.,1.45983193964168E-32));
#58098=DIRECTION('ref_axis',(1.,0.,0.));
#58099=DIRECTION('center_axis',(-0.763055658654184,0.601098528025735,0.237542883288733));
#58100=DIRECTION('ref_axis',(0.3156558309711,0.0258668540830143,0.948521113225105));
#58101=DIRECTION('center_axis',(-0.731752133462375,-0.601098523429036,0.321277730794861));
#58102=DIRECTION('ref_axis',(0.383262015888094,0.0268944802402911,0.923248024157105));
#58103=DIRECTION('center_axis',(0.764063590022611,-0.601098518825436,-0.234280603268019));
#58104=DIRECTION('ref_axis',(0.313053074944991,0.0279222149704815,0.949325087722129));
#58105=DIRECTION('center_axis',(0.733118084397875,0.601098531882569,-0.318148439093156));
#58106=DIRECTION('ref_axis',(0.37931414459962,0.0268942877291573,0.924877006414474));
#58107=DIRECTION('center_axis',(0.,-1.,1.45983193964168E-32));
#58108=DIRECTION('ref_axis',(1.,0.,0.));
#58109=DIRECTION('center_axis',(-0.680008326307634,0.601098526530791,0.419844301562856));
#58110=DIRECTION('ref_axis',(0.502751902272055,-0.0345384959278909,0.863740480156435));
#58111=DIRECTION('center_axis',(-0.731752192868383,-0.601098528530253,0.321277585945668));
#58112=DIRECTION('ref_axis',(0.424736152881488,-0.0335099985284445,0.904696789225018));
#58113=DIRECTION('center_axis',(0.681795729173495,-0.60109852804082,-0.416935418581753));
#58114=DIRECTION('ref_axis',(0.500433501629634,-0.0324816859338729,0.8651654469092));
#58115=DIRECTION('center_axis',(0.733118040771723,0.601098527035837,-0.318148548779305));
#58116=DIRECTION('ref_axis',(0.420867355674219,-0.0335100257314689,0.906503032043063));
#58117=DIRECTION('center_axis',(0.,-1.,1.45983193964168E-32));
#58118=DIRECTION('ref_axis',(1.,0.,0.));
#58119=DIRECTION('center_axis',(-0.727266707321978,0.60109852793785,0.331306046023914));
#58120=DIRECTION('ref_axis',(0.411591638996172,-0.00432799832780596,0.911358102580385));
#58121=DIRECTION('center_axis',(-0.731752194190079,-0.601098528072251,0.321277583792239));
#58122=DIRECTION('ref_axis',(0.40428211487033,-0.00330183696942516,0.914628377795376));
#58123=DIRECTION('center_axis',(0.728675428745706,-0.601098528032884,-0.328196098604113));
#58124=DIRECTION('ref_axis',(0.409106312832959,-0.00227572372044445,0.91248388801215));
#58125=DIRECTION('center_axis',(0.733118028917691,0.601098528044534,-0.318148574189064));
#58126=DIRECTION('ref_axis',(0.400371098715705,-0.00330184579683318,0.916347140077118));
#58127=DIRECTION('center_axis',(-0.752014581596804,0.584827952222568,0.304056467395354));
#58128=DIRECTION('ref_axis',(0.372659392286658,-0.00326197145442373,0.927962465233788));
#58129=DIRECTION('center_axis',(0.913719848261096,-4.35909436812389E-10,
-0.406344729132445));
#58130=DIRECTION('ref_axis',(-0.406294753104332,-0.0156832196307687,-0.913607470537486));
#58131=DIRECTION('',(-0.913719871391209,8.32139862540962E-8,0.406344677121314));
#58132=DIRECTION('center_axis',(-0.764516880406,0.584827969931467,0.271090732339042));
#58133=DIRECTION('ref_axis',(0.338976908816905,0.00704480134891643,0.940768316889387));
#58134=DIRECTION('center_axis',(-0.937431471416932,5.26575514447819E-10,
0.348169838436769));
#58135=DIRECTION('ref_axis',(-0.348127081105987,0.0156715280544189,-0.937316349270119));
#58136=DIRECTION('',(0.937431446874141,-1.44328993199741E-11,-0.348169904517111));
#58137=DIRECTION('',(-0.358768424268643,-3.07809289805637E-8,0.933426600085831));
#58138=DIRECTION('center_axis',(0.257928020713531,0.793626260375571,0.551026764298329));
#58139=DIRECTION('ref_axis',(3.86526474988473E-16,-0.570324176014851,0.821419706516091));
#58140=DIRECTION('center_axis',(-0.833069808886043,0.471546674515063,-0.289203090018688));
#58141=DIRECTION('ref_axis',(-0.0947709949961845,0.393417043001799,0.914462404248066));
#58142=DIRECTION('',(0.909057433470377,5.19500677922194E-12,0.416670832495209));
#58143=DIRECTION('center_axis',(-0.707980627189437,0.584828255987165,0.3959031984254));
#58144=DIRECTION('ref_axis',(0.466848718284166,-0.0330815410864286,0.883718216331303));
#58145=DIRECTION('center_axis',(0.886386495251401,-1.08055804801194E-7,
-0.462945980688812));
#58146=DIRECTION('ref_axis',(-0.462889103293546,-0.0156751635321578,-0.886277590431089));
#58147=DIRECTION('',(-0.886402259955067,3.8857805861861E-13,0.462915795308984));
#58148=DIRECTION('center_axis',(-0.724512896583829,0.584827952226093,0.364770241355767));
#58149=DIRECTION('ref_axis',(0.434856856698299,-0.0227607295918755,0.900211899149817));
#58150=DIRECTION('center_axis',(-0.913719892390152,3.99854364386318E-10,
0.406344629902412));
#58151=DIRECTION('ref_axis',(-0.406294589028634,0.0156933905087666,-0.913607368851846));
#58152=DIRECTION('',(0.91371987086034,-2.24265050970685E-11,-0.406344678315053));
#58153=DIRECTION('',(-0.299450150892402,0.,0.954111946854518));
#58154=DIRECTION('',(0.933426594324386,8.00811321699435E-12,0.358768439258496));
#58155=DIRECTION('',(-0.855586424288614,8.32667268468143E-13,0.517659995144519));
#58156=DIRECTION('center_axis',(-0.673082061317715,0.584827952146517,0.452699464457831));
#58157=DIRECTION('ref_axis',(0.525411830022407,-0.052656272840452,0.849217125241276));
#58158=DIRECTION('center_axis',(-0.886402289863428,4.66216806888189E-10,
0.462915738039734));
#58159=DIRECTION('ref_axis',(-0.462858150621278,0.0157729998159349,-0.886292020092845));
#58160=DIRECTION('',(0.886402259954025,-1.76136882834176E-10,-0.462915795310981));
#58161=DIRECTION('',(-0.238950069590315,0.,0.971031855421223));
#58162=DIRECTION('',(0.95411194684388,6.73708191429212E-11,0.299450150926296));
#58163=DIRECTION('center_axis',(-0.784193107368798,0.58482795138977,0.207406455127399));
#58164=DIRECTION('ref_axis',(0.274059996359373,0.0265489690028562,0.961346072255141));
#58165=DIRECTION('center_axis',(0.937431447265939,-2.66968652048685E-11,
-0.348169903462213));
#58166=DIRECTION('ref_axis',(-0.348126729081251,-0.015747767055638,-0.937315202230259));
#58167=DIRECTION('center_axis',(-0.957443409380817,7.95312786477369E-12,
0.288621062698544));
#58168=DIRECTION('ref_axis',(0.00472526695421307,-0.999865971929401,0.0156751405061303));
#58169=DIRECTION('',(0.957443409235807,-6.06126260028942E-10,-0.288621063179587));
#58170=DIRECTION('',(0.881100638180641,2.24206636473677E-10,0.472928816417088));
#58171=DIRECTION('center_axis',(0.,-1.,1.45983193964168E-32));
#58172=DIRECTION('ref_axis',(1.,0.,0.));
#58173=DIRECTION('center_axis',(-0.724030222887723,0.601098530184123,0.338320548231469));
#58174=DIRECTION('ref_axis',(0.457541092754366,0.0514849742756542,0.887696708265259));
#58175=DIRECTION('center_axis',(0.635677057400638,0.601098532148273,-0.484350320887329));
#58176=DIRECTION('ref_axis',(0.573333811124451,0.0525165478891726,0.817637054700505));
#58177=DIRECTION('center_axis',(-0.704116787165796,0.58482793005043,0.402735449475516));
#58178=DIRECTION('ref_axis',(0.510055965204231,0.0219594825838839,0.859860857048527));
#58179=DIRECTION('center_axis',(0.821392007966856,-9.6282449769448E-9,-0.570364067283499));
#58180=DIRECTION('ref_axis',(-0.570293417594276,-0.0157391393474235,-0.821290263756513));
#58181=DIRECTION('',(-0.821393979885945,4.44089209849773E-13,0.570361227475297));
#58182=DIRECTION('center_axis',(-0.720953072810683,0.584827952320198,0.371756550701933));
#58183=DIRECTION('ref_axis',(0.478628082816279,0.032283433065689,0.877424035623088));
#58184=DIRECTION('center_axis',(-0.855586463236559,5.60123081497593E-10,
0.517659930771502));
#58185=DIRECTION('ref_axis',(-0.517596110925291,0.0157020800827716,-0.855480982042317));
#58186=DIRECTION('',(0.855586424289034,-3.88578058618695E-13,-0.517659995143825));
#58187=DIRECTION('',(-0.177506961529512,-1.6426898906565E-13,0.984119544876821));
#58188=DIRECTION('center_axis',(0.677733657883253,-0.601098528047542,-0.423506373684346));
#58189=DIRECTION('ref_axis',(0.544549134368899,0.0232723709346554,0.838406009645185));
#58190=DIRECTION('',(0.971031855421274,0.,0.23895006959011));
#58191=DIRECTION('center_axis',(0.,-1.,1.45983193964168E-32));
#58192=DIRECTION('ref_axis',(1.,0.,0.));
#58193=DIRECTION('center_axis',(-0.675918226413701,0.601098528713118,0.426397830647251));
#58194=DIRECTION('ref_axis',(0.546857279595311,0.0212181223337183,0.836956932606599));
#58195=DIRECTION('center_axis',(-0.633602050443839,-0.601098527883255,0.487061599235606));
#58196=DIRECTION('ref_axis',(0.595954168650271,0.0222452135891341,0.802710271107041));
#58197=DIRECTION('center_axis',(0.635677009826813,0.601098527945971,-0.484350388539979));
#58198=DIRECTION('ref_axis',(0.592519529931851,0.0222452123180939,0.805248879029497));
#58199=DIRECTION('center_axis',(-0.64808802673632,0.584827954381773,0.487809566710878));
#58200=DIRECTION('ref_axis',(0.596826823270977,-0.00784635390048773,0.802331713043142));
#58201=DIRECTION('center_axis',(0.783959299467165,-2.39970101787109E-9,
-0.620812223445183));
#58202=DIRECTION('ref_axis',(-0.620735922539111,-0.015677848198522,-0.783862946914435));
#58203=DIRECTION('',(-0.783959868703779,7.77156117237062E-13,0.620811504614689));
#58204=DIRECTION('center_axis',(-0.668674692280572,0.584827952254079,0.459184518647769));
#58205=DIRECTION('ref_axis',(0.567546154955955,0.00246180457167309,0.823337902390605));
#58206=DIRECTION('center_axis',(-0.821394026637575,6.22329750071602E-10,
0.570361160146894));
#58207=DIRECTION('ref_axis',(-0.570291123441637,0.0156707406185681,-0.821293164717776));
#58208=DIRECTION('',(0.821393979885603,-6.37823127618236E-11,-0.57036122747579));
#58209=DIRECTION('',(-0.115363314586758,1.6426898906571E-13,0.993323364090243));
#58210=DIRECTION('center_axis',(0.619310103140169,-0.601098528052553,-0.50510944924993));
#58211=DIRECTION('ref_axis',(0.627981801754453,-0.00691952358516004,0.778197260891212));
#58212=DIRECTION('',(0.984119544874613,2.34493981894299E-11,0.177506961541753));
#58213=DIRECTION('center_axis',(0.,-1.,1.45983193964168E-32));
#58214=DIRECTION('ref_axis',(1.,0.,0.));
#58215=DIRECTION('center_axis',(-0.617146594133584,0.601098527826761,0.507750569860653));
#58216=DIRECTION('ref_axis',(0.630092201514216,-0.00897201270892481,0.776468492972458));
#58217=DIRECTION('center_axis',(-0.63360204568641,-0.601098528143562,0.487061605103133));
#58218=DIRECTION('ref_axis',(0.614163633400353,-0.00794573548312544,0.789138705612714));
#58219=DIRECTION('center_axis',(0.635677020797868,0.601098527942322,-0.484350374145742));
#58220=DIRECTION('ref_axis',(0.610786790306842,-0.00794575219278953,0.791755241099645));
#58221=DIRECTION('center_axis',(-0.58183871533142,0.584827952227705,0.56519021190625));
#58222=DIRECTION('ref_axis',(0.687206831862969,-0.0181546317512861,0.726234934154806));
#58223=DIRECTION('center_axis',(0.743431881697495,6.52231953694037E-10,
-0.668811660541084));
#58224=DIRECTION('ref_axis',(-0.668729442833958,-0.0156795066147268,-0.743340490864922));
#58225=DIRECTION('',(-0.743431828237324,2.06171160587007E-7,0.668811719965842));
#58226=DIRECTION('center_axis',(-0.605846879053264,0.58482778253678,0.539375587058343));
#58227=DIRECTION('ref_axis',(0.649836813198125,-0.0273551074048852,0.759581341471321));
#58228=DIRECTION('center_axis',(-0.78395992854951,6.42204840304423E-10,
0.620811429041579));
#58229=DIRECTION('ref_axis',(-0.620734889719503,0.0157023279254214,-0.783863274801568));
#58230=DIRECTION('',(-0.783959869213338,-1.29267420091223E-5,0.620811503836636));
#58231=DIRECTION('',(-0.0527643416803028,-7.62630514906024E-8,0.998606991887719));
#58232=DIRECTION('center_axis',(0.74343182608437,8.46488594574043E-12,-0.668811722359036));
#58233=DIRECTION('ref_axis',(-0.516239882040292,-0.635772805085321,-0.573837367644325));
#58234=DIRECTION('',(-0.993323364090019,0.,-0.115363314588682));
#58235=DIRECTION('center_axis',(-0.644048861750252,0.398564391579836,0.652952899865527));
#58236=DIRECTION('ref_axis',(0.711944358623391,-1.48341292504493E-16,0.702235879334237));
#58237=DIRECTION('center_axis',(0.694956629954641,5.74456464726726E-5,-0.719051652652357));
#58238=DIRECTION('ref_axis',(0.719051591959292,0.000363044425646409,0.694956600299294));
#58239=DIRECTION('',(-0.699970449419061,5.94973699395165E-5,0.714171804540155));
#58240=DIRECTION('center_axis',(-0.60996563275169,0.590180063807912,0.528799980281315));
#58241=DIRECTION('ref_axis',(-0.329667630782392,-0.795820412202847,0.507926298527272));
#58242=DIRECTION('center_axis',(0.295192624134886,0.550037558023661,0.781229799367464));
#58243=DIRECTION('ref_axis',(-2.99006832900842E-16,-0.817666865875968,0.575691667864467));
#58244=DIRECTION('center_axis',(-0.878790409509715,-0.477126090119163,0.00883800211288844));
#58245=DIRECTION('ref_axis',(0.0430053759461772,-0.09762677183074,-0.994293493422157));
#58246=DIRECTION('center_axis',(0.,-1.,1.45983193964168E-32));
#58247=DIRECTION('ref_axis',(1.,0.,0.));
#58248=DIRECTION('center_axis',(-0.786810691452641,0.601098536565918,0.140033871453045));
#58249=DIRECTION('ref_axis',(0.194285827458928,0.0258666594739602,0.98060386149365));
#58250=DIRECTION('center_axis',(-0.766248820041582,-0.601098522588609,0.227031521878956));
#58251=DIRECTION('ref_axis',(0.264526238238669,0.0268944948231608,0.964003400114079));
#58252=DIRECTION('center_axis',(0.787401802212211,-0.601098527961809,-0.136670997490725));
#58253=DIRECTION('ref_axis',(0.191602837697934,0.0279220147745897,0.981075284408402));
#58254=DIRECTION('center_axis',(0.767211803203183,0.601098532171143,-0.223755678469661));
#58255=DIRECTION('ref_axis',(0.26040530923369,0.0268942848435636,0.96512474445828));
#58256=DIRECTION('center_axis',(0.,-1.,1.45983193964168E-32));
#58257=DIRECTION('ref_axis',(1.,0.,0.));
#58258=DIRECTION('center_axis',(-0.763055658742142,0.601098528049379,0.237542882946354));
#58259=DIRECTION('ref_axis',(0.294122635795175,-0.0043279808307652,0.955757889684845));
#58260=DIRECTION('center_axis',(-0.766248826143083,-0.601098528566415,0.227031485458818));
#58261=DIRECTION('ref_axis',(0.286461009557513,-0.00330174912324799,0.958086211390195));
#58262=DIRECTION('center_axis',(0.76406357716492,-0.601098528929575,-0.234280619276642));
#58263=DIRECTION('ref_axis',(0.29151558545289,-0.00227553083980164,0.956563372389648));
#58264=DIRECTION('center_axis',(0.767211806619316,0.601098527379421,-0.223755679628956));
#58265=DIRECTION('ref_axis',(0.28236518714665,-0.00330193682016637,0.959301307359097));
#58266=DIRECTION('center_axis',(0.,-1.,1.45983193964168E-32));
#58267=DIRECTION('ref_axis',(1.,0.,0.));
#58268=DIRECTION('center_axis',(-0.760723836756566,0.60109853016227,0.244907740235234));
#58269=DIRECTION('ref_axis',(0.34267534538575,0.0514849745188543,0.93804205932546));
#58270=DIRECTION('center_axis',(0.691369743499754,0.601098531888471,-0.40085961724101));
#58271=DIRECTION('ref_axis',(0.466335810284432,0.0525165508876074,0.88304752076501));
#58272=DIRECTION('center_axis',(0.,-1.,1.45983193964168E-32));
#58273=DIRECTION('ref_axis',(1.,0.,0.));
#58274=DIRECTION('center_axis',(-0.727266700096615,0.601098526413129,0.331306064651021));
#58275=DIRECTION('ref_axis',(0.390532168548934,-0.0345384980101142,0.919941148924034));
#58276=DIRECTION('center_axis',(-0.766248865328599,-0.601098528706299,0.227031352834265));
#58277=DIRECTION('ref_axis',(0.307998411581329,-0.0335099952893715,0.950796539055062));
#58278=DIRECTION('center_axis',(0.72867543016971,-0.601098528022213,-0.328196095462021));
#58279=DIRECTION('ref_axis',(0.388053451412226,-0.0324816862907586,0.921064307691253));
#58280=DIRECTION('center_axis',(0.767211772309541,0.601098527048624,-0.223755798158681));
#58281=DIRECTION('ref_axis',(0.30393373490876,-0.0335100255164653,0.952103651381664));
#58282=DIRECTION('center_axis',(-0.75201458167613,0.584827952239124,0.304056467167315));
#58283=DIRECTION('ref_axis',(0.352415118267461,-0.0330869090612141,0.935258702640775));
#58284=DIRECTION('center_axis',(0.937431427900636,-4.26563368083218E-10,
-0.348169955602397));
#58285=DIRECTION('ref_axis',(-0.348127178393669,-0.0156751701946118,-0.937316252234555));
#58286=DIRECTION('',(-0.93743144687371,3.88578058618708E-13,0.348169904518272));
#58287=DIRECTION('center_axis',(-0.764517729851838,0.584827952226204,0.271088374957497));
#58288=DIRECTION('ref_axis',(0.318601412279502,-0.0227607295886048,0.94761547543405));
#58289=DIRECTION('center_axis',(-0.957443432644625,6.20247471359333E-10,
0.288620985525443));
#58290=DIRECTION('ref_axis',(-0.288585442177813,0.0156933905085329,-0.957325524603508));
#58291=DIRECTION('',(0.957443409238553,-2.2482016248302E-11,-0.288621063170478));
#58292=DIRECTION('',(-0.416670832492711,-1.43735365432645E-13,0.909057433471522));
#58293=DIRECTION('',(0.881100638234107,8.00811321699514E-12,0.472928816317476));
#58294=DIRECTION('',(-0.913719870860275,3.88578058618767E-13,0.4063446783152));
#58295=DIRECTION('center_axis',(-0.724512895938863,0.584827952146669,0.364770242764149));
#58296=DIRECTION('ref_axis',(0.414833672503379,-0.0526562728382997,0.908372358170446));
#58297=DIRECTION('center_axis',(-0.937431470815378,4.98983339446778E-10,
0.348169840056427));
#58298=DIRECTION('ref_axis',(-0.348126527198881,0.015772999815457,-0.937314852937511));
#58299=DIRECTION('',(0.937431446873072,-1.7691403895138E-10,-0.348169904519991));
#58300=DIRECTION('',(-0.358768439254574,0.,0.933426594325894));
#58301=DIRECTION('',(0.909057433457252,6.51326541667565E-11,0.416670832523844));
#58302=DIRECTION('center_axis',(-0.749040752138178,0.584827930050797,0.311310526434255));
#58303=DIRECTION('ref_axis',(0.398264879952269,0.0219594825763105,0.917007560776674));
#58304=DIRECTION('center_axis',(0.886400663547062,-9.55911743639789E-9,
-0.462918852136449));
#58305=DIRECTION('ref_axis',(-0.462861511471999,-0.015739139347479,-0.886290866866209));
#58306=DIRECTION('',(-0.886402259955305,7.77156117237576E-13,0.462915795308529));
#58307=DIRECTION('center_axis',(-0.761861593087581,0.584827952320615,0.278465759407741));
#58308=DIRECTION('ref_axis',(0.36488356584029,0.0322834330592784,0.930493290319485));
#58309=DIRECTION('center_axis',(-0.913719901723408,5.65380501737239E-10,
0.406344608915347));
#58310=DIRECTION('ref_axis',(-0.406294512606847,0.0157020800825024,-0.913607253532199));
#58311=DIRECTION('',(0.913719870860467,-3.88578058618884E-13,-0.406344678314768));
#58312=DIRECTION('',(-0.299450150892451,-1.64268989065695E-13,0.954111946854502));
#58313=DIRECTION('center_axis',(0.72546894837819,-0.601098528071751,-0.335224349487053));
#58314=DIRECTION('ref_axis',(0.435175066285531,0.0232723703371241,0.900045031352474));
#58315=DIRECTION('',(0.933426594325836,0.,0.358768439254726));
#58316=DIRECTION('center_axis',(-0.804004432171644,0.584827951390059,0.10748553540481));
#58317=DIRECTION('ref_axis',(0.151410339629092,0.0265489689966038,0.988114396868409));
#58318=DIRECTION('center_axis',(0.973676780287623,-1.28906918013669E-11,
-0.22793316460912));
#58319=DIRECTION('ref_axis',(-0.227904900037124,-0.0157477670551488,-0.973556040694035));
#58320=DIRECTION('center_axis',(-0.98606749399318,4.96891179130181E-11,
0.166345716175714));
#58321=DIRECTION('ref_axis',(0.00272900050446146,-0.999865419160101,0.0161770245732108));
#58322=DIRECTION('',(0.986067493102596,-6.06514838087271E-10,-0.166345721454935));
#58323=DIRECTION('',(0.814879198669332,2.24062901110924E-10,0.579630823521341));
#58324=DIRECTION('center_axis',(-0.784193102249395,0.584827952222746,0.207406472134837));
#58325=DIRECTION('ref_axis',(0.253416325277267,-0.00326197145543368,0.967351810679646));
#58326=DIRECTION('center_axis',(0.957443386600224,-6.15197396809075E-10,
-0.288621138268657));
#58327=DIRECTION('ref_axis',(-0.288585640979932,-0.0156832196320613,-0.957325631351305));
#58328=DIRECTION('',(-0.957443409615588,8.32144303432537E-8,0.288621061919726));
#58329=DIRECTION('center_axis',(-0.792465114529435,0.584827969931237,0.173133728198635));
#58330=DIRECTION('ref_axis',(0.218394439445317,0.00704480135457211,0.975835149804126));
#58331=DIRECTION('center_axis',(-0.973676797222046,5.70223093254237E-10,
0.227933092269243));
#58332=DIRECTION('ref_axis',(-0.227905100723701,0.0156715280547446,-0.973557223933215));
#58333=DIRECTION('',(0.973676779881275,-1.40998324126016E-11,-0.227933166344942));
#58334=DIRECTION('',(-0.472928802167949,-3.07808057783763E-8,0.881100645828834));
#58335=DIRECTION('center_axis',(0.186832215081918,0.793626260376337,0.579008706539594));
#58336=DIRECTION('ref_axis',(-9.49913119975713E-19,-0.589386723434917,0.807851032207457));
#58337=DIRECTION('center_axis',(-0.790254046147588,0.471546674542655,-0.391333970254474));
#58338=DIRECTION('ref_axis',(-0.208641931036127,0.393409230472831,0.895375743468792));
#58339=DIRECTION('',(0.849666541316565,4.90753604829622E-12,0.527320366160028));
#58340=DIRECTION('center_axis',(0.,-1.,1.45983193964168E-32));
#58341=DIRECTION('ref_axis',(1.,0.,0.));
#58342=DIRECTION('center_axis',(-0.72403023283582,0.6010985284829,0.338320529964412));
#58343=DIRECTION('ref_axis',(0.437646620241063,0.0212181286726185,0.89889667193021));
#58344=DIRECTION('center_axis',(-0.689650913839443,-0.601098527866504,0.403809579922447));
#58345=DIRECTION('ref_axis',(0.490648618647226,0.0222452140406601,0.871073523574132));
#58346=DIRECTION('center_axis',(0.691369707533585,0.601098527966793,-0.400859685153146));
#58347=DIRECTION('ref_axis',(0.486922890027579,0.0222452117933845,0.873161640087022));
#58348=DIRECTION('center_axis',(-0.704116346384031,0.584827953375261,0.402736186238222));
#58349=DIRECTION('ref_axis',(0.491561927830823,-0.00784642890357389,0.870807271823511));
#58350=DIRECTION('center_axis',(0.855586176495259,-1.17960254227111E-9,
-0.51766040469619));
#58351=DIRECTION('ref_axis',(-0.517596781651614,-0.015677848278934,-0.855481020652846));
#58352=DIRECTION('',(-0.85558642428887,3.88578058618816E-13,0.517659995144097));
#58353=DIRECTION('center_axis',(-0.720953073140382,0.584827952253987,0.371756550166701));
#58354=DIRECTION('ref_axis',(0.459879282372611,0.0024618045807253,0.887978031914449));
#58355=DIRECTION('center_axis',(-0.886402301307037,6.8040664922404E-10,
0.462915716127234));
#58356=DIRECTION('ref_axis',(-0.462858873032855,0.0156707406196535,-0.886293456786852));
#58357=DIRECTION('',(0.886402259955158,-6.3782312761799E-11,-0.462915795308811));
#58358=DIRECTION('',(-0.238950069590406,1.64268989065784E-13,0.971031855421201));
#58359=DIRECTION('center_axis',(0.677733656698397,-0.60109852802926,-0.423506375606408));
#58360=DIRECTION('ref_axis',(0.525496001044302,-0.0069195257270167,0.850767931371511));
#58361=DIRECTION('',(0.954111946850913,2.37574025439388E-11,0.299450150903886));
#58362=DIRECTION('center_axis',(0.,-1.,1.45983193964168E-32));
#58363=DIRECTION('ref_axis',(1.,0.,0.));
#58364=DIRECTION('center_axis',(-0.675918227587769,0.601098527795593,0.426397830079587));
#58365=DIRECTION('ref_axis',(0.527806431987649,-0.00897201507403433,0.849317298362619));
#58366=DIRECTION('center_axis',(-0.689650908208436,-0.601098528172786,0.403809589083505));
#58367=DIRECTION('ref_axis',(0.510415466722804,-0.0079457331077057,0.859891223734446));
#58368=DIRECTION('center_axis',(0.691369715830186,0.601098527946894,-0.400859670873694));
#58369=DIRECTION('ref_axis',(0.506737309962297,-0.00794575175649518,0.86206389770202));
#58370=DIRECTION('center_axis',(-0.648087860160526,0.584827952230098,0.487809790597627));
#58371=DIRECTION('ref_axis',(0.590766628055431,-0.0181546317021972,0.806638209189085));
#58372=DIRECTION('center_axis',(0.82139394033835,-5.4349324088216E-10,-0.570361284428947));
#58373=DIRECTION('ref_axis',(-0.570291169341544,-0.0156795066169794,-0.82129296553867));
#58374=DIRECTION('',(-0.821393981728642,2.06171937742879E-7,0.570361224821538));
#58375=DIRECTION('center_axis',(-0.668671281884745,0.584827782536624,0.45918970105601));
#58376=DIRECTION('ref_axis',(0.549511870148897,-0.0273551074063184,0.835037964804146));
#58377=DIRECTION('center_axis',(-0.855586480187597,7.32921391904566E-10,
0.517659902754887));
#58378=DIRECTION('ref_axis',(-0.517596080894988,0.0157023279262901,-0.855480995662583));
#58379=DIRECTION('',(-0.855586424696769,-1.29267420091793E-5,0.517659994308522));
#58380=DIRECTION('',(-0.177506922439442,-7.62631952260005E-8,0.984119551927545));
#58381=DIRECTION('center_axis',(0.82139397988059,-7.72262198065806E-12,
-0.570361227483009));
#58382=DIRECTION('ref_axis',(-0.440248283571863,-0.635772805084867,-0.634014502299867));
#58383=DIRECTION('',(-0.971031855420821,0.,-0.23895006959195));
#58384=DIRECTION('center_axis',(-0.720807042413305,0.39856439157804,0.567083444806328));
#58385=DIRECTION('ref_axis',(0.618316971226236,-4.58880547466017E-16,0.785928828262212));
#58386=DIRECTION('center_axis',(0.779597758089364,5.74456436517556E-5,-0.62628055397085));
#58387=DIRECTION('ref_axis',(0.626280497553244,0.000362750097935672,0.77959772113368));
#58388=DIRECTION('',(-0.783960434937737,5.9497369157871E-5,0.620810786723538));
#58389=DIRECTION('center_axis',(-0.671432082927573,0.590180063811423,0.448181269460343));
#58390=DIRECTION('ref_axis',(-0.390733176690629,-0.795821494105799,0.462596729509043));
#58391=DIRECTION('center_axis',(0.194950885198616,0.550037558002531,0.812067015182176));
#58392=DIRECTION('ref_axis',(1.0056084917372E-16,-0.827952943501162,0.560797577872588));
#58393=DIRECTION('center_axis',(-0.872968580275457,-0.47712608966723,-0.101373331851685));
#58394=DIRECTION('ref_axis',(0.167281242125899,-0.0976209729541355,-0.98106428518844));
#58395=DIRECTION('center_axis',(0.,-1.,1.45983193964168E-32));
#58396=DIRECTION('ref_axis',(1.,0.,0.));
#58397=DIRECTION('center_axis',(-0.786810699055945,0.601098526818443,0.140033870573491));
#58398=DIRECTION('ref_axis',(0.172015417774543,-0.0043281742326977,0.985084749123476));
#58399=DIRECTION('center_axis',(-0.788661315181863,-0.601098528412519,0.12920483379471));
#58400=DIRECTION('ref_axis',(0.164122137841156,-0.00330174737487977,0.986434499769103));
#58401=DIRECTION('center_axis',(0.787401802179485,-0.601098528054466,-0.136670997271746));
#58402=DIRECTION('ref_axis',(0.169327964798454,-0.00227571930843304,0.985557132508736));
#58403=DIRECTION('center_axis',(0.789206135165619,0.601098527541506,-0.125834162310476));
#58404=DIRECTION('ref_axis',(0.159906318021571,-0.0033019368237457,0.987126672048728));
#58405=DIRECTION('center_axis',(0.,-1.,1.45983193964168E-32));
#58406=DIRECTION('ref_axis',(1.,0.,0.));
#58407=DIRECTION('center_axis',(-0.763055658010031,0.601098527992998,0.237542885440774));
#58408=DIRECTION('ref_axis',(0.272153471330359,-0.0345384700759067,0.961633808748242));
#58409=DIRECTION('center_axis',(-0.788661313920426,-0.601098533000795,0.129204820148475));
#58410=DIRECTION('ref_axis',(0.186403448113438,-0.0335099185808696,0.981901644711997));
#58411=DIRECTION('center_axis',(0.76406356176432,-0.601098537476189,-0.234280647574671));
#58412=DIRECTION('ref_axis',(0.26955334695223,-0.032481514321347,0.962437501541914));
#58413=DIRECTION('center_axis',(0.789206140541634,0.601098522388829,-0.125834153207089));
#58414=DIRECTION('ref_axis',(0.182206791918155,-0.0335101061238788,0.982689044289424));
#58415=DIRECTION('center_axis',(0.,-1.,1.45983193964168E-32));
#58416=DIRECTION('ref_axis',(1.,0.,0.));
#58417=DIRECTION('center_axis',(-0.798157352253882,0.601098536492064,0.0403161316369818));
#58418=DIRECTION('ref_axis',(0.0698515706646391,0.0258666611243446,0.997221978256577));
#58419=DIRECTION('center_axis',(-0.788661314308054,-0.601098522653569,0.129204865920715));
#58420=DIRECTION('ref_axis',(0.141618704730856,0.0268944934460804,0.989555874467245));
#58421=DIRECTION('center_axis',(0.798322321900873,-0.601098527948964,-0.0369056913278559));
#58422=DIRECTION('ref_axis',(0.0671306538928277,0.027922015095456,0.997353415986996));
#58423=DIRECTION('center_axis',(0.789206130815412,0.601098532003673,-0.125834168278713));
#58424=DIRECTION('ref_axis',(0.137389735591166,0.0268942886600805,0.99015188622335));
#58425=DIRECTION('center_axis',(0.,-1.,1.45983193964168E-32));
#58426=DIRECTION('ref_axis',(1.,0.,0.));
#58427=DIRECTION('center_axis',(-0.760723846485499,0.601098528328861,0.244907714515458));
#58428=DIRECTION('ref_axis',(0.321534013967133,0.0212181329446819,0.946660271003556));
#58429=DIRECTION('center_axis',(-0.734823571847927,-0.60109852793342,0.314189239110651));
#58430=DIRECTION('ref_axis',(0.377605244297892,0.0222452123488197,0.925699427463518));
#58431=DIRECTION('center_axis',(0.761763160169678,-0.601098528110665,-0.241655637864085));
#58432=DIRECTION('ref_axis',(0.318938028103574,0.0232723692944289,0.947489805252187));
#58433=DIRECTION('center_axis',(0.73615909432316,0.601098528132069,-0.31104717861245));
#58434=DIRECTION('ref_axis',(0.373647180134697,0.0222452071622992,0.927304122462364));
#58435=DIRECTION('center_axis',(0.,-1.,1.45983193964168E-32));
#58436=DIRECTION('ref_axis',(1.,0.,0.));
#58437=DIRECTION('center_axis',(-0.785420383285721,0.601098529650706,0.147632581671769));
#58438=DIRECTION('ref_axis',(0.22240539569108,0.0514849804187075,0.973593928061787));
#58439=DIRECTION('center_axis',(0.736159119253747,0.601098531981097,-0.311047112170677));
#58440=DIRECTION('ref_axis',(0.351983410607425,0.0525165497891723,0.934531802912777));
#58441=DIRECTION('',(-0.957443409238448,3.88578058618629E-13,0.288621063170827));
#58442=DIRECTION('center_axis',(-0.764517729382288,0.58482795214616,0.271088376454395));
#58443=DIRECTION('ref_axis',(0.29771334017134,-0.0526562728465342,0.953202016371102));
#58444=DIRECTION('center_axis',(-0.973676803711829,7.80713441197243E-10,
0.227933064546407));
#58445=DIRECTION('ref_axis',(-0.227904709319416,0.0157729998142581,-0.973555676860287));
#58446=DIRECTION('',(0.973676779880511,-1.76914038951382E-10,-0.227933166348205));
#58447=DIRECTION('',(-0.472928816313912,0.,0.88110063823602));
#58448=DIRECTION('',(0.849666541299393,6.73708191429312E-11,0.527320366187697));
#58449=DIRECTION('center_axis',(-0.782151896996921,0.584827930051179,0.214976050424628));
#58450=DIRECTION('ref_axis',(0.280192919632944,0.0219594825691283,0.959692507479798));
#58451=DIRECTION('center_axis',(0.937430225687632,-1.00225340753624E-8,
-0.348173192487928));
#58452=DIRECTION('ref_axis',(-0.348130065144794,-0.0157391393476006,-0.937314108095508));
#58453=DIRECTION('',(-0.937431446873868,0.,0.348169904517848));
#58454=DIRECTION('center_axis',(-0.790755100933366,0.584827952320552,0.180783396727721));
#58455=DIRECTION('ref_axis',(0.245384617050075,0.0322834330615039,0.968888109982237));
#58456=DIRECTION('center_axis',(-0.957443430531097,5.48477399997537E-10,
0.288620992536655));
#58457=DIRECTION('ref_axis',(-0.28858540981457,0.0157020800817192,-0.957325391872201));
#58458=DIRECTION('',(0.95744340923852,-1.22124532708705E-12,-0.288621063170588));
#58459=DIRECTION('',(-0.41667083249281,0.,0.909057433471477));
#58460=DIRECTION('',(0.881100638236075,1.43735365432681E-13,0.47292881631381));
#58461=DIRECTION('center_axis',(-0.749040407174815,0.584827953375321,0.311311312628085));
#58462=DIRECTION('ref_axis',(0.378544724024558,-0.00784642890859345,0.925549742297276));
#58463=DIRECTION('center_axis',(0.913719640106859,-1.87941711854915E-9,
-0.406345197194444));
#58464=DIRECTION('ref_axis',(-0.406295255358328,-0.0156778482813538,-0.913607339367728));
#58465=DIRECTION('',(-0.913719870860235,3.88578058618638E-13,0.406344678315288));
#58466=DIRECTION('center_axis',(-0.76186159335239,0.584827952253948,0.278465758823256));
#58467=DIRECTION('ref_axis',(0.344959838796073,0.00246180458216537,0.938614217416286));
#58468=DIRECTION('center_axis',(-0.937431470422838,5.10643621529069E-10,
0.348169841113322));
#58469=DIRECTION('ref_axis',(-0.348127088079396,0.0156707406182868,-0.937316359845402));
#58470=DIRECTION('',(0.937431446873923,-6.41708908203887E-11,-0.348169904517699));
#58471=DIRECTION('',(-0.35876843925459,1.64268989065808E-13,0.933426594325888));
#58472=DIRECTION('center_axis',(0.725468946368522,-0.601098528002572,-0.335224353960282));
#58473=DIRECTION('ref_axis',(0.414722814901041,-0.00691952791939243,0.909921483939098));
#58474=DIRECTION('',(0.909057433466349,2.35931335548692E-11,0.416670832503999));
#58475=DIRECTION('center_axis',(-0.811136126793454,0.584827951389749,0.00586950456028211));
#58476=DIRECTION('ref_axis',(0.0263728513782388,0.0265489690017877,0.99929956717449));
#58477=DIRECTION('center_axis',(0.994566648832187,8.50721872347641E-12,
-0.104101782072709));
#58478=DIRECTION('ref_axis',(-0.104088873058919,-0.0157477670547349,-0.994443318816168));
#58479=DIRECTION('center_axis',(-0.998722132347498,-0.000115441181840488,
0.0505379959297901));
#58480=DIRECTION('ref_axis',(0.00137233352454056,-0.999690590777516,0.0248362519635856));
#58481=DIRECTION('',(0.999140703554945,-6.069034161454E-10,-0.041447008332686));
#58482=DIRECTION('',(0.735806627409681,2.24206636476401E-10,0.677191706284115));
#58483=DIRECTION('center_axis',(-0.80400442922631,0.584827952222711,0.107485552905802));
#58484=DIRECTION('ref_axis',(0.130176731431605,-0.00326197145312202,0.991485440203749));
#58485=DIRECTION('center_axis',(0.986067481394172,-5.51759956911657E-10,
-0.166345790860347));
#58486=DIRECTION('ref_axis',(-0.166325332124458,-0.0156832196314432,-0.985946205690595));
#58487=DIRECTION('',(-0.986067493321454,8.32135976760707E-8,0.16634572015756));
#58488=DIRECTION('center_axis',(-0.807915700396783,0.584827969931553,0.0724463017559439));
#58489=DIRECTION('ref_axis',(0.0943677593143437,0.00704480134984,0.995512479467702));
#58490=DIRECTION('center_axis',(-0.994566657124383,6.29001243004044E-10,
0.104101702850767));
#58491=DIRECTION('ref_axis',(-0.104088918533863,0.0156715280532925,-0.994444518435758));
#58492=DIRECTION('',(0.994566648423263,-1.40443212613673E-11,-0.104101785979482));
#58493=DIRECTION('',(-0.579630810343145,-3.07808057783809E-8,0.814879208043099));
#58494=DIRECTION('center_axis',(0.112789953813512,0.793626260378774,0.597859335593205));
#58495=DIRECTION('ref_axis',(-8.52455597729631E-17,-0.601698864106725,0.798723028923467));
#58496=DIRECTION('center_axis',(-0.734975505034963,0.4715466745576,-0.487293279978568));
#58497=DIRECTION('ref_axis',(-0.319218617798124,0.393407181090822,0.862166030366094));
#58498=DIRECTION('',(0.776875900240113,5.05127141378944E-12,0.629653742644411));
#58499=DIRECTION('center_axis',(-0.784195235649416,0.584828255987556,0.207397549125613));
#58500=DIRECTION('ref_axis',(0.232410023807321,-0.0330815410766171,0.972055138597537));
#58501=DIRECTION('center_axis',(0.973669013264507,-1.08193100855599E-7,
-0.227966340955215));
#58502=DIRECTION('ref_axis',(-0.227938333995393,-0.0156751635311225,-0.973549385056391));
#58503=DIRECTION('',(-0.973676779881119,7.77156117237206E-13,0.22793316634561));
#58504=DIRECTION('center_axis',(-0.792465661813423,0.584827952226059,0.17313128296668));
#58505=DIRECTION('ref_axis',(0.197321433282868,-0.022760729597827,0.980074589587634));
#58506=DIRECTION('center_axis',(-0.986067510765312,8.16820737104964E-10,
0.166345616753496));
#58507=DIRECTION('ref_axis',(-0.166325131471838,0.015693390508592,-0.985946077701626));
#58508=DIRECTION('',(0.986067493104091,-2.20934381896923E-11,-0.166345721446069));
#58509=DIRECTION('',(-0.527320366157622,0.,0.849666541318058));
#58510=DIRECTION('',(0.814879198734754,8.17238220596398E-12,0.579630823429366));
#58511=DIRECTION('center_axis',(0.,-1.,1.45983193964168E-32));
#58512=DIRECTION('ref_axis',(1.,0.,0.));
#58513=DIRECTION('center_axis',(-0.724030231397888,0.601098527836107,0.338320534190856));
#58514=DIRECTION('ref_axis',(0.417196833668173,-0.00897201206616011,0.908771866299092));
#58515=DIRECTION('center_axis',(-0.734823570967135,-0.601098528090507,0.314189240870107));
#58516=DIRECTION('ref_axis',(0.398617732222085,-0.00794574009299561,0.917082749141263));
#58517=DIRECTION('center_axis',(0.736159098339688,0.601098527936454,-0.311047169484511));
#58518=DIRECTION('ref_axis',(0.394696278215606,-0.00794575246477388,0.91877729237314));
#58519=DIRECTION('center_axis',(-0.704116272226526,0.584827952230066,0.402736317553072));
#58520=DIRECTION('ref_axis',(0.485009681668631,-0.0181546317046172,0.874320317752804));
#58521=DIRECTION('center_axis',(0.886402227295928,-5.52722010689124E-10,
-0.462915857845481));
#58522=DIRECTION('ref_axis',(-0.462858951134617,-0.015679506619194,-0.886293260962048));
#58523=DIRECTION('',(-0.88640226145087,2.06171882231894E-7,0.462915792444739));
#58524=DIRECTION('center_axis',(-0.720950339151385,0.584827782536519,0.37176211917155));
#58525=DIRECTION('ref_axis',(0.440520796653547,-0.0273551074137171,0.897325540600572));
#58526=DIRECTION('center_axis',(-0.913719924310483,9.17652330754914E-10,
0.406344558125301));
#58527=DIRECTION('ref_axis',(-0.406294460236443,0.0157023279264494,-0.913607272562378));
#58528=DIRECTION('',(-0.91371987116053,-1.29267419736916E-5,0.406344677434421));
#58529=DIRECTION('',(-0.299450112994252,-7.6263051490643E-8,0.954111958748932));
#58530=DIRECTION('center_axis',(0.886402259958573,5.51249576955609E-12,
-0.462915795302272));
#58531=DIRECTION('ref_axis',(-0.357313706641208,-0.635772805085359,-0.68419284953894));
#58532=DIRECTION('',(-0.933426594325549,0.,-0.358768439255471));
#58533=DIRECTION('center_axis',(-0.786197665429277,0.398564391573593,0.472270745063811));
#58534=DIRECTION('ref_axis',(0.514938355828264,6.04616573156442E-16,0.857227210077284));
#58535=DIRECTION('center_axis',(0.85194416384702,5.74456530678644E-5,-0.52363263686195));
#58536=DIRECTION('ref_axis',(0.523632585407709,0.000363224037420787,0.851944119979437));
#58537=DIRECTION('',(-0.855586896082275,5.94973699395157E-5,0.517659211945815));
#58538=DIRECTION('center_axis',(-0.722309648058218,0.590180063816037,0.360494472351674));
#58539=DIRECTION('ref_axis',(-0.445631531500632,-0.795821662861919,0.409976120099806));
#58540=DIRECTION('center_axis',(0.0916346543585759,0.550037558005875,0.830097449040484));
#58541=DIRECTION('ref_axis',(-1.25152671372798E-16,-0.833604678715212,0.552361511715025));
#58542=DIRECTION('center_axis',(-0.853379514155569,-0.477126090889111,-0.209985947654791));
#58543=DIRECTION('ref_axis',(0.288925961123907,-0.0976286666970697,-0.952360452994337));
#58544=DIRECTION('center_axis',(0.,-1.,1.45983193964168E-32));
#58545=DIRECTION('ref_axis',(1.,0.,0.));
#58546=DIRECTION('center_axis',(-0.786810702938747,0.601098516361292,0.140033893644677));
#58547=DIRECTION('ref_axis',(0.149483054325176,-0.0345386753521871,0.988160865636022));
#58548=DIRECTION('center_axis',(-0.798636142119035,-0.601098532740246,0.0293405255363244));
#58549=DIRECTION('ref_axis',(0.0618686902012185,-0.0335099203682645,0.997521603981437));
#58550=DIRECTION('center_axis',(0.787401802117191,-0.60109852815296,-0.136670997197453));
#58551=DIRECTION('ref_axis',(0.1468026567879,-0.0324816839227375,0.988632348332563));
#58552=DIRECTION('center_axis',(0.798754216513376,0.601098522019537,-0.0259281396947761));
#58553=DIRECTION('ref_axis',(0.057606428403082,-0.0335101155912361,0.997776814502974));
#58554=DIRECTION('center_axis',(0.,-1.,1.45983193964168E-32));
#58555=DIRECTION('ref_axis',(1.,0.,0.));
#58556=DIRECTION('center_axis',(-0.797730380527669,0.60109852822162,0.0480291510749676));
#58557=DIRECTION('ref_axis',(0.0986279656220281,0.051484996853496,0.993791637867946));
#58558=DIRECTION('center_axis',(0.769338807450739,0.601098527991798,-0.216329283723609));
#58559=DIRECTION('ref_axis',(0.232080081996,0.0525165954341669,0.971277943095968));
#58560=DIRECTION('center_axis',(0.,-1.,1.45983193964168E-32));
#58561=DIRECTION('ref_axis',(1.,0.,0.));
#58562=DIRECTION('center_axis',(-0.798157359514994,0.60109852682156,0.0403161320689704));
#58563=DIRECTION('ref_axis',(0.047195167488092,-0.00432817393868725,0.998876310198679));
#58564=DIRECTION('center_axis',(-0.79863614492077,-0.601098528403341,0.0293405381243889));
#58565=DIRECTION('ref_axis',(0.0391949569049173,-0.00330174988199066,0.999226127461116));
#58566=DIRECTION('center_axis',(0.798322321310044,-0.601098528021013,-0.036905702934847));
#58567=DIRECTION('ref_axis',(0.0444697099494423,-0.00227572610152403,0.999008141091815));
#58568=DIRECTION('center_axis',(0.798754211449592,0.601098527548076,-0.0259281675225105));
#58569=DIRECTION('ref_axis',(0.03492563283816,-0.00330193561822562,0.999384459250807));
#58570=DIRECTION('center_axis',(0.,-1.,1.45983193964168E-32));
#58571=DIRECTION('ref_axis',(1.,0.,0.));
#58572=DIRECTION('center_axis',(-0.796916594028537,0.601098536374166,-0.0600374194214937));
#58573=DIRECTION('ref_axis',(-0.0556842885238396,0.0258666638057379,0.998113308054328));
#58574=DIRECTION('center_axis',(-0.798636147949864,-0.601098522706458,0.0293405723856551));
#58575=DIRECTION('ref_axis',(0.0164777599185274,0.0268944923173048,0.999502461083044));
#58576=DIRECTION('center_axis',(0.796652821507865,-0.601098527915204,0.0634416402824783));
#58577=DIRECTION('ref_axis',(-0.0584002209349251,0.0279220158115366,0.99790268825561));
#58578=DIRECTION('center_axis',(0.798754207866941,0.601098531819143,-0.025928178874069));
#58579=DIRECTION('ref_axis',(0.0122074444057763,0.0268942928144612,0.999563742497241));
#58580=DIRECTION('center_axis',(0.,-1.,1.45983193964168E-32));
#58581=DIRECTION('ref_axis',(1.,0.,0.));
#58582=DIRECTION('center_axis',(-0.760723845934306,0.601098527910175,0.24490771725517));
#58583=DIRECTION('ref_axis',(0.300007788767924,-0.00897200679300414,0.953894559043444));
#58584=DIRECTION('center_axis',(-0.768407619804461,-0.601098528125849,0.219613955183591));
#58585=DIRECTION('ref_axis',(0.280533569597203,-0.00794573722101145,0.959811326037084));
#58586=DIRECTION('center_axis',(0.761763161499585,-0.601098528053865,-0.241655633813147));
#58587=DIRECTION('ref_axis',(0.297409194101466,-0.00691952345940434,0.954725034477996));
#58588=DIRECTION('center_axis',(0.769338810340699,0.601098527970217,-0.216329273505912));
#58589=DIRECTION('ref_axis',(0.276430654457888,-0.00794574992649899,0.961001018903773));
#58590=DIRECTION('center_axis',(0.,-1.,1.45983193964168E-32));
#58591=DIRECTION('ref_axis',(1.,0.,0.));
#58592=DIRECTION('center_axis',(-0.785420387740065,0.601098528306397,0.147632563447667));
#58593=DIRECTION('ref_axis',(0.200350628531198,0.0212181335979679,0.979494469843384));
#58594=DIRECTION('center_axis',(-0.768407622369157,-0.601098527984367,0.219613946597221));
#58595=DIRECTION('ref_axis',(0.258606809898566,0.0222452109926528,0.965726497752847));
#58596=DIRECTION('center_axis',(0.786043913939973,-0.601098527958986,-0.144275864383021));
#58597=DIRECTION('ref_axis',(0.197671140201316,0.0232723733017627,0.979992100464292));
#58598=DIRECTION('center_axis',(0.769338810009928,0.601098528244495,-0.216329273920128));
#58599=DIRECTION('ref_axis',(0.254478832329244,0.0222452039836464,0.966822462914506));
#58600=DIRECTION('center_axis',(-0.802928197021279,0.584827908067885,0.115250285783159));
#58601=DIRECTION('ref_axis',(0.157701346099928,0.021960067734333,0.987242645383279));
#58602=DIRECTION('center_axis',(0.973675213540049,-1.90745723150787E-8,
-0.227939857282003));
#58603=DIRECTION('ref_axis',(-0.227911623139389,-0.0157391387082283,-0.973554606352767));
#58604=DIRECTION('',(-0.973676779881003,0.,0.227933166346105));
#58605=DIRECTION('center_axis',(-0.807177928462317,0.584827952320411,0.0802499718878338));
#58606=DIRECTION('ref_axis',(0.122015806264322,0.0322834330627758,0.992002985364131));
#58607=DIRECTION('center_axis',(-0.986067506113591,5.83269785121389E-10,
0.166345644328079));
#58608=DIRECTION('ref_axis',(-0.16632513635319,0.015702080082056,-0.985945938527153));
#58609=DIRECTION('',(0.986067493104161,-4.44089209849969E-13,-0.166345721445658));
#58610=DIRECTION('',(-0.527320366157736,0.,0.849666541317987));
#58611=DIRECTION('',(0.814879198737098,1.43735365432635E-13,0.579630823426072));
#58612=DIRECTION('center_axis',(-0.782151653290743,0.58482795337546,0.214976873652094));
#58613=DIRECTION('ref_axis',(0.259557643791007,-0.00784642891460876,0.965695740439476));
#58614=DIRECTION('center_axis',(0.957443242800339,-1.9481252264197E-9,-0.288621615295826));
#58615=DIRECTION('ref_axis',(-0.28858614228077,-0.0156778482810863,-0.957325568214272));
#58616=DIRECTION('',(-0.95744340923868,-3.88578058618785E-13,0.288621063170055));
#58617=DIRECTION('center_axis',(-0.790755101119389,0.584827952254179,0.180783396128763));
#58618=DIRECTION('ref_axis',(0.224600172503117,0.00246180457544701,0.974447896005632));
#58619=DIRECTION('center_axis',(-0.97367679496501,4.99433705161115E-10,
0.227933101910772));
#58620=DIRECTION('ref_axis',(-0.227905113178174,0.0156707406176226,-0.973557233692883));
#58621=DIRECTION('',(0.973676779880786,-6.4614980030186E-11,-0.227933166347032));
#58622=DIRECTION('',(-0.472928816313917,1.64268989065853E-13,0.881100638236018));
#58623=DIRECTION('',(0.849666541311608,2.34493981894313E-11,0.527320366168015));
#58624=DIRECTION('center_axis',(-0.749021847116042,0.584826536165524,0.311358627854613));
#58625=DIRECTION('ref_axis',(0.371641576311207,-0.0181846249388088,0.928198178285627));
#58626=DIRECTION('center_axis',(0.93743142220389,-5.5501891853302E-10,-0.348169970940619));
#58627=DIRECTION('ref_axis',(-0.348127170059145,-0.0156795066183704,-0.937316182800028));
#58628=DIRECTION('',(-0.937431447998895,2.06171549165055E-7,0.348169901488703));
#58629=DIRECTION('center_axis',(-0.761859578893809,0.584827782536394,0.278471626600113));
#58630=DIRECTION('ref_axis',(0.32458244704978,-0.0273551074290013,0.945461756584963));
#58631=DIRECTION('center_axis',(-0.957443434474091,5.7096507072109E-10,
0.288620979456547));
#58632=DIRECTION('ref_axis',(-0.288585395612374,0.0157023279254197,-0.957325392088276));
#58633=DIRECTION('',(-0.957443409425798,-1.29267425264385E-5,0.288621062259848));
#58634=DIRECTION('',(-0.416670796384237,-7.6262907755298E-8,0.90905745002201));
#58635=DIRECTION('center_axis',(0.937431446872798,-2.82675655164576E-12,
-0.348169904520728));
#58636=DIRECTION('ref_axis',(-0.268744079138403,-0.635772805084965,-0.723581066807615));
#58637=DIRECTION('',(-0.8811006382351,0.,-0.472928816315627));
#58638=DIRECTION('center_axis',(-0.80547572014595,0.584827951390055,-0.0958390918585707));
#58639=DIRECTION('ref_axis',(-0.099080552477698,0.0265489689961426,0.994725186353475));
#58640=DIRECTION('center_axis',(0.999771606780537,-3.77560611900383E-11,
0.0213713423879551));
#58641=DIRECTION('ref_axis',(0.0213686922602901,-0.0157477670553484,-0.999647631330088));
#58642=DIRECTION('center_axis',(-0.996456868435036,-1.82930342323839E-11,
-0.0841053467304035));
#58643=DIRECTION('ref_axis',(0.00137653801704517,0.999866054443186,-0.0163088416297004));
#58644=DIRECTION('',(0.996456868254416,-6.06792393843473E-10,0.0841053488703394));
#58645=DIRECTION('',(0.645129946086367,2.242066364764E-10,0.76407287130391));
#58646=DIRECTION('center_axis',(-0.81113612606466,0.584827952222608,0.00586952229118291));
#58647=DIRECTION('ref_axis',(0.00488417276115256,-0.00326197144681202,0.999982752050614));
#58648=DIRECTION('center_axis',(0.999140699079624,-8.46367557917498E-10,
-0.0414471162167002));
#58649=DIRECTION('ref_axis',(-0.0414420186801338,-0.0156832196316866,-0.999017815511665));
#58650=DIRECTION('',(-0.999140703609447,8.32139862541118E-8,0.041447007018758));
#58651=DIRECTION('center_axis',(-0.810624973045738,0.584827969931961,-0.0293836461293935));
#58652=DIRECTION('ref_axis',(-0.0311471567426006,0.0070448013376867,0.999489982641629));
#58653=DIRECTION('center_axis',(-0.999771605135594,5.82131145152661E-10,
-0.021371419339818));
#58654=DIRECTION('ref_axis',(0.0213687948117744,0.0156715280532176,-0.999648827247234));
#58655=DIRECTION('',(0.99977160679441,-1.48769885298236E-11,0.0213713417389642));
#58656=DIRECTION('',(-0.677191694384739,-3.07809495137633E-8,0.735806638361142));
#58657=DIRECTION('center_axis',(0.0369689275944231,0.793626260379842,0.607281365783626));
#58658=DIRECTION('ref_axis',(2.85820292298768E-17,-0.607696777849814,0.794169142054105));
#58659=DIRECTION('center_axis',(-0.668105961212897,0.471546674538878,-0.575567683529154));
#58660=DIRECTION('ref_axis',(-0.424756903944142,0.393410586642562,0.815358622245048));
#58661=DIRECTION('',(0.691833462133554,5.05127141378853E-12,0.722057103470564));
#58662=DIRECTION('center_axis',(-0.804005427452842,0.584828255987393,0.107476432882369));
#58663=DIRECTION('ref_axis',(0.108746587635101,-0.0330815410815246,0.993518893286581));
#58664=DIRECTION('center_axis',(0.994563100012491,-1.08262028849995E-7,
-0.104135681173802));
#58665=DIRECTION('ref_axis',(-0.10412288844737,-0.0156751635309253,-0.994440904905694));
#58666=DIRECTION('',(-0.994566648423227,3.88578058618661E-13,0.104101785979821));
#58667=DIRECTION('center_axis',(-0.807915936897736,0.584827952226153,0.0724438071999103));
#58668=DIRECTION('ref_axis',(0.0729295773933777,-0.0227607295944781,0.997077341999882));
#58669=DIRECTION('center_axis',(-0.999140706646079,5.68849416964949E-10,
0.0414469338163077));
#58670=DIRECTION('ref_axis',(-0.0414418296657482,0.0156933905078002,-0.999017663631792));
#58671=DIRECTION('',(0.999140703555315,-2.24820162483055E-11,-0.041447008323772));
#58672=DIRECTION('',(-0.62965374264226,0.,0.776875900241856));
#58673=DIRECTION('',(0.735806627486024,8.0286468406269E-12,0.677191706201164));
#58674=DIRECTION('',(-0.986067493104082,7.77156117237022E-13,0.166345721446123));
#58675=DIRECTION('center_axis',(-0.792465661535707,0.584827952145603,0.173131284509631));
#58676=DIRECTION('ref_axis',(0.175897890621741,-0.0526562728545463,0.98299910936068));
#58677=DIRECTION('center_axis',(-0.994566657961751,6.7861735203041E-10,
0.104101694850723));
#58678=DIRECTION('ref_axis',(-0.104088744433143,0.0157729998146477,-0.994442932379319));
#58679=DIRECTION('',(0.994566648423056,-1.76525460892884E-10,-0.104101785981459));
#58680=DIRECTION('',(-0.579630823425941,0.,0.814879198737191));
#58681=DIRECTION('',(0.776875900220228,6.51531877903912E-11,0.629653742668945));
#58682=DIRECTION('center_axis',(-0.83918948161091,0.39856439156716,0.370010053550321));
#58683=DIRECTION('ref_axis',(-0.429012364341953,-0.903298616871369,3.62132827148377E-16));
#58684=DIRECTION('center_axis',(0.910854901238292,5.74456698535606E-5,-0.412726720228018));
#58685=DIRECTION('ref_axis',(0.412726674652397,0.000363348493937081,0.910854851229463));
#58686=DIRECTION('',(-0.913720240772838,5.94973707566566E-5,0.406343842160909));
#58687=DIRECTION('center_axis',(-0.761795958691224,0.590180063811968,0.267122461804732));
#58688=DIRECTION('ref_axis',(0.493495347852432,0.795819764955679,-0.350903467286796));
#58689=DIRECTION('center_axis',(-0.0131267097189408,0.550037558010457,0.835036750251058));
#58690=DIRECTION('ref_axis',(6.76045893512397E-18,-0.835108702353105,0.550084952761038));
#58691=DIRECTION('center_axis',(-0.820332144360729,-0.477126090118974,-0.315286959857698));
#58692=DIRECTION('ref_axis',(0.406006491071471,-0.0976208218760109,-0.908641240723798));
#58693=DIRECTION('center_axis',(-0.87894677835708,0.398564391567542,0.261914082458552));
#58694=DIRECTION('ref_axis',(-0.412981067386498,-0.910739610415792,-1.42150438893369E-16));
#58695=DIRECTION('center_axis',(0.955400912707171,5.74456423295275E-5,-0.295311856684258));
#58696=DIRECTION('ref_axis',(0.295311817796603,0.000362973412833882,0.955400857504308));
#58697=DIRECTION('',(-0.957443671436405,5.94973691223933E-5,0.288620187246907));
#58698=DIRECTION('center_axis',(-0.789268291903739,0.590180063813734,0.169537770635844));
#58699=DIRECTION('ref_axis',(0.533588748824947,0.795821946541685,-0.2862699364761));
#58700=DIRECTION('center_axis',(-0.117681057741536,0.550037558015597,0.826807023084028));
#58701=DIRECTION('ref_axis',(4.25184181647116E-17,-0.832592338318892,0.553886268265137));
#58702=DIRECTION('center_axis',(-0.774347645955717,-0.477126090634454,-0.415615708123167));
#58703=DIRECTION('ref_axis',(0.516691144115654,-0.0976284509969061,-0.850587412996689));
#58704=DIRECTION('center_axis',(-0.0394351207028803,0.793626260377946,0.607126206067294));
#58705=DIRECTION('ref_axis',(-1.39708533644483E-17,-0.607598837097768,0.794244076564276));
#58706=DIRECTION('center_axis',(-0.590699987197054,0.471546674561303,-0.654765040938791));
#58707=DIRECTION('ref_axis',(-0.523594102005531,0.3934170135974,0.75569323786648));
#58708=DIRECTION('center_axis',(-1.19900741137893E-16,-1.,1.45983193964168E-32));
#58709=DIRECTION('ref_axis',(-1.,1.19900741137893E-16,0.));
#58710=DIRECTION('center_axis',(-1.19900741137893E-16,-1.,1.45983193964168E-32));
#58711=DIRECTION('ref_axis',(-1.,1.19900741137893E-16,0.));
#58712=DIRECTION('center_axis',(-1.19900741137893E-16,-1.,1.45983193964168E-32));
#58713=DIRECTION('ref_axis',(-1.,1.19900741137893E-16,0.));
#58714=DIRECTION('center_axis',(-0.796301631197733,-0.584827952229447,0.154531480426938));
#58715=DIRECTION('ref_axis',(0.174895616737967,0.0219588922001345,0.984342079918962));
#58716=DIRECTION('center_axis',(-0.78883375237848,-0.58482795222954,0.188990945284396));
#58717=DIRECTION('ref_axis',(0.210169515934559,0.0322834340869575,0.977131799940717));
#58718=DIRECTION('center_axis',(-0.811140170796249,-0.584827952229906,-0.00528106156067749));
#58719=DIRECTION('ref_axis',(0.0314665010204262,-0.0526562713691229,0.998116815006657));
#58720=DIRECTION('center_axis',(-0.811140170796482,-0.584827952229454,-0.00528106157488254));
#58721=DIRECTION('ref_axis',(0.00990171161333319,-0.0227607290413202,0.999691905199114));
#58722=DIRECTION('center_axis',(-0.81014435690596,-0.584827952229489,-0.0405263773916719));
#58723=DIRECTION('ref_axis',(-0.0260944005329791,-0.0330869094618765,0.999111774869602));
#58724=DIRECTION('center_axis',(-0.811140170796523,-0.584827952229448,-0.00528106156919257));
#58725=DIRECTION('ref_axis',(-0.0115903885860303,0.00704626726206911,0.999908002273257));
#58726=DIRECTION('center_axis',(-0.810144356905825,-0.584827952229486,-0.0405263773944057));
#58727=DIRECTION('ref_axis',(-0.0476118958772688,-0.00326197171456771,0.998860584321709));
#58728=DIRECTION('center_axis',(-0.810144356905296,-0.584827952229881,-0.0405263773992749));
#58729=DIRECTION('ref_axis',(-0.0690517656280587,0.0265489589827359,0.997259748731784));
#58730=DIRECTION('center_axis',(-0.811140170795812,-0.584827952230272,-0.00528106158720195));
#58731=DIRECTION('ref_axis',(-0.0330971952597666,0.0368858773873733,0.99877124894307));
#58732=DIRECTION('center_axis',(0.814941485545711,-0.572651970021063,0.0891072183807034));
#58733=DIRECTION('ref_axis',(0.574939054737167,0.81819623767036,-3.64197201067138E-17));
#58734=DIRECTION('center_axis',(0.876234650030245,-0.398672303280863,-0.270690289229419));
#58735=DIRECTION('ref_axis',(0.414133355848299,0.910216218034938,7.98171504109407E-18));
#58736=DIRECTION('center_axis',(-0.788833752377747,-0.584827952229584,0.18899094528732));
#58737=DIRECTION('ref_axis',(0.252033915040477,-0.0273514773899239,0.967331795380446));
#58738=DIRECTION('center_axis',(-0.796301631197723,-0.584827952229588,0.154531480426454));
#58739=DIRECTION('ref_axis',(0.216973405116302,-0.0376838387932248,0.975449880704305));
#58740=DIRECTION('center_axis',(-0.796301631197232,-0.584827952229512,0.154531480429274));
#58741=DIRECTION('ref_axis',(0.196052058349387,-0.0078465155714681,0.980562095234338));
#58742=DIRECTION('center_axis',(-0.788833752378357,-0.584827952229601,0.18899094528472));
#58743=DIRECTION('ref_axis',(0.231262112084199,0.0024618052359846,0.972888367198075));
#58744=DIRECTION('center_axis',(0.819683524323173,-0.572651970037011,-0.0137346702134645));
#58745=DIRECTION('ref_axis',(0.572705990547634,0.819760848291045,1.96554044353146E-18));
#58746=DIRECTION('center_axis',(0.835398788851755,-0.39867230328298,-0.378377137496526));
#58747=DIRECTION('ref_axis',(0.430693725907008,0.902498152055914,1.54228934430356E-17));
#58748=DIRECTION('center_axis',(-0.758926716337915,-0.584827952229656,0.286367780169868));
#58749=DIRECTION('ref_axis',(0.371285374189789,-0.0273514773865269,0.928115869704598));
#58750=DIRECTION('center_axis',(-0.770654624865961,-0.58482795222928,0.253116011868101));
#58751=DIRECTION('ref_axis',(0.337518792731011,-0.0376838387990361,0.940564188584048));
#58752=DIRECTION('center_axis',(-0.805405980798282,-0.584827952229224,0.0964234016498613));
#58753=DIRECTION('ref_axis',(0.156315586147125,-0.0526562713792445,0.986302567477098));
#58754=DIRECTION('center_axis',(-0.805405980797294,-0.584827952229503,0.0964234016564226));
#58755=DIRECTION('ref_axis',(0.135118252709478,-0.0227607290393984,0.990568022398428));
#58756=DIRECTION('center_axis',(-0.808835428595534,-0.584827952229771,0.0613311971137978));
#58757=DIRECTION('ref_axis',(0.0993332710549336,-0.0330869094570363,0.994503975700504));
#58758=DIRECTION('center_axis',(-0.805405980797101,-0.5848279522295,0.0964234016580494));
#58759=DIRECTION('ref_axis',(0.113822708281416,0.00704626726155522,0.993476089897066));
#58760=DIRECTION('center_axis',(-0.808835428596934,-0.584827952229517,0.0613311970977501));
#58761=DIRECTION('ref_axis',(0.0779539650531781,-0.0032619717164415,0.996951623135751));
#58762=DIRECTION('center_axis',(-0.808835428596281,-0.584827952229553,0.0613311971060317));
#58763=DIRECTION('ref_axis',(0.0564825171890357,0.0265489589884549,0.998050538814854));
#58764=DIRECTION('center_axis',(-0.80540598079873,-0.584827952230285,0.0964234016396851));
#58765=DIRECTION('ref_axis',(0.0923430162306484,0.0368858773872494,0.995043817830551));
#58766=DIRECTION('center_axis',(-0.758926716341125,-0.584827952229569,0.286367780161537));
#58767=DIRECTION('ref_axis',(0.351373786213101,0.00246180523518679,0.93623202352689));
#58768=DIRECTION('center_axis',(-0.770654624866236,-0.584827952229576,0.25311601186658));
#58769=DIRECTION('ref_axis',(0.317403147406832,-0.00784651558018333,0.948258231817413));
#58770=DIRECTION('center_axis',(-0.770654624861251,-0.584827952229353,0.253116011882271));
#58771=DIRECTION('ref_axis',(0.2968872883741,0.02195889220305,0.954660015427005));
#58772=DIRECTION('center_axis',(-0.75892671634115,-0.584827952229477,0.286367780161659));
#58773=DIRECTION('ref_axis',(0.330979354631449,0.0322834340865671,0.943085598814513));
#58774=DIRECTION('center_axis',(0.811498664278269,-0.572651970034831,-0.116359954837616));
#58775=DIRECTION('ref_axis',(0.576568537396316,0.817048787824003,-1.47601094058414E-16));
#58776=DIRECTION('center_axis',(0.781388189730918,-0.398672303283029,-0.480096752274001));
#58777=DIRECTION('ref_axis',(-0.523498180784514,8.42991561846578E-17,-0.852026792252042));
#58778=DIRECTION('center_axis',(-0.717050952619425,-0.584827952229777,0.379228424090681));
#58779=DIRECTION('ref_axis',(0.484681441192821,-0.0273514773836963,0.874263002332924));
#58780=DIRECTION('center_axis',(-0.732853934721158,-0.584827952229817,0.347708752628398));
#58781=DIRECTION('ref_axis',(0.452741307384835,-0.0376838387856906,0.890845237334659));
#58782=DIRECTION('center_axis',(-0.717050952628536,-0.584827952229634,0.379228424073675));
#58783=DIRECTION('ref_axis',(0.465944085829832,0.00246180523198907,0.884810741568615));
#58784=DIRECTION('center_axis',(-0.73285393472127,-0.584827952229536,0.347708752628632));
#58785=DIRECTION('ref_axis',(0.433748599251106,-0.00784651556579437,0.900999769612168));
#58786=DIRECTION('center_axis',(-0.794770682400051,-0.584827952229808,0.162221541997498));
#58787=DIRECTION('ref_axis',(0.223194397613665,-0.0330869094539688,0.974212254745678));
#58788=DIRECTION('center_axis',(-0.786970057354105,-0.584827952229501,0.196607210241956));
#58789=DIRECTION('ref_axis',(0.258203898243506,-0.0227607290377056,0.96582229014738));
#58790=DIRECTION('center_axis',(-0.786970057353186,-0.584827952229392,0.196607210245963));
#58791=DIRECTION('ref_axis',(0.237440753049131,0.00704626726436888,0.971376466108327));
#58792=DIRECTION('center_axis',(-0.794770682404231,-0.584827952229529,0.162221541978031));
#58793=DIRECTION('ref_axis',(0.202290445390172,-0.00326197171572208,0.979320139302961));
#58794=DIRECTION('center_axis',(-0.794770682403762,-0.58482795222973,0.162221541979603));
#58795=DIRECTION('ref_axis',(0.181126036956144,0.0265489589848099,0.983101475694846));
#58796=DIRECTION('center_axis',(-0.786970057355164,-0.584827952229715,0.196607210237081));
#58797=DIRECTION('ref_axis',(0.216326923204146,0.0368858773959806,0.97562395129771));
#58798=DIRECTION('center_axis',(-0.7170509526256,-0.58482795222946,0.379228424079493));
#58799=DIRECTION('ref_axis',(0.446569451189646,0.0322834340870415,0.894166374422415));
#58800=DIRECTION('center_axis',(-0.732853934732519,-0.584827952229878,0.34770875260435));
#58801=DIRECTION('ref_axis',(0.41419687010375,0.021958892191509,0.909922392212643));
#58802=DIRECTION('center_axis',(-0.786970057358417,-0.584827952228838,0.196607210226671));
#58803=DIRECTION('ref_axis',(0.278699481110547,-0.0526562713830886,0.95893373927125));
#58804=DIRECTION('center_axis',(0.790515985532476,-0.572651970032463,-0.217150173464257));
#58805=DIRECTION('ref_axis',(0.586650501972613,0.809840224078356,9.70824530985733E-17));
#58806=DIRECTION('center_axis',(0.715054632080185,-0.398672303280797,-0.574244954472788));
#58807=DIRECTION('ref_axis',(-0.626157514223935,-2.26629648864061E-16,-0.779696586744422));
#58808=DIRECTION('center_axis',(-0.663866867041266,-0.584827952229466,0.4661084092096));
#58809=DIRECTION('ref_axis',(0.590433792322176,-0.0273514773905273,0.806622485161807));
#58810=DIRECTION('center_axis',(-0.683495700249331,-0.584827952229789,0.436817918624441));
#58811=DIRECTION('ref_axis',(0.560823821147073,-0.0376838387877329,0.827077124534475));
#58812=DIRECTION('center_axis',(-0.663866867041324,-0.584827952229674,0.466108409209256));
#58813=DIRECTION('ref_axis',(0.573166168880506,0.00246180523643346,0.819435465650481));
#58814=DIRECTION('center_axis',(-0.683495700253782,-0.584827952229443,0.436817918617939));
#58815=DIRECTION('ref_axis',(0.543253576549997,-0.00784651557252715,0.839532002820028));
#58816=DIRECTION('center_axis',(-0.663866867043481,-0.584827952229547,0.466108409206343));
#58817=DIRECTION('ref_axis',(0.555116880732246,0.0322834340855692,0.831145612158149));
#58818=DIRECTION('center_axis',(-0.683495700251026,-0.584827952229332,0.4368179186224));
#58819=DIRECTION('ref_axis',(0.524974319790862,0.0219588922038162,0.850834749298183));
#58820=DIRECTION('center_axis',(-0.768171927774257,-0.584827952229491,0.260553556242555));
#58821=DIRECTION('ref_axis',(0.323436684567506,-0.00326197171076301,0.946244191853529));
#58822=DIRECTION('center_axis',(-0.756123145994201,-0.58482795222951,0.293690405670444));
#58823=DIRECTION('ref_axis',(0.357314215292318,0.0070462672613232,0.93395765517914));
#58824=DIRECTION('center_axis',(-0.768171927771648,-0.584827952229115,0.260553556251089));
#58825=DIRECTION('ref_axis',(0.302913090937847,0.0265489589946694,0.952648315022275));
#58826=DIRECTION('center_axis',(-0.756123145985551,-0.584827952228401,0.293690405694923));
#58827=DIRECTION('ref_axis',(0.336899225382093,0.036885877413158,0.94081791223616));
#58828=DIRECTION('center_axis',(-0.756123145993946,-0.584827952229542,0.293690405671039));
#58829=DIRECTION('ref_axis',(0.396688118786568,-0.0526562713743675,0.916441953152802));
#58830=DIRECTION('center_axis',(-0.768171927778807,-0.584827952229177,0.260553556229844));
#58831=DIRECTION('ref_axis',(0.343535615169486,-0.033086909467639,0.93855662457414));
#58832=DIRECTION('center_axis',(-0.756123145992398,-0.584827952229551,0.293690405675006));
#58833=DIRECTION('ref_axis',(0.377217514059134,-0.0227607290356258,0.925844963425742));
#58834=DIRECTION('center_axis',(0.757066397461466,-0.572651970032553,-0.31451580413797));
#58835=DIRECTION('ref_axis',(0.603266389976478,0.797539756203255,-8.73256628124952E-19));
#58836=DIRECTION('center_axis',(0.637444235727302,-0.398672303282526,-0.659336970701205));
#58837=DIRECTION('ref_axis',(-0.7189419696157,-2.63290852888377E-16,-0.695070100295717));
#58838=DIRECTION('center_axis',(-0.600213204385386,-0.584827952229503,0.545637586290088));
#58839=DIRECTION('ref_axis',(0.686874649850214,-0.0273514773867845,0.726261049539286));
#58840=DIRECTION('center_axis',(-0.623358330286889,-0.584827952229631,0.519038205099431));
#58841=DIRECTION('ref_axis',(0.66006180822835,-0.037683838791864,0.750265511410614));
#58842=DIRECTION('center_axis',(-0.600213204401377,-0.584827952229736,0.545637586272247));
#58843=DIRECTION('ref_axis',(0.671349079039191,0.00246180522602489,0.741137202944407));
#58844=DIRECTION('center_axis',(-0.623358330292484,-0.584827952229444,0.519038205092922));
#58845=DIRECTION('ref_axis',(0.644191120426613,-0.00784651557700974,0.764824314831063));
#58846=DIRECTION('center_axis',(-0.60021320438963,-0.584827952229362,0.54563758628557));
#58847=DIRECTION('ref_axis',(0.654909785459053,0.0322834340879301,0.755017187084815));
#58848=DIRECTION('center_axis',(-0.623358330277944,-0.584827952229089,0.519038205110784));
#58849=DIRECTION('ref_axis',(0.627472610842218,0.0219588922095925,0.778328934124755));
#58850=DIRECTION('center_axis',(-0.713351720932154,-0.58482795222982,0.386141927966661));
#58851=DIRECTION('ref_axis',(0.508420747851833,-0.0526562713708326,0.85949732997788));
#58852=DIRECTION('center_axis',(-0.729458642968396,-0.584827952230075,0.354776485253861));
#58853=DIRECTION('ref_axis',(0.419923024492709,0.0265489589792049,0.907171321348959));
#58854=DIRECTION('center_axis',(-0.713351720928075,-0.584827952228853,0.38614192797566));
#58855=DIRECTION('ref_axis',(0.452158425492064,0.0368858774076047,0.891174612690694));
#58856=DIRECTION('center_axis',(-0.713351720932402,-0.584827952229603,0.386141927966532));
#58857=DIRECTION('ref_axis',(0.490282184337812,-0.0227607290347429,0.871266508557945));
#58858=DIRECTION('center_axis',(-0.729458642960928,-0.584827952229548,0.354776485270086));
#58859=DIRECTION('ref_axis',(0.458459070886996,-0.0330869094602276,0.888099395756918));
#58860=DIRECTION('center_axis',(-0.729458642954225,-0.584827952229394,0.354776485284121));
#58861=DIRECTION('ref_axis',(0.439482134022233,-0.00326197170103793,0.898245408235347));
#58862=DIRECTION('center_axis',(-0.713351720929657,-0.584827952229258,0.386141927972125));
#58863=DIRECTION('ref_axis',(0.471552618924881,0.00704626726875167,0.881809774102478));
#58864=DIRECTION('center_axis',(0.711677420049753,-0.572651970035769,-0.406921332698939));
#58865=DIRECTION('ref_axis',(0.626902064777995,0.779098069036939,-3.10242901956412E-17));
#58866=DIRECTION('center_axis',(0.549780962987417,-0.39867230327996,-0.734030849034344));
#58867=DIRECTION('ref_axis',(-0.800388280671653,2.40386410672042E-16,-0.599481943150479));
#58868=DIRECTION('center_axis',(-0.527093820965332,-0.584827952229272,0.616561732668744));
#58869=DIRECTION('ref_axis',(0.772483083816642,-0.0273514773988447,0.634446043333262));
#58870=DIRECTION('center_axis',(-0.553390227092773,-0.584827952228929,0.593072949012115));
#58871=DIRECTION('ref_axis',(0.748890226283988,-0.037683838805149,0.661621762995463));
#58872=DIRECTION('center_axis',(-0.527093820963167,-0.584827952229652,0.616561732670234));
#58873=DIRECTION('ref_axis',(0.758944413191785,0.00246180522996503,0.651150763802045));
#58874=DIRECTION('center_axis',(-0.553390227069166,-0.584827952229485,0.593072949033594));
#58875=DIRECTION('ref_axis',(0.734969385527659,-0.00784651556621632,0.678054890499703));
#58876=DIRECTION('center_axis',(-0.527093820963804,-0.584827952229951,0.616561732669406));
#58877=DIRECTION('ref_axis',(0.74437437163618,0.0322834340803733,0.666981689954995));
#58878=DIRECTION('center_axis',(-0.553390227069857,-0.584827952229117,0.593072949033312));
#58879=DIRECTION('ref_axis',(0.720075283975828,0.0219588922066651,0.693548406717359));
#58880=DIRECTION('center_axis',(-0.659330313116227,-0.584827952228385,0.47250376135901));
#58881=DIRECTION('ref_axis',(0.612135277983495,-0.0526562713886202,0.788997920486181));
#58882=DIRECTION('center_axis',(-0.659330313105025,-0.584827952229428,0.47250376137335));
#58883=DIRECTION('ref_axis',(0.595614811680486,-0.0227607290416661,0.802947660386598));
#58884=DIRECTION('center_axis',(-0.679241359589837,-0.584827952229611,0.443404377192501));
#58885=DIRECTION('ref_axis',(0.566152353175322,-0.0330869094578101,0.823636308947448));
#58886=DIRECTION('center_axis',(-0.659330313103211,-0.584827952229385,0.472503761375935));
#58887=DIRECTION('ref_axis',(0.57835435604605,0.00704626726010693,0.815755226131134));
#58888=DIRECTION('center_axis',(-0.679241359601283,-0.58482795222964,0.443404377174929));
#58889=DIRECTION('ref_axis',(0.548596687653687,-0.0032619717215567,0.836080757962944));
#58890=DIRECTION('center_axis',(-0.679241359595714,-0.584827952229845,0.443404377183191));
#58891=DIRECTION('ref_axis',(0.530310521127004,0.0265489589845896,0.84738769400956));
#58892=DIRECTION('center_axis',(-0.65933031310547,-0.584827952230006,0.472503761372014));
#58893=DIRECTION('ref_axis',(0.560286817117969,0.0368858773936832,0.827476957149088));
#58894=DIRECTION('center_axis',(0.65506486458811,-0.572651970038989,-0.492909468759352));
#58895=DIRECTION('ref_axis',(0.658159678661854,0.752878368253282,-3.22303153492065E-17));
#58896=DIRECTION('center_axis',(0.453447316037979,-0.398672303276905,-0.797148622389728));
#58897=DIRECTION('ref_axis',(-0.869211990412565,-4.27068266829703E-16,-0.494439597648718));
#58898=DIRECTION('center_axis',(-0.445661853072599,-0.584827952229858,0.677762332242305));
#58899=DIRECTION('ref_axis',(0.845908998121008,-0.0273514773765865,0.532625443987828));
#58900=DIRECTION('center_axis',(-0.474694829399016,-0.584827952229825,0.657754578267995));
#58901=DIRECTION('ref_axis',(0.825908198133754,-0.0376838387877635,0.562543844113215));
#58902=DIRECTION('center_axis',(-0.445661853116207,-0.5848279522299,0.677762332213594));
#58903=DIRECTION('ref_axis',(0.834570740565636,0.0024618052198936,0.550895288150829));
#58904=DIRECTION('center_axis',(-0.47469482939812,-0.584827952229606,0.657754578268837));
#58905=DIRECTION('ref_axis',(0.814156744357949,-0.00784651556705881,0.580592135504711));
#58906=DIRECTION('center_axis',(-0.445661853115868,-0.584827952230675,0.677762332213148));
#58907=DIRECTION('ref_axis',(0.822099729305151,0.0322834340707679,0.568427493143141));
#58908=DIRECTION('center_axis',(-0.474694829418479,-0.584827952230029,0.657754578253768));
#58909=DIRECTION('ref_axis',(0.801321939720788,0.0219588921910951,0.597830206643871));
#58910=DIRECTION('center_axis',(-0.594910872368468,-0.584827952229229,0.55141392821469));
#58911=DIRECTION('ref_axis',(0.706196069142412,-0.0526562713766156,0.706055542441611));
#58912=DIRECTION('center_axis',(-0.594910872346582,-0.584827952229776,0.551413928237722));
#58913=DIRECTION('ref_axis',(0.691554237667827,-0.0227607290218153,0.721965847930541));
#58914=DIRECTION('center_axis',(-0.618312034235857,-0.584827952229107,0.52503951718954));
#58915=DIRECTION('ref_axis',(0.664917074636038,-0.0330869094734788,0.746183985541735));
#58916=DIRECTION('center_axis',(-0.594910872357871,-0.584827952229404,0.551413928225937));
#58917=DIRECTION('ref_axis',(0.676035099498984,0.00704626726817664,0.736835730921746));
#58918=DIRECTION('center_axis',(-0.618312034234228,-0.584827952229657,0.525039517190846));
#58919=DIRECTION('ref_axis',(0.649059543819316,-0.00326197170423922,0.760730614684109));
#58920=DIRECTION('center_axis',(-0.618312034217777,-0.584827952229191,0.525039517210739));
#58921=DIRECTION('ref_axis',(0.632334704053358,0.0265489589935709,0.774240256526428));
#58922=DIRECTION('center_axis',(-0.594910872361907,-0.584827952229308,0.551413928221684));
#58923=DIRECTION('ref_axis',(0.659579150962401,0.0368858774011951,0.750729495666757));
#58924=DIRECTION('center_axis',(0.588121544899005,-0.57265197003845,-0.571124128046338));
#58925=DIRECTION('ref_axis',(0.697621253169909,0.716466738324708,1.05871245547361E-16));
#58926=DIRECTION('center_axis',(0.349962534037925,-0.398672303273708,-0.847694885776829));
#58927=DIRECTION('ref_axis',(2.03396851858332E-16,0.904918591666238,-0.425584706558861));
#58928=DIRECTION('center_axis',(-0.357201531544164,-0.584827952230252,0.728274214944257));
#58929=DIRECTION('ref_axis',(0.905994422190039,-0.0273514773660029,0.422405023225855));
#58930=DIRECTION('center_axis',(-0.388513210696198,-0.58482795222995,0.712063024882668));
#58931=DIRECTION('ref_axis',(0.889901104310132,-0.0376838387861378,0.454594272777328));
#58932=DIRECTION('center_axis',(-0.357201531572555,-0.584827952229513,0.728274214930926));
#58933=DIRECTION('ref_axis',(0.897035388835196,0.0024618052425906,0.441951864677859));
#58934=DIRECTION('center_axis',(-0.388513210688937,-0.584827952229398,0.712063024887083));
#58935=DIRECTION('ref_axis',(0.880504364980544,-0.00784651556111698,0.473973095696115));
#58936=DIRECTION('center_axis',(-0.357201531589311,-0.584827952229665,0.728274214922585));
#58937=DIRECTION('ref_axis',(0.886860083159802,0.0322834340828434,0.460908855178124));
#58938=DIRECTION('center_axis',(-0.38851321069286,-0.5848279522291,0.712063024885188));
#58939=DIRECTION('ref_axis',(0.869931269815895,0.0219588922094773,0.492683867048067));
#58940=DIRECTION('center_axis',(-0.5211093317958,-0.584827952229009,0.621627968005751));
#58941=DIRECTION('ref_axis',(0.789119726415041,-0.0526562713785744,0.611978246727085));
#58942=DIRECTION('center_axis',(-0.521109331771439,-0.584827952229721,0.621627968025504));
#58943=DIRECTION('ref_axis',(0.776587440188631,-0.0227607290239678,0.629598202789341));
#58944=DIRECTION('center_axis',(-0.547631558727778,-0.584827952229038,0.598394470376335));
#58945=DIRECTION('ref_axis',(0.753195656642439,-0.0330869094743024,0.656963894926049));
#58946=DIRECTION('center_axis',(-0.521109331759202,-0.584827952228686,0.621627968036734));
#58947=DIRECTION('ref_axis',(0.763054365594531,0.00704626728573874,0.646295896060361));
#58948=DIRECTION('center_axis',(-0.547631558700224,-0.584827952229441,0.598394470401158));
#58949=DIRECTION('ref_axis',(0.739286343288302,-0.00326197170241592,0.673383295135856));
#58950=DIRECTION('center_axis',(-0.547631558691036,-0.584827952228464,0.59839447041052));
#58951=DIRECTION('ref_axis',(0.724386590960141,0.026548959005902,0.688882587683016));
#58952=DIRECTION('center_axis',(-0.52110933176397,-0.584827952227933,0.621627968033447));
#58953=DIRECTION('ref_axis',(0.748469527589275,0.036885877418764,0.662142581561808));
#58954=DIRECTION('center_axis',(0.511903197111928,-0.572651970045343,-0.640331818661055));
#58955=DIRECTION('ref_axis',(2.78623697967282E-17,0.745401236176701,-0.666616079243702));
#58956=DIRECTION('center_axis',(0.240958633818126,-0.398672303272877,-0.884872494425949));
#58957=DIRECTION('ref_axis',(2.16461393462878E-16,0.91173645657313,-0.41077564893196));
#58958=DIRECTION('center_axis',(-0.263107928487425,-0.584827952230399,0.767300778220024));
#58959=DIRECTION('ref_axis',(0.951791773000886,-0.0273514773604094,0.305523022919768));
#58960=DIRECTION('center_axis',(-0.296204506617227,-0.584827952228624,0.755141812212593));
#58961=DIRECTION('ref_axis',(0.939859738456232,-0.0376838388117045,0.339475478232811));
#58962=DIRECTION('center_axis',(-0.263107928520809,-0.584827952229402,0.767300778209336));
#58963=DIRECTION('ref_axis',(0.945353253144115,0.00246180524621462,0.326038596311492));
#58964=DIRECTION('center_axis',(-0.296204506602731,-0.584827952229629,0.755141812217501));
#58965=DIRECTION('ref_axis',(0.932965905764073,-0.00784651558281844,0.359879217064603));
#58966=DIRECTION('center_axis',(-0.263107928561358,-0.584827952230673,0.767300778194463));
#58967=DIRECTION('ref_axis',(0.937634123704886,0.0322834340717656,0.346121409260833));
#58968=DIRECTION('center_axis',(-0.29620450658635,-0.584827952229493,0.755141812224032));
#58969=DIRECTION('ref_axis',(0.924821264095292,0.0219588922008965,0.379767608585166));
#58970=DIRECTION('center_axis',(-0.439089585745395,-0.584827952229949,0.682038563411529));
#58971=DIRECTION('ref_axis',(0.859598494215755,-0.0526562713668447,0.508249688467931));
#58972=DIRECTION('center_axis',(-0.439089585734235,-0.584827952229727,0.682038563418904));
#58973=DIRECTION('ref_axis',(0.849373394870101,-0.0227607290228192,0.52730141788278));
#58974=DIRECTION('center_axis',(-0.468314606414701,-0.584827952228701,0.662312385291585));
#58975=DIRECTION('ref_axis',(0.829595893198059,-0.0330869094862335,0.557383091248349));
#58976=DIRECTION('center_axis',(-0.439089585749168,-0.584827952229422,0.682038563409552));
#58977=DIRECTION('ref_axis',(0.838039808487152,0.00704626726651889,0.545563588877068));
#58978=DIRECTION('center_axis',(-0.468314606376331,-0.58482795222944,0.662312385318063));
#58979=DIRECTION('ref_axis',(0.817854155460095,-0.00326197170855117,0.575416318796424));
#58980=DIRECTION('center_axis',(-0.468314606377336,-0.584827952229433,0.662312385317358));
#58981=DIRECTION('ref_axis',(0.805014468575665,0.0265489589911354,0.592660828940404));
#58982=DIRECTION('center_axis',(-0.439089585747537,-0.584827952229093,0.682038563410884));
#58983=DIRECTION('ref_axis',(0.825556092624422,0.036885877404233,0.563113283433109));
#58984=DIRECTION('center_axis',(0.427611830115045,-0.57265197004781,-0.699441093978631));
#58985=DIRECTION('ref_axis',(2.4296297475095E-16,0.773750158489481,-0.633490877785547));
#58986=DIRECTION('center_axis',(0.128154672001504,-0.398672303267734,-0.908095135242661));
#58987=DIRECTION('ref_axis',(1.3304126858695E-16,0.915645369915158,-0.401987010428115));
#58988=DIRECTION('center_axis',(-0.16486495623335,-0.584827952230397,0.794226549856007));
#58989=DIRECTION('ref_axis',(0.982578798975358,-0.0273514773601188,0.18382274203798));
#58990=DIRECTION('center_axis',(-0.199224480487903,-0.584827952228576,0.786311562083666));
#58991=DIRECTION('ref_axis',(0.974996223098389,-0.0376838388125904,0.219002952574214));
#58992=DIRECTION('center_axis',(-0.164864956274359,-0.5848279522295,0.794226549848155));
#58993=DIRECTION('ref_axis',(0.97876233192126,0.00246180524259714,0.204983504524156));
#58994=DIRECTION('center_axis',(-0.19922448045893,-0.584827952229542,0.786311562090289));
#58995=DIRECTION('ref_axis',(0.970714016903537,-0.00784651557515089,0.240109828162715));
#58996=DIRECTION('center_axis',(-0.164864956292685,-0.58482795222969,0.794226549844211));
#58997=DIRECTION('ref_axis',(0.973621114013237,0.0322834340827729,0.225875421928651));
#58998=DIRECTION('center_axis',(-0.199224480444615,-0.584827952229133,0.78631156209422));
#58999=DIRECTION('ref_axis',(0.965126274586139,0.0219588922067689,0.260862188054405));
#59000=DIRECTION('center_axis',(-0.350145134677076,-0.584827952228389,0.731693003215366));
#59001=DIRECTION('ref_axis',(0.916520880240436,-0.0526562713881566,0.396505729046623));
#59002=DIRECTION('center_axis',(-0.350145134629644,-0.584827952229829,0.731693003236914));
#59003=DIRECTION('ref_axis',(0.908764223723316,-0.0227607290213395,0.416688774620791));
#59004=DIRECTION('center_axis',(-0.381612052959433,-0.584827952229268,0.715785238271514));
#59005=DIRECTION('ref_axis',(0.892912906963496,-0.0330869094685037,0.449012023224125));
#59006=DIRECTION('center_axis',(-0.350145134628676,-0.584827952228926,0.731693003238098));
#59007=DIRECTION('ref_axis',(0.899808863003385,0.00704626727932487,0.436227417957633));
#59008=DIRECTION('center_axis',(-0.381612052930085,-0.584827952229394,0.715785238287057));
#59009=DIRECTION('ref_axis',(0.883523919049835,-0.00326197169889307,0.468374683354531));
#59010=DIRECTION('center_axis',(-0.381612052925238,-0.584827952228613,0.71578523829028));
#59011=DIRECTION('ref_axis',(0.87294678715174,0.0265489590050242,0.487092454855548));
#59012=DIRECTION('center_axis',(-0.350145134606279,-0.584827952227175,0.731693003250216));
#59013=DIRECTION('ref_axis',(0.889623144943821,0.0368858774309471,0.455203352389253));
#59014=DIRECTION('center_axis',(0.336576769114371,-0.572651970050439,-0.747519765417533));
#59015=DIRECTION('ref_axis',(1.19211448397068E-16,0.793835266537866,-0.608132855222241));
#59016=DIRECTION('center_axis',(0.0133296344508691,-0.398672303267143,-0.916996573304981));
#59017=DIRECTION('ref_axis',(5.21908896690381E-18,0.917078049750596,-0.398707725866508));
#59018=DIRECTION('center_axis',(-0.06402196519388,-0.584827952229365,0.808626894348636));
#59019=DIRECTION('ref_axis',(0.997869970321849,-0.0273514773948857,0.0592234667525383));
#59020=DIRECTION('center_axis',(-0.0991025652750874,-0.584827952228812,
0.805080708902996));
#59021=DIRECTION('ref_axis',(0.994756434869629,-0.0376838388044832,0.095076619515121));
#59022=DIRECTION('center_axis',(-0.0640219651807408,-0.584827952229592,
0.808626894349513));
#59023=DIRECTION('ref_axis',(0.996735744040993,0.00246180523994048,0.080695700418357));
#59024=DIRECTION('center_axis',(-0.0991025652440291,-0.584827952229419,
0.805080708906379));
#59025=DIRECTION('ref_axis',(0.993153388117747,-0.00784651556606208,0.116553763833314));
#59026=DIRECTION('center_axis',(-0.0640219652106609,-0.584827952230345,
0.808626894346599));
#59027=DIRECTION('ref_axis',(0.994253517734721,0.0322834340735004,0.102067244288046));
#59028=DIRECTION('center_axis',(-0.0991025652547514,-0.584827952229472,
0.80508070890502));
#59029=DIRECTION('ref_axis',(0.990210667184292,0.0219588922006542,0.137842815002304));
#59030=DIRECTION('center_axis',(-0.25567868561861,-0.584827952229395,0.769808207290305));
#59031=DIRECTION('ref_axis',(0.95898918450145,-0.0526562713766554,0.278508637377643));
#59032=DIRECTION('center_axis',(-0.255678685641103,-0.584827952229286,0.769808207282917));
#59033=DIRECTION('ref_axis',(0.953823297883429,-0.0227607290544355,0.299504700510177));
#59034=DIRECTION('center_axis',(-0.288891249511358,-0.584827952228646,0.757969730429794));
#59035=DIRECTION('ref_axis',(0.942148150765216,-0.0330869094820139,0.333559767404004));
#59036=DIRECTION('center_axis',(-0.255678685610651,-0.584827952229358,0.769808207292976));
#59037=DIRECTION('ref_axis',(0.947387394214282,0.00704626726439204,0.320011680101699));
#59038=DIRECTION('center_axis',(-0.288891249468051,-0.584827952229451,0.757969730445679));
#59039=DIRECTION('ref_axis',(0.935259982633899,-0.00326197170485859,0.353946499381242));
#59040=DIRECTION('center_axis',(-0.288891249461548,-0.584827952228912,0.757969730448573));
#59041=DIRECTION('ref_axis',(0.9271122134078,0.0265489589997462,0.373842341804832));
#59042=DIRECTION('center_axis',(-0.255678685595091,-0.584827952228579,0.769808207298736));
#59043=DIRECTION('ref_axis',(0.939660308803962,0.0368858774105686,0.34011459260975));
#59044=DIRECTION('center_axis',(0.240233691412443,-0.572651970044448,-0.783809603612104));
#59045=DIRECTION('ref_axis',(1.40955751182557E-16,0.807455881609291,-0.589927961071995));
#59046=DIRECTION('center_axis',(-0.101705619397937,-0.398672303265427,-0.911436427619569));
#59047=DIRECTION('ref_axis',(-2.04923865621488E-17,0.916187281044667,-0.400750378729677));
#59048=DIRECTION('center_axis',(0.0378306905445431,-0.584827952229437,0.810274709678173));
#59049=DIRECTION('ref_axis',(0.997424136147349,-0.0273514773922417,-0.0663097980329947));
#59050=DIRECTION('center_axis',(0.00258225663246541,-0.584827952230405,
0.811153252006472));
#59051=DIRECTION('ref_axis',(0.99882874342139,-0.0376838387736332,-0.030349128661775));
#59052=DIRECTION('center_axis',(0.0378306905688722,-0.584827952229421,0.810274709677048));
#59053=DIRECTION('ref_axis',(0.998990038056263,0.00246180524922385,-0.044864723104699));
#59054=DIRECTION('center_axis',(0.00258225662327451,-0.584827952229373,
0.811153252007245));
#59055=DIRECTION('ref_axis',(0.999930137117185,-0.0078465155589794,-0.00884042297572202));
#59056=DIRECTION('center_axis',(0.0378306905186115,-0.584827952230635,0.810274709678518));
#59057=DIRECTION('ref_axis',(0.999205949546035,0.0322834340709376,-0.02335059477601));
#59058=DIRECTION('center_axis',(0.00258225662696415,-0.584827952228561,
0.811153252007819));
#59059=DIRECTION('ref_axis',(0.999678846039727,0.0219588922164569,0.0126495783845262));
#59060=DIRECTION('center_axis',(-0.157180030979881,-0.584827952228931,0.795783076065883));
#59061=DIRECTION('ref_axis',(0.986333656442174,-0.0526562713819141,0.156119298145892));
#59062=DIRECTION('center_axis',(-0.157180030981607,-0.584827952229301,0.79578307606527));
#59063=DIRECTION('ref_axis',(0.983840008871071,-0.0227607290469234,0.177597258306043));
#59064=DIRECTION('center_axis',(-0.191614458434911,-0.584827952229383,0.788200587166669));
#59065=DIRECTION('ref_axis',(0.976525155431572,-0.0330869094653137,0.2128470747541));
#59066=DIRECTION('center_axis',(-0.157180030964318,-0.584827952229441,0.795783076068582));
#59067=DIRECTION('ref_axis',(0.980025060285253,0.00704626726332402,0.198749166867535));
#59068=DIRECTION('center_axis',(-0.19161445842515,-0.584827952229539,0.788200587168926));
#59069=DIRECTION('ref_axis',(0.972246437596987,-0.00326197170944447,0.233936367674064));
#59070=DIRECTION('center_axis',(-0.191614458432366,-0.584827952229689,0.788200587167061));
#59071=DIRECTION('ref_axis',(0.966656526227481,0.0265489589867337,0.254696511712548));
#59072=DIRECTION('center_axis',(-0.157180030995559,-0.584827952230838,0.795783076061385));
#59073=DIRECTION('ref_axis',(0.974878468272374,0.0368858773811864,0.219662022545385));
#59074=DIRECTION('center_axis',(0.140101984886909,-0.572651970039226,-0.807738296133681));
#59075=DIRECTION('ref_axis',(-2.73695913613894E-16,0.815784312933643,-0.578356252470209));
#59076=DIRECTION('center_axis',(-0.215136914873053,-0.398672303262503,-0.891502385005377));
#59077=DIRECTION('ref_axis',(-1.40757177117324E-16,0.912878440606828,-0.408231493977676));
#59078=DIRECTION('center_axis',(0.139086733702938,-0.584827952229738,0.799144008798552));
#59079=DIRECTION('ref_axis',(0.98124832751129,-0.0273514773842728,-0.190797317699161));
#59080=DIRECTION('center_axis',(0.104226354693529,-0.584827952228692,0.804433423770602));
#59081=DIRECTION('ref_axis',(0.987148926019581,-0.037683838811534,-0.155296252855032));
#59082=DIRECTION('center_axis',(0.13908673371138,-0.58482795222936,0.799144008797359));
#59083=DIRECTION('ref_axis',(0.985489662402947,0.00246180524800965,-0.169717603128984));
#59084=DIRECTION('center_axis',(0.104226354730604,-0.584827952229458,0.804433423765242));
#59085=DIRECTION('ref_axis',(0.990937390525656,-0.00784651556961726,-0.13409519100855));
#59086=DIRECTION('center_axis',(0.139086733689145,-0.584827952229692,0.799144008800986));
#59087=DIRECTION('ref_axis',(0.98840030663301,0.0322834340858216,-0.1484001810356));
#59088=DIRECTION('center_axis',(0.104226354733429,-0.584827952229202,0.804433423765062));
#59089=DIRECTION('ref_axis',(0.993381492313261,0.0219588922051712,-0.112743149603864));
#59090=DIRECTION('center_axis',(-0.0562025533330101,-0.584827952229683,
0.809207970357241));
#59091=DIRECTION('ref_axis',(0.998123057416868,-0.0526562713724056,0.0312678643012303));
#59092=DIRECTION('center_axis',(-0.0562025533235253,-0.58482795222968,0.809207970357902));
#59093=DIRECTION('ref_axis',(0.998340975199547,-0.0227607290307561,0.052889001234716));
#59094=DIRECTION('center_axis',(-0.0913157929052481,-0.584827952229324,
0.806001049786749));
#59095=DIRECTION('ref_axis',(0.995501775041207,-0.0330869094618318,0.0887776566038487));
#59096=DIRECTION('center_axis',(-0.0562025533135293,-0.584827952229175,
0.809207970358962));
#59097=DIRECTION('ref_axis',(0.997207145718442,0.00704626727498444,0.0743522605276269));
#59098=DIRECTION('center_axis',(-0.0913157929007026,-0.584827952229465,
0.806001049787162));
#59099=DIRECTION('ref_axis',(0.993899985449488,-0.00326197170932218,0.110236919696055));
#59100=DIRECTION('center_axis',(-0.0913157928690418,-0.584827952228333,
0.80600104979157));
#59101=DIRECTION('ref_axis',(0.990956088185965,0.0265489590098869,0.131533965433503));
#59102=DIRECTION('center_axis',(-0.0562025532929524,-0.584827952227329,
0.809207970361725));
#59103=DIRECTION('ref_axis',(0.994722211948922,0.0368858774239052,0.095745251068202));
#59104=DIRECTION('center_axis',(0.037760786365144,-0.572651970035092,-0.818928473206308));
#59105=DIRECTION('ref_axis',(3.16831373149503E-17,0.819512943950104,-0.573060672789744));
#59106=DIRECTION('center_axis',(-0.325175372684327,-0.398672303260341,-0.857508817221551));
#59107=DIRECTION('ref_axis',(-3.37422109478849E-16,0.90678944104826,-0.421583810888634));
#59108=DIRECTION('center_axis',(0.238149295968193,-0.584827952229663,0.775410329516388));
#59109=DIRECTION('ref_axis',(0.949597646582202,-0.0273514773858706,-0.312275849675177));
#59110=DIRECTION('center_axis',(0.204226740955095,-0.584827952228983,0.785027199892154));
#59111=DIRECTION('ref_axis',(0.95990118035779,-0.0376838388049021,-0.277794262432916));
#59112=DIRECTION('center_axis',(0.238149295966526,-0.584827952229582,0.775410329516961));
#59113=DIRECTION('ref_axis',(0.956447526073562,0.00246180524043142,-0.291893935159196));
#59114=DIRECTION('center_axis',(0.204226740979238,-0.584827952229625,0.785027199885395));
#59115=DIRECTION('ref_axis',(0.966316969328394,-0.00784651557037047,-0.257235197788701));
#59116=DIRECTION('center_axis',(0.238149295946062,-0.584827952230011,0.775410329522922));
#59117=DIRECTION('ref_axis',(0.962007000446442,0.0322834340790003,-0.271109407760236));
#59118=DIRECTION('center_axis',(0.204226740987369,-0.584827952229167,0.78502719988362));
#59119=DIRECTION('ref_axis',(0.971417919034731,0.0219588922077158,-0.236357850792486));
#59120=DIRECTION('center_axis',(0.0456612721466382,-0.584827952230221,0.809871171555178));
#59121=DIRECTION('ref_axis',(0.994171461523332,-0.052656271367303,-0.0940766824364801));
#59122=DIRECTION('center_axis',(0.0456612721394024,-0.5848279522294,0.809871171556179));
#59123=DIRECTION('ref_axis',(0.997097507965193,-0.0227607290354471,-0.0726533469523378));
#59124=DIRECTION('center_axis',(0.0104229772374144,-0.584827952229693,0.811090394368182));
#59125=DIRECTION('ref_axis',(0.998778736973264,-0.0330869094538148,-0.0366918382325957));
#59126=DIRECTION('center_axis',(0.0456612721423449,-0.584827952229337,0.809871171556059));
#59127=DIRECTION('ref_axis',(0.998662678758543,0.00704626726621081,-0.0512172253487444));
#59128=DIRECTION('center_axis',(0.010422977223353,-0.584827952229428,0.811090394368554));
#59129=DIRECTION('ref_axis',(0.999879136804397,-0.00326197171151358,-0.0152010303548121));
#59130=DIRECTION('center_axis',(0.0104229772140677,-0.584827952229834,0.81109039436838));
#59131=DIRECTION('ref_axis',(0.999627680658168,0.0265489589835582,0.00629705001267351));
#59132=DIRECTION('center_axis',(0.0456612721716982,-0.584827952227699,0.809871171555587));
#59133=DIRECTION('ref_axis',(0.99887859211368,0.0368858774200037,-0.0296814801509117));
#59134=DIRECTION('center_axis',(-0.065175922335569,-0.572651970056052,-0.817203659034045));
#59135=DIRECTION('ref_axis',(-3.98584692492418E-17,0.818944908553334,-0.573872143211858));
#59136=DIRECTION('center_axis',(-0.430085620617851,-0.398672303259856,-0.809991823138505));
#59137=DIRECTION('ref_axis',(-0.883216234749031,-3.21399618696842E-16,0.468965971767402));
#59138=DIRECTION('center_axis',(0.333456101558182,-0.584827952229417,0.73944796613742));
#59139=DIRECTION('ref_axis',(0.902971243510296,-0.0273514773966886,-0.428829604945471));
#59140=DIRECTION('center_axis',(0.301006349518998,-0.584827952229591,0.753240628113082));
#59141=DIRECTION('ref_axis',(0.917515219660035,-0.0376838387937564,-0.395911290551259));
#59142=DIRECTION('center_axis',(0.333456101576296,-0.58482795222948,0.739447966129201));
#59143=DIRECTION('ref_axis',(0.912321640901148,0.00246180524209912,-0.409466925475535));
#59144=DIRECTION('center_axis',(0.301006349521064,-0.584827952229532,0.753240628112302));
#59145=DIRECTION('ref_axis',(0.926457152276119,-0.00784651557254989,-0.376318451832746));
#59146=DIRECTION('center_axis',(0.333456101560606,-0.584827952229806,0.739447966136019));
#59147=DIRECTION('ref_axis',(0.920442269183709,0.0322834340832547,-0.389543077186254));
#59148=DIRECTION('center_axis',(0.301006349541005,-0.584827952228975,0.753240628104766));
#59149=DIRECTION('ref_axis',(0.934134504873787,0.0219588922130655,-0.356245047484144));
#59150=DIRECTION('center_axis',(0.146804992065436,-0.584827952229486,0.797762220586895));
#59151=DIRECTION('ref_axis',(0.974541187793879,-0.0526562713753265,-0.217937583675104));
#59152=DIRECTION('center_axis',(0.146804992111045,-0.584827952229952,0.79776222057816));
#59153=DIRECTION('ref_axis',(0.980129217387624,-0.0227607290121625,-0.197049908495181));
#59154=DIRECTION('center_axis',(0.111997370786089,-0.584827952229844,0.803388358907229));
#59155=DIRECTION('ref_axis',(0.986304361580666,-0.0330869094541399,-0.161582680847079));
#59156=DIRECTION('center_axis',(0.146804992081053,-0.584827952229384,0.797762220584096));
#59157=DIRECTION('ref_axis',(0.984368704782361,0.00704626726995306,-0.175978985002918));
#59158=DIRECTION('center_axis',(0.111997370781047,-0.584827952229584,0.803388358908122));
#59159=DIRECTION('ref_axis',(0.990089596872588,-0.00326197170726883,-0.140399251085102));
#59160=DIRECTION('center_axis',(0.111997370753232,-0.584827952230296,0.80338835891148));
#59161=DIRECTION('ref_axis',(0.992534547463153,0.0265489589767518,-0.119039173675579));
#59162=DIRECTION('center_axis',(0.146804992125695,-0.584827952226961,0.797762220577657));
#59163=DIRECTION('ref_axis',(0.98728206017675,0.0368858774329538,-0.154640116719929));
#59164=DIRECTION('center_axis',(-0.167084767789042,-0.572651970057299,-0.802591054997734));
#59165=DIRECTION('ref_axis',(1.04024676683625E-16,0.814034314690017,-0.580816782218932));
#59166=DIRECTION('center_axis',(-0.528213161393386,-0.398672303260503,-0.749700774138436));
#59167=DIRECTION('ref_axis',(-0.817474789260881,-2.1562309484241E-16,0.57596438164428));
#59168=DIRECTION('center_axis',(0.423504105275545,-0.584827952229947,0.691824066584335));
#59169=DIRECTION('ref_axis',(0.842104444500713,-0.0273514773774933,-0.538620461213101));
#59170=DIRECTION('center_axis',(0.393038908107982,-0.584827952229038,0.709575001676973));
#59171=DIRECTION('ref_axis',(0.86065949586068,-0.0376838388021038,-0.507784561086665));
#59172=DIRECTION('center_axis',(0.423504105240179,-0.584827952229838,0.691824066606078));
#59173=DIRECTION('ref_axis',(0.853807898469918,0.00246180522579648,-0.520582377751507));
#59174=DIRECTION('center_axis',(0.393038908152261,-0.584827952229443,0.709575001652113));
#59175=DIRECTION('ref_axis',(0.871986552479397,-0.00784651555265927,-0.489466939117218));
#59176=DIRECTION('center_axis',(0.423504105258982,-0.584827952229269,0.691824066595048));
#59177=DIRECTION('ref_axis',(0.864361613487515,0.0322834340894379,-0.501833419585277));
#59178=DIRECTION('center_axis',(0.39303890813514,-0.584827952229147,0.70957500166184));
#59179=DIRECTION('ref_axis',(0.88211923155067,0.0219588922095178,-0.470514046954377));
#59180=DIRECTION('center_axis',(0.24563350955146,-0.584827952228278,0.773072082847332));
#59181=DIRECTION('ref_axis',(0.93954181737605,-0.0526562713904792,-0.338361479020532));
#59182=DIRECTION('center_axis',(0.245633509623877,-0.584827952230061,0.773072082822973));
#59183=DIRECTION('ref_axis',(0.947703703551881,-0.0227607290100421,-0.31833887523986));
#59184=DIRECTION('center_axis',(0.211805498867834,-0.584827952229117,0.783016409113402));
#59185=DIRECTION('ref_axis',(0.958275377222213,-0.0330869094709953,-0.283925268039469));
#59186=DIRECTION('center_axis',(0.245633509610189,-0.584827952228881,0.773072082828215));
#59187=DIRECTION('ref_axis',(0.954550648293822,0.00704626728150651,-0.297965450949));
#59188=DIRECTION('center_axis',(0.211805498906855,-0.584827952229244,0.783016409102751));
#59189=DIRECTION('ref_axis',(0.964685752543678,-0.00326197169741844,-0.26338329176294));
#59190=DIRECTION('center_axis',(0.211805498865265,-0.584827952230204,0.783016409113284));
#59191=DIRECTION('ref_axis',(0.969788551542686,0.0265489589781888,-0.242498078495303));
#59192=DIRECTION('center_axis',(0.245633509565711,-0.584827952229986,0.773072082841512));
#59193=DIRECTION('ref_axis',(0.960115500395768,0.0368858773910101,-0.277159986197286));
#59194=DIRECTION('center_axis',(-0.266358586643225,-0.572651970059613,-0.775321110578235));
#59195=DIRECTION('ref_axis',(-2.48492576229079E-16,0.804380141111197,-0.594114962432299));
#59196=DIRECTION('center_axis',(-0.618010465074973,-0.39867230325935,-0.677586496081276));
#59197=DIRECTION('ref_axis',(-0.738841278010305,-1.09179488801154E-16,0.673879489158187));
#59198=DIRECTION('center_axis',(0.506873196223756,-0.584827952229664,0.633289688247623));
#59199=DIRECTION('ref_axis',(0.767957155370104,-0.0273514773849234,-0.639916951018427));
#59200=DIRECTION('center_axis',(0.478873008347111,-0.584827952229356,0.654718953573062));
#59201=DIRECTION('ref_axis',(0.790230657669329,-0.0376838387963876,-0.611649765775372));
#59202=DIRECTION('center_axis',(0.506873196218676,-0.584827952229412,0.633289688251922));
#59203=DIRECTION('ref_axis',(0.781829095418921,0.00246180523862598,-0.623487934984631));
#59204=DIRECTION('center_axis',(0.478873008373498,-0.584827952229322,0.654718953553793));
#59205=DIRECTION('ref_axis',(0.803764203864772,-0.00784651555737207,-0.594896240347203));
#59206=DIRECTION('center_axis',(0.506873196212247,-0.584827952229583,0.633289688256909));
#59207=DIRECTION('ref_axis',(0.794649458809522,0.0322834340848596,-0.606209549163837));
#59208=DIRECTION('center_axis',(0.478873008348126,-0.584827952229779,0.654718953571943));
#59209=DIRECTION('ref_axis',(0.816192411000741,0.0219588921980096,-0.57736275882519));
#59210=DIRECTION('center_axis',(0.340588239909505,-0.584827952229418,0.736190136531651));
#59211=DIRECTION('ref_axis',(0.889725311229054,-0.0526562713735081,-0.453449211757394));
#59212=DIRECTION('center_axis',(0.340588239911442,-0.584827952229579,0.736190136530627));
#59213=DIRECTION('ref_axis',(0.900332336196276,-0.0227607290358304,-0.434607447719333));
#59214=DIRECTION('center_axis',(0.308273327752867,-0.584827952229647,0.750295822783955));
#59215=DIRECTION('ref_axis',(0.915133817709533,-0.033086909459052,-0.401790184184263));
#59216=DIRECTION('center_axis',(0.340588239920696,-0.58482795222925,0.736190136526607));
#59217=DIRECTION('ref_axis',(0.909678757870439,0.00704626726974534,-0.415252823707268));
#59218=DIRECTION('center_axis',(0.308273327749158,-0.584827952229474,0.750295822785613));
#59219=DIRECTION('ref_axis',(0.924068237631228,-0.0032619717112851,-0.382213620560115));
#59220=DIRECTION('center_axis',(0.308273327756663,-0.584827952229327,0.750295822782644));
#59221=DIRECTION('ref_axis',(0.931748410832705,0.0265489589938174,-0.362132643774451));
#59222=DIRECTION('center_axis',(0.340588239932968,-0.584827952228373,0.736190136521626));
#59223=DIRECTION('ref_axis',(0.917807345604216,0.0368858774140981,-0.39530887721165));
#59224=DIRECTION('center_axis',(-0.361431771470631,-0.572651970061988,-0.735823889090131));
#59225=DIRECTION('ref_axis',(1.05608455141898E-18,0.789173129075047,-0.614170800629515));
#59226=DIRECTION('center_axis',(-0.698061374540006,-0.398672303260801,-0.594786274209522));
#59227=DIRECTION('ref_axis',(-0.648555798443099,3.71019517064062E-16,0.76116711457198));
#59228=DIRECTION('center_axis',(0.582248594100823,-0.58482795222998,0.5647679531968));
#59229=DIRECTION('ref_axis',(0.6816987231266,-0.0273514773733327,-0.731121568258699));
#59230=DIRECTION('center_axis',(0.557154995178035,-0.584827952229649,0.589537596459326));
#59231=DIRECTION('ref_axis',(0.707339409944258,-0.0376838387904544,-0.705868888274391));
#59232=DIRECTION('center_axis',(0.582248594074075,-0.584827952229764,0.5647679532246));
#59233=DIRECTION('ref_axis',(0.697520380507347,0.00246180523187029,-0.716560715007379));
#59234=DIRECTION('center_axis',(0.557154995173542,-0.584827952229435,0.589537596463785));
#59235=DIRECTION('ref_axis',(0.722866013622932,-0.00784651557421879,-0.690943672481508));
#59236=DIRECTION('center_axis',(0.582248594082303,-0.584827952229179,0.564767953216724));
#59237=DIRECTION('ref_axis',(0.712405207457628,0.0322834340894324,-0.70102539202988));
#59238=DIRECTION('center_axis',(0.557154995173226,-0.584827952229562,0.589537596463957));
#59239=DIRECTION('ref_axis',(0.737393748550908,0.0219588921987813,-0.675106115104464));
#59240=DIRECTION('center_axis',(0.430171690230978,-0.584827952229147,0.687698031998992));
#59241=DIRECTION('ref_axis',(0.825877305439295,-0.0526562713786458,-0.561385779517817));
#59242=DIRECTION('center_axis',(0.430171690255798,-0.584827952229872,0.687698031982849));
#59243=DIRECTION('ref_axis',(0.838762190047532,-0.0227607290251598,-0.544022001173584));
#59244=DIRECTION('center_axis',(0.39987950204304,-0.584827952228486,0.705742623155245));
#59245=DIRECTION('ref_axis',(0.857560051241502,-0.0330869094880703,-0.513318629055288));
#59246=DIRECTION('center_axis',(0.430171690277,-0.584827952228745,0.687698031970545));
#59247=DIRECTION('ref_axis',(0.850460690000747,0.00704626728869317,-0.525991411413484));
#59248=DIRECTION('center_axis',(0.39987950209059,-0.584827952229427,0.705742623127523));
#59249=DIRECTION('ref_axis',(0.868877614590822,-0.00326197170616806,-0.495016212263348));
#59250=DIRECTION('center_axis',(0.399879502092047,-0.584827952229158,0.705742623126921));
#59251=DIRECTION('ref_axis',(0.879014041089011,0.0265489589953712,-0.476056160914475));
#59252=DIRECTION('center_axis',(0.430171690237065,-0.584827952229516,0.68769803199487));
#59253=DIRECTION('ref_axis',(0.86102482072266,0.0368858773983956,-0.50722351103637));
#59254=DIRECTION('center_axis',(-0.450804961352599,-0.572651970064768,-0.684722285310491));
#59255=DIRECTION('ref_axis',(3.11886164380238E-16,0.767090570529824,-0.641538819249645));
#59256=DIRECTION('center_axis',(-0.767103439127705,-0.398672303259429,-0.502605917486323));
#59257=DIRECTION('ref_axis',(-0.548042206506147,4.1389735132999E-17,0.83645067988966));
#59258=DIRECTION('center_axis',(0.648441583792624,-0.584827952229372,0.487339490191091));
#59259=DIRECTION('ref_axis',(0.584689494827209,-0.0273514773949,-0.810795961585293));
#59260=DIRECTION('center_axis',(0.62665031490309,-0.58482795222999,0.515058879277248));
#59261=DIRECTION('ref_axis',(0.613292997180565,-0.0376838387864848,-0.788956036736898));
#59262=DIRECTION('center_axis',(0.648441583795839,-0.584827952229595,0.487339490186545));
#59263=DIRECTION('ref_axis',(0.602211352506359,0.0024618052356761,-0.798332904512549));
#59264=DIRECTION('center_axis',(0.62665031489973,-0.584827952229372,0.515058879282038));
#59265=DIRECTION('ref_axis',(0.630567794508368,-0.00784651556989916,-0.776094510174028));
#59266=DIRECTION('center_axis',(0.648441583795029,-0.584827952229575,0.487339490187648));
#59267=DIRECTION('ref_axis',(0.618925900421918,0.0322834340860392,-0.784785645683285));
#59268=DIRECTION('center_axis',(0.626650314909146,-0.584827952228887,0.515058879271132));
#59269=DIRECTION('ref_axis',(0.646965946175702,0.0219588922115843,-0.762202644669919));
#59270=DIRECTION('center_axis',(0.512971076023869,-0.584827952228682,0.628360518695216));
#59271=DIRECTION('ref_axis',(0.74900472119103,-0.0526562713861267,-0.660468958178398));
#59272=DIRECTION('center_axis',(0.512971076037276,-0.584827952229498,0.628360518683511));
#59273=DIRECTION('ref_axis',(0.763964263128389,-0.0227607290396375,-0.644857002657397));
#59274=DIRECTION('center_axis',(0.485179337823022,-0.584827952230446,0.650059440697201));
#59275=DIRECTION('ref_axis',(0.786462050426737,-0.0330869094385312,-0.616751732597793));
#59276=DIRECTION('center_axis',(0.512971076019171,-0.584827952229899,0.628360518697919));
#59277=DIRECTION('ref_axis',(0.777830349057598,0.00704626724669506,-0.628434800279889));
#59278=DIRECTION('center_axis',(0.485179337808214,-0.584827952229516,0.65005944070909));
#59279=DIRECTION('ref_axis',(0.799984272523417,-0.00326197169936234,-0.600012102591116));
#59280=DIRECTION('center_axis',(0.48517933779427,-0.584827952229414,0.650059440719588));
#59281=DIRECTION('ref_axis',(0.812417094824369,0.0265489589910001,-0.582471988007686));
#59282=DIRECTION('center_axis',(0.512971076053233,-0.584827952228724,0.628360518671205));
#59283=DIRECTION('ref_axis',(0.790663420048422,0.0368858774084628,-0.611138927123072));
#59284=DIRECTION('center_axis',(-0.533068687695661,-0.572651970068508,-0.622822202056961));
#59285=DIRECTION('ref_axis',(3.61729072720274E-16,0.736133834918718,-0.676836004574122));
#59286=DIRECTION('center_axis',(-0.824047824234184,-0.398672303260603,-0.402499165201362));
#59287=DIRECTION('ref_axis',(-0.438885661587862,2.2735551145057E-16,0.898542918314192));
#59288=DIRECTION('center_axis',(0.704408262379738,-0.584827952229673,0.402225392264096));
#59289=DIRECTION('ref_axis',(0.478459363886856,-0.027351477387215,-0.877683618278091));
#59290=DIRECTION('center_axis',(0.68626298482074,-0.584827952230173,0.432457375882516));
#59291=DIRECTION('ref_axis',(0.509574587483431,-0.0376838387798185,-0.859600877201686));
#59292=DIRECTION('center_axis',(0.704408262376566,-0.584827952229622,0.402225392269725));
#59293=DIRECTION('ref_axis',(0.49740509173617,0.00246180523631316,-0.867514907209041));
#59294=DIRECTION('center_axis',(0.686262984799087,-0.584827952229561,0.432457375917704));
#59295=DIRECTION('ref_axis',(0.528325144612044,-0.00784651558329287,-0.849005873809989));
#59296=DIRECTION('center_axis',(0.704408262374531,-0.584827952229628,0.402225392273281));
#59297=DIRECTION('ref_axis',(0.515685762206007,0.0322834340851825,-0.856169360898694));
#59298=DIRECTION('center_axis',(0.686262984814354,-0.584827952229256,0.43245737589389));
#59299=DIRECTION('ref_axis',(0.546335104369736,0.0219588922059708,-0.837278783193744));
#59300=DIRECTION('center_axis',(0.587680601530481,-0.584827952229076,0.559113384633491));
#59301=DIRECTION('ref_axis',(0.660319885045023,-0.05265627138097,-0.749136146837396));
#59302=DIRECTION('center_axis',(0.587680601544024,-0.584827952229498,0.559113384618814));
#59303=DIRECTION('ref_axis',(0.677118163392339,-0.0227607290334116,-0.735522224013696));
#59304=DIRECTION('center_axis',(0.56282760551461,-0.584827952229546,0.584124432601211));
#59305=DIRECTION('ref_axis',(0.702961073322399,-0.0330869094577009,-0.710458292805397));
#59306=DIRECTION('center_axis',(0.587680601535344,-0.584827952229505,0.55911338462793));
#59307=DIRECTION('ref_axis',(0.692933158812551,0.00704626725934919,-0.720967396999178));
#59308=DIRECTION('center_axis',(0.562827605520547,-0.584827952229568,0.584124432595469));
#59309=DIRECTION('ref_axis',(0.718474700600097,-0.00326197170431984,-0.695545443618316));
#59310=DIRECTION('center_axis',(0.562827605513519,-0.584827952229463,0.584124432602346));
#59311=DIRECTION('ref_axis',(0.733007845657271,0.0265489589905533,-0.679701883903086));
#59312=DIRECTION('center_axis',(0.58768060156272,-0.584827952227991,0.559113384600739));
#59313=DIRECTION('ref_axis',(0.707832784918237,0.0368858774180847,-0.705416317249602));
#59314=DIRECTION('center_axis',(-0.606925602392853,-0.572651970070417,-0.551099840622861));
#59315=DIRECTION('ref_axis',(0.686271561910537,-0.7273454085322,-1.7200576857839E-16));
#59316=DIRECTION('center_axis',(-0.867996482891093,-0.398672303259356,-0.296044760640299));
#59317=DIRECTION('ref_axis',(0.417381833030164,-0.908731206384143,-2.70851097314861E-16));
#59318=DIRECTION('center_axis',(0.749266001871889,-0.584827952229832,0.310767959625145));
#59319=DIRECTION('ref_axis',(0.364683642961482,-0.0273514773819596,-0.930729680004547));
#59320=DIRECTION('center_axis',(0.73505287750409,-0.5848279522301,0.343035761347566));
#59321=DIRECTION('ref_axis',(0.397819882148946,-0.0376838387832597,-0.916689298323896));
#59322=DIRECTION('center_axis',(0.749266001868941,-0.584827952229526,0.310767959632829));
#59323=DIRECTION('ref_axis',(0.384754455528877,0.00246180524083023,-0.923015681592482));
#59324=DIRECTION('center_axis',(0.735052877494717,-0.584827952229498,0.343035761368678));
#59325=DIRECTION('ref_axis',(0.417750491554942,-0.00784651557676579,-0.908527907661018));
#59326=DIRECTION('center_axis',(0.749266001867358,-0.584827952229307,0.310767959637058));
#59327=DIRECTION('ref_axis',(0.404312951457465,0.0322834340889155,-0.914050773845294));
#59328=DIRECTION('center_axis',(0.735052877499929,-0.584827952229289,0.343035761357865));
#59329=DIRECTION('ref_axis',(0.437088231600138,0.0219588922034376,-0.899150535144067));
#59330=DIRECTION('center_axis',(0.65312205288754,-0.584827952229456,0.481048698494307));
#59331=DIRECTION('ref_axis',(0.561221409852641,-0.0526562713746137,-0.825989010948655));
#59332=DIRECTION('center_axis',(0.653122052890733,-0.584827952229576,0.481048698489826));
#59333=DIRECTION('ref_axis',(0.579593505736634,-0.0227607290348539,-0.814587820509072));
#59334=DIRECTION('center_axis',(0.631599745689671,-0.584827952230062,0.508977433227776));
#59335=DIRECTION('ref_axis',(0.608373980132682,-0.0330869094484406,-0.792960501362249));
#59336=DIRECTION('center_axis',(0.65312205289568,-0.584827952229212,0.481048698483552));
#59337=DIRECTION('ref_axis',(0.597107998714186,0.00704626726938554,-0.802129907177826));
#59338=DIRECTION('center_axis',(0.631599745685247,-0.584827952229501,0.508977433233911));
#59339=DIRECTION('ref_axis',(0.625634353446796,-0.00326197170274169,-0.780109617507578));
#59340=DIRECTION('center_axis',(0.631599745674331,-0.584827952229705,0.508977433247222));
#59341=DIRECTION('ref_axis',(0.642038624889269,0.0265489589877621,-0.766212475053077));
#59342=DIRECTION('center_axis',(0.653122052899692,-0.584827952228688,0.481048698478743));
#59343=DIRECTION('ref_axis',(0.61383920394949,0.0368858774095715,-0.788568870639961));
#59344=DIRECTION('center_axis',(-0.671210937779911,-0.572651970073183,-0.470686305490095));
#59345=DIRECTION('ref_axis',(0.649044045255814,-0.760750831296272,-1.68693210803163E-16));
#59346=DIRECTION('center_axis',(-0.898256318494365,-0.398672303264004,-0.184921553354722));
#59347=DIRECTION('ref_axis',(0.405668756710548,-0.914020163797779,-1.89095079954371E-16));
#59348=DIRECTION('center_axis',(0.782307368915401,-0.584827952229458,0.21440953064582));
#59349=DIRECTION('ref_axis',(0.245156643157,-0.0273514773929348,-0.96909757867844));
#59350=DIRECTION('center_axis',(0.772250547205598,-0.584827952229256,0.248204267956837));
#59351=DIRECTION('ref_axis',(0.279791319643253,-0.037683838798696,-0.95932098160401));
#59352=DIRECTION('center_axis',(0.782307368913366,-0.584827952229746,0.214409530652459));
#59353=DIRECTION('ref_axis',(0.266036011735809,0.00246180523015953,-0.9639599472876));
#59354=DIRECTION('center_axis',(0.772250547211137,-0.584827952229511,0.248204267939002));
#59355=DIRECTION('ref_axis',(0.300587663690744,-0.00784651556811171,-0.953721913678395));
#59356=DIRECTION('center_axis',(0.782307368912528,-0.584827952230018,0.214409530654777));
#59357=DIRECTION('ref_axis',(0.2865638839574,0.0322834340798274,-0.957517060054422));
#59358=DIRECTION('center_axis',(0.77225054720522,-0.584827952229822,0.248204267956682));
#59359=DIRECTION('ref_axis',(0.320948216323777,0.0219588921948035,-0.94684214602655));
#59360=DIRECTION('center_axis',(0.708263379303267,-0.584827952229123,0.395397587030329));
#59361=DIRECTION('ref_axis',(0.45327213778181,-0.052656271378629,-0.889815534925755));
#59362=DIRECTION('center_axis',(0.708263379307223,-0.584827952229426,0.395397587022796));
#59363=DIRECTION('ref_axis',(0.472928312264079,-0.0227607290376266,-0.880806880464001));
#59364=DIRECTION('center_axis',(0.690411180536856,-0.584827952228857,0.425803555740798));
#59365=DIRECTION('ref_axis',(0.504192465897799,-0.0330869094779533,-0.862957249087749));
#59366=DIRECTION('center_axis',(0.70826337931017,-0.584827952229283,0.395397587017728));
#59367=DIRECTION('ref_axis',(0.491866088796126,0.00704626726564717,-0.870642349538559));
#59368=DIRECTION('center_axis',(0.690411180559335,-0.584827952229379,0.425803555703633));
#59369=DIRECTION('ref_axis',(0.522927378805018,-0.00326197170296729,-0.852370996712536));
#59370=DIRECTION('center_axis',(0.690411180556875,-0.584827952229177,0.4258035557079));
#59371=DIRECTION('ref_axis',(0.540944071460083,0.0265489589947329,-0.840639437766563));
#59372=DIRECTION('center_axis',(0.708263379302448,-0.584827952229935,0.395397587030597));
#59373=DIRECTION('ref_axis',(0.510165012055972,0.036885877393939,-0.859285221869205));
#59374=DIRECTION('center_axis',(-0.724910875715219,-0.572651970076974,-0.382849766144314));
#59375=DIRECTION('ref_axis',(0.619880264826496,-0.784696410899548,-6.375267076676E-18));
#59376=DIRECTION('center_axis',(-0.914350115364004,-0.398672303265294,-0.070882022706601));
#59377=DIRECTION('ref_axis',(0.399677609928807,-0.916655774062214,1.06579819070638E-17));
#59378=DIRECTION('center_axis',(0.803011281433564,-0.584827952229893,0.114669735244374));
#59379=DIRECTION('ref_axis',(0.121763376606092,-0.0273514773793618,-0.992182229634581));
#59380=DIRECTION('center_axis',(0.79726936447069,-0.584827952229677,0.149458444951582));
#59381=DIRECTION('ref_axis',(0.157350280855911,-0.0376838387905617,-0.986823599945083));
#59382=DIRECTION('center_axis',(0.803011281429913,-0.584827952229658,0.114669735271145));
#59383=DIRECTION('ref_axis',(0.143122021098843,0.00246180523247351,-0.989701988778228));
#59384=DIRECTION('center_axis',(0.797269364468822,-0.584827952229543,0.149458444962072));
#59385=DIRECTION('ref_axis',(0.178684388830733,-0.00784651557677228,-0.983875155383797));
#59386=DIRECTION('center_axis',(0.803011281429729,-0.584827952229772,0.114669735271848));
#59387=DIRECTION('ref_axis',(0.164295532805841,0.0322834340834813,-0.985882730239161));
#59388=DIRECTION('center_axis',(0.797269364472123,-0.584827952229213,0.149458444945752));
#59389=DIRECTION('ref_axis',(0.199746655922415,0.021958892206408,-0.979601490658768));
#59390=DIRECTION('center_axis',(0.752234969135609,-0.584827952229195,0.303510819413338));
#59391=DIRECTION('ref_axis',(0.338174493321089,-0.0526562713785287,-0.939609136370829));
#59392=DIRECTION('center_axis',(0.752234969141854,-0.584827952229689,0.303510819396908));
#59393=DIRECTION('ref_axis',(0.358804756783703,-0.0227607290319074,-0.933135089750312));
#59394=DIRECTION('center_axis',(0.738334418684743,-0.584827952229868,0.335914501735312));
#59395=DIRECTION('ref_axis',(0.392059535219292,-0.0330869094523403,-0.919344645531003));
#59396=DIRECTION('center_axis',(0.752234969145643,-0.584827952229108,0.303510819388636));
#59397=DIRECTION('ref_axis',(0.378867156817279,0.00704626727295211,-0.925424241957552));
#59398=DIRECTION('center_axis',(0.738334418680268,-0.584827952229459,0.335914501745859));
#59399=DIRECTION('ref_axis',(0.411973527025067,-0.00326197170852844,-0.911189976114256));
#59400=DIRECTION('center_axis',(0.73833441867766,-0.584827952229559,0.335914501751417));
#59401=DIRECTION('ref_axis',(0.43131850689555,0.0265489589884161,-0.901809014362811));
#59402=DIRECTION('center_axis',(0.752234969147248,-0.584827952228465,0.303510819385897));
#59403=DIRECTION('ref_axis',(0.398445213122471,0.0368858774114973,-0.916450131860634));
#59404=DIRECTION('center_axis',(-0.767178536098743,-0.572651970080584,-0.288975457283513));
#59405=DIRECTION('ref_axis',(0.598172081278793,-0.801367681640954,1.80237087757503E-16));
#59406=DIRECTION('center_axis',(-0.916024064707328,-0.398672303268271,0.0442753597821266));
#59407=DIRECTION('ref_axis',(0.399063638865775,-0.916923231320488,-3.58065846580494E-17));
#59408=DIRECTION('center_axis',(0.811051226341725,-0.584827952229574,0.0131215296572828));
#59409=DIRECTION('ref_axis',(-0.00355017109927834,-0.0273514773886332,-0.999619574122989));
#59410=DIRECTION('center_axis',(0.809714767587711,-0.584827952229316,0.0483555730153735));
#59411=DIRECTION('ref_axis',(0.0324277341660284,-0.0376838387987105,-0.998763420610832));
#59412=DIRECTION('center_axis',(0.811051226341597,-0.584827952229581,0.0131215296648961));
#59413=DIRECTION('ref_axis',(0.0179509106930064,0.00246180523465447,-0.99983583868567));
#59414=DIRECTION('center_axis',(0.809714767588841,-0.584827952229489,0.0483555729943428));
#59415=DIRECTION('ref_axis',(0.0539631543924302,-0.00784651556639407,-0.998512098154792));
#59416=DIRECTION('center_axis',(0.811051226341607,-0.584827952229582,0.0131215296642423));
#59417=DIRECTION('ref_axis',(0.0394361429572599,0.0322834340863139,-0.998700440829105));
#59418=DIRECTION('center_axis',(0.809714767588954,-0.584827952229199,0.0483555729959739));
#59419=DIRECTION('ref_axis',(0.0753949714509705,0.0219588922059928,-0.996911934592516));
#59420=DIRECTION('center_axis',(0.784343364141097,-0.584827952229295,0.206837504865814));
#59421=DIRECTION('ref_axis',(0.217743635085388,-0.0526562713782781,-0.974584540439842));
#59422=DIRECTION('center_axis',(0.784343364146169,-0.5848279522297,0.206837504845436));
#59423=DIRECTION('ref_axis',(0.239022635952717,-0.0227607290302773,-0.97074720124048));
#59424=DIRECTION('center_axis',(0.774613681968537,-0.584827952229984,0.240727875406297));
#59425=DIRECTION('ref_axis',(0.273743591493593,-0.033086909449576,-0.961233427705916));
#59426=DIRECTION('center_axis',(0.784343364145265,-0.584827952229309,0.206837504849971));
#59427=DIRECTION('ref_axis',(0.25989326346829,0.00704626726723805,-0.96561164125201));
#59428=DIRECTION('center_axis',(0.774613681964187,-0.584827952229543,0.240727875421367));
#59429=DIRECTION('ref_axis',(0.294522606615922,-0.00326197170818176,-0.955638945278361));
#59430=DIRECTION('center_axis',(0.77461368196608,-0.584827952229136,0.240727875416265));
#59431=DIRECTION('ref_axis',(0.314890791803105,0.0265489589951922,-0.948756524095558));
#59432=DIRECTION('center_axis',(0.784343364146824,-0.584827952228856,0.206837504845337));
#59433=DIRECTION('ref_axis',(0.280441695187659,0.0368858774073383,-0.959162075797497));
#59434=DIRECTION('center_axis',(-0.797347332677702,-0.572651970082362,-0.190543832837863));
#59435=DIRECTION('ref_axis',(0.583339514953269,-0.812228422485993,1.43682251946218E-17));
#59436=DIRECTION('center_axis',(-0.903251767344807,-0.398672303269224,0.158734493398553));
#59437=DIRECTION('ref_axis',(0.403791856799519,-0.914850882047122,-3.65899417434021E-17));
#59438=DIRECTION('center_axis',(0.806300408914237,-0.584827952229579,-0.0886336103049619));
#59439=DIRECTION('ref_axis',(-0.128807730497183,-0.0273514773898677,-0.991292320785729));
#59440=DIRECTION('center_axis',(0.809390485122122,-0.584827952229272,-0.0535098952072579));
#59441=DIRECTION('ref_axis',(-0.0930062172741409,-0.0376838387986781,-0.994952145503366));
#59442=DIRECTION('center_axis',(0.806300408914354,-0.584827952229474,-0.0886336103045866));
#59443=DIRECTION('ref_axis',(-0.107503296299766,0.0024618052375083,-0.994201680143248));
#59444=DIRECTION('center_axis',(0.809390485121829,-0.584827952229487,-0.0535098952093429));
#59445=DIRECTION('ref_axis',(-0.0716091111974473,-0.00784651557791117,-0.997401908654078));
#59446=DIRECTION('center_axis',(0.806300408914507,-0.584827952229418,-0.0886336103035621));
#59447=DIRECTION('ref_axis',(-0.0860451784234849,0.0322834340877071,-0.995768048871611));
#59448=DIRECTION('center_axis',(0.809390485121477,-0.584827952229612,-0.0535098952133025));
#59449=DIRECTION('ref_axis',(-0.0501457367486247,0.0219588921980094,-0.998500481792259));
#59450=DIRECTION('center_axis',(0.804082195749088,-0.584827952228849,0.106902239317689));
#59451=DIRECTION('ref_axis',(0.0938788296586372,-0.0526562713838044,-0.994190164116443));
#59452=DIRECTION('center_axis',(0.804082195752539,-0.584827952229685,0.106902239287161));
#59453=DIRECTION('ref_axis',(0.115470985370648,-0.022760729030197,-0.993050049469585));
#59454=DIRECTION('center_axis',(0.798676824751148,-0.584827952229572,0.141744826700622));
#59455=DIRECTION('ref_axis',(0.15111054782177,-0.0330869094600406,-0.987962984508725));
#59456=DIRECTION('center_axis',(0.80408219575091,-0.584827952229495,0.106902239300454));
#59457=DIRECTION('ref_axis',(0.136820698101175,0.00704626726231543,-0.99057076813763));
#59458=DIRECTION('center_axis',(0.798676824749585,-0.584827952229556,0.141744826709496));
#59459=DIRECTION('ref_axis',(0.172426888770446,-0.00326197171537725,-0.985016917402677));
#59460=DIRECTION('center_axis',(0.798676824752703,-0.584827952229169,0.141744826693526));
#59461=DIRECTION('ref_axis',(0.193497060827057,0.0265489589948573,-0.980741576679392));
#59462=DIRECTION('center_axis',(0.804082195751867,-0.584827952229202,0.106902239294854));
#59463=DIRECTION('ref_axis',(0.15801544419156,0.0368858774025659,-0.986747460825305));
#59464=DIRECTION('center_axis',(-0.814941485506432,-0.572651970086207,-0.089107218321276));
#59465=DIRECTION('ref_axis',(0.574939054799503,-0.818196237626558,-1.3031285787327E-18));
#59466=DIRECTION('center_axis',(-0.876234650033272,-0.398672303273934,0.270690289229825));
#59467=DIRECTION('ref_axis',(0.41413335584115,-0.910216218038191,-5.40282558576922E-17));
#59468=DIRECTION('center_axis',(0.788833752374882,-0.584827952229736,-0.188990945298809));
#59469=DIRECTION('ref_axis',(-0.252033915049667,-0.0273514773827825,-0.967331795378254));
#59470=DIRECTION('center_axis',(0.79630163119712,-0.584827952229675,-0.154531480429235));
#59471=DIRECTION('ref_axis',(-0.216973405118666,-0.0376838387916993,-0.975449880703838));
#59472=DIRECTION('center_axis',(0.788833752376995,-0.584827952229461,-0.188990945290837));
#59473=DIRECTION('ref_axis',(-0.231262112088917,0.00246180523997023,-0.972888367196943));
#59474=DIRECTION('center_axis',(0.796301631196168,-0.584827952229549,-0.154531480434615));
#59475=DIRECTION('ref_axis',(-0.196052058353707,-0.00784651556825947,-0.9805620952335));
#59476=DIRECTION('center_axis',(0.788833752376159,-0.584827952229035,-0.188990945295645));
#59477=DIRECTION('ref_axis',(-0.210169515943608,0.0322834340937078,-0.977131799938548));
#59478=DIRECTION('center_axis',(0.796301631197679,-0.584827952229497,-0.154531480427026));
#59479=DIRECTION('ref_axis',(-0.174895616738131,0.0219588922000665,-0.984342079918935));
#59480=DIRECTION('center_axis',(0.811140170796625,-0.584827952229234,0.00528106157723248));
#59481=DIRECTION('ref_axis',(-0.0314665010067795,-0.0526562713785295,-0.998116815006591));
#59482=DIRECTION('center_axis',(0.811140170796457,-0.584827952229611,0.00528106156134455));
#59483=DIRECTION('ref_axis',(-0.00990171162426306,-0.0227607290333322,-0.999691905199187));
#59484=DIRECTION('center_axis',(0.810144356906057,-0.58482795222952,0.0405263773892647));
#59485=DIRECTION('ref_axis',(0.0260944005297899,-0.033086909462181,-0.999111774869675));
#59486=DIRECTION('center_axis',(0.811140170796392,-0.584827952229608,0.00528106157163474));
#59487=DIRECTION('ref_axis',(0.0115903885878127,0.00704626726036128,-0.999908002273249));
#59488=DIRECTION('center_axis',(0.810144356906541,-0.584827952229447,0.0405263773806528));
#59489=DIRECTION('ref_axis',(0.0476118958662175,-0.00326197170636763,-0.998860584322262));
#59490=DIRECTION('center_axis',(0.810144356906329,-0.584827952229399,0.0405263773855901));
#59491=DIRECTION('ref_axis',(0.0690517656170743,0.0265489589909614,-0.997259748732325));
#59492=DIRECTION('center_axis',(0.811140170795799,-0.584827952230299,0.00528106158617268));
#59493=DIRECTION('ref_axis',(0.0330971952593657,0.0368858773885729,-0.998771248943039));
#59494=DIRECTION('center_axis',(-0.819683524284951,-0.572651970090649,0.0137346702581644));
#59495=DIRECTION('ref_axis',(0.572705990601629,-0.819760848253323,6.03749681350753E-18));
#59496=DIRECTION('center_axis',(-0.835398788855164,-0.39867230327499,0.378377137497418));
#59497=DIRECTION('ref_axis',(0.430693725898546,-0.902498152059952,2.31475229891537E-16));
#59498=DIRECTION('center_axis',(0.758926716336079,-0.584827952229742,-0.286367780174555));
#59499=DIRECTION('ref_axis',(-0.371285374193801,-0.0273514773838731,-0.928115869703071));
#59500=DIRECTION('center_axis',(0.770654624860523,-0.584827952229746,-0.25311601188358));
#59501=DIRECTION('ref_axis',(-0.337518792743693,-0.0376838387894886,-0.94056418857988));
#59502=DIRECTION('center_axis',(0.758926716343912,-0.584827952229653,-0.286367780153981));
#59503=DIRECTION('ref_axis',(-0.351373786207065,0.00246180523036329,-0.936232023529167));
#59504=DIRECTION('center_axis',(0.770654624862685,-0.584827952229546,-0.253116011877459));
#59505=DIRECTION('ref_axis',(-0.317403147415658,-0.00784651557350236,-0.948258231814514));
#59506=DIRECTION('center_axis',(0.758926716336075,-0.584827952228924,-0.286367780176238));
#59507=DIRECTION('ref_axis',(-0.330979354643143,0.0322834340956424,-0.943085598810098));
#59508=DIRECTION('center_axis',(0.7706546248633,-0.584827952229544,-0.25311601187559));
#59509=DIRECTION('ref_axis',(-0.296887288368979,0.0219588921985787,-0.9546600154287));
#59510=DIRECTION('center_axis',(0.805405980797642,-0.584827952229345,-0.0964234016544657));
#59511=DIRECTION('ref_axis',(-0.156315586151049,-0.0526562713767823,-0.986302567476608));
#59512=DIRECTION('center_axis',(0.805405980796604,-0.584827952229569,-0.0964234016617822));
#59513=DIRECTION('ref_axis',(-0.135118252713833,-0.0227607290362419,-0.990568022397907));
#59514=DIRECTION('center_axis',(0.808835428597436,-0.584827952229255,-0.0613311970936381));
#59515=DIRECTION('ref_axis',(-0.0993332710383858,-0.0330869094686513,-0.994503975701771));
#59516=DIRECTION('center_axis',(0.805405980795944,-0.584827952229344,-0.0964234016686599));
#59517=DIRECTION('ref_axis',(-0.113822708290088,0.00704626726769293,-0.993476089896029));
#59518=DIRECTION('center_axis',(0.808835428596014,-0.584827952229492,-0.0613311971101359));
#59519=DIRECTION('ref_axis',(-0.077953965063628,-0.003261971709741,-0.996951623134956));
#59520=DIRECTION('center_axis',(0.808835428596344,-0.584827952229524,-0.0613311971054644));
#59521=DIRECTION('ref_axis',(-0.0564825171882718,0.0265489589885428,-0.998050538814895));
#59522=DIRECTION('center_axis',(0.805405980796467,-0.584827952229193,-0.0964234016652054));
#59523=DIRECTION('ref_axis',(-0.0923430162513425,0.0368858774021895,-0.995043817828077));
#59524=DIRECTION('center_axis',(-0.811498664230888,-0.572651970093207,0.116359954880761));
#59525=DIRECTION('ref_axis',(0.576568537458026,-0.817048787780456,6.33336117189426E-17));
#59526=DIRECTION('center_axis',(-0.781388189732742,-0.398672303278799,0.480096752274545));
#59527=DIRECTION('ref_axis',(0.523498180784058,-3.57703746127638E-16,0.852026792252322));
#59528=DIRECTION('center_axis',(0.717050952625024,-0.584827952229473,-0.379228424080563));
#59529=DIRECTION('ref_axis',(-0.484681441184531,-0.0273514773904689,-0.874263002337308));
#59530=DIRECTION('center_axis',(0.732853934726112,-0.584827952229606,-0.347708752618311));
#59531=DIRECTION('ref_axis',(-0.452741307376777,-0.0376838387925448,-0.890845237338464));
#59532=DIRECTION('center_axis',(0.717050952631686,-0.584827952229711,-0.379228424067599));
#59533=DIRECTION('ref_axis',(-0.465944085825003,0.00246180522786322,-0.884810741571169));
#59534=DIRECTION('center_axis',(0.732853934727818,-0.584827952229481,-0.347708752614925));
#59535=DIRECTION('ref_axis',(-0.433748599240115,-0.00784651557489748,-0.900999769617379));
#59536=DIRECTION('center_axis',(0.717050952622112,-0.584827952229132,-0.379228424086595));
#59537=DIRECTION('ref_axis',(-0.44656945119513,0.0322834340919662,-0.894166374419498));
#59538=DIRECTION('center_axis',(0.732853934728052,-0.58482795222954,-0.347708752614334));
#59539=DIRECTION('ref_axis',(-0.414196870111794,0.0219588921978709,-0.909922392208828));
#59540=DIRECTION('center_axis',(0.786970057351451,-0.584827952229999,-0.196607210251102));
#59541=DIRECTION('ref_axis',(-0.278699481130594,-0.0526562713682668,-0.958933739266238));
#59542=DIRECTION('center_axis',(0.786970057355849,-0.584827952229471,-0.196607210235065));
#59543=DIRECTION('ref_axis',(-0.258203898238116,-0.022760729042155,-0.965822290148716));
#59544=DIRECTION('center_axis',(0.794770682406187,-0.584827952229128,-0.162221541969888));
#59545=DIRECTION('ref_axis',(-0.223194397591495,-0.0330869094709643,-0.97421225475018));
#59546=DIRECTION('center_axis',(0.786970057353973,-0.584827952229482,-0.196607210242542));
#59547=DIRECTION('ref_axis',(-0.237440753046596,0.00704626726199184,-0.971376466108963));
#59548=DIRECTION('center_axis',(0.794770682402583,-0.584827952229557,-0.162221541986002));
#59549=DIRECTION('ref_axis',(-0.202290445396925,-0.00326197171136405,-0.979320139301581));
#59550=DIRECTION('center_axis',(0.794770682401897,-0.584827952229347,-0.162221541990116));
#59551=DIRECTION('ref_axis',(-0.181126036964189,0.0265489589916822,-0.983101475693179));
#59552=DIRECTION('center_axis',(0.786970057353212,-0.584827952229266,-0.196607210246233));
#59553=DIRECTION('ref_axis',(-0.216326923211641,0.0368858774012871,-0.975623951295848));
#59554=DIRECTION('center_axis',(-0.790515985477339,-0.572651970093842,0.217150173503114));
#59555=DIRECTION('ref_axis',(0.586650502040687,-0.809840224029042,2.50717685812128E-16));
#59556=DIRECTION('center_axis',(-0.715054632079823,-0.398672303282021,0.57424495447239));
#59557=DIRECTION('ref_axis',(0.626157514223864,1.11353316466764E-16,0.77969658674448));
#59558=DIRECTION('center_axis',(0.663866867044535,-0.584827952229405,-0.46610840920502));
#59559=DIRECTION('ref_axis',(-0.590433792318414,-0.0273514773937692,-0.806622485164451));
#59560=DIRECTION('center_axis',(0.683495700250236,-0.584827952229823,-0.436817918622978));
#59561=DIRECTION('ref_axis',(-0.560823821146066,-0.0376838387890247,-0.827077124535099));
#59562=DIRECTION('center_axis',(0.663866867042483,-0.584827952229439,-0.466108409207899));
#59563=DIRECTION('ref_axis',(-0.573166168879147,0.0024618052356994,-0.819435465651434));
#59564=DIRECTION('center_axis',(0.683495700255293,-0.584827952229569,-0.436817918615406));
#59565=DIRECTION('ref_axis',(-0.543253576548145,-0.00784651557452022,-0.839532002821207));
#59566=DIRECTION('center_axis',(0.663866867031427,-0.584827952228639,-0.466108409224651));
#59567=DIRECTION('ref_axis',(-0.555116880746585,0.032283434098762,-0.83114561214806));
#59568=DIRECTION('center_axis',(0.68349570025321,-0.584827952229423,-0.436817918618862));
#59569=DIRECTION('ref_axis',(-0.524974319787969,0.0219588922014649,-0.850834749300029));
#59570=DIRECTION('center_axis',(0.756123145990597,-0.584827952229889,-0.293690405678969));
#59571=DIRECTION('ref_axis',(-0.396688118793096,-0.0526562713693517,-0.916441953150265));
#59572=DIRECTION('center_axis',(0.756123146001629,-0.584827952229234,-0.29369040565187));
#59573=DIRECTION('ref_axis',(-0.377217514040846,-0.0227607290510223,-0.925844963432815));
#59574=DIRECTION('center_axis',(0.768171927774616,-0.584827952229541,-0.260553556241384));
#59575=DIRECTION('ref_axis',(-0.343535615178875,-0.0330869094603869,-0.938556624570959));
#59576=DIRECTION('center_axis',(0.756123145995835,-0.584827952229549,-0.293690405666161));
#59577=DIRECTION('ref_axis',(-0.357314215289047,0.0070462672583536,-0.933957655180414));
#59578=DIRECTION('center_axis',(0.768171927772525,-0.584827952229534,-0.260553556247562));
#59579=DIRECTION('ref_axis',(-0.323436684571794,-0.00326197170798405,-0.946244191852073));
#59580=DIRECTION('center_axis',(0.768171927771508,-0.58482795222913,-0.260553556251471));
#59581=DIRECTION('ref_axis',(-0.302913090938082,0.0265489589950167,-0.95264831502219));
#59582=DIRECTION('center_axis',(0.75612314599938,-0.584827952230302,-0.293690405655535));
#59583=DIRECTION('ref_axis',(-0.336899225350735,0.0368858773883775,-0.940817912248361));
#59584=DIRECTION('center_axis',(-0.75706639739712,-0.572651970098847,0.314515804172152));
#59585=DIRECTION('ref_axis',(0.603266390053514,-0.797539756144985,-4.43056783040492E-17));
#59586=DIRECTION('center_axis',(-0.637444235726239,-0.398672303285474,0.65933697070045));
#59587=DIRECTION('ref_axis',(0.718941969615881,5.05113636903814E-16,0.69507010029553));
#59588=DIRECTION('center_axis',(0.600213204389163,-0.584827952229446,-0.545637586285995));
#59589=DIRECTION('ref_axis',(-0.686874649847015,-0.0273514773903244,-0.726261049542179));
#59590=DIRECTION('center_axis',(0.623358330292039,-0.584827952229342,-0.519038205093572));
#59591=DIRECTION('ref_axis',(-0.6600618082234,-0.037683838796267,-0.750265511414747));
#59592=DIRECTION('center_axis',(0.600213204391252,-0.584827952229486,-0.545637586283653));
#59593=DIRECTION('ref_axis',(-0.671349079048087,0.00246180523542522,-0.741137202936317));
#59594=DIRECTION('center_axis',(0.623358330295149,-0.58482795222947,-0.519038205089691));
#59595=DIRECTION('ref_axis',(-0.644191120423901,-0.00784651557927282,-0.764824314833324));
#59596=DIRECTION('center_axis',(0.600213204390774,-0.584827952229604,-0.545637586284054));
#59597=DIRECTION('ref_axis',(-0.654909785457995,0.0322834340866717,-0.755017187085787));
#59598=DIRECTION('center_axis',(0.623358330287479,-0.584827952229354,-0.519038205099034));
#59599=DIRECTION('ref_axis',(-0.6274726108324,0.0219588922014093,-0.778328934132901));
#59600=DIRECTION('center_axis',(0.713351720938627,-0.584827952229213,-0.386141927955623));
#59601=DIRECTION('ref_axis',(-0.508420747842796,-0.0526562713784942,-0.859497329982756));
#59602=DIRECTION('center_axis',(0.713351720938112,-0.584827952229473,-0.38614192795618));
#59603=DIRECTION('ref_axis',(-0.490282184329536,-0.0227607290419115,-0.871266508562414));
#59604=DIRECTION('center_axis',(0.729458642964286,-0.584827952229379,-0.354776485263458));
#59605=DIRECTION('ref_axis',(-0.458459070881828,-0.0330869094649778,-0.888099395759409));
#59606=DIRECTION('center_axis',(0.713351720936875,-0.584827952229576,-0.386141927958309));
#59607=DIRECTION('ref_axis',(-0.471552618913885,0.00704626725944046,-0.881809774108433));
#59608=DIRECTION('center_axis',(0.729458642961595,-0.584827952229519,-0.354776485268762));
#59609=DIRECTION('ref_axis',(-0.439482134009922,-0.00326197171117806,-0.898245408241334));
#59610=DIRECTION('center_axis',(0.729458642961771,-0.58482795222943,-0.354776485268546));
#59611=DIRECTION('ref_axis',(-0.419923024504176,0.0265489589890718,-0.907171321343362));
#59612=DIRECTION('center_axis',(0.713351720934301,-0.584827952229366,-0.386141927963382));
#59613=DIRECTION('ref_axis',(-0.452158425482432,0.0368858773992535,-0.891174612695927));
#59614=DIRECTION('center_axis',(-0.711677419984127,-0.572651970099548,0.406921332723959));
#59615=DIRECTION('ref_axis',(0.626902064855465,-0.779098068974602,-1.93769385385326E-16));
#59616=DIRECTION('center_axis',(-0.549780962986053,-0.39867230328459,0.734030849032851));
#59617=DIRECTION('ref_axis',(0.800388280671782,3.1365307998394E-16,0.599481943150308));
#59618=DIRECTION('center_axis',(0.527093820944015,-0.58482795222981,-0.616561732686457));
#59619=DIRECTION('ref_axis',(-0.772483083831191,-0.0273514773824917,-0.634446043316253));
#59620=DIRECTION('center_axis',(0.553390227073648,-0.584827952229816,-0.593072949029086));
#59621=DIRECTION('ref_axis',(-0.748890226298068,-0.0376838387900128,-0.661621762980388));
#59622=DIRECTION('center_axis',(0.52709382095827,-0.584827952229528,-0.616561732674538));
#59623=DIRECTION('ref_axis',(-0.758944413195169,0.00246180523388964,-0.651150763798087));
#59624=DIRECTION('center_axis',(0.553390227071032,-0.584827952229476,-0.593072949031862));
#59625=DIRECTION('ref_axis',(-0.734969385526333,-0.00784651556787667,-0.678054890501121));
#59626=DIRECTION('center_axis',(0.527093820954421,-0.584827952229462,-0.616561732677892));
#59627=DIRECTION('ref_axis',(-0.744374371642847,0.0322834340877894,-0.666981689947195));
#59628=DIRECTION('center_axis',(0.553390227083124,-0.584827952229677,-0.593072949020381));
#59629=DIRECTION('ref_axis',(-0.720075283965554,0.0219588921958596,-0.693548406728368));
#59630=DIRECTION('center_axis',(0.659330313101025,-0.584827952229551,-0.472503761378779));
#59631=DIRECTION('ref_axis',(-0.61213527799987,-0.0526562713738629,-0.788997920474461));
#59632=DIRECTION('center_axis',(0.659330313100206,-0.584827952229568,-0.472503761379902));
#59633=DIRECTION('ref_axis',(-0.595614811685905,-0.0227607290370077,-0.80294766038271));
#59634=DIRECTION('center_axis',(0.679241359593035,-0.584827952229435,-0.443404377187834));
#59635=DIRECTION('ref_axis',(-0.566152353171553,-0.0330869094612513,-0.823636308949901));
#59636=DIRECTION('center_axis',(0.659330313104009,-0.584827952229546,-0.472503761374621));
#59637=DIRECTION('ref_axis',(-0.578354356045136,0.00704626725904472,-0.815755226131792));
#59638=DIRECTION('center_axis',(0.679241359593601,-0.584827952229575,-0.443404377186782));
#59639=DIRECTION('ref_axis',(-0.54859668766339,-0.00326197171347784,-0.836080757956609));
#59640=DIRECTION('center_axis',(0.679241359592077,-0.584827952229497,-0.443404377189219));
#59641=DIRECTION('ref_axis',(-0.530310521131489,0.0265489589891908,-0.847387694006609));
#59642=DIRECTION('center_axis',(0.659330313101111,-0.584827952229377,-0.472503761378876));
#59643=DIRECTION('ref_axis',(-0.560286817122907,0.0368858773991434,-0.827476957145501));
#59644=DIRECTION('center_axis',(-0.655064864523098,-0.572651970099649,0.492909468775278));
#59645=DIRECTION('ref_axis',(0.658159678738397,-0.75287836818637,3.33585939142612E-17));
#59646=DIRECTION('center_axis',(-0.453447316035864,-0.398672303285154,0.797148622386806));
#59647=DIRECTION('ref_axis',(0.869211990412778,-3.92406044704623E-16,0.494439597648345));
#59648=DIRECTION('center_axis',(0.445661853117017,-0.584827952228927,-0.677762332213901));
#59649=DIRECTION('ref_axis',(-0.845908998097638,-0.0273514774077798,-0.532625444023342));
#59650=DIRECTION('center_axis',(0.474694829402545,-0.584827952229701,-0.657754578265559));
#59651=DIRECTION('ref_axis',(-0.825908198131717,-0.0376838387902702,-0.562543844116038));
#59652=DIRECTION('center_axis',(0.445661853094375,-0.584827952229501,-0.677762332228294));
#59653=DIRECTION('ref_axis',(-0.834570740577306,0.00246180523543606,-0.550895288133081));
#59654=DIRECTION('center_axis',(0.474694829395997,-0.584827952229462,-0.657754578270496));
#59655=DIRECTION('ref_axis',(-0.814156744359243,-0.00784651556552523,-0.580592135502918));
#59656=DIRECTION('center_axis',(0.44566185310384,-0.584827952230146,-0.677762332221514));
#59657=DIRECTION('ref_axis',(-0.822099729311578,0.0322834340795859,-0.568427493133345));
#59658=DIRECTION('center_axis',(0.47469482941652,-0.584827952229831,-0.657754578255358));
#59659=DIRECTION('ref_axis',(-0.801321939721966,0.0219588921926168,-0.597830206642236));
#59660=DIRECTION('center_axis',(0.594910872379941,-0.584827952228667,-0.551413928202908));
#59661=DIRECTION('ref_axis',(-0.706196069132843,-0.0526562713866946,-0.706055542450431));
#59662=DIRECTION('center_axis',(0.59491087235748,-0.584827952229707,-0.551413928226038));
#59663=DIRECTION('ref_axis',(-0.691554237658444,-0.0227607290313939,-0.721965847939227));
#59664=DIRECTION('center_axis',(0.618312034230551,-0.584827952229208,-0.525039517195676));
#59665=DIRECTION('ref_axis',(-0.664917074641091,-0.0330869094688109,-0.746183985537439));
#59666=DIRECTION('center_axis',(0.594910872366718,-0.584827952229429,-0.551413928216366));
#59667=DIRECTION('ref_axis',(-0.676035099491233,0.00704626726054901,-0.73683573092893));
#59668=DIRECTION('center_axis',(0.618312034217811,-0.584827952229436,-0.525039517210426));
#59669=DIRECTION('ref_axis',(-0.649059543844922,-0.00326197170724836,-0.760730614662249));
#59670=DIRECTION('center_axis',(0.618312034220884,-0.584827952229394,-0.525039517206855));
#59671=DIRECTION('ref_axis',(-0.632334704050471,0.0265489589903301,-0.774240256528898));
#59672=DIRECTION('center_axis',(0.594910872389116,-0.584827952230958,-0.551413928190579));
#59673=DIRECTION('ref_axis',(-0.659579150937677,0.0368858773772172,-0.750729495689657));
#59674=DIRECTION('center_axis',(-0.588121544827873,-0.572651970103301,0.571124128054562));
#59675=DIRECTION('ref_axis',(0.697621253253775,-0.716466738243048,-6.26947218563319E-16));
#59676=DIRECTION('center_axis',(-0.349962534036297,-0.398672303280935,0.847694885774102));
#59677=DIRECTION('ref_axis',(8.44177824649252E-17,-0.90491859166274,-0.4255847065663));
#59678=DIRECTION('center_axis',(0.357201531611052,-0.584827952228913,-0.728274214912525));
#59679=DIRECTION('ref_axis',(-0.905994422163722,-0.0273514774097695,-0.422405023279467));
#59680=DIRECTION('center_axis',(0.388513210693687,-0.584827952230087,-0.712063024883926));
#59681=DIRECTION('ref_axis',(-0.889901104311223,-0.0376838387844891,-0.454594272775329));
#59682=DIRECTION('center_axis',(0.357201531563024,-0.58482795222909,-0.72827421493594));
#59683=DIRECTION('ref_axis',(-0.897035388838967,0.00246180524912005,-0.441951864670168));
#59684=DIRECTION('center_axis',(0.388513210718662,-0.584827952229685,-0.712063024870629));
#59685=DIRECTION('ref_axis',(-0.88050436496746,-0.00784651558132259,-0.473973095720087));
#59686=DIRECTION('center_axis',(0.357201531562618,-0.58482795222851,-0.728274214936605));
#59687=DIRECTION('ref_axis',(-0.886860083170569,0.0322834341005172,-0.460908855156168));
#59688=DIRECTION('center_axis',(0.388513210725782,-0.584827952230155,-0.712063024866358));
#59689=DIRECTION('ref_axis',(-0.869931269801255,0.0219588921870204,-0.492683867074917));
#59690=DIRECTION('center_axis',(0.521109331790668,-0.584827952229543,-0.62162796800955));
#59691=DIRECTION('ref_axis',(-0.789119726418472,-0.0526562713750646,-0.611978246722963));
#59692=DIRECTION('center_axis',(0.521109331792446,-0.584827952229465,-0.621627968008134));
#59693=DIRECTION('ref_axis',(-0.776587440174645,-0.022760729040405,-0.629598202805998));
#59694=DIRECTION('center_axis',(0.547631558707113,-0.584827952229693,-0.598394470394607));
#59695=DIRECTION('ref_axis',(-0.753195656657539,-0.0330869094581457,-0.656963894909551));
#59696=DIRECTION('center_axis',(0.521109331798352,-0.58482795222975,-0.621627968002915));
#59697=DIRECTION('ref_axis',(-0.76305436556791,0.00704626725475995,-0.64629589609213));
#59698=DIRECTION('center_axis',(0.547631558727812,-0.584827952229681,-0.598394470375676));
#59699=DIRECTION('ref_axis',(-0.73928634326801,-0.00326197172494508,-0.673383295158025));
#59700=DIRECTION('center_axis',(0.547631558699565,-0.584827952228912,-0.598394470402278));
#59701=DIRECTION('ref_axis',(-0.724386590953742,0.0265489589987662,-0.688882587690019));
#59702=DIRECTION('center_axis',(0.521109331796591,-0.584827952229941,-0.621627968004211));
#59703=DIRECTION('ref_axis',(-0.748469527566617,0.0368858773927419,-0.66214258158887));
#59704=DIRECTION('center_axis',(-0.511903197047791,-0.572651970103374,0.640331818660431));
#59705=DIRECTION('ref_axis',(-3.39450182657419E-16,-0.745401236142811,-0.666616079281597));
#59706=DIRECTION('center_axis',(-0.240958633816367,-0.398672303283347,0.884872494421711));
#59707=DIRECTION('ref_axis',(3.01927584586609E-17,-0.911736456568353,-0.410775648942563));
#59708=DIRECTION('center_axis',(0.263107928563467,-0.584827952229085,-0.767300778194951));
#59709=DIRECTION('ref_axis',(-0.951791772979906,-0.0273514774076893,-0.305523022980894));
#59710=DIRECTION('center_axis',(0.296204506578728,-0.584827952229886,-0.755141812226717));
#59711=DIRECTION('ref_axis',(-0.939859738468349,-0.0376838387875407,-0.339475478201949));
#59712=DIRECTION('center_axis',(0.26310792852108,-0.584827952229321,-0.767300778209305));
#59713=DIRECTION('ref_axis',(-0.94535325314404,0.00246180524608073,-0.326038596311711));
#59714=DIRECTION('center_axis',(0.296204506588777,-0.584827952229501,-0.755141812223074));
#59715=DIRECTION('ref_axis',(-0.932965905768518,-0.00784651557401198,-0.359879217053272));
#59716=DIRECTION('center_axis',(0.263107928504294,-0.584827952228226,-0.767300778215896));
#59717=DIRECTION('ref_axis',(-0.93763412372089,0.0322834341076045,-0.346121409214134));
#59718=DIRECTION('center_axis',(0.296204506582971,-0.584827952229374,-0.75514181222545));
#59719=DIRECTION('ref_axis',(-0.924821264096414,0.0219588922029174,-0.379767608582316));
#59720=DIRECTION('center_axis',(0.43908958573722,-0.584827952230541,-0.682038563416284));
#59721=DIRECTION('ref_axis',(-0.859598494219977,-0.0526562713614962,-0.508249688461343));
#59722=DIRECTION('center_axis',(0.439089585757463,-0.584827952229602,-0.682038563404057));
#59723=DIRECTION('ref_axis',(-0.849373394858158,-0.0227607290393782,-0.527301417901302));
#59724=DIRECTION('center_axis',(0.468314606413799,-0.584827952228568,-0.66231238529234));
#59725=DIRECTION('ref_axis',(-0.829595893198619,-0.0330869094855917,-0.557383091247553));
#59726=DIRECTION('center_axis',(0.439089585767504,-0.584827952229721,-0.682038563397491));
#59727=DIRECTION('ref_axis',(-0.838039808477603,0.00704626725346033,-0.545563588891904));
#59728=DIRECTION('center_axis',(0.468314606372224,-0.584827952229452,-0.662312385320956));
#59729=DIRECTION('ref_axis',(-0.817854155462514,-0.00326197170577599,-0.575416318793));
#59730=DIRECTION('center_axis',(0.468314606377903,-0.584827952229227,-0.662312385317139));
#59731=DIRECTION('ref_axis',(-0.805014468575387,0.0265489589908086,-0.592660828940796));
#59732=DIRECTION('center_axis',(0.439089585738317,-0.584827952228573,-0.682038563417265));
#59733=DIRECTION('ref_axis',(-0.825556092629325,0.0368858774108551,-0.563113283425487));
#59734=DIRECTION('center_axis',(-0.427611830052617,-0.572651970104803,0.699441093970135));
#59735=DIRECTION('ref_axis',(-1.75302949851223E-16,-0.773750158454805,-0.6334908778279));
#59736=DIRECTION('center_axis',(-0.128154671999727,-0.398672303284917,0.908095135235368));
#59737=DIRECTION('ref_axis',(-2.92400519014607E-17,-0.915645369907592,-0.401987010445348));
#59738=DIRECTION('center_axis',(0.1648649562964,-0.584827952229255,-0.79422654984376));
#59739=DIRECTION('ref_axis',(-0.982578798964788,-0.0273514773978768,-0.183822742088859));
#59740=DIRECTION('center_axis',(0.199224480465946,-0.584827952229349,-0.786311562088655));
#59741=DIRECTION('ref_axis',(-0.974996223102871,-0.0376838387993657,-0.219002952556533));
#59742=DIRECTION('center_axis',(0.164864956283302,-0.584827952229486,-0.794226549846309));
#59743=DIRECTION('ref_axis',(-0.978762331919751,0.00246180523728022,-0.204983504531425));
#59744=DIRECTION('center_axis',(0.199224480450776,-0.584827952229559,-0.786311562092342));
#59745=DIRECTION('ref_axis',(-0.970714016905226,-0.00784651557031847,-0.240109828156044));
#59746=DIRECTION('center_axis',(0.164864956289079,-0.584827952229657,-0.794226549844983));
#59747=DIRECTION('ref_axis',(-0.97362111401387,0.0322834340847991,-0.225875421925633));
#59748=DIRECTION('center_axis',(0.199224480466149,-0.58482795222989,-0.786311562088201));
#59749=DIRECTION('ref_axis',(-0.965126274581717,0.0219588921935203,-0.26086218807188));
#59750=DIRECTION('center_axis',(0.350145134649513,-0.584827952229794,-0.731693003227434));
#59751=DIRECTION('ref_axis',(-0.916520880250958,-0.0526562713704369,-0.396505729024655));
#59752=DIRECTION('center_axis',(0.350145134667601,-0.584827952229321,-0.731693003219155));
#59753=DIRECTION('ref_axis',(-0.908764223708701,-0.0227607290460544,-0.416688774651315));
#59754=DIRECTION('center_axis',(0.381612052951492,-0.584827952229456,-0.715785238275594));
#59755=DIRECTION('ref_axis',(-0.892912906966885,-0.0330869094632203,-0.449012023217774));
#59756=DIRECTION('center_axis',(0.350145134675522,-0.584827952229961,-0.731693003214853));
#59757=DIRECTION('ref_axis',(-0.899808862985237,0.00704626724822561,-0.436227417995569));
#59758=DIRECTION('center_axis',(0.381612052944737,-0.584827952229599,-0.715785238279079));
#59759=DIRECTION('ref_axis',(-0.883523919043546,-0.00326197170887951,-0.468374683366324));
#59760=DIRECTION('center_axis',(0.381612052960543,-0.584827952229905,-0.715785238270402));
#59761=DIRECTION('ref_axis',(-0.872946787136347,0.0265489589811143,-0.487092454884438));
#59762=DIRECTION('center_axis',(0.350145134633492,-0.584827952228301,-0.731693003236293));
#59763=DIRECTION('ref_axis',(-0.889623144933142,0.0368858774129701,-0.455203352411579));
#59764=DIRECTION('center_axis',(-0.336576769080192,-0.572651970082322,0.747519765408497));
#59765=DIRECTION('ref_axis',(4.05335326092723E-16,-0.793835266517972,-0.60813285524821));
#59766=DIRECTION('center_axis',(-0.01332963444991,-0.398672303291145,0.91699657329456));
#59767=DIRECTION('ref_axis',(1.50046340237098E-17,-0.917078049740163,-0.398707725890507));
#59768=DIRECTION('center_axis',(0.0640219651873326,-0.584827952229454,-0.808626894349091));
#59769=DIRECTION('ref_axis',(-0.997869970322272,-0.0273514773912274,-0.0592234667471015));
#59770=DIRECTION('center_axis',(0.0991025652636654,-0.584827952229383,-0.805080708903988));
#59771=DIRECTION('ref_axis',(-0.994756434870767,-0.037683838797787,-0.0950766195058686));
#59772=DIRECTION('center_axis',(0.0640219651883166,-0.584827952229605,-0.808626894348903));
#59773=DIRECTION('ref_axis',(-0.996735744040505,0.0024618052355194,-0.0806957004245199));
#59774=DIRECTION('center_axis',(0.0991025652509091,-0.584827952229481,-0.805080708905487));
#59775=DIRECTION('ref_axis',(-0.993153388117073,-0.00784651557029387,-0.116553763838773));
#59776=DIRECTION('center_axis',(0.0640219652154374,-0.584827952230895,-0.808626894345823));
#59777=DIRECTION('ref_axis',(-0.994253517734423,0.0322834340705456,-0.102067244291878));
#59778=DIRECTION('center_axis',(0.0991025652721308,-0.584827952229959,-0.805080708902527));
#59779=DIRECTION('ref_axis',(-0.990210667182516,0.0219588921906706,-0.137842815016649));
#59780=DIRECTION('center_axis',(0.255678685621909,-0.584827952229304,-0.769808207289278));
#59781=DIRECTION('ref_axis',(-0.958989184500568,-0.0526562713786804,-0.278508637380299));
#59782=DIRECTION('center_axis',(0.255678685634193,-0.584827952229256,-0.769808207285234));
#59783=DIRECTION('ref_axis',(-0.953823297885295,-0.0227607290501976,-0.299504700504554));
#59784=DIRECTION('center_axis',(0.288891249491466,-0.58482795222929,-0.757969730436879));
#59785=DIRECTION('ref_axis',(-0.942148150771053,-0.0330869094683896,-0.333559767388869));
#59786=DIRECTION('center_axis',(0.255678685607245,-0.584827952229379,-0.769808207294092));
#59787=DIRECTION('ref_axis',(-0.947387394215224,0.00704626726637755,-0.320011680098865));
#59788=DIRECTION('center_axis',(0.288891249475173,-0.58482795222939,-0.757969730443012));
#59789=DIRECTION('ref_axis',(-0.935259982631717,-0.00326197170936511,-0.353946499386967));
#59790=DIRECTION('center_axis',(0.288891249477309,-0.584827952229552,-0.757969730442073));
#59791=DIRECTION('ref_axis',(-0.927112213402921,0.0265489589896012,-0.373842341817651));
#59792=DIRECTION('center_axis',(0.255678685630505,-0.584827952230323,-0.769808207285649));
#59793=DIRECTION('ref_axis',(-0.939660308794284,0.0368858773885189,-0.340114592638878));
#59794=DIRECTION('center_axis',(-0.240233691368199,-0.572651970087536,0.783809603594185));
#59795=DIRECTION('ref_axis',(1.07498383400422E-17,-0.807455881581724,-0.589927961109729));
#59796=DIRECTION('center_axis',(0.101705619397328,-0.398672303296703,0.911436427605956));
#59797=DIRECTION('ref_axis',(1.56250901277415E-16,-0.916187281030926,-0.400750378761092));
#59798=DIRECTION('center_axis',(-0.0378306905315764,-0.584827952229299,
-0.810274709678878));
#59799=DIRECTION('ref_axis',(-0.997424136147838,-0.0273514773998618,0.0663097980224935));
#59800=DIRECTION('center_axis',(-0.00258225658073046,-0.584827952229025,
-0.811153252007632));
#59801=DIRECTION('ref_axis',(-0.998828743421528,-0.0376838388038362,0.030349128619739));
#59802=DIRECTION('center_axis',(-0.0378306905364861,-0.584827952229633,
-0.810274709678407));
#59803=DIRECTION('ref_axis',(-0.998990038057491,0.00246180523032482,0.0448647230783922));
#59804=DIRECTION('center_axis',(-0.00258225661252645,-0.584827952229595,
-0.81115325200712));
#59805=DIRECTION('ref_axis',(-0.999930137117214,-0.00784651556523036,0.00884042296698303));
#59806=DIRECTION('center_axis',(-0.0378306905424066,-0.584827952229676,
-0.8102747096781));
#59807=DIRECTION('ref_axis',(-0.999205949545135,0.0322834340848084,0.0233505947953502));
#59808=DIRECTION('center_axis',(-0.00258225660711838,-0.584827952229256,
-0.811153252007381));
#59809=DIRECTION('ref_axis',(-0.99967884603978,0.0219588922047833,-0.0126495784005934));
#59810=DIRECTION('center_axis',(0.157180030989646,-0.584827952228585,-0.795783076064208));
#59811=DIRECTION('ref_axis',(-0.986333656440618,-0.0526562713877413,-0.156119298153757));
#59812=DIRECTION('center_axis',(0.157180030957695,-0.584827952229673,-0.79578307606972));
#59813=DIRECTION('ref_axis',(-0.983840008874882,-0.0227607290325835,-0.177597258286768));
#59814=DIRECTION('center_axis',(0.191614458464428,-0.584827952228724,-0.788200587159982));
#59815=DIRECTION('ref_axis',(-0.976525155425776,-0.0330869094830448,-0.212847074777938));
#59816=DIRECTION('center_axis',(0.157180030967844,-0.584827952229568,-0.795783076067793));
#59817=DIRECTION('ref_axis',(-0.980025060284695,0.00704626726114766,-0.198749166870366));
#59818=DIRECTION('center_axis',(0.191614458419219,-0.584827952229447,-0.788200587170436));
#59819=DIRECTION('ref_axis',(-0.972246437598155,-0.00326197170583667,-0.233936367669261));
#59820=DIRECTION('center_axis',(0.191614458440564,-0.584827952229784,-0.788200587164998));
#59821=DIRECTION('ref_axis',(-0.966656526225866,0.0265489589817698,-0.254696511719196));
#59822=DIRECTION('center_axis',(0.157180030962411,-0.584827952229387,-0.795783076068999));
#59823=DIRECTION('ref_axis',(-0.974878468277728,0.0368858774010781,-0.219662022518284));
#59824=DIRECTION('center_axis',(-0.140101984835677,-0.572651970092198,0.807738296105012));
#59825=DIRECTION('ref_axis',(4.34107268269613E-17,-0.815784312898716,-0.578356252519474));
#59826=DIRECTION('center_axis',(0.215136914870904,-0.398672303292247,0.891502384992595));
#59827=DIRECTION('ref_axis',(-2.23020076991194E-16,-0.912878440593297,-0.408231494007935));
#59828=DIRECTION('center_axis',(-0.139086733705889,-0.584827952229799,-0.799144008797993));
#59829=DIRECTION('ref_axis',(-0.981248327510859,-0.0273514773825953,0.190797317701617));
#59830=DIRECTION('center_axis',(-0.104226354737577,-0.584827952229801,-0.804433423764089));
#59831=DIRECTION('ref_axis',(-0.987148926014928,-0.0376838387855637,0.155296252890911));
#59832=DIRECTION('center_axis',(-0.139086733679773,-0.584827952229591,-0.799144008802691));
#59833=DIRECTION('ref_axis',(-0.98548966240741,0.00246180522930748,0.169717603103337));
#59834=DIRECTION('center_axis',(-0.104226354689701,-0.584827952229773,-0.804433423770312));
#59835=DIRECTION('ref_axis',(-0.990937390529949,-0.00784651559373285,0.13409519097541));
#59836=DIRECTION('center_axis',(-0.139086733682762,-0.584827952229986,-0.799144008801882));
#59837=DIRECTION('ref_axis',(-0.988400306633913,0.0322834340821356,0.148400181030382));
#59838=DIRECTION('center_axis',(-0.104226354709108,-0.584827952229878,-0.804433423767722));
#59839=DIRECTION('ref_axis',(-0.993381492315826,0.021958892191087,0.112743149584011));
#59840=DIRECTION('center_axis',(0.0562025533357102,-0.584827952229681,-0.809207970357055));
#59841=DIRECTION('ref_axis',(-0.998123057416714,-0.0526562713740524,-0.0312678643033671));
#59842=DIRECTION('center_axis',(0.0562025533502697,-0.584827952229286,-0.80920797035633));
#59843=DIRECTION('ref_axis',(-0.998340975198042,-0.0227607290464764,-0.0528890012563592));
#59844=DIRECTION('center_axis',(0.0913157928915538,-0.584827952229636,-0.806001049788074));
#59845=DIRECTION('ref_axis',(-0.995501775042467,-0.0330869094538936,-0.0887776565926787));
#59846=DIRECTION('center_axis',(0.0562025533307129,-0.584827952229465,-0.809207970357558));
#59847=DIRECTION('ref_axis',(-0.997207145717477,0.00704626726482406,-0.0743522605415241));
#59848=DIRECTION('center_axis',(0.0913157928957569,-0.584827952229292,-0.806001049787848));
#59849=DIRECTION('ref_axis',(-0.993899985449946,-0.00326197170642138,-0.11023691969202));
#59850=DIRECTION('center_axis',(0.0913157929462842,-0.584827952230976,-0.806001049780901));
#59851=DIRECTION('ref_axis',(-0.990956088178859,0.0265489589641095,-0.131533965496278));
#59852=DIRECTION('center_axis',(0.0562025533008339,-0.584827952227875,-0.809207970360782));
#59853=DIRECTION('ref_axis',(-0.994722211948487,0.036885877419139,-0.095745251074552));
#59854=DIRECTION('center_axis',(-0.0377607863096941,-0.572651970097324,
0.818928473165348));
#59855=DIRECTION('ref_axis',(-2.66091658816507E-19,-0.819512943907396,-0.573060672850819));
#59856=DIRECTION('center_axis',(0.325175372679881,-0.398672303295285,0.857508817206991));
#59857=DIRECTION('ref_axis',(-1.86469491306704E-16,-0.906789441031397,-0.421583810924905));
#59858=DIRECTION('center_axis',(-0.238149295947369,-0.584827952229357,-0.775410329523014));
#59859=DIRECTION('ref_axis',(-0.949597646587419,-0.0273514773986001,0.312275849658199));
#59860=DIRECTION('center_axis',(-0.204226740992109,-0.584827952230219,-0.785027199881604));
#59861=DIRECTION('ref_axis',(-0.95990118034991,-0.0376838387824492,0.277794262463191));
#59862=DIRECTION('center_axis',(-0.238149295926173,-0.584827952229801,-0.775410329529189));
#59863=DIRECTION('ref_axis',(-0.956447526083613,0.00246180521581662,0.29189393512647));
#59864=DIRECTION('center_axis',(-0.20422674096961,-0.584827952229362,-0.785027199888095));
#59865=DIRECTION('ref_axis',(-0.966316969330447,-0.00784651557616204,0.257235197780811));
#59866=DIRECTION('center_axis',(-0.238149295974102,-0.584827952228874,-0.775410329515168));
#59867=DIRECTION('ref_axis',(-0.962007000439502,0.0322834340959872,0.271109407782839));
#59868=DIRECTION('center_axis',(-0.204226740951319,-0.58482795223023,-0.785027199892207));
#59869=DIRECTION('ref_axis',(-0.971417919042336,0.0219588921862599,0.236357850763224));
#59870=DIRECTION('center_axis',(-0.0456612721227857,-0.584827952229086,
-0.809871171557343));
#59871=DIRECTION('ref_axis',(-0.994171461524437,-0.0526562713812391,0.0940766824170002));
#59872=DIRECTION('center_axis',(-0.045661272150223,-0.584827952229654,-0.809871171555386));
#59873=DIRECTION('ref_axis',(-0.997097507964699,-0.0227607290290802,0.0726533469611127));
#59874=DIRECTION('center_axis',(-0.0104229772031832,-0.584827952228972,
-0.811090394369141));
#59875=DIRECTION('ref_axis',(-0.998778736973622,-0.0330869094738195,0.0366918382047993));
#59876=DIRECTION('center_axis',(-0.045661272103643,-0.584827952229944,-0.809871171557803));
#59877=DIRECTION('ref_axis',(-0.998662678760311,0.00704626724351014,0.0512172253173974));
#59878=DIRECTION('center_axis',(-0.0104229772141451,-0.584827952229454,
-0.811090394368653));
#59879=DIRECTION('ref_axis',(-0.999879136804493,-0.00326197171688232,0.0152010303473315));
#59880=DIRECTION('center_axis',(-0.0104229772060856,-0.584827952230127,
-0.811090394368271));
#59881=DIRECTION('ref_axis',(-0.999627680658252,0.026548958978832,-0.00629705001911262));
#59882=DIRECTION('center_axis',(-0.0456612721438079,-0.584827952229114,
-0.809871171556137));
#59883=DIRECTION('ref_axis',(-0.998878592114955,0.0368858774036614,0.0296814801283008));
#59884=DIRECTION('center_axis',(0.0651759223724451,-0.572651970102054,0.817203658998868));
#59885=DIRECTION('ref_axis',(-1.00418082817833E-16,-0.818944908520059,-0.573872143259343));
#59886=DIRECTION('center_axis',(0.430085620611463,-0.398672303296099,0.809991823124059));
#59887=DIRECTION('ref_axis',(0.883216234748452,-1.85852527887398E-17,-0.468965971768493));
#59888=DIRECTION('center_axis',(-0.333456101556104,-0.584827952229228,-0.739447966138506));
#59889=DIRECTION('ref_axis',(-0.902971243511053,-0.0273514773981376,0.428829604943784));
#59890=DIRECTION('center_axis',(-0.301006349552527,-0.58482795223066,-0.753240628098854));
#59891=DIRECTION('ref_axis',(-0.917515219648999,-0.0376838387726605,0.395911290578843));
#59892=DIRECTION('center_axis',(-0.333456101558463,-0.584827952229472,-0.73944796613725));
#59893=DIRECTION('ref_axis',(-0.912321640907653,0.00246180523059358,0.409466925461109));
#59894=DIRECTION('center_axis',(-0.301006349518084,-0.584827952229521,-0.753240628113502));
#59895=DIRECTION('ref_axis',(-0.926457152277091,-0.00784651557441018,0.376318451830314));
#59896=DIRECTION('center_axis',(-0.333456101577383,-0.584827952229164,-0.739447966128961));
#59897=DIRECTION('ref_axis',(-0.920442269177619,0.0322834340938364,0.389543077199768));
#59898=DIRECTION('center_axis',(-0.30100634950513,-0.584827952230014,-0.753240628118295));
#59899=DIRECTION('ref_axis',(-0.934134504885361,0.0219588921907591,0.356245047455169));
#59900=DIRECTION('center_axis',(-0.146804992071868,-0.584827952229856,-0.79776222058544));
#59901=DIRECTION('ref_axis',(-0.974541187792916,-0.0526562713714318,0.217937583680351));
#59902=DIRECTION('center_axis',(-0.14680499205743,-0.584827952229402,-0.79776222058843));
#59903=DIRECTION('ref_axis',(-0.980129217395657,-0.0227607290439648,0.197049908451549));
#59904=DIRECTION('center_axis',(-0.111997370784885,-0.584827952229807,-0.803388358907424));
#59905=DIRECTION('ref_axis',(-0.986304361580781,-0.033086909454995,0.161582680846199));
#59906=DIRECTION('center_axis',(-0.146804992063548,-0.584827952229562,-0.797762220587186));
#59907=DIRECTION('ref_axis',(-0.98436870478496,0.00704626725946665,0.175978984988801));
#59908=DIRECTION('center_axis',(-0.111997370782148,-0.58482795222945,-0.803388358908065));
#59909=DIRECTION('ref_axis',(-0.990089596872472,-0.00326197170656146,0.140399251085937));
#59910=DIRECTION('center_axis',(-0.11199737074419,-0.584827952230717,-0.803388358912434));
#59911=DIRECTION('ref_axis',(-0.992534547464178,0.0265489589715222,0.119039173668203));
#59912=DIRECTION('center_axis',(-0.146804992029651,-0.584827952231123,-0.79776222059228));
#59913=DIRECTION('ref_axis',(-0.987282060191029,0.0368858773761462,0.154640116642314));
#59914=DIRECTION('center_axis',(0.167084767814961,-0.572651970094166,0.802591054966034));
#59915=DIRECTION('ref_axis',(1.54173804028222E-16,-0.814034314661491,-0.580816782258912));
#59916=DIRECTION('center_axis',(0.528213161385387,-0.398672303295916,0.74970077412524));
#59917=DIRECTION('ref_axis',(0.817474789260215,5.18362180146966E-17,-0.575964381645226));
#59918=DIRECTION('center_axis',(-0.423504105258802,-0.584827952229492,-0.691824066594969));
#59919=DIRECTION('ref_axis',(-0.842104444509155,-0.0273514773890005,0.538620461199319));
#59920=DIRECTION('center_axis',(-0.393038908136311,-0.584827952230094,-0.709575001660411));
#59921=DIRECTION('ref_axis',(-0.860659495847695,-0.037683838783106,0.507784561110084));
#59922=DIRECTION('center_axis',(-0.423504105256182,-0.584827952229402,-0.69182406659665));
#59923=DIRECTION('ref_axis',(-0.853807898461964,0.00246180523642254,0.520582377764501));
#59924=DIRECTION('center_axis',(-0.39303890811573,-0.584827952229416,-0.709575001672369));
#59925=DIRECTION('ref_axis',(-0.871986552495883,-0.00784651557689437,0.489466939087459));
#59926=DIRECTION('center_axis',(-0.423504105251284,-0.584827952229727,-0.691824066599373));
#59927=DIRECTION('ref_axis',(-0.864361613491274,0.0322834340843171,0.501833419579131));
#59928=DIRECTION('center_axis',(-0.393038908128715,-0.584827952229044,-0.709575001665483));
#59929=DIRECTION('ref_axis',(-0.88211923155341,0.0219588922046995,0.470514046949466));
#59930=DIRECTION('center_axis',(-0.245633509582242,-0.584827952229828,-0.773072082836379));
#59931=DIRECTION('ref_axis',(-0.939541817367972,-0.0526562713714979,0.338361479045916));
#59932=DIRECTION('center_axis',(-0.24563350958476,-0.584827952229614,-0.773072082835741));
#59933=DIRECTION('ref_axis',(-0.947703703562037,-0.0227607290339116,0.31833887520792));
#59934=DIRECTION('center_axis',(-0.211805498835859,-0.584827952228281,-0.783016409122675));
#59935=DIRECTION('ref_axis',(-0.958275377229305,-0.033086909490308,0.283925268013282));
#59936=DIRECTION('center_axis',(-0.245633509587554,-0.584827952229358,-0.773072082835046));
#59937=DIRECTION('ref_axis',(-0.95455064829962,0.00704626726762763,0.297965450930756));
#59938=DIRECTION('center_axis',(-0.211805498854265,-0.584827952229578,-0.783016409116728));
#59939=DIRECTION('ref_axis',(-0.964685752555244,-0.00326197172903191,0.263383291720189));
#59940=DIRECTION('center_axis',(-0.211805498885655,-0.584827952229335,-0.783016409108418));
#59941=DIRECTION('ref_axis',(-0.969788551538211,0.0265489589902435,0.242498078511879));
#59942=DIRECTION('center_axis',(-0.245633509521976,-0.584827952232075,-0.773072082853827));
#59943=DIRECTION('ref_axis',(-0.960115500406961,0.0368858773645434,0.277159986162033));
#59944=DIRECTION('center_axis',(0.266358586659695,-0.572651970087279,0.775321110552143));
#59945=DIRECTION('ref_axis',(1.19124006870652E-16,-0.804380141087925,-0.594114962463807));
#59946=DIRECTION('center_axis',(0.61801046506436,-0.39867230329826,0.677586496068062));
#59947=DIRECTION('ref_axis',(0.738841278009524,-2.52796011405891E-16,-0.673879489159044));
#59948=DIRECTION('center_axis',(-0.506873196214637,-0.584827952229441,-0.633289688255127));
#59949=DIRECTION('ref_axis',(-0.76795715537621,-0.0273514773915847,0.639916951010815));
#59950=DIRECTION('center_axis',(-0.47887300834826,-0.584827952229484,-0.654718953572108));
#59951=DIRECTION('ref_axis',(-0.790230657668672,-0.037683838795387,0.611649765776283));
#59952=DIRECTION('center_axis',(-0.506873196222743,-0.584827952229388,-0.633289688248689));
#59953=DIRECTION('ref_axis',(-0.781829095416187,0.00246180524143953,0.623487934988048));
#59954=DIRECTION('center_axis',(-0.478873008346566,-0.584827952229558,-0.654718953573281));
#59955=DIRECTION('ref_axis',(-0.803764203880813,-0.0078465155765271,0.594896240325278));
#59956=DIRECTION('center_axis',(-0.506873196212754,-0.584827952229607,-0.633289688256482));
#59957=DIRECTION('ref_axis',(-0.794649458809219,0.032283434085324,0.606209549164209));
#59958=DIRECTION('center_axis',(-0.478873008327432,-0.584827952230354,-0.654718953586565));
#59959=DIRECTION('ref_axis',(-0.816192411012875,0.0219588921831804,0.5773627588086));
#59960=DIRECTION('center_axis',(-0.340588239910082,-0.584827952229608,-0.736190136531233));
#59961=DIRECTION('ref_axis',(-0.889725311228872,-0.0526562713729305,0.453449211757819));
#59962=DIRECTION('center_axis',(-0.340588239919936,-0.584827952229746,-0.736190136526565));
#59963=DIRECTION('ref_axis',(-0.900332336193019,-0.0227607290304719,0.434607447726361));
#59964=DIRECTION('center_axis',(-0.308273327736802,-0.584827952229275,-0.750295822790845));
#59965=DIRECTION('ref_axis',(-0.915133817714972,-0.0330869094691202,0.401790184171045));
#59966=DIRECTION('center_axis',(-0.340588239870387,-0.584827952230211,-0.736190136549119));
#59967=DIRECTION('ref_axis',(-0.909678757889288,0.00704626723776923,0.415252823666518));
#59968=DIRECTION('center_axis',(-0.308273327748204,-0.584827952229549,-0.750295822785946));
#59969=DIRECTION('ref_axis',(-0.924068237631525,-0.00326197171192395,0.382213620559391));
#59970=DIRECTION('center_axis',(-0.308273327756411,-0.584827952229156,-0.750295822782881));
#59971=DIRECTION('ref_axis',(-0.931748410832772,0.0265489589935049,0.362132643774301));
#59972=DIRECTION('center_axis',(-0.340588239917826,-0.584827952229112,-0.736190136528045));
#59973=DIRECTION('ref_axis',(-0.917807345609863,0.0368858774046296,0.395308877199423));
#59974=DIRECTION('center_axis',(0.361431771479317,-0.572651970079971,0.735823889071869));
#59975=DIRECTION('ref_axis',(-1.63914301419145E-16,-0.789173129058311,-0.61417080065102));
#59976=DIRECTION('center_axis',(0.698061374528685,-0.398672303296788,0.594786274198688));
#59977=DIRECTION('ref_axis',(0.648555798442348,-1.26241681070733E-16,-0.76116711457262));
#59978=DIRECTION('center_axis',(-0.582248594085411,-0.584827952229698,-0.564767953212982));
#59979=DIRECTION('ref_axis',(-0.6816987231398,-0.0273514773860545,0.731121568245916));
#59980=DIRECTION('center_axis',(-0.557154995166819,-0.584827952229244,-0.589537596470328));
#59981=DIRECTION('ref_axis',(-0.707339409953029,-0.0376838387996158,0.705868888265112));
#59982=DIRECTION('center_axis',(-0.582248594079238,-0.584827952229526,-0.564767953219524));
#59983=DIRECTION('ref_axis',(-0.697520380503128,0.00246180523609652,0.716560715011471));
#59984=DIRECTION('center_axis',(-0.557154995173368,-0.584827952229518,-0.589537596463867));
#59985=DIRECTION('ref_axis',(-0.72286601362311,-0.00784651557417456,0.690943672481324));
#59986=DIRECTION('center_axis',(-0.58224859407526,-0.584827952229825,-0.564767953223315));
#59987=DIRECTION('ref_axis',(-0.712405207463399,0.0322834340840874,0.701025392024262));
#59988=DIRECTION('center_axis',(-0.557154995166649,-0.58482795222981,-0.589537596469928));
#59989=DIRECTION('ref_axis',(-0.737393748555925,0.0219588921937242,0.675106115099149));
#59990=DIRECTION('center_axis',(-0.430171690231809,-0.584827952229279,-0.68769803199836));
#59991=DIRECTION('ref_axis',(-0.825877305438824,-0.0526562713780784,0.561385779518564));
#59992=DIRECTION('center_axis',(-0.430171690235322,-0.58482795222936,-0.687698031996093));
#59993=DIRECTION('ref_axis',(-0.838762190057943,-0.0227607290396216,0.544022001156927));
#59994=DIRECTION('center_axis',(-0.399879502055293,-0.584827952228838,-0.70574262314801));
#59995=DIRECTION('ref_axis',(-0.857560051235848,-0.033086909479653,0.513318629065277));
#59996=DIRECTION('center_axis',(-0.430171690229828,-0.584827952229611,-0.687698031999316));
#59997=DIRECTION('ref_axis',(-0.850460690024639,0.00704626725670269,0.525991411375283));
#59998=DIRECTION('center_axis',(-0.399879502057685,-0.584827952229754,-0.705742623145897));
#59999=DIRECTION('ref_axis',(-0.868877614606056,-0.00326197172774871,0.495016212236466));
#60000=DIRECTION('center_axis',(-0.399879502062724,-0.584827952230319,-0.705742623142573));
#60001=DIRECTION('ref_axis',(-0.879014041102351,0.0265489589760492,0.476056160890921));
#60002=DIRECTION('center_axis',(-0.430171690221956,-0.584827952230244,-0.687698032003702));
#60003=DIRECTION('ref_axis',(-0.861024820730134,0.0368858773879713,0.50722351102444));
#60004=DIRECTION('center_axis',(-0.648441583796989,-0.58482795222928,-0.487339490185394));
#60005=DIRECTION('ref_axis',(-0.584689494821897,-0.0273514773918109,0.810795961589228));
#60006=DIRECTION('center_axis',(-0.626650314901459,-0.584827952229821,-0.515058879279423));
#60007=DIRECTION('ref_axis',(-0.613292997182075,-0.0376838387884075,0.788956036735632));
#60008=DIRECTION('center_axis',(0.450804961350449,-0.572651970056101,0.684722285319155));
#60009=DIRECTION('ref_axis',(1.61865499994955E-17,-0.767090570538598,-0.641538819239155));
#60010=DIRECTION('center_axis',(0.767103439114685,-0.398672303296782,0.502605917476567));
#60011=DIRECTION('ref_axis',(0.548042206505212,9.68883205373909E-18,-0.836450679890272));
#60012=DIRECTION('center_axis',(-0.648441583787969,-0.584827952229667,-0.487339490196932));
#60013=DIRECTION('ref_axis',(-0.602211352514835,0.0024618052280988,0.798332904506179));
#60014=DIRECTION('center_axis',(-0.626650314887279,-0.584827952229558,-0.515058879296975));
#60015=DIRECTION('ref_axis',(-0.630567794520706,-0.00784651558099585,0.776094510163891));
#60016=DIRECTION('center_axis',(-0.648441583795828,-0.584827952229534,-0.487339490186635));
#60017=DIRECTION('ref_axis',(-0.618925900421077,0.0322834340867861,0.784785645683918));
#60018=DIRECTION('center_axis',(-0.626650314895806,-0.584827952229403,-0.515058879286777));
#60019=DIRECTION('ref_axis',(-0.646965946188594,0.0219588921995646,0.762202644659322));
#60020=DIRECTION('center_axis',(-0.512971076047556,-0.584827952230014,-0.628360518674639));
#60021=DIRECTION('ref_axis',(-0.749004721174768,-0.0526562713680577,0.66046895819828));
#60022=DIRECTION('center_axis',(-0.512971076038393,-0.584827952229598,-0.628360518682507));
#60023=DIRECTION('ref_axis',(-0.763964263127642,-0.0227607290387081,0.644857002658314));
#60024=DIRECTION('center_axis',(-0.48517933779571,-0.584827952229707,-0.65005944071825));
#60025=DIRECTION('ref_axis',(-0.786462050443622,-0.0330869094583757,0.616751732575197));
#60026=DIRECTION('center_axis',(-0.512971076036445,-0.584827952229604,-0.628360518684092));
#60027=DIRECTION('ref_axis',(-0.777830349046253,0.00704626725964967,0.628434800293785));
#60028=DIRECTION('center_axis',(-0.485179337811888,-0.584827952229374,-0.650059440706475));
#60029=DIRECTION('ref_axis',(-0.79998427252114,-0.00326197169693252,0.600012102594165));
#60030=DIRECTION('center_axis',(-0.485179337790077,-0.584827952229588,-0.650059440722562));
#60031=DIRECTION('ref_axis',(-0.812417094826833,0.0265489589879128,0.58247198800439));
#60032=DIRECTION('center_axis',(-0.512971076046306,-0.584827952229162,-0.628360518676453));
#60033=DIRECTION('ref_axis',(-0.790663420052944,0.0368858774035164,0.611138927117521));
#60034=DIRECTION('center_axis',(0.533068687695702,-0.572651970066448,0.622822202058821));
#60035=DIRECTION('ref_axis',(-4.08993525798431E-16,-0.736133834920939,-0.676836004571707));
#60036=DIRECTION('center_axis',(0.824047824221018,-0.398672303295535,0.402499165193716));
#60037=DIRECTION('ref_axis',(0.438885661586792,-5.28466665497678E-17,-0.898542918314715));
#60038=DIRECTION('center_axis',(-0.704408262376733,-0.584827952229495,-0.402225392269618));
#60039=DIRECTION('ref_axis',(-0.478459363891251,-0.027351477390948,0.877683618275579));
#60040=DIRECTION('center_axis',(-0.686262984817355,-0.58482795222998,-0.432457375888148));
#60041=DIRECTION('ref_axis',(-0.509574587487999,-0.0376838387835741,0.859600877198813));
#60042=DIRECTION('center_axis',(-0.704408262374728,-0.584827952229583,-0.402225392273001));
#60043=DIRECTION('ref_axis',(-0.497405091738635,0.00246180523382742,0.867514907207634));
#60044=DIRECTION('center_axis',(-0.686262984804124,-0.584827952229589,-0.432457375909674));
#60045=DIRECTION('ref_axis',(-0.52832514460542,-0.00784651557794266,0.849005873814161));
#60046=DIRECTION('center_axis',(-0.704408262374556,-0.584827952229765,-0.402225392273037));
#60047=DIRECTION('ref_axis',(-0.515685762205737,0.0322834340851159,0.856169360898859));
#60048=DIRECTION('center_axis',(-0.686262984807675,-0.584827952229569,-0.432457375904064));
#60049=DIRECTION('ref_axis',(-0.546335104378128,0.0219588921989141,0.837278783188453));
#60050=DIRECTION('center_axis',(-0.587680601548565,-0.584827952230265,-0.559113384613239));
#60051=DIRECTION('ref_axis',(-0.660319885028862,-0.0526562713654081,0.749136146852736));
#60052=DIRECTION('center_axis',(-0.587680601532822,-0.58482795222935,-0.559113384630743));
#60053=DIRECTION('ref_axis',(-0.677118163401999,-0.0227607290428999,0.735522224004509));
#60054=DIRECTION('center_axis',(-0.56282760550518,-0.584827952229442,-0.584124432610402));
#60055=DIRECTION('ref_axis',(-0.702961073329084,-0.033086909466746,0.710458292798361));
#60056=DIRECTION('center_axis',(-0.587680601533554,-0.58482795222962,-0.559113384629692));
#60057=DIRECTION('ref_axis',(-0.692933158813929,0.00704626725769116,0.720967396997869));
#60058=DIRECTION('center_axis',(-0.562827605502354,-0.584827952229588,-0.584124432612979));
#60059=DIRECTION('ref_axis',(-0.718474700614503,-0.0032619717187004,0.695545443603368));
#60060=DIRECTION('center_axis',(-0.562827605517478,-0.584827952229182,-0.584124432598812));
#60061=DIRECTION('ref_axis',(-0.733007845654138,0.0265489589933554,0.679701883906355));
#60062=DIRECTION('center_axis',(-0.587680601554992,-0.584827952228574,-0.559113384608252));
#60063=DIRECTION('ref_axis',(-0.707832784924696,0.0368858774120165,0.705416317243438));
#60064=DIRECTION('center_axis',(0.60692560239257,-0.572651970058496,0.551099840635561));
#60065=DIRECTION('ref_axis',(0.686271561903148,0.727345408539171,-3.55494846067791E-17));
#60066=DIRECTION('center_axis',(0.867996482877091,-0.398672303294177,0.296044760634463));
#60067=DIRECTION('ref_axis',(0.417381833065828,0.908731206367763,3.03903854002256E-16));
#60068=DIRECTION('center_axis',(-0.749266001865758,-0.584827952229527,-0.3107679596405));
#60069=DIRECTION('ref_axis',(-0.364683642974061,-0.0273514773913525,0.930729679999342));
#60070=DIRECTION('center_axis',(-0.73505287749892,-0.5848279522297,-0.343035761359327));
#60071=DIRECTION('ref_axis',(-0.397819882158354,-0.0376838387908347,0.916689298319501));
#60072=DIRECTION('center_axis',(-0.74926600186879,-0.584827952229442,-0.31076795963335));
#60073=DIRECTION('ref_axis',(-0.38475445552896,0.00246180524003201,0.923015681592449));
#60074=DIRECTION('center_axis',(-0.735052877495005,-0.584827952229528,-0.343035761368011));
#60075=DIRECTION('ref_axis',(-0.417750490545346,-0.00784651710898623,0.908527908112008));
#60076=DIRECTION('center_axis',(-0.74926600186846,-0.584827952229323,-0.31076795963437));
#60077=DIRECTION('ref_axis',(-0.404312951455422,0.0322834340908156,0.91405077384613));
#60078=DIRECTION('center_axis',(-0.735052877496047,-0.584827952229571,-0.343035761365705));
#60079=DIRECTION('ref_axis',(-0.437088231606847,0.0219588921987504,0.89915053514092));
#60080=DIRECTION('center_axis',(-0.653122052884241,-0.584827952229301,-0.481048698498975));
#60081=DIRECTION('ref_axis',(-0.561221409856519,-0.0526562713777249,0.825989010945821));
#60082=DIRECTION('center_axis',(-0.653122052875048,-0.584827952229324,-0.481048698511428));
#60083=DIRECTION('ref_axis',(-0.57959350575428,-0.0227607290501129,0.814587820496091));
#60084=DIRECTION('center_axis',(-0.631599745679082,-0.584827952229646,-0.508977433241395));
#60085=DIRECTION('ref_axis',(-0.608373980143524,-0.0330869094586271,0.792960501353506));
#60086=DIRECTION('center_axis',(-0.653122052875627,-0.584827952229884,-0.481048698509961));
#60087=DIRECTION('ref_axis',(-0.597107998736065,0.0070462672503748,0.802129907161706));
#60088=DIRECTION('center_axis',(-0.631599745672695,-0.584827952229487,-0.508977433249503));
#60089=DIRECTION('ref_axis',(-0.62563435345937,-0.00326197171456914,0.780109617497445));
#60090=DIRECTION('center_axis',(-0.631599745668354,-0.584827952229863,-0.508977433254457));
#60091=DIRECTION('ref_axis',(-0.642038624895127,0.0265489589821433,0.766212475048363));
#60092=DIRECTION('center_axis',(-0.653122052893968,-0.584827952229045,-0.481048698486079));
#60093=DIRECTION('ref_axis',(-0.613839203955641,0.0368858774042529,0.788568870635421));
#60094=DIRECTION('center_axis',(0.67121093778181,-0.572651970054142,0.470686305510552));
#60095=DIRECTION('ref_axis',(0.649044045242262,0.760750831307834,-7.92593106383196E-16));
#60096=DIRECTION('center_axis',(0.898256318482264,-0.398672303292889,0.184921553351231));
#60097=DIRECTION('ref_axis',(0.405668756739668,0.914020163784854,4.40549150587367E-17));
#60098=DIRECTION('center_axis',(-0.782307368915369,-0.584827952229426,-0.214409530646024));
#60099=DIRECTION('ref_axis',(-0.245156643157368,-0.0273514773927631,0.969097578678352));
#60100=DIRECTION('center_axis',(-0.772250547206547,-0.584827952229391,-0.248204267953567));
#60101=DIRECTION('ref_axis',(-0.279791319640618,-0.0376838387967089,0.959320981604856));
#60102=DIRECTION('center_axis',(-0.782307368914677,-0.584827952229587,-0.214409530648112));
#60103=DIRECTION('ref_axis',(-0.266036011731999,0.00246180523244144,0.963959947288646));
#60104=DIRECTION('center_axis',(-0.772250547207055,-0.584827952229545,-0.248204267951624));
#60105=DIRECTION('ref_axis',(-0.300587663701301,-0.00784651557541538,0.953721913675007));
#60106=DIRECTION('center_axis',(-0.782307368917322,-0.584827952229332,-0.214409530639156));
#60107=DIRECTION('ref_axis',(-0.286563883944476,0.0322834340891994,0.957517060057974));
#60108=DIRECTION('center_axis',(-0.772250547207065,-0.584827952229574,-0.248204267951522));
#60109=DIRECTION('ref_axis',(-0.320948216319338,0.0219588921977076,0.946842146027988));
#60110=DIRECTION('center_axis',(-0.708263379304496,-0.58482795222933,-0.395397587027824));
#60111=DIRECTION('ref_axis',(-0.453272137779791,-0.0526562713770493,0.889815534926877));
#60112=DIRECTION('center_axis',(-0.708263379298612,-0.584827952229271,-0.395397587038451));
#60113=DIRECTION('ref_axis',(-0.472928312276866,-0.0227607290478678,0.880806880456871));
#60114=DIRECTION('center_axis',(-0.690411180541906,-0.584827952229035,-0.425803555732365));
#60115=DIRECTION('ref_axis',(-0.504192465890993,-0.0330869094722355,0.862957249091944));
#60116=DIRECTION('center_axis',(-0.708263379302418,-0.584827952229702,-0.395397587030994));
#60117=DIRECTION('ref_axis',(-0.491866088807356,0.00704626725721685,0.870642349532283));
#60118=DIRECTION('center_axis',(-0.690411180544678,-0.584827952229611,-0.42580355572708));
#60119=DIRECTION('ref_axis',(-0.522927378824416,-0.00326197171863667,0.852370996700576));
#60120=DIRECTION('center_axis',(-0.690411180551283,-0.584827952229555,-0.425803555716447));
#60121=DIRECTION('ref_axis',(-0.540944071467078,0.0265489589886524,0.840639437762255));
#60122=DIRECTION('center_axis',(-0.708263379298778,-0.58482795223008,-0.395397587036955));
#60123=DIRECTION('ref_axis',(-0.510165012061082,0.0368858773894978,0.859285221866362));
#60124=DIRECTION('center_axis',(0.724910875721522,-0.572651970049502,0.38284976617347));
#60125=DIRECTION('ref_axis',(0.619880264804866,0.784696410916635,-2.87690912095748E-16));
#60126=DIRECTION('center_axis',(0.914350115353379,-0.398672303289966,0.0708820227048915));
#60127=DIRECTION('ref_axis',(0.399677609953492,0.916655774051451,9.93161652328719E-17));
#60128=DIRECTION('center_axis',(-0.803011281431714,-0.5848279522296,-0.114669735258827));
#60129=DIRECTION('ref_axis',(-0.12176337661821,-0.0273514773873073,0.992182229632875));
#60130=DIRECTION('center_axis',(-0.797269364471594,-0.584827952229905,-0.149458444945867));
#60131=DIRECTION('ref_axis',(-0.157350280851449,-0.0376838387869603,0.986823599945932));
#60132=DIRECTION('center_axis',(-0.803011281430099,-0.584827952229649,-0.114669735269889));
#60133=DIRECTION('ref_axis',(-0.143122021097682,0.00246180523301818,0.989701988778395));
#60134=DIRECTION('center_axis',(-0.79726936446997,-0.584827952229467,-0.149458444956243));
#60135=DIRECTION('ref_axis',(-0.178684388826315,-0.00784651557285187,0.983875155384631));
#60136=DIRECTION('center_axis',(-0.803011281431542,-0.584827952229375,-0.114669735261181));
#60137=DIRECTION('ref_axis',(-0.164295532796555,0.0322834340889757,0.985882730240529));
#60138=DIRECTION('center_axis',(-0.797269364469036,-0.58482795222959,-0.149458444960745));
#60139=DIRECTION('ref_axis',(-0.199746655934583,0.0219588921973963,0.979601490656488));
#60140=DIRECTION('center_axis',(-0.75223496913832,-0.584827952229617,-0.303510819405804));
#60141=DIRECTION('ref_axis',(-0.338174493315121,-0.0526562713737487,0.939609136373245));
#60142=DIRECTION('center_axis',(-0.752234969135657,-0.584827952229478,-0.303510819412674));
#60143=DIRECTION('ref_axis',(-0.35880475679657,-0.0227607290416326,0.933135089745128));
#60144=DIRECTION('center_axis',(-0.738334418673682,-0.584827952229299,-0.335914501760613));
#60145=DIRECTION('ref_axis',(-0.392059535240024,-0.0330869094679849,0.919344645521598));
#60146=DIRECTION('center_axis',(-0.752234969136256,-0.584827952229545,-0.303510819411061));
#60147=DIRECTION('ref_axis',(-0.378867156835913,0.00704626725925369,0.925424241950027));
#60148=DIRECTION('center_axis',(-0.738334418678639,-0.584827952229531,-0.335914501749314));
#60149=DIRECTION('ref_axis',(-0.411973527028004,-0.00326197171058358,0.911189976112921));
#60150=DIRECTION('center_axis',(-0.738334418681027,-0.584827952229172,-0.335914501744689));
#60151=DIRECTION('ref_axis',(-0.431318506889835,0.0265489589925769,0.901809014365422));
#60152=DIRECTION('center_axis',(-0.752234969138981,-0.58482795222936,-0.303510819404664));
#60153=DIRECTION('ref_axis',(-0.398445213138042,0.0368858773996949,0.916450131854339));
#60154=DIRECTION('center_axis',(0.767178536111651,-0.572651970044602,0.288975457320548));
#60155=DIRECTION('ref_axis',(0.598172081248193,0.801367681663795,-4.17053780108495E-16));
#60156=DIRECTION('center_axis',(0.916024064699777,-0.398672303285569,-0.0442753597825917));
#60157=DIRECTION('ref_axis',(0.399063638883099,0.916923231312949,8.19224667888075E-18));
#60158=DIRECTION('center_axis',(-0.811051226341668,-0.584827952229427,-0.0131215296673966));
#60159=DIRECTION('ref_axis',(0.0035501710909852,-0.0273514773944228,0.99961957412286));
#60160=DIRECTION('center_axis',(-0.809714767588102,-0.58482795222959,-0.0483555730055123));
#60161=DIRECTION('ref_axis',(-0.0324277341580232,-0.0376838387929533,0.998763420611309));
#60162=DIRECTION('center_axis',(-0.811051226342032,-0.584827952229353,-0.0131215296481657));
#60163=DIRECTION('ref_axis',(-0.0179509106794282,0.00246180524443599,0.99983583868589));
#60164=DIRECTION('center_axis',(-0.809714767588315,-0.584827952229458,-0.0483555730035268));
#60165=DIRECTION('ref_axis',(-0.0539631543998079,-0.00784651557187224,0.99851209815435));
#60166=DIRECTION('center_axis',(-0.811051226341268,-0.584827952229893,-0.0131215296713105));
#60167=DIRECTION('ref_axis',(-0.0394361429627812,0.0322834340818623,0.998700440829031));
#60168=DIRECTION('center_axis',(-0.809714767588765,-0.58482795222925,-0.0483555729985027));
#60169=DIRECTION('ref_axis',(-0.0753949714532756,0.0219588922048596,0.996911934592367));
#60170=DIRECTION('center_axis',(-0.784343364140843,-0.584827952229176,-0.206837504867116));
#60171=DIRECTION('ref_axis',(-0.217743635086438,-0.0526562713790471,0.974584540439566));
#60172=DIRECTION('center_axis',(-0.784343364142726,-0.58482795222944,-0.206837504859228));
#60173=DIRECTION('ref_axis',(-0.239022635964213,-0.0227607290381041,0.970747201237466));
#60174=DIRECTION('center_axis',(-0.7746136819609,-0.584827952229385,-0.240727875432328));
#60175=DIRECTION('ref_axis',(-0.273743591514971,-0.0330869094649303,0.961233427699299));
#60176=DIRECTION('center_axis',(-0.784343364141514,-0.58482795222953,-0.20683750486357));
#60177=DIRECTION('ref_axis',(-0.259893263479541,0.00704626725925445,0.96561164124904));
#60178=DIRECTION('center_axis',(-0.774613681957867,-0.584827952229589,-0.240727875441592));
#60179=DIRECTION('ref_axis',(-0.29452260663248,-0.00326197172036406,0.955638945273216));
#60180=DIRECTION('center_axis',(-0.774613681963109,-0.584827952229387,-0.240727875425216));
#60181=DIRECTION('ref_axis',(-0.314890791810213,0.0265489589893783,0.948756524093362));
#60182=DIRECTION('center_axis',(-0.784343364140797,-0.584827952229724,-0.206837504865741));
#60183=DIRECTION('ref_axis',(-0.280441695204173,0.0368858773946116,0.959162075793158));
#60184=DIRECTION('center_axis',(0.797347332705084,-0.572651970025819,0.190543832893213));
#60185=DIRECTION('ref_axis',(0.583339514902054,0.812228422522775,1.92994765983885E-17));
#60186=DIRECTION('center_axis',(0.903251767338709,-0.398672303283214,-0.158734493398112));
#60187=DIRECTION('ref_axis',(0.40379185681366,0.91485088204088,-1.37857755134463E-16));
#60188=DIRECTION('center_axis',(-0.806300408914473,-0.584827952229552,0.0886336103029912));
#60189=DIRECTION('ref_axis',(0.128807730495229,-0.0273514773905314,0.991292320785965));
#60190=DIRECTION('center_axis',(-0.809390485121178,-0.584827952229607,0.0535098952178855));
#60191=DIRECTION('ref_axis',(0.0930062172828468,-0.0376838387925279,0.994952145502785));
#60192=DIRECTION('center_axis',(-0.806300408913409,-0.584827952229407,0.0886336103136302));
#60193=DIRECTION('ref_axis',(0.107503296306928,0.0024618052430626,0.99420168014246));
#60194=DIRECTION('center_axis',(-0.809390485121514,-0.584827952229481,0.0535098952141856));
#60195=DIRECTION('ref_axis',(0.0716091112012576,-0.00784651557490987,0.997401908653828));
#60196=DIRECTION('center_axis',(-0.806300408914069,-0.584827952229266,0.0886336103085555));
#60197=DIRECTION('ref_axis',(0.0860451784273227,0.0322834340909248,0.995768048871175));
#60198=DIRECTION('center_axis',(-0.809390485121174,-0.58482795222938,0.0535098952204267));
#60199=DIRECTION('ref_axis',(0.0501457366864746,0.0219588922963099,0.998500481793219));
#60200=DIRECTION('center_axis',(-0.804082195749635,-0.584827952229121,-0.106902239312084));
#60201=DIRECTION('ref_axis',(-0.093878829653998,-0.0526562713806529,0.994190164117048));
#60202=DIRECTION('center_axis',(-0.804082195750617,-0.584827952229495,-0.10690223930266));
#60203=DIRECTION('ref_axis',(-0.115470985383714,-0.0227607290386235,0.993050049467873));
#60204=DIRECTION('center_axis',(-0.798676824748701,-0.584827952229234,-0.141744826715803));
#60205=DIRECTION('ref_axis',(-0.15111054783433,-0.0330869094686492,0.987962984506516));
#60206=DIRECTION('center_axis',(-0.804082195750302,-0.584827952229587,-0.106902239304525));
#60207=DIRECTION('ref_axis',(-0.136820698104582,0.00704626726004378,0.990570768137176));
#60208=DIRECTION('center_axis',(-0.798676824749339,-0.584827952229491,-0.14174482671115));
#60209=DIRECTION('ref_axis',(-0.172426888771917,-0.0032619717161641,0.985016917402417));
#60210=DIRECTION('center_axis',(-0.798676824749257,-0.584827952229734,-0.141744826710606));
#60211=DIRECTION('ref_axis',(-0.193497060841072,0.0265489589847928,0.980741576676899));
#60212=DIRECTION('center_axis',(-0.804082195752222,-0.584827952229105,-0.10690223929272));
#60213=DIRECTION('ref_axis',(-0.158015444189677,0.0368858774036313,0.986747460825567));
#63522=CARTESIAN_POINT('',(0.,0.,0.));
#63523=CARTESIAN_POINT('Origin',(0.00812378219310841,-0.0355241814719619,
0.07415));
#63524=CARTESIAN_POINT('',(0.00962378219312842,-0.0201741814719718,0.07415000000001));
#63525=CARTESIAN_POINT('Origin',(0.00812378219311841,-0.0201741814719718,
0.07415000000001));
#63526=CARTESIAN_POINT('',(0.00962378219312842,-0.0315241814719718,0.07415000000001));
#63527=CARTESIAN_POINT('',(0.00962378219310841,-0.0355241814719619,0.07415));
#63528=CARTESIAN_POINT('Origin',(0.00812378219311841,-0.0315241814719718,
0.07415000000001));
#63529=CARTESIAN_POINT('Origin',(0.00812378219310841,-0.0320241814719619,
0.07415));
#63530=CARTESIAN_POINT('',(0.00800089067195264,-0.0317744765475852,0.0798989817472979));
#63531=CARTESIAN_POINT('',(0.00812378219307299,-0.031774544307656,0.0799003628356941));
#63532=CARTESIAN_POINT('Ctrl Pts',(0.00812378219303757,-0.031774544307656,
0.0799003628356941));
#63533=CARTESIAN_POINT('Ctrl Pts',(0.00811348867094932,-0.0317744296023842,
0.0799002481304222));
#63534=CARTESIAN_POINT('Ctrl Pts',(0.00810319488311751,-0.0317743418685778,
0.0799001327570061));
#63535=CARTESIAN_POINT('Ctrl Pts',(0.00806223108536668,-0.0317741013472404,
0.0798996722309655));
#63536=CARTESIAN_POINT('Ctrl Pts',(0.00803155944442365,-0.031774163538908,
0.0798993242496632));
#63537=CARTESIAN_POINT('Ctrl Pts',(0.00800089067195264,-0.0317744765475852,
0.079898981747298));
#63538=CARTESIAN_POINT('',(0.00812378219310841,-0.0315241814719669,0.0796500000000049));
#63539=CARTESIAN_POINT('',(0.00812378219310841,-0.0320241814719619,0.08015));
#63540=CARTESIAN_POINT('Origin',(0.00812378219311841,-0.0315241814719718,
0.07415000000001));
#63541=CARTESIAN_POINT('',(0.00818490370815573,-0.0317755400071256,0.0799010337471101));
#63542=CARTESIAN_POINT('Ctrl Pts',(0.00818490370815573,-0.0317755400071257,
0.0799010337471101));
#63543=CARTESIAN_POINT('Ctrl Pts',(0.00816453180595947,-0.0317751040881875,
0.0799008143144595));
#63544=CARTESIAN_POINT('Ctrl Pts',(0.0081441575200755,-0.0317747713589418,
0.0799005898869801));
#63545=CARTESIAN_POINT('Ctrl Pts',(0.00812378219303757,-0.031774544307656,
0.0799003628356941));
#63546=CARTESIAN_POINT('',(0.00836641386969367,-0.0318824481878403,0.0800032400262193));
#63547=CARTESIAN_POINT('Origin',(0.0125782760148201,-0.0332583300628553,
0.0708159433682903));
#63548=CARTESIAN_POINT('',(0.00853918443652277,-0.0317755397360895,0.0798863371607593));
#63549=CARTESIAN_POINT('Origin',(0.00345819158879964,-0.0326853491204495,
0.0717801654791084));
#63550=CARTESIAN_POINT('',(0.00872239818039313,-0.0317744765475852,0.0798690517008071));
#63551=CARTESIAN_POINT('Ctrl Pts',(0.00853918446518101,-0.0317755400678203,
0.0798863373898779));
#63552=CARTESIAN_POINT('Ctrl Pts',(0.00856971630102154,-0.0317748838920054,
0.0798834685041633));
#63553=CARTESIAN_POINT('Ctrl Pts',(0.00860025258788743,-0.0317744615155934,
0.0798805878692076));
#63554=CARTESIAN_POINT('Ctrl Pts',(0.00866132551949298,-0.0317741013465794,
0.079874820213224));
#63555=CARTESIAN_POINT('Ctrl Pts',(0.00869186305200621,-0.0317741635377597,
0.0798719331080806));
#63556=CARTESIAN_POINT('Ctrl Pts',(0.00872239818037093,-0.0317744765473203,
0.0798690517005431));
#63557=CARTESIAN_POINT('',(0.00890521740261619,-0.0317755400071256,0.0798480245711424));
#63558=CARTESIAN_POINT('Ctrl Pts',(0.00872239818039312,-0.0317744765475851,
0.079869051700807));
#63559=CARTESIAN_POINT('Ctrl Pts',(0.00875287145286697,-0.0317741635039241,
0.0798655472943847));
#63560=CARTESIAN_POINT('Ctrl Pts',(0.00878333832390794,-0.0317741013272851,
0.0798620491063663));
#63561=CARTESIAN_POINT('Ctrl Pts',(0.00884428421652555,-0.0317744615102831,
0.0798550449672046));
#63562=CARTESIAN_POINT('Ctrl Pts',(0.00887475419897025,-0.0317748838659619,
0.0798515400556039));
#63563=CARTESIAN_POINT('Ctrl Pts',(0.00890521740261618,-0.0317755400071256,
0.0798480245711423));
#63564=CARTESIAN_POINT('',(0.00909810614576694,-0.0318824481878404,0.0799266756677436));
#63565=CARTESIAN_POINT('Origin',(0.0121252829034405,-0.0332583300636472,
0.070283937281488));
#63566=CARTESIAN_POINT('',(0.00925486255046764,-0.0317755397364823,0.0797890407230367));
#63567=CARTESIAN_POINT('Origin',(0.00319796214065289,-0.0326853491204372,
0.0723836058889708));
#63568=CARTESIAN_POINT('',(0.0094344651571187,-0.0317744765475852,0.0797489287925986));
#63569=CARTESIAN_POINT('Ctrl Pts',(0.00925486260762856,-0.0317755400683138,
0.0797890409468029));
#63570=CARTESIAN_POINT('Ctrl Pts',(0.00928479412963376,-0.0317748838922174,
0.0797823680280026));
#63571=CARTESIAN_POINT('Ctrl Pts',(0.00931472858696256,-0.0317744615158803,
0.0797756828966261));
#63572=CARTESIAN_POINT('Ctrl Pts',(0.00937459705300773,-0.0317741013468556,
0.0797623062541212));
#63573=CARTESIAN_POINT('Ctrl Pts',(0.00940453194095072,-0.0317741635379398,
0.0797556145462587));
#63574=CARTESIAN_POINT('Ctrl Pts',(0.00943446515711872,-0.0317744765475852,
0.0797489287925987));
#63575=CARTESIAN_POINT('',(0.00961320739701597,-0.0317755400071255,0.0797051541438529));
#63576=CARTESIAN_POINT('Ctrl Pts',(0.00943446515711872,-0.0317744765475852,
0.0797489287925987));
#63577=CARTESIAN_POINT('Ctrl Pts',(0.00946425568272709,-0.0317741635379398,
0.0797416334984917));
#63578=CARTESIAN_POINT('Ctrl Pts',(0.00949405034927215,-0.0317741013468556,
0.0797343427978588));
#63579=CARTESIAN_POINT('Ctrl Pts',(0.00955363457623872,-0.0317744615102831,
0.079719756135239));
#63580=CARTESIAN_POINT('Ctrl Pts',(0.0095834250118687,-0.0317748838659621,
0.0797124599594862));
#63581=CARTESIAN_POINT('Ctrl Pts',(0.00961320739701597,-0.0317755400071257,
0.0797051541438529));
#63582=CARTESIAN_POINT('',(0.00981443275107406,-0.0318824481878406,0.0797590096831689));
#63583=CARTESIAN_POINT('Origin',(0.0116091837302405,-0.0332583300607984,
0.0698129013353744));
#63584=CARTESIAN_POINT('',(0.00995270285202925,-0.0317755397364837,0.0796028132440281));
#63585=CARTESIAN_POINT('Origin',(0.00301541581737871,-0.0326853491204465,
0.0730149033892818));
#63586=CARTESIAN_POINT('',(0.0101258618805387,-0.0317744765475852,0.0795405074326928));
#63587=CARTESIAN_POINT('Ctrl Pts',(0.00995270293678456,-0.0317755400683137,
0.0796028134588651));
#63588=CARTESIAN_POINT('Ctrl Pts',(0.00998156209550537,-0.0317748838923493,
0.0795924417456697));
#63589=CARTESIAN_POINT('Ctrl Pts',(0.0100104226445564,-0.0317744615158499,
0.0795820575451456));
#63590=CARTESIAN_POINT('Ctrl Pts',(0.0100681425004938,-0.0317741013467719,
0.079561282869969));
#63591=CARTESIAN_POINT('Ctrl Pts',(0.0100970026465938,-0.0317741635379696,
0.0795508920929727));
#63592=CARTESIAN_POINT('Ctrl Pts',(0.0101258618805387,-0.0317744765475852,
0.0795405074326928));
#63593=CARTESIAN_POINT('',(0.0102977082662106,-0.0317755400071256,0.0794746756172265));
#63594=CARTESIAN_POINT('Ctrl Pts',(0.0101258618805387,-0.0317744765475851,
0.0795405074326927));
#63595=CARTESIAN_POINT('Ctrl Pts',(0.0101545062686811,-0.0317741635039241,
0.0795295347289502));
#63596=CARTESIAN_POINT('Ctrl Pts',(0.0101831460029575,-0.031774101327285,
0.0795185696402207));
#63597=CARTESIAN_POINT('Ctrl Pts',(0.0102404353097176,-0.0317744615102831,
0.079496628921809));
#63598=CARTESIAN_POINT('Ctrl Pts',(0.0102690763855666,-0.0317748838659622,
0.0794856565469538));
#63599=CARTESIAN_POINT('Ctrl Pts',(0.0102977082662106,-0.0317755400071257,
0.0794746756172266));
#63600=CARTESIAN_POINT('',(0.0105040967871363,-0.0318824481878407,0.0795028862652307));
#63601=CARTESIAN_POINT('Origin',(0.0110381176980832,-0.0332583300612685,
0.0694102640075936));
#63602=CARTESIAN_POINT('',(0.0106216999825734,-0.0317755397360894,0.0793305916421598));
#63603=CARTESIAN_POINT('Origin',(0.00291343148364639,-0.0326853491206454,
0.0736641020412303));
#63604=CARTESIAN_POINT('',(0.0107856846113026,-0.0317744765475852,0.0792470745504406));
#63605=CARTESIAN_POINT('Ctrl Pts',(0.0106217000935633,-0.0317755400678203,
0.079330591844639));
#63606=CARTESIAN_POINT('Ctrl Pts',(0.0106490317714279,-0.0317748838919549,
0.0793166849026812));
#63607=CARTESIAN_POINT('Ctrl Pts',(0.0106763632593857,-0.0317744615156049,
0.0793027653996415));
#63608=CARTESIAN_POINT('Ctrl Pts',(0.0107310242162656,-0.0317741013466114,
0.0792749203246661));
#63609=CARTESIAN_POINT('Ctrl Pts',(0.0107583544827035,-0.0317741635377483,
0.0792609943461551));
#63610=CARTESIAN_POINT('Ctrl Pts',(0.0107856846111848,-0.0317744765473203,
0.0792470745502033));
#63611=CARTESIAN_POINT('',(0.010947925022592,-0.0317755400071255,0.0791602237753096));
#63612=CARTESIAN_POINT('Ctrl Pts',(0.0107856846113026,-0.0317744765475852,
0.0792470745504406));
#63613=CARTESIAN_POINT('Ctrl Pts',(0.0108127249443218,-0.0317741635379697,
0.079232599850341));
#63614=CARTESIAN_POINT('Ctrl Pts',(0.0108397704303659,-0.0317741013467719,
0.0792181285696829));
#63615=CARTESIAN_POINT('Ctrl Pts',(0.0108938551617572,-0.0317744615102529,
0.0791891821749494));
#63616=CARTESIAN_POINT('Ctrl Pts',(0.0109208951937506,-0.0317748838660943,
0.0791747066403946));
#63617=CARTESIAN_POINT('Ctrl Pts',(0.010947925022592,-0.0317755400071257,
0.0791602237753096));
#63618=CARTESIAN_POINT('',(0.0111562218401201,-0.031882448187841,0.0791623446332304));
#63619=CARTESIAN_POINT('Origin',(0.0104210908503211,-0.033258330069597,
0.0690823750888361));
#63620=CARTESIAN_POINT('',(0.0112513034569997,-0.0317755397360895,0.0789766690159622));
#63621=CARTESIAN_POINT('Origin',(0.00289361749240266,-0.0326853491202809,
0.0743209635941413));
#63622=CARTESIAN_POINT('',(0.0114035275507881,-0.0317744765475852,0.0788732577576833));
#63623=CARTESIAN_POINT('Ctrl Pts',(0.0112513035924919,-0.0317755400678203,
0.0789766692029341));
#63624=CARTESIAN_POINT('Ctrl Pts',(0.0112766767526801,-0.0317748838918833,
0.0789594463519205));
#63625=CARTESIAN_POINT('Ctrl Pts',(0.0113020481459377,-0.0317744615156214,
0.0789422110655245));
#63626=CARTESIAN_POINT('Ctrl Pts',(0.0113527909245682,-0.0317741013270863,
0.0789077328522199));
#63627=CARTESIAN_POINT('Ctrl Pts',(0.0113781547830805,-0.0317741635037164,
0.0788904950389542));
#63628=CARTESIAN_POINT('Ctrl Pts',(0.0114035275506415,-0.0317744765473203,
0.0788732577574627));
#63629=CARTESIAN_POINT('',(0.0115536033594913,-0.0317755400071255,0.0787667577114933));
#63630=CARTESIAN_POINT('Ctrl Pts',(0.0114035275507881,-0.0317744765475852,
0.0788732577576833));
#63631=CARTESIAN_POINT('Ctrl Pts',(0.0114285405028257,-0.031774163537956,
0.0788555081417705));
#63632=CARTESIAN_POINT('Ctrl Pts',(0.0114535589958953,-0.0317741013468101,
0.0788377612724408));
#63633=CARTESIAN_POINT('Ctrl Pts',(0.0115035893044095,-0.0317744615102667,
0.0788022645167903));
#63634=CARTESIAN_POINT('Ctrl Pts',(0.011528601850937,-0.0317748838660339,
0.0787845141123455));
#63635=CARTESIAN_POINT('Ctrl Pts',(0.0115536033594913,-0.0317755400071257,
0.0787667577114933));
#63636=CARTESIAN_POINT('',(0.0117605235083789,-0.0318824481878413,0.0787427553321347));
#63637=CARTESIAN_POINT('Origin',(0.00976783406872409,-0.0332583300697538,
0.0688344057025907));
#63638=CARTESIAN_POINT('',(0.0118315840528038,-0.0317755397360895,0.0785466269360707));
#63639=CARTESIAN_POINT('Origin',(0.00295628632343493,-0.0326853491203905,
0.0749751289491354));
#63640=CARTESIAN_POINT('',(0.0119696469467589,-0.0317744765475852,0.0784249523685494));
#63641=CARTESIAN_POINT('Ctrl Pts',(0.0118315842106613,-0.0317755400678203,
0.0785466271045866));
#63642=CARTESIAN_POINT('Ctrl Pts',(0.0118545986960121,-0.0317748838920054,
0.0785263599644561));
#63643=CARTESIAN_POINT('Ctrl Pts',(0.0118776098762876,-0.0317744615155934,
0.0785060807027428));
#63644=CARTESIAN_POINT('Ctrl Pts',(0.0119236287727241,-0.0317741013465795,
0.0784655168025234));
#63645=CARTESIAN_POINT('Ctrl Pts',(0.0119466371576691,-0.0317741635377597,
0.0784452315741446));
#63646=CARTESIAN_POINT('Ctrl Pts',(0.0119696469465858,-0.0317744765473203,
0.0784249523683489));
#63647=CARTESIAN_POINT('',(0.0121051913677208,-0.0317755400071256,0.0783004826206495));
#63648=CARTESIAN_POINT('Ctrl Pts',(0.0119696469467589,-0.0317744765475852,
0.0784249523685494));
#63649=CARTESIAN_POINT('Ctrl Pts',(0.0119922405024809,-0.0317741635039404,
0.0784042055051241));
#63650=CARTESIAN_POINT('Ctrl Pts',(0.0120148325343447,-0.0317741013272396,
0.0783834674352309));
#63651=CARTESIAN_POINT('Ctrl Pts',(0.0120600218711234,-0.0317744615102667,
0.0783419778674282));
#63652=CARTESIAN_POINT('Ctrl Pts',(0.0120826124706645,-0.0317748838660339,
0.0783212325268882));
#63653=CARTESIAN_POINT('Ctrl Pts',(0.0121051913677208,-0.0317755400071257,
0.0783004826206495));
#63654=CARTESIAN_POINT('',(0.0123074715936121,-0.0318824481878415,0.078250735535872));
#63655=CARTESIAN_POINT('Origin',(0.00908864960674653,-0.0332583300699432,
0.0686702664128971));
#63656=CARTESIAN_POINT('',(0.012353390398347,-0.0317755397360894,0.0780472474229795));
#63657=CARTESIAN_POINT('Origin',(0.00310044965113113,-0.0326853491203657,
0.0756162815277102));
#63658=CARTESIAN_POINT('',(0.0124751147581572,-0.0317744765475852,0.0779092284268295));
#63659=CARTESIAN_POINT('Ctrl Pts',(0.0123533905760804,-0.0317755400678203,
0.0780472475703818));
#63660=CARTESIAN_POINT('Ctrl Pts',(0.0123736834429088,-0.0317748838918832,
0.0780242557585583));
#63661=CARTESIAN_POINT('Ctrl Pts',(0.0123939715057635,-0.0317744615156213,
0.0780012523414514));
#63662=CARTESIAN_POINT('Ctrl Pts',(0.0124345457237183,-0.0317741013270862,
0.0779552381087258));
#63663=CARTESIAN_POINT('Ctrl Pts',(0.0124548258601386,-0.0317741635037164,
0.0779322341179504));
#63664=CARTESIAN_POINT('Ctrl Pts',(0.0124751147579603,-0.0317744765473203,
0.0779092284266523));
#63665=CARTESIAN_POINT('',(0.0125939901748882,-0.0317755400071256,0.0777687519394998));
#63666=CARTESIAN_POINT('Ctrl Pts',(0.0124751147581572,-0.0317744765475852,
0.0779092284268295));
#63667=CARTESIAN_POINT('Ctrl Pts',(0.0124949277333584,-0.0317741635379398,
0.0778858159783074));
#63668=CARTESIAN_POINT('Ctrl Pts',(0.0125147467586242,-0.0317741013468556,
0.0778624048120024));
#63669=CARTESIAN_POINT('Ctrl Pts',(0.0125543775856657,-0.0317744615102831,
0.0778155812241751));
#63670=CARTESIAN_POINT('Ctrl Pts',(0.012574189969852,-0.0317748838659619,
0.0777921681152774));
#63671=CARTESIAN_POINT('Ctrl Pts',(0.0125939901748881,-0.0317755400071256,
0.0777687519394998));
#63672=CARTESIAN_POINT('',(0.0127884403977845,-0.0318824481878419,0.0776940446905479));
#63673=CARTESIAN_POINT('Origin',(0.00839424863624071,-0.0332583300607026,
0.0685925458525311));
#63674=CARTESIAN_POINT('',(0.0128084932958481,-0.0317755397360895,0.0774864059899253));
#63675=CARTESIAN_POINT('Origin',(0.00332383393396606,-0.0326853491205201,
0.0762343099705962));
#63676=CARTESIAN_POINT('',(0.0129119594556425,-0.0317744765475852,0.0773342192071665));
#63677=CARTESIAN_POINT('Ctrl Pts',(0.0128084934906545,-0.0317755400678204,
0.0774864061138895));
#63678=CARTESIAN_POINT('Ctrl Pts',(0.0128257447040448,-0.0317748838918833,
0.0774610522287524));
#63679=CARTESIAN_POINT('Ctrl Pts',(0.0128429896968152,-0.0317744615156214,
0.0774356874319397));
#63680=CARTESIAN_POINT('Ctrl Pts',(0.0128774768623651,-0.0317741013270863,
0.0773849507372473));
#63681=CARTESIAN_POINT('Ctrl Pts',(0.0128947139193034,-0.0317741635037164,
0.0773595863647356));
#63682=CARTESIAN_POINT('Ctrl Pts',(0.012911959455425,-0.0317744765473203,
0.0773342192070154));
#63683=CARTESIAN_POINT('',(0.01301229113181,-0.0317755400071255,0.0771799513785266));
#63684=CARTESIAN_POINT('Ctrl Pts',(0.0129119594556425,-0.0317744765475851,
0.0773342192071665));
#63685=CARTESIAN_POINT('Ctrl Pts',(0.0129286836574135,-0.031774163503954,
0.0773085053569013));
#63686=CARTESIAN_POINT('Ctrl Pts',(0.0129454085700161,-0.0317741013272014,
0.0772828004029442));
#63687=CARTESIAN_POINT('Ctrl Pts',(0.0129788601669899,-0.0317744615102528,
0.0772313761716959));
#63688=CARTESIAN_POINT('Ctrl Pts',(0.0129955818856934,-0.0317748838660939,
0.0772056645293147));
#63689=CARTESIAN_POINT('Ctrl Pts',(0.01301229113181,-0.0317755400071256,
0.0771799513785267));
#63690=CARTESIAN_POINT('',(0.0131958447555375,-0.0318824481878423,0.0770814621433442));
#63691=CARTESIAN_POINT('Origin',(0.00769558219568638,-0.0332583300696311,
0.0686024695523869));
#63692=CARTESIAN_POINT('',(0.0131897155007483,-0.0317755397360896,0.0768729474413377));
#63693=CARTESIAN_POINT('Origin',(0.00362291626787834,-0.0326853491204316,
0.076819467600236));
#63694=CARTESIAN_POINT('',(0.0132732917373798,-0.0317744765475852,0.0767089929484456));
#63695=CARTESIAN_POINT('Ctrl Pts',(0.0131897157095554,-0.0317755400678204,
0.0768729475399086));
#63696=CARTESIAN_POINT('Ctrl Pts',(0.0132036532060474,-0.031774883891955,
0.0768456314303515));
#63697=CARTESIAN_POINT('Ctrl Pts',(0.0132175831656799,-0.031774461515605,
0.0768183052702963));
#63698=CARTESIAN_POINT('Ctrl Pts',(0.0132454393978449,-0.031774101327041,
0.0767636462572597));
#63699=CARTESIAN_POINT('Ctrl Pts',(0.0132593615358501,-0.0317741635037326,
0.0767363215158222));
#63700=CARTESIAN_POINT('Ctrl Pts',(0.0132732917371451,-0.0317744765473204,
0.076708992948323));
#63701=CARTESIAN_POINT('',(0.0133534973825149,-0.0317755400071256,0.0765433666743088));
#63702=CARTESIAN_POINT('Ctrl Pts',(0.0132732917373799,-0.0317744765475852,
0.0767089929484456));
#63703=CARTESIAN_POINT('Ctrl Pts',(0.0132866612644048,-0.0317741635039404,
0.076681385760083));
#63704=CARTESIAN_POINT('Ctrl Pts',(0.0133000326116973,-0.0317741013272397,
0.0766537873087095));
#63705=CARTESIAN_POINT('Ctrl Pts',(0.0133267752658551,-0.0317744615102666,
0.0765985759797762));
#63706=CARTESIAN_POINT('Ctrl Pts',(0.0133401426049004,-0.0317748838660336,
0.0765709712956067));
#63707=CARTESIAN_POINT('Ctrl Pts',(0.0133534973825149,-0.0317755400071256,
0.0765433666743088));
#63708=CARTESIAN_POINT('',(0.0135232596567777,-0.0318824481878426,0.0764226486869691));
#63709=CARTESIAN_POINT('Origin',(0.0070036687906888,-0.0332583300606654,
0.0686998812247189));
#63710=CARTESIAN_POINT('',(0.0134910449111451,-0.0317755397360896,0.0762165463849901));
#63711=CARTESIAN_POINT('Origin',(0.00399297994630453,-0.0326853491203843,
0.0773625261311474));
#63712=CARTESIAN_POINT('',(0.0135534131774357,-0.0317744765475852,0.0760434098422606));
#63713=CARTESIAN_POINT('Ctrl Pts',(0.0134910451306599,-0.0317755400678204,
0.0762165464566133));
#63714=CARTESIAN_POINT('Ctrl Pts',(0.0135014491094886,-0.031774883891955,
0.0761876989112398));
#63715=CARTESIAN_POINT('Ctrl Pts',(0.0135118443512286,-0.031774461515605,
0.0761588423392328));
#63716=CARTESIAN_POINT('Ctrl Pts',(0.0135326303378373,-0.0317741013270409,
0.0761011230171825));
#63717=CARTESIAN_POINT('Ctrl Pts',(0.0135430179974245,-0.0317741635037327,
0.0760722688329206));
#63718=CARTESIAN_POINT('Ctrl Pts',(0.0135534131771875,-0.0317744765473204,
0.0760434098421683));
#63719=CARTESIAN_POINT('',(0.0136122279006024,-0.0317755400071255,0.0758690371479093));
#63720=CARTESIAN_POINT('Ctrl Pts',(0.0135534131774357,-0.0317744765475851,
0.0760434098422606));
#63721=CARTESIAN_POINT('Ctrl Pts',(0.0135632161178193,-0.0317741635379696,
0.076014347858285));
#63722=CARTESIAN_POINT('Ctrl Pts',(0.0135730251553652,-0.0317741013467718,
0.0759852848394868));
#63723=CARTESIAN_POINT('Ctrl Pts',(0.0135926360570299,-0.0317744615102528,
0.0759271602795009));
#63724=CARTESIAN_POINT('Ctrl Pts',(0.0136024382067509,-0.0317748838660941,
0.0758980978933012));
#63725=CARTESIAN_POINT('Ctrl Pts',(0.0136122279006023,-0.0317755400071256,
0.0758690371479093));
#63726=CARTESIAN_POINT('',(0.0137655215729243,-0.031882448187843,0.075727994203186));
#63727=CARTESIAN_POINT('Origin',(0.0063294202056316,-0.0332583300615265,
0.068883244469716));
#63728=CARTESIAN_POINT('',(0.0137077293822312,-0.0317755397360894,0.0755275546576563));
#63729=CARTESIAN_POINT('Origin',(0.00442818884366834,-0.0326853491202104,
0.0778549212059884));
#63730=CARTESIAN_POINT('',(0.0137479060933655,-0.0317744765475852,0.075347966531792));
#63731=CARTESIAN_POINT('Ctrl Pts',(0.0137077296089918,-0.0317755400678203,
0.0755275547012022));
#63732=CARTESIAN_POINT('Ctrl Pts',(0.0137144359939304,-0.0317748838918833,
0.0754976306597627));
#63733=CARTESIAN_POINT('Ctrl Pts',(0.013721132578227,-0.0317744615156214,
0.0754676987628676));
#63734=CARTESIAN_POINT('Ctrl Pts',(0.0137345205107817,-0.0317741013270863,
0.0754078294047801));
#63735=CARTESIAN_POINT('Ctrl Pts',(0.0137412098727239,-0.0317741635037165,
0.0753779008237642));
#63736=CARTESIAN_POINT('Ctrl Pts',(0.0137479060931077,-0.0317744765473204,
0.0753479665317316));
#63737=CARTESIAN_POINT('',(0.0137844023512441,-0.0317755400071256,0.0751675973787842));
#63738=CARTESIAN_POINT('Ctrl Pts',(0.0137479060933655,-0.0317744765475852,
0.075347966531792));
#63739=CARTESIAN_POINT('Ctrl Pts',(0.0137539893027907,-0.0317741635379398,
0.075317905073158));
#63740=CARTESIAN_POINT('Ctrl Pts',(0.0137600784316405,-0.0317741013468556,
0.0752878418234986));
#63741=CARTESIAN_POINT('Ctrl Pts',(0.0137722497546434,-0.0317744615102831,
0.0752277177041611));
#63742=CARTESIAN_POINT('Ctrl Pts',(0.013778332128021,-0.0317748838659621,
0.0751976559515538));
#63743=CARTESIAN_POINT('Ctrl Pts',(0.0137844023512441,-0.0317755400071257,
0.0751675973787842));
#63744=CARTESIAN_POINT('',(0.0139188098888395,-0.0318824481878434,0.0750084538081706));
#63745=CARTESIAN_POINT('Origin',(0.00568346973988991,-0.0332583300694759,
0.0691496675676217));
#63746=CARTESIAN_POINT('',(0.0138363516704564,-0.0317755397360895,0.0748168380704599));
#63747=CARTESIAN_POINT('Origin',(0.00492167945582895,-0.032685349120183,
0.0782888874601413));
#63748=CARTESIAN_POINT('',(0.0138537032156988,-0.0317744765475852,0.0746336305734897));
#63749=CARTESIAN_POINT('Ctrl Pts',(0.0138363519008867,-0.0317755400678203,
0.0748168380852418));
#63750=CARTESIAN_POINT('Ctrl Pts',(0.0138392549267852,-0.0317748838919549,
0.0747863094742291));
#63751=CARTESIAN_POINT('Ctrl Pts',(0.013842147245254,-0.031774461515605,
0.0747557742930014));
#63752=CARTESIAN_POINT('Ctrl Pts',(0.0138479259901821,-0.0317741013270409,
0.0746946990649327));
#63753=CARTESIAN_POINT('Ctrl Pts',(0.0138508115585138,-0.0317741635037327,
0.074664168082036));
#63754=CARTESIAN_POINT('Ctrl Pts',(0.0138537032154354,-0.0317744765473203,
0.074633630573462));
#63755=CARTESIAN_POINT('',(0.0138673054405015,-0.0317755400071255,0.0744501094911124));
#63756=CARTESIAN_POINT('Ctrl Pts',(0.0138537032156987,-0.0317744765475851,
0.0746336305734897));
#63757=CARTESIAN_POINT('Ctrl Pts',(0.0138559710036869,-0.0317741635039403,
0.0746030404077552));
#63758=CARTESIAN_POINT('Ctrl Pts',(0.0138582437004173,-0.0317741013272395,
0.0745724576953827));
#63759=CARTESIAN_POINT('Ctrl Pts',(0.0138627837456575,-0.0317744615102666,
0.0745112788723768));
#63760=CARTESIAN_POINT('Ctrl Pts',(0.0138650504211692,-0.0317748838660337,
0.0744806918404243));
#63761=CARTESIAN_POINT('Ctrl Pts',(0.0138673054405015,-0.0317755400071256,
0.0744501094911124));
#63762=CARTESIAN_POINT('',(0.0139807071562112,-0.0318824481878437,0.074275375083785));
#63763=CARTESIAN_POINT('Origin',(0.00507600449970732,-0.0332583300693116,
0.0694949489328749));
#63764=CARTESIAN_POINT('',(0.0138748833255002,-0.0317755397360895,0.0740956050485428));
#63765=CARTESIAN_POINT('Origin',(0.00546566914113827,-0.0326853491204145,
0.078657580986387));
#63766=CARTESIAN_POINT('',(0.0138691360606172,-0.0317744765475852,0.0739116674721342));
#63767=CARTESIAN_POINT('Ctrl Pts',(0.0138748835559661,-0.0317755400678203,
0.0740956050343276));
#63768=CARTESIAN_POINT('Ctrl Pts',(0.0138739374410007,-0.0317748838918833,
0.074064953301563));
#63769=CARTESIAN_POINT('Ctrl Pts',(0.0138729798797259,-0.0317744615156214,
0.0740342963974567));
#63770=CARTESIAN_POINT('Ctrl Pts',(0.0138710584062604,-0.0317741013466568,
0.0739729818335607));
#63771=CARTESIAN_POINT('Ctrl Pts',(0.0138700944656008,-0.0317741635377321,
0.0739423232741826));
#63772=CARTESIAN_POINT('Ctrl Pts',(0.0138691360603524,-0.0317744765473203,
0.0739116674721398));
#63773=CARTESIAN_POINT('',(0.013859629737133,-0.0317755400071255,0.0737278886974891));
#63774=CARTESIAN_POINT('Ctrl Pts',(0.0138691360606172,-0.0317744765475852,
0.0739116674721342));
#63775=CARTESIAN_POINT('Ctrl Pts',(0.0138675521742271,-0.0317741635379696,
0.0738810376197538));
#63776=CARTESIAN_POINT('Ctrl Pts',(0.0138659735758916,-0.031774101346772,
0.0738504045607044));
#63777=CARTESIAN_POINT('Ctrl Pts',(0.0138628102534823,-0.0317744615102528,
0.0737891424571854));
#63778=CARTESIAN_POINT('Ctrl Pts',(0.0138612254838846,-0.0317748838660939,
0.0737585125218971));
#63779=CARTESIAN_POINT('Ctrl Pts',(0.013859629737133,-0.0317755400071256,
0.0737278886974891));
#63780=CARTESIAN_POINT('',(0.0139502372181573,-0.0318824481878442,0.0735403191194324));
#63781=CARTESIAN_POINT('Origin',(0.00451660453409808,-0.0332583300694264,
0.0699136432343077));
#63782=CARTESIAN_POINT('',(0.013822716680145,-0.0317755397360895,0.073375229867504));
#63783=CARTESIAN_POINT('Origin',(0.00605157885713282,-0.032685349120609,
0.0789551872677681));
#63784=CARTESIAN_POINT('',(0.0137939612429368,-0.0317744765475852,0.0731934630171163));
#63785=CARTESIAN_POINT('Ctrl Pts',(0.013822716907012,-0.0317755400678204,
0.0733752298245158));
#63786=CARTESIAN_POINT('Ctrl Pts',(0.0138179365721851,-0.0317748838919549,
0.0733449383727703));
#63787=CARTESIAN_POINT('Ctrl Pts',(0.0138131442323767,-0.031774461515605,
0.0733146432200586));
#63788=CARTESIAN_POINT('Ctrl Pts',(0.0138035526358299,-0.0317741013270409,
0.0732540496671673));
#63789=CARTESIAN_POINT('Ctrl Pts',(0.0137987548020344,-0.0317741635037326,
0.0732237602595771));
#63790=CARTESIAN_POINT('Ctrl Pts',(0.0137939612426747,-0.0317744765473203,
0.073193463017155));
#63791=CARTESIAN_POINT('',(0.0137614962915661,-0.0317755400071256,0.0730123248512634));
#63792=CARTESIAN_POINT('Ctrl Pts',(0.0137939612429368,-0.0317744765475851,
0.0731934630171163));
#63793=CARTESIAN_POINT('Ctrl Pts',(0.0137885503195655,-0.031774163503954,
0.0731632699230634));
#63794=CARTESIAN_POINT('Ctrl Pts',(0.0137831460043102,-0.0317741013272014,
0.0731330828275425));
#63795=CARTESIAN_POINT('Ctrl Pts',(0.0137723288603643,-0.0317744615102528,
0.0730726969823686));
#63796=CARTESIAN_POINT('Ctrl Pts',(0.0137669176383144,-0.031774883866094,
0.0730425071975653));
#63797=CARTESIAN_POINT('Ctrl Pts',(0.013761496291566,-0.0317755400071256,
0.0730123248512635));
#63798=CARTESIAN_POINT('',(0.0138278806038027,-0.0318824481878444,0.0728148781867722));
#63799=CARTESIAN_POINT('Origin',(0.00401409197564931,-0.0332583300606848,
0.0703991474283218));
#63800=CARTESIAN_POINT('',(0.0136806744335506,-0.0317755397360895,0.0726670732742799));
#63801=CARTESIAN_POINT('Origin',(0.00667016845759922,-0.0326853491205027,
0.0791770128756238));
#63802=CARTESIAN_POINT('',(0.01362936431444,-0.0317744765475852,0.072490343721727));
#63803=CARTESIAN_POINT('Ctrl Pts',(0.0136806746532409,-0.0317755400678203,
0.0726670732031967));
#63804=CARTESIAN_POINT('Ctrl Pts',(0.0136721354862546,-0.0317748838918833,
0.0726376197402067));
#63805=CARTESIAN_POINT('Ctrl Pts',(0.0136635839465049,-0.0317744615156214,
0.0726081641149218));
#63806=CARTESIAN_POINT('Ctrl Pts',(0.0136464745276844,-0.0317741013466568,
0.072549253711818));
#63807=CARTESIAN_POINT('Ctrl Pts',(0.013637916397321,-0.0317741635377321,
0.0725197980697543));
#63808=CARTESIAN_POINT('Ctrl Pts',(0.0136293643141849,-0.0317744765473204,
0.0724903437217983));
#63809=CARTESIAN_POINT('',(0.0135744527268592,-0.0317755400071255,0.0723147028217476));
#63810=CARTESIAN_POINT('Ctrl Pts',(0.01362936431444,-0.0317744765475851,
0.072490343721727));
#63811=CARTESIAN_POINT('Ctrl Pts',(0.0136202118588346,-0.0317741635039241,
0.0724610668749721));
#63812=CARTESIAN_POINT('Ctrl Pts',(0.0136110667109972,-0.031774101327285,
0.0724317951510505));
#63813=CARTESIAN_POINT('Ctrl Pts',(0.0135927665129182,-0.031774461510283,
0.0723732412225488));
#63814=CARTESIAN_POINT('Ctrl Pts',(0.0135836141775723,-0.0317748838659619,
0.0723439677022079));
#63815=CARTESIAN_POINT('Ctrl Pts',(0.0135744527268593,-0.0317755400071256,
0.0723147028217477));
#63816=CARTESIAN_POINT('',(0.0136155669500483,-0.0318824481878448,0.0721104929226697));
#63817=CARTESIAN_POINT('Origin',(0.00357639162872483,-0.0332583300605841,
0.0709438047849521));
#63818=CARTESIAN_POINT('',(0.0134509966767981,-0.0317755397360895,0.0719823033213779));
#63819=CARTESIAN_POINT('Origin',(0.00731168241481123,-0.0326853491200009,
0.0793195594880205));
#63820=CARTESIAN_POINT('',(0.0133779410670143,-0.0317744765475852,0.0718133981972761));
#63821=CARTESIAN_POINT('Ctrl Pts',(0.0134509968858469,-0.0317755400678204,
0.0719823032233207));
#63822=CARTESIAN_POINT('Ctrl Pts',(0.0134388335549863,-0.0317748838918833,
0.0719541522510933));
#63823=CARTESIAN_POINT('Ctrl Pts',(0.0134266576779183,-0.0317744615156214,
0.0719260006843409));
#63824=CARTESIAN_POINT('Ctrl Pts',(0.0134022984171264,-0.0317741013270863,
0.0718696961268912));
#63825=CARTESIAN_POINT('Ctrl Pts',(0.0133901186460761,-0.0317741635037165,
0.0718415514879352));
#63826=CARTESIAN_POINT('Ctrl Pts',(0.0133779410667702,-0.0317744765473203,
0.0718133981973787));
#63827=CARTESIAN_POINT('',(0.0133014488317624,-0.0317755400071256,0.0716460245250861));
#63828=CARTESIAN_POINT('Ctrl Pts',(0.0133779410670143,-0.0317744765475851,
0.0718133981972761));
#63829=CARTESIAN_POINT('Ctrl Pts',(0.0133651928047721,-0.0317741635379398,
0.0717855023455787));
#63830=CARTESIAN_POINT('Ctrl Pts',(0.0133524482787067,-0.0317741013468555,
0.0717576015655608));
#63831=CARTESIAN_POINT('Ctrl Pts',(0.013326955015208,-0.031774461510283,
0.0717018060070864));
#63832=CARTESIAN_POINT('Ctrl Pts',(0.0133142059037977,-0.0317748838659619,
0.07167391040898));
#63833=CARTESIAN_POINT('Ctrl Pts',(0.0133014488317624,-0.0317755400071256,
0.0716460245250861));
#63834=CARTESIAN_POINT('',(0.0133166445700436,-0.0318824481878451,0.0714382719035195));
#63835=CARTESIAN_POINT('Origin',(0.00321040634813816,-0.0332583300608944,
0.0715390257557646));
#63836=CARTESIAN_POINT('',(0.0131373055653141,-0.0317755397360895,0.071331719240017));
#63837=CARTESIAN_POINT('Origin',(0.00796600367088492,-0.0326853491205882,
0.0793805790579488));
#63838=CARTESIAN_POINT('',(0.0130436565954646,-0.0317744765475852,0.0711733022790721));
#63839=CARTESIAN_POINT('Ctrl Pts',(0.0131373057604247,-0.0317755400678204,
0.0713317191165323));
#63840=CARTESIAN_POINT('Ctrl Pts',(0.013121710088684,-0.0317748838918834,
0.0713053145927175));
#63841=CARTESIAN_POINT('Ctrl Pts',(0.0131061018951522,-0.0317744615156214,
0.0712789110515214));
#63842=CARTESIAN_POINT('Ctrl Pts',(0.0130748778821574,-0.0317741013270863,
0.0712261034972461));
#63843=CARTESIAN_POINT('Ctrl Pts',(0.013059266693632,-0.0317741635037165,
0.0711997073172645));
#63844=CARTESIAN_POINT('Ctrl Pts',(0.0130436565952352,-0.0317744765473204,
0.0711733022792046));
#63845=CARTESIAN_POINT('',(0.0129467900407859,-0.0317755400071255,0.0710168354174665));
#63846=CARTESIAN_POINT('Ctrl Pts',(0.0130436565954646,-0.0317744765475852,
0.0711733022790721));
#63847=CARTESIAN_POINT('Ctrl Pts',(0.0130275108253663,-0.0317741635039242,
0.0711472213414462));
#63848=CARTESIAN_POINT('Ctrl Pts',(0.0130113734074458,-0.031774101327285,
0.0711211435483423));
#63849=CARTESIAN_POINT('Ctrl Pts',(0.0129790863738693,-0.0317744615102831,
0.0710689802733736));
#63850=CARTESIAN_POINT('Ctrl Pts',(0.0129629415474981,-0.0317748838659619,
0.0710429025277493));
#63851=CARTESIAN_POINT('Ctrl Pts',(0.0129467900407859,-0.0317755400071256,
0.0710168354174665));
#63852=CARTESIAN_POINT('',(0.012935827648289,-0.0318824481878454,0.0708088164563586));
#63853=CARTESIAN_POINT('Origin',(0.00292190787764685,-0.033258330069175,
0.0721754233574242));
#63854=CARTESIAN_POINT('',(0.0127445481953167,-0.0317755397360895,0.0707255811298004));
#63855=CARTESIAN_POINT('Origin',(0.00862281318846725,-0.0326853491205626,
0.0793591092720414));
#63856=CARTESIAN_POINT('',(0.0126317827655993,-0.0317744765475852,0.0705801506621206));
#63857=CARTESIAN_POINT('Ctrl Pts',(0.012744548373412,-0.0317755400678204,
0.0707255809828356));
#63858=CARTESIAN_POINT('Ctrl Pts',(0.0127257663158992,-0.0317748838919549,
0.0707013393251905));
#63859=CARTESIAN_POINT('Ctrl Pts',(0.0127069719553852,-0.031774461515605,
0.0706771002078058));
#63860=CARTESIAN_POINT('Ctrl Pts',(0.0126693756085247,-0.0317741013270409,
0.0706286224595139));
#63861=CARTESIAN_POINT('Ctrl Pts',(0.0126505792013278,-0.0317741635037326,
0.0706043910233677));
#63862=CARTESIAN_POINT('Ctrl Pts',(0.0126317827653884,-0.0317744765473203,
0.0705801506622807));
#63863=CARTESIAN_POINT('',(0.0125160695349263,-0.0317755400071255,0.0704370581869752));
#63864=CARTESIAN_POINT('Ctrl Pts',(0.0126317827655993,-0.0317744765475851,
0.0705801506621206));
#63865=CARTESIAN_POINT('Ctrl Pts',(0.0126124975990844,-0.0317741635379696,
0.0705563015760721));
#63866=CARTESIAN_POINT('Ctrl Pts',(0.0125932148258627,-0.0317741013467719,
0.0705324467875334));
#63867=CARTESIAN_POINT('Ctrl Pts',(0.0125546466832984,-0.0317744615102529,
0.0704847440589314));
#63868=CARTESIAN_POINT('Ctrl Pts',(0.0125353607535185,-0.0317748838660941,
0.0704608954249417));
#63869=CARTESIAN_POINT('Ctrl Pts',(0.0125160695349263,-0.0317755400071257,
0.0704370581869752));
#63870=CARTESIAN_POINT('',(0.0124791218951295,-0.0318824481878456,0.0702320534696074));
#63871=CARTESIAN_POINT('Origin',(0.00271544613521357,-0.0332583300697618,
0.0728429612128157));
#63872=CARTESIAN_POINT('',(0.0122789185851526,-0.0317755397360895,0.0701734481508155));
#63873=CARTESIAN_POINT('Origin',(0.00927175268908372,-0.0326853491204069,
0.079255488721487));
#63874=CARTESIAN_POINT('',(0.012148815073757,-0.0317744765475852,0.0700432977017521));
#63875=CARTESIAN_POINT('Ctrl Pts',(0.012278918743424,-0.0317755400678203,
0.0701734479826883));
#63876=CARTESIAN_POINT('Ctrl Pts',(0.0122572465003417,-0.0317748838918833,
0.0701517514913895));
#63877=CARTESIAN_POINT('Ctrl Pts',(0.0122355623732302,-0.0317744615156213,
0.0701300590658809));
#63878=CARTESIAN_POINT('Ctrl Pts',(0.012192186615306,-0.0317741013270862,
0.0700866756542975));
#63879=CARTESIAN_POINT('Ctrl Pts',(0.012170501417954,-0.0317741635037164,
0.0700649911035623));
#63880=CARTESIAN_POINT('Ctrl Pts',(0.0121488150735677,-0.0317744765473202,
0.0700432977019375));
#63881=CARTESIAN_POINT('',(0.0120160800338609,-0.0317755400071255,0.0699158362668794));
#63882=CARTESIAN_POINT('Ctrl Pts',(0.012148815073757,-0.0317744765475851,
0.0700432977017521));
#63883=CARTESIAN_POINT('Ctrl Pts',(0.0121266928934662,-0.0317741635379696,
0.0700220537451477));
#63884=CARTESIAN_POINT('Ctrl Pts',(0.0121045723728852,-0.031774101346772,
0.0700008038310598));
#63885=CARTESIAN_POINT('Ctrl Pts',(0.0120603296144284,-0.0317744615102528,
0.0699583111227498));
#63886=CARTESIAN_POINT('Ctrl Pts',(0.0120382067335565,-0.0317748838660938,
0.0699370677103091));
#63887=CARTESIAN_POINT('Ctrl Pts',(0.012016080033861,-0.0317755400071257,
0.0699158362668794));
#63888=CARTESIAN_POINT('',(0.0119537298331154,-0.0318824481878458,0.0697170788401083));
#63889=CARTESIAN_POINT('Origin',(0.0025942770824451,-0.0332583300694133,
0.0735311118503182));
#63890=CARTESIAN_POINT('',(0.0117477599919279,-0.0317755397360895,0.0696840277699691));
#63891=CARTESIAN_POINT('Origin',(0.00990258800930164,-0.0326853491203117,
0.0790713515635572));
#63892=CARTESIAN_POINT('',(0.0116023702089484,-0.0317744765475852,0.0695712098898517));
#63893=CARTESIAN_POINT('Ctrl Pts',(0.0117477601278794,-0.0317755400678204,
0.069684027583331));
#63894=CARTESIAN_POINT('Ctrl Pts',(0.011723539485495,-0.0317748838918833,
0.0696652184276502));
#63895=CARTESIAN_POINT('Ctrl Pts',(0.0116993075623698,-0.0317744615156214,
0.069646414795164));
#63896=CARTESIAN_POINT('Ctrl Pts',(0.0116508364519961,-0.0317741013270863,
0.0696088098987382));
#63897=CARTESIAN_POINT('Ctrl Pts',(0.0116266044540401,-0.0317741635037165,
0.0695900142130668));
#63898=CARTESIAN_POINT('Ctrl Pts',(0.0116023702087839,-0.0317744765473203,
0.0695712098900593));
#63899=CARTESIAN_POINT('',(0.0114547066707008,-0.0317755400071255,0.0694613896382215));
#63900=CARTESIAN_POINT('Ctrl Pts',(0.0116023702089483,-0.0317744765475851,
0.0695712098898518));
#63901=CARTESIAN_POINT('Ctrl Pts',(0.0115777572180677,-0.0317741635039241,
0.0695529041017128));
#63902=CARTESIAN_POINT('Ctrl Pts',(0.0115531531504213,-0.031774101327285,
0.0695345981626347));
#63903=CARTESIAN_POINT('Ctrl Pts',(0.0115039308435332,-0.0317744615102831,
0.0694979836259309));
#63904=CARTESIAN_POINT('Ctrl Pts',(0.0114793199051569,-0.0317748838659621,
0.0694796804582271));
#63905=CARTESIAN_POINT('Ctrl Pts',(0.0114547066707008,-0.0317755400071257,
0.0694613896382215));
#63906=CARTESIAN_POINT('',(0.0113679372089185,-0.0318824481878459,0.0692720140253997));
#63907=CARTESIAN_POINT('Origin',(0.00256031164226087,-0.0332583300673947,
0.0742290227164587));
#63908=CARTESIAN_POINT('',(0.0111594491039563,-0.0317755397360895,0.0692650384390329));
#63909=CARTESIAN_POINT('Origin',(0.0105053704991273,-0.0326853491202493,
0.078809601752004));
#63910=CARTESIAN_POINT('',(0.0110010659331233,-0.0317744765475852,0.0691713323332258));
#63911=CARTESIAN_POINT('Ctrl Pts',(0.0111594492154439,-0.0317755400678204,
0.0692650382368272));
#63912=CARTESIAN_POINT('Ctrl Pts',(0.0111330621477567,-0.0317748838918834,
0.0692494130483858));
#63913=CARTESIAN_POINT('Ctrl Pts',(0.0111066645805211,-0.0317744615156214,
0.0692337947534391));
#63914=CARTESIAN_POINT('Ctrl Pts',(0.0110538625360635,-0.0317741013270863,
0.0692025614238513));
#63915=CARTESIAN_POINT('Ctrl Pts',(0.0110274658905872,-0.0317741635037164,
0.0691869510224353));
#63916=CARTESIAN_POINT('Ctrl Pts',(0.0110010659329861,-0.0317744765473203,
0.0691713323334524));
#63917=CARTESIAN_POINT('',(0.0108408026387313,-0.0317755400071255,0.069080885195809));
#63918=CARTESIAN_POINT('Ctrl Pts',(0.0110010659331233,-0.0317744765475851,
0.0691713323332258));
#63919=CARTESIAN_POINT('Ctrl Pts',(0.0109743526994062,-0.0317741635039241,
0.0691562557174284));
#63920=CARTESIAN_POINT('Ctrl Pts',(0.0109476482996434,-0.031774101327285,
0.0691411778335043));
#63921=CARTESIAN_POINT('Ctrl Pts',(0.0108942251070701,-0.031774461510283,
0.0691110212042464));
#63922=CARTESIAN_POINT('Ctrl Pts',(0.0108675142381039,-0.0317748838659619,
0.0690959469309762));
#63923=CARTESIAN_POINT('Ctrl Pts',(0.0108408026387313,-0.0317755400071256,
0.0690808851958091));
#63924=CARTESIAN_POINT('',(0.0107309823221581,-0.031882448187846,0.0689038779634784));
#63925=CARTESIAN_POINT('Origin',(0.00261408542943201,-0.0332583300691909,
0.0749256873615116));
#63926=CARTESIAN_POINT('',(0.0105232639353812,-0.0317755397360894,0.0689230878700478));
#63927=CARTESIAN_POINT('Origin',(0.0110705939186843,-0.0326853491202391,
0.0784743672369037));
#63928=CARTESIAN_POINT('',(0.0103543851739103,-0.0317744765475852,0.0688499713398157));
#63929=CARTESIAN_POINT('Ctrl Pts',(0.0105232640206465,-0.0317755400678203,
0.0689230876554634));
#63930=CARTESIAN_POINT('Ctrl Pts',(0.0104951266674769,-0.0317748838918833,
0.0689108928528174));
#63931=CARTESIAN_POINT('Ctrl Pts',(0.0104669797615349,-0.0317744615156213,
0.068898706205251));
#63932=CARTESIAN_POINT('Ctrl Pts',(0.0104106795027757,-0.0317741013270862,
0.0688743370107661));
#63933=CARTESIAN_POINT('Ctrl Pts',(0.0103825345006468,-0.0317741635037164,
0.0688621580789607));
#63934=CARTESIAN_POINT('Ctrl Pts',(0.0103543851738026,-0.0317744765473203,
0.0688499713400577));
#63935=CARTESIAN_POINT('',(0.0101840495712649,-0.0317755400071255,0.068780323722001));
#63936=CARTESIAN_POINT('Ctrl Pts',(0.0103543851739103,-0.0317744765475851,
0.0688499713398158));
#63937=CARTESIAN_POINT('Ctrl Pts',(0.0103259929824784,-0.0317741635039403,
0.0688383616641979));
#63938=CARTESIAN_POINT('Ctrl Pts',(0.0102976093964995,-0.0317741013272397,
0.0688267496233041));
#63939=CARTESIAN_POINT('Ctrl Pts',(0.0102408278293677,-0.0317744615102666,
0.0688035264876947));
#63940=CARTESIAN_POINT('Ctrl Pts',(0.0102124382745739,-0.0317748838660335,
0.0687919188385002));
#63941=CARTESIAN_POINT('Ctrl Pts',(0.0101840495712649,-0.0317755400071256,
0.068780323722001));
#63942=CARTESIAN_POINT('',(0.0100529103318967,-0.0318824481878461,0.0686184763799545));
#63943=CARTESIAN_POINT('Origin',(0.00275475047964434,-0.0332583300614187,
0.0756101189085328));
#63944=CARTESIAN_POINT('',(0.00984923750634952,-0.0317755397360895,0.0686635688277579));
#63945=CARTESIAN_POINT('Origin',(0.0115893443567482,-0.0326853491205606,
0.0780709348670765));
#63946=CARTESIAN_POINT('',(0.00967252647319418,-0.0317744765475852,0.0686121949644612));
#63947=CARTESIAN_POINT('Ctrl Pts',(0.00984923756404795,-0.0317755400678203,
0.068663568604179));
#63948=CARTESIAN_POINT('Ctrl Pts',(0.00981979367147625,-0.0317748838919549,
0.0686549965075861));
#63949=CARTESIAN_POINT('Ctrl Pts',(0.00979034131869444,-0.0317744615156049,
0.0686464336976297));
#63950=CARTESIAN_POINT('Ctrl Pts',(0.00973143393050001,-0.0317741013466114,
0.0686293138838769));
#63951=CARTESIAN_POINT('Ctrl Pts',(0.0097019780353993,-0.0317741635377482,
0.0686207566305228));
#63952=CARTESIAN_POINT('Ctrl Pts',(0.00967252647311763,-0.0317744765473203,
0.0686121949647148));
#63953=CARTESIAN_POINT('',(0.00949480485650097,-0.0317755400071255,0.0685644452507862));
#63954=CARTESIAN_POINT('Ctrl Pts',(0.00967252647319419,-0.0317744765475852,
0.0686121949644612));
#63955=CARTESIAN_POINT('Ctrl Pts',(0.00964290630339529,-0.031774163537956,
0.0686042361846668));
#63956=CARTESIAN_POINT('Ctrl Pts',(0.00961328471788823,-0.0317741013468101,
0.0685962713846959));
#63957=CARTESIAN_POINT('Ctrl Pts',(0.00955404347873013,-0.0317744615102666,
0.0685803488530575));
#63958=CARTESIAN_POINT('Ctrl Pts',(0.00952442295984559,-0.0317748838660336,
0.068572390888345));
#63959=CARTESIAN_POINT('Ctrl Pts',(0.00949480485650097,-0.0317755400071256,
0.0685644452507862));
#63960=CARTESIAN_POINT('',(0.00934441483848152,-0.0318824481878461,0.0684203102282909));
#63961=CARTESIAN_POINT('Origin',(0.00298008830923749,-0.0332583300645355,
0.0762715235567863));
#63962=CARTESIAN_POINT('',(0.00914799961629096,-0.0317755397360895,0.0684905740824893));
#63963=CARTESIAN_POINT('Origin',(0.0120534408096581,-0.0326853491203047,
0.0776056670125974));
#63964=CARTESIAN_POINT('',(0.00896624315000526,-0.0317744765475852,0.0684617530826412));
#63965=CARTESIAN_POINT('Ctrl Pts',(0.00914799964551254,-0.0317755400678203,
0.0684905738534419));
#63966=CARTESIAN_POINT('Ctrl Pts',(0.0091177135549392,-0.0317748838918833,
0.0684857596481305));
#63967=CARTESIAN_POINT('Ctrl Pts',(0.00908742023979814,-0.0317744615156213,
0.0684809557173699));
#63968=CARTESIAN_POINT('Ctrl Pts',(0.00902682838497098,-0.0317741013270862,
0.0684713534309399));
#63969=CARTESIAN_POINT('Ctrl Pts',(0.00899653883266233,-0.0317741635037163,
0.0684665565000764));
#63970=CARTESIAN_POINT('Ctrl Pts',(0.00896624314996109,-0.0317744765473202,
0.0684617530829025));
#63971=CARTESIAN_POINT('',(0.00878393829532611,-0.0317755400071255,0.0684366543146152));
#63972=CARTESIAN_POINT('Ctrl Pts',(0.00896624315000525,-0.0317744765475851,
0.0684617530826413));
#63973=CARTESIAN_POINT('Ctrl Pts',(0.00893585904291267,-0.0317741635379398,
0.0684575694516458));
#63974=CARTESIAN_POINT('Ctrl Pts',(0.00890547277664513,-0.0317741013468555,
0.0684533800253657));
#63975=CARTESIAN_POINT('Ctrl Pts',(0.00884470305483108,-0.031774461510283,
0.0684450079443782));
#63976=CARTESIAN_POINT('Ctrl Pts',(0.00881431870684405,-0.031774883865962,
0.0684408251662397));
#63977=CARTESIAN_POINT('Ctrl Pts',(0.00878393829532611,-0.0317755400071256,
0.0684366543146152));
#63978=CARTESIAN_POINT('',(0.00861666923907833,-0.0318824481878461,0.068312504707078));
#63979=CARTESIAN_POINT('Origin',(0.00328654529439703,-0.0332583300606616,
0.0768994704731398));
#63980=CARTESIAN_POINT('',(0.00843060920563109,-0.0317755397360895,0.0684068318647171));
#63981=CARTESIAN_POINT('Origin',(0.0124555641985925,-0.0326853491202919,
0.0770859012249049));
#63982=CARTESIAN_POINT('',(0.0082466737142653,-0.0317744765475852,0.0684010182527021));
#63983=CARTESIAN_POINT('Ctrl Pts',(0.008430609205915,-0.0317755400678204,
0.0684068316338133));
#63984=CARTESIAN_POINT('Ctrl Pts',(0.00839995855029356,-0.0317748838918834,
0.0684058512436123));
#63985=CARTESIAN_POINT('Ctrl Pts',(0.00836930201481447,-0.0317744615156214,
0.0684048819524226));
#63986=CARTESIAN_POINT('Ctrl Pts',(0.00830798445925291,-0.0317741013270863,
0.0684029495559823));
#63987=CARTESIAN_POINT('Ctrl Pts',(0.008277332534255,-0.0317741635037165,
0.0684019867378854));
#63988=CARTESIAN_POINT('Ctrl Pts',(0.00824667371425424,-0.0317744765473203,
0.0684010182529667));
#63989=CARTESIAN_POINT('',(0.00806266067806107,-0.0317755400071255,0.0683989662528899));
#63990=CARTESIAN_POINT('Ctrl Pts',(0.0082466737142653,-0.0317744765475852,
0.068401018252702));
#63991=CARTESIAN_POINT('Ctrl Pts',(0.00821600484693169,-0.0317741635379398,
0.0684006757492774));
#63992=CARTESIAN_POINT('Ctrl Pts',(0.00818533311110706,-0.0317741013468556,
0.0684003277668821));
#63993=CARTESIAN_POINT('Ctrl Pts',(0.00812399327671767,-0.0317744615102831,
0.0683996381679916));
#63994=CARTESIAN_POINT('Ctrl Pts',(0.00809332427727973,-0.031774883865962,
0.0683992965408911));
#63995=CARTESIAN_POINT('Ctrl Pts',(0.00806266067806107,-0.0317755400071256,
0.06839896625289));
#63996=CARTESIAN_POINT('',(0.00788115051652376,-0.031882448187846,0.0682967599737853));
#63997=CARTESIAN_POINT('Origin',(0.00366928835036435,-0.0332583300693303,
0.0774840566758911));
#63998=CARTESIAN_POINT('',(0.00770837994969399,-0.0317755397360895,0.0684136628392406));
#63999=CARTESIAN_POINT('Origin',(0.0127893735271636,-0.0326853484021168,
0.0765198349424559));
#64000=CARTESIAN_POINT('',(0.00752516620582388,-0.0317744765475852,0.0684309482991929));
#64001=CARTESIAN_POINT('Ctrl Pts',(0.00770837992103575,-0.0317755400678203,
0.0684136626101221));
#64002=CARTESIAN_POINT('Ctrl Pts',(0.00767784808519083,-0.0317748838920053,
0.0684165314958372));
#64003=CARTESIAN_POINT('Ctrl Pts',(0.00764731179832722,-0.0317744615155934,
0.0684194121307926));
#64004=CARTESIAN_POINT('Ctrl Pts',(0.00758623886673111,-0.0317741013465795,
0.0684251797867753));
#64005=CARTESIAN_POINT('Ctrl Pts',(0.00755570133421423,-0.0317741635377596,
0.0684280668919191));
#64006=CARTESIAN_POINT('Ctrl Pts',(0.00752516620584607,-0.0317744765473203,
0.0684309482994569));
#64007=CARTESIAN_POINT('',(0.00734234698360057,-0.0317755400071256,0.0684519754288576));
#64008=CARTESIAN_POINT('Ctrl Pts',(0.00752516620582388,-0.0317744765475852,
0.0684309482991929));
#64009=CARTESIAN_POINT('Ctrl Pts',(0.00749469293335161,-0.0317741635039242,
0.068434452705615));
#64010=CARTESIAN_POINT('Ctrl Pts',(0.0074642260623123,-0.0317741013272851,
0.0684379508936332));
#64011=CARTESIAN_POINT('Ctrl Pts',(0.00740328016968802,-0.0317744615102832,
0.0684449550327957));
#64012=CARTESIAN_POINT('Ctrl Pts',(0.00737281018723983,-0.0317748838659622,
0.0684484599443968));
#64013=CARTESIAN_POINT('Ctrl Pts',(0.00734234698360056,-0.0317755400071257,
0.0684519754288575));
#64014=CARTESIAN_POINT('',(0.00714945824045025,-0.0318824481878459,0.0683733243322622));
#64015=CARTESIAN_POINT('Origin',(0.00412228148793428,-0.0332583300609497,
0.0780160627022593));
#64016=CARTESIAN_POINT('',(0.00699270183528492,-0.0317755397360895,0.068510959277511));
#64017=CARTESIAN_POINT('Origin',(0.0130496030223191,-0.0326853484020826,
0.0759163944377061));
#64018=CARTESIAN_POINT('',(0.00681309922909792,-0.0317744765475852,0.0685510712074014));
#64019=CARTESIAN_POINT('Ctrl Pts',(0.00699270177813648,-0.0317755400678204,
0.068510959053791));
#64020=CARTESIAN_POINT('Ctrl Pts',(0.00696277025609412,-0.0317748838918833,
0.0685176319724393));
#64021=CARTESIAN_POINT('Ctrl Pts',(0.00693283579913468,-0.0317744615156214,
0.0685243171036637));
#64022=CARTESIAN_POINT('Ctrl Pts',(0.00687296733296115,-0.0317741013466568,
0.0685376937461372));
#64023=CARTESIAN_POINT('Ctrl Pts',(0.00684303244542577,-0.0317741635377321,
0.0685443854539173));
#64024=CARTESIAN_POINT('Ctrl Pts',(0.00681309922915301,-0.0317744765473203,
0.0685510712076604));
#64025=CARTESIAN_POINT('',(0.00663435698920081,-0.0317755400071256,0.0685948458561471));
#64026=CARTESIAN_POINT('Ctrl Pts',(0.00681309922909793,-0.0317744765475851,
0.0685510712074014));
#64027=CARTESIAN_POINT('Ctrl Pts',(0.00678330546761347,-0.0317741635039403,
0.0685583672939304));
#64028=CARTESIAN_POINT('Ctrl Pts',(0.00675351727781274,-0.0317741013272395,
0.0685656564087527));
#64029=CARTESIAN_POINT('Ctrl Pts',(0.00669392980840041,-0.0317744615102666,
0.0685802438651471));
#64030=CARTESIAN_POINT('Ctrl Pts',(0.00666413937109456,-0.0317748838660337,
0.068587540041312));
#64031=CARTESIAN_POINT('Ctrl Pts',(0.00663435698920084,-0.0317755400071256,
0.0685948458561471));
#64032=CARTESIAN_POINT('',(0.00643313163514339,-0.0318824481878457,0.0685409903168382));
#64033=CARTESIAN_POINT('Origin',(0.00463838065616737,-0.033258330061087,
0.0784870986645944));
#64034=CARTESIAN_POINT('',(0.00629486153379326,-0.0317755397360894,0.0686971867565749));
#64035=CARTESIAN_POINT('Origin',(0.0132321485687967,-0.0326853491204153,
0.0752850966106633));
#64036=CARTESIAN_POINT('',(0.00612170250567762,-0.0317744765475852,0.0687594925673074));
#64037=CARTESIAN_POINT('Ctrl Pts',(0.0062948614490559,-0.0317755400678203,
0.0686971865417816));
#64038=CARTESIAN_POINT('Ctrl Pts',(0.00626600228762614,-0.0317748838919548,
0.0687075582557843));
#64039=CARTESIAN_POINT('Ctrl Pts',(0.00623714174029079,-0.0317744615156049,
0.0687179424556203));
#64040=CARTESIAN_POINT('Ctrl Pts',(0.00617941875177804,-0.0317741013270409,
0.0687387182582189));
#64041=CARTESIAN_POINT('Ctrl Pts',(0.00615056487727383,-0.0317741635037326,
0.0687491067781996));
#64042=CARTESIAN_POINT('Ctrl Pts',(0.00612170250576476,-0.0317744765473203,
0.0687594925675575));
#64043=CARTESIAN_POINT('',(0.00594985612000611,-0.0317755400071255,0.0688253243827735));
#64044=CARTESIAN_POINT('Ctrl Pts',(0.00612170250567763,-0.0317744765475851,
0.0687594925673074));
#64045=CARTESIAN_POINT('Ctrl Pts',(0.00609306123154383,-0.031774163537956,
0.0687704640781778));
#64046=CARTESIAN_POINT('Ctrl Pts',(0.00606441527350702,-0.0317741013468101,
0.0687814315507554));
#64047=CARTESIAN_POINT('Ctrl Pts',(0.00600712907498679,-0.0317744615102666,
0.0688033710787701));
#64048=CARTESIAN_POINT('Ctrl Pts',(0.00597848799753159,-0.0317748838660335,
0.0688143434542423));
#64049=CARTESIAN_POINT('Ctrl Pts',(0.0059498561200061,-0.0317755400071256,
0.0688253243827735));
#64050=CARTESIAN_POINT('',(0.00574346759908138,-0.0318824481878455,0.0687971137347777));
#64051=CARTESIAN_POINT('Origin',(0.00520944668414427,-0.0332583300692591,
0.078889736052037));
#64052=CARTESIAN_POINT('',(0.00562586440364342,-0.0317755397360894,0.0689694083578402));
#64053=CARTESIAN_POINT('Origin',(0.0133341329028461,-0.0326853491203037,
0.0746358979587515));
#64054=CARTESIAN_POINT('',(0.00546187977491395,-0.0317744765475852,0.0690529254495596));
#64055=CARTESIAN_POINT('Ctrl Pts',(0.00562586429265349,-0.0317755400678202,
0.068969408155361));
#64056=CARTESIAN_POINT('Ctrl Pts',(0.00559853261180286,-0.0317748838918832,
0.0689833150988382));
#64057=CARTESIAN_POINT('Ctrl Pts',(0.00557120112538377,-0.0317744615156213,
0.068997234601096));
#64058=CARTESIAN_POINT('Ctrl Pts',(0.00551654017287186,-0.0317741013466567,
0.0690250796738461));
#64059=CARTESIAN_POINT('Ctrl Pts',(0.00548920990492778,-0.031774163537732,
0.0690390056531245));
#64060=CARTESIAN_POINT('Ctrl Pts',(0.00546187977503177,-0.0317744765473203,
0.0690529254497969));
#64061=CARTESIAN_POINT('',(0.00529963936362479,-0.0317755400071255,0.0691397762246904));
#64062=CARTESIAN_POINT('Ctrl Pts',(0.00546187977491393,-0.0317744765475852,
0.0690529254495596));
#64063=CARTESIAN_POINT('Ctrl Pts',(0.00543483650076778,-0.0317741635039242,
0.0690674017240456));
#64064=CARTESIAN_POINT('Ctrl Pts',(0.00540779688937628,-0.031774101327285,
0.0690818698602811));
#64065=CARTESIAN_POINT('Ctrl Pts',(0.00535370922709989,-0.031774461510283,
0.0691108178236381));
#64066=CARTESIAN_POINT('Ctrl Pts',(0.0053266691979104,-0.031774883865962,
0.0691252933566885));
#64067=CARTESIAN_POINT('Ctrl Pts',(0.00529963936362484,-0.0317755400071256,
0.0691397762246905));
#64068=CARTESIAN_POINT('',(0.00509134254609834,-0.0318824481878453,0.0691376553667789));
#64069=CARTESIAN_POINT('Origin',(0.00582647353396789,-0.0332583300652073,
0.0792176248812057));
#64070=CARTESIAN_POINT('',(0.00499626092921708,-0.0317755397360894,0.0693233309840378));
#64071=CARTESIAN_POINT('Origin',(0.0133539468935739,-0.0326853491203005,
0.0739790364057491));
#64072=CARTESIAN_POINT('',(0.00484403683542784,-0.0317744765475852,0.0694267422423173));
#64073=CARTESIAN_POINT('Ctrl Pts',(0.00499626079372497,-0.0317755400678203,
0.0693233307970659));
#64074=CARTESIAN_POINT('Ctrl Pts',(0.00497088763825794,-0.0317748838920054,
0.0693405536448749));
#64075=CARTESIAN_POINT('Ctrl Pts',(0.00494551624256691,-0.0317744615155934,
0.0693577889329206));
#64076=CARTESIAN_POINT('Ctrl Pts',(0.00489477621409276,-0.0317741013465794,
0.0693922652775759));
#64077=CARTESIAN_POINT('Ctrl Pts',(0.0048694068438692,-0.0317741635377597,
0.0694095068355857));
#64078=CARTESIAN_POINT('Ctrl Pts',(0.00484403683557445,-0.0317744765473203,
0.0694267422425379));
#64079=CARTESIAN_POINT('',(0.00469396102672551,-0.0317755400071256,0.0695332422885067));
#64080=CARTESIAN_POINT('Ctrl Pts',(0.00484403683542785,-0.0317744765475851,
0.0694267422423173));
#64081=CARTESIAN_POINT('Ctrl Pts',(0.00481902388447747,-0.0317741635379696,
0.0694444918574586));
#64082=CARTESIAN_POINT('Ctrl Pts',(0.00479400539256557,-0.031774101346772,
0.0694622387259671));
#64083=CARTESIAN_POINT('Ctrl Pts',(0.00474397508069731,-0.0317744615102528,
0.0694977354839971));
#64084=CARTESIAN_POINT('Ctrl Pts',(0.00471896253299177,-0.0317748838660939,
0.0695154858892795));
#64085=CARTESIAN_POINT('Ctrl Pts',(0.00469396102672552,-0.0317755400071256,
0.0695332422885067));
#64086=CARTESIAN_POINT('',(0.00448704087784028,-0.0318824481878451,0.0695572446678755));
#64087=CARTESIAN_POINT('Origin',(0.00647973031733237,-0.0332583300693583,
0.079465594297633));
#64088=CARTESIAN_POINT('',(0.00441598033341292,-0.0317755397360894,0.0697533730639295));
#64089=CARTESIAN_POINT('Origin',(0.0132912780623905,-0.0326853491205531,
0.0733248710508142));
#64090=CARTESIAN_POINT('',(0.00427791743945781,-0.0317744765475852,0.0698750476314508));
#64091=CARTESIAN_POINT('Ctrl Pts',(0.00441598017555541,-0.0317755400678203,
0.0697533728954136));
#64092=CARTESIAN_POINT('Ctrl Pts',(0.00439296568843473,-0.0317748838919549,
0.0697736400371027));
#64093=CARTESIAN_POINT('Ctrl Pts',(0.00436995450907151,-0.0317744615156049,
0.0697939192980136));
#64094=CARTESIAN_POINT('Ctrl Pts',(0.00432393561522292,-0.0317741013466114,
0.0698344831959516));
#64095=CARTESIAN_POINT('Ctrl Pts',(0.00430092722938568,-0.0317741635377482,
0.069854768425117));
#64096=CARTESIAN_POINT('Ctrl Pts',(0.0042779174396309,-0.0317744765473203,
0.0698750476316513));
#64097=CARTESIAN_POINT('',(0.00414237301849599,-0.0317755400071255,0.0699995173793506));
#64098=CARTESIAN_POINT('Ctrl Pts',(0.00427791743945776,-0.0317744765475852,
0.0698750476314508));
#64099=CARTESIAN_POINT('Ctrl Pts',(0.00425532388256617,-0.0317741635039242,
0.06989579449595));
#64100=CARTESIAN_POINT('Ctrl Pts',(0.00423273184945642,-0.0317741013272851,
0.0699165325669869));
#64101=CARTESIAN_POINT('Ctrl Pts',(0.00418754251629321,-0.0317744615102831,
0.0699580221314705));
#64102=CARTESIAN_POINT('Ctrl Pts',(0.00416495191802581,-0.031774883865962,
0.0699787674708386));
#64103=CARTESIAN_POINT('Ctrl Pts',(0.00414237301849597,-0.0317755400071257,
0.0699995173793505));
#64104=CARTESIAN_POINT('',(0.00394009279260827,-0.0318824481878447,0.0700492644641388));
#64105=CARTESIAN_POINT('Origin',(0.00715891477913272,-0.0332583300694027,
0.079629733586828));
#64106=CARTESIAN_POINT('',(0.00389417398786977,-0.0317755397360895,0.0702527525770204));
#64107=CARTESIAN_POINT('Origin',(0.0131471147347495,-0.0326853491205069,
0.0726837184722928));
#64108=CARTESIAN_POINT('',(0.00377244962806149,-0.0317744765475852,0.0703907715731684));
#64109=CARTESIAN_POINT('Ctrl Pts',(0.00389417381013636,-0.0317755400678204,
0.0702527524296181));
#64110=CARTESIAN_POINT('Ctrl Pts',(0.00387388094330818,-0.0317748838918833,
0.0702757442414414));
#64111=CARTESIAN_POINT('Ctrl Pts',(0.0038535928804539,-0.0317744615156214,
0.0702987476585478));
#64112=CARTESIAN_POINT('Ctrl Pts',(0.00381302086706254,-0.0317741013466568,
0.0703447593911317));
#64113=CARTESIAN_POINT('Ctrl Pts',(0.00379273632146808,-0.0317741635377321,
0.070367768381869));
#64114=CARTESIAN_POINT('Ctrl Pts',(0.00377244962825834,-0.0317744765473203,
0.0703907715733456));
#64115=CARTESIAN_POINT('',(0.00365357421132868,-0.0317755400071255,0.0705312480605002));
#64116=CARTESIAN_POINT('Ctrl Pts',(0.00377244962806147,-0.0317744765475851,
0.0703907715731684));
#64117=CARTESIAN_POINT('Ctrl Pts',(0.00375263449972844,-0.0317741635039242,
0.0704141865659871));
#64118=CARTESIAN_POINT('Ctrl Pts',(0.00373281978104871,-0.031774101327285,
0.0704375926437021));
#64119=CARTESIAN_POINT('Ctrl Pts',(0.00369318680055041,-0.031774461510283,
0.0704844187758258));
#64120=CARTESIAN_POINT('Ctrl Pts',(0.00367337441636236,-0.031774883865962,
0.0705078318847255));
#64121=CARTESIAN_POINT('Ctrl Pts',(0.00365357421132872,-0.0317755400071256,
0.0705312480605002));
#64122=CARTESIAN_POINT('',(0.00345912398843712,-0.0318824481878444,0.0706059553094632));
#64123=CARTESIAN_POINT('Origin',(0.00785331577631647,-0.0332583300696887,
0.0797074542031271));
#64124=CARTESIAN_POINT('',(0.00343907109036868,-0.0317755397360895,0.0708135940100747));
#64125=CARTESIAN_POINT('Origin',(0.0129237304522124,-0.0326853491203865,
0.0720656900293326));
#64126=CARTESIAN_POINT('',(0.00333560493057455,-0.0317744765475852,0.0709657807928331));
#64127=CARTESIAN_POINT('Ctrl Pts',(0.00343907089556234,-0.0317755400678203,
0.0708135938861105));
#64128=CARTESIAN_POINT('Ctrl Pts',(0.00342181968217177,-0.0317748838918833,
0.0708389477712479));
#64129=CARTESIAN_POINT('Ctrl Pts',(0.00340457468940154,-0.0317744615156214,
0.0708643125680603));
#64130=CARTESIAN_POINT('Ctrl Pts',(0.00337008752385169,-0.0317741013270863,
0.0709150492627527));
#64131=CARTESIAN_POINT('Ctrl Pts',(0.00335285046691346,-0.0317741635037165,
0.0709404136352643));
#64132=CARTESIAN_POINT('Ctrl Pts',(0.00333560493079202,-0.0317744765473204,
0.0709657807929842));
#64133=CARTESIAN_POINT('',(0.00323527325440675,-0.0317755400071256,0.0711200486214734));
#64134=CARTESIAN_POINT('Ctrl Pts',(0.00333560493057454,-0.0317744765475852,
0.0709657807928331));
#64135=CARTESIAN_POINT('Ctrl Pts',(0.0033188807272107,-0.0317741635039242,
0.0709914946455473));
#64136=CARTESIAN_POINT('Ctrl Pts',(0.00330215581291114,-0.0317741013272851,
0.0710171996021129));
#64137=CARTESIAN_POINT('Ctrl Pts',(0.00326870422085706,-0.0317744615102831,
0.0710686238257989));
#64138=CARTESIAN_POINT('Ctrl Pts',(0.00325198250388255,-0.0317748838659619,
0.0710943354655161));
#64139=CARTESIAN_POINT('Ctrl Pts',(0.00323527325440685,-0.0317755400071256,
0.0711200486214734));
#64140=CARTESIAN_POINT('',(0.00305171963068536,-0.031882448187844,0.0712185378566669));
#64141=CARTESIAN_POINT('Origin',(0.00855198215770979,-0.0332583300606185,
0.079697530396209));
#64142=CARTESIAN_POINT('',(0.00305784888546854,-0.0317755397360895,0.0714270525586625));
#64143=CARTESIAN_POINT('Origin',(0.0126246481179549,-0.0326853491205759,
0.0714805323998506));
#64144=CARTESIAN_POINT('',(0.00297427264883722,-0.0317744765475852,0.0715910070515539));
#64145=CARTESIAN_POINT('Ctrl Pts',(0.00305784867666147,-0.0317755400678203,
0.0714270524600915));
#64146=CARTESIAN_POINT('Ctrl Pts',(0.00304391117864933,-0.0317748838918833,
0.0714543685726279));
#64147=CARTESIAN_POINT('Ctrl Pts',(0.00302998121980092,-0.0317744615156213,
0.0714816947311485));
#64148=CARTESIAN_POINT('Ctrl Pts',(0.00300212650340108,-0.0317741013466568,
0.0715363507699768));
#64149=CARTESIAN_POINT('Ctrl Pts',(0.00298820133741727,-0.031774163537732,
0.0715636814523147));
#64150=CARTESIAN_POINT('Ctrl Pts',(0.00297427264907201,-0.0317744765473203,
0.0715910070516766));
#64151=CARTESIAN_POINT('',(0.00289406700370193,-0.0317755400071256,0.0717566333256912));
#64152=CARTESIAN_POINT('Ctrl Pts',(0.00297427264883726,-0.0317744765475851,
0.0715910070515539));
#64153=CARTESIAN_POINT('Ctrl Pts',(0.00296090457455914,-0.031774163537956,
0.0716186112400905));
#64154=CARTESIAN_POINT('Ctrl Pts',(0.00294753032146113,-0.03177410134681,
0.0716462156911905));
#64155=CARTESIAN_POINT('Ctrl Pts',(0.0029207891203601,-0.0317744615102666,
0.0717014240202273));
#64156=CARTESIAN_POINT('Ctrl Pts',(0.00290742178131277,-0.0317748838660337,
0.0717290287044008));
#64157=CARTESIAN_POINT('Ctrl Pts',(0.00289406700370195,-0.0317755400071256,
0.0717566333256912));
#64158=CARTESIAN_POINT('',(0.00272430472944635,-0.0318824481878437,0.0718773513130417));
#64159=CARTESIAN_POINT('Origin',(0.00924389559598285,-0.0332583300610094,
0.0796001187756036));
#64160=CARTESIAN_POINT('',(0.00275651947507167,-0.0317755397360895,0.07208345361501));
#64161=CARTESIAN_POINT('Origin',(0.0122545844395361,-0.0326853491205966,
0.0709374738690273));
#64162=CARTESIAN_POINT('',(0.00269415120878019,-0.0317744765475852,0.0722565901577418));
#64163=CARTESIAN_POINT('Ctrl Pts',(0.0027565192555569,-0.0317755400678203,
0.0720834535433868));
#64164=CARTESIAN_POINT('Ctrl Pts',(0.00274611527559222,-0.0317748838918833,
0.0721123010919102));
#64165=CARTESIAN_POINT('Ctrl Pts',(0.0027357200344381,-0.0317744615156214,
0.0721411576622954));
#64166=CARTESIAN_POINT('Ctrl Pts',(0.00271493404948892,-0.0317741013270863,
0.072198876979737));
#64167=CARTESIAN_POINT('Ctrl Pts',(0.00270454638932916,-0.0317741635037164,
0.072227731165589));
#64168=CARTESIAN_POINT('Ctrl Pts',(0.00269415120902848,-0.0317744765473203,
0.0722565901578341));
#64169=CARTESIAN_POINT('',(0.00263533648561441,-0.0317755400071256,0.0724309628520908));
#64170=CARTESIAN_POINT('Ctrl Pts',(0.0026941512087802,-0.0317744765475851,
0.0722565901577418));
#64171=CARTESIAN_POINT('Ctrl Pts',(0.00268434826746197,-0.0317741635379398,
0.0722856521444882));
#64172=CARTESIAN_POINT('Ctrl Pts',(0.00267453922892048,-0.0317741013468556,
0.0723147151662367));
#64173=CARTESIAN_POINT('Ctrl Pts',(0.00265492833014389,-0.0317744615102831,
0.0723728397176637));
#64174=CARTESIAN_POINT('Ctrl Pts',(0.00264512618143677,-0.0317748838659621,
0.072401902100848));
#64175=CARTESIAN_POINT('Ctrl Pts',(0.0026353364856144,-0.0317755400071257,
0.0724309628520908));
#64176=CARTESIAN_POINT('',(0.00248204281330085,-0.0318824481878432,0.072572005796824));
#64177=CARTESIAN_POINT('Origin',(0.00991814422157668,-0.0332583300700225,
0.0794167555683928));
#64178=CARTESIAN_POINT('',(0.00253983500398563,-0.0317755397360895,0.0727724453423437));
#64179=CARTESIAN_POINT('Origin',(0.011819375542347,-0.0326853491204354,
0.0704450787941925));
#64180=CARTESIAN_POINT('',(0.00249965829285137,-0.0317744765475852,0.0729520334682077));
#64181=CARTESIAN_POINT('Ctrl Pts',(0.00253983477722505,-0.0317755400678203,
0.0727724452987978));
#64182=CARTESIAN_POINT('Ctrl Pts',(0.0025331283922866,-0.0317748838918833,
0.0728023693402364));
#64183=CARTESIAN_POINT('Ctrl Pts',(0.00252643180798999,-0.0317744615156214,
0.0728323012371319));
#64184=CARTESIAN_POINT('Ctrl Pts',(0.00251304460285598,-0.0317741013466568,
0.0728921673422743));
#64185=CARTESIAN_POINT('Ctrl Pts',(0.00250635378587497,-0.0317741635377321,
0.0729221024289259));
#64186=CARTESIAN_POINT('Ctrl Pts',(0.00249965829310926,-0.0317744765473203,
0.0729520334682682));
#64187=CARTESIAN_POINT('',(0.00246316203497268,-0.0317755400071255,0.0731324026212159));
#64188=CARTESIAN_POINT('Ctrl Pts',(0.0024996582928514,-0.0317744765475851,
0.0729520334682077));
#64189=CARTESIAN_POINT('Ctrl Pts',(0.00249357508374126,-0.031774163537956,
0.0729820949252851));
#64190=CARTESIAN_POINT('Ctrl Pts',(0.00248748595522708,-0.0317741013468101,
0.073012158173287));
#64191=CARTESIAN_POINT('Ctrl Pts',(0.00247531463125164,-0.0317744615102666,
0.0730722822974274));
#64192=CARTESIAN_POINT('Ctrl Pts',(0.00246923225753412,-0.0317748838660336,
0.0731023440517231));
#64193=CARTESIAN_POINT('Ctrl Pts',(0.00246316203497269,-0.0317755400071256,
0.0731324026212159));
#64194=CARTESIAN_POINT('',(0.00232875449738658,-0.0318824481878429,0.0732915461918387));
#64195=CARTESIAN_POINT('Origin',(0.010564094601645,-0.0332583300617367,
0.0791503323998404));
#64196=CARTESIAN_POINT('',(0.00241121271576042,-0.0317755397360895,0.0734831619295401));
#64197=CARTESIAN_POINT('Origin',(0.0113258849301056,-0.0326853491204514,
0.0700111125401321));
#64198=CARTESIAN_POINT('',(0.002393861170518,-0.0317744765475852,0.073666369426511));
#64199=CARTESIAN_POINT('Ctrl Pts',(0.00241121248533015,-0.0317755400678203,
0.0734831619147582));
#64200=CARTESIAN_POINT('Ctrl Pts',(0.00240830945911483,-0.0317748838918833,
0.0735136905291024));
#64201=CARTESIAN_POINT('Ctrl Pts',(0.00240541714081022,-0.0317744615156214,
0.073544225708614));
#64202=CARTESIAN_POINT('Ctrl Pts',(0.0023996387103257,-0.0317741013466568,
0.0736052976133437));
#64203=CARTESIAN_POINT('Ctrl Pts',(0.00239675251364211,-0.0317741635377321,
0.0736358352346231));
#64204=CARTESIAN_POINT('Ctrl Pts',(0.00239386117078142,-0.0317744765473203,
0.0736663694265387));
#64205=CARTESIAN_POINT('',(0.0023802589457153,-0.0317755400071255,0.0738498905088876));
#64206=CARTESIAN_POINT('Ctrl Pts',(0.00239386117051799,-0.0317744765475851,
0.073666369426511));
#64207=CARTESIAN_POINT('Ctrl Pts',(0.0023915933825296,-0.0317741635039404,
0.0736969595922481));
#64208=CARTESIAN_POINT('Ctrl Pts',(0.00238932068579902,-0.0317741013272396,
0.0737275423046233));
#64209=CARTESIAN_POINT('Ctrl Pts',(0.00238478064055958,-0.0317744615102666,
0.0737887211276194));
#64210=CARTESIAN_POINT('Ctrl Pts',(0.00238251396504818,-0.0317748838660336,
0.0738193081595674));
#64211=CARTESIAN_POINT('Ctrl Pts',(0.00238025894571531,-0.0317755400071256,
0.0738498905088876));
#64212=CARTESIAN_POINT('',(0.0022668572300156,-0.0318824481878425,0.0740246249162233));
#64213=CARTESIAN_POINT('Origin',(0.0111715598869108,-0.0332583300696574,
0.0788050510671788));
#64214=CARTESIAN_POINT('',(0.00237268106071657,-0.0317755397360895,0.0742043949514572));
#64215=CARTESIAN_POINT('Origin',(0.0107818952449207,-0.0326853491204138,
0.0696424190137116));
#64216=CARTESIAN_POINT('',(0.00237842832559961,-0.0317744765475852,0.0743883325278656));
#64217=CARTESIAN_POINT('Ctrl Pts',(0.00237268083025065,-0.0317755400678204,
0.0742043949656725));
#64218=CARTESIAN_POINT('Ctrl Pts',(0.00237362694521611,-0.0317748838918833,
0.0742350466984364));
#64219=CARTESIAN_POINT('Ctrl Pts',(0.00237458450649089,-0.0317744615156214,
0.074265703602543));
#64220=CARTESIAN_POINT('Ctrl Pts',(0.00237650608436353,-0.0317741013270863,
0.0743270214980914));
#64221=CARTESIAN_POINT('Ctrl Pts',(0.00237746981646342,-0.0317741635037165,
0.0743576733943658));
#64222=CARTESIAN_POINT('Ctrl Pts',(0.00237842832586444,-0.0317744765473203,
0.07438833252786));
#64223=CARTESIAN_POINT('',(0.00238793464908376,-0.0317755400071256,0.074572111302511));
#64224=CARTESIAN_POINT('Ctrl Pts',(0.00237842832559961,-0.0317744765475852,
0.0743883325278656));
#64225=CARTESIAN_POINT('Ctrl Pts',(0.00238001238426591,-0.0317741635039242,
0.0744189657117954));
#64226=CARTESIAN_POINT('Ctrl Pts',(0.00238159063874809,-0.0317741013272851,
0.0744495921164671));
#64227=CARTESIAN_POINT('Ctrl Pts',(0.00238475413258085,-0.0317744615102831,
0.0745108575398308));
#64228=CARTESIAN_POINT('Ctrl Pts',(0.00238633890201153,-0.0317748838659621,
0.0745414874719487));
#64229=CARTESIAN_POINT('Ctrl Pts',(0.00238793464908377,-0.0317755400071257,
0.074572111302511));
#64230=CARTESIAN_POINT('',(0.00229732716806982,-0.0318824481878422,0.0747596808805746));
#64231=CARTESIAN_POINT('Origin',(0.0117309598519367,-0.0332583300698019,
0.0783863567654003));
#64232=CARTESIAN_POINT('',(0.00242484770607189,-0.0317755397360895,0.0749247701324961));
#64233=CARTESIAN_POINT('Origin',(0.0101959855290228,-0.0326853491203767,
0.0693448127321306));
#64234=CARTESIAN_POINT('',(0.0024536031432799,-0.0317744765475852,0.0751065369828829));
#64235=CARTESIAN_POINT('Ctrl Pts',(0.00242484747920488,-0.0317755400678203,
0.0749247701754843));
#64236=CARTESIAN_POINT('Ctrl Pts',(0.00242962781403169,-0.0317748838919549,
0.0749550616272295));
#64237=CARTESIAN_POINT('Ctrl Pts',(0.00243442015384011,-0.031774461515605,
0.0749853567799411));
#64238=CARTESIAN_POINT('Ctrl Pts',(0.00244401175038665,-0.031774101327041,
0.0750459503328312));
#64239=CARTESIAN_POINT('Ctrl Pts',(0.0024488095841822,-0.0317741635037326,
0.0750762397404218));
#64240=CARTESIAN_POINT('Ctrl Pts',(0.00245360314354193,-0.0317744765473203,
0.0751065369828442));
#64241=CARTESIAN_POINT('',(0.00248606809465078,-0.0317755400071256,0.0752876751487366));
#64242=CARTESIAN_POINT('Ctrl Pts',(0.0024536031432799,-0.0317744765475851,
0.0751065369828829));
#64243=CARTESIAN_POINT('Ctrl Pts',(0.00245901347869469,-0.0317741635379696,
0.0751367267961233));
#64244=CARTESIAN_POINT('Ctrl Pts',(0.00246441896965501,-0.0317741013467719,
0.075166920453516));
#64245=CARTESIAN_POINT('Ctrl Pts',(0.00247523552585244,-0.0317744615102528,
0.0752273030176307));
#64246=CARTESIAN_POINT('Ctrl Pts',(0.00248064674790228,-0.031774883866094,
0.0752574928024337));
#64247=CARTESIAN_POINT('Ctrl Pts',(0.00248606809465078,-0.0317755400071256,
0.0752876751487366));
#64248=CARTESIAN_POINT('',(0.00241968378242437,-0.0318824481878419,0.0754851218132336));
#64249=CARTESIAN_POINT('Origin',(0.0122334724704804,-0.0332583300697356,
0.0779008525869336));
#64250=CARTESIAN_POINT('',(0.00256688995266614,-0.0317755397360895,0.0756329267257202));
#64251=CARTESIAN_POINT('Origin',(0.00957739592850816,-0.0326853491203207,
0.0691229871243551));
#64252=CARTESIAN_POINT('',(0.00261820007177698,-0.0317744765475852,0.0758096562782736));
#64253=CARTESIAN_POINT('Ctrl Pts',(0.00256688973297591,-0.0317755400678204,
0.0756329267968033));
#64254=CARTESIAN_POINT('Ctrl Pts',(0.0025754288999625,-0.0317748838918833,
0.0756623802597942));
#64255=CARTESIAN_POINT('Ctrl Pts',(0.0025839804397121,-0.0317744615156214,
0.0756918358850788));
#64256=CARTESIAN_POINT('Ctrl Pts',(0.0026010907882075,-0.0317741013270863,
0.0757507494891987));
#64257=CARTESIAN_POINT('Ctrl Pts',(0.0026096470595172,-0.0317741635037165,
0.0757801987293597));
#64258=CARTESIAN_POINT('Ctrl Pts',(0.0026182000720321,-0.0317744765473204,
0.0758096562782024));
#64259=CARTESIAN_POINT('',(0.00267311165935758,-0.0317755400071256,0.0759852971782525));
#64260=CARTESIAN_POINT('Ctrl Pts',(0.002618200071777,-0.0317744765475852,
0.0758096562782736));
#64261=CARTESIAN_POINT('Ctrl Pts',(0.00262735252738243,-0.0317741635039242,
0.0758389331250288));
#64262=CARTESIAN_POINT('Ctrl Pts',(0.00263649767521997,-0.0317741013272851,
0.0758682048489508));
#64263=CARTESIAN_POINT('Ctrl Pts',(0.00265479787330016,-0.0317744615102831,
0.075926758777456));
#64264=CARTESIAN_POINT('Ctrl Pts',(0.00266395020864746,-0.0317748838659621,
0.0759560322978017));
#64265=CARTESIAN_POINT('Ctrl Pts',(0.00267311165935761,-0.0317755400071257,
0.0759852971782525));
#64266=CARTESIAN_POINT('',(0.00263199743617858,-0.0318824481878415,0.0761895070773348));
#64267=CARTESIAN_POINT('Origin',(0.0126711728188753,-0.0332583300697157,
0.0773561952226392));
#64268=CARTESIAN_POINT('',(0.00279656770941877,-0.0317755397360895,0.0763176966786222));
#64269=CARTESIAN_POINT('Origin',(0.00893588197120081,-0.0326853491203759,
0.0689804405125556));
#64270=CARTESIAN_POINT('',(0.00286962331920213,-0.0317744765475852,0.0764866018027231));
#64271=CARTESIAN_POINT('Ctrl Pts',(0.00279656750036996,-0.0317755400678203,
0.0763176967766793));
#64272=CARTESIAN_POINT('Ctrl Pts',(0.00280873083123078,-0.0317748838918833,
0.0763458477489071));
#64273=CARTESIAN_POINT('Ctrl Pts',(0.00282090670829858,-0.0317744615156214,
0.0763739993156591));
#64274=CARTESIAN_POINT('Ctrl Pts',(0.00284526596909028,-0.0317741013270863,
0.0764303038731084));
#64275=CARTESIAN_POINT('Ctrl Pts',(0.00285744574014045,-0.0317741635037164,
0.0764584485120642));
#64276=CARTESIAN_POINT('Ctrl Pts',(0.00286962331944631,-0.0317744765473203,
0.0764866018026204));
#64277=CARTESIAN_POINT('',(0.00294611555445444,-0.0317755400071255,0.0766539754749139));
#64278=CARTESIAN_POINT('Ctrl Pts',(0.00286962331920212,-0.0317744765475852,
0.0764866018027231));
#64279=CARTESIAN_POINT('Ctrl Pts',(0.0028823729661738,-0.0317741635039404,
0.0765145006844968));
#64280=CARTESIAN_POINT('Ctrl Pts',(0.00289511472089743,-0.0317741013272396,
0.0765423953996442));
#64281=CARTESIAN_POINT('Ctrl Pts',(0.00292060937168583,-0.0317744615102667,
0.076598193994396));
#64282=CARTESIAN_POINT('Ctrl Pts',(0.00293335848381762,-0.0317748838660339,
0.0766260895940772));
#64283=CARTESIAN_POINT('Ctrl Pts',(0.00294611555445441,-0.0317755400071257,
0.0766539754749139));
#64284=CARTESIAN_POINT('',(0.00293091981618271,-0.0318824481878412,0.076861728096484));
#64285=CARTESIAN_POINT('Origin',(0.0130371580999669,-0.033258330069632,
0.0767609742442826));
#64286=CARTESIAN_POINT('',(0.00311025882090281,-0.0317755397360895,0.076968280759983));
#64287=CARTESIAN_POINT('Origin',(0.00828156071521838,-0.032685349120703,
0.0689194209423546));
#64288=CARTESIAN_POINT('',(0.00320390779075248,-0.0317744765475852,0.0771266977209283));
#64289=CARTESIAN_POINT('Ctrl Pts',(0.00311025862579223,-0.0317755400678203,
0.0769682808834677));
#64290=CARTESIAN_POINT('Ctrl Pts',(0.00312585429753271,-0.0317748838918833,
0.0769946854072822));
#64291=CARTESIAN_POINT('Ctrl Pts',(0.00314146249106465,-0.0317744615156213,
0.0770210889484786));
#64292=CARTESIAN_POINT('Ctrl Pts',(0.00317268480753182,-0.0317741013466568,
0.0770738936335047));
#64293=CARTESIAN_POINT('Ctrl Pts',(0.00318829938879392,-0.0317741635377321,
0.0771002955519336));
#64294=CARTESIAN_POINT('Ctrl Pts',(0.00320390779098185,-0.0317744765473203,
0.0771266977207958));
#64295=CARTESIAN_POINT('',(0.00330077434543096,-0.0317755400071256,0.0772831645825335));
#64296=CARTESIAN_POINT('Ctrl Pts',(0.00320390779075249,-0.0317744765475851,
0.0771266977209283));
#64297=CARTESIAN_POINT('Ctrl Pts',(0.00322005180560095,-0.031774163537956,
0.0771527758232258));
#64298=CARTESIAN_POINT('Ctrl Pts',(0.0032361927313619,-0.0317741013468102,
0.0771788592831621));
#64299=CARTESIAN_POINT('Ctrl Pts',(0.00326847801320322,-0.0317744615102666,
0.0772310197280091));
#64300=CARTESIAN_POINT('Ctrl Pts',(0.00328462284048518,-0.0317748838660336,
0.0772570974751015));
#64301=CARTESIAN_POINT('Ctrl Pts',(0.00330077434543096,-0.0317755400071256,
0.0772831645825335));
#64302=CARTESIAN_POINT('',(0.00331173673793648,-0.0318824481878409,0.077491183543644));
#64303=CARTESIAN_POINT('Origin',(0.013325656508119,-0.0332583300697143,
0.0761245766423453));
#64304=CARTESIAN_POINT('',(0.00350301619090027,-0.0317755397360894,0.0775744188701997));
#64305=CARTESIAN_POINT('Origin',(0.00762475119780743,-0.0326853491204433,
0.0689408907276665));
#64306=CARTESIAN_POINT('',(0.00361578162061684,-0.0317744765475852,0.0777198493378787));
#64307=CARTESIAN_POINT('Ctrl Pts',(0.00350301601280495,-0.0317755400678203,
0.0775744190171645));
#64308=CARTESIAN_POINT('Ctrl Pts',(0.00352179807236654,-0.0317748838918833,
0.077598660677454));
#64309=CARTESIAN_POINT('Ctrl Pts',(0.00354059243182567,-0.0317744615156214,
0.0776228997934755));
#64310=CARTESIAN_POINT('Ctrl Pts',(0.00357818673292297,-0.0317741013466568,
0.0776713749039054));
#64311=CARTESIAN_POINT('Ctrl Pts',(0.00359698722635675,-0.0317741635377321,
0.0776956116093609));
#64312=CARTESIAN_POINT('Ctrl Pts',(0.00361578162082781,-0.0317744765473204,
0.0777198493377185));
#64313=CARTESIAN_POINT('',(0.00373149485129061,-0.0317755400071255,0.0778629418130248));
#64314=CARTESIAN_POINT('Ctrl Pts',(0.00361578162061688,-0.0317744765475852,
0.0777198493378787));
#64315=CARTESIAN_POINT('Ctrl Pts',(0.00363506888290464,-0.031774163503954,
0.0777437010156738));
#64316=CARTESIAN_POINT('Ctrl Pts',(0.00365434746464147,-0.0317741013272014,
0.0777675506203995));
#64317=CARTESIAN_POINT('Ctrl Pts',(0.00369291770291779,-0.0317744615102528,
0.0778152559410678));
#64318=CARTESIAN_POINT('Ctrl Pts',(0.00371220363269735,-0.031774883866094,
0.0778391045750569));
#64319=CARTESIAN_POINT('Ctrl Pts',(0.00373149485129058,-0.0317755400071256,
0.0778629418130247));
#64320=CARTESIAN_POINT('',(0.00376844249109501,-0.0318824481878408,0.0780679465303945));
#64321=CARTESIAN_POINT('Origin',(0.0135321181980821,-0.0332583300620928,
0.0754570388007481));
#64322=CARTESIAN_POINT('',(0.00396864580106426,-0.0317755397360895,0.0781265518491845));
#64323=CARTESIAN_POINT('Origin',(0.00697581169705831,-0.0326853491203594,
0.0690445112786724));
#64324=CARTESIAN_POINT('',(0.00409874931245924,-0.0317744765475852,0.0782567022982473));
#64325=CARTESIAN_POINT('Ctrl Pts',(0.00396864564279281,-0.0317755400678204,
0.0781265520173118));
#64326=CARTESIAN_POINT('Ctrl Pts',(0.00399031788587653,-0.0317748838918833,
0.078148248508612));
#64327=CARTESIAN_POINT('Ctrl Pts',(0.00401200201298715,-0.0317744615156214,
0.0781699409341198));
#64328=CARTESIAN_POINT('Ctrl Pts',(0.00405537777091025,-0.0317741013270863,
0.0782133243457021));
#64329=CARTESIAN_POINT('Ctrl Pts',(0.00407706296826219,-0.0317741635037165,
0.0782350088964372));
#64330=CARTESIAN_POINT('Ctrl Pts',(0.00409874931264841,-0.0317744765473204,
0.078256702298062));
#64331=CARTESIAN_POINT('',(0.00423148435235597,-0.0317755400071255,0.0783841637331207));
#64332=CARTESIAN_POINT('Ctrl Pts',(0.00409874931245925,-0.0317744765475851,
0.0782567022982473));
#64333=CARTESIAN_POINT('Ctrl Pts',(0.0041208738989355,-0.0317741635039241,
0.0782779485655145));
#64334=CARTESIAN_POINT('Ctrl Pts',(0.00414298961362218,-0.031774101327285,
0.0782991938641527));
#64335=CARTESIAN_POINT('Ctrl Pts',(0.00418723476963576,-0.031774461510283,
0.0783416888751821));
#64336=CARTESIAN_POINT('Ctrl Pts',(0.00420935764821783,-0.031774883865962,
0.0783629322854281));
#64337=CARTESIAN_POINT('Ctrl Pts',(0.00423148435235597,-0.0317755400071256,
0.0783841637331206));
#64338=CARTESIAN_POINT('',(0.00429383455310798,-0.0318824481878405,0.078582921159893));
#64339=CARTESIAN_POINT('Origin',(0.0136532872535296,-0.033258330061942,
0.0747688881694887));
#64340=CARTESIAN_POINT('',(0.004499804394289,-0.0317755397360895,0.0786159722300308));
#64341=CARTESIAN_POINT('Origin',(0.00634497637698724,-0.0326853491204427,
0.0692286484364096));
#64342=CARTESIAN_POINT('',(0.00464519417726763,-0.0317744765475852,0.0787287901101476));
#64343=CARTESIAN_POINT('Ctrl Pts',(0.00449980425833748,-0.0317755400678204,
0.078615972416669));
#64344=CARTESIAN_POINT('Ctrl Pts',(0.00452402489621148,-0.0317748838920056,
0.0786347815688472));
#64345=CARTESIAN_POINT('Ctrl Pts',(0.00454825682165911,-0.0317744615155934,
0.0786535852031391));
#64346=CARTESIAN_POINT('Ctrl Pts',(0.00459672793863523,-0.0317741013270089,
0.0786911901046868));
#64347=CARTESIAN_POINT('Ctrl Pts',(0.0046209599343138,-0.0317741635037441,
0.0787099857885914));
#64348=CARTESIAN_POINT('Ctrl Pts',(0.00464519417743208,-0.0317744765473204,
0.0787287901099401));
#64349=CARTESIAN_POINT('',(0.00479285771551606,-0.0317755400071256,0.0788386103617785));
#64350=CARTESIAN_POINT('Ctrl Pts',(0.0046451941772676,-0.0317744765475852,
0.0787287901101476));
#64351=CARTESIAN_POINT('Ctrl Pts',(0.00466980716687401,-0.0317741635039404,
0.0787470958973389));
#64352=CARTESIAN_POINT('Ctrl Pts',(0.00469441123316321,-0.0317741013272396,
0.0787654018354073));
#64353=CARTESIAN_POINT('Ctrl Pts',(0.00474363354398586,-0.0317744615102667,
0.0788020163750381));
#64354=CARTESIAN_POINT('Ctrl Pts',(0.00476824448374763,-0.0317748838660338,
0.0788203195437703));
#64355=CARTESIAN_POINT('Ctrl Pts',(0.00479285771551602,-0.0317755400071257,
0.0788386103617786));
#64356=CARTESIAN_POINT('',(0.00487962717730369,-0.0318824481878404,0.0790279859746015));
#64357=CARTESIAN_POINT('Origin',(0.0136872527565295,-0.0332583300699954,
0.0740709772763413));
#64358=CARTESIAN_POINT('',(0.00508811528226063,-0.0317755397360895,0.0790349615609672));
#64359=CARTESIAN_POINT('Origin',(0.00574219388719208,-0.0326853491204695,
0.0694903982482642));
#64360=CARTESIAN_POINT('',(0.00524649845309392,-0.0317744765475852,0.0791286676667744));
#64361=CARTESIAN_POINT('Ctrl Pts',(0.00508811517077312,-0.0317755400678204,
0.0790349617631729));
#64362=CARTESIAN_POINT('Ctrl Pts',(0.00511450223846017,-0.0317748838918833,
0.0790505869516141));
#64363=CARTESIAN_POINT('Ctrl Pts',(0.00514089980569581,-0.0317744615156214,
0.0790662052465609));
#64364=CARTESIAN_POINT('Ctrl Pts',(0.00519369898120271,-0.0317741013466568,
0.0790974368791144));
#64365=CARTESIAN_POINT('Ctrl Pts',(0.00522010136427528,-0.0317741635377321,
0.079113050674707));
#64366=CARTESIAN_POINT('Ctrl Pts',(0.00524649845323109,-0.0317744765473204,
0.0791286676665479));
#64367=CARTESIAN_POINT('',(0.00540676174748558,-0.0317755400071255,0.079219114804191));
#64368=CARTESIAN_POINT('Ctrl Pts',(0.00524649845309391,-0.0317744765475852,
0.0791286676667744));
#64369=CARTESIAN_POINT('Ctrl Pts',(0.00527320878412476,-0.0317741635379398,
0.079143742644332));
#64370=CARTESIAN_POINT('Ctrl Pts',(0.00529991898931921,-0.0317741013468556,
0.0791588238050543));
#64371=CARTESIAN_POINT('Ctrl Pts',(0.00535333927914465,-0.0317744615102831,
0.0791889787957524));
#64372=CARTESIAN_POINT('Ctrl Pts',(0.00538005014810841,-0.0317748838659619,
0.0792040530690213));
#64373=CARTESIAN_POINT('Ctrl Pts',(0.00540676174748559,-0.0317755400071256,
0.079219114804191));
#64374=CARTESIAN_POINT('',(0.00551658206406282,-0.0318824481878402,0.079396122036523));
#64375=CARTESIAN_POINT('Origin',(0.0136334789566357,-0.0332583300695342,
0.0733743126384046));
#64376=CARTESIAN_POINT('',(0.0057243004508357,-0.0317755397360895,0.0793769121299523));
#64377=CARTESIAN_POINT('Origin',(0.00517697046763587,-0.0326853491204486,
0.0698256327630568));
#64378=CARTESIAN_POINT('',(0.00589317921230553,-0.0317744765475852,0.0794500286601838));
#64379=CARTESIAN_POINT('Ctrl Pts',(0.0057243003655704,-0.0317755400678203,
0.0793769123445366));
#64380=CARTESIAN_POINT('Ctrl Pts',(0.00575243771566211,-0.0317748838919551,
0.0793891071458487));
#64381=CARTESIAN_POINT('Ctrl Pts',(0.00578058462318907,-0.0317744615156049,
0.0794012937941031));
#64382=CARTESIAN_POINT('Ctrl Pts',(0.00583688488645091,-0.0317741013270408,
0.0794256629905367));
#64383=CARTESIAN_POINT('Ctrl Pts',(0.00586502988702687,-0.0317741635037327,
0.0794378419216701));
#64384=CARTESIAN_POINT('Ctrl Pts',(0.00589317921241321,-0.0317744765473204,
0.0794500286599419));
#64385=CARTESIAN_POINT('',(0.00606351481495193,-0.0317755400071256,0.079519676277999));
#64386=CARTESIAN_POINT('Ctrl Pts',(0.00589317921230552,-0.0317744765475851,
0.0794500286601838));
#64387=CARTESIAN_POINT('Ctrl Pts',(0.00592156832008162,-0.0317741635379398,
0.0794616370748831));
#64388=CARTESIAN_POINT('Ctrl Pts',(0.00594995807796962,-0.0317741013468556,
0.0794732516397625));
#64389=CARTESIAN_POINT('Ctrl Pts',(0.00600673655534851,-0.0317744615102831,
0.0794964735116913));
#64390=CARTESIAN_POINT('Ctrl Pts',(0.00603512610854758,-0.031774883865962,
0.0795080811602356));
#64391=CARTESIAN_POINT('Ctrl Pts',(0.0060635148149519,-0.0317755400071257,
0.079519676277999));
#64392=CARTESIAN_POINT('',(0.00619465405432301,-0.0318824481878401,0.0796815236200473));
#64393=CARTESIAN_POINT('Origin',(0.0134928139021324,-0.0332583300607513,
0.0726898810955411));
#64394=CARTESIAN_POINT('',(0.00639832687986726,-0.0317755397360895,0.0796364311722422));
#64395=CARTESIAN_POINT('Origin',(0.00465821950616128,-0.0326853484023168,
0.0702290644721585));
#64396=CARTESIAN_POINT('',(0.00657503791302196,-0.0317744765475852,0.0796878050355386));
#64397=CARTESIAN_POINT('Ctrl Pts',(0.00639832682216884,-0.0317755400678204,
0.0796364313958211));
#64398=CARTESIAN_POINT('Ctrl Pts',(0.00642777071795408,-0.0317748838918833,
0.0796450034933495));
#64399=CARTESIAN_POINT('Ctrl Pts',(0.00645722306908044,-0.0317744615156214,
0.079653566302823));
#64400=CARTESIAN_POINT('Ctrl Pts',(0.00651613045257276,-0.0317741013466568,
0.0796706861152094));
#64401=CARTESIAN_POINT('Ctrl Pts',(0.0065455863492945,-0.0317741635377321,
0.0796792433690345));
#64402=CARTESIAN_POINT('Ctrl Pts',(0.0065750379130985,-0.0317744765473203,
0.079687805035285));
#64403=CARTESIAN_POINT('',(0.00675275952971589,-0.0317755400071255,0.0797355547492138));
#64404=CARTESIAN_POINT('Ctrl Pts',(0.00657503791302196,-0.0317744765475852,
0.0796878050355386));
#64405=CARTESIAN_POINT('Ctrl Pts',(0.00660465808435497,-0.0317741635379398,
0.0796957638157452));
#64406=CARTESIAN_POINT('Ctrl Pts',(0.00663427967149549,-0.0317741013468556,
0.0797037286161553));
#64407=CARTESIAN_POINT('Ctrl Pts',(0.00669352090591582,-0.0317744615102831,
0.0797196511465201));
#64408=CARTESIAN_POINT('Ctrl Pts',(0.00672314142313093,-0.0317748838659618,
0.0797276091107857));
#64409=CARTESIAN_POINT('Ctrl Pts',(0.00675275952971588,-0.0317755400071256,
0.0797355547492138));
#64410=CARTESIAN_POINT('',(0.0069031495477372,-0.0318824481878401,0.0798796897717117));
#64411=CARTESIAN_POINT('Origin',(0.0132674760598083,-0.0332583300604723,
0.072028476464189));
#64412=CARTESIAN_POINT('',(0.00709956476929273,-0.0317755397364821,0.079809425917849));
#64413=CARTESIAN_POINT('Origin',(0.00419412357676368,-0.0326853491206543,
0.0706943329874522));
#64414=CARTESIAN_POINT('',(0.00728132123621136,-0.0317744765475735,0.0798382469173586));
#64415=CARTESIAN_POINT('Ctrl Pts',(0.00709956474006579,-0.0317755400683136,
0.0798094261469438));
#64416=CARTESIAN_POINT('Ctrl Pts',(0.00712985083066187,-0.0317748838922172,
0.0798142403521005));
#64417=CARTESIAN_POINT('Ctrl Pts',(0.00716014414620153,-0.0317744615158801,
0.0798190442828555));
#64418=CARTESIAN_POINT('Ctrl Pts',(0.00722073270871306,-0.0317741013468555,
0.079828646047477));
#64419=CARTESIAN_POINT('Ctrl Pts',(0.0072510288455948,-0.0317741635379398,
0.0798334440220898));
#64420=CARTESIAN_POINT('Ctrl Pts',(0.0072813212362112,-0.0317744765475852,
0.0798382469173588));
#64421=CARTESIAN_POINT('',(0.0074636260908907,-0.0317755400071255,0.0798633456853848));
#64422=CARTESIAN_POINT('Ctrl Pts',(0.00728132123621146,-0.0317744765475851,
0.0798382469173587));
#64423=CARTESIAN_POINT('Ctrl Pts',(0.00731170534173171,-0.031774163537956,
0.0798424305481377));
#64424=CARTESIAN_POINT('Ctrl Pts',(0.00734209160632505,-0.0317741013468101,
0.0798466199741871));
#64425=CARTESIAN_POINT('Ctrl Pts',(0.00740286133299313,-0.0317744615102666,
0.0798549920558435));
#64426=CARTESIAN_POINT('Ctrl Pts',(0.00743324568268853,-0.0317748838660336,
0.0798591748342155));
#64427=CARTESIAN_POINT('Ctrl Pts',(0.00746362609089069,-0.0317755400071256,
0.0798633456853848));
#64428=CARTESIAN_POINT('',(0.00763089514713966,-0.0318824481878402,0.0799874952929255));
#64429=CARTESIAN_POINT('Origin',(0.0129610190916437,-0.0332583300609749,
0.0714005295268761));
#64430=CARTESIAN_POINT('',(0.00781695517999998,-0.0317755397364822,0.079893168135698));
#64431=CARTESIAN_POINT('Origin',(0.00379200018792774,-0.0326853491206267,
0.0712140987753191));
#64432=CARTESIAN_POINT('Ctrl Pts',(0.0078169551797167,-0.0317755400683137,
0.0798931683666495));
#64433=CARTESIAN_POINT('Ctrl Pts',(0.00784760582917376,-0.0317748838923494,
0.0798941487564968));
#64434=CARTESIAN_POINT('Ctrl Pts',(0.00787826236822532,-0.0317744615158499,
0.0798951180477344));
#64435=CARTESIAN_POINT('Ctrl Pts',(0.00793957660105809,-0.0317741013467719,
0.0798970503394014));
#64436=CARTESIAN_POINT('Ctrl Pts',(0.00797023518641224,-0.0317741635379696,
0.0798980133676535));
#64437=CARTESIAN_POINT('Ctrl Pts',(0.00800089067195264,-0.0317744765475852,
0.079898981747298));
#64438=CARTESIAN_POINT('Origin',(0.00812378219310841,-0.0355241814719619,
0.07415));
#64439=CARTESIAN_POINT('',(0.00808309105517532,-0.0351949306059337,0.0683208911579615));
#64440=CARTESIAN_POINT('',(0.00812378219275222,-0.0351704285080635,0.0682962470361016));
#64441=CARTESIAN_POINT('Ctrl Pts',(0.00812378219239603,-0.0351704285080635,
0.0682962470361016));
#64442=CARTESIAN_POINT('Ctrl Pts',(0.00811019485630785,-0.0351786035562758,
0.0683044220843155));
#64443=CARTESIAN_POINT('Ctrl Pts',(0.00809663611840715,-0.0351867679503489,
0.0683126337499256));
#64444=CARTESIAN_POINT('Ctrl Pts',(0.00808309105565127,-0.035194930606244,
0.0683208911584355));
#64445=CARTESIAN_POINT('',(0.00812378219310841,-0.0355241814719745,0.0686500000000126));
#64446=CARTESIAN_POINT('',(0.00812378219310841,-0.0355241814719619,0.06865));
#64447=CARTESIAN_POINT('Origin',(0.00812378219311841,-0.0355241814719719,
0.07415000000001));
#64448=CARTESIAN_POINT('',(0.00825051023896004,-0.035094370708599,0.0682215435661843));
#64449=CARTESIAN_POINT('Ctrl Pts',(0.00825051024267582,-0.035094370714152,
0.0682215435714773));
#64450=CARTESIAN_POINT('Ctrl Pts',(0.00822342491110835,-0.0351105857202016,
0.0682371832994888));
#64451=CARTESIAN_POINT('Ctrl Pts',(0.00819642805189303,-0.0351267738254377,
0.0682529789241719));
#64452=CARTESIAN_POINT('Ctrl Pts',(0.00815423794672532,-0.035152112510921,
0.0682779903654756));
#64453=CARTESIAN_POINT('Ctrl Pts',(0.00813899690518094,-0.035161274321419,
0.0682870928494552));
#64454=CARTESIAN_POINT('Ctrl Pts',(0.00812378219239603,-0.0351704285080635,
0.0682962470361016));
#64455=CARTESIAN_POINT('',(0.0084138644635775,-0.035195137125492,0.0683281780970644));
#64456=CARTESIAN_POINT('Origin',(0.00335368224046308,-0.0338370705272818,
0.0771371906830081));
#64457=CARTESIAN_POINT('',(0.00842661992254915,-0.0352722979006255,0.0684060942064975));
#64458=CARTESIAN_POINT('Origin',(0.0137020032039043,-0.0346069579033217,
0.0681231525239146));
#64459=CARTESIAN_POINT('',(0.00860741083993109,-0.0352740680168103,0.0684201085860881));
#64460=CARTESIAN_POINT('Origin',(0.00861719186418346,-0.0305802162291841,
0.06765606648571));
#64461=CARTESIAN_POINT('',(0.00878811029711487,-0.0352728165321731,0.0684371314675367));
#64462=CARTESIAN_POINT('Origin',(0.0085644044276215,-0.0288496123715138,
0.069309525093856));
#64463=CARTESIAN_POINT('',(0.00881399297514621,-0.0351949306052073,0.0683617554737295));
#64464=CARTESIAN_POINT('Ctrl Pts',(0.00878811029168475,-0.0352728165303531,
0.0684371314675542));
#64465=CARTESIAN_POINT('Ctrl Pts',(0.00879672353338646,-0.0352468764909534,
0.068412018231727));
#64466=CARTESIAN_POINT('Ctrl Pts',(0.00880535111903101,-0.0352209141752707,
0.0683868926325456));
#64467=CARTESIAN_POINT('Ctrl Pts',(0.00881399297658388,-0.035194930607398,
0.0683617554719593));
#64468=CARTESIAN_POINT('',(0.00899254353630529,-0.0350943706855873,0.0682841744236151));
#64469=CARTESIAN_POINT('Origin',(0.0123257004762265,-0.0338370705480914,
0.0778944685611667));
#64470=CARTESIAN_POINT('',(0.00914124484256304,-0.0351951371254925,0.06841044185062));
#64471=CARTESIAN_POINT('Origin',(0.00301690163542675,-0.0338370705272569,
0.076515783741189));
#64472=CARTESIAN_POINT('',(0.00914413424298837,-0.0352722979006256,0.0684893422511767));
#64473=CARTESIAN_POINT('Origin',(0.0144133815475748,-0.0346069579035747,
0.0688698124929622));
#64474=CARTESIAN_POINT('',(0.00932174310247744,-0.0352740680168102,0.0685259052334733));
#64475=CARTESIAN_POINT('Origin',(0.00942720686743619,-0.0305802162290654,
0.0677691137207357));
#64476=CARTESIAN_POINT('',(0.00949888415769095,-0.035272816532173,0.0685654415316891));
#64477=CARTESIAN_POINT('Origin',(0.00916760236170185,-0.0288496123710761,
0.0694029182935395));
#64478=CARTESIAN_POINT('',(0.00953400986011256,-0.0351949306052073,0.0684939038598372));
#64479=CARTESIAN_POINT('Ctrl Pts',(0.00949888415230144,-0.0352728165303531,
0.0685654415310259));
#64480=CARTESIAN_POINT('Ctrl Pts',(0.00951057699907121,-0.0352468764909533,
0.068541605845998));
#64481=CARTESIAN_POINT('Ctrl Pts',(0.0095222856262167,-0.0352209141752705,
0.0685177596928773));
#64482=CARTESIAN_POINT('Ctrl Pts',(0.00953400986176051,-0.0351949306073977,
0.0684939038582614));
#64483=CARTESIAN_POINT('',(0.00972087598064153,-0.0350943706855873,0.0684393128786594));
#64484=CARTESIAN_POINT('Origin',(0.0118232607428322,-0.0338370705484021,
0.0783915823134132));
#64485=CARTESIAN_POINT('',(0.00985257922776396,-0.035195137125493,0.0685832218648373));
#64486=CARTESIAN_POINT('Origin',(0.00276065961398387,-0.0338370705322628,
0.0758570669485549));
#64487=CARTESIAN_POINT('',(0.00984555700207224,-0.0352722979006258,0.068661862250068));
#64488=CARTESIAN_POINT('Origin',(0.0150255691519021,-0.0346069579032499,
0.0696997441737871));
#64489=CARTESIAN_POINT('',(0.010017182805856,-0.0352740680168101,0.0687203972149985));
#64490=CARTESIAN_POINT('Origin',(0.0102166660849917,-0.0305802162292844,
0.0679827913439425));
#64491=CARTESIAN_POINT('',(0.0101879718388395,-0.035272816532173,0.0687818234189402));
#64492=CARTESIAN_POINT('Origin',(0.00975433862813941,-0.0288496123715215,
0.069571175807738));
#64493=CARTESIAN_POINT('',(0.0102317866123413,-0.0351949306052074,0.0687152522608634));
#64494=CARTESIAN_POINT('Ctrl Pts',(0.0101879718335757,-0.035272816530353,
0.0687818234176067));
#64495=CARTESIAN_POINT('Ctrl Pts',(0.010202559882235,-0.0352468764909531,
0.0687596411863698));
#64496=CARTESIAN_POINT('Ctrl Pts',(0.010217164898837,-0.0352209141752703,
0.0687374505473897));
#64497=CARTESIAN_POINT('Ctrl Pts',(0.0102317866141735,-0.0351949306073974,
0.0687152522595068));
#64498=CARTESIAN_POINT('',(0.010424021301891,-0.0350943706855873,0.0686845122810066));
#64499=CARTESIAN_POINT('Origin',(0.0112624780227344,-0.0338370705483178,
0.0788218037795066));
#64500=CARTESIAN_POINT('',(0.0105366494509951,-0.0351951371254935,0.0688437932956783));
#64501=CARTESIAN_POINT('Origin',(0.00258899722437033,-0.0338370705329863,
0.0751714287151622));
#64502=CARTESIAN_POINT('',(0.0105198263438801,-0.0352722979006259,0.0689209334597304));
#64503=CARTESIAN_POINT('Origin',(0.0155289113492698,-0.0346069579166609,
0.0705998590110601));
#64504=CARTESIAN_POINT('',(0.0106827624505072,-0.0352740680168103,0.0690005172759302));
#64505=CARTESIAN_POINT('Origin',(0.010973119273292,-0.0305802162291668,
0.0682937295319573));
#64506=CARTESIAN_POINT('',(0.0108445060161877,-0.0352728165321731,0.069082864657668));
#64507=CARTESIAN_POINT('Origin',(0.0103153600492251,-0.0288496124320004,
0.0698116441084991));
#64508=CARTESIAN_POINT('',(0.0108963188756178,-0.0351949306052075,0.0690223098802967));
#64509=CARTESIAN_POINT('Ctrl Pts',(0.0108445060111324,-0.0352728165303531,
0.0690828646556853));
#64510=CARTESIAN_POINT('Ctrl Pts',(0.0108617591994395,-0.0352468764909531,
0.0690626857052769));
#64511=CARTESIAN_POINT('Ctrl Pts',(0.0108790302756615,-0.0352209141752702,
0.0690425005400701));
#64512=CARTESIAN_POINT('Ctrl Pts',(0.0108963188776054,-0.0351949306073972,
0.0690223098791807));
#64513=CARTESIAN_POINT('',(0.0110908904782989,-0.0350943706855873,0.0690159056896065));
#64514=CARTESIAN_POINT('Origin',(0.0106521961942472,-0.0338370705480734,
0.0791783481085643));
#64515=CARTESIAN_POINT('',(0.0111826673161923,-0.0351951371254939,0.0691880467760207));
#64516=CARTESIAN_POINT('Origin',(0.00250462165323249,-0.0338370705271412,
0.0744696819722123));
#64517=CARTESIAN_POINT('',(0.0111563086381029,-0.0352722979006261,0.0692624701724259));
#64518=CARTESIAN_POINT('Origin',(0.0159154704425166,-0.0346069579032674,
0.0715559617640655));
#64519=CARTESIAN_POINT('',(0.0113079854478385,-0.0352740680168103,0.0693618477555725));
#64520=CARTESIAN_POINT('Origin',(0.0116846367137315,-0.0305802162290746,
0.0686970246035787));
#64521=CARTESIAN_POINT('',(0.0114581327535644,-0.035272816532173,0.0694638176477042));
#64522=CARTESIAN_POINT('Origin',(0.0108418189710028,-0.0288496123714861,
0.0701205308855496));
#64523=CARTESIAN_POINT('',(0.0115171265791785,-0.0351949306052074,0.0694102342360514));
#64524=CARTESIAN_POINT('Ctrl Pts',(0.0114581327487975,-0.0352728165303531,
0.0694638176451035));
#64525=CARTESIAN_POINT('Ctrl Pts',(0.0114777789836662,-0.0352468764909529,
0.069445960209626));
#64526=CARTESIAN_POINT('Ctrl Pts',(0.0114974437443192,-0.0352209141752698,
0.0694280988503058));
#64527=CARTESIAN_POINT('Ctrl Pts',(0.01151712658129,-0.0351949306073967,
0.0694102342351935));
#64528=CARTESIAN_POINT('',(0.011710966584585,-0.0350943706855873,0.0694282668324408));
#64529=CARTESIAN_POINT('Origin',(0.0100020397743013,-0.0338370705544373,
0.0794555923382736));
#64530=CARTESIAN_POINT('',(0.0117804447357093,-0.0351951371254944,0.0696105532228325));
#64531=CARTESIAN_POINT('Origin',(0.00250886368030171,-0.0338370705332249,
0.0737628936041924));
#64532=CARTESIAN_POINT('',(0.0117449661787447,-0.0352722979006265,0.0696810861501711));
#64533=CARTESIAN_POINT('Origin',(0.0161791498534244,-0.0346069579034337,
0.0725529740133547));
#64534=CARTESIAN_POINT('',(0.0118829916576916,-0.0352740680168101,0.0697986902564126));
#64535=CARTESIAN_POINT('Origin',(0.0123399973512426,-0.0305802162291525,
0.0691863163546208));
#64536=CARTESIAN_POINT('',(0.0120191747907581,-0.0352728165321731,0.0699186745328258));
#64537=CARTESIAN_POINT('Origin',(0.0113254128382053,-0.0288496124326838,
0.0704929647860157));
#64538=CARTESIAN_POINT('',(0.0120844192146853,-0.0351949306052073,0.0698729075293024));
#64539=CARTESIAN_POINT('Ctrl Pts',(0.0120191747863548,-0.0352728165303531,
0.0699186745296482));
#64540=CARTESIAN_POINT('Ctrl Pts',(0.0120409042349252,-0.0352468764909528,
0.0699034202315265));
#64541=CARTESIAN_POINT('Ctrl Pts',(0.0120626525549864,-0.0352209141752695,
0.0698881643623993));
#64542=CARTESIAN_POINT('Ctrl Pts',(0.0120844192168873,-0.0351949306073962,
0.0698729075287162));
#64543=CARTESIAN_POINT('',(0.0122744706501375,-0.0350943706855873,0.0699150925279542));
#64544=CARTESIAN_POINT('Origin',(0.00932226209534658,-0.0338370705483705,
0.0796491642990803));
#64545=CARTESIAN_POINT('',(0.012320554402545,-0.0351951371254947,0.0701046494570542));
#64546=CARTESIAN_POINT('Origin',(0.00260165624639857,-0.0338370705282117,
0.073062210172673));
#64547=CARTESIAN_POINT('',(0.0122765154847423,-0.0352722979006269,0.0701701795689278));
#64548=CARTESIAN_POINT('Origin',(0.0163157913041077,-0.0346069579032108,
0.0735751723167505));
#64549=CARTESIAN_POINT('',(0.0123987128886455,-0.0352740680168101,0.0703041555112558));
#64550=CARTESIAN_POINT('Origin',(0.0129288657570403,-0.0305802162290188,
0.0697538883619407));
#64551=CARTESIAN_POINT('',(0.0125187841596924,-0.035272816532173,0.070440261948236));
#64552=CARTESIAN_POINT('Origin',(0.0117585150668984,-0.0288496123714419,
0.0709230723270721));
#64553=CARTESIAN_POINT('',(0.0125892502383923,-0.035194930605207,0.0704030331258278));
#64554=CARTESIAN_POINT('Ctrl Pts',(0.012518784155722,-0.035272816530353,
0.0704402619445316));
#64555=CARTESIAN_POINT('Ctrl Pts',(0.0125422541316097,-0.0352468764909525,
0.0704278513531597));
#64556=CARTESIAN_POINT('Ctrl Pts',(0.0125657430270801,-0.035220914175269,
0.070415441568395));
#64557=CARTESIAN_POINT('Ctrl Pts',(0.0125892502406501,-0.0351949306073955,
0.0704030331255223));
#64558=CARTESIAN_POINT('',(0.0127725158792218,-0.0350943706855873,0.0704687052441133));
#64559=CARTESIAN_POINT('Origin',(0.00862358367950969,-0.0338370705479122,
0.0797560111077919));
#64560=CARTESIAN_POINT('',(0.012794478464608,-0.0351951371254951,0.0706625432859136));
#64561=CARTESIAN_POINT('Origin',(0.002781536070095,-0.0338370705270207,
0.0723786818205332));
#64562=CARTESIAN_POINT('',(0.0127425737060082,-0.0352722979006273,0.0707220371333118));
#64563=CARTESIAN_POINT('Origin',(0.01632323987826,-0.0346069579035876,0.0746064359959854));
#64564=CARTESIAN_POINT('',(0.0128470159088111,-0.0352740680168102,0.0708702720310826));
#64565=CARTESIAN_POINT('Origin',(0.013441955124631,-0.0305802162290379,
0.0703907896758804));
#64566=CARTESIAN_POINT('',(0.0129490817221664,-0.0352728165321731,0.0710203541488127));
#64567=CARTESIAN_POINT('Origin',(0.0121342953984036,-0.0288496124323702,
0.0714040704362385));
#64568=CARTESIAN_POINT('',(0.0130236581634837,-0.0351949306052069,0.0709922506282884));
#64569=CARTESIAN_POINT('Ctrl Pts',(0.0129490817186916,-0.0352728165303531,
0.0710203541446399));
#64570=CARTESIAN_POINT('Ctrl Pts',(0.0129739220863566,-0.0352468764909524,
0.0710109829824574));
#64571=CARTESIAN_POINT('Ctrl Pts',(0.0129987811233229,-0.0352209141752687,
0.0710016149917742));
#64572=CARTESIAN_POINT('Ctrl Pts',(0.0130236581657616,-0.035194930607395,
0.0709922506282686));
#64573=CARTESIAN_POINT('',(0.0131972478006323,-0.0350943706857667,0.0710803741771032));
#64574=CARTESIAN_POINT('Origin',(0.00791702309657988,-0.0338370705483001,
0.0797744477714516));
#64575=CARTESIAN_POINT('',(0.0131947428563309,-0.0351951371254954,0.0712754363904597));
#64576=CARTESIAN_POINT('Origin',(0.003045666357819,-0.0338370705334225,
0.0717230882096386));
#64577=CARTESIAN_POINT('',(0.0131357908259834,-0.0352722979006277,0.0713279557198694));
#64578=CARTESIAN_POINT('Origin',(0.0162013781061114,-0.0346069579034164,
0.075630501407276));
#64579=CARTESIAN_POINT('',(0.0132208307117569,-0.0352740680168102,0.0714881118201936));
#64580=CARTESIAN_POINT('Origin',(0.0138711737281729,-0.0305802162290074,
0.0710869759822714));
#64581=CARTESIAN_POINT('',(0.0133032814285732,-0.035272816532173,0.0716498027340223));
#64582=CARTESIAN_POINT('Origin',(0.012446827528811,-0.0288496123715279,
0.0719283735020433));
#64583=CARTESIAN_POINT('',(0.0133807921174785,-0.0351949306052067,0.0716312677246893));
#64584=CARTESIAN_POINT('Ctrl Pts',(0.0133032814256488,-0.035272816530353,
0.0716498027294469));
#64585=CARTESIAN_POINT('Ctrl Pts',(0.013329100437654,-0.0352468764909521,
0.0716436187852796));
#64586=CARTESIAN_POINT('Ctrl Pts',(0.0133549375742533,-0.0352209141752683,
0.0716374403274873));
#64587=CARTESIAN_POINT('Ctrl Pts',(0.0133807921197406,-0.0351949306073944,
0.0716312677249552));
#64588=CARTESIAN_POINT('',(0.013541968139514,-0.0350943706855873,0.0717404529441539));
#64589=CARTESIAN_POINT('Origin',(0.00721372322735028,-0.0338370705482336,
0.0797041835349999));
#64590=CARTESIAN_POINT('',(0.0135150351691498,-0.0351951371254956,0.0719336630803094));
#64591=CARTESIAN_POINT('Origin',(0.00338988147407706,-0.0338370705268427,
0.0711057684529389));
#64592=CARTESIAN_POINT('',(0.0134499655757892,-0.0352722979006282,0.0719783796305319));
#64593=CARTESIAN_POINT('Origin',(0.0159521278207605,-0.0346069579033098,
0.0766312184265049));
#64594=CARTESIAN_POINT('',(0.0135142620147343,-0.0352740680168101,0.072147931176035));
#64595=CARTESIAN_POINT('Origin',(0.0142097525339431,-0.0305802162291656,
0.0718314680071569));
#64596=CARTESIAN_POINT('',(0.0135757973379538,-0.035272816532173,0.072318680923662));
#64597=CARTESIAN_POINT('Origin',(0.0126911826582227,-0.0288496123714389,
0.0724877129411867));
#64598=CARTESIAN_POINT('',(0.0136550198845806,-0.0351949306052065,0.0723100067336897));
#64599=CARTESIAN_POINT('Ctrl Pts',(0.0135757973356259,-0.035272816530353,
0.0723186809187561));
#64600=CARTESIAN_POINT('Ctrl Pts',(0.0136021878107285,-0.0352468764909519,
0.0723157817170976));
#64601=CARTESIAN_POINT('Ctrl Pts',(0.0136285955798824,-0.0352209141752679,
0.0723128902301664));
#64602=CARTESIAN_POINT('Ctrl Pts',(0.0136550198867911,-0.0351949306073937,
0.0723100067342372));
#64603=CARTESIAN_POINT('',(0.0138012404489288,-0.0350943706855873,0.0724385317071006));
#64604=CARTESIAN_POINT('Origin',(0.00652477553238292,-0.0338370705485876,
0.0795463265056502));
#64605=CARTESIAN_POINT('',(0.0137503042019585,-0.0351951371254957,0.0726268427273582));
#64606=CARTESIAN_POINT('Origin',(0.00380875312443852,-0.0338370705334268,
0.0705364580523133));
#64607=CARTESIAN_POINT('',(0.0136801432319426,-0.0352722979006287,0.0726630512916841));
#64608=CARTESIAN_POINT('Origin',(0.0155794198489981,-0.0346069579034531,
0.0775928051493414));
#64609=CARTESIAN_POINT('',(0.0137226822308082,-0.0352740680168101,0.0728393243532072));
#64610=CARTESIAN_POINT('Origin',(0.0144523519517679,-0.030580216229071,
0.072612524666635));
#64611=CARTESIAN_POINT('',(0.0137623317116241,-0.035272816532173,0.0730164401091124));
#64612=CARTESIAN_POINT('Origin',(0.0128635071531246,-0.0288496123714632,
0.0730732676405112));
#64613=CARTESIAN_POINT('',(0.013842016729087,-0.0351949306052061,0.0730177635356588));
#64614=CARTESIAN_POINT('Ctrl Pts',(0.0137623317099295,-0.035272816530353,
0.0730164401039535));
#64615=CARTESIAN_POINT('Ctrl Pts',(0.0137888774545723,-0.0352468764909517,
0.0730168713669459));
#64616=CARTESIAN_POINT('Ctrl Pts',(0.0138154393899859,-0.0352209141752674,
0.0730173124513521));
#64617=CARTESIAN_POINT('Ctrl Pts',(0.0138420167312112,-0.035194930607393,
0.0730177635364791));
#64618=CARTESIAN_POINT('',(0.0139709758501003,-0.0350943706855873,0.0731636013474081));
#64619=CARTESIAN_POINT('Origin',(0.00586104512645934,-0.0338370705482262,
0.0793033661844569));
#64620=CARTESIAN_POINT('',(0.0138968396215665,-0.0351951371254958,0.0733440434744868));
#64621=CARTESIAN_POINT('Origin',(0.00429567531282297,-0.0338370705328629,
0.070024135363444));
#64622=CARTESIAN_POINT('',(0.0138226937553044,-0.0352722979006292,0.0733711730222263));
#64623=CARTESIAN_POINT('Origin',(0.0150891320168613,-0.0346069579032025,
0.0785000967776752));
#64624=CARTESIAN_POINT('',(0.0138428044486668,-0.0352740680168103,0.0735513876682886));
#64625=CARTESIAN_POINT('Origin',(0.0145951460440602,-0.0305802162291541,
0.0734178282305441));
#64626=CARTESIAN_POINT('',(0.0138599427910812,-0.0352728165321731,0.073732076211198));
#64627=CARTESIAN_POINT('Origin',(0.0129610833543958,-0.0288496123719289,
0.073675803052224));
#64628=CARTESIAN_POINT('',(0.0139388335990533,-0.0351949306052057,0.0737433763830361));
#64629=CARTESIAN_POINT('Ctrl Pts',(0.0138599427900465,-0.0352728165303531,
0.0737320762058673));
#64630=CARTESIAN_POINT('Ctrl Pts',(0.013886225161979,-0.0352468764909514,
0.0737358311322358));
#64631=CARTESIAN_POINT('Ctrl Pts',(0.0139125223660635,-0.0352209141752669,
0.0737395978318148));
#64632=CARTESIAN_POINT('Ctrl Pts',(0.0139388336010576,-0.0351949306073923,
0.0737433763841162));
#64633=CARTESIAN_POINT('',(0.0140484975143569,-0.0350943706855873,0.0739042270837131));
#64634=CARTESIAN_POINT('Origin',(0.00523299947751265,-0.033837070554829,
0.0789791341757105));
#64635=CARTESIAN_POINT('',(0.0139523304768704,-0.0351951371254958,0.074073954637478));
#64636=CARTESIAN_POINT('Origin',(0.00484296903637281,-0.0338370705331573,
0.0695768800252357));
#64637=CARTESIAN_POINT('',(0.0138753690389657,-0.0352722979006297,0.0740915773194568));
#64638=CARTESIAN_POINT('Origin',(0.0144889964576451,-0.0346069579032552,
0.0793387847816124));
#64639=CARTESIAN_POINT('',(0.0138727342691775,-0.0352740680168102,0.0742728914574353));
#64640=CARTESIAN_POINT('Origin',(0.0146358828626028,-0.0305802162292082,
0.0742346785806469));
#64641=CARTESIAN_POINT('',(0.0138670911912921,-0.035272816532173,0.0744543032210886));
#64642=CARTESIAN_POINT('Origin',(0.0129823724269125,-0.0288496123714457,
0.0742858168330627));
#64643=CARTESIAN_POINT('',(0.0139439436346045,-0.0351949306052053,0.0744754019277582));
#64644=CARTESIAN_POINT('Ctrl Pts',(0.0138670911909336,-0.035272816530353,
0.0744543032156703));
#64645=CARTESIAN_POINT('Ctrl Pts',(0.0138926957014499,-0.0352468764909512,
0.0744613225879828));
#64646=CARTESIAN_POINT('Ctrl Pts',(0.0139183134515877,-0.0352209141752664,
0.0744683554996323));
#64647=CARTESIAN_POINT('Ctrl Pts',(0.0139439436364572,-0.0351949306073916,
0.0744754019290811));
#64648=CARTESIAN_POINT('',(0.0140325828787443,-0.0350943706855873,0.0746487288057257));
#64649=CARTESIAN_POINT('Origin',(0.0046505431174405,-0.0338370705478985,
0.078578743883373));
#64650=CARTESIAN_POINT('',(0.0139159016439338,-0.0351951371254958,0.0748050650812635));
#64651=CARTESIAN_POINT('Origin',(0.0054420031031212,-0.0338370705270375,
0.0692017454954627));
#64652=CARTESIAN_POINT('',(0.0138373383622366,-0.0352722979006302,0.0748129029772593));
#64653=CARTESIAN_POINT('Origin',(0.0137884776670116,-0.0346069579032201,
0.0800956425500761));
#64654=CARTESIAN_POINT('',(0.0138119996811912,-0.0352740680168102,0.0749924571748874));
#64655=CARTESIAN_POINT('Origin',(0.0145739199633192,-0.0305802162289763,
0.075050193498937));
#64656=CARTESIAN_POINT('',(0.0137836641777151,-0.035272816532173,0.0751717311874006));
#64657=CARTESIAN_POINT('Origin',(0.0129270386287473,-0.0288496123715092,
0.0748936887013136));
#64658=CARTESIAN_POINT('',(0.0138572662474272,-0.035194930605205,0.0752022956896942));
#64659=CARTESIAN_POINT('Ctrl Pts',(0.0137836641780386,-0.035272816530353,
0.0751717311819801));
#64660=CARTESIAN_POINT('Ctrl Pts',(0.0138081870287124,-0.035246876490951,
0.0751819043005423));
#64661=CARTESIAN_POINT('Ctrl Pts',(0.0138327213176805,-0.035220914175266,
0.0751920925110443));
#64662=CARTESIAN_POINT('Ctrl Pts',(0.0138572662490992,-0.035194930607391,
0.0752022956912388));
#64663=CARTESIAN_POINT('',(0.0139234829265729,-0.0350943706855873,0.075385365276546));
#64664=CARTESIAN_POINT('Origin',(0.00412286189794218,-0.0338370705537578,
0.0781085096178728));
#64665=CARTESIAN_POINT('',(0.0137881276272134,-0.0351951371254958,0.0755258447574009));
#64666=CARTESIAN_POINT('Origin',(0.00608333050192936,-0.033837070532533,
0.0689046479421592));
#64667=CARTESIAN_POINT('',(0.0137092014916075,-0.0352722979006308,0.0755237742591112));
#64668=CARTESIAN_POINT('Origin',(0.0129986232703443,-0.0346069579246078,
0.0807587338069652));
#64669=CARTESIAN_POINT('',(0.013661558505442,-0.03527406801681,0.0756987368394292));
#64670=CARTESIAN_POINT('Origin',(0.0144102345384795,-0.0305802162291997,
0.0758515118280225));
#64671=CARTESIAN_POINT('',(0.0136109774441913,-0.0352728165321729,0.0758730458425347));
#64672=CARTESIAN_POINT('Origin',(0.0127959546074294,-0.0288496123713882,
0.0754898321545026));
#64673=CARTESIAN_POINT('',(0.0136801683916959,-0.0351949306052046,0.0759125941199928));
#64674=CARTESIAN_POINT('Ctrl Pts',(0.0136109774451917,-0.0352728165303529,
0.0758730458371975));
#64675=CARTESIAN_POINT('Ctrl Pts',(0.0136340318960186,-0.0352468764909507,
0.0758862122658525));
#64676=CARTESIAN_POINT('Ctrl Pts',(0.0136570958034239,-0.0352209141752656,
0.0758993951010413));
#64677=CARTESIAN_POINT('Ctrl Pts',(0.0136801683931609,-0.0351949306073904,
0.0759125941217349));
#64678=CARTESIAN_POINT('',(0.0137229182292617,-0.0350943706855873,0.076102519298984));
#64679=CARTESIAN_POINT('Origin',(0.00365827753959396,-0.0338370705548003,
0.0775758473097735));
#64680=CARTESIAN_POINT('',(0.0135710234992816,-0.0351951371254955,0.0762249265398243));
#64681=CARTESIAN_POINT('Origin',(0.00675683701100066,-0.0338370705333701,
0.0686902727050293));
#64682=CARTESIAN_POINT('',(0.0134929792220735,-0.0352722979006312,0.0762129803002442));
#64683=CARTESIAN_POINT('Origin',(0.0121318897028376,-0.0346069579193411,
0.0813176016052952));
#64684=CARTESIAN_POINT('',(0.0134237832891401,-0.03527406801681,0.0763805919988452));
#64685=CARTESIAN_POINT('Origin',(0.0141474080046922,-0.0305802162291773,
0.0766259962991262));
#64686=CARTESIAN_POINT('',(0.0133517543636662,-0.0352728165321731,0.0765471870354345));
#64687=CARTESIAN_POINT('Origin',(0.0125911876422138,-0.0288496124320617,
0.0760648456574108));
#64688=CARTESIAN_POINT('',(0.0134154430063885,-0.0351949306052041,0.0765950953880969));
#64689=CARTESIAN_POINT('Ctrl Pts',(0.0133517543653276,-0.0352728165303531,
0.0765471870302647));
#64690=CARTESIAN_POINT('Ctrl Pts',(0.0133729768338461,-0.0352468764909506,
0.0765631391265675));
#64691=CARTESIAN_POINT('Ctrl Pts',(0.0133942066280911,-0.0352209141752652,
0.0765791086852571));
#64692=CARTESIAN_POINT('Ctrl Pts',(0.0134154430076234,-0.0351949306073897,
0.0765950953900088));
#64693=CARTESIAN_POINT('',(0.0134340518118987,-0.0350943706855873,0.0767888809256985));
#64694=CARTESIAN_POINT('Origin',(0.0032641168098965,-0.0338370705480144,
0.0769891573437204));
#64695=CARTESIAN_POINT('',(0.0132680131219274,-0.0351951371254952,0.076891285491214));
#64696=CARTESIAN_POINT('Origin',(0.0074519010555576,-0.0338370705327029,
0.0685620006219173));
#64697=CARTESIAN_POINT('',(0.0131920815079901,-0.0352722979006317,0.0768696519096777));
#64698=CARTESIAN_POINT('Origin',(0.0112019458402663,-0.0346069579032916,
0.0817634321243535));
#64699=CARTESIAN_POINT('',(0.0131024238894872,-0.03527406801681,0.0770272693899471));
#64700=CARTESIAN_POINT('Origin',(0.0137895852935984,-0.0305802162292673,
0.0773614328295466));
#64701=CARTESIAN_POINT('',(0.0130100830389724,-0.035272816532173,0.0771835231567753));
#64702=CARTESIAN_POINT('Origin',(0.0123159670119983,-0.0288496123715262,
0.0766096608940125));
#64703=CARTESIAN_POINT('',(0.0130672649689706,-0.0351949306052037,0.0772390360413014));
#64704=CARTESIAN_POINT('Ctrl Pts',(0.0130100830412686,-0.035272816530353,
0.0771835231518545));
#64705=CARTESIAN_POINT('Ctrl Pts',(0.0130291388364723,-0.0352468764909504,
0.0772020093417171));
#64706=CARTESIAN_POINT('Ctrl Pts',(0.0130481997110196,-0.0352209141752648,
0.0772205137744273));
#64707=CARTESIAN_POINT('Ctrl Pts',(0.0130672649699559,-0.0351949306073892,
0.0772390360433531));
#64708=CARTESIAN_POINT('',(0.0130614392704462,-0.0350943706855874,0.0774336258238241));
#64709=CARTESIAN_POINT('Origin',(0.00294659599916159,-0.0338370705541986,
0.076357692168123));
#64710=CARTESIAN_POINT('',(0.0128838751498114,-0.0351951371254949,0.077514412732843));
#64711=CARTESIAN_POINT('Origin',(0.00815756107015764,-0.0338370705324253,
0.0685218546307288));
#64712=CARTESIAN_POINT('',(0.012811253686056,-0.0352722979006321,0.0774834329838542));
#64713=CARTESIAN_POINT('Origin',(0.0102234575330089,-0.034606957902553,
0.0820891941414742));
#64714=CARTESIAN_POINT('',(0.0127025483361862,-0.03527406801681,0.0776285705239727));
#64715=CARTESIAN_POINT('Origin',(0.0133424094829901,-0.0305802162293828,
0.0780462231458248));
#64716=CARTESIAN_POINT('',(0.0125913518310046,-0.035272816532173,0.0777720188057947));
#64717=CARTESIAN_POINT('Origin',(0.0119746331291439,-0.0288496123712106,
0.0771156858121774));
#64718=CARTESIAN_POINT('',(0.0126411252550837,-0.0351949306052034,0.0778342607508339));
#64719=CARTESIAN_POINT('Ctrl Pts',(0.0125913518338994,-0.035272816530353,
0.0777720188012005));
#64720=CARTESIAN_POINT('Ctrl Pts',(0.0126079404345147,-0.0352468764909503,
0.0777927475463656));
#64721=CARTESIAN_POINT('Ctrl Pts',(0.0126245317879862,-0.0352209141752645,
0.0778134950271386));
#64722=CARTESIAN_POINT('Ctrl Pts',(0.0126411252558039,-0.0351949306073887,
0.0778342607529929));
#64723=CARTESIAN_POINT('',(0.0126109569272709,-0.0350943706855874,0.0780265859811649));
#64724=CARTESIAN_POINT('Origin',(0.00271072246036746,-0.0338370705542837,
0.0756914103695427));
#64725=CARTESIAN_POINT('',(0.0124246676682262,-0.0351951371254947,0.0780844811758725));
#64726=CARTESIAN_POINT('Origin',(0.00886268837342121,-0.0338370705330453,
0.0685704678582771));
#64727=CARTESIAN_POINT('',(0.0123565016385186,-0.0352722979006325,0.0780446438285792));
#64728=CARTESIAN_POINT('Origin',(0.00921185609345463,-0.0346069579033713,
0.0822897503235107));
#64729=CARTESIAN_POINT('',(0.0122304629055867,-0.0352740680168101,0.0781750125228384));
#64730=CARTESIAN_POINT('Origin',(0.0128129328025127,-0.0305802162293653,
0.0786695676955698));
#64731=CARTESIAN_POINT('',(0.0121021643810505,-0.035272816532173,0.0783033930545577));
#64732=CARTESIAN_POINT('Origin',(0.0115725690272512,-0.0288496123714179,
0.0775749400940305));
#64733=CARTESIAN_POINT('',(0.0121437443425793,-0.035194930605203,0.0783713824674553));
#64734=CARTESIAN_POINT('Ctrl Pts',(0.0121021643844982,-0.035272816530353,
0.0783033930503626));
#64735=CARTESIAN_POINT('Ctrl Pts',(0.0121160241783837,-0.0352468764909501,
0.0783260374461362));
#64736=CARTESIAN_POINT('Ctrl Pts',(0.0121298843552239,-0.0352209141752643,
0.0783487007748063));
#64737=CARTESIAN_POINT('Ctrl Pts',(0.0121437443430231,-0.0351949306073883,
0.0783713824696875));
#64738=CARTESIAN_POINT('',(0.0120897091580298,-0.0350943706855874,0.0785584100618229));
#64739=CARTESIAN_POINT('Origin',(0.00256021610683366,-0.0338370705542768,
0.0750008196084603));
#64740=CARTESIAN_POINT('',(0.0118976326534744,-0.0351951371254942,0.0785925005004138));
#64741=CARTESIAN_POINT('Origin',(0.00955616268257527,-0.0338370705333592,
0.0687070736356047));
#64742=CARTESIAN_POINT('',(0.0118349970768232,-0.0352722979006328,0.07854443381358));
#64743=CARTESIAN_POINT('Origin',(0.00818309507620666,-0.0346069579027949,
0.0823619377817764));
#64744=CARTESIAN_POINT('',(0.0116936126669398,-0.0352740680168101,0.078657977669793));
#64745=CARTESIAN_POINT('Origin',(0.0122095054157723,-0.0305802162292943,
0.0792216359629003));
#64746=CARTESIAN_POINT('',(0.0115502354674222,-0.035272816532173,0.0787692658137335));
#64747=CARTESIAN_POINT('Origin',(0.011116115495978,-0.0288496123715395,
0.0779801810239078));
#64748=CARTESIAN_POINT('',(0.0115829662255687,-0.0351949306052026,0.0788419304608332));
#64749=CARTESIAN_POINT('Ctrl Pts',(0.0115502354713685,-0.035272816530353,
0.0787692658100036));
#64750=CARTESIAN_POINT('Ctrl Pts',(0.0115611478812951,-0.03524687649095,
0.0787934687407373));
#64751=CARTESIAN_POINT('Ctrl Pts',(0.0115720582982357,-0.035220914175264,
0.0788176905030729));
#64752=CARTESIAN_POINT('Ctrl Pts',(0.0115829662257291,-0.0351949306073879,
0.0788419304631035));
#64753=CARTESIAN_POINT('',(0.0115059163514221,-0.0350943706855873,0.0790207108823495));
#64754=CARTESIAN_POINT('Origin',(0.00249745047290323,-0.0338370705482644,
0.0742968108926817));
#64755=CARTESIAN_POINT('',(0.0113110817625737,-0.0351951371254938,0.0790304589382426));
#64756=CARTESIAN_POINT('Origin',(0.0102270474902958,-0.0338370705270455,
0.068929517567728));
#64757=CARTESIAN_POINT('',(0.0112549644394394,-0.0352722979006331,0.0789749209522334));
#64758=CARTESIAN_POINT('Origin',(0.00715339866134947,-0.0346069579035208,
0.082304618075051));
#64759=CARTESIAN_POINT('',(0.0111004640692083,-0.03527406801681,0.0790698493159593));
#64760=CARTESIAN_POINT('Origin',(0.0115416437331749,-0.0305802162294728,
0.0796937215015325));
#64761=CARTESIAN_POINT('',(0.0109442693387939,-0.0352728165321731,0.0791622899916112));
#64762=CARTESIAN_POINT('Origin',(0.0106124710845554,-0.0288496124319553,
0.0783250177177809));
#64763=CARTESIAN_POINT('',(0.0109676347099497,-0.0351949306052022,0.0792384839080203));
#64764=CARTESIAN_POINT('Ctrl Pts',(0.0109442693431767,-0.0352728165303531,
0.0791622899884052));
#64765=CARTESIAN_POINT('Ctrl Pts',(0.010952062273921,-0.0352468764909499,
0.0791876697594232));
#64766=CARTESIAN_POINT('Ctrl Pts',(0.0109598508671691,-0.0352209141752638,
0.0792130679637629));
#64767=CARTESIAN_POINT('Ctrl Pts',(0.0109676347098241,-0.0351949306073876,
0.079238483910293));
#64768=CARTESIAN_POINT('',(0.0108687852687488,-0.0350943706855873,0.07940619768264));
#64769=CARTESIAN_POINT('Origin',(0.00252341553365714,-0.0338370705543086,
0.0735904869236782));
#64770=CARTESIAN_POINT('',(0.0106742652534621,-0.0351951371254933,0.0793914496231707));
#64771=CARTESIAN_POINT('Origin',(0.0108647625592668,-0.0338370705271384,
0.0692342916717644));
#64772=CARTESIAN_POINT('',(0.0106255511875536,-0.0352722979006333,0.0793293162052023));
#64773=CARTESIAN_POINT('Origin',(0.00613900577330561,-0.0346069579032824,
0.0821186951698965));
#64774=CARTESIAN_POINT('',(0.0104603714201079,-0.03527406801681,0.0794041319994378));
#64775=CARTESIAN_POINT('Origin',(0.0108198803322818,-0.0305802162294855,
0.0800783792403199));
#64776=CARTESIAN_POINT('',(0.0102938224430008,-0.0352728165321731,0.0794762673621242));
#64777=CARTESIAN_POINT('Origin',(0.0100695785560694,-0.028849612371461,
0.0786040118752345));
#64778=CARTESIAN_POINT('',(0.0103074539413048,-0.0351949306052018,0.0795547889242649));
#64779=CARTESIAN_POINT('Ctrl Pts',(0.0102938224477508,-0.0352728165303531,
0.0794762673594928));
#64780=CARTESIAN_POINT('Ctrl Pts',(0.0102983730001398,-0.0352468764909498,
0.079502423716645));
#64781=CARTESIAN_POINT('Ctrl Pts',(0.0103029169389272,-0.0352209141752636,
0.0795285978181342));
#64782=CARTESIAN_POINT('Ctrl Pts',(0.0103074539408953,-0.0351949306073873,
0.0795547889265041));
#64783=CARTESIAN_POINT('',(0.0101883638484256,-0.0350943706857666,0.079708791105264));
#64784=CARTESIAN_POINT('Origin',(0.00263770164532897,-0.0338370705486574,
0.0728929867578665));
#64785=CARTESIAN_POINT('',(0.00999722610290667,-0.0351951371254956,0.0796697795164551));
#64786=CARTESIAN_POINT('Origin',(0.0114592507464863,-0.0338370705486561,
0.0696165894085452));
#64787=CARTESIAN_POINT('',(0.00995668354414125,-0.0352722979006335,0.0796020305476417));
#64788=CARTESIAN_POINT('Origin',(0.00515591409378127,-0.0346069579414847,
0.0818071011663319));
#64789=CARTESIAN_POINT('',(0.00978342936308381,-0.0352740680168101,0.0796555538826207));
#64790=CARTESIAN_POINT('Origin',(0.0100555978531566,-0.0305802162293099,
0.0803695428969902));
#64791=CARTESIAN_POINT('',(0.00960915271614781,-0.035272816532173,0.0797062463145787));
#64792=CARTESIAN_POINT('Origin',(0.00949599965990695,-0.028849612371569,
0.0788127636112503));
#64793=CARTESIAN_POINT('',(0.00961283536472869,-0.0351949306052016,0.0797858571905092));
#64794=CARTESIAN_POINT('Ctrl Pts',(0.00960915272119017,-0.035272816530353,
0.0797062463125634));
#64795=CARTESIAN_POINT('Ctrl Pts',(0.00961038913029425,-0.0352468764909497,
0.0797327667544723));
#64796=CARTESIAN_POINT('Ctrl Pts',(0.0096116167539918,-0.0352209141752635,
0.0797593039718948));
#64797=CARTESIAN_POINT('Ctrl Pts',(0.00961283536404159,-0.0351949306073873,
0.0797858571926796));
#64798=CARTESIAN_POINT('',(0.00947538274148284,-0.0350943706857667,0.0799237190718858));
#64799=CARTESIAN_POINT('Origin',(0.00283850659495694,-0.0338370705540077,
0.0722153105035223));
#64800=CARTESIAN_POINT('',(0.00929064162275147,-0.035195137125491,0.079861059189403));
#64801=CARTESIAN_POINT('Origin',(0.0120011365590591,-0.0338370705323713,
0.0700703818276128));
#64802=CARTESIAN_POINT('',(0.00925890995150084,-0.0352722979006337,0.0797887631114598));
#64803=CARTESIAN_POINT('Origin',(0.00421962723954973,-0.0346069578981706,
0.0813747501428187));
#64804=CARTESIAN_POINT('',(0.00908031367876579,-0.0352740680168079,0.0798201498922159));
#64805=CARTESIAN_POINT('Origin',(0.0092608494871027,-0.0305802162292691,
0.0805626206468866));
#64806=CARTESIAN_POINT('',(0.00890105780882915,-0.0352728165321731,0.0798485999435113));
#64807=CARTESIAN_POINT('Origin',(0.00890078007252705,-0.0288496123647477,
0.0789479807675767));
#64808=CARTESIAN_POINT('',(0.00889473353011883,-0.0351949306052013,0.0799280446221614));
#64809=CARTESIAN_POINT('Ctrl Pts',(0.00890105781408429,-0.0352728165303532,
0.0798485999421439));
#64810=CARTESIAN_POINT('Ctrl Pts',(0.00889896058099329,-0.0352468764909498,
0.0798750662255982));
#64811=CARTESIAN_POINT('Ctrl Pts',(0.00889685252924194,-0.0352209141752635,
0.0799015480511828));
#64812=CARTESIAN_POINT('Ctrl Pts',(0.008894733529165,-0.0351949306073872,
0.0799280446242287));
#64813=CARTESIAN_POINT('',(0.0087410860864854,-0.0350943706857667,0.0800475920396916));
#64814=CARTESIAN_POINT('Origin',(0.00312266345952377,-0.0338370705537815,
0.0715681454234068));
#64815=CARTESIAN_POINT('',(0.00856565507233699,-0.0351951371254918,0.0799622720473137));
#64816=CARTESIAN_POINT('Origin',(0.0124818742154735,-0.0338370705274226,
0.0705885121561095));
#64817=CARTESIAN_POINT('',(0.00854323471601816,-0.0352722979006337,0.0798865690125767));
#64818=CARTESIAN_POINT('Origin',(0.00334491140344038,-0.0346069579038024,
0.0808284604609533));
#64819=CARTESIAN_POINT('',(0.00836211292151624,-0.0352740680168079,0.0798953242508273));
#64820=CARTESIAN_POINT('Origin',(0.00844816889056077,-0.0305802162291152,
0.0806545675384037));
#64821=CARTESIAN_POINT('',(0.00818070480072852,-0.0352728165321732,0.0799010832471564));
#64822=CARTESIAN_POINT('Origin',(0.00829330676799402,-0.0288496123650155,
0.0790075309130333));
#64823=CARTESIAN_POINT('',(0.0081644733313186,-0.0351949306058011,0.0799791088412712));
#64824=CARTESIAN_POINT('Ctrl Pts',(0.00818070480611361,-0.0352728165303532,
0.0799010832464584));
#64825=CARTESIAN_POINT('Ctrl Pts',(0.00817530700536458,-0.0352468764905577,
0.0799270779827507));
#64826=CARTESIAN_POINT('Ctrl Pts',(0.00816989652331777,-0.0352209141744786,
0.0799530867826816));
#64827=CARTESIAN_POINT('Ctrl Pts',(0.00816447333092876,-0.0351949306062089,
0.0799791088415971));
#64828=CARTESIAN_POINT('',(0.00799705416196017,-0.0350943707007864,0.08007845644402));
#64829=CARTESIAN_POINT('Origin',(0.00348535491286147,-0.0338373859475111,
0.0709614461967262));
#64830=CARTESIAN_POINT('',(0.00783369992265928,-0.0351951371254912,0.0799718219029567));
#64831=CARTESIAN_POINT('Origin',(0.0128938821456517,-0.0338370705272571,
0.0711628093171656));
#64832=CARTESIAN_POINT('',(0.0078209444636804,-0.0352722979006336,0.0798939057935052));
#64833=CARTESIAN_POINT('Origin',(0.0025455611822975,-0.0346069579031932,
0.0801768474759825));
#64834=CARTESIAN_POINT('',(0.00764015354630635,-0.0352740680168098,0.0798798914139134));
#64835=CARTESIAN_POINT('Origin',(0.00763037252202439,-0.0305802162295736,
0.0806439335144828));
#64836=CARTESIAN_POINT('',(0.00745945408910196,-0.035272816532173,0.0798628685324633));
#64837=CARTESIAN_POINT('Origin',(0.00768315995856749,-0.0288496123710585,
0.0789904749064774));
#64838=CARTESIAN_POINT('',(0.00743357141106809,-0.0351949306052011,0.0799382445262853));
#64839=CARTESIAN_POINT('Ctrl Pts',(0.00745945409453209,-0.035272816530353,
0.0798628685324458));
#64840=CARTESIAN_POINT('Ctrl Pts',(0.00745084085282929,-0.0352468764909498,
0.0798879817682764));
#64841=CARTESIAN_POINT('Ctrl Pts',(0.00744221326718366,-0.0352209141752637,
0.0799131073674612));
#64842=CARTESIAN_POINT('Ctrl Pts',(0.00743357140962971,-0.0351949306073875,
0.0799382445280509));
#64843=CARTESIAN_POINT('',(0.00725502085064003,-0.0350943706857667,0.0800158255764398));
#64844=CARTESIAN_POINT('Origin',(0.00392186390992144,-0.0338370705483594,
0.0704055314389981));
#64845=CARTESIAN_POINT('',(0.00710631954367321,-0.0351951371254908,0.0798895581494023));
#64846=CARTESIAN_POINT('Origin',(0.0132306627505617,-0.033837070527115,
0.0717842162590107));
#64847=CARTESIAN_POINT('',(0.00710343014324219,-0.0352722979006335,0.0798106577488273));
#64848=CARTESIAN_POINT('Origin',(0.00183418283858109,-0.0346069579033387,
0.0794301875068299));
#64849=CARTESIAN_POINT('',(0.00692582128376252,-0.03527406801681,0.0797740947665314));
#64850=CARTESIAN_POINT('Origin',(0.00682035751875458,-0.0305802162293907,
0.0805308862794182));
#64851=CARTESIAN_POINT('',(0.0067486802285259,-0.0352728165321729,0.0797345584683111));
#64852=CARTESIAN_POINT('Origin',(0.00707996202453286,-0.0288496123715112,
0.0788970817063622));
#64853=CARTESIAN_POINT('',(0.00671355452610057,-0.035194930605201,0.0798060961401762));
#64854=CARTESIAN_POINT('Ctrl Pts',(0.00674868023391541,-0.0352728165303529,
0.0797345584689743));
#64855=CARTESIAN_POINT('Ctrl Pts',(0.00673698738714423,-0.0352468764909498,
0.0797583941540052));
#64856=CARTESIAN_POINT('Ctrl Pts',(0.00672527875999732,-0.0352209141752638,
0.0797822403071289));
#64857=CARTESIAN_POINT('Ctrl Pts',(0.00671355452445208,-0.0351949306073877,
0.0798060961417479));
#64858=CARTESIAN_POINT('',(0.00652668840559494,-0.0350943706855873,0.0798606871213604));
#64859=CARTESIAN_POINT('Origin',(0.00442430365356226,-0.0338370705545198,
0.0699084177326389));
#64860=CARTESIAN_POINT('',(0.00639498515847155,-0.0351951371254902,0.0797167781351863));
#64861=CARTESIAN_POINT('Origin',(0.0134869047874854,-0.0338370705288107,
0.0724429330351057));
#64862=CARTESIAN_POINT('',(0.00640200738415908,-0.0352722979006334,0.0796381377499374));
#64863=CARTESIAN_POINT('Origin',(0.00122199523403942,-0.0346069579031278,
0.078600255826089));
#64864=CARTESIAN_POINT('',(0.00623038158038529,-0.0352740680168099,0.0795796027850097));
#64865=CARTESIAN_POINT('Origin',(0.00603089830120988,-0.0305802162294044,
0.0803172086561122));
#64866=CARTESIAN_POINT('',(0.00605959254737729,-0.035272816532173,0.0795181765810599));
#64867=CARTESIAN_POINT('Origin',(0.00649322575805522,-0.0288496123718448,
0.0787288241923079));
#64868=CARTESIAN_POINT('',(0.00601577777387097,-0.0351949306052009,0.0795847477391485));
#64869=CARTESIAN_POINT('Ctrl Pts',(0.0060595925526412,-0.035272816530353,
0.0795181765823933));
#64870=CARTESIAN_POINT('Ctrl Pts',(0.00604500450398018,-0.03524687649095,
0.0795403588136329));
#64871=CARTESIAN_POINT('Ctrl Pts',(0.00603039948737651,-0.035220914175264,
0.0795625494526157));
#64872=CARTESIAN_POINT('Ctrl Pts',(0.00601577777203827,-0.035194930607388,
0.0795847477405013));
#64873=CARTESIAN_POINT('',(0.0058235430843454,-0.0350943706855874,0.0796154877190134));
#64874=CARTESIAN_POINT('Origin',(0.00498508636730859,-0.0338370705537688,
0.0694781962621798));
#64875=CARTESIAN_POINT('',(0.0057109149352393,-0.0351951371254898,0.0794562067043462));
#64876=CARTESIAN_POINT('Origin',(0.0136585671622885,-0.0338370705331965,
0.0731285712846959));
#64877=CARTESIAN_POINT('',(0.00572773804235142,-0.0352722979006333,0.0793790665402766));
#64878=CARTESIAN_POINT('Origin',(0.000718652933226445,-0.0346069579030036,
0.0777001409526867));
#64879=CARTESIAN_POINT('',(0.00556480193573351,-0.035274068016808,0.0792994827240814));
#64880=CARTESIAN_POINT('Origin',(0.0052744451129475,-0.0305802162290773,
0.0800062704680069));
#64881=CARTESIAN_POINT('',(0.00540305837002919,-0.0352728165321732,0.0792171353423319));
#64882=CARTESIAN_POINT('Origin',(0.00593220434223688,-0.0288496124253593,
0.0784883558809479));
#64883=CARTESIAN_POINT('',(0.0053512455105937,-0.0351949306052009,0.0792776901197134));
#64884=CARTESIAN_POINT('Ctrl Pts',(0.00540305837508442,-0.0352728165303532,
0.0792171353443146));
#64885=CARTESIAN_POINT('Ctrl Pts',(0.00538580518677541,-0.0352468764909502,
0.0792373142947253));
#64886=CARTESIAN_POINT('Ctrl Pts',(0.00536853411055141,-0.0352209141752643,
0.0792574994599344));
#64887=CARTESIAN_POINT('Ctrl Pts',(0.00535124550860563,-0.0351949306073883,
0.0792776901208262));
#64888=CARTESIAN_POINT('',(0.00515667390793764,-0.0350943706855873,0.0792840943104133));
#64889=CARTESIAN_POINT('Origin',(0.00559536819040455,-0.0338370705541392,
0.0691216519384616));
#64890=CARTESIAN_POINT('',(0.00506489707003965,-0.0351951371254925,0.0791119532240087));
#64891=CARTESIAN_POINT('Origin',(0.0137429427619029,-0.0338370705482579,
0.0738303180245431));
#64892=CARTESIAN_POINT('',(0.00509125574812847,-0.0352722979006329,0.0790375298275827));
#64893=CARTESIAN_POINT('Origin',(0.000332093925861045,-0.0346069579299659,
0.0767440382573458));
#64894=CARTESIAN_POINT('',(0.00493957893840163,-0.0352740680168099,0.0789381522444425));
#64895=CARTESIAN_POINT('Origin',(0.00456292767242667,-0.0305802162293321,
0.079602975396522));
#64896=CARTESIAN_POINT('',(0.0047894316326524,-0.035272816532173,0.0788361823522959));
#64897=CARTESIAN_POINT('Origin',(0.00540574541516571,-0.02884961237144,
0.0781794691145221));
#64898=CARTESIAN_POINT('',(0.00473043780703324,-0.035194930605201,0.078889765763957));
#64899=CARTESIAN_POINT('Ctrl Pts',(0.00478943163741931,-0.035272816530353,
0.0788361823548966));
#64900=CARTESIAN_POINT('Ctrl Pts',(0.00476978540254869,-0.0352468764909502,
0.0788540397903759));
#64901=CARTESIAN_POINT('Ctrl Pts',(0.00475012064189385,-0.0352209141752646,
0.0788719011496979));
#64902=CARTESIAN_POINT('Ctrl Pts',(0.0047304378049211,-0.0351949306073888,
0.078889765764812));
#64903=CARTESIAN_POINT('',(0.00453659780165151,-0.0350943706855874,0.0788717331675791));
#64904=CARTESIAN_POINT('Origin',(0.00624552461956904,-0.0338370705480265,
0.0688444076153873));
#64905=CARTESIAN_POINT('',(0.00446711965052249,-0.035195137125489,0.078689446777193));
#64906=CARTESIAN_POINT('Origin',(0.0137387007491635,-0.0338370705274849,
0.074537106376181));
#64907=CARTESIAN_POINT('',(0.00450259820748627,-0.0352722979006326,0.0786189138498392));
#64908=CARTESIAN_POINT('Origin',(6.8414532284294E-5,-0.0346069579036642,
0.0757470259866494));
#64909=CARTESIAN_POINT('',(0.00436457272854574,-0.0352740680168099,0.0785013097436045));
#64910=CARTESIAN_POINT('Origin',(0.00390756703492207,-0.0305802162292527,
0.0791136836454428));
#64911=CARTESIAN_POINT('',(0.00422838959545862,-0.035272816532173,0.0783813254671743));
#64912=CARTESIAN_POINT('Origin',(0.00492215155327239,-0.0288496123718619,
0.0778070352087378));
#64913=CARTESIAN_POINT('',(0.00416314517152701,-0.0351949306052012,0.0784270924707041));
#64914=CARTESIAN_POINT('Ctrl Pts',(0.00422838959986201,-0.035272816530353,
0.078381325470352));
#64915=CARTESIAN_POINT('Ctrl Pts',(0.00420666015128976,-0.0352468764909504,
0.0783965797684749));
#64916=CARTESIAN_POINT('Ctrl Pts',(0.00418491183122674,-0.035220914175265,
0.0784118356376035));
#64917=CARTESIAN_POINT('Ctrl Pts',(0.00416314516932403,-0.0351949306073894,
0.0784270924712879));
#64918=CARTESIAN_POINT('',(0.00397309373609907,-0.0350943706855873,0.0783849074720655));
#64919=CARTESIAN_POINT('Origin',(0.00692530227733226,-0.0338370705548223,
0.0686508357466448));
#64920=CARTESIAN_POINT('',(0.00392700998368523,-0.0351951371254887,0.0781953505429711));
#64921=CARTESIAN_POINT('Origin',(0.0136459081016941,-0.0338370705330285,
0.0752377898391803));
#64922=CARTESIAN_POINT('',(0.00397104890148771,-0.0352722979006322,0.0781298204310839));
#64923=CARTESIAN_POINT('Origin',(-6.82269184376445E-5,-0.0346069579035453,
0.0747248276832768));
#64924=CARTESIAN_POINT('',(0.00384885149759004,-0.03527406801681,0.0779958444887646));
#64925=CARTESIAN_POINT('Origin',(0.00331869862899803,-0.0305802162295164,
0.0785461116382315));
#64926=CARTESIAN_POINT('',(0.00372878022652447,-0.035272816532173,0.077859738051764));
#64927=CARTESIAN_POINT('Origin',(0.00448904931912108,-0.0288496123714666,
0.0773769276730949));
#64928=CARTESIAN_POINT('',(0.00365831414782088,-0.0351949306052012,0.0778969668741772));
#64929=CARTESIAN_POINT('Ctrl Pts',(0.00372878023049487,-0.035272816530353,
0.0778597380554684));
#64930=CARTESIAN_POINT('Ctrl Pts',(0.0037053102546055,-0.0352468764909506,
0.0778721486468413));
#64931=CARTESIAN_POINT('Ctrl Pts',(0.00368182135913347,-0.0352209141752653,
0.0778845584316069));
#64932=CARTESIAN_POINT('Ctrl Pts',(0.00365831414556175,-0.0351949306073898,
0.0778969668744805));
#64933=CARTESIAN_POINT('',(0.00347504850701491,-0.0350943706855874,0.0778312947559066));
#64934=CARTESIAN_POINT('Origin',(0.007623980706386,-0.0338370705483359,
0.0685439888925231));
#64935=CARTESIAN_POINT('',(0.0034530859216209,-0.0351951371254883,0.0776374567141115));
#64936=CARTESIAN_POINT('Origin',(0.0134660283161429,-0.0338370705272378,
0.0759213181795987));
#64937=CARTESIAN_POINT('',(0.00350499068022065,-0.0352722979006318,0.0775779628667008));
#64938=CARTESIAN_POINT('Origin',(-7.56754917528666E-5,-0.0346069579032585,
0.0736935640038484));
#64939=CARTESIAN_POINT('',(0.00340054847742131,-0.0352740680168101,0.0774297279689394));
#64940=CARTESIAN_POINT('Origin',(0.00280560926146734,-0.0305802162293396,
0.0779092103242104));
#64941=CARTESIAN_POINT('',(0.0032984826640503,-0.0352728165321729,0.0772796458511875));
#64942=CARTESIAN_POINT('Origin',(0.00411326899362973,-0.0288496123714065,
0.0768959295603915));
#64943=CARTESIAN_POINT('',(0.00322390622273076,-0.0351949306052015,0.0773077493717152));
#64944=CARTESIAN_POINT('Ctrl Pts',(0.00329848266752508,-0.0352728165303529,
0.0772796458553603));
#64945=CARTESIAN_POINT('Ctrl Pts',(0.00327364229985878,-0.0352468764909508,
0.0772890170175433));
#64946=CARTESIAN_POINT('Ctrl Pts',(0.00324878326289108,-0.0352209141752657,
0.077298385008227));
#64947=CARTESIAN_POINT('Ctrl Pts',(0.00322390622045105,-0.0351949306073906,
0.0773077493717331));
#64948=CARTESIAN_POINT('',(0.00305031658517945,-0.0350943706855873,0.0772196258223481));
#64949=CARTESIAN_POINT('Origin',(0.00833054129011836,-0.0338370705479401,
0.0685255522280844));
#64950=CARTESIAN_POINT('',(0.00305282152989682,-0.035195137125488,0.0770245636095646));
#64951=CARTESIAN_POINT('Origin',(0.0132018980278313,-0.0338370705330224,
0.0765769117901669));
#64952=CARTESIAN_POINT('',(0.00311177356024406,-0.0352722979006314,0.0769720442801441));
#64953=CARTESIAN_POINT('Origin',(4.61862801057515E-5,-0.0346069579036435,
0.0726694985930505));
#64954=CARTESIAN_POINT('',(0.00302673367447229,-0.0352740680168101,0.0768118881798294));
#64955=CARTESIAN_POINT('Origin',(0.00237639065787438,-0.0305802162294318,
0.0772130240178286));
#64956=CARTESIAN_POINT('',(0.00294428295764374,-0.035272816532173,0.0766501972659778));
#64957=CARTESIAN_POINT('Origin',(0.00380073685025004,-0.0288496124326153,
0.0763716265010679));
#64958=CARTESIAN_POINT('',(0.00286677226873748,-0.0351949306052018,0.0766687322753135));
#64959=CARTESIAN_POINT('Ctrl Pts',(0.0029442829605681,-0.0352728165303531,
0.0766501972705532));
#64960=CARTESIAN_POINT('Ctrl Pts',(0.00291846394856184,-0.0352468764909511,
0.0766563812147208));
#64961=CARTESIAN_POINT('Ctrl Pts',(0.00289262681196146,-0.0352209141752662,
0.0766625596725133));
#64962=CARTESIAN_POINT('Ctrl Pts',(0.00286677226647317,-0.0351949306073912,
0.0766687322750457));
#64963=CARTESIAN_POINT('',(0.00270559624672265,-0.0350943706855873,0.076559547055866));
#64964=CARTESIAN_POINT('Origin',(0.00903384112997155,-0.033837070554224,
0.0685958165021795));
#64965=CARTESIAN_POINT('',(0.00273252921707685,-0.0351951371254877,0.0763663369197139));
#64966=CARTESIAN_POINT('Origin',(0.0128576828699685,-0.0338370705326189,
0.0771942315442123));
#64967=CARTESIAN_POINT('',(0.00279759881043661,-0.0352722979006309,0.0763216203694819));
#64968=CARTESIAN_POINT('Origin',(0.000295436565332532,-0.0346069579034067,
0.0716687815734711));
#64969=CARTESIAN_POINT('',(0.00273330237149167,-0.03527406801681,0.076152068823989));
#64970=CARTESIAN_POINT('Origin',(0.00203781185220466,-0.0305802162292972,
0.0764685319928733));
#64971=CARTESIAN_POINT('',(0.00267176704826306,-0.035272816532173,0.0759813190763382));
#64972=CARTESIAN_POINT('Origin',(0.00355638172827499,-0.0288496123714443,
0.0758122870587156));
#64973=CARTESIAN_POINT('',(0.00259254450163696,-0.035194930605202,0.0759899932663124));
#64974=CARTESIAN_POINT('Ctrl Pts',(0.00267176705059093,-0.035272816530353,
0.075981319081244));
#64975=CARTESIAN_POINT('Ctrl Pts',(0.00264537657548761,-0.0352468764909512,
0.0759842182829025));
#64976=CARTESIAN_POINT('Ctrl Pts',(0.00261896880633315,-0.0352209141752666,
0.0759871097698338));
#64977=CARTESIAN_POINT('Ctrl Pts',(0.00259254449942374,-0.0351949306073918,
0.075989993265763));
#64978=CARTESIAN_POINT('',(0.00244632393730788,-0.0350943706855874,0.0758614682929193));
#64979=CARTESIAN_POINT('Origin',(0.00972278885438708,-0.0338370705482382,
0.0687536734940358));
#64980=CARTESIAN_POINT('',(0.00249726018426747,-0.0351951371254876,0.0756731572726638));
#64981=CARTESIAN_POINT('Origin',(0.0124388113078349,-0.0338370705268928,
0.0777635419566633));
#64982=CARTESIAN_POINT('',(0.00256742115428162,-0.0352722979006304,0.0756369487083298));
#64983=CARTESIAN_POINT('Origin',(0.000668144537672311,-0.034606957903352,
0.0707071948512846));
#64984=CARTESIAN_POINT('',(0.0025248821554141,-0.0352740680168102,0.0754606756468147));
#64985=CARTESIAN_POINT('Origin',(0.00179521243424888,-0.0305802162295,0.0756874753334203));
#64986=CARTESIAN_POINT('',(0.00248523267459275,-0.035272816532173,0.0752835598908876));
#64987=CARTESIAN_POINT('Origin',(0.00338405722560929,-0.0288496124323458,
0.075226732360674));
#64988=CARTESIAN_POINT('',(0.00240554765713235,-0.0351949306052022,0.0752822364643431));
#64989=CARTESIAN_POINT('Ctrl Pts',(0.0024852326762874,-0.0352728165303531,
0.0752835598960465));
#64990=CARTESIAN_POINT('Ctrl Pts',(0.00245868693164429,-0.0352468764909515,
0.0752831286330541));
#64991=CARTESIAN_POINT('Ctrl Pts',(0.00243212499623051,-0.035220914175267,
0.0752826875486479));
#64992=CARTESIAN_POINT('Ctrl Pts',(0.00240554765500504,-0.0351949306073924,
0.0752822364635208));
#64993=CARTESIAN_POINT('',(0.00227658853613647,-0.0350943706855873,0.0751363986526118));
#64994=CARTESIAN_POINT('Origin',(0.010386519222081,-0.0338370705546125,
0.0689966338444921));
#64995=CARTESIAN_POINT('',(0.0023507247646591,-0.0351951371254875,0.0749559565255339));
#64996=CARTESIAN_POINT('Origin',(0.0119518891160215,-0.0338370705273412,
0.078275864650999));
#64997=CARTESIAN_POINT('',(0.00242487063091823,-0.0352722979006299,0.074928826977787));
#64998=CARTESIAN_POINT('Origin',(0.00115843236911722,-0.034606957903392,
0.0697999032221867));
#64999=CARTESIAN_POINT('',(0.00240475993755276,-0.0352740680168099,0.0747486123317347));
#65000=CARTESIAN_POINT('Origin',(0.00165241834197848,-0.0305802162295103,
0.0748821717694814));
#65001=CARTESIAN_POINT('',(0.00238762159513567,-0.0352728165321731,0.0745679237888021));
#65002=CARTESIAN_POINT('Origin',(0.00328648102428352,-0.0288496124320948,
0.0746241969480168));
#65003=CARTESIAN_POINT('',(0.00230873078716791,-0.0351949306052026,0.0745566236169663));
#65004=CARTESIAN_POINT('Ctrl Pts',(0.00238762159617038,-0.0352728165303531,
0.0745679237941327));
#65005=CARTESIAN_POINT('Ctrl Pts',(0.0023613392242382,-0.0352468764909518,
0.0745641688677643));
#65006=CARTESIAN_POINT('Ctrl Pts',(0.00233504202015395,-0.0352209141752675,
0.0745604021681853));
#65007=CARTESIAN_POINT('Ctrl Pts',(0.00230873078516012,-0.0351949306073931,
0.0745566236158839));
#65008=CARTESIAN_POINT('',(0.00219906687187978,-0.0350943706855873,0.0743957729163068));
#65009=CARTESIAN_POINT('Origin',(0.0110145649089121,-0.0338370705544943,
0.0693208658243919));
#65010=CARTESIAN_POINT('',(0.00229523390935503,-0.0351951371254875,0.0742260453625414));
#65011=CARTESIAN_POINT('Origin',(0.0114045953917401,-0.0338370705268584,
0.0787231199947708));
#65012=CARTESIAN_POINT('',(0.00237219534725549,-0.0352722979006293,0.0742084226805557));
#65013=CARTESIAN_POINT('Origin',(0.0017585679285661,-0.0346069579032107,
0.0689612152181359));
#65014=CARTESIAN_POINT('',(0.0023748301170392,-0.0352740680168101,0.0740271085425837));
#65015=CARTESIAN_POINT('Origin',(0.00161168152344718,-0.030580216229527,
0.0740653214193561));
#65016=CARTESIAN_POINT('',(0.0023804731949247,-0.035272816532173,0.0738456967789116));
#65017=CARTESIAN_POINT('Origin',(0.00326519195932053,-0.0288496123714054,
0.0740141831669405));
#65018=CARTESIAN_POINT('',(0.00230362075161854,-0.0351949306052031,0.0738245980722451));
#65019=CARTESIAN_POINT('Ctrl Pts',(0.00238047319528312,-0.035272816530353,
0.0738456967843299));
#65020=CARTESIAN_POINT('Ctrl Pts',(0.00235486868476764,-0.035246876490952,
0.0738386774120175));
#65021=CARTESIAN_POINT('Ctrl Pts',(0.0023292509346306,-0.035220914175268,
0.0738316445003683));
#65022=CARTESIAN_POINT('Ctrl Pts',(0.00230362074976191,-0.0351949306073939,
0.0738245980709196));
#65023=CARTESIAN_POINT('',(0.0022149815074924,-0.0350943706855873,0.0736512711942942));
#65024=CARTESIAN_POINT('Origin',(0.0115970212688448,-0.0338370705480172,
0.0697212561165514));
#65025=CARTESIAN_POINT('',(0.00233166274229183,-0.0351951371254875,0.0734949349187544));
#65026=CARTESIAN_POINT('Origin',(0.01080556128334,-0.0338370705272959,0.0790982545048888));
#65027=CARTESIAN_POINT('',(0.00241022602398344,-0.0352722979006288,0.0734870970227522));
#65028=CARTESIAN_POINT('Origin',(0.0024590867190163,-0.0346069579034221,
0.0682043574498562));
#65029=CARTESIAN_POINT('',(0.00243556470502341,-0.0352740680168101,0.0733075428251295));
#65030=CARTESIAN_POINT('Origin',(0.00167364442279193,-0.0305802162292074,
0.0732498065010526));
#65031=CARTESIAN_POINT('',(0.00246390020850166,-0.035272816532173,0.0731282688125995));
#65032=CARTESIAN_POINT('Origin',(0.00332052575741809,-0.028849612371474,
0.0734063112986791));
#65033=CARTESIAN_POINT('',(0.00239029813879711,-0.0351949306052035,0.0730977043103102));
#65034=CARTESIAN_POINT('Ctrl Pts',(0.00246390020817816,-0.035272816530353,
0.07312826881802));
#65035=CARTESIAN_POINT('Ctrl Pts',(0.0024393773575055,-0.0352468764909522,
0.0731180956994582));
#65036=CARTESIAN_POINT('Ctrl Pts',(0.00241484306853851,-0.0352209141752684,
0.0731079074889567));
#65037=CARTESIAN_POINT('Ctrl Pts',(0.00239029813712095,-0.0351949306073946,
0.0730977043087625));
#65038=CARTESIAN_POINT('',(0.00232408145966373,-0.0350943706855874,0.0729146347234738));
#65039=CARTESIAN_POINT('Origin',(0.0121247025115712,-0.0338370705513202,
0.0701914903750677));
#65040=CARTESIAN_POINT('',(0.00245943675901277,-0.0351951371254877,0.0727741552426159));
#65041=CARTESIAN_POINT('Origin',(0.01016423388182,-0.03383707053302,0.0793953520558185));
#65042=CARTESIAN_POINT('',(0.00253836289461168,-0.0352722979006283,0.0727762257408987));
#65043=CARTESIAN_POINT('Origin',(0.00324894114125073,-0.0346069579033883,
0.0675412660163024));
#65044=CARTESIAN_POINT('',(0.00258600588077167,-0.0352740680168102,0.0726012631605823));
#65045=CARTESIAN_POINT('Origin',(0.00183732984760715,-0.0305802162294387,
0.0724484881719455));
#65046=CARTESIAN_POINT('',(0.00263658694202549,-0.035272816532173,0.0724269541574653));
#65047=CARTESIAN_POINT('Origin',(0.00345160977874861,-0.0288496123715095,
0.0728101678454856));
#65048=CARTESIAN_POINT('',(0.00256739599452954,-0.0351949306052039,0.0723874058800131));
#65049=CARTESIAN_POINT('Ctrl Pts',(0.00263658694102517,-0.035272816530353,
0.0724269541628026));
#65050=CARTESIAN_POINT('Ctrl Pts',(0.00261353249019967,-0.0352468764909524,
0.0724137877341483));
#65051=CARTESIAN_POINT('Ctrl Pts',(0.00259046858279584,-0.0352209141752689,
0.0724006048989603));
#65052=CARTESIAN_POINT('Ctrl Pts',(0.0025673959930603,-0.0351949306073953,
0.0723874058782675));
#65053=CARTESIAN_POINT('',(0.00252464615697504,-0.0350943706855873,0.0721974807010359));
#65054=CARTESIAN_POINT('Origin',(0.0125892868464681,-0.0338370705546861,
0.0707241526903459));
#65055=CARTESIAN_POINT('',(0.00267654088694574,-0.0351951371254879,0.0720750734601912));
#65056=CARTESIAN_POINT('Origin',(0.00949072738717799,-0.0338370705310109,
0.0796097273078675));
#65057=CARTESIAN_POINT('',(0.00275458516414511,-0.0352722979006279,0.0720870196997644));
#65058=CARTESIAN_POINT('Origin',(0.00411567467158826,-0.034606957924588,
0.0669823984380814));
#65059=CARTESIAN_POINT('',(0.00282378109707297,-0.0352740680168102,0.0719194080011641));
#65060=CARTESIAN_POINT('Origin',(0.00210015638139261,-0.030580216229448,
0.0716740037008217));
#65061=CARTESIAN_POINT('',(0.00289581002255045,-0.035272816532173,0.0717528129645656));
#65062=CARTESIAN_POINT('Origin',(0.00365637675003213,-0.0288496123718428,
0.0722351543457127));
#65063=CARTESIAN_POINT('',(0.00283212137983757,-0.0351949306052042,0.0717049046119108));
#65064=CARTESIAN_POINT('Ctrl Pts',(0.00289581002088911,-0.035272816530353,
0.0717528129697354));
#65065=CARTESIAN_POINT('Ctrl Pts',(0.00287458755237228,-0.0352468764909526,
0.0717368608734338));
#65066=CARTESIAN_POINT('Ctrl Pts',(0.00285335775812898,-0.0352209141752692,
0.0717208913147453));
#65067=CARTESIAN_POINT('Ctrl Pts',(0.00283212137859842,-0.0351949306073958,
0.0717049046099949));
#65068=CARTESIAN_POINT('',(0.00281351257433806,-0.0350943706855873,0.0715111190743214));
#65069=CARTESIAN_POINT('Origin',(0.0129834475299402,-0.0338370705542504,
0.0713108426575205));
#65070=CARTESIAN_POINT('',(0.00297955126430113,-0.0351951371254881,0.0714087145088007));
#65071=CARTESIAN_POINT('Origin',(0.00879566332822816,-0.033837070532911,
0.0797379993743328));
#65072=CARTESIAN_POINT('',(0.00305548287822846,-0.0352722979006274,0.0714303480903293));
#65073=CARTESIAN_POINT('Origin',(0.00504561854555748,-0.0346069579034451,
0.066536567876592));
#65074=CARTESIAN_POINT('',(0.00314514049672617,-0.0352740680168102,0.0712727306100589));
#65075=CARTESIAN_POINT('Origin',(0.00245797909256947,-0.0305802162293691,
0.0709385671704278));
#65076=CARTESIAN_POINT('',(0.00323748134724438,-0.0352728165321731,0.0711164768432249));
#65077=CARTESIAN_POINT('Origin',(0.00393159737382974,-0.0288496123719026,
0.0716903391057524));
#65078=CARTESIAN_POINT('',(0.00318029941725562,-0.0351949306052047,0.0710609639587081));
#65079=CARTESIAN_POINT('Ctrl Pts',(0.00323748134494819,-0.0352728165303531,
0.0711164768481458));
#65080=CARTESIAN_POINT('Ctrl Pts',(0.00321842554974618,-0.0352468764909528,
0.0710979906582848));
#65081=CARTESIAN_POINT('Ctrl Pts',(0.00319936467520065,-0.0352209141752696,
0.0710794862255762));
#65082=CARTESIAN_POINT('Ctrl Pts',(0.00318029941626621,-0.0351949306073963,
0.071060963956652));
#65083=CARTESIAN_POINT('',(0.00318612511579046,-0.0350943706855874,0.0708663741761959));
#65084=CARTESIAN_POINT('Origin',(0.0133009684340317,-0.0338370705483989,
0.0719423078362993));
#65085=CARTESIAN_POINT('',(0.00336368923641856,-0.0351951371254884,0.0707855872671713));
#65086=CARTESIAN_POINT('Origin',(0.00809000333431659,-0.0338370705278078,
0.0797781454036159));
#65087=CARTESIAN_POINT('',(0.00343631070016287,-0.035272297900627,0.0708165670161512));
#65088=CARTESIAN_POINT('Origin',(0.00602410685206571,-0.0346069579033739,
0.0662108058592296));
#65089=CARTESIAN_POINT('',(0.00354501605002859,-0.0352740680168101,0.07067142947603));
#65090=CARTESIAN_POINT('Origin',(0.00290515490327304,-0.0305802162292641,
0.0702537768542104));
#65091=CARTESIAN_POINT('',(0.00365621255521218,-0.035272816532173,0.0705279811942054));
#65092=CARTESIAN_POINT('Origin',(0.00427293125686862,-0.0288496123715293,
0.071184314187666));
#65093=CARTESIAN_POINT('',(0.00360643913114228,-0.035194930605205,0.0704657392491771));
#65094=CARTESIAN_POINT('Ctrl Pts',(0.00365621255231737,-0.035272816530353,
0.0705279811987995));
#65095=CARTESIAN_POINT('Ctrl Pts',(0.00363962395170388,-0.0352468764909529,
0.0705072524536365));
#65096=CARTESIAN_POINT('Ctrl Pts',(0.00362303259823409,-0.0352209141752699,
0.0704865049728655));
#65097=CARTESIAN_POINT('Ctrl Pts',(0.00360643913041818,-0.0351949306073968,
0.0704657392470133));
#65098=CARTESIAN_POINT('',(0.00363660745896575,-0.0350943706855873,0.0702734140188551));
#65099=CARTESIAN_POINT('Origin',(0.0135368419257299,-0.0338370705541201,
0.0726085896305422));
#65100=CARTESIAN_POINT('',(0.00382289671800493,-0.0351951371254887,0.0702155188241416));
#65101=CARTESIAN_POINT('Origin',(0.00738487602467975,-0.0338370705289731,
0.0797295321728266));
#65102=CARTESIAN_POINT('',(0.00389106274770099,-0.0352722979006266,0.0702553561714247));
#65103=CARTESIAN_POINT('Origin',(0.00703570829280538,-0.0346069579035862,
0.0660102496760509));
#65104=CARTESIAN_POINT('',(0.00401710148062903,-0.0352740680168101,0.0701249874771627));
#65105=CARTESIAN_POINT('Origin',(0.00343463158368949,-0.0305802162293682,
0.069630432304418));
#65106=CARTESIAN_POINT('',(0.00414540000516627,-0.035272816532173,0.0699966069454424));
#65107=CARTESIAN_POINT('Origin',(0.00467499535910736,-0.0288496123713801,
0.0707250599061107));
#65108=CARTESIAN_POINT('',(0.0041038200436459,-0.0351949306052054,0.0699286175325576));
#65109=CARTESIAN_POINT('Ctrl Pts',(0.00414540000171849,-0.035272816530353,
0.0699966069496375));
#65110=CARTESIAN_POINT('Ctrl Pts',(0.00413154020783471,-0.035246876490953,
0.0699739625538664));
#65111=CARTESIAN_POINT('Ctrl Pts',(0.00411768003099606,-0.0352209141752702,
0.0699512992251989));
#65112=CARTESIAN_POINT('Ctrl Pts',(0.00410382004319857,-0.0351949306073972,
0.0699286175303201));
#65113=CARTESIAN_POINT('',(0.00415785522820683,-0.0350943706855873,0.0697415899381972));
#65114=CARTESIAN_POINT('Origin',(0.0136873482790303,-0.0338370705545973,
0.0732991803912815));
#65115=CARTESIAN_POINT('',(0.00434993173275813,-0.035195137125489,0.0697074994996005));
#65116=CARTESIAN_POINT('Origin',(0.00669140170371844,-0.0338370705330846,
0.0795929263638979));
#65117=CARTESIAN_POINT('',(0.00441256730939742,-0.0352722979006262,0.0697555661864226));
#65118=CARTESIAN_POINT('Origin',(0.00806446930900352,-0.0346069579035356,
0.0659380622183925));
#65119=CARTESIAN_POINT('',(0.00455395171927896,-0.0352740680168101,0.0696420223302055));
#65120=CARTESIAN_POINT('Origin',(0.00403805897045731,-0.0305802162293176,
0.0690783640371152));
#65121=CARTESIAN_POINT('',(0.00469732891879462,-0.035272816532173,0.0695307341862665));
#65122=CARTESIAN_POINT('Origin',(0.00513144889000808,-0.0288496123713709,
0.0703198189757993));
#65123=CARTESIAN_POINT('',(0.00466459816065547,-0.0351949306052058,0.0694580695391812));
#65124=CARTESIAN_POINT('Ctrl Pts',(0.00469732891484825,-0.035272816530353,
0.0695307341899964));
#65125=CARTESIAN_POINT('Ctrl Pts',(0.00468641650492311,-0.0352468764909532,
0.0695065312592657));
#65126=CARTESIAN_POINT('Ctrl Pts',(0.00467550608798394,-0.0352209141752704,
0.069482309496933));
#65127=CARTESIAN_POINT('Ctrl Pts',(0.00466459816049193,-0.0351949306073975,
0.0694580695369053));
#65128=CARTESIAN_POINT('',(0.00474164803481453,-0.0350943706855873,0.0692792891176706));
#65129=CARTESIAN_POINT('Origin',(0.013750113884078,-0.0338370705527406,
0.0740031890922119));
#65130=CARTESIAN_POINT('',(0.00493648262366037,-0.0351951371254895,0.0692695410617723));
#65131=CARTESIAN_POINT('Origin',(0.0060205168904824,-0.0338370705331194,
0.0793704823860861));
#65132=CARTESIAN_POINT('',(0.00499259994678247,-0.035272297900626,0.0693250790477682));
#65133=CARTESIAN_POINT('Origin',(0.00909416572563785,-0.0346069579029593,
0.0659953819249899));
#65134=CARTESIAN_POINT('',(0.00514710031701445,-0.0352740680168101,0.0692301506840371));
#65135=CARTESIAN_POINT('Origin',(0.00470592065312846,-0.0305802162291783,
0.0686062784986003));
#65136=CARTESIAN_POINT('',(0.00530329504742269,-0.035272816532173,0.069137710008389));
#65137=CARTESIAN_POINT('Origin',(0.00563509330511477,-0.0288496123712193,
0.0699749822889916));
#65138=CARTESIAN_POINT('',(0.00527992967627283,-0.0351949306052063,0.0690615160919956));
#65139=CARTESIAN_POINT('Ctrl Pts',(0.00530329504303985,-0.035272816530353,
0.0691377100115949));
#65140=CARTESIAN_POINT('Ctrl Pts',(0.00529550211229662,-0.0352468764909533,
0.0691123302405803));
#65141=CARTESIAN_POINT('Ctrl Pts',(0.00528771351904963,-0.0352209141752707,
0.0690869320362439));
#65142=CARTESIAN_POINT('Ctrl Pts',(0.00527992967639571,-0.035194930607398,
0.0690615160897173));
#65143=CARTESIAN_POINT('',(0.00537877911748765,-0.0350943706855873,0.0688938023173803));
#65144=CARTESIAN_POINT('Origin',(0.0137241488906242,-0.0338370705481307,
0.0747095131024691));
#65145=CARTESIAN_POINT('',(0.00557329913277311,-0.03519513712549,0.0689085503768451));
#65146=CARTESIAN_POINT('Origin',(0.00538280182741146,-0.0338370705333044,
0.0790657082803801));
#65147=CARTESIAN_POINT('',(0.00562201319866981,-0.0352722979006257,0.0689706837947988));
#65148=CARTESIAN_POINT('Origin',(0.0101085586128168,-0.0346069579030927,
0.0661813048304526));
#65149=CARTESIAN_POINT('',(0.00578719296611978,-0.0352740680168101,0.0688958680005572));
#65150=CARTESIAN_POINT('Origin',(0.00542768405399171,-0.0305802162292022,
0.0682216207597974));
#65151=CARTESIAN_POINT('',(0.0059537419432158,-0.035272816532173,0.0688237326378758));
#65152=CARTESIAN_POINT('Origin',(0.00617798583012386,-0.0288496123715834,
0.069695988124715));
#65153=CARTESIAN_POINT('',(0.00594011044491611,-0.0351949306052065,0.0687452110757515));
#65154=CARTESIAN_POINT('Ctrl Pts',(0.00595374193846581,-0.035272816530353,
0.0688237326405072));
#65155=CARTESIAN_POINT('Ctrl Pts',(0.00594919138607751,-0.0352468764909533,
0.0687975762833586));
#65156=CARTESIAN_POINT('Ctrl Pts',(0.00594464744729082,-0.0352209141752707,
0.068771402181873));
#65157=CARTESIAN_POINT('Ctrl Pts',(0.00594011044532344,-0.0351949306073981,
0.0687452110735067));
#65158=CARTESIAN_POINT('',(0.00605920053781098,-0.0350943706857667,0.068591208894756));
#65159=CARTESIAN_POINT('Origin',(0.013609862705455,-0.0338370705544637,
0.0754070132109463));
#65160=CARTESIAN_POINT('',(0.00625033828333205,-0.0351951371254905,0.0686302204835654));
#65161=CARTESIAN_POINT('Origin',(0.00478831365572456,-0.0338370705271894,
0.0786834105677195));
#65162=CARTESIAN_POINT('',(0.00629088084208389,-0.0352722979006255,0.0686979694523592));
#65163=CARTESIAN_POINT('Origin',(0.0110916503910954,-0.0346069579032766,
0.0664928988182023));
#65164=CARTESIAN_POINT('',(0.00646413502314418,-0.0352740680168103,0.0686444461173757));
#65165=CARTESIAN_POINT('Origin',(0.0061919665330451,-0.0305802162293461,
0.0679304571029579));
#65166=CARTESIAN_POINT('',(0.00663841167006886,-0.0352728165321731,0.0685937536854215));
#65167=CARTESIAN_POINT('Origin',(0.00675156472634297,-0.0288496123711304,
0.0694872363888643));
#65168=CARTESIAN_POINT('',(0.00663472902149044,-0.0351949306052067,0.0685141428095075));
#65169=CARTESIAN_POINT('Ctrl Pts',(0.00663841166502647,-0.0352728165303531,
0.0685937536874368));
#65170=CARTESIAN_POINT('Ctrl Pts',(0.00663717525592264,-0.0352468764909534,
0.0685672332455315));
#65171=CARTESIAN_POINT('Ctrl Pts',(0.00663594763222532,-0.0352209141752708,
0.0685406960281127));
#65172=CARTESIAN_POINT('Ctrl Pts',(0.00663472902217576,-0.0351949306073982,
0.0685141428073316));
#65173=CARTESIAN_POINT('',(0.00677218164542555,-0.0350943706855873,0.0683762809279056));
#65174=CARTESIAN_POINT('Origin',(0.0134090578226959,-0.0338370705483153,
0.0760846895319725));
#65175=CARTESIAN_POINT('',(0.00695692276348947,-0.035195137125491,0.0684389408106166));
#65176=CARTESIAN_POINT('Origin',(0.00424642782830705,-0.0338370705333258,
0.0782296181675427));
#65177=CARTESIAN_POINT('',(0.00698865443472587,-0.0352722979006255,0.0685112368885413));
#65178=CARTESIAN_POINT('Origin',(0.0120279371145698,-0.034606957903202,
0.0669252498662866));
#65179=CARTESIAN_POINT('',(0.00716725070746612,-0.0352740680168103,0.0684798501077816));
#65180=CARTESIAN_POINT('Origin',(0.00698671489911995,-0.0305802162291834,
0.0677373793531191));
#65181=CARTESIAN_POINT('',(0.00734650657738756,-0.035272816532173,0.0684514000564886));
#65182=CARTESIAN_POINT('Origin',(0.00734678431164021,-0.0288496123715145,
0.0693520192202523));
#65183=CARTESIAN_POINT('',(0.00735283085609856,-0.0351949306052069,0.0683719553778551));
#65184=CARTESIAN_POINT('Ctrl Pts',(0.00734650657213241,-0.035272816530353,
0.0684514000578559));
#65185=CARTESIAN_POINT('Ctrl Pts',(0.0073486038052232,-0.0352468764909534,
0.0684249337744054));
#65186=CARTESIAN_POINT('Ctrl Pts',(0.00735071185697431,-0.0352209141752708,
0.0683984519488246));
#65187=CARTESIAN_POINT('Ctrl Pts',(0.00735283085705102,-0.0351949306073981,
0.0683719553757825));
#65188=CARTESIAN_POINT('',(0.00750647830044633,-0.0350943706855873,0.0682524079601858));
#65189=CARTESIAN_POINT('Origin',(0.0131249009244661,-0.0338370705545213,
0.0767318545731042));
#65190=CARTESIAN_POINT('',(0.0076819093138999,-0.0351951371254915,0.068337727952706));
#65191=CARTESIAN_POINT('Origin',(0.00376569017080977,-0.0338370705271979,
0.0777114878440688));
#65192=CARTESIAN_POINT('',(0.00770432967021006,-0.0352722979006254,0.068413430987425));
#65193=CARTESIAN_POINT('Origin',(0.0129026529829984,-0.0346069579031808,
0.0674715395396379));
#65194=CARTESIAN_POINT('',(0.00788545146471963,-0.0352740680168103,0.0684046757491718));
#65195=CARTESIAN_POINT('Origin',(0.007799395495655,-0.0305802162292729,
0.0676454324615505));
#65196=CARTESIAN_POINT('',(0.00806685958548826,-0.035272816532173,0.0683989167528435));
#65197=CARTESIAN_POINT('Origin',(0.00795425761772123,-0.0288496123715584,
0.0692924690748105));
#65198=CARTESIAN_POINT('Ctrl Pts',(0.00806685958010319,-0.035272816530353,
0.0683989167535414));
#65199=CARTESIAN_POINT('Ctrl Pts',(0.00807225738087576,-0.0352468764904448,
0.0683729220171362));
#65200=CARTESIAN_POINT('Ctrl Pts',(0.00807766786294621,-0.0352209141742528,
0.0683469132170922));
#65201=CARTESIAN_POINT('Ctrl Pts',(0.00808309105535896,-0.0351949306058699,
0.0683208911580634));
#65202=CARTESIAN_POINT('Ctrl Pts',(0.00611239953422995,-0.0321934096636941,
0.0795381792420887));
#65203=CARTESIAN_POINT('Ctrl Pts',(0.0062088453767827,-0.0320508460844199,
0.0795741820338511));
#65204=CARTESIAN_POINT('Ctrl Pts',(0.00630618582282729,-0.0319086045662818,
0.0796075663699033));
#65205=CARTESIAN_POINT('Ctrl Pts',(0.00640420536345943,-0.0317669892867522,
0.0796382776227359));
#65206=CARTESIAN_POINT('Ctrl Pts',(0.00619157146001148,-0.0321934096636941,
0.0795657879145643));
#65207=CARTESIAN_POINT('Ctrl Pts',(0.00628851148465414,-0.0320508460844199,
0.0796003735665574));
#65208=CARTESIAN_POINT('Ctrl Pts',(0.00638630766442437,-0.0319086045662818,
0.0796323285536707));
#65209=CARTESIAN_POINT('Ctrl Pts',(0.00648474376251334,-0.0317669892867522,
0.079661601406819));
#65210=CARTESIAN_POINT('Ctrl Pts',(0.00627074338579301,-0.0321934096636941,
0.07959339658704));
#65211=CARTESIAN_POINT('Ctrl Pts',(0.00636817759252559,-0.0320508460844199,
0.0796265650992637));
#65212=CARTESIAN_POINT('Ctrl Pts',(0.00646642950602144,-0.0319086045662818,
0.0796570907374381));
#65213=CARTESIAN_POINT('Ctrl Pts',(0.00656528216156726,-0.0317669892867522,
0.0796849251909021));
#65214=CARTESIAN_POINT('Ctrl Pts',(0.00634991531157455,-0.0321934096636941,
0.0796210052595158));
#65215=CARTESIAN_POINT('Ctrl Pts',(0.00644784370039705,-0.0320508460844199,
0.07965275663197));
#65216=CARTESIAN_POINT('Ctrl Pts',(0.00654655134761852,-0.0319086045662818,
0.0796818529212054));
#65217=CARTESIAN_POINT('Ctrl Pts',(0.00664582056062116,-0.0317669892867522,
0.0797082489749852));
#65218=CARTESIAN_POINT('',(0.00634849891017779,-0.0321934096636941,0.0796205113349072));
#65219=CARTESIAN_POINT('',(0.00657475148852131,-0.0318665617511335,0.0796888291962702));
#65220=CARTESIAN_POINT('Origin',(0.0120877674127181,-0.0326371944420803,
0.0639272420168472));
#65221=CARTESIAN_POINT('Origin',(0.00362254235843933,-0.0316939261509517,
0.0902449672848619));
#65222=CARTESIAN_POINT('',(0.00623028697057217,-0.0320197221621733,0.0795806781352575));
#65223=CARTESIAN_POINT('Ctrl Pts',(0.006230440319499,-0.0320197392094662,
0.0795807815711654));
#65224=CARTESIAN_POINT('Ctrl Pts',(0.00625807389753705,-0.0319792716575961,
0.0795904154589886));
#65225=CARTESIAN_POINT('Ctrl Pts',(0.00628590671902399,-0.0319386439829625,
0.0795998825366595));
#65226=CARTESIAN_POINT('Ctrl Pts',(0.00631397072666642,-0.0318979099381557,
0.0796091847358133));
#65227=CARTESIAN_POINT('Ctrl Pts',(0.00634203417960238,-0.0318571766984883,
0.0796184867511021));
#65228=CARTESIAN_POINT('Ctrl Pts',(0.00637018561218629,-0.0318163871833556,
0.0796275783066765));
#65229=CARTESIAN_POINT('Ctrl Pts',(0.00639832711295821,-0.0317755399638303,
0.0796364314820802));
#65230=CARTESIAN_POINT('',(0.00623046951091843,-0.0321934096636184,0.0795793523635383));
#65231=CARTESIAN_POINT('Origin',(0.00549057998102661,-0.032411138515515,
0.0817649442849136));
#65232=CARTESIAN_POINT('',(0.00628948421055811,-0.0321934096636663,0.0795999318492328));
#65233=CARTESIAN_POINT('Ctrl Pts',(0.00634761694800813,-0.0321934096636618,
0.0796186849094062));
#65234=CARTESIAN_POINT('Ctrl Pts',(0.00642303437495258,-0.0320835708272592,
0.0796431796123983));
#65235=CARTESIAN_POINT('Ctrl Pts',(0.00649891497332981,-0.0319739230346488,
0.0796660993477363));
#65236=CARTESIAN_POINT('Ctrl Pts',(0.00657515940862739,-0.0318646057455573,
0.0796874222421317));
#65237=CARTESIAN_POINT('Ctrl Pts',(0.0063968930671626,-0.0321934096636618,
0.0797207291588613));
#65238=CARTESIAN_POINT('Ctrl Pts',(0.00647371776383567,-0.0320835708272592,
0.0797445443057667));
#65239=CARTESIAN_POINT('Ctrl Pts',(0.00655099075229,-0.0319739230346488,
0.0797667557558143));
#65240=CARTESIAN_POINT('Ctrl Pts',(0.0066286109860951,-0.0318646057455573,
0.0797873426786399));
#65241=CARTESIAN_POINT('Ctrl Pts',(0.00644616918631708,-0.0321934096636618,
0.0798227734083164));
#65242=CARTESIAN_POINT('Ctrl Pts',(0.00652440115271877,-0.0320835708272592,
0.0798459089991351));
#65243=CARTESIAN_POINT('Ctrl Pts',(0.00660306653125019,-0.0319739230346488,
0.0798674121638922));
#65244=CARTESIAN_POINT('Ctrl Pts',(0.00668206256356282,-0.0318646057455573,
0.0798872631151482));
#65245=CARTESIAN_POINT('Ctrl Pts',(0.00649544530547155,-0.0321934096636618,
0.0799248176577715));
#65246=CARTESIAN_POINT('Ctrl Pts',(0.00657508454160187,-0.0320835708272592,
0.0799472736925035));
#65247=CARTESIAN_POINT('Ctrl Pts',(0.00665514231021038,-0.0319739230346488,
0.0799680685719702));
#65248=CARTESIAN_POINT('Ctrl Pts',(0.00673551414103053,-0.0318646057455573,
0.0799871835516564));
#65249=CARTESIAN_POINT('',(0.00650778413467281,-0.0321763980308508,0.0799282826387235));
#65250=CARTESIAN_POINT('',(0.00649544530549579,-0.0321934096636184,0.0799248176577655));
#65251=CARTESIAN_POINT('Origin',(0.0115523914991793,-0.032638623128404,
0.0641682690361009));
#65252=CARTESIAN_POINT('Ctrl Pts',(0.00650778413552138,-0.0321763980306373,
0.0799282826356648));
#65253=CARTESIAN_POINT('Ctrl Pts',(0.00651934361022421,-0.0321259596176374,
0.0798869497196757));
#65254=CARTESIAN_POINT('Ctrl Pts',(0.00653070280202329,-0.0320749164634477,
0.0798463329500821));
#65255=CARTESIAN_POINT('Ctrl Pts',(0.00655302976147259,-0.0319716057793998,
0.0797664990161937));
#65256=CARTESIAN_POINT('Ctrl Pts',(0.00656398882969326,-0.0319193786690191,
0.079727312958225));
#65257=CARTESIAN_POINT('Ctrl Pts',(0.00657475148901346,-0.0318665617525394,
0.0796888291944782));
#65258=CARTESIAN_POINT('',(0.00642197210784679,-0.0321934096636663,0.0797726644963464));
#65259=CARTESIAN_POINT('Ctrl Pts',(0.00642018079033925,-0.0327445246967098,
0.0796432565260038));
#65260=CARTESIAN_POINT('Ctrl Pts',(0.0066273623471771,-0.032443687833936,
0.0797075089032933));
#65261=CARTESIAN_POINT('Ctrl Pts',(0.00683879507475351,-0.0321434074405927,
0.0797559729847424));
#65262=CARTESIAN_POINT('Ctrl Pts',(0.00666051466053194,-0.0327445246967098,
0.0797121015028591));
#65263=CARTESIAN_POINT('Ctrl Pts',(0.00687029274811941,-0.032443687833936,
0.0797672895400524));
#65264=CARTESIAN_POINT('Ctrl Pts',(0.00708363186683336,-0.0321434074405927,
0.0798065194509301));
#65265=CARTESIAN_POINT('',(0.00669549827496981,-0.0326943950436612,0.0797211874900408));
#65266=CARTESIAN_POINT('',(0.00692559410938842,-0.0323666188837389,0.0797751640257003));
#65267=CARTESIAN_POINT('Origin',(0.0107966333535284,-0.032639557911179,
0.063418158651594));
#65268=CARTESIAN_POINT('',(0.00692587713480487,-0.0321934096636183,0.0797738352990901));
#65269=CARTESIAN_POINT('Origin',(0.0046246570713615,-0.0321933825603155,
0.0905774351089828));
#65270=CARTESIAN_POINT('',(0.0068036198394134,-0.032193409653269,0.0797477938830148));
#65271=CARTESIAN_POINT('',(0.00686474848660418,-0.0321934096584275,0.0797608145910825));
#65272=CARTESIAN_POINT('',(0.00657475148825586,-0.0325210109756238,0.0796888291971702));
#65273=CARTESIAN_POINT('Origin',(0.0112554365552375,-0.032639312915934,
0.0635619781636827));
#65274=CARTESIAN_POINT('',(0.00657511738662487,-0.0326943950436595,0.0796875208638126));
#65275=CARTESIAN_POINT('Origin',(0.00359563216993536,-0.0326943765538142,
0.0903411861737025));
#65276=CARTESIAN_POINT('',(0.00663530783080734,-0.0326943950436703,0.0797043541769368));
#65277=CARTESIAN_POINT('Ctrl Pts',(0.00680357784751435,-0.0321934096636941,
0.0797477849389554));
#65278=CARTESIAN_POINT('Ctrl Pts',(0.00695375916615836,-0.0319797282159868,
0.0797832043113791));
#65279=CARTESIAN_POINT('Ctrl Pts',(0.00710562359026252,-0.0317669959604736,
0.0798105201877894));
#65280=CARTESIAN_POINT('Ctrl Pts',(0.00704813442386174,-0.0321934096636941,
0.0797998767133908));
#65281=CARTESIAN_POINT('Ctrl Pts',(0.00719971329733514,-0.0319797282159868,
0.0798287349496652));
#65282=CARTESIAN_POINT('Ctrl Pts',(0.0073526214655046,-0.0317669959604736,
0.0798494241930394));
#65283=CARTESIAN_POINT('Ctrl Pts',(0.00704960156178621,-0.0321934096636941,
0.0798001892211097));
#65284=CARTESIAN_POINT('Ctrl Pts',(0.00720118881943688,-0.0319797282159868,
0.0798290080959742));
#65285=CARTESIAN_POINT('Ctrl Pts',(0.00735410324921062,-0.0317669959604736,
0.0798496575850109));
#65286=CARTESIAN_POINT('',(0.00692586345786333,-0.0320197259213208,0.079775175606695));
#65287=CARTESIAN_POINT('Ctrl Pts',(0.00692602729464874,-0.0320197391311198,
0.0797752572332416));
#65288=CARTESIAN_POINT('Ctrl Pts',(0.00695465041516763,-0.0319792715672862,
0.0797813517959236));
#65289=CARTESIAN_POINT('Ctrl Pts',(0.00698345031945878,-0.0319386438886458,
0.0797872558098532));
#65290=CARTESIAN_POINT('Ctrl Pts',(0.00701245886379329,-0.0318979098685799,
0.079792967204071));
#65291=CARTESIAN_POINT('Ctrl Pts',(0.00704146683463511,-0.0318571766538168,
0.0797986784853758));
#65292=CARTESIAN_POINT('Ctrl Pts',(0.00707053584027515,-0.031816387180722,
0.0798041699052481));
#65293=CARTESIAN_POINT('Ctrl Pts',(0.00709956503935144,-0.0317755399642094,
0.0798094261960755));
#65294=CARTESIAN_POINT('Origin',(0.00652527656989749,-0.0323427478904392,
0.0816545449409095));
#65295=CARTESIAN_POINT('',(0.00704813442396921,-0.0321934096636941,0.0797998767134112));
#65296=CARTESIAN_POINT('',(0.00698700577939704,-0.0321934096636663,0.0797868560062607));
#65297=CARTESIAN_POINT('',(0.00728116543148289,-0.0318665617561286,0.0798392989017126));
#65298=CARTESIAN_POINT('Origin',(0.0107752588915392,-0.0326371944422002,
0.0635110324311407));
#65299=CARTESIAN_POINT('Origin',(0.00567527026384143,-0.0316939261508471,
0.0906822086115865));
#65300=CARTESIAN_POINT('Ctrl Pts',(0.00669450361246156,-0.0326943950436604,
0.0797194204763658));
#65301=CARTESIAN_POINT('Ctrl Pts',(0.00677126066483236,-0.0325844576448134,
0.0797391186139606));
#65302=CARTESIAN_POINT('Ctrl Pts',(0.00684843053920001,-0.0324744968375322,
0.0797572306839354));
#65303=CARTESIAN_POINT('Ctrl Pts',(0.00692591404093729,-0.0323646534831894,
0.0797737348438269));
#65304=CARTESIAN_POINT('Ctrl Pts',(0.00675008982741099,-0.0326943950436604,
0.0798181691487118));
#65305=CARTESIAN_POINT('Ctrl Pts',(0.00682820782156145,-0.0325844576448134,
0.079837101204085));
#65306=CARTESIAN_POINT('Ctrl Pts',(0.00690672289018837,-0.0324744968375322,
0.079854418991114));
#65307=CARTESIAN_POINT('Ctrl Pts',(0.0069855341291601,-0.0323646534831894,
0.07987010170879));
#65308=CARTESIAN_POINT('Ctrl Pts',(0.00680567604236041,-0.0326943950436604,
0.0799169178210579));
#65309=CARTESIAN_POINT('Ctrl Pts',(0.00688515497829054,-0.0325844576448134,
0.0799350837942094));
#65310=CARTESIAN_POINT('Ctrl Pts',(0.00696501524117674,-0.0324744968375322,
0.0799516072982926));
#65311=CARTESIAN_POINT('Ctrl Pts',(0.00704515421738291,-0.0323646534831894,
0.0799664685737531));
#65312=CARTESIAN_POINT('Ctrl Pts',(0.00686126225730983,-0.0326943950436604,
0.080015666493404));
#65313=CARTESIAN_POINT('Ctrl Pts',(0.00694210213501962,-0.0325844576448134,
0.0800330663843338));
#65314=CARTESIAN_POINT('Ctrl Pts',(0.0070233075921651,-0.0324744968375322,
0.0800487956054711));
#65315=CARTESIAN_POINT('Ctrl Pts',(0.00710477430560572,-0.0323646534831894,
0.0800628354387162));
#65316=CARTESIAN_POINT('',(0.00687379430653122,-0.0326773559991385,0.0800183498757061));
#65317=CARTESIAN_POINT('',(0.00686126225730346,-0.0326943950436594,0.0800156664933914));
#65318=CARTESIAN_POINT('Origin',(0.0102840270947223,-0.0326395669596865,
0.0637670848817632));
#65319=CARTESIAN_POINT('Ctrl Pts',(0.00687379430722387,-0.0326773559987502,
0.0800183498724243));
#65320=CARTESIAN_POINT('Ctrl Pts',(0.00688274285206967,-0.0326267922587361,
0.0799763389116804));
#65321=CARTESIAN_POINT('Ctrl Pts',(0.00689153279042086,-0.0325756109582127,
0.0799350725648748));
#65322=CARTESIAN_POINT('Ctrl Pts',(0.00690880293489446,-0.0324719985462384,
0.0798539939790238));
#65323=CARTESIAN_POINT('Ctrl Pts',(0.00691727621436546,-0.0324196091621787,
0.0798142142587047));
#65324=CARTESIAN_POINT('Ctrl Pts',(0.0069255941093985,-0.0323666188837757,
0.0797751640256525));
#65325=CARTESIAN_POINT('',(0.00677838026614664,-0.0326943950436703,0.0798684269917262));
#65326=CARTESIAN_POINT('Ctrl Pts',(0.0070470305045208,-0.0321934096636617,
0.0797981752289914));
#65327=CARTESIAN_POINT('Ctrl Pts',(0.00712492324285888,-0.0320835708272592,
0.0798130244739482));
#65328=CARTESIAN_POINT('Ctrl Pts',(0.00720307810459581,-0.0319739230346488,
0.0798262531195679));
#65329=CARTESIAN_POINT('Ctrl Pts',(0.00728139379705147,-0.0318646057455573,
0.079837851914955));
#65330=CARTESIAN_POINT('Ctrl Pts',(0.00710870760250867,-0.0321934096636617,
0.0798932388937096));
#65331=CARTESIAN_POINT('Ctrl Pts',(0.00718791134287151,-0.0320835708272592,
0.0799072375634168));
#65332=CARTESIAN_POINT('Ctrl Pts',(0.00726735884358815,-0.0319739230346488,
0.0799195889960363));
#65333=CARTESIAN_POINT('Ctrl Pts',(0.00734694724427252,-0.0318646057455573,
0.0799302851899337));
#65334=CARTESIAN_POINT('Ctrl Pts',(0.00717038470049655,-0.0321934096636617,
0.0799883025584277));
#65335=CARTESIAN_POINT('Ctrl Pts',(0.00725089944288413,-0.0320835708272592,
0.0800014506528853));
#65336=CARTESIAN_POINT('Ctrl Pts',(0.00733163958258048,-0.0319739230346488,
0.0800129248725047));
#65337=CARTESIAN_POINT('Ctrl Pts',(0.00741250069149358,-0.0318646057455573,
0.0800227184649123));
#65338=CARTESIAN_POINT('Ctrl Pts',(0.00723206179848442,-0.0321934096636617,
0.0800833662231458));
#65339=CARTESIAN_POINT('Ctrl Pts',(0.00731388754289675,-0.0320835708272592,
0.0800956637423538));
#65340=CARTESIAN_POINT('Ctrl Pts',(0.00739592032157282,-0.0319739230346488,
0.0801062607489731));
#65341=CARTESIAN_POINT('Ctrl Pts',(0.00747805413871463,-0.0318646057455573,
0.080115151739891));
#65342=CARTESIAN_POINT('',(0.00723206179850728,-0.0321934096636184,0.0800833662231361));
#65343=CARTESIAN_POINT('',(0.00714009811124825,-0.0321934096636663,0.0799416214682837));
#65344=CARTESIAN_POINT('',(0.0072447376095977,-0.0321763980308323,0.0800852574163262));
#65345=CARTESIAN_POINT('Origin',(0.0102743132755924,-0.032638623121943,
0.0638172591966035));
#65346=CARTESIAN_POINT('Ctrl Pts',(0.0072447376100568,-0.032176398030638,
0.0800852574131847));
#65347=CARTESIAN_POINT('Ctrl Pts',(0.00725102554679725,-0.0321259596179443,
0.0800428016334987));
#65348=CARTESIAN_POINT('Ctrl Pts',(0.00725720453687498,-0.0320749164640583,
0.0800010814552825));
#65349=CARTESIAN_POINT('Ctrl Pts',(0.00726934959633817,-0.0319716057814242,
0.0799190787268633));
#65350=CARTESIAN_POINT('Ctrl Pts',(0.00727531093351594,-0.0319193786724658,
0.0798788281282486));
#65351=CARTESIAN_POINT('Ctrl Pts',(0.00728116543149043,-0.0318665617561676,
0.0798392989016617));
#65352=CARTESIAN_POINT('Origin',(0.00812378219310841,-0.0315241814719618,
0.07415));
#65353=CARTESIAN_POINT('',(0.00650778413457271,-0.032210423332376,0.0799282826390797));
#65354=CARTESIAN_POINT('',(0.00652013033595527,-0.0321934096636183,0.0799317212593733));
#65355=CARTESIAN_POINT('Origin',(0.011510859167661,-0.0326387222458553,
0.064150091005772));
#65356=CARTESIAN_POINT('Origin',(0.0103707261840096,-0.0326386250403645,
0.0638377917879493));
#65357=CARTESIAN_POINT('Origin',(0.0104156615022366,-0.0326387237688314,
0.0638438037632278));
#65358=CARTESIAN_POINT('Ctrl Pts',(0.00628253620983209,-0.0325229783203769,
0.0798605002608448));
#65359=CARTESIAN_POINT('Ctrl Pts',(0.00636125533104743,-0.032413025309245,
0.0798858817964589));
#65360=CARTESIAN_POINT('Ctrl Pts',(0.00644048756263473,-0.0323031222208069,
0.0799096310763216));
#65361=CARTESIAN_POINT('Ctrl Pts',(0.00652013034027635,-0.0321934096576658,
0.0799317212605718));
#65362=CARTESIAN_POINT('Ctrl Pts',(0.00638006773521382,-0.0325229783203769,
0.0798028049942006));
#65363=CARTESIAN_POINT('Ctrl Pts',(0.00645799152844019,-0.032413025309245,
0.0798268420598701));
#65364=CARTESIAN_POINT('Ctrl Pts',(0.00653640074057769,-0.0323031222208069,
0.0798492635260847));
#65365=CARTESIAN_POINT('Ctrl Pts',(0.00661519392155494,-0.0321934096576658,
0.0798700442166176));
#65366=CARTESIAN_POINT('Ctrl Pts',(0.00647759926059556,-0.0325229783203769,
0.0797451097275563));
#65367=CARTESIAN_POINT('Ctrl Pts',(0.00655472772583294,-0.032413025309245,
0.0797678023232814));
#65368=CARTESIAN_POINT('Ctrl Pts',(0.00663231391852064,-0.0323031222208069,
0.0797888959758477));
#65369=CARTESIAN_POINT('Ctrl Pts',(0.00671025750283354,-0.0321934096576658,
0.0798083671726634));
#65370=CARTESIAN_POINT('Ctrl Pts',(0.00657513078597729,-0.0325229783203769,
0.0796874144609121));
#65371=CARTESIAN_POINT('Ctrl Pts',(0.0066514639232257,-0.032413025309245,
0.0797087625866926));
#65372=CARTESIAN_POINT('Ctrl Pts',(0.00672822709646359,-0.0323031222208069,
0.0797285284256107));
#65373=CARTESIAN_POINT('Ctrl Pts',(0.00680532108411213,-0.0321934096576658,
0.0797466901287092));
#65374=CARTESIAN_POINT('',(0.00666187508717938,-0.0321934096584275,0.0798397575712243));
#65375=CARTESIAN_POINT('Ctrl Pts',(0.00650778413550527,-0.0322104233328919,
0.0799282826357219));
#65376=CARTESIAN_POINT('Ctrl Pts',(0.00651935927351475,-0.032260942183129,
0.0798868937128506));
#65377=CARTESIAN_POINT('Ctrl Pts',(0.00653072611711976,-0.0323120888240578,
0.0798462495829169));
#65378=CARTESIAN_POINT('Ctrl Pts',(0.00655305324555121,-0.0324156524631808,
0.0797664150448035));
#65379=CARTESIAN_POINT('Ctrl Pts',(0.00656400435275298,-0.0324680267167312,
0.0797272574528198));
#65380=CARTESIAN_POINT('Ctrl Pts',(0.00657475148827184,-0.0325210109755912,
0.0796888291971297));
#65381=CARTESIAN_POINT('Origin',(0.000857015991460974,-0.0262834582511143,
0.0711337946337778));
#65382=CARTESIAN_POINT('Origin',(-4.30651632228096E-5,-0.0342770750354629,
0.0831569757493063));
#65383=CARTESIAN_POINT('Origin',(0.00812378219310841,-0.0315241814719618,
0.07415));
#65384=CARTESIAN_POINT('',(0.00687379430654047,-0.0327114338379849,0.0800183498756619));
#65385=CARTESIAN_POINT('',(0.00688633205822609,-0.0326943950436593,0.080021006486431));
#65386=CARTESIAN_POINT('Origin',(0.0102395545876542,-0.0326395654975294,
0.0637584004514019));
#65387=CARTESIAN_POINT('Origin',(0.0103823027994842,-0.0326395685578362,
0.0637880142693136));
#65388=CARTESIAN_POINT('Origin',(0.0104264524945685,-0.0326395670824504,
0.0637982142985762));
#65389=CARTESIAN_POINT('Origin',(0.00812378219310841,-0.0315241814719618,
0.07415));
#65390=CARTESIAN_POINT('',(0.00724473760954337,-0.0322104233323761,0.0800852574166919));
#65391=CARTESIAN_POINT('Origin',(0.00910588055929315,-0.0326387236910637,
0.0636378225172512));
#65392=CARTESIAN_POINT('',(0.00725741743084164,-0.0321934096636185,0.0800871215330948));
#65393=CARTESIAN_POINT('Origin',(0.0102308302744509,-0.0326387223938502,
0.063804430290524));
#65394=CARTESIAN_POINT('Origin',(0.00906054610542325,-0.032638624887444,
0.0636374902704471));
#65395=CARTESIAN_POINT('Ctrl Pts',(0.00676850500884118,-0.0332451089994433,
0.0797393960992048));
#65396=CARTESIAN_POINT('Ctrl Pts',(0.00697931253171443,-0.0329451141710254,
0.0797905112144965));
#65397=CARTESIAN_POINT('Ctrl Pts',(0.00719337137210792,-0.0326442513127493,
0.0798256022327296));
#65398=CARTESIAN_POINT('Ctrl Pts',(0.00701268781257067,-0.0332451089994433,
0.0797930128723526));
#65399=CARTESIAN_POINT('Ctrl Pts',(0.00722551752512797,-0.0329451141710254,
0.0798349184825263));
#65400=CARTESIAN_POINT('Ctrl Pts',(0.00744089911280378,-0.0326442513127493,
0.0798606738392798));
#65401=CARTESIAN_POINT('Ctrl Pts',(0.00701512964060797,-0.0332451089994433,
0.0797935490400841));
#65402=CARTESIAN_POINT('Ctrl Pts',(0.0072279795750621,-0.0329451141710254,
0.0798353625552067));
#65403=CARTESIAN_POINT('Ctrl Pts',(0.00744337439021074,-0.0326442513127493,
0.0798610245553452));
#65404=CARTESIAN_POINT('',(0.00704813442391742,-0.0331951640388616,0.0797998767134014));
#65405=CARTESIAN_POINT('',(0.00728116544438958,-0.0328677532355034,0.0798392989097624));
#65406=CARTESIAN_POINT('Origin',(0.00942570137070009,-0.0326402808280126,
0.0632053166742233));
#65407=CARTESIAN_POINT('',(0.00728136446697921,-0.0326943950436593,0.0798379550257279));
#65408=CARTESIAN_POINT('Origin',(0.0056617568152294,-0.0326944278779099,
0.0907760213917055));
#65409=CARTESIAN_POINT('',(0.00715771327076763,-0.0326943950436593,0.0798196415968991));
#65410=CARTESIAN_POINT('',(0.00721953886888343,-0.0326943950436693,0.0798287983113235));
#65411=CARTESIAN_POINT('',(0.00692559410938562,-0.0330220786163545,0.0797751640256997));
#65412=CARTESIAN_POINT('Origin',(0.00990488328926026,-0.0326396682763397,
0.06324452552734));
#65413=CARTESIAN_POINT('',(0.00692587713480482,-0.0331951640388587,0.0797738352990901));
#65414=CARTESIAN_POINT('Origin',(0.00462763753303142,-0.0331952026560205,
0.0905634351200403));
#65415=CARTESIAN_POINT('',(0.00698700577937112,-0.0331951640388701,0.0797868560062557));
#65416=CARTESIAN_POINT('Ctrl Pts',(0.00712210179944357,-0.0327445246967096,
0.0798134584300539));
#65417=CARTESIAN_POINT('Ctrl Pts',(0.00733570262603343,-0.032443687833936,
0.0798512374237038));
#65418=CARTESIAN_POINT('Ctrl Pts',(0.00755154230344066,-0.0321434074405928,
0.0798728198039668));
#65419=CARTESIAN_POINT('Ctrl Pts',(0.00736916912884946,-0.0327445246967096,
0.0798516387226174));
#65420=CARTESIAN_POINT('Ctrl Pts',(0.00758420994871405,-0.032443687833936,
0.0798800994196052));
#65421=CARTESIAN_POINT('Ctrl Pts',(0.00780078363633826,-0.0321434074405928,
0.079892281509324));
#65422=CARTESIAN_POINT('Ctrl Pts',(0.00737163980214352,-0.0327445246967096,
0.079852020525543));
#65423=CARTESIAN_POINT('Ctrl Pts',(0.00758669502194085,-0.032443687833936,
0.0798803880395643));
#65424=CARTESIAN_POINT('Ctrl Pts',(0.00780327604966724,-0.0321434074405928,
0.0798924761263776));
#65425=CARTESIAN_POINT('',(0.00728116543147845,-0.0325210109756238,0.079839298901712));
#65426=CARTESIAN_POINT('',(0.00751561932206926,-0.032193409653269,0.079869113822887));
#65427=CARTESIAN_POINT('Origin',(0.00990371151108213,-0.0326393129157963,
0.0632529675118896));
#65428=CARTESIAN_POINT('Origin',(0.00566063188032259,-0.0326943765538233,
0.0907810415460278));
#65429=CARTESIAN_POINT('',(0.00740501566319187,-0.0326943950436612,0.079856268454557));
#65430=CARTESIAN_POINT('',(0.00734319006509555,-0.0326943950436702,0.0798471117401525));
#65431=CARTESIAN_POINT('',(0.00764006217698056,-0.0323666188837389,0.0798809807141534));
#65432=CARTESIAN_POINT('Origin',(0.00943050074521163,-0.0326395579110436,
0.0631677853481666));
#65433=CARTESIAN_POINT('',(0.00764017643705447,-0.0321934096636184,0.0798796269924588));
#65434=CARTESIAN_POINT('Origin',(0.00671115127334794,-0.0321933825602894,
0.0908864564610883));
#65435=CARTESIAN_POINT('',(0.00757789787906403,-0.0321934096584275,0.0798743704077667));
#65436=CARTESIAN_POINT('Ctrl Pts',(0.00664473569757571,-0.0330240426238172,
0.0799648449217574));
#65437=CARTESIAN_POINT('Ctrl Pts',(0.00672484085150183,-0.032914277406352,
0.0799852202281985));
#65438=CARTESIAN_POINT('Ctrl Pts',(0.00680540715526839,-0.0328043479726691,
0.0800039496951787));
#65439=CARTESIAN_POINT('Ctrl Pts',(0.00688633205822612,-0.0326943950436593,
0.080021006486431));
#65440=CARTESIAN_POINT('Ctrl Pts',(0.00673845201798835,-0.0330240426238172,
0.0799011394488928));
#65441=CARTESIAN_POINT('Ctrl Pts',(0.00681767956696052,-0.032914277406352,
0.0799202237217169));
#65442=CARTESIAN_POINT('Ctrl Pts',(0.00689734113898388,-0.0328043479726691,
0.0799376796539984));
#65443=CARTESIAN_POINT('Ctrl Pts',(0.00697733529750685,-0.0326943950436593,
0.079953482072883));
#65444=CARTESIAN_POINT('Ctrl Pts',(0.00683216833840099,-0.0330240426238172,
0.0798374339760282));
#65445=CARTESIAN_POINT('Ctrl Pts',(0.00691051828241921,-0.032914277406352,
0.0798552272152352));
#65446=CARTESIAN_POINT('Ctrl Pts',(0.00698927512269936,-0.0328043479726691,
0.0798714096128182));
#65447=CARTESIAN_POINT('Ctrl Pts',(0.00706833853678758,-0.0326943950436593,
0.079885957659335));
#65448=CARTESIAN_POINT('Ctrl Pts',(0.00692588465881363,-0.0330240426238172,
0.0797737285031636));
#65449=CARTESIAN_POINT('Ctrl Pts',(0.00700335699787791,-0.032914277406352,
0.0797902307087535));
#65450=CARTESIAN_POINT('Ctrl Pts',(0.00708120910641484,-0.0328043479726691,
0.0798051395716379));
#65451=CARTESIAN_POINT('Ctrl Pts',(0.00715934177606831,-0.0326943950436593,
0.079818433245787));
#65452=CARTESIAN_POINT('',(0.00702202266450686,-0.0326943950436694,0.0799203240416751));
#65453=CARTESIAN_POINT('Ctrl Pts',(0.00687379430722661,-0.0327114338383317,
0.0800183498724113));
#65454=CARTESIAN_POINT('Ctrl Pts',(0.00688274136365943,-0.0327619876830968,
0.0799763458993577));
#65455=CARTESIAN_POINT('Ctrl Pts',(0.00689153057501085,-0.0328131562604328,
0.0799350829656163));
#65456=CARTESIAN_POINT('Ctrl Pts',(0.00690880070357794,-0.0329167375858765,
0.079854004454442));
#65457=CARTESIAN_POINT('Ctrl Pts',(0.00691727473948476,-0.032969108892062,
0.0798142211828647));
#65458=CARTESIAN_POINT('Ctrl Pts',(0.00692559410939825,-0.0330220786163187,
0.0797751640256538));
#65459=CARTESIAN_POINT('Ctrl Pts',(0.00701277044732563,-0.0325229783203769,
0.0800462405735153));
#65460=CARTESIAN_POINT('Ctrl Pts',(0.00709404999468926,-0.032413025309245,
0.0800615558461347));
#65461=CARTESIAN_POINT('Ctrl Pts',(0.00717563403050498,-0.032303122220807,
0.0800751874240448));
#65462=CARTESIAN_POINT('Ctrl Pts',(0.00725741743527886,-0.0321934096576659,
0.0800871215337423));
#65463=CARTESIAN_POINT('Ctrl Pts',(0.00710230177316844,-0.0325229783203769,
0.0799767763098309));
#65464=CARTESIAN_POINT('Ctrl Pts',(0.00718262375717627,-0.032413025309245,
0.0799908573950815));
#65465=CARTESIAN_POINT('Ctrl Pts',(0.00726322484411828,-0.032303122220807,
0.0800032747812394));
#65466=CARTESIAN_POINT('Ctrl Pts',(0.00734400122846935,-0.0321934096576659,
0.080014016205666));
#65467=CARTESIAN_POINT('Ctrl Pts',(0.00719183309901126,-0.0325229783203769,
0.0799073120461464));
#65468=CARTESIAN_POINT('Ctrl Pts',(0.00727119751966328,-0.032413025309245,
0.0799201589440282));
#65469=CARTESIAN_POINT('Ctrl Pts',(0.00735081565773157,-0.032303122220807,
0.0799313621384341));
#65470=CARTESIAN_POINT('Ctrl Pts',(0.00743058502165983,-0.0321934096576659,
0.0799409108775897));
#65471=CARTESIAN_POINT('Ctrl Pts',(0.00728136442485407,-0.0325229783203769,
0.079837847782462));
#65472=CARTESIAN_POINT('Ctrl Pts',(0.00735977128215028,-0.032413025309245,
0.0798494604929749));
#65473=CARTESIAN_POINT('Ctrl Pts',(0.00743840647134487,-0.032303122220807,
0.0798594494956288));
#65474=CARTESIAN_POINT('Ctrl Pts',(0.00751716881485032,-0.0321934096576659,
0.0798678055495134));
#65475=CARTESIAN_POINT('Ctrl Pts',(0.0072447376100483,-0.0322104233328924,
0.0800852574132425));
#65476=CARTESIAN_POINT('Ctrl Pts',(0.00725103406710004,-0.0322609421831292,
0.0800427441049149));
#65477=CARTESIAN_POINT('Ctrl Pts',(0.00725721721951797,-0.0323120888240568,
0.0800009958228221));
#65478=CARTESIAN_POINT('Ctrl Pts',(0.0072693623710612,-0.032415652463181,
0.0799189924726836));
#65479=CARTESIAN_POINT('Ctrl Pts',(0.00727531937788986,-0.0324680267167315,
0.0798787711123318));
#65480=CARTESIAN_POINT('Ctrl Pts',(0.00728116543148923,-0.0325210109755912,
0.0798392989016698));
#65481=CARTESIAN_POINT('',(0.00738651837595761,-0.0321934096584275,0.0799781176780848));
#65482=CARTESIAN_POINT('Ctrl Pts',(0.0070470305962444,-0.0331951640388604,
0.0797981753703263));
#65483=CARTESIAN_POINT('Ctrl Pts',(0.00716380300075277,-0.0330306422010619,
0.0798204365192424));
#65484=CARTESIAN_POINT('Ctrl Pts',(0.00728139570075475,-0.0328657861914644,
0.0798378523198839));
#65485=CARTESIAN_POINT('Ctrl Pts',(0.00704813442391434,-0.0331951640388604,
0.0797998767134008));
#65486=CARTESIAN_POINT('Ctrl Pts',(0.00716494200259997,-0.0330306422010619,
0.0798221150413876));
#65487=CARTESIAN_POINT('Ctrl Pts',(0.00728256890351013,-0.0328657861914644,
0.0798395065868143));
#65488=CARTESIAN_POINT('Ctrl Pts',(0.00723206179851563,-0.0331951640388604,
0.0800833662231506));
#65489=CARTESIAN_POINT('Ctrl Pts',(0.00735473034105878,-0.0330306422010619,
0.0801018019705908));
#65490=CARTESIAN_POINT('Ctrl Pts',(0.00747805603302103,-0.0328657861914644,
0.0801151519449496));
#65491=CARTESIAN_POINT('',(0.0072447376087371,-0.0331781648281939,0.0800852574177228));
#65492=CARTESIAN_POINT('',(0.00723206179850726,-0.0331951640388588,0.0800833662231361));
#65493=CARTESIAN_POINT('Origin',(0.00895854672991136,-0.0326412092321598,
0.0636520794477061));
#65494=CARTESIAN_POINT('Ctrl Pts',(0.0072447376074011,-0.033178164828644,
0.0800852574164436));
#65495=CARTESIAN_POINT('Ctrl Pts',(0.00725103492480123,-0.0331276811546784,
0.080042738216493));
#65496=CARTESIAN_POINT('Ctrl Pts',(0.00725721849869883,-0.0330765663497804,
0.0800009867766641));
#65497=CARTESIAN_POINT('Ctrl Pts',(0.00726936363266433,-0.0329730614463303,
0.0799189835691956));
#65498=CARTESIAN_POINT('Ctrl Pts',(0.00727532029166565,-0.0329207133374016,
0.079878764929847));
#65499=CARTESIAN_POINT('Ctrl Pts',(0.00728116542928284,-0.0328677532289389,
0.079839298916334));
#65500=CARTESIAN_POINT('',(0.00714009811122234,-0.0331951640388701,0.0799416214682788));
#65501=CARTESIAN_POINT('Ctrl Pts',(0.00740380737835698,-0.0326943950436604,
0.0798546400385811));
#65502=CARTESIAN_POINT('Ctrl Pts',(0.00752174670447765,-0.0325294772287039,
0.079869524999578));
#65503=CARTESIAN_POINT('Ctrl Pts',(0.00764020046178808,-0.0323646534831895,
0.0798795227037504));
#65504=CARTESIAN_POINT('Ctrl Pts',(0.00740501566318987,-0.0326943950436604,
0.0798562684545567));
#65505=CARTESIAN_POINT('Ctrl Pts',(0.00752298865563857,-0.0325294772287039,
0.0798711284351345));
#65506=CARTESIAN_POINT('Ctrl Pts',(0.00764147501804653,-0.0323646534831895,
0.0798810997887738));
#65507=CARTESIAN_POINT('Ctrl Pts',(0.00760638055272833,-0.0326943950436604,
0.0801276496671071));
#65508=CARTESIAN_POINT('Ctrl Pts',(0.00772996415638362,-0.0325294772287039,
0.080138346573553));
#65509=CARTESIAN_POINT('Ctrl Pts',(0.00785388427222964,-0.0323646534831895,
0.0801439265187721));
#65510=CARTESIAN_POINT('',(0.00760638055272024,-0.0326943950436594,0.0801276496670952));
#65511=CARTESIAN_POINT('',(0.00750569810796606,-0.0326943950436702,0.0799919590608361));
#65512=CARTESIAN_POINT('',(0.00761915009913651,-0.0326773559992498,0.080128741208886));
#65513=CARTESIAN_POINT('Origin',(0.0089656686821606,-0.0326395670106896,
0.0635782065413069));
#65514=CARTESIAN_POINT('Ctrl Pts',(0.00761915009765573,-0.0326773559997669,
0.0801287412078143));
#65515=CARTESIAN_POINT('Ctrl Pts',(0.00762276268675555,-0.0326267924002059,
0.0800859400983815));
#65516=CARTESIAN_POINT('Ctrl Pts',(0.00762631123906512,-0.0325756107621957,
0.0800438972503982));
#65517=CARTESIAN_POINT('Ctrl Pts',(0.00763328334109336,-0.0324719987229943,
0.0799612937629902));
#65518=CARTESIAN_POINT('Ctrl Pts',(0.00763670417734596,-0.0324196089019014,
0.079920765339583));
#65519=CARTESIAN_POINT('Ctrl Pts',(0.00764006217694614,-0.0323666188837573,
0.079880980714126));
#65520=CARTESIAN_POINT('Origin',(0.00812378219310841,-0.0315241814719618,
0.07415));
#65521=CARTESIAN_POINT('',(0.00724473760960414,-0.0332121607144381,0.0800852574162843));
#65522=CARTESIAN_POINT('',(0.00725741743084167,-0.0331951640388587,0.0800871215330948));
#65523=CARTESIAN_POINT('Origin',(0.00891321520677268,-0.0326413632176459,
0.0636532890694186));
#65524=CARTESIAN_POINT('Origin',(0.0103677068612828,-0.0326412105375278,
0.0638607799806587));
#65525=CARTESIAN_POINT('Origin',(0.0104107413389209,-0.032641364003851,
0.0638750845771472));
#65526=CARTESIAN_POINT('Origin',(0.00812378219310841,-0.0315241814719618,
0.07415));
#65527=CARTESIAN_POINT('',(0.00761915009998218,-0.0327114338379849,0.0801287412078418));
#65528=CARTESIAN_POINT('Origin',(0.0091108725407328,-0.0326395670427101,
0.0635912399722349));
#65529=CARTESIAN_POINT('',(0.00763192194936946,-0.0326943950436594,0.0801298054734803));
#65530=CARTESIAN_POINT('Origin',(0.00892045828662401,-0.0326395654740188,
0.0635751647114222));
#65531=CARTESIAN_POINT('Origin',(0.00906579254212087,-0.0326395685432592,
0.063586653804524));
#65532=CARTESIAN_POINT('Ctrl Pts',(0.00712211991050009,-0.0337436976235975,
0.0798134616332768));
#65533=CARTESIAN_POINT('Ctrl Pts',(0.00717305794275089,-0.0336723290703325,
0.0798224707356528));
#65534=CARTESIAN_POINT('Ctrl Pts',(0.00722414977978394,-0.033601104548885,
0.0798305621659212));
#65535=CARTESIAN_POINT('Ctrl Pts',(0.0073872758947078,-0.0333736987606856,
0.0798563964999464));
#65536=CARTESIAN_POINT('Ctrl Pts',(0.00755161571374524,-0.0331450831799191,
0.0798728271439816));
#65537=CARTESIAN_POINT('Ctrl Pts',(0.00736918736200067,-0.0337436976235975,
0.079851641135749));
#65538=CARTESIAN_POINT('Ctrl Pts',(0.00742046878648296,-0.0336723290703325,
0.079858428076022));
#65539=CARTESIAN_POINT('Ctrl Pts',(0.00747186399050261,-0.033601104548885,
0.0798642915271371));
#65540=CARTESIAN_POINT('Ctrl Pts',(0.00763595869612106,-0.0333736987606856,
0.0798830123650636));
#65541=CARTESIAN_POINT('Ctrl Pts',(0.00780085729627007,-0.0331450831799191,
0.07989228565216));
#65542=CARTESIAN_POINT('Ctrl Pts',(0.00737165803651567,-0.0337436976235975,
0.0798520229307737));
#65543=CARTESIAN_POINT('Ctrl Pts',(0.00742294289492028,-0.0336723290703325,
0.0798587876494257));
#65544=CARTESIAN_POINT('Ctrl Pts',(0.0074743411326098,-0.033601104548885,
0.0798646288207493));
#65545=CARTESIAN_POINT('Ctrl Pts',(0.00763844552413519,-0.0333736987606856,
0.0798832785237148));
#65546=CARTESIAN_POINT('Ctrl Pts',(0.00780334971209532,-0.0331450831799191,
0.0798924802372417));
#65547=CARTESIAN_POINT('',(0.0074050156632065,-0.0336938721132548,0.0798562684545589));
#65548=CARTESIAN_POINT('',(0.00764006219165131,-0.0333679870047996,0.0798809807154008));
#65549=CARTESIAN_POINT('Ctrl Pts',(0.00740501566320096,-0.0336938721132527,
0.0798562684545586));
#65550=CARTESIAN_POINT('Ctrl Pts',(0.00742728990584582,-0.0336629187933873,
0.0798590741375051));
#65551=CARTESIAN_POINT('Ctrl Pts',(0.00744957345305481,-0.0336319952301012,
0.0798617484984804));
#65552=CARTESIAN_POINT('Ctrl Pts',(0.00747186399050984,-0.0336011045488922,
0.0798642915271382));
#65553=CARTESIAN_POINT('Ctrl Pts',(0.00752779857637719,-0.0335235892595425,
0.0798706728562161));
#65554=CARTESIAN_POINT('Ctrl Pts',(0.00758387658419767,-0.0334458668665543,
0.0798762384027458));
#65555=CARTESIAN_POINT('Ctrl Pts',(0.00764006217985969,-0.0333679869962467,
0.0798809807146459));
#65556=CARTESIAN_POINT('',(0.00764017643705453,-0.0331951640388586,0.0798796269924588));
#65557=CARTESIAN_POINT('Ctrl Pts',(0.00764010643901735,-0.0333679692468943,
0.0798809851401499));
#65558=CARTESIAN_POINT('Ctrl Pts',(0.00764013865025297,-0.0333391895417487,
0.0798805330337325));
#65559=CARTESIAN_POINT('Ctrl Pts',(0.00764015955517311,-0.0333104081136032,
0.0798801939271189));
#65560=CARTESIAN_POINT('Ctrl Pts',(0.00764018169841457,-0.033253269932262,
0.0798797447215171));
#65561=CARTESIAN_POINT('Ctrl Pts',(0.00764018322692077,-0.0332249176543048,
0.0798796312789282));
#65562=CARTESIAN_POINT('Ctrl Pts',(0.00764017665659403,-0.0331960985149987,
0.0798796270408481));
#65563=CARTESIAN_POINT('Ctrl Pts',(0.00764017654790957,-0.0331956312777104,
0.0798796270018154));
#65564=CARTESIAN_POINT('Ctrl Pts',(0.00764017643705271,-0.0331951640388586,
0.0798796269924586));
#65565=CARTESIAN_POINT('',(0.0075156193285227,-0.0331951640388587,0.0798691138238489));
#65566=CARTESIAN_POINT('',(0.00757789788279861,-0.0331951640388687,0.0798743704081638));
#65567=CARTESIAN_POINT('',(0.00728116543138446,-0.0335216366567661,0.0798392989013045));
#65568=CARTESIAN_POINT('Origin',(0.0085168111349089,-0.0326434571526396,
0.0632307515618159));
#65569=CARTESIAN_POINT('',(0.00728136446697911,-0.0336938721132327,0.0798379550257279));
#65570=CARTESIAN_POINT('Origin',(0.00568141891782992,-0.0336938867896335,
0.0906406863567228));
#65571=CARTESIAN_POINT('',(0.00734319006510281,-0.0336938721132538,0.0798471117401534));
#65572=CARTESIAN_POINT('Ctrl Pts',(0.00747972886102596,-0.0332451089994432,
0.0798651833133709));
#65573=CARTESIAN_POINT('Ctrl Pts',(0.00769528052629965,-0.0329451141710253,
0.0798894741822098));
#65574=CARTESIAN_POINT('Ctrl Pts',(0.00791204951958449,-0.0326442513127494,
0.0798974598106435));
#65575=CARTESIAN_POINT('Ctrl Pts',(0.00772870617396611,-0.0332451089994432,
0.0798877730818758));
#65576=CARTESIAN_POINT('Ctrl Pts',(0.0079451098262982,-0.0329451141710253,
0.0799026736177233));
#65577=CARTESIAN_POINT('Ctrl Pts',(0.00816202106796723,-0.0326442513127494,
0.0799012314149623));
#65578=CARTESIAN_POINT('',(0.00764006217697776,-0.0330220786163545,0.0798809807141532));
#65579=CARTESIAN_POINT('',(0.0078759255272611,-0.0326943950436594,0.0798960153213506));
#65580=CARTESIAN_POINT('Origin',(0.00852402039608933,-0.0326396682764816,
0.0631072872915801));
#65581=CARTESIAN_POINT('Origin',(0.00671235452142551,-0.0331952026559979,
0.0908721933899018));
#65582=CARTESIAN_POINT('',(0.00776473354558816,-0.0331951640388616,0.0798901401610688));
#65583=CARTESIAN_POINT('',(0.00770245499133134,-0.0331951640388701,0.0798848835767737));
#65584=CARTESIAN_POINT('',(0.00800086794439122,-0.0328677532092643,0.0799000449639514));
#65585=CARTESIAN_POINT('Origin',(0.0080435778561186,-0.0326401908898621,
0.0631284489558804));
#65586=CARTESIAN_POINT('',(0.00800089697811041,-0.0326943950436593,0.0798986867390679));
#65587=CARTESIAN_POINT('Origin',(0.00776458814375024,-0.032694427913436,
0.0909534764247798));
#65588=CARTESIAN_POINT('',(0.00793841125269576,-0.0326943950436694,0.0798973510302193));
#65589=CARTESIAN_POINT('Ctrl Pts',(0.00701277233604355,-0.0335235895815171,
0.0800462409294017));
#65590=CARTESIAN_POINT('Ctrl Pts',(0.00709394570106689,-0.0334144449262748,
0.0800615361674614));
#65591=CARTESIAN_POINT('Ctrl Pts',(0.00717552831255958,-0.0333049234473147,
0.0800751719972648));
#65592=CARTESIAN_POINT('Ctrl Pts',(0.00725741743084065,-0.0331951640388587,
0.0800871215330957));
#65593=CARTESIAN_POINT('Ctrl Pts',(0.00710230374508894,-0.0335235895815171,
0.07997677655522));
#65594=CARTESIAN_POINT('Ctrl Pts',(0.0071825207962389,-0.0334144449262748,
0.079990839217163));
#65595=CARTESIAN_POINT('Ctrl Pts',(0.00726312053107448,-0.0333049234473147,
0.0800032608114941));
#65596=CARTESIAN_POINT('Ctrl Pts',(0.00734400132606785,-0.0331951640388587,
0.0800140161189775));
#65597=CARTESIAN_POINT('Ctrl Pts',(0.00719183515413433,-0.0335235895815171,
0.0799073121810384));
#65598=CARTESIAN_POINT('Ctrl Pts',(0.00727109589141091,-0.0334144449262748,
0.0799201422668647));
#65599=CARTESIAN_POINT('Ctrl Pts',(0.00735071274958938,-0.0333049234473147,
0.0799313496257235));
#65600=CARTESIAN_POINT('Ctrl Pts',(0.00743058522129505,-0.0331951640388587,
0.0799409107048593));
#65601=CARTESIAN_POINT('Ctrl Pts',(0.00728136656317972,-0.0335235895815171,
0.0798378478068567));
#65602=CARTESIAN_POINT('Ctrl Pts',(0.00735967098658292,-0.0334144449262748,
0.0798494453165664));
#65603=CARTESIAN_POINT('Ctrl Pts',(0.00743830496810428,-0.0333049234473147,
0.0798594384399528));
#65604=CARTESIAN_POINT('Ctrl Pts',(0.00751716911652226,-0.0331951640388587,
0.0798678052907411));
#65605=CARTESIAN_POINT('',(0.00738651837969219,-0.0331951640388687,0.0799781176784819));
#65606=CARTESIAN_POINT('Ctrl Pts',(0.0072447376100579,-0.0332121607145959,
0.0800852574131777));
#65607=CARTESIAN_POINT('Ctrl Pts',(0.00725102434571237,-0.0332625444109769,
0.0800428097431533));
#65608=CARTESIAN_POINT('Ctrl Pts',(0.00725720275104595,-0.033313530074687,
0.0800010935130951));
#65609=CARTESIAN_POINT('Ctrl Pts',(0.00726934780540806,-0.0334167203140549,
0.0799190908191178));
#65610=CARTESIAN_POINT('Ctrl Pts',(0.00727530975055819,-0.0334688847587227,
0.0798788361155094));
#65611=CARTESIAN_POINT('Ctrl Pts',(0.00728116543164366,-0.0335216366562291,
0.0798392989006264));
#65612=CARTESIAN_POINT('Ctrl Pts',(0.00738519173768159,-0.0330240426238172,
0.0801043668126164));
#65613=CARTESIAN_POINT('Ctrl Pts',(0.00746721894158385,-0.032914277406352,
0.0801145416157137));
#65614=CARTESIAN_POINT('Ctrl Pts',(0.00754949738064075,-0.0328043479726691,
0.0801230257598851));
#65615=CARTESIAN_POINT('Ctrl Pts',(0.00763192194936942,-0.0326943950436594,
0.0801298054734803));
#65616=CARTESIAN_POINT('Ctrl Pts',(0.00747018466400619,-0.0330240426238172,
0.0800294179069582));
#65617=CARTESIAN_POINT('Ctrl Pts',(0.00755117937371382,-0.032914277406352,
0.0800384218496908));
#65618=CARTESIAN_POINT('Ctrl Pts',(0.00763240059888571,-0.0328043479726691,
0.08004575589432));
#65619=CARTESIAN_POINT('Ctrl Pts',(0.00771374454783255,-0.0326943950436594,
0.0800514077798578));
#65620=CARTESIAN_POINT('Ctrl Pts',(0.00755517759033078,-0.0330240426238172,
0.0799544690012999));
#65621=CARTESIAN_POINT('Ctrl Pts',(0.00763513980584379,-0.032914277406352,
0.0799623020836678));
#65622=CARTESIAN_POINT('Ctrl Pts',(0.00771530381713068,-0.0328043479726691,
0.0799684860287549));
#65623=CARTESIAN_POINT('Ctrl Pts',(0.00779556714629568,-0.0326943950436594,
0.0799730100862353));
#65624=CARTESIAN_POINT('Ctrl Pts',(0.00764017051665538,-0.0330240426238172,
0.0798795200956417));
#65625=CARTESIAN_POINT('Ctrl Pts',(0.00771910023797376,-0.032914277406352,
0.0798861823176449));
#65626=CARTESIAN_POINT('Ctrl Pts',(0.00779820703537564,-0.0328043479726691,
0.0798912161631897));
#65627=CARTESIAN_POINT('Ctrl Pts',(0.00787738974475881,-0.0326943950436594,
0.0798946123926128));
#65628=CARTESIAN_POINT('Ctrl Pts',(0.00761915010025602,-0.0327114338383318,
0.0801287412045299));
#65629=CARTESIAN_POINT('Ctrl Pts',(0.00762276211271095,-0.0327619876830942,
0.0800859470818386));
#65630=CARTESIAN_POINT('Ctrl Pts',(0.00762631040159336,-0.0328131562604278,
0.0800439079383769));
#65631=CARTESIAN_POINT('Ctrl Pts',(0.00763328251806064,-0.0329167375858763,
0.079961304234419));
#65632=CARTESIAN_POINT('Ctrl Pts',(0.00763670356759461,-0.0329691088920606,
0.0799207725875));
#65633=CARTESIAN_POINT('Ctrl Pts',(0.00764006217698454,-0.0330220786163186,
0.079880980714106));
#65634=CARTESIAN_POINT('',(0.00775392373832528,-0.0326943950436694,0.0800129103974254));
#65635=CARTESIAN_POINT('Ctrl Pts',(0.00740380746807937,-0.0336938721132523,
0.079854640159517));
#65636=CARTESIAN_POINT('Ctrl Pts',(0.00743719861993812,-0.0336474569765025,
0.0798588544104961));
#65637=CARTESIAN_POINT('Ctrl Pts',(0.00747063681694241,-0.033601104548885,
0.0798626774871199));
#65638=CARTESIAN_POINT('Ctrl Pts',(0.00755529464382165,-0.0334837508592655,
0.0798723566381497));
#65639=CARTESIAN_POINT('Ctrl Pts',(0.0076402021085357,-0.0333660264659096,
0.0798795229518747));
#65640=CARTESIAN_POINT('Ctrl Pts',(0.00740501566317657,-0.0336938721132523,
0.0798562684545551));
#65641=CARTESIAN_POINT('Ctrl Pts',(0.0074384163459865,-0.0336474569765025,
0.0798604756335674));
#65642=CARTESIAN_POINT('Ctrl Pts',(0.00747186399050261,-0.033601104548885,
0.0798642915271371));
#65643=CARTESIAN_POINT('Ctrl Pts',(0.00755654573630964,-0.0334837508592655,
0.0798739524923255));
#65644=CARTESIAN_POINT('Ctrl Pts',(0.00764147657056388,-0.0333660264659096,
0.0798810999194275));
#65645=CARTESIAN_POINT('Ctrl Pts',(0.00760758874208749,-0.0336938721132523,
0.0801292779544295));
#65646=CARTESIAN_POINT('Ctrl Pts',(0.00764258744009457,-0.0336474569765025,
0.0801322994059899));
#65647=CARTESIAN_POINT('Ctrl Pts',(0.00767761910987388,-0.033601104548885,
0.080134910946569));
#65648=CARTESIAN_POINT('Ctrl Pts',(0.00776631124345654,-0.0334837508592655,
0.0801415227668837));
#65649=CARTESIAN_POINT('Ctrl Pts',(0.00785516035193512,-0.0333660264659096,
0.0801455035519669));
#65650=CARTESIAN_POINT('',(0.00761915009983477,-0.0336769361243754,0.0801287412095221));
#65651=CARTESIAN_POINT('',(0.00760638055271975,-0.0336938721132321,0.0801276496670952));
#65652=CARTESIAN_POINT('Ctrl Pts',(0.00761915009983503,-0.0336769361243751,
0.0801287412095222));
#65653=CARTESIAN_POINT('Ctrl Pts',(0.00761702148825769,-0.0336797586670475,
0.0801285615453289));
#65654=CARTESIAN_POINT('Ctrl Pts',(0.00761489305313471,-0.0336825812713744,
0.0801283807511564));
#65655=CARTESIAN_POINT('Ctrl Pts',(0.00761063654794096,-0.0336882265870973,
0.0801280169044073));
#65656=CARTESIAN_POINT('Ctrl Pts',(0.00760850847778055,-0.0336910492986195,
0.0801278338518592));
#65657=CARTESIAN_POINT('Ctrl Pts',(0.00760638055272642,-0.033693872113238,
0.0801276496671085));
#65658=CARTESIAN_POINT('Ctrl Pts',(0.00761915009983475,-0.0336769361243754,
0.0801287412095221));
#65659=CARTESIAN_POINT('Ctrl Pts',(0.00762267519166302,-0.0336279018525385,
0.0800869768983302));
#65660=CARTESIAN_POINT('Ctrl Pts',(0.00762625099640256,-0.033576782605156,
0.0800446117546109));
#65661=CARTESIAN_POINT('Ctrl Pts',(0.00763325751955493,-0.0334733172106825,
0.0799616004097819));
#65662=CARTESIAN_POINT('Ctrl Pts',(0.00763669294690799,-0.0334209631477589,
0.079920898418453));
#65663=CARTESIAN_POINT('Ctrl Pts',(0.00764006217698056,-0.0333679869844681,
0.0798809807141533));
#65664=CARTESIAN_POINT('',(0.00750569810797312,-0.0336938721132534,0.079991959060837));
#65665=CARTESIAN_POINT('Ctrl Pts',(0.00776342518707949,-0.0331951640388604,
0.0798885905798627));
#65666=CARTESIAN_POINT('Ctrl Pts',(0.00788206687599759,-0.0330306421900773,
0.0798960407304203));
#65667=CARTESIAN_POINT('Ctrl Pts',(0.00800091510898811,-0.0328657861694599,
0.0798985809287791));
#65668=CARTESIAN_POINT('Ctrl Pts',(0.00776473354558501,-0.0331951640388604,
0.0798901401610685));
#65669=CARTESIAN_POINT('Ctrl Pts',(0.00788340727110318,-0.0330306421900773,
0.0798975632621511));
#65670=CARTESIAN_POINT('Ctrl Pts',(0.00800228639533539,-0.0328657861694599,
0.0799000751100419));
#65671=CARTESIAN_POINT('Ctrl Pts',(0.00798274125483999,-0.0331951640388604,
0.0801483420587605));
#65672=CARTESIAN_POINT('Ctrl Pts',(0.0081067531394057,-0.0330306421900773,
0.0801512579899268));
#65673=CARTESIAN_POINT('Ctrl Pts',(0.00823077957518043,-0.0328657861694599,
0.0801490458875051));
#65674=CARTESIAN_POINT('',(0.00798274125482956,-0.0331951640388588,0.0801483420587467));
#65675=CARTESIAN_POINT('',(0.00787373740021886,-0.0331951640388701,0.0800192411099177));
#65676=CARTESIAN_POINT('',(0.0079955541420418,-0.0331781648281943,0.0801486296404161));
#65677=CARTESIAN_POINT('Origin',(0.00763622598507471,-0.0326412091981293,
0.0636302351063101));
#65678=CARTESIAN_POINT('Ctrl Pts',(0.00799555414055663,-0.033178164828644,
0.0801486296393133));
#65679=CARTESIAN_POINT('Ctrl Pts',(0.00799647273296179,-0.033127681151819,
0.0801056564503676));
#65680=CARTESIAN_POINT('Ctrl Pts',(0.00799737470460111,-0.0330765663440246,
0.080063459223434));
#65681=CARTESIAN_POINT('Ctrl Pts',(0.00799914634354069,-0.032973061432112,
0.0799805804403965));
#65682=CARTESIAN_POINT('Ctrl Pts',(0.00800001530045004,-0.0329207133203635,
0.0799399323678051));
#65683=CARTESIAN_POINT('Ctrl Pts',(0.00800086794435749,-0.0328677532092815,
0.0799000449639279));
#65684=CARTESIAN_POINT('Origin',(0.00812378219310841,-0.0315241814719618,
0.07415));
#65685=CARTESIAN_POINT('',(0.00761915009994875,-0.0337108120655531,0.080128741208238));
#65686=CARTESIAN_POINT('',(0.00763192194936942,-0.0336938721132327,0.0801298054734803));
#65687=CARTESIAN_POINT('Origin',(0.0101088601348352,-0.0345562507257751,
0.0639194914324974));
#65688=CARTESIAN_POINT('Ctrl Pts',(0.00763192194936625,-0.0336938721132348,
0.080129805473485));
#65689=CARTESIAN_POINT('Ctrl Pts',(0.00762979326524268,-0.0336910493096957,
0.0801296303816536));
#65690=CARTESIAN_POINT('Ctrl Pts',(0.00762766461530371,-0.0336882265926354,
0.0801294541482935));
#65691=CARTESIAN_POINT('Ctrl Pts',(0.00762340733835879,-0.033682581271277,
0.0801290993943332));
#65692=CARTESIAN_POINT('Ctrl Pts',(0.00762127871137503,-0.0336797586669988,
0.0801289208737123));
#65693=CARTESIAN_POINT('Ctrl Pts',(0.00761915009983449,-0.0336769361243751,
0.0801287412095221));
#65694=CARTESIAN_POINT('Origin',(0.00788156968309789,-0.0345562519616818,
0.0637315024488479));
#65695=CARTESIAN_POINT('Origin',(0.00812378219310841,-0.0315241814719618,
0.07415));
#65696=CARTESIAN_POINT('',(0.00799555414272147,-0.0332121607144207,0.080148629638879));
#65697=CARTESIAN_POINT('Origin',(0.0091049176852243,-0.0326413654380319,
0.0636694742416528));
#65698=CARTESIAN_POINT('',(0.00800836761556968,-0.0331951640388587,0.0801488898535752));
#65699=CARTESIAN_POINT('Origin',(0.00759140414320651,-0.0326413636678921,
0.0636371177732643));
#65700=CARTESIAN_POINT('Origin',(0.00906043161709704,-0.0326412105475495,
0.063660675157574));
#65701=CARTESIAN_POINT('Ctrl Pts',(0.00747965684771335,-0.034243627687391,
0.0798651751976138));
#65702=CARTESIAN_POINT('Ctrl Pts',(0.00769520823370105,-0.0339430054201809,
0.0798894687855002));
#65703=CARTESIAN_POINT('Ctrl Pts',(0.00791197715337794,-0.0336441434784052,
0.0798974571442634));
#65704=CARTESIAN_POINT('Ctrl Pts',(0.00772863387599453,-0.034243627687391,
0.0798877681033205));
#65705=CARTESIAN_POINT('Ctrl Pts',(0.0079450373674681,-0.0339430054201809,
0.0799026713677838));
#65706=CARTESIAN_POINT('Ctrl Pts',(0.00816194865425262,-0.0336441434784052,
0.0799012318959718));
#65707=CARTESIAN_POINT('',(0.00776473354558619,-0.034193496108874,0.0798901401610687));
#65708=CARTESIAN_POINT('',(0.00800086794805514,-0.0338664212895224,0.0799000449648617));
#65709=CARTESIAN_POINT('Origin',(0.00931760079658415,-0.0345610818075694,
0.0632275564000169));
#65710=CARTESIAN_POINT('',(0.00800089697811059,-0.0336938721132326,0.0798986867390679));
#65711=CARTESIAN_POINT('Origin',(0.00776658026320743,-0.0336938005044392,
0.0908637967520959));
#65712=CARTESIAN_POINT('',(0.00787592552726112,-0.0336938721132327,0.0798960153213506));
#65713=CARTESIAN_POINT('',(0.00793841125269586,-0.0336938721132427,0.0798973510302193));
#65714=CARTESIAN_POINT('',(0.00764006217697529,-0.0340203938281606,0.0798809807141529));
#65715=CARTESIAN_POINT('Origin',(0.00978408309822432,-0.0345589643244979,
0.0633455303789544));
#65716=CARTESIAN_POINT('',(0.00764017643705448,-0.034193496108874,0.0798796269924588));
#65717=CARTESIAN_POINT('Origin',(0.00671338119780292,-0.0341934220717617,
0.0908600308491757));
#65718=CARTESIAN_POINT('',(0.00770245499133034,-0.0341934961088841,0.0798848835767737));
#65719=CARTESIAN_POINT('Ctrl Pts',(0.00783983827644646,-0.0337436976235975,
0.0798943451195232));
#65720=CARTESIAN_POINT('Ctrl Pts',(0.00789150378703078,-0.0336723290703325,
0.0798968989541427));
#65721=CARTESIAN_POINT('Ctrl Pts',(0.00794320687478813,-0.033601104548885,
0.0798985230759225));
#65722=CARTESIAN_POINT('Ctrl Pts',(0.0081082845921927,-0.0333736987606857,
0.0799037085750454));
#65723=CARTESIAN_POINT('Ctrl Pts',(0.00827338784841755,-0.0331450831799192,
0.0798994124176215));
#65724=CARTESIAN_POINT('Ctrl Pts',(0.00808974268779718,-0.0337436976235975,
0.0799012578026096));
#65725=CARTESIAN_POINT('Ctrl Pts',(0.00814147037210082,-0.0336723290703325,
0.0799015639590792));
#65726=CARTESIAN_POINT('Ctrl Pts',(0.00819319519487387,-0.033601104548885,
0.0799009396480215));
#65727=CARTESIAN_POINT('Ctrl Pts',(0.00835834230787811,-0.0333736987606857,
0.0798989463464833));
#65728=CARTESIAN_POINT('Ctrl Pts',(0.00852310288436963,-0.0331450831799192,
0.0798874792361743));
#65729=CARTESIAN_POINT('Ctrl Pts',(0.00809224173191068,-0.0337436976235975,
0.0799013269294405));
#65730=CARTESIAN_POINT('Ctrl Pts',(0.00814397003795152,-0.0336723290703325,
0.0799016106091286));
#65731=CARTESIAN_POINT('Ctrl Pts',(0.00819569507807473,-0.033601104548885,
0.0799009638137425));
#65732=CARTESIAN_POINT('Ctrl Pts',(0.00836084288503496,-0.0333736987606857,
0.0798988987241977));
#65733=CARTESIAN_POINT('Ctrl Pts',(0.00852560003472915,-0.0331450831799192,
0.0798873599043598));
#65734=CARTESIAN_POINT('',(0.00800086794424164,-0.0335216366567656,0.07990004496356));
#65735=CARTESIAN_POINT('',(0.00823720990302466,-0.0331951640388587,0.0799002399214836));
#65736=CARTESIAN_POINT('Origin',(0.00714516726941353,-0.0326434571526036,
0.063267593509416));
#65737=CARTESIAN_POINT('Origin',(0.00776750895290892,-0.0336938867896287,
0.0908167616606058));
#65738=CARTESIAN_POINT('',(0.00812586842897576,-0.0336938721132548,0.0799013581567853));
#65739=CARTESIAN_POINT('',(0.00806338270355318,-0.0336938721132536,0.0799000224479366));
#65740=CARTESIAN_POINT('',(0.00836215880828412,-0.0333679869984219,0.079896416412814));
#65741=CARTESIAN_POINT('Ctrl Pts',(0.00812586842898595,-0.0336938721132649,
0.0799013581567863));
#65742=CARTESIAN_POINT('Ctrl Pts',(0.00814831867788204,-0.0336629187933933,
0.0799013500132285));
#65743=CARTESIAN_POINT('Ctrl Pts',(0.00817076169896996,-0.0336319952301041,
0.0799012104170416));
#65744=CARTESIAN_POINT('Ctrl Pts',(0.00819319519488396,-0.0336011045488951,
0.0799009396480218));
#65745=CARTESIAN_POINT('Ctrl Pts',(0.00824948851244248,-0.0335235892595455,
0.079900260195899));
#65746=CARTESIAN_POINT('Ctrl Pts',(0.00830582187881451,-0.033445866867327,
0.0798987534184142));
#65747=CARTESIAN_POINT('Ctrl Pts',(0.00836215880829256,-0.0333679869984152,
0.0798964164132425));
#65748=CARTESIAN_POINT('',(0.00836210249096915,-0.0331951640388588,0.0798950590454431));
#65749=CARTESIAN_POINT('Ctrl Pts',(0.00836220326593144,-0.0333679692463177,
0.0798964152568053));
#65750=CARTESIAN_POINT('Ctrl Pts',(0.00836217855921108,-0.0333391895390484,
0.0798959626782118));
#65751=CARTESIAN_POINT('Ctrl Pts',(0.00836215679795873,-0.0333104081088491,
0.0798956236254674));
#65752=CARTESIAN_POINT('Ctrl Pts',(0.00836212246616085,-0.03325326985216,
0.0798951751861306));
#65753=CARTESIAN_POINT('Ctrl Pts',(0.00836210976142365,-0.0332249172665086,
0.0798950624471958));
#65754=CARTESIAN_POINT('Ctrl Pts',(0.00836210271505692,-0.0331960985307702,
0.0798950590659285));
#65755=CARTESIAN_POINT('Ctrl Pts',(0.00836210260212061,-0.033195631261781,
0.0798950590408323));
#65756=CARTESIAN_POINT('Ctrl Pts',(0.00836210249096896,-0.0331951640388603,
0.0798950590454432));
#65757=CARTESIAN_POINT('',(0.00829965619700691,-0.0331951640388688,0.0798976494834734));
#65758=CARTESIAN_POINT('Ctrl Pts',(0.00738518997603143,-0.0340223579322397,
0.0801043665940979));
#65759=CARTESIAN_POINT('Ctrl Pts',(0.00746731622100408,-0.0339125849573575,
0.0801145537071008));
#65760=CARTESIAN_POINT('Ctrl Pts',(0.00754959560638283,-0.0338030433565231,
0.0801230338393014));
#65761=CARTESIAN_POINT('Ctrl Pts',(0.00763192194936947,-0.0336938721132327,
0.0801298054734804));
#65762=CARTESIAN_POINT('Ctrl Pts',(0.00747018306963347,-0.0340223579322397,
0.08002941758563));
#65763=CARTESIAN_POINT('Ctrl Pts',(0.00755127557230412,-0.0339125849573575,
0.0800384324222008));
#65764=CARTESIAN_POINT('Ctrl Pts',(0.00763249767838148,-0.0338030433565231,
0.080045762497778));
#65765=CARTESIAN_POINT('Ctrl Pts',(0.00771374468752323,-0.0336938721132327,
0.0800514076460144));
#65766=CARTESIAN_POINT('Ctrl Pts',(0.00755517616323551,-0.0340223579322397,
0.0799544685771621));
#65767=CARTESIAN_POINT('Ctrl Pts',(0.00763523492360417,-0.0339125849573575,
0.0799623111373008));
#65768=CARTESIAN_POINT('Ctrl Pts',(0.00771539975038013,-0.0338030433565231,
0.0799684911562546));
#65769=CARTESIAN_POINT('Ctrl Pts',(0.00779556742567699,-0.0336938721132327,
0.0799730098185483));
#65770=CARTESIAN_POINT('Ctrl Pts',(0.00764016925683755,-0.0340223579322397,
0.0798795195686942));
#65771=CARTESIAN_POINT('Ctrl Pts',(0.00771919427490421,-0.0339125849573575,
0.0798861898524009));
#65772=CARTESIAN_POINT('Ctrl Pts',(0.00779830182237878,-0.0338030433565231,
0.0798912198147312));
#65773=CARTESIAN_POINT('Ctrl Pts',(0.00787739016383075,-0.0336938721132327,
0.0798946119910823));
#65774=CARTESIAN_POINT('',(0.00775392373832528,-0.0336938721132427,0.0800129103974254));
#65775=CARTESIAN_POINT('Ctrl Pts',(0.00761915010024686,-0.0337108120662688,
0.0801287412046396));
#65776=CARTESIAN_POINT('Ctrl Pts',(0.00762276656768743,-0.0337611408994229,
0.0800858943005123));
#65777=CARTESIAN_POINT('Ctrl Pts',(0.00762631704262065,-0.0338121088781167,
0.080043829257326));
#65778=CARTESIAN_POINT('Ctrl Pts',(0.00763328924190049,-0.0339153382773235,
0.0799612245722275));
#65779=CARTESIAN_POINT('Ctrl Pts',(0.00763670801657843,-0.0339675558473111,
0.0799207198771726));
#65780=CARTESIAN_POINT('Ctrl Pts',(0.00764006217698382,-0.0340203938281305,
0.0798809807141136));
#65781=CARTESIAN_POINT('Ctrl Pts',(0.0077605279221661,-0.0335235895815172,
0.0801389937664584));
#65782=CARTESIAN_POINT('Ctrl Pts',(0.00784297821260505,-0.0334144449262748,
0.0801439946766798));
#65783=CARTESIAN_POINT('Ctrl Pts',(0.00792562654348016,-0.0333049234473147,
0.0801472979713915));
#65784=CARTESIAN_POINT('Ctrl Pts',(0.00800836761556974,-0.0331951640388588,
0.0801488898535752));
#65785=CARTESIAN_POINT('Ctrl Pts',(0.00784064715467543,-0.0335235895815172,
0.0800588558786143));
#65786=CARTESIAN_POINT('Ctrl Pts',(0.00792199418931122,-0.0334144449262748,
0.0800627537898599));
#65787=CARTESIAN_POINT('Ctrl Pts',(0.00800351520974718,-0.0333049234473147,
0.0800649756108182));
#65788=CARTESIAN_POINT('Ctrl Pts',(0.00808510623297895,-0.0331951640388588,
0.0800655090579198));
#65789=CARTESIAN_POINT('Ctrl Pts',(0.00792076638718476,-0.0335235895815172,
0.0799787179907701));
#65790=CARTESIAN_POINT('Ctrl Pts',(0.00800101016601739,-0.0334144449262748,
0.07998151290304));
#65791=CARTESIAN_POINT('Ctrl Pts',(0.0080814038760142,-0.0333049234473147,
0.079982653250245));
#65792=CARTESIAN_POINT('Ctrl Pts',(0.00816184485038816,-0.0331951640388588,
0.0799821282622644));
#65793=CARTESIAN_POINT('Ctrl Pts',(0.00800088561969408,-0.0335235895815172,
0.0798985801029259));
#65794=CARTESIAN_POINT('Ctrl Pts',(0.00808002614272356,-0.0334144449262748,
0.0799002720162201));
#65795=CARTESIAN_POINT('Ctrl Pts',(0.00815929254228122,-0.0333049234473147,
0.0799003308896717));
#65796=CARTESIAN_POINT('Ctrl Pts',(0.00823858346779737,-0.0331951640388588,
0.0798987474666089));
#65797=CARTESIAN_POINT('Ctrl Pts',(0.00799555414278324,-0.0332121607145974,
0.080148629635739));
#65798=CARTESIAN_POINT('Ctrl Pts',(0.00799647120190776,-0.0332625444109692,
0.080105728741371));
#65799=CARTESIAN_POINT('Ctrl Pts',(0.00799737245866444,-0.033313530074669,
0.080063567096736));
#65800=CARTESIAN_POINT('Ctrl Pts',(0.00799914408284852,-0.0334167203140551,
0.0799806888395441));
#65801=CARTESIAN_POINT('Ctrl Pts',(0.00800001376411097,-0.033468884758723,
0.0799400043264331));
#65802=CARTESIAN_POINT('Ctrl Pts',(0.00800086794441465,-0.0335216366562283,
0.0799000449628543));
#65803=CARTESIAN_POINT('',(0.00812278875930717,-0.0331951640388687,0.0800245648875394));
#65804=CARTESIAN_POINT('Ctrl Pts',(0.00776342512837748,-0.0341934961088741,
0.0798885905103364));
#65805=CARTESIAN_POINT('Ctrl Pts',(0.0078425568931179,-0.0340836138583034,
0.0798935596208554));
#65806=CARTESIAN_POINT('Ctrl Pts',(0.00792175351426542,-0.0339738896647349,
0.0798968888812743));
#65807=CARTESIAN_POINT('Ctrl Pts',(0.00800091334428685,-0.033864463329982,
0.0798985808253354));
#65808=CARTESIAN_POINT('Ctrl Pts',(0.00783653050386538,-0.0341934961088741,
0.0799751743598111));
#65809=CARTESIAN_POINT('Ctrl Pts',(0.00791685620861504,-0.0340836138583034,
0.0799791353904951));
#65810=CARTESIAN_POINT('Ctrl Pts',(0.00799722533680004,-0.0339738896647349,
0.0799814323486915));
#65811=CARTESIAN_POINT('Ctrl Pts',(0.00807753482879076,-0.033864463329982,
0.0799820691899589));
#65812=CARTESIAN_POINT('Ctrl Pts',(0.00790963587935328,-0.0341934961088741,
0.0800617582092858));
#65813=CARTESIAN_POINT('Ctrl Pts',(0.00799115552411218,-0.0340836138583034,
0.0800647111601349));
#65814=CARTESIAN_POINT('Ctrl Pts',(0.00807269715933465,-0.0339738896647349,
0.0800659758161088));
#65815=CARTESIAN_POINT('Ctrl Pts',(0.00815415631329468,-0.033864463329982,
0.0800655575545823));
#65816=CARTESIAN_POINT('Ctrl Pts',(0.00798274125484118,-0.0341934961088741,
0.0801483420587605));
#65817=CARTESIAN_POINT('Ctrl Pts',(0.00806545483960932,-0.0340836138583034,
0.0801502869297746));
#65818=CARTESIAN_POINT('Ctrl Pts',(0.00814816898186926,-0.0339738896647349,
0.080150519283526));
#65819=CARTESIAN_POINT('Ctrl Pts',(0.0082307777977986,-0.033864463329982,
0.0801490459192057));
#65820=CARTESIAN_POINT('',(0.00799555414272003,-0.0341764758832475,0.0801486296389534));
#65821=CARTESIAN_POINT('',(0.00798274125482951,-0.034193496108874,0.0801483420587467));
#65822=CARTESIAN_POINT('Origin',(0.008861397458876,-0.0345621026442791,
0.0636056055471864));
#65823=CARTESIAN_POINT('Ctrl Pts',(0.00799555414278307,-0.0341764758830276,
0.0801486296357497));
#65824=CARTESIAN_POINT('Ctrl Pts',(0.00799647149735682,-0.0341260048548319,
0.0801057149199867));
#65825=CARTESIAN_POINT('Ctrl Pts',(0.00799737289797397,-0.034074927129329,
0.0800635465454208));
#65826=CARTESIAN_POINT('Ctrl Pts',(0.00799914452350784,-0.033971543442925,
0.0799806682250842));
#65827=CARTESIAN_POINT('Ctrl Pts',(0.00800001405517191,-0.0339192781035257,
0.0799399907103279));
#65828=CARTESIAN_POINT('Ctrl Pts',(0.00800086794432318,-0.0338664212877424,
0.0799000449671372));
#65829=CARTESIAN_POINT('',(0.00787373740021786,-0.0341934961088841,0.0800192411099177));
#65830=CARTESIAN_POINT('Ctrl Pts',(0.00812586842894504,-0.033693872113253,
0.0799013581567852));
#65831=CARTESIAN_POINT('Ctrl Pts',(0.00815953303674479,-0.0336474569765028,
0.0799013459453546));
#65832=CARTESIAN_POINT('Ctrl Pts',(0.00819319519487387,-0.033601104548885,
0.0799009396480215));
#65833=CARTESIAN_POINT('Ctrl Pts',(0.0082784200398284,-0.0334837508592655,
0.0798999109965879));
#65834=CARTESIAN_POINT('Ctrl Pts',(0.00836357697923725,-0.0333660264659097,
0.0798963574080059));
#65835=CARTESIAN_POINT('Ctrl Pts',(0.00836106132202396,-0.033693872113253,
0.0801468257561836));
#65836=CARTESIAN_POINT('Ctrl Pts',(0.00839616273313799,-0.0336474569765028,
0.0801454368827042));
#65837=CARTESIAN_POINT('Ctrl Pts',(0.00843124548056321,-0.033601104548885,
0.0801436371980553));
#65838=CARTESIAN_POINT('Ctrl Pts',(0.00852006693100108,-0.0334837508592655,
0.0801390808102985));
#65839=CARTESIAN_POINT('Ctrl Pts',(0.00860871436238776,-0.0333660264659097,
0.0801318944596376));
#65840=CARTESIAN_POINT('',(0.00835965858108673,-0.0336938721132327,0.0801453617346741));
#65841=CARTESIAN_POINT('',(0.00824276350504124,-0.0336938721132538,0.0800233599457397));
#65842=CARTESIAN_POINT('',(0.00837246424305004,-0.0336769361243754,0.0801448442213319));
#65843=CARTESIAN_POINT('Ctrl Pts',(0.0083724642430503,-0.0336769361243751,
0.0801448442213319));
#65844=CARTESIAN_POINT('Ctrl Pts',(0.00837032989836826,-0.0336797586669794,
0.0801449327596143));
#65845=CARTESIAN_POINT('Ctrl Pts',(0.00836819558712512,-0.0336825812712383,
0.0801450201547123));
#65846=CARTESIAN_POINT('Ctrl Pts',(0.00836392704416631,-0.0336882265862871,
0.0801451926585425));
#65847=CARTESIAN_POINT('Ctrl Pts',(0.00836179281252015,-0.0336910492969991,
0.0801452777673101));
#65848=CARTESIAN_POINT('Ctrl Pts',(0.00835965858109482,-0.0336938721132384,
0.0801453617346872));
#65849=CARTESIAN_POINT('Ctrl Pts',(0.00837246424305002,-0.0336769361243754,
0.0801448442213319));
#65850=CARTESIAN_POINT('Ctrl Pts',(0.00837072712806767,-0.0336279031442069,
0.0801029685261757));
#65851=CARTESIAN_POINT('Ctrl Pts',(0.00836896502031064,-0.0335767852183815,
0.0800604903436776));
#65852=CARTESIAN_POINT('Ctrl Pts',(0.00836551221211579,-0.0334733199151731,
0.0799772553564356));
#65853=CARTESIAN_POINT('Ctrl Pts',(0.00836381919334894,-0.0334209645163069,
0.0799364426649829));
#65854=CARTESIAN_POINT('Ctrl Pts',(0.00836215879818742,-0.0333679869844682,
0.0798964164132224));
#65855=CARTESIAN_POINT('Origin',(0.00812378219310841,-0.0315241814719618,
0.07415));
#65856=CARTESIAN_POINT('',(0.00799555414271336,-0.0342105180190348,0.0801486296392591));
#65857=CARTESIAN_POINT('',(0.00800836761556967,-0.034193496108874,0.0801488898535753));
#65858=CARTESIAN_POINT('Origin',(0.0088164943374163,-0.0345621696908114,
0.0635994077056605));
#65859=CARTESIAN_POINT('Origin',(0.00783743114609163,-0.0345621044702029,
0.0635837134576787));
#65860=CARTESIAN_POINT('Origin',(0.00788255835472517,-0.0345621711986352,
0.0635794480198904));
#65861=CARTESIAN_POINT('Origin',(0.00812378219310841,-0.0315241814719618,
0.07415));
#65862=CARTESIAN_POINT('',(0.00837246424300171,-0.0337108120655824,0.0801448442200445));
#65863=CARTESIAN_POINT('Origin',(0.00657769573536795,-0.0345562518668543,
0.0638440125869785));
#65864=CARTESIAN_POINT('',(0.00838526877037957,-0.0336938721132327,0.0801442993560502));
#65865=CARTESIAN_POINT('Origin',(0.00881098448054971,-0.0345562507319043,
0.0637513655757208));
#65866=CARTESIAN_POINT('Ctrl Pts',(0.00838526877037628,-0.0336938721132354,
0.0801442993560566));
#65867=CARTESIAN_POINT('Ctrl Pts',(0.00838313492427463,-0.0336910493064383,
0.0801443924398485));
#65868=CARTESIAN_POINT('Ctrl Pts',(0.00838100097271145,-0.0336882265910066,
0.0801444843866646));
#65869=CARTESIAN_POINT('Ctrl Pts',(0.0083767328044364,-0.0336825812712758,
0.0801446660082786));
#65870=CARTESIAN_POINT('Ctrl Pts',(0.00837459858774597,-0.0336797586669982,
0.0801447556830489));
#65871=CARTESIAN_POINT('Ctrl Pts',(0.00837246424304975,-0.0336769361243751,
0.0801448442213319));
#65872=CARTESIAN_POINT('Ctrl Pts',(0.00787442585994672,-0.0346945769586966,
0.0798959832641261));
#65873=CARTESIAN_POINT('Ctrl Pts',(0.00799477778035788,-0.0345275153357699,
0.0799012061323774));
#65874=CARTESIAN_POINT('Ctrl Pts',(0.00811532508433994,-0.0343603235954687,
0.0799026453943974));
#65875=CARTESIAN_POINT('Ctrl Pts',(0.00823571118321104,-0.0341934961073027,
0.0799003020923843));
#65876=CARTESIAN_POINT('Ctrl Pts',(0.00795824004961583,-0.0346945769586966,
0.0798977748950125));
#65877=CARTESIAN_POINT('Ctrl Pts',(0.00807862949645335,-0.0345275153357699,
0.0799012422414983));
#65878=CARTESIAN_POINT('Ctrl Pts',(0.00819915912702418,-0.0343603235954687,
0.0799009243475134));
#65879=CARTESIAN_POINT('Ctrl Pts',(0.00831947248215584,-0.0341934961073027,
0.0798968274513665));
#65880=CARTESIAN_POINT('Ctrl Pts',(0.00804205423928495,-0.0346945769586966,
0.0798995665258989));
#65881=CARTESIAN_POINT('Ctrl Pts',(0.00816248121254882,-0.0345275153357699,
0.0799012783506192));
#65882=CARTESIAN_POINT('Ctrl Pts',(0.00828299316970842,-0.0343603235954687,
0.0798992033006293));
#65883=CARTESIAN_POINT('Ctrl Pts',(0.00840323378110064,-0.0341934961073027,
0.0798933528103488));
#65884=CARTESIAN_POINT('Ctrl Pts',(0.00812586842895406,-0.0346945769586966,
0.0799013581567853));
#65885=CARTESIAN_POINT('Ctrl Pts',(0.00824633292864429,-0.0345275153357699,
0.0799013144597401));
#65886=CARTESIAN_POINT('Ctrl Pts',(0.00836682721239266,-0.0343603235954687,
0.0798974822537453));
#65887=CARTESIAN_POINT('Ctrl Pts',(0.00848699508004543,-0.0341934961073027,
0.079889878169331));
#65888=CARTESIAN_POINT('',(0.00812586842896553,-0.0346945769586966,0.0799013581567853));
#65889=CARTESIAN_POINT('',(0.00836215879841123,-0.0343667727831679,0.0798964164132529));
#65890=CARTESIAN_POINT('Origin',(0.00793680313391798,-0.0345626457064672,
0.0630888181481351));
#65891=CARTESIAN_POINT('',(0.00836210249096924,-0.0341934961088739,0.0798950590454431));
#65892=CARTESIAN_POINT('Origin',(0.00882024320446819,-0.0341934771029012,
0.0909390978419296));
#65893=CARTESIAN_POINT('',(0.00823720990226415,-0.0341934961076211,0.079900239921759));
#65894=CARTESIAN_POINT('',(0.00829965619643977,-0.034193496108098,0.0798976494834846));
#65895=CARTESIAN_POINT('',(0.00800086794439598,-0.0345211942962625,0.0799000449639508));
#65896=CARTESIAN_POINT('Origin',(0.00841742866201907,-0.0345625558918781,
0.0631024169485933));
#65897=CARTESIAN_POINT('',(0.00800089697811051,-0.0346945769586885,0.0798986867390679));
#65898=CARTESIAN_POINT('Origin',(0.00776445294209699,-0.0346945685854053,
0.0909597269016649));
#65899=CARTESIAN_POINT('',(0.00806338270354802,-0.0346945769587026,0.0799000224479366));
#65900=CARTESIAN_POINT('Ctrl Pts',(0.00819853890223646,-0.034243627687391,
0.079900927549921));
#65901=CARTESIAN_POINT('Ctrl Pts',(0.00841543871042038,-0.033943005420181,
0.0798981080541562));
#65902=CARTESIAN_POINT('Ctrl Pts',(0.00863150995301438,-0.0336441434784053,
0.0798789587860116));
#65903=CARTESIAN_POINT('Ctrl Pts',(0.00820103735635621,-0.034243627687391,
0.0799008396464996));
#65904=CARTESIAN_POINT('Ctrl Pts',(0.00841793384920793,-0.033943005420181,
0.0798979259199843));
#65905=CARTESIAN_POINT('Ctrl Pts',(0.00863399468804203,-0.0336441434784053,
0.0798786829385132));
#65906=CARTESIAN_POINT('Ctrl Pts',(0.00845088276833138,-0.034243627687391,
0.079892049304359));
#65907=CARTESIAN_POINT('Ctrl Pts',(0.00866744772796387,-0.033943005420181,
0.0798797125027897));
#65908=CARTESIAN_POINT('Ctrl Pts',(0.00888246819080694,-0.0336441434784053,
0.0798510981886735));
#65909=CARTESIAN_POINT('',(0.00836215879818212,-0.0340203938281605,0.0798964164132226));
#65910=CARTESIAN_POINT('',(0.00859804663143739,-0.0336938721132327,0.0798817709516813));
#65911=CARTESIAN_POINT('Origin',(0.00841683201496112,-0.0345589643243666,
0.0632226359681015));
#65912=CARTESIAN_POINT('Origin',(0.00881882493712156,-0.0341934220717763,
0.0909050373789402));
#65913=CARTESIAN_POINT('',(0.00848699507891361,-0.0341934961088741,0.0798898781694027));
#65914=CARTESIAN_POINT('',(0.00842454878495143,-0.0341934961088841,0.079892468607433));
#65915=CARTESIAN_POINT('',(0.00872250889090621,-0.0338664212874645,0.0798701093824915));
#65916=CARTESIAN_POINT('Origin',(0.0079392327225337,-0.0345610751537147,
0.0631640572814627));
#65917=CARTESIAN_POINT('',(0.0087223674624904,-0.0336938721132328,0.0798687582284338));
#65918=CARTESIAN_POINT('Origin',(0.00986416572584789,-0.0336938005063908,
0.09077677479047));
#65919=CARTESIAN_POINT('',(0.0086602070469739,-0.0336938721132427,0.0798752645900675));
#65920=CARTESIAN_POINT('Ctrl Pts',(0.00776052615137487,-0.0345231616327895,
0.0801389936590533));
#65921=CARTESIAN_POINT('Ctrl Pts',(0.00784307599736326,-0.0344132092794018,
0.0801440006321788));
#65922=CARTESIAN_POINT('Ctrl Pts',(0.007925725149449,-0.0343032738552988,
0.0801472998685129));
#65923=CARTESIAN_POINT('Ctrl Pts',(0.00800836761624737,-0.0341934961079738,
0.0801488898535884));
#65924=CARTESIAN_POINT('Ctrl Pts',(0.00784064529399383,-0.0345231616327895,
0.0800588559085098));
#65925=CARTESIAN_POINT('Ctrl Pts',(0.00792209055391287,-0.0344132092794018,
0.08006275855205));
#65926=CARTESIAN_POINT('Ctrl Pts',(0.00800361233473437,-0.0343032738552988,
0.0800649763632687));
#65927=CARTESIAN_POINT('Ctrl Pts',(0.00808510612485482,-0.0341934961079738,
0.0800655091761332));
#65928=CARTESIAN_POINT('Ctrl Pts',(0.00792076443661279,-0.0345231616327895,
0.0799787181579662));
#65929=CARTESIAN_POINT('Ctrl Pts',(0.00800110511046248,-0.0344132092794018,
0.0799815164719211));
#65930=CARTESIAN_POINT('Ctrl Pts',(0.00808149952001974,-0.0343032738552988,
0.0799826528580245));
#65931=CARTESIAN_POINT('Ctrl Pts',(0.00816184463346228,-0.0341934961079738,
0.079982128498678));
#65932=CARTESIAN_POINT('Ctrl Pts',(0.00800088357923175,-0.0345231616327895,
0.0798985804074227));
#65933=CARTESIAN_POINT('Ctrl Pts',(0.00808011966701209,-0.0344132092794018,
0.0799002743917923));
#65934=CARTESIAN_POINT('Ctrl Pts',(0.00815938670530511,-0.0343032738552988,
0.0799003293527803));
#65935=CARTESIAN_POINT('Ctrl Pts',(0.00823858314206973,-0.0341934961079738,
0.0798987478212229));
#65936=CARTESIAN_POINT('',(0.00812278875873998,-0.034193496108098,0.0800245648875506));
#65937=CARTESIAN_POINT('Ctrl Pts',(0.00799555414278203,-0.0342105180195385,
0.0801486296357966));
#65938=CARTESIAN_POINT('Ctrl Pts',(0.00799647252560746,-0.0342610556241125,
0.0801056668174451));
#65939=CARTESIAN_POINT('Ctrl Pts',(0.00799737442852795,-0.0343122189869793,
0.0800634749446548));
#65940=CARTESIAN_POINT('Ctrl Pts',(0.00799914606515046,-0.0344158119695101,
0.0799805961055804));
#65941=CARTESIAN_POINT('Ctrl Pts',(0.00800001507423936,-0.034468199044999,
0.0799399430373854));
#65942=CARTESIAN_POINT('Ctrl Pts',(0.00800086794439187,-0.0345211942962383,
0.0799000449639186));
#65943=CARTESIAN_POINT('Ctrl Pts',(0.00813729401533547,-0.0340223579322397,
0.0801499847858721));
#65944=CARTESIAN_POINT('Ctrl Pts',(0.00822004945414989,-0.0339125849573575,
0.0801497984226033));
#65945=CARTESIAN_POINT('Ctrl Pts',(0.008302742884389,-0.0338030433565231,
0.0801478993450034));
#65946=CARTESIAN_POINT('Ctrl Pts',(0.00838526877037963,-0.0336938721132327,
0.0801442993560502));
#65947=CARTESIAN_POINT('Ctrl Pts',(0.00821222331142454,-0.0340223579322397,
0.0800649743134704));
#65948=CARTESIAN_POINT('Ctrl Pts',(0.00829380623410792,-0.0339125849573575,
0.0800637544797847));
#65949=CARTESIAN_POINT('Ctrl Pts',(0.00837530658169332,-0.0338030433565231,
0.080060846926335));
#65950=CARTESIAN_POINT('Ctrl Pts',(0.00845662045858306,-0.0336938721132327,
0.0800562646105182));
#65951=CARTESIAN_POINT('Ctrl Pts',(0.00828715260751361,-0.0340223579322397,
0.0799799638410686));
#65952=CARTESIAN_POINT('Ctrl Pts',(0.00836756301406595,-0.0339125849573575,
0.0799777105369661));
#65953=CARTESIAN_POINT('Ctrl Pts',(0.00844787027899764,-0.0338030433565231,
0.0799737945076665));
#65954=CARTESIAN_POINT('Ctrl Pts',(0.00852797214678649,-0.0336938721132327,
0.0799682298649861));
#65955=CARTESIAN_POINT('Ctrl Pts',(0.00836208190360268,-0.0340223579322397,
0.0798949533686669));
#65956=CARTESIAN_POINT('Ctrl Pts',(0.00844131979402398,-0.0339125849573575,
0.0798916665941474));
#65957=CARTESIAN_POINT('Ctrl Pts',(0.00852043397630197,-0.0338030433565231,
0.0798867420889981));
#65958=CARTESIAN_POINT('Ctrl Pts',(0.00859932383498993,-0.0336938721132327,
0.0798801951194541));
#65959=CARTESIAN_POINT('Ctrl Pts',(0.00837246424284696,-0.0337108120662689,
0.080144844216436));
#65960=CARTESIAN_POINT('Ctrl Pts',(0.00837068205231926,-0.0337611408994186,
0.0801018819093909));
#65961=CARTESIAN_POINT('Ctrl Pts',(0.00836893238281478,-0.0338121088781076,
0.0800597035691341));
#65962=CARTESIAN_POINT('Ctrl Pts',(0.00836549649192956,-0.0339153382773238,
0.079976876398362));
#65963=CARTESIAN_POINT('Ctrl Pts',(0.00836381172414221,-0.0339675558473122,
0.0799362626088399));
#65964=CARTESIAN_POINT('Ctrl Pts',(0.00836215879818578,-0.0340203938281304,
0.0798964164131825));
#65965=CARTESIAN_POINT('',(0.00849165770091848,-0.0336938721132427,0.0800130351538757));
#65966=CARTESIAN_POINT('Ctrl Pts',(0.00812446563227316,-0.0346945769586931,
0.079899894077111));
#65967=CARTESIAN_POINT('Ctrl Pts',(0.00820370207897374,-0.034584662917547,
0.0798998846589738));
#65968=CARTESIAN_POINT('Ctrl Pts',(0.00828295186469101,-0.0344746925049099,
0.0798982366620499));
#65969=CARTESIAN_POINT('Ctrl Pts',(0.00836211345418758,-0.034364806625142,
0.0798949526173048));
#65970=CARTESIAN_POINT('Ctrl Pts',(0.00820286328188074,-0.0346945769586931,
0.0799817166296364));
#65971=CARTESIAN_POINT('Ctrl Pts',(0.00828322728471282,-0.034584662917547,
0.0799806268522611));
#65972=CARTESIAN_POINT('Ctrl Pts',(0.00836358247776556,-0.0344746925049099,
0.0799778749941733));
#65973=CARTESIAN_POINT('Ctrl Pts',(0.00844382591526756,-0.034364806625142,
0.0799734650065821));
#65974=CARTESIAN_POINT('Ctrl Pts',(0.00828126093148832,-0.0346945769586931,
0.0800635391821619));
#65975=CARTESIAN_POINT('Ctrl Pts',(0.00836275249045189,-0.034584662917547,
0.0800613690455484));
#65976=CARTESIAN_POINT('Ctrl Pts',(0.0084442130908401,-0.0344746925049099,
0.0800575133262967));
#65977=CARTESIAN_POINT('Ctrl Pts',(0.00852553837634755,-0.034364806625142,
0.0800519773958594));
#65978=CARTESIAN_POINT('Ctrl Pts',(0.0083596585810959,-0.0346945769586931,
0.0801453617346874));
#65979=CARTESIAN_POINT('Ctrl Pts',(0.00844227769619097,-0.034584662917547,
0.0801421112388358));
#65980=CARTESIAN_POINT('Ctrl Pts',(0.00852484370391465,-0.0344746925049099,
0.0801371516584202));
#65981=CARTESIAN_POINT('Ctrl Pts',(0.00860725083742753,-0.034364806625142,
0.0801304897851367));
#65982=CARTESIAN_POINT('',(0.00837246424298863,-0.0346775396663494,0.0801448442197254));
#65983=CARTESIAN_POINT('',(0.00835965858108672,-0.0346945769586886,0.0801453617346741));
#65984=CARTESIAN_POINT('Origin',(0.00753182116752839,-0.0345626618000782,
0.0635645479677025));
#65985=CARTESIAN_POINT('Ctrl Pts',(0.00837246424284332,-0.0346775396659518,
0.0801448442163483));
#65986=CARTESIAN_POINT('Ctrl Pts',(0.0083706837491285,-0.0346269748529746,
0.0801019228134568));
#65987=CARTESIAN_POINT('Ctrl Pts',(0.00836893491328795,-0.0345757904818327,
0.0800597645698871));
#65988=CARTESIAN_POINT('Ctrl Pts',(0.00836549905757979,-0.0344721679344127,
0.0799769382471099));
#65989=CARTESIAN_POINT('Ctrl Pts',(0.00836381342224014,-0.0344197716859661,
0.0799363035439716));
#65990=CARTESIAN_POINT('Ctrl Pts',(0.00836215879819277,-0.0343667727831003,
0.0798964164133518));
#65991=CARTESIAN_POINT('',(0.00824276350503612,-0.0346945769587026,0.0800233599457397));
#65992=CARTESIAN_POINT('Ctrl Pts',(0.00848550275512826,-0.0341934961088741,
0.0798885047252767));
#65993=CARTESIAN_POINT('Ctrl Pts',(0.00856463333733548,-0.0340836138577592,
0.0798835168129129));
#65994=CARTESIAN_POINT('Ctrl Pts',(0.00864362273682097,-0.0339738896636479,
0.0798768938524777));
#65995=CARTESIAN_POINT('Ctrl Pts',(0.00872237042513336,-0.0338644633283559,
0.0798686510975485));
#65996=CARTESIAN_POINT('Ctrl Pts',(0.00856888350709102,-0.0341934961088741,
0.0799652433024739));
#65997=CARTESIAN_POINT('Ctrl Pts',(0.00864907226883839,-0.0340836138577592,
0.0799591056189129));
#65998=CARTESIAN_POINT('Ctrl Pts',(0.00872909554802715,-0.0339738896636479,
0.0799513115421572));
#65999=CARTESIAN_POINT('Ctrl Pts',(0.00880885159344511,-0.0338644633283559,
0.0799418779133713));
#66000=CARTESIAN_POINT('Ctrl Pts',(0.00865226425905377,-0.0341934961088741,
0.080041981879671));
#66001=CARTESIAN_POINT('Ctrl Pts',(0.0087335112003413,-0.0340836138577592,
0.0800346944249129));
#66002=CARTESIAN_POINT('Ctrl Pts',(0.00881456835923333,-0.0339738896636479,
0.0800257292318366));
#66003=CARTESIAN_POINT('Ctrl Pts',(0.00889533276175687,-0.0338644633283559,
0.0800151047291941));
#66004=CARTESIAN_POINT('Ctrl Pts',(0.00873564501101654,-0.0341934961088741,
0.0801187204568681));
#66005=CARTESIAN_POINT('Ctrl Pts',(0.00881795013184422,-0.0340836138577592,
0.0801102832309129));
#66006=CARTESIAN_POINT('Ctrl Pts',(0.00890004117043951,-0.0339738896636479,
0.080100146921516));
#66007=CARTESIAN_POINT('Ctrl Pts',(0.00898181393006862,-0.0338644633283559,
0.0800883315450169));
#66008=CARTESIAN_POINT('',(0.00873564501100223,-0.034193496108874,0.080118720456855));
#66009=CARTESIAN_POINT('',(0.00861132004496793,-0.0341934961088841,0.0800042993131389));
#66010=CARTESIAN_POINT('',(0.00874839290880158,-0.0341764758832693,0.0801173998887386));
#66011=CARTESIAN_POINT('Origin',(0.00753402011430365,-0.0345621044320822,
0.063596300007772));
#66012=CARTESIAN_POINT('Ctrl Pts',(0.00874839290846302,-0.0341764758830294,
0.0801173998855504));
#66013=CARTESIAN_POINT('Ctrl Pts',(0.00874392438930416,-0.0341260048545657,
0.0800747085898974));
#66014=CARTESIAN_POINT('Ctrl Pts',(0.00873953358334686,-0.0340749271287874,
0.0800327597498871));
#66015=CARTESIAN_POINT('Ctrl Pts',(0.00873090383116496,-0.033971543441884,
0.0799503129059302));
#66016=CARTESIAN_POINT('Ctrl Pts',(0.00872666826184563,-0.0339192781023551,
0.0799098471642289));
#66017=CARTESIAN_POINT('Ctrl Pts',(0.00872250888864519,-0.0338664212862971,
0.079870109384281));
#66018=CARTESIAN_POINT('Origin',(0.00812378219310841,-0.0315241814719618,
0.07415));
#66019=CARTESIAN_POINT('',(0.00837246424298395,-0.0347116136489624,0.0801448442196129));
#66020=CARTESIAN_POINT('',(0.00838526877038213,-0.0346945769586885,0.0801442993560471));
#66021=CARTESIAN_POINT('Origin',(0.00748666597710875,-0.0345626706594334,
0.0635682954795692));
#66022=CARTESIAN_POINT('Origin',(0.00783699278750874,-0.034562661800787,
0.0635518887600696));
#66023=CARTESIAN_POINT('Origin',(0.007882302937497,-0.0345626708902314,
0.063551884177655));
#66024=CARTESIAN_POINT('Origin',(0.00812378219310841,-0.0315241814719618,
0.07415));
#66025=CARTESIAN_POINT('',(0.00874839290883282,-0.0342105180190378,0.0801173998890376));
#66026=CARTESIAN_POINT('Origin',(0.00655961767461394,-0.0345621724972048,
0.0636930371683406));
#66027=CARTESIAN_POINT('',(0.00876113795713322,-0.034193496108874,0.0801160520974983));
#66028=CARTESIAN_POINT('Origin',(0.00748869677100344,-0.0345621724912701,
0.0635957898356987));
#66029=CARTESIAN_POINT('Origin',(0.00651538230794598,-0.0345621044227283,
0.0637029211023602));
#66030=CARTESIAN_POINT('Ctrl Pts',(0.00819861739708981,-0.0352450361874067,
0.0799009265290252));
#66031=CARTESIAN_POINT('Ctrl Pts',(0.00841551715029151,-0.0349452760959492,
0.0798981040729926));
#66032=CARTESIAN_POINT('Ctrl Pts',(0.00863158811518962,-0.0346444289841739,
0.0798789518583681));
#66033=CARTESIAN_POINT('Ctrl Pts',(0.00820111585000953,-0.0352450361874067,
0.0799008385915021));
#66034=CARTESIAN_POINT('Ctrl Pts',(0.00841801228659313,-0.0349452760959492,
0.0798979219047714));
#66035=CARTESIAN_POINT('Ctrl Pts',(0.00863407284645355,-0.0346444289841739,
0.0798786759769696));
#66036=CARTESIAN_POINT('Ctrl Pts',(0.008450961145774,-0.0352450361874067,
0.0798920448390692));
#66037=CARTESIAN_POINT('Ctrl Pts',(0.00866752592054227,-0.0349452760959492,
0.0798797050823835));
#66038=CARTESIAN_POINT('Ctrl Pts',(0.00888254597661861,-0.0346444289841739,
0.0798510878367011));
#66039=CARTESIAN_POINT('',(0.00848696272951962,-0.035195163346716,0.0798898823170016));
#66040=CARTESIAN_POINT('',(0.00872250888900978,-0.0348678972936559,0.0798701093821336));
#66041=CARTESIAN_POINT('Origin',(0.00655853854367246,-0.0345631633298701,
0.063255429313764));
#66042=CARTESIAN_POINT('',(0.00872236746249042,-0.0346945769586885,0.0798687582284338));
#66043=CARTESIAN_POINT('Origin',(0.00987283268348529,-0.0346946199326914,
0.0908599115959569));
#66044=CARTESIAN_POINT('',(0.00859804661349631,-0.0346945769330289,0.0798817709530099));
#66045=CARTESIAN_POINT('',(0.00866020703771396,-0.0346945769458128,0.0798752645908338));
#66046=CARTESIAN_POINT('',(0.00836215879816735,-0.0350221583435275,0.0798964164132232));
#66047=CARTESIAN_POINT('Origin',(0.00703135310806099,-0.0345628458714274,
0.0631648023821488));
#66048=CARTESIAN_POINT('',(0.00836210451100454,-0.035195136029876,0.0798951807167968));
#66049=CARTESIAN_POINT('Origin',(0.00881881006648593,-0.035195183836695,
0.0909046886051022));
#66050=CARTESIAN_POINT('',(0.00848699507357902,-0.0351951371328746,0.0798898781697402));
#66051=CARTESIAN_POINT('Ctrl Pts',(0.00859655477161187,-0.0346945769586965,
0.0798819271053914));
#66052=CARTESIAN_POINT('Ctrl Pts',(0.00871661227977268,-0.0345275153362944,
0.0798720246944468));
#66053=CARTESIAN_POINT('Ctrl Pts',(0.00883638941924486,-0.0343603235965185,
0.0798583440241053));
#66054=CARTESIAN_POINT('Ctrl Pts',(0.00895553254378017,-0.034193496108874,
0.0798409308207588));
#66055=CARTESIAN_POINT('Ctrl Pts',(0.00867993261225376,-0.0346945769586965,
0.0798731999053233));
#66056=CARTESIAN_POINT('Ctrl Pts',(0.00879980732571497,-0.0345275153362944,
0.0798615511121238));
#66057=CARTESIAN_POINT('Ctrl Pts',(0.00891934670109299,-0.0343603235965185,
0.0798461293565485));
#66058=CARTESIAN_POINT('Ctrl Pts',(0.00903819787187309,-0.034193496108874,
0.0798269855038953));
#66059=CARTESIAN_POINT('Ctrl Pts',(0.00876331045289566,-0.0346945769586965,
0.0798644727052552));
#66060=CARTESIAN_POINT('Ctrl Pts',(0.00888300237165726,-0.0345275153362944,
0.0798510775298008));
#66061=CARTESIAN_POINT('Ctrl Pts',(0.00900230398294112,-0.0343603235965185,
0.0798339146889917));
#66062=CARTESIAN_POINT('Ctrl Pts',(0.00912086319996601,-0.034193496108874,
0.0798130401870318));
#66063=CARTESIAN_POINT('Ctrl Pts',(0.00884668829353756,-0.0346945769586965,
0.0798557455051871));
#66064=CARTESIAN_POINT('Ctrl Pts',(0.00896619741759955,-0.0345275153362944,
0.0798406039474778));
#66065=CARTESIAN_POINT('Ctrl Pts',(0.00908526126478925,-0.0343603235965185,
0.0798217000214349));
#66066=CARTESIAN_POINT('Ctrl Pts',(0.00920352852805893,-0.034193496108874,
0.0797990948701682));
#66067=CARTESIAN_POINT('',(0.00872250888843107,-0.034521194296262,0.0798701093821982));
#66068=CARTESIAN_POINT('',(0.00895701165478282,-0.034193496108874,0.0798406813005297));
#66069=CARTESIAN_POINT('Origin',(0.00703048902793496,-0.0345625596120563,
0.0631527265340316));
#66070=CARTESIAN_POINT('Origin',(0.00987410394469407,-0.0346945685853843,
0.090872213061757));
#66071=CARTESIAN_POINT('',(0.00884668829354895,-0.0346945769586965,0.0798557455051857));
#66072=CARTESIAN_POINT('',(0.00878452787802969,-0.0346945769587025,0.0798622518668198));
#66073=CARTESIAN_POINT('',(0.00908049607825518,-0.0343667727833008,0.0798212276927166));
#66074=CARTESIAN_POINT('Origin',(0.00655194445142138,-0.0345626461565819,
0.0631994734902468));
#66075=CARTESIAN_POINT('',(0.00908027009142088,-0.034193496108874,0.079819888085349));
#66076=CARTESIAN_POINT('Origin',(0.010918983977091,-0.034193477102776,0.090719421010809));
#66077=CARTESIAN_POINT('',(0.00901864087311185,-0.034193496108884,0.0798302846929494));
#66078=CARTESIAN_POINT('Ctrl Pts',(0.00813729593822262,-0.0350241211494342,
0.0801499847815393));
#66079=CARTESIAN_POINT('Ctrl Pts',(0.00821994326849878,-0.0349144232818961,
0.0801497986352412));
#66080=CARTESIAN_POINT('Ctrl Pts',(0.00830263621940882,-0.0348045283579412,
0.0801479039981522));
#66081=CARTESIAN_POINT('Ctrl Pts',(0.00838526878148375,-0.0346945769439157,
0.0801442993555636));
#66082=CARTESIAN_POINT('Ctrl Pts',(0.00821222509612046,-0.0350241211494342,
0.0800649744109982));
#66083=CARTESIAN_POINT('Ctrl Pts',(0.00829370144339803,-0.0349144232818961,
0.0800637561462722));
#66084=CARTESIAN_POINT('Ctrl Pts',(0.00837520137579429,-0.0348045283579412,
0.080060852978038));
#66085=CARTESIAN_POINT('Ctrl Pts',(0.00845662036387449,-0.0346945769439157,
0.0800562647402515));
#66086=CARTESIAN_POINT('Ctrl Pts',(0.0082871542540183,-0.0350241211494342,
0.0799799640404571));
#66087=CARTESIAN_POINT('Ctrl Pts',(0.00836745961829727,-0.0349144232818961,
0.0799777136573032));
#66088=CARTESIAN_POINT('Ctrl Pts',(0.00844776653217976,-0.0348045283579412,
0.0799738019579238));
#66089=CARTESIAN_POINT('Ctrl Pts',(0.00852797194626523,-0.0346945769439157,
0.0799682301249394));
#66090=CARTESIAN_POINT('Ctrl Pts',(0.00836208341191614,-0.0350241211494342,
0.079894953669916));
#66091=CARTESIAN_POINT('Ctrl Pts',(0.00844121779319652,-0.0349144232818961,
0.0798916711683342));
#66092=CARTESIAN_POINT('Ctrl Pts',(0.00852033168856522,-0.0348045283579412,
0.0798867509378095));
#66093=CARTESIAN_POINT('Ctrl Pts',(0.00859932352865597,-0.0346945769439157,
0.0798801955096272));
#66094=CARTESIAN_POINT('',(0.00849165769165981,-0.0346945769458128,0.0800130351546404));
#66095=CARTESIAN_POINT('Ctrl Pts',(0.00837246424284203,-0.0347116136492819,
0.080144844216319));
#66096=CARTESIAN_POINT('Ctrl Pts',(0.00837068446168699,-0.0347621546532086,
0.0801019399907227));
#66097=CARTESIAN_POINT('Ctrl Pts',(0.00836893597389417,-0.0348133084096554,
0.0800597901373518));
#66098=CARTESIAN_POINT('Ctrl Pts',(0.00836550012579731,-0.0349168561544585,
0.0799769639980557));
#66099=CARTESIAN_POINT('Ctrl Pts',(0.00836381412832226,-0.0349692089015929,
0.0799363205651147));
#66100=CARTESIAN_POINT('Ctrl Pts',(0.00836215879818583,-0.0350221583435,
0.0798964164131859));
#66101=CARTESIAN_POINT('Ctrl Pts',(0.00851401047485387,-0.0345231616327841,
0.0801372967095463));
#66102=CARTESIAN_POINT('Ctrl Pts',(0.00859653693055541,-0.0344132092796988,
0.0801319179620799));
#66103=CARTESIAN_POINT('Ctrl Pts',(0.00867894787312256,-0.034303273855898,
0.0801248324974919));
#66104=CARTESIAN_POINT('Ctrl Pts',(0.00876113795713209,-0.034193496108874,
0.0801160520974999));
#66105=CARTESIAN_POINT('Ctrl Pts',(0.00858345393086496,-0.0345231616327841,
0.0800477492776698));
#66106=CARTESIAN_POINT('Ctrl Pts',(0.00866474610129079,-0.0344132092796988,
0.0800414133499308));
#66107=CARTESIAN_POINT('Ctrl Pts',(0.00874590302374674,-0.034303273855898,
0.0800333962846738));
#66108=CARTESIAN_POINT('Ctrl Pts',(0.00882682098992594,-0.034193496108874,
0.080023711015952));
#66109=CARTESIAN_POINT('Ctrl Pts',(0.00865289738687605,-0.0345231616327841,
0.0799582018457932));
#66110=CARTESIAN_POINT('Ctrl Pts',(0.00873295527202617,-0.0344132092796988,
0.0799509087377818));
#66111=CARTESIAN_POINT('Ctrl Pts',(0.00881285817437092,-0.034303273855898,
0.0799419600718556));
#66112=CARTESIAN_POINT('Ctrl Pts',(0.00889250402271978,-0.034193496108874,
0.0799313699344041));
#66113=CARTESIAN_POINT('Ctrl Pts',(0.00872234084288715,-0.0345231616327841,
0.0798686544139167));
#66114=CARTESIAN_POINT('Ctrl Pts',(0.00880116444276154,-0.0344132092796988,
0.0798604041256328));
#66115=CARTESIAN_POINT('Ctrl Pts',(0.00887981332499511,-0.034303273855898,
0.0798505238590375));
#66116=CARTESIAN_POINT('Ctrl Pts',(0.00895818705551363,-0.034193496108874,
0.0798390288528561));
#66117=CARTESIAN_POINT('Ctrl Pts',(0.00874839290846746,-0.0342105180195409,
0.0801173998855935));
#66118=CARTESIAN_POINT('Ctrl Pts',(0.00874391938062411,-0.0342610556241027,
0.0800746607380183));
#66119=CARTESIAN_POINT('Ctrl Pts',(0.00873952612792476,-0.0343122189869566,
0.0800326885223474));
#66120=CARTESIAN_POINT('Ctrl Pts',(0.00873089632176624,-0.03441581196951,
0.0799502411627092));
#66121=CARTESIAN_POINT('Ctrl Pts',(0.00872666329796788,-0.0344681990449968,
0.0799097997403819));
#66122=CARTESIAN_POINT('Ctrl Pts',(0.00872250888842384,-0.0345211942962374,
0.0798701093821663));
#66123=CARTESIAN_POINT('',(0.00885907480596801,-0.0341934961088839,0.079978366699024));
#66124=CARTESIAN_POINT('Ctrl Pts',(0.00848591858107241,-0.0351951371254931,
0.079888887426213));
#66125=CARTESIAN_POINT('Ctrl Pts',(0.00856495229917834,-0.0350856248738967,
0.0798839002251971));
#66126=CARTESIAN_POINT('Ctrl Pts',(0.00864394783125726,-0.0349758427086611,
0.0798772756007074));
#66127=CARTESIAN_POINT('Ctrl Pts',(0.00872280354676591,-0.0348659306906667,
0.079869016093009));
#66128=CARTESIAN_POINT('Ctrl Pts',(0.00854641813340751,-0.0351951371254931,
0.0799445675377254));
#66129=CARTESIAN_POINT('Ctrl Pts',(0.00862621865628073,-0.0350856248738967,
0.0799387471604839));
#66130=CARTESIAN_POINT('Ctrl Pts',(0.00870596440399965,-0.0349758427086611,
0.0799312728288274));
#66131=CARTESIAN_POINT('Ctrl Pts',(0.00878555272167216,-0.0348659306906667,
0.0799221481144213));
#66132=CARTESIAN_POINT('Ctrl Pts',(0.00860691768574261,-0.0351951371254931,
0.0800002476492377));
#66133=CARTESIAN_POINT('Ctrl Pts',(0.00868748501338313,-0.0350856248738967,
0.0799935940957707));
#66134=CARTESIAN_POINT('Ctrl Pts',(0.00876798097674204,-0.0349758427086611,
0.0799852700569474));
#66135=CARTESIAN_POINT('Ctrl Pts',(0.00884830189657841,-0.0348659306906667,
0.0799752801358336));
#66136=CARTESIAN_POINT('Ctrl Pts',(0.00866741723807771,-0.0351951371254931,
0.0800559277607501));
#66137=CARTESIAN_POINT('Ctrl Pts',(0.00874875137048552,-0.0350856248738967,
0.0800484410310575));
#66138=CARTESIAN_POINT('Ctrl Pts',(0.00882999754948443,-0.0349758427086611,
0.0800392672850673));
#66139=CARTESIAN_POINT('Ctrl Pts',(0.00891105107148466,-0.0348659306906667,
0.0800284121572459));
#66140=CARTESIAN_POINT('Origin',(0.00927614291461343,-0.030860918850898,
0.0851593964693888));
#66141=CARTESIAN_POINT('',(0.00856565507232487,-0.0351951371254931,0.0799622720473082));
#66142=CARTESIAN_POINT('Ctrl Pts',(0.00884511306056555,-0.0346945769586931,
0.0798544687873255));
#66143=CARTESIAN_POINT('Ctrl Pts',(0.00892372352378627,-0.0345846629175835,
0.0798445284833742));
#66144=CARTESIAN_POINT('Ctrl Pts',(0.00900214185246384,-0.034474692504983,
0.0798329608494984));
#66145=CARTESIAN_POINT('Ctrl Pts',(0.00908026762921077,-0.0343648066252516,
0.0798197811224456));
#66146=CARTESIAN_POINT('Ctrl Pts',(0.00893314760635036,-0.0346945769586931,
0.0799258203136349));
#66147=CARTESIAN_POINT('Ctrl Pts',(0.00901274132966835,-0.0345846629175835,
0.0799146668491456));
#66148=CARTESIAN_POINT('Ctrl Pts',(0.00909211799872473,-0.034474692504983,
0.0799018655141058));
#66149=CARTESIAN_POINT('Ctrl Pts',(0.00917117597472416,-0.0343648066252516,
0.0798874331310947));
#66150=CARTESIAN_POINT('Ctrl Pts',(0.00902118215213519,-0.0346945769586931,
0.0799971718399444));
#66151=CARTESIAN_POINT('Ctrl Pts',(0.00910175913555044,-0.0345846629175835,
0.079984805214917));
#66152=CARTESIAN_POINT('Ctrl Pts',(0.00918209414498561,-0.034474692504983,
0.0799707701787133));
#66153=CARTESIAN_POINT('Ctrl Pts',(0.00926208432023754,-0.0343648066252516,
0.0799550851397438));
#66154=CARTESIAN_POINT('Ctrl Pts',(0.00910921669792,-0.0346945769586931,
0.0800685233662539));
#66155=CARTESIAN_POINT('Ctrl Pts',(0.00919077694143253,-0.0345846629175835,
0.0800549435806884));
#66156=CARTESIAN_POINT('Ctrl Pts',(0.00927207029124649,-0.034474692504983,
0.0800396748433208));
#66157=CARTESIAN_POINT('Ctrl Pts',(0.00935299266575093,-0.0343648066252516,
0.0800227371483928));
#66158=CARTESIAN_POINT('',(0.009109216697909,-0.0346945769586885,0.0800685233662417));
#66159=CARTESIAN_POINT('',(0.00897795249573898,-0.0346945769587025,0.0799621344357236));
#66160=CARTESIAN_POINT('',(0.00912185652151936,-0.0346775396663496,0.0800664049570397));
#66161=CARTESIAN_POINT('Origin',(0.00620977999082163,-0.0345626617704269,
0.0637222098416));
#66162=CARTESIAN_POINT('Ctrl Pts',(0.00912185652095255,-0.0346775396659521,
0.0800664049537068));
#66163=CARTESIAN_POINT('Ctrl Pts',(0.00911471058875113,-0.03462697485299,
0.0800240451539444));
#66164=CARTESIAN_POINT('Ctrl Pts',(0.00910769171401761,-0.0345757904818634,
0.0799824385279803));
#66165=CARTESIAN_POINT('Ctrl Pts',(0.0090939020602039,-0.0344721679344743,
0.0799006959424259));
#66166=CARTESIAN_POINT('Ctrl Pts',(0.00908713683786502,-0.0344197716860438,
0.079860592922198));
#66167=CARTESIAN_POINT('Ctrl Pts',(0.0090804960779661,-0.0343667727831938,
0.0798212276929094));
#66168=CARTESIAN_POINT('Origin',(0.00812378219310841,-0.0315241814719618,
0.07415));
#66169=CARTESIAN_POINT('',(0.00912185652150067,-0.0347116136489619,0.0800664049569289));
#66170=CARTESIAN_POINT('Origin',(0.00655591106685294,-0.0345626706845752,
0.0636657179185765));
#66171=CARTESIAN_POINT('',(0.00913449179186378,-0.0346945769586886,0.0800642595569509));
#66172=CARTESIAN_POINT('Origin',(0.00616545050053386,-0.0345626706260411,
0.0637315869851469));
#66173=CARTESIAN_POINT('Origin',(0.00651095856197596,-0.0345626618561295,
0.0636714021604937));
#66174=CARTESIAN_POINT('Origin',(0.00788233303269208,-0.0351840467447537,
0.0732031905879628));
#66175=CARTESIAN_POINT('',(0.00908028734499586,-0.035195136029876,0.0798200085441095));
#66176=CARTESIAN_POINT('Origin',(0.0101570089533248,-0.0352322613584381,
0.0859412120342698));
#66177=CARTESIAN_POINT('',(0.00895731903566345,-0.0351951142564677,0.0798406090109526));
#66178=CARTESIAN_POINT('',(0.00908027014552778,-0.0351951372916786,0.0798198880762214));
#66179=CARTESIAN_POINT('Origin',(0.00838011388044975,-0.0352875103405805,
0.0739259169494507));
#66180=CARTESIAN_POINT('Ctrl Pts',(0.00891880951702706,-0.0352450361874076,
0.079846199417526));
#66181=CARTESIAN_POINT('Ctrl Pts',(0.00913364520334914,-0.0349452760959497,
0.0798162144699741));
#66182=CARTESIAN_POINT('Ctrl Pts',(0.00934561197516326,-0.0346444289841739,
0.0797701324035723));
#66183=CARTESIAN_POINT('Ctrl Pts',(0.00892127724740515,-0.0352450361874076,
0.0798457990342332));
#66184=CARTESIAN_POINT('Ctrl Pts',(0.00913609783302355,-0.0349452760959497,
0.079815721014703));
#66185=CARTESIAN_POINT('Ctrl Pts',(0.00934804253647126,-0.0346444289841739,
0.0797695472781772));
#66186=CARTESIAN_POINT('Ctrl Pts',(0.00916805028897418,-0.0352450361874076,
0.0798057607043536));
#66187=CARTESIAN_POINT('Ctrl Pts',(0.00938136080420208,-0.0349452760959497,
0.0797663754868366));
#66188=CARTESIAN_POINT('Ctrl Pts',(0.00959109867097598,-0.0346444289841739,
0.0797110347377743));
#66189=CARTESIAN_POINT('',(0.00908049607791315,-0.0350221583435275,0.0798212276927154));
#66190=CARTESIAN_POINT('',(0.00931268828447517,-0.0346945769330289,0.079777133133678));
#66191=CARTESIAN_POINT('Origin',(0.005663156899118,-0.0345628458716139,
0.0633883416159371));
#66192=CARTESIAN_POINT('Origin',(0.0109132497041071,-0.0351951838366848,
0.0906854626481361));
#66193=CARTESIAN_POINT('',(0.00920349695358097,-0.0351951633467166,0.0797991030395162));
#66194=CARTESIAN_POINT('',(0.00920352852280879,-0.0351951371328746,0.0797990948711718));
#66195=CARTESIAN_POINT('',(0.00943470755481608,-0.0348678972925388,0.0797499642584603));
#66196=CARTESIAN_POINT('Origin',(0.00520542918551106,-0.0345631633303276,
0.0635375133050744));
#66197=CARTESIAN_POINT('',(0.00943439789959453,-0.0346945769586885,0.0797486414843168));
#66198=CARTESIAN_POINT('Origin',(0.0119533318496204,-0.0346946199340818,
0.0905089382316885));
#66199=CARTESIAN_POINT('',(0.00937354309177105,-0.0346945769458128,0.0797628873091441));
#66200=CARTESIAN_POINT('Origin',(0.000623215658025582,-0.0298325076523077,
0.0739584486183963));
#66201=CARTESIAN_POINT('Origin',(0.00630463286954172,-0.033873312329463,
0.082331557296228));
#66202=CARTESIAN_POINT('Ctrl Pts',(0.00888918687231204,-0.0350241211494342,
0.0801009793880569));
#66203=CARTESIAN_POINT('Ctrl Pts',(0.00897115917338596,-0.0349144232818962,
0.080090436252429));
#66204=CARTESIAN_POINT('Ctrl Pts',(0.00905296260468609,-0.0348045283579412,
0.0800781923801888));
#66205=CARTESIAN_POINT('Ctrl Pts',(0.00913449180281645,-0.0346945769439158,
0.0800642595550811));
#66206=CARTESIAN_POINT('Ctrl Pts',(0.0089528705667935,-0.0350241211494342,
0.0800072482360308));
#66207=CARTESIAN_POINT('Ctrl Pts',(0.00903355175967953,-0.0349144232818962,
0.0799958278836228));
#66208=CARTESIAN_POINT('Ctrl Pts',(0.00911404517730361,-0.0348045283579412,
0.0799827329576747));
#66209=CARTESIAN_POINT('Ctrl Pts',(0.00919424709366599,-0.0346945769439158,
0.079967976394464));
#66210=CARTESIAN_POINT('Ctrl Pts',(0.00901655426127497,-0.0350241211494342,
0.0799135170840048));
#66211=CARTESIAN_POINT('Ctrl Pts',(0.0090959443459731,-0.0349144232818962,
0.0799012195148165));
#66212=CARTESIAN_POINT('Ctrl Pts',(0.00917512774992114,-0.0348045283579412,
0.0798872735351606));
#66213=CARTESIAN_POINT('Ctrl Pts',(0.00925400238451553,-0.0346945769439158,
0.0798716932338468));
#66214=CARTESIAN_POINT('Ctrl Pts',(0.00908023795575643,-0.0350241211494342,
0.0798197859319787));
#66215=CARTESIAN_POINT('Ctrl Pts',(0.00915833693226667,-0.0349144232818962,
0.0798066111460103));
#66216=CARTESIAN_POINT('Ctrl Pts',(0.00923621032253866,-0.0348045283579412,
0.0797918141126465));
#66217=CARTESIAN_POINT('Ctrl Pts',(0.00931375767536507,-0.0346945769439158,
0.0797754100732296));
#66218=CARTESIAN_POINT('Ctrl Pts',(0.00912185652094782,-0.0347116136492809,
0.0800664049536785));
#66219=CARTESIAN_POINT('Ctrl Pts',(0.00911471344857282,-0.0347621546531963,
0.0800240621064524));
#66220=CARTESIAN_POINT('Ctrl Pts',(0.00910769597071279,-0.0348133084096308,
0.0799824637609031));
#66221=CARTESIAN_POINT('Ctrl Pts',(0.00909390634743964,-0.0349168561544574,
0.0799007213563877));
#66222=CARTESIAN_POINT('Ctrl Pts',(0.00908713967168468,-0.0349692089015915,
0.0798606097205706));
#66223=CARTESIAN_POINT('Ctrl Pts',(0.00908049607792671,-0.0350221583435,
0.0798212276926761));
#66224=CARTESIAN_POINT('',(0.00922359003790568,-0.0346945769458128,0.0799206963454612));
#66225=CARTESIAN_POINT('Ctrl Pts',(0.00920233634567586,-0.0351951371254938,
0.0797982468602394));
#66226=CARTESIAN_POINT('Ctrl Pts',(0.00928012179748727,-0.0350856248736035,
0.0797833934333025));
#66227=CARTESIAN_POINT('Ctrl Pts',(0.00935766414079992,-0.0349758427080725,
0.0797669202804344));
#66228=CARTESIAN_POINT('Ctrl Pts',(0.00943486286483655,-0.0348659306897825,
0.0797488426595543));
#66229=CARTESIAN_POINT('Ctrl Pts',(0.00926933740939195,-0.0351951371254938,
0.0798459053129186));
#66230=CARTESIAN_POINT('Ctrl Pts',(0.00934777919481731,-0.0350856248736035,
0.079830129173476));
#66231=CARTESIAN_POINT('Ctrl Pts',(0.00942595934155043,-0.0349758427080725,
0.0798127189866814));
#66232=CARTESIAN_POINT('Ctrl Pts',(0.00950377645181123,-0.0348659306897825,
0.0797936911621062));
#66233=CARTESIAN_POINT('Ctrl Pts',(0.00933633847310804,-0.0351951371254938,
0.0798935637655978));
#66234=CARTESIAN_POINT('Ctrl Pts',(0.00941543659214735,-0.0350856248736035,
0.0798768649136495));
#66235=CARTESIAN_POINT('Ctrl Pts',(0.00949425454230094,-0.0349758427080725,
0.0798585176929283));
#66236=CARTESIAN_POINT('Ctrl Pts',(0.00957269003878591,-0.0348659306897825,
0.0798385396646581));
#66237=CARTESIAN_POINT('Ctrl Pts',(0.00940333953682413,-0.0351951371254938,
0.079941222218277));
#66238=CARTESIAN_POINT('Ctrl Pts',(0.0094830939894774,-0.0350856248736035,
0.079923600653823));
#66239=CARTESIAN_POINT('Ctrl Pts',(0.00956254974305145,-0.0349758427080725,
0.0799043163991753));
#66240=CARTESIAN_POINT('Ctrl Pts',(0.00964160362576058,-0.0348659306897825,
0.07988338816721));
#66241=CARTESIAN_POINT('',(0.0092906416227406,-0.0351951371254938,0.079861059189401));
#66242=CARTESIAN_POINT('Origin',(0.0106468975549029,-0.0308609197410635,
0.0849281543167568));
#66243=CARTESIAN_POINT('Ctrl Pts',(0.00545294195983083,-0.0321934096636941,
0.0792435987468211));
#66244=CARTESIAN_POINT('Ctrl Pts',(0.00554411495180879,-0.0320508460844048,
0.079291405515133));
#66245=CARTESIAN_POINT('Ctrl Pts',(0.00563650367258421,-0.0319086045662519,
0.0793367265985879));
#66246=CARTESIAN_POINT('Ctrl Pts',(0.00572990115924722,-0.0317669892867074,
0.0793794807900028));
#66247=CARTESIAN_POINT('Ctrl Pts',(0.00552802930713434,-0.0321934096636941,
0.0792809125901338));
#66248=CARTESIAN_POINT('Ctrl Pts',(0.0056198701991386,-0.0320508460844048,
0.0793273753306858));
#66249=CARTESIAN_POINT('Ctrl Pts',(0.00571289020496758,-0.0319086045662519,
0.0793713354546265));
#66250=CARTESIAN_POINT('Ctrl Pts',(0.00580688124369109,-0.0317669892867074,
0.0794127147970611));
#66251=CARTESIAN_POINT('Ctrl Pts',(0.00560311665443784,-0.0321934096636941,
0.0793182264334465));
#66252=CARTESIAN_POINT('Ctrl Pts',(0.00569562544646842,-0.0320508460844048,
0.0793633451462386));
#66253=CARTESIAN_POINT('Ctrl Pts',(0.00578927673735094,-0.0319086045662519,
0.0794059443106649));
#66254=CARTESIAN_POINT('Ctrl Pts',(0.00588386132813497,-0.0317669892867074,
0.0794459488041194));
#66255=CARTESIAN_POINT('Ctrl Pts',(0.00567820400174134,-0.0321934096636941,
0.0793555402767591));
#66256=CARTESIAN_POINT('Ctrl Pts',(0.00577138069379823,-0.0320508460844048,
0.0793993149617914));
#66257=CARTESIAN_POINT('Ctrl Pts',(0.00586566326973432,-0.0319086045662518,
0.0794405531667035));
#66258=CARTESIAN_POINT('Ctrl Pts',(0.00596084141257884,-0.0317669892867074,
0.0794791828111777));
#66259=CARTESIAN_POINT('',(0.00567686067426102,-0.0321934096636941,0.0793548727247266));
#66260=CARTESIAN_POINT('',(0.00589276668497216,-0.0318665617511328,0.0794510088465921));
#66261=CARTESIAN_POINT('Origin',(0.0133377615190161,-0.0326371944419888,
0.064504670602517));
#66262=CARTESIAN_POINT('Origin',(0.00164080164324394,-0.0316939261509349,
0.089553898701131));
#66263=CARTESIAN_POINT('',(0.00556457329482249,-0.0320197221621744,0.0793005377371172));
#66264=CARTESIAN_POINT('Ctrl Pts',(0.00556471247059017,-0.0320197392094667,
0.0793006595771184));
#66265=CARTESIAN_POINT('Ctrl Pts',(0.00559092070329904,-0.0319792716575964,
0.0793136809045492));
#66266=CARTESIAN_POINT('Ctrl Pts',(0.00561734751521862,-0.0319386439829625,
0.0793265617090013));
#66267=CARTESIAN_POINT('Ctrl Pts',(0.0056440243550796,-0.0318979099381557,
0.0793393079103611));
#66268=CARTESIAN_POINT('Ctrl Pts',(0.00567070066765265,-0.0318571766984881,
0.0793520538597826));
#66269=CARTESIAN_POINT('Ctrl Pts',(0.00569749064372408,-0.0318163871833553,
0.079364602035801));
#66270=CARTESIAN_POINT('Ctrl Pts',(0.00572430064325569,-0.0317755399638303,
0.0793769124665612));
#66271=CARTESIAN_POINT('',(0.0055649205590403,-0.0321934096636183,0.0792992452978757));
#66272=CARTESIAN_POINT('Origin',(0.004556373628744,-0.0324113149036198,
0.0813760325455046));
#66273=CARTESIAN_POINT('',(0.00562089061666066,-0.0321934096636663,0.0793270590113111));
#66274=CARTESIAN_POINT('Ctrl Pts',(0.00567621457844038,-0.0321934096636618,
0.0793529501619655));
#66275=CARTESIAN_POINT('Ctrl Pts',(0.00574796731611607,-0.0320835708272592,
0.0793867040268945));
#66276=CARTESIAN_POINT('Ctrl Pts',(0.00582037696876832,-0.0319739230346488,
0.0794189533940329));
#66277=CARTESIAN_POINT('Ctrl Pts',(0.00589334772661693,-0.0318646057455573,
0.0794496641126543));
#66278=CARTESIAN_POINT('Ctrl Pts',(0.00571231260492629,-0.0321934096636618,
0.0794603656973853));
#66279=CARTESIAN_POINT('Ctrl Pts',(0.0057855466865502,-0.0320835708272592,
0.0794936217423959));
#66280=CARTESIAN_POINT('Ctrl Pts',(0.00585942652155362,-0.0319739230346488,
0.0795253429220357));
#66281=CARTESIAN_POINT('Ctrl Pts',(0.00593385447102425,-0.0318646057455573,
0.0795554959057187));
#66282=CARTESIAN_POINT('Ctrl Pts',(0.0057484106314122,-0.0321934096636618,
0.0795677812328052));
#66283=CARTESIAN_POINT('Ctrl Pts',(0.00582312605698432,-0.0320835708272592,
0.0796005394578972));
#66284=CARTESIAN_POINT('Ctrl Pts',(0.00589847607433893,-0.0319739230346488,
0.0796317324500384));
#66285=CARTESIAN_POINT('Ctrl Pts',(0.00597436121543156,-0.0318646057455573,
0.0796613276987831));
#66286=CARTESIAN_POINT('Ctrl Pts',(0.00578450865789812,-0.0321934096636618,
0.079675196768225));
#66287=CARTESIAN_POINT('Ctrl Pts',(0.00586070542741844,-0.0320835708272592,
0.0797074571733986));
#66288=CARTESIAN_POINT('Ctrl Pts',(0.00593752562712424,-0.0319739230346488,
0.0797381219780412));
#66289=CARTESIAN_POINT('Ctrl Pts',(0.00601486795983887,-0.0318646057455573,
0.0797671594918474));
#66290=CARTESIAN_POINT('',(0.00579631591447991,-0.0321763980308314,0.0796801808921294));
#66291=CARTESIAN_POINT('',(0.00578450865792329,-0.0321934096636184,0.079675196768223));
#66292=CARTESIAN_POINT('Origin',(0.0127763985114372,-0.0326386231203367,
0.06467669662428));
#66293=CARTESIAN_POINT('Ctrl Pts',(0.00579631591570451,-0.0321763980306366,
0.0796801808892017));
#66294=CARTESIAN_POINT('Ctrl Pts',(0.00581296462851228,-0.0321259596176305,
0.0796406226819386));
#66295=CARTESIAN_POINT('Ctrl Pts',(0.00582932488076331,-0.032074916463434,
0.079601749871939));
#66296=CARTESIAN_POINT('Ctrl Pts',(0.005861481630547,-0.0319716057793989,
0.0795253437624975));
#66297=CARTESIAN_POINT('Ctrl Pts',(0.00587726559859713,-0.0319193786690187,
0.0794878402337576));
#66298=CARTESIAN_POINT('Ctrl Pts',(0.00589276668568432,-0.0318665617525382,
0.0794510088448763));
#66299=CARTESIAN_POINT('',(0.00573068466610216,-0.0321934096636663,0.0795150347464848));
#66300=CARTESIAN_POINT('Origin',(0.00812378219310841,-0.0315241814719618,
0.07415));
#66301=CARTESIAN_POINT('',(0.0057963159143359,-0.0322104233323592,0.0796801808924703));
#66302=CARTESIAN_POINT('',(0.00580813378883182,-0.0321934096636183,0.0796851397875583));
#66303=CARTESIAN_POINT('Origin',(0.0127374721225919,-0.0326387223296586,
0.0646534565409408));
#66304=CARTESIAN_POINT('Origin',(0.0116454707300995,-0.0326386250315982,
0.0642007234862707));
#66305=CARTESIAN_POINT('Origin',(0.0116892981152757,-0.0326387238142873,
0.0642123200058464));
#66306=CARTESIAN_POINT('Ctrl Pts',(0.00574512659303898,-0.0327445246967097,
0.0793864226850263));
#66307=CARTESIAN_POINT('Ctrl Pts',(0.00594262150320909,-0.032443687833936,
0.079476135147583));
#66308=CARTESIAN_POINT('Ctrl Pts',(0.00614631286053686,-0.0321434074405928,
0.0795507166227029));
#66309=CARTESIAN_POINT('Ctrl Pts',(0.00597493679531699,-0.0327445246967097,
0.0794848466197624));
#66310=CARTESIAN_POINT('Ctrl Pts',(0.00617614382487061,-0.032443687833936,
0.0795658916488468));
#66311=CARTESIAN_POINT('Ctrl Pts',(0.00638288388932941,-0.0321434074405928,
0.0796315507017539));
#66312=CARTESIAN_POINT('',(0.00600850577735225,-0.0326943950436612,0.0794982455707406));
#66313=CARTESIAN_POINT('',(0.00623002218363936,-0.0323666188837389,0.0795806351402517));
#66314=CARTESIAN_POINT('Origin',(0.0121206135023099,-0.0326395579113119,
0.0638377795047609));
#66315=CARTESIAN_POINT('Origin',(0.00259334537534946,-0.0321933825603034,
0.0900093432880409));
#66316=CARTESIAN_POINT('',(0.00611244010570222,-0.032193409653269,0.0795381933896475));
#66317=CARTESIAN_POINT('',(0.00617145480780626,-0.0321934096584275,0.0795587728765589));
#66318=CARTESIAN_POINT('',(0.00589276668459501,-0.0325210109756239,0.0794510088474529));
#66319=CARTESIAN_POINT('Origin',(0.0125577735393507,-0.0326393129161412,
0.0640379682458832));
#66320=CARTESIAN_POINT('',(0.00589329367539631,-0.0326943950436593,0.0794497566899203));
#66321=CARTESIAN_POINT('Origin',(0.00160204435036457,-0.0326943765538151,
0.0896459861852913));
#66322=CARTESIAN_POINT('',(0.00595089972638428,-0.0326943950436702,0.0794740011303405));
#66323=CARTESIAN_POINT('Ctrl Pts',(0.00558133952140229,-0.0325229783203769,
0.079584701947773));
#66324=CARTESIAN_POINT('Ctrl Pts',(0.00565625676890326,-0.032413025309245,
0.079619749464403));
#66325=CARTESIAN_POINT('Ctrl Pts',(0.00573188765663896,-0.032303122220807,
0.0796532419058877));
#66326=CARTESIAN_POINT('Ctrl Pts',(0.00580813379296862,-0.0321934096576658,
0.079685139789289));
#66327=CARTESIAN_POINT('Ctrl Pts',(0.00568533311590499,-0.0325229783203769,
0.0795396855669895));
#66328=CARTESIAN_POINT('Ctrl Pts',(0.0057596298135813,-0.032413025309245,
0.0795732995341935));
#66329=CARTESIAN_POINT('Ctrl Pts',(0.00583461059079949,-0.032303122220807,
0.0796053714805483));
#66330=CARTESIAN_POINT('Ctrl Pts',(0.00591017795287016,-0.0321934096576658,
0.0796358637132843));
#66331=CARTESIAN_POINT('Ctrl Pts',(0.00578932671040769,-0.0325229783203769,
0.079494669186206));
#66332=CARTESIAN_POINT('Ctrl Pts',(0.00586300285825935,-0.032413025309245,
0.079526849603984));
#66333=CARTESIAN_POINT('Ctrl Pts',(0.00593733352496002,-0.032303122220807,
0.0795575010552089));
#66334=CARTESIAN_POINT('Ctrl Pts',(0.00601222211277171,-0.0321934096576658,
0.0795865876372795));
#66335=CARTESIAN_POINT('Ctrl Pts',(0.0058933203049104,-0.0325229783203769,
0.0794496528054225));
#66336=CARTESIAN_POINT('Ctrl Pts',(0.00596637590293739,-0.032413025309245,
0.0794803996737744));
#66337=CARTESIAN_POINT('Ctrl Pts',(0.00604005645912054,-0.032303122220807,
0.0795096306298695));
#66338=CARTESIAN_POINT('Ctrl Pts',(0.00611426627267325,-0.0321934096576658,
0.0795373115612748));
#66339=CARTESIAN_POINT('',(0.00596028694676296,-0.0321934096584275,0.079611666588569));
#66340=CARTESIAN_POINT('Ctrl Pts',(0.00579631591568124,-0.0322104233328918,
0.0796801808892569));
#66341=CARTESIAN_POINT('Ctrl Pts',(0.00581298718780795,-0.0322609421831307,
0.0796405690798791));
#66342=CARTESIAN_POINT('Ctrl Pts',(0.00582935846068635,-0.0323120888240607,
0.0796016700843133));
#66343=CARTESIAN_POINT('Ctrl Pts',(0.00586151545385223,-0.0324156524631807,
0.0795252633965831));
#66344=CARTESIAN_POINT('Ctrl Pts',(0.00587728795592471,-0.0324680267167312,
0.0794877871115846));
#66345=CARTESIAN_POINT('Ctrl Pts',(0.00589276668461587,-0.0325210109755912,
0.0794510088474146));
#66346=CARTESIAN_POINT('Origin',(0.00129234738506729,-0.0262834582510987,
0.0702468110083525));
#66347=CARTESIAN_POINT('Origin',(-0.00110757709133214,-0.0342770866417274,
0.0820623878212155));
#66348=CARTESIAN_POINT('Ctrl Pts',(0.00600774042359261,-0.0326943950436604,
0.0794963678262276));
#66349=CARTESIAN_POINT('Ctrl Pts',(0.00608142339239928,-0.0325844576448134,
0.0795255308476965));
#66350=CARTESIAN_POINT('Ctrl Pts',(0.00615571471496154,-0.0324744968375322,
0.079553172048478));
#66351=CARTESIAN_POINT('Ctrl Pts',(0.00623051871641797,-0.0323646534831894,
0.0795792573259598));
#66352=CARTESIAN_POINT('Ctrl Pts',(0.00605051183421898,-0.0326943950436604,
0.0796013046358585));
#66353=CARTESIAN_POINT('Ctrl Pts',(0.00612564102893491,-0.0325844576448134,
0.0796298781871268));
#66354=CARTESIAN_POINT('Ctrl Pts',(0.00620136648854788,-0.0324744968375322,
0.079656899965667));
#66355=CARTESIAN_POINT('Ctrl Pts',(0.00627759071164313,-0.0323646534831894,
0.0796823366878515));
#66356=CARTESIAN_POINT('Ctrl Pts',(0.00609328324484535,-0.0326943950436604,
0.0797062414454894));
#66357=CARTESIAN_POINT('Ctrl Pts',(0.00616985866547053,-0.0325844576448134,
0.0797342255265571));
#66358=CARTESIAN_POINT('Ctrl Pts',(0.00624701826213421,-0.0324744968375322,
0.079760627882856));
#66359=CARTESIAN_POINT('Ctrl Pts',(0.00632466270686829,-0.0323646534831894,
0.0797854160497432));
#66360=CARTESIAN_POINT('Ctrl Pts',(0.00613605465547172,-0.0326943950436605,
0.0798111782551203));
#66361=CARTESIAN_POINT('Ctrl Pts',(0.00621407630200616,-0.0325844576448134,
0.0798385728659873));
#66362=CARTESIAN_POINT('Ctrl Pts',(0.00629267003572055,-0.0324744968375322,
0.079864355800045));
#66363=CARTESIAN_POINT('Ctrl Pts',(0.00637173470209345,-0.0323646534831894,
0.0798884954116349));
#66364=CARTESIAN_POINT('',(0.0061481515687621,-0.0326773559991203,0.0798154111604032));
#66365=CARTESIAN_POINT('',(0.00613605465546716,-0.0326943950436594,0.0798111782551076));
#66366=CARTESIAN_POINT('Origin',(0.0115683174553085,-0.0326395670534535,
0.0641197075211798));
#66367=CARTESIAN_POINT('Ctrl Pts',(0.0061481515698599,-0.0326773559987499,
0.0798154111572346));
#66368=CARTESIAN_POINT('Ctrl Pts',(0.00616229492231307,-0.0326267922587316,
0.0797748530155223));
#66369=CARTESIAN_POINT('Ctrl Pts',(0.00617618759405846,-0.0325756109582041,
0.0797350137375803));
#66370=CARTESIAN_POINT('Ctrl Pts',(0.00620348339961995,-0.032471998546238,
0.0796567390036529));
#66371=CARTESIAN_POINT('Ctrl Pts',(0.00621687558572942,-0.0324196091621781,
0.0796183349418251));
#66372=CARTESIAN_POINT('Ctrl Pts',(0.00623002218365545,-0.0323666188837756,
0.0795806351402057));
#66373=CARTESIAN_POINT('',(0.00607228021641971,-0.0326943950436703,0.0796547119129341));
#66374=CARTESIAN_POINT('Ctrl Pts',(0.00607865468745572,-0.0332451089994434,
0.0795254607696106));
#66375=CARTESIAN_POINT('Ctrl Pts',(0.00628139350736245,-0.0329451141710254,
0.0796025940154523));
#66376=CARTESIAN_POINT('Ctrl Pts',(0.00648936635907893,-0.0326442513127494,
0.0796642370171651));
#66377=CARTESIAN_POINT('Ctrl Pts',(0.00631419207329205,-0.0332451089994434,
0.07960925897886));
#66378=CARTESIAN_POINT('Ctrl Pts',(0.00652009139436912,-0.0329451141710254,
0.0796775087868542));
#66379=CARTESIAN_POINT('Ctrl Pts',(0.00673054663175123,-0.0326442513127494,
0.0797300555257605));
#66380=CARTESIAN_POINT('Ctrl Pts',(0.00631654744715042,-0.0332451089994434,
0.0796100969609525));
#66381=CARTESIAN_POINT('Ctrl Pts',(0.00652247837323919,-0.0329451141710254,
0.0796782579345683));
#66382=CARTESIAN_POINT('Ctrl Pts',(0.00673295843447796,-0.0326442513127494,
0.0797307137108465));
#66383=CARTESIAN_POINT('',(0.00634849891012766,-0.0331951640388616,0.0796205113348909));
#66384=CARTESIAN_POINT('',(0.00657475150005643,-0.0328677532355031,0.0796888292067752));
#66385=CARTESIAN_POINT('Origin',(0.0107871679007543,-0.0326402808280936,
0.0634547925117744));
#66386=CARTESIAN_POINT('Origin',(0.00359737778299924,-0.0326944278779056,
0.0903363466980259));
#66387=CARTESIAN_POINT('',(0.00645473649828102,-0.0326943950436593,0.0796538542375847));
#66388=CARTESIAN_POINT('',(0.00651492694246295,-0.0326943950436694,0.0796706875507087));
#66389=CARTESIAN_POINT('',(0.0062300221836367,-0.0330220786163545,0.0795806351402508));
#66390=CARTESIAN_POINT('Origin',(0.0112576571543798,-0.0326396682763637,
0.0635537496105579));
#66391=CARTESIAN_POINT('',(0.00623046951091848,-0.0331951640388588,0.0795793523635383));
#66392=CARTESIAN_POINT('Origin',(0.00259805675387946,-0.033195202656003,
0.0899958271549816));
#66393=CARTESIAN_POINT('',(0.00628948421053307,-0.0331951640388702,0.0795999318492247));
#66394=CARTESIAN_POINT('Ctrl Pts',(0.00634761702129453,-0.0331951640388604,
0.0796186850611225));
#66395=CARTESIAN_POINT('Ctrl Pts',(0.00646067857873859,-0.0330306422010619,
0.0796554061372785));
#66396=CARTESIAN_POINT('Ctrl Pts',(0.00657516124656832,-0.0328657861914645,
0.0796874228824649));
#66397=CARTESIAN_POINT('Ctrl Pts',(0.00634849891012466,-0.0331951640388604,
0.0796205113348899));
#66398=CARTESIAN_POINT('Ctrl Pts',(0.00646159822460796,-0.0330306422010619,
0.0796572141785598));
#66399=CARTESIAN_POINT('Ctrl Pts',(0.00657611786364599,-0.0328657861914645,
0.0796892111463014));
#66400=CARTESIAN_POINT('Ctrl Pts',(0.00649544530550182,-0.0331951640388604,
0.07992481765778));
#66401=CARTESIAN_POINT('Ctrl Pts',(0.00661483595810781,-0.033030642201062,
0.0799584824789388));
#66402=CARTESIAN_POINT('Ctrl Pts',(0.00673551599469892,-0.0328657861914645,
0.0799871839925174));
#66403=CARTESIAN_POINT('',(0.00650778413364387,-0.0331781648281935,0.0799282826400012));
#66404=CARTESIAN_POINT('',(0.00649544530549579,-0.0331951640388588,0.0799248176577655));
#66405=CARTESIAN_POINT('Origin',(0.0102677027280972,-0.0326412092317192,
0.0638394822911415));
#66406=CARTESIAN_POINT('Ctrl Pts',(0.00650778413247788,-0.033178164828644,
0.0799282826385656));
#66407=CARTESIAN_POINT('Ctrl Pts',(0.00651936086246763,-0.0331276811546791,
0.0798868879783595));
#66408=CARTESIAN_POINT('Ctrl Pts',(0.00653072851999776,-0.0330765663497815,
0.0798462407684161));
#66409=CARTESIAN_POINT('Ctrl Pts',(0.0065530556131091,-0.0329730614463311,
0.0797664063696435));
#66410=CARTESIAN_POINT('Ctrl Pts',(0.00656400603419346,-0.0329207133374058,
0.0797272514336151));
#66411=CARTESIAN_POINT('Ctrl Pts',(0.00657475148424507,-0.0328677532289387,
0.0796888292114015));
#66412=CARTESIAN_POINT('',(0.00642197210782172,-0.0331951640388701,0.0797726644963382));
#66413=CARTESIAN_POINT('Origin',(0.00812378219310841,-0.0315241814719618,
0.07415));
#66414=CARTESIAN_POINT('',(0.00614815156877667,-0.0327114338380032,0.0798154111603605));
#66415=CARTESIAN_POINT('',(0.00616025749492682,-0.0326943950436593,0.0798196182199214));
#66416=CARTESIAN_POINT('Origin',(0.011525283954854,-0.0326395656488183,
0.0641055182638404));
#66417=CARTESIAN_POINT('Origin',(0.0116631949407086,-0.0326395684957492,
0.0641527893530563));
#66418=CARTESIAN_POINT('Origin',(0.0117057178917446,-0.0326395671683965,
0.0641684423746073));
#66419=CARTESIAN_POINT('Ctrl Pts',(0.005927605104244,-0.0330240426238172,
0.0797336194528622));
#66420=CARTESIAN_POINT('Ctrl Pts',(0.00600452490206404,-0.032914277406352,
0.079763873931893));
#66421=CARTESIAN_POINT('Ctrl Pts',(0.00608210849180188,-0.0328043479726691,
0.0797925533467991));
#66422=CARTESIAN_POINT('Ctrl Pts',(0.00616025749492681,-0.0326943950436593,
0.0798196182199214));
#66423=CARTESIAN_POINT('Ctrl Pts',(0.00602856685638832,-0.0330240426238172,
0.0796821620861541));
#66424=CARTESIAN_POINT('Ctrl Pts',(0.00610477777884947,-0.032914277406352,
0.0797110257186868));
#66425=CARTESIAN_POINT('Ctrl Pts',(0.00618162338714594,-0.0328043479726691,
0.079738328248141));
#66426=CARTESIAN_POINT('Ctrl Pts',(0.00625900619957894,-0.0326943950436593,
0.0797640319867867));
#66427=CARTESIAN_POINT('Ctrl Pts',(0.00612952860853264,-0.0330240426238172,
0.079630704719446));
#66428=CARTESIAN_POINT('Ctrl Pts',(0.00620503065563489,-0.0329142774063519,
0.0796581775054807));
#66429=CARTESIAN_POINT('Ctrl Pts',(0.00628113828249001,-0.0328043479726691,
0.0796841031494829));
#66430=CARTESIAN_POINT('Ctrl Pts',(0.00635775490423107,-0.0326943950436593,
0.0797084457536519));
#66431=CARTESIAN_POINT('Ctrl Pts',(0.00623049036067695,-0.0330240426238172,
0.079579247352738));
#66432=CARTESIAN_POINT('Ctrl Pts',(0.00630528353242032,-0.0329142774063519,
0.0796053292922745));
#66433=CARTESIAN_POINT('Ctrl Pts',(0.00638065317783408,-0.0328043479726691,
0.0796298780508248));
#66434=CARTESIAN_POINT('Ctrl Pts',(0.00645650360888319,-0.0326943950436593,
0.0796528595205172));
#66435=CARTESIAN_POINT('',(0.00630749699661392,-0.0326943950436693,0.0797367362287631));
#66436=CARTESIAN_POINT('Ctrl Pts',(0.00614815156986408,-0.0327114338383317,
0.0798154111572224));
#66437=CARTESIAN_POINT('Ctrl Pts',(0.00616229256985094,-0.0327619876831005,
0.079774859761553));
#66438=CARTESIAN_POINT('Ctrl Pts',(0.00617618409255887,-0.0328131562604407,
0.0797350237786449));
#66439=CARTESIAN_POINT('Ctrl Pts',(0.00620347987297984,-0.0329167375858766,
0.0796567491168115));
#66440=CARTESIAN_POINT('Ctrl Pts',(0.00621687325465107,-0.0329691088920625,
0.0796183416265345));
#66441=CARTESIAN_POINT('Ctrl Pts',(0.00623002218365494,-0.0330220786163187,
0.0795806351402068));
#66442=CARTESIAN_POINT('Origin',(0.00812378219310841,-0.0315241814719618,
0.07415));
#66443=CARTESIAN_POINT('',(0.0065077841346841,-0.0332121607144207,0.0799282826386817));
#66444=CARTESIAN_POINT('',(0.00652013033595562,-0.033195164038859,0.0799317212593731));
#66445=CARTESIAN_POINT('Origin',(0.0102225774597537,-0.0326413637773631,
0.063835002134874));
#66446=CARTESIAN_POINT('Origin',(0.0116395938759324,-0.032641210696683,
0.0642231517663572));
#66447=CARTESIAN_POINT('Origin',(0.0116804941341952,-0.032641365556836,
0.0642427376336306));
#66448=CARTESIAN_POINT('Ctrl Pts',(0.00642019835711451,-0.0337436976235975,
0.0796432619738859));
#66449=CARTESIAN_POINT('Ctrl Pts',(0.00646960558783428,-0.0336723290703325,
0.079658584265092));
#66450=CARTESIAN_POINT('Ctrl Pts',(0.00651928042535222,-0.033601104548885,
0.0796730153971601));
#66451=CARTESIAN_POINT('Ctrl Pts',(0.0066778823415161,-0.0333736987606857,
0.0797190911432073));
#66452=CARTESIAN_POINT('Ctrl Pts',(0.00683886698624801,-0.0331450831799192,
0.0797559894676301));
#66453=CARTESIAN_POINT('Ctrl Pts',(0.00666053244746381,-0.0337436976235975,
0.0797121061821823));
#66454=CARTESIAN_POINT('Ctrl Pts',(0.00671055887342662,-0.0336723290703325,
0.0797252668721563));
#66455=CARTESIAN_POINT('Ctrl Pts',(0.00676081392562346,-0.033601104548885,
0.0797375256153175));
#66456=CARTESIAN_POINT('Ctrl Pts',(0.00692126835232302,-0.0333736987606857,
0.0797766653539112));
#66457=CARTESIAN_POINT('Ctrl Pts',(0.00708370442669944,-0.0331450831799192,
0.0798065327931359));
#66458=CARTESIAN_POINT('Ctrl Pts',(0.0066629357883673,-0.0337436976235975,
0.0797127946242653));
#66459=CARTESIAN_POINT('Ctrl Pts',(0.00671296840628254,-0.0336723290703325,
0.0797259336982269));
#66460=CARTESIAN_POINT('Ctrl Pts',(0.00676322926062617,-0.033601104548885,
0.0797381707174991));
#66461=CARTESIAN_POINT('Ctrl Pts',(0.00692370221243109,-0.0333736987606857,
0.0797772410960182));
#66462=CARTESIAN_POINT('Ctrl Pts',(0.00708615280110395,-0.0331450831799192,
0.079807038226391));
#66463=CARTESIAN_POINT('',(0.00669549827498406,-0.0336938721132548,0.0797211874900445));
#66464=CARTESIAN_POINT('',(0.00692559412378843,-0.0333679870047995,0.0797751640287754));
#66465=CARTESIAN_POINT('Ctrl Pts',(0.00669549827497859,-0.033693872113252,
0.0797211874900436));
#66466=CARTESIAN_POINT('Ctrl Pts',(0.00671724523325145,-0.0336629187933862,
0.079726762752198));
#66467=CARTESIAN_POINT('Ctrl Pts',(0.00673901788172619,-0.0336319952301,
0.0797322088940652));
#66468=CARTESIAN_POINT('Ctrl Pts',(0.00676081392563053,-0.0336011045488914,
0.0797375256153195));
#66469=CARTESIAN_POINT('Ctrl Pts',(0.00681550765797378,-0.0335235892595418,
0.0797508670882265));
#66470=CARTESIAN_POINT('Ctrl Pts',(0.00687044592600969,-0.0334458668665535,
0.0797634171868114));
#66471=CARTESIAN_POINT('Ctrl Pts',(0.00692559411218311,-0.0333679869962459,
0.0797751640265497));
#66472=CARTESIAN_POINT('Ctrl Pts',(0.00692563746768464,-0.0333679692468944,
0.0797751739643015));
#66473=CARTESIAN_POINT('Ctrl Pts',(0.0069257260888849,-0.0333391895413371,
0.07977472946001));
#66474=CARTESIAN_POINT('Ctrl Pts',(0.00692578933029035,-0.0333104081127898,
0.0797743956474309));
#66475=CARTESIAN_POINT('Ctrl Pts',(0.00692586759951753,-0.0332532697859831,
0.079773952758113));
#66476=CARTESIAN_POINT('Ctrl Pts',(0.00692588332869693,-0.0332249169284244,
0.0797738404015532));
#66477=CARTESIAN_POINT('Ctrl Pts',(0.00692587734690751,-0.0331960985446588,
0.0797738353746939));
#66478=CARTESIAN_POINT('Ctrl Pts',(0.00692587724360892,-0.0331956312477754,
0.0797738353222659));
#66479=CARTESIAN_POINT('Ctrl Pts',(0.00692587713480589,-0.0331951640388594,
0.0797738352990903));
#66480=CARTESIAN_POINT('',(0.00680361984569412,-0.0331951640388587,0.0797477938847791));
#66481=CARTESIAN_POINT('',(0.00686474849025947,-0.0331951640388687,0.0797608145919446));
#66482=CARTESIAN_POINT('',(0.00657475148821477,-0.0335216366567667,0.0796888291967531));
#66483=CARTESIAN_POINT('Origin',(0.00988225669933695,-0.0326434571528327,
0.0633661126856979));
#66484=CARTESIAN_POINT('',(0.00657511738662483,-0.0336938721132327,0.0796875208638126));
#66485=CARTESIAN_POINT('Origin',(0.00363384684509192,-0.0336938867896251,
0.0902045431394953));
#66486=CARTESIAN_POINT('',(0.00663530783081445,-0.0336938721132537,0.0797043541769385));
#66487=CARTESIAN_POINT('Ctrl Pts',(0.00628253803905408,-0.0335235895815172,
0.0798605008506432));
#66488=CARTESIAN_POINT('Ctrl Pts',(0.00636115432620475,-0.0334144449262748,
0.0798858492014999));
#66489=CARTESIAN_POINT('Ctrl Pts',(0.00644038461179668,-0.0333049234473147,
0.0799096025212135));
#66490=CARTESIAN_POINT('Ctrl Pts',(0.00652013033595572,-0.0331951640388587,
0.0799317212593731));
#66491=CARTESIAN_POINT('Ctrl Pts',(0.00638006966083075,-0.0335235895815172,
0.0798028054848014));
#66492=CARTESIAN_POINT('Ctrl Pts',(0.00645789165767889,-0.0334144449262748,
0.0798268111208623));
#66493=CARTESIAN_POINT('Ctrl Pts',(0.00653629900094778,-0.0333049234473147,
0.0798492365926033));
#66494=CARTESIAN_POINT('Ctrl Pts',(0.00661519402924983,-0.0331951640388587,
0.0798700441428444));
#66495=CARTESIAN_POINT('Ctrl Pts',(0.00647760128260742,-0.0335235895815172,
0.0797451101189596));
#66496=CARTESIAN_POINT('Ctrl Pts',(0.00655462898915302,-0.0334144449262748,
0.0797677730402246));
#66497=CARTESIAN_POINT('Ctrl Pts',(0.00663221339009887,-0.0333049234473147,
0.0797888706639931));
#66498=CARTESIAN_POINT('Ctrl Pts',(0.00671025772254394,-0.0331951640388587,
0.0798083670263157));
#66499=CARTESIAN_POINT('Ctrl Pts',(0.00657513290438409,-0.0335235895815172,
0.0796874147531178));
#66500=CARTESIAN_POINT('Ctrl Pts',(0.00665136632062716,-0.0334144449262748,
0.079708734959587));
#66501=CARTESIAN_POINT('Ctrl Pts',(0.00672812777924997,-0.0333049234473147,
0.0797285047353828));
#66502=CARTESIAN_POINT('Ctrl Pts',(0.00680532141583805,-0.0331951640388587,
0.079746689909787));
#66503=CARTESIAN_POINT('',(0.00666187509083487,-0.0331951640388689,0.0798397575720862));
#66504=CARTESIAN_POINT('Ctrl Pts',(0.00650778413552333,-0.0332121607145972,
0.0799282826356574));
#66505=CARTESIAN_POINT('Ctrl Pts',(0.00651934140213031,-0.0332625444109758,
0.0798869576150997));
#66506=CARTESIAN_POINT('Ctrl Pts',(0.00653069951889734,-0.0333135300746838,
0.0798463446894959));
#66507=CARTESIAN_POINT('Ctrl Pts',(0.00655302646867632,-0.0334167203140557,
0.0797665107901856));
#66508=CARTESIAN_POINT('Ctrl Pts',(0.00656398665427754,-0.0334688847587232,
0.0797273207368029));
#66509=CARTESIAN_POINT('Ctrl Pts',(0.00657475148855615,-0.0335216366562301,
0.0796888291961133));
#66510=CARTESIAN_POINT('Ctrl Pts',(0.00669450368631926,-0.0336938721132516,
0.0797194206075927));
#66511=CARTESIAN_POINT('Ctrl Pts',(0.00672710335326963,-0.0336474569765021,
0.079727786648979));
#66512=CARTESIAN_POINT('Ctrl Pts',(0.00675979872154734,-0.033601104548885,
0.0797357704968567));
#66513=CARTESIAN_POINT('Ctrl Pts',(0.00684257587687882,-0.0334837508592655,
0.0797559837640789));
#66514=CARTESIAN_POINT('Ctrl Pts',(0.00692591564360106,-0.0333660264659097,
0.0797737352963861));
#66515=CARTESIAN_POINT('Ctrl Pts',(0.00669549827495535,-0.0336938721132516,
0.0797211874900371));
#66516=CARTESIAN_POINT('Ctrl Pts',(0.00672810828405499,-0.0336474569765021,
0.0797295477097661));
#66517=CARTESIAN_POINT('Ctrl Pts',(0.00676081392562346,-0.033601104548885,
0.0797375256153175));
#66518=CARTESIAN_POINT('Ctrl Pts',(0.00684361709056516,-0.0334837508592655,
0.0797577238379356));
#66519=CARTESIAN_POINT('Ctrl Pts',(0.00692698240967332,-0.0333660264659097,
0.0797754595615265));
#66520=CARTESIAN_POINT('Ctrl Pts',(0.00686225684122005,-0.0336938721132516,
0.0800174333674734));
#66521=CARTESIAN_POINT('Ctrl Pts',(0.00689660087574535,-0.0336474569765021,
0.0800248174939775));
#66522=CARTESIAN_POINT('Ctrl Pts',(0.00693102899751936,-0.033601104548885,
0.0800317990742297));
#66523=CARTESIAN_POINT('Ctrl Pts',(0.00701819308631786,-0.0334837508592655,
0.08004947483026));
#66524=CARTESIAN_POINT('Ctrl Pts',(0.00710584266837151,-0.0333660264659097,
0.0800645599717287));
#66525=CARTESIAN_POINT('',(0.00687379430618294,-0.0336769361243754,0.0800183498773113));
#66526=CARTESIAN_POINT('',(0.00686126225730294,-0.033693872113232,0.0800156664933913));
#66527=CARTESIAN_POINT('Ctrl Pts',(0.00687379430618319,-0.0336769361243751,
0.0800183498773114));
#66528=CARTESIAN_POINT('Ctrl Pts',(0.00687170499727109,-0.0336797586670031,
0.080017904844059));
#66529=CARTESIAN_POINT('Ctrl Pts',(0.00686961600504582,-0.0336825812712857,
0.0800174587118532));
#66530=CARTESIAN_POINT('Ctrl Pts',(0.00686543866504512,-0.03368822658797,
0.0800165642524324));
#66531=CARTESIAN_POINT('Ctrl Pts',(0.00686335031727572,-0.0336910493003646,
0.0800161159252534));
#66532=CARTESIAN_POINT('Ctrl Pts',(0.00686126225730768,-0.0336938721132377,
0.0800156664934046));
#66533=CARTESIAN_POINT('Ctrl Pts',(0.00687379430618294,-0.0336769361243754,
0.0800183498773113));
#66534=CARTESIAN_POINT('Ctrl Pts',(0.00688252605777871,-0.0336279018525375,
0.0799773567013441));
#66535=CARTESIAN_POINT('Ctrl Pts',(0.00689138342668254,-0.0335767826051552,
0.0799357737866078));
#66536=CARTESIAN_POINT('Ctrl Pts',(0.00690873878157675,-0.0334733172106835,
0.0798542951612311));
#66537=CARTESIAN_POINT('Ctrl Pts',(0.00691724843174461,-0.033420963147761,
0.0798143446904805));
#66538=CARTESIAN_POINT('Ctrl Pts',(0.00692559410938842,-0.0333679869844681,
0.0797751640257003));
#66539=CARTESIAN_POINT('',(0.00677838026615351,-0.0336938721132534,0.0798684269917279));
#66540=CARTESIAN_POINT('Origin',(0.00812378219310841,-0.0315241814719618,
0.07415));
#66541=CARTESIAN_POINT('',(0.00687379430645763,-0.0337108120655533,0.0800183498760507));
#66542=CARTESIAN_POINT('',(0.00688633205822611,-0.0336938721132327,0.080021006486431));
#66543=CARTESIAN_POINT('Origin',(0.0113754299909055,-0.0345562507997293,
0.0642489584326503));
#66544=CARTESIAN_POINT('Ctrl Pts',(0.00688633205822346,-0.0336938721132342,
0.080021006486434));
#66545=CARTESIAN_POINT('Ctrl Pts',(0.00688424210681475,-0.0336910493131789,
0.0800205659809332));
#66546=CARTESIAN_POINT('Ctrl Pts',(0.00688215232852207,-0.0336882265943771,
0.0800201243463767));
#66547=CARTESIAN_POINT('Ctrl Pts',(0.00687797308262314,-0.033682581271242,
0.080019238811193));
#66548=CARTESIAN_POINT('Ctrl Pts',(0.00687588361507858,-0.0336797586669812,
0.0800187949105602));
#66549=CARTESIAN_POINT('Ctrl Pts',(0.00687379430618269,-0.0336769361243751,
0.0800183498773113));
#66550=CARTESIAN_POINT('Origin',(0.00918926354515599,-0.0345562519797235,
0.0637832982217835));
#66551=CARTESIAN_POINT('Ctrl Pts',(0.00676843458054931,-0.034243627687391,
0.0797393790217815));
#66552=CARTESIAN_POINT('Ctrl Pts',(0.0069792414855517,-0.0339430054201809,
0.0797904967996763));
#66553=CARTESIAN_POINT('Ctrl Pts',(0.00719329991071649,-0.0336441434784052,
0.079825590517484));
#66554=CARTESIAN_POINT('Ctrl Pts',(0.00701261670866883,-0.034243627687391,
0.0797929988717162));
#66555=CARTESIAN_POINT('Ctrl Pts',(0.00722544591964964,-0.0339430054201809,
0.0798349071688289));
#66556=CARTESIAN_POINT('Ctrl Pts',(0.0074408272098064,-0.0336441434784052,
0.0798606652406512));
#66557=CARTESIAN_POINT('',(0.00704813442391549,-0.0341934961088741,0.079799876713401));
#66558=CARTESIAN_POINT('',(0.00728116543324923,-0.0338664212863488,0.0798392989023731));
#66559=CARTESIAN_POINT('Origin',(0.0106771194136505,-0.0345610720405296,
0.0634633038873715));
#66560=CARTESIAN_POINT('Origin',(0.00567456591739579,-0.0336938005072874,
0.0906872278499356));
#66561=CARTESIAN_POINT('',(0.00715771327076761,-0.0336938721132327,0.0798196415968991));
#66562=CARTESIAN_POINT('',(0.00721953886888336,-0.0336938721132427,0.0798287983113235));
#66563=CARTESIAN_POINT('',(0.00692559410938321,-0.0340203938281605,0.0797751640256991));
#66564=CARTESIAN_POINT('Origin',(0.0111251502442658,-0.0345589643244944,
0.0636388177300196));
#66565=CARTESIAN_POINT('',(0.00692587713480481,-0.034193496108874,0.07977383529909));
#66566=CARTESIAN_POINT('Origin',(0.00463018030827809,-0.0341934220717773,
0.0905514971227124));
#66567=CARTESIAN_POINT('',(0.00698700577937015,-0.034193496108884,0.0797868560062556));
#66568=CARTESIAN_POINT('Ctrl Pts',(0.00664473397720439,-0.0340223579322397,
0.0799648444841687));
#66569=CARTESIAN_POINT('Ctrl Pts',(0.00672493584839216,-0.0339125849573575,
0.0799852444165857));
#66570=CARTESIAN_POINT('Ctrl Pts',(0.00680550359385178,-0.0338030433565231,
0.0800039700218362));
#66571=CARTESIAN_POINT('Ctrl Pts',(0.00688633205822612,-0.0336938721132327,
0.080021006486431));
#66572=CARTESIAN_POINT('Ctrl Pts',(0.00673845047646088,-0.0340223579322397,
0.0799011389302705));
#66573=CARTESIAN_POINT('Ctrl Pts',(0.00681777368190933,-0.0339125849573575,
0.0799202462677398));
#66574=CARTESIAN_POINT('Ctrl Pts',(0.00689743662534604,-0.0338030433565231,
0.0799376983726733));
#66575=CARTESIAN_POINT('Ctrl Pts',(0.00697733545287098,-0.0336938721132327,
0.0799534819576028));
#66576=CARTESIAN_POINT('Ctrl Pts',(0.00683216697571736,-0.0340223579322397,
0.0798374333763723));
#66577=CARTESIAN_POINT('Ctrl Pts',(0.0069106115154265,-0.0339125849573575,
0.079855248118894));
#66578=CARTESIAN_POINT('Ctrl Pts',(0.00698936965684029,-0.0338030433565231,
0.0798714267235104));
#66579=CARTESIAN_POINT('Ctrl Pts',(0.00706833884751585,-0.0336938721132327,
0.0798859574287746));
#66580=CARTESIAN_POINT('Ctrl Pts',(0.00692588347497385,-0.0340223579322397,
0.0797737278224742));
#66581=CARTESIAN_POINT('Ctrl Pts',(0.00700344934894367,-0.0339125849573575,
0.0797902499700482));
#66582=CARTESIAN_POINT('Ctrl Pts',(0.00708130268833455,-0.0338030433565231,
0.0798051550743475));
#66583=CARTESIAN_POINT('Ctrl Pts',(0.00715934224216072,-0.0336938721132327,
0.0798184328999464));
#66584=CARTESIAN_POINT('',(0.00702202266450686,-0.0336938721132427,0.079920324041675));
#66585=CARTESIAN_POINT('Ctrl Pts',(0.00687379430720368,-0.0337108120662689,
0.0800183498725188));
#66586=CARTESIAN_POINT('Ctrl Pts',(0.00688275239876129,-0.0337611408994256,
0.0799762940925845));
#66587=CARTESIAN_POINT('Ctrl Pts',(0.00689154702502222,-0.0338121088781224,
0.0799350057373299));
#66588=CARTESIAN_POINT('Ctrl Pts',(0.00690881735871832,-0.0339153382773237,
0.0798539262631313));
#66589=CARTESIAN_POINT('Ctrl Pts',(0.00691728575974262,-0.0339675558473116,
0.07981416944578));
#66590=CARTESIAN_POINT('Ctrl Pts',(0.00692559410939671,-0.0340203938281304,
0.0797751640256612));
#66591=CARTESIAN_POINT('Ctrl Pts',(0.00704703054551019,-0.0341934961088741,
0.0797981752921274));
#66592=CARTESIAN_POINT('Ctrl Pts',(0.00716380211997548,-0.0340287516182428,
0.0798204362841637));
#66593=CARTESIAN_POINT('Ctrl Pts',(0.00728139397905306,-0.0338644633275951,
0.0798378519968459));
#66594=CARTESIAN_POINT('Ctrl Pts',(0.00704813442391546,-0.0341934961088741,
0.079799876713401));
#66595=CARTESIAN_POINT('Ctrl Pts',(0.00716494117392518,-0.0340287516182428,
0.0798221148836209));
#66596=CARTESIAN_POINT('Ctrl Pts',(0.00728256723524739,-0.0338644633275951,
0.0798395063401556));
#66597=CARTESIAN_POINT('Ctrl Pts',(0.00723206179851671,-0.0341934961088741,
0.0800833662231507));
#66598=CARTESIAN_POINT('Ctrl Pts',(0.00735472947080411,-0.0340287516182428,
0.0801018018398009));
#66599=CARTESIAN_POINT('Ctrl Pts',(0.00747805428393412,-0.0338644633275951,
0.080115151755611));
#66600=CARTESIAN_POINT('',(0.00724473760860792,-0.0341764758832429,0.0800852574172649));
#66601=CARTESIAN_POINT('',(0.00723206179850727,-0.034193496108874,0.0800833662231361));
#66602=CARTESIAN_POINT('Origin',(0.0101771442443428,-0.0345621026889891,
0.0637811990244643));
#66603=CARTESIAN_POINT('Ctrl Pts',(0.00724473760714494,-0.0341764758837536,
0.0800852574161694));
#66604=CARTESIAN_POINT('Ctrl Pts',(0.0072510263338492,-0.0341260050040345,
0.0800427962089692));
#66605=CARTESIAN_POINT('Ctrl Pts',(0.00725720570985234,-0.0340749269147931,
0.0800010730721234));
#66606=CARTESIAN_POINT('Ctrl Pts',(0.00726935073097967,-0.0339715436305673,
0.0799190706301537));
#66607=CARTESIAN_POINT('Ctrl Pts',(0.00727531177446978,-0.0339192778236826,
0.0798788224358291));
#66608=CARTESIAN_POINT('Ctrl Pts',(0.00728116543122125,-0.0338664212854931,
0.079839298903217));
#66609=CARTESIAN_POINT('',(0.00714009811122139,-0.0341934961088841,0.0799416214682786));
#66610=CARTESIAN_POINT('Origin',(0.00812378219310841,-0.0315241814719618,
0.07415));
#66611=CARTESIAN_POINT('',(0.00724473760954819,-0.0342105180190349,0.0800852574166593));
#66612=CARTESIAN_POINT('',(0.00725741743084159,-0.034193496108874,0.0800871215330949));
#66613=CARTESIAN_POINT('Origin',(0.0101333719713516,-0.034562169737374,
0.0637694223670492));
#66614=CARTESIAN_POINT('Origin',(0.00916399607309383,-0.0345621043777391,
0.063631142614299));
#66615=CARTESIAN_POINT('Origin',(0.00920930196589667,-0.0345621711700108,
0.0636325666787368));
#66616=CARTESIAN_POINT('Ctrl Pts',(0.00715622944660961,-0.0346945769586966,
0.079819421834301));
#66617=CARTESIAN_POINT('Ctrl Pts',(0.00727497775684171,-0.0345275153362944,
0.0798396876139634));
#66618=CARTESIAN_POINT('Ctrl Pts',(0.00739439412158621,-0.0343603235965185,
0.0798562241103379));
#66619=CARTESIAN_POINT('Ctrl Pts',(0.00751412463335077,-0.034193496108874,
0.0798689876649925));
#66620=CARTESIAN_POINT('Ctrl Pts',(0.00723915818567159,-0.0346945769586966,
0.0798317040410828));
#66621=CARTESIAN_POINT('Ctrl Pts',(0.00735816375164226,-0.0345275153362944,
0.0798502328451027));
#66622=CARTESIAN_POINT('Ctrl Pts',(0.00747778281237967,-0.0343603235965185,
0.0798650238261077));
#66623=CARTESIAN_POINT('Ctrl Pts',(0.00759766093763429,-0.034193496108874,
0.0798760384970352));
#66624=CARTESIAN_POINT('Ctrl Pts',(0.0073220869247337,-0.0346945769586966,
0.0798439862478629));
#66625=CARTESIAN_POINT('Ctrl Pts',(0.0074413497464428,-0.0345275153362944,
0.0798607780762401));
#66626=CARTESIAN_POINT('Ctrl Pts',(0.00756117150317306,-0.0343603235965185,
0.0798738235418762));
#66627=CARTESIAN_POINT('Ctrl Pts',(0.00768119724191778,-0.034193496108874,
0.079883089329078));
#66628=CARTESIAN_POINT('Ctrl Pts',(0.00740501566379556,-0.0346945769586966,
0.0798562684546465));
#66629=CARTESIAN_POINT('Ctrl Pts',(0.00752453574124338,-0.0345275153362944,
0.0798713233073814));
#66630=CARTESIAN_POINT('Ctrl Pts',(0.00764456019396659,-0.0343603235965185,
0.0798826232576472));
#66631=CARTESIAN_POINT('Ctrl Pts',(0.00776473354620134,-0.034193496108874,
0.0798901401611205));
#66632=CARTESIAN_POINT('',(0.00740501566319633,-0.0346945769586966,0.0798562684545576));
#66633=CARTESIAN_POINT('',(0.0076400621771997,-0.0343667727831673,0.0798809807142107));
#66634=CARTESIAN_POINT('Origin',(0.00932461120802878,-0.0345626457063345,
0.0631526041805093));
#66635=CARTESIAN_POINT('Origin',(0.00671051934626394,-0.0341934771029274,
0.0908940004869859));
#66636=CARTESIAN_POINT('',(0.00751561932852272,-0.034193496108874,0.0798691138238489));
#66637=CARTESIAN_POINT('',(0.0075778978827986,-0.034193496108884,0.0798743704081639));
#66638=CARTESIAN_POINT('',(0.00728116543148868,-0.034521194296263,0.0798392989017116));
#66639=CARTESIAN_POINT('Origin',(0.00979974754044332,-0.0345625596120374,
0.0632263351489356));
#66640=CARTESIAN_POINT('',(0.00728136446697915,-0.0346945769586885,0.0798379550257279));
#66641=CARTESIAN_POINT('Origin',(0.00566046893509098,-0.0346945685854079,
0.0907821412878401));
#66642=CARTESIAN_POINT('',(0.00734319006509773,-0.0346945769587026,0.0798471117401527));
#66643=CARTESIAN_POINT('Ctrl Pts',(0.00701277059268193,-0.0345231616327842,
0.0800462406009045));
#66644=CARTESIAN_POINT('Ctrl Pts',(0.00709404196812263,-0.0344132092796988,
0.0800615543316371));
#66645=CARTESIAN_POINT('Ctrl Pts',(0.00717562590277485,-0.034303273855898,
0.0800751862379566));
#66646=CARTESIAN_POINT('Ctrl Pts',(0.00725741743084155,-0.034193496108874,
0.0800871215330949));
#66647=CARTESIAN_POINT('Ctrl Pts',(0.00710230189555469,-0.0345231616327842,
0.0799767763515059));
#66648=CARTESIAN_POINT('Ctrl Pts',(0.00718261580411526,-0.0344132092796988,
0.0799908560192784));
#66649=CARTESIAN_POINT('Ctrl Pts',(0.00726321679566934,-0.034303273855898,
0.080003273730757));
#66650=CARTESIAN_POINT('Ctrl Pts',(0.00734400120352891,-0.034193496108874,
0.0800140162224409));
#66651=CARTESIAN_POINT('Ctrl Pts',(0.00719183319842744,-0.0345231616327842,
0.0799073121021073));
#66652=CARTESIAN_POINT('Ctrl Pts',(0.0072711896401079,-0.0344132092796988,
0.0799201577069198));
#66653=CARTESIAN_POINT('Ctrl Pts',(0.00735080768856383,-0.034303273855898,
0.0799313612235574));
#66654=CARTESIAN_POINT('Ctrl Pts',(0.00743058497621627,-0.034193496108874,
0.0799409109117868));
#66655=CARTESIAN_POINT('Ctrl Pts',(0.00728136450130019,-0.0345231616327842,
0.0798378478527087));
#66656=CARTESIAN_POINT('Ctrl Pts',(0.00735976347610053,-0.0344132092796988,
0.079849459394561));
#66657=CARTESIAN_POINT('Ctrl Pts',(0.00743839858145832,-0.034303273855898,
0.0798594487163577));
#66658=CARTESIAN_POINT('Ctrl Pts',(0.00751716874890363,-0.034193496108874,
0.0798678056011328));
#66659=CARTESIAN_POINT('',(0.00738651837969215,-0.0341934961088839,0.0799781176784819));
#66660=CARTESIAN_POINT('Ctrl Pts',(0.00724473761004957,-0.0342105180195384,
0.0800852574132335));
#66661=CARTESIAN_POINT('Ctrl Pts',(0.00725103342009984,-0.0342610556241179,
0.0800427484734217));
#66662=CARTESIAN_POINT('Ctrl Pts',(0.00725721625509396,-0.0343122189869899,
0.0800010023345559));
#66663=CARTESIAN_POINT('Ctrl Pts',(0.00726936139472658,-0.0344158119695101,
0.0799189990648373));
#66664=CARTESIAN_POINT('Ctrl Pts',(0.00727531873191037,-0.0344681990449985,
0.079878775473947));
#66665=CARTESIAN_POINT('Ctrl Pts',(0.00728116543148774,-0.0345211942962392,
0.0798392989016795));
#66666=CARTESIAN_POINT('Ctrl Pts',(0.00740380742581461,-0.0346945769586932,
0.0798546401025433));
#66667=CARTESIAN_POINT('Ctrl Pts',(0.00748242024987177,-0.034584662917547,
0.079864561718752));
#66668=CARTESIAN_POINT('Ctrl Pts',(0.00756125167614127,-0.0344746925049099,
0.0798728593486793));
#66669=CARTESIAN_POINT('Ctrl Pts',(0.00764020065280731,-0.034364806625142,
0.0798795227775937));
#66670=CARTESIAN_POINT('Ctrl Pts',(0.00747133180145219,-0.0346945769586932,
0.0799456432907319));
#66671=CARTESIAN_POINT('Ctrl Pts',(0.00755119869544069,-0.034584662917547,
0.0799546343869138));
#66672=CARTESIAN_POINT('Ctrl Pts',(0.00763126516306773,-0.0344746925049099,
0.0799619754042279));
#66673=CARTESIAN_POINT('Ctrl Pts',(0.00771142857510226,-0.034364806625142,
0.0799676573602005));
#66674=CARTESIAN_POINT('Ctrl Pts',(0.00753885617708977,-0.0346945769586932,
0.0800366464789205));
#66675=CARTESIAN_POINT('Ctrl Pts',(0.00761997714100961,-0.034584662917547,
0.0800447070550755));
#66676=CARTESIAN_POINT('Ctrl Pts',(0.00770127864999419,-0.0344746925049099,
0.0800510914597765));
#66677=CARTESIAN_POINT('Ctrl Pts',(0.00778265649739722,-0.034364806625142,
0.0800557919428073));
#66678=CARTESIAN_POINT('Ctrl Pts',(0.00760638055272735,-0.0346945769586932,
0.0801276496671091));
#66679=CARTESIAN_POINT('Ctrl Pts',(0.00768875558657853,-0.034584662917547,
0.0801347797232373));
#66680=CARTESIAN_POINT('Ctrl Pts',(0.00777129213692066,-0.0344746925049099,
0.0801402075153251));
#66681=CARTESIAN_POINT('Ctrl Pts',(0.00785388441969217,-0.034364806625142,
0.0801439265254142));
#66682=CARTESIAN_POINT('',(0.00761915009997584,-0.0346775396663668,0.0801287412079197));
#66683=CARTESIAN_POINT('',(0.00760638055272025,-0.0346945769586886,0.0801276496670952));
#66684=CARTESIAN_POINT('Origin',(0.00886319787775422,-0.0345626617929341,
0.0635738250497379));
#66685=CARTESIAN_POINT('Ctrl Pts',(0.00761915010025431,-0.0346775396659514,
0.0801287412045515));
#66686=CARTESIAN_POINT('Ctrl Pts',(0.00762276312447797,-0.0346269748529709,
0.0800859350947044));
#66687=CARTESIAN_POINT('Ctrl Pts',(0.0076263119077185,-0.0345757904818262,
0.0800438900942244));
#66688=CARTESIAN_POINT('Ctrl Pts',(0.00763328403561633,-0.0344721679344123,
0.0799612862548403));
#66689=CARTESIAN_POINT('Ctrl Pts',(0.00763670457075407,-0.0344197716859653,
0.0799207607023451));
#66690=CARTESIAN_POINT('Ctrl Pts',(0.00764006217696968,-0.0343667727830994,
0.0798809807142818));
#66691=CARTESIAN_POINT('',(0.00750569810796829,-0.0346945769587026,0.0799919590608363));
#66692=CARTESIAN_POINT('Origin',(0.00812378219310841,-0.0315241814719618,
0.07415));
#66693=CARTESIAN_POINT('',(0.00761915009998483,-0.0347116136489593,0.0801287412078104));
#66694=CARTESIAN_POINT('',(0.00763192194936935,-0.0346945769586885,0.0801298054734804));
#66695=CARTESIAN_POINT('Origin',(0.00881792530718465,-0.0345626673615202,
0.0635718759458564));
#66696=CARTESIAN_POINT('Origin',(0.00916754804003983,-0.0345626633401097,
0.0635995098234622));
#66697=CARTESIAN_POINT('Origin',(0.00921250601583,-0.0345626690505617,0.0636051839189239));
#66698=CARTESIAN_POINT('Ctrl Pts',(0.00747724508128081,-0.0352450361874068,
0.0798649580937247));
#66699=CARTESIAN_POINT('Ctrl Pts',(0.00769278826268485,-0.0349452760959492,
0.0798893426410291));
#66700=CARTESIAN_POINT('Ctrl Pts',(0.00790955585247625,-0.034644428984174,
0.0798974223200474));
#66701=CARTESIAN_POINT('Ctrl Pts',(0.00747973485464712,-0.0352450361874068,
0.0798651839887987));
#66702=CARTESIAN_POINT('Ctrl Pts',(0.00769528655582368,-0.0349452760959492,
0.0798894746327597));
#66703=CARTESIAN_POINT('Ctrl Pts',(0.00791205556799978,-0.034644428984174,
0.07989746003346));
#66704=CARTESIAN_POINT('Ctrl Pts',(0.00772871219127743,-0.0352450361874068,
0.0798877734961964));
#66705=CARTESIAN_POINT('Ctrl Pts',(0.00794511586970579,-0.0349452760959492,
0.0799026738058181));
#66706=CARTESIAN_POINT('Ctrl Pts',(0.00816202712035146,-0.034644428984174,
0.079901231374718));
#66707=CARTESIAN_POINT('Ctrl Pts',(0.0077312268623774,-0.0352450361874068,
0.0798880016502211));
#66708=CARTESIAN_POINT('Ctrl Pts',(0.007947639145776,-0.0349452760959492,
0.079902807117466));
#66709=CARTESIAN_POINT('Ctrl Pts',(0.00816455183303021,-0.034644428984174,
0.0799012694652647));
#66710=CARTESIAN_POINT('',(0.0077647011018514,-0.0351951634053305,0.0798901405098147));
#66711=CARTESIAN_POINT('',(0.00800086794471331,-0.0348678972939192,0.0799000449641624));
#66712=CARTESIAN_POINT('Origin',(0.00793593353284433,-0.0345628965658585,
0.0631458627386298));
#66713=CARTESIAN_POINT('Origin',(0.00776473386622734,-0.0346946199326787,
0.0909473631118738));
#66714=CARTESIAN_POINT('',(0.00787592550929624,-0.0346945769330289,0.079896015320419));
#66715=CARTESIAN_POINT('',(0.00793841124341285,-0.0346945769458128,0.0798973510298189));
#66716=CARTESIAN_POINT('',(0.00764006217696069,-0.0350221583435276,0.0798809807141517));
#66717=CARTESIAN_POINT('Origin',(0.00841677757682629,-0.0345628458716598,
0.0631145062762775));
#66718=CARTESIAN_POINT('',(0.00764016319169323,-0.0351951360298762,0.0798797479575789));
#66719=CARTESIAN_POINT('Origin',(0.00671341033859371,-0.0351951838366723,
0.0908596829756913));
#66720=CARTESIAN_POINT('',(0.00776473354557716,-0.0351951371328746,0.0798901401611844));
#66721=CARTESIAN_POINT('Ctrl Pts',(0.00738519188429683,-0.0350241211494343,
0.080104366830803));
#66722=CARTESIAN_POINT('Ctrl Pts',(0.00746721084600568,-0.0349144232818962,
0.0801145406094731));
#66723=CARTESIAN_POINT('Ctrl Pts',(0.00754948919929143,-0.0348045283579412,
0.0801230250870939));
#66724=CARTESIAN_POINT('Ctrl Pts',(0.00763192196044475,-0.0346945769439158,
0.0801298054743914));
#66725=CARTESIAN_POINT('Ctrl Pts',(0.00747018482803159,-0.0350241211494343,
0.0800294179060719));
#66726=CARTESIAN_POINT('Ctrl Pts',(0.00755117139903253,-0.0349144232818962,
0.0800384209417905));
#66727=CARTESIAN_POINT('Ctrl Pts',(0.00763239254358138,-0.0348045283579412,
0.0800457553159674));
#66728=CARTESIAN_POINT('Ctrl Pts',(0.00771374457730006,-0.0346945769439158,
0.0800514077628559));
#66729=CARTESIAN_POINT('Ctrl Pts',(0.00755517777176635,-0.0350241211494343,
0.0799544689813407));
#66730=CARTESIAN_POINT('Ctrl Pts',(0.00763513195205937,-0.0349144232818962,
0.0799623012741078));
#66731=CARTESIAN_POINT('Ctrl Pts',(0.00771529588787134,-0.0348045283579412,
0.0799684855448408));
#66732=CARTESIAN_POINT('Ctrl Pts',(0.00779556719415537,-0.0346945769439158,
0.0799730100513204));
#66733=CARTESIAN_POINT('Ctrl Pts',(0.00764017071550111,-0.0350241211494343,
0.0798795200566096));
#66734=CARTESIAN_POINT('Ctrl Pts',(0.00771909250508621,-0.0349144232818962,
0.0798861816064252));
#66735=CARTESIAN_POINT('Ctrl Pts',(0.00779819923216129,-0.0348045283579412,
0.0798912157737143));
#66736=CARTESIAN_POINT('Ctrl Pts',(0.00787738981101069,-0.0346945769439158,
0.079894612339785));
#66737=CARTESIAN_POINT('',(0.00775392372904227,-0.0346945769458128,0.080012910397025));
#66738=CARTESIAN_POINT('Ctrl Pts',(0.00761915010025643,-0.034711613649279,
0.0801287412045252));
#66739=CARTESIAN_POINT('Ctrl Pts',(0.00762276167853553,-0.0347621546532138,
0.0800859522258283));
#66740=CARTESIAN_POINT('Ctrl Pts',(0.00762630975550902,-0.03481330840967,
0.0800439155930049));
#66741=CARTESIAN_POINT('Ctrl Pts',(0.00763328186796119,-0.0349168561544569,
0.0799613119366169));
#66742=CARTESIAN_POINT('Ctrl Pts',(0.00763670313795349,-0.0349692089015916,
0.0799207776777686));
#66743=CARTESIAN_POINT('Ctrl Pts',(0.00764006217698359,-0.0350221583435,
0.0798809807141169));
#66744=CARTESIAN_POINT('Ctrl Pts',(0.00776378970930018,-0.0351951371254924,
0.0798890223092295));
#66745=CARTESIAN_POINT('Ctrl Pts',(0.0078428252849622,-0.0350856248738962,
0.0798939799852341));
#66746=CARTESIAN_POINT('Ctrl Pts',(0.00792202819928413,-0.0349758427086608,
0.0798973083633598));
#66747=CARTESIAN_POINT('Ctrl Pts',(0.00800129730473024,-0.0348659306906667,
0.0798989972261563));
#66748=CARTESIAN_POINT('Ctrl Pts',(0.00781683363617358,-0.0351951371254924,
0.079951845970955));
#66749=CARTESIAN_POINT('Ctrl Pts',(0.00789673439478874,-0.0350856248738962,
0.0799560731466983));
#66750=CARTESIAN_POINT('Ctrl Pts',(0.00797678810562306,-0.0349758427086608,
0.0799586525448041));
#66751=CARTESIAN_POINT('Ctrl Pts',(0.00805689247560053,-0.0348659306906667,
0.0799595748427044));
#66752=CARTESIAN_POINT('Ctrl Pts',(0.00786987756304698,-0.0351951371254924,
0.0800146696326804));
#66753=CARTESIAN_POINT('Ctrl Pts',(0.00795064350461529,-0.0350856248738962,
0.0800181663081626));
#66754=CARTESIAN_POINT('Ctrl Pts',(0.008031548011962,-0.0349758427086608,
0.0800199967262483));
#66755=CARTESIAN_POINT('Ctrl Pts',(0.00811248764647081,-0.0348659306906667,
0.0800201524592524));
#66756=CARTESIAN_POINT('Ctrl Pts',(0.00792292148992038,-0.0351951371254924,
0.0800774932944058));
#66757=CARTESIAN_POINT('Ctrl Pts',(0.00800455261444184,-0.0350856248738962,
0.0800802594696268));
#66758=CARTESIAN_POINT('Ctrl Pts',(0.00808630791830094,-0.0349758427086608,
0.0800813409076926));
#66759=CARTESIAN_POINT('Ctrl Pts',(0.0081680828173411,-0.0348659306906667,
0.0800807300758005));
#66760=CARTESIAN_POINT('Origin',(0.00788721294704829,-0.0308609188508779,
0.0852170131853622));
#66761=CARTESIAN_POINT('',(0.00783369992264697,-0.0351951371254924,0.0799718219029499));
#66762=CARTESIAN_POINT('Origin',(0.00800290361662291,-0.035184046744755,
0.0731803948590619));
#66763=CARTESIAN_POINT('Origin',(0.00866315573714708,-0.0352322612474718,
0.0861032743007049));
#66764=CARTESIAN_POINT('',(0.00823752392040189,-0.0351951142564675,0.0799002067269712));
#66765=CARTESIAN_POINT('',(0.00836210254579337,-0.0351951372916786,0.0798950590431689));
#66766=CARTESIAN_POINT('Origin',(0.00840618459976702,-0.0352875121144073,
0.0739596041588875));
#66767=CARTESIAN_POINT('Origin',(0.000706367619496166,-0.0298325076522946,
0.0730198888008274));
#66768=CARTESIAN_POINT('Origin',(0.00529310284598232,-0.0338731063892672,
0.0820393710964081));
#66769=CARTESIAN_POINT('Ctrl Pts',(0.00483560513139321,-0.0321934096636941,
0.0788686891565478));
#66770=CARTESIAN_POINT('Ctrl Pts',(0.0049200674202468,-0.0320508460843909,
0.0789275459601164));
#66771=CARTESIAN_POINT('Ctrl Pts',(0.00500604739043419,-0.0319086045662242,
0.0789840890504166));
#66772=CARTESIAN_POINT('Ctrl Pts',(0.00509334988896869,-0.0317669892866659,
0.0790382119212771));
#66773=CARTESIAN_POINT('Ctrl Pts',(0.00490542372789669,-0.0321934096636941,
0.0789151197090981));
#66774=CARTESIAN_POINT('Ctrl Pts',(0.00499071710153061,-0.0320508460843909,
0.0789727267930371));
#66775=CARTESIAN_POINT('Ctrl Pts',(0.00507749395235713,-0.0319086045662242,
0.0790279987763921));
#66776=CARTESIAN_POINT('Ctrl Pts',(0.00516555763688526,-0.0317669892866659,
0.0790808320311662));
#66777=CARTESIAN_POINT('Ctrl Pts',(0.00497524232440018,-0.0321934096636941,
0.0789615502616486));
#66778=CARTESIAN_POINT('Ctrl Pts',(0.00506136678281444,-0.0320508460843909,
0.0790179076259579));
#66779=CARTESIAN_POINT('Ctrl Pts',(0.00514894051428005,-0.0319086045662242,
0.0790719085023677));
#66780=CARTESIAN_POINT('Ctrl Pts',(0.00523776538480183,-0.0317669892866659,
0.0791234521410554));
#66781=CARTESIAN_POINT('Ctrl Pts',(0.00504506092090366,-0.0321934096636941,
0.079007980814199));
#66782=CARTESIAN_POINT('Ctrl Pts',(0.00513201646409826,-0.0320508460843909,
0.0790630884588786));
#66783=CARTESIAN_POINT('Ctrl Pts',(0.00522038707620298,-0.0319086045662242,
0.0791158182283434));
#66784=CARTESIAN_POINT('Ctrl Pts',(0.0053099731327184,-0.0317669892866659,
0.0791660722509446));
#66785=CARTESIAN_POINT('',(0.00504381185241653,-0.0321934096636941,0.0790071501624367));
#66786=CARTESIAN_POINT('',(0.00524596632873056,-0.0318665617511322,0.0791295884207342));
#66787=CARTESIAN_POINT('Origin',(0.0145055280571824,-0.0326371944419857,
0.0652342117938775));
#66788=CARTESIAN_POINT('Origin',(-0.000238698541601191,-0.0316939261508872,
0.0886199014530148));
#66789=CARTESIAN_POINT('',(0.00493921987219606,-0.0320197221621748,0.0789391702820801));
#66790=CARTESIAN_POINT('Ctrl Pts',(0.00493934267991975,-0.0320197392094669,
0.0789393086046855));
#66791=CARTESIAN_POINT('Ctrl Pts',(0.00496371224781349,-0.0319792716575967,
0.0789555120176116));
#66792=CARTESIAN_POINT('Ctrl Pts',(0.00498831628355511,-0.0319386439829624,
0.0789716034108641));
#66793=CARTESIAN_POINT('Ctrl Pts',(0.00501318524593401,-0.0318979099381556,
0.0789875925992203));
#66794=CARTESIAN_POINT('Ctrl Pts',(0.00503805371675908,-0.031857176698488,
0.0790035814715382));
#66795=CARTESIAN_POINT('Ctrl Pts',(0.00506305974239178,-0.0318163871833551,
0.0790193883757689));
#66796=CARTESIAN_POINT('Ctrl Pts',(0.00508811543097495,-0.0317755399638303,
0.0790349619190384));
#66797=CARTESIAN_POINT('',(0.0049397263837213,-0.0321934096636185,0.0789379315578555));
#66798=CARTESIAN_POINT('Origin',(0.0036795163241933,-0.0324111462521584,
0.0808709034511289));
#66799=CARTESIAN_POINT('',(0.00499176911807891,-0.0321934096636663,0.0789725408601561));
#66800=CARTESIAN_POINT('Ctrl Pts',(0.005043411812262,-0.0321934096636618,
0.079005161782379));
#66801=CARTESIAN_POINT('Ctrl Pts',(0.0051103682771328,-0.0320835708272592,
0.0790476424906311));
#66802=CARTESIAN_POINT('Ctrl Pts',(0.00517816504058231,-0.0319739230346488,
0.0790887128977855));
#66803=CARTESIAN_POINT('Ctrl Pts',(0.0052467113285401,-0.0318646057455572,
0.0791283271142545));
#66804=CARTESIAN_POINT('Ctrl Pts',(0.00506576245863784,-0.0321934096636618,
0.0791162545966029));
#66805=CARTESIAN_POINT('Ctrl Pts',(0.00513425097999746,-0.0320835708272592,
0.0791584270720224));
#66806=CARTESIAN_POINT('Ctrl Pts',(0.00520357253241831,-0.0319739230346488,
0.0791991577193024));
#66807=CARTESIAN_POINT('Ctrl Pts',(0.00527363442433022,-0.0318646057455572,
0.0792384012332775));
#66808=CARTESIAN_POINT('Ctrl Pts',(0.00508811310501367,-0.0321934096636617,
0.0792273474108269));
#66809=CARTESIAN_POINT('Ctrl Pts',(0.00515813368286211,-0.0320835708272592,
0.0792692116534138));
#66810=CARTESIAN_POINT('Ctrl Pts',(0.00522898002425432,-0.0319739230346488,
0.0793096025408193));
#66811=CARTESIAN_POINT('Ctrl Pts',(0.00530055752012034,-0.0318646057455572,
0.0793484753523005));
#66812=CARTESIAN_POINT('Ctrl Pts',(0.0051104637513895,-0.0321934096636617,
0.0793384402250508));
#66813=CARTESIAN_POINT('Ctrl Pts',(0.00518201638572676,-0.0320835708272592,
0.0793799962348052));
#66814=CARTESIAN_POINT('Ctrl Pts',(0.00525438751609032,-0.0319739230346488,
0.0794200473623362));
#66815=CARTESIAN_POINT('Ctrl Pts',(0.00532748061591046,-0.0318646057455572,
0.0794585494713235));
#66816=CARTESIAN_POINT('',(0.00512155322786208,-0.0321763980308309,0.0793448648892966));
#66817=CARTESIAN_POINT('',(0.00511046375141491,-0.0321934096636184,0.0793384402250532));
#66818=CARTESIAN_POINT('Origin',(0.0139270308064902,-0.0326386230501741,
0.0653345240239085));
#66819=CARTESIAN_POINT('Ctrl Pts',(0.00512155322944348,-0.0321763980306358,
0.0793448648865458));
#66820=CARTESIAN_POINT('Ctrl Pts',(0.00514302862021074,-0.032125959617624,
0.0793077052445692));
#66821=CARTESIAN_POINT('Ctrl Pts',(0.00516413192196313,-0.0320749164634223,
0.0792711894416004));
#66822=CARTESIAN_POINT('Ctrl Pts',(0.0052056113309264,-0.0319716057793972,
0.0791994161265915));
#66823=CARTESIAN_POINT('Ctrl Pts',(0.00522597127620166,-0.0319193786690153,
0.0791641865801306));
#66824=CARTESIAN_POINT('Ctrl Pts',(0.00524596632965145,-0.0318665617525372,
0.0791295884191216));
#66825=CARTESIAN_POINT('',(0.00507713780192571,-0.0321934096636663,0.079172795193755));
#66826=CARTESIAN_POINT('Origin',(0.00812378219310841,-0.0315241814719618,
0.07415));
#66827=CARTESIAN_POINT('',(0.00512155322767646,-0.0322104233323594,0.0793448648896169));
#66828=CARTESIAN_POINT('',(0.00513265640034521,-0.0321934096636183,0.0793512658547612));
#66829=CARTESIAN_POINT('Origin',(0.0138913242442269,-0.0326387223796466,
0.0653065885275257));
#66830=CARTESIAN_POINT('Origin',(0.0128646762507391,-0.0326386249609679,
0.0647205611477657));
#66831=CARTESIAN_POINT('Origin',(0.0129067043389715,-0.0326387238634907,
0.0647375594113493));
#66832=CARTESIAN_POINT('Ctrl Pts',(0.00510758521549168,-0.0327445246967097,
0.0790470073302188));
#66833=CARTESIAN_POINT('Ctrl Pts',(0.00529227886628301,-0.032443687833936,
0.0791607650589165));
#66834=CARTESIAN_POINT('Ctrl Pts',(0.00548501651897787,-0.0321434074405927,
0.0792602877332916));
#66835=CARTESIAN_POINT('Ctrl Pts',(0.00532324750568314,-0.0327445246967097,
0.0791734580185892));
#66836=CARTESIAN_POINT('Ctrl Pts',(0.00551271032215167,-0.032443687833936,
0.0792790819110421));
#66837=CARTESIAN_POINT('Ctrl Pts',(0.00570959091803836,-0.0321434074405927,
0.0793701346234916));
#66838=CARTESIAN_POINT('',(0.00535487245241603,-0.0326943950436612,0.0791909586239028));
#66839=CARTESIAN_POINT('',(0.00556431598451705,-0.0323666188837389,0.0793004618945372));
#66840=CARTESIAN_POINT('Origin',(0.0133815612327477,-0.0326395579110695,
0.0644200302362526));
#66841=CARTESIAN_POINT('Origin',(0.000649251549682753,-0.0321933825603001,
0.0891911400034396));
#66842=CARTESIAN_POINT('',(0.00545298043822705,-0.032193409653269,0.0792436178677751));
#66843=CARTESIAN_POINT('',(0.00550895049813857,-0.0321934096584275,0.079271431582728));
#66844=CARTESIAN_POINT('',(0.00524596632824741,-0.0325210109756239,0.079129588421542));
#66845=CARTESIAN_POINT('Origin',(0.0137901838302527,-0.0326393129158855,
0.064673431109986));
#66846=CARTESIAN_POINT('',(0.00524664610052126,-0.0326943950436593,0.0791284121871067));
#66847=CARTESIAN_POINT('Origin',(-0.000288691790634326,-0.0326943765538279,
0.0887064052524144));
#66848=CARTESIAN_POINT('',(0.00530075927647864,-0.0326943950436702,0.0791596854055147));
#66849=CARTESIAN_POINT('Ctrl Pts',(0.00492023867268703,-0.0325229783203769,
0.0792231951384511));
#66850=CARTESIAN_POINT('Ctrl Pts',(0.00499017255672714,-0.032413025309245,
0.0792673559158233));
#66851=CARTESIAN_POINT('Ctrl Pts',(0.00506100935633197,-0.0323031222208069,
0.0793100633231205));
#66852=CARTESIAN_POINT('Ctrl Pts',(0.00513265640423252,-0.0321934096576658,
0.0793512658569968));
#66853=CARTESIAN_POINT('Ctrl Pts',(0.0050290542952026,-0.0325229783203769,
0.0791915675787449));
#66854=CARTESIAN_POINT('Ctrl Pts',(0.00509855219402381,-0.032413025309245,
0.0792342283351404));
#66855=CARTESIAN_POINT('Ctrl Pts',(0.00516892204467461,-0.0323031222208069,
0.0792754449678827));
#66856=CARTESIAN_POINT('Ctrl Pts',(0.0052400718453971,-0.0321934096576658,
0.0793151678620962));
#66857=CARTESIAN_POINT('Ctrl Pts',(0.00513786991771817,-0.0325229783203769,
0.0791599400190387));
#66858=CARTESIAN_POINT('Ctrl Pts',(0.00520693183132047,-0.032413025309245,
0.0792011007544574));
#66859=CARTESIAN_POINT('Ctrl Pts',(0.00527683473301726,-0.0323031222208069,
0.0792408266126449));
#66860=CARTESIAN_POINT('Ctrl Pts',(0.00534748728656168,-0.0321934096576658,
0.0792790698671956));
#66861=CARTESIAN_POINT('Ctrl Pts',(0.00524668554023373,-0.0325229783203769,
0.0791283124593325));
#66862=CARTESIAN_POINT('Ctrl Pts',(0.00531531146861714,-0.032413025309245,
0.0791679731737744));
#66863=CARTESIAN_POINT('Ctrl Pts',(0.0053847474213599,-0.0323031222208069,
0.0792062082574071));
#66864=CARTESIAN_POINT('Ctrl Pts',(0.00545490272772627,-0.0321934096576658,
0.0792429718722951));
#66865=CARTESIAN_POINT('',(0.00529281841879103,-0.0321934096584275,0.0792974418611707));
#66866=CARTESIAN_POINT('Ctrl Pts',(0.00512155322941316,-0.0322104233328919,
0.0793448648865983));
#66867=CARTESIAN_POINT('Ctrl Pts',(0.00514305771973737,-0.0322609421831331,
0.0793076548926103));
#66868=CARTESIAN_POINT('Ctrl Pts',(0.00516417523713712,-0.0323120888240662,
0.0792711144918086));
#66869=CARTESIAN_POINT('Ctrl Pts',(0.00520565496004409,-0.0324156524631809,
0.0791993406335716));
#66870=CARTESIAN_POINT('Ctrl Pts',(0.00522600011520745,-0.0324680267167312,
0.0791641366789603));
#66871=CARTESIAN_POINT('Ctrl Pts',(0.00524596632827296,-0.0325210109755913,
0.0791295884215067));
#66872=CARTESIAN_POINT('Origin',(0.00183541458650297,-0.0262834582510794,
0.0694213830049663));
#66873=CARTESIAN_POINT('Origin',(-0.00202648219799944,-0.0342770903299606,
0.0808430025345483));
#66874=CARTESIAN_POINT('Ctrl Pts',(0.00535434847749101,-0.0326943950436604,
0.0791889997617047));
#66875=CARTESIAN_POINT('Ctrl Pts',(0.0054237953382994,-0.0325844576448134,
0.0792271677487778));
#66876=CARTESIAN_POINT('Ctrl Pts',(0.00549403649051997,-0.0324744968375322,
0.0792639021621176));
#66877=CARTESIAN_POINT('Ctrl Pts',(0.00556498128790682,-0.0323646534831894,
0.0792991571767813));
#66878=CARTESIAN_POINT('Ctrl Pts',(0.00538363055309838,-0.0326943950436604,
0.0792984697924462));
#66879=CARTESIAN_POINT('Ctrl Pts',(0.00545458611609909,-0.0325844576448134,
0.0793362342176371));
#66880=CARTESIAN_POINT('Ctrl Pts',(0.00552632773096381,-0.0324744968375322,
0.0793725338380989));
#66881=CARTESIAN_POINT('Ctrl Pts',(0.00559876283665023,-0.0323646534831894,
0.0794073234124879));
#66882=CARTESIAN_POINT('Ctrl Pts',(0.00541291262870576,-0.0326943950436604,
0.0794079398231878));
#66883=CARTESIAN_POINT('Ctrl Pts',(0.00548537689389879,-0.0325844576448134,
0.0794453006864963));
#66884=CARTESIAN_POINT('Ctrl Pts',(0.00555861897140765,-0.0324744968375322,
0.0794811655140802));
#66885=CARTESIAN_POINT('Ctrl Pts',(0.00563254438539363,-0.0323646534831894,
0.0795154896481944));
#66886=CARTESIAN_POINT('Ctrl Pts',(0.00544219470431313,-0.0326943950436604,
0.0795174098539293));
#66887=CARTESIAN_POINT('Ctrl Pts',(0.00551616767169849,-0.0325844576448134,
0.0795543671553555));
#66888=CARTESIAN_POINT('Ctrl Pts',(0.0055909102118515,-0.0324744968375322,
0.0795897971900614));
#66889=CARTESIAN_POINT('Ctrl Pts',(0.00566632593413703,-0.0323646534831894,
0.0796236558839009));
#66890=CARTESIAN_POINT('',(0.00545366570612353,-0.0326773559991379,0.0795231255267482));
#66891=CARTESIAN_POINT('',(0.00544219470431034,-0.0326943950436594,0.0795174098539166));
#66892=CARTESIAN_POINT('Origin',(0.0127982851832748,-0.0326395670423499,
0.0646305142286374));
#66893=CARTESIAN_POINT('Ctrl Pts',(0.00545366570760913,-0.0326773559987494,
0.0795231255237429));
#66894=CARTESIAN_POINT('Ctrl Pts',(0.00547278081855304,-0.0326267922587283,
0.0794846598271862));
#66895=CARTESIAN_POINT('Ctrl Pts',(0.00549155712796076,-0.0325756109581972,
0.0794468759073205));
#66896=CARTESIAN_POINT('Ctrl Pts',(0.00552844812344945,-0.0324719985462383,
0.0793726394646285));
#66897=CARTESIAN_POINT('Ctrl Pts',(0.00554654801342227,-0.0324196091621783,
0.0793362167162885));
#66898=CARTESIAN_POINT('Ctrl Pts',(0.00556431598453872,-0.0323666188837756,
0.0793004618944936));
#66899=CARTESIAN_POINT('',(0.00539853357837318,-0.0326943950436703,0.0793541842389197));
#66900=CARTESIAN_POINT('Origin',(0.00812378219310841,-0.0315241814719618,
0.07415));
#66901=CARTESIAN_POINT('',(0.00545366570614322,-0.0327114338380033,0.0795231255267077));
#66902=CARTESIAN_POINT('',(0.00546514888907058,-0.0326943950436593,0.079528816687218));
#66903=CARTESIAN_POINT('Origin',(0.0127573694918815,-0.0326395657042319,
0.064611043345139));
#66904=CARTESIAN_POINT('Origin',(0.0128882682879769,-0.0326395684985889,
0.0646752265085024));
#66905=CARTESIAN_POINT('Origin',(0.0129284940098363,-0.032639567221667,
0.0646960856478551));
#66906=CARTESIAN_POINT('Ctrl Pts',(0.0054210572485344,-0.0332451089994434,
0.0792267512125353));
#66907=CARTESIAN_POINT('Ctrl Pts',(0.00561253005317438,-0.0329451141710254,
0.0793286861515629));
#66908=CARTESIAN_POINT('Ctrl Pts',(0.00581113706010535,-0.0326442513127493,
0.0794159089897944));
#66909=CARTESIAN_POINT('Ctrl Pts',(0.00564423465119968,-0.0332451089994434,
0.0793394093100675));
#66910=CARTESIAN_POINT('Ctrl Pts',(0.00583995642550487,-0.0329451141710254,
0.0794329269756397));
#66911=CARTESIAN_POINT('Ctrl Pts',(0.00604216630777994,-0.0326442513127493,
0.0795114364032364));
#66912=CARTESIAN_POINT('Ctrl Pts',(0.00564646642522633,-0.0332451089994434,
0.0793405358910428));
#66913=CARTESIAN_POINT('Ctrl Pts',(0.00584223068922818,-0.0329451141710254,
0.0794339693838805));
#66914=CARTESIAN_POINT('Ctrl Pts',(0.00604447660025668,-0.0326442513127493,
0.0795123916773708));
#66915=CARTESIAN_POINT('',(0.0056768606742133,-0.0331951640388616,0.0793548727247041));
#66916=CARTESIAN_POINT('',(0.00589276669509876,-0.0328677532355027,0.0794510088584609));
#66917=CARTESIAN_POINT('Origin',(0.0121066312472922,-0.0326402808281404,
0.0638729381599424));
#66918=CARTESIAN_POINT('Origin',(0.00160438252152576,-0.0326944278779215,
0.0896414035572649));
#66919=CARTESIAN_POINT('',(0.00577808157344145,-0.0326943950436593,0.0794012678091005));
#66920=CARTESIAN_POINT('',(0.00583568762442888,-0.0326943950436694,0.0794255122495204));
#66921=CARTESIAN_POINT('',(0.00556431598451448,-0.0330220786163545,0.0793004618945359));
#66922=CARTESIAN_POINT('Origin',(0.0125610079397382,-0.0326396682764704,
0.0640300828915743));
#66923=CARTESIAN_POINT('',(0.00556492055904027,-0.0331951640388588,0.0792992452978757));
#66924=CARTESIAN_POINT('Origin',(0.000655619978475284,-0.033195202656007,
0.0891783210318515));
#66925=CARTESIAN_POINT('',(0.00562089061663679,-0.0331951640388702,0.0793270590112999));
#66926=CARTESIAN_POINT('Ctrl Pts',(0.00524510953553629,-0.0330240426238172,
0.0794143369697029));
#66927=CARTESIAN_POINT('Ctrl Pts',(0.00531763090608894,-0.0329142774063519,
0.0794539934901158));
#66928=CARTESIAN_POINT('Ctrl Pts',(0.00539100824224168,-0.0328043479726691,
0.0794921705614427));
#66929=CARTESIAN_POINT('Ctrl Pts',(0.00546514888907057,-0.0326943950436593,
0.079528816687218));
#66930=CARTESIAN_POINT('Ctrl Pts',(0.00535172449226936,-0.0330240426238172,
0.0793759392225634));
#66931=CARTESIAN_POINT('Ctrl Pts',(0.00542371689644606,-0.0329142774063519,
0.0794141270180774));
#66932=CARTESIAN_POINT('Ctrl Pts',(0.00549653463986747,-0.0328043479726691,
0.079450845567505));
#66933=CARTESIAN_POINT('Ctrl Pts',(0.00557008573303214,-0.0326943950436593,
0.0794860452625987));
#66934=CARTESIAN_POINT('Ctrl Pts',(0.00545833944900243,-0.0330240426238172,
0.079337541475424));
#66935=CARTESIAN_POINT('Ctrl Pts',(0.00552980288680317,-0.0329142774063519,
0.0793742605460391));
#66936=CARTESIAN_POINT('Ctrl Pts',(0.00560206103749325,-0.0328043479726691,
0.0794095205735674));
#66937=CARTESIAN_POINT('Ctrl Pts',(0.00567502257699371,-0.0326943950436593,
0.0794432738379793));
#66938=CARTESIAN_POINT('Ctrl Pts',(0.0055649544057355,-0.0330240426238172,
0.0792991437282845));
#66939=CARTESIAN_POINT('Ctrl Pts',(0.00563588887716028,-0.0329142774063519,
0.0793343940740007));
#66940=CARTESIAN_POINT('Ctrl Pts',(0.00570758743511903,-0.0328043479726691,
0.0793681955796297));
#66941=CARTESIAN_POINT('Ctrl Pts',(0.00577995942095528,-0.0326943950436593,
0.07940050241336));
#66942=CARTESIAN_POINT('',(0.00562161523126602,-0.0326943950436693,0.0794650422481693));
#66943=CARTESIAN_POINT('Ctrl Pts',(0.00545366570761464,-0.0327114338383316,
0.0795231255237316));
#66944=CARTESIAN_POINT('Ctrl Pts',(0.0054727776391388,-0.0327619876831034,
0.0794846662251811));
#66945=CARTESIAN_POINT('Ctrl Pts',(0.00549155239559205,-0.0328131562604465,
0.0794468854303548));
#66946=CARTESIAN_POINT('Ctrl Pts',(0.00552844335710324,-0.0329167375858767,
0.0793726490560364));
#66947=CARTESIAN_POINT('Ctrl Pts',(0.0055465448629089,-0.032969108892062,
0.0793362230561256));
#66948=CARTESIAN_POINT('Ctrl Pts',(0.00556431598453815,-0.0330220786163187,
0.0793004618944946));
#66949=CARTESIAN_POINT('Ctrl Pts',(0.00567621463213379,-0.0331951640388604,
0.0793529503216706));
#66950=CARTESIAN_POINT('Ctrl Pts',(0.00578378229421297,-0.0330306422010619,
0.0794035522117594));
#66951=CARTESIAN_POINT('Ctrl Pts',(0.00589334946981015,-0.0328657861914644,
0.0794496649782933));
#66952=CARTESIAN_POINT('Ctrl Pts',(0.00567686067421046,-0.0331951640388604,
0.0793548727247027));
#66953=CARTESIAN_POINT('Ctrl Pts',(0.00578446808073979,-0.0330306422010619,
0.0794054612582857));
#66954=CARTESIAN_POINT('Ctrl Pts',(0.00589407441478735,-0.0328657861914644,
0.079451559037047));
#66955=CARTESIAN_POINT('Ctrl Pts',(0.00578450865792718,-0.0331951640388604,
0.0796751967682374));
#66956=CARTESIAN_POINT('Ctrl Pts',(0.00589873855868392,-0.0330306422010619,
0.0797235597487747));
#66957=CARTESIAN_POINT('Ctrl Pts',(0.00601486974363614,-0.0328657861914644,
0.0797671601615587));
#66958=CARTESIAN_POINT('',(0.00579631591329893,-0.0331781648281931,0.0796801808932682));
#66959=CARTESIAN_POINT('',(0.00578450865792326,-0.0331951640388588,0.079675196768223));
#66960=CARTESIAN_POINT('Origin',(0.0115430477417567,-0.0326412091917871,
0.0641894882940049));
#66961=CARTESIAN_POINT('Ctrl Pts',(0.00579631591232129,-0.033178164828644,
0.0796801808916987));
#66962=CARTESIAN_POINT('Ctrl Pts',(0.00581298948295319,-0.033127681154679,
0.079640563589756));
#66963=CARTESIAN_POINT('Ctrl Pts',(0.00582936194936585,-0.0330765663497816,
0.0796016616404801));
#66964=CARTESIAN_POINT('Ctrl Pts',(0.00586151889002797,-0.0329730614463284,
0.0795252550865608));
#66965=CARTESIAN_POINT('Ctrl Pts',(0.00587729037851306,-0.0329207133374053,
0.0794877813505832));
#66966=CARTESIAN_POINT('Ctrl Pts',(0.00589276667883221,-0.0328677532289383,
0.079451008861069));
#66967=CARTESIAN_POINT('',(0.00573068466607828,-0.0331951640388701,0.0795150347464736));
#66968=CARTESIAN_POINT('Ctrl Pts',(0.0057451433384942,-0.0337436976235975,
0.079386430291651));
#66969=CARTESIAN_POINT('Ctrl Pts',(0.00579224058614003,-0.0336723290703325,
0.0794078241300019));
#66970=CARTESIAN_POINT('Ctrl Pts',(0.0058397150222809,-0.033601104548885,
0.0794283673762962));
#66971=CARTESIAN_POINT('Ctrl Pts',(0.00599129149272274,-0.0333736987606857,
0.079493957892326));
#66972=CARTESIAN_POINT('Ctrl Pts',(0.00614638213913415,-0.0331450831799192,
0.0795507419885182));
#66973=CARTESIAN_POINT('Ctrl Pts',(0.00597495385551883,-0.0337436976235975,
0.0794848534914815));
#66974=CARTESIAN_POINT('Ctrl Pts',(0.00602293633634038,-0.0336723290703325,
0.0795041803792137));
#66975=CARTESIAN_POINT('Ctrl Pts',(0.00607125868452036,-0.033601104548885,
0.0795226410867183));
#66976=CARTESIAN_POINT('Ctrl Pts',(0.00622554237014116,-0.0333736987606857,
0.0795815824689207));
#66977=CARTESIAN_POINT('Ctrl Pts',(0.00638295420481749,-0.0331450831799192,
0.0796315730329152));
#66978=CARTESIAN_POINT('Ctrl Pts',(0.00597725196068907,-0.0337436976235975,
0.0794858377234798));
#66979=CARTESIAN_POINT('Ctrl Pts',(0.00602524329384239,-0.0336723290703325,
0.0795051439417057));
#66980=CARTESIAN_POINT('Ctrl Pts',(0.00607357412114276,-0.033601104548885,
0.0795235838238225));
#66981=CARTESIAN_POINT('Ctrl Pts',(0.00622788487891534,-0.0333736987606857,
0.0795824587146866));
#66982=CARTESIAN_POINT('Ctrl Pts',(0.00638531992547433,-0.0331450831799192,
0.0796323813433592));
#66983=CARTESIAN_POINT('',(0.00600850577736595,-0.0336938721132548,0.079498245570746));
#66984=CARTESIAN_POINT('',(0.00623002219053035,-0.0333679869945434,0.0795806351426612));
#66985=CARTESIAN_POINT('Ctrl Pts',(0.00600850577737769,-0.0336938721132649,
0.0794982455707519));
#66986=CARTESIAN_POINT('Ctrl Pts',(0.00602938248874717,-0.0336629187933932,
0.0795065024868959));
#66987=CARTESIAN_POINT('Ctrl Pts',(0.00605030087081092,-0.033631995230104,
0.0795146345207427));
#66988=CARTESIAN_POINT('Ctrl Pts',(0.00607125868453239,-0.033601104548895,
0.0795226410867234));
#66989=CARTESIAN_POINT('Ctrl Pts',(0.00612384901051982,-0.0335235892595454,
0.0795427323004617));
#66990=CARTESIAN_POINT('Ctrl Pts',(0.00617678113087338,-0.0334458668660369,
0.0795620690291126));
#66991=CARTESIAN_POINT('Ctrl Pts',(0.00623002219042159,-0.0333679869945385,
0.0795806351429525));
#66992=CARTESIAN_POINT('Ctrl Pts',(0.00623006395440777,-0.0333679692459669,
0.0795806504347048));
#66993=CARTESIAN_POINT('Ctrl Pts',(0.00623020758797247,-0.0333391895376564,
0.079580220542604));
#66994=CARTESIAN_POINT('Ctrl Pts',(0.00623031216851744,-0.0333104081064338,
0.0795798972884828));
#66995=CARTESIAN_POINT('Ctrl Pts',(0.00623044532910061,-0.0332532698692968,
0.0795794677019095));
#66996=CARTESIAN_POINT('Ctrl Pts',(0.00623047501916999,-0.0332249173570707,
0.0795793582030702));
#66997=CARTESIAN_POINT('Ctrl Pts',(0.00623046971168589,-0.0331960985270736,
0.0795793524650619));
#66998=CARTESIAN_POINT('Ctrl Pts',(0.00623046961596248,-0.0331956312655128,
0.0795793524001691));
#66999=CARTESIAN_POINT('Ctrl Pts',(0.00623046951091808,-0.0331951640388606,
0.0795793523635382));
#67000=CARTESIAN_POINT('',(0.00611244011171099,-0.0331951640388587,0.0795381933921863));
#67001=CARTESIAN_POINT('',(0.00617145481132473,-0.0331951640388687,0.0795587728778723));
#67002=CARTESIAN_POINT('',(0.00589276668460748,-0.0335216366567672,0.0794510088470328));
#67003=CARTESIAN_POINT('Origin',(0.0112199700697491,-0.0326434571526922,
0.063671542154586));
#67004=CARTESIAN_POINT('',(0.00589329367539628,-0.0336938721132328,0.0794497566899203));
#67005=CARTESIAN_POINT('Origin',(0.00165708336615458,-0.0336938867896174,
0.0895152100896136));
#67006=CARTESIAN_POINT('',(0.00595089972639112,-0.0336938721132538,0.0794740011303432));
#67007=CARTESIAN_POINT('Ctrl Pts',(0.00600812838762901,-0.0336938721132389,
0.0794973196701799));
#67008=CARTESIAN_POINT('Ctrl Pts',(0.00603942802408733,-0.0336474569764957,
0.0795097032939517));
#67009=CARTESIAN_POINT('Ctrl Pts',(0.00607087048182631,-0.033601104548885,
0.0795217196674262));
#67010=CARTESIAN_POINT('Ctrl Pts',(0.00615047555574723,-0.0334837508592656,
0.079552142362326));
#67011=CARTESIAN_POINT('Ctrl Pts',(0.00623094716051302,-0.0333660264659097,
0.0795801928344315));
#67012=CARTESIAN_POINT('Ctrl Pts',(0.00600850577734697,-0.0336938721132389,
0.0794982455707385));
#67013=CARTESIAN_POINT('Ctrl Pts',(0.00603981083340851,-0.0336474569764957,
0.079510626985523));
#67014=CARTESIAN_POINT('Ctrl Pts',(0.00607125868452036,-0.033601104548885,
0.0795226410867183));
#67015=CARTESIAN_POINT('Ctrl Pts',(0.00615087741322139,-0.0334837508592656,
0.0795530580287297));
#67016=CARTESIAN_POINT('Ctrl Pts',(0.0062313624963011,-0.0333660264659097,
0.0795811023458535));
#67017=CARTESIAN_POINT('Ctrl Pts',(0.00613681994874161,-0.0336938721132389,
0.079813055851237));
#67018=CARTESIAN_POINT('Ctrl Pts',(0.00616996769384003,-0.0336474569764957,
0.0798246862005972));
#67019=CARTESIAN_POINT('Ctrl Pts',(0.00620324931555745,-0.033601104548885,
0.0798359277168299));
#67020=CARTESIAN_POINT('Ctrl Pts',(0.00628751072982149,-0.0334837508592656,
0.0798643886513444));
#67021=CARTESIAN_POINT('Ctrl Pts',(0.00637257849918126,-0.0333660264659097,
0.0798903402475066));
#67022=CARTESIAN_POINT('',(0.00614815156821454,-0.0336769361243754,0.079815411161953));
#67023=CARTESIAN_POINT('',(0.00613605465546666,-0.033693872113232,0.0798111782551074));
#67024=CARTESIAN_POINT('Ctrl Pts',(0.00614815156821478,-0.0336769361243751,
0.0798154111619531));
#67025=CARTESIAN_POINT('Ctrl Pts',(0.00614613451157701,-0.033679758667013,
0.0798147077780765));
#67026=CARTESIAN_POINT('Ctrl Pts',(0.00614411790686429,-0.0336825812713055,
0.0798140033436034));
#67027=CARTESIAN_POINT('Ctrl Pts',(0.00614008561141594,-0.0336882265887076,
0.0798125923775529));
#67028=CARTESIAN_POINT('Ctrl Pts',(0.00613806992066078,-0.0336910493018399,
0.0798118858460027));
#67029=CARTESIAN_POINT('Ctrl Pts',(0.0061360546554696,-0.0336938721132374,
0.0798111782551204));
#67030=CARTESIAN_POINT('Ctrl Pts',(0.00614815156821451,-0.0336769361243754,
0.079815411161953));
#67031=CARTESIAN_POINT('Ctrl Pts',(0.00616195191148716,-0.0336279031428251,
0.0797758366494754));
#67032=CARTESIAN_POINT('Ctrl Pts',(0.00617595080743692,-0.0335767852155831,
0.079735692758015));
#67033=CARTESIAN_POINT('Ctrl Pts',(0.00620338130999196,-0.0334733199122754,
0.079657031760663));
#67034=CARTESIAN_POINT('Ctrl Pts',(0.00621683133435809,-0.0334209645148399,
0.0796184618391355));
#67035=CARTESIAN_POINT('Ctrl Pts',(0.00623002218363935,-0.033367986984468,
0.0795806351402516));
#67036=CARTESIAN_POINT('',(0.00607228021642631,-0.0336938721132534,0.0796547119129367));
#67037=CARTESIAN_POINT('Origin',(0.00812378219310841,-0.0315241814719618,
0.07415));
#67038=CARTESIAN_POINT('',(0.00579631591449628,-0.0332121607144398,0.0796801808920896));
#67039=CARTESIAN_POINT('',(0.00580813378883238,-0.0331951640388587,0.079685139787558));
#67040=CARTESIAN_POINT('Origin',(0.0114988399443315,-0.0326413638235096,
0.0641793877490522));
#67041=CARTESIAN_POINT('Origin',(0.0128560347686871,-0.032641210522979,
0.0647420762614981));
#67042=CARTESIAN_POINT('Origin',(0.0128941577392383,-0.0326413654357388,
0.0647666337109076));
#67043=CARTESIAN_POINT('Ctrl Pts',(0.00558134126227887,-0.0335235895815172,
0.0795847027621829));
#67044=CARTESIAN_POINT('Ctrl Pts',(0.00565616064574541,-0.0334144449262749,
0.0796197044672014));
#67045=CARTESIAN_POINT('Ctrl Pts',(0.0057317890965029,-0.0333049234473147,
0.0796532006727838));
#67046=CARTESIAN_POINT('Ctrl Pts',(0.00580813378883215,-0.0331951640388587,
0.0796851397875581));
#67047=CARTESIAN_POINT('Ctrl Pts',(0.00568533496484918,-0.0335235895815172,
0.0795396862950656));
#67048=CARTESIAN_POINT('Ctrl Pts',(0.00575953460801659,-0.0334144449262749,
0.0795732563220234));
#67049=CARTESIAN_POINT('Ctrl Pts',(0.00583451302907715,-0.0333049234473147,
0.0796053320080887));
#67050=CARTESIAN_POINT('Ctrl Pts',(0.00591017806896196,-0.0331951640388587,
0.0796358636535905));
#67051=CARTESIAN_POINT('Ctrl Pts',(0.0057893286674195,-0.0335235895815172,
0.0794946698279483));
#67052=CARTESIAN_POINT('Ctrl Pts',(0.00586290857028777,-0.0334144449262749,
0.0795268081768454));
#67053=CARTESIAN_POINT('Ctrl Pts',(0.00593723696165139,-0.0333049234473147,
0.0795574633433936));
#67054=CARTESIAN_POINT('Ctrl Pts',(0.00601222234909177,-0.0331951640388587,
0.0795865875196228));
#67055=CARTESIAN_POINT('Ctrl Pts',(0.00589332236998982,-0.0335235895815172,
0.079449653360831));
#67056=CARTESIAN_POINT('Ctrl Pts',(0.00596628253255895,-0.0334144449262749,
0.0794803600316675));
#67057=CARTESIAN_POINT('Ctrl Pts',(0.00603996089422564,-0.0333049234473147,
0.0795095946786985));
#67058=CARTESIAN_POINT('Ctrl Pts',(0.00611426662922157,-0.0331951640388587,
0.0795373113856552));
#67059=CARTESIAN_POINT('',(0.00596028695028169,-0.0331951640388687,0.0796116665898822));
#67060=CARTESIAN_POINT('Ctrl Pts',(0.00579631591570712,-0.033212160714597,
0.0796801808891952));
#67061=CARTESIAN_POINT('Ctrl Pts',(0.00581296144826987,-0.0332625444109796,
0.0796406302383598));
#67062=CARTESIAN_POINT('Ctrl Pts',(0.0058293201521852,-0.0333135300746914,
0.0796017611073038));
#67063=CARTESIAN_POINT('Ctrl Pts',(0.00586147688804284,-0.0334167203140563,
0.0795253550309514));
#67064=CARTESIAN_POINT('Ctrl Pts',(0.0058772624654211,-0.0334688847587242,
0.0794878476783467));
#67065=CARTESIAN_POINT('Ctrl Pts',(0.00589276668502568,-0.0335216366562311,
0.0794510088464411));
#67066=CARTESIAN_POINT('Origin',(0.00812378219310841,-0.0315241814719618,
0.07415));
#67067=CARTESIAN_POINT('',(0.00614815156864569,-0.0337108120655533,0.0798154111607359));
#67068=CARTESIAN_POINT('',(0.00616025749492669,-0.0336938721132327,0.0798196182199215));
#67069=CARTESIAN_POINT('Origin',(0.0125907192491432,-0.0345562507698484,
0.0647345707538487));
#67070=CARTESIAN_POINT('Ctrl Pts',(0.00616025749492479,-0.0336938721132337,
0.0798196182199231));
#67071=CARTESIAN_POINT('Ctrl Pts',(0.00615823923547568,-0.0336910493161011,
0.0798189192482954));
#67072=CARTESIAN_POINT('Ctrl Pts',(0.00615622128614975,-0.0336882265958383,
0.0798182191771287));
#67073=CARTESIAN_POINT('Ctrl Pts',(0.00615218598084661,-0.0336825812713121,
0.0798168168259064));
#67074=CARTESIAN_POINT('Ctrl Pts',(0.00615016862485449,-0.0336797586670165,
0.0798161145458304));
#67075=CARTESIAN_POINT('Ctrl Pts',(0.00614815156821449,-0.0336769361243755,
0.079815411161953));
#67076=CARTESIAN_POINT('Origin',(0.0104801540985315,-0.0345562519801551,
0.0639985831636916));
#67077=CARTESIAN_POINT('Ctrl Pts',(0.00607858695488061,-0.0342436276873911,
0.0795254349998424));
#67078=CARTESIAN_POINT('Ctrl Pts',(0.00628132482807593,-0.033943005420181,
0.0796025708098521));
#67079=CARTESIAN_POINT('Ctrl Pts',(0.00648929692949157,-0.0336441434784052,
0.0796642164378105));
#67080=CARTESIAN_POINT('Ctrl Pts',(0.00631412328481066,-0.0342436276873911,
0.0796092361769408));
#67081=CARTESIAN_POINT('Ctrl Pts',(0.00652002177150363,-0.033943005420181,
0.0796774885878225));
#67082=CARTESIAN_POINT('Ctrl Pts',(0.00673047637342439,-0.0336441434784052,
0.0797300379830996));
#67083=CARTESIAN_POINT('Ctrl Pts',(0.00631647864810996,-0.0342436276873911,
0.0796100741887117));
#67084=CARTESIAN_POINT('Ctrl Pts',(0.0065224087409379,-0.033943005420181,
0.0796782377656022));
#67085=CARTESIAN_POINT('Ctrl Pts',(0.00673288816786372,-0.0336441434784052,
0.0797306961985525));
#67086=CARTESIAN_POINT('',(0.00634849891012578,-0.0341934961088741,0.0796205113348903));
#67087=CARTESIAN_POINT('',(0.00657475148961899,-0.0338664212863112,0.079688829198174));
#67088=CARTESIAN_POINT('Origin',(0.0119963837668672,-0.0345610720404866,
0.0638675896884594));
#67089=CARTESIAN_POINT('Origin',(0.00362121447950633,-0.0336938005073021,
0.0902498586722073));
#67090=CARTESIAN_POINT('',(0.00645473649828104,-0.0336938721132327,0.0796538542375847));
#67091=CARTESIAN_POINT('',(0.00651492694246293,-0.0336938721132427,0.0796706875507087));
#67092=CARTESIAN_POINT('',(0.00623002218363433,-0.0340203938281605,0.07958063514025));
#67093=CARTESIAN_POINT('Origin',(0.0124188840229564,-0.0345589643243816,
0.0640978727049483));
#67094=CARTESIAN_POINT('',(0.00623046951091836,-0.034193496108874,0.0795793523635383));
#67095=CARTESIAN_POINT('Origin',(0.00260207576277473,-0.0341934220717541,
0.0899843020048005));
#67096=CARTESIAN_POINT('',(0.00628948421053207,-0.0341934961088841,0.0795999318492243));
#67097=CARTESIAN_POINT('Ctrl Pts',(0.00592760345228274,-0.0340223579322396,
0.0797336188031044));
#67098=CARTESIAN_POINT('Ctrl Pts',(0.00600461611826673,-0.0339125849573575,
0.079763909835815));
#67099=CARTESIAN_POINT('Ctrl Pts',(0.00608220162233248,-0.0338030433565231,
0.0797925856001345));
#67100=CARTESIAN_POINT('Ctrl Pts',(0.00616025749492674,-0.0336938721132327,
0.0798196182199215));
#67101=CARTESIAN_POINT('Ctrl Pts',(0.00602856539201688,-0.0340223579322396,
0.0796821613784168));
#67102=CARTESIAN_POINT('Ctrl Pts',(0.00610486832590783,-0.0339125849573575,
0.0797110598826587));
#67103=CARTESIAN_POINT('Ctrl Pts',(0.00618171577449755,-0.0338030433565231,
0.0797383587868282));
#67104=CARTESIAN_POINT('Ctrl Pts',(0.00625900636816637,-0.0336938721132327,
0.0797640318918879));
#67105=CARTESIAN_POINT('Ctrl Pts',(0.00612952733175102,-0.0340223579322396,
0.0796307039537292));
#67106=CARTESIAN_POINT('Ctrl Pts',(0.00620512053354894,-0.0339125849573575,
0.0796582099295023));
#67107=CARTESIAN_POINT('Ctrl Pts',(0.00628122992666263,-0.0338030433565231,
0.0796841319735219));
#67108=CARTESIAN_POINT('Ctrl Pts',(0.00635775524140601,-0.0336938721132327,
0.0797084455638543));
#67109=CARTESIAN_POINT('Ctrl Pts',(0.00623048927148517,-0.0340223579322396,
0.0795792465290416));
#67110=CARTESIAN_POINT('Ctrl Pts',(0.00630537274119004,-0.0339125849573575,
0.079605359976346));
#67111=CARTESIAN_POINT('Ctrl Pts',(0.0063807440788277,-0.0338030433565231,
0.0796299051602156));
#67112=CARTESIAN_POINT('Ctrl Pts',(0.00645650411464565,-0.0336938721132327,
0.0796528592358206));
#67113=CARTESIAN_POINT('',(0.00630749699661386,-0.0336938721132427,0.0797367362287631));
#67114=CARTESIAN_POINT('Ctrl Pts',(0.00614815156982787,-0.0337108120662688,
0.0798154111573263));
#67115=CARTESIAN_POINT('Ctrl Pts',(0.00616231001104801,-0.0337611408994286,
0.0797748097463572));
#67116=CARTESIAN_POINT('Ctrl Pts',(0.00617621009212749,-0.0338121088781288,
0.0797349492210609));
#67117=CARTESIAN_POINT('Ctrl Pts',(0.00620350619675928,-0.0339153382773237,
0.0796566736295054));
#67118=CARTESIAN_POINT('Ctrl Pts',(0.00621689067238685,-0.0339675558473111,
0.0796182916786175));
#67119=CARTESIAN_POINT('Ctrl Pts',(0.00623002218365246,-0.0340203938281304,
0.0795806351402141));
#67120=CARTESIAN_POINT('Ctrl Pts',(0.00634761698076121,-0.0341934961088741,
0.0796186849771815));
#67121=CARTESIAN_POINT('Ctrl Pts',(0.00646067773436962,-0.0340287516182427,
0.0796554057936628));
#67122=CARTESIAN_POINT('Ctrl Pts',(0.00657515957893013,-0.033864463327595,
0.0796874223461877));
#67123=CARTESIAN_POINT('Ctrl Pts',(0.00634849891012574,-0.0341934961088741,
0.0796205113348903));
#67124=CARTESIAN_POINT('Ctrl Pts',(0.00646159742224096,-0.0340287516182427,
0.0796572139181767));
#67125=CARTESIAN_POINT('Ctrl Pts',(0.00657611623945257,-0.033864463327595,
0.079689210692499));
#67126=CARTESIAN_POINT('Ctrl Pts',(0.00649544530550296,-0.0341934961088741,
0.0799248176577804));
#67127=CARTESIAN_POINT('Ctrl Pts',(0.00661483511110781,-0.0340287516182427,
0.0799584822401085));
#67128=CARTESIAN_POINT('Ctrl Pts',(0.00673551428313467,-0.033864463327595,
0.0799871835854533));
#67129=CARTESIAN_POINT('',(0.00650778413357308,-0.0341764758832424,0.0799282826395307));
#67130=CARTESIAN_POINT('',(0.00649544530549579,-0.034193496108874,0.0799248176577655));
#67131=CARTESIAN_POINT('Origin',(0.0114605081543549,-0.0345621026563146,
0.0641203147158454));
#67132=CARTESIAN_POINT('Ctrl Pts',(0.00650778413225823,-0.034176475883753,
0.079928282638261));
#67133=CARTESIAN_POINT('Ctrl Pts',(0.00651934507087322,-0.0341260050040351,
0.079886944436816));
#67134=CARTESIAN_POINT('Ctrl Pts',(0.00653070501630605,-0.0340749269147945,
0.0798463247805428));
#67135=CARTESIAN_POINT('Ctrl Pts',(0.00655303190152458,-0.0339715436305775,
0.0797664911270974));
#67136=CARTESIAN_POINT('Ctrl Pts',(0.00656399037672683,-0.0339192778237867,
0.0797273074187317));
#67137=CARTESIAN_POINT('Ctrl Pts',(0.00657475148779686,-0.0338664212855678,
0.0796888291986856));
#67138=CARTESIAN_POINT('',(0.00642197210782079,-0.0341934961088841,0.0797726644963379));
#67139=CARTESIAN_POINT('Origin',(0.00812378219310841,-0.0315241814719618,
0.07415));
#67140=CARTESIAN_POINT('',(0.00650778413458173,-0.034210518019035,0.0799282826390478));
#67141=CARTESIAN_POINT('',(0.00652013033595573,-0.034193496108874,0.079931721259373));
#67142=CARTESIAN_POINT('Origin',(0.011418557203585,-0.0345621698369096,
0.0641031448877212));
#67143=CARTESIAN_POINT('Origin',(0.010474156061617,-0.0345621043539572,
0.063844460519104));
#67144=CARTESIAN_POINT('Origin',(0.0105189261518166,-0.0345621712241411,
0.0638515515515507));
#67145=CARTESIAN_POINT('Ctrl Pts',(0.00645329191808031,-0.0346945769586966,
0.0796534502354016));
#67146=CARTESIAN_POINT('Ctrl Pts',(0.00656856388672206,-0.0345275153362944,
0.0796884393230398));
#67147=CARTESIAN_POINT('Ctrl Pts',(0.00668496604520018,-0.0343603235965185,
0.0797198122633351));
#67148=CARTESIAN_POINT('Ctrl Pts',(0.00680215274854109,-0.034193496108874,
0.0797474813857446));
#67149=CARTESIAN_POINT('Ctrl Pts',(0.00653402737037455,-0.0346945769586966,
0.0796760293202807));
#67150=CARTESIAN_POINT('Ctrl Pts',(0.00664977226698927,-0.0345275153362944,
0.079709327371546));
#67151=CARTESIAN_POINT('Ctrl Pts',(0.00676659429422632,-0.0343603235965185,
0.0797389939649302));
#67152=CARTESIAN_POINT('Ctrl Pts',(0.00688414664033257,-0.034193496108874,
0.0797649464949634));
#67153=CARTESIAN_POINT('Ctrl Pts',(0.0066147628226688,-0.0346945769586966,
0.0796986084051599));
#67154=CARTESIAN_POINT('Ctrl Pts',(0.00673098064725648,-0.0345275153362944,
0.0797302154200521));
#67155=CARTESIAN_POINT('Ctrl Pts',(0.00684822254325245,-0.0343603235965185,
0.0797581756665252));
#67156=CARTESIAN_POINT('Ctrl Pts',(0.00696614053212405,-0.034193496108874,
0.0797824116041821));
#67157=CARTESIAN_POINT('Ctrl Pts',(0.00669549827496304,-0.0346945769586966,
0.079721187490039));
#67158=CARTESIAN_POINT('Ctrl Pts',(0.00681218902752369,-0.0345275153362944,
0.0797511034685582));
#67159=CARTESIAN_POINT('Ctrl Pts',(0.00692985079227859,-0.0343603235965185,
0.0797773573681202));
#67160=CARTESIAN_POINT('Ctrl Pts',(0.00704813442391553,-0.034193496108874,
0.0797998767134009));
#67161=CARTESIAN_POINT('',(0.00669549827497416,-0.0346945769586966,0.079721187490042));
#67162=CARTESIAN_POINT('',(0.00692559410958799,-0.0343667727831515,0.0797751640257857));
#67163=CARTESIAN_POINT('Origin',(0.0106934814914887,-0.034562645706343,
0.0633898257144464));
#67164=CARTESIAN_POINT('Origin',(0.00462308388846954,-0.0341934771029066,
0.0905848402985495));
#67165=CARTESIAN_POINT('',(0.00680361984569412,-0.034193496108874,0.0797477938847791));
#67166=CARTESIAN_POINT('',(0.00686474849025947,-0.034193496108884,0.0797608145919446));
#67167=CARTESIAN_POINT('',(0.00657475148826711,-0.0345211942962637,0.07968882919717));
#67168=CARTESIAN_POINT('Origin',(0.0111556302912778,-0.0345625596120658,
0.0635225256653779));
#67169=CARTESIAN_POINT('',(0.00657511738662482,-0.0346945769586885,0.0796875208638126));
#67170=CARTESIAN_POINT('Origin',(0.00359533271229314,-0.0346945685853929,
0.0903422568304037));
#67171=CARTESIAN_POINT('',(0.00663530783080949,-0.0346945769587026,0.0797043541769372));
#67172=CARTESIAN_POINT('Ctrl Pts',(0.00628253635060995,-0.0345231616327842,
0.0798605003062357));
#67173=CARTESIAN_POINT('Ctrl Pts',(0.00636124755759006,-0.0344132092796988,
0.0798858792879077));
#67174=CARTESIAN_POINT('Ctrl Pts',(0.00644047964765093,-0.034303273855898,
0.0799096288809111));
#67175=CARTESIAN_POINT('Ctrl Pts',(0.00652013033595567,-0.034193496108874,
0.079931721259373));
#67176=CARTESIAN_POINT('Ctrl Pts',(0.00638006785141206,-0.0345231616327842,
0.0798028050508859));
#67177=CARTESIAN_POINT('Ctrl Pts',(0.00645798381052559,-0.0344132092796988,
0.0798268396981327));
#67178=CARTESIAN_POINT('Ctrl Pts',(0.00653639288725383,-0.034303273855898,
0.0798492614751472));
#67179=CARTESIAN_POINT('Ctrl Pts',(0.00661519389470903,-0.034193496108874,
0.0798700442301341));
#67180=CARTESIAN_POINT('Ctrl Pts',(0.00647759935221417,-0.0345231616327842,
0.0797451097955361));
#67181=CARTESIAN_POINT('Ctrl Pts',(0.00655472006346112,-0.0344132092796988,
0.0797678001083577));
#67182=CARTESIAN_POINT('Ctrl Pts',(0.00663230612685673,-0.034303273855898,
0.0797888940693834));
#67183=CARTESIAN_POINT('Ctrl Pts',(0.00671025745346239,-0.034193496108874,
0.0798083672008952));
#67184=CARTESIAN_POINT('Ctrl Pts',(0.00657513085301627,-0.0345231616327842,
0.0796874145401863));
#67185=CARTESIAN_POINT('Ctrl Pts',(0.00665145631639665,-0.0344132092796988,
0.0797087605185827));
#67186=CARTESIAN_POINT('Ctrl Pts',(0.00672821936645963,-0.034303273855898,
0.0797285266636195));
#67187=CARTESIAN_POINT('Ctrl Pts',(0.00680532101221575,-0.034193496108874,
0.0797466901716563));
#67188=CARTESIAN_POINT('',(0.00666187509083492,-0.0341934961088839,0.079839757572086));
#67189=CARTESIAN_POINT('Ctrl Pts',(0.00650778413550785,-0.0342105180195384,
0.0799282826357127));
#67190=CARTESIAN_POINT('Ctrl Pts',(0.00651935808409803,-0.0342610556241207,
0.0798868979658173));
#67191=CARTESIAN_POINT('Ctrl Pts',(0.00653072434416499,-0.0343122189869959,
0.0798462559224256));
#67192=CARTESIAN_POINT('Ctrl Pts',(0.0065530514506996,-0.0344158119695109,
0.0797664214626082));
#67193=CARTESIAN_POINT('Ctrl Pts',(0.00656400316521219,-0.0344681990449993,
0.079727261699079));
#67194=CARTESIAN_POINT('Ctrl Pts',(0.00657475148826946,-0.0345211942962403,
0.0796888291971384));
#67195=CARTESIAN_POINT('Ctrl Pts',(0.00669450365152847,-0.0346945769586932,
0.0797194205457717));
#67196=CARTESIAN_POINT('Ctrl Pts',(0.00680964748051673,-0.034529677707698,
0.0797489698682939));
#67197=CARTESIAN_POINT('Ctrl Pts',(0.00692591422119528,-0.034364806625142,
0.0797737349410289));
#67198=CARTESIAN_POINT('Ctrl Pts',(0.0066954982749654,-0.0346945769586932,
0.0797211874900396));
#67199=CARTESIAN_POINT('Ctrl Pts',(0.00681067863427614,-0.034529677707698,
0.079750716249426));
#67200=CARTESIAN_POINT('Ctrl Pts',(0.00692698102416918,-0.034364806625142,
0.0797754592667644));
#67201=CARTESIAN_POINT('Ctrl Pts',(0.00686126225730843,-0.0346945769586932,
0.0800156664934055));
#67202=CARTESIAN_POINT('Ctrl Pts',(0.00698253076164711,-0.034529677707698,
0.0800417681997477));
#67203=CARTESIAN_POINT('Ctrl Pts',(0.00710477445107272,-0.034364806625142,
0.0800628354637875));
#67204=CARTESIAN_POINT('',(0.00687379430557909,-0.0346775396665011,0.0800183498766304));
#67205=CARTESIAN_POINT('',(0.00686126225730344,-0.0346945769586886,0.0800156664933914));
#67206=CARTESIAN_POINT('Origin',(0.0101829135396672,-0.0345626617741161,
0.0637498947265812));
#67207=CARTESIAN_POINT('Ctrl Pts',(0.00687379430425578,-0.0346775396670097,
0.0800183498753647));
#67208=CARTESIAN_POINT('Ctrl Pts',(0.00688274382668006,-0.0346269749928203,
0.0799763342633121));
#67209=CARTESIAN_POINT('Ctrl Pts',(0.00689153426098909,-0.0345757902890825,
0.0799350653549555));
#67210=CARTESIAN_POINT('Ctrl Pts',(0.00690880436139023,-0.0344721681087976,
0.0798539869941608));
#67211=CARTESIAN_POINT('Ctrl Pts',(0.0069172772623034,-0.0344197714289672,
0.0798142093294302));
#67212=CARTESIAN_POINT('Ctrl Pts',(0.00692559410932243,-0.0343667727830727,
0.0797751640258361));
#67213=CARTESIAN_POINT('',(0.0067783802661488,-0.0346945769587026,0.0798684269917267));
#67214=CARTESIAN_POINT('Origin',(0.00812378219310841,-0.0315241814719618,
0.07415));
#67215=CARTESIAN_POINT('',(0.00687379430654705,-0.0347116136489777,0.0800183498756309));
#67216=CARTESIAN_POINT('',(0.00688633205822579,-0.034694576958689,0.0800210064864313));
#67217=CARTESIAN_POINT('Origin',(0.0101382425443413,-0.0345626675611879,
0.0637422868206545));
#67218=CARTESIAN_POINT('Origin',(0.0104816443016738,-0.0345626636336016,
0.0638135220613863));
#67219=CARTESIAN_POINT('Origin',(0.0105255369531395,-0.0345626690763649,
0.0638247862753589));
#67220=CARTESIAN_POINT('Ctrl Pts',(0.0067660446236618,-0.0352450361874069,
0.0797388559936841));
#67221=CARTESIAN_POINT('Ctrl Pts',(0.00697683178632017,-0.0349452760959493,
0.0797900639063986));
#67222=CARTESIAN_POINT('Ctrl Pts',(0.00719087731434947,-0.034644428984174,
0.0798252489912614));
#67223=CARTESIAN_POINT('Ctrl Pts',(0.00676851087054738,-0.0352450361874069,
0.0797393975205065));
#67224=CARTESIAN_POINT('Ctrl Pts',(0.006979318457225,-0.0349452760959493,
0.0797905124171933));
#67225=CARTESIAN_POINT('Ctrl Pts',(0.00719337734490327,-0.034644428984174,
0.0798256032118566));
#67226=CARTESIAN_POINT('Ctrl Pts',(0.00701269373050567,-0.0352450361874069,
0.0797930140375753));
#67227=CARTESIAN_POINT('Ctrl Pts',(0.00722552349730697,-0.0349452760959493,
0.0798349194265778));
#67228=CARTESIAN_POINT('Ctrl Pts',(0.00744090512250706,-0.034644428984174,
0.0798606745579176));
#67229=CARTESIAN_POINT('Ctrl Pts',(0.00701513555910525,-0.0352450361874069,
0.079793550202746));
#67230=CARTESIAN_POINT('Ctrl Pts',(0.00722798554770779,-0.0349452760959493,
0.0798353634966716));
#67231=CARTESIAN_POINT('Ctrl Pts',(0.00744338040028309,-0.034644428984174,
0.0798610252713782));
#67232=CARTESIAN_POINT('',(0.00704810219230022,-0.0351951634053299,0.0797998729931193));
#67233=CARTESIAN_POINT('',(0.00728116543148293,-0.0348678972925388,0.0798392989017126));
#67234=CARTESIAN_POINT('Origin',(0.00931659888056036,-0.0345628965653863,
0.0632090899675132));
#67235=CARTESIAN_POINT('Origin',(0.00566228227765515,-0.0346946199340971,
0.0907699076031147));
#67236=CARTESIAN_POINT('',(0.00715771325306242,-0.0346945769330289,0.079819641593722));
#67237=CARTESIAN_POINT('',(0.00721953885972381,-0.0346945769458128,0.0798287983097628));
#67238=CARTESIAN_POINT('',(0.00692559410936888,-0.0350221583435276,0.0797751640256961));
#67239=CARTESIAN_POINT('Origin',(0.00979758133306995,-0.0345628458716864,
0.0632382464995736));
#67240=CARTESIAN_POINT('',(0.00692584883293436,-0.0351951360298761,0.0797739536502795));
#67241=CARTESIAN_POINT('Origin',(0.00463025283431429,-0.0351951838366627,
0.0905511556451489));
#67242=CARTESIAN_POINT('',(0.00704813442389201,-0.0351951371328747,0.0797998767135148));
#67243=CARTESIAN_POINT('Ctrl Pts',(0.0066447358407554,-0.0350241211494343,
0.0799648449581764));
#67244=CARTESIAN_POINT('Ctrl Pts',(0.00672483294587503,-0.0349144232818962,
0.0799852182152474));
#67245=CARTESIAN_POINT('Ctrl Pts',(0.00680539912275446,-0.0348045283579412,
0.0800039480022977));
#67246=CARTESIAN_POINT('Ctrl Pts',(0.00688633206909981,-0.0346945769439157,
0.0800210064887231));
#67247=CARTESIAN_POINT('Ctrl Pts',(0.00673845218083138,-0.0350241211494343,
0.0799011394685713));
#67248=CARTESIAN_POINT('Ctrl Pts',(0.00681767176895197,-0.0349144232818962,
0.079920221821483));
#67249=CARTESIAN_POINT('Ctrl Pts',(0.00689733321968474,-0.0348045283579412,
0.079937678070609));
#67250=CARTESIAN_POINT('Ctrl Pts',(0.00697733532887279,-0.0346945769439157,
0.0799534820597085));
#67251=CARTESIAN_POINT('Ctrl Pts',(0.00683216852090737,-0.0350241211494343,
0.0798374339789663));
#67252=CARTESIAN_POINT('Ctrl Pts',(0.00691051059202892,-0.0349144232818962,
0.0798552254277186));
#67253=CARTESIAN_POINT('Ctrl Pts',(0.00698926731661502,-0.0348045283579412,
0.0798714081389203));
#67254=CARTESIAN_POINT('Ctrl Pts',(0.00706833858864577,-0.0346945769439157,
0.0798859576306939));
#67255=CARTESIAN_POINT('Ctrl Pts',(0.00692588486098336,-0.0350241211494343,
0.0797737284893613));
#67256=CARTESIAN_POINT('Ctrl Pts',(0.00700334941510587,-0.0349144232818962,
0.0797902290339543));
#67257=CARTESIAN_POINT('Ctrl Pts',(0.00708120141354529,-0.0348045283579412,
0.0798051382072316));
#67258=CARTESIAN_POINT('Ctrl Pts',(0.00715934184841875,-0.0346945769439157,
0.0798184332016793));
#67259=CARTESIAN_POINT('',(0.00702202265534713,-0.0346945769458131,0.0799203240401144));
#67260=CARTESIAN_POINT('Ctrl Pts',(0.00687379430722754,-0.0347116136492789,
0.0800183498724067));
#67261=CARTESIAN_POINT('Ctrl Pts',(0.00688274028816434,-0.034762154653045,
0.0799763509485115));
#67262=CARTESIAN_POINT('Ctrl Pts',(0.0068915289745913,-0.0348133084093162,
0.0799350904791837));
#67263=CARTESIAN_POINT('Ctrl Pts',(0.00690879909330109,-0.0349168561546272,
0.0798540120142869));
#67264=CARTESIAN_POINT('Ctrl Pts',(0.00691727367530838,-0.0349692089019536,
0.0798142261788806));
#67265=CARTESIAN_POINT('Ctrl Pts',(0.00692559410939604,-0.0350221583435,
0.0797751640256645));
#67266=CARTESIAN_POINT('Ctrl Pts',(0.00704733813404601,-0.0351951371254917,
0.0797986493821031));
#67267=CARTESIAN_POINT('Ctrl Pts',(0.00712512912923097,-0.035085624873602,
0.0798134737496555));
#67268=CARTESIAN_POINT('Ctrl Pts',(0.0072032903487341,-0.0349758427080718,
0.0798267026399164));
#67269=CARTESIAN_POINT('Ctrl Pts',(0.00728172272318351,-0.0348659306897824,
0.0798383132388551));
#67270=CARTESIAN_POINT('Ctrl Pts',(0.00709208990104423,-0.0351951371254917,
0.0798676258273673));
#67271=CARTESIAN_POINT('Ctrl Pts',(0.00717083081291874,-0.035085624873602,
0.0798818338910469));
#67272=CARTESIAN_POINT('Ctrl Pts',(0.00724992999223989,-0.0349758427080718,
0.0798944263402952));
#67273=CARTESIAN_POINT('Ctrl Pts',(0.00732928712096993,-0.0348659306897824,
0.0799053811053336));
#67274=CARTESIAN_POINT('Ctrl Pts',(0.00713684166804246,-0.0351951371254917,
0.0799366022726316));
#67275=CARTESIAN_POINT('Ctrl Pts',(0.0072165324966065,-0.035085624873602,
0.0799501940324382));
#67276=CARTESIAN_POINT('Ctrl Pts',(0.00729656963574569,-0.0349758427080718,
0.079962150040674));
#67277=CARTESIAN_POINT('Ctrl Pts',(0.00737685151875635,-0.0348659306897824,
0.0799724489718121));
#67278=CARTESIAN_POINT('Ctrl Pts',(0.00718159343504069,-0.0351951371254917,
0.0800055787178959));
#67279=CARTESIAN_POINT('Ctrl Pts',(0.00726223418029427,-0.035085624873602,
0.0800185541738295));
#67280=CARTESIAN_POINT('Ctrl Pts',(0.00734320927925149,-0.0349758427080718,
0.0800298737410528));
#67281=CARTESIAN_POINT('Ctrl Pts',(0.00742441591654277,-0.0348659306897824,
0.0800395168382905));
#67282=CARTESIAN_POINT('Origin',(0.00650201229109275,-0.0308609197410636,
0.0851000951589266));
#67283=CARTESIAN_POINT('',(0.00710631954366105,-0.0351951371254917,0.0798895581493945));
#67284=CARTESIAN_POINT('Origin',(0.00812538052117974,-0.0351840467441193,
0.0731728904387266));
#67285=CARTESIAN_POINT('Origin',(0.00716077028536051,-0.0352322613422822,
0.086076488883645));
#67286=CARTESIAN_POINT('',(0.00751593503015258,-0.0351951142564676,0.0798691202478984));
#67287=CARTESIAN_POINT('',(0.00764017649173142,-0.0351951372916787,0.0798796269970737));
#67288=CARTESIAN_POINT('Origin',(0.00842780899661044,-0.0352875115375133,
0.0739965727786824));
#67289=CARTESIAN_POINT('Origin',(0.000906496639794719,-0.0298325076523213,
0.0720991515120198));
#67290=CARTESIAN_POINT('Origin',(0.00432725982884279,-0.0338733733910703,
0.0816220350393757));
#67291=CARTESIAN_POINT('Ctrl Pts',(0.0042701248194806,-0.0321934096636942,
0.0784193630194674));
#67292=CARTESIAN_POINT('Ctrl Pts',(0.00434654438445685,-0.0320508460843789,
0.0784883416513423));
#67293=CARTESIAN_POINT('Ctrl Pts',(0.00442475964856207,-0.0319086045662002,
0.0785552150301777));
#67294=CARTESIAN_POINT('Ctrl Pts',(0.00450459034641189,-0.0317669892866302,
0.0786198530304804));
#67295=CARTESIAN_POINT('Ctrl Pts',(0.00433357358420958,-0.0321934096636942,
0.0784741780437055));
#67296=CARTESIAN_POINT('Ctrl Pts',(0.00441097431201675,-0.0320508460843789,
0.0785420209729062));
#67297=CARTESIAN_POINT('Ctrl Pts',(0.00449013948506295,-0.0319086045662002,
0.0786077331434814));
#67298=CARTESIAN_POINT('Ctrl Pts',(0.00457088699848174,-0.0317669892866302,
0.0786711870986076));
#67299=CARTESIAN_POINT('Ctrl Pts',(0.00439702234893855,-0.0321934096636942,
0.0785289930679436));
#67300=CARTESIAN_POINT('Ctrl Pts',(0.00447540423957666,-0.0320508460843789,
0.07859570029447));
#67301=CARTESIAN_POINT('Ctrl Pts',(0.00455551932156381,-0.0319086045662002,
0.0786602512567852));
#67302=CARTESIAN_POINT('Ctrl Pts',(0.00463718365055159,-0.0317669892866302,
0.0787225211667348));
#67303=CARTESIAN_POINT('Ctrl Pts',(0.00446047111366753,-0.0321934096636942,
0.0785838080921818));
#67304=CARTESIAN_POINT('Ctrl Pts',(0.00453983416713657,-0.0320508460843789,
0.0786493796160338));
#67305=CARTESIAN_POINT('Ctrl Pts',(0.00462089915806469,-0.0319086045662002,
0.078712769370089));
#67306=CARTESIAN_POINT('Ctrl Pts',(0.00470348030262144,-0.0317669892866302,
0.0787738552348621));
#67307=CARTESIAN_POINT('',(0.00445933600272986,-0.0321934096636942,0.0785828274405644));
#67308=CARTESIAN_POINT('',(0.00464455084779424,-0.0318665617511316,0.0787296369108196));
#67309=CARTESIAN_POINT('Origin',(0.0155726506501712,-0.0326371944419261,
0.0661043602921911));
#67310=CARTESIAN_POINT('Origin',(-0.00198631738476063,-0.0316939261508961,
0.0874577052339979));
#67311=CARTESIAN_POINT('',(0.00436408889973575,-0.0320197221621755,0.0785022747507831));
#67312=CARTESIAN_POINT('Ctrl Pts',(0.00436419340266429,-0.0320197392094673,
0.0785024273745623));
#67313=CARTESIAN_POINT('Ctrl Pts',(0.00438633998309954,-0.0319792716575971,
0.0785215573354824));
#67314=CARTESIAN_POINT('Ctrl Pts',(0.00440873322232175,-0.0319386439829625,
0.0785406055466512));
#67315=CARTESIAN_POINT('Ctrl Pts',(0.00443140210882574,-0.0318979099381557,
0.078559585562952));
#67316=CARTESIAN_POINT('Ctrl Pts',(0.00445407054726213,-0.0318571766984879,
0.0785785652040986));
#67317=CARTESIAN_POINT('Ctrl Pts',(0.00447689826249396,-0.031816387183355,
0.0785973815522193));
#67318=CARTESIAN_POINT('Ctrl Pts',(0.00449980449695246,-0.0317755399638304,
0.0786159726039175));
#67319=CARTESIAN_POINT('',(0.00436474667057906,-0.0321934096636182,0.0785011092769962));
#67320=CARTESIAN_POINT('Origin',(0.00287114878390623,-0.0324113699142621,
0.0802621419685801));
#67321=CARTESIAN_POINT('',(0.00441204133666445,-0.0321934096636662,0.0785419683587903));
#67322=CARTESIAN_POINT('Ctrl Pts',(0.0044591883271136,-0.0321934096636618,
0.0785808046011513));
#67323=CARTESIAN_POINT('Ctrl Pts',(0.00452029257573062,-0.0320835708272592,
0.0786313422065808));
#67324=CARTESIAN_POINT('Ctrl Pts',(0.00458240725451797,-0.0319739230346488,
0.0786805859488959));
#67325=CARTESIAN_POINT('Ctrl Pts',(0.00464544805667624,-0.0318646057455573,
0.0787284789233544));
#67326=CARTESIAN_POINT('Ctrl Pts',(0.00446743911033446,-0.0321934096636618,
0.0786938226941353));
#67327=CARTESIAN_POINT('Ctrl Pts',(0.00453010196653488,-0.0320835708272592,
0.0787442465148339));
#67328=CARTESIAN_POINT('Ctrl Pts',(0.0045937719940808,-0.0319739230346488,
0.0787933442831149));
#67329=CARTESIAN_POINT('Ctrl Pts',(0.00465836291054557,-0.0318646057455573,
0.0788410594337238));
#67330=CARTESIAN_POINT('Ctrl Pts',(0.00447568989355532,-0.0321934096636618,
0.0788068407871193));
#67331=CARTESIAN_POINT('Ctrl Pts',(0.00453991135733915,-0.0320835708272592,
0.078857150823087));
#67332=CARTESIAN_POINT('Ctrl Pts',(0.00460513673364362,-0.0319739230346488,
0.078906102617334));
#67333=CARTESIAN_POINT('Ctrl Pts',(0.00467127776441489,-0.0318646057455573,
0.0789536399440932));
#67334=CARTESIAN_POINT('Ctrl Pts',(0.00448394067677619,-0.0321934096636618,
0.0789198588801033));
#67335=CARTESIAN_POINT('Ctrl Pts',(0.00454972074814341,-0.0320835708272592,
0.07897005513134));
#67336=CARTESIAN_POINT('Ctrl Pts',(0.00461650147320646,-0.0319739230346488,
0.079018860951553));
#67337=CARTESIAN_POINT('Ctrl Pts',(0.00468419261828422,-0.0318646057455573,
0.0790662204544626));
#67338=CARTESIAN_POINT('',(0.00449413748547113,-0.0321763980308493,0.0789276227638977));
#67339=CARTESIAN_POINT('',(0.00448394067680125,-0.0321934096636184,0.0789198588801103));
#67340=CARTESIAN_POINT('Origin',(0.0149861426078369,-0.032638623058885,
0.0661313765646252));
#67341=CARTESIAN_POINT('Ctrl Pts',(0.00449413748738438,-0.0321763980306348,
0.0789276227613674));
#67342=CARTESIAN_POINT('Ctrl Pts',(0.00452010087637376,-0.0321259596176119,
0.0788934477144262));
#67343=CARTESIAN_POINT('Ctrl Pts',(0.00454561441595596,-0.032074916463399,
0.0788598647945113));
#67344=CARTESIAN_POINT('Ctrl Pts',(0.0045957623290327,-0.031971605779397,
0.0787938561819953));
#67345=CARTESIAN_POINT('Ctrl Pts',(0.00462037716303247,-0.0319193786690168,
0.0787614562088084));
#67346=CARTESIAN_POINT('Ctrl Pts',(0.00464455084890938,-0.0318665617525361,
0.0787296369093355));
#67347=CARTESIAN_POINT('',(0.00447163833977556,-0.0321934096636663,0.0787513431603474));
#67348=CARTESIAN_POINT('Origin',(0.00812378219310841,-0.0315241814719618,
0.07415));
#67349=CARTESIAN_POINT('',(0.0044941374852466,-0.0322104233323594,0.0789276227641925));
#67350=CARTESIAN_POINT('',(0.00450435085242233,-0.0321934096636183,0.0789353648523491));
#67351=CARTESIAN_POINT('Origin',(0.014954218876609,-0.0326387224538279,
0.0660991862359572));
#67352=CARTESIAN_POINT('Origin',(0.0140091149074795,-0.0326386249602914,
0.0653891067255413));
#67353=CARTESIAN_POINT('Origin',(0.0140486811808949,-0.0326387238743361,
0.0654112383954586));
#67354=CARTESIAN_POINT('Ctrl Pts',(0.00451761106607016,-0.0327445246967097,
0.0786303632444832));
#67355=CARTESIAN_POINT('Ctrl Pts',(0.00468659072827904,-0.032443687833936,
0.0787663722119848));
#67356=CARTESIAN_POINT('Ctrl Pts',(0.004865335088422,-0.0321434074405928,
0.0788892665535882));
#67357=CARTESIAN_POINT('Ctrl Pts',(0.00471572432102837,-0.0327445246967097,
0.0787828464835944));
#67358=CARTESIAN_POINT('Ctrl Pts',(0.00489045498261643,-0.032443687833936,
0.0789113834875353));
#67359=CARTESIAN_POINT('Ctrl Pts',(0.00507437118532303,-0.0321434074405928,
0.0790263939038594));
#67360=CARTESIAN_POINT('',(0.00474490648815703,-0.0326943950436612,0.0788041727482432));
#67361=CARTESIAN_POINT('',(0.0049389740964552,-0.0323666188837389,0.0789390627880091));
#67362=CARTESIAN_POINT('Origin',(0.0145595906482954,-0.0326395579112012,
0.065155728401725));
#67363=CARTESIAN_POINT('Origin',(-0.00117696400785318,-0.032193382560303,
0.088135729191429));
#67364=CARTESIAN_POINT('',(0.0048356409098863,-0.032193409653269,0.0788687129493481));
#67365=CARTESIAN_POINT('',(0.00488768364632547,-0.0321934096584275,0.0789033222534424));
#67366=CARTESIAN_POINT('',(0.00464455084721257,-0.0325210109756239,0.0787296369115615));
#67367=CARTESIAN_POINT('Origin',(0.0149332315833509,-0.0326393129160891,
0.065458345125981));
#67368=CARTESIAN_POINT('',(0.00464537268054427,-0.0326943950436593,0.0787285551501433));
#67369=CARTESIAN_POINT('Origin',(-0.00204675831664323,-0.0326943765538239,
0.0875372610391569));
#67370=CARTESIAN_POINT('',(0.00469513958436065,-0.0326943950436702,0.0787663639492033));
#67371=CARTESIAN_POINT('Ctrl Pts',(0.00430965961899282,-0.0325229783203769,
0.0787816810112161));
#67372=CARTESIAN_POINT('Ctrl Pts',(0.00437350724044426,-0.032413025309245,
0.078834258607491));
#67373=CARTESIAN_POINT('Ctrl Pts',(0.00443843281327257,-0.032303122220807,
0.0788855074592754));
#67374=CARTESIAN_POINT('Ctrl Pts',(0.00450435085599873,-0.0321934096576658,
0.0789353648550541));
#67375=CARTESIAN_POINT('Ctrl Pts',(0.00442158118215094,-0.0325229783203769,
0.0787639410580971));
#67376=CARTESIAN_POINT('Ctrl Pts',(0.00448518425873659,-0.032413025309245,
0.0788149758180713));
#67377=CARTESIAN_POINT('Ctrl Pts',(0.00454983340823832,-0.032303122220807,
0.0788646871262812));
#67378=CARTESIAN_POINT('Ctrl Pts',(0.00461544357275238,-0.0321934096576658,
0.0789130142282012));
#67379=CARTESIAN_POINT('Ctrl Pts',(0.00453350274530907,-0.0325229783203769,
0.078746201104978));
#67380=CARTESIAN_POINT('Ctrl Pts',(0.00459686127702891,-0.032413025309245,
0.0787956930286517));
#67381=CARTESIAN_POINT('Ctrl Pts',(0.00466123400320407,-0.0323031222208069,
0.078843866793287));
#67382=CARTESIAN_POINT('Ctrl Pts',(0.00472653628950603,-0.0321934096576658,
0.0788906636013482));
#67383=CARTESIAN_POINT('Ctrl Pts',(0.00464542430846719,-0.0325229783203769,
0.078728461151859));
#67384=CARTESIAN_POINT('Ctrl Pts',(0.00470853829532123,-0.032413025309245,
0.0787764102392321));
#67385=CARTESIAN_POINT('Ctrl Pts',(0.00477263459816983,-0.0323031222208069,
0.0788230464602929));
#67386=CARTESIAN_POINT('Ctrl Pts',(0.00483762900625968,-0.0321934096576658,
0.0788683129744954));
#67387=CARTESIAN_POINT('',(0.004669995880676,-0.0321934096584275,0.0789020389006892));
#67388=CARTESIAN_POINT('Ctrl Pts',(0.00449413748734713,-0.0322104233328918,
0.0789276227614162));
#67389=CARTESIAN_POINT('Ctrl Pts',(0.00452013605721095,-0.0322609421831359,
0.0788934014066515));
#67390=CARTESIAN_POINT('Ctrl Pts',(0.00454566678326801,-0.0323120888240719,
0.078859795864563));
#67391=CARTESIAN_POINT('Ctrl Pts',(0.00459581507590604,-0.032415652463181,
0.0787937867524388));
#67392=CARTESIAN_POINT('Ctrl Pts',(0.00462041202890994,-0.0324680267167315,
0.0787614103156084));
#67393=CARTESIAN_POINT('Ctrl Pts',(0.00464455084724232,-0.0325210109755913,
0.0787296369115297));
#67394=CARTESIAN_POINT('Origin',(0.00247765310163461,-0.0262834582511612,
0.0686705281165161));
#67395=CARTESIAN_POINT('Origin',(-0.00278525371840213,-0.034277076391757,
0.0795180575115256));
#67396=CARTESIAN_POINT('Ctrl Pts',(0.00474463215546422,-0.0326943950436604,
0.0788021636607871));
#67397=CARTESIAN_POINT('Ctrl Pts',(0.00480874768979384,-0.0325844576448134,
0.078848734681508));
#67398=CARTESIAN_POINT('Ctrl Pts',(0.00487383092674217,-0.0324744968375322,
0.0788939829837636));
#67399=CARTESIAN_POINT('Ctrl Pts',(0.00493979767822429,-0.0323646534831894,
0.0789378517429675));
#67400=CARTESIAN_POINT('Ctrl Pts',(0.00475996310022805,-0.0326943950436604,
0.0789144405048603));
#67401=CARTESIAN_POINT('Ctrl Pts',(0.00482562601989823,-0.0325844576448134,
0.078960800236429));
#67402=CARTESIAN_POINT('Ctrl Pts',(0.00489225238189191,-0.0324744968375322,
0.0790058052321134));
#67403=CARTESIAN_POINT('Ctrl Pts',(0.00495975602528217,-0.0323646534831894,
0.0790493990063364));
#67404=CARTESIAN_POINT('Ctrl Pts',(0.00477529404499188,-0.0326943950436604,
0.0790267173489334));
#67405=CARTESIAN_POINT('Ctrl Pts',(0.00484250435000262,-0.0325844576448134,
0.0790728657913501));
#67406=CARTESIAN_POINT('Ctrl Pts',(0.00491067383704165,-0.0324744968375322,
0.0791176274804633));
#67407=CARTESIAN_POINT('Ctrl Pts',(0.00497971437234006,-0.0323646534831894,
0.0791609462697054));
#67408=CARTESIAN_POINT('Ctrl Pts',(0.00479062498975571,-0.0326943950436604,
0.0791389941930066));
#67409=CARTESIAN_POINT('Ctrl Pts',(0.00485938268010701,-0.0325844576448134,
0.0791849313462711));
#67410=CARTESIAN_POINT('Ctrl Pts',(0.00492909529219139,-0.0324744968375322,
0.0792294497288132));
#67411=CARTESIAN_POINT('Ctrl Pts',(0.00499967271939794,-0.0323646534831894,
0.0792724935330743));
#67412=CARTESIAN_POINT('',(0.00480128917553514,-0.0326773559991376,0.0791461024937869));
#67413=CARTESIAN_POINT('',(0.00479062498975458,-0.0326943950436594,0.0791389941929943));
#67414=CARTESIAN_POINT('Origin',(0.0139545330167376,-0.0326395669258199,
0.0652914488846738));
#67415=CARTESIAN_POINT('Ctrl Pts',(0.00480128917738503,-0.0326773559987491,
0.0791461024909921));
#67416=CARTESIAN_POINT('Ctrl Pts',(0.0048250745901028,-0.032626792258723,
0.079110335866603));
#67417=CARTESIAN_POINT('Ctrl Pts',(0.00484843842355853,-0.0325756109581861,
0.0790752031797998));
#67418=CARTESIAN_POINT('Ctrl Pts',(0.00489434281593506,-0.0324719985462381,
0.0790061757813931));
#67419=CARTESIAN_POINT('Ctrl Pts',(0.00491686496369439,-0.0324196091621773,
0.0789723087550395));
#67420=CARTESIAN_POINT('Ctrl Pts',(0.00493897409648217,-0.0323666188837757,
0.0789390627879684));
#67421=CARTESIAN_POINT('',(0.00476776573896581,-0.0326943950436702,0.0789715834706288));
#67422=CARTESIAN_POINT('Origin',(0.00812378219310841,-0.0315241814719618,
0.07415));
#67423=CARTESIAN_POINT('',(0.0048012891755597,-0.0327114338379852,0.0791461024937492));
#67424=CARTESIAN_POINT('',(0.00481196851860964,-0.0326943950436593,0.0791531880022078));
#67425=CARTESIAN_POINT('Origin',(0.0139163806071854,-0.0326395657591289,
0.0652670033992444));
#67426=CARTESIAN_POINT('Origin',(0.0140382027957248,-0.0326395684823877,
0.0653470865582513));
#67427=CARTESIAN_POINT('Origin',(0.0140754969351185,-0.0326395672488115,
0.065372822803197));
#67428=CARTESIAN_POINT('Ctrl Pts',(0.0048060833965187,-0.0332451089994433,
0.078847978256134));
#67429=CARTESIAN_POINT('Ctrl Pts',(0.0049832705453824,-0.0329451141710254,
0.0789731073134659));
#67430=CARTESIAN_POINT('Ctrl Pts',(0.00516937955638642,-0.0326442513127493,
0.0790845344319531));
#67431=CARTESIAN_POINT('Ctrl Pts',(0.00501338117505318,-0.0332451089994433,
0.0789877195564523));
#67432=CARTESIAN_POINT('Ctrl Pts',(0.00519583875328712,-0.0329451141710254,
0.0791050302501518));
#67433=CARTESIAN_POINT('Ctrl Pts',(0.00538661430981726,-0.0326442513127493,
0.0792082642258664));
#67434=CARTESIAN_POINT('Ctrl Pts',(0.00501545415283852,-0.0332451089994433,
0.0789891169694555));
#67435=CARTESIAN_POINT('Ctrl Pts',(0.00519796443536617,-0.0329451141710254,
0.0791063494795187));
#67436=CARTESIAN_POINT('Ctrl Pts',(0.00538878665735157,-0.0326442513127493,
0.0792095015238055));
#67437=CARTESIAN_POINT('',(0.00504381185237201,-0.0331951640388616,0.0790071501624085));
#67438=CARTESIAN_POINT('',(0.0052459663372888,-0.0328677532355024,0.0791295884337797));
#67439=CARTESIAN_POINT('Origin',(0.0133632826850496,-0.0326402808283654,
0.0644531592131837));
#67440=CARTESIAN_POINT('Origin',(-0.000285797768402256,-0.032694427877906,
0.0887021517708994));
#67441=CARTESIAN_POINT('',(0.00513841974862762,-0.0326943950436593,0.0790658657503114));
#67442=CARTESIAN_POINT('',(0.00519253292458443,-0.0326943950436694,0.0790971389687191));
#67443=CARTESIAN_POINT('',(0.00493897409645284,-0.0330220786163545,0.0789390627880075));
#67444=CARTESIAN_POINT('Origin',(0.0137943810235266,-0.0326396682763673,
0.0646660133120013));
#67445=CARTESIAN_POINT('',(0.00493972638372129,-0.0331951640388587,0.0789379315578555));
#67446=CARTESIAN_POINT('Origin',(-0.00116903923235206,-0.033195202656002,
0.0881238094238224));
#67447=CARTESIAN_POINT('',(0.00499176911805666,-0.0331951640388701,0.0789725408601421));
#67448=CARTESIAN_POINT('Ctrl Pts',(0.00460801235427424,-0.0330240426238172,
0.0790120327477688));
#67449=CARTESIAN_POINT('Ctrl Pts',(0.00467499159222374,-0.0329142774063519,
0.0790604659025474));
#67450=CARTESIAN_POINT('Ctrl Pts',(0.00474300547036676,-0.0328043479726691,
0.0791075385550743));
#67451=CARTESIAN_POINT('Ctrl Pts',(0.00481196851860963,-0.0326943950436593,
0.0791531880022078));
#67452=CARTESIAN_POINT('Ctrl Pts',(0.00471859913403964,-0.0330240426238172,
0.0789873001756081));
#67453=CARTESIAN_POINT('Ctrl Pts',(0.00478523765671186,-0.0329142774063519,
0.0790342098897559));
#67454=CARTESIAN_POINT('Ctrl Pts',(0.00485287915594523,-0.0328043479726691,
0.0790797653856978));
#67455=CARTESIAN_POINT('Ctrl Pts',(0.00492143858516508,-0.0326943950436593,
0.0791239059170205));
#67456=CARTESIAN_POINT('Ctrl Pts',(0.00482918591380505,-0.0330240426238172,
0.0789625676034474));
#67457=CARTESIAN_POINT('Ctrl Pts',(0.00489548372119997,-0.0329142774063519,
0.0790079538769644));
#67458=CARTESIAN_POINT('Ctrl Pts',(0.0049627528415237,-0.0328043479726691,
0.0790519922163214));
#67459=CARTESIAN_POINT('Ctrl Pts',(0.00503090865172054,-0.0326943950436593,
0.0790946238318333));
#67460=CARTESIAN_POINT('Ctrl Pts',(0.00493977269357046,-0.0330240426238172,
0.0789378350312866));
#67461=CARTESIAN_POINT('Ctrl Pts',(0.00500572978568809,-0.0329142774063519,
0.0789816978641729));
#67462=CARTESIAN_POINT('Ctrl Pts',(0.00507262652710217,-0.0328043479726691,
0.079024219046945));
#67463=CARTESIAN_POINT('Ctrl Pts',(0.005140378718276,-0.0326943950436593,
0.079065341746646));
#67464=CARTESIAN_POINT('',(0.00497519413362863,-0.0326943950436693,0.0791095268762696));
#67465=CARTESIAN_POINT('Ctrl Pts',(0.0048012891773917,-0.0327114338383317,
0.0791461024909819));
#67466=CARTESIAN_POINT('Ctrl Pts',(0.00482507063387641,-0.0327619876831058,
0.0791103418156636));
#67467=CARTESIAN_POINT('Ctrl Pts',(0.00484843253495084,-0.0328131562604521,
0.0790752120346227));
#67468=CARTESIAN_POINT('Ctrl Pts',(0.00489433688505058,-0.0329167375858765,
0.0790061846997884));
#67469=CARTESIAN_POINT('Ctrl Pts',(0.00491686104343086,-0.0329691088920616,
0.078972314650022));
#67470=CARTESIAN_POINT('Ctrl Pts',(0.00493897409648142,-0.0330220786163187,
0.0789390627879694));
#67471=CARTESIAN_POINT('Ctrl Pts',(0.00504341184551566,-0.0331951640388604,
0.0790051619475543));
#67472=CARTESIAN_POINT('Ctrl Pts',(0.00514378920594111,-0.0330306422010619,
0.079068846629541));
#67473=CARTESIAN_POINT('Ctrl Pts',(0.00524671294949429,-0.0328657861914645,
0.0791283281915476));
#67474=CARTESIAN_POINT('Ctrl Pts',(0.00504381185236937,-0.0331951640388604,
0.0790071501624067));
#67475=CARTESIAN_POINT('Ctrl Pts',(0.00514423031786217,-0.0330306422010619,
0.0790708265745082));
#67476=CARTESIAN_POINT('Ctrl Pts',(0.00524719478955565,-0.0328657861914645,
0.0791302981747805));
#67477=CARTESIAN_POINT('Ctrl Pts',(0.00511046375141672,-0.0331951640388604,
0.0793384402250667));
#67478=CARTESIAN_POINT('Ctrl Pts',(0.00521773142655159,-0.0330306422010619,
0.0794007386518885));
#67479=CARTESIAN_POINT('Ctrl Pts',(0.00532748230170476,-0.0328657861914645,
0.0794585503593227));
#67480=CARTESIAN_POINT('',(0.00512155322654768,-0.0331781648281926,0.0793448648902783));
#67481=CARTESIAN_POINT('',(0.00511046375141491,-0.0331951640388588,0.0793384402250532));
#67482=CARTESIAN_POINT('Origin',(0.012764468923795,-0.0326412092392991,
0.0646965776852704));
#67483=CARTESIAN_POINT('Ctrl Pts',(0.00512155322577364,-0.033178164828644,
0.0793448648885998));
#67484=CARTESIAN_POINT('Ctrl Pts',(0.00514306068487822,-0.0331276811546798,
0.0793076497334389));
#67485=CARTESIAN_POINT('Ctrl Pts',(0.00516417975659762,-0.0330765663497826,
0.0792711065518096));
#67486=CARTESIAN_POINT('Ctrl Pts',(0.00520565941064976,-0.03297306144632,
0.0791993328197377));
#67487=CARTESIAN_POINT('Ctrl Pts',(0.00522600324074536,-0.0329207133373855,
0.0791641312670039));
#67488=CARTESIAN_POINT('Ctrl Pts',(0.00524596632082362,-0.032867753228938,
0.0791295884343284));
#67489=CARTESIAN_POINT('',(0.00507713780190345,-0.0331951640388701,0.0791727951937408));
#67490=CARTESIAN_POINT('Origin',(0.00812378219310841,-0.0315241814719618,
0.07415));
#67491=CARTESIAN_POINT('',(0.00512155322788321,-0.0332121607144399,0.0793448648892593));
#67492=CARTESIAN_POINT('',(0.00513265640034574,-0.0331951640388587,0.0793512658547611));
#67493=CARTESIAN_POINT('Origin',(0.0127218757545504,-0.0326413639142849,
0.0646810160177423));
#67494=CARTESIAN_POINT('Origin',(0.013997845151354,-0.0326412104312054,
0.0654093691303759));
#67495=CARTESIAN_POINT('Origin',(0.0140325894827513,-0.032641365465698,
0.0654385109720689));
#67496=CARTESIAN_POINT('Ctrl Pts',(0.00510760087554114,-0.0337436976235975,
0.0790470169756248));
#67497=CARTESIAN_POINT('Ctrl Pts',(0.00515164538838314,-0.0336723290703325,
0.0790741449675099));
#67498=CARTESIAN_POINT('Ctrl Pts',(0.00519617072292914,-0.033601104548885,
0.0791004763487643));
#67499=CARTESIAN_POINT('Ctrl Pts',(0.00533833129616268,-0.0333736987606857,
0.079184547233157));
#67500=CARTESIAN_POINT('Ctrl Pts',(0.00548508207211302,-0.0331450831799192,
0.0792603215820004));
#67501=CARTESIAN_POINT('Ctrl Pts',(0.00532326357010544,-0.0337436976235975,
0.0791734669743328));
#67502=CARTESIAN_POINT('Ctrl Pts',(0.00536844539339983,-0.0336723290703325,
0.0791986552632584));
#67503=CARTESIAN_POINT('Ctrl Pts',(0.00541407296526578,-0.033601104548885,
0.0792230267987213));
#67504=CARTESIAN_POINT('Ctrl Pts',(0.00555975276392098,-0.0333736987606857,
0.0793008402837251));
#67505=CARTESIAN_POINT('Ctrl Pts',(0.00570965788023112,-0.0331450831799192,
0.0793701655914324));
#67506=CARTESIAN_POINT('Ctrl Pts',(0.00532542019705108,-0.0337436976235975,
0.07917473147432));
#67507=CARTESIAN_POINT('Ctrl Pts',(0.00537061339345001,-0.0336723290703325,
0.0791999003662159));
#67508=CARTESIAN_POINT('Ctrl Pts',(0.00541625198768915,-0.033601104548885,
0.0792242523032209));
#67509=CARTESIAN_POINT('Ctrl Pts',(0.00556196697859858,-0.0333736987606857,
0.0793020032142308));
#67510=CARTESIAN_POINT('Ctrl Pts',(0.0057119036383123,-0.0331450831799192,
0.0793712640315267));
#67511=CARTESIAN_POINT('',(0.00535487245242893,-0.0336938721132548,0.0791909586239099));
#67512=CARTESIAN_POINT('',(0.00556431599105305,-0.0333679869945434,0.0793004618977903));
#67513=CARTESIAN_POINT('Ctrl Pts',(0.00535487245244038,-0.0336938721132648,
0.0791909586239173));
#67514=CARTESIAN_POINT('Ctrl Pts',(0.00537454967870561,-0.0336629187933932,
0.0792017669775535));
#67515=CARTESIAN_POINT('Ctrl Pts',(0.00539428389898122,-0.033631995230104,
0.0792124566563494));
#67516=CARTESIAN_POINT('Ctrl Pts',(0.00541407296527756,-0.033601104548895,
0.0792230267987281));
#67517=CARTESIAN_POINT('Ctrl Pts',(0.00546373050405251,-0.0335235892595454,
0.0792495509028554));
#67518=CARTESIAN_POINT('Ctrl Pts',(0.00551382170409883,-0.0334458668660369,
0.0792753693094286));
#67519=CARTESIAN_POINT('Ctrl Pts',(0.00556431599090787,-0.0333679869945385,
0.079300461898067));
#67520=CARTESIAN_POINT('Ctrl Pts',(0.00556435550900939,-0.0333679692459669,
0.0793004823036556));
#67521=CARTESIAN_POINT('Ctrl Pts',(0.00556455188975413,-0.0333391895374597,
0.079300073803441));
#67522=CARTESIAN_POINT('Ctrl Pts',(0.00556469616012824,-0.0333104081060613,
0.0792997662056888));
#67523=CARTESIAN_POINT('Ctrl Pts',(0.00556488211226626,-0.0332532698405432,
0.0792993566957794));
#67524=CARTESIAN_POINT('Ctrl Pts',(0.00556492529106622,-0.03322491721508,
0.0792992517812584));
#67525=CARTESIAN_POINT('Ctrl Pts',(0.00556492074556344,-0.0331960985328607,
0.0792992454237937));
#67526=CARTESIAN_POINT('Ctrl Pts',(0.00556492065866469,-0.0331956312596703,
0.0792992453473829));
#67527=CARTESIAN_POINT('Ctrl Pts',(0.0055649205590409,-0.0331951640388594,
0.0792992452978759));
#67528=CARTESIAN_POINT('',(0.00545298044386901,-0.0331951640388587,0.0792436178710481));
#67529=CARTESIAN_POINT('',(0.00550895050146465,-0.0331951640388687,0.0792714315844719));
#67530=CARTESIAN_POINT('',(0.00524596632831351,-0.0335216366567679,0.0791295884211258));
#67531=CARTESIAN_POINT('Origin',(0.0125088547087134,-0.0326434571528773,
0.0641422231621661));
#67532=CARTESIAN_POINT('',(0.00524664610052128,-0.0336938721132327,0.0791284121871067));
#67533=CARTESIAN_POINT('Origin',(-0.000217696129839952,-0.0336938867896336,
0.088583558613889));
#67534=CARTESIAN_POINT('',(0.0053007592764851,-0.0336938721132537,0.0791596854055182));
#67535=CARTESIAN_POINT('Ctrl Pts',(0.00492024029776362,-0.0335235895815172,
0.079223196164629));
#67536=CARTESIAN_POINT('Ctrl Pts',(0.00499008283117384,-0.0334144449262748,
0.079267299226012));
#67537=CARTESIAN_POINT('Ctrl Pts',(0.00506091674125023,-0.0333049234473147,
0.0793100100622914));
#67538=CARTESIAN_POINT('Ctrl Pts',(0.00513265640034556,-0.0331951640388587,
0.0793512658547612));
#67539=CARTESIAN_POINT('Ctrl Pts',(0.00502905603831519,-0.0335235895815172,
0.0791915685328141));
#67540=CARTESIAN_POINT('Ctrl Pts',(0.0050984631551044,-0.0334144449262748,
0.0792341735312899));
#67541=CARTESIAN_POINT('Ctrl Pts',(0.00516883019946658,-0.0333049234473147,
0.0792753935789491));
#67542=CARTESIAN_POINT('Ctrl Pts',(0.00524007196805507,-0.0331951640388587,
0.0793151678174233));
#67543=CARTESIAN_POINT('Ctrl Pts',(0.00513787177886675,-0.0335235895815172,
0.0791599409009992));
#67544=CARTESIAN_POINT('Ctrl Pts',(0.00520684347903495,-0.0334144449262748,
0.0792010478365679));
#67545=CARTESIAN_POINT('Ctrl Pts',(0.00527674365768294,-0.0333049234473147,
0.0792407770956068));
#67546=CARTESIAN_POINT('Ctrl Pts',(0.00534748753576459,-0.0331951640388587,
0.0792790697800854));
#67547=CARTESIAN_POINT('Ctrl Pts',(0.00524668751941831,-0.0335235895815172,
0.0791283132691844));
#67548=CARTESIAN_POINT('Ctrl Pts',(0.00531522380296551,-0.0334144449262748,
0.0791679221418459));
#67549=CARTESIAN_POINT('Ctrl Pts',(0.00538465711589929,-0.0333049234473147,
0.0792061606122645));
#67550=CARTESIAN_POINT('Ctrl Pts',(0.00545490310347411,-0.0331951640388587,
0.0792429717427476));
#67551=CARTESIAN_POINT('',(0.00529281842211738,-0.0331951640388687,0.0792974418629146));
#67552=CARTESIAN_POINT('Ctrl Pts',(0.00512155322944654,-0.033212160714597,
0.0793448648865405));
#67553=CARTESIAN_POINT('Ctrl Pts',(0.00514302451797355,-0.0332625444109832,
0.0793077123428178));
#67554=CARTESIAN_POINT('Ctrl Pts',(0.00516412582250511,-0.0333135300746992,
0.0792711999957257));
#67555=CARTESIAN_POINT('Ctrl Pts',(0.00520560521350614,-0.0334167203140571,
0.0791994267117975));
#67556=CARTESIAN_POINT('Ctrl Pts',(0.00522596723467659,-0.0334688847587259,
0.0791641935733269));
#67557=CARTESIAN_POINT('Ctrl Pts',(0.00524596632880189,-0.0335216366562323,
0.0791295884205915));
#67558=CARTESIAN_POINT('Ctrl Pts',(0.0053546140846346,-0.033693872113239,
0.0791899927248701));
#67559=CARTESIAN_POINT('Ctrl Pts',(0.00538411483450019,-0.0336474569764958,
0.0792062015847164));
#67560=CARTESIAN_POINT('Ctrl Pts',(0.00541380330812527,-0.033601104548885,
0.0792220639903966));
#67561=CARTESIAN_POINT('Ctrl Pts',(0.00548896769753591,-0.0334837508592656,
0.079262223954583));
#67562=CARTESIAN_POINT('Ctrl Pts',(0.00556528910329043,-0.0333660264659097,
0.0793001390067731));
#67563=CARTESIAN_POINT('Ctrl Pts',(0.00535487245241095,-0.033693872113239,
0.0791909586238999));
#67564=CARTESIAN_POINT('Ctrl Pts',(0.00538437885600408,-0.0336474569764958,
0.0792071659714339));
#67565=CARTESIAN_POINT('Ctrl Pts',(0.00541407296526578,-0.033601104548885,
0.0792230267987213));
#67566=CARTESIAN_POINT('Ctrl Pts',(0.00548925162281262,-0.0334837508592656,
0.0792631827667802));
#67567=CARTESIAN_POINT('Ctrl Pts',(0.00556558717202429,-0.0333660264659097,
0.0793010934018032));
#67568=CARTESIAN_POINT('Ctrl Pts',(0.00544271863782408,-0.033693872113239,
0.0795193685613193));
#67569=CARTESIAN_POINT('Ctrl Pts',(0.0054741473337589,-0.0336474569764958,
0.0795350617159796));
#67570=CARTESIAN_POINT('Ctrl Pts',(0.00550575758436879,-0.033601104548885,
0.0795503858827673));
#67571=CARTESIAN_POINT('Ctrl Pts',(0.00558578747126071,-0.0334837508592656,
0.0795891831498267));
#67572=CARTESIAN_POINT('Ctrl Pts',(0.0056669318583874,-0.0333660264659097,
0.0796255919285078));
#67573=CARTESIAN_POINT('',(0.00545366570538521,-0.0336769361243753,0.0795231255282181));
#67574=CARTESIAN_POINT('',(0.00544219470431035,-0.0336938721132327,0.0795174098539167));
#67575=CARTESIAN_POINT('Ctrl Pts',(0.00545366570538547,-0.033676936124375,
0.0795231255282182));
#67576=CARTESIAN_POINT('Ctrl Pts',(0.00545175271121779,-0.0336797586670124,
0.079522174886503));
#67577=CARTESIAN_POINT('Ctrl Pts',(0.00544984029708625,-0.0336825812713044,
0.079521223259117));
#67578=CARTESIAN_POINT('Ctrl Pts',(0.00544601663813532,-0.0336882265891408,
0.0795193180381814));
#67579=CARTESIAN_POINT('Ctrl Pts',(0.00544410539329454,-0.0336910493027062,
0.079518364444656));
#67580=CARTESIAN_POINT('Ctrl Pts',(0.00544219470431098,-0.0336938721132374,
0.0795174098539292));
#67581=CARTESIAN_POINT('Ctrl Pts',(0.00545366570538519,-0.0336769361243754,
0.079523125528218));
#67582=CARTESIAN_POINT('Ctrl Pts',(0.00547231772202003,-0.0336279018505232,
0.0794855917250323));
#67583=CARTESIAN_POINT('Ctrl Pts',(0.00549123807150779,-0.0335767826010773,
0.0794475179506085));
#67584=CARTESIAN_POINT('Ctrl Pts',(0.00552831108612262,-0.0334733172064623,
0.0793729152274124));
#67585=CARTESIAN_POINT('Ctrl Pts',(0.00554648866729878,-0.0334209631456245,
0.0793363361396069));
#67586=CARTESIAN_POINT('Ctrl Pts',(0.00556431598451702,-0.0333679869844681,
0.0793004618945372));
#67587=CARTESIAN_POINT('',(0.00539853357837964,-0.0336938721132538,0.0793541842389233));
#67588=CARTESIAN_POINT('Ctrl Pts',(0.00542099327985926,-0.0342436276873911,
0.0792267171568266));
#67589=CARTESIAN_POINT('Ctrl Pts',(0.00561246482387742,-0.0339430054201811,
0.0793286545211486));
#67590=CARTESIAN_POINT('Ctrl Pts',(0.00581107075726798,-0.0336441434784053,
0.0794158798708794));
#67591=CARTESIAN_POINT('Ctrl Pts',(0.00564416926297431,-0.0342436276873911,
0.0793393780664654));
#67592=CARTESIAN_POINT('Ctrl Pts',(0.00583988988324642,-0.0339430054201811,
0.0794328982098245));
#67593=CARTESIAN_POINT('Ctrl Pts',(0.00604209880213932,-0.0336441434784053,
0.0795114101932013));
#67594=CARTESIAN_POINT('Ctrl Pts',(0.00564640102280546,-0.0342436276873911,
0.0793405046755617));
#67595=CARTESIAN_POINT('Ctrl Pts',(0.00584216413384011,-0.0339430054201811,
0.0794339406467113));
#67596=CARTESIAN_POINT('Ctrl Pts',(0.00604440908258803,-0.0336441434784053,
0.0795123654964246));
#67597=CARTESIAN_POINT('',(0.00567686067421152,-0.034193496108874,0.0793548727247033));
#67598=CARTESIAN_POINT('',(0.0058927666861224,-0.0338664212863787,0.0794510088485209));
#67599=CARTESIAN_POINT('Origin',(0.0132545748800529,-0.0345610720405186,
0.0644340352423985));
#67600=CARTESIAN_POINT('Origin',(0.00163887119202861,-0.0336938005073097,
0.0895585850922207));
#67601=CARTESIAN_POINT('',(0.00577808157344143,-0.0336938721132327,0.0794012678091005));
#67602=CARTESIAN_POINT('',(0.00583568762442886,-0.0336938721132427,0.0794255122495204));
#67603=CARTESIAN_POINT('',(0.00556431598451228,-0.0340203938281605,0.0793004618945348));
#67604=CARTESIAN_POINT('Origin',(0.0136448814808393,-0.0345589643246379,
0.0647154557314726));
#67605=CARTESIAN_POINT('',(0.00556492055904032,-0.034193496108874,0.0792992452978757));
#67606=CARTESIAN_POINT('Origin',(0.000661051947683549,-0.0341934220717601,
0.0891673905593451));
#67607=CARTESIAN_POINT('',(0.00562089061663592,-0.0341934961088841,0.0793270590112994));
#67608=CARTESIAN_POINT('Ctrl Pts',(0.00567621460244076,-0.0341934961088741,
0.0793529502333115));
#67609=CARTESIAN_POINT('Ctrl Pts',(0.00578378149956862,-0.0340287516182428,
0.0794035517650258));
#67610=CARTESIAN_POINT('Ctrl Pts',(0.00589334788253513,-0.0338644633275951,
0.0794496642372343));
#67611=CARTESIAN_POINT('Ctrl Pts',(0.00567686067421154,-0.0341934961088741,
0.0793548727247032));
#67612=CARTESIAN_POINT('Ctrl Pts',(0.00578446731733436,-0.0340287516182428,
0.0794054608993926));
#67613=CARTESIAN_POINT('Ctrl Pts',(0.00589407286027767,-0.0338644633275951,
0.0794515583832574));
#67614=CARTESIAN_POINT('Ctrl Pts',(0.00578450865792822,-0.0341934961088741,
0.0796751967682377));
#67615=CARTESIAN_POINT('Ctrl Pts',(0.00589873774829603,-0.0340287516182428,
0.0797235594056701));
#67616=CARTESIAN_POINT('Ctrl Pts',(0.00601486809658658,-0.0338644633275951,
0.0797671595431882));
#67617=CARTESIAN_POINT('',(0.00579631591328774,-0.034176475883242,0.0796801808927925));
#67618=CARTESIAN_POINT('',(0.00578450865792329,-0.034193496108874,0.079675196768223));
#67619=CARTESIAN_POINT('Origin',(0.0126912500153698,-0.0345621026823869,
0.0646176043969201));
#67620=CARTESIAN_POINT('Ctrl Pts',(0.0057963159121418,-0.0341764758837524,
0.0796801808913685));
#67621=CARTESIAN_POINT('Ctrl Pts',(0.00581296673976368,-0.034126005004022,
0.0796406176237988));
#67622=CARTESIAN_POINT('Ctrl Pts',(0.00582932810150455,-0.034074926914769,
0.079601742044333));
#67623=CARTESIAN_POINT('Ctrl Pts',(0.00586148474250247,-0.0339715436305362,
0.0795253362037994));
#67624=CARTESIAN_POINT('Ctrl Pts',(0.00587726782772358,-0.0339192778237569,
0.0794878349318182));
#67625=CARTESIAN_POINT('Ctrl Pts',(0.00589276668396639,-0.0338664212855109,
0.0794510088488591));
#67626=CARTESIAN_POINT('',(0.00573068466607741,-0.0341934961088841,0.0795150347464732));
#67627=CARTESIAN_POINT('Origin',(0.00812378219310841,-0.0315241814719618,
0.07415));
#67628=CARTESIAN_POINT('',(0.00545366570596618,-0.0337108120655526,0.0795231255270644));
#67629=CARTESIAN_POINT('',(0.00546514888907052,-0.0336938721132327,0.079528816687218));
#67630=CARTESIAN_POINT('Origin',(0.0137355626301267,-0.0345562507985583,
0.0653686693265288));
#67631=CARTESIAN_POINT('Ctrl Pts',(0.0054651488890697,-0.0336938721132331,
0.0795288166872185));
#67632=CARTESIAN_POINT('Ctrl Pts',(0.00546323415082136,-0.0336910493194145,
0.079527870273319));
#67633=CARTESIAN_POINT('Ctrl Pts',(0.00546131985468562,-0.033688226597495,
0.0795269228057549));
#67634=CARTESIAN_POINT('Ctrl Pts',(0.00545749212905528,-0.033682581271305,
0.0795250257540697));
#67635=CARTESIAN_POINT('Ctrl Pts',(0.00545557869955279,-0.0336797586670127,
0.0795240761699332));
#67636=CARTESIAN_POINT('Ctrl Pts',(0.00545366570538492,-0.033676936124375,
0.0795231255282179));
#67637=CARTESIAN_POINT('Origin',(0.011733884582879,-0.0345562512720826,
0.0643739613533162));
#67638=CARTESIAN_POINT('Ctrl Pts',(0.0052451079780368,-0.0340223579322397,
0.0794143361180231));
#67639=CARTESIAN_POINT('Ctrl Pts',(0.00531771690306934,-0.0339125849573575,
0.0794540405433465));
#67640=CARTESIAN_POINT('Ctrl Pts',(0.00539109659599479,-0.0338030433565231,
0.0794922142328016));
#67641=CARTESIAN_POINT('Ctrl Pts',(0.00546514888906988,-0.0336938721132327,
0.0795288166872183));
#67642=CARTESIAN_POINT('Ctrl Pts',(0.00535172312814745,-0.0340223579322397,
0.0793759383368725));
#67643=CARTESIAN_POINT('Ctrl Pts',(0.0054238024476323,-0.0339125849573575,
0.0794141722612119));
#67644=CARTESIAN_POINT('Ctrl Pts',(0.00549662247120436,-0.0338030433565231,
0.0794508874445912));
#67645=CARTESIAN_POINT('Ctrl Pts',(0.00557008591218377,-0.0336938721132327,
0.0794860451895779));
#67646=CARTESIAN_POINT('Ctrl Pts',(0.0054583382782581,-0.0340223579322397,
0.0793375405557219));
#67647=CARTESIAN_POINT('Ctrl Pts',(0.00552988799219527,-0.0339125849573575,
0.0793743039790773));
#67648=CARTESIAN_POINT('Ctrl Pts',(0.00560214834641393,-0.0338030433565231,
0.0794095606563807));
#67649=CARTESIAN_POINT('Ctrl Pts',(0.00567502293529766,-0.0336938721132327,
0.0794432736919375));
#67650=CARTESIAN_POINT('Ctrl Pts',(0.00556495342836875,-0.0340223579322397,
0.0792991427745713));
#67651=CARTESIAN_POINT('Ctrl Pts',(0.00563597353675823,-0.0339125849573575,
0.0793344356969426));
#67652=CARTESIAN_POINT('Ctrl Pts',(0.0057076742216235,-0.0338030433565231,
0.0793682338681703));
#67653=CARTESIAN_POINT('Ctrl Pts',(0.00577995995841156,-0.0336938721132327,
0.0794005021942971));
#67654=CARTESIAN_POINT('',(0.00562161523126597,-0.0336938721132427,0.0794650422481692));
#67655=CARTESIAN_POINT('Ctrl Pts',(0.00545366570756543,-0.033710812066268,
0.0795231255238306));
#67656=CARTESIAN_POINT('Ctrl Pts',(0.00547280121137372,-0.0337611408994333,
0.0794846187903303));
#67657=CARTESIAN_POINT('Ctrl Pts',(0.0054915875346911,-0.0338121088781394,
0.0794468147192862));
#67658=CARTESIAN_POINT('Ctrl Pts',(0.00552847893437984,-0.0339153382773234,
0.0793725774632149));
#67659=CARTESIAN_POINT('Ctrl Pts',(0.00554656840343498,-0.0339675558473119,
0.0793361756850831));
#67660=CARTESIAN_POINT('Ctrl Pts',(0.00556431598453475,-0.0340203938281304,
0.0793004618945015));
#67661=CARTESIAN_POINT('Origin',(0.00812378219310841,-0.0315241814719618,
0.07415));
#67662=CARTESIAN_POINT('',(0.00579631591434876,-0.034210518019052,0.07968018089244));
#67663=CARTESIAN_POINT('',(0.00580813378883227,-0.034193496108874,0.0796851397875581));
#67664=CARTESIAN_POINT('Origin',(0.0126517817243141,-0.0345621697916885,
0.0645953120688972));
#67665=CARTESIAN_POINT('Origin',(0.0117472492764006,-0.0345621043445321,
0.0642203026984108));
#67666=CARTESIAN_POINT('Origin',(0.0117907777614704,-0.0345621710836054,
0.0642329490599898));
#67667=CARTESIAN_POINT('Ctrl Pts',(0.00577669901908363,-0.0346945769586965,
0.0794006859386861));
#67668=CARTESIAN_POINT('Ctrl Pts',(0.00588667673832936,-0.0345275153362944,
0.0794498465354869));
#67669=CARTESIAN_POINT('Ctrl Pts',(0.00599822895896659,-0.0343603235965185,
0.0794955611496933));
#67670=CARTESIAN_POINT('Ctrl Pts',(0.00611102374956819,-0.034193496108874,
0.0795376994812688));
#67671=CARTESIAN_POINT('Ctrl Pts',(0.005853967938694,-0.0346945769586965,
0.0794332058161165));
#67672=CARTESIAN_POINT('Ctrl Pts',(0.00596462679979276,-0.0345275153362944,
0.0794807479844593));
#67673=CARTESIAN_POINT('Ctrl Pts',(0.00607680944037584,-0.0343603235965185,
0.0795248223303149));
#67674=CARTESIAN_POINT('Ctrl Pts',(0.00619018213661502,-0.034193496108874,
0.0795653034325437));
#67675=CARTESIAN_POINT('Ctrl Pts',(0.00593123685830434,-0.0346945769586965,
0.0794657256935453));
#67676=CARTESIAN_POINT('Ctrl Pts',(0.00604257686125612,-0.0345275153362944,
0.0795116494334311));
#67677=CARTESIAN_POINT('Ctrl Pts',(0.00615538992178506,-0.0343603235965185,
0.0795540835109363));
#67678=CARTESIAN_POINT('Ctrl Pts',(0.00626934052366183,-0.034193496108874,
0.0795929073838184));
#67679=CARTESIAN_POINT('Ctrl Pts',(0.00600850577791472,-0.0346945769586965,
0.0794982455709775));
#67680=CARTESIAN_POINT('Ctrl Pts',(0.00612052692271955,-0.0345275153362944,
0.0795425508824042));
#67681=CARTESIAN_POINT('Ctrl Pts',(0.00623397040319434,-0.0343603235965185,
0.079583344691558));
#67682=CARTESIAN_POINT('Ctrl Pts',(0.00634849891070869,-0.034193496108874,
0.0796205113350935));
#67683=CARTESIAN_POINT('',(0.0060085057773564,-0.0346945769586966,0.0794982455707422));
#67684=CARTESIAN_POINT('',(0.00623002218382771,-0.0343667727831509,0.0795806351403604));
#67685=CARTESIAN_POINT('Origin',(0.0120218260819249,-0.0345626457063868,
0.0637967416251167));
#67686=CARTESIAN_POINT('Origin',(0.00259085538939692,-0.0341934771029017,
0.090016492532288));
#67687=CARTESIAN_POINT('',(0.00611244011171101,-0.034193496108874,0.0795381933921864));
#67688=CARTESIAN_POINT('',(0.00617145481132468,-0.034193496108884,0.0795587728778723));
#67689=CARTESIAN_POINT('',(0.0058927666846072,-0.0345211942962644,0.0794510088474529));
#67690=CARTESIAN_POINT('Origin',(0.0124636989864353,-0.0345625596120814,
0.063986317800692));
#67691=CARTESIAN_POINT('',(0.00589329367539629,-0.0346945769586885,0.0794497566899203));
#67692=CARTESIAN_POINT('Origin',(0.00160161318766902,-0.03469456858539,
0.0896470109187123));
#67693=CARTESIAN_POINT('',(0.00595089972638634,-0.0346945769587026,0.0794740011303412));
#67694=CARTESIAN_POINT('Ctrl Pts',(0.00558133965538096,-0.0345231616327842,
0.0795847020104502));
#67695=CARTESIAN_POINT('Ctrl Pts',(0.0056562493711466,-0.0344132092796988,
0.07961974600136));
#67696=CARTESIAN_POINT('Ctrl Pts',(0.00573188007922492,-0.034303273855898,
0.0796532387357783));
#67697=CARTESIAN_POINT('Ctrl Pts',(0.00580813378883211,-0.034193496108874,
0.0796851397875582));
#67698=CARTESIAN_POINT('Ctrl Pts',(0.00568533322408234,-0.0345231616327842,
0.0795396856377914));
#67699=CARTESIAN_POINT('Ctrl Pts',(0.00575962245252887,-0.0344132092796988,
0.0795732962237679));
#67700=CARTESIAN_POINT('Ctrl Pts',(0.00583460305645197,-0.034303273855898,
0.0796053684615008));
#67701=CARTESIAN_POINT('Ctrl Pts',(0.00591017792454178,-0.034193496108874,
0.0796358637233295));
#67702=CARTESIAN_POINT('Ctrl Pts',(0.00578932679278373,-0.0345231616327842,
0.0794946692651327));
#67703=CARTESIAN_POINT('Ctrl Pts',(0.00586299553391114,-0.0344132092796988,
0.0795268464461759));
#67704=CARTESIAN_POINT('Ctrl Pts',(0.00593732603367902,-0.034303273855898,
0.0795574981872233));
#67705=CARTESIAN_POINT('Ctrl Pts',(0.00601222206025146,-0.034193496108874,
0.0795865876591009));
#67706=CARTESIAN_POINT('Ctrl Pts',(0.00589332036148511,-0.0345231616327842,
0.079449652892474));
#67707=CARTESIAN_POINT('Ctrl Pts',(0.0059663686152934,-0.0344132092796988,
0.0794803966685838));
#67708=CARTESIAN_POINT('Ctrl Pts',(0.00604004901090607,-0.034303273855898,
0.0795096279129457));
#67709=CARTESIAN_POINT('Ctrl Pts',(0.00611426619596113,-0.034193496108874,
0.0795373115948722));
#67710=CARTESIAN_POINT('',(0.00596028695028164,-0.0341934961088839,0.0796116665898822));
#67711=CARTESIAN_POINT('Ctrl Pts',(0.00579631591568478,-0.0342105180195382,
0.0796801808892483));
#67712=CARTESIAN_POINT('Ctrl Pts',(0.00581298547473257,-0.0342610556241241,
0.0796405731502351));
#67713=CARTESIAN_POINT('Ctrl Pts',(0.00582935590716231,-0.0343122189870039,
0.0796016761516192));
#67714=CARTESIAN_POINT('Ctrl Pts',(0.00586151286878964,-0.0344158119695117,
0.0795252695388263));
#67715=CARTESIAN_POINT('Ctrl Pts',(0.00587728624555107,-0.0344681990450007,
0.0794877911755215));
#67716=CARTESIAN_POINT('Ctrl Pts',(0.00589276668461278,-0.0345211942962415,
0.0794510088474223));
#67717=CARTESIAN_POINT('Ctrl Pts',(0.00600774045365258,-0.0346945769586931,
0.0794963678999827));
#67718=CARTESIAN_POINT('Ctrl Pts',(0.00611827282701614,-0.034529677707698,
0.0795401155656829));
#67719=CARTESIAN_POINT('Ctrl Pts',(0.00623051888307191,-0.034364806625142,
0.0795792574449877));
#67720=CARTESIAN_POINT('Ctrl Pts',(0.00600850577734801,-0.0346945769586931,
0.0794982455707389));
#67721=CARTESIAN_POINT('Ctrl Pts',(0.00611907697022586,-0.034529677707698,
0.0795419774139132));
#67722=CARTESIAN_POINT('Ctrl Pts',(0.0062313611586656,-0.034364806625142,
0.0795811018797661));
#67723=CARTESIAN_POINT('Ctrl Pts',(0.00613605465547,-0.0346945769586931,
0.0798111782551212));
#67724=CARTESIAN_POINT('Ctrl Pts',(0.00625309551017338,-0.034529677707698,
0.0798522731154911));
#67725=CARTESIAN_POINT('Ctrl Pts',(0.00637173484327099,-0.034364806625142,
0.07988849545474));
#67726=CARTESIAN_POINT('',(0.00614815156770165,-0.0346775396665006,0.0798154111612007));
#67727=CARTESIAN_POINT('',(0.00613605465546712,-0.0346945769586885,0.0798111782551075));
#67728=CARTESIAN_POINT('Origin',(0.01147015549346,-0.0345626617707366,0.0640899802503613));
#67729=CARTESIAN_POINT('Ctrl Pts',(0.00614815156654657,-0.0346775396670096,
0.0798154111597802));
#67730=CARTESIAN_POINT('Ctrl Pts',(0.00616229647183186,-0.0346269749928212,
0.0797748485259631));
#67731=CARTESIAN_POINT('Ctrl Pts',(0.00617618995667073,-0.0345757902890838,
0.0797350067688319));
#67732=CARTESIAN_POINT('Ctrl Pts',(0.00620348569030341,-0.0344721681087949,
0.0796567322526532));
#67733=CARTESIAN_POINT('Ctrl Pts',(0.00621687724320778,-0.034419771428959,
0.0796183301827554));
#67734=CARTESIAN_POINT('Ctrl Pts',(0.00623002218355715,-0.0343667727830716,
0.0795806351403776));
#67735=CARTESIAN_POINT('',(0.00607228021642176,-0.0346945769587026,0.0796547119129349));
#67736=CARTESIAN_POINT('Origin',(0.00812378219310841,-0.0315241814719618,
0.07415));
#67737=CARTESIAN_POINT('',(0.00614815156878709,-0.0347116136489779,0.0798154111603306));
#67738=CARTESIAN_POINT('',(0.00616025749492668,-0.0346945769586885,0.0798196182199215));
#67739=CARTESIAN_POINT('Origin',(0.0114267900940531,-0.0345626675620375,
0.0640768340854252));
#67740=CARTESIAN_POINT('Origin',(0.0117585564508999,-0.0345626632792103,
0.0641905470644617));
#67741=CARTESIAN_POINT('Origin',(0.0118006907407996,-0.0345626691098713,
0.0642072234592839));
#67742=CARTESIAN_POINT('Ctrl Pts',(0.00607630495006719,-0.0352450361874068,
0.0795246249347493));
#67743=CARTESIAN_POINT('Ctrl Pts',(0.00627901225575353,-0.0349452760959492,
0.0796018468061226));
#67744=CARTESIAN_POINT('Ctrl Pts',(0.00648696035864053,-0.034644428984174,
0.0796635805546132));
#67745=CARTESIAN_POINT('Ctrl Pts',(0.00607866032480437,-0.0352450361874068,
0.0795254629143717));
#67746=CARTESIAN_POINT('Ctrl Pts',(0.00628139923541077,-0.0349452760959492,
0.079602595951329));
#67747=CARTESIAN_POINT('Ctrl Pts',(0.0064893721620599,-0.034644428984174,
0.0796642387371611));
#67748=CARTESIAN_POINT('Ctrl Pts',(0.00631419779852133,-0.0352450361874068,
0.0796092608766085));
#67749=CARTESIAN_POINT('Ctrl Pts',(0.00652009720113476,-0.0349452760959492,
0.0796775104719741));
#67750=CARTESIAN_POINT('Ctrl Pts',(0.00673055250399705,-0.034644428984174,
0.0797300569919472));
#67751=CARTESIAN_POINT('',(0.0063484673055885,-0.0351951633467143,0.0796205032826253));
#67752=CARTESIAN_POINT('',(0.0065747514882603,-0.0348678972925388,0.0796888291971714));
#67753=CARTESIAN_POINT('Origin',(0.010679534327633,-0.0345636767885608,
0.063445017347961));
#67754=CARTESIAN_POINT('Origin',(0.00359866410323816,-0.0346946199340881,
0.0903303466244583));
#67755=CARTESIAN_POINT('',(0.00645473648111493,-0.0346945769330289,0.0796538542322125));
#67756=CARTESIAN_POINT('',(0.00651492693357118,-0.0346945769458128,0.0796706875480123));
#67757=CARTESIAN_POINT('',(0.00623002218362052,-0.0350221583435276,0.0795806351402451));
#67758=CARTESIAN_POINT('Origin',(0.0111519882768809,-0.0345628458717012,
0.0635340715940157));
#67759=CARTESIAN_POINT('',(0.0062304265988768,-0.035195136029876,0.0795794662343274));
#67760=CARTESIAN_POINT('Origin',(0.00260219061514371,-0.0351951838366748,
0.0899839723495549));
#67761=CARTESIAN_POINT('',(0.00634849890504161,-0.0351951371328747,0.0796205113332404));
#67762=CARTESIAN_POINT('Ctrl Pts',(0.00592760524173035,-0.0350241211494343,
0.0797336195069392));
#67763=CARTESIAN_POINT('Ctrl Pts',(0.00600451731106532,-0.0349144232818962,
0.0797638709439768));
#67764=CARTESIAN_POINT('Ctrl Pts',(0.00608210073480112,-0.0348045283579412,
0.0797925506605261));
#67765=CARTESIAN_POINT('Ctrl Pts',(0.00616025750542763,-0.0346945769439157,
0.0798196182235583));
#67766=CARTESIAN_POINT('Ctrl Pts',(0.00602856701548103,-0.0350241211494343,
0.0796821621260871));
#67767=CARTESIAN_POINT('Ctrl Pts',(0.00610477028049311,-0.0349144232818962,
0.0797110228560873));
#67768=CARTESIAN_POINT('Ctrl Pts',(0.00618161572874426,-0.0348045283579412,
0.0797383256846858));
#67769=CARTESIAN_POINT('Ctrl Pts',(0.00625900623234884,-0.0346945769439157,
0.0797640319776473));
#67770=CARTESIAN_POINT('Ctrl Pts',(0.00612952878923171,-0.0350241211494343,
0.0796307047452351));
#67771=CARTESIAN_POINT('Ctrl Pts',(0.0062050232499209,-0.0349144232818962,
0.0796581747681978));
#67772=CARTESIAN_POINT('Ctrl Pts',(0.0062811307226874,-0.0348045283579412,
0.0796841007088454));
#67773=CARTESIAN_POINT('Ctrl Pts',(0.00635775495927005,-0.0346945769439157,
0.0797084457317363));
#67774=CARTESIAN_POINT('Ctrl Pts',(0.0062304905629824,-0.0350241211494343,
0.0795792473643831));
#67775=CARTESIAN_POINT('Ctrl Pts',(0.00630527621934869,-0.0349144232818962,
0.0796053266803083));
#67776=CARTESIAN_POINT('Ctrl Pts',(0.00638064571663054,-0.0348045283579412,
0.079629875733005));
#67777=CARTESIAN_POINT('Ctrl Pts',(0.00645650368619125,-0.0346945769439157,
0.0796528594858253));
#67778=CARTESIAN_POINT('',(0.00630749698772211,-0.0346945769458128,0.0797367362260666));
#67779=CARTESIAN_POINT('Ctrl Pts',(0.00614815156986566,-0.034711613649279,
0.079815411157218));
#67780=CARTESIAN_POINT('Ctrl Pts',(0.00616229087005735,-0.0347621546532189,
0.079774864635961));
#67781=CARTESIAN_POINT('Ctrl Pts',(0.00617618156314332,-0.0348133084096807,
0.0797350310321158));
#67782=CARTESIAN_POINT('Ctrl Pts',(0.00620347732784562,-0.0349168561544566,
0.079656756415358));
#67783=CARTESIAN_POINT('Ctrl Pts',(0.00621687157260909,-0.0349692089015912,
0.0796183464500372));
#67784=CARTESIAN_POINT('Ctrl Pts',(0.00623002218365135,-0.0350221583435,
0.0795806351402172));
#67785=CARTESIAN_POINT('Ctrl Pts',(0.00634786272464048,-0.035195137125491,
0.0796191938798822));
#67786=CARTESIAN_POINT('Ctrl Pts',(0.00646093487661855,-0.0350307338980939,
0.0796559099006431));
#67787=CARTESIAN_POINT('Ctrl Pts',(0.00657542792186249,-0.0348659306897824,
0.0796879211537307));
#67788=CARTESIAN_POINT('Ctrl Pts',(0.0063484989101211,-0.035195137125491,
0.0796205113348887));
#67789=CARTESIAN_POINT('Ctrl Pts',(0.00646159829965483,-0.0350307338980939,
0.079657214202914));
#67790=CARTESIAN_POINT('Ctrl Pts',(0.00657611801556334,-0.0348659306897824,
0.0796892111887473));
#67791=CARTESIAN_POINT('Ctrl Pts',(0.00645512425971208,-0.035195137125491,
0.0798413181670515));
#67792=CARTESIAN_POINT('Ctrl Pts',(0.00657278869196188,-0.0350307338980939,
0.0798758166228729));
#67793=CARTESIAN_POINT('Ctrl Pts',(0.00669177843904926,-0.0348659306897824,
0.0799054224020185));
#67794=CARTESIAN_POINT('Origin',(0.00514238959704072,-0.0308609197409829,
0.0848104887221482));
#67795=CARTESIAN_POINT('',(0.00639498515845967,-0.035195137125491,0.0797167781351773));
#67796=CARTESIAN_POINT('Origin',(0.00824783221874499,-0.0351840467441202,
0.0731807955630989));
#67797=CARTESIAN_POINT('Origin',(0.00567356812171042,-0.035232261387866,
0.0858617980372858));
#67798=CARTESIAN_POINT('',(0.00680393225277577,-0.0351951142564674,0.0797478398260794));
#67799=CARTESIAN_POINT('',(0.00692587718847221,-0.0351951372916787,0.0797738353105215));
#67800=CARTESIAN_POINT('Origin',(0.00844465116790654,-0.0352875118344055,
0.0740358531781859));
#67801=CARTESIAN_POINT('Origin',(0.00122044656463087,-0.029832507652323,
0.0712107573289516));
#67802=CARTESIAN_POINT('Origin',(0.00342050335947712,-0.0338732948498643,
0.0810873635885459));
#67803=CARTESIAN_POINT('Ctrl Pts',(0.00376541898641349,-0.0321934096636941,
0.0779027064771762));
#67804=CARTESIAN_POINT('Ctrl Pts',(0.00383259064532129,-0.032050846084365,
0.0779807191031296));
#67805=CARTESIAN_POINT('Ctrl Pts',(0.0039018077019054,-0.0319086045661724,
0.0780568681373702));
#67806=CARTESIAN_POINT('Ctrl Pts',(0.00397290762127662,-0.0317669892865887,
0.0781310018872401));
#67807=CARTESIAN_POINT('Ctrl Pts',(0.0038214972944457,-0.0321934096636941,
0.077965041507425));
#67808=CARTESIAN_POINT('Ctrl Pts',(0.00388978472071109,-0.032050846084365,
0.0780420503583689));
#67809=CARTESIAN_POINT('Ctrl Pts',(0.00396008973390662,-0.0319086045661724,
0.0781171663959826));
#67810=CARTESIAN_POINT('Ctrl Pts',(0.00403224763969298,-0.0317669892865887,
0.0781902403446855));
#67811=CARTESIAN_POINT('Ctrl Pts',(0.0038775756024779,-0.0321934096636941,
0.0780273765376737));
#67812=CARTESIAN_POINT('Ctrl Pts',(0.00394697879610091,-0.032050846084365,
0.0781033816136083));
#67813=CARTESIAN_POINT('Ctrl Pts',(0.00401837176590785,-0.0319086045661724,
0.078177464654595));
#67814=CARTESIAN_POINT('Ctrl Pts',(0.00409158765810936,-0.0317669892865887,
0.078249478802131));
#67815=CARTESIAN_POINT('Ctrl Pts',(0.00393365391051011,-0.0321934096636941,
0.0780897115679225));
#67816=CARTESIAN_POINT('Ctrl Pts',(0.00400417287149071,-0.032050846084365,
0.0781647128688477));
#67817=CARTESIAN_POINT('Ctrl Pts',(0.00407665379790908,-0.0319086045661724,
0.0782377629132073));
#67818=CARTESIAN_POINT('Ctrl Pts',(0.00415092767652572,-0.0317669892865887,
0.0783087172595763));
#67819=CARTESIAN_POINT('',(0.0039326506584995,-0.0321934096636941,0.0780885963819116));
#67820=CARTESIAN_POINT('',(0.00409800492356571,-0.0318665617511309,0.0782574617910789));
#67821=CARTESIAN_POINT('Origin',(0.0165223001385245,-0.0326371944419616,
0.0671013933342569));
#67822=CARTESIAN_POINT('Origin',(-0.00357449398580896,-0.0316939261508776,
0.0860856385078435));
#67823=CARTESIAN_POINT('',(0.00384825053644379,-0.0320197221621765,0.0779967412467433));
#67824=CARTESIAN_POINT('Ctrl Pts',(0.0038483350865036,-0.0320197392094679,
0.077996905764728));
#67825=CARTESIAN_POINT('Ctrl Pts',(0.00386790941467717,-0.0319792716575976,
0.0780186605827307));
#67826=CARTESIAN_POINT('Ctrl Pts',(0.0038877387026203,-0.0319386439829627,
0.0780403652101468));
#67827=CARTESIAN_POINT('Ctrl Pts',(0.00390785001136752,-0.0318979099381559,
0.0780620367281972));
#67828=CARTESIAN_POINT('Ctrl Pts',(0.00392796092259969,-0.0318571766984879,
0.0780837078178938));
#67829=CARTESIAN_POINT('Ctrl Pts',(0.0039482503207249,-0.0318163871833547,
0.0781052368648544));
#67830=CARTESIAN_POINT('Ctrl Pts',(0.00396864585605781,-0.0317755399638304,
0.0781265522329901));
#67831=CARTESIAN_POINT('',(0.00384904919316622,-0.0321934096636183,0.0779956674036122));
#67832=CARTESIAN_POINT('Origin',(0.00212289893016235,-0.0324157424817443,
0.0795772528035699));
#67833=CARTESIAN_POINT('',(0.00389084992584285,-0.0321934096636663,0.0780421318927719));
#67834=CARTESIAN_POINT('Ctrl Pts',(0.00393275767635423,-0.0321934096636618,
0.0780865709845288));
#67835=CARTESIAN_POINT('Ctrl Pts',(0.00398704605821487,-0.0320835708272592,
0.0781443684789084));
#67836=CARTESIAN_POINT('Ctrl Pts',(0.00404249906675006,-0.0319739230346488,
0.0782010089531512));
#67837=CARTESIAN_POINT('Ctrl Pts',(0.00409904019200004,-0.0318646057455572,
0.0782564253847822));
#67838=CARTESIAN_POINT('Ctrl Pts',(0.00392677847664008,-0.0321934096636618,
0.0781997319934329));
#67839=CARTESIAN_POINT('Ctrl Pts',(0.00398262743700604,-0.0320835708272592,
0.0782576119456364));
#67840=CARTESIAN_POINT('Ctrl Pts',(0.00403964182530797,-0.0319739230346488,
0.0783143025337832));
#67841=CARTESIAN_POINT('Ctrl Pts',(0.00409774312898821,-0.0318646057455572,
0.0783697368245971));
#67842=CARTESIAN_POINT('Ctrl Pts',(0.00392079927692593,-0.0321934096636617,
0.0783128930023369));
#67843=CARTESIAN_POINT('Ctrl Pts',(0.0039782088157972,-0.0320835708272592,
0.0783708554123644));
#67844=CARTESIAN_POINT('Ctrl Pts',(0.00403678458386588,-0.0319739230346488,
0.0784275961144152));
#67845=CARTESIAN_POINT('Ctrl Pts',(0.00409644606597639,-0.0318646057455572,
0.078483048264412));
#67846=CARTESIAN_POINT('Ctrl Pts',(0.00391482007721177,-0.0321934096636617,
0.0784260540112409));
#67847=CARTESIAN_POINT('Ctrl Pts',(0.00397379019458837,-0.0320835708272592,
0.0784840988790923));
#67848=CARTESIAN_POINT('Ctrl Pts',(0.00403392734242379,-0.0319739230346488,
0.0785408896950472));
#67849=CARTESIAN_POINT('Ctrl Pts',(0.00409514900296457,-0.0318646057455572,
0.078596359704227));
#67850=CARTESIAN_POINT('',(0.00392396340836445,-0.0321763980308298,0.0784350346734988));
#67851=CARTESIAN_POINT('',(0.00391482007723565,-0.0321934096636184,0.0784260540112524));
#67852=CARTESIAN_POINT('Origin',(0.0159370310552557,-0.0326386231710662,
0.0670546876297493));
#67853=CARTESIAN_POINT('Ctrl Pts',(0.00392396341057931,-0.0321763980306338,
0.0784350346712286));
#67854=CARTESIAN_POINT('Ctrl Pts',(0.00395400533963687,-0.0321259596176027,
0.0784043831802315));
#67855=CARTESIAN_POINT('Ctrl Pts',(0.0039835267532891,-0.0320749164633809,
0.0783742627660816));
#67856=CARTESIAN_POINT('Ctrl Pts',(0.00404155230793302,-0.0319716057793957,
0.0783150598513033));
#67857=CARTESIAN_POINT('Ctrl Pts',(0.0040700338400219,-0.0319193786690148,
0.0782860004183207));
#67858=CARTESIAN_POINT('Ctrl Pts',(0.00409800492485757,-0.0318665617525349,
0.0782574617897467));
#67859=CARTESIAN_POINT('',(0.00392373536787758,-0.0321934096636663,0.078257325196592));
#67860=CARTESIAN_POINT('Origin',(0.00812378219310841,-0.0315241814719618,
0.07415));
#67861=CARTESIAN_POINT('',(0.00392396340810453,-0.0322104233323765,0.0784350346737633));
#67862=CARTESIAN_POINT('',(0.00393312589888556,-0.0321934096636183,0.0784439957875769));
#67863=CARTESIAN_POINT('Origin',(0.0159093932547248,-0.0326387224835572,
0.067018750192623));
#67864=CARTESIAN_POINT('Origin',(0.015060738398086,-0.0326386249044207,
0.0661958168573123));
#67865=CARTESIAN_POINT('Origin',(0.0150972187277074,-0.0326387239258707,
0.0662227328979937));
#67866=CARTESIAN_POINT('Ctrl Pts',(0.00398450838954435,-0.0327445246967095,
0.078143061153943));
#67867=CARTESIAN_POINT('Ctrl Pts',(0.00413510915295419,-0.0324436878339359,
0.0782991764175831));
#67868=CARTESIAN_POINT('Ctrl Pts',(0.00429704131520911,-0.0321434074405927,
0.0784435043092344));
#67869=CARTESIAN_POINT('Ctrl Pts',(0.00416194824489146,-0.0327445246967095,
0.0783191721920251));
#67870=CARTESIAN_POINT('Ctrl Pts',(0.00431919114468679,-0.0324436878339359,
0.0784685952021174));
#67871=CARTESIAN_POINT('Ctrl Pts',(0.00448724248583043,-0.0321434074405927,
0.078605749539347));
#67872=CARTESIAN_POINT('',(0.00418822741220764,-0.0326943950436612,0.0783439877880759));
#67873=CARTESIAN_POINT('',(0.00436385853458972,-0.0323666188837389,0.0785021373004665));
#67874=CARTESIAN_POINT('Origin',(0.0156361235182012,-0.0326395579108916,
0.0660332716046196));
#67875=CARTESIAN_POINT('Origin',(-0.00285650192840184,-0.0321933825603126,
0.0868597545804409));
#67876=CARTESIAN_POINT('',(0.00427015733382251,-0.032193409653269,0.0784193911088875));
#67877=CARTESIAN_POINT('',(0.00431745200174686,-0.0321934096584275,0.0784602501927232));
#67878=CARTESIAN_POINT('',(0.00409800492289456,-0.032521010975624,0.0782574617917432));
#67879=CARTESIAN_POINT('Origin',(0.0159688902513804,-0.0326393129162593,
0.0663803317319811));
#67880=CARTESIAN_POINT('',(0.00409895585648136,-0.0326943950436592,0.0782564915633657));
#67881=CARTESIAN_POINT('Origin',(-0.00364442915373624,-0.0326943765538,
0.0861569918797376));
#67882=CARTESIAN_POINT('',(0.0041435916343545,-0.0326943950436702,0.0783002396757309));
#67883=CARTESIAN_POINT('Ctrl Pts',(0.00375923155673887,-0.0325229783203769,
0.0782671225076021));
#67884=CARTESIAN_POINT('Ctrl Pts',(0.00381598600047065,-0.032413025309245,
0.0783272877426781));
#67885=CARTESIAN_POINT('Ctrl Pts',(0.00387397643145428,-0.032303122220807,
0.0783862698139424));
#67886=CARTESIAN_POINT('Ctrl Pts',(0.00393312590209474,-0.0321934096576658,
0.0784439957907088));
#67887=CARTESIAN_POINT('Ctrl Pts',(0.0038724939906298,-0.0325229783203769,
0.0782635499307282));
#67888=CARTESIAN_POINT('Ctrl Pts',(0.0039291991864675,-0.032413025309245,
0.0783221538456299));
#67889=CARTESIAN_POINT('Ctrl Pts',(0.003987108079113,-0.032303122220807,
0.0783795758522807));
#67890=CARTESIAN_POINT('Ctrl Pts',(0.00404614389593064,-0.0321934096576658,
0.0784357450146406));
#67891=CARTESIAN_POINT('Ctrl Pts',(0.00398575642452073,-0.0325229783203769,
0.0782599773538543));
#67892=CARTESIAN_POINT('Ctrl Pts',(0.00404241237246435,-0.032413025309245,
0.0783170199485817));
#67893=CARTESIAN_POINT('Ctrl Pts',(0.00410023972677172,-0.032303122220807,
0.078372881890619));
#67894=CARTESIAN_POINT('Ctrl Pts',(0.00415916188976654,-0.0321934096576658,
0.0784274942385725));
#67895=CARTESIAN_POINT('Ctrl Pts',(0.00409901885841167,-0.0325229783203769,
0.0782564047769805));
#67896=CARTESIAN_POINT('Ctrl Pts',(0.00415562555846121,-0.032413025309245,
0.0783118860515336));
#67897=CARTESIAN_POINT('Ctrl Pts',(0.00421337137443044,-0.032303122220807,
0.0783661879289573));
#67898=CARTESIAN_POINT('Ctrl Pts',(0.00427217988360243,-0.0321934096576658,
0.0784192434625043));
#67899=CARTESIAN_POINT('',(0.00410164161590011,-0.0321934096584275,0.0784316934480136));
#67900=CARTESIAN_POINT('Ctrl Pts',(0.00392396341053566,-0.0322104233328918,
0.0784350346712731));
#67901=CARTESIAN_POINT('Ctrl Pts',(0.0039540460469616,-0.032260942183138,
0.0784043416469399));
#67902=CARTESIAN_POINT('Ctrl Pts',(0.00398358734687533,-0.0323120888240771,
0.0783742009430386));
#67903=CARTESIAN_POINT('Ctrl Pts',(0.00404161334071153,-0.0324156524631808,
0.0783149975801566));
#67904=CARTESIAN_POINT('Ctrl Pts',(0.00407007418291316,-0.0324680267167307,
0.0782859592568571));
#67905=CARTESIAN_POINT('Ctrl Pts',(0.00409800492292809,-0.0325210109755913,
0.0782574617917153));
#67906=CARTESIAN_POINT('Origin',(0.00320893444532068,-0.0262834582511651,
0.0680060877728064));
#67907=CARTESIAN_POINT('Origin',(-0.0033720415137391,-0.0342770802866463,
0.0781084632927795));
#67908=CARTESIAN_POINT('Ctrl Pts',(0.00418820704813744,-0.0326943950436604,
0.0783419601598709));
#67909=CARTESIAN_POINT('Ctrl Pts',(0.00424598011571114,-0.0325844576448134,
0.0783961997614225));
#67910=CARTESIAN_POINT('Ctrl Pts',(0.00430487903586174,-0.0324744968375322,
0.0784492483598374));
#67911=CARTESIAN_POINT('Ctrl Pts',(0.00436482740636163,-0.0323646534831894,
0.078501039027043));
#67912=CARTESIAN_POINT('Ctrl Pts',(0.00418934508390059,-0.0326943950436604,
0.0784552731443737));
#67913=CARTESIAN_POINT('Ctrl Pts',(0.00424867981677191,-0.0325844576448134,
0.0785094970616596));
#67914=CARTESIAN_POINT('Ctrl Pts',(0.00430914018836527,-0.0324744968375322,
0.0785624976769));
#67915=CARTESIAN_POINT('Ctrl Pts',(0.0043706477966784,-0.0323646534831894,
0.0786142081510959));
#67916=CARTESIAN_POINT('Ctrl Pts',(0.00419048311966374,-0.0326943950436604,
0.0785685861288765));
#67917=CARTESIAN_POINT('Ctrl Pts',(0.00425137951783268,-0.0325844576448134,
0.0786227943618967));
#67918=CARTESIAN_POINT('Ctrl Pts',(0.0043134013408688,-0.0324744968375322,
0.0786757469939626));
#67919=CARTESIAN_POINT('Ctrl Pts',(0.00437646818699518,-0.0323646534831894,
0.0787273772751487));
#67920=CARTESIAN_POINT('Ctrl Pts',(0.00419162115542689,-0.0326943950436604,
0.0786818991133793));
#67921=CARTESIAN_POINT('Ctrl Pts',(0.00425407921889344,-0.0325844576448134,
0.0787360916621338));
#67922=CARTESIAN_POINT('Ctrl Pts',(0.00431766249337233,-0.0324744968375322,
0.0787889963110252));
#67923=CARTESIAN_POINT('Ctrl Pts',(0.00438228857731196,-0.0323646534831894,
0.0788405463992016));
#67924=CARTESIAN_POINT('',(0.00420131034459516,-0.0326773559991372,0.0786902879399716));
#67925=CARTESIAN_POINT('',(0.00419162115542731,-0.0326943950436594,0.0786818991133677));
#67926=CARTESIAN_POINT('Origin',(0.0150188268209347,-0.0326395669851025,
0.0660920879965544));
#67927=CARTESIAN_POINT('Ctrl Pts',(0.00420131034678007,-0.0326773559987487,
0.0786902879374314));
#67928=CARTESIAN_POINT('Ctrl Pts',(0.00422939095110529,-0.0326267922587177,
0.0786577844462431));
#67929=CARTESIAN_POINT('Ctrl Pts',(0.00425697384699894,-0.0325756109581761,
0.0786258570559618));
#67930=CARTESIAN_POINT('Ctrl Pts',(0.00431116769657224,-0.032471998546238,
0.0785631273051464));
#67931=CARTESIAN_POINT('Ctrl Pts',(0.00433775691439304,-0.0324196091621782,
0.0785323501040173));
#67932=CARTESIAN_POINT('Ctrl Pts',(0.00436385853462161,-0.0323666188837756,
0.0785021373004296));
#67933=CARTESIAN_POINT('',(0.00418992428382747,-0.0326943950436702,0.0785129434507318));
#67934=CARTESIAN_POINT('Origin',(0.00812378219310841,-0.0315241814719618,
0.07415));
#67935=CARTESIAN_POINT('',(0.00420131034462419,-0.0327114338380035,0.0786902879399374));
#67936=CARTESIAN_POINT('',(0.00421101742817708,-0.0326943950436593,0.0786986560536431));
#67937=CARTESIAN_POINT('Origin',(0.014984038863885,-0.0326395658097383,
0.0660630537460898));
#67938=CARTESIAN_POINT('Origin',(0.0150948635439747,-0.0326395684242205,
0.0661577736041775));
#67939=CARTESIAN_POINT('Origin',(0.0151286377925338,-0.0326395672933506,
0.0661879811385929));
#67940=CARTESIAN_POINT('Ctrl Pts',(0.00424343163642233,-0.0332451089994433,
0.0783951153761972));
#67941=CARTESIAN_POINT('Ctrl Pts',(0.00440353878232574,-0.0329451141710254,
0.0785414651918511));
#67942=CARTESIAN_POINT('Ctrl Pts',(0.00457421474712319,-0.0326442513127493,
0.0786753393183718));
#67943=CARTESIAN_POINT('Ctrl Pts',(0.00443158058102485,-0.0332451089994433,
0.0785597360755183));
#67944=CARTESIAN_POINT('Ctrl Pts',(0.00459789649818397,-0.0329451141710254,
0.0786989897376274));
#67945=CARTESIAN_POINT('Ctrl Pts',(0.00477422908447897,-0.0326442513127493,
0.0788253201999939));
#67946=CARTESIAN_POINT('Ctrl Pts',(0.00443346207047087,-0.0332451089994433,
0.0785613822825115));
#67947=CARTESIAN_POINT('Ctrl Pts',(0.00459984007534255,-0.0329451141710254,
0.0787005649830851));
#67948=CARTESIAN_POINT('Ctrl Pts',(0.00477622922785252,-0.0326442513127493,
0.0788268200088102));
#67949=CARTESIAN_POINT('',(0.00445933600268922,-0.0331951640388616,0.0785828274405308));
#67950=CARTESIAN_POINT('',(0.00464455085464897,-0.032867753235502,0.0787296369248357));
#67951=CARTESIAN_POINT('Origin',(0.01453730406965,-0.0326402808282098,0.0651863052379474));
#67952=CARTESIAN_POINT('Origin',(-0.00204335396685721,-0.0326944278779124,
0.0875334038494764));
#67953=CARTESIAN_POINT('',(0.00454583887293236,-0.0326943950436593,0.078652937552044));
#67954=CARTESIAN_POINT('',(0.00459560577674832,-0.0326943950436694,0.0786907463511037));
#67955=CARTESIAN_POINT('',(0.0043638585345876,-0.0330220786163546,0.0785021373004647));
#67956=CARTESIAN_POINT('Origin',(0.0149383253770748,-0.0326396682765928,
0.0654515118674726));
#67957=CARTESIAN_POINT('',(0.00436474667057916,-0.0331951640388587,0.0785011092769963));
#67958=CARTESIAN_POINT('Origin',(-0.00284714542766966,-0.0331952026560193,
0.0868489222798781));
#67959=CARTESIAN_POINT('',(0.00441204133664418,-0.0331951640388701,0.0785419683587736));
#67960=CARTESIAN_POINT('Ctrl Pts',(0.00402636096358964,-0.0330240426238173,
0.0785330513649649));
#67961=CARTESIAN_POINT('Ctrl Pts',(0.00408674176634207,-0.032914277406352,
0.0785894973343257));
#67962=CARTESIAN_POINT('Ctrl Pts',(0.00414831956698752,-0.0328043479726691,
0.0786447232042023));
#67963=CARTESIAN_POINT('Ctrl Pts',(0.00421101742817707,-0.0326943950436593,
0.0786986560536431));
#67964=CARTESIAN_POINT('Ctrl Pts',(0.00413917554680919,-0.0330240426238173,
0.0785223740152204));
#67965=CARTESIAN_POINT('Ctrl Pts',(0.00419940925866645,-0.032914277406352,
0.0785772658537874));
#67966=CARTESIAN_POINT('Ctrl Pts',(0.0042608077668618,-0.0328043479726691,
0.078630939858859));
#67967=CARTESIAN_POINT('Ctrl Pts',(0.00432329430898262,-0.0326943950436593,
0.0786833251038636));
#67968=CARTESIAN_POINT('Ctrl Pts',(0.00425199013002873,-0.0330240426238173,
0.0785116966654759));
#67969=CARTESIAN_POINT('Ctrl Pts',(0.00431207675099082,-0.032914277406352,
0.078565034373249));
#67970=CARTESIAN_POINT('Ctrl Pts',(0.00437329596673607,-0.0328043479726691,
0.0786171565135158));
#67971=CARTESIAN_POINT('Ctrl Pts',(0.00443557118978818,-0.0326943950436593,
0.078667994154084));
#67972=CARTESIAN_POINT('Ctrl Pts',(0.00436480471324827,-0.0330240426238173,
0.0785010193157314));
#67973=CARTESIAN_POINT('Ctrl Pts',(0.0044247442433152,-0.032914277406352,
0.0785528028927107));
#67974=CARTESIAN_POINT('Ctrl Pts',(0.00448578416661034,-0.0328043479726691,
0.0786033731681725));
#67975=CARTESIAN_POINT('Ctrl Pts',(0.00454784807059373,-0.0326943950436593,
0.0786526632043045));
#67976=CARTESIAN_POINT('',(0.00437842815056471,-0.0326943950436694,0.0786757968028536));
#67977=CARTESIAN_POINT('Ctrl Pts',(0.00420131034678774,-0.0327114338383316,
0.0786902879374224));
#67978=CARTESIAN_POINT('Ctrl Pts',(0.00422938628036045,-0.0327619876829319,
0.078657789852662));
#67979=CARTESIAN_POINT('Ctrl Pts',(0.00425696689483702,-0.0328131562600878,
0.0786258651031487));
#67980=CARTESIAN_POINT('Ctrl Pts',(0.00431116069478636,-0.0329167375860513,
0.0785631354097734));
#67981=CARTESIAN_POINT('Ctrl Pts',(0.00433775228638831,-0.032969108892433,
0.0785323554609643));
#67982=CARTESIAN_POINT('Ctrl Pts',(0.00436385853462079,-0.0330220786163188,
0.0785021373004306));
#67983=CARTESIAN_POINT('Ctrl Pts',(0.00445918833940328,-0.0331951640388604,
0.0785808047691941));
#67984=CARTESIAN_POINT('Ctrl Pts',(0.00455079238723864,-0.0330306422010619,
0.0786565678976004));
#67985=CARTESIAN_POINT('Ctrl Pts',(0.00464544952982838,-0.0328657861914645,
0.0787284801953144));
#67986=CARTESIAN_POINT('Ctrl Pts',(0.00445933600268683,-0.0331951640388604,
0.0785828274405288));
#67987=CARTESIAN_POINT('Ctrl Pts',(0.00455098186795523,-0.0330306422010619,
0.0786585875160914));
#67988=CARTESIAN_POINT('Ctrl Pts',(0.00464568066606805,-0.0328657861914645,
0.0787304950352118));
#67989=CARTESIAN_POINT('Ctrl Pts',(0.00448394067680124,-0.0331951640388604,
0.0789198588801225));
#67990=CARTESIAN_POINT('Ctrl Pts',(0.00458255445099879,-0.0330306422010619,
0.0789951102698229));
#67991=CARTESIAN_POINT('Ctrl Pts',(0.00468419417948977,-0.0328657861914645,
0.0790662215467457));
#67992=CARTESIAN_POINT('',(0.00449413748404394,-0.0331781648281924,0.0789276227647071));
#67993=CARTESIAN_POINT('',(0.00448394067680124,-0.0331951640388588,0.0789198588801103));
#67994=CARTESIAN_POINT('Origin',(0.0139127037144764,-0.0326412092261607,
0.065352752982653));
#67995=CARTESIAN_POINT('Ctrl Pts',(0.00449413748348554,-0.033178164828644,
0.0789276227629457));
#67996=CARTESIAN_POINT('Ctrl Pts',(0.00452013964558557,-0.0331276811546787,
0.0788933966597935));
#67997=CARTESIAN_POINT('Ctrl Pts',(0.00454567226223526,-0.0330765663497806,
0.0788597885536142));
#67998=CARTESIAN_POINT('Ctrl Pts',(0.00459582047074767,-0.0329730614463256,
0.0787937795580319));
#67999=CARTESIAN_POINT('Ctrl Pts',(0.00462041580809327,-0.0329207133374001,
0.0787614053380697));
#68000=CARTESIAN_POINT('Ctrl Pts',(0.00464455083824491,-0.0328677532289377,
0.0787296369233164));
#68001=CARTESIAN_POINT('',(0.00447163833975523,-0.0331951640388701,0.0787513431603306));
#68002=CARTESIAN_POINT('Origin',(0.00812378219310841,-0.0315241814719618,
0.07415));
#68003=CARTESIAN_POINT('',(0.00449413748549661,-0.0332121607144209,0.0789276227638636));
#68004=CARTESIAN_POINT('',(0.00450435085242291,-0.0331951640388587,0.0789353648523489));
#68005=CARTESIAN_POINT('Origin',(0.0138723966468389,-0.0326413639619036,
0.0653319760184241));
#68006=CARTESIAN_POINT('Origin',(0.0150470180937759,-0.0326412103396109,
0.0662145069192957));
#68007=CARTESIAN_POINT('Origin',(0.0150778355420318,-0.0326413655861837,
0.0662477737448309));
#68008=CARTESIAN_POINT('Ctrl Pts',(0.00451762539374549,-0.0337436976235975,
0.0786303747765571));
#68009=CARTESIAN_POINT('Ctrl Pts',(0.00455792256350522,-0.0336723290703325,
0.0786628090973386));
#68010=CARTESIAN_POINT('Ctrl Pts',(0.00459879660533242,-0.033601104548885,
0.0786945133519412));
#68011=CARTESIAN_POINT('Ctrl Pts',(0.00472929932419518,-0.0333736987606857,
0.0787957387566284));
#68012=CARTESIAN_POINT('Ctrl Pts',(0.00486539588228306,-0.0331450831799191,
0.0788893083513764));
#68013=CARTESIAN_POINT('Ctrl Pts',(0.00471573913632553,-0.0337436976235975,
0.0787828573821255));
#68014=CARTESIAN_POINT('Ctrl Pts',(0.00475740775774911,-0.0336723290703325,
0.0788135098378812));
#68015=CARTESIAN_POINT('Ctrl Pts',(0.00479962097923611,-0.033601104548885,
0.0788434078476292));
#68016=CARTESIAN_POINT('Ctrl Pts',(0.00493439943347605,-0.0333736987606857,
0.0789388662702924));
#68017=CARTESIAN_POINT('Ctrl Pts',(0.00507443373818682,-0.0331450831799191,
0.079026433020197));
#68018=CARTESIAN_POINT('Ctrl Pts',(0.00471772027375133,-0.0337436976235975,
0.0787843822081812));
#68019=CARTESIAN_POINT('Ctrl Pts',(0.00475940260969155,-0.0336723290703325,
0.0788150168452867));
#68020=CARTESIAN_POINT('Ctrl Pts',(0.00480162922297515,-0.033601104548885,
0.0788448967925861));
#68021=CARTESIAN_POINT('Ctrl Pts',(0.00493645043456887,-0.0333736987606857,
0.0789402975454291));
#68022=CARTESIAN_POINT('Ctrl Pts',(0.00507652411674586,-0.0331450831799191,
0.0790278042668852));
#68023=CARTESIAN_POINT('',(0.00474490648816895,-0.0336938721132548,0.0788041727482519));
#68024=CARTESIAN_POINT('',(0.00493897410253327,-0.0333679869945434,0.0789390627920544));
#68025=CARTESIAN_POINT('Ctrl Pts',(0.00474490648817959,-0.0336938721132648,
0.078804172748261));
#68026=CARTESIAN_POINT('Ctrl Pts',(0.00476307390772768,-0.0336629187933932,
0.0788173620851958));
#68027=CARTESIAN_POINT('Ctrl Pts',(0.00478131274577295,-0.0336319952301039,
0.0788304408263207));
#68028=CARTESIAN_POINT('Ctrl Pts',(0.00479962097924727,-0.0336011045488949,
0.0788434078476377));
#68029=CARTESIAN_POINT('Ctrl Pts',(0.00484556260175928,-0.0335235892595453,
0.078875946541187));
#68030=CARTESIAN_POINT('Ctrl Pts',(0.00489202291335045,-0.0334458668660369,
0.0789078394539877));
#68031=CARTESIAN_POINT('Ctrl Pts',(0.00493897410235363,-0.0333679869945385,
0.0789390627923123));
#68032=CARTESIAN_POINT('Ctrl Pts',(0.00493901075134363,-0.0333679692460369,
0.0789390879899287));
#68033=CARTESIAN_POINT('Ctrl Pts',(0.00493925678222502,-0.0333391895373844,
0.0789387073238942));
#68034=CARTESIAN_POINT('Ctrl Pts',(0.00493943846720192,-0.0333104081058565,
0.0789384202335114));
#68035=CARTESIAN_POINT('Ctrl Pts',(0.00493967427870374,-0.0332532697311741,
0.0789380372579631));
#68036=CARTESIAN_POINT('Ctrl Pts',(0.00493973026308562,-0.0332249166699368,
0.0789379385812724));
#68037=CARTESIAN_POINT('Ctrl Pts',(0.00493972655318134,-0.0331960985551544,
0.0789379317062876));
#68038=CARTESIAN_POINT('Ctrl Pts',(0.00493972647635046,-0.0331956312372016,
0.0789379316194554));
#68039=CARTESIAN_POINT('Ctrl Pts',(0.00493972638372156,-0.0331951640388589,
0.0789379315578557));
#68040=CARTESIAN_POINT('',(0.00483564091507221,-0.0331951640388587,0.0788687129533036));
#68041=CARTESIAN_POINT('',(0.00488768364940674,-0.0331951640388687,0.0789033222555896));
#68042=CARTESIAN_POINT('',(0.0046445508473314,-0.0335216366567685,0.0787296369111558));
#68043=CARTESIAN_POINT('Origin',(0.013728584133644,-0.0326434571527307,
0.0647707327897084));
#68044=CARTESIAN_POINT('',(0.00464537268054423,-0.0336938721132327,0.0787285551501433));
#68045=CARTESIAN_POINT('Origin',(-0.00196092565071937,-0.0336938867896245,
0.0874242812441565));
#68046=CARTESIAN_POINT('',(0.00469513958436659,-0.0336938721132537,0.0787663639492076));
#68047=CARTESIAN_POINT('Ctrl Pts',(0.00430966110264114,-0.0335235895815172,
0.0787816822329784));
#68048=CARTESIAN_POINT('Ctrl Pts',(0.00437342532752126,-0.0334144449262748,
0.0788341911191021));
#68049=CARTESIAN_POINT('Ctrl Pts',(0.00443834760384049,-0.0333049234473147,
0.0788854430106762));
#68050=CARTESIAN_POINT('Ctrl Pts',(0.00450435085242276,-0.0331951640388587,
0.078935364852349));
#68051=CARTESIAN_POINT('Ctrl Pts',(0.00442158279194207,-0.0335235895815172,
0.0787639422231131));
#68052=CARTESIAN_POINT('Ctrl Pts',(0.00448510279065953,-0.0334144449262748,
0.07881491028683));
#68053=CARTESIAN_POINT('Ctrl Pts',(0.0045497487279985,-0.0333049234473147,
0.0788646246313078));
#68054=CARTESIAN_POINT('Ctrl Pts',(0.00461544370004225,-0.0331951640388587,
0.0789130141992537));
#68055=CARTESIAN_POINT('Ctrl Pts',(0.004533504481243,-0.0335235895815172,
0.0787462022132478));
#68056=CARTESIAN_POINT('Ctrl Pts',(0.00459678025379779,-0.0334144449262748,
0.078795629454558));
#68057=CARTESIAN_POINT('Ctrl Pts',(0.00466114985215651,-0.0333049234473147,
0.0788438062519395));
#68058=CARTESIAN_POINT('Ctrl Pts',(0.00472653654766174,-0.0331951640388587,
0.0788906635461584));
#68059=CARTESIAN_POINT('Ctrl Pts',(0.00464542617054393,-0.0335235895815172,
0.0787284622033826));
#68060=CARTESIAN_POINT('Ctrl Pts',(0.00470845771693606,-0.0334144449262748,
0.078776348622286));
#68061=CARTESIAN_POINT('Ctrl Pts',(0.00477255097631451,-0.0333049234473147,
0.0788229878725712));
#68062=CARTESIAN_POINT('Ctrl Pts',(0.00483762939528123,-0.0331951640388587,
0.0788683128930631));
#68063=CARTESIAN_POINT('',(0.00466999588375756,-0.0331951640388687,0.0789020389028363));
#68064=CARTESIAN_POINT('Ctrl Pts',(0.0044941374873876,-0.0332121607145971,
0.078927622761363));
#68065=CARTESIAN_POINT('Ctrl Pts',(0.00452009591683222,-0.033262544410985,
0.0788934542425632));
#68066=CARTESIAN_POINT('Ctrl Pts',(0.00454560704180172,-0.0333135300747026,
0.078859874500962));
#68067=CARTESIAN_POINT('Ctrl Pts',(0.00459575493317219,-0.0334167203140575,
0.0787938659170176));
#68068=CARTESIAN_POINT('Ctrl Pts',(0.00462037227689717,-0.0334688847587267,
0.0787614626403224));
#68069=CARTESIAN_POINT('Ctrl Pts',(0.00464455084788231,-0.0335216366562334,
0.0787296369106874));
#68070=CARTESIAN_POINT('Ctrl Pts',(0.00474477121693191,-0.0336938721132388,
0.0788031820835436));
#68071=CARTESIAN_POINT('Ctrl Pts',(0.00477200783575637,-0.0336474569764957,
0.0788229605560618));
#68072=CARTESIAN_POINT('Ctrl Pts',(0.00479947412030335,-0.033601104548885,
0.0788424188343343));
#68073=CARTESIAN_POINT('Ctrl Pts',(0.00486901243788165,-0.0334837508592656,
0.0788916827211816));
#68074=CARTESIAN_POINT('Ctrl Pts',(0.00493998001046396,-0.0333660264659097,
0.0789388644104339));
#68075=CARTESIAN_POINT('Ctrl Pts',(0.00474490648815247,-0.0336938721132388,
0.0788041727482399));
#68076=CARTESIAN_POINT('Ctrl Pts',(0.00477214890566613,-0.0336474569764957,
0.0788239504289708));
#68077=CARTESIAN_POINT('Ctrl Pts',(0.00479962097923612,-0.033601104548885,
0.0788434078476292));
#68078=CARTESIAN_POINT('Ctrl Pts',(0.00486917395328969,-0.0334837508592656,
0.0788926695581313));
#68079=CARTESIAN_POINT('Ctrl Pts',(0.0049401561114216,-0.0333660264659097,
0.0789398486376924));
#68080=CARTESIAN_POINT('Ctrl Pts',(0.00479089930076365,-0.0336938721132388,
0.0791410031216843));
#68081=CARTESIAN_POINT('Ctrl Pts',(0.00482011329822525,-0.0336474569764957,
0.079160511591221));
#68082=CARTESIAN_POINT('Ctrl Pts',(0.00484955366519232,-0.033601104548885,
0.0791796767372991));
#68083=CARTESIAN_POINT('Ctrl Pts',(0.00492408990558829,-0.0334837508592656,
0.0792281984808254));
#68084=CARTESIAN_POINT('Ctrl Pts',(0.00500003121502358,-0.0333660264659097,
0.079274490253836));
#68085=CARTESIAN_POINT('',(0.00480128917461756,-0.0336769361243754,0.0791461024951536));
#68086=CARTESIAN_POINT('',(0.00479062498975413,-0.033693872113232,0.0791389941929939));
#68087=CARTESIAN_POINT('Ctrl Pts',(0.00480128917461775,-0.033676936124375,
0.0791461024951537));
#68088=CARTESIAN_POINT('Ctrl Pts',(0.00479951041199867,-0.0336797586669838,
0.0791449195877995));
#68089=CARTESIAN_POINT('Ctrl Pts',(0.0047977323483792,-0.0336825812712471,
0.0791437357752447));
#68090=CARTESIAN_POINT('Ctrl Pts',(0.00479417762654158,-0.0336882265907989,
0.0791413663452849));
#68091=CARTESIAN_POINT('Ctrl Pts',(0.00479240096835471,-0.0336910493060223,
0.0791401807279334));
#68092=CARTESIAN_POINT('Ctrl Pts',(0.00479062498975387,-0.0336938721132366,
0.0791389941930052));
#68093=CARTESIAN_POINT('Ctrl Pts',(0.00480128917461751,-0.0336769361243754,
0.0791461024951536));
#68094=CARTESIAN_POINT('Ctrl Pts',(0.00482449834745087,-0.0336279018505242,
0.0791112023747748));
#68095=CARTESIAN_POINT('Ctrl Pts',(0.00484804141359443,-0.0335767826010779,
0.0790758001720155));
#68096=CARTESIAN_POINT('Ctrl Pts',(0.00489417229694787,-0.0334733172064603,
0.0790064321943725));
#68097=CARTESIAN_POINT('Ctrl Pts',(0.00491679111782316,-0.033420963145621,
0.0789724197986262));
#68098=CARTESIAN_POINT('Ctrl Pts',(0.00493897409645518,-0.033367986984468,
0.078939062788009));
#68099=CARTESIAN_POINT('',(0.00476776573897154,-0.0336938721132534,0.0789715834706329));
#68100=CARTESIAN_POINT('Origin',(0.00812378219310841,-0.0315241814719618,
0.07415));
#68101=CARTESIAN_POINT('',(0.00480128917533939,-0.0337108120655664,0.0791461024940809));
#68102=CARTESIAN_POINT('',(0.00481196851860953,-0.0336938721132327,0.0791531880022078));
#68103=CARTESIAN_POINT('Origin',(0.0147919046467725,-0.0345562508791708,
0.0661412555029351));
#68104=CARTESIAN_POINT('Ctrl Pts',(0.00481196851861003,-0.0336938721132325,
0.0791531880022075));
#68105=CARTESIAN_POINT('Ctrl Pts',(0.00481018749777614,-0.0336910493226109,
0.0791520090720634));
#68106=CARTESIAN_POINT('Ctrl Pts',(0.00480840704459998,-0.0336882265990933,
0.0791508291499735));
#68107=CARTESIAN_POINT('Ctrl Pts',(0.00480484726436342,-0.0336825812713364,
0.0791484673152215));
#68108=CARTESIAN_POINT('Ctrl Pts',(0.00480306793726456,-0.0336797586670285,
0.0791472854025262));
#68109=CARTESIAN_POINT('Ctrl Pts',(0.00480128917461733,-0.0336769361243751,
0.0791461024951534));
#68110=CARTESIAN_POINT('Origin',(0.0129306800696285,-0.0345562513805278,
0.0649035143543814));
#68111=CARTESIAN_POINT('Ctrl Pts',(0.00480602420056776,-0.034243627687391,
0.0788479364515639));
#68112=CARTESIAN_POINT('Ctrl Pts',(0.00498320979478004,-0.0339430054201809,
0.0789730677570683));
#68113=CARTESIAN_POINT('Ctrl Pts',(0.00516931742593454,-0.0336441434784052,
0.0790844972327005));
#68114=CARTESIAN_POINT('Ctrl Pts',(0.00501332021829518,-0.034243627687391,
0.0789876803638976));
#68115=CARTESIAN_POINT('Ctrl Pts',(0.00519577634104691,-0.0339430054201809,
0.0791049933712071));
#68116=CARTESIAN_POINT('Ctrl Pts',(0.00538655062146727,-0.0336441434784052,
0.0792082297618051));
#68117=CARTESIAN_POINT('Ctrl Pts',(0.00501539317847246,-0.034243627687391,
0.078989077803021));
#68118=CARTESIAN_POINT('Ctrl Pts',(0.00519790200650957,-0.0339430054201809,
0.0791063126273486));
#68119=CARTESIAN_POINT('Ctrl Pts',(0.00538872295342259,-0.0336441434784052,
0.0792094670870962));
#68120=CARTESIAN_POINT('',(0.00504381185237035,-0.0341934961088741,0.0790071501624075));
#68121=CARTESIAN_POINT('',(0.00524596632995467,-0.0338664212894231,0.0791295884229386));
#68122=CARTESIAN_POINT('Origin',(0.0144318607449391,-0.0345610818077284,
0.0651537162091521));
#68123=CARTESIAN_POINT('Origin',(-0.000241169198642399,-0.0336938005044516,
0.0886243284210318));
#68124=CARTESIAN_POINT('',(0.00513841974862763,-0.0336938721132327,0.0790658657503114));
#68125=CARTESIAN_POINT('',(0.00519253292458446,-0.0336938721132427,0.079097138968719));
#68126=CARTESIAN_POINT('',(0.00493897409645077,-0.0340203938281605,0.0789390627880061));
#68127=CARTESIAN_POINT('Origin',(0.0147838079042916,-0.0345589643245868,
0.0654818271573763));
#68128=CARTESIAN_POINT('',(0.00493972638372135,-0.034193496108874,0.0789379315578555));
#68129=CARTESIAN_POINT('Origin',(-0.00116228036178326,-0.0341934220717766,
0.088113645806421));
#68130=CARTESIAN_POINT('',(0.00499176911805584,-0.0341934961088841,0.0789725408601415));
#68131=CARTESIAN_POINT('Ctrl Pts',(0.00460801091579982,-0.0340223579322397,
0.0790120317075984));
#68132=CARTESIAN_POINT('Ctrl Pts',(0.00467507101375865,-0.0339125849573575,
0.0790605233630289));
#68133=CARTESIAN_POINT('Ctrl Pts',(0.00474308765395145,-0.0338030433565231,
0.079107592955733));
#68134=CARTESIAN_POINT('Ctrl Pts',(0.00481196851860885,-0.0336938721132327,
0.079153188002208));
#68135=CARTESIAN_POINT('Ctrl Pts',(0.00471859789168073,-0.0340223579322397,
0.0789872991259313));
#68136=CARTESIAN_POINT('Ctrl Pts',(0.0047853168628331,-0.0339125849573575,
0.0790342654985415));
#68137=CARTESIAN_POINT('Ctrl Pts',(0.00485296104611517,-0.0338030433565231,
0.0790798179407561));
#68138=CARTESIAN_POINT('Ctrl Pts',(0.00492143877205597,-0.0336938721132327,
0.0791239058670292));
#68139=CARTESIAN_POINT('Ctrl Pts',(0.00482918486756165,-0.0340223579322397,
0.0789625665442643));
#68140=CARTESIAN_POINT('Ctrl Pts',(0.00489556271190754,-0.0339125849573575,
0.0790080076340541));
#68141=CARTESIAN_POINT('Ctrl Pts',(0.00496283443827889,-0.0338030433565231,
0.0790520429257791));
#68142=CARTESIAN_POINT('Ctrl Pts',(0.00503090902550308,-0.0336938721132327,
0.0790946237318504));
#68143=CARTESIAN_POINT('Ctrl Pts',(0.00493977184344256,-0.0340223579322397,
0.0789378339625972));
#68144=CARTESIAN_POINT('Ctrl Pts',(0.00500580856098198,-0.0339125849573575,
0.0789817497695667));
#68145=CARTESIAN_POINT('Ctrl Pts',(0.00507270783044261,-0.0338030433565231,
0.0790242679108022));
#68146=CARTESIAN_POINT('Ctrl Pts',(0.0051403792789502,-0.0336938721132327,
0.0790653415966716));
#68147=CARTESIAN_POINT('',(0.00497519413362858,-0.0336938721132427,0.0791095268762696));
#68148=CARTESIAN_POINT('Ctrl Pts',(0.00480128917733045,-0.0337108120662679,
0.0791461024910741));
#68149=CARTESIAN_POINT('Ctrl Pts',(0.00482509996540099,-0.0337611408994367,
0.0791102977092344));
#68150=CARTESIAN_POINT('Ctrl Pts',(0.00484847625941539,-0.033812108878147,
0.0790751462852275));
#68151=CARTESIAN_POINT('Ctrl Pts',(0.0048943811547497,-0.0339153382773236,
0.0790061181305126));
#68152=CARTESIAN_POINT('Ctrl Pts',(0.00491689033549877,-0.0339675558473114,
0.0789722706029247));
#68153=CARTESIAN_POINT('Ctrl Pts',(0.00493897409647724,-0.0340203938281304,
0.0789390627879758));
#68154=CARTESIAN_POINT('Ctrl Pts',(0.00504341182756386,-0.0341934961088741,
0.0790051618583216));
#68155=CARTESIAN_POINT('Ctrl Pts',(0.00514378847330114,-0.0340287516194401,
0.0790688460884141));
#68156=CARTESIAN_POINT('Ctrl Pts',(0.00524671146664077,-0.033864463329982,
0.0791283272586611));
#68157=CARTESIAN_POINT('Ctrl Pts',(0.00504381185237033,-0.0341934961088741,
0.0790071501624074));
#68158=CARTESIAN_POINT('Ctrl Pts',(0.00514422960472787,-0.0340287516194401,
0.0790708261223022));
#68159=CARTESIAN_POINT('Ctrl Pts',(0.00524719332774941,-0.033864463329982,
0.0791302973304505));
#68160=CARTESIAN_POINT('Ctrl Pts',(0.00511046375141771,-0.0341934961088741,
0.0793384402250671));
#68161=CARTESIAN_POINT('Ctrl Pts',(0.00521773066477672,-0.0340287516194401,
0.0794007382094683));
#68162=CARTESIAN_POINT('Ctrl Pts',(0.00532748074355059,-0.033864463329982,
0.0794585495385583));
#68163=CARTESIAN_POINT('',(0.00512155322659617,-0.0341764758832416,0.079344864889805));
#68164=CARTESIAN_POINT('',(0.0051104637514149,-0.034193496108874,0.0793384402250532));
#68165=CARTESIAN_POINT('Origin',(0.0138499602326468,-0.0345621026920888,
0.0652652255464296));
#68166=CARTESIAN_POINT('Ctrl Pts',(0.00512155322563717,-0.0341764758837518,
0.0793448648882492));
#68167=CARTESIAN_POINT('Ctrl Pts',(0.00514303134858548,-0.0341260050044428,
0.079307700491239));
#68168=CARTESIAN_POINT('Ctrl Pts',(0.00516413609801035,-0.034074926915621,
0.0792711820800005));
#68169=CARTESIAN_POINT('Ctrl Pts',(0.00520561536501873,-0.0339715436322559,
0.0791994090187048));
#68170=CARTESIAN_POINT('Ctrl Pts',(0.00522597415170171,-0.0339192778251916,
0.0791641816003481));
#68171=CARTESIAN_POINT('Ctrl Pts',(0.00524596632672147,-0.0338664212874305,
0.0791295884241146));
#68172=CARTESIAN_POINT('',(0.00507713780190263,-0.0341934961088841,0.0791727951937404));
#68173=CARTESIAN_POINT('Ctrl Pts',(0.00513712102382444,-0.0346945769586966,
0.0790651151881108));
#68174=CARTESIAN_POINT('Ctrl Pts',(0.00524007007934417,-0.0345275153362944,
0.0791276720020953));
#68175=CARTESIAN_POINT('Ctrl Pts',(0.005345013116983,-0.0343603235965185,
0.0791870073434382));
#68176=CARTESIAN_POINT('Ctrl Pts',(0.00545163715361716,-0.034193496108874,
0.0792429503375184));
#68177=CARTESIAN_POINT('Ctrl Pts',(0.0052097048335311,-0.0346945769586966,
0.0791070630001433));
#68178=CARTESIAN_POINT('Ctrl Pts',(0.00531353250276884,-0.0345275153362944,
0.0791680995171725));
#68179=CARTESIAN_POINT('Ctrl Pts',(0.00541930656944027,-0.0343603235965185,
0.0792258865367407));
#68180=CARTESIAN_POINT('Ctrl Pts',(0.00552671166066623,-0.034193496108874,
0.0792802578000049));
#68181=CARTESIAN_POINT('Ctrl Pts',(0.00528228864323767,-0.0346945769586966,
0.0791490108121771));
#68182=CARTESIAN_POINT('Ctrl Pts',(0.00538699492619351,-0.0345275153362944,
0.0792085270322502));
#68183=CARTESIAN_POINT('Ctrl Pts',(0.00549360002189762,-0.0343603235965185,
0.079264765730044));
#68184=CARTESIAN_POINT('Ctrl Pts',(0.00560178616771541,-0.034193496108874,
0.0793175652624937));
#68185=CARTESIAN_POINT('Ctrl Pts',(0.00535487245294441,-0.0346945769586966,
0.0791909586242082));
#68186=CARTESIAN_POINT('Ctrl Pts',(0.00546045734961816,-0.0345275153362944,
0.0792489545473269));
#68187=CARTESIAN_POINT('Ctrl Pts',(0.00556789347435482,-0.0343603235965185,
0.0793036449233458));
#68188=CARTESIAN_POINT('Ctrl Pts',(0.00567686067476436,-0.034193496108874,
0.0793548727249779));
#68189=CARTESIAN_POINT('',(0.00535487245241997,-0.0346945769586966,0.0791909586239049));
#68190=CARTESIAN_POINT('',(0.00556431598469133,-0.0343667727831502,0.0793004618946675));
#68191=CARTESIAN_POINT('Origin',(0.0132886961920314,-0.0345626457065727,
0.0643669346046938));
#68192=CARTESIAN_POINT('Origin',(0.000645886075255295,-0.0341934771029131,
0.0891979212485602));
#68193=CARTESIAN_POINT('',(0.00545298044386904,-0.034193496108874,0.0792436178710481));
#68194=CARTESIAN_POINT('',(0.00550895050146468,-0.034193496108884,0.0792714315844719));
#68195=CARTESIAN_POINT('',(0.00524596632826059,-0.034521194296265,0.0791295884215426));
#68196=CARTESIAN_POINT('Origin',(0.0137033246011917,-0.0345625596120016,
0.0646103972754862));
#68197=CARTESIAN_POINT('',(0.00524664610052137,-0.0346945769586885,0.0791284121871068));
#68198=CARTESIAN_POINT('Origin',(-0.00028924817164534,-0.0346945685853917,
0.0887073677574834));
#68199=CARTESIAN_POINT('',(0.00530075927648067,-0.0346945769587026,0.0791596854055159));
#68200=CARTESIAN_POINT('Ctrl Pts',(0.00535434849807001,-0.0346945769586932,
0.0791889998386456));
#68201=CARTESIAN_POINT('Ctrl Pts',(0.00545852625425208,-0.034529677707698,
0.079246255920702));
#68202=CARTESIAN_POINT('Ctrl Pts',(0.00556498143832853,-0.034364806625142,
0.0792991573157578));
#68203=CARTESIAN_POINT('Ctrl Pts',(0.00535487245241206,-0.0346945769586932,
0.0791909586239005));
#68204=CARTESIAN_POINT('Ctrl Pts',(0.00545909070509329,-0.034529677707698,
0.0792482038735716));
#68205=CARTESIAN_POINT('Ctrl Pts',(0.0055655859033527,-0.034364806625142,
0.0793010927717408));
#68206=CARTESIAN_POINT('Ctrl Pts',(0.00544219470431115,-0.0346945769586932,
0.0795174098539296));
#68207=CARTESIAN_POINT('Ctrl Pts',(0.00555316210518375,-0.034529677707698,
0.0795728497778299));
#68208=CARTESIAN_POINT('Ctrl Pts',(0.00566632606879868,-0.034364806625142,
0.0796236559443599));
#68209=CARTESIAN_POINT('',(0.00545366570497139,-0.0346775396665004,0.0795231255274065));
#68210=CARTESIAN_POINT('',(0.00544219470431032,-0.0346945769586885,0.0795174098539166));
#68211=CARTESIAN_POINT('Origin',(0.0127046232047038,-0.0345626618182689,
0.064588718319839));
#68212=CARTESIAN_POINT('Ctrl Pts',(0.00545366570400267,-0.0346775396670097,
0.0795231255258533));
#68213=CARTESIAN_POINT('Ctrl Pts',(0.00547278291854349,-0.0346269749928203,
0.0794846555672365));
#68214=CARTESIAN_POINT('Ctrl Pts',(0.0054915603453571,-0.0345757902890819,
0.0794468692896402));
#68215=CARTESIAN_POINT('Ctrl Pts',(0.00552845124219787,-0.0344721681087867,
0.0793726330539552));
#68216=CARTESIAN_POINT('Ctrl Pts',(0.00554655025430632,-0.0344197714289421,
0.0793362122024711));
#68217=CARTESIAN_POINT('Ctrl Pts',(0.00556431598442007,-0.0343667727830705,
0.0793004618946509));
#68218=CARTESIAN_POINT('',(0.00539853357837515,-0.0346945769587026,0.0793541842389209));
#68219=CARTESIAN_POINT('Origin',(0.00812378219310841,-0.0315241814719618,
0.07415));
#68220=CARTESIAN_POINT('',(0.00512155322769303,-0.0342105180190352,0.0793448648895882));
#68221=CARTESIAN_POINT('',(0.00513265640034568,-0.0341934961088739,0.0793512658547611));
#68222=CARTESIAN_POINT('Origin',(0.0138135968724053,-0.034562169891954,
0.0652381629999228));
#68223=CARTESIAN_POINT('Origin',(0.012963198382615,-0.0345621042509321,
0.0647527421530786));
#68224=CARTESIAN_POINT('Origin',(0.0130047980182236,-0.0345621713291986,
0.0647707445053555));
#68225=CARTESIAN_POINT('Ctrl Pts',(0.00492023879775385,-0.0345231616327842,
0.0792231952174262));
#68226=CARTESIAN_POINT('Ctrl Pts',(0.00499016565133852,-0.0344132092796988,
0.0792673515529028));
#68227=CARTESIAN_POINT('Ctrl Pts',(0.0050610022359883,-0.0343032738558979,
0.0793100592283065));
#68228=CARTESIAN_POINT('Ctrl Pts',(0.00513265640034569,-0.0341934961088739,
0.0793512658547611));
#68229=CARTESIAN_POINT('Ctrl Pts',(0.00502905439365322,-0.0345231616327842,
0.0791915676625468));
#68230=CARTESIAN_POINT('Ctrl Pts',(0.00509854530592192,-0.0344132092796988,
0.079234224128234));
#68231=CARTESIAN_POINT('Ctrl Pts',(0.00516891494812477,-0.0343032738558979,
0.0792754410283371));
#68232=CARTESIAN_POINT('Ctrl Pts',(0.0052400718160332,-0.0341934961088739,
0.0793151678685117));
#68233=CARTESIAN_POINT('Ctrl Pts',(0.0051378699895526,-0.0345231616327842,
0.0791599401076674));
#68234=CARTESIAN_POINT('Ctrl Pts',(0.00520692496050531,-0.0344132092796988,
0.0792010967035653));
#68235=CARTESIAN_POINT('Ctrl Pts',(0.00527682766026125,-0.0343032738558979,
0.0792408228283676));
#68236=CARTESIAN_POINT('Ctrl Pts',(0.00534748723172071,-0.0341934961088739,
0.0792790698822624));
#68237=CARTESIAN_POINT('Ctrl Pts',(0.00524668558545197,-0.0345231616327842,
0.079128312552788));
#68238=CARTESIAN_POINT('Ctrl Pts',(0.00531530461508871,-0.0344132092796988,
0.0791679692788966));
#68239=CARTESIAN_POINT('Ctrl Pts',(0.00538474037239772,-0.0343032738558979,
0.0792062046283982));
#68240=CARTESIAN_POINT('Ctrl Pts',(0.00545490264740822,-0.0341934961088739,
0.079242971896013));
#68241=CARTESIAN_POINT('',(0.00529281842211735,-0.0341934961088839,0.0792974418629146));
#68242=CARTESIAN_POINT('Ctrl Pts',(0.00512155322941782,-0.0342105180195384,
0.0793448648865901));
#68243=CARTESIAN_POINT('Ctrl Pts',(0.0051430555100191,-0.0342610556241263,
0.0793076587161653));
#68244=CARTESIAN_POINT('Ctrl Pts',(0.0051641719433129,-0.0343122189870085,
0.0792711201912312));
#68245=CARTESIAN_POINT('Ctrl Pts',(0.00520565162553852,-0.0344158119695126,
0.0791993464033866));
#68246=CARTESIAN_POINT('Ctrl Pts',(0.00522599790897453,-0.0344681990450014,
0.0791641404964846));
#68247=CARTESIAN_POINT('Ctrl Pts',(0.00524596632826922,-0.0345211942962425,
0.0791295884215131));
#68248=CARTESIAN_POINT('Origin',(0.00812378219310841,-0.0315241814719618,
0.07415));
#68249=CARTESIAN_POINT('',(0.00545366570615726,-0.034711613648978,0.0795231255266795));
#68250=CARTESIAN_POINT('',(0.00546514888907038,-0.0346945769586885,0.0795288166872181));
#68251=CARTESIAN_POINT('Origin',(0.0126632473294917,-0.0345626675282767,
0.0645702406010984));
#68252=CARTESIAN_POINT('Origin',(0.0129781455413861,-0.0345626632992206,
0.0647246384176518));
#68253=CARTESIAN_POINT('Origin',(0.0130178575616,-0.034562669103339,0.06474646406225));
#68254=CARTESIAN_POINT('Ctrl Pts',(0.00542106257343935,-0.0352450361861256,
0.079226754047367));
#68255=CARTESIAN_POINT('Ctrl Pts',(0.00561253548933533,-0.0349452761023744,
0.0793286887878722));
#68256=CARTESIAN_POINT('Ctrl Pts',(0.0058111425924016,-0.034644428998343,
0.0794159114194262));
#68257=CARTESIAN_POINT('Ctrl Pts',(0.00564424009426933,-0.0352450361861256,
0.0793394119108128));
#68258=CARTESIAN_POINT('Ctrl Pts',(0.00583996197109809,-0.0349452761023744,
0.0794329293732153));
#68259=CARTESIAN_POINT('Ctrl Pts',(0.00604217194043589,-0.034644428998343,
0.0795114385901518));
#68260=CARTESIAN_POINT('Ctrl Pts',(0.00564647186947763,-0.0352450361861256,
0.0793405384894472));
#68261=CARTESIAN_POINT('Ctrl Pts',(0.00584223623591572,-0.0349452761023744,
0.0794339717790687));
#68262=CARTESIAN_POINT('Ctrl Pts',(0.00604448223391623,-0.034644428998343,
0.0795123938618591));
#68263=CARTESIAN_POINT('',(0.00567683038040905,-0.0351951634053288,0.0793548611056252));
#68264=CARTESIAN_POINT('',(0.00589276668460222,-0.0348678972925434,0.0794510088474559));
#68265=CARTESIAN_POINT('Origin',(0.0120010715500606,-0.034563676788786,
0.0638497500128052));
#68266=CARTESIAN_POINT('Origin',(0.00160641038181471,-0.0346946199340732,
0.0896356118820766));
#68267=CARTESIAN_POINT('',(0.00577808157344129,-0.0346945769586883,0.0794012678091004));
#68268=CARTESIAN_POINT('',(0.00583568762442879,-0.0346945769586984,0.0794255122495203));
#68269=CARTESIAN_POINT('',(0.00556431598449918,-0.0350221583435276,0.0793004618945283));
#68270=CARTESIAN_POINT('Origin',(0.0124587166940046,-0.0345629067284135,
0.0639973484499783));
#68271=CARTESIAN_POINT('',(0.00556486371357888,-0.035195136029876,0.0792993528924502));
#68272=CARTESIAN_POINT('Origin',(0.000661207092376949,-0.0351951838366793,
0.0891670778385463));
#68273=CARTESIAN_POINT('',(0.00567686067416044,-0.0351951371328747,0.0793548727248077));
#68274=CARTESIAN_POINT('Ctrl Pts',(0.00524510966521925,-0.0350241211493459,
0.079414337040617));
#68275=CARTESIAN_POINT('Ctrl Pts',(0.0053176237462245,-0.03491442328675,
0.0794539895726004));
#68276=CARTESIAN_POINT('Ctrl Pts',(0.00539100087653385,-0.0348045283677551,
0.079492166920732));
#68277=CARTESIAN_POINT('Ctrl Pts',(0.00546514888907046,-0.0346945769586885,
0.0795288166872181));
#68278=CARTESIAN_POINT('Ctrl Pts',(0.00535172464515648,-0.0350241211493459,
0.0793759392821534));
#68279=CARTESIAN_POINT('Ctrl Pts',(0.00542370981280642,-0.03491442328675,
0.0794141232365683));
#68280=CARTESIAN_POINT('Ctrl Pts',(0.00549652735663397,-0.0348045283677551,
0.0794508420611333));
#68281=CARTESIAN_POINT('Ctrl Pts',(0.00557008575680197,-0.0346945769586885,
0.0794860452529104));
#68282=CARTESIAN_POINT('Ctrl Pts',(0.00545833962509371,-0.0350241211493459,
0.0793375415236899));
#68283=CARTESIAN_POINT('Ctrl Pts',(0.00552979587938833,-0.03491442328675,
0.0793742569005361));
#68284=CARTESIAN_POINT('Ctrl Pts',(0.00560205383673409,-0.0348045283677551,
0.0794095172015345));
#68285=CARTESIAN_POINT('Ctrl Pts',(0.00567502262453347,-0.0346945769586885,
0.0794432738186027));
#68286=CARTESIAN_POINT('Ctrl Pts',(0.00556495460503094,-0.0350241211493459,
0.0792991437652263));
#68287=CARTESIAN_POINT('Ctrl Pts',(0.00563588194597025,-0.03491442328675,
0.0793343905645039));
#68288=CARTESIAN_POINT('Ctrl Pts',(0.0057075803168342,-0.0348045283677551,
0.0793681923419358));
#68289=CARTESIAN_POINT('Ctrl Pts',(0.00577995949226498,-0.0346945769586885,
0.0794005023842949));
#68290=CARTESIAN_POINT('',(0.00562161523126584,-0.0346945769586984,0.0794650422481692));
#68291=CARTESIAN_POINT('Ctrl Pts',(0.00545366570761676,-0.0347116136492789,
0.0795231255237274));
#68292=CARTESIAN_POINT('Ctrl Pts',(0.00547277534182364,-0.0347621546532227,
0.0794846708481116));
#68293=CARTESIAN_POINT('Ctrl Pts',(0.00549154897702143,-0.0348133084096884,
0.0794468923096087));
#68294=CARTESIAN_POINT('Ctrl Pts',(0.0055284399172878,-0.0349168561544569,
0.0793726559780416));
#68295=CARTESIAN_POINT('Ctrl Pts',(0.00554654258958549,-0.0349692089015918,
0.0793362276307771));
#68296=CARTESIAN_POINT('Ctrl Pts',(0.0055643159845333,-0.0350221583435,
0.0793004618945045));
#68297=CARTESIAN_POINT('Ctrl Pts',(0.00567639462613548,-0.0351951371254904,
0.0793534859230376));
#68298=CARTESIAN_POINT('Ctrl Pts',(0.00578397343281551,-0.0350307338980949,
0.0794040841254413));
#68299=CARTESIAN_POINT('Ctrl Pts',(0.00589355159233925,-0.0348659306897851,
0.0794501927438176));
#68300=CARTESIAN_POINT('Ctrl Pts',(0.00567686067420752,-0.0351951371254904,
0.0793548727247014));
#68301=CARTESIAN_POINT('Ctrl Pts',(0.00578446815214185,-0.0350307338980949,
0.0794054612918536));
#68302=CARTESIAN_POINT('Ctrl Pts',(0.00589407456018512,-0.0348659306897851,
0.0794515590981978));
#68303=CARTESIAN_POINT('Ctrl Pts',(0.00575497081680124,-0.0351951371254904,
0.079587302128884));
#68304=CARTESIAN_POINT('Ctrl Pts',(0.00586738362683585,-0.0350307338980949,
0.079636275817846));
#68305=CARTESIAN_POINT('Ctrl Pts',(0.00598172451619324,-0.0348659306897851,
0.0796805615163434));
#68306=CARTESIAN_POINT('Origin',(0.00382978524874992,-0.0308609197384744,
0.084352760014669));
#68307=CARTESIAN_POINT('',(0.00571091493522803,-0.0351951371254904,0.0794562067043364));
#68308=CARTESIAN_POINT('Origin',(0.00836832757329725,-0.03518404674412,
0.0732039856204225));
#68309=CARTESIAN_POINT('Origin',(0.00422499454032104,-0.0352322614457976,
0.0854624028434309));
#68310=CARTESIAN_POINT('',(0.00611274429739835,-0.0351951142564672,0.0795382781262157));
#68311=CARTESIAN_POINT('',(0.00623046956272987,-0.0351951372916786,0.0795793523816059));
#68312=CARTESIAN_POINT('Origin',(0.00845646098340635,-0.0352875126228133,
0.0740768915355774));
#68313=CARTESIAN_POINT('Origin',(0.00164326621622433,-0.0298325076523774,
0.0703687167587176));
#68314=CARTESIAN_POINT('Origin',(0.00258859523071002,-0.033873480203009,
0.0804430596755119));
#68315=CARTESIAN_POINT('Ctrl Pts',(0.00332944714467594,-0.0321934096636941,
0.0773268675119815));
#68316=CARTESIAN_POINT('Ctrl Pts',(0.00338631156032693,-0.0320508460843488,
0.0774126838263026));
#68317=CARTESIAN_POINT('Ctrl Pts',(0.00344543881505853,-0.0319086045661401,
0.0774969076001925));
#68318=CARTESIAN_POINT('Ctrl Pts',(0.00350668666774897,-0.0317669892865405,
0.0775793679661119));
#68319=CARTESIAN_POINT('Ctrl Pts',(0.00337727060759419,-0.0321934096636941,
0.0773957394875768));
#68320=CARTESIAN_POINT('Ctrl Pts',(0.00343536779881174,-0.0320508460843488,
0.077480699784685));
#68321=CARTESIAN_POINT('Ctrl Pts',(0.00349570390009959,-0.0319086045661401,
0.0775640350645548));
#68322=CARTESIAN_POINT('Ctrl Pts',(0.00355813422497361,-0.0317669892865405,
0.0776455765870144));
#68323=CARTESIAN_POINT('Ctrl Pts',(0.00342509407051245,-0.0321934096636941,
0.0774646114631721));
#68324=CARTESIAN_POINT('Ctrl Pts',(0.00348442403729657,-0.0320508460843488,
0.0775487157430673));
#68325=CARTESIAN_POINT('Ctrl Pts',(0.00354596898514065,-0.0319086045661401,
0.0776311625289171));
#68326=CARTESIAN_POINT('Ctrl Pts',(0.00360958178219824,-0.0317669892865405,
0.0777117852079169));
#68327=CARTESIAN_POINT('Ctrl Pts',(0.00347291753343071,-0.0321934096636941,
0.0775334834387674));
#68328=CARTESIAN_POINT('Ctrl Pts',(0.00353348027578138,-0.0320508460843488,
0.0776167317014498));
#68329=CARTESIAN_POINT('Ctrl Pts',(0.00359623407018171,-0.0319086045661401,
0.0776982899932795));
#68330=CARTESIAN_POINT('Ctrl Pts',(0.00366102933942288,-0.0317669892865405,
0.0777779938288193));
#68331=CARTESIAN_POINT('',(0.00347206196223053,-0.0321934096636941,0.0775322513055127));
#68332=CARTESIAN_POINT('',(0.00361494791176087,-0.0318665617511303,0.0777205095452145));
#68333=CARTESIAN_POINT('Origin',(0.0173394999816654,-0.0326371944420774,
0.0682095871144943));
#68334=CARTESIAN_POINT('Origin',(-0.00497818172410554,-0.0316939261509784,
0.0845253396750685));
#68335=CARTESIAN_POINT('',(0.00339983986145632,-0.0320197221621766,0.0774305423353098));
#68336=CARTESIAN_POINT('Ctrl Pts',(0.00339990312524244,-0.0320197392094684,
0.0774307161529535));
#68337=CARTESIAN_POINT('Ctrl Pts',(0.00341659650230586,-0.0319792716575983,
0.0774547527415632));
#68338=CARTESIAN_POINT('Ctrl Pts',(0.00343354911925363,-0.031938643982963,
0.0774787714902867));
#68339=CARTESIAN_POINT('Ctrl Pts',(0.00345078568289115,-0.0318979099381562,
0.0775027927373011));
#68340=CARTESIAN_POINT('Ctrl Pts',(0.00346802190583522,-0.031857176698488,
0.0775268135095177));
#68341=CARTESIAN_POINT('Ctrl Pts',(0.00348545301092505,-0.0318163871833546,
0.0775507157293868));
#68342=CARTESIAN_POINT('Ctrl Pts',(0.00350301619735661,-0.0317755399638303,
0.0775744192578713));
#68343=CARTESIAN_POINT('',(0.00340076680876396,-0.0321934096636184,0.0774295770579827));
#68344=CARTESIAN_POINT('Origin',(0.00151749285991017,-0.0324111438667224,
0.0787628845887113));
#68345=CARTESIAN_POINT('',(0.00343641438550725,-0.0321934096636663,0.0774809141817577));
#68346=CARTESIAN_POINT('Ctrl Pts',(0.00347242198582075,-0.0321934096636618,
0.0775302552918872));
#68347=CARTESIAN_POINT('Ctrl Pts',(0.00351903834071276,-0.0320835708272592,
0.0775944011742037));
#68348=CARTESIAN_POINT('Ctrl Pts',(0.00356695515192517,-0.0319739230346488,
0.07765754512626));
#68349=CARTESIAN_POINT('Ctrl Pts',(0.00361610491294562,-0.0318646057455573,
0.0777196110648324));
#68350=CARTESIAN_POINT('Ctrl Pts',(0.00345230709872301,-0.0321934096636618,
0.0776417746000015));
#68351=CARTESIAN_POINT('Ctrl Pts',(0.00350046139178699,-0.0320835708272592,
0.0777061978822878));
#68352=CARTESIAN_POINT('Ctrl Pts',(0.00354992098988267,-0.0319739230346488,
0.0777695872458599));
#68353=CARTESIAN_POINT('Ctrl Pts',(0.0036006163885113,-0.0318646057455573,
0.0778318664449979));
#68354=CARTESIAN_POINT('Ctrl Pts',(0.00343219221162527,-0.0321934096636618,
0.0777532939081159));
#68355=CARTESIAN_POINT('Ctrl Pts',(0.00348188444286121,-0.0320835708272592,
0.0778179945903719));
#68356=CARTESIAN_POINT('Ctrl Pts',(0.00353288682784016,-0.0319739230346488,
0.0778816293654599));
#68357=CARTESIAN_POINT('Ctrl Pts',(0.00358512786407699,-0.0318646057455573,
0.0779441218251635));
#68358=CARTESIAN_POINT('Ctrl Pts',(0.00341207732452753,-0.0321934096636618,
0.0778648132162302));
#68359=CARTESIAN_POINT('Ctrl Pts',(0.00346330749393543,-0.0320835708272592,
0.0779297912984559));
#68360=CARTESIAN_POINT('Ctrl Pts',(0.00351585266579766,-0.0319739230346488,
0.0779936714850599));
#68361=CARTESIAN_POINT('Ctrl Pts',(0.00356963933964267,-0.0318646057455573,
0.078056377205329));
#68362=CARTESIAN_POINT('',(0.00342002298234353,-0.0321763980308481,0.0778748690265434));
#68363=CARTESIAN_POINT('',(0.00341207732454946,-0.0321934096636184,0.0778648132162463));
#68364=CARTESIAN_POINT('Origin',(0.0167646994888026,-0.0326386230218105,
0.0680898959435203));
#68365=CARTESIAN_POINT('Ctrl Pts',(0.00342002298482514,-0.0321763980306328,
0.0778748690245691));
#68366=CARTESIAN_POINT('Ctrl Pts',(0.00345366967478655,-0.0321259596175906,
0.0778482244818392));
#68367=CARTESIAN_POINT('Ctrl Pts',(0.00348673339218307,-0.0320749164633572,
0.0778220415903783));
#68368=CARTESIAN_POINT('Ctrl Pts',(0.00355172149072844,-0.0319716057793949,
0.0777705780386704));
#68369=CARTESIAN_POINT('Ctrl Pts',(0.00358362055013076,-0.0319193786690143,
0.0777453174305103));
#68370=CARTESIAN_POINT('Ctrl Pts',(0.00361494791320901,-0.0318665617525338,
0.0777205095440551));
#68371=CARTESIAN_POINT('',(0.0034420696434,-0.0321934096636663,0.0776985322608896));
#68372=CARTESIAN_POINT('Origin',(0.00812378219310841,-0.0315241814719618,
0.07415));
#68373=CARTESIAN_POINT('',(0.00342002298205243,-0.0322104233323598,0.0778748690267733));
#68374=CARTESIAN_POINT('',(0.00342799009848551,-0.0321934096636183,0.0778849078441259));
#68375=CARTESIAN_POINT('Origin',(0.0167417837500709,-0.0326387225284402,
0.0680507782985828));
#68376=CARTESIAN_POINT('Origin',(0.0160029617252066,-0.032638624895482,
0.0671279692888624));
#68377=CARTESIAN_POINT('Origin',(0.0160357811135996,-0.0326387239005177,
0.0671592451620444));
#68378=CARTESIAN_POINT('Ctrl Pts',(0.00351668453358277,-0.0327445246967098,
0.0775927861036656));
#68379=CARTESIAN_POINT('Ctrl Pts',(0.00364653133419014,-0.032443687833936,
0.0777665456324781));
#68380=CARTESIAN_POINT('Ctrl Pts',(0.00378909753162478,-0.0321434074405927,
0.0779300309371087));
#68381=CARTESIAN_POINT('Ctrl Pts',(0.00367065265680256,-0.0327445246967098,
0.0777897475644447));
#68382=CARTESIAN_POINT('Ctrl Pts',(0.0038079279803431,-0.032443687833936,
0.0779577000905583));
#68383=CARTESIAN_POINT('Ctrl Pts',(0.00395746418988505,-0.0321434074405927,
0.0781148353428632));
#68384=CARTESIAN_POINT('',(0.0036936143861395,-0.0326943950436612,0.0778176611351237));
#68385=CARTESIAN_POINT('',(0.0038480392148886,-0.0323666188837389,0.0779965760078549));
#68386=CARTESIAN_POINT('Origin',(0.0165941822790158,-0.0326395579109043,
0.0670388204620943));
#68387=CARTESIAN_POINT('Origin',(-0.00436287349293982,-0.0321933825603008,
0.0853833401400488));
#68388=CARTESIAN_POINT('',(0.00376544772383368,-0.032193409653269,0.0779027384202294));
#68389=CARTESIAN_POINT('',(0.00380724845807768,-0.0321934096584275,0.0779492029116465));
#68390=CARTESIAN_POINT('',(0.00361494791101053,-0.0325210109756239,0.0777205095457903));
#68391=CARTESIAN_POINT('Origin',(0.016880826878996,-0.0326393129161898,
0.0674248506473343));
#68392=CARTESIAN_POINT('',(0.00361601294806189,-0.0326943950436595,0.0777196661515348));
#68393=CARTESIAN_POINT('Origin',(-0.005056508717713,-0.0326943765538189,
0.0845873647954996));
#68394=CARTESIAN_POINT('',(0.0036548136671107,-0.0326943950436703,0.0777686636433393));
#68395=CARTESIAN_POINT('Ctrl Pts',(0.00327763506527675,-0.0325229783203769,
0.0776876345225935));
#68396=CARTESIAN_POINT('Ctrl Pts',(0.00332640127980775,-0.032413025309245,
0.0777544385547724));
#68397=CARTESIAN_POINT('Ctrl Pts',(0.00337654202520829,-0.032303122220807,
0.0778202236630187));
#68398=CARTESIAN_POINT('Ctrl Pts',(0.00342799010127687,-0.0321934096576658,
0.0778849078476354));
#68399=CARTESIAN_POINT('Ctrl Pts',(0.00339045215365831,-0.0325229783203769,
0.0776982856636362));
#68400=CARTESIAN_POINT('Ctrl Pts',(0.00343936519393565,-0.032413025309245,
0.077763534514719));
#68401=CARTESIAN_POINT('Ctrl Pts',(0.0034896205718948,-0.032303122220807,
0.0778277616404636));
#68402=CARTESIAN_POINT('Ctrl Pts',(0.00354115101091851,-0.0321934096576658,
0.0778908870420193));
#68403=CARTESIAN_POINT('Ctrl Pts',(0.00350326924203986,-0.0325229783203769,
0.077708936804679));
#68404=CARTESIAN_POINT('Ctrl Pts',(0.00355232910806356,-0.032413025309245,
0.0777726304746655));
#68405=CARTESIAN_POINT('Ctrl Pts',(0.0036026991185813,-0.032303122220807,
0.0778352996179085));
#68406=CARTESIAN_POINT('Ctrl Pts',(0.00365431192056015,-0.0321934096576658,
0.0778968662364032));
#68407=CARTESIAN_POINT('Ctrl Pts',(0.00361608633042141,-0.0325229783203769,
0.0777195879457217));
#68408=CARTESIAN_POINT('Ctrl Pts',(0.00366529302219146,-0.032413025309245,
0.0777817264346121));
#68409=CARTESIAN_POINT('Ctrl Pts',(0.00371577766526781,-0.032303122220807,
0.0778428375953534));
#68410=CARTESIAN_POINT('Ctrl Pts',(0.00376747283020179,-0.0321934096576658,
0.0779028454307871));
#68411=CARTESIAN_POINT('',(0.00359671891073733,-0.0321934096584275,0.0778938231319032));
#68412=CARTESIAN_POINT('Ctrl Pts',(0.00342002298477554,-0.0322104233328918,
0.0778748690246083));
#68413=CARTESIAN_POINT('Ctrl Pts',(0.00345371526661704,-0.0322609421831403,
0.0778481883780358));
#68414=CARTESIAN_POINT('Ctrl Pts',(0.00348680125644047,-0.0323120888240814,
0.0778219878492282));
#68415=CARTESIAN_POINT('Ctrl Pts',(0.00355178984688891,-0.0324156524631808,
0.0777705239079862));
#68416=CARTESIAN_POINT('Ctrl Pts',(0.00358366573380517,-0.0324680267167304,
0.0777452816499224));
#68417=CARTESIAN_POINT('Ctrl Pts',(0.00361494791104727,-0.0325210109755912,
0.0777205095457668));
#68418=CARTESIAN_POINT('Origin',(0.00401772587397361,-0.0262834582511791,
0.067438540595134));
#68419=CARTESIAN_POINT('Origin',(-0.00377752765640774,-0.0342770824103611,
0.0766364395902537));
#68420=CARTESIAN_POINT('Ctrl Pts',(0.00369384831184546,-0.0326943950436604,
0.077815646943078));
#68421=CARTESIAN_POINT('Ctrl Pts',(0.00374436779687566,-0.0325844576448134,
0.0778766997345428));
#68422=CARTESIAN_POINT('Ctrl Pts',(0.00379615352907322,-0.0324744968375322,
0.0779367120210303));
#68423=CARTESIAN_POINT('Ctrl Pts',(0.00384913809697668,-0.0323646534831894,
0.0779956078264775));
#68424=CARTESIAN_POINT('Ctrl Pts',(0.0036807754911042,-0.0326943950436604,
0.0779282090545546));
#68425=CARTESIAN_POINT('Ctrl Pts',(0.00373284629299443,-0.0325844576448134,
0.0779894420139903));
#68426=CARTESIAN_POINT('Ctrl Pts',(0.00378618717801016,-0.0324744968375322,
0.0780496023974234));
#68427=CARTESIAN_POINT('Ctrl Pts',(0.00384072873952019,-0.0323646534831894,
0.0781086140665237));
#68428=CARTESIAN_POINT('Ctrl Pts',(0.00366770267036294,-0.0326943950436604,
0.0780407711660313));
#68429=CARTESIAN_POINT('Ctrl Pts',(0.00372132478911321,-0.0325844576448134,
0.0781021842934379));
#68430=CARTESIAN_POINT('Ctrl Pts',(0.00377622082694709,-0.0324744968375322,
0.0781624927738165));
#68431=CARTESIAN_POINT('Ctrl Pts',(0.00383231938206371,-0.0323646534831894,
0.0782216203065699));
#68432=CARTESIAN_POINT('Ctrl Pts',(0.00365462984962169,-0.0326943950436604,
0.078153333277508));
#68433=CARTESIAN_POINT('Ctrl Pts',(0.00370980328523198,-0.0325844576448134,
0.0782149265728854));
#68434=CARTESIAN_POINT('Ctrl Pts',(0.00376625447588403,-0.0324744968375322,
0.0782753831502096));
#68435=CARTESIAN_POINT('Ctrl Pts',(0.00382391002460722,-0.0323646534831894,
0.0783346265466161));
#68436=CARTESIAN_POINT('',(0.0036631912378776,-0.0326773559991367,0.0781628703331065));
#68437=CARTESIAN_POINT('',(0.00365462984962342,-0.0326943950436594,0.078153333277498));
#68438=CARTESIAN_POINT('Origin',(0.0159743814683323,-0.0326395669855557,
0.0670198053090934));
#68439=CARTESIAN_POINT('Ctrl Pts',(0.00366319124036326,-0.0326773559987476,
0.0781628703308607));
#68440=CARTESIAN_POINT('Ctrl Pts',(0.0036951241883951,-0.0326267922587068,
0.0781341425723436));
#68441=CARTESIAN_POINT('Ctrl Pts',(0.00372649114798488,-0.032575610958155,
0.0781059239925992));
#68442=CARTESIAN_POINT('Ctrl Pts',(0.0037881197853654,-0.0324719985462377,
0.0780504811750229));
#68443=CARTESIAN_POINT('Ctrl Pts',(0.0038183567453997,-0.0324196091621775,
0.0780232791739646));
#68444=CARTESIAN_POINT('Ctrl Pts',(0.00384803921492484,-0.0323666188837756,
0.0779965760078223));
#68445=CARTESIAN_POINT('',(0.00367412211789146,-0.0326943950436703,0.0779854972063209));
#68446=CARTESIAN_POINT('Origin',(0.00812378219310841,-0.0315241814719618,
0.07415));
#68447=CARTESIAN_POINT('',(0.0036631912379105,-0.0327114338379855,0.0781628703330763));
#68448=CARTESIAN_POINT('',(0.00367177297545987,-0.0326943950436593,0.0781723890818771));
#68449=CARTESIAN_POINT('Origin',(0.0159435067138025,-0.0326395658227958,
0.066986639998606));
#68450=CARTESIAN_POINT('Origin',(0.0160415858996068,-0.0326395684850483,
0.067094502901923));
#68451=CARTESIAN_POINT('Origin',(0.0160713078331,-0.032639567343421,0.067128705283839));
#68452=CARTESIAN_POINT('Ctrl Pts',(0.00374197532261405,-0.0332451089994432,
0.0778753044908689));
#68453=CARTESIAN_POINT('Ctrl Pts',(0.00388247748022288,-0.0329451141710253,
0.0780405670408267));
#68454=CARTESIAN_POINT('Ctrl Pts',(0.00403502873689203,-0.0326442513127493,
0.0781947769004333));
#68455=CARTESIAN_POINT('Ctrl Pts',(0.00390800821203346,-0.0332451089994432,
0.0780622084224248));
#68456=CARTESIAN_POINT('Ctrl Pts',(0.00405555956675183,-0.0329451141710253,
0.0782212089395058));
#68457=CARTESIAN_POINT('Ctrl Pts',(0.00421466831258984,-0.0326442513127493,
0.0783686435816667));
#68458=CARTESIAN_POINT('Ctrl Pts',(0.00390966854092765,-0.0332451089994432,
0.0780640774617403));
#68459=CARTESIAN_POINT('Ctrl Pts',(0.00405729038761712,-0.0329451141710253,
0.0782230153584925));
#68460=CARTESIAN_POINT('Ctrl Pts',(0.00421646470834681,-0.0326442513127493,
0.078370382248479));
#68461=CARTESIAN_POINT('',(0.00393265065846339,-0.0331951640388616,0.0780885963818732));
#68462=CARTESIAN_POINT('',(0.00409800492860871,-0.0328677532355016,0.0782574618058445));
#68463=CARTESIAN_POINT('Origin',(0.0156101803831019,-0.0326402808282682,
0.0660608140840406));
#68464=CARTESIAN_POINT('Origin',(-0.00364056838794087,-0.0326944278779144,
0.0861535916169325));
#68465=CARTESIAN_POINT('',(0.004009684300756,-0.0326943950436593,0.0781689953386565));
#68466=CARTESIAN_POINT('',(0.00405432007862868,-0.0326943950436692,0.0782127434510212));
#68467=CARTESIAN_POINT('',(0.0038480392148867,-0.0330220786163545,0.0779965760078528));
#68468=CARTESIAN_POINT('Origin',(0.0159748003131234,-0.0326396682764862,
0.06637419077711));
#68469=CARTESIAN_POINT('',(0.00384904919316599,-0.0331951640388587,0.077995667403612));
#68470=CARTESIAN_POINT('Origin',(-0.00435223336755533,-0.0331952026560077,
0.085373765661119));
#68471=CARTESIAN_POINT('',(0.00389084992582468,-0.0331951640388701,0.0780421318927526));
#68472=CARTESIAN_POINT('Ctrl Pts',(0.0035093283533754,-0.0330240426238172,
0.0779849466438276));
#68473=CARTESIAN_POINT('Ctrl Pts',(0.0035621584796016,-0.032914277406352,
0.0780485152411145));
#68474=CARTESIAN_POINT('Ctrl Pts',(0.00361632908404852,-0.0328043479726691,
0.0781110233833827));
#68475=CARTESIAN_POINT('Ctrl Pts',(0.00367177297545988,-0.0326943950436593,
0.0781723890818771));
#68476=CARTESIAN_POINT('Ctrl Pts',(0.00362259158667951,-0.0330240426238172,
0.0779884929046831));
#68477=CARTESIAN_POINT('Ctrl Pts',(0.00367547056610395,-0.032914277406352,
0.0780505011905842));
#68478=CARTESIAN_POINT('Ctrl Pts',(0.00372965779210934,-0.0328043479726691,
0.0781114472336624));
#68479=CARTESIAN_POINT('Ctrl Pts',(0.00378508599703424,-0.0326943950436593,
0.0781712510457416));
#68480=CARTESIAN_POINT('Ctrl Pts',(0.00373585481998362,-0.0330240426238172,
0.0779920391655386));
#68481=CARTESIAN_POINT('Ctrl Pts',(0.00378878265260629,-0.032914277406352,
0.0780524871400539));
#68482=CARTESIAN_POINT('Ctrl Pts',(0.00384298650017017,-0.0328043479726691,
0.0781118710839421));
#68483=CARTESIAN_POINT('Ctrl Pts',(0.00389839901860859,-0.0326943950436593,
0.0781701130096061));
#68484=CARTESIAN_POINT('Ctrl Pts',(0.00384911805328772,-0.0330240426238172,
0.0779955854263941));
#68485=CARTESIAN_POINT('Ctrl Pts',(0.00390209473910864,-0.032914277406352,
0.0780544730895236));
#68486=CARTESIAN_POINT('Ctrl Pts',(0.003956315208231,-0.0328043479726691,
0.0781122949342219));
#68487=CARTESIAN_POINT('Ctrl Pts',(0.00401171204018295,-0.0326943950436593,
0.0781689749734706));
#68488=CARTESIAN_POINT('',(0.00384072863811794,-0.0326943950436694,0.0781706922102768));
#68489=CARTESIAN_POINT('Ctrl Pts',(0.00366319124037136,-0.0327114338383316,
0.0781628703308533));
#68490=CARTESIAN_POINT('Ctrl Pts',(0.00369511887698221,-0.0327619876831102,
0.0781341473506367));
#68491=CARTESIAN_POINT('Ctrl Pts',(0.00372648324226078,-0.0328131562604614,
0.078105931104806));
#68492=CARTESIAN_POINT('Ctrl Pts',(0.00378811182289566,-0.0329167375858765,
0.0780504883382796));
#68493=CARTESIAN_POINT('Ctrl Pts',(0.00381835148227642,-0.0329691088920623,
0.078023283908815));
#68494=CARTESIAN_POINT('Ctrl Pts',(0.00384803921492386,-0.0330220786163187,
0.0779965760078231));
#68495=CARTESIAN_POINT('Ctrl Pts',(0.00393275766748565,-0.0331951640388604,
0.078086571152787));
#68496=CARTESIAN_POINT('Ctrl Pts',(0.00401414375217492,-0.0330306422010619,
0.0781732178978193));
#68497=CARTESIAN_POINT('Ctrl Pts',(0.00409904149411709,-0.0328657861914645,
0.0782564268313473));
#68498=CARTESIAN_POINT('Ctrl Pts',(0.00393265065846129,-0.0331951640388604,
0.078088596381871));
#68499=CARTESIAN_POINT('Ctrl Pts',(0.00401407861346341,-0.0330306422010619,
0.0781752453392462));
#68500=CARTESIAN_POINT('Ctrl Pts',(0.00409901828137901,-0.0328657861914645,
0.0782584547526827));
#68501=CARTESIAN_POINT('Ctrl Pts',(0.00391482007723423,-0.0331951640388604,
0.0784260540112631));
#68502=CARTESIAN_POINT('Ctrl Pts',(0.00400322475236632,-0.0330306422010619,
0.0785130716044733));
#68503=CARTESIAN_POINT('Ctrl Pts',(0.00409515041496016,-0.0328657861914645,
0.0785963609835681));
#68504=CARTESIAN_POINT('',(0.00392396340684694,-0.033178164828192,0.0784350346741231));
#68505=CARTESIAN_POINT('',(0.00391482007723563,-0.0331951640388588,0.0784260540112524));
#68506=CARTESIAN_POINT('Origin',(0.0149696437100718,-0.0326412091873849,
0.0661476661280231));
#68507=CARTESIAN_POINT('Ctrl Pts',(0.00392396340651288,-0.033178164828644,
0.0784350346723065));
#68508=CARTESIAN_POINT('Ctrl Pts',(0.00395405020197888,-0.0331276811546783,
0.0784043373872559));
#68509=CARTESIAN_POINT('Ctrl Pts',(0.00398359369894219,-0.0330765663497789,
0.0783741943764374));
#68510=CARTESIAN_POINT('Ctrl Pts',(0.00404161959471262,-0.0329730614463239,
0.0783149911186314));
#68511=CARTESIAN_POINT('Ctrl Pts',(0.00407007855615157,-0.0329207133373932,
0.0782859547922208));
#68512=CARTESIAN_POINT('Ctrl Pts',(0.00409800491252451,-0.0328677532289374,
0.0782574618022812));
#68513=CARTESIAN_POINT('',(0.00392373536785951,-0.0331951640388702,0.0782573251965728));
#68514=CARTESIAN_POINT('Origin',(0.00812378219310841,-0.0315241814719618,
0.07415));
#68515=CARTESIAN_POINT('',(0.00392396340839382,-0.0332121607144402,0.0784350346734683));
#68516=CARTESIAN_POINT('',(0.00393312589888615,-0.0331951640388587,0.0784439957875769));
#68517=CARTESIAN_POINT('Origin',(0.0149322586422581,-0.0326413640258274,
0.0661220012505349));
#68518=CARTESIAN_POINT('Origin',(0.0159870069992313,-0.0326412104640766,
0.0671447922847213));
#68519=CARTESIAN_POINT('Origin',(0.0160134126578002,-0.0326413654427593,
0.0671816590824428));
#68520=CARTESIAN_POINT('Ctrl Pts',(0.00398452115888946,-0.0337436976235975,
0.0781430743908167));
#68521=CARTESIAN_POINT('Ctrl Pts',(0.00402043547512745,-0.0336723290703325,
0.0781803035318806));
#68522=CARTESIAN_POINT('Ctrl Pts',(0.00405701361617926,-0.033601104548885,
0.0782168806647972));
#68523=CARTESIAN_POINT('Ctrl Pts',(0.0041738003748362,-0.0333736987606857,
0.0783336642046779));
#68524=CARTESIAN_POINT('Ctrl Pts',(0.00429709639104041,-0.0331450831799192,
0.0784435533969256));
#68525=CARTESIAN_POINT('Ctrl Pts',(0.00416196157741737,-0.0337436976235975,
0.0783191848614669));
#68526=CARTESIAN_POINT('Ctrl Pts',(0.00419945985791865,-0.0336723290703325,
0.0783548180765149));
#68527=CARTESIAN_POINT('Ctrl Pts',(0.00423759300130689,-0.033601104548885,
0.078389771051074));
#68528=CARTESIAN_POINT('Ctrl Pts',(0.00435934457439544,-0.0333736987606857,
0.0785013689750472));
#68529=CARTESIAN_POINT('Ctrl Pts',(0.00448729964286908,-0.0331450831799192,
0.0786057961871931));
#68530=CARTESIAN_POINT('Ctrl Pts',(0.00416373598160265,-0.0337436976235975,
0.0783209459661734));
#68531=CARTESIAN_POINT('Ctrl Pts',(0.00420125010174657,-0.0336723290703325,
0.0783565632219612));
#68532=CARTESIAN_POINT('Ctrl Pts',(0.00423939879515817,-0.033601104548885,
0.0783914999549368));
#68533=CARTESIAN_POINT('Ctrl Pts',(0.00436120001639104,-0.0333736987606857,
0.0785030460227508));
#68534=CARTESIAN_POINT('Ctrl Pts',(0.00448920167538737,-0.0331450831799192,
0.0786074186150958));
#68535=CARTESIAN_POINT('',(0.00418822741221839,-0.0336938721132548,0.078343987788086));
#68536=CARTESIAN_POINT('',(0.00436385854011419,-0.0333679869945434,0.0785021373052407));
#68537=CARTESIAN_POINT('Ctrl Pts',(0.00418822741222797,-0.0336938721132648,
0.0783439877880965));
#68538=CARTESIAN_POINT('Ctrl Pts',(0.00420459851399994,-0.0336629187933931,
0.0783593501046076));
#68539=CARTESIAN_POINT('Ctrl Pts',(0.0042210543324433,-0.0336319952301039,
0.0783746116485008));
#68540=CARTESIAN_POINT('Ctrl Pts',(0.00423759300131699,-0.0336011045488949,
0.0783897710510839));
#68541=CARTESIAN_POINT('Ctrl Pts',(0.00427909418073509,-0.0335235892595453,
0.0784278111794205));
#68542=CARTESIAN_POINT('Ctrl Pts',(0.00432119089700305,-0.0334458668660368,
0.0784652756281618));
#68543=CARTESIAN_POINT('Ctrl Pts',(0.00436385853990239,-0.0333679869945384,
0.0785021373054752));
#68544=CARTESIAN_POINT('Ctrl Pts',(0.00436389174180533,-0.0333679692460741,
0.078502166897738));
#68545=CARTESIAN_POINT('Ctrl Pts',(0.00436418354275695,-0.033339189537532,
0.0785018200692105));
#68546=CARTESIAN_POINT('Ctrl Pts',(0.00436439977706645,-0.0333104081060831,
0.0785015580137926));
#68547=CARTESIAN_POINT('Ctrl Pts',(0.00436468172845928,-0.0332532697777497,
0.0785012076134217));
#68548=CARTESIAN_POINT('Ctrl Pts',(0.00436474964008472,-0.0332249169019147,
0.0785011167321469));
#68549=CARTESIAN_POINT('Ctrl Pts',(0.00436474682003064,-0.0331960985456441,
0.0785011094454358));
#68550=CARTESIAN_POINT('Ctrl Pts',(0.00436474675475889,-0.0331956312467839,
0.0785011093497213));
#68551=CARTESIAN_POINT('Ctrl Pts',(0.00436474667057917,-0.0331951640388602,
0.0785011092769963));
#68552=CARTESIAN_POINT('',(0.00427015733847041,-0.0331951640388587,0.078419391113463));
#68553=CARTESIAN_POINT('',(0.00431745200453479,-0.0331951640388687,0.0784602501952397));
#68554=CARTESIAN_POINT('',(0.00409800492306439,-0.0335216366567692,0.0782574617913545));
#68555=CARTESIAN_POINT('Origin',(0.0148599224840116,-0.0326434571526649,
0.065547159063874));
#68556=CARTESIAN_POINT('',(0.00409895585648141,-0.0336938721132328,0.0782564915633658));
#68557=CARTESIAN_POINT('Origin',(-0.00354511341528025,-0.0336938867896257,
0.0860556604238307));
#68558=CARTESIAN_POINT('',(0.0041435916343599,-0.0336938721132538,0.0783002396757359));
#68559=CARTESIAN_POINT('Ctrl Pts',(0.00375923287556075,-0.0335235895815172,
0.0782671239056808));
#68560=CARTESIAN_POINT('Ctrl Pts',(0.00381591319199349,-0.0334144449262748,
0.0783272105200437));
#68561=CARTESIAN_POINT('Ctrl Pts',(0.00387389997147532,-0.0333049234473147,
0.078386195193966));
#68562=CARTESIAN_POINT('Ctrl Pts',(0.00393312589888597,-0.0331951640388587,
0.0784439957875769));
#68563=CARTESIAN_POINT('Ctrl Pts',(0.00387249544171201,-0.0335235895815172,
0.0782635512883181));
#68564=CARTESIAN_POINT('Ctrl Pts',(0.00392912657403291,-0.0334144449262748,
0.0783220786204644));
#68565=CARTESIAN_POINT('Ctrl Pts',(0.00398703189929923,-0.0333049234473147,
0.0783795032368506));
#68566=CARTESIAN_POINT('Ctrl Pts',(0.00404614402584485,-0.0331951640388587,
0.0784357450018751));
#68567=CARTESIAN_POINT('Ctrl Pts',(0.00398575800786327,-0.0335235895815172,
0.0782599786709554));
#68568=CARTESIAN_POINT('Ctrl Pts',(0.00404233995607234,-0.0334144449262748,
0.0783169467208852));
#68569=CARTESIAN_POINT('Ctrl Pts',(0.00410016382712313,-0.0333049234473147,
0.0783728112797351));
#68570=CARTESIAN_POINT('Ctrl Pts',(0.00415916215280372,-0.0331951640388587,
0.0784274942161733));
#68571=CARTESIAN_POINT('Ctrl Pts',(0.00409902057401453,-0.0335235895815172,
0.0782564060535926));
#68572=CARTESIAN_POINT('Ctrl Pts',(0.00415555333811177,-0.0334144449262748,
0.0783118148213059));
#68573=CARTESIAN_POINT('Ctrl Pts',(0.00421329575494704,-0.0333049234473147,
0.0783661193226197));
#68574=CARTESIAN_POINT('Ctrl Pts',(0.0042721802797626,-0.0331951640388587,
0.0784192434304715));
#68575=CARTESIAN_POINT('',(0.00410164161868828,-0.0331951640388687,0.0784316934505299));
#68576=CARTESIAN_POINT('Ctrl Pts',(0.00392396341058244,-0.033212160714597,
0.0784350346712254));
#68577=CARTESIAN_POINT('Ctrl Pts',(0.00395399960100596,-0.033262544410987,
0.0784043890353013));
#68578=CARTESIAN_POINT('Ctrl Pts',(0.00398351822073386,-0.0333135300747073,
0.0783742714717752));
#68579=CARTESIAN_POINT('Ctrl Pts',(0.00404154375026909,-0.0334167203140585,
0.078315068582615));
#68580=CARTESIAN_POINT('Ctrl Pts',(0.00407002818633233,-0.0334688847587279,
0.0782860061867257));
#68581=CARTESIAN_POINT('Ctrl Pts',(0.00409800492366914,-0.0335216366562345,
0.0782574617909592));
#68582=CARTESIAN_POINT('Ctrl Pts',(0.00418821737084671,-0.0336938721132389,
0.0783429879810832));
#68583=CARTESIAN_POINT('Ctrl Pts',(0.00421276032088089,-0.0336474569764957,
0.0783660241479467));
#68584=CARTESIAN_POINT('Ctrl Pts',(0.00423757125663496,-0.033601104548885,
0.0783887714301394));
#68585=CARTESIAN_POINT('Ctrl Pts',(0.00430038684157254,-0.0334837508592656,
0.0784463623187233));
#68586=CARTESIAN_POINT('Ctrl Pts',(0.00436488137996903,-0.0333660264659097,
0.0785020665616132));
#68587=CARTESIAN_POINT('Ctrl Pts',(0.00418822741220353,-0.0336938721132389,
0.078343987788072));
#68588=CARTESIAN_POINT('Ctrl Pts',(0.00421277621443978,-0.0336474569764957,
0.0783670238961601));
#68589=CARTESIAN_POINT('Ctrl Pts',(0.00423759300130689,-0.033601104548885,
0.078389771051074));
#68590=CARTESIAN_POINT('Ctrl Pts',(0.00430042339991743,-0.0334837508592656,
0.0784473616174172));
#68591=CARTESIAN_POINT('Ctrl Pts',(0.00436493273593315,-0.0333660264659097,
0.0785030650992483));
#68592=CARTESIAN_POINT('Ctrl Pts',(0.00419164151788341,-0.0336938721132389,
0.0786839265813392));
#68593=CARTESIAN_POINT('Ctrl Pts',(0.00421818009468031,-0.0336474569764957,
0.0787069427055339));
#68594=CARTESIAN_POINT('Ctrl Pts',(0.00424498628583072,-0.033601104548885,
0.0787296465851001));
#68595=CARTESIAN_POINT('Ctrl Pts',(0.0043128533986939,-0.0334837508592656,
0.0787871275882126));
#68596=CARTESIAN_POINT('Ctrl Pts',(0.00438239399062286,-0.0333660264659097,
0.0788425723066389));
#68597=CARTESIAN_POINT('',(0.00420131034351263,-0.0336769361243753,0.0786902879412135));
#68598=CARTESIAN_POINT('',(0.00419162115542691,-0.033693872113232,0.0786818991133673));
#68599=CARTESIAN_POINT('Ctrl Pts',(0.00420131034351287,-0.033676936124375,
0.0786902879412137));
#68600=CARTESIAN_POINT('Ctrl Pts',(0.00419969386454803,-0.0336797586670257,
0.0786888914233459));
#68601=CARTESIAN_POINT('Ctrl Pts',(0.00419807819252284,-0.0336825812713308,
0.0786874940950229));
#68602=CARTESIAN_POINT('Ctrl Pts',(0.00419484846833955,-0.0336882265921195,
0.0786846978233311));
#68603=CARTESIAN_POINT('Ctrl Pts',(0.00419323441613566,-0.0336910493086635,
0.0786832988799539));
#68604=CARTESIAN_POINT('Ctrl Pts',(0.00419162115542556,-0.0336938721132361,
0.0786818991133772));
#68605=CARTESIAN_POINT('Ctrl Pts',(0.00420131034351269,-0.0336769361243753,
0.0786902879412135));
#68606=CARTESIAN_POINT('Ctrl Pts',(0.00422870993497068,-0.0336279031301507,
0.0786585727270677));
#68607=CARTESIAN_POINT('Ctrl Pts',(0.00425650373818913,-0.0335767851899387,
0.0786264012101173));
#68608=CARTESIAN_POINT('Ctrl Pts',(0.00431096501853182,-0.0334733198857322,
0.0785633619063608));
#68609=CARTESIAN_POINT('Ctrl Pts',(0.00433766906313391,-0.0334209645014062,
0.0785324517924494));
#68610=CARTESIAN_POINT('Ctrl Pts',(0.00436385853458973,-0.033367986984468,
0.0785021373004666));
#68611=CARTESIAN_POINT('',(0.00418992428383265,-0.0336938721132534,0.0785129434507367));
#68612=CARTESIAN_POINT('Origin',(0.00812378219310841,-0.0315241814719618,
0.07415));
#68613=CARTESIAN_POINT('',(0.00420131034436393,-0.0337108120655529,0.0786902879402389));
#68614=CARTESIAN_POINT('',(0.00421101742817701,-0.0336938721132327,0.0786986560536431));
#68615=CARTESIAN_POINT('Origin',(0.0157430862401175,-0.0345562509322005,
0.0670401444338427));
#68616=CARTESIAN_POINT('Ctrl Pts',(0.00421101742817892,-0.0336938721132319,
0.0786986560536424));
#68617=CARTESIAN_POINT('Ctrl Pts',(0.0042093982121299,-0.0336910493257073,
0.0786972632001427));
#68618=CARTESIAN_POINT('Ctrl Pts',(0.00420777968091916,-0.0336882266006415,
0.0786958694313745));
#68619=CARTESIAN_POINT('Ctrl Pts',(0.00420454398607452,-0.0336825812712706,
0.0786930800608296));
#68620=CARTESIAN_POINT('Ctrl Pts',(0.00420292682246003,-0.0336797586669955,
0.0786916844590663));
#68621=CARTESIAN_POINT('Ctrl Pts',(0.00420131034351245,-0.033676936124375,
0.0786902879412133));
#68622=CARTESIAN_POINT('Origin',(0.0140516683263155,-0.0345562513563432,
0.0655788895999354));
#68623=CARTESIAN_POINT('Ctrl Pts',(0.00424337814675107,-0.034243627687391,
0.0783950664820488));
#68624=CARTESIAN_POINT('Ctrl Pts',(0.00440348346849126,-0.0339430054201809,
0.078541418333298));
#68625=CARTESIAN_POINT('Ctrl Pts',(0.00457415776889112,-0.0336441434784052,
0.078675294625436));
#68626=CARTESIAN_POINT('Ctrl Pts',(0.00443152501705866,-0.034243627687391,
0.0785596895521011));
#68627=CARTESIAN_POINT('Ctrl Pts',(0.00459783920024025,-0.0339430054201809,
0.0786989453271564));
#68628=CARTESIAN_POINT('Ctrl Pts',(0.00477417021782287,-0.0336441434784052,
0.0788252780254251));
#68629=CARTESIAN_POINT('Ctrl Pts',(0.00443340648576174,-0.034243627687391,
0.0785613357828016));
#68630=CARTESIAN_POINT('Ctrl Pts',(0.00459978275755775,-0.0339430054201809,
0.078700520597095));
#68631=CARTESIAN_POINT('Ctrl Pts',(0.00477617034231219,-0.0336441434784052,
0.0788267778594251));
#68632=CARTESIAN_POINT('',(0.00445933600268769,-0.0341934961088741,0.0785828274405296));
#68633=CARTESIAN_POINT('',(0.00464455084769837,-0.033866421286606,0.0787296369122528));
#68634=CARTESIAN_POINT('Origin',(0.0155096437724735,-0.0345610720405944,
0.0660152563958636));
#68635=CARTESIAN_POINT('Origin',(-0.00198935276394271,-0.0336938005073003,
0.087461764218862));
#68636=CARTESIAN_POINT('',(0.00454583887293236,-0.0336938721132327,0.078652937552044));
#68637=CARTESIAN_POINT('',(0.0045956057767483,-0.0336938721132427,0.0786907463511036));
#68638=CARTESIAN_POINT('',(0.00436385853458568,-0.0340203938281605,0.0785021373004631));
#68639=CARTESIAN_POINT('Origin',(0.0158177017432013,-0.0345589643243796,
0.0663849008475276));
#68640=CARTESIAN_POINT('',(0.00436474667057904,-0.034193496108874,0.0785011092769962));
#68641=CARTESIAN_POINT('Origin',(-0.00283916590558952,-0.0341934220717559,
0.0868396860044658));
#68642=CARTESIAN_POINT('',(0.00441204133664336,-0.0341934961088841,0.078541968358773));
#68643=CARTESIAN_POINT('Ctrl Pts',(0.00402635966682603,-0.0340223579322397,
0.078533050152708));
#68644=CARTESIAN_POINT('Ctrl Pts',(0.00408681335990656,-0.0339125849573575,
0.078589564295872));
#68645=CARTESIAN_POINT('Ctrl Pts',(0.00414839428431968,-0.0338030433565231,
0.0786447874762301));
#68646=CARTESIAN_POINT('Ctrl Pts',(0.0042110174281763,-0.0336938721132327,
0.0786986560536433));
#68647=CARTESIAN_POINT('Ctrl Pts',(0.00413917444580609,-0.0340223579322397,
0.0785223728181119));
#68648=CARTESIAN_POINT('Ctrl Pts',(0.00419948087059488,-0.0339125849573575,
0.0785773309512404));
#68649=CARTESIAN_POINT('Ctrl Pts',(0.00426088242440792,-0.0338030433565231,
0.0786310022630648));
#68650=CARTESIAN_POINT('Ctrl Pts',(0.00432329450066539,-0.0336938721132327,
0.0786833250776902));
#68651=CARTESIAN_POINT('Ctrl Pts',(0.00425198922478615,-0.0340223579322397,
0.0785116954835158));
#68652=CARTESIAN_POINT('Ctrl Pts',(0.0043121483812832,-0.0339125849573575,
0.0785650976066089));
#68653=CARTESIAN_POINT('Ctrl Pts',(0.00437337056449616,-0.0338030433565231,
0.0786172170498995));
#68654=CARTESIAN_POINT('Ctrl Pts',(0.00443557157315449,-0.0336938721132327,
0.078667994101737));
#68655=CARTESIAN_POINT('Ctrl Pts',(0.00436480400376621,-0.0340223579322397,
0.0785010181489197));
#68656=CARTESIAN_POINT('Ctrl Pts',(0.00442481589197153,-0.0339125849573575,
0.0785528642619773));
#68657=CARTESIAN_POINT('Ctrl Pts',(0.0044858587045844,-0.0338030433565231,
0.0786034318367342));
#68658=CARTESIAN_POINT('Ctrl Pts',(0.00454784864564359,-0.0336938721132327,
0.0786526631257839));
#68659=CARTESIAN_POINT('',(0.00437842815056468,-0.0336938721132427,0.0786757968028536));
#68660=CARTESIAN_POINT('Ctrl Pts',(0.00420131034671543,-0.033710812066268,
0.0786902879375062));
#68661=CARTESIAN_POINT('Ctrl Pts',(0.00422942090869603,-0.0337611408994384,
0.0786577497701273));
#68662=CARTESIAN_POINT('Ctrl Pts',(0.00425701851528578,-0.03381210887815,
0.0786258053521147));
#68663=CARTESIAN_POINT('Ctrl Pts',(0.00431121295864493,-0.0339153382773232,
0.0785630749139882));
#68664=CARTESIAN_POINT('Ctrl Pts',(0.00433778686786166,-0.0339675558473116,
0.0785323154326729));
#68665=CARTESIAN_POINT('Ctrl Pts',(0.00436385853461576,-0.0340203938281304,
0.0785021373004364));
#68666=CARTESIAN_POINT('Ctrl Pts',(0.00445918833261691,-0.0341934961088741,
0.0785808046762242));
#68667=CARTESIAN_POINT('Ctrl Pts',(0.00455079172865743,-0.0340287516182427,
0.0786565672672794));
#68668=CARTESIAN_POINT('Ctrl Pts',(0.00464544817671417,-0.0338644633275951,
0.0787284790827956));
#68669=CARTESIAN_POINT('Ctrl Pts',(0.0044593360026877,-0.0341934961088741,
0.0785828274405296));
#68670=CARTESIAN_POINT('Ctrl Pts',(0.00455098121778667,-0.0340287516182427,
0.0786585869786223));
#68671=CARTESIAN_POINT('Ctrl Pts',(0.00464567932298703,-0.0338644633275951,
0.0787304940153715));
#68672=CARTESIAN_POINT('Ctrl Pts',(0.00448394067680217,-0.0341934961088741,
0.0789198588801231));
#68673=CARTESIAN_POINT('Ctrl Pts',(0.00458255375139738,-0.0340287516182427,
0.0789951097359624));
#68674=CARTESIAN_POINT('Ctrl Pts',(0.00468419273796784,-0.0338644633275951,
0.0790662205381982));
#68675=CARTESIAN_POINT('',(0.00449413748415137,-0.0341764758832413,0.0789276227642436));
#68676=CARTESIAN_POINT('',(0.00448394067680121,-0.034193496108874,0.0789198588801102));
#68677=CARTESIAN_POINT('Origin',(0.0149183650452552,-0.0345621026722942,
0.0660529651115736));
#68678=CARTESIAN_POINT('Ctrl Pts',(0.00449413748339433,-0.0341764758837513,
0.0789276227625805));
#68679=CARTESIAN_POINT('Ctrl Pts',(0.00452010417916289,-0.0341260050040843,
0.0788934433402988));
#68680=CARTESIAN_POINT('Ctrl Pts',(0.00454561948207761,-0.0340749269148962,
0.0788598580138956));
#68681=CARTESIAN_POINT('Ctrl Pts',(0.00459576722287304,-0.0339715436307836,
0.0787938496348361));
#68682=CARTESIAN_POINT('Ctrl Pts',(0.00462038064066904,-0.0339192778237455,
0.0787614516277956));
#68683=CARTESIAN_POINT('Ctrl Pts',(0.00464455084621759,-0.0338664212855905,
0.078729636912815));
#68684=CARTESIAN_POINT('',(0.00447163833975446,-0.0341934961088841,0.0787513431603299));
#68685=CARTESIAN_POINT('Origin',(0.00812378219310841,-0.0315241814719618,
0.07415));
#68686=CARTESIAN_POINT('',(0.00449413748526666,-0.0342105180190354,0.0789276227641661));
#68687=CARTESIAN_POINT('',(0.00450435085242285,-0.0341934961088739,0.0789353648523489));
#68688=CARTESIAN_POINT('Origin',(0.0148856805237589,-0.0345621700122827,
0.0660215583807938));
#68689=CARTESIAN_POINT('Origin',(0.0141028267023117,-0.0345621042433387,
0.0654333822330383));
#68690=CARTESIAN_POINT('Origin',(0.0141418420727513,-0.0345621713716514,
0.0654564562677148));
#68691=CARTESIAN_POINT('Ctrl Pts',(0.00454464445934973,-0.0346945769586966,
0.0786520301348715));
#68692=CARTESIAN_POINT('Ctrl Pts',(0.00463894128303914,-0.0345275153362944,
0.0787269966077136));
#68693=CARTESIAN_POINT('Ctrl Pts',(0.00473562012328609,-0.0343603235965186,
0.0787990169224147));
#68694=CARTESIAN_POINT('Ctrl Pts',(0.00483439188120101,-0.034193496108874,
0.0788678823245642));
#68695=CARTESIAN_POINT('Ctrl Pts',(0.00461139846911413,-0.0346945769586966,
0.0787027443394518));
#68696=CARTESIAN_POINT('Ctrl Pts',(0.00470675752212333,-0.0345275153362944,
0.0787763126228326));
#68697=CARTESIAN_POINT('Ctrl Pts',(0.00480445489466537,-0.0343603235965186,
0.0788469009802945));
#68698=CARTESIAN_POINT('Ctrl Pts',(0.0049041985384288,-0.034193496108874,
0.0789143049372926));
#68699=CARTESIAN_POINT('Ctrl Pts',(0.00467815247887855,-0.0346945769586966,
0.0787534585440321));
#68700=CARTESIAN_POINT('Ctrl Pts',(0.0047745737612075,-0.0345275153362944,
0.0788256286379508));
#68701=CARTESIAN_POINT('Ctrl Pts',(0.00487328966604467,-0.0343603235965186,
0.0788947850381736));
#68702=CARTESIAN_POINT('Ctrl Pts',(0.00497400519565672,-0.034193496108874,
0.0789607275500208));
#68703=CARTESIAN_POINT('Ctrl Pts',(0.00474490648864292,-0.0346945769586966,
0.0788041727486125));
#68704=CARTESIAN_POINT('Ctrl Pts',(0.00484239000029171,-0.0345275153362944,
0.0788749446530705));
#68705=CARTESIAN_POINT('Ctrl Pts',(0.00494212443742393,-0.0343603235965186,
0.0789426690960541));
#68706=CARTESIAN_POINT('Ctrl Pts',(0.00504381185288439,-0.034193496108874,
0.0790071501627492));
#68707=CARTESIAN_POINT('',(0.00474490648816067,-0.0346945769586966,0.0788041727482459));
#68708=CARTESIAN_POINT('',(0.00493897409661285,-0.0343667727831496,0.0789390627881592));
#68709=CARTESIAN_POINT('Origin',(0.0144741125225068,-0.0345626457065151,
0.0650914123699995));
#68710=CARTESIAN_POINT('Origin',(-0.00118115406393903,-0.0341934771028877,
0.0881420343625942));
#68711=CARTESIAN_POINT('',(0.00483564091507222,-0.034193496108874,0.0788687129533036));
#68712=CARTESIAN_POINT('',(0.00488768364940678,-0.034193496108884,0.0789033222555896));
#68713=CARTESIAN_POINT('',(0.00464455084722664,-0.0345211942962657,0.0787296369115627));
#68714=CARTESIAN_POINT('Origin',(0.0148549574993365,-0.0345625596120213,
0.0653849219839156));
#68715=CARTESIAN_POINT('',(0.00464537268054424,-0.0346945769586886,0.0787285551501433));
#68716=CARTESIAN_POINT('Origin',(-0.00204743084295042,-0.0346945685853865,
0.0875381462982233));
#68717=CARTESIAN_POINT('',(0.00469513958436245,-0.0346945769587026,0.0787663639492045));
#68718=CARTESIAN_POINT('Ctrl Pts',(0.00430965973317534,-0.0345231616327842,
0.0787816811052434));
#68719=CARTESIAN_POINT('Ctrl Pts',(0.00437350093632571,-0.0344132092796988,
0.0788342534134986));
#68720=CARTESIAN_POINT('Ctrl Pts',(0.00443842626229129,-0.034303273855898,
0.0788855025043345));
#68721=CARTESIAN_POINT('Ctrl Pts',(0.00450435085242282,-0.0341934961088739,
0.078935364852349));
#68722=CARTESIAN_POINT('Ctrl Pts',(0.00442158126932214,-0.0345231616327842,
0.0787639411535772));
#68723=CARTESIAN_POINT('Ctrl Pts',(0.00448517795221465,-0.0344132092796988,
0.0788149707810296));
#68724=CARTESIAN_POINT('Ctrl Pts',(0.00454982686140292,-0.034303273855898,
0.0788646823283665));
#68725=CARTESIAN_POINT('Ctrl Pts',(0.00461544354281598,-0.0341934961088739,
0.0789130142308859));
#68726=CARTESIAN_POINT('Ctrl Pts',(0.00453350280546893,-0.0345231616327842,
0.0787462012019111));
#68727=CARTESIAN_POINT('Ctrl Pts',(0.00459685496810358,-0.0344132092796988,
0.0787956881485606));
#68728=CARTESIAN_POINT('Ctrl Pts',(0.00466122746051455,-0.0343032738558979,
0.0788438621523986));
#68729=CARTESIAN_POINT('Ctrl Pts',(0.00472653623320913,-0.0341934961088739,
0.0788906636094228));
#68730=CARTESIAN_POINT('Ctrl Pts',(0.00464542434161573,-0.0345231616327842,
0.0787284612502449));
#68731=CARTESIAN_POINT('Ctrl Pts',(0.00470853198399252,-0.0344132092796988,
0.0787764055160916));
#68732=CARTESIAN_POINT('Ctrl Pts',(0.00477262805962619,-0.0343032738558979,
0.0788230419764306));
#68733=CARTESIAN_POINT('Ctrl Pts',(0.00483762892360229,-0.0341934961088739,
0.0788683129879597));
#68734=CARTESIAN_POINT('',(0.00466999588375753,-0.0341934961088839,0.0789020389028363));
#68735=CARTESIAN_POINT('Ctrl Pts',(0.00449413748735283,-0.0342105180195383,
0.0789276227614087));
#68736=CARTESIAN_POINT('Ctrl Pts',(0.00452013338569833,-0.0342610556241287,
0.0788934049231057));
#68737=CARTESIAN_POINT('Ctrl Pts',(0.00454566280108907,-0.0343122189870131,
0.0788598011062189));
#68738=CARTESIAN_POINT('Ctrl Pts',(0.00459581104454471,-0.0344158119695132,
0.0787937920588325));
#68739=CARTESIAN_POINT('Ctrl Pts',(0.0046204093616113,-0.034468199045002,
0.0787614138265159));
#68740=CARTESIAN_POINT('Ctrl Pts',(0.00464455084723834,-0.0345211942962437,
0.0787296369115348));
#68741=CARTESIAN_POINT('Ctrl Pts',(0.00474463216623766,-0.0346945769586932,
0.0788021637397005));
#68742=CARTESIAN_POINT('Ctrl Pts',(0.00484081235979049,-0.034529677707698,
0.0788720252754961));
#68743=CARTESIAN_POINT('Ctrl Pts',(0.00493979781004147,-0.034364806625142,
0.078937851899701));
#68744=CARTESIAN_POINT('Ctrl Pts',(0.00474490648815338,-0.0346945769586932,
0.0788041727482405));
#68745=CARTESIAN_POINT('Ctrl Pts',(0.00484112821653624,-0.034529677707698,
0.0788740286126247));
#68746=CARTESIAN_POINT('Ctrl Pts',(0.00494015493172163,-0.034364806625142,
0.0789398478535915));
#68747=CARTESIAN_POINT('Ctrl Pts',(0.0047906249897536,-0.0346945769586932,
0.0791389941930059));
#68748=CARTESIAN_POINT('Ctrl Pts',(0.00489376891459494,-0.034529677707698,
0.0792079048597189));
#68749=CARTESIAN_POINT('Ctrl Pts',(0.00499967284542011,-0.034364806625142,
0.0792724936099335));
#68750=CARTESIAN_POINT('',(0.00480128917430954,-0.0346775396665,0.0791461024942956));
#68751=CARTESIAN_POINT('',(0.00479062498975458,-0.0346945769586886,0.0791389941929943));
#68752=CARTESIAN_POINT('Origin',(0.0138668481856376,-0.0345626618035967,
0.065238243567384));
#68753=CARTESIAN_POINT('Ctrl Pts',(0.00480128917354233,-0.0346775396670097,
0.0791461024926342));
#68754=CARTESIAN_POINT('Ctrl Pts',(0.004825077207445,-0.0346269749928202,
0.0791103319034466));
#68755=CARTESIAN_POINT('Ctrl Pts',(0.00484844244499505,-0.034575790289082,
0.079075197017556));
#68756=CARTESIAN_POINT('Ctrl Pts',(0.00489434671355866,-0.0344721681087932,
0.079006169812157));
#68757=CARTESIAN_POINT('Ctrl Pts',(0.00491686775263628,-0.0344197714289493,
0.0789723045576773));
#68758=CARTESIAN_POINT('Ctrl Pts',(0.0049389740963452,-0.0343667727830694,
0.078939062788109));
#68759=CARTESIAN_POINT('',(0.00476776573896762,-0.0346945769587026,0.0789715834706301));
#68760=CARTESIAN_POINT('Ctrl Pts',(0.00480399461433585,-0.0352450361874068,
0.0788465703505273));
#68761=CARTESIAN_POINT('Ctrl Pts',(0.00498112867174079,-0.0349452760959493,
0.0789717781936259));
#68762=CARTESIAN_POINT('Ctrl Pts',(0.00516719067698568,-0.0346444289841739,
0.0790832878724453));
#68763=CARTESIAN_POINT('Ctrl Pts',(0.00480608832337919,-0.0352450361874068,
0.0788479817354648));
#68764=CARTESIAN_POINT('Ctrl Pts',(0.00498327561204054,-0.0349452760959493,
0.0789731106130311));
#68765=CARTESIAN_POINT('Ctrl Pts',(0.00516938474931044,-0.0346444289841739,
0.0790845375410549));
#68766=CARTESIAN_POINT('Ctrl Pts',(0.00501338624846292,-0.0352450361874068,
0.078987722818386));
#68767=CARTESIAN_POINT('Ctrl Pts',(0.00519584395855024,-0.0349452760959493,
0.0791050333264142));
#68768=CARTESIAN_POINT('Ctrl Pts',(0.00538661963294988,-0.0346444289841739,
0.0792082671063583));
#68769=CARTESIAN_POINT('Ctrl Pts',(0.00501545922771376,-0.0352450361874068,
0.0789891202292151));
#68770=CARTESIAN_POINT('Ctrl Pts',(0.00519796964201533,-0.0349452760959493,
0.0791063525535481));
#68771=CARTESIAN_POINT('Ctrl Pts',(0.00538879198178627,-0.0346444289841739,
0.0792095044020113));
#68772=CARTESIAN_POINT('',(0.00504378325369919,-0.0351951634053304,0.0790071348381277));
#68773=CARTESIAN_POINT('',(0.00524596632825134,-0.0348678972925388,0.0791295884215443));
#68774=CARTESIAN_POINT('Origin',(0.0132614616026492,-0.0345636767886549,
0.0644169237729676));
#68775=CARTESIAN_POINT('Origin',(-0.000283058594760006,-0.0346946199341104,
0.0886966607326437));
#68776=CARTESIAN_POINT('',(0.00513841973333968,-0.0346945769330289,0.0790658657408367));
#68777=CARTESIAN_POINT('',(0.00519253291664268,-0.0346945769458128,0.0790971389638961));
#68778=CARTESIAN_POINT('',(0.00493897409645518,-0.0350221583435553,0.0789390627880089));
#68779=CARTESIAN_POINT('Origin',(0.013696925733086,-0.0345628459369985,
0.0646206747760047));
#68780=CARTESIAN_POINT('',(0.00493965650132374,-0.0351951360298761,0.0789380311793917));
#68781=CARTESIAN_POINT('Origin',(-0.00116208724412833,-0.0351951838366679,
0.0881133549896872));
#68782=CARTESIAN_POINT('',(0.00504381185230669,-0.0351951371328748,0.0790071501625045));
#68783=CARTESIAN_POINT('Ctrl Pts',(0.00504352329155854,-0.0351951371254922,
0.0790057158847739));
#68784=CARTESIAN_POINT('Ctrl Pts',(0.00514391217089723,-0.0350307338980945,
0.0790693983049438));
#68785=CARTESIAN_POINT('Ctrl Pts',(0.00524684733166884,-0.0348659306897824,
0.0791288771281542));
#68786=CARTESIAN_POINT('Ctrl Pts',(0.00504381185236551,-0.0351951371254922,
0.0790071501624043));
#68787=CARTESIAN_POINT('Ctrl Pts',(0.00514423038449431,-0.0350307338980945,
0.0790708266167605));
#68788=CARTESIAN_POINT('Ctrl Pts',(0.00524719492614438,-0.0348659306897824,
0.0791302982536733));
#68789=CARTESIAN_POINT('Ctrl Pts',(0.00509217494435261,-0.0351951371254922,
0.0792475365880562));
#68790=CARTESIAN_POINT('Ctrl Pts',(0.00519756331500823,-0.0350307338980945,
0.0793102131658296));
#68791=CARTESIAN_POINT('Ctrl Pts',(0.00530545212250922,-0.0348659306897824,
0.0793684803717592));
#68792=CARTESIAN_POINT('Origin',(0.0025848997906258,-0.0308609197411455,
0.0837341276772471));
#68793=CARTESIAN_POINT('',(0.00506489707002948,-0.0351951371254922,0.0791119532239969));
#68794=CARTESIAN_POINT('Origin',(0.00812378219310841,-0.0315241814719618,
0.07415));
#68795=CARTESIAN_POINT('',(0.0048012891755772,-0.0347116136489781,0.0791461024937229));
#68796=CARTESIAN_POINT('',(0.00481196851860944,-0.0346945769586885,0.0791531880022078));
#68797=CARTESIAN_POINT('Origin',(0.0138281143311945,-0.0345626675566824,
0.0652147260523571));
#68798=CARTESIAN_POINT('Origin',(0.0141211786267606,-0.0345626631941208,
0.0654073732970256));
#68799=CARTESIAN_POINT('Origin',(0.0141578417119078,-0.0345626691539936,
0.0654340041758359));
#68800=CARTESIAN_POINT('Ctrl Pts',(0.00460801247398302,-0.0350241211494502,
0.0790120328343313));
#68801=CARTESIAN_POINT('Ctrl Pts',(0.00467498498276811,-0.0349144232819069,
0.0790604611206929));
#68802=CARTESIAN_POINT('Ctrl Pts',(0.00474299862511201,-0.0348045283579466,
0.0791075340241056));
#68803=CARTESIAN_POINT('Ctrl Pts',(0.00481196852787608,-0.0346945769439158,
0.0791531880083418));
#68804=CARTESIAN_POINT('Ctrl Pts',(0.00471859927819826,-0.0350241211494502,
0.0789873002538434));
#68805=CARTESIAN_POINT('Ctrl Pts',(0.00478523110582786,-0.0349144232819069,
0.0790342052523193));
#68806=CARTESIAN_POINT('Ctrl Pts',(0.0048528723756531,-0.0348045283579466,
0.0790797609982078));
#68807=CARTESIAN_POINT('Ctrl Pts',(0.00492143861918303,-0.0346945769439158,
0.0791239059163165));
#68808=CARTESIAN_POINT('Ctrl Pts',(0.00482918608241349,-0.0350241211494502,
0.0789625676733555));
#68809=CARTESIAN_POINT('Ctrl Pts',(0.00489547722888761,-0.0349144232819069,
0.0790079493839456));
#68810=CARTESIAN_POINT('Ctrl Pts',(0.00496274612619419,-0.0348045283579466,
0.0790519879723101));
#68811=CARTESIAN_POINT('Ctrl Pts',(0.00503090871048998,-0.0346945769439158,
0.0790946238242913));
#68812=CARTESIAN_POINT('Ctrl Pts',(0.00493977288662872,-0.0350241211494502,
0.0789378350928677));
#68813=CARTESIAN_POINT('Ctrl Pts',(0.00500572335194736,-0.0349144232819069,
0.078981693515572));
#68814=CARTESIAN_POINT('Ctrl Pts',(0.00507261987673527,-0.0348045283579466,
0.0790242149464124));
#68815=CARTESIAN_POINT('Ctrl Pts',(0.00514037880179692,-0.0346945769439158,
0.079065341732266));
#68816=CARTESIAN_POINT('',(0.00497519412568671,-0.0346945769458128,0.0791095268714466));
#68817=CARTESIAN_POINT('Ctrl Pts',(0.00480128917739434,-0.0347116136492789,
0.079146102490978));
#68818=CARTESIAN_POINT('Ctrl Pts',(0.00482506777527153,-0.0347621546532295,
0.0791103461142078));
#68819=CARTESIAN_POINT('Ctrl Pts',(0.00484842828114121,-0.0348133084097021,
0.0790752184311656));
#68820=CARTESIAN_POINT('Ctrl Pts',(0.0048943326048069,-0.0349168561544683,
0.0790061911360808));
#68821=CARTESIAN_POINT('Ctrl Pts',(0.00491685821468387,-0.0349692089016065,
0.0789723189036683));
#68822=CARTESIAN_POINT('Ctrl Pts',(0.00493897409648279,-0.0350221583435177,
0.0789390627879674));
#68823=CARTESIAN_POINT('Origin',(0.0084849663280849,-0.0351840467447566,
0.0732420948397483));
#68824=CARTESIAN_POINT('Origin',(0.00283797433828648,-0.0352322613188162,
0.0848844373324612));
#68825=CARTESIAN_POINT('',(0.00545327161097464,-0.0351951142564667,0.0792437400615015));
#68826=CARTESIAN_POINT('',(0.0055649206081788,-0.0351951372916786,0.0792992453222945));
#68827=CARTESIAN_POINT('Origin',(0.00846304037582862,-0.0352875132321111,
0.0741190968493382));
#68828=CARTESIAN_POINT('Origin',(0.0021682874759184,-0.0298325076522524,
0.0695863092837193));
#68829=CARTESIAN_POINT('Origin',(0.00184281903255471,-0.033873222743243,
0.0796997796762625));
#68830=CARTESIAN_POINT('Ctrl Pts',(0.0029690848306492,-0.0321934096636942,
0.0767009274483544));
#68831=CARTESIAN_POINT('Ctrl Pts',(0.00301474521723456,-0.0320508460843402,
0.0767931940764988));
#68832=CARTESIAN_POINT('Ctrl Pts',(0.00306285019798059,-0.0319086045661229,
0.0768841643308079));
#68833=CARTESIAN_POINT('Ctrl Pts',(0.00311328006876048,-0.0317669892865148,
0.0769736508635441));
#68834=CARTESIAN_POINT('Ctrl Pts',(0.00300789924387488,-0.0321934096636942,
0.0767752502170988));
#68835=CARTESIAN_POINT('Ctrl Pts',(0.0030548899726286,-0.0320508460843402,
0.0768668220857297));
#68836=CARTESIAN_POINT('Ctrl Pts',(0.00310430562564333,-0.0319086045661229,
0.0769570623607072));
#68837=CARTESIAN_POINT('Ctrl Pts',(0.00315602380608249,-0.0317669892865148,
0.0770457854984011));
#68838=CARTESIAN_POINT('Ctrl Pts',(0.00304671365710054,-0.0321934096636942,
0.0768495729858433));
#68839=CARTESIAN_POINT('Ctrl Pts',(0.00309503472802263,-0.0320508460843402,
0.0769404500949606));
#68840=CARTESIAN_POINT('Ctrl Pts',(0.00314576105330607,-0.0319086045661229,
0.0770299603906066));
#68841=CARTESIAN_POINT('Ctrl Pts',(0.00319876754340448,-0.0317669892865148,
0.077117920133258));
#68842=CARTESIAN_POINT('Ctrl Pts',(0.00308552807032622,-0.0321934096636942,
0.0769238957545877));
#68843=CARTESIAN_POINT('Ctrl Pts',(0.00313517948341667,-0.0320508460843402,
0.0770140781041916));
#68844=CARTESIAN_POINT('Ctrl Pts',(0.00318721648096881,-0.0319086045661229,
0.0771028584205059));
#68845=CARTESIAN_POINT('Ctrl Pts',(0.00324151128072648,-0.0317669892865148,
0.0771900547681149));
#68846=CARTESIAN_POINT('',(0.00308483367280552,-0.0321934096636942,0.0769225661055668));
#68847=CARTESIAN_POINT('',(0.0032029979100201,-0.0318665617511297,0.0771272482309031));
#68848=CARTESIAN_POINT('Origin',(0.0180113624498778,-0.0326371944420234,
0.069411464754423));
#68849=CARTESIAN_POINT('Origin',(-0.00617524371148055,-0.0316939261508981,
0.0828014155067585));
#68850=CARTESIAN_POINT('',(0.00302592857898553,-0.032019722162177,0.0768126073115477));
#68851=CARTESIAN_POINT('Ctrl Pts',(0.0030259695587903,-0.032019739209469,
0.0768127876876422));
#68852=CARTESIAN_POINT('Ctrl Pts',(0.00303951872021519,-0.0319792716575989,
0.0768387269754978));
#68853=CARTESIAN_POINT('Ctrl Pts',(0.00305332731327124,-0.0319386439829633,
0.0768646810555132));
#68854=CARTESIAN_POINT('Ctrl Pts',(0.0030674173008937,-0.0318979099381565,
0.0768906732020765));
#68855=CARTESIAN_POINT('Ctrl Pts',(0.00308150701001716,-0.0318571766984882,
0.0769166648348857));
#68856=CARTESIAN_POINT('Ctrl Pts',(0.00309580492313141,-0.0318163871833546,
0.0769425632753775));
#68857=CARTESIAN_POINT('Ctrl Pts',(0.00311025877872009,-0.0317755399638303,
0.0769682811454069));
#68858=CARTESIAN_POINT('',(0.00302696919836558,-0.0321934096636183,0.0768117658230244));
#68859=CARTESIAN_POINT('Origin',(0.000990947553938459,-0.0324112197412341,
0.0778987847009924));
#68860=CARTESIAN_POINT('',(0.00305590143559555,-0.0321934096636663,0.0768671659643057));
#68861=CARTESIAN_POINT('Ctrl Pts',(0.00308544102434413,-0.0321934096636618,
0.0769206309540255));
#68862=CARTESIAN_POINT('Ctrl Pts',(0.00312365018450362,-0.0320835708272592,
0.0769901136053962));
#68863=CARTESIAN_POINT('Ctrl Pts',(0.00316327512165632,-0.0319739230346489,
0.0770587652174217));
#68864=CARTESIAN_POINT('Ctrl Pts',(0.00320425839735533,-0.0318646057455573,
0.0771265018460079));
#68865=CARTESIAN_POINT('Ctrl Pts',(0.00305150767364851,-0.0321934096636618,
0.0770287498352429));
#68866=CARTESIAN_POINT('Ctrl Pts',(0.00309120787744292,-0.0320835708272592,
0.0770987004539658));
#68867=CARTESIAN_POINT('Ctrl Pts',(0.00313233267792466,-0.0319739230346489,
0.0771677889048329));
#68868=CARTESIAN_POINT('Ctrl Pts',(0.00317482267478138,-0.0318646057455573,
0.0772359308321207));
#68869=CARTESIAN_POINT('Ctrl Pts',(0.0030175743229529,-0.0321934096636618,
0.0771368687164603));
#68870=CARTESIAN_POINT('Ctrl Pts',(0.00305876557038222,-0.0320835708272592,
0.0772072873025354));
#68871=CARTESIAN_POINT('Ctrl Pts',(0.00310139023419301,-0.0319739230346489,
0.0772768125922441));
#68872=CARTESIAN_POINT('Ctrl Pts',(0.00314538695220742,-0.0318646057455573,
0.0773453598182336));
#68873=CARTESIAN_POINT('Ctrl Pts',(0.00298364097225728,-0.0321934096636618,
0.0772449875976778));
#68874=CARTESIAN_POINT('Ctrl Pts',(0.00302632326332152,-0.0320835708272592,
0.0773158741511051));
#68875=CARTESIAN_POINT('Ctrl Pts',(0.00307044779046135,-0.0319739230346489,
0.0773858362796553));
#68876=CARTESIAN_POINT('Ctrl Pts',(0.00311595122963347,-0.0318646057455573,
0.0774547888043465));
#68877=CARTESIAN_POINT('',(0.00299026364896617,-0.0321763980308285,0.0772559599699106));
#68878=CARTESIAN_POINT('',(0.00298364097227652,-0.0321934096636184,0.0772449875976981));
#68879=CARTESIAN_POINT('Origin',(0.0174560957059853,-0.0326386229898935,
0.0692206757338883));
#68880=CARTESIAN_POINT('Ctrl Pts',(0.00299026365167526,-0.0321763980306317,
0.0772559599682634));
#68881=CARTESIAN_POINT('Ctrl Pts',(0.00302698447414228,-0.0321259596175778,
0.0772337425741577));
#68882=CARTESIAN_POINT('Ctrl Pts',(0.00306306906071051,-0.0320749164633317,
0.0772119101252265));
#68883=CARTESIAN_POINT('Ctrl Pts',(0.00313399480201706,-0.0319716057793942,
0.0771689975475394));
#68884=CARTESIAN_POINT('Ctrl Pts',(0.00316880832151041,-0.0319193786690141,
0.0771479341390824));
#68885=CARTESIAN_POINT('Ctrl Pts',(0.00320299791160168,-0.0318665617525326,
0.0771272482299349));
#68886=CARTESIAN_POINT('',(0.00303423732255102,-0.0321934096636663,0.0770837768516425));
#68887=CARTESIAN_POINT('Origin',(0.00812378219310841,-0.0315241814719618,
0.07415));
#68888=CARTESIAN_POINT('',(0.00299026364864828,-0.0322104233323768,0.0772559599701025));
#68889=CARTESIAN_POINT('',(0.00299690974454782,-0.0321934096636183,0.0772669181728473));
#68890=CARTESIAN_POINT('Origin',(0.0174382634095364,-0.0326387226163109,
0.0691789946233088));
#68891=CARTESIAN_POINT('Origin',(0.0168209260078138,-0.0326386248122561,
0.0681708631843273));
#68892=CARTESIAN_POINT('Origin',(0.0168495664139399,-0.0326387239598755,
0.0682060057493927));
#68893=CARTESIAN_POINT('Ctrl Pts',(0.00312151735985888,-0.0327445246967096,
0.0769882162599131));
#68894=CARTESIAN_POINT('Ctrl Pts',(0.00322856243605139,-0.032443687833936,
0.0771768797623295));
#68895=CARTESIAN_POINT('Ctrl Pts',(0.00334951431456717,-0.0321434074405928,
0.0773569442190236));
#68896=CARTESIAN_POINT('Ctrl Pts',(0.00324958558167206,-0.0327445246967096,
0.0772029219434933));
#68897=CARTESIAN_POINT('Ctrl Pts',(0.00336472841510119,-0.032443687833936,
0.0773867552739614));
#68898=CARTESIAN_POINT('Ctrl Pts',(0.00349339121768822,-0.0321434074405928,
0.0775613933245446));
#68899=CARTESIAN_POINT('',(0.00326886775284126,-0.0326943950436612,0.0772334932751161));
#68900=CARTESIAN_POINT('',(0.00339965091615906,-0.0323666188837389,0.0774303519137662));
#68901=CARTESIAN_POINT('Origin',(0.0174186577702613,-0.0326395579108609,
0.0681565168690591));
#68902=CARTESIAN_POINT('Origin',(-0.00567232325795304,-0.032193382560304,
0.0837297690636582));
#68903=CARTESIAN_POINT('',(0.00332947165196833,-0.0321934096532689,0.0773269028049071));
#68904=CARTESIAN_POINT('',(0.00336511922998225,-0.0321934096584275,0.0773782399311192));
#68905=CARTESIAN_POINT('',(0.00320299790920229,-0.0325210109756239,0.0771272482313813));
#68906=CARTESIAN_POINT('Origin',(0.0176546596804715,-0.0326393129161776,
0.0685754291857115));
#68907=CARTESIAN_POINT('',(0.0032041602534476,-0.0326943950436593,0.077126544972079));
#68908=CARTESIAN_POINT('Origin',(-0.00626072666954365,-0.0326943765538048,
0.0828531348999376));
#68909=CARTESIAN_POINT('',(0.00323651400315443,-0.0326943950436702,0.0771800191236075));
#68910=CARTESIAN_POINT('Ctrl Pts',(0.00287246520896839,-0.0325229783203769,
0.0770523559278832));
#68911=CARTESIAN_POINT('Ctrl Pts',(0.00291247412196393,-0.032413025309245,
0.0771247452176709));
#68912=CARTESIAN_POINT('Ctrl Pts',(0.00295397443227379,-0.032303122220807,
0.077196295892444));
#68913=CARTESIAN_POINT('Ctrl Pts',(0.0029969097468773,-0.0321934096576658,
0.077266918176679));
#68914=CARTESIAN_POINT('Ctrl Pts',(0.00298305775896316,-0.0325229783203769,
0.0770770628119856));
#68915=CARTESIAN_POINT('Ctrl Pts',(0.00302340725581576,-0.032413025309245,
0.0771479275858901));
#68916=CARTESIAN_POINT('Ctrl Pts',(0.00306521656175702,-0.032303122220807,
0.0772179469305881));
#68917=CARTESIAN_POINT('Ctrl Pts',(0.00310842895718062,-0.0321934096576658,
0.0772870330460477));
#68918=CARTESIAN_POINT('Ctrl Pts',(0.00309365030895794,-0.0325229783203769,
0.0771017696960881));
#68919=CARTESIAN_POINT('Ctrl Pts',(0.00313434038966758,-0.032413025309245,
0.0771711099541094));
#68920=CARTESIAN_POINT('Ctrl Pts',(0.00317645869124026,-0.032303122220807,
0.0772395979687324));
#68921=CARTESIAN_POINT('Ctrl Pts',(0.00321994816748395,-0.0321934096576658,
0.0773071479154165));
#68922=CARTESIAN_POINT('Ctrl Pts',(0.00320424285895271,-0.0325229783203769,
0.0771264765801905));
#68923=CARTESIAN_POINT('Ctrl Pts',(0.0032452735235194,-0.032413025309245,
0.0771942923223286));
#68924=CARTESIAN_POINT('Ctrl Pts',(0.00328770082072349,-0.032303122220807,
0.0772612490068766));
#68925=CARTESIAN_POINT('Ctrl Pts',(0.00333146737778727,-0.0321934096576658,
0.0773272627847852));
#68926=CARTESIAN_POINT('',(0.00316319069787418,-0.0321934096584275,0.0772969104885515));
#68927=CARTESIAN_POINT('Ctrl Pts',(0.00299026365162035,-0.0322104233328919,
0.0772559599682966));
#68928=CARTESIAN_POINT('Ctrl Pts',(0.00302703423146573,-0.0322609421831417,
0.0772337124692202));
#68929=CARTESIAN_POINT('Ctrl Pts',(0.00306314312537439,-0.0323120888240841,
0.0772118653134978));
#68930=CARTESIAN_POINT('Ctrl Pts',(0.00313406940354204,-0.0324156524631809,
0.0771689524109907));
#68931=CARTESIAN_POINT('Ctrl Pts',(0.00316885763339512,-0.0324680267167311,
0.077147904303651));
#68932=CARTESIAN_POINT('Ctrl Pts',(0.00320299790924169,-0.0325210109755913,
0.0771272482313627));
#68933=CARTESIAN_POINT('Origin',(0.00489127226361921,-0.0262834582511723,
0.0669768371414704));
#68934=CARTESIAN_POINT('Origin',(-0.00399534140117125,-0.0342770905168603,
0.0751251954865947));
#68935=CARTESIAN_POINT('Ctrl Pts',(0.00326935227917528,-0.0326943950436604,
0.0772315242842415));
#68936=CARTESIAN_POINT('Ctrl Pts',(0.00331182145920417,-0.0325844576448134,
0.0772984274266268));
#68937=CARTESIAN_POINT('Ctrl Pts',(0.00335567731151665,-0.0324744968375322,
0.0773644569715792));
#68938=CARTESIAN_POINT('Ctrl Pts',(0.00340086247853638,-0.0323646534831894,
0.0774295290932336));
#68939=CARTESIAN_POINT('Ctrl Pts',(0.00324227476812217,-0.0326943950436604,
0.0773415603509526));
#68940=CARTESIAN_POINT('Ctrl Pts',(0.00328626045137991,-0.0325844576448134,
0.0774088366721889));
#68941=CARTESIAN_POINT('Ctrl Pts',(0.003331640632197,-0.0324744968375322,
0.0774752080586296));
#68942=CARTESIAN_POINT('Ctrl Pts',(0.00337835599389737,-0.0323646534831894,
0.0775405902733609));
#68943=CARTESIAN_POINT('Ctrl Pts',(0.00321519725706906,-0.0326943950436604,
0.0774515964176637));
#68944=CARTESIAN_POINT('Ctrl Pts',(0.00326069944355565,-0.0325844576448134,
0.077519245917751));
#68945=CARTESIAN_POINT('Ctrl Pts',(0.00330760395287735,-0.0324744968375322,
0.0775859591456801));
#68946=CARTESIAN_POINT('Ctrl Pts',(0.00335584950925836,-0.0323646534831894,
0.0776516514534883));
#68947=CARTESIAN_POINT('Ctrl Pts',(0.00318811974601596,-0.0326943950436604,
0.0775616324843749));
#68948=CARTESIAN_POINT('Ctrl Pts',(0.00323513843573139,-0.0325844576448134,
0.0776296551633131));
#68949=CARTESIAN_POINT('Ctrl Pts',(0.0032835672735577,-0.0324744968375322,
0.0776967102327305));
#68950=CARTESIAN_POINT('Ctrl Pts',(0.00333334302461935,-0.0323646534831894,
0.0777627126336156));
#68951=CARTESIAN_POINT('',(0.00319541831515216,-0.0326773559991361,0.077572167363916));
#68952=CARTESIAN_POINT('',(0.0031881197460185,-0.0326943950436594,0.0775616324843668));
#68953=CARTESIAN_POINT('Origin',(0.0168061277761233,-0.0326395670836268,
0.0680599699871882));
#68954=CARTESIAN_POINT('Ctrl Pts',(0.00319541831789935,-0.0326773559987466,
0.0775721673619998));
#68955=CARTESIAN_POINT('Ctrl Pts',(0.00323070000797244,-0.0326267922586965,
0.0775476683900689));
#68956=CARTESIAN_POINT('Ctrl Pts',(0.00326535635556921,-0.0325756109581347,
0.0775236036447224));
#68957=CARTESIAN_POINT('Ctrl Pts',(0.00333344786032804,-0.0324719985462373,
0.0774763221267347));
#68958=CARTESIAN_POINT('Ctrl Pts',(0.00336685570765316,-0.032419609162177,
0.0774531243175539));
#68959=CARTESIAN_POINT('Ctrl Pts',(0.00339965091619911,-0.0323666188837756,
0.0774303519137384));
#68960=CARTESIAN_POINT('',(0.00322849374943987,-0.0326943950436702,0.0773975628797515));
#68961=CARTESIAN_POINT('Origin',(0.00812378219310841,-0.0315241814719618,
0.07415));
#68962=CARTESIAN_POINT('',(0.0031954183151884,-0.0327114338379857,0.0775721673638903));
#68963=CARTESIAN_POINT('',(0.00320273936760646,-0.0326943950436593,0.0775826866314311));
#68964=CARTESIAN_POINT('Origin',(0.0167796527206399,-0.0326395659357401,
0.0680231969149709));
#68965=CARTESIAN_POINT('Origin',(0.0168634398053643,-0.0326395684527436,
0.0681425016757454));
#68966=CARTESIAN_POINT('Origin',(0.0168886406309284,-0.0326395674034263,
0.068180159390258));
#68967=CARTESIAN_POINT('Ctrl Pts',(0.00330962272071791,-0.0332451089994433,
0.0772967433283306));
#68968=CARTESIAN_POINT('Ctrl Pts',(0.00342830408707474,-0.0329451141710254,
0.0774783123234561));
#68969=CARTESIAN_POINT('Ctrl Pts',(0.00356032481116817,-0.0326442513127494,
0.0776504259345422));
#68970=CARTESIAN_POINT('Ctrl Pts',(0.00345092111710486,-0.0332451089994433,
0.0775029829054696));
#68971=CARTESIAN_POINT('Ctrl Pts',(0.00357738093637565,-0.0329451141710254,
0.0776792227443859));
#68972=CARTESIAN_POINT('Ctrl Pts',(0.0037167566017878,-0.0326442513127494,
0.0778454364339609));
#68973=CARTESIAN_POINT('Ctrl Pts',(0.00345233410106873,-0.0332451089994433,
0.0775050453012409));
#68974=CARTESIAN_POINT('Ctrl Pts',(0.00357887170486866,-0.0329451141710254,
0.0776812318485952));
#68975=CARTESIAN_POINT('Ctrl Pts',(0.00371832091969399,-0.0326442513127494,
0.077847386538955));
#68976=CARTESIAN_POINT('',(0.00347206196219953,-0.0331951640388616,0.0775322513054701));
#68977=CARTESIAN_POINT('',(0.00361494791491237,-0.0328677532355012,0.0777205095604965));
#68978=CARTESIAN_POINT('Origin',(0.0165649917248435,-0.0326402808281325,
0.0670628942239344));
#68979=CARTESIAN_POINT('Origin',(-0.00505225171976446,-0.0326944278779135,
0.0845844758664123));
#68980=CARTESIAN_POINT('',(0.003538411509985,-0.0326943950436593,0.0776216711679468));
#68981=CARTESIAN_POINT('',(0.00357721222903344,-0.0326943950436694,0.0776706686597508));
#68982=CARTESIAN_POINT('',(0.00339965091615746,-0.0330220786163545,0.0774303519137639));
#68983=CARTESIAN_POINT('Origin',(0.0168874600041524,-0.0326396682766063,
0.0674194988430164));
#68984=CARTESIAN_POINT('',(0.003400766808764,-0.0331951640388587,0.0774295770579827));
#68985=CARTESIAN_POINT('Origin',(-0.00566056714797226,-0.0331952026560148,
0.0837216034790517));
#68986=CARTESIAN_POINT('',(0.00343641438549177,-0.0331951640388701,0.0774809141817364));
#68987=CARTESIAN_POINT('Ctrl Pts',(0.00306506843675485,-0.0330240426238172,
0.0773763625232311));
#68988=CARTESIAN_POINT('Ctrl Pts',(0.00310951472380506,-0.032914277406352,
0.0774460512336908));
#68989=CARTESIAN_POINT('Ctrl Pts',(0.00315542382926138,-0.0328043479726691,
0.0775148558576064));
#68990=CARTESIAN_POINT('Ctrl Pts',(0.00320273936760645,-0.0326943950436593,
0.0775826866314311));
#68991=CARTESIAN_POINT('Ctrl Pts',(0.00317699409129416,-0.0330240426238172,
0.0773940764680345));
#68992=CARTESIAN_POINT('Ctrl Pts',(0.0032216844051919,-0.032914277406352,
0.0774622232935591));
#68993=CARTESIAN_POINT('Ctrl Pts',(0.00326780578408337,-0.0328043479726691,
0.077529480219137));
#68994=CARTESIAN_POINT('Ctrl Pts',(0.00331530151590948,-0.0326943950436593,
0.0775957594564494));
#68995=CARTESIAN_POINT('Ctrl Pts',(0.00328891974583347,-0.0330240426238172,
0.0774117904128379));
#68996=CARTESIAN_POINT('Ctrl Pts',(0.00333385408657873,-0.032914277406352,
0.0774783953534273));
#68997=CARTESIAN_POINT('Ctrl Pts',(0.00338018773890536,-0.0328043479726691,
0.0775441045806676));
#68998=CARTESIAN_POINT('Ctrl Pts',(0.00342786366421251,-0.0326943950436593,
0.0776088322814676));
#68999=CARTESIAN_POINT('Ctrl Pts',(0.00340084540037278,-0.0330240426238172,
0.0774295043576413));
#69000=CARTESIAN_POINT('Ctrl Pts',(0.00344602376796557,-0.032914277406352,
0.0774945674132956));
#69001=CARTESIAN_POINT('Ctrl Pts',(0.00349256969372735,-0.0328043479726691,
0.0775587289421982));
#69002=CARTESIAN_POINT('Ctrl Pts',(0.00354042581251554,-0.0326943950436593,
0.0776219051064858));
#69003=CARTESIAN_POINT('',(0.00337057543880573,-0.0326943950436693,0.077602178899699));
#69004=CARTESIAN_POINT('Ctrl Pts',(0.00319541831790758,-0.0327114338383316,
0.077572167361994));
#69005=CARTESIAN_POINT('Ctrl Pts',(0.00323069413955649,-0.0327619876831115,
0.0775476724649914));
#69006=CARTESIAN_POINT('Ctrl Pts',(0.00326534762077641,-0.0328131562604638,
0.0775236097100055));
#69007=CARTESIAN_POINT('Ctrl Pts',(0.00333343906285031,-0.0329167375858765,
0.0774763282355452));
#69008=CARTESIAN_POINT('Ctrl Pts',(0.00336684989259642,-0.0329691088920617,
0.0774531283554249));
#69009=CARTESIAN_POINT('Ctrl Pts',(0.00339965091619805,-0.0330220786163187,
0.0774303519137392));
#69010=CARTESIAN_POINT('Ctrl Pts',(0.00347242195593373,-0.0331951640388604,
0.077530255457707));
#69011=CARTESIAN_POINT('Ctrl Pts',(0.00354230657030366,-0.0330306422010619,
0.0776264193484358));
#69012=CARTESIAN_POINT('Ctrl Pts',(0.0036161060234924,-0.0328657861914644,
0.0777196126631896));
#69013=CARTESIAN_POINT('Ctrl Pts',(0.00347206196219772,-0.0331951640388604,
0.0775322513054674));
#69014=CARTESIAN_POINT('Ctrl Pts',(0.00354198783944048,-0.0330306422010619,
0.077628422638836));
#69015=CARTESIAN_POINT('Ctrl Pts',(0.00361582882785534,-0.0328657861914644,
0.0777216216844319));
#69016=CARTESIAN_POINT('Ctrl Pts',(0.00341207732454699,-0.0331951640388604,
0.0778648132162551));
#69017=CARTESIAN_POINT('Ctrl Pts',(0.00348887870607642,-0.0330306422010619,
0.0779622246935485));
#69018=CARTESIAN_POINT('Ctrl Pts',(0.0035696405801603,-0.0328657861914644,
0.0780563786515523));
#69019=CARTESIAN_POINT('',(0.00342002298075961,-0.0331781648281916,0.0778748690269726));
#69020=CARTESIAN_POINT('',(0.00341207732454947,-0.0331951640388588,0.0778648132162463));
#69021=CARTESIAN_POINT('Origin',(0.0159186204347069,-0.0326412091816574,
0.0670687808657489));
#69022=CARTESIAN_POINT('Ctrl Pts',(0.00342002298065486,-0.033178164828644,
0.0778748690251295));
#69023=CARTESIAN_POINT('Ctrl Pts',(0.00345371992274879,-0.0331276811546788,
0.077848184672704));
#69024=CARTESIAN_POINT('Ctrl Pts',(0.00348680838142885,-0.0330765663497807,
0.0778219821305349));
#69025=CARTESIAN_POINT('Ctrl Pts',(0.00355179686141659,-0.0329730614463279,
0.0777705182812483));
#69026=CARTESIAN_POINT('Ctrl Pts',(0.0035836706321198,-0.0329207133374049,
0.0777452777686087));
#69027=CARTESIAN_POINT('Ctrl Pts',(0.0036149478994017,-0.0328677532289369,
0.0777205095549454));
#69028=CARTESIAN_POINT('',(0.0034420696433845,-0.0331951640388701,0.0776985322608681));
#69029=CARTESIAN_POINT('Origin',(0.00812378219310841,-0.0315241814719618,
0.07415));
#69030=CARTESIAN_POINT('',(0.00342002298237634,-0.0332121607144211,0.0778748690265169));
#69031=CARTESIAN_POINT('',(0.00342799009848604,-0.0331951640388587,0.077884907844126));
#69032=CARTESIAN_POINT('Origin',(0.0158847466979892,-0.0326413640993599,
0.0670386330042486));
#69033=CARTESIAN_POINT('Origin',(0.016802988518155,-0.0326412103775044,
0.0681855539297036));
#69034=CARTESIAN_POINT('Origin',(0.0168245650622733,-0.0326413655647481,
0.0682254393833421));
#69035=CARTESIAN_POINT('Ctrl Pts',(0.00351669554321774,-0.0337436976235975,
0.0775928008365862));
#69036=CARTESIAN_POINT('Ctrl Pts',(0.00354766061571275,-0.0336723290703325,
0.0776342376721385));
#69037=CARTESIAN_POINT('Ctrl Pts',(0.00357936599685407,-0.033601104548885,
0.0776751108401327));
#69038=CARTESIAN_POINT('Ctrl Pts',(0.00368059499835616,-0.0333736987606857,
0.0778056107690198));
#69039=CARTESIAN_POINT('Ctrl Pts',(0.00378914602084772,-0.0331450831799191,
0.0779300865405608));
#69040=CARTESIAN_POINT('Ctrl Pts',(0.00367066429629554,-0.0337436976235975,
0.0777897618049929));
#69041=CARTESIAN_POINT('Ctrl Pts',(0.00370340086559064,-0.0336723290703325,
0.0778298138222454));
#69042=CARTESIAN_POINT('Ctrl Pts',(0.00373685254842926,-0.033601104548885,
0.0778692705323269));
#69043=CARTESIAN_POINT('Ctrl Pts',(0.00384365714532796,-0.0333736987606857,
0.0779952479916836));
#69044=CARTESIAN_POINT('Ctrl Pts',(0.00395751504969802,-0.0331450831799191,
0.0781148887865536));
#69045=CARTESIAN_POINT('Ctrl Pts',(0.00367220398382631,-0.0337436976235975,
0.077791731414677));
#69046=CARTESIAN_POINT('Ctrl Pts',(0.00370495826808942,-0.0336723290703325,
0.0778317695837464));
#69047=CARTESIAN_POINT('Ctrl Pts',(0.00373842741394501,-0.033601104548885,
0.0778712121292489));
#69048=CARTESIAN_POINT('Ctrl Pts',(0.00384528776679768,-0.0333736987606857,
0.0779971443639103));
#69049=CARTESIAN_POINT('Ctrl Pts',(0.00395919873998652,-0.0331450831799191,
0.0781167368090136));
#69050=CARTESIAN_POINT('',(0.00369361438614891,-0.0336938721132548,0.0778176611351351));
#69051=CARTESIAN_POINT('',(0.00384803921977251,-0.0333679869945434,0.0779965760132826));
#69052=CARTESIAN_POINT('Ctrl Pts',(0.00369361438615697,-0.0336938721132648,
0.0778176611351466));
#69053=CARTESIAN_POINT('Ctrl Pts',(0.0037079309880983,-0.0336629187933931,
0.0778349541583256));
#69054=CARTESIAN_POINT('Ctrl Pts',(0.00372234426885285,-0.0336319952301039,
0.0778521578213233));
#69055=CARTESIAN_POINT('Ctrl Pts',(0.00373685254843802,-0.0336011045488949,
0.0778692705323379));
#69056=CARTESIAN_POINT('Ctrl Pts',(0.0037732587863711,-0.0335235892595452,
0.077912212179914));
#69057=CARTESIAN_POINT('Ctrl Pts',(0.00381032801695305,-0.0334458668660367,
0.077954657327859));
#69058=CARTESIAN_POINT('Ctrl Pts',(0.00384803921953166,-0.0333679869945384,
0.0779965760134899));
#69059=CARTESIAN_POINT('Ctrl Pts',(0.00384806845073468,-0.0333679692460368,
0.077996609533711));
#69060=CARTESIAN_POINT('Ctrl Pts',(0.00384840141990203,-0.0333391895371364,
0.0779963020123921));
#69061=CARTESIAN_POINT('Ctrl Pts',(0.0038486487933833,-0.0333104081053817,
0.0779960691246925));
#69062=CARTESIAN_POINT('Ctrl Pts',(0.00384897243894554,-0.0332532696655993,
0.0779957568246079));
#69063=CARTESIAN_POINT('Ctrl Pts',(0.00384905120287359,-0.0332249163443174,
0.0779956751698193));
#69064=CARTESIAN_POINT('Ctrl Pts',(0.00384904932046599,-0.0331960985684305,
0.0779956675896123));
#69065=CARTESIAN_POINT('Ctrl Pts',(0.00384904926756352,-0.0331956312238387,
0.07799566748631));
#69066=CARTESIAN_POINT('Ctrl Pts',(0.0038490491931661,-0.03319516403886,
0.077995667403612));
#69067=CARTESIAN_POINT('',(0.00376544772787017,-0.0331951640388587,0.0779027384253525));
#69068=CARTESIAN_POINT('',(0.00380724846052808,-0.0331951640388687,0.0779492029144923));
#69069=CARTESIAN_POINT('',(0.00361494791122898,-0.0335216366567698,0.0777205095454249));
#69070=CARTESIAN_POINT('Origin',(0.0158850278782498,-0.032643457152887,
0.0664592572789629));
#69071=CARTESIAN_POINT('',(0.00361601294806183,-0.0336938721132325,0.0777196661515348));
#69072=CARTESIAN_POINT('Origin',(-0.00494527546920406,-0.0336938867896149,
0.0844992804885138));
#69073=CARTESIAN_POINT('',(0.00365481366711538,-0.0336938721132536,0.0777686636433449));
#69074=CARTESIAN_POINT('Ctrl Pts',(0.00327763619847352,-0.0335235895815172,
0.0776876360749402));
#69075=CARTESIAN_POINT('Ctrl Pts',(0.00332633872400957,-0.0334144449262749,
0.0777543528157398));
#69076=CARTESIAN_POINT('Ctrl Pts',(0.00337647552050197,-0.0333049234473147,
0.0778201400484667));
#69077=CARTESIAN_POINT('Ctrl Pts',(0.00342799009848586,-0.0331951640388587,
0.0778849078441259));
#69078=CARTESIAN_POINT('Ctrl Pts',(0.00339045342314712,-0.0335235895815172,
0.0776982871923899));
#69079=CARTESIAN_POINT('Ctrl Pts',(0.00343930258228498,-0.0334144449262749,
0.0777634507819752));
#69080=CARTESIAN_POINT('Ctrl Pts',(0.00348955409390823,-0.0333049234473147,
0.0778276800497654));
#69081=CARTESIAN_POINT('Ctrl Pts',(0.00354115114140821,-0.0331951640388587,
0.0778908870456369));
#69082=CARTESIAN_POINT('Ctrl Pts',(0.00350327064782071,-0.0335235895815172,
0.0777089383098397));
#69083=CARTESIAN_POINT('Ctrl Pts',(0.00355226644056039,-0.0334144449262749,
0.0777725487482107));
#69084=CARTESIAN_POINT('Ctrl Pts',(0.00360263266731449,-0.0333049234473147,
0.0778352200510641));
#69085=CARTESIAN_POINT('Ctrl Pts',(0.00365431218433055,-0.0331951640388587,
0.0778968662471479));
#69086=CARTESIAN_POINT('Ctrl Pts',(0.00361608787249431,-0.0335235895815172,
0.0777195894272895));
#69087=CARTESIAN_POINT('Ctrl Pts',(0.0036652302988358,-0.0334144449262749,
0.0777816467144461));
#69088=CARTESIAN_POINT('Ctrl Pts',(0.00371571124072075,-0.0333049234473147,
0.0778427600523629));
#69089=CARTESIAN_POINT('Ctrl Pts',(0.00376747322725289,-0.0331951640388587,
0.0779028454486589));
#69090=CARTESIAN_POINT('',(0.0035967189131881,-0.0331951640388687,0.0778938231347492));
#69091=CARTESIAN_POINT('Ctrl Pts',(0.00342002298482788,-0.033212160714597,
0.0778748690245668));
#69092=CARTESIAN_POINT('Ctrl Pts',(0.00345366324756589,-0.0332625444109904,
0.0778482295715033));
#69093=CARTESIAN_POINT('Ctrl Pts',(0.00348672383578633,-0.0333135300747143,
0.0778220491580205));
#69094=CARTESIAN_POINT('Ctrl Pts',(0.00355171190622051,-0.033416720314059,
0.0777705856285736));
#69095=CARTESIAN_POINT('Ctrl Pts',(0.00358361421804985,-0.0334688847587291,
0.0777453224448341));
#69096=CARTESIAN_POINT('Ctrl Pts',(0.003614947911878,-0.0335216366562357,
0.0777205095451091));
#69097=CARTESIAN_POINT('Ctrl Pts',(0.00369372973300097,-0.033693872113239,
0.0778166679533916));
#69098=CARTESIAN_POINT('Ctrl Pts',(0.00371519195726162,-0.0336474569764958,
0.0778425985204879));
#69099=CARTESIAN_POINT('Ctrl Pts',(0.00373695626094463,-0.033601104548885,
0.077868276068372));
#69100=CARTESIAN_POINT('Ctrl Pts',(0.00379205847394283,-0.0334837508592656,
0.0779332857159763));
#69101=CARTESIAN_POINT('Ctrl Pts',(0.00384906286075581,-0.0333660264659097,
0.0779966340233174));
#69102=CARTESIAN_POINT('Ctrl Pts',(0.00369361438613585,-0.033693872113239,
0.0778176611351193));
#69103=CARTESIAN_POINT('Ctrl Pts',(0.00371508242381872,-0.0336474569764958,
0.0778435923773791));
#69104=CARTESIAN_POINT('Ctrl Pts',(0.00373685254842926,-0.033601104548885,
0.077869270532327));
#69105=CARTESIAN_POINT('Ctrl Pts',(0.00379196949867764,-0.0334837508592656,
0.0779342817168771));
#69106=CARTESIAN_POINT('Ctrl Pts',(0.00384898866181219,-0.0333660264659097,
0.077997631123794));
#69107=CARTESIAN_POINT('Ctrl Pts',(0.00365439594239875,-0.033693872113239,
0.0781553473103698));
#69108=CARTESIAN_POINT('Ctrl Pts',(0.00367784056932152,-0.0336474569764958,
0.0781815081111948));
#69109=CARTESIAN_POINT('Ctrl Pts',(0.00370158983500764,-0.033601104548885,
0.0782073926705059));
#69110=CARTESIAN_POINT('Ctrl Pts',(0.00376171751542633,-0.0334837508592656,
0.0782729264234479));
#69111=CARTESIAN_POINT('Ctrl Pts',(0.0038237606931727,-0.0333660264659097,
0.0783366496909593));
#69112=CARTESIAN_POINT('',(0.00366319123664695,-0.0336769361243753,0.078162870334204));
#69113=CARTESIAN_POINT('',(0.00365462984962344,-0.0336938721132327,0.078153333277498));
#69114=CARTESIAN_POINT('Ctrl Pts',(0.00366319123664715,-0.033676936124375,
0.0781628703342042));
#69115=CARTESIAN_POINT('Ctrl Pts',(0.00366176253420729,-0.0336797586670149,
0.0781612822297672));
#69116=CARTESIAN_POINT('Ctrl Pts',(0.00366033473392105,-0.0336825812713094,
0.0781596934224022));
#69117=CARTESIAN_POINT('Ctrl Pts',(0.00365748094242724,-0.0336882265929357,
0.0781565144079007));
#69118=CARTESIAN_POINT('Ctrl Pts',(0.00365605495119278,-0.0336910493102957,
0.0781549242007668));
#69119=CARTESIAN_POINT('Ctrl Pts',(0.00365462984962063,-0.033693872113236,
0.0781533332775063));
#69120=CARTESIAN_POINT('Ctrl Pts',(0.00366319123664697,-0.0336769361243754,
0.0781628703342039));
#69121=CARTESIAN_POINT('Ctrl Pts',(0.00369435055763764,-0.0336279018505218,
0.0781348385518554));
#69122=CARTESIAN_POINT('Ctrl Pts',(0.00372595814487436,-0.0335767826010767,
0.0781064034968595));
#69123=CARTESIAN_POINT('Ctrl Pts',(0.00378789085622976,-0.0334733172064618,
0.0780506871259704));
#69124=CARTESIAN_POINT('Ctrl Pts',(0.00381825760411366,-0.033420963145624,
0.0780233683641929));
#69125=CARTESIAN_POINT('Ctrl Pts',(0.00384803921488857,-0.0333679869844681,
0.077996576007855));
#69126=CARTESIAN_POINT('',(0.00367412211789618,-0.0336938721132538,0.0779854972063266));
#69127=CARTESIAN_POINT('Origin',(0.00812378219310841,-0.0315241814719618,
0.07415));
#69128=CARTESIAN_POINT('',(0.00366319123761458,-0.0337108120655385,0.0781628703333429));
#69129=CARTESIAN_POINT('',(0.00367177297545981,-0.0336938721132327,0.0781723890818771));
#69130=CARTESIAN_POINT('Origin',(0.0165741070031077,-0.0345562509814765,
0.068051159813424));
#69131=CARTESIAN_POINT('Ctrl Pts',(0.00367177297546312,-0.0336938721132315,
0.0781723890818763));
#69132=CARTESIAN_POINT('Ctrl Pts',(0.00367034109970152,-0.0336910493285698,
0.0781708042714665));
#69133=CARTESIAN_POINT('Ctrl Pts',(0.00366891001591097,-0.0336882266020728,
0.0781692186364285));
#69134=CARTESIAN_POINT('Ctrl Pts',(0.00366604943561649,-0.0336825812713202,
0.0781660457200292));
#69135=CARTESIAN_POINT('Ctrl Pts',(0.00366461993908932,-0.0336797586670204,
0.0781644584386437));
#69136=CARTESIAN_POINT('Ctrl Pts',(0.00366319123664674,-0.033676936124375,
0.0781628703342038));
#69137=CARTESIAN_POINT('Origin',(0.015079169887541,-0.0345562514173524,
0.06638943663483));
#69138=CARTESIAN_POINT('Ctrl Pts',(0.0037419283827865,-0.034243627687391,
0.0778752492782319));
#69139=CARTESIAN_POINT('Ctrl Pts',(0.00388242847548842,-0.033943005420181,
0.0780405136191053));
#69140=CARTESIAN_POINT('Ctrl Pts',(0.0040349778094604,-0.0336441434784053,
0.0781947254186484));
#69141=CARTESIAN_POINT('Ctrl Pts',(0.00390795891713605,-0.034243627687391,
0.078062155301847));
#69142=CARTESIAN_POINT('Ctrl Pts',(0.00405550828672741,-0.033943005420181,
0.078221157697888));
#69143=CARTESIAN_POINT('Ctrl Pts',(0.0042146151959899,-0.0336441434784053,
0.0783685943617086));
#69144=CARTESIAN_POINT('Ctrl Pts',(0.00390961922247955,-0.034243627687391,
0.0780640243620831));
#69145=CARTESIAN_POINT('Ctrl Pts',(0.0040572390848398,-0.033943005420181,
0.0782229641386759));
#69146=CARTESIAN_POINT('Ctrl Pts',(0.00421641156985519,-0.0336441434784053,
0.0783703330511392));
#69147=CARTESIAN_POINT('',(0.00393265065846204,-0.0341934961088741,0.0780885963818718));
#69148=CARTESIAN_POINT('',(0.00409800492354329,-0.0338664212864431,0.0782574617933473));
#69149=CARTESIAN_POINT('Origin',(0.0164709577679441,-0.0345610720405665,
0.0670050951932994));
#69150=CARTESIAN_POINT('Origin',(-0.00357801441268596,-0.0336938005072879,
0.0860892848005765));
#69151=CARTESIAN_POINT('',(0.004009684300756,-0.0336938721132327,0.0781689953386565));
#69152=CARTESIAN_POINT('',(0.00405432007862871,-0.0336938721132427,0.0782127434510211));
#69153=CARTESIAN_POINT('',(0.00384803921488506,-0.0340203938281605,0.0779965760078509));
#69154=CARTESIAN_POINT('Origin',(0.0167302578751519,-0.0345589643243195,
0.0674104347896106));
#69155=CARTESIAN_POINT('',(0.00384904919316617,-0.034193496108874,0.0779956674036122));
#69156=CARTESIAN_POINT('Origin',(-0.00434315919637213,-0.0341934220717669,
0.0853656022723086));
#69157=CARTESIAN_POINT('',(0.0038908499258241,-0.0341934961088841,0.0780421318927521));
#69158=CARTESIAN_POINT('Ctrl Pts',(0.00350932721877318,-0.0340223579322397,
0.077984945278602));
#69159=CARTESIAN_POINT('Ctrl Pts',(0.00356222111612229,-0.0339125849573575,
0.0780485906477019));
#69160=CARTESIAN_POINT('Ctrl Pts',(0.0036163951567911,-0.0338030433565231,
0.0781110965131711));
#69161=CARTESIAN_POINT('Ctrl Pts',(0.0036717729754591,-0.0336938721132327,
0.0781723890818771));
#69162=CARTESIAN_POINT('Ctrl Pts',(0.0036225906443956,-0.0340223579322397,
0.0779884915790218));
#69163=CARTESIAN_POINT('Ctrl Pts',(0.00367553345447663,-0.0339125849573575,
0.0780505747500789));
#69164=CARTESIAN_POINT('Ctrl Pts',(0.00372972403963752,-0.0338030433565231,
0.078111518502864));
#69165=CARTESIAN_POINT('Ctrl Pts',(0.00378508619048596,-0.0336938721132327,
0.0781712510437988));
#69166=CARTESIAN_POINT('Ctrl Pts',(0.00373585407001801,-0.0340223579322397,
0.0779920378794416));
#69167=CARTESIAN_POINT('Ctrl Pts',(0.00378884579283097,-0.0339125849573575,
0.0780525588524559));
#69168=CARTESIAN_POINT('Ctrl Pts',(0.00384305292248394,-0.0338030433565231,
0.0781119404925568));
#69169=CARTESIAN_POINT('Ctrl Pts',(0.00389839940551282,-0.0336938721132327,
0.0781701130057204));
#69170=CARTESIAN_POINT('Ctrl Pts',(0.00384911749564042,-0.0340223579322397,
0.0779955841798613));
#69171=CARTESIAN_POINT('Ctrl Pts',(0.00390215813118531,-0.0339125849573575,
0.078054542954833));
#69172=CARTESIAN_POINT('Ctrl Pts',(0.00395638180533036,-0.0338030433565231,
0.0781123624822497));
#69173=CARTESIAN_POINT('Ctrl Pts',(0.00401171262053968,-0.0336938721132327,
0.078168974967642));
#69174=CARTESIAN_POINT('',(0.00384072863811791,-0.0336938721132427,0.0781706922102768));
#69175=CARTESIAN_POINT('Ctrl Pts',(0.00366319124028913,-0.0337108120662679,
0.0781628703309272));
#69176=CARTESIAN_POINT('Ctrl Pts',(0.00369515825582565,-0.0337611408994407,
0.0781341119243458));
#69177=CARTESIAN_POINT('Ctrl Pts',(0.00372654194424991,-0.0338121088781551,
0.0781058782948817));
#69178=CARTESIAN_POINT('Ctrl Pts',(0.00378817125688635,-0.0339153382773233,
0.0780504348698266));
#69179=CARTESIAN_POINT('Ctrl Pts',(0.00381839080814706,-0.0339675558473107,
0.07802324853018));
#69180=CARTESIAN_POINT('Ctrl Pts',(0.00384803921491822,-0.0340203938281304,
0.0779965760078282));
#69181=CARTESIAN_POINT('Ctrl Pts',(0.003932757672405,-0.0341934961088741,
0.0780865710596998));
#69182=CARTESIAN_POINT('Ctrl Pts',(0.00401414317778697,-0.0340287516182428,
0.0781732171899265));
#69183=CARTESIAN_POINT('Ctrl Pts',(0.00409904029110814,-0.0338644633275951,
0.0782564255580111));
#69184=CARTESIAN_POINT('Ctrl Pts',(0.00393265065846206,-0.0341934961088741,
0.0780885963818717));
#69185=CARTESIAN_POINT('Ctrl Pts',(0.00401407803578436,-0.0340287516182428,
0.0781752447245274));
#69186=CARTESIAN_POINT('Ctrl Pts',(0.00409901707670845,-0.033864463327595,
0.0782584535725514));
#69187=CARTESIAN_POINT('Ctrl Pts',(0.00391482007723506,-0.0341934961088741,
0.0784260540112638));
#69188=CARTESIAN_POINT('Ctrl Pts',(0.00400322412519192,-0.0340287516182428,
0.0785130709871392));
#69189=CARTESIAN_POINT('Ctrl Pts',(0.00409514911120959,-0.033864463327595,
0.0785963598023026));
#69190=CARTESIAN_POINT('',(0.00392396340701163,-0.0341764758832409,0.0784350346736767));
#69191=CARTESIAN_POINT('',(0.00391482007723565,-0.034193496108874,0.0784260540112524));
#69192=CARTESIAN_POINT('Origin',(0.0158796153722629,-0.0345621027314363,
0.066968399723049));
#69193=CARTESIAN_POINT('Ctrl Pts',(0.00392396340646852,-0.0341764758837506,
0.0784350346719325));
#69194=CARTESIAN_POINT('Ctrl Pts',(0.00395400916461337,-0.0341260050040629,
0.0784043792545373));
#69195=CARTESIAN_POINT('Ctrl Pts',(0.00398353262931382,-0.0340749269148536,
0.0783742566738718));
#69196=CARTESIAN_POINT('Ctrl Pts',(0.00404155798382064,-0.0339715436306741,
0.07831505396907));
#69197=CARTESIAN_POINT('Ctrl Pts',(0.00407003786434501,-0.0339192778238253,
0.0782859963093393));
#69198=CARTESIAN_POINT('Ctrl Pts',(0.00409800492169441,-0.033866421285696,
0.0782574617929191));
#69199=CARTESIAN_POINT('',(0.00392373536785884,-0.0341934961088841,0.0782573251965721));
#69200=CARTESIAN_POINT('Origin',(0.00812378219310841,-0.0315241814719618,
0.07415));
#69201=CARTESIAN_POINT('',(0.00392396340812783,-0.0342105180190355,0.0784350346737397));
#69202=CARTESIAN_POINT('',(0.00393312589888613,-0.0341934961088739,0.0784439957875769));
#69203=CARTESIAN_POINT('Origin',(0.0158511247668744,-0.0345621700984072,
0.0669331443589828));
#69204=CARTESIAN_POINT('Origin',(0.015148162081767,-0.0345621041817851,
0.0662514884247236));
#69205=CARTESIAN_POINT('Origin',(0.015183977864322,-0.0345621713726151,
0.0662792703143448));
#69206=CARTESIAN_POINT('Ctrl Pts',(0.00400861303500967,-0.0346945769586966,
0.0781679453770228));
#69207=CARTESIAN_POINT('Ctrl Pts',(0.00409277050962898,-0.0345275153362944,
0.0782541392426631));
#69208=CARTESIAN_POINT('Ctrl Pts',(0.0041796604694202,-0.0343603235965185,
0.0783377087273367));
#69209=CARTESIAN_POINT('Ctrl Pts',(0.00426902225899016,-0.034193496108874,
0.0784184104890255));
#69210=CARTESIAN_POINT('Ctrl Pts',(0.00406848449422091,-0.0346945769586966,
0.0782266261808496));
#69211=CARTESIAN_POINT('Ctrl Pts',(0.00415387106177088,-0.0345275153362944,
0.0783115660148054));
#69212=CARTESIAN_POINT('Ctrl Pts',(0.00424195099425694,-0.0343603235965185,
0.0783938424895965));
#69213=CARTESIAN_POINT('Ctrl Pts',(0.00433246017371171,-0.034193496108874,
0.0784732161396614));
#69214=CARTESIAN_POINT('Ctrl Pts',(0.00412835595343221,-0.0346945769586966,
0.078285306984677));
#69215=CARTESIAN_POINT('Ctrl Pts',(0.00421497161391285,-0.0345275153362944,
0.0783689927869475));
#69216=CARTESIAN_POINT('Ctrl Pts',(0.00430424151909371,-0.0343603235965185,
0.0784499762518558));
#69217=CARTESIAN_POINT('Ctrl Pts',(0.00439589808843326,-0.034193496108874,
0.0785280217902974));
#69218=CARTESIAN_POINT('Ctrl Pts',(0.00418822741264338,-0.0346945769586966,
0.0783439877885032));
#69219=CARTESIAN_POINT('Ctrl Pts',(0.00427607216605468,-0.0345275153362944,
0.0784264195590902));
#69220=CARTESIAN_POINT('Ctrl Pts',(0.0043665320439304,-0.0343603235965185,
0.078506110014116));
#69221=CARTESIAN_POINT('Ctrl Pts',(0.00445933600315482,-0.034193496108874,
0.0785828274409331));
#69222=CARTESIAN_POINT('',(0.00418822741221091,-0.0346945769586966,0.078343987788079));
#69223=CARTESIAN_POINT('',(0.00436385853472848,-0.0343667727831489,0.0785021373006342));
#69224=CARTESIAN_POINT('Origin',(0.0155593803504305,-0.0345626457066645,
0.0659587494736872));
#69225=CARTESIAN_POINT('Origin',(-0.00286144870193541,-0.0341934771029068,
0.0868654853021026));
#69226=CARTESIAN_POINT('',(0.00427015733847042,-0.034193496108874,0.0784193911134631));
#69227=CARTESIAN_POINT('',(0.00431745200453473,-0.034193496108884,0.0784602501952396));
#69228=CARTESIAN_POINT('',(0.00409800492290952,-0.0345211942962664,0.078257461791745));
#69229=CARTESIAN_POINT('Origin',(0.015900435741368,-0.0345625596118997,
0.0662976772090484));
#69230=CARTESIAN_POINT('',(0.00409895585648141,-0.0346945769586885,0.0782564915633657));
#69231=CARTESIAN_POINT('Origin',(-0.00364520733230665,-0.0346945685853842,
0.0861577858689212));
#69232=CARTESIAN_POINT('',(0.00414359163435617,-0.0346945769587025,0.0783002396757324));
#69233=CARTESIAN_POINT('Ctrl Pts',(0.00375923165823636,-0.0345231616327841,
0.0782671226151987));
#69234=CARTESIAN_POINT('Ctrl Pts',(0.00381598039704188,-0.0344132092796987,
0.0783272817995263));
#69235=CARTESIAN_POINT('Ctrl Pts',(0.00387397055314826,-0.0343032738558979,
0.0783862640770171));
#69236=CARTESIAN_POINT('Ctrl Pts',(0.00393312589888613,-0.0341934961088739,
0.0784439957875769));
#69237=CARTESIAN_POINT('Ctrl Pts',(0.00387249406514685,-0.0345231616327841,
0.0782635500363809));
#69238=CARTESIAN_POINT('Ctrl Pts',(0.00392919356098316,-0.0344132092796987,
0.0783221480578899));
#69239=CARTESIAN_POINT('Ctrl Pts',(0.00398710218523956,-0.0343032738558979,
0.078379570271663));
#69240=CARTESIAN_POINT('Ctrl Pts',(0.00404614386589386,-0.0341934961088739,
0.0784357450135522));
#69241=CARTESIAN_POINT('Ctrl Pts',(0.00398575647205734,-0.0345231616327841,
0.0782599774575631));
#69242=CARTESIAN_POINT('Ctrl Pts',(0.00404240672492443,-0.0344132092796987,
0.0783170143162536));
#69243=CARTESIAN_POINT('Ctrl Pts',(0.00410023381733086,-0.0343032738558979,
0.0783728764663089));
#69244=CARTESIAN_POINT('Ctrl Pts',(0.00415916183290159,-0.0341934961088739,
0.0784274942395275));
#69245=CARTESIAN_POINT('Ctrl Pts',(0.00409901887896783,-0.0345231616327841,
0.0782564048787452));
#69246=CARTESIAN_POINT('Ctrl Pts',(0.00415561988886571,-0.0344132092796987,
0.0783118805746172));
#69247=CARTESIAN_POINT('Ctrl Pts',(0.00421336544942216,-0.0343032738558979,
0.0783661826609548));
#69248=CARTESIAN_POINT('Ctrl Pts',(0.00427217979990932,-0.0341934961088739,
0.0784192434655028));
#69249=CARTESIAN_POINT('',(0.00410164161868827,-0.0341934961088839,0.0784316934505299));
#69250=CARTESIAN_POINT('Ctrl Pts',(0.0039239634105423,-0.0342105180195383,
0.0784350346712663));
#69251=CARTESIAN_POINT('Ctrl Pts',(0.00395404295578628,-0.0342610556241312,
0.0784043448008363));
#69252=CARTESIAN_POINT('Ctrl Pts',(0.00398358273914332,-0.0343122189870182,
0.0783742056442631));
#69253=CARTESIAN_POINT('Ctrl Pts',(0.00404160867607172,-0.0344158119695139,
0.0783150023394436));
#69254=CARTESIAN_POINT('Ctrl Pts',(0.00407007109661467,-0.0344681990450033,
0.0782859624057777));
#69255=CARTESIAN_POINT('Ctrl Pts',(0.00409800492292408,-0.0345211942962448,
0.0782574617917192));
#69256=CARTESIAN_POINT('Ctrl Pts',(0.00418820704893545,-0.0346945769586932,
0.0783419602395123));
#69257=CARTESIAN_POINT('Ctrl Pts',(0.00427487286075145,-0.034529677707698,
0.0784233254708944));
#69258=CARTESIAN_POINT('Ctrl Pts',(0.00436482751749549,-0.034364806625142,
0.0785010391990618));
#69259=CARTESIAN_POINT('Ctrl Pts',(0.00418822741220435,-0.0346945769586932,
0.0783439877880727));
#69260=CARTESIAN_POINT('Ctrl Pts',(0.0042749351421522,-0.034529677707698,
0.0784253525984587));
#69261=CARTESIAN_POINT('Ctrl Pts',(0.00436493166380939,-0.034364806625142,
0.0785030641734747));
#69262=CARTESIAN_POINT('Ctrl Pts',(0.00419162115542487,-0.0346945769586932,
0.0786818991133777));
#69263=CARTESIAN_POINT('Ctrl Pts',(0.00428531496292501,-0.034529677707698,
0.0787631937605239));
#69264=CARTESIAN_POINT('Ctrl Pts',(0.00438228869270736,-0.034364806625142,
0.0788405464912489));
#69265=CARTESIAN_POINT('',(0.00420131034331547,-0.0346775396664996,0.0786902879403227));
#69266=CARTESIAN_POINT('',(0.00419162115542729,-0.0346945769586885,0.0786818991133677));
#69267=CARTESIAN_POINT('Origin',(0.0149385014674794,-0.0345626616892411,
0.0660283124331721));
#69268=CARTESIAN_POINT('Ctrl Pts',(0.0042013103427617,-0.0346775396670096,
0.0786902879385792));
#69269=CARTESIAN_POINT('Ctrl Pts',(0.00422939404452155,-0.0346269749928197,
0.0786577808423804));
#69270=CARTESIAN_POINT('Ctrl Pts',(0.0042569786090545,-0.034575790289081,
0.0786258514463341));
#69271=CARTESIAN_POINT('Ctrl Pts',(0.00431117231160473,-0.0344721681087947,
0.0785631218714823));
#69272=CARTESIAN_POINT('Ctrl Pts',(0.00433776020740688,-0.0344197714289613,
0.0785323462893058));
#69273=CARTESIAN_POINT('Ctrl Pts',(0.00436385853446865,-0.0343667727830683,
0.0785021373005513));
#69274=CARTESIAN_POINT('',(0.0041899242838291,-0.0346945769587026,0.0785129434507333));
#69275=CARTESIAN_POINT('Origin',(0.00812378219310841,-0.0315241814719618,
0.07415));
#69276=CARTESIAN_POINT('',(0.00420131034464479,-0.0347116136489782,0.0786902879399135));
#69277=CARTESIAN_POINT('',(0.0042110174281769,-0.0346945769586885,0.0786986560536431));
#69278=CARTESIAN_POINT('Origin',(0.014903020832005,-0.0345626676565481,
0.0660001258509192));
#69279=CARTESIAN_POINT('Origin',(0.0151696289895262,-0.0345626631767773,
0.0662279847007374));
#69280=CARTESIAN_POINT('Origin',(0.0152026653345296,-0.0345626691251745,
0.0662590006051623));
#69281=CARTESIAN_POINT('Ctrl Pts',(0.00424153578227314,-0.0352450361874068,
0.0783934567785217));
#69282=CARTESIAN_POINT('Ctrl Pts',(0.00440158038088488,-0.0349452760959493,
0.0785398781045686));
#69283=CARTESIAN_POINT('Ctrl Pts',(0.00457219936302422,-0.034644428984174,
0.0786738282490249));
#69284=CARTESIAN_POINT('Ctrl Pts',(0.0042434360883573,-0.0352450361874068,
0.078395119445592));
#69285=CARTESIAN_POINT('Ctrl Pts',(0.00440354339548659,-0.0349452760959493,
0.0785414691004188));
#69286=CARTESIAN_POINT('Ctrl Pts',(0.00457421950942565,-0.034644428984174,
0.0786753430538034));
#69287=CARTESIAN_POINT('Ctrl Pts',(0.00443158520560055,-0.0352450361874068,
0.0785597399475977));
#69288=CARTESIAN_POINT('Ctrl Pts',(0.00459790127684407,-0.0349452760959493,
0.0786989934420251));
#69289=CARTESIAN_POINT('Ctrl Pts',(0.00477423400461568,-0.034644428984174,
0.0788253237249377));
#69290=CARTESIAN_POINT('Ctrl Pts',(0.00443346669677299,-0.0352450361874068,
0.0785613861526177));
#69291=CARTESIAN_POINT('Ctrl Pts',(0.00459984485565765,-0.0349452760959493,
0.0787005686854411));
#69292=CARTESIAN_POINT('Ctrl Pts',(0.00477623414956757,-0.034644428984174,
0.078826823531649));
#69293=CARTESIAN_POINT('',(0.0044593095501685,-0.0351951634053279,0.0785828086527249));
#69294=CARTESIAN_POINT('',(0.00464455084721618,-0.0348678972925388,0.0787296369115643));
#69295=CARTESIAN_POINT('Origin',(0.0144408273820345,-0.0345636767886177,
0.0651375939594543));
#69296=CARTESIAN_POINT('Origin',(-0.00203994926337658,-0.0346946199340828,
0.0875282986026686));
#69297=CARTESIAN_POINT('',(0.0045458388589538,-0.0346945769330289,0.0786529375407269));
#69298=CARTESIAN_POINT('',(0.00459560576947358,-0.0346945769458128,0.0786907463453233));
#69299=CARTESIAN_POINT('',(0.00436385853457462,-0.0350221583435276,0.0785021373004535));
#69300=CARTESIAN_POINT('Origin',(0.0148473209008226,-0.0345628458719425,
0.0653943164018214));
#69301=CARTESIAN_POINT('',(0.00436466485333552,-0.0351951360298761,0.0785011993543997));
#69302=CARTESIAN_POINT('Origin',(-0.00283893782162353,-0.0351951838366924,
0.0868394217306688));
#69303=CARTESIAN_POINT('',(0.00445933600261231,-0.0351951371328748,0.078582827440618));
#69304=CARTESIAN_POINT('Ctrl Pts',(0.00402636107151413,-0.0350241211494343,
0.0785330514658565));
#69305=CARTESIAN_POINT('Ctrl Pts',(0.00408673580833524,-0.0349144232818962,
0.0785894917617984));
#69306=CARTESIAN_POINT('Ctrl Pts',(0.00414831334359367,-0.0348045283579412,
0.0786447178510264));
#69307=CARTESIAN_POINT('Ctrl Pts',(0.00421101743660167,-0.0346945769439157,
0.0786986560608902));
#69308=CARTESIAN_POINT('Ctrl Pts',(0.0041391756800295,-0.0350241211494343,
0.0785223741109151));
#69309=CARTESIAN_POINT('Ctrl Pts',(0.00419940334066417,-0.0349144232818962,
0.0785772604318805));
#69310=CARTESIAN_POINT('Ctrl Pts',(0.0042608015899308,-0.0348045283579412,
0.0786309346561729));
#69311=CARTESIAN_POINT('Ctrl Pts',(0.00432329434281574,-0.0346945769439157,
0.0786833251074294));
#69312=CARTESIAN_POINT('Ctrl Pts',(0.00425199028854486,-0.0350241211494343,
0.0785116967559738));
#69313=CARTESIAN_POINT('Ctrl Pts',(0.0043120708729931,-0.0349144232818962,
0.0785650291019626));
#69314=CARTESIAN_POINT('Ctrl Pts',(0.00437328983626794,-0.0348045283579412,
0.0786171514613195));
#69315=CARTESIAN_POINT('Ctrl Pts',(0.00443557124902981,-0.0346945769439157,
0.0786679941539687));
#69316=CARTESIAN_POINT('Ctrl Pts',(0.00436480489706022,-0.0350241211494343,
0.0785010194010324));
#69317=CARTESIAN_POINT('Ctrl Pts',(0.00442473840532203,-0.0349144232818962,
0.0785527977720447));
#69318=CARTESIAN_POINT('Ctrl Pts',(0.00448577808260507,-0.0348045283579412,
0.078603368266466));
#69319=CARTESIAN_POINT('Ctrl Pts',(0.00454784815524387,-0.0346945769439157,
0.0786526632005079));
#69320=CARTESIAN_POINT('',(0.00437842814328991,-0.0346945769458128,0.0786757967970733));
#69321=CARTESIAN_POINT('Ctrl Pts',(0.00420131034679082,-0.0347116136492788,
0.0786902879374189));
#69322=CARTESIAN_POINT('Ctrl Pts',(0.00422938290564181,-0.0347621546532281,
0.0786577937589219));
#69323=CARTESIAN_POINT('Ctrl Pts',(0.00425696187304804,-0.0348133084096997,
0.0786258709158915));
#69324=CARTESIAN_POINT('Ctrl Pts',(0.00431115564150317,-0.0349168561544567,
0.078563141258971));
#69325=CARTESIAN_POINT('Ctrl Pts',(0.0043377489466328,-0.0349692089015913,
0.0785323593267541));
#69326=CARTESIAN_POINT('Ctrl Pts',(0.00436385853461358,-0.0350221583435,
0.0785021373004389));
#69327=CARTESIAN_POINT('Ctrl Pts',(0.00445922947991934,-0.0351951371254893,
0.0785813683063454));
#69328=CARTESIAN_POINT('Ctrl Pts',(0.00455084523931787,-0.035030733898093,
0.0786571306344719));
#69329=CARTESIAN_POINT('Ctrl Pts',(0.00464551405235916,-0.0348659306897825,
0.0787290416459421));
#69330=CARTESIAN_POINT('Ctrl Pts',(0.00445933600268492,-0.0351951371254893,
0.0785828274405272));
#69331=CARTESIAN_POINT('Ctrl Pts',(0.00455098192876717,-0.035030733898093,
0.0786585875663624));
#69332=CARTESIAN_POINT('Ctrl Pts',(0.00464568079169184,-0.0348659306897825,
0.0787304951306015));
#69333=CARTESIAN_POINT('Ctrl Pts',(0.00447718932921445,-0.0351951371254893,
0.0788273798501157));
#69334=CARTESIAN_POINT('Ctrl Pts',(0.00457389122292753,-0.035030733898093,
0.0789027708696265));
#69335=CARTESIAN_POINT('Ctrl Pts',(0.00467362647762573,-0.0348659306897825,
0.0789741006743426));
#69336=CARTESIAN_POINT('Origin',(0.00142736582007893,-0.0308609197411502,
0.0829643479260305));
#69337=CARTESIAN_POINT('',(0.00446711965051264,-0.0351951371254893,0.0786894467771819));
#69338=CARTESIAN_POINT('Origin',(0.00859590893976371,-0.03518404674412,
0.0732945223648207));
#69339=CARTESIAN_POINT('Origin',(0.00153424433607435,-0.0352322612301065,
0.0841373491110821));
#69340=CARTESIAN_POINT('',(0.00483591447171173,-0.0351951142564667,0.0788688706731626));
#69341=CARTESIAN_POINT('',(0.00493972642941176,-0.0351951372916787,0.0789379315882405));
#69342=CARTESIAN_POINT('Origin',(0.00846414469139679,-0.0352875119101824,
0.0741619812508536));
#69343=CARTESIAN_POINT('Origin',(0.00278723044504516,-0.0298325076522633,
0.0688758739377672));
#69344=CARTESIAN_POINT('Origin',(0.00119730982211957,-0.0338734199020578,
0.0788688060512241));
#69345=CARTESIAN_POINT('Ctrl Pts',(0.00269001517329539,-0.0321934096636942,
0.0760347577350164));
#69346=CARTESIAN_POINT('Ctrl Pts',(0.00272375143924168,-0.0320508460843289,
0.0761320195771432));
#69347=CARTESIAN_POINT('Ctrl Pts',(0.00276007550171859,-0.0319086045661005,
0.0762283016566206));
#69348=CARTESIAN_POINT('Ctrl Pts',(0.00279889208139986,-0.0317669892864814,
0.0763234031000984));
#69349=CARTESIAN_POINT('Ctrl Pts',(0.0027192084103453,-0.0321934096636942,
0.0761133591824487));
#69350=CARTESIAN_POINT('Ctrl Pts',(0.00275435160477109,-0.0320508460843289,
0.076210098479534));
#69351=CARTESIAN_POINT('Ctrl Pts',(0.00279206749514457,-0.0319086045661005,
0.0763058206065784));
#69352=CARTESIAN_POINT('Ctrl Pts',(0.00283225790454788,-0.0317669892864814,
0.076400326142627));
#69353=CARTESIAN_POINT('Ctrl Pts',(0.00274840164739521,-0.0321934096636942,
0.076191960629881));
#69354=CARTESIAN_POINT('Ctrl Pts',(0.0027849517703005,-0.0320508460843289,
0.0762881773819247));
#69355=CARTESIAN_POINT('Ctrl Pts',(0.00282405948857053,-0.0319086045661005,
0.0763833395565361));
#69356=CARTESIAN_POINT('Ctrl Pts',(0.00286562372769592,-0.0317669892864814,
0.0764772491851556));
#69357=CARTESIAN_POINT('Ctrl Pts',(0.00277759488444513,-0.0321934096636942,
0.0762705620773133));
#69358=CARTESIAN_POINT('Ctrl Pts',(0.0028155519358299,-0.0320508460843289,
0.0763662562843156));
#69359=CARTESIAN_POINT('Ctrl Pts',(0.00285605148199651,-0.0319086045661005,
0.0764608585064939));
#69360=CARTESIAN_POINT('Ctrl Pts',(0.00289898955084395,-0.0317669892864814,
0.0765541722276842));
#69361=CARTESIAN_POINT('',(0.00277707261166756,-0.0321934096636942,0.0762691558818855));
#69362=CARTESIAN_POINT('',(0.0028686516159578,-0.031866561751129,0.0764870339334687));
#69363=CARTESIAN_POINT('Origin',(0.0185272918711739,-0.0326371944421996,
0.0706880719260468));
#69364=CARTESIAN_POINT('Origin',(-0.00714680149905182,-0.031693926150899,
0.0809410533642363));
#69365=CARTESIAN_POINT('',(0.00273241349331969,-0.0320197221621774,0.0761526813799176));
#69366=CARTESIAN_POINT('Ctrl Pts',(0.00273243154286703,-0.0320197392094698,
0.076152865469824));
#69367=CARTESIAN_POINT('Ctrl Pts',(0.00274262281028387,-0.0319792716575996,
0.0761802983788608));
#69368=CARTESIAN_POINT('Ctrl Pts',(0.00275306960968677,-0.0319386439829638,
0.076207778478822));
#69369=CARTESIAN_POINT('Ctrl Pts',(0.00276379081377242,-0.031897909938157,
0.0762353316132561));
#69370=CARTESIAN_POINT('Ctrl Pts',(0.00277451180594564,-0.0318571766984884,
0.0762628842030822));
#69371=CARTESIAN_POINT('Ctrl Pts',(0.00278545104045337,-0.0318163871833545,
0.0762903704303193));
#69372=CARTESIAN_POINT('Ctrl Pts',(0.00279656761926225,-0.0317755399638303,
0.07631769705572));
#69373=CARTESIAN_POINT('',(0.00273355137358275,-0.0321934096636182,0.0761519769509753));
#69374=CARTESIAN_POINT('Origin',(0.000577389415186222,-0.0324112132163665,
0.0769752261397524));
#69375=CARTESIAN_POINT('',(0.00275531199263515,-0.0321934096636662,0.0762105664164404));
#69376=CARTESIAN_POINT('Ctrl Pts',(0.00277791771285805,-0.0321934096636618,
0.0762673121109242));
#69377=CARTESIAN_POINT('Ctrl Pts',(0.00280711709700424,-0.0320835708272592,
0.07634103574843));
#69378=CARTESIAN_POINT('Ctrl Pts',(0.00283782525116754,-0.0319739230346489,
0.0764141123434925));
#69379=CARTESIAN_POINT('Ctrl Pts',(0.00286999571080509,-0.0318646057455573,
0.0764864514149958));
#69380=CARTESIAN_POINT('Ctrl Pts',(0.00273070104777598,-0.0321934096636618,
0.0763703254659009));
#69381=CARTESIAN_POINT('Ctrl Pts',(0.00276132106637121,-0.0320835708272592,
0.0764447002580166));
#69382=CARTESIAN_POINT('Ctrl Pts',(0.00279346250656865,-0.0319739230346489,
0.0765183982300369));
#69383=CARTESIAN_POINT('Ctrl Pts',(0.0028270770090207,-0.0318646057455573,
0.0765913282465753));
#69384=CARTESIAN_POINT('Ctrl Pts',(0.00268348438269391,-0.0321934096636618,
0.0764733388208775));
#69385=CARTESIAN_POINT('Ctrl Pts',(0.00271552503573818,-0.0320835708272592,
0.0765483647676032));
#69386=CARTESIAN_POINT('Ctrl Pts',(0.00274909976196975,-0.0319739230346489,
0.0766226841165813));
#69387=CARTESIAN_POINT('Ctrl Pts',(0.0027841583072363,-0.0318646057455573,
0.0766962050781548));
#69388=CARTESIAN_POINT('Ctrl Pts',(0.00263626771761184,-0.0321934096636618,
0.0765763521758541));
#69389=CARTESIAN_POINT('Ctrl Pts',(0.00266972900510516,-0.0320835708272592,
0.0766520292771898));
#69390=CARTESIAN_POINT('Ctrl Pts',(0.00270473701737086,-0.0319739230346489,
0.0767269700031256));
#69391=CARTESIAN_POINT('Ctrl Pts',(0.0027412396054519,-0.0318646057455573,
0.0768010819097342));
#69392=CARTESIAN_POINT('',(0.0026414629696454,-0.0321763980308278,0.076588068069142));
#69393=CARTESIAN_POINT('',(0.00263626771762764,-0.0321934096636185,0.0765763521758782));
#69394=CARTESIAN_POINT('Origin',(0.0180003159370518,-0.032638623175221,
0.070429194154957));
#69395=CARTESIAN_POINT('Ctrl Pts',(0.00264146297253932,-0.0321763980306305,
0.0765880680678479));
#69396=CARTESIAN_POINT('Ctrl Pts',(0.00268067881820687,-0.032125959617565,
0.0765706282039456));
#69397=CARTESIAN_POINT('Ctrl Pts',(0.00271921519846222,-0.0320749164633059,
0.0765534905083077));
#69398=CARTESIAN_POINT('Ctrl Pts',(0.00279496004121797,-0.0319716057793932,
0.076519805661622));
#69399=CARTESIAN_POINT('Ctrl Pts',(0.00283213899080369,-0.031919378669013,
0.0765032716354018));
#69400=CARTESIAN_POINT('Ctrl Pts',(0.00286865161764783,-0.0318665617525314,
0.076487033932707));
#69401=CARTESIAN_POINT('',(0.0027066701646576,-0.0321934096636664,0.0764227540288918));
#69402=CARTESIAN_POINT('Origin',(0.00812378219310841,-0.0315241814719618,
0.07415));
#69403=CARTESIAN_POINT('',(0.00264146296930577,-0.032210423332377,0.0765880680692927));
#69404=CARTESIAN_POINT('',(0.00264668323176904,-0.0321934096636183,0.0765997728400262));
#69405=CARTESIAN_POINT('Origin',(0.0179878480322056,-0.0326387226476407,
0.0703856066204022));
#69406=CARTESIAN_POINT('Origin',(0.0175017309251695,-0.0326386247673746,
0.0693080517117185));
#69407=CARTESIAN_POINT('Origin',(0.0175257409011946,-0.0326387239810024,
0.0693465066926255));
#69408=CARTESIAN_POINT('Ctrl Pts',(0.00280523889076349,-0.0327445246967095,
0.0763388860502735));
#69409=CARTESIAN_POINT('Ctrl Pts',(0.00288779407774399,-0.0324436878339359,
0.0765394781901585));
#69410=CARTESIAN_POINT('Ctrl Pts',(0.00298522415396361,-0.0321434074405927,
0.0767332820748691));
#69411=CARTESIAN_POINT('Ctrl Pts',(0.00290538749880782,-0.0327445246967095,
0.0765679499197658));
#69412=CARTESIAN_POINT('Ctrl Pts',(0.0029965819708594,-0.0324436878339359,
0.0767647648931502));
#69413=CARTESIAN_POINT('Ctrl Pts',(0.00310234227723534,-0.0321434074405927,
0.0769541515956304));
#69414=CARTESIAN_POINT('',(0.00292068602045132,-0.0326943950436612,0.0766006968841704));
#69415=CARTESIAN_POINT('',(0.00302576498972626,-0.0323666188837389,0.0768123947104103));
#69416=CARTESIAN_POINT('Origin',(0.0180965475217363,-0.0326395579112048,
0.0693687340856444));
#69417=CARTESIAN_POINT('Origin',(-0.006764200291473,-0.0321933825603,0.0819251191929099));
#69418=CARTESIAN_POINT('',(0.00296910472131925,-0.0321934096532689,0.0767009655345619));
#69419=CARTESIAN_POINT('',(0.00299803695950301,-0.0321934096584275,0.0767563656784212));
#69420=CARTESIAN_POINT('',(0.00286865161508525,-0.0325210109756238,0.0764870339338416));
#69421=CARTESIAN_POINT('Origin',(0.0182781848506571,-0.0326393129160331,
0.0698139220355885));
#69422=CARTESIAN_POINT('',(0.00286989293566145,-0.0326943950436593,0.0764864819003117));
#69423=CARTESIAN_POINT('Origin',(-0.00723809272765096,-0.0326943765538153,
0.0809816506985317));
#69424=CARTESIAN_POINT('',(0.00289528947806638,-0.0326943950436702,0.076543589392251));
#69425=CARTESIAN_POINT('Ctrl Pts',(0.00255011175848464,-0.0325229783203769,
0.0763713054464067));
#69426=CARTESIAN_POINT('Ctrl Pts',(0.00258073240548661,-0.0324130253092449,
0.0764481383714599));
#69427=CARTESIAN_POINT('Ctrl Pts',(0.00261293779602111,-0.0323031222208069,
0.0765243262158763));
#69428=CARTESIAN_POINT('Ctrl Pts',(0.00264668323359993,-0.0321934096576657,
0.0765997728441197));
#69429=CARTESIAN_POINT('Ctrl Pts',(0.00265673565951443,-0.0325229783203769,
0.0764096784312474));
#69430=CARTESIAN_POINT('Ctrl Pts',(0.00268788527727328,-0.0324130253092449,
0.0764850415481566));
#69431=CARTESIAN_POINT('Ctrl Pts',(0.0027205891534663,-0.0323031222208069,
0.0765597488649146));
#69432=CARTESIAN_POINT('Ctrl Pts',(0.00275480202000012,-0.0321934096576657,
0.0766337061649673));
#69433=CARTESIAN_POINT('Ctrl Pts',(0.00276335956054423,-0.0325229783203769,
0.076448051416088));
#69434=CARTESIAN_POINT('Ctrl Pts',(0.00279503814905994,-0.0324130253092449,
0.0765219447248533));
#69435=CARTESIAN_POINT('Ctrl Pts',(0.0028282405109115,-0.0323031222208069,
0.0765951715139529));
#69436=CARTESIAN_POINT('Ctrl Pts',(0.00286292080640031,-0.0321934096576657,
0.0766676394858149));
#69437=CARTESIAN_POINT('Ctrl Pts',(0.00286998346157403,-0.0325229783203769,
0.0764864244009287));
#69438=CARTESIAN_POINT('Ctrl Pts',(0.00290219102084661,-0.0324130253092449,
0.07655884790155));
#69439=CARTESIAN_POINT('Ctrl Pts',(0.00293589186835669,-0.0323031222208069,
0.0766305941629912));
#69440=CARTESIAN_POINT('Ctrl Pts',(0.00297103959280049,-0.0321934096576657,
0.0767015728066625));
#69441=CARTESIAN_POINT('',(0.00280789397620474,-0.0321934096584275,0.0766503691869222));
#69442=CARTESIAN_POINT('Ctrl Pts',(0.00264146297247978,-0.0322104233328919,
0.0765880680678742));
#69443=CARTESIAN_POINT('Ctrl Pts',(0.00268073195631818,-0.0322609421831417,
0.0765706045726451));
#69444=CARTESIAN_POINT('Ctrl Pts',(0.00271929429548424,-0.0323120888240844,
0.0765534553327049));
#69445=CARTESIAN_POINT('Ctrl Pts',(0.0027950397115963,-0.0324156524631806,
0.0765197702310391));
#69446=CARTESIAN_POINT('Ctrl Pts',(0.00283219165321953,-0.0324680267167308,
0.07650324821565));
#69447=CARTESIAN_POINT('Ctrl Pts',(0.00286865161512663,-0.0325210109755912,
0.076487033933828));
#69448=CARTESIAN_POINT('Origin',(0.00581579726585811,-0.0262834582511792,
0.0666282587511482));
#69449=CARTESIAN_POINT('Origin',(-0.00402200473973704,-0.0342770910835669,
0.073598576003963));
#69450=CARTESIAN_POINT('Ctrl Pts',(0.00292141350614364,-0.0326943950436604,
0.076598804146629));
#69451=CARTESIAN_POINT('Ctrl Pts',(0.00295516261683231,-0.0325844576448134,
0.0766705025374135));
#69452=CARTESIAN_POINT('Ctrl Pts',(0.00299039695627052,-0.0324744968375323,
0.076741508015463));
#69453=CARTESIAN_POINT('Ctrl Pts',(0.00302707012533032,-0.0323646534831895,
0.0768117302270937));
#69454=CARTESIAN_POINT('Ctrl Pts',(0.00288075833330346,-0.0326943950436604,
0.0767045788340702));
#69455=CARTESIAN_POINT('Ctrl Pts',(0.00291596521742796,-0.0325844576448134,
0.0767768375293324));
#69456=CARTESIAN_POINT('Ctrl Pts',(0.00295266902148612,-0.0324744968375323,
0.0768483732023684));
#69457=CARTESIAN_POINT('Ctrl Pts',(0.00299082145421641,-0.0323646534831895,
0.0769190948461468));
#69458=CARTESIAN_POINT('Ctrl Pts',(0.00284010316046328,-0.0326943950436604,
0.0768103535215114));
#69459=CARTESIAN_POINT('Ctrl Pts',(0.00287676781802361,-0.0325844576448134,
0.0768831725212512));
#69460=CARTESIAN_POINT('Ctrl Pts',(0.00291494108670172,-0.0324744968375323,
0.0769552383892738));
#69461=CARTESIAN_POINT('Ctrl Pts',(0.0029545727831025,-0.0323646534831895,
0.0770264594652));
#69462=CARTESIAN_POINT('Ctrl Pts',(0.0027994479876231,-0.0326943950436604,
0.0769161282089526));
#69463=CARTESIAN_POINT('Ctrl Pts',(0.00283757041861926,-0.0325844576448134,
0.07698950751317));
#69464=CARTESIAN_POINT('Ctrl Pts',(0.00287721315191733,-0.0324744968375323,
0.0770621035761792));
#69465=CARTESIAN_POINT('Ctrl Pts',(0.00291832411198859,-0.0323646534831895,
0.0771338240842531));
#69466=CARTESIAN_POINT('',(0.0028053686348441,-0.0326773559991174,0.0769274947710929));
#69467=CARTESIAN_POINT('',(0.00279944798762602,-0.0326943950436594,0.0769161282089466));
#69468=CARTESIAN_POINT('Origin',(0.0175009479672079,-0.0326395670470851,
0.069196178123875));
#69469=CARTESIAN_POINT('Ctrl Pts',(0.00280536863780952,-0.0326773559987453,
0.0769274947695367));
#69470=CARTESIAN_POINT('Ctrl Pts',(0.00284344265659943,-0.0326267922586819,
0.0769076109476141));
#69471=CARTESIAN_POINT('Ctrl Pts',(0.00288084184090237,-0.0325756109581063,
0.0768880795520755));
#69472=CARTESIAN_POINT('Ctrl Pts',(0.00295432236932552,-0.0324719985462371,
0.0768497049914597));
#69473=CARTESIAN_POINT('Ctrl Pts',(0.00299037424223145,-0.0324196091621781,
0.0768308772174652));
#69474=CARTESIAN_POINT('Ctrl Pts',(0.00302576498976948,-0.0323666188837757,
0.0768123947103877));
#69475=CARTESIAN_POINT('',(0.00286006700404867,-0.0326943950436703,0.0767584125465685));
#69476=CARTESIAN_POINT('Origin',(0.00812378219310841,-0.0315241814719618,
0.07415));
#69477=CARTESIAN_POINT('',(0.00280536863488315,-0.0327114338379858,0.0769274947710722));
#69478=CARTESIAN_POINT('',(0.00281131354479966,-0.0326943950436593,0.07693884866222));
#69479=CARTESIAN_POINT('Origin',(0.0174792905163763,-0.0326395659724961,
0.0691563769486344));
#69480=CARTESIAN_POINT('Origin',(0.0175474642808288,-0.0326395683304246,
0.0692852422766188));
#69481=CARTESIAN_POINT('Origin',(0.0175677465258632,-0.0326395673934692,
0.0693257614342945));
#69482=CARTESIAN_POINT('Ctrl Pts',(0.00295319228954088,-0.0332451089994432,
0.0766685561437311));
#69483=CARTESIAN_POINT('Ctrl Pts',(0.00304818118860149,-0.0329451141710253,
0.0768635681325073));
#69484=CARTESIAN_POINT('Ctrl Pts',(0.00315758933443493,-0.0326442513127493,
0.0770508711606103));
#69485=CARTESIAN_POINT('Ctrl Pts',(0.00306752783277678,-0.0332451089994432,
0.0768908788451202));
#69486=CARTESIAN_POINT('Ctrl Pts',(0.00317090176970667,-0.0329451141710253,
0.0770815785983315));
#69487=CARTESIAN_POINT('Ctrl Pts',(0.00328834631719047,-0.0326442513127493,
0.0772639500461449));
#69488=CARTESIAN_POINT('Ctrl Pts',(0.00306867118820914,-0.0332451089994432,
0.0768931020721341));
#69489=CARTESIAN_POINT('Ctrl Pts',(0.00317212897551773,-0.0329451141710253,
0.0770837587029898));
#69490=CARTESIAN_POINT('Ctrl Pts',(0.00328965388701803,-0.0326442513127493,
0.0772660808350003));
#69491=CARTESIAN_POINT('',(0.00308483367278007,-0.0331951640388616,0.0769225661055207));
#69492=CARTESIAN_POINT('',(0.00320299791123032,-0.0328677532355008,0.0771272482464603));
#69493=CARTESIAN_POINT('Origin',(0.017386680150143,-0.0326402808282017,
0.0681767422555932));
#69494=CARTESIAN_POINT('Origin',(-0.00625614153616046,-0.0326944278779117,
0.0828508016780252));
#69495=CARTESIAN_POINT('',(0.00313945275405452,-0.0326943950436593,0.0770195966690428));
#69496=CARTESIAN_POINT('',(0.00317180650376106,-0.0326943950436694,0.0770730708205709));
#69497=CARTESIAN_POINT('',(0.00302576498972491,-0.0330220786163545,0.0768123947104077));
#69498=CARTESIAN_POINT('Origin',(0.0176619112604149,-0.0326396682765736,
0.068570950932937));
#69499=CARTESIAN_POINT('',(0.00302696919836557,-0.0331951640388587,0.0768117658230245));
#69500=CARTESIAN_POINT('Origin',(-0.0067515135471169,-0.0331952026560048,
0.0819184912642713));
#69501=CARTESIAN_POINT('',(0.00305590143558282,-0.0331951640388701,0.0768671659642826));
#69502=CARTESIAN_POINT('Ctrl Pts',(0.00270058745800114,-0.0330240426238172,
0.0767168967383076));
#69503=CARTESIAN_POINT('Ctrl Pts',(0.00273594896137764,-0.0329142774063519,
0.0767916065293464));
#69504=CARTESIAN_POINT('Ctrl Pts',(0.00277287255382553,-0.0328043479726691,
0.0768656225448883));
#69505=CARTESIAN_POINT('Ctrl Pts',(0.00281131354479966,-0.0326943950436593,
0.0769388486622199));
#69506=CARTESIAN_POINT('Ctrl Pts',(0.0028094103993424,-0.0330240426238172,
0.0767484990075675));
#69507=CARTESIAN_POINT('Ctrl Pts',(0.00284520725476656,-0.0329142774063519,
0.0768217096565682));
#69508=CARTESIAN_POINT('Ctrl Pts',(0.0028825354248474,-0.0328043479726691,
0.0768942167827522));
#69509=CARTESIAN_POINT('Ctrl Pts',(0.00292134964751124,-0.0326943950436593,
0.076965926182132));
#69510=CARTESIAN_POINT('Ctrl Pts',(0.00291823334068367,-0.0330240426238172,
0.0767801012768274));
#69511=CARTESIAN_POINT('Ctrl Pts',(0.00295446554815548,-0.0329142774063519,
0.07685181278379));
#69512=CARTESIAN_POINT('Ctrl Pts',(0.00299219829586928,-0.0328043479726691,
0.0769228110206161));
#69513=CARTESIAN_POINT('Ctrl Pts',(0.00303138575022282,-0.0326943950436593,
0.076993003702044));
#69514=CARTESIAN_POINT('Ctrl Pts',(0.00302705628202493,-0.0330240426238172,
0.0768117035460873));
#69515=CARTESIAN_POINT('Ctrl Pts',(0.0030637238415444,-0.0329142774063519,
0.0768819159110119));
#69516=CARTESIAN_POINT('Ctrl Pts',(0.00310186116689115,-0.0328043479726691,
0.0769514052584801));
#69517=CARTESIAN_POINT('Ctrl Pts',(0.00314142185293441,-0.0326943950436593,
0.077020081221956));
#69518=CARTESIAN_POINT('',(0.00297538314943708,-0.0326943950436693,0.0769792226656414));
#69519=CARTESIAN_POINT('Ctrl Pts',(0.00280536863781758,-0.0327114338383317,
0.0769274947695324));
#69520=CARTESIAN_POINT('Ctrl Pts',(0.00284343632372475,-0.0327619876831131,
0.0769076142549022));
#69521=CARTESIAN_POINT('Ctrl Pts',(0.00288083241478682,-0.0328131562604672,
0.0768880844747814));
#69522=CARTESIAN_POINT('Ctrl Pts',(0.00295431287558149,-0.0329167375858766,
0.0768497099494839));
#69523=CARTESIAN_POINT('Ctrl Pts',(0.00299036796694966,-0.0329691088920619,
0.0768308804946759));
#69524=CARTESIAN_POINT('Ctrl Pts',(0.00302576498976837,-0.0330220786163186,
0.0768123947103882));
#69525=CARTESIAN_POINT('Ctrl Pts',(0.0030854409739107,-0.0331951640388604,
0.0769206311147899));
#69526=CARTESIAN_POINT('Ctrl Pts',(0.00314272199584558,-0.0330306422010619,
0.0770247955892129));
#69527=CARTESIAN_POINT('Ctrl Pts',(0.00320425929881839,-0.0328657861914645,
0.0771265035709478));
#69528=CARTESIAN_POINT('Ctrl Pts',(0.00308483367277861,-0.0331951640388604,
0.0769225661055178));
#69529=CARTESIAN_POINT('Ctrl Pts',(0.0031421546994062,-0.0330306422010619,
0.0770267431355024));
#69530=CARTESIAN_POINT('Ctrl Pts',(0.00320373249182254,-0.0328657861914645,
0.0771284620086342));
#69531=CARTESIAN_POINT('Ctrl Pts',(0.0029836409722735,-0.0331951640388604,
0.0772449875977048));
#69532=CARTESIAN_POINT('Ctrl Pts',(0.00304762785653462,-0.0330306422010619,
0.0773512567218936));
#69533=CARTESIAN_POINT('Ctrl Pts',(0.00311595227910942,-0.0328657861914645,
0.0774547903946437));
#69534=CARTESIAN_POINT('',(0.00299026364734075,-0.0331781648281913,0.0772559599701381));
#69535=CARTESIAN_POINT('',(0.00298364097227652,-0.0331951640388588,0.0772449875976981));
#69536=CARTESIAN_POINT('Origin',(0.0167446679814435,-0.0326412092246788,
0.0681015706921973));
#69537=CARTESIAN_POINT('Ctrl Pts',(0.00299026364746687,-0.033178164828644,
0.0772559599682971));
#69538=CARTESIAN_POINT('Ctrl Pts',(0.00302703931528364,-0.0331276811546775,
0.0772337093766741));
#69539=CARTESIAN_POINT('Ctrl Pts',(0.00306315091092208,-0.0330765663497785,
0.077211860532896));
#69540=CARTESIAN_POINT('Ctrl Pts',(0.0031340770679752,-0.032973061446328,
0.0771689477077748));
#69541=CARTESIAN_POINT('Ctrl Pts',(0.00316886297954141,-0.0329207133374062,
0.0771479010668649));
#69542=CARTESIAN_POINT('Ctrl Pts',(0.0032029978965378,-0.0328677532289367,
0.0771272482390092));
#69543=CARTESIAN_POINT('',(0.0030342373225383,-0.0331951640388701,0.0770837768516194));
#69544=CARTESIAN_POINT('Origin',(0.00812378219310841,-0.0315241814719618,
0.07415));
#69545=CARTESIAN_POINT('',(0.00299026364900185,-0.0332121607144214,0.0772559599698887));
#69546=CARTESIAN_POINT('',(0.00299690974454838,-0.0331951640388587,0.0772669181728474));
#69547=CARTESIAN_POINT('Origin',(0.0167148396002469,-0.0326413641344407,
0.068067415206876));
#69548=CARTESIAN_POINT('Origin',(0.0174820935607263,-0.0326412103657649,
0.0693203784622903));
#69549=CARTESIAN_POINT('Origin',(0.0174985010147094,-0.0326413655906454,
0.0693626535943588));
#69550=CARTESIAN_POINT('Ctrl Pts',(0.00312152643615495,-0.0337436976235975,
0.0769882322565332));
#69551=CARTESIAN_POINT('Ctrl Pts',(0.00314705392721609,-0.0336723290703325,
0.0770332233029239));
#69552=CARTESIAN_POINT('Ctrl Pts',(0.00317338653564643,-0.033601104548885,
0.0770777479117201));
#69553=CARTESIAN_POINT('Ctrl Pts',(0.00325746133816869,-0.0333736987606857,
0.0772199061677783));
#69554=CARTESIAN_POINT('Ctrl Pts',(0.00334955545247764,-0.0331450831799191,
0.0773570054613371));
#69555=CARTESIAN_POINT('Ctrl Pts',(0.00324959534457015,-0.0337436976235975,
0.0772029375305657));
#69556=CARTESIAN_POINT('Ctrl Pts',(0.00327705392740539,-0.0336723290703325,
0.0772467767057847));
#69557=CARTESIAN_POINT('Ctrl Pts',(0.00330529659667296,-0.033601104548885,
0.0772901148955005));
#69558=CARTESIAN_POINT('Ctrl Pts',(0.00339546984508672,-0.0333736987606857,
0.0774284851504514));
#69559=CARTESIAN_POINT('Ctrl Pts',(0.00349343497818585,-0.0331450831799191,
0.0775614527212405));
#69560=CARTESIAN_POINT('Ctrl Pts',(0.0032508760336543,-0.0337436976235975,
0.077205084583306));
#69561=CARTESIAN_POINT('Ctrl Pts',(0.00327835392740729,-0.0336723290703325,
0.0772489122398133));
#69562=CARTESIAN_POINT('Ctrl Pts',(0.00330661569728322,-0.033601104548885,
0.0772922385653383));
#69563=CARTESIAN_POINT('Ctrl Pts',(0.0033968499301559,-0.0333736987606857,
0.0774305709402782));
#69564=CARTESIAN_POINT('Ctrl Pts',(0.00349487377344293,-0.0331450831799191,
0.0775634971938395));
#69565=CARTESIAN_POINT('',(0.00326886775284914,-0.0336938721132548,0.0772334932751286));
#69566=CARTESIAN_POINT('',(0.0033996509203255,-0.0333679869945434,0.0774303519197621));
#69567=CARTESIAN_POINT('Ctrl Pts',(0.00326886775285565,-0.0336938721132647,
0.0772334932751408));
#69568=CARTESIAN_POINT('Ctrl Pts',(0.00328090407360133,-0.0336629187933931,
0.0772524442836817));
#69569=CARTESIAN_POINT('Ctrl Pts',(0.00329304751061946,-0.0336319952301039,
0.0772713187537415));
#69570=CARTESIAN_POINT('Ctrl Pts',(0.0033052965966801,-0.0336011045488949,
0.0772901148955123));
#69571=CARTESIAN_POINT('Ctrl Pts',(0.00333603374500763,-0.0335235892595453,
0.077337280846893));
#69572=CARTESIAN_POINT('Ctrl Pts',(0.0033674908859935,-0.0334458668660368,
0.0773840373087036));
#69573=CARTESIAN_POINT('Ctrl Pts',(0.00339965092005911,-0.0333679869945384,
0.0774303519199386));
#69574=CARTESIAN_POINT('Ctrl Pts',(0.00339967571956702,-0.0333679692460368,
0.077430388839483));
#69575=CARTESIAN_POINT('Ctrl Pts',(0.00340004460580707,-0.033339189537481,
0.0774301254751632));
#69576=CARTESIAN_POINT('Ctrl Pts',(0.00340031921724595,-0.0333104081060444,
0.077429925427979));
#69577=CARTESIAN_POINT('Ctrl Pts',(0.00340067945138924,-0.0332532698185305,
0.0774296561547328));
#69578=CARTESIAN_POINT('Ctrl Pts',(0.00340076783166611,-0.0332249171053087,
0.0774295850184696));
#69579=CARTESIAN_POINT('Ctrl Pts',(0.00340076691158274,-0.0331960985374019,
0.0774295772582261));
#69580=CARTESIAN_POINT('Ctrl Pts',(0.00340076687221496,-0.0331956312550877,
0.0774295771493602));
#69581=CARTESIAN_POINT('Ctrl Pts',(0.00340076680876476,-0.0331951640388587,
0.0774295770579837));
#69582=CARTESIAN_POINT('',(0.00332947165532952,-0.0331951640388587,0.0773269028104969));
#69583=CARTESIAN_POINT('',(0.00336511923205677,-0.0331951640388687,0.0773782399342498));
#69584=CARTESIAN_POINT('',(0.00320299790946593,-0.0335216366567704,0.0771272482310453));
#69585=CARTESIAN_POINT('Origin',(0.0167877337917752,-0.0326434571527087,
0.0674926431002186));
#69586=CARTESIAN_POINT('',(0.00320416025344758,-0.0336938721132327,0.077126544972079));
#69587=CARTESIAN_POINT('Origin',(-0.00613933112997888,-0.0336938867896225,
0.0827796855776315));
#69588=CARTESIAN_POINT('',(0.00323651400315836,-0.0336938721132537,0.0771800191236138));
#69589=CARTESIAN_POINT('Ctrl Pts',(0.00287246613866903,-0.0335235895815172,
0.0770523576100163));
#69590=CARTESIAN_POINT('Ctrl Pts',(0.00291242280538719,-0.0334144449262748,
0.0771246523143955));
#69591=CARTESIAN_POINT('Ctrl Pts',(0.00295391893165918,-0.0333049234473147,
0.0771962046019677));
#69592=CARTESIAN_POINT('Ctrl Pts',(0.0029969097445482,-0.0331951640388587,
0.0772669181728474));
#69593=CARTESIAN_POINT('Ctrl Pts',(0.0029830588268381,-0.0335235895815172,
0.0770770644877937));
#69594=CARTESIAN_POINT('Ctrl Pts',(0.00302335563237224,-0.0334144449262748,
0.0771478366660834));
#69595=CARTESIAN_POINT('Ctrl Pts',(0.00306516083399531,-0.0333049234473147,
0.077217857651356));
#69596=CARTESIAN_POINT('Ctrl Pts',(0.00310842908618799,-0.0331951640388587,
0.0772870330659916));
#69597=CARTESIAN_POINT('Ctrl Pts',(0.00309365151500718,-0.0335235895815172,
0.0771017713655712));
#69598=CARTESIAN_POINT('Ctrl Pts',(0.00313428845935728,-0.0334144449262748,
0.0771710210177712));
#69599=CARTESIAN_POINT('Ctrl Pts',(0.00317640273633143,-0.0333049234473147,
0.0772395107007442));
#69600=CARTESIAN_POINT('Ctrl Pts',(0.00321994842782777,-0.0331951640388587,
0.0773071479591357));
#69601=CARTESIAN_POINT('Ctrl Pts',(0.00320424420317625,-0.0335235895815172,
0.0771264782433486));
#69602=CARTESIAN_POINT('Ctrl Pts',(0.00324522128634233,-0.0334144449262748,
0.077194205369459));
#69603=CARTESIAN_POINT('Ctrl Pts',(0.00328764463866756,-0.0333049234473147,
0.0772611637501324));
#69604=CARTESIAN_POINT('Ctrl Pts',(0.00333146776946756,-0.0331951640388587,
0.0773272628522799));
#69605=CARTESIAN_POINT('',(0.00316319069994895,-0.0331951640388687,0.0772969104916822));
#69606=CARTESIAN_POINT('Ctrl Pts',(0.00299026365167755,-0.0332121607145971,
0.077255959968262));
#69607=CARTESIAN_POINT('Ctrl Pts',(0.00302697745968889,-0.0332625444109906,
0.0772337468181496));
#69608=CARTESIAN_POINT('Ctrl Pts',(0.00306305863117457,-0.0333135300747148,
0.0772119164354719));
#69609=CARTESIAN_POINT('Ctrl Pts',(0.00313398434181871,-0.0334167203140597,
0.0771690038763366));
#69610=CARTESIAN_POINT('Ctrl Pts',(0.00316880141089817,-0.033468884758729,
0.0771479383202467));
#69611=CARTESIAN_POINT('Ctrl Pts',(0.00320299791014901,-0.0335216366562368,
0.0771272482308138));
#69612=CARTESIAN_POINT('Ctrl Pts',(0.00326910666883635,-0.0336938721132388,
0.0772325223817137));
#69613=CARTESIAN_POINT('Ctrl Pts',(0.00328714969522587,-0.0336474569764957,
0.0772609384085093));
#69614=CARTESIAN_POINT('Ctrl Pts',(0.00330552413076729,-0.033601104548885,
0.0772891412718158));
#69615=CARTESIAN_POINT('Ctrl Pts',(0.00335204397701066,-0.0334837508592655,
0.0773605444374629));
#69616=CARTESIAN_POINT('Ctrl Pts',(0.00340065921900735,-0.0333660264659097,
0.0774305377686061));
#69617=CARTESIAN_POINT('Ctrl Pts',(0.00326886775283826,-0.0336938721132388,
0.0772334932751113));
#69618=CARTESIAN_POINT('Ctrl Pts',(0.00328691646218901,-0.0336474569764957,
0.0772619107003615));
#69619=CARTESIAN_POINT('Ctrl Pts',(0.00330529659667295,-0.033601104548885,
0.0772901148955005));
#69620=CARTESIAN_POINT('Ctrl Pts',(0.00335183087132848,-0.0334837508592655,
0.0773615214330415));
#69621=CARTESIAN_POINT('Ctrl Pts',(0.00340046063531764,-0.0333660264659097,
0.077431517707054));
#69622=CARTESIAN_POINT('Ctrl Pts',(0.00318763525797031,-0.0336938721132388,
0.0775636013196375));
#69623=CARTESIAN_POINT('Ctrl Pts',(0.00320761619924714,-0.0336474569764957,
0.077592494225636));
#69624=CARTESIAN_POINT('Ctrl Pts',(0.00322793399936187,-0.033601104548885,
0.0776211512497286));
#69625=CARTESIAN_POINT('Ctrl Pts',(0.00327937399789735,-0.0334837508592655,
0.0776937042460684));
#69626=CARTESIAN_POINT('Ctrl Pts',(0.00333294130348528,-0.0333660264659097,
0.0777647011086698));
#69627=CARTESIAN_POINT('',(0.00319541831379252,-0.0336769361243753,0.0775721673648515));
#69628=CARTESIAN_POINT('',(0.00318811974601819,-0.033693872113232,0.0775616324843663));
#69629=CARTESIAN_POINT('Ctrl Pts',(0.0031954183137927,-0.033676936124375,
0.0775721673648517));
#69630=CARTESIAN_POINT('Ctrl Pts',(0.00319419991937076,-0.0336797586669961,
0.0775704127192077));
#69631=CARTESIAN_POINT('Ctrl Pts',(0.00319298250808888,-0.0336825812712718,
0.0775686574892483));
#69632=CARTESIAN_POINT('Ctrl Pts',(0.00319054965489436,-0.0336882265949077,
0.0775651458660598));
#69633=CARTESIAN_POINT('Ctrl Pts',(0.0031893342129824,-0.0336910493142397,
0.0775633894728613));
#69634=CARTESIAN_POINT('Ctrl Pts',(0.00318811974601561,-0.0336938721132351,
0.077561632484373));
#69635=CARTESIAN_POINT('Ctrl Pts',(0.00319541831379256,-0.0336769361243753,
0.0775721673648515));
#69636=CARTESIAN_POINT('Ctrl Pts',(0.00322984434082938,-0.033627903142825,
0.0775482625499652));
#69637=CARTESIAN_POINT('Ctrl Pts',(0.00326476567292551,-0.0335767852155825,
0.0775240138041409));
#69638=CARTESIAN_POINT('Ctrl Pts',(0.00333319318983,-0.0334733199122762,
0.0774764989653541));
#69639=CARTESIAN_POINT('Ctrl Pts',(0.00336674531917255,-0.0334209645148413,
0.0774532009693323));
#69640=CARTESIAN_POINT('Ctrl Pts',(0.00339965091615904,-0.0333679869844681,
0.0774303519137662));
#69641=CARTESIAN_POINT('',(0.00322849374944367,-0.0336938721132534,0.0773975628797575));
#69642=CARTESIAN_POINT('Origin',(0.00812378219310841,-0.0315241814719618,
0.07415));
#69643=CARTESIAN_POINT('',(0.0031954183148614,-0.0337108120655386,0.0775721673641177));
#69644=CARTESIAN_POINT('',(0.00320273936760633,-0.0336938721132327,0.0775826866314311));
#69645=CARTESIAN_POINT('Origin',(0.0172718609241822,-0.0345562510848324,
0.0691583577627806));
#69646=CARTESIAN_POINT('Ctrl Pts',(0.00320273936761098,-0.033693872113231,
0.0775826866314307));
#69647=CARTESIAN_POINT('Ctrl Pts',(0.0032015174131691,-0.0336910493311992,
0.0775809348577371));
#69648=CARTESIAN_POINT('Ctrl Pts',(0.00320029634609684,-0.0336882266033876,
0.0775791823627307));
#69649=CARTESIAN_POINT('Ctrl Pts',(0.00319785599361853,-0.0336825812712792,
0.0775756759391047));
#69650=CARTESIAN_POINT('Ctrl Pts',(0.00319663670821591,-0.0336797586669998,
0.0775739220104976));
#69651=CARTESIAN_POINT('Ctrl Pts',(0.00319541831379236,-0.033676936124375,
0.0775721673648512));
#69652=CARTESIAN_POINT('Origin',(0.0159969813080498,-0.0345562513515122,
0.0673223721723791));
#69653=CARTESIAN_POINT('Ctrl Pts',(0.00330958307100335,-0.0342436276873909,
0.0772966826679415));
#69654=CARTESIAN_POINT('Ctrl Pts',(0.00342826216427442,-0.0339430054201809,
0.0774782531810595));
#69655=CARTESIAN_POINT('Ctrl Pts',(0.00356028073769327,-0.0336441434784051,
0.0776503684758071));
#69656=CARTESIAN_POINT('Ctrl Pts',(0.0034508788686863,-0.0342436276873909,
0.0775029240254747));
#69657=CARTESIAN_POINT('Ctrl Pts',(0.00357733648298728,-0.0339430054201809,
0.0776791654797324));
#69658=CARTESIAN_POINT('Ctrl Pts',(0.00371671007292475,-0.0336441434784051,
0.0778453809448418));
#69659=CARTESIAN_POINT('Ctrl Pts',(0.00345229182666312,-0.0342436276873909,
0.07750498643905));
#69660=CARTESIAN_POINT('Ctrl Pts',(0.00357882722617441,-0.0339430054201809,
0.0776811746027192));
#69661=CARTESIAN_POINT('Ctrl Pts',(0.00371827436627707,-0.0336441434784051,
0.0778473310695321));
#69662=CARTESIAN_POINT('',(0.00347206196219838,-0.0341934961088741,0.0775322513054685));
#69663=CARTESIAN_POINT('',(0.00361494791185617,-0.0338664212863469,0.0777205095474807));
#69664=CARTESIAN_POINT('Origin',(0.0173006318178325,-0.0345610720403646,
0.0681076134076986));
#69665=CARTESIAN_POINT('Origin',(-0.00498213160236743,-0.0336938005072949,
0.0845285157372853));
#69666=CARTESIAN_POINT('',(0.003538411509985,-0.0336938721132327,0.0776216711679468));
#69667=CARTESIAN_POINT('',(0.00357721222903342,-0.0336938721132426,0.0776706686597508));
#69668=CARTESIAN_POINT('',(0.00339965091615601,-0.0340203938281605,0.0774303519137619));
#69669=CARTESIAN_POINT('Origin',(0.0175070847443505,-0.0345589643243467,
0.0685422557012214));
#69670=CARTESIAN_POINT('',(0.00340076680876393,-0.0341934961088739,0.0774295770579827));
#69671=CARTESIAN_POINT('Origin',(-0.00565054137690369,-0.0341934220717627,
0.0837146417663959));
#69672=CARTESIAN_POINT('',(0.00343641438549115,-0.034193496108884,0.0774809141817356));
#69673=CARTESIAN_POINT('Ctrl Pts',(0.00306506748220749,-0.0340223579322396,
0.0773763610265673));
#69674=CARTESIAN_POINT('Ctrl Pts',(0.00310956741546666,-0.0339125849573574,
0.0774461338961124));
#69675=CARTESIAN_POINT('Ctrl Pts',(0.00315548021540779,-0.0338030433565231,
0.0775149366918551));
#69676=CARTESIAN_POINT('Ctrl Pts',(0.00320273936760564,-0.0336938721132327,
0.0775826866314311));
#69677=CARTESIAN_POINT('Ctrl Pts',(0.00317699332258989,-0.0340223579322396,
0.0773940750347268));
#69678=CARTESIAN_POINT('Ctrl Pts',(0.00322173757822165,-0.0339125849573574,
0.0774623041550182));
#69679=CARTESIAN_POINT('Ctrl Pts',(0.0032678625768305,-0.0338030433565231,
0.0775295592293766));
#69680=CARTESIAN_POINT('Ctrl Pts',(0.00331530170807924,-0.0336938721132327,
0.0775957594787677));
#69681=CARTESIAN_POINT('Ctrl Pts',(0.00328891916297228,-0.0340223579322396,
0.0774117890428864));
#69682=CARTESIAN_POINT('Ctrl Pts',(0.00333390774097664,-0.0339125849573574,
0.0774784744139241));
#69683=CARTESIAN_POINT('Ctrl Pts',(0.0033802449382532,-0.0338030433565231,
0.077544181766898));
#69684=CARTESIAN_POINT('Ctrl Pts',(0.00342786404855284,-0.0336938721132327,
0.0776088323261044));
#69685=CARTESIAN_POINT('Ctrl Pts',(0.00340084500335468,-0.0340223579322396,
0.0774295030510459));
#69686=CARTESIAN_POINT('Ctrl Pts',(0.00344607790373163,-0.0339125849573574,
0.0774946446728299));
#69687=CARTESIAN_POINT('Ctrl Pts',(0.00349262729967591,-0.0338030433565231,
0.0775588043044195));
#69688=CARTESIAN_POINT('Ctrl Pts',(0.00354042638902644,-0.0336938721132327,
0.0776219051734411));
#69689=CARTESIAN_POINT('',(0.00337057543880566,-0.0336938721132427,0.077602178899699));
#69690=CARTESIAN_POINT('Ctrl Pts',(0.00319541831781671,-0.033710812066268,
0.0775721673620571));
#69691=CARTESIAN_POINT('Ctrl Pts',(0.00323073764797705,-0.0337611408994413,
0.0775476422535255));
#69692=CARTESIAN_POINT('Ctrl Pts',(0.00326541247872095,-0.0338121088781569,
0.0775235646738136));
#69693=CARTESIAN_POINT('Ctrl Pts',(0.00333350472956026,-0.0339153382773232,
0.0774762826377611));
#69694=CARTESIAN_POINT('Ctrl Pts',(0.00336689334249021,-0.0339675558473112,
0.0774530981845989));
#69695=CARTESIAN_POINT('Ctrl Pts',(0.00339965091619176,-0.0340203938281304,
0.0774303519137434));
#69696=CARTESIAN_POINT('Ctrl Pts',(0.00347242197248126,-0.0341934961088741,
0.0775302553659703));
#69697=CARTESIAN_POINT('Ctrl Pts',(0.00354230608916746,-0.0340287516182428,
0.077626418574135));
#69698=CARTESIAN_POINT('Ctrl Pts',(0.00361610498956091,-0.0338644633275951,
0.0777196112491169));
#69699=CARTESIAN_POINT('Ctrl Pts',(0.00347206196219839,-0.0341934961088741,
0.0775322513054685));
#69700=CARTESIAN_POINT('Ctrl Pts',(0.0035419873433613,-0.0340287516182428,
0.0776284219565622));
#69701=CARTESIAN_POINT('Ctrl Pts',(0.00361582778059364,-0.0338644633275951,
0.077721620362621));
#69702=CARTESIAN_POINT('Ctrl Pts',(0.00341207732454776,-0.0341934961088741,
0.0778648132162559));
#69703=CARTESIAN_POINT('Ctrl Pts',(0.00348887816121998,-0.0340287516182428,
0.0779622240024765));
#69704=CARTESIAN_POINT('Ctrl Pts',(0.00356963943474203,-0.0338644633275951,
0.0780563773161981));
#69705=CARTESIAN_POINT('',(0.00342002298097895,-0.0341764758832406,0.0778748690265504));
#69706=CARTESIAN_POINT('',(0.00341207732454946,-0.034193496108874,0.0778648132162463));
#69707=CARTESIAN_POINT('Origin',(0.0167185512793139,-0.0345621025955202,
0.0679970923786799));
#69708=CARTESIAN_POINT('Ctrl Pts',(0.00342002298065817,-0.0341764758837501,
0.0778748690247524));
#69709=CARTESIAN_POINT('Ctrl Pts',(0.00345367396163459,-0.0341260050040318,
0.0778482210664868));
#69710=CARTESIAN_POINT('Ctrl Pts',(0.00348673998545543,-0.0340749269147912,
0.0778220362826484));
#69711=CARTESIAN_POINT('Ctrl Pts',(0.00355172785916549,-0.0339715436305661,
0.0777705729141452));
#69712=CARTESIAN_POINT('Ctrl Pts',(0.00358362505779547,-0.0339192778236895,
0.0777453138582455));
#69713=CARTESIAN_POINT('Ctrl Pts',(0.00361494790979576,-0.0338664212854881,
0.077720509546709));
#69714=CARTESIAN_POINT('',(0.00344206964338392,-0.0341934961088841,0.0776985322608674));
#69715=CARTESIAN_POINT('Origin',(0.00812378219310841,-0.0315241814719618,
0.07415));
#69716=CARTESIAN_POINT('',(0.00342002298207836,-0.0342105180190357,0.0778748690267528));
#69717=CARTESIAN_POINT('',(0.00342799009848599,-0.0341934961088739,0.0778849078441259));
#69718=CARTESIAN_POINT('Origin',(0.0166947039403234,-0.0345621700238114,
0.0679585443454162));
#69719=CARTESIAN_POINT('Origin',(0.0160827186936042,-0.034562104145154,
0.067194158895128));
#69720=CARTESIAN_POINT('Origin',(0.0161147699170915,-0.0345621714440594,
0.0672262105569304));
#69721=CARTESIAN_POINT('Ctrl Pts',(0.0035374802865757,-0.0346945769586966,
0.0776204952203742));
#69722=CARTESIAN_POINT('Ctrl Pts',(0.00361017119847693,-0.0345275153362944,
0.0777165571500617));
#69723=CARTESIAN_POINT('Ctrl Pts',(0.00368590197124099,-0.0343603235965186,
0.0778103578640126));
#69724=CARTESIAN_POINT('Ctrl Pts',(0.00376444450366233,-0.034193496108874,
0.0779016232702499));
#69725=CARTESIAN_POINT('Ctrl Pts',(0.00358952498655659,-0.0346945769586966,
0.0776862171921169));
#69726=CARTESIAN_POINT('Ctrl Pts',(0.00366359247146961,-0.0345275153362944,
0.0777811890247257));
#69727=CARTESIAN_POINT('Ctrl Pts',(0.00374066589074799,-0.0343603235965186,
0.0778738560676888));
#69728=CARTESIAN_POINT('Ctrl Pts',(0.00382051322206656,-0.034193496108874,
0.0779639476409435));
#69729=CARTESIAN_POINT('Ctrl Pts',(0.00364156968653757,-0.0346945769586966,
0.0777519391638623));
#69730=CARTESIAN_POINT('Ctrl Pts',(0.00371701374446233,-0.0345275153362944,
0.0778458208993921));
#69731=CARTESIAN_POINT('Ctrl Pts',(0.00379542981025503,-0.0343603235965186,
0.0779373542713669));
#69732=CARTESIAN_POINT('Ctrl Pts',(0.00387658194047087,-0.034193496108874,
0.078026272011638));
#69733=CARTESIAN_POINT('Ctrl Pts',(0.00369361438651835,-0.0346945769586966,
0.0778176611356023));
#69734=CARTESIAN_POINT('Ctrl Pts',(0.00377043501745496,-0.0345275153362944,
0.0779104527740538));
#69735=CARTESIAN_POINT('Ctrl Pts',(0.00385019372976199,-0.0343603235965186,
0.0780008524750413));
#69736=CARTESIAN_POINT('Ctrl Pts',(0.00393265065887501,-0.034193496108874,
0.0780885963823307));
#69737=CARTESIAN_POINT('',(0.00369361438614239,-0.0346945769586966,0.0778176611351273));
#69738=CARTESIAN_POINT('',(0.00384803921500643,-0.0343667727831482,0.0779965760080376));
#69739=CARTESIAN_POINT('Origin',(0.0165273843527379,-0.0345626457063339,
0.0669552674912437));
#69740=CARTESIAN_POINT('Origin',(-0.0043684998350524,-0.0341934771029004,
0.0853884053149871));
#69741=CARTESIAN_POINT('',(0.00376544772787017,-0.034193496108874,0.0779027384253525));
#69742=CARTESIAN_POINT('',(0.00380724846052817,-0.034193496108884,0.0779492029144924));
#69743=CARTESIAN_POINT('',(0.00361494791102639,-0.0345211942962673,0.0777205095457931));
#69744=CARTESIAN_POINT('Origin',(0.0168232715116394,-0.0345625596118009,
0.0673342682550502));
#69745=CARTESIAN_POINT('',(0.00361601294806193,-0.0346945769586885,0.0777196661515349));
#69746=CARTESIAN_POINT('Origin',(-0.00505738028098554,-0.0346945685853854,
0.0845880549798203));
#69747=CARTESIAN_POINT('',(0.00365481366711216,-0.0346945769587026,0.077768663643341));
#69748=CARTESIAN_POINT('Ctrl Pts',(0.00327763515248835,-0.0345231616327842,
0.0776876346420627));
#69749=CARTESIAN_POINT('Ctrl Pts',(0.003326396465438,-0.0344132092796988,
0.0777544319561883));
#69750=CARTESIAN_POINT('Ctrl Pts',(0.00337653691228175,-0.034303273855898,
0.0778202172345836));
#69751=CARTESIAN_POINT('Ctrl Pts',(0.00342799009848597,-0.034193496108874,
0.077884907844126));
#69752=CARTESIAN_POINT('Ctrl Pts',(0.00339045221434589,-0.0345231616327842,
0.0776982857777953));
#69753=CARTESIAN_POINT('Ctrl Pts',(0.00343936033820601,-0.0344132092796988,
0.077763528067557));
#69754=CARTESIAN_POINT('Ctrl Pts',(0.00348961542393308,-0.034303273855898,
0.0778277553651525));
#69755=CARTESIAN_POINT('Ctrl Pts',(0.00354115098125492,-0.034193496108874,
0.0778908870371748));
#69756=CARTESIAN_POINT('Ctrl Pts',(0.00350326927620343,-0.0345231616327842,
0.0777089369135279));
#69757=CARTESIAN_POINT('Ctrl Pts',(0.00355232421097402,-0.0344132092796988,
0.0777726241789256));
#69758=CARTESIAN_POINT('Ctrl Pts',(0.00360269393558442,-0.034303273855898,
0.0778352934957214));
#69759=CARTESIAN_POINT('Ctrl Pts',(0.00365431186402386,-0.034193496108874,
0.0778968662302236));
#69760=CARTESIAN_POINT('Ctrl Pts',(0.00361608633806097,-0.0345231616327842,
0.0777195880492606));
#69761=CARTESIAN_POINT('Ctrl Pts',(0.00366528808374204,-0.0344132092796988,
0.0777817202902942));
#69762=CARTESIAN_POINT('Ctrl Pts',(0.00371577244723576,-0.034303273855898,
0.0778428316262903));
#69763=CARTESIAN_POINT('Ctrl Pts',(0.00376747274679281,-0.034193496108874,
0.0779028454232725));
#69764=CARTESIAN_POINT('',(0.00359671891318807,-0.0341934961088839,0.0778938231347492));
#69765=CARTESIAN_POINT('Ctrl Pts',(0.00342002298478292,-0.0342105180195383,
0.0778748690246025));
#69766=CARTESIAN_POINT('Ctrl Pts',(0.00345371180452855,-0.0342610556241335,
0.0778481911196357));
#69767=CARTESIAN_POINT('Ctrl Pts',(0.00348679609582259,-0.0343122189870233,
0.07782199193588));
#69768=CARTESIAN_POINT('Ctrl Pts',(0.00355178462253462,-0.0344158119695144,
0.0777705280451103));
#69769=CARTESIAN_POINT('Ctrl Pts',(0.00358366227717941,-0.0344681990450042,
0.0777452843871966));
#69770=CARTESIAN_POINT('Ctrl Pts',(0.00361494791104364,-0.0345211942962462,
0.0777205095457699));
#69771=CARTESIAN_POINT('Ctrl Pts',(0.00369384830265547,-0.0346945769586932,
0.0778156470221916));
#69772=CARTESIAN_POINT('Ctrl Pts',(0.00376963296111065,-0.034529677707698,
0.0779072327708561));
#69773=CARTESIAN_POINT('Ctrl Pts',(0.00384913818567455,-0.034364806625142,
0.0779956080110687));
#69774=CARTESIAN_POINT('Ctrl Pts',(0.00369361438613664,-0.0346945769586932,
0.0778176611351202));
#69775=CARTESIAN_POINT('Ctrl Pts',(0.00376944068495148,-0.034529677707698,
0.0779092517198432));
#69776=CARTESIAN_POINT('Ctrl Pts',(0.00384898771417262,-0.034364806625142,
0.0779976300709476));
#69777=CARTESIAN_POINT('Ctrl Pts',(0.00365462984961993,-0.0346945769586932,
0.078153333277506));
#69778=CARTESIAN_POINT('Ctrl Pts',(0.00373739593246461,-0.034529677707698,
0.0782457298399369));
#69779=CARTESIAN_POINT('Ctrl Pts',(0.00382391012755614,-0.034364806625142,
0.0783346266524003));
#69780=CARTESIAN_POINT('',(0.0036631912365639,-0.0346775396664992,0.0781628703332946));
#69781=CARTESIAN_POINT('',(0.00365462984962341,-0.0346945769586885,0.078153333277498));
#69782=CARTESIAN_POINT('Origin',(0.0159026830614759,-0.0345626618374433,
0.0669464651399987));
#69783=CARTESIAN_POINT('Ctrl Pts',(0.00366319123623208,-0.0346775396670096,
0.0781628703314963));
#69784=CARTESIAN_POINT('Ctrl Pts',(0.0036951277090955,-0.0346269749928201,
0.0781341393846126));
#69785=CARTESIAN_POINT('Ctrl Pts',(0.00372649657555011,-0.0345757902890816,
0.0781059190240606));
#69786=CARTESIAN_POINT('Ctrl Pts',(0.00378812504502702,-0.0344721681087921,
0.0780504763626206));
#69787=CARTESIAN_POINT('Ctrl Pts',(0.0038183604905615,-0.034419771428953,
0.0780232758020536));
#69788=CARTESIAN_POINT('Ctrl Pts',(0.00384803921475855,-0.034366772783067,
0.0779965760079231));
#69789=CARTESIAN_POINT('',(0.0036741221178929,-0.0346945769587026,0.0779854972063226));
#69790=CARTESIAN_POINT('Origin',(0.00812378219310841,-0.0315241814719618,
0.07415));
#69791=CARTESIAN_POINT('',(0.00366319123793398,-0.0347116136489784,0.0781628703330552));
#69792=CARTESIAN_POINT('',(0.00367177297545972,-0.0346945769586885,0.0781723890818771));
#69793=CARTESIAN_POINT('Origin',(0.0158710147657852,-0.034562667817165,
0.0669140540721872));
#69794=CARTESIAN_POINT('Origin',(0.0161069622412668,-0.034562663129058,
0.0671735309468892));
#69795=CARTESIAN_POINT('Origin',(0.0161358505580842,-0.0345626691923073,
0.0672084428109901));
#69796=CARTESIAN_POINT('Ctrl Pts',(0.00374030229525091,-0.0352450361874067,
0.0778734213582005));
#69797=CARTESIAN_POINT('Ctrl Pts',(0.00388073343614336,-0.0349452760959492,
0.0780387470154162));
#69798=CARTESIAN_POINT('Ctrl Pts',(0.00403321863190598,-0.034644428984174,
0.0781930251517135));
#69799=CARTESIAN_POINT('Ctrl Pts',(0.00374197922941375,-0.0352450361874067,
0.0778753090861507));
#69800=CARTESIAN_POINT('Ctrl Pts',(0.00388248156713411,-0.0349452760959492,
0.0780405714967564));
#69801=CARTESIAN_POINT('Ctrl Pts',(0.00403503299346854,-0.034644428984174,
0.0781947812032845));
#69802=CARTESIAN_POINT('Ctrl Pts',(0.00390801231484276,-0.0352450361874067,
0.0780622128435846));
#69803=CARTESIAN_POINT('Ctrl Pts',(0.0040555638434466,-0.0349452760959492,
0.0782212132136182));
#69804=CARTESIAN_POINT('Ctrl Pts',(0.00421467275213715,-0.034644428984174,
0.0783686476954718));
#69805=CARTESIAN_POINT('Ctrl Pts',(0.00390967264569706,-0.0352450361874067,
0.078064081881159));
#69806=CARTESIAN_POINT('Ctrl Pts',(0.00405729466620972,-0.0349452760959492,
0.0782230196307868));
#69807=CARTESIAN_POINT('Ctrl Pts',(0.00421646914972384,-0.034644428984174,
0.0783703863603937));
#69808=CARTESIAN_POINT('',(0.00393262676926531,-0.0351951634053276,0.0780885744268352));
#69809=CARTESIAN_POINT('',(0.00409800492289777,-0.0348678972925388,0.0782574617917464));
#69810=CARTESIAN_POINT('Origin',(0.0155205695846266,-0.0345636767882058,
0.066000395172796));
#69811=CARTESIAN_POINT('Origin',(-0.00363654968017413,-0.0346946199341113,
0.0861489543183961));
#69812=CARTESIAN_POINT('',(0.0040096842883074,-0.0346945769330289,0.0781689953256754));
#69813=CARTESIAN_POINT('',(0.00405432007213583,-0.0346945769458128,0.0782127434443747));
#69814=CARTESIAN_POINT('',(0.00384803921487524,-0.0350221583435276,0.0779965760078401));
#69815=CARTESIAN_POINT('Origin',(0.0158916819271418,-0.0345628458718783,
0.0663060404294573));
#69816=CARTESIAN_POINT('',(0.00384895673138347,-0.035195136029876,0.0779957465163086));
#69817=CARTESIAN_POINT('Origin',(-0.00434289989842977,-0.0351951838366823,
0.085365368543244));
#69818=CARTESIAN_POINT('',(0.00393265065837624,-0.0351951371328748,0.0780885963819501));
#69819=CARTESIAN_POINT('Ctrl Pts',(0.00350932844780378,-0.0350241211494342,
0.0779849467574502));
#69820=CARTESIAN_POINT('Ctrl Pts',(0.00356215326699826,-0.0349144232818962,
0.078048508965792));
#69821=CARTESIAN_POINT('Ctrl Pts',(0.0036163235806588,-0.0348045283579412,
0.07811101729242));
#69822=CARTESIAN_POINT('Ctrl Pts',(0.00367177298290972,-0.0346945769439158,
0.0781723890901229));
#69823=CARTESIAN_POINT('Ctrl Pts',(0.0036225917068556,-0.0350241211494342,
0.0779884930163202));
#69824=CARTESIAN_POINT('Ctrl Pts',(0.00367546537431199,-0.0349144232818962,
0.0780504950697084));
#69825=CARTESIAN_POINT('Ctrl Pts',(0.00372965231595476,-0.0348045283579412,
0.0781114412978262));
#69826=CARTESIAN_POINT('Ctrl Pts',(0.00378508603015364,-0.0346945769439158,
0.0781712510535197));
#69827=CARTESIAN_POINT('Ctrl Pts',(0.00373585496590742,-0.0350241211494342,
0.0779920392751902));
#69828=CARTESIAN_POINT('Ctrl Pts',(0.00378877748162572,-0.0349144232818962,
0.0780524811736247));
#69829=CARTESIAN_POINT('Ctrl Pts',(0.00384298105125072,-0.0348045283579412,
0.0781118653032324));
#69830=CARTESIAN_POINT('Ctrl Pts',(0.00389839907739756,-0.0346945769439158,
0.0781701130169165));
#69831=CARTESIAN_POINT('Ctrl Pts',(0.00384911822495923,-0.0350241211494342,
0.0779955855340602));
#69832=CARTESIAN_POINT('Ctrl Pts',(0.00390208958893945,-0.0349144232818962,
0.078054467277541));
#69833=CARTESIAN_POINT('Ctrl Pts',(0.00395630978654668,-0.0348045283579412,
0.0781122893086386));
#69834=CARTESIAN_POINT('Ctrl Pts',(0.00401171212464148,-0.0346945769439158,
0.0781689749803132));
#69835=CARTESIAN_POINT('',(0.00384072863162498,-0.0346945769458128,0.0781706922036303));
#69836=CARTESIAN_POINT('Ctrl Pts',(0.00366319124037487,-0.0347116136492789,
0.0781628703308502));
#69837=CARTESIAN_POINT('Ctrl Pts',(0.00369511503917859,-0.0347621546532298,
0.0781341508032303));
#69838=CARTESIAN_POINT('Ctrl Pts',(0.00372647753133189,-0.0348133084097032,
0.0781059362425147));
#69839=CARTESIAN_POINT('Ctrl Pts',(0.00378810607647596,-0.0349168561544566,
0.0780504935079169));
#69840=CARTESIAN_POINT('Ctrl Pts',(0.00381834768455198,-0.0349692089015916,
0.0780232873253524));
#69841=CARTESIAN_POINT('Ctrl Pts',(0.00384803921491572,-0.0350221583435,
0.0779965760078304));
#69842=CARTESIAN_POINT('Ctrl Pts',(0.00393272785366326,-0.0351951371254888,
0.0780871354025537));
#69843=CARTESIAN_POINT('Ctrl Pts',(0.00401412565786805,-0.0350307338980928,
0.0781737828214646));
#69844=CARTESIAN_POINT('Ctrl Pts',(0.00409903513944573,-0.0348659306897824,
0.0782569919415866));
#69845=CARTESIAN_POINT('Ctrl Pts',(0.0039326506584598,-0.0351951371254888,
0.0780885963818693));
#69846=CARTESIAN_POINT('Ctrl Pts',(0.0040140786674953,-0.0350307338980928,
0.0781752453967426));
#69847=CARTESIAN_POINT('Ctrl Pts',(0.00409901839405667,-0.0348659306897824,
0.0782584548630651));
#69848=CARTESIAN_POINT('Ctrl Pts',(0.00391971266190752,-0.0351951371254888,
0.0783334580378068));
#69849=CARTESIAN_POINT('Ctrl Pts',(0.00400620303204808,-0.0350307338980928,
0.0784203745376411));
#69850=CARTESIAN_POINT('Ctrl Pts',(0.00409621184939875,-0.0348659306897825,
0.0785036420275136));
#69851=CARTESIAN_POINT('Origin',(0.000375438335953373,-0.0308609197411229,
0.0820555606426193));
#69852=CARTESIAN_POINT('',(0.00392700998367615,-0.0351951371254888,0.0781953505429598));
#69853=CARTESIAN_POINT('Origin',(0.00869940585763844,-0.035184046744121,
0.0733604412332708));
#69854=CARTESIAN_POINT('Origin',(0.000334508268153806,-0.0352322613438187,
0.0832326488377673));
#69855=CARTESIAN_POINT('',(0.00427040897049458,-0.0351951142564664,0.0784195818753924));
#69856=CARTESIAN_POINT('',(0.00436474671210107,-0.0351951372916787,0.0785011093128683));
#69857=CARTESIAN_POINT('Origin',(0.00845998783042524,-0.0352875122321978,
0.0742045170014701));
#69858=CARTESIAN_POINT('Origin',(0.00349033402313407,-0.0298325076522552,
0.0682486147103869));
#69859=CARTESIAN_POINT('Origin',(0.000660065224870908,-0.0338732569609108,
0.0779634230108649));
#69860=CARTESIAN_POINT('Ctrl Pts',(0.00249663926781917,-0.0321934096636942,
0.0753388642662976));
#69861=CARTESIAN_POINT('Ctrl Pts',(0.00251791937205675,-0.0320508460843224,
0.0754395874450527));
#69862=CARTESIAN_POINT('Ctrl Pts',(0.00254188966409757,-0.0319086045660874,
0.0755396629237864));
#69863=CARTESIAN_POINT('Ctrl Pts',(0.00256848079202786,-0.0317669892864618,
0.0756388794714287));
#69864=CARTESIAN_POINT('Ctrl Pts',(0.00251575093390584,-0.0321934096636942,
0.0754205048006375));
#69865=CARTESIAN_POINT('Ctrl Pts',(0.00253849236483141,-0.0320508460843224,
0.0755208858896705));
#69866=CARTESIAN_POINT('Ctrl Pts',(0.00256391369043927,-0.0319086045660874,
0.0756205802736542));
#69867=CARTESIAN_POINT('Ctrl Pts',(0.00259194250203898,-0.0317669892864618,
0.0757193777992968));
#69868=CARTESIAN_POINT('Ctrl Pts',(0.00253486259999249,-0.0321934096636942,
0.0755021453349773));
#69869=CARTESIAN_POINT('Ctrl Pts',(0.00255906535760608,-0.0320508460843224,
0.0756021843342883));
#69870=CARTESIAN_POINT('Ctrl Pts',(0.00258593771678096,-0.0319086045660874,
0.0757014976235219));
#69871=CARTESIAN_POINT('Ctrl Pts',(0.00261540421205009,-0.0317669892864618,
0.0757998761271649));
#69872=CARTESIAN_POINT('Ctrl Pts',(0.00255397426607915,-0.0321934096636942,
0.0755837858693173));
#69873=CARTESIAN_POINT('Ctrl Pts',(0.00257963835038075,-0.0320508460843224,
0.075683482778906));
#69874=CARTESIAN_POINT('Ctrl Pts',(0.00260796174312265,-0.0319086045660874,
0.0757824149733896));
#69875=CARTESIAN_POINT('Ctrl Pts',(0.0026388659220612,-0.0317669892864618,
0.075880374455033));
#69876=CARTESIAN_POINT('',(0.00255363235459846,-0.0321934096636942,0.0755823253040244));
#69877=CARTESIAN_POINT('',(0.00261718187036008,-0.0318665617511284,0.0758099632148273));
#69878=CARTESIAN_POINT('Origin',(0.0188791517298509,-0.0326371944422352,
0.0720192757713647));
#69879=CARTESIAN_POINT('Origin',(-0.00787753306643577,-0.0316939261509106,
0.0789735922318573));
#69880=CARTESIAN_POINT('',(0.00252392351269698,-0.0320197221621786,0.0754611719665832));
#69881=CARTESIAN_POINT('Ctrl Pts',(0.00252391834733507,-0.0320197392094706,
0.0754613568670933));
#69882=CARTESIAN_POINT('Ctrl Pts',(0.0025305909983687,-0.0319792716576002,
0.075489850763948));
#69883=CARTESIAN_POINT('Ctrl Pts',(0.00253751125185122,-0.0319386439829642,
0.0755184235062629));
#69884=CARTESIAN_POINT('Ctrl Pts',(0.00254469459260698,-0.0318979099381574,
0.0755471030991781));
#69885=CARTESIAN_POINT('Ctrl Pts',(0.00255187779137879,-0.0318571766984887,
0.0755757821252203));
#69886=CARTESIAN_POINT('Ctrl Pts',(0.00255928582901695,-0.0318163871833547,
0.0756044226649795));
#69887=CARTESIAN_POINT('Ctrl Pts',(0.00256688981595761,-0.0317755399638303,
0.0756329270885448));
#69888=CARTESIAN_POINT('',(0.00252514070879166,-0.0321934096636184,0.0754606157064861));
#69889=CARTESIAN_POINT('Origin',(0.000283209708318734,-0.0324111556700518,
0.0760070347756993));
#69890=CARTESIAN_POINT('',(0.00253938653170505,-0.0321934096636663,0.0755214705052652));
#69891=CARTESIAN_POINT('Ctrl Pts',(0.00255470187769009,-0.0321934096636618,
0.0755806019910128));
#69892=CARTESIAN_POINT('Ctrl Pts',(0.00257443099409214,-0.0320835708272592,
0.0756574039488498));
#69893=CARTESIAN_POINT('Ctrl Pts',(0.00259573807933072,-0.0319739230346488,
0.0757337530653914));
#69894=CARTESIAN_POINT('Ctrl Pts',(0.00261858837554064,-0.0318646057455573,
0.0758095537494409));
#69895=CARTESIAN_POINT('Ctrl Pts',(0.00249494653323593,-0.0321934096636618,
0.0756768852376034));
#69896=CARTESIAN_POINT('Ctrl Pts',(0.00251600347064723,-0.0320835708272592,
0.075754511268211));
#69897=CARTESIAN_POINT('Ctrl Pts',(0.00253865466084808,-0.0319739230346488,
0.0758316565003408));
#69898=CARTESIAN_POINT('Ctrl Pts',(0.00256286354811148,-0.0318646057455573,
0.0759082244562026));
#69899=CARTESIAN_POINT('Ctrl Pts',(0.00243519118878176,-0.0321934096636618,
0.0757731684841941));
#69900=CARTESIAN_POINT('Ctrl Pts',(0.00245757594720233,-0.0320835708272592,
0.0758516185875722));
#69901=CARTESIAN_POINT('Ctrl Pts',(0.00248157124236545,-0.0319739230346488,
0.0759295599352901));
#69902=CARTESIAN_POINT('Ctrl Pts',(0.00250713872068231,-0.0318646057455573,
0.0760068951629643));
#69903=CARTESIAN_POINT('Ctrl Pts',(0.0023754358443276,-0.0321934096636618,
0.0758694517307847));
#69904=CARTESIAN_POINT('Ctrl Pts',(0.00239914842375743,-0.0320835708272592,
0.0759487259069335));
#69905=CARTESIAN_POINT('Ctrl Pts',(0.00242448782388281,-0.0319739230346488,
0.0760274633702395));
#69906=CARTESIAN_POINT('Ctrl Pts',(0.00245141389325315,-0.0318646057455573,
0.076105565869726));
#69907=CARTESIAN_POINT('',(0.00237912173945756,-0.0321763980308272,0.075881726378492));
#69908=CARTESIAN_POINT('',(0.00237543584433933,-0.0321934096636185,0.0758694517308122));
#69909=CARTESIAN_POINT('Origin',(0.0183887770136759,-0.0326386230590182,
0.0716963916098026));
#69910=CARTESIAN_POINT('Ctrl Pts',(0.00237912174249056,-0.0321763980306293,
0.0758817263775713));
#69911=CARTESIAN_POINT('Ctrl Pts',(0.00242021415404723,-0.0321259596175519,
0.0758693390809465));
#69912=CARTESIAN_POINT('Ctrl Pts',(0.00246059458625344,-0.03207491646328,
0.075857166410302));
#69913=CARTESIAN_POINT('Ctrl Pts',(0.00253996398903856,-0.0319716057793918,
0.0758332405247676));
#69914=CARTESIAN_POINT('Ctrl Pts',(0.00257892203447221,-0.0319193786690113,
0.0758214966322547));
#69915=CARTESIAN_POINT('Ctrl Pts',(0.00261718187213179,-0.0318665617525305,
0.075809963214284));
#69916=CARTESIAN_POINT('',(0.0024645340994789,-0.0321934096636664,0.0757258885174283));
#69917=CARTESIAN_POINT('Origin',(0.00812378219310841,-0.0315241814719618,
0.07415));
#69918=CARTESIAN_POINT('',(0.00237912173910149,-0.0322104233323771,0.0758817263785991));
#69919=CARTESIAN_POINT('',(0.002382833841471,-0.0321934096636183,0.0758939931260947));
#69920=CARTESIAN_POINT('Origin',(0.0183818702993081,-0.0326387227710374,
0.0716515854926586));
#69921=CARTESIAN_POINT('Origin',(0.018034639889298,-0.0326386247628077,
0.0705216006089351));
#69922=CARTESIAN_POINT('Origin',(0.0180536409609535,-0.032638723939034,
0.070562761627751));
#69923=CARTESIAN_POINT('Ctrl Pts',(0.00257283702668973,-0.0327445246967098,
0.0756550358000437));
#69924=CARTESIAN_POINT('Ctrl Pts',(0.00262960037984349,-0.032443687833936,
0.0758643931195237));
#69925=CARTESIAN_POINT('Ctrl Pts',(0.00270197212326312,-0.0321434074405926,
0.0760688800292161));
#69926=CARTESIAN_POINT('Ctrl Pts',(0.00264348661759046,-0.0327445246967098,
0.0758948453813902));
#69927=CARTESIAN_POINT('Ctrl Pts',(0.00270929453696334,-0.032443687833936,
0.0761015381079892));
#69928=CARTESIAN_POINT('Ctrl Pts',(0.00279048444391856,-0.0321434074405926,
0.0763026867209342));
#69929=CARTESIAN_POINT('',(0.0026545602228832,-0.0326943950436612,0.0759292515393858));
#69930=CARTESIAN_POINT('',(0.00273227783999863,-0.0323666188837389,0.0761524499520336));
#69931=CARTESIAN_POINT('Origin',(0.0186171608058684,-0.0326395579111834,
0.0706563547216975));
#69932=CARTESIAN_POINT('Origin',(-0.00762128491708506,-0.0321933825603066,
0.0799978511097441));
#69933=CARTESIAN_POINT('',(0.00269003013365542,-0.0321934096532689,0.0760347980138639));
#69934=CARTESIAN_POINT('',(0.00271179075332963,-0.0321934096584274,0.0760933874820075));
#69935=CARTESIAN_POINT('',(0.00261718186944653,-0.0325210109756239,0.0758099632150888));
#69936=CARTESIAN_POINT('Origin',(0.0187415690246258,-0.0326393129157209,
0.0711207974251109));
#69937=CARTESIAN_POINT('',(0.00261848258998651,-0.0326943950436594,0.0758095711132296));
#69938=CARTESIAN_POINT('Origin',(-0.00797319251360476,-0.0326943765538147,
0.079002428014876));
#69939=CARTESIAN_POINT('',(0.00263652140644485,-0.0326943950436703,0.0758694113263177));
#69940=CARTESIAN_POINT('Ctrl Pts',(0.00231565842030428,-0.0325229783203769,
0.0756552236510969));
#69941=CARTESIAN_POINT('Ctrl Pts',(0.00233640789541759,-0.032413025309245,
0.0757352885102898));
#69942=CARTESIAN_POINT('Ctrl Pts',(0.00235881046792943,-0.0323031222208069,
0.0758149119965307));
#69943=CARTESIAN_POINT('Ctrl Pts',(0.0023828338427744,-0.0321934096576658,
0.0758939931303853));
#69944=CARTESIAN_POINT('Ctrl Pts',(0.0024166321497558,-0.0325229783203769,
0.075706657571782));
#69945=CARTESIAN_POINT('Ctrl Pts',(0.00243809064034096,-0.032413025309245,
0.0757853305103225));
#69946=CARTESIAN_POINT('Ctrl Pts',(0.00246117332712184,-0.0323031222208069,
0.0758635476201272));
#69947=CARTESIAN_POINT('Ctrl Pts',(0.00248584710742285,-0.0321934096576658,
0.0759412097539712));
#69948=CARTESIAN_POINT('Ctrl Pts',(0.00251760587920732,-0.0325229783203769,
0.075758091492467));
#69949=CARTESIAN_POINT('Ctrl Pts',(0.00253977338526434,-0.032413025309245,
0.0758353725103551));
#69950=CARTESIAN_POINT('Ctrl Pts',(0.00256353618631424,-0.0323031222208069,
0.0759121832437238));
#69951=CARTESIAN_POINT('Ctrl Pts',(0.0025888603720713,-0.0321934096576658,
0.0759884263775571));
#69952=CARTESIAN_POINT('Ctrl Pts',(0.00261857960865884,-0.0325229783203769,
0.075809525413152));
#69953=CARTESIAN_POINT('Ctrl Pts',(0.00264145613018772,-0.032413025309245,
0.0758854145103878));
#69954=CARTESIAN_POINT('Ctrl Pts',(0.00266589904550664,-0.0323031222208069,
0.0759608188673203));
#69955=CARTESIAN_POINT('Ctrl Pts',(0.00269187363671976,-0.0321934096576658,
0.0760356430011429));
#69956=CARTESIAN_POINT('',(0.00253643198727375,-0.0321934096584275,0.0759643955695672));
#69957=CARTESIAN_POINT('Ctrl Pts',(0.00237912174242734,-0.032210423332892,
0.0758817263775903));
#69958=CARTESIAN_POINT('Ctrl Pts',(0.00242026983492637,-0.032260942183143,
0.0758693222959601));
#69959=CARTESIAN_POINT('Ctrl Pts',(0.00246067746822554,-0.0323120888240864,
0.0758571414255604));
#69960=CARTESIAN_POINT('Ctrl Pts',(0.00254004747182089,-0.0324156524631809,
0.0758332153589119));
#69961=CARTESIAN_POINT('Ctrl Pts',(0.00257897721690126,-0.0324680267167309,
0.0758214799975259));
#69962=CARTESIAN_POINT('Ctrl Pts',(0.00261718186948933,-0.0325210109755912,
0.0758099632150805));
#69963=CARTESIAN_POINT('Origin',(0.00677672056911715,-0.0262834582511889,
0.0663983027135962));
#69964=CARTESIAN_POINT('Origin',(-0.00385709242765191,-0.0342770814131407,
0.0720806704906369));
#69965=CARTESIAN_POINT('Ctrl Pts',(0.0026555191950499,-0.0326943950436605,
0.0759274649047795));
#69966=CARTESIAN_POINT('Ctrl Pts',(0.00268001599276205,-0.0325844576448134,
0.0760028278175099));
#69967=CARTESIAN_POINT('Ctrl Pts',(0.00270607315274507,-0.0324744968375323,
0.076077689429851));
#69968=CARTESIAN_POINT('Ctrl Pts',(0.00273365596606139,-0.0323646534831895,
0.0761519542852319));
#69969=CARTESIAN_POINT('Ctrl Pts',(0.00260192751678469,-0.0326943950436605,
0.0760273100829432));
#69970=CARTESIAN_POINT('Ctrl Pts',(0.00262780036818173,-0.0325844576448134,
0.0761034115894416));
#69971=CARTESIAN_POINT('Ctrl Pts',(0.00265524895456519,-0.0324744968375323,
0.0761789833887758));
#69972=CARTESIAN_POINT('Ctrl Pts',(0.00268423677167008,-0.0323646534831895,
0.076253929139032));
#69973=CARTESIAN_POINT('Ctrl Pts',(0.00254833583851947,-0.0326943950436605,
0.0761271552611068));
#69974=CARTESIAN_POINT('Ctrl Pts',(0.00257558474360142,-0.0325844576448134,
0.0762039953613732));
#69975=CARTESIAN_POINT('Ctrl Pts',(0.0026044247563853,-0.0324744968375323,
0.0762802773477006));
#69976=CARTESIAN_POINT('Ctrl Pts',(0.00263481757727878,-0.0323646534831895,
0.0763559039928319));
#69977=CARTESIAN_POINT('Ctrl Pts',(0.00249474416025426,-0.0326943950436605,
0.0762270004392705));
#69978=CARTESIAN_POINT('Ctrl Pts',(0.00252336911902111,-0.0325844576448134,
0.0763045791333049));
#69979=CARTESIAN_POINT('Ctrl Pts',(0.00255360055820541,-0.0324744968375323,
0.0763815713066255));
#69980=CARTESIAN_POINT('Ctrl Pts',(0.00258539838288748,-0.0323646534831895,
0.0764578788466319));
#69981=CARTESIAN_POINT('',(0.00249919351341637,-0.0326773559991168,0.076239019426535));
#69982=CARTESIAN_POINT('',(0.00249474416025706,-0.0326943950436595,0.0762270004392665));
#69983=CARTESIAN_POINT('Origin',(0.0180478846633527,-0.0326395669977758,
0.0704105109512779));
#69984=CARTESIAN_POINT('Ctrl Pts',(0.00249919351655316,-0.0326773559987442,
0.0762390194253633));
#69985=CARTESIAN_POINT('Ctrl Pts',(0.00253945941403874,-0.0326267922586696,
0.076224064333202));
#69986=CARTESIAN_POINT('Ctrl Pts',(0.00257901162757038,-0.0325756109580818,
0.0762093743092491));
#69987=CARTESIAN_POINT('Ctrl Pts',(0.00265672234782972,-0.0324719985462368,
0.0761805118957437));
#69988=CARTESIAN_POINT('Ctrl Pts',(0.00269484968674601,-0.0324196091621767,
0.0761663510821778));
#69989=CARTESIAN_POINT('Ctrl Pts',(0.00273227784004436,-0.0323666188837757,
0.0761524499520166));
#69990=CARTESIAN_POINT('',(0.00257465219158013,-0.0326943950436703,0.0760781259893362));
#69991=CARTESIAN_POINT('Origin',(0.00812378219310841,-0.0315241814719618,
0.07415));
#69992=CARTESIAN_POINT('',(0.00249919351345739,-0.032711433837986,0.0762390194265195));
#69993=CARTESIAN_POINT('',(0.00250366852609158,-0.0326943950436593,0.0762510288836281));
#69994=CARTESIAN_POINT('Origin',(0.0180313865054977,-0.0326395661194546,
0.0703683094605398));
#69995=CARTESIAN_POINT('Origin',(0.0180828715748333,-0.0326395682947654,
0.0705047029332642));
#69996=CARTESIAN_POINT('Origin',(0.0180979155018327,-0.0326395673551978,
0.0705474446243651));
#69997=CARTESIAN_POINT('Ctrl Pts',(0.00267830514990377,-0.0332451089994434,
0.0760006498242324));
#69998=CARTESIAN_POINT('Ctrl Pts',(0.00274810354998636,-0.0329451141710254,
0.0762060293511019));
#69999=CARTESIAN_POINT('Ctrl Pts',(0.00283317368574278,-0.0326442513127492,
0.0764055679155792));
#70000=CARTESIAN_POINT('Ctrl Pts',(0.00276387470017103,-0.0332451089994434,
0.0762355494880615));
#70001=CARTESIAN_POINT('Ctrl Pts',(0.00284253248602208,-0.0329451141710254,
0.0764377017065412));
#70002=CARTESIAN_POINT('Ctrl Pts',(0.00293619374490576,-0.0326442513127492,
0.0766333548059177));
#70003=CARTESIAN_POINT('Ctrl Pts',(0.0027647303956737,-0.0332451089994434,
0.0762378984846998));
#70004=CARTESIAN_POINT('Ctrl Pts',(0.00284347677538243,-0.0329451141710254,
0.0764400184300957));
#70005=CARTESIAN_POINT('Ctrl Pts',(0.00293722394549739,-0.0326442513127492,
0.076635632674821));
#70006=CARTESIAN_POINT('',(0.00277707261164815,-0.0331951640388616,0.0762691558818365));
#70007=CARTESIAN_POINT('',(0.00286865161520751,-0.0328677532355005,0.0764870339490556));
#70008=CARTESIAN_POINT('Origin',(0.0180622871415354,-0.0326402808284701,
0.0693847921303757));
#70009=CARTESIAN_POINT('Origin',(-0.00723325094578848,-0.0326944278779115,
0.0809799113798173));
#70010=CARTESIAN_POINT('',(0.00281909985087197,-0.0326943950436593,0.0763722669164541));
#70011=CARTESIAN_POINT('',(0.00284449639327671,-0.0326943950436692,0.0764293744083929));
#70012=CARTESIAN_POINT('',(0.00273227783999764,-0.0330220786163545,0.0761524499520309));
#70013=CARTESIAN_POINT('Origin',(0.0182859405234867,-0.0326396682762467,
0.0698103879589332));
#70014=CARTESIAN_POINT('',(0.00273355137358273,-0.0331951640388588,0.0761519769509752));
#70015=CARTESIAN_POINT('Origin',(-0.00760786748069256,-0.0331952026560122,
0.0799928656019648));
#70016=CARTESIAN_POINT('',(0.00275531199262544,-0.0331951640388701,0.0762105664164158));
#70017=CARTESIAN_POINT('Ctrl Pts',(0.00242163349987949,-0.0330240426238172,
0.0760169494584312));
#70018=CARTESIAN_POINT('Ctrl Pts',(0.00244735254755011,-0.0329142774063519,
0.0760955021120148));
#70019=CARTESIAN_POINT('Ctrl Pts',(0.00247470831987959,-0.032804347972669,
0.076173562242403));
#70020=CARTESIAN_POINT('Ctrl Pts',(0.00250366852609159,-0.0326943950436592,
0.0762510288836281));
#70021=CARTESIAN_POINT('Ctrl Pts',(0.00252563752523012,-0.0330240426238172,
0.0760619416654831));
#70022=CARTESIAN_POINT('Ctrl Pts',(0.00255197638438667,-0.0329142774063519,
0.0761390615622913));
#70023=CARTESIAN_POINT('Ctrl Pts',(0.00257992265811595,-0.032804347972669,
0.0762156754083878));
#70024=CARTESIAN_POINT('Ctrl Pts',(0.00260944324813962,-0.0326943950436592,
0.0762916840697697));
#70025=CARTESIAN_POINT('Ctrl Pts',(0.00262964155058076,-0.0330240426238172,
0.0761069338725351));
#70026=CARTESIAN_POINT('Ctrl Pts',(0.00265660022122323,-0.0329142774063519,
0.0761826210125678));
#70027=CARTESIAN_POINT('Ctrl Pts',(0.0026851369963523,-0.032804347972669,
0.0762577885743726));
#70028=CARTESIAN_POINT('Ctrl Pts',(0.00271521797018765,-0.0326943950436592,
0.0763323392559112));
#70029=CARTESIAN_POINT('Ctrl Pts',(0.00273364557593139,-0.0330240426238172,
0.076151926079587));
#70030=CARTESIAN_POINT('Ctrl Pts',(0.00276122405805979,-0.0329142774063519,
0.0762261804628443));
#70031=CARTESIAN_POINT('Ctrl Pts',(0.00279035133458866,-0.032804347972669,
0.0762999017403575));
#70032=CARTESIAN_POINT('Ctrl Pts',(0.00282099269223568,-0.0326943950436592,
0.0763729944420527));
#70033=CARTESIAN_POINT('',(0.00266138418849177,-0.0326943950436693,0.0763116479000511));
#70034=CARTESIAN_POINT('Ctrl Pts',(0.00249919351656075,-0.0327114338383317,
0.0762390194253603));
#70035=CARTESIAN_POINT('Ctrl Pts',(0.00253945271657824,-0.0327619876831137,
0.0762240668206949));
#70036=CARTESIAN_POINT('Ctrl Pts',(0.0025790016587862,-0.0328131562604681,
0.076209378011739));
#70037=CARTESIAN_POINT('Ctrl Pts',(0.00265671230754119,-0.0329167375858765,
0.0761805156247909));
#70038=CARTESIAN_POINT('Ctrl Pts',(0.0026948430502022,-0.0329691088920619,
0.0761663535470457));
#70039=CARTESIAN_POINT('Ctrl Pts',(0.00273227784004319,-0.0330220786163186,
0.0761524499520169));
#70040=CARTESIAN_POINT('Ctrl Pts',(0.00277791764267319,-0.0331951640388604,
0.0762673122641001));
#70041=CARTESIAN_POINT('Ctrl Pts',(0.00282169171623913,-0.0330306422010619,
0.0763778345862308));
#70042=CARTESIAN_POINT('Ctrl Pts',(0.00286999638896757,-0.0328657861914645,
0.0764864532393173));
#70043=CARTESIAN_POINT('Ctrl Pts',(0.00277707261164708,-0.0331951640388604,
0.0762691558818335));
#70044=CARTESIAN_POINT('Ctrl Pts',(0.00282088480082764,-0.0330306422010619,
0.0763796956744389));
#70045=CARTESIAN_POINT('Ctrl Pts',(0.00286922827867427,-0.0328657861914645,
0.0764883302077133));
#70046=CARTESIAN_POINT('Ctrl Pts',(0.00263626771762459,-0.0331951640388604,
0.0765763521758829));
#70047=CARTESIAN_POINT('Ctrl Pts',(0.00268643099322868,-0.0330306422010619,
0.0766898030193965));
#70048=CARTESIAN_POINT('Ctrl Pts',(0.00274124044733536,-0.0328657861914645,
0.0768010836190257));
#70049=CARTESIAN_POINT('',(0.00264146296800414,-0.0331781648281909,0.0765880680691641));
#70050=CARTESIAN_POINT('',(0.00263626771762763,-0.0331951640388588,0.0765763521758782));
#70051=CARTESIAN_POINT('Origin',(0.0174347589091698,-0.0326412092064642,
0.0692297478366806));
#70052=CARTESIAN_POINT('Ctrl Pts',(0.00264146296835899,-0.033178164828644,
0.0765880680673543));
#70053=CARTESIAN_POINT('Ctrl Pts',(0.00268073738764738,-0.0331276811546776,
0.0765706021416561));
#70054=CARTESIAN_POINT('Ctrl Pts',(0.00271930261880876,-0.0330765663497784,
0.0765534515655876));
#70055=CARTESIAN_POINT('Ctrl Pts',(0.00279504790506716,-0.0329730614463218,
0.0765197665255157));
#70056=CARTESIAN_POINT('Ctrl Pts',(0.00283219736290148,-0.0329207133373851,
0.0765032456744304));
#70057=CARTESIAN_POINT('Ctrl Pts',(0.00286865160156484,-0.0328677532289363,
0.0764870339398219));
#70058=CARTESIAN_POINT('',(0.00270667016464789,-0.0331951640388702,0.0764227540288673));
#70059=CARTESIAN_POINT('Origin',(0.00812378219310841,-0.0315241814719618,
0.07415));
#70060=CARTESIAN_POINT('',(0.0026414629696845,-0.0332121607144215,0.0765880680691276));
#70061=CARTESIAN_POINT('',(0.00264668323176962,-0.0331951640388587,0.0765997728400264));
#70062=CARTESIAN_POINT('Origin',(0.0174094462810411,-0.0326413640761601,
0.0691921232523155));
#70063=CARTESIAN_POINT('Origin',(0.0180136125105183,-0.0326412103205533,
0.0705313689848069));
#70064=CARTESIAN_POINT('Origin',(0.0180245920194116,-0.0326413657162226,
0.0705753669552167));
#70065=CARTESIAN_POINT('Ctrl Pts',(0.00280524589058206,-0.0337436976235975,
0.076338903058317));
#70066=CARTESIAN_POINT('Ctrl Pts',(0.00282493321642591,-0.0336723290703325,
0.0763867387798682));
#70067=CARTESIAN_POINT('Ctrl Pts',(0.00284547777117999,-0.033601104548885,
0.0764342126497879));
#70068=CARTESIAN_POINT('Ctrl Pts',(0.00291107246486281,-0.0333736987606857,
0.0765857873123978));
#70069=CARTESIAN_POINT('Ctrl Pts',(0.00298525729179216,-0.0331450831799191,
0.0767333479902159));
#70070=CARTESIAN_POINT('Ctrl Pts',(0.00290539523114428,-0.0337436976235975,
0.0765679666075451));
#70071=CARTESIAN_POINT('Ctrl Pts',(0.00292714278926541,-0.0336723290703325,
0.0766149015707493));
#70072=CARTESIAN_POINT('Ctrl Pts',(0.00294973104119621,-0.033601104548885,
0.0766614377709584));
#70073=CARTESIAN_POINT('Ctrl Pts',(0.00302185085513068,-0.0333736987606857,
0.0768100186399245));
#70074=CARTESIAN_POINT('Ctrl Pts',(0.00310237824828838,-0.0331450831799191,
0.0769542160086103));
#70075=CARTESIAN_POINT('Ctrl Pts',(0.00290639672454991,-0.0337436976235975,
0.0765702572430374));
#70076=CARTESIAN_POINT('Ctrl Pts',(0.0029281648849938,-0.0336723290703325,
0.076617183198658));
#70077=CARTESIAN_POINT('Ctrl Pts',(0.00295077357389638,-0.033601104548885,
0.0766637100221701));
#70078=CARTESIAN_POINT('Ctrl Pts',(0.00302295863903336,-0.0333736987606857,
0.0768122609531998));
#70079=CARTESIAN_POINT('Ctrl Pts',(0.00310354945785334,-0.0331450831799191,
0.0769564246887942));
#70080=CARTESIAN_POINT('',(0.00292068602045762,-0.0336938721132548,0.0766006968841836));
#70081=CARTESIAN_POINT('',(0.00302576499310969,-0.0333679869945434,0.0768123947168798));
#70082=CARTESIAN_POINT('Ctrl Pts',(0.00292068602046224,-0.0336938721132647,
0.0766006968841961));
#70083=CARTESIAN_POINT('Ctrl Pts',(0.00293025224004404,-0.0336629187933931,
0.0766210070093736));
#70084=CARTESIAN_POINT('Ctrl Pts',(0.00293993432406981,-0.0336319952301038,
0.0766412546248275));
#70085=CARTESIAN_POINT('Ctrl Pts',(0.00294973104120162,-0.0336011045488948,
0.0766614377709706));
#70086=CARTESIAN_POINT('Ctrl Pts',(0.00297431435673327,-0.0335235892595452,
0.0767120841909275));
#70087=CARTESIAN_POINT('Ctrl Pts',(0.0029996633102178,-0.0334458668660368,
0.0767624145892694));
#70088=CARTESIAN_POINT('Ctrl Pts',(0.0030257649928217,-0.0333679869945383,
0.0768123947170223));
#70089=CARTESIAN_POINT('Ctrl Pts',(0.0030257849695321,-0.0333679692460369,
0.0768124344536474));
#70090=CARTESIAN_POINT('Ctrl Pts',(0.00302618395529592,-0.033339189537351,
0.0768122193997352));
#70091=CARTESIAN_POINT('Ctrl Pts',(0.00302648147390406,-0.0333104081057743,
0.0768120553479233));
#70092=CARTESIAN_POINT('Ctrl Pts',(0.00302687261701995,-0.033253269724522,
0.0768118333469244));
#70093=CARTESIAN_POINT('Ctrl Pts',(0.00302696921424088,-0.0332249166372877,
0.0768117738464262));
#70094=CARTESIAN_POINT('Ctrl Pts',(0.0030269692753617,-0.0331960985564874,
0.0768117660347441));
#70095=CARTESIAN_POINT('Ctrl Pts',(0.00302696924986029,-0.0331956312358587,
0.0768117659216277));
#70096=CARTESIAN_POINT('Ctrl Pts',(0.00302696919836504,-0.0331951640388587,
0.0768117658230233));
#70097=CARTESIAN_POINT('',(0.00296910472395193,-0.0331951640388587,0.07670096554053));
#70098=CARTESIAN_POINT('',(0.00299803696116874,-0.0331951640388687,0.0767563656817873));
#70099=CARTESIAN_POINT('',(0.00286865161539024,-0.0335216366567711,0.0764870339335403));
#70100=CARTESIAN_POINT('Origin',(0.0175538040129587,-0.0326434571528625,
0.0686310194173281));
#70101=CARTESIAN_POINT('',(0.00286989293566143,-0.0336938721132327,0.0764864819003116));
#70102=CARTESIAN_POINT('Origin',(-0.00710844836118518,-0.0336938867896263,
0.0809239963976862));
#70103=CARTESIAN_POINT('',(0.00289528947806953,-0.0336938721132538,0.0765435893922577));
#70104=CARTESIAN_POINT('Ctrl Pts',(0.00255011247002711,-0.0335235895815172,
0.0763713072317981));
#70105=CARTESIAN_POINT('Ctrl Pts',(0.0025806931374243,-0.0334144449262749,
0.0764480397690822));
#70106=CARTESIAN_POINT('Ctrl Pts',(0.00261289417477601,-0.0333049234473147,
0.0765242286891813));
#70107=CARTESIAN_POINT('Ctrl Pts',(0.00264668323176944,-0.0331951640388587,
0.0765997728400264));
#70108=CARTESIAN_POINT('Ctrl Pts',(0.00265673650893439,-0.0335235895815172,
0.0764096802276814));
#70109=CARTESIAN_POINT('Ctrl Pts',(0.00268784545616939,-0.0334144449262749,
0.0764849448751466));
#70110=CARTESIAN_POINT('Ctrl Pts',(0.00272054505478949,-0.0333049234473147,
0.0765596533051353));
#70111=CARTESIAN_POINT('Ctrl Pts',(0.00275480214549061,-0.0331951640388587,
0.0766337062009227));
#70112=CARTESIAN_POINT('Ctrl Pts',(0.00276336054784166,-0.0335235895815172,
0.0764480532235648));
#70113=CARTESIAN_POINT('Ctrl Pts',(0.00279499777491448,-0.0334144449262749,
0.0765218499812109));
#70114=CARTESIAN_POINT('Ctrl Pts',(0.00282819593480297,-0.0333049234473147,
0.0765950779210892));
#70115=CARTESIAN_POINT('Ctrl Pts',(0.00286292105921177,-0.0331951640388587,
0.076667639561819));
#70116=CARTESIAN_POINT('Ctrl Pts',(0.00286998458674894,-0.0335235895815172,
0.0764864262194482));
#70117=CARTESIAN_POINT('Ctrl Pts',(0.00290215009365957,-0.0334144449262749,
0.0765587550872753));
#70118=CARTESIAN_POINT('Ctrl Pts',(0.00293584681481645,-0.0333049234473147,
0.0766305025370432));
#70119=CARTESIAN_POINT('Ctrl Pts',(0.00297103997293294,-0.0331951640388587,
0.0767015729227154));
#70120=CARTESIAN_POINT('',(0.00280789397787078,-0.0331951640388687,0.0766503691902882));
#70121=CARTESIAN_POINT('Ctrl Pts',(0.00264146297254081,-0.0332121607145971,
0.0765880680678471));
#70122=CARTESIAN_POINT('Ctrl Pts',(0.00268067132715015,-0.0332625444110019,
0.0765706315353287));
#70123=CARTESIAN_POINT('Ctrl Pts',(0.0027192040602785,-0.0333135300747347,
0.0765534954616293));
#70124=CARTESIAN_POINT('Ctrl Pts',(0.0027949488702927,-0.0334167203140606,
0.0765198106295043));
#70125=CARTESIAN_POINT('Ctrl Pts',(0.00283213161064489,-0.0334688847587302,
0.076503274917467));
#70126=CARTESIAN_POINT('Ctrl Pts',(0.0028686516160965,-0.033521636656238,
0.0764870339333968));
#70127=CARTESIAN_POINT('Ctrl Pts',(0.00292104473773195,-0.033693872113239,
0.0765997635906665));
#70128=CARTESIAN_POINT('Ctrl Pts',(0.00293538401694588,-0.0336474569764958,
0.0766302169394442));
#70129=CARTESIAN_POINT('Ctrl Pts',(0.00295007880852096,-0.033601104548885,
0.076660500342171));
#70130=CARTESIAN_POINT('Ctrl Pts',(0.00298728264224462,-0.0334837508592656,
0.0767371709552845));
#70131=CARTESIAN_POINT('Ctrl Pts',(0.00302674204801737,-0.0333660264659097,
0.0768127054735856));
#70132=CARTESIAN_POINT('Ctrl Pts',(0.0029206860204489,-0.033693872113239,
0.0766006968841651));
#70133=CARTESIAN_POINT('Ctrl Pts',(0.00293503076253938,-0.0336474569764958,
0.076631152332634));
#70134=CARTESIAN_POINT('Ctrl Pts',(0.00294973104119621,-0.033601104548885,
0.0766614377709584));
#70135=CARTESIAN_POINT('Ctrl Pts',(0.00298694876694935,-0.0334837508592656,
0.0767381135377368));
#70136=CARTESIAN_POINT('Ctrl Pts',(0.00302642221136499,-0.0333660264659097,
0.0768136527957902));
#70137=CARTESIAN_POINT('Ctrl Pts',(0.00279872055942052,-0.033693872113239,
0.0769180207969077));
#70138=CARTESIAN_POINT('Ctrl Pts',(0.00281492270367152,-0.0336474569764958,
0.0769491901496925));
#70139=CARTESIAN_POINT('Ctrl Pts',(0.00283148861436989,-0.033601104548885,
0.0769801677001781));
#70140=CARTESIAN_POINT('Ctrl Pts',(0.00287342969151647,-0.0334837508592656,
0.0770585957358222));
#70141=CARTESIAN_POINT('Ctrl Pts',(0.00291767633653727,-0.0333660264659097,
0.0771357465305788));
#70142=CARTESIAN_POINT('',(0.00280536863337681,-0.0336769361243753,0.0769274947718516));
#70143=CARTESIAN_POINT('',(0.00279944798762601,-0.0336938721132327,0.0769161282089466));
#70144=CARTESIAN_POINT('Ctrl Pts',(0.00280536863337695,-0.033676936124375,
0.0769274947718519));
#70145=CARTESIAN_POINT('Ctrl Pts',(0.00280437976177307,-0.0336797586669909,
0.0769256012568036));
#70146=CARTESIAN_POINT('Ctrl Pts',(0.00280339193879104,-0.0336825812712615,
0.0769237072852676));
#70147=CARTESIAN_POINT('Ctrl Pts',(0.00280141839210353,-0.0336882265959168,
0.076919918434235));
#70148=CARTESIAN_POINT('Ctrl Pts',(0.00280043266840231,-0.0336910493162576,
0.0769180235547777));
#70149=CARTESIAN_POINT('Ctrl Pts',(0.00279944798762285,-0.0336938721132349,
0.0769161282089515));
#70150=CARTESIAN_POINT('Ctrl Pts',(0.00280536863337684,-0.0336769361243753,
0.0769274947718516));
#70151=CARTESIAN_POINT('Ctrl Pts',(0.0028425210803906,-0.0336279007516201,
0.0769080922326953));
#70152=CARTESIAN_POINT('Ctrl Pts',(0.00288020252032072,-0.0335767878632067,
0.0768884134316338));
#70153=CARTESIAN_POINT('Ctrl Pts',(0.00295404756158169,-0.033473319885732,
0.0768498485073897));
#70154=CARTESIAN_POINT('Ctrl Pts',(0.00299025512618674,-0.0334209645014077,
0.0768309394247733));
#70155=CARTESIAN_POINT('Ctrl Pts',(0.00302576498972625,-0.0333679869844681,
0.0768123947104102));
#70156=CARTESIAN_POINT('',(0.00286006700405182,-0.0336938721132538,0.0767584125465751));
#70157=CARTESIAN_POINT('Origin',(0.00812378219310841,-0.0315241814719618,
0.07415));
#70158=CARTESIAN_POINT('',(0.00280536863453025,-0.0337108120655389,0.0769274947712568));
#70159=CARTESIAN_POINT('',(0.00281131354479959,-0.0336938721132327,0.07693884866222));
#70160=CARTESIAN_POINT('Origin',(0.0178253440299299,-0.0345562511534441,
0.0703442768603358));
#70161=CARTESIAN_POINT('Ctrl Pts',(0.00281131354480541,-0.0336938721132305,
0.0769388486622202));
#70162=CARTESIAN_POINT('Ctrl Pts',(0.002810320782198,-0.0336910493337498,
0.076936957551993));
#70163=CARTESIAN_POINT('Ctrl Pts',(0.00280932898901947,-0.0336882266046629,
0.0769350658347944));
#70164=CARTESIAN_POINT('Ctrl Pts',(0.00280734735042096,-0.033682581271302,
0.0769312812022592));
#70165=CARTESIAN_POINT('Ctrl Pts',(0.00280635750498768,-0.0336797586670112,
0.0769293882869132));
#70166=CARTESIAN_POINT('Ctrl Pts',(0.00280536863337669,-0.033676936124375,
0.0769274947718514));
#70167=CARTESIAN_POINT('Origin',(0.0167906271279013,-0.0345562514784053,
0.0683629835414773));
#70168=CARTESIAN_POINT('Ctrl Pts',(0.00295316055523882,-0.034243627687391,
0.0766684909922402));
#70169=CARTESIAN_POINT('Ctrl Pts',(0.00304814700888272,-0.0339430054201809,
0.076863504202146));
#70170=CARTESIAN_POINT('Ctrl Pts',(0.00315755280998154,-0.0336441434784052,
0.0770508086310832));
#70171=CARTESIAN_POINT('Ctrl Pts',(0.00306749329711971,-0.034243627687391,
0.0768908151342806));
#70172=CARTESIAN_POINT('Ctrl Pts',(0.00317086484401067,-0.0339430054201809,
0.07708151621374));
#70173=CARTESIAN_POINT('Ctrl Pts',(0.00328830710985207,-0.0336441434784052,
0.0772638891629611));
#70174=CARTESIAN_POINT('Ctrl Pts',(0.00306863662453852,-0.034243627687391,
0.076893038375701));
#70175=CARTESIAN_POINT('Ctrl Pts',(0.00317209202236195,-0.0339430054201809,
0.0770836963338559));
#70176=CARTESIAN_POINT('Ctrl Pts',(0.00328961465285077,-0.0336441434784052,
0.0772660199682799));
#70177=CARTESIAN_POINT('',(0.00308483367277913,-0.034193496108874,0.0769225661055189));
#70178=CARTESIAN_POINT('',(0.0032029979098032,-0.033866421286425,0.0771272482330836));
#70179=CARTESIAN_POINT('Origin',(0.0179855814678328,-0.0345610720404878,
0.0693054236682199));
#70180=CARTESIAN_POINT('Origin',(-0.00617955990394535,-0.0336938005073058,
0.0828040724588024));
#70181=CARTESIAN_POINT('',(0.0031394527540545,-0.0336938721132327,0.0770195966690428));
#70182=CARTESIAN_POINT('',(0.00317180650376104,-0.0336938721132427,0.077073070820571));
#70183=CARTESIAN_POINT('',(0.00302576498972379,-0.0340203938281605,0.0768123947104055));
#70184=CARTESIAN_POINT('Origin',(0.018135931327103,-0.034558964324261,0.0697625140900591));
#70185=CARTESIAN_POINT('',(0.00302696919836559,-0.034193496108874,0.0768117658230245));
#70186=CARTESIAN_POINT('Origin',(-0.00674069408269382,-0.034193422071769,
0.0819128414261462));
#70187=CARTESIAN_POINT('',(0.00305590143558237,-0.034193496108884,0.0768671659642817));
#70188=CARTESIAN_POINT('Ctrl Pts',(0.00270058669856236,-0.0340223579322397,
0.0767168951338089));
#70189=CARTESIAN_POINT('Ctrl Pts',(0.00273599087720114,-0.0339125849573575,
0.0767916951439664));
#70190=CARTESIAN_POINT('Ctrl Pts',(0.00277291836413257,-0.0338030433565231,
0.0768657098087929));
#70191=CARTESIAN_POINT('Ctrl Pts',(0.00281131354479889,-0.0336938721132327,
0.0769388486622199));
#70192=CARTESIAN_POINT('Ctrl Pts',(0.00280940981634064,-0.0340223579322397,
0.0767484974892177));
#70193=CARTESIAN_POINT('Ctrl Pts',(0.00284524987388292,-0.0339125849573575,
0.0768217965447584));
#70194=CARTESIAN_POINT('Ctrl Pts',(0.00288258186715795,-0.0338030433565231,
0.0768943022879911));
#70195=CARTESIAN_POINT('Ctrl Pts',(0.00292134983536847,-0.0336938721132327,
0.0769659262283597));
#70196=CARTESIAN_POINT('Ctrl Pts',(0.00291823293411893,-0.0340223579322397,
0.0767800998446266));
#70197=CARTESIAN_POINT('Ctrl Pts',(0.00295450887056471,-0.0339125849573575,
0.0768518979455505));
#70198=CARTESIAN_POINT('Ctrl Pts',(0.00299224537018333,-0.0338030433565231,
0.0769228947671894));
#70199=CARTESIAN_POINT('Ctrl Pts',(0.00303138612593806,-0.0336938721132327,
0.0769930037944996));
#70200=CARTESIAN_POINT('Ctrl Pts',(0.00302705605189722,-0.0340223579322397,
0.0768117022000354));
#70201=CARTESIAN_POINT('Ctrl Pts',(0.00306376786724649,-0.0339125849573575,
0.0768819993463426));
#70202=CARTESIAN_POINT('Ctrl Pts',(0.00310190887320872,-0.0338030433565231,
0.0769514872463876));
#70203=CARTESIAN_POINT('Ctrl Pts',(0.00314142241650764,-0.0336938721132327,
0.0770200813606394));
#70204=CARTESIAN_POINT('',(0.00297538314943704,-0.0336938721132427,0.0769792226656414));
#70205=CARTESIAN_POINT('Ctrl Pts',(0.00280536863771951,-0.0337108120662681,
0.0769274947695836));
#70206=CARTESIAN_POINT('Ctrl Pts',(0.00284348327556921,-0.0337611408994431,
0.0769075897347138));
#70207=CARTESIAN_POINT('Ctrl Pts',(0.00288090240583828,-0.0338121088781598,
0.0768880479225696));
#70208=CARTESIAN_POINT('Ctrl Pts',(0.00295438373940751,-0.0339153382773233,
0.0768496729414733));
#70209=CARTESIAN_POINT('Ctrl Pts',(0.00299041485563483,-0.0339675558473109,
0.0768308560074719));
#70210=CARTESIAN_POINT('Ctrl Pts',(0.00302576498976157,-0.0340203938281304,
0.0768123947103918));
#70211=CARTESIAN_POINT('Ctrl Pts',(0.00308544100182471,-0.0341934961088741,
0.0769206310258527));
#70212=CARTESIAN_POINT('Ctrl Pts',(0.00314272161554826,-0.0340287516182428,
0.0770247947607176));
#70213=CARTESIAN_POINT('Ctrl Pts',(0.00320425845026947,-0.033864463327595,
0.0771265020384417));
#70214=CARTESIAN_POINT('Ctrl Pts',(0.00308483367277917,-0.0341934961088741,
0.0769225661055188));
#70215=CARTESIAN_POINT('Ctrl Pts',(0.00314215429275034,-0.0340287516182428,
0.0770267423964333));
#70216=CARTESIAN_POINT('Ctrl Pts',(0.00320373161848564,-0.033864463327595,
0.0771284605659895));
#70217=CARTESIAN_POINT('Ctrl Pts',(0.00298364097227414,-0.0341934961088741,
0.0772449875977058));
#70218=CARTESIAN_POINT('Ctrl Pts',(0.0030476274025888,-0.0340287516182428,
0.0773512559679823));
#70219=CARTESIAN_POINT('Ctrl Pts',(0.00311595131008736,-0.033864463327595,
0.0774547889262603));
#70220=CARTESIAN_POINT('',(0.00299026364761127,-0.0341764758832402,0.0772559599697467));
#70221=CARTESIAN_POINT('',(0.00298364097227651,-0.034193496108874,0.0772449875976981));
#70222=CARTESIAN_POINT('Origin',(0.0174219428488388,-0.0345621026098399,
0.0691228200665612));
#70223=CARTESIAN_POINT('Ctrl Pts',(0.00299026364751781,-0.0341764758837495,
0.0772559599679233));
#70224=CARTESIAN_POINT('Ctrl Pts',(0.00302698915521971,-0.0341260050040528,
0.0772337397230359));
#70225=CARTESIAN_POINT('Ctrl Pts',(0.00306307626717999,-0.0340749269148341,
0.0772119056857348));
#70226=CARTESIAN_POINT('Ctrl Pts',(0.00313400176244441,-0.0339715436306629,
0.0771689932616394));
#70227=CARTESIAN_POINT('Ctrl Pts',(0.0031688132413406,-0.0339192778237096,
0.0771479311599543));
#70228=CARTESIAN_POINT('Ctrl Pts',(0.0032029979078558,-0.0338664212855284,
0.0771272482321564));
#70229=CARTESIAN_POINT('',(0.00303423732253782,-0.0341934961088841,0.0770837768516186));
#70230=CARTESIAN_POINT('Origin',(0.00812378219310841,-0.0315241814719618,
0.07415));
#70231=CARTESIAN_POINT('',(0.00299026364867667,-0.0342105180190358,0.0772559599700854));
#70232=CARTESIAN_POINT('',(0.0029969097445483,-0.0341934961088739,0.0772669181728474));
#70233=CARTESIAN_POINT('Origin',(0.0174031147408198,-0.0345621700815362,
0.0690815872974236));
#70234=CARTESIAN_POINT('Origin',(0.0168917581452915,-0.0345621040926577,
0.0682465271175147));
#70235=CARTESIAN_POINT('Origin',(0.0169195395759662,-0.0345621714000146,
0.0682823430648086));
#70236=CARTESIAN_POINT('Ctrl Pts',(0.00313867625893174,-0.0346945769586966,
0.0770183132809271));
#70237=CARTESIAN_POINT('Ctrl Pts',(0.00319875422901076,-0.0345275153362943,
0.077122728320646));
#70238=CARTESIAN_POINT('Ctrl Pts',(0.00326213149522179,-0.0343603235965184,
0.0772252809705813));
#70239=CARTESIAN_POINT('Ctrl Pts',(0.0033286161078392,-0.0341934961088739,
0.0773256707113915));
#70240=CARTESIAN_POINT('Ctrl Pts',(0.00318207342367352,-0.0346945769586966,
0.0770900399458308));
#70241=CARTESIAN_POINT('Ctrl Pts',(0.00324365373746674,-0.0345275153362943,
0.0771935460145589));
#70242=CARTESIAN_POINT('Ctrl Pts',(0.003308505149674,-0.0343603235965184,
0.07729514221107));
#70243=CARTESIAN_POINT('Ctrl Pts',(0.00337643139274299,-0.0341934961088739,
0.0773945309095862));
#70244=CARTESIAN_POINT('Ctrl Pts',(0.00322547058841523,-0.0346945769586966,
0.0771617666107346));
#70245=CARTESIAN_POINT('Ctrl Pts',(0.00328855324592267,-0.0345275153362943,
0.0772643637084713));
#70246=CARTESIAN_POINT('Ctrl Pts',(0.00335487880412618,-0.0343603235965184,
0.0773650034515584));
#70247=CARTESIAN_POINT('Ctrl Pts',(0.00342424667764678,-0.0341934961088739,
0.0774633911077818));
#70248=CARTESIAN_POINT('Ctrl Pts',(0.00326886775315709,-0.0346945769586966,
0.0772334932756384));
#70249=CARTESIAN_POINT('Ctrl Pts',(0.00333345275437871,-0.0345275153362943,
0.0773351814023849));
#70250=CARTESIAN_POINT('Ctrl Pts',(0.00340125245857841,-0.0343603235965184,
0.0774348646920475));
#70251=CARTESIAN_POINT('Ctrl Pts',(0.00347206196255056,-0.0341934961088739,
0.0775322513059756));
#70252=CARTESIAN_POINT('',(0.00326886775284368,-0.0346945769586966,0.0772334932751199));
#70253=CARTESIAN_POINT('',(0.00339965091625427,-0.0343667727831474,0.0774303519139613));
#70254=CARTESIAN_POINT('Origin',(0.017362858530093,-0.0345626457066266,
0.068065250738478));
#70255=CARTESIAN_POINT('Origin',(-0.00567854003290058,-0.0341934771029006,
0.0837340891832016));
#70256=CARTESIAN_POINT('',(0.0033294716553295,-0.0341934961088739,0.0773269028104969));
#70257=CARTESIAN_POINT('',(0.00336511923205672,-0.0341934961088839,0.0773782399342499));
#70258=CARTESIAN_POINT('',(0.0032029979092189,-0.0345211942962679,0.077127248231385));
#70259=CARTESIAN_POINT('Origin',(0.0176089111386796,-0.034562559611928,
0.0684783474624671));
#70260=CARTESIAN_POINT('',(0.00320416025344759,-0.0346945769586885,0.0771265449720789));
#70261=CARTESIAN_POINT('Origin',(-0.00626167783094857,-0.0346945685853958,
0.082853710465351));
#70262=CARTESIAN_POINT('',(0.00323651400315563,-0.0346945769587025,0.0771800191236094));
#70263=CARTESIAN_POINT('Ctrl Pts',(0.00287246528051888,-0.0345231616327842,
0.0770523560573407));
#70264=CARTESIAN_POINT('Ctrl Pts',(0.00291247017257885,-0.0344132092796988,
0.077124738067718));
#70265=CARTESIAN_POINT('Ctrl Pts',(0.0029539701653608,-0.034303273855898,
0.0771962888738794));
#70266=CARTESIAN_POINT('Ctrl Pts',(0.00299690974454829,-0.0341934961088739,
0.0772669181728474));
#70267=CARTESIAN_POINT('Ctrl Pts',(0.0029830578048643,-0.0345231616327842,
0.0770770629328505));
#70268=CARTESIAN_POINT('Ctrl Pts',(0.00302340324641867,-0.0344132092796988,
0.0771479205809815));
#70269=CARTESIAN_POINT('Ctrl Pts',(0.00306521224089357,-0.034303273855898,
0.077217940059549));
#70270=CARTESIAN_POINT('Ctrl Pts',(0.00310842892835813,-0.0341934961088739,
0.0772870330375236));
#70271=CARTESIAN_POINT('Ctrl Pts',(0.00309365032920972,-0.0345231616327842,
0.0771017698083604));
#70272=CARTESIAN_POINT('Ctrl Pts',(0.00313433632025849,-0.0344132092796988,
0.0771711030942451));
#70273=CARTESIAN_POINT('Ctrl Pts',(0.00317645431642635,-0.034303273855898,
0.0772395912452187));
#70274=CARTESIAN_POINT('Ctrl Pts',(0.00321994811216796,-0.0341934961088739,
0.0773071479021997));
#70275=CARTESIAN_POINT('Ctrl Pts',(0.00320424285355514,-0.0345231616327842,
0.0771264766838702));
#70276=CARTESIAN_POINT('Ctrl Pts',(0.00324526939409831,-0.0344132092796988,
0.0771942856075086));
#70277=CARTESIAN_POINT('Ctrl Pts',(0.00328769639195912,-0.034303273855898,
0.0772612424308884));
#70278=CARTESIAN_POINT('Ctrl Pts',(0.00333146729597779,-0.0341934961088739,
0.0773272627668758));
#70279=CARTESIAN_POINT('',(0.0031631906999489,-0.0341934961088839,0.0772969104916822));
#70280=CARTESIAN_POINT('Ctrl Pts',(0.00299026365162846,-0.0342105180195383,
0.0772559599682917));
#70281=CARTESIAN_POINT('Ctrl Pts',(0.00302703045306284,-0.0342610556241344,
0.0772337147552873));
#70282=CARTESIAN_POINT('Ctrl Pts',(0.00306313749325517,-0.0343122189870244,
0.0772118687211287));
#70283=CARTESIAN_POINT('Ctrl Pts',(0.00313406370186486,-0.0344158119695154,
0.0771689558607066));
#70284=CARTESIAN_POINT('Ctrl Pts',(0.00316885386095482,-0.0344681990450055,
0.0771479065861105));
#70285=CARTESIAN_POINT('Ctrl Pts',(0.00320299790923847,-0.0345211942962474,
0.0771272482313646));
#70286=CARTESIAN_POINT('Ctrl Pts',(0.00326935226014221,-0.0346945769586932,
0.0772315243615793));
#70287=CARTESIAN_POINT('Ctrl Pts',(0.00333306059590116,-0.034529677707698,
0.0773318862655589));
#70288=CARTESIAN_POINT('Ctrl Pts',(0.00340086254339944,-0.0343648066251421,
0.0774295292874859));
#70289=CARTESIAN_POINT('Ctrl Pts',(0.00326886775283886,-0.0346945769586932,
0.0772334932751123));
#70290=CARTESIAN_POINT('Ctrl Pts',(0.00333261679449195,-0.034529677707698,
0.0773338651959376));
#70291=CARTESIAN_POINT('Ctrl Pts',(0.00340045982710713,-0.0343648066251421,
0.077431516543739));
#70292=CARTESIAN_POINT('Ctrl Pts',(0.00318811974601443,-0.0346945769586932,
0.0775616324843726));
#70293=CARTESIAN_POINT('Ctrl Pts',(0.00325865283363512,-0.034529677707698,
0.0776636738131036));
#70294=CARTESIAN_POINT('Ctrl Pts',(0.00333334311349819,-0.0343648066251421,
0.0777627127514686));
#70295=CARTESIAN_POINT('',(0.00319541831382511,-0.0346775396664988,0.0775721673639379));
#70296=CARTESIAN_POINT('',(0.00318811974601852,-0.0346945769586886,0.0775616324843668));
#70297=CARTESIAN_POINT('Origin',(0.0167441863132882,-0.0345626618330746,
0.067978222031336));
#70298=CARTESIAN_POINT('Ctrl Pts',(0.00319541831372028,-0.0346775396670096,
0.0775721673621132));
#70299=CARTESIAN_POINT('Ctrl Pts',(0.00323070390043304,-0.0346269749928193,
0.0775476656687395));
#70300=CARTESIAN_POINT('Ctrl Pts',(0.00326536236304662,-0.0345757902890807,
0.0775235993956254));
#70301=CARTESIAN_POINT('Ctrl Pts',(0.00333345368166626,-0.0344721681087968,
0.0774763180114924));
#70302=CARTESIAN_POINT('Ctrl Pts',(0.0033668598458875,-0.0344197714289659,
0.0774531214416305));
#70303=CARTESIAN_POINT('Ctrl Pts',(0.00339965091602227,-0.0343667727830658,
0.0774303519138172));
#70304=CARTESIAN_POINT('',(0.0032284937494411,-0.0346945769587026,0.0773975628797533));
#70305=CARTESIAN_POINT('Origin',(0.00812378219310841,-0.0315241814719618,
0.07415));
#70306=CARTESIAN_POINT('',(0.00319541831521432,-0.0347116136489601,0.0775721673638723));
#70307=CARTESIAN_POINT('',(0.00320273936760624,-0.0346945769586885,0.0775826866314311));
#70308=CARTESIAN_POINT('Origin',(0.0167168297805645,-0.034562667741533,
0.0679420974235828));
#70309=CARTESIAN_POINT('Origin',(0.0169183957182655,-0.0345626631704672,
0.0682291003233101));
#70310=CARTESIAN_POINT('Origin',(0.0169426807811622,-0.0345626691855843,
0.0682673575323138));
#70311=CARTESIAN_POINT('Ctrl Pts',(0.00330819890478178,-0.0352450361874069,
0.0772946653587965));
#70312=CARTESIAN_POINT('Ctrl Pts',(0.00342680190497358,-0.0349452760959493,
0.0774762880628058));
#70313=CARTESIAN_POINT('Ctrl Pts',(0.00355874853173212,-0.034644428984174,
0.0776484611325734));
#70314=CARTESIAN_POINT('Ctrl Pts',(0.00330962602076979,-0.0352450361874069,
0.0772967483770289));
#70315=CARTESIAN_POINT('Ctrl Pts',(0.00342830758328338,-0.0349452760959493,
0.0774783172564756));
#70316=CARTESIAN_POINT('Ctrl Pts',(0.00356032849489012,-0.034644428984174,
0.0776504307369548));
#70317=CARTESIAN_POINT('Ctrl Pts',(0.00345092463344402,-0.0352450361874069,
0.0775029878059855));
#70318=CARTESIAN_POINT('Ctrl Pts',(0.0035773846436591,-0.0349452760959493,
0.0776792275208075));
#70319=CARTESIAN_POINT('Ctrl Pts',(0.00371676049073153,-0.034644428984174,
0.0778454410717504));
#70320=CARTESIAN_POINT('Ctrl Pts',(0.00345233761957076,-0.0352450361874069,
0.077505050200275));
#70321=CARTESIAN_POINT('Ctrl Pts',(0.00357887541426286,-0.0349452760959493,
0.0776812366234508));
#70322=CARTESIAN_POINT('Ctrl Pts',(0.00371832481068995,-0.034644428984174,
0.0778473911750983));
#70323=CARTESIAN_POINT('',(0.00347204101307095,-0.0351951634053271,0.0775322265294441));
#70324=CARTESIAN_POINT('',(0.00361494791101335,-0.0348678972925388,0.0777205095457939));
#70325=CARTESIAN_POINT('Origin',(0.0164836600325524,-0.0345636767887041,
0.0669917205232383));
#70326=CARTESIAN_POINT('Origin',(-0.00504768341986911,-0.034694619934111,
0.0845803789055665));
#70327=CARTESIAN_POINT('',(0.00353841149926285,-0.0346945769330288,0.0776216711535067));
#70328=CARTESIAN_POINT('',(0.0035772122234248,-0.0346945769458128,0.0776706686523429));
#70329=CARTESIAN_POINT('',(0.00339965091614769,-0.0350221583435276,0.0774303519137499));
#70330=CARTESIAN_POINT('Origin',(0.0168135385341327,-0.0345628458717477,
0.067341468385268));
#70331=CARTESIAN_POINT('',(0.00340066516062048,-0.0351951360298761,0.0774296439583182));
#70332=CARTESIAN_POINT('Origin',(-0.0056502547616421,-0.0351951838366929,
0.0837144424795535));
#70333=CARTESIAN_POINT('',(0.00347206196210342,-0.0351951371328749,0.0775322513055353));
#70334=CARTESIAN_POINT('Ctrl Pts',(0.00306506851619793,-0.0350241211494343,
0.0773763626477927));
#70335=CARTESIAN_POINT('Ctrl Pts',(0.00310951033881109,-0.0349144232818962,
0.0774460443545387));
#70336=CARTESIAN_POINT('Ctrl Pts',(0.00315541913266755,-0.0348045283579412,
0.0775148491249152));
#70337=CARTESIAN_POINT('Ctrl Pts',(0.00320273937396406,-0.0346945769439157,
0.0775826866405456));
#70338=CARTESIAN_POINT('Ctrl Pts',(0.00317699419653077,-0.0350241211494343,
0.0773940765938533));
#70339=CARTESIAN_POINT('Ctrl Pts',(0.00322168002148792,-0.0349144232818962,
0.0774622165702441));
#70340=CARTESIAN_POINT('Ctrl Pts',(0.00326780109506742,-0.0348045283579412,
0.0775294736437625));
#70341=CARTESIAN_POINT('Ctrl Pts',(0.00331530154779286,-0.0346945769439157,
0.0775957594683171));
#70342=CARTESIAN_POINT('Ctrl Pts',(0.00328891987686361,-0.0350241211494343,
0.0774117905399139));
#70343=CARTESIAN_POINT('Ctrl Pts',(0.00333384970416474,-0.0349144232818962,
0.0774783887859494));
#70344=CARTESIAN_POINT('Ctrl Pts',(0.0033801830574673,-0.0348045283579412,
0.0775440981626099));
#70345=CARTESIAN_POINT('Ctrl Pts',(0.00342786372162167,-0.0346945769439157,
0.0776088322960885));
#70346=CARTESIAN_POINT('Ctrl Pts',(0.00340084555719646,-0.0350241211494343,
0.0774295044859745));
#70347=CARTESIAN_POINT('Ctrl Pts',(0.00344601938684157,-0.0349144232818962,
0.0774945610016548));
#70348=CARTESIAN_POINT('Ctrl Pts',(0.00349256501986717,-0.0348045283579412,
0.0775587226814572));
#70349=CARTESIAN_POINT('Ctrl Pts',(0.00354042589545047,-0.0346945769439157,
0.07762190512386));
#70350=CARTESIAN_POINT('',(0.00337057543319695,-0.0346945769458128,0.0776021788922911));
#70351=CARTESIAN_POINT('Ctrl Pts',(0.00319541831791141,-0.0347116136492788,
0.0775721673619913));
#70352=CARTESIAN_POINT('Ctrl Pts',(0.00323068989929081,-0.0347621546532318,
0.0775476754093557));
#70353=CARTESIAN_POINT('Ctrl Pts',(0.00326534131095514,-0.034813308409707,
0.077523614091432));
#70354=CARTESIAN_POINT('Ctrl Pts',(0.00333343271381562,-0.0349168561544567,
0.0774763326442009));
#70355=CARTESIAN_POINT('Ctrl Pts',(0.00336684569661273,-0.0349692089015914,
0.0774531312690406));
#70356=CARTESIAN_POINT('Ctrl Pts',(0.00339965091618907,-0.0350221583435,
0.0774303519137454));
#70357=CARTESIAN_POINT('Ctrl Pts',(0.00347232165795471,-0.0351951371254882,
0.0775308115215332));
#70358=CARTESIAN_POINT('Ctrl Pts',(0.00354221781496879,-0.0350307338980925,
0.0776269775496714));
#70359=CARTESIAN_POINT('Ctrl Pts',(0.00361602889183594,-0.0348659306897825,
0.0777201725209142));
#70360=CARTESIAN_POINT('Ctrl Pts',(0.0034720619621967,-0.0351951371254882,
0.077532251305466));
#70361=CARTESIAN_POINT('Ctrl Pts',(0.00354198788584025,-0.0350307338980925,
0.0776284227026511));
#70362=CARTESIAN_POINT('Ctrl Pts',(0.00361582892580994,-0.0348659306897825,
0.077721621808066));
#70363=CARTESIAN_POINT('Ctrl Pts',(0.00342853668249728,-0.0351951371254882,
0.077773560593165));
#70364=CARTESIAN_POINT('Ctrl Pts',(0.00350345152426138,-0.0350307338980925,
0.0778706318481992));
#70365=CARTESIAN_POINT('Ctrl Pts',(0.00358231441144628,-0.0348659306897825,
0.0779645238451709));
#70366=CARTESIAN_POINT('Origin',(-0.000554293137037344,-0.0308609197410472,
0.0810220979452573));
#70367=CARTESIAN_POINT('',(0.00345308592161264,-0.0351951371254882,0.0776374567141));
#70368=CARTESIAN_POINT('Origin',(0.00879382484640623,-0.0351840467441214,
0.0734388119151953));
#70369=CARTESIAN_POINT('Origin',(-0.000742447723436461,-0.0352322614715386,
0.0821847918805444));
#70370=CARTESIAN_POINT('',(0.00376567346689154,-0.0351951142564663,0.0779029592209228));
#70371=CARTESIAN_POINT('',(0.00384904922986462,-0.0351951372916786,0.0779956674444053));
#70372=CARTESIAN_POINT('Origin',(0.00845049893136249,-0.0352875121748006,
0.0742462287415656));
#70373=CARTESIAN_POINT('Origin',(0.00426650984675451,-0.0298325076522592,
0.0677144238543658));
#70374=CARTESIAN_POINT('Origin',(0.00024036384308776,-0.0338730261438308,
0.076997743730105));
#70375=CARTESIAN_POINT('Ctrl Pts',(0.00239200676776708,-0.0321934096636942,
0.0746242216979064));
#70376=CARTESIAN_POINT('Ctrl Pts',(0.00240049511033863,-0.0320508460843189,
0.0747268177485896));
#70377=CARTESIAN_POINT('Ctrl Pts',(0.0024117336061173,-0.0319086045660805,
0.0748291083764958));
#70378=CARTESIAN_POINT('Ctrl Pts',(0.00242567992432284,-0.0317669892864515,
0.0749308753240754));
#70379=CARTESIAN_POINT('Ctrl Pts',(0.00240073546049954,-0.0321934096636942,
0.0747076137991576));
#70380=CARTESIAN_POINT('Ctrl Pts',(0.00241071648197276,-0.0320508460843189,
0.0748100536103974));
#70381=CARTESIAN_POINT('Ctrl Pts',(0.00242344233332272,-0.0319086045660805,
0.0749121480113285));
#70382=CARTESIAN_POINT('Ctrl Pts',(0.00243886751601472,-0.0317669892864515,
0.0750136794305652));
#70383=CARTESIAN_POINT('Ctrl Pts',(0.00240946415323199,-0.0321934096636942,
0.0747910059004088));
#70384=CARTESIAN_POINT('Ctrl Pts',(0.00242093785360689,-0.0320508460843189,
0.0748932894722052));
#70385=CARTESIAN_POINT('Ctrl Pts',(0.00243515106052814,-0.0319086045660805,
0.0749951876461612));
#70386=CARTESIAN_POINT('Ctrl Pts',(0.0024520551077066,-0.0317669892864515,
0.0750964835370549));
#70387=CARTESIAN_POINT('Ctrl Pts',(0.00241819284596445,-0.0321934096636942,
0.07487439800166));
#70388=CARTESIAN_POINT('Ctrl Pts',(0.00243115922524102,-0.0320508460843189,
0.0749765253340131));
#70389=CARTESIAN_POINT('Ctrl Pts',(0.00244685978773356,-0.0319086045660805,
0.0750782272809939));
#70390=CARTESIAN_POINT('Ctrl Pts',(0.00246524269939848,-0.0317669892864515,
0.0751792876435447));
#70391=CARTESIAN_POINT('',(0.00241803668792887,-0.0321934096636942,0.0748729061004892));
#70392=CARTESIAN_POINT('',(0.00245255450133589,-0.0318665617511279,0.0751067138846742));
#70393=CARTESIAN_POINT('Origin',(0.019061392985984,-0.0326371944421208,
0.0733840824103799));
#70394=CARTESIAN_POINT('Origin',(-0.0083559143282543,-0.03169392615091,
0.0769300601821768));
#70395=CARTESIAN_POINT('',(0.00240374664865815,-0.032019722162179,0.0747489845880791));
#70396=CARTESIAN_POINT('Ctrl Pts',(0.00240371834984765,-0.0320197392094712,
0.0747491673832019));
#70397=CARTESIAN_POINT('Ctrl Pts',(0.00240676715280521,-0.0319792716576009,
0.0747782729020997));
#70398=CARTESIAN_POINT('Ctrl Pts',(0.00241005172383592,-0.0319386439829649,
0.0748074876775532));
#70399=CARTESIAN_POINT('Ctrl Pts',(0.0024135839156869,-0.031897909938158,
0.0748368414346369));
#70400=CARTESIAN_POINT('Ctrl Pts',(0.00241711603772156,-0.031857176698489,
0.0748661946115224));
#70401=CARTESIAN_POINT('Ctrl Pts',(0.00242087604931126,-0.0318163871833547,
0.0748955377853829));
#70402=CARTESIAN_POINT('Ctrl Pts',(0.00242484752496734,-0.0317755399638303,
0.0749247704753257));
#70403=CARTESIAN_POINT('',(0.00240502396467459,-0.0321934096636183,0.0747485852693819));
#70404=CARTESIAN_POINT('Origin',(0.000111662229081881,-0.0324112415123257,
0.075009778339421));
#70405=CARTESIAN_POINT('',(0.00241153032631172,-0.0321934096636663,0.0748107456849456));
#70406=CARTESIAN_POINT('Ctrl Pts',(0.00241931376590365,-0.0321934096636618,
0.0748713304231029));
#70407=CARTESIAN_POINT('Ctrl Pts',(0.00242926147461029,-0.0320835708272592,
0.0749499994885167));
#70408=CARTESIAN_POINT('Ctrl Pts',(0.00244083146546171,-0.0319739230346489,
0.0750284170553609));
#70409=CARTESIAN_POINT('Ctrl Pts',(0.00245400123542266,-0.0318646057455573,
0.0751064839298879));
#70410=CARTESIAN_POINT('Ctrl Pts',(0.00234796211955568,-0.0321934096636618,
0.0749593651169921));
#70411=CARTESIAN_POINT('Ctrl Pts',(0.00235912389530128,-0.0320835708272592,
0.0750390181772173));
#70412=CARTESIAN_POINT('Ctrl Pts',(0.00237192761270491,-0.0319739230346489,
0.0751183940430615));
#70413=CARTESIAN_POINT('Ctrl Pts',(0.00238634909616581,-0.0318646057455573,
0.0751973924158433));
#70414=CARTESIAN_POINT('Ctrl Pts',(0.0022766104732077,-0.0321934096636618,
0.0750473998108813));
#70415=CARTESIAN_POINT('Ctrl Pts',(0.00228898631599226,-0.0320835708272592,
0.0751280368659178));
#70416=CARTESIAN_POINT('Ctrl Pts',(0.00230302375994811,-0.0319739230346489,
0.0752083710307621));
#70417=CARTESIAN_POINT('Ctrl Pts',(0.00231869695690897,-0.0318646057455573,
0.0752883009017987));
#70418=CARTESIAN_POINT('Ctrl Pts',(0.00220525882685973,-0.0321934096636618,
0.0751354345047705));
#70419=CARTESIAN_POINT('Ctrl Pts',(0.00221884873668325,-0.0320835708272592,
0.0752170555546183));
#70420=CARTESIAN_POINT('Ctrl Pts',(0.00223411990719132,-0.0319739230346489,
0.0752983480184628));
#70421=CARTESIAN_POINT('Ctrl Pts',(0.00225104481765213,-0.0318646057455573,
0.0753792093877541));
#70422=CARTESIAN_POINT('',(0.00220737723631769,-0.0321763980308456,0.0751480743283701));
#70423=CARTESIAN_POINT('',(0.00220525882686676,-0.0321934096636184,0.0751354345048006));
#70424=CARTESIAN_POINT('Origin',(0.0186153532276283,-0.0326386231974675,
0.0730022842093011));
#70425=CARTESIAN_POINT('Ctrl Pts',(0.00220737723944192,-0.0321763980306282,
0.0751480743278375));
#70426=CARTESIAN_POINT('Ctrl Pts',(0.00224969816501251,-0.032125959617537,
0.0751409349535598));
#70427=CARTESIAN_POINT('Ctrl Pts',(0.00229128582563289,-0.0320749164632513,
0.0751339192781986));
#70428=CARTESIAN_POINT('Ctrl Pts',(0.00237302808554854,-0.0319716057793908,
0.0751201296793188));
#70429=CARTESIAN_POINT('Ctrl Pts',(0.00241315083518113,-0.0319193786690101,
0.0751133611287137));
#70430=CARTESIAN_POINT('Ctrl Pts',(0.00245255450316127,-0.0318665617525295,
0.075106713884358));
#70431=CARTESIAN_POINT('',(0.00231164775740781,-0.0321934096636663,0.0750041703026549));
#70432=CARTESIAN_POINT('Origin',(0.00812378219310841,-0.0315241814719618,
0.07415));
#70433=CARTESIAN_POINT('',(0.0022073772359508,-0.0322104233323605,0.0751480743284319));
#70434=CARTESIAN_POINT('',(0.0022095226361545,-0.0321934096636183,0.0751607095987536));
#70435=CARTESIAN_POINT('Origin',(0.0186141164605679,-0.0326387227552032,
0.0729569655886994));
#70436=CARTESIAN_POINT('Origin',(0.0184112488701724,-0.032638624733196,
0.0717923714997738));
#70437=CARTESIAN_POINT('Origin',(0.0184249411132221,-0.0326387240321869,
0.071835589278331));
#70438=CARTESIAN_POINT('Ctrl Pts',(0.00242797688386437,-0.0327445246967097,
0.0749474502361826));
#70439=CARTESIAN_POINT('Ctrl Pts',(0.00245805321120333,-0.032443687833936,
0.0751622710452652));
#70440=CARTESIAN_POINT('Ctrl Pts',(0.00250422527619636,-0.0321434074405927,
0.0753742160992186));
#70441=CARTESIAN_POINT('Ctrl Pts',(0.00246801327136899,-0.0327445246967097,
0.0751942235890301));
#70442=CARTESIAN_POINT('Ctrl Pts',(0.00250739680786285,-0.032443687833936,
0.0754075344010728));
#70443=CARTESIAN_POINT('Ctrl Pts',(0.00256273590206407,-0.0321434074405927,
0.075617272690696));
#70444=CARTESIAN_POINT('',(0.00247468732294034,-0.0326943950436612,0.0752297463349518));
#70445=CARTESIAN_POINT('',(0.00252381793464815,-0.0323666188837389,0.0754609253617077));
#70446=CARTESIAN_POINT('Origin',(0.018972287240742,-0.0326395579110082,
0.0719990722305594));
#70447=CARTESIAN_POINT('Origin',(-0.0082300605462127,-0.0321933825603015,
0.0779783584721712));
#70448=CARTESIAN_POINT('',(0.00249664906193553,-0.0321934096532689,0.0753389061025637));
#70449=CARTESIAN_POINT('',(0.00251089488512872,-0.0321934096584275,0.0753997609040791));
#70450=CARTESIAN_POINT('',(0.00245255450039553,-0.0325210109756239,0.0751067138848201));
#70451=CARTESIAN_POINT('Origin',(0.0190375043577656,-0.032639312916037,
0.0724754451495563));
#70452=CARTESIAN_POINT('',(0.00245389410775943,-0.0326943950436593,0.0751064878983125));
#70453=CARTESIAN_POINT('Origin',(-0.0084544335388826,-0.032694376553816,
0.0769466793692213));
#70454=CARTESIAN_POINT('',(0.00246429071535988,-0.0326943950436702,0.0751681171166422));
#70455=CARTESIAN_POINT('Ctrl Pts',(0.00217280266362598,-0.0325229783203769,
0.0749154035796323));
#70456=CARTESIAN_POINT('Ctrl Pts',(0.00218335373523294,-0.032413025309245,
0.0749974377023069));
#70457=CARTESIAN_POINT('Ctrl Pts',(0.00219560018777097,-0.0323031222208069,
0.0750792411204294));
#70458=CARTESIAN_POINT('Ctrl Pts',(0.0022095226369099,-0.0321934096576658,
0.0751607096031737));
#70459=CARTESIAN_POINT('Ctrl Pts',(0.00226653380546701,-0.0325229783203769,
0.0749790872925074));
#70460=CARTESIAN_POINT('Ctrl Pts',(0.00227796275566328,-0.032413025309245,
0.0750598293334414));
#70461=CARTESIAN_POINT('Ctrl Pts',(0.00229106022527254,-0.0323031222208069,
0.0751403227057466));
#70462=CARTESIAN_POINT('Ctrl Pts',(0.002305805799086,-0.0321934096576658,
0.0752204648951381));
#70463=CARTESIAN_POINT('Ctrl Pts',(0.00236026494730804,-0.0325229783203769,
0.0750427710053824));
#70464=CARTESIAN_POINT('Ctrl Pts',(0.00237257177609363,-0.032413025309245,
0.075122220964576));
#70465=CARTESIAN_POINT('Ctrl Pts',(0.00238652026277411,-0.0323031222208069,
0.0752014042910639));
#70466=CARTESIAN_POINT('Ctrl Pts',(0.0024020889612621,-0.0321934096576658,
0.0752802201871025));
#70467=CARTESIAN_POINT('Ctrl Pts',(0.00245399608914908,-0.0325229783203769,
0.0751064547182575));
#70468=CARTESIAN_POINT('Ctrl Pts',(0.00246718079652397,-0.032413025309245,
0.0751846125957105));
#70469=CARTESIAN_POINT('Ctrl Pts',(0.00248198030027568,-0.0323031222208069,
0.0752624858763811));
#70470=CARTESIAN_POINT('Ctrl Pts',(0.0024983721234382,-0.0321934096576658,
0.0753399754790668));
#70471=CARTESIAN_POINT('',(0.00235308584881014,-0.0321934096584275,0.0752498078502129));
#70472=CARTESIAN_POINT('Ctrl Pts',(0.00220737723937597,-0.0322104233328921,
0.0751480743278485));
#70473=CARTESIAN_POINT('Ctrl Pts',(0.00224975551053476,-0.0322609421831422,
0.0751409252795949));
#70474=CARTESIAN_POINT('Ctrl Pts',(0.00229137118545055,-0.0323120888240851,
0.0751339048783387));
#70475=CARTESIAN_POINT('Ctrl Pts',(0.00237311406416133,-0.0324156524631807,
0.0751201151750706));
#70476=CARTESIAN_POINT('Ctrl Pts',(0.00241320766736387,-0.0324680267167312,
0.075113351541347));
#70477=CARTESIAN_POINT('Ctrl Pts',(0.00245255450043899,-0.0325210109755913,
0.0751067138848172));
#70478=CARTESIAN_POINT('Origin',(0.00775888783888567,-0.0262834582511916,
0.0662905955728784));
#70479=CARTESIAN_POINT('Origin',(-0.00350327331151527,-0.0342770850501676,
0.0705953783460784));
#70480=CARTESIAN_POINT('Ctrl Pts',(0.00247586265801749,-0.0326943950436604,
0.0752280939795756));
#70481=CARTESIAN_POINT('Ctrl Pts',(0.00249072081361951,-0.0325844576448134,
0.0753059328960985));
#70482=CARTESIAN_POINT('Ctrl Pts',(0.00250718985716863,-0.0324744968375322,
0.0753834700303844));
#70483=CARTESIAN_POINT('Ctrl Pts',(0.00252524731729828,-0.0323646534831894,
0.0754606063283826));
#70484=CARTESIAN_POINT('Ctrl Pts',(0.00241017964710776,-0.0326943950436604,
0.0753204350303575));
#70485=CARTESIAN_POINT('Ctrl Pts',(0.00242631043545513,-0.0325844576448134,
0.0753991791818738));
#70486=CARTESIAN_POINT('Ctrl Pts',(0.00244407092355962,-0.0324744968375322,
0.0754775952950863));
#70487=CARTESIAN_POINT('Ctrl Pts',(0.00246343696984689,-0.0323646534831894,
0.0755555832125682));
#70488=CARTESIAN_POINT('Ctrl Pts',(0.00234449663619804,-0.0326943950436604,
0.0754127760811394));
#70489=CARTESIAN_POINT('Ctrl Pts',(0.00236190005729076,-0.0325844576448134,
0.0754924254676492));
#70490=CARTESIAN_POINT('Ctrl Pts',(0.0023809519899506,-0.0324744968375322,
0.0755717205597883));
#70491=CARTESIAN_POINT('Ctrl Pts',(0.00240162662239551,-0.0323646534831894,
0.0756505600967539));
#70492=CARTESIAN_POINT('Ctrl Pts',(0.00227881362528831,-0.0326943950436604,
0.0755051171319213));
#70493=CARTESIAN_POINT('Ctrl Pts',(0.00229748967912638,-0.0325844576448134,
0.0755856717534245));
#70494=CARTESIAN_POINT('Ctrl Pts',(0.00231783305634159,-0.0324744968375322,
0.0756658458244902));
#70495=CARTESIAN_POINT('Ctrl Pts',(0.00233981627494412,-0.0323646534831894,
0.0757455369809395));
#70496=CARTESIAN_POINT('',(0.0022817215154339,-0.0326773559991162,0.0755175989977011));
#70497=CARTESIAN_POINT('',(0.0022788136252905,-0.0326943950436594,0.0755051171319192));
#70498=CARTESIAN_POINT('Origin',(0.018438312426154,-0.0326395669990593,
0.0716838177891191));
#70499=CARTESIAN_POINT('Ctrl Pts',(0.00228172151869258,-0.032677355998743,
0.0755175989969323));
#70500=CARTESIAN_POINT('Ctrl Pts',(0.00232354427761802,-0.0326267922586569,
0.0755078084852715));
#70501=CARTESIAN_POINT('Ctrl Pts',(0.00236462575834461,-0.0325756109580565,
0.0754981915033596));
#70502=CARTESIAN_POINT('Ctrl Pts',(0.00244534112595734,-0.0324719985462364,
0.0754792964144627));
#70503=CARTESIAN_POINT('Ctrl Pts',(0.0024849426399717,-0.032419609162177,
0.0754700258858152));
#70504=CARTESIAN_POINT('Ctrl Pts',(0.00252381793469563,-0.0323666188837756,
0.0754609253616966));
#70505=CARTESIAN_POINT('',(0.00237675047412542,-0.0326943950436703,0.0753674317334455));
#70506=CARTESIAN_POINT('Origin',(0.00812378219310841,-0.0315241814719618,
0.07415));
#70507=CARTESIAN_POINT('',(0.00228172151547635,-0.0327114338380045,0.0755175989976911));
#70508=CARTESIAN_POINT('',(0.00228465605720561,-0.0326943950436593,0.0755300746244477));
#70509=CARTESIAN_POINT('Origin',(0.0184272333273719,-0.0326395661562076,
0.0716398814172339));
#70510=CARTESIAN_POINT('Origin',(0.0184612178671954,-0.0326395683361966,
0.0717816520510706));
#70511=CARTESIAN_POINT('Origin',(0.0184707862139934,-0.0326395674444665,
0.0718259421494922));
#70512=CARTESIAN_POINT('Ctrl Pts',(0.00248929643620834,-0.0332451089994433,
0.075303557651481));
#70513=CARTESIAN_POINT('Ctrl Pts',(0.00253280357484802,-0.0329451141710254,
0.0755160657586173));
#70514=CARTESIAN_POINT('Ctrl Pts',(0.00259219409366805,-0.0326442513127494,
0.0757246930171084));
#70515=CARTESIAN_POINT('Ctrl Pts',(0.00254475051058248,-0.0332451089994433,
0.0755473297697295));
#70516=CARTESIAN_POINT('Ctrl Pts',(0.00259745166508388,-0.0329451141710254,
0.0757577463922322));
#70517=CARTESIAN_POINT('Ctrl Pts',(0.00266585254136425,-0.0326442513127494,
0.0759635955769168));
#70518=CARTESIAN_POINT('Ctrl Pts',(0.00254530505132622,-0.0332451089994433,
0.0755497674909119));
#70519=CARTESIAN_POINT('Ctrl Pts',(0.00259809814598624,-0.0329451141710254,
0.0757601631985683));
#70520=CARTESIAN_POINT('Ctrl Pts',(0.0026665891258412,-0.0326442513127494,
0.0759659846025148));
#70521=CARTESIAN_POINT('',(0.00255363235458533,-0.0331951640388616,0.0755823253039733));
#70522=CARTESIAN_POINT('',(0.0026171818676611,-0.0328677532355001,0.0758099632301979));
#70523=CARTESIAN_POINT('Origin',(0.0185811579717228,-0.0326402808281015,
0.0706679921793711));
#70524=CARTESIAN_POINT('Origin',(-0.00796817111841373,-0.0326944278779144,
0.0790013085759663));
#70525=CARTESIAN_POINT('',(0.0025824049570902,-0.0326943950436593,0.0756898906870749));
#70526=CARTESIAN_POINT('',(0.00260044377354836,-0.0326943950436694,0.0757497309001623));
#70527=CARTESIAN_POINT('',(0.00252381793464749,-0.0330220786163545,0.0754609253617049));
#70528=CARTESIAN_POINT('Origin',(0.0187497064791712,-0.0326396682763934,
0.0711182632598278));
#70529=CARTESIAN_POINT('',(0.00252514070879168,-0.0331951640388587,0.0754606157064861));
#70530=CARTESIAN_POINT('Origin',(-0.00821612393864679,-0.0331952026560115,
0.0779750944438362));
#70531=CARTESIAN_POINT('',(0.0025393865316985,-0.0331951640388701,0.0755214705052398));
#70532=CARTESIAN_POINT('Ctrl Pts',(0.00223260583294866,-0.0330240426238172,
0.075287559270334));
#70533=CARTESIAN_POINT('Ctrl Pts',(0.00224827682016781,-0.032914277406352,
0.0753687159641902));
#70534=CARTESIAN_POINT('Ctrl Pts',(0.00226563335550769,-0.0328043479726691,
0.0754495891545376));
#70535=CARTESIAN_POINT('Ctrl Pts',(0.00228465605720559,-0.0326943950436593,
0.0755300746244477));
#70536=CARTESIAN_POINT('Ctrl Pts',(0.00233015073669985,-0.0330240426238172,
0.0753452318611957));
#70537=CARTESIAN_POINT('Ctrl Pts',(0.00234661622004579,-0.032914277406352,
0.0754250447789693));
#70538=CARTESIAN_POINT('Ctrl Pts',(0.00236473986799249,-0.0328043479726691,
0.0755045570988585));
#70539=CARTESIAN_POINT('Ctrl Pts',(0.00238450126803657,-0.0326943950436593,
0.075583666320247));
#70540=CARTESIAN_POINT('Ctrl Pts',(0.00242769564045103,-0.0330240426238172,
0.0754029044520574));
#70541=CARTESIAN_POINT('Ctrl Pts',(0.00244495561992378,-0.032914277406352,
0.0754813735937484));
#70542=CARTESIAN_POINT('Ctrl Pts',(0.00246384638047729,-0.0328043479726691,
0.0755595250431793));
#70543=CARTESIAN_POINT('Ctrl Pts',(0.00248434647886754,-0.0326943950436593,
0.0756372580160463));
#70544=CARTESIAN_POINT('Ctrl Pts',(0.00252524054420221,-0.0330240426238172,
0.075460577042919));
#70545=CARTESIAN_POINT('Ctrl Pts',(0.00254329501980176,-0.032914277406352,
0.0755377024085275));
#70546=CARTESIAN_POINT('Ctrl Pts',(0.00256295289296209,-0.0328043479726691,
0.0756144929875002));
#70547=CARTESIAN_POINT('Ctrl Pts',(0.00258419168969852,-0.0326943950436593,
0.0756908497118456));
#70548=CARTESIAN_POINT('',(0.0024335305071579,-0.0326943950436694,0.0756099826557714));
#70549=CARTESIAN_POINT('Ctrl Pts',(0.00228172151869955,-0.0327114338383318,
0.0755175989969306));
#70550=CARTESIAN_POINT('Ctrl Pts',(0.00232353732119333,-0.0327619876831142,
0.0755078101137379));
#70551=CARTESIAN_POINT('Ctrl Pts',(0.00236461540410392,-0.03281315626047,
0.0754981939272388));
#70552=CARTESIAN_POINT('Ctrl Pts',(0.00244533069746579,-0.0329167375858767,
0.0754792988557237));
#70553=CARTESIAN_POINT('Ctrl Pts',(0.00248493574682939,-0.0329691088920618,
0.0754700274994674));
#70554=CARTESIAN_POINT('Ctrl Pts',(0.00252381793469442,-0.0330220786163187,
0.0754609253616968));
#70555=CARTESIAN_POINT('Ctrl Pts',(0.00255470178886066,-0.0331951640388604,
0.0755806021341843));
#70556=CARTESIAN_POINT('Ctrl Pts',(0.00258427857076817,-0.033030642201062,
0.0756957393009799));
#70557=CARTESIAN_POINT('Ctrl Pts',(0.00261858881970751,-0.0328657861914645,
0.0758095556443734));
#70558=CARTESIAN_POINT('Ctrl Pts',(0.00255363235458461,-0.0331951640388604,
0.0755823253039703));
#70559=CARTESIAN_POINT('Ctrl Pts',(0.00258324476192266,-0.033030642201062,
0.0756974845806339));
#70560=CARTESIAN_POINT('Ctrl Pts',(0.00261759151967494,-0.0328657861914645,
0.0758113215425662));
#70561=CARTESIAN_POINT('Ctrl Pts',(0.00237543584433657,-0.0331951640388604,
0.0758694517308149));
#70562=CARTESIAN_POINT('Ctrl Pts',(0.00241098440646129,-0.033030642201062,
0.075988295106079));
#70563=CARTESIAN_POINT('Ctrl Pts',(0.00245141451426703,-0.0328657861914645,
0.0761055676710554));
#70564=CARTESIAN_POINT('',(0.00237912173782625,-0.0331781648281905,0.0758817263783082));
#70565=CARTESIAN_POINT('',(0.00237543584433932,-0.0331951640388588,0.0758694517308122));
#70566=CARTESIAN_POINT('Origin',(0.017978010182919,-0.0326412092170369,
0.0704355203308688));
#70567=CARTESIAN_POINT('Ctrl Pts',(0.00237912173840406,-0.033178164828644,
0.0758817263765579));
#70568=CARTESIAN_POINT('Ctrl Pts',(0.00242027552811085,-0.0331276811546774,
0.0758693205648664));
#70569=CARTESIAN_POINT('Ctrl Pts',(0.00246068619806179,-0.0330765663497782,
0.0758571387313375));
#70570=CARTESIAN_POINT('Ctrl Pts',(0.00254005606509915,-0.0329730614463344,
0.0758332127095248));
#70571=CARTESIAN_POINT('Ctrl Pts',(0.00257898320003413,-0.0329207133374209,
0.0758214781919652));
#70572=CARTESIAN_POINT('Ctrl Pts',(0.00261718185528346,-0.032867753228936,
0.0758099632193273));
#70573=CARTESIAN_POINT('',(0.00246453409947232,-0.0331951640388702,0.0757258885174028));
#70574=CARTESIAN_POINT('Origin',(0.00812378219310841,-0.0315241814719618,
0.07415));
#70575=CARTESIAN_POINT('',(0.00237912173949705,-0.0332121607144409,0.07588172637848));
#70576=CARTESIAN_POINT('',(0.00238283384147147,-0.0331951640388587,0.0758939931260949));
#70577=CARTESIAN_POINT('Origin',(0.0179576128667686,-0.0326413642951286,
0.0703950201715192));
#70578=CARTESIAN_POINT('Origin',(0.0183891629845607,-0.0326412102338043,
0.0717994275002161));
#70579=CARTESIAN_POINT('Origin',(0.0183945413997972,-0.0326413657341333,
0.0718444545186698));
#70580=CARTESIAN_POINT('Ctrl Pts',(0.00257284183963962,-0.0337436976235976,
0.0756550535512837));
#70581=CARTESIAN_POINT('Ctrl Pts',(0.00258637851937698,-0.0336723290703325,
0.0757049795500909));
#70582=CARTESIAN_POINT('Ctrl Pts',(0.00260081102055362,-0.033601104548885,
0.075754653989846));
#70583=CARTESIAN_POINT('Ctrl Pts',(0.00264689113789323,-0.0333736987606857,
0.075913254636032));
#70584=CARTESIAN_POINT('Ctrl Pts',(0.00270199673840641,-0.0331450831799192,
0.0760689495780717));
#70585=CARTESIAN_POINT('Ctrl Pts',(0.00264349219742188,-0.0337436976235976,
0.0758948629067002));
#70586=CARTESIAN_POINT('Ctrl Pts',(0.00265918575884595,-0.0336723290703325,
0.0759441534654821));
#70587=CARTESIAN_POINT('Ctrl Pts',(0.00267576336321349,-0.033601104548885,
0.075993153772508));
#70588=CARTESIAN_POINT('Ctrl Pts',(0.00272869237012062,-0.0333736987606857,
0.0761496020464278));
#70589=CARTESIAN_POINT('Ctrl Pts',(0.00279051205824203,-0.0331450831799192,
0.0763027551343668));
#70590=CARTESIAN_POINT('Ctrl Pts',(0.0026441987009997,-0.0337436976235976,
0.0758972610002543));
#70591=CARTESIAN_POINT('Ctrl Pts',(0.00265991383124064,-0.0336723290703325,
0.075946545204636));
#70592=CARTESIAN_POINT('Ctrl Pts',(0.00267651288664009,-0.033601104548885,
0.0759955387703346));
#70593=CARTESIAN_POINT('Ctrl Pts',(0.00272951038244289,-0.0333736987606857,
0.0761519655205318));
#70594=CARTESIAN_POINT('Ctrl Pts',(0.00279139721144039,-0.0331450831799192,
0.0763050931899297));
#70595=CARTESIAN_POINT('',(0.00265456022288775,-0.0336938721132548,0.0759292515393999));
#70596=CARTESIAN_POINT('',(0.00273227784254589,-0.0333679869945435,0.076152449958875));
#70597=CARTESIAN_POINT('Ctrl Pts',(0.00265456022289061,-0.0336938721132647,
0.075929251539412));
#70598=CARTESIAN_POINT('Ctrl Pts',(0.00266150547631112,-0.033662918793393,
0.0759506004784193));
#70599=CARTESIAN_POINT('Ctrl Pts',(0.00266857351509565,-0.0336319952301038,
0.0759719019222763));
#70600=CARTESIAN_POINT('Ctrl Pts',(0.00267576336321711,-0.0336011045488948,
0.07599315377252));
#70601=CARTESIAN_POINT('Ctrl Pts',(0.00269380515238141,-0.033523589259545,
0.0760464819367554));
#70602=CARTESIAN_POINT('Ctrl Pts',(0.00271264615022564,-0.0334458668660368,
0.0760995925311814));
#70603=CARTESIAN_POINT('Ctrl Pts',(0.0027322778422408,-0.0333679869945384,
0.0761524499589809));
#70604=CARTESIAN_POINT('Ctrl Pts',(0.00273229268110906,-0.033367969246074,
0.076152491886018));
#70605=CARTESIAN_POINT('Ctrl Pts',(0.0027327154741517,-0.0333391895375,
0.0761523285340469));
#70606=CARTESIAN_POINT('Ctrl Pts',(0.00273303120788034,-0.0333104081060346,
0.0761522030648029));
#70607=CARTESIAN_POINT('Ctrl Pts',(0.00273344709022916,-0.0332532698060263,
0.0761520318378214));
#70608=CARTESIAN_POINT('Ctrl Pts',(0.00273355038452273,-0.0332249170431269,
0.0761519849153727));
#70609=CARTESIAN_POINT('Ctrl Pts',(0.0027335514233815,-0.0331960985399096,
0.0761519771705221));
#70610=CARTESIAN_POINT('Ctrl Pts',(0.00273355141231489,-0.0331956312525604,
0.0761519770552596));
#70611=CARTESIAN_POINT('Ctrl Pts',(0.00273355137358271,-0.0331951640388588,
0.076151976950975));
#70612=CARTESIAN_POINT('',(0.00269003013551804,-0.0331951640388587,0.076034798020116));
#70613=CARTESIAN_POINT('',(0.00271179075456039,-0.0331951640388687,0.0760933874855556));
#70614=CARTESIAN_POINT('',(0.00261718186978805,-0.0335216366567717,0.0758099632148271));
#70615=CARTESIAN_POINT('Origin',(0.0181711571565241,-0.0326434571525561,
0.069856433354535));
#70616=CARTESIAN_POINT('',(0.00261848258998653,-0.0336938721132327,0.0758095711132298));
#70617=CARTESIAN_POINT('Origin',(-0.00783734462861687,-0.0336938867896231,
0.0789614764282001));
#70618=CARTESIAN_POINT('',(0.00263652140644714,-0.0336938721132538,0.0758694113263247));
#70619=CARTESIAN_POINT('Ctrl Pts',(0.00231565890246709,-0.0335235895815172,
0.0756552255115898));
#70620=CARTESIAN_POINT('Ctrl Pts',(0.00233638129515044,-0.0334144449262748,
0.0757351857638279));
#70621=CARTESIAN_POINT('Ctrl Pts',(0.00235877941398685,-0.0333049234473147,
0.075814809771671));
#70622=CARTESIAN_POINT('Ctrl Pts',(0.00238283384147129,-0.0331951640388587,
0.0758939931260949));
#70623=CARTESIAN_POINT('Ctrl Pts',(0.00241663276732491,-0.0335235895815172,
0.0757066594605111));
#70624=CARTESIAN_POINT('Ctrl Pts',(0.00243806324957928,-0.0334144449262748,
0.0757852296087002));
#70625=CARTESIAN_POINT('Ctrl Pts',(0.00246114155299237,-0.0333049234473147,
0.0758634472868355));
#70626=CARTESIAN_POINT('Ctrl Pts',(0.00248584722741736,-0.0331951640388587,
0.0759412098053713));
#70627=CARTESIAN_POINT('Ctrl Pts',(0.00251760663218272,-0.0335235895815172,
0.0757580934094324));
#70628=CARTESIAN_POINT('Ctrl Pts',(0.00253974520400812,-0.0334144449262748,
0.0758352734535725));
#70629=CARTESIAN_POINT('Ctrl Pts',(0.00256350369199788,-0.0333049234473147,
0.0759120848019999));
#70630=CARTESIAN_POINT('Ctrl Pts',(0.00258886061336342,-0.0331951640388587,
0.0759884264846476));
#70631=CARTESIAN_POINT('Ctrl Pts',(0.00261858049704053,-0.0335235895815172,
0.0758095273583538));
#70632=CARTESIAN_POINT('Ctrl Pts',(0.00264142715843697,-0.0334144449262748,
0.0758853172984448));
#70633=CARTESIAN_POINT('Ctrl Pts',(0.0026658658310034,-0.0333049234473147,
0.0759607223171644));
#70634=CARTESIAN_POINT('Ctrl Pts',(0.00269187399930949,-0.0331951640388587,
0.076035643163924));
#70635=CARTESIAN_POINT('',(0.00253643198850476,-0.0331951640388687,0.0759643955731154));
#70636=CARTESIAN_POINT('Ctrl Pts',(0.00237912174249123,-0.0332121607145971,
0.0758817263775711));
#70637=CARTESIAN_POINT('Ctrl Pts',(0.00242020630450993,-0.0332625444109943,
0.0758693414471874));
#70638=CARTESIAN_POINT('Ctrl Pts',(0.00246058291505227,-0.033313530074722,
0.0758571699285895));
#70639=CARTESIAN_POINT('Ctrl Pts',(0.00253995228355812,-0.0334167203140611,
0.0758332440533886));
#70640=CARTESIAN_POINT('Ctrl Pts',(0.00257891430115607,-0.0334688847587314,
0.0758214989634607));
#70641=CARTESIAN_POINT('Ctrl Pts',(0.00261718187050628,-0.0335216366562391,
0.075809963214774));
#70642=CARTESIAN_POINT('Ctrl Pts',(0.00265503308426364,-0.0336938721132391,
0.0759283705643767));
#70643=CARTESIAN_POINT('Ctrl Pts',(0.00266544247730287,-0.0336474569764958,
0.0759603809676342));
#70644=CARTESIAN_POINT('Ctrl Pts',(0.00267622587927018,-0.033601104548885,
0.0759922673224299));
#70645=CARTESIAN_POINT('Ctrl Pts',(0.00270352697379182,-0.0334837508592656,
0.0760729962416402));
#70646=CARTESIAN_POINT('Ctrl Pts',(0.00273320824493969,-0.0333660264659097,
0.0761528807226235));
#70647=CARTESIAN_POINT('Ctrl Pts',(0.00265456022288147,-0.0336938721132391,
0.0759292515393802));
#70648=CARTESIAN_POINT('Ctrl Pts',(0.00266497477255974,-0.0336474569764958,
0.0759612647104523));
#70649=CARTESIAN_POINT('Ctrl Pts',(0.00267576336321351,-0.033601104548885,
0.075993153772508));
#70650=CARTESIAN_POINT('Ctrl Pts',(0.00270307759429631,-0.0334837508592656,
0.076073889545878));
#70651=CARTESIAN_POINT('Ctrl Pts',(0.00273277219933971,-0.0333660264659097,
0.0761537804887477));
#70652=CARTESIAN_POINT('Ctrl Pts',(0.00249378526387214,-0.0336938721132391,
0.0762287869326754));
#70653=CARTESIAN_POINT('Ctrl Pts',(0.00250595309360374,-0.0336474569764958,
0.0762617411729333));
#70654=CARTESIAN_POINT('Ctrl Pts',(0.002518505860578,-0.033601104548885,
0.0762945507153355));
#70655=CARTESIAN_POINT('Ctrl Pts',(0.00255028658049469,-0.0334837508592656,
0.0763776169333112));
#70656=CARTESIAN_POINT('Ctrl Pts',(0.00258451476892472,-0.0333660264659097,
0.0764597049461023));
#70657=CARTESIAN_POINT('',(0.00249919351186432,-0.0336769361243754,0.0762390194271047));
#70658=CARTESIAN_POINT('',(0.00249474416025707,-0.0336938721132328,0.0762270004392665));
#70659=CARTESIAN_POINT('Ctrl Pts',(0.00249919351186441,-0.0336769361243751,
0.076239019427105));
#70660=CARTESIAN_POINT('Ctrl Pts',(0.00249844975816789,-0.0336797586670077,
0.0762370169045009));
#70661=CARTESIAN_POINT('Ctrl Pts',(0.00249770710203766,-0.0336825812712949,
0.0762350140604358));
#70662=CARTESIAN_POINT('Ctrl Pts',(0.00249622398589853,-0.0336882265975037,
0.0762310077335349));
#70663=CARTESIAN_POINT('Ctrl Pts',(0.00249548352587924,-0.0336910493194312,
0.0762290042507009));
#70664=CARTESIAN_POINT('Ctrl Pts',(0.00249474416025435,-0.0336938721132344,
0.0762270004392697));
#70665=CARTESIAN_POINT('Ctrl Pts',(0.00249919351186432,-0.0336769361243754,
0.0762390194271047));
#70666=CARTESIAN_POINT('Ctrl Pts',(0.0025384839031759,-0.0336279018505215,
0.0762244266461211));
#70667=CARTESIAN_POINT('Ctrl Pts',(0.00257833953646447,-0.0335767826010774,
0.0762096239295242));
#70668=CARTESIAN_POINT('Ctrl Pts',(0.00265643367930056,-0.0334733172064629,
0.0761806191096568));
#70669=CARTESIAN_POINT('Ctrl Pts',(0.00269472467439516,-0.0334209631456252,
0.0761663975128138));
#70670=CARTESIAN_POINT('Ctrl Pts',(0.00273227783999864,-0.0333679869844681,
0.0761524499520336));
#70671=CARTESIAN_POINT('',(0.00257465219158242,-0.0336938721132539,0.0760781259893432));
#70672=CARTESIAN_POINT('Origin',(0.00812378219310841,-0.0315241814719618,
0.07415));
#70673=CARTESIAN_POINT('',(0.00249919351308419,-0.0337108120655673,0.0762390194266585));
#70674=CARTESIAN_POINT('',(0.00250366852609151,-0.0336938721132327,0.0762510288836281));
#70675=CARTESIAN_POINT('Origin',(0.0182258276927463,-0.034556251066585,
0.0715902141959668));
#70676=CARTESIAN_POINT('Ctrl Pts',(0.00250366852609819,-0.0336938721132302,
0.0762510288836292));
#70677=CARTESIAN_POINT('Ctrl Pts',(0.00250292061121399,-0.0336910493357639,
0.076249028260651));
#70678=CARTESIAN_POINT('Ctrl Pts',(0.00250217373338578,-0.03368822660567,
0.0762470271548477));
#70679=CARTESIAN_POINT('Ctrl Pts',(0.00250068206056199,-0.0336825812712835,
0.0762430239993698));
#70680=CARTESIAN_POINT('Ctrl Pts',(0.00249993726555925,-0.033679758667002,
0.0762410219497045));
#70681=CARTESIAN_POINT('Ctrl Pts',(0.00249919351186424,-0.0336769361243751,
0.0762390194271045));
#70682=CARTESIAN_POINT('Origin',(0.0174475919152087,-0.0345562514648014,
0.0694948596281702));
#70683=CARTESIAN_POINT('Ctrl Pts',(0.00267828183148321,-0.034243627687391,
0.0760005812091178));
#70684=CARTESIAN_POINT('Ctrl Pts',(0.00274807765238379,-0.033943005420181,
0.0762059616409958));
#70685=CARTESIAN_POINT('Ctrl Pts',(0.00283314528632338,-0.0336441434784052,
0.0764055013013883));
#70686=CARTESIAN_POINT('Ctrl Pts',(0.00276384842192349,-0.034243627687391,
0.0762354819511355));
#70687=CARTESIAN_POINT('Ctrl Pts',(0.00284250367035878,-0.033943005420181,
0.0764376351858541));
#70688=CARTESIAN_POINT('Ctrl Pts',(0.00293616247741516,-0.0336441434784052,
0.0766332894888336));
#70689=CARTESIAN_POINT('Ctrl Pts',(0.00276470408782789,-0.034243627687391,
0.0762378309585557));
#70690=CARTESIAN_POINT('Ctrl Pts',(0.00284344793053853,-0.033943005420181,
0.0764399519213026));
#70691=CARTESIAN_POINT('Ctrl Pts',(0.00293719264932608,-0.0336441434784052,
0.076635567370708));
#70692=CARTESIAN_POINT('',(0.00277707261164741,-0.0341934961088741,0.0762691558818346));
#70693=CARTESIAN_POINT('',(0.00286865161518105,-0.0338664212863057,0.076487033935523));
#70694=CARTESIAN_POINT('Origin',(0.018515004651897,-0.0345610720405401,
0.0705796357915323));
#70695=CARTESIAN_POINT('Origin',(-0.00715141688422835,-0.0336938005073012,
0.0809431479026955));
#70696=CARTESIAN_POINT('',(0.00281909985087202,-0.0336938721132327,0.0763722669164541));
#70697=CARTESIAN_POINT('',(0.00284449639327672,-0.0336938721132427,0.0764293744083928));
#70698=CARTESIAN_POINT('',(0.00273227783999677,-0.0340203938281605,0.0761524499520286));
#70699=CARTESIAN_POINT('Origin',(0.0186068803369215,-0.0345589643243687,
0.0710519657530197));
#70700=CARTESIAN_POINT('',(0.00273355137358276,-0.034193496108874,0.0761519769509753));
#70701=CARTESIAN_POINT('Origin',(-0.00759642532336942,-0.0341934220717646,
0.0799886160664778));
#70702=CARTESIAN_POINT('',(0.00275531199262508,-0.034193496108884,0.0762105664164149));
#70703=CARTESIAN_POINT('Ctrl Pts',(0.00242163294752614,-0.0340223579322396,
0.0760169477714017));
#70704=CARTESIAN_POINT('Ctrl Pts',(0.00244738302649796,-0.0339125849573574,
0.0760955952813278));
#70705=CARTESIAN_POINT('Ctrl Pts',(0.00247474283189135,-0.0338030433565231,
0.0761736545597596));
#70706=CARTESIAN_POINT('Ctrl Pts',(0.00250366852609084,-0.0336938721132327,
0.0762510288836279));
#70707=CARTESIAN_POINT('Ctrl Pts',(0.00252563713712521,-0.0340223579322396,
0.0760619400860366));
#70708=CARTESIAN_POINT('Ctrl Pts',(0.00255200777746074,-0.0339125849573574,
0.0761391531069339));
#70709=CARTESIAN_POINT('Ctrl Pts',(0.00257995801756693,-0.0338030433565231,
0.0762157660601573));
#70710=CARTESIAN_POINT('Ctrl Pts',(0.00260944342872167,-0.0336938721132327,
0.0762916841391776));
#70711=CARTESIAN_POINT('Ctrl Pts',(0.00262964132672429,-0.0340223579322396,
0.0761069324006715));
#70712=CARTESIAN_POINT('Ctrl Pts',(0.00265663252842351,-0.0339125849573574,
0.0761827109325399));
#70713=CARTESIAN_POINT('Ctrl Pts',(0.00268517320324251,-0.0338030433565231,
0.076257877560555));
#70714=CARTESIAN_POINT('Ctrl Pts',(0.0027152183313525,-0.0336938721132327,
0.0763323393947272));
#70715=CARTESIAN_POINT('Ctrl Pts',(0.00273364551632336,-0.0340223579322396,
0.0761519247153065));
#70716=CARTESIAN_POINT('Ctrl Pts',(0.00276125727938629,-0.0339125849573574,
0.076226268758146));
#70717=CARTESIAN_POINT('Ctrl Pts',(0.00279038838891809,-0.0338030433565231,
0.0762999890609528));
#70718=CARTESIAN_POINT('Ctrl Pts',(0.00282099323398333,-0.0336938721132327,
0.0763729946502769));
#70719=CARTESIAN_POINT('',(0.00266138418849176,-0.0336938721132427,0.0763116479000511));
#70720=CARTESIAN_POINT('Ctrl Pts',(0.00249919351645708,-0.0337108120662681,
0.0762390194253988));
#70721=CARTESIAN_POINT('Ctrl Pts',(0.0025395023713875,-0.0337611408994432,
0.0762240483784822));
#70722=CARTESIAN_POINT('Ctrl Pts',(0.00257907567914348,-0.0338121088781598,
0.0762093505199573));
#70723=CARTESIAN_POINT('Ctrl Pts',(0.00265678725091846,-0.0339153382773232,
0.0761804877901918));
#70724=CARTESIAN_POINT('Ctrl Pts',(0.00269489263821679,-0.0339675558473112,
0.076166335129641));
#70725=CARTESIAN_POINT('Ctrl Pts',(0.00273227784003597,-0.0340203938281304,
0.0761524499520196));
#70726=CARTESIAN_POINT('Ctrl Pts',(0.00277791768151383,-0.0341934961088741,
0.0762673121793628));
#70727=CARTESIAN_POINT('Ctrl Pts',(0.00282169144277852,-0.0340287516182428,
0.0763778337166045));
#70728=CARTESIAN_POINT('Ctrl Pts',(0.0028699957391836,-0.0338644633275951,
0.0764864516125442));
#70729=CARTESIAN_POINT('Ctrl Pts',(0.00277707261164746,-0.0341934961088741,
0.0762691558818346));
#70730=CARTESIAN_POINT('Ctrl Pts',(0.00282088449000827,-0.0340287516182428,
0.0763796948902301));
#70731=CARTESIAN_POINT('Ctrl Pts',(0.00286922759303518,-0.0338644633275951,
0.0764883286669863));
#70732=CARTESIAN_POINT('Ctrl Pts',(0.00263626771762503,-0.0341934961088741,
0.0765763521758839));
#70733=CARTESIAN_POINT('Ctrl Pts',(0.00268643063735243,-0.0340287516182428,
0.0766898022145356));
#70734=CARTESIAN_POINT('Ctrl Pts',(0.00274123966999151,-0.0338644633275951,
0.0768010820407703));
#70735=CARTESIAN_POINT('',(0.00264146296832161,-0.0341764758832398,0.0765880680688096));
#70736=CARTESIAN_POINT('',(0.00263626771762762,-0.034193496108874,0.0765763521758782));
#70737=CARTESIAN_POINT('Origin',(0.0179786966131428,-0.0345621025081795,
0.0703278293545461));
#70738=CARTESIAN_POINT('Ctrl Pts',(0.00264146296845681,-0.0341764758837489,
0.0765880680669895));
#70739=CARTESIAN_POINT('Ctrl Pts',(0.0026806838197208,-0.0341260050040299,
0.0765706259619968));
#70740=CARTESIAN_POINT('Ctrl Pts',(0.00271922290453729,-0.0340749269147893,
0.0765534870070261));
#70741=CARTESIAN_POINT('Ctrl Pts',(0.00279496748398733,-0.0339715436305769,
0.0765198022818631));
#70742=CARTESIAN_POINT('Ctrl Pts',(0.00283214424516812,-0.0339192778237878,
0.0765032692964079));
#70743=CARTESIAN_POINT('Ctrl Pts',(0.00286865161362882,-0.0338664212855625,
0.0764870339344522));
#70744=CARTESIAN_POINT('',(0.00270667016464752,-0.0341934961088841,0.0764227540288665));
#70745=CARTESIAN_POINT('Origin',(0.00812378219310841,-0.0315241814719618,
0.07415));
#70746=CARTESIAN_POINT('',(0.00264146296933602,-0.0342105180190531,0.0765880680692793));
#70747=CARTESIAN_POINT('',(0.00264668323176958,-0.0341934961088739,0.0765997728400264));
#70748=CARTESIAN_POINT('Origin',(0.0179651848135109,-0.0345621701778859,
0.0702845622155633));
#70749=CARTESIAN_POINT('Origin',(0.0175625212072795,-0.0345621041234899,
0.0693919965751807));
#70750=CARTESIAN_POINT('Origin',(0.0175855946343702,-0.0345621714878735,
0.0694310119607774));
#70751=CARTESIAN_POINT('Ctrl Pts',(0.00281849032982699,-0.0346945769586965,
0.0763708963275908));
#70752=CARTESIAN_POINT('Ctrl Pts',(0.00286500789260676,-0.0345275153362944,
0.0764820177897902));
#70753=CARTESIAN_POINT('Ctrl Pts',(0.00291503215491682,-0.0343603235965185,
0.0765917050591585));
#70754=CARTESIAN_POINT('Ctrl Pts',(0.00296841034567327,-0.034193496108874,
0.0766996359283591));
#70755=CARTESIAN_POINT('Ctrl Pts',(0.00285255556015485,-0.0346945769586965,
0.0764474965133866));
#70756=CARTESIAN_POINT('Ctrl Pts',(0.00290067754449516,-0.0345275153362944,
0.0765579044656978));
#70757=CARTESIAN_POINT('Ctrl Pts',(0.0029522842041221,-0.0343603235965185,
0.0766668275830464));
#70758=CARTESIAN_POINT('Ctrl Pts',(0.00300721812151278,-0.034193496108874,
0.0767739459876756));
#70759=CARTESIAN_POINT('Ctrl Pts',(0.00288662079048272,-0.0346945769586965,
0.0765240966991827));
#70760=CARTESIAN_POINT('Ctrl Pts',(0.00293634719638359,-0.0345275153362944,
0.0766337911416053));
#70761=CARTESIAN_POINT('Ctrl Pts',(0.00298953625332745,-0.0343603235965185,
0.0767419501069332));
#70762=CARTESIAN_POINT('Ctrl Pts',(0.00304602589735237,-0.034193496108874,
0.0768482560469898));
#70763=CARTESIAN_POINT('Ctrl Pts',(0.00292068602081057,-0.0346945769586965,
0.0766006968849783));
#70764=CARTESIAN_POINT('Ctrl Pts',(0.00297201684827194,-0.0345275153362944,
0.0767096778175131));
#70765=CARTESIAN_POINT('Ctrl Pts',(0.00302678830253266,-0.0343603235965185,
0.0768170726308223));
#70766=CARTESIAN_POINT('Ctrl Pts',(0.00308483367319179,-0.034193496108874,
0.0769225661063088));
#70767=CARTESIAN_POINT('',(0.00292068602045324,-0.0346945769586966,0.0766006968841744));
#70768=CARTESIAN_POINT('',(0.00302576498982647,-0.0343667727832792,0.0768123947107075));
#70769=CARTESIAN_POINT('Origin',(0.0180526272124075,-0.0345626461567138,
0.0692711946845922));
#70770=CARTESIAN_POINT('Origin',(-0.00677090826187286,-0.0341934771027846,
0.0819286285336233));
#70771=CARTESIAN_POINT('',(0.00296910472395195,-0.034193496108874,0.07670096554053));
#70772=CARTESIAN_POINT('',(0.00299803696116878,-0.034193496108884,0.0767563656817873));
#70773=CARTESIAN_POINT('',(0.00286865161510245,-0.0345211942962685,0.0764870339338463));
#70774=CARTESIAN_POINT('Origin',(0.0182449646160614,-0.0345625596118157,
0.0697118720181048));
#70775=CARTESIAN_POINT('',(0.00286989293566145,-0.0346945769586886,0.0764864819003117));
#70776=CARTESIAN_POINT('Origin',(-0.00723910855075123,-0.0346945685853894,
0.0809821024537475));
#70777=CARTESIAN_POINT('',(0.00289528947806735,-0.0346945769587026,0.0765435893922531));
#70778=CARTESIAN_POINT('Ctrl Pts',(0.00255011181324564,-0.0345231616327842,
0.0763713055838112));
#70779=CARTESIAN_POINT('Ctrl Pts',(0.00258072938337036,-0.0344132092796988,
0.0764481307828973));
#70780=CARTESIAN_POINT('Ctrl Pts',(0.00261293444241344,-0.0343032738558979,
0.0765243187178692));
#70781=CARTESIAN_POINT('Ctrl Pts',(0.00264668323176956,-0.0341934961088739,
0.0765997728400264));
#70782=CARTESIAN_POINT('Ctrl Pts',(0.00265673568990527,-0.0345231616327842,
0.0764096785569123));
#70783=CARTESIAN_POINT('Ctrl Pts',(0.00268788217743937,-0.0344132092796988,
0.0764850340959731));
#70784=CARTESIAN_POINT('Ctrl Pts',(0.00272058572784374,-0.0343032738558979,
0.0765597415065079));
#70785=CARTESIAN_POINT('Ctrl Pts',(0.0027548019924733,-0.0341934961088739,
0.0766337061528979));
#70786=CARTESIAN_POINT('Ctrl Pts',(0.00276335956656489,-0.0345231616327842,
0.0764480515300134));
#70787=CARTESIAN_POINT('Ctrl Pts',(0.00279503497150837,-0.0344132092796988,
0.0765219374090489));
#70788=CARTESIAN_POINT('Ctrl Pts',(0.00282823701327404,-0.0343032738558979,
0.0765951642951466));
#70789=CARTESIAN_POINT('Ctrl Pts',(0.00286292075317704,-0.0341934961088739,
0.0766676394657694));
#70790=CARTESIAN_POINT('Ctrl Pts',(0.00286998344322452,-0.0345231616327842,
0.0764864245031145));
#70791=CARTESIAN_POINT('Ctrl Pts',(0.00290218776557737,-0.0344132092796988,
0.0765588407221246));
#70792=CARTESIAN_POINT('Ctrl Pts',(0.00293588829870434,-0.0343032738558979,
0.0766305870837853));
#70793=CARTESIAN_POINT('Ctrl Pts',(0.00297103951388078,-0.0341934961088739,
0.0767015727786409));
#70794=CARTESIAN_POINT('',(0.00280789397787076,-0.0341934961088839,0.0766503691902882));
#70795=CARTESIAN_POINT('Ctrl Pts',(0.00264146297248843,-0.0342105180195384,
0.0765880680678703));
#70796=CARTESIAN_POINT('Ctrl Pts',(0.00268072792119011,-0.034261055624136,
0.0765706063671259));
#70797=CARTESIAN_POINT('Ctrl Pts',(0.00271928828068896,-0.034312218987028,
0.0765534580075728));
#70798=CARTESIAN_POINT('Ctrl Pts',(0.00279503362251527,-0.0344158119695162,
0.0765197729389431));
#70799=CARTESIAN_POINT('Ctrl Pts',(0.00283218762445906,-0.0344681990450067,
0.0765032500072992));
#70800=CARTESIAN_POINT('Ctrl Pts',(0.00286865161512399,-0.0345211942962485,
0.0764870339338293));
#70801=CARTESIAN_POINT('Ctrl Pts',(0.00292141347753173,-0.0346945769586932,
0.076598804221065));
#70802=CARTESIAN_POINT('Ctrl Pts',(0.00297204077206713,-0.0345296777077528,
0.0767063595131458));
#70803=CARTESIAN_POINT('Ctrl Pts',(0.00302707016526706,-0.0343648066252516,
0.0768117304279686));
#70804=CARTESIAN_POINT('Ctrl Pts',(0.00292068602044944,-0.0346945769586932,
0.0766006968841661));
#70805=CARTESIAN_POINT('Ctrl Pts',(0.00297135244445524,-0.0345296777077528,
0.0767082672159074));
#70806=CARTESIAN_POINT('Ctrl Pts',(0.0030264215552929,-0.0343648066252516,
0.0768136515402825));
#70807=CARTESIAN_POINT('Ctrl Pts',(0.00279944798762186,-0.0346945769586932,
0.0769161282089503));
#70808=CARTESIAN_POINT('Ctrl Pts',(0.00285663573107336,-0.0345296777077528,
0.0770262050512342));
#70809=CARTESIAN_POINT('Ctrl Pts',(0.00291832418535472,-0.0343648066252516,
0.0771338242122447));
#70810=CARTESIAN_POINT('',(0.00280536863352462,-0.0346775396664985,0.0769274947709485));
#70811=CARTESIAN_POINT('',(0.002799447987626,-0.0346945769586885,0.0769161282089466));
#70812=CARTESIAN_POINT('Origin',(0.0174497406703401,-0.0345626617476886,
0.0691073113763725));
#70813=CARTESIAN_POINT('Ctrl Pts',(0.00280536863364831,-0.0346775396670096,
0.0769274947691259));
#70814=CARTESIAN_POINT('Ctrl Pts',(0.00284344685941726,-0.0346269749928347,
0.0769076087356097));
#70815=CARTESIAN_POINT('Ctrl Pts',(0.00288084833351958,-0.0345757902891115,
0.0768880760894427));
#70816=CARTESIAN_POINT('Ctrl Pts',(0.00295432866049844,-0.0344721681088523,
0.0768497016382947));
#70817=CARTESIAN_POINT('Ctrl Pts',(0.00299037870823899,-0.0344197714290315,
0.0768308748829006));
#70818=CARTESIAN_POINT('Ctrl Pts',(0.00302576498952295,-0.0343667727831574,
0.0768123947104756));
#70819=CARTESIAN_POINT('',(0.00286006700404961,-0.0346945769587026,0.0767584125465705));
#70820=CARTESIAN_POINT('Origin',(0.00812378219310841,-0.0315241814719618,
0.07415));
#70821=CARTESIAN_POINT('',(0.00280536863491102,-0.0347116136489604,0.0769274947710576));
#70822=CARTESIAN_POINT('',(0.00281131354479945,-0.0346945769586885,0.0769388486622199));
#70823=CARTESIAN_POINT('Origin',(0.0174271276195662,-0.0345626679652983,
0.0690680433225043));
#70824=CARTESIAN_POINT('Origin',(0.0175911330836941,-0.0345626630821519,
0.0693780458598815));
#70825=CARTESIAN_POINT('Origin',(0.0176104315067095,-0.03456266930565,0.069419044940195));
#70826=CARTESIAN_POINT('Ctrl Pts',(0.00295204013945966,-0.0352450361874068,
0.0766663161081523));
#70827=CARTESIAN_POINT('Ctrl Pts',(0.00304694455878776,-0.0349452760959492,
0.0768613715604168));
#70828=CARTESIAN_POINT('Ctrl Pts',(0.00315627173941708,-0.034644428984174,
0.0770487242914932));
#70829=CARTESIAN_POINT('Ctrl Pts',(0.0029531949308012,-0.0352450361874068,
0.0766685615662252));
#70830=CARTESIAN_POINT('Ctrl Pts',(0.0030481840389702,-0.0349452760959492,
0.0768635734648196));
#70831=CARTESIAN_POINT('Ctrl Pts',(0.0031575923872077,-0.034644428984174,
0.0770508763868473));
#70832=CARTESIAN_POINT('Ctrl Pts',(0.00306753070719105,-0.0352450361874068,
0.0768908841477084));
#70833=CARTESIAN_POINT('Ctrl Pts',(0.0031709048491127,-0.0349452760959492,
0.0770815838017356));
#70834=CARTESIAN_POINT('Ctrl Pts',(0.00328834959419955,-0.034644428984174,
0.0772639551347779));
#70835=CARTESIAN_POINT('Ctrl Pts',(0.00306867406495496,-0.0352450361874068,
0.0768931073735232));
#70836=CARTESIAN_POINT('Ctrl Pts',(0.00317213205721413,-0.0349452760959492,
0.0770837639051047));
#70837=CARTESIAN_POINT('Ctrl Pts',(0.00328965716626947,-0.034644428984174,
0.0772660859222573));
#70838=CARTESIAN_POINT('',(0.00308481599410115,-0.0351951634053267,0.0769225388992395));
#70839=CARTESIAN_POINT('',(0.00320299790920465,-0.0348678972925388,0.0771272482313852));
#70840=CARTESIAN_POINT('Origin',(0.0173149102123577,-0.0345636767888238,
0.0680959362170143));
#70841=CARTESIAN_POINT('Origin',(-0.00625109662106326,-0.0346946199340714,
0.0828473081894833));
#70842=CARTESIAN_POINT('',(0.00313945274522816,-0.0346945769330289,0.0770195966533715));
#70843=CARTESIAN_POINT('',(0.00317180649912508,-0.0346945769458128,0.0770730708125184));
#70844=CARTESIAN_POINT('',(0.00302576498971699,-0.0350221583435276,0.0768123947103925));
#70845=CARTESIAN_POINT('Origin',(0.0175983524926475,-0.0345628458717151,
0.0684842709518878));
#70846=CARTESIAN_POINT('',(0.00302685996691316,-0.0351951360298762,0.0768118194559413));
#70847=CARTESIAN_POINT('Origin',(-0.0067403848516491,-0.0351951838366744,
0.0819126794330099));
#70848=CARTESIAN_POINT('',(0.00308483367267652,-0.0351951371328749,0.0769225661055733));
#70849=CARTESIAN_POINT('Ctrl Pts',(0.00270058752120605,-0.0350241211494343,
0.0767168968718439));
#70850=CARTESIAN_POINT('Ctrl Pts',(0.00273594547314701,-0.0349144232818962,
0.0767915991548529));
#70851=CARTESIAN_POINT('Ctrl Pts',(0.00277286873809569,-0.0348045283579412,
0.076865615276647));
#70852=CARTESIAN_POINT('Ctrl Pts',(0.00281131354996476,-0.0346945769439158,
0.0769388486720593));
#70853=CARTESIAN_POINT('Ctrl Pts',(0.00280941048797988,-0.0350241211494343,
0.0767484991455839));
#70854=CARTESIAN_POINT('Ctrl Pts',(0.00284520374828418,-0.0349144232818962,
0.0768217024368448));
#70855=CARTESIAN_POINT('Ctrl Pts',(0.00288253159691867,-0.0348045283579412,
0.076894209671537));
#70856=CARTESIAN_POINT('Ctrl Pts',(0.00292134967765577,-0.0346945769439158,
0.0769659261979021));
#70857=CARTESIAN_POINT('Ctrl Pts',(0.00291823345475372,-0.0350241211494343,
0.0767801014193239));
#70858=CARTESIAN_POINT('Ctrl Pts',(0.00295446202342134,-0.0349144232818962,
0.0768518057188366));
#70859=CARTESIAN_POINT('Ctrl Pts',(0.00299219445574165,-0.0348045283579412,
0.0769228040664269));
#70860=CARTESIAN_POINT('Ctrl Pts',(0.00303138580534677,-0.0346945769439158,
0.0769930037237449));
#70861=CARTESIAN_POINT('Ctrl Pts',(0.00302705642152756,-0.0350241211494343,
0.0768117036930639));
#70862=CARTESIAN_POINT('Ctrl Pts',(0.00306372029855851,-0.0349144232818962,
0.0768819090008284));
#70863=CARTESIAN_POINT('Ctrl Pts',(0.00310185731456463,-0.0348045283579412,
0.0769513984613169));
#70864=CARTESIAN_POINT('Ctrl Pts',(0.00314142193303777,-0.0346945769439158,
0.0770200812495877));
#70865=CARTESIAN_POINT('',(0.00297538314480101,-0.0346945769458128,0.076979222657589));
#70866=CARTESIAN_POINT('Ctrl Pts',(0.00280536863782169,-0.0347116136492789,
0.0769274947695302));
#70867=CARTESIAN_POINT('Ctrl Pts',(0.00284343174786804,-0.0347621546532333,
0.0769076166446031));
#70868=CARTESIAN_POINT('Ctrl Pts',(0.00288082560558245,-0.034813308409711,
0.0768880880308286));
#70869=CARTESIAN_POINT('Ctrl Pts',(0.00295430602405962,-0.0349168561544566,
0.0768497135276311));
#70870=CARTESIAN_POINT('Ctrl Pts',(0.0029903634388798,-0.0349692089015919,
0.0768308828594206));
#70871=CARTESIAN_POINT('Ctrl Pts',(0.00302576498975863,-0.0350221583435,
0.0768123947103933));
#70872=CARTESIAN_POINT('Ctrl Pts',(0.00308527177353325,-0.0351951371254878,
0.0769211702232192));
#70873=CARTESIAN_POINT('Ctrl Pts',(0.00314256397920663,-0.0350307338980923,
0.0770253382648744));
#70874=CARTESIAN_POINT('Ctrl Pts',(0.0032041126065885,-0.0348659306897825,
0.0771270493468694));
#70875=CARTESIAN_POINT('Ctrl Pts',(0.00308483367277792,-0.0351951371254878,
0.0769225661055166));
#70876=CARTESIAN_POINT('Ctrl Pts',(0.003142154737442,-0.0350307338980923,
0.07702674320463));
#70877=CARTESIAN_POINT('Ctrl Pts',(0.00320373257350924,-0.0348659306897825,
0.0771284621435705));
#70878=CARTESIAN_POINT('Ctrl Pts',(0.00301140752959325,-0.0351951371254878,
0.0771565174333589));
#70879=CARTESIAN_POINT('Ctrl Pts',(0.00307356539117437,-0.0350307338980923,
0.0772622125719135));
#70880=CARTESIAN_POINT('Ctrl Pts',(0.00314003863335222,-0.0348659306897825,
0.0773652483431038));
#70881=CARTESIAN_POINT('Origin',(-0.00134716617794425,-0.0308609197410127,
0.0798802581581213));
#70882=CARTESIAN_POINT('',(0.00305282152988927,-0.0351951371254878,0.0770245636095533));
#70883=CARTESIAN_POINT('Origin',(0.0088776768623139,-0.0351840467441197,
0.0735283984580129));
#70884=CARTESIAN_POINT('Origin',(-0.00167966696799405,-0.0352322612925457,
0.0810102763570714));
#70885=CARTESIAN_POINT('',(0.00332966794130894,-0.0351951142564661,0.07732715015763));
#70886=CARTESIAN_POINT('',(0.00340076684006047,-0.0351951372916787,0.0774295771030537));
#70887=CARTESIAN_POINT('Origin',(0.00843588221042041,-0.0352875123163659,
0.074286406577489));
#70888=CARTESIAN_POINT('Origin',(0.00510351715950868,-0.0298325076522393,
0.0672817258785396));
#70889=CARTESIAN_POINT('Origin',(-5.41234501965848E-5,-0.033873131987072,
0.0759873405662144));
#70890=CARTESIAN_POINT('Ctrl Pts',(0.00237776779016926,-0.0321934096636941,
0.0739021003700527));
#70891=CARTESIAN_POINT('Ctrl Pts',(0.00237333050484116,-0.0320508460843169,
0.0740049512916559));
#70892=CARTESIAN_POINT('Ctrl Pts',(0.00237165996656505,-0.0319086045660766,
0.0741078438844261));
#70893=CARTESIAN_POINT('Ctrl Pts',(0.00237274153327594,-0.0317669892864456,
0.0742105563063861));
#70894=CARTESIAN_POINT('Ctrl Pts',(0.00237597585284884,-0.0321934096636941,
0.0739859288949626));
#70895=CARTESIAN_POINT('Ctrl Pts',(0.00237303905819812,-0.0320508460843169,
0.0740888118913904));
#70896=CARTESIAN_POINT('Ctrl Pts',(0.00237286874101169,-0.0319086045660766,
0.0741916962195769));
#70897=CARTESIAN_POINT('Ctrl Pts',(0.00237544703044969,-0.0317669892864456,
0.0742943603212735));
#70898=CARTESIAN_POINT('Ctrl Pts',(0.00237418391552844,-0.0321934096636941,
0.0740697574198723));
#70899=CARTESIAN_POINT('Ctrl Pts',(0.00237274761155508,-0.0320508460843169,
0.074172672491125));
#70900=CARTESIAN_POINT('Ctrl Pts',(0.00237407751545835,-0.0319086045660766,
0.0742755485547279));
#70901=CARTESIAN_POINT('Ctrl Pts',(0.00237815252762344,-0.0317669892864456,
0.074378164336161));
#70902=CARTESIAN_POINT('Ctrl Pts',(0.00237239197820803,-0.0321934096636941,
0.0741535859447821));
#70903=CARTESIAN_POINT('Ctrl Pts',(0.00237245616491203,-0.0320508460843169,
0.0742565330908595));
#70904=CARTESIAN_POINT('Ctrl Pts',(0.00237528628990499,-0.0319086045660766,
0.0743594008898788));
#70905=CARTESIAN_POINT('Ctrl Pts',(0.00238085802479719,-0.0317669892864456,
0.0744619683510483));
#70906=CARTESIAN_POINT('',(0.00237242403632313,-0.0321934096636941,0.0741520862359061));
#70907=CARTESIAN_POINT('',(0.00237736578083819,-0.0318665617511273,0.0743883766050468));
#70908=CARTESIAN_POINT('Origin',(0.0190711415859749,-0.0326371944419006,
0.0747609680271806));
#70909=CARTESIAN_POINT('Origin',(-0.0085744009303593,-0.0316939261509138,
0.0748426849382173));
#70910=CARTESIAN_POINT('',(0.00237377816213862,-0.0320197221621803,0.0740273508648053));
#70911=CARTESIAN_POINT('Ctrl Pts',(0.00237372717616906,-0.0320197392094719,
0.074027528671752));
#70912=CARTESIAN_POINT('Ctrl Pts',(0.00237310404960662,-0.0319792716576016,
0.0740567868012731));
#70913=CARTESIAN_POINT('Ctrl Pts',(0.00237270113853826,-0.0319386439829655,
0.0740861828754044));
#70914=CARTESIAN_POINT('Ctrl Pts',(0.00237252647670892,-0.0318979099381587,
0.0741157478703721));
#70915=CARTESIAN_POINT('Ctrl Pts',(0.0023723518183319,-0.0318571766984894,
0.0741453122809667));
#70916=CARTESIAN_POINT('Ctrl Pts',(0.00237240450624418,-0.0318163871833549,
0.0741748953295478));
#70917=CARTESIAN_POINT('Ctrl Pts',(0.00237268083807216,-0.0317755399638303,
0.0742043952688851));
#70918=CARTESIAN_POINT('',(0.00237509545404048,-0.0321934096636183,0.074027114785002));
#70919=CARTESIAN_POINT('Origin',(6.75629272769168E-5,-0.03241117574553,
0.0739988197263972));
#70920=CARTESIAN_POINT('',(0.0023737597451918,-0.0321934096636663,0.074089600510464));
#70921=CARTESIAN_POINT('Ctrl Pts',(0.00237388852889845,-0.0321934096636617,
0.0741506830435188));
#70922=CARTESIAN_POINT('Ctrl Pts',(0.00237389794860091,-0.0320835708272591,
0.0742299785583533));
#70923=CARTESIAN_POINT('Ctrl Pts',(0.00237554837939786,-0.0319739230346488,
0.0743092278836263));
#70924=CARTESIAN_POINT('Ctrl Pts',(0.00237882992797032,-0.0318646057455572,
0.0743883297873848));
#70925=CARTESIAN_POINT('Ctrl Pts',(0.00229206583874311,-0.0321934096636617,
0.0742290808249946));
#70926=CARTESIAN_POINT('Ctrl Pts',(0.00229315642495177,-0.0320835708272591,
0.0743095047384952));
#70927=CARTESIAN_POINT('Ctrl Pts',(0.00229591074728617,-0.0319739230346488,
0.0743898594332326));
#70928=CARTESIAN_POINT('Ctrl Pts',(0.00230031739153543,-0.0318646057455572,
0.0744700423714043));
#70929=CARTESIAN_POINT('Ctrl Pts',(0.00221024314858776,-0.0321934096636617,
0.0743074786064704));
#70930=CARTESIAN_POINT('Ctrl Pts',(0.00221241490130264,-0.0320835708272591,
0.0743890309186371));
#70931=CARTESIAN_POINT('Ctrl Pts',(0.00221627311517448,-0.0319739230346488,
0.074470490982839));
#70932=CARTESIAN_POINT('Ctrl Pts',(0.00222180485510055,-0.0318646057455572,
0.0745517549554239));
#70933=CARTESIAN_POINT('Ctrl Pts',(0.00212842045843242,-0.0321934096636617,
0.0743858763879462));
#70934=CARTESIAN_POINT('Ctrl Pts',(0.0021316733776535,-0.0320835708272591,
0.0744685570987791));
#70935=CARTESIAN_POINT('Ctrl Pts',(0.00213663548306279,-0.0319739230346488,
0.0745511225324453));
#70936=CARTESIAN_POINT('Ctrl Pts',(0.00214329231866566,-0.0318646057455572,
0.0746334675394434));
#70937=CARTESIAN_POINT('',(0.00212893797363555,-0.0321763980308259,0.0743986820498694));
#70938=CARTESIAN_POINT('',(0.00212842045843431,-0.0321934096636184,0.0743858763879783));
#70939=CARTESIAN_POINT('Origin',(0.018676471018924,-0.0326386230645992,
0.0743262766362804));
#70940=CARTESIAN_POINT('Ctrl Pts',(0.00212893797680168,-0.0321763980306269,
0.0743986820497332));
#70941=CARTESIAN_POINT('Ctrl Pts',(0.0021718199901083,-0.0321259596175228,
0.0743969031900029));
#70942=CARTESIAN_POINT('Ctrl Pts',(0.00221395901689214,-0.0320749164632234,
0.0743951551513188));
#70943=CARTESIAN_POINT('Ctrl Pts',(0.00229678500966819,-0.0319716057793904,
0.0743917193093));
#70944=CARTESIAN_POINT('Ctrl Pts',(0.00233743970376939,-0.0319193786690102,
0.0743900328446889));
#70945=CARTESIAN_POINT('Ctrl Pts',(0.0023773657826883,-0.0318665617525285,
0.0743883766049627));
#70946=CARTESIAN_POINT('',(0.00225042224738872,-0.0321934096636663,0.0742689813119522));
#70947=CARTESIAN_POINT('Origin',(0.00812378219310841,-0.0315241814719618,
0.07415));
#70948=CARTESIAN_POINT('',(0.00212893797326352,-0.0322104233323776,0.0743986820498849));
#70949=CARTESIAN_POINT('',(0.00212948283705857,-0.0321934096636183,0.0744114865772715));
#70950=CARTESIAN_POINT('Origin',(0.0186809237928152,-0.032638722891123,
0.0742811607215313));
#70951=CARTESIAN_POINT('Origin',(0.0186256182595173,-0.0326386247204135,
0.07310032358825));
#70952=CARTESIAN_POINT('Origin',(0.0186337858873733,-0.0326387241141357,
0.0731449165497552));
#70953=CARTESIAN_POINT('Ctrl Pts',(0.00237294299327498,-0.0327445246967096,
0.0742272884057232));
#70954=CARTESIAN_POINT('Ctrl Pts',(0.0023758579731503,-0.0324436878339359,
0.0744441848519215));
#70955=CARTESIAN_POINT('Ctrl Pts',(0.00239510219866997,-0.0321434074405927,
0.0746602455500255));
#70956=CARTESIAN_POINT('Ctrl Pts',(0.00238173477963596,-0.0327445246967096,
0.0744771337668821));
#70957=CARTESIAN_POINT('Ctrl Pts',(0.00239407283135373,-0.0324436878339359,
0.0746936986254369));
#70958=CARTESIAN_POINT('Ctrl Pts',(0.00242268838222746,-0.0321434074405927,
0.0749087188936194));
#70959=CARTESIAN_POINT('',(0.00238390402370576,-0.0326943950436612,0.0745132128858064));
#70960=CARTESIAN_POINT('',(0.00240367281091007,-0.0323666188837389,0.0747487266953189));
#70961=CARTESIAN_POINT('Origin',(0.019156326270843,-0.0326395579110921,
0.0733757111555328));
#70962=CARTESIAN_POINT('Origin',(-0.00858092611035353,-0.0321933825603038,
0.0758984911828047));
#70963=CARTESIAN_POINT('',(0.00239201124118077,-0.0321934096532689,0.0746242644318081));
#70964=CARTESIAN_POINT('',(0.00239851760275117,-0.0321934096584275,0.0746864248501227));
#70965=CARTESIAN_POINT('',(0.00237736577988581,-0.0325210109756238,0.0743883766050745));
#70966=CARTESIAN_POINT('Origin',(0.0191613237731052,-0.0326393129154959,
0.0738565016030731));
#70967=CARTESIAN_POINT('',(0.00237872314766527,-0.0326943950436593,0.0743883202978606));
#70968=CARTESIAN_POINT('Origin',(-0.00867422623493687,-0.032694376553816,
0.0748468250876423));
#70969=CARTESIAN_POINT('',(0.00238131358569552,-0.0326943950436702,0.0744507665918435));
#70970=CARTESIAN_POINT('Ctrl Pts',(0.00212379740907037,-0.0325229783203769,
0.074163512636487));
#70971=CARTESIAN_POINT('Ctrl Pts',(0.00212398368046884,-0.032413025309245,
0.0742462222955239));
#70972=CARTESIAN_POINT('Ctrl Pts',(0.00212588087916087,-0.0323031222208069,
0.0743289155567573));
#70973=CARTESIAN_POINT('Ctrl Pts',(0.00212948283725399,-0.0321934096576658,
0.0744114865817515));
#70974=CARTESIAN_POINT('Ctrl Pts',(0.00220880776720183,-0.0325229783203769,
0.0742384418113572));
#70975=CARTESIAN_POINT('Ctrl Pts',(0.0022100269356373,-0.032413025309245,
0.0743199796044664));
#70976=CARTESIAN_POINT('Ctrl Pts',(0.00221293263315515,-0.0323031222208069,
0.0744014798107064));
#70977=CARTESIAN_POINT('Ctrl Pts',(0.00221751745397346,-0.0321934096576658,
0.074482838165444));
#70978=CARTESIAN_POINT('Ctrl Pts',(0.00229381812533329,-0.0325229783203769,
0.0743133709862274));
#70979=CARTESIAN_POINT('Ctrl Pts',(0.00229607019080575,-0.032413025309245,
0.0743937369134088));
#70980=CARTESIAN_POINT('Ctrl Pts',(0.00229998438714944,-0.0323031222208069,
0.0744740440646555));
#70981=CARTESIAN_POINT('Ctrl Pts',(0.00230555207069293,-0.0321934096576658,
0.0745541897491365));
#70982=CARTESIAN_POINT('Ctrl Pts',(0.00237882848346475,-0.0325229783203769,
0.0743883001610976));
#70983=CARTESIAN_POINT('Ctrl Pts',(0.0023821134459742,-0.032413025309245,
0.0744674942223513));
#70984=CARTESIAN_POINT('Ctrl Pts',(0.00238703614114373,-0.0323031222208069,
0.0745466083186045));
#70985=CARTESIAN_POINT('Ctrl Pts',(0.00239358668741239,-0.0321934096576658,
0.074625541332829));
#70986=CARTESIAN_POINT('',(0.00226074703894315,-0.0321934096584275,0.0745178755040674));
#70987=CARTESIAN_POINT('Ctrl Pts',(0.0021289379767339,-0.0322104233328922,
0.074398682049736));
#70988=CARTESIAN_POINT('Ctrl Pts',(0.00217187809590104,-0.0322609421831419,
0.0743969007796203));
#70989=CARTESIAN_POINT('Ctrl Pts',(0.00221404550838051,-0.0323120888240847,
0.0743951515634291));
#70990=CARTESIAN_POINT('Ctrl Pts',(0.00229687212817822,-0.032415652463181,
0.0743917156953997));
#70991=CARTESIAN_POINT('Ctrl Pts',(0.00233749728942868,-0.0324680267167306,
0.0743900304558829));
#70992=CARTESIAN_POINT('Ctrl Pts',(0.00237736577992929,-0.0325210109755912,
0.0743883766050771));
#70993=CARTESIAN_POINT('Origin',(0.0087468097105921,-0.0262834582511982,
0.0663068359349611));
#70994=CARTESIAN_POINT('Origin',(-0.00296606493112828,-0.0342770791904115,
0.0691661651794213));
#70995=CARTESIAN_POINT('Ctrl Pts',(0.00238527718595703,-0.0326943950436604,
0.0745117208682917));
#70996=CARTESIAN_POINT('Ctrl Pts',(0.00239026237745925,-0.0325844576448134,
0.0745908082223948));
#70997=CARTESIAN_POINT('Ctrl Pts',(0.00239688357791956,-0.0324744968375322,
0.0746697980716994));
#70998=CARTESIAN_POINT('Ctrl Pts',(0.0024051309079293,-0.0323646534831894,
0.0747485893268164));
#70999=CARTESIAN_POINT('Ctrl Pts',(0.00230853870272208,-0.0326943950436604,
0.0745951015181593));
#71000=CARTESIAN_POINT('Ctrl Pts',(0.00231467303585146,-0.0325844576448134,
0.0746752464723846));
#71001=CARTESIAN_POINT('Ctrl Pts',(0.00232246533216997,-0.0324744968375322,
0.0747552702305265));
#71002=CARTESIAN_POINT('Ctrl Pts',(0.00233190419352096,-0.0323646534831894,
0.0748350703991877));
#71003=CARTESIAN_POINT('Ctrl Pts',(0.00223180021948713,-0.0326943950436604,
0.0746784821680268));
#71004=CARTESIAN_POINT('Ctrl Pts',(0.00223908369424368,-0.0325844576448134,
0.0747596847223744));
#71005=CARTESIAN_POINT('Ctrl Pts',(0.00224804708642038,-0.0324744968375322,
0.0748407423893536));
#71006=CARTESIAN_POINT('Ctrl Pts',(0.00225867747911263,-0.0323646534831894,
0.0749215514715591));
#71007=CARTESIAN_POINT('Ctrl Pts',(0.00215506173625218,-0.0326943950436604,
0.0747618628178944));
#71008=CARTESIAN_POINT('Ctrl Pts',(0.0021634943526359,-0.0325844576448134,
0.0748441229723642));
#71009=CARTESIAN_POINT('Ctrl Pts',(0.0021736288406708,-0.0324744968375322,
0.0749262145481808));
#71010=CARTESIAN_POINT('Ctrl Pts',(0.0021854507647043,-0.0323646534831894,
0.0750080325439304));
#71011=CARTESIAN_POINT('',(0.00215638230421628,-0.0326773559991335,0.0747746107157097));
#71012=CARTESIAN_POINT('',(0.00215506173625341,-0.0326943950436594,0.0747618628178938));
#71013=CARTESIAN_POINT('Origin',(0.0186660739182752,-0.0326395670545172,
0.0729960178679478));
#71014=CARTESIAN_POINT('Ctrl Pts',(0.00215638230754539,-0.0326773559987419,
0.074774610715356));
#71015=CARTESIAN_POINT('Ctrl Pts',(0.00219910235802171,-0.0326267922586414,
0.0747701391864154));
#71016=CARTESIAN_POINT('Ctrl Pts',(0.00224106522645314,-0.0325756109580267,
0.0747657469120963));
#71017=CARTESIAN_POINT('Ctrl Pts',(0.0023235123118499,-0.0324719985462364,
0.0747571171346427));
#71018=CARTESIAN_POINT('Ctrl Pts',(0.00236396346142973,-0.0324196091621776,
0.074752883092688));
#71019=CARTESIAN_POINT('Ctrl Pts',(0.00240367281095859,-0.0323666188837757,
0.0747487266953138));
#71020=CARTESIAN_POINT('',(0.00226948287998959,-0.0326943950436702,0.0746375378518601));
#71021=CARTESIAN_POINT('Origin',(0.00812378219310841,-0.0315241814719618,
0.07415));
#71022=CARTESIAN_POINT('',(0.00215638230425946,-0.0327114338380047,0.0747746107157052));
#71023=CARTESIAN_POINT('',(0.00215773009560762,-0.0326943950436593,0.0747873557640231));
#71024=CARTESIAN_POINT('Origin',(0.0186605887082149,-0.0326395662378234,
0.0729510394200869));
#71025=CARTESIAN_POINT('Origin',(0.0186765368098082,-0.0326395681387481,
0.0730959516853406));
#71026=CARTESIAN_POINT('Origin',(0.0186804785953922,-0.0326395674485255,
0.0731410915149567));
#71027=CARTESIAN_POINT('Ctrl Pts',(0.00238914692877785,-0.0332451089994433,
0.0745882731854638));
#71028=CARTESIAN_POINT('Ctrl Pts',(0.00240567667240838,-0.0329451141710254,
0.074804558493071));
#71029=CARTESIAN_POINT('Ctrl Pts',(0.00243845095033208,-0.0326442513127494,
0.0750189842690818));
#71030=CARTESIAN_POINT('Ctrl Pts',(0.00241361098337932,-0.0332451089994433,
0.0748370733262042));
#71031=CARTESIAN_POINT('Ctrl Pts',(0.00243952437784246,-0.0329451141710254,
0.0750524359568965));
#71032=CARTESIAN_POINT('Ctrl Pts',(0.0024815861488399,-0.0326442513127494,
0.0752652348622784));
#71033=CARTESIAN_POINT('Ctrl Pts',(0.00241385562392534,-0.0332451089994433,
0.0748395613276117));
#71034=CARTESIAN_POINT('Ctrl Pts',(0.0024398628548968,-0.0329451141710254,
0.0750549147315347));
#71035=CARTESIAN_POINT('Ctrl Pts',(0.00248201750082498,-0.0326442513127494,
0.0752676973682104));
#71036=CARTESIAN_POINT('',(0.00241803668792225,-0.0331951640388616,0.0748729061004368));
#71037=CARTESIAN_POINT('',(0.00245255449673062,-0.0328677532354998,0.0751067138995858));
#71038=CARTESIAN_POINT('Origin',(0.0189351097397747,-0.0326402808282397,
0.0720061055721766));
#71039=CARTESIAN_POINT('Origin',(-0.00844931148379163,-0.0326944278779101,
0.076946197824319));
#71040=CARTESIAN_POINT('',(0.00243310089257869,-0.0326943950436593,0.0749832294616745));
#71041=CARTESIAN_POINT('',(0.00244349750017906,-0.0326943950436693,0.0750448586800035));
#71042=CARTESIAN_POINT('',(0.00240367281090978,-0.0330220786163545,0.074748726695316));
#71043=CARTESIAN_POINT('Origin',(0.0190458952612445,-0.0326396682766514,
0.0724739508603131));
#71044=CARTESIAN_POINT('',(0.00240502396467458,-0.0331951640388587,0.0747485852693819));
#71045=CARTESIAN_POINT('Origin',(-0.00856669033432262,-0.0331952026560096,
0.0758969993447738));
#71046=CARTESIAN_POINT('',(0.00241153032630842,-0.0331951640388701,0.0748107456849194));
#71047=CARTESIAN_POINT('Ctrl Pts',(0.00213648553643562,-0.0330240426238172,
0.0745402290929985));
#71048=CARTESIAN_POINT('Ctrl Pts',(0.00214186132237346,-0.032914277406352,
0.0746227099375847));
#71049=CARTESIAN_POINT('Ctrl Pts',(0.00214894489779314,-0.0328043479726691,
0.0747051207693682));
#71050=CARTESIAN_POINT('Ctrl Pts',(0.00215773009560757,-0.0326943950436594,
0.0747873557640232));
#71051=CARTESIAN_POINT('Ctrl Pts',(0.00222603297718474,-0.0330240426238172,
0.0746096725364601));
#71052=CARTESIAN_POINT('Ctrl Pts',(0.00223236541421173,-0.032914277406352,
0.0746909197778081));
#71053=CARTESIAN_POINT('Ctrl Pts',(0.00224038061562119,-0.0328043479726691,
0.0747720766147069));
#71054=CARTESIAN_POINT('Ctrl Pts',(0.0022500711766021,-0.0326943950436594,
0.0748530387964234));
#71055=CARTESIAN_POINT('Ctrl Pts',(0.00231558041793386,-0.0330240426238172,
0.0746791159799217));
#71056=CARTESIAN_POINT('Ctrl Pts',(0.00232286950605001,-0.032914277406352,
0.0747591296180316));
#71057=CARTESIAN_POINT('Ctrl Pts',(0.00233181633344924,-0.0328043479726691,
0.0748390324600457));
#71058=CARTESIAN_POINT('Ctrl Pts',(0.00234241225759662,-0.0326943950436594,
0.0749187218288236));
#71059=CARTESIAN_POINT('Ctrl Pts',(0.00240512785868298,-0.0330240426238172,
0.0747485594233833));
#71060=CARTESIAN_POINT('Ctrl Pts',(0.00241337359788828,-0.032914277406352,
0.074827339458255));
#71061=CARTESIAN_POINT('Ctrl Pts',(0.00242325205127729,-0.0328043479726691,
0.0749059883053845));
#71062=CARTESIAN_POINT('Ctrl Pts',(0.00243475333859115,-0.0326943950436594,
0.0749844048612238));
#71063=CARTESIAN_POINT('',(0.00229541549410315,-0.0326943950436694,0.0748852926128588));
#71064=CARTESIAN_POINT('Ctrl Pts',(0.00215638230755161,-0.0327114338383319,
0.0747746107153553));
#71065=CARTESIAN_POINT('Ctrl Pts',(0.00219909525233674,-0.0327619876831146,
0.074770139930171));
#71066=CARTESIAN_POINT('Ctrl Pts',(0.00224105465004281,-0.0328131562604706,
0.0747657480191344));
#71067=CARTESIAN_POINT('Ctrl Pts',(0.00232350165961882,-0.0329167375858765,
0.074757118249617));
#71068=CARTESIAN_POINT('Ctrl Pts',(0.00236395642039812,-0.0329691088920619,
0.0747528838296762));
#71069=CARTESIAN_POINT('Ctrl Pts',(0.00240367281095737,-0.0330220786163186,
0.0747487266953138));
#71070=CARTESIAN_POINT('Ctrl Pts',(0.00241931365983049,-0.0331951640388604,
0.0748713305540121));
#71071=CARTESIAN_POINT('Ctrl Pts',(0.00243422670656056,-0.0330306422010619,
0.0749892667835727));
#71072=CARTESIAN_POINT('Ctrl Pts',(0.00245400143858907,-0.0328657861914645,
0.0751064858655472));
#71073=CARTESIAN_POINT('Ctrl Pts',(0.00241803668792191,-0.0331951640388604,
0.0748729061004337));
#71074=CARTESIAN_POINT('Ctrl Pts',(0.00243298230806411,-0.0330306422010619,
0.0749908687305697));
#71075=CARTESIAN_POINT('Ctrl Pts',(0.00245279067683453,-0.0328657861914645,
0.0751081128442673));
#71076=CARTESIAN_POINT('Ctrl Pts',(0.0022052588268649,-0.0331951640388604,
0.0751354345048016));
#71077=CARTESIAN_POINT('Ctrl Pts',(0.00222563205344984,-0.0330306422010619,
0.0752577961807944));
#71078=CARTESIAN_POINT('Ctrl Pts',(0.00225104520800275,-0.0328657861914645,
0.0753792112527129));
#71079=CARTESIAN_POINT('',(0.00220737723472213,-0.0331781648281902,0.0751480743279835));
#71080=CARTESIAN_POINT('',(0.00220525882686678,-0.0331951640388588,0.0751354345048006));
#71081=CARTESIAN_POINT('Origin',(0.0183658543510097,-0.0326412091878594,
0.0716998723397664));
#71082=CARTESIAN_POINT('Ctrl Pts',(0.00220737723551375,-0.033178164828644,
0.0751480743263201));
#71083=CARTESIAN_POINT('Ctrl Pts',(0.00224976137579082,-0.0331276811546775,
0.0751409242756966));
#71084=CARTESIAN_POINT('Ctrl Pts',(0.00229138018412607,-0.0330765663497782,
0.075133903299499));
#71085=CARTESIAN_POINT('Ctrl Pts',(0.00237312292174858,-0.0329730614463176,
0.0751201136235957));
#71086=CARTESIAN_POINT('Ctrl Pts',(0.00241321382965176,-0.0329207133373706,
0.0751133504999028));
#71087=CARTESIAN_POINT('Ctrl Pts',(0.00245255448581311,-0.0328677532289357,
0.0751067138872499));
#71088=CARTESIAN_POINT('',(0.00231164775740451,-0.0331951640388701,0.0750041703026287));
#71089=CARTESIAN_POINT('Origin',(0.00812378219310841,-0.0315241814719618,
0.07415));
#71090=CARTESIAN_POINT('',(0.00220737723635824,-0.033212160714422,0.0751480743283634));
#71091=CARTESIAN_POINT('',(0.00220952263615501,-0.0331951640388587,0.0751607095987539));
#71092=CARTESIAN_POINT('Origin',(0.0183506938193972,-0.0326413645221128,
0.0716571354312258));
#71093=CARTESIAN_POINT('Origin',(0.0186028220668772,-0.0326412102403194,
0.0731045558557979));
#71094=CARTESIAN_POINT('Origin',(0.0186025147681812,-0.0326413657479853,
0.0731499018936054));
#71095=CARTESIAN_POINT('Ctrl Pts',(0.00242797943404241,-0.0337436976235975,
0.0749474684506714));
#71096=CARTESIAN_POINT('Ctrl Pts',(0.00243515198614739,-0.0336723290703325,
0.074998697363909));
#71097=CARTESIAN_POINT('Ctrl Pts',(0.00244324482458147,-0.033601104548885,
0.0750497889779105));
#71098=CARTESIAN_POINT('Ctrl Pts',(0.00246908365460051,-0.0333736987606857,
0.0752129143807388));
#71099=CARTESIAN_POINT('Ctrl Pts',(0.00250424098045896,-0.0331450831799192,
0.0753742881847566));
#71100=CARTESIAN_POINT('Ctrl Pts',(0.002468016610698,-0.0337436976235975,
0.0751942416754861));
#71101=CARTESIAN_POINT('Ctrl Pts',(0.00247740867858648,-0.0336723290703325,
0.075245110488289));
#71102=CARTESIAN_POINT('Ctrl Pts',(0.00248771419666688,-0.033601104548885,
0.0752958021380185));
#71103=CARTESIAN_POINT('Ctrl Pts',(0.00252061767448949,-0.0333736987606857,
0.0754576505341546));
#71104=CARTESIAN_POINT('Ctrl Pts',(0.00256275472416368,-0.0331450831799192,
0.0756173440256608));
#71105=CARTESIAN_POINT('Ctrl Pts',(0.00246841698246456,-0.0337436976235975,
0.0751967094077343));
#71106=CARTESIAN_POINT('Ctrl Pts',(0.00247783124551087,-0.0336723290703325,
0.0752475746195329));
#71107=CARTESIAN_POINT('Ctrl Pts',(0.00248815889038774,-0.033601104548885,
0.0752982622696196));
#71108=CARTESIAN_POINT('Ctrl Pts',(0.00252113301468838,-0.0333736987606857,
0.0754600978956887));
#71109=CARTESIAN_POINT('Ctrl Pts',(0.00256333986160073,-0.0331450831799192,
0.0756197745840699));
#71110=CARTESIAN_POINT('',(0.00247468732294312,-0.0336938721132548,0.0752297463349663));
#71111=CARTESIAN_POINT('',(0.00252381793631918,-0.0333679869945435,0.0754609253688133));
#71112=CARTESIAN_POINT('Ctrl Pts',(0.00247468732294426,-0.0336938721132647,
0.0752297463349778));
#71113=CARTESIAN_POINT('Ctrl Pts',(0.00247890207940818,-0.033662918793393,
0.0752517974022936));
#71114=CARTESIAN_POINT('Ctrl Pts',(0.00248324460575755,-0.0336319952301038,
0.0752738167380591));
#71115=CARTESIAN_POINT('Ctrl Pts',(0.00248771419666878,-0.0336011045488948,
0.0752958021380299));
#71116=CARTESIAN_POINT('Ctrl Pts',(0.00249892992967298,-0.0335235892595452,
0.075350971029537));
#71117=CARTESIAN_POINT('Ctrl Pts',(0.00251096583808578,-0.0334458668660367,
0.0754060242342462));
#71118=CARTESIAN_POINT('Ctrl Pts',(0.0025238179360017,-0.0333679869945383,
0.0754609253688804));
#71119=CARTESIAN_POINT('Ctrl Pts',(0.00252382740301007,-0.033367969246074,
0.0754609688251143));
#71120=CARTESIAN_POINT('Ctrl Pts',(0.00252426733563364,-0.0333391895375059,
0.0754608597512404));
#71121=CARTESIAN_POINT('Ctrl Pts',(0.00252459630517395,-0.0333104081060432,
0.0754607748432893));
#71122=CARTESIAN_POINT('Ctrl Pts',(0.00252503036866947,-0.0332532697965678,
0.0754606570903441));
#71123=CARTESIAN_POINT('Ctrl Pts',(0.0025251387292648,-0.0332249169959204,
0.0754606234838277));
#71124=CARTESIAN_POINT('Ctrl Pts',(0.00252514073068577,-0.0331960985418316,
0.0754606159305638));
#71125=CARTESIAN_POINT('Ctrl Pts',(0.00252514073414812,-0.0331956312506232,
0.0754606158148028));
#71126=CARTESIAN_POINT('Ctrl Pts',(0.00252514070879179,-0.0331951640388587,
0.0754606157064865));
#71127=CARTESIAN_POINT('',(0.00249664906299847,-0.0331951640388587,0.075338906109001));
#71128=CARTESIAN_POINT('',(0.00251089488590508,-0.0331951640388687,0.0753997609077536));
#71129=CARTESIAN_POINT('',(0.00245255450076835,-0.0335216366567723,0.0751067138846023));
#71130=CARTESIAN_POINT('Origin',(0.0186300571953353,-0.0326434571528621,
0.0711495594033536));
#71131=CARTESIAN_POINT('',(0.00245389410775942,-0.0336938721132327,0.0751064878983125));
#71132=CARTESIAN_POINT('Origin',(-0.00831452423081074,-0.0336938867896226,
0.0769230771272436));
#71133=CARTESIAN_POINT('',(0.00246429071536126,-0.0336938721132538,0.0751681171166494));
#71134=CARTESIAN_POINT('Ctrl Pts',(0.0021728029088052,-0.0335235895815172,
0.0749154054858857));
#71135=CARTESIAN_POINT('Ctrl Pts',(0.00218334022226314,-0.0334144449262749,
0.0749973324321342));
#71136=CARTESIAN_POINT('Ctrl Pts',(0.00219558219087022,-0.0333049234473147,
0.0750791358095524));
#71137=CARTESIAN_POINT('Ctrl Pts',(0.00220952263615483,-0.0331951640388588,
0.0751607095987539));
#71138=CARTESIAN_POINT('Ctrl Pts',(0.00226653418144584,-0.0335235895815172,
0.0749790892437453));
#71139=CARTESIAN_POINT('Ctrl Pts',(0.00227794822721251,-0.0334144449262749,
0.075059725794486));
#71140=CARTESIAN_POINT('Ctrl Pts',(0.00229104127678745,-0.0333049234473147,
0.0751402191812586));
#71141=CARTESIAN_POINT('Ctrl Pts',(0.00230580591169218,-0.0331951640388588,
0.0752204649611722));
#71142=CARTESIAN_POINT('Ctrl Pts',(0.00236026545408649,-0.0335235895815172,
0.0750427730016049));
#71143=CARTESIAN_POINT('Ctrl Pts',(0.00237255623216187,-0.0334144449262749,
0.0751221191568377));
#71144=CARTESIAN_POINT('Ctrl Pts',(0.00238650036270467,-0.0333049234473147,
0.0752013025529648));
#71145=CARTESIAN_POINT('Ctrl Pts',(0.00240208918722953,-0.0331951640388588,
0.0752802203235906));
#71146=CARTESIAN_POINT('Ctrl Pts',(0.00245399672672714,-0.0335235895815172,
0.0751064567594644));
#71147=CARTESIAN_POINT('Ctrl Pts',(0.00246716423711124,-0.0334144449262749,
0.0751845125191895));
#71148=CARTESIAN_POINT('Ctrl Pts',(0.0024819594486219,-0.0333049234473147,
0.075262385924671));
#71149=CARTESIAN_POINT('Ctrl Pts',(0.00249837246276688,-0.0331951640388588,
0.075339975686009));
#71150=CARTESIAN_POINT('',(0.00235308584958674,-0.0331951640388687,0.0752498078538875));
#71151=CARTESIAN_POINT('Ctrl Pts',(0.00220737723944181,-0.0332121607145973,
0.0751480743278375));
#71152=CARTESIAN_POINT('Ctrl Pts',(0.00224969008078945,-0.0332625444109937,
0.0751409363173366));
#71153=CARTESIAN_POINT('Ctrl Pts',(0.00229127380548083,-0.0333135300747213,
0.075133921305958));
#71154=CARTESIAN_POINT('Ctrl Pts',(0.00237301603011546,-0.0334167203140618,
0.07512013171303));
#71155=CARTESIAN_POINT('Ctrl Pts',(0.00241314287066596,-0.0334688847587314,
0.0751133624722961));
#71156=CARTESIAN_POINT('Ctrl Pts',(0.00245255450148716,-0.03352163665624,
0.0751067138846404));
#71157=CARTESIAN_POINT('Ctrl Pts',(0.00247526687111416,-0.033693872113239,
0.0752289315719396));
#71158=CARTESIAN_POINT('Ctrl Pts',(0.00248158221563218,-0.0336474569764958,
0.0752619942064954));
#71159=CARTESIAN_POINT('Ctrl Pts',(0.002488284167301,-0.033601104548885,
0.075294980646497));
#71160=CARTESIAN_POINT('Ctrl Pts',(0.00250525196805112,-0.0334837508592656,
0.0753784947285229));
#71161=CARTESIAN_POINT('Ctrl Pts',(0.00252468701319737,-0.0333660264659098,
0.0754614693462026));
#71162=CARTESIAN_POINT('Ctrl Pts',(0.00247468732293934,-0.033693872113239,
0.0752297463349461));
#71163=CARTESIAN_POINT('Ctrl Pts',(0.00248100743653561,-0.0336474569764958,
0.0752628123617897));
#71164=CARTESIAN_POINT('Ctrl Pts',(0.00248771419666689,-0.033601104548885,
0.0752958021380185));
#71165=CARTESIAN_POINT('Ctrl Pts',(0.00250469417133847,-0.0334837508592656,
0.0753793246666048));
#71166=CARTESIAN_POINT('Ctrl Pts',(0.00252414163534938,-0.0333660264659098,
0.0754623073663972));
#71167=CARTESIAN_POINT('Ctrl Pts',(0.00227763838309537,-0.033693872113239,
0.075506769356708));
#71168=CARTESIAN_POINT('Ctrl Pts',(0.002285580004364,-0.0336474569764958,
0.0755409887763842));
#71169=CARTESIAN_POINT('Ctrl Pts',(0.00229392166298028,-0.033601104548885,
0.0755751128846199));
#71170=CARTESIAN_POINT('Ctrl Pts',(0.00231504082472912,-0.0334837508592656,
0.0756615072810482));
#71171=CARTESIAN_POINT('Ctrl Pts',(0.00233871075758991,-0.0333660264659098,
0.0757472379348749));
#71172=CARTESIAN_POINT('',(0.00228172151382143,-0.0336769361243754,0.0755175989980726));
#71173=CARTESIAN_POINT('',(0.00227881362529051,-0.0336938721132327,0.0755051171319192));
#71174=CARTESIAN_POINT('Ctrl Pts',(0.00228172151382151,-0.0336769361243751,
0.0755175989980729));
#71175=CARTESIAN_POINT('Ctrl Pts',(0.00228123460747909,-0.0336797586670031,
0.0755155190489053));
#71176=CARTESIAN_POINT('Ctrl Pts',(0.00228074883033805,-0.0336825812712857,
0.075513438918373));
#71177=CARTESIAN_POINT('Ctrl Pts',(0.00227977953466158,-0.0336882265989872,
0.0755092782977148));
#71178=CARTESIAN_POINT('Ctrl Pts',(0.00227929601612137,-0.0336910493223981,
0.0755071978075978));
#71179=CARTESIAN_POINT('Ctrl Pts',(0.00227881362528851,-0.0336938721132338,
0.0755051171319211));
#71180=CARTESIAN_POINT('Ctrl Pts',(0.00228172151382143,-0.0336769361243754,
0.0755175989980726));
#71181=CARTESIAN_POINT('Ctrl Pts',(0.00232253195311806,-0.0336279007642953,
0.0755080454656879));
#71182=CARTESIAN_POINT('Ctrl Pts',(0.0023639234699351,-0.0335767878888531,
0.0754983559057812));
#71183=CARTESIAN_POINT('Ctrl Pts',(0.00244503924067831,-0.0334733199122762,
0.0754793670843899));
#71184=CARTESIAN_POINT('Ctrl Pts',(0.00248481178595621,-0.0334209645148418,
0.0754700565181263));
#71185=CARTESIAN_POINT('Ctrl Pts',(0.00252381793464815,-0.0333679869844682,
0.0754609253617077));
#71186=CARTESIAN_POINT('',(0.00237675047412682,-0.0336938721132538,0.0753674317334528));
#71187=CARTESIAN_POINT('Origin',(0.00812378219310841,-0.0315241814719618,
0.07415));
#71188=CARTESIAN_POINT('',(0.00228172151508861,-0.033710812065583,0.0755175989977821));
#71189=CARTESIAN_POINT('',(0.00228465605720548,-0.0336938721132327,0.0755300746244476));
#71190=CARTESIAN_POINT('Origin',(0.0184669961080924,-0.034556251000384,
0.0728765208499561));
#71191=CARTESIAN_POINT('Ctrl Pts',(0.00228465605721286,-0.0336938721132298,
0.0755300746244498));
#71192=CARTESIAN_POINT('Ctrl Pts',(0.00228416478475723,-0.0336910493377706,
0.0755279960398684));
#71193=CARTESIAN_POINT('Ctrl Pts',(0.00228367460116839,-0.0336882266066734,
0.0755259171040297));
#71194=CARTESIAN_POINT('Ctrl Pts',(0.00228269641887757,-0.0336825812712869,
0.0755217585577134));
#71195=CARTESIAN_POINT('Ctrl Pts',(0.00228220842016392,-0.0336797586670037,
0.0755196789472403));
#71196=CARTESIAN_POINT('Ctrl Pts',(0.00228172151382139,-0.0336769361243751,
0.0755175989980724));
#71197=CARTESIAN_POINT('Origin',(0.0179575146465307,-0.0345562514382243,
0.0707001500671947));
#71198=CARTESIAN_POINT('Ctrl Pts',(0.00248928190141467,-0.0342436276873911,
0.0753034866548439));
#71199=CARTESIAN_POINT('Ctrl Pts',(0.00253278636778234,-0.033943005420181,
0.0755159953365952));
#71200=CARTESIAN_POINT('Ctrl Pts',(0.00259217426715855,-0.0336441434784052,
0.0757246233687993));
#71201=CARTESIAN_POINT('Ctrl Pts',(0.00254473290416811,-0.0342436276873911,
0.0755472594718143));
#71202=CARTESIAN_POINT('Ctrl Pts',(0.00259743141389354,-0.033943005420181,
0.0757576767845201));
#71203=CARTESIAN_POINT('Ctrl Pts',(0.00266582970682857,-0.0336441434784052,
0.0759635268560216));
#71204=CARTESIAN_POINT('Ctrl Pts',(0.00254528741419565,-0.0342436276873911,
0.075549697199984));
#71205=CARTESIAN_POINT('Ctrl Pts',(0.00259807786435466,-0.033943005420181,
0.0757600935989994));
#71206=CARTESIAN_POINT('Ctrl Pts',(0.00266656626122527,-0.0336441434784052,
0.0759659158908939));
#71207=CARTESIAN_POINT('',(0.00255363235458484,-0.0341934961088741,0.0755823253039714));
#71208=CARTESIAN_POINT('',(0.00261718186963272,-0.0338664212862875,0.0758099632168831));
#71209=CARTESIAN_POINT('Origin',(0.0188805520503518,-0.0345610720404299,
0.0719101546910196));
#71210=CARTESIAN_POINT('Origin',(-0.00788237466357971,-0.0336938005072939,
0.0789750915015038));
#71211=CARTESIAN_POINT('',(0.00258240495709018,-0.0336938721132327,0.0756898906870749));
#71212=CARTESIAN_POINT('',(0.00260044377354836,-0.0336938721132427,0.0757497309001623));
#71213=CARTESIAN_POINT('',(0.00252381793464694,-0.0340203938281605,0.0754609253617025));
#71214=CARTESIAN_POINT('Origin',(0.0189125046270622,-0.0345589643243083,
0.0723902752663712));
#71215=CARTESIAN_POINT('',(0.00252514070879169,-0.034193496108874,0.0754606157064862));
#71216=CARTESIAN_POINT('Origin',(-0.00820423943531576,-0.0341934220717692,
0.0779723123442933));
#71217=CARTESIAN_POINT('',(0.00253938653169827,-0.0341934961088841,0.0755214705052389));
#71218=CARTESIAN_POINT('Ctrl Pts',(0.0022326054963916,-0.0340223579322397,
0.0752875575273789));
#71219=CARTESIAN_POINT('Ctrl Pts',(0.00224829538156874,-0.0339125849573575,
0.0753688122188604));
#71220=CARTESIAN_POINT('Ctrl Pts',(0.00226565602494908,-0.0338030433565231,
0.0754496850694462));
#71221=CARTESIAN_POINT('Ctrl Pts',(0.00228465605720486,-0.0336938721132327,
0.0755300746244473));
#71222=CARTESIAN_POINT('Ctrl Pts',(0.00233015054961238,-0.0340223579322397,
0.075345230245561));
#71223=CARTESIAN_POINT('Ctrl Pts',(0.00234663589199001,-0.0339125849573575,
0.0754251395363505));
#71224=CARTESIAN_POINT('Ctrl Pts',(0.00236476358694424,-0.0338030433565231,
0.075504651467526));
#71225=CARTESIAN_POINT('Ctrl Pts',(0.00238450143849556,-0.0336938721132327,
0.0755836664117405));
#71226=CARTESIAN_POINT('Ctrl Pts',(0.00242769560283315,-0.0340223579322397,
0.0754029029637432));
#71227=CARTESIAN_POINT('Ctrl Pts',(0.00244497640241129,-0.0339125849573575,
0.0754814668538405));
#71228=CARTESIAN_POINT('Ctrl Pts',(0.00246387114893939,-0.0338030433565231,
0.0755596178656058));
#71229=CARTESIAN_POINT('Ctrl Pts',(0.00248434681978626,-0.0336938721132327,
0.0756372581990337));
#71230=CARTESIAN_POINT('Ctrl Pts',(0.00252524065605393,-0.0340223579322397,
0.0754605756819253));
#71231=CARTESIAN_POINT('Ctrl Pts',(0.00254331691283256,-0.0339125849573575,
0.0755377941713306));
#71232=CARTESIAN_POINT('Ctrl Pts',(0.00256297871093455,-0.0338030433565231,
0.0756145842636856));
#71233=CARTESIAN_POINT('Ctrl Pts',(0.00258419220107697,-0.0336938721132327,
0.0756908499863269));
#71234=CARTESIAN_POINT('',(0.00243353050715783,-0.0336938721132427,0.0756099826557713));
#71235=CARTESIAN_POINT('Ctrl Pts',(0.00228172151859185,-0.0337108120662681,
0.0755175989969558));
#71236=CARTESIAN_POINT('Ctrl Pts',(0.00232358889588207,-0.033761140899444,
0.0755077980403452));
#71237=CARTESIAN_POINT('Ctrl Pts',(0.00236469228642256,-0.0338121088781616,
0.0754981759294487));
#71238=CARTESIAN_POINT('Ctrl Pts',(0.00244540853849247,-0.0339153382773234,
0.0754792806335045));
#71239=CARTESIAN_POINT('Ctrl Pts',(0.00248498725214032,-0.0339675558473108,
0.0754700154423158));
#71240=CARTESIAN_POINT('Ctrl Pts',(0.00252381793468696,-0.0340203938281304,
0.0754609253616985));
#71241=CARTESIAN_POINT('Ctrl Pts',(0.00255470183801549,-0.0341934961088741,
0.0755806020549832));
#71242=CARTESIAN_POINT('Ctrl Pts',(0.00258427840845701,-0.0340287516182428,
0.0756957384039372));
#71243=CARTESIAN_POINT('Ctrl Pts',(0.00261858837893608,-0.0338644633275951,
0.0758095539489883));
#71244=CARTESIAN_POINT('Ctrl Pts',(0.00255363235458491,-0.0341934961088741,
0.0755823253039714));
#71245=CARTESIAN_POINT('Ctrl Pts',(0.00258324455184167,-0.0340287516182428,
0.0756974837636528));
#71246=CARTESIAN_POINT('Ctrl Pts',(0.00261759103254668,-0.0338644633275951,
0.0758113199280548));
#71247=CARTESIAN_POINT('Ctrl Pts',(0.00237543584433704,-0.0341934961088741,
0.075869451730816));
#71248=CARTESIAN_POINT('Ctrl Pts',(0.00241098415426721,-0.0340287516182428,
0.0759882942629614));
#71249=CARTESIAN_POINT('Ctrl Pts',(0.00245141394086077,-0.0338644633275951,
0.0761055660078178));
#71250=CARTESIAN_POINT('',(0.00237912173818566,-0.0341764758832395,0.0758817263779963));
#71251=CARTESIAN_POINT('',(0.00237543584433932,-0.034193496108874,0.0758694517308122));
#71252=CARTESIAN_POINT('Origin',(0.0183800328338216,-0.0345621026367731,
0.0715931167332867));
#71253=CARTESIAN_POINT('Ctrl Pts',(0.0023791217385473,-0.0341764758837485,
0.0758817263762082));
#71254=CARTESIAN_POINT('Ctrl Pts',(0.00242021939710316,-0.0341260050040296,
0.0758693374835352));
#71255=CARTESIAN_POINT('Ctrl Pts',(0.0024606026703716,-0.0340749269147885,
0.0758571639024622));
#71256=CARTESIAN_POINT('Ctrl Pts',(0.00253997179671667,-0.0339715436305742,
0.0758332381044852));
#71257=CARTESIAN_POINT('Ctrl Pts',(0.0025789275406577,-0.0339192778236512,
0.0758214949702209));
#71258=CARTESIAN_POINT('Ctrl Pts',(0.00261718186802259,-0.0338664212854278,
0.0758099632154826));
#71259=CARTESIAN_POINT('',(0.00246453409947208,-0.0341934961088841,0.0757258885174018));
#71260=CARTESIAN_POINT('Origin',(0.00812378219310841,-0.0315241814719618,
0.07415));
#71261=CARTESIAN_POINT('',(0.00237912173913322,-0.0342105180190362,0.0758817263785895));
#71262=CARTESIAN_POINT('',(0.00238283384147144,-0.0341934961088739,0.0758939931260949));
#71263=CARTESIAN_POINT('Origin',(0.0183720500414141,-0.0345621701000461,
0.0715484971096708));
#71264=CARTESIAN_POINT('Origin',(0.0180844299120316,-0.0345621040084784,
0.0706125026862545));
#71265=CARTESIAN_POINT('Origin',(0.0181024312949348,-0.0345621715591868,
0.0706541020864207));
#71266=CARTESIAN_POINT('Ctrl Pts',(0.00258197202263347,-0.0346945769586965,
0.0756884545124663));
#71267=CARTESIAN_POINT('Ctrl Pts',(0.00261419556836066,-0.0345275153362944,
0.0758045299453067));
#71268=CARTESIAN_POINT('Ctrl Pts',(0.00265007791427002,-0.0343603235965185,
0.075919622000346));
#71269=CARTESIAN_POINT('Ctrl Pts',(0.00268950787721066,-0.034193496108874,
0.0760333918636549));
#71270=CARTESIAN_POINT('Ctrl Pts',(0.00260616808954228,-0.0346945769586965,
0.0757687201886334));
#71271=CARTESIAN_POINT('Ctrl Pts',(0.00264007283199341,-0.0345275153362944,
0.0758842888251648));
#71272=CARTESIAN_POINT('Ctrl Pts',(0.00267762087119285,-0.0343603235965185,
0.0759988210807221));
#71273=CARTESIAN_POINT('Ctrl Pts',(0.00271869612221547,-0.034193496108874,
0.0761119798702332));
#71274=CARTESIAN_POINT('Ctrl Pts',(0.00263036415645107,-0.0346945769586965,
0.0758489858648032));
#71275=CARTESIAN_POINT('Ctrl Pts',(0.00266595009562619,-0.0345275153362944,
0.0759640477050237));
#71276=CARTESIAN_POINT('Ctrl Pts',(0.00270516382811572,-0.0343603235965185,
0.0760780201610976));
#71277=CARTESIAN_POINT('Ctrl Pts',(0.00274788436722025,-0.034193496108874,
0.07619056787681));
#71278=CARTESIAN_POINT('Ctrl Pts',(0.00265456022335989,-0.0346945769586965,
0.0759292515409676));
#71279=CARTESIAN_POINT('Ctrl Pts',(0.00269182735925891,-0.0345275153362944,
0.076043806584881));
#71280=CARTESIAN_POINT('Ctrl Pts',(0.00273270678503852,-0.0343603235965185,
0.0761572192414743));
#71281=CARTESIAN_POINT('Ctrl Pts',(0.00277707261222508,-0.034193496108874,
0.0762691558833898));
#71282=CARTESIAN_POINT('',(0.00265456022288458,-0.0346945769586966,0.0759292515393901));
#71283=CARTESIAN_POINT('',(0.00273227784011006,-0.0343667727836499,0.0761524499526084));
#71284=CARTESIAN_POINT('Origin',(0.018585812268892,-0.034562647418524,0.0705540814451111));
#71285=CARTESIAN_POINT('Origin',(-0.00762837865205597,-0.0341934771024016,
0.0800004955552602));
#71286=CARTESIAN_POINT('',(0.00269003013551803,-0.034193496108874,0.076034798020116));
#71287=CARTESIAN_POINT('',(0.0027117907545604,-0.034193496108884,0.0760933874855557));
#71288=CARTESIAN_POINT('',(0.00261718186946422,-0.0345211942962691,0.0758099632150947));
#71289=CARTESIAN_POINT('Origin',(0.0187214010005133,-0.0345625596118379,
0.0710153885034588));
#71290=CARTESIAN_POINT('',(0.00261848258998653,-0.0346945769586885,0.0758095711132297));
#71291=CARTESIAN_POINT('Origin',(-0.00797425693574556,-0.0346945685853909,
0.0790027489276701));
#71292=CARTESIAN_POINT('',(0.00263652140644556,-0.0346945769587026,0.0758694113263199));
#71293=CARTESIAN_POINT('Ctrl Pts',(0.00231565845741203,-0.0345231616327842,
0.0756552237942812));
#71294=CARTESIAN_POINT('Ctrl Pts',(0.00233640584823061,-0.0344132092796988,
0.0757352806027937));
#71295=CARTESIAN_POINT('Ctrl Pts',(0.00235880808051535,-0.0343032738558979,
0.075814904137329));
#71296=CARTESIAN_POINT('Ctrl Pts',(0.0023828338414714,-0.0341934961088739,
0.0758939931260949));
#71297=CARTESIAN_POINT('Ctrl Pts',(0.00241663216415694,-0.0345231616327842,
0.0757066577002648));
#71298=CARTESIAN_POINT('Ctrl Pts',(0.00243808849895635,-0.0344132092796988,
0.0757853227283894));
#71299=CARTESIAN_POINT('Ctrl Pts',(0.00246117085076418,-0.0343032738558979,
0.0758635398903994));
#71300=CARTESIAN_POINT('Ctrl Pts',(0.00248584708162573,-0.0341934961088739,
0.075941209738547));
#71301=CARTESIAN_POINT('Ctrl Pts',(0.00251760587090184,-0.0345231616327842,
0.0757580916062485));
#71302=CARTESIAN_POINT('Ctrl Pts',(0.0025397711496821,-0.0344132092796988,
0.0758353648539852));
#71303=CARTESIAN_POINT('Ctrl Pts',(0.002563533621013,-0.0343032738558979,
0.0759121756434697));
#71304=CARTESIAN_POINT('Ctrl Pts',(0.00258886032178006,-0.0341934961088739,
0.075988426350999));
#71305=CARTESIAN_POINT('Ctrl Pts',(0.00261857957764675,-0.0345231616327842,
0.0758095255122321));
#71306=CARTESIAN_POINT('Ctrl Pts',(0.00264145380040784,-0.0344132092796988,
0.075885406979581));
#71307=CARTESIAN_POINT('Ctrl Pts',(0.00266589639126183,-0.0343032738558979,
0.07596081139654));
#71308=CARTESIAN_POINT('Ctrl Pts',(0.00269187356193439,-0.0341934961088739,
0.076035642963451));
#71309=CARTESIAN_POINT('',(0.00253643198850474,-0.0341934961088839,0.0759643955731155));
#71310=CARTESIAN_POINT('Ctrl Pts',(0.00237912174243639,-0.0342105180195385,
0.0758817263775875));
#71311=CARTESIAN_POINT('Ctrl Pts',(0.00242026560670682,-0.0342610556241352,
0.0758693235705557));
#71312=CARTESIAN_POINT('Ctrl Pts',(0.00246067116560645,-0.0343122189870268,
0.0758571433254832));
#71313=CARTESIAN_POINT('Ctrl Pts',(0.00254004109136414,-0.034415811969517,
0.0758332172822989));
#71314=CARTESIAN_POINT('Ctrl Pts',(0.00257897299535572,-0.0344681990450069,
0.0758214812701097));
#71315=CARTESIAN_POINT('Ctrl Pts',(0.00261718186948729,-0.0345211942962495,
0.0758099632150811));
#71316=CARTESIAN_POINT('Ctrl Pts',(0.00265551915720157,-0.0346945769586932,
0.0759274649752898));
#71317=CARTESIAN_POINT('Ctrl Pts',(0.00269226698782536,-0.0345296777079064,
0.0760405174441954));
#71318=CARTESIAN_POINT('Ctrl Pts',(0.00273365598030741,-0.0343648066255586,
0.0761519544895733));
#71319=CARTESIAN_POINT('Ctrl Pts',(0.00265456022288184,-0.0346945769586932,
0.0759292515393815));
#71320=CARTESIAN_POINT('Ctrl Pts',(0.00269134498945405,-0.0345296777079064,
0.0760423238335756));
#71321=CARTESIAN_POINT('Ctrl Pts',(0.0027327717057206,-0.0343648066255586,
0.0761537791607048));
#71322=CARTESIAN_POINT('Ctrl Pts',(0.00249474416025337,-0.0346945769586932,
0.076227000439268));
#71323=CARTESIAN_POINT('Ctrl Pts',(0.00253768467464258,-0.0345296777079064,
0.0763433768174706));
#71324=CARTESIAN_POINT('Ctrl Pts',(0.00258539843954466,-0.0343648066255586,
0.0764578789825962));
#71325=CARTESIAN_POINT('',(0.00249919351212516,-0.0346775396664981,0.0762390194262264));
#71326=CARTESIAN_POINT('',(0.00249474416025707,-0.0346945769586886,0.0762270004392665));
#71327=CARTESIAN_POINT('Origin',(0.0180082191875373,-0.034562661794297,
0.0703159270750803));
#71328=CARTESIAN_POINT('Ctrl Pts',(0.00249919351247531,-0.0346775396670096,
0.0762390194244345));
#71329=CARTESIAN_POINT('Ctrl Pts',(0.00253946386091069,-0.0346269749928766,
0.0762240626654086));
#71330=CARTESIAN_POINT('Ctrl Pts',(0.0025790185028908,-0.0345757902891958,
0.0762093716876919));
#71331=CARTESIAN_POINT('Ctrl Pts',(0.00265672900953741,-0.0344721681090152,
0.0761805093575572));
#71332=CARTESIAN_POINT('Ctrl Pts',(0.0026948544099873,-0.0344197714292358,
0.0761663493258164));
#71333=CARTESIAN_POINT('Ctrl Pts',(0.0027322778396058,-0.0343667727834165,
0.0761524499521408));
#71334=CARTESIAN_POINT('',(0.00257465219158083,-0.0346945769587026,0.0760781259893383));
#71335=CARTESIAN_POINT('Origin',(0.00812378219310841,-0.0315241814719618,
0.07415));
#71336=CARTESIAN_POINT('',(0.002499193513487,-0.0347116136489789,0.0762390194265086));
#71337=CARTESIAN_POINT('',(0.00250366852609143,-0.0346945769586885,0.0762510288836281));
#71338=CARTESIAN_POINT('Origin',(0.0179907058082699,-0.0345626680065938,
0.0702741345734983));
#71339=CARTESIAN_POINT('Origin',(0.0181145644536158,-0.0345626631243122,
0.0706022478523321));
#71340=CARTESIAN_POINT('Origin',(0.018128572272324,-0.0345626692914332,
0.0706453424126909));
#71341=CARTESIAN_POINT('Ctrl Pts',(0.00267744283577248,-0.0352450361874069,
0.0759982830493078));
#71342=CARTESIAN_POINT('Ctrl Pts',(0.00274715197485094,-0.0349452760959493,
0.076203695108825));
#71343=CARTESIAN_POINT('Ctrl Pts',(0.00283213555440364,-0.034644428984174,
0.0764032728367221));
#71344=CARTESIAN_POINT('Ctrl Pts',(0.00267830709071825,-0.0352450361874069,
0.0760006555350061));
#71345=CARTESIAN_POINT('Ctrl Pts',(0.00274810570956311,-0.0349452760959493,
0.0762060349986132));
#71346=CARTESIAN_POINT('Ctrl Pts',(0.0028331760594223,-0.034644428984174,
0.0764055734832195));
#71347=CARTESIAN_POINT('Ctrl Pts',(0.00276387688732919,-0.0352450361874069,
0.0762355551090968));
#71348=CARTESIAN_POINT('Ctrl Pts',(0.00284253488898659,-0.0349452760959493,
0.0764377072548668));
#71349=CARTESIAN_POINT('Ctrl Pts',(0.00293619635829975,-0.034644428984174,
0.0766333602651433));
#71350=CARTESIAN_POINT('Ctrl Pts',(0.0027647325852953,-0.0352450361874069,
0.0762379041048377));
#71351=CARTESIAN_POINT('Ctrl Pts',(0.00284347918078083,-0.0349452760959493,
0.0764400239774293));
#71352=CARTESIAN_POINT('Ctrl Pts',(0.00293722656128853,-0.034644428984174,
0.0766356381329626));
#71353=CARTESIAN_POINT('',(0.00277705848222208,-0.0351951634053265,0.0762691266743592));
#71354=CARTESIAN_POINT('',(0.00286865161508712,-0.0348678972925388,0.0764870339338457));
#71355=CARTESIAN_POINT('Origin',(0.0180012108129683,-0.0345636767889768,
0.0692956281131201));
#71356=CARTESIAN_POINT('Origin',(-0.00722780739889109,-0.0346946199341087,
0.0809770789890401));
#71357=CARTESIAN_POINT('',(0.00281909984408069,-0.0346945769330289,0.076372266899799));
#71358=CARTESIAN_POINT('',(0.00284449638968655,-0.0346945769458129,0.0764293743998229));
#71359=CARTESIAN_POINT('',(0.00273227783999167,-0.0350221583435276,0.0761524499520148));
#71360=CARTESIAN_POINT('Origin',(0.0182337468182862,-0.0345628458716235,
0.0697164254497386));
#71361=CARTESIAN_POINT('',(0.00273343628146693,-0.0351951360298763,0.0761520164706515));
#71362=CARTESIAN_POINT('Origin',(-0.00759609818597462,-0.0351951838366788,
0.079988494223648));
#71363=CARTESIAN_POINT('',(0.00277707261153886,-0.0351951371328749,0.0762691558818757));
#71364=CARTESIAN_POINT('Ctrl Pts',(0.00242163354584956,-0.0350241211494342,
0.0760169495988363));
#71365=CARTESIAN_POINT('Ctrl Pts',(0.00244735001109438,-0.0349144232818962,
0.0760954943584803));
#71366=CARTESIAN_POINT('Ctrl Pts',(0.00247470544519014,-0.0348045283579412,
0.0761735545532363));
#71367=CARTESIAN_POINT('Ctrl Pts',(0.00250366852998279,-0.0346945769439158,
0.0762510288940373));
#71368=CARTESIAN_POINT('Ctrl Pts',(0.00252563759587068,-0.0350241211494342,
0.0760619418135205));
#71369=CARTESIAN_POINT('Ctrl Pts',(0.00255197381042526,-0.0349144232818962,
0.0761390539600188));
#71370=CARTESIAN_POINT('Ctrl Pts',(0.00257991975164319,-0.0348045283579412,
0.07621566787348));
#71371=CARTESIAN_POINT('Ctrl Pts',(0.00260944327606993,-0.0346945769439158,
0.0762916840891936));
#71372=CARTESIAN_POINT('Ctrl Pts',(0.00262964164589181,-0.0350241211494342,
0.0761069340282047));
#71373=CARTESIAN_POINT('Ctrl Pts',(0.00265659760975614,-0.0349144232818962,
0.0761826135615573));
#71374=CARTESIAN_POINT('Ctrl Pts',(0.00268513405809624,-0.0348045283579412,
0.0762577811937236));
#71375=CARTESIAN_POINT('Ctrl Pts',(0.00271521802215706,-0.0346945769439158,
0.0763323392843498));
#71376=CARTESIAN_POINT('Ctrl Pts',(0.00273364569591294,-0.0350241211494342,
0.076151926242889));
#71377=CARTESIAN_POINT('Ctrl Pts',(0.00276122140908702,-0.0349144232818962,
0.0762261731630958));
#71378=CARTESIAN_POINT('Ctrl Pts',(0.00279034836454929,-0.0348045283579412,
0.0762998945139673));
#71379=CARTESIAN_POINT('Ctrl Pts',(0.00282099276824419,-0.0346945769439158,
0.0763729944795061));
#71380=CARTESIAN_POINT('',(0.00266138418490153,-0.0346945769458128,0.0763116478914811));
#71381=CARTESIAN_POINT('Ctrl Pts',(0.00249919351656515,-0.0347116136492789,
0.0762390194253587));
#71382=CARTESIAN_POINT('Ctrl Pts',(0.00253944787729479,-0.0347621546532341,
0.0762240686180454));
#71383=CARTESIAN_POINT('Ctrl Pts',(0.0025789944575839,-0.0348133084097124,
0.076209380686326));
#71384=CARTESIAN_POINT('Ctrl Pts',(0.0026567050615848,-0.0349168561544564,
0.0761805183159999));
#71385=CARTESIAN_POINT('Ctrl Pts',(0.00269483826145598,-0.0349692089015912,
0.0761663553256262));
#71386=CARTESIAN_POINT('Ctrl Pts',(0.00273227784003292,-0.0350221583435,
0.0761524499520208));
#71387=CARTESIAN_POINT('Ctrl Pts',(0.00277768220828862,-0.0351951371254875,
0.0762678259150681));
#71388=CARTESIAN_POINT('Ctrl Pts',(0.00282146693031317,-0.0350307338980921,
0.0763783531779963));
#71389=CARTESIAN_POINT('Ctrl Pts',(0.00286978244958865,-0.0348659306897825,
0.0764869763262212));
#71390=CARTESIAN_POINT('Ctrl Pts',(0.0027770726116466,-0.0351951371254875,
0.0762691558818324));
#71391=CARTESIAN_POINT('Ctrl Pts',(0.00282088482989956,-0.0350307338980921,
0.0763796957477886));
#71392=CARTESIAN_POINT('Ctrl Pts',(0.00286922834280482,-0.0348659306897825,
0.0764883303518237));
#71393=CARTESIAN_POINT('Ctrl Pts',(0.00267490357911754,-0.0351951371254875,
0.0764920596976223));
#71394=CARTESIAN_POINT('Ctrl Pts',(0.00272332419390732,-0.0350307338980921,
0.0766047118442231));
#71395=CARTESIAN_POINT('Ctrl Pts',(0.00277635946833986,-0.0348659306897825,
0.0767152664539698));
#71396=CARTESIAN_POINT('Origin',(-0.00199067670531014,-0.0308609197410307,
0.0786480487766916));
#71397=CARTESIAN_POINT('',(0.00273252921706985,-0.0351951371254875,0.0763663369197028));
#71398=CARTESIAN_POINT('Origin',(0.00894963950894094,-0.0351840467441202,
0.0736277880284817));
#71399=CARTESIAN_POINT('Origin',(-0.00246205922185187,-0.0352322613882021,
0.0797274165207997));
#71400=CARTESIAN_POINT('',(0.00296926846134209,-0.035195114256466,0.0767012355384141));
#71401=CARTESIAN_POINT('',(0.00302696922376633,-0.0351951372916787,0.0768117658716625));
#71402=CARTESIAN_POINT('Origin',(0.0084163362896763,-0.0352875124680666,
0.0743244425502087));
#71403=CARTESIAN_POINT('Origin',(0.00598815585604378,-0.0298325076522621,
0.0669573446885997));
#71404=CARTESIAN_POINT('Origin',(-0.000219626886901942,-0.0338732543834639,
0.0749480502568973));
#71405=CARTESIAN_POINT('Ctrl Pts',(0.00245414689220848,-0.0321934096636941,
0.0731838885674513));
#71406=CARTESIAN_POINT('Ctrl Pts',(0.00243685395761994,-0.0320508460843085,
0.0732853723395051));
#71407=CARTESIAN_POINT('Ctrl Pts',(0.00242230073067469,-0.0319086045660596,
0.0733872442194909));
#71408=CARTESIAN_POINT('Ctrl Pts',(0.00241050048893715,-0.0317669892864203,
0.0734892822795843));
#71409=CARTESIAN_POINT('Ctrl Pts',(0.00244186258475718,-0.0321934096636941,
0.0732668314901052));
#71410=CARTESIAN_POINT('Ctrl Pts',(0.00242605428898742,-0.0320508460843085,
0.0733685351454127));
#71411=CARTESIAN_POINT('Ctrl Pts',(0.00241299048926756,-0.0319086045660596,
0.0734705868535438));
#71412=CARTESIAN_POINT('Ctrl Pts',(0.00240268122428634,-0.0317669892864203,
0.0735727645634927));
#71413=CARTESIAN_POINT('Ctrl Pts',(0.00242957827730588,-0.0321934096636941,
0.0733497744127592));
#71414=CARTESIAN_POINT('Ctrl Pts',(0.00241525462035492,-0.0320508460843085,
0.0734516979513203));
#71415=CARTESIAN_POINT('Ctrl Pts',(0.00240368024786043,-0.0319086045660596,
0.0735539294875968));
#71416=CARTESIAN_POINT('Ctrl Pts',(0.00239486195963552,-0.0317669892864203,
0.073656246847401));
#71417=CARTESIAN_POINT('Ctrl Pts',(0.00241729396985459,-0.0321934096636941,
0.073432717335413));
#71418=CARTESIAN_POINT('Ctrl Pts',(0.0024044549517224,-0.0320508460843085,
0.0735348607572279));
#71419=CARTESIAN_POINT('Ctrl Pts',(0.00239437000645331,-0.0319086045660596,
0.0736372721216497));
#71420=CARTESIAN_POINT('Ctrl Pts',(0.0023870426949847,-0.0317669892864203,
0.0737397291313093));
#71421=CARTESIAN_POINT('',(0.0024175137385447,-0.0321934096636941,0.0734312334701365));
#71422=CARTESIAN_POINT('',(0.00239280147990483,-0.0318665617511268,0.0736662799839588));
#71423=CARTESIAN_POINT('Origin',(0.0189082437893042,-0.0326371944417531,
0.0761282183133339));
#71424=CARTESIAN_POINT('Origin',(-0.00852954720918482,-0.0316939261509197,
0.0727443856010129));
#71425=CARTESIAN_POINT('',(0.0024344906740738,-0.0320197221621809,0.07330765139166));
#71426=CARTESIAN_POINT('Ctrl Pts',(0.00243441780502418,-0.0320197392094727,
0.0733078214063092));
#71427=CARTESIAN_POINT('Ctrl Pts',(0.0024301325760199,-0.0319792716576025,
0.073336770728273));
#71428=CARTESIAN_POINT('Ctrl Pts',(0.00242604853700066,-0.0319386439829662,
0.0733658845074326));
#71429=CARTESIAN_POINT('Ctrl Pts',(0.00242216977601236,-0.0318979099381593,
0.0733951944826528));
#71430=CARTESIAN_POINT('Ctrl Pts',(0.00241829109169051,-0.0318571766984898,
0.0734245038785406));
#71431=CARTESIAN_POINT('Ctrl Pts',(0.00241463562500548,-0.031816387183355,
0.0734538602594943));
#71432=CARTESIAN_POINT('Ctrl Pts',(0.00241121245508737,-0.0317755399638303,
0.0734831622165602));
#71433=CARTESIAN_POINT('',(0.00243582716738047,-0.0321934096636184,0.0733075822738708));
#71434=CARTESIAN_POINT('Origin',(0.000149372311971935,-0.0324112673258503,
0.0729902076274767));
#71435=CARTESIAN_POINT('',(0.00242667045297258,-0.0321934096636663,0.0733694078720137));
#71436=CARTESIAN_POINT('Ctrl Pts',(0.00241914254979784,-0.0321934096636617,
0.0734300248919303));
#71437=CARTESIAN_POINT('Ctrl Pts',(0.00240921353194178,-0.0320835708272592,
0.0735086963185477));
#71438=CARTESIAN_POINT('Ctrl Pts',(0.00240091837440467,-0.0319739230346488,
0.0735875275930489));
#71439=CARTESIAN_POINT('Ctrl Pts',(0.00239425994960734,-0.0318646057455573,
0.0736664170417633));
#71440=CARTESIAN_POINT('Ctrl Pts',(0.00232813920853723,-0.0321934096636617,
0.0734975493811466));
#71441=CARTESIAN_POINT('Ctrl Pts',(0.00231914140601297,-0.0320835708272592,
0.0735774758147638));
#71442=CARTESIAN_POINT('Ctrl Pts',(0.00231180289596956,-0.0319739230346488,
0.0736575420968569));
#71443=CARTESIAN_POINT('Ctrl Pts',(0.00230612520559497,-0.0318646057455573,
0.0737376450675846));
#71444=CARTESIAN_POINT('Ctrl Pts',(0.00223713586727661,-0.0321934096636617,
0.0735650738703629));
#71445=CARTESIAN_POINT('Ctrl Pts',(0.00222906928008416,-0.0320835708272592,
0.07364625531098));
#71446=CARTESIAN_POINT('Ctrl Pts',(0.00222268741753445,-0.0319739230346488,
0.0737275566006649));
#71447=CARTESIAN_POINT('Ctrl Pts',(0.0022179904615826,-0.0318646057455573,
0.0738088730934058));
#71448=CARTESIAN_POINT('Ctrl Pts',(0.002146132526016,-0.0321934096636617,
0.0736325983595793));
#71449=CARTESIAN_POINT('Ctrl Pts',(0.00213899715415534,-0.0320835708272592,
0.0737150348071961));
#71450=CARTESIAN_POINT('Ctrl Pts',(0.00213357193909934,-0.0319739230346488,
0.073797571104473));
#71451=CARTESIAN_POINT('Ctrl Pts',(0.00212985571757023,-0.0318646057455573,
0.0738801011192271));
#71452=CARTESIAN_POINT('',(0.00214504098544081,-0.0321763980308447,0.0736453679068871));
#71453=CARTESIAN_POINT('',(0.00214613252601318,-0.0321934096636184,0.0736325983596118));
#71454=CARTESIAN_POINT('Origin',(0.0185711665253974,-0.0326386231815108,
0.0756474894054743));
#71455=CARTESIAN_POINT('Ctrl Pts',(0.00214504098859838,-0.0321763980306265,
0.0736453679071493));
#71456=CARTESIAN_POINT('Ctrl Pts',(0.00218780781467109,-0.0321259596175139,
0.0736489776156494));
#71457=CARTESIAN_POINT('Ctrl Pts',(0.00222983364998933,-0.0320749164632061,
0.0736525247812591));
#71458=CARTESIAN_POINT('Ctrl Pts',(0.0023124371602503,-0.0319716057793898,
0.0736594968813775));
#71459=CARTESIAN_POINT('Ctrl Pts',(0.00235298265000875,-0.0319193786690093,
0.0736629190993149));
#71460=CARTESIAN_POINT('Ctrl Pts',(0.0023928014817504,-0.0318665617525277,
0.0736662799841081));
#71461=CARTESIAN_POINT('',(0.00228182313228894,-0.0321934096636663,0.0735319159148842));
#71462=CARTESIAN_POINT('Origin',(0.00812378219310841,-0.0315241814719618,
0.07415));
#71463=CARTESIAN_POINT('',(0.00214504098506965,-0.0322104233323609,0.0736453679068559));
#71464=CARTESIAN_POINT('',(0.00214397671962842,-0.0321934096636183,0.0736581397562614));
#71465=CARTESIAN_POINT('Origin',(0.0185812385183085,-0.0326387230348049,
0.0756032873434876));
#71466=CARTESIAN_POINT('Origin',(0.0186743673869259,-0.0326386245818049,
0.0744248298492832));
#71467=CARTESIAN_POINT('Origin',(0.0186768816158389,-0.0326387241480481,
0.074470094625862));
#71468=CARTESIAN_POINT('Ctrl Pts',(0.00240860327225173,-0.0327445246967097,
0.0735059076909357));
#71469=CARTESIAN_POINT('Ctrl Pts',(0.00238431093368944,-0.032443687833936,
0.0737214591877253));
#71470=CARTESIAN_POINT('Ctrl Pts',(0.00237632382680337,-0.0321434074405927,
0.0739382281237025));
#71471=CARTESIAN_POINT('Ctrl Pts',(0.0023860118057462,-0.0327445246967097,
0.07375488484981));
#71472=CARTESIAN_POINT('Ctrl Pts',(0.00237110979424191,-0.032443687833936,
0.073971288397688));
#71473=CARTESIAN_POINT('Ctrl Pts',(0.00237255051745677,-0.0321434074405927,
0.0741881996463537));
#71474=CARTESIAN_POINT('',(0.00238364203203967,-0.0326943950436611,0.073790951352479));
#71475=CARTESIAN_POINT('',(0.00237373722915698,-0.0323666188837389,0.0740270857512829));
#71476=CARTESIAN_POINT('Origin',(0.0191663754899599,-0.0326395579109917,
0.074764561077896));
#71477=CARTESIAN_POINT('Origin',(-0.0086683485399123,-0.0321933825603029,
0.0737910482320124));
#71478=CARTESIAN_POINT('',(0.00237776687233203,-0.0321934096532689,0.0739021433276513));
#71479=CARTESIAN_POINT('',(0.00237643116307099,-0.0321934096584275,0.0739646290558353));
#71480=CARTESIAN_POINT('',(0.00239280147895539,-0.0325210109756238,0.0736662799838677));
#71481=CARTESIAN_POINT('Origin',(0.0191110745637306,-0.0326393129159087,
0.0752421867029637));
#71482=CARTESIAN_POINT('',(0.00239415520064964,-0.0326943950436593,0.0736663942439461));
#71483=CARTESIAN_POINT('Origin',(-0.00862910428412556,-0.0326943765538171,
0.0727359819515683));
#71484=CARTESIAN_POINT('',(0.00238889861635466,-0.0326943950436702,0.0737286727982226));
#71485=CARTESIAN_POINT('Ctrl Pts',(0.00216941549877631,-0.0325229783203769,
0.0734114085909923));
#71486=CARTESIAN_POINT('Ctrl Pts',(0.00215923403235506,-0.032413025309245,
0.0734934894056602));
#71487=CARTESIAN_POINT('Ctrl Pts',(0.00215075205724437,-0.0323031222208069,
0.0735757683878763));
#71488=CARTESIAN_POINT('Ctrl Pts',(0.00214397671926085,-0.0321934096576658,
0.0736581397607305));
#71489=CARTESIAN_POINT('Ctrl Pts',(0.00224436440906771,-0.0325229783203769,
0.0734964015500094));
#71490=CARTESIAN_POINT('Ctrl Pts',(0.00223535456872785,-0.032413025309245,
0.073577449195588));
#71491=CARTESIAN_POINT('Ctrl Pts',(0.00222802266956867,-0.0323031222208069,
0.0736586709288246));
#71492=CARTESIAN_POINT('Ctrl Pts',(0.00222237443202867,-0.0321934096576658,
0.0737399623790529));
#71493=CARTESIAN_POINT('Ctrl Pts',(0.00231931331935912,-0.0325229783203769,
0.0735813945090266));
#71494=CARTESIAN_POINT('Ctrl Pts',(0.00231147510510064,-0.032413025309245,
0.0736614089855159));
#71495=CARTESIAN_POINT('Ctrl Pts',(0.00230529328189297,-0.0323031222208069,
0.0737415734697729));
#71496=CARTESIAN_POINT('Ctrl Pts',(0.00230077214479649,-0.0321934096576658,
0.0738217849973754));
#71497=CARTESIAN_POINT('Ctrl Pts',(0.00239426222965053,-0.0325229783203769,
0.0736663874680437));
#71498=CARTESIAN_POINT('Ctrl Pts',(0.00238759564147342,-0.032413025309245,
0.0737453687754437));
#71499=CARTESIAN_POINT('Ctrl Pts',(0.00238256389421727,-0.0323031222208069,
0.0738244760107211));
#71500=CARTESIAN_POINT('Ctrl Pts',(0.00237916985756431,-0.0321934096576658,
0.0739036076156978));
#71501=CARTESIAN_POINT('',(0.00226087179586497,-0.0321934096584275,0.073780141541465));
#71502=CARTESIAN_POINT('Ctrl Pts',(0.00214504098853049,-0.0322104233328923,
0.0736453679071436));
#71503=CARTESIAN_POINT('Ctrl Pts',(0.00218786576437557,-0.0322609421831417,
0.0736489825068597));
#71504=CARTESIAN_POINT('Ctrl Pts',(0.00222991990913416,-0.0323120888240843,
0.0736525320619177));
#71505=CARTESIAN_POINT('Ctrl Pts',(0.00231252404474623,-0.0324156524631811,
0.0736595042148185));
#71506=CARTESIAN_POINT('Ctrl Pts',(0.0023530400809842,-0.0324680267167309,
0.0736629239467422));
#71507=CARTESIAN_POINT('Ctrl Pts',(0.00239280147899819,-0.0325210109755912,
0.0736662799838758));
#71508=CARTESIAN_POINT('Origin',(0.0097249060661641,-0.0262834582512067,
0.0664467676796293));
#71509=CARTESIAN_POINT('Origin',(-0.00225402174624506,-0.0342771013831326,
0.0678154784922417));
#71510=CARTESIAN_POINT('Ctrl Pts',(0.00238519136587608,-0.0326943950436604,
0.0737896432028331));
#71511=CARTESIAN_POINT('Ctrl Pts',(0.0023802249738305,-0.0325844576448134,
0.0738687317396979));
#71512=CARTESIAN_POINT('Ctrl Pts',(0.00237689391091544,-0.0324744968375322,
0.0739479285869114));
#71513=CARTESIAN_POINT('Ctrl Pts',(0.00237520104548429,-0.0323646534831895,
0.0740271322139863));
#71514=CARTESIAN_POINT('Ctrl Pts',(0.00229860762203796,-0.0326943950436604,
0.0738627484891289));
#71515=CARTESIAN_POINT('Ctrl Pts',(0.00229464875785145,-0.0325844576448134,
0.073943030312259));
#71516=CARTESIAN_POINT('Ctrl Pts',(0.00229234997321614,-0.0324744968375322,
0.0740233996928605));
#71517=CARTESIAN_POINT('Ctrl Pts',(0.00229171279314884,-0.0323646534831895,
0.0741037536163709));
#71518=CARTESIAN_POINT('Ctrl Pts',(0.00221202387819984,-0.0326943950436604,
0.0739358537754246));
#71519=CARTESIAN_POINT('Ctrl Pts',(0.00220907254187239,-0.0325844576448134,
0.0740173288848201));
#71520=CARTESIAN_POINT('Ctrl Pts',(0.00220780603551685,-0.0324744968375322,
0.0740988707988096));
#71521=CARTESIAN_POINT('Ctrl Pts',(0.00220822454081339,-0.0323646534831895,
0.0741803750187554));
#71522=CARTESIAN_POINT('Ctrl Pts',(0.00212544013436172,-0.0326943950436604,
0.0740089590617204));
#71523=CARTESIAN_POINT('Ctrl Pts',(0.00212349632589333,-0.0325844576448134,
0.0740916274573811));
#71524=CARTESIAN_POINT('Ctrl Pts',(0.00212326209781756,-0.0324744968375322,
0.0741743419047587));
#71525=CARTESIAN_POINT('Ctrl Pts',(0.00212473628847795,-0.0323646534831895,
0.07425699642114));
#71526=CARTESIAN_POINT('',(0.00212515255399853,-0.0326773559991329,0.0740217719496073));
#71527=CARTESIAN_POINT('',(0.00212544013436172,-0.0326943950436594,0.0740089590617211));
#71528=CARTESIAN_POINT('Origin',(0.0187275769404676,-0.0326395670532496,
0.0743264168673391));
#71529=CARTESIAN_POINT('Ctrl Pts',(0.00212515255734552,-0.0326773559987408,
0.0740217719496743));
#71530=CARTESIAN_POINT('Ctrl Pts',(0.00216809617865336,-0.0326267922586304,
0.0740226899221395));
#71531=CARTESIAN_POINT('Ctrl Pts',(0.00221027865528394,-0.032575610958006,
0.0740235916242056));
#71532=CARTESIAN_POINT('Ctrl Pts',(0.00229315721868346,-0.0324719985462361,
0.0740253632549352));
#71533=CARTESIAN_POINT('Ctrl Pts',(0.00233382006503627,-0.0324196091621767,
0.0740262324730443));
#71534=CARTESIAN_POINT('Ctrl Pts',(0.00237373722920576,-0.0323666188837757,
0.0740270857512839));
#71535=CARTESIAN_POINT('',(0.0022545410832107,-0.0326943950436702,0.0738999552071101));
#71536=CARTESIAN_POINT('Origin',(0.00812378219310841,-0.0315241814719618,
0.07415));
#71537=CARTESIAN_POINT('',(0.00212515255404165,-0.0327114338379866,0.0740217719496084));
#71538=CARTESIAN_POINT('',(0.00212489233953398,-0.0326943950436593,0.074034585422462));
#71539=CARTESIAN_POINT('Origin',(0.0187277723063497,-0.0326395662664893,
0.0742811056495937));
#71540=CARTESIAN_POINT('Origin',(0.0187254324157374,-0.032639568123537,
0.0744268740492791));
#71541=CARTESIAN_POINT('Origin',(0.0187236855789967,-0.0326395675150339,
0.0744721518653795));
#71542=CARTESIAN_POINT('Ctrl Pts',(0.00237943604517094,-0.0332451089994432,
0.0738660768895002));
#71543=CARTESIAN_POINT('Ctrl Pts',(0.00236872770986089,-0.0329451141710252,
0.0740827284490749));
#71544=CARTESIAN_POINT('Ctrl Pts',(0.00237436887694699,-0.0326442513127493,
0.0742995711200258));
#71545=CARTESIAN_POINT('Ctrl Pts',(0.00237252426724457,-0.0332451089994432,
0.0741159813258873));
#71546=CARTESIAN_POINT('Ctrl Pts',(0.00237124123195885,-0.0329451141710252,
0.0743328935674314));
#71547=CARTESIAN_POINT('Ctrl Pts',(0.00238630055841826,-0.0326442513127493,
0.0745492862276531));
#71548=CARTESIAN_POINT('Ctrl Pts',(0.0023724551494653,-0.0332451089994432,
0.0741184803702511));
#71549=CARTESIAN_POINT('Ctrl Pts',(0.00237126636717983,-0.0329451141710252,
0.0743353952186149));
#71550=CARTESIAN_POINT('Ctrl Pts',(0.00238641987523298,-0.0326442513127493,
0.0745517833787293));
#71551=CARTESIAN_POINT('',(0.00237242403632311,-0.0331951640388616,0.0741520862358533));
#71552=CARTESIAN_POINT('',(0.00237736577183239,-0.0328677532463079,0.0743883766242067));
#71553=CARTESIAN_POINT('Origin',(0.0191185650576716,-0.0326403163409216,
0.0733780785999388));
#71554=CARTESIAN_POINT('Origin',(-0.00866908174770781,-0.0326944278639077,
0.0748471381129464));
#71555=CARTESIAN_POINT('',(0.00237354227162478,-0.0326943950436593,0.0742634277099163));
#71556=CARTESIAN_POINT('',(0.00237613270965503,-0.0326943950436693,0.0743258740038985));
#71557=CARTESIAN_POINT('',(0.00237373722915705,-0.0330220786163545,0.07402708575128));
#71558=CARTESIAN_POINT('Origin',(0.0191698357957509,-0.0326396682760288,
0.0738560707557115));
#71559=CARTESIAN_POINT('',(0.00237509545404048,-0.0331951640388586,0.074027114785002));
#71560=CARTESIAN_POINT('Origin',(-0.00865403804678937,-0.0331952026560058,
0.0737913527080536));
#71561=CARTESIAN_POINT('',(0.0023737597451918,-0.0331951640388701,0.0740896005104377));
#71562=CARTESIAN_POINT('Ctrl Pts',(0.00213478848483599,-0.0330240426238172,
0.073786744769755));
#71563=CARTESIAN_POINT('Ctrl Pts',(0.00212978429013694,-0.0329142774063519,
0.0738692489928803));
#71564=CARTESIAN_POINT('Ctrl Pts',(0.00212648319342054,-0.0328043479726691,
0.0739518977980528));
#71565=CARTESIAN_POINT('Ctrl Pts',(0.00212489233953394,-0.0326943950436593,
0.0740345854224621));
#71566=CARTESIAN_POINT('Ctrl Pts',(0.00221492624594939,-0.0330240426238172,
0.0738668639012297));
#71567=CARTESIAN_POINT('Ctrl Pts',(0.0022110257703427,-0.0329142774063519,
0.0739482641486212));
#71568=CARTESIAN_POINT('Ctrl Pts',(0.00220880612070064,-0.0328043479726691,
0.074029785610731));
#71569=CARTESIAN_POINT('Ctrl Pts',(0.00220827301668285,-0.0326943950436593,
0.0741113239308051));
#71570=CARTESIAN_POINT('Ctrl Pts',(0.00229506400706279,-0.0330240426238172,
0.0739469830327043));
#71571=CARTESIAN_POINT('Ctrl Pts',(0.00229226725054845,-0.0329142774063519,
0.074027279304362));
#71572=CARTESIAN_POINT('Ctrl Pts',(0.00229112904798074,-0.0328043479726691,
0.0741076734234092));
#71573=CARTESIAN_POINT('Ctrl Pts',(0.00229165369383175,-0.0326943950436593,
0.0741880624391481));
#71574=CARTESIAN_POINT('Ctrl Pts',(0.0023752017681762,-0.0330240426238172,
0.0740271021641789));
#71575=CARTESIAN_POINT('Ctrl Pts',(0.0023735087307542,-0.0329142774063519,
0.0741062944601029));
#71576=CARTESIAN_POINT('Ctrl Pts',(0.00237345197526084,-0.0328043479726691,
0.0741855612360874));
#71577=CARTESIAN_POINT('Ctrl Pts',(0.00237503437098066,-0.0326943950436593,
0.0742648009474911));
#71578=CARTESIAN_POINT('',(0.00224921730558938,-0.0326943950436693,0.0741490065661991));
#71579=CARTESIAN_POINT('Ctrl Pts',(0.0021251525573509,-0.0327114338383319,
0.0740217719496745));
#71580=CARTESIAN_POINT('Ctrl Pts',(0.00216808903577093,-0.032761987683113,
0.0740226897694516));
#71581=CARTESIAN_POINT('Ctrl Pts',(0.00221026802350364,-0.032813156260467,
0.0740235913969382));
#71582=CARTESIAN_POINT('Ctrl Pts',(0.00229314651070481,-0.0329167375858765,
0.074025363026039));
#71583=CARTESIAN_POINT('Ctrl Pts',(0.00233381298715526,-0.0329691088920615,
0.0740262323217458));
#71584=CARTESIAN_POINT('Ctrl Pts',(0.00237373722920451,-0.0330220786163187,
0.0740270857512838));
#71585=CARTESIAN_POINT('Ctrl Pts',(0.00237388840724671,-0.0331951640388604,
0.0741506831601087));
#71586=CARTESIAN_POINT('Ctrl Pts',(0.00237390253114358,-0.0330306422053993,
0.0742695585245084));
#71587=CARTESIAN_POINT('Ctrl Pts',(0.00237882988666516,-0.0328657862001532,
0.0743883317269922));
#71588=CARTESIAN_POINT('Ctrl Pts',(0.00237242403632318,-0.0331951640388604,
0.0741520862358502));
#71589=CARTESIAN_POINT('Ctrl Pts',(0.00237246716791067,-0.0330306422053993,
0.0742709918751792));
#71590=CARTESIAN_POINT('Ctrl Pts',(0.00237742475763063,-0.0328657862001532,
0.0743897941278041));
#71591=CARTESIAN_POINT('Ctrl Pts',(0.00212842045843366,-0.0331951640388604,
0.0743858763879778));
#71592=CARTESIAN_POINT('Ctrl Pts',(0.00213329705139667,-0.0330306422053993,
0.074509826644706));
#71593=CARTESIAN_POINT('Ctrl Pts',(0.00214329247167014,-0.0328657862001532,
0.0746334694321039));
#71594=CARTESIAN_POINT('',(0.0021289379721009,-0.0331781648281899,0.0743986820492859));
#71595=CARTESIAN_POINT('',(0.00212842045843432,-0.0331951640388588,0.0743858763879783));
#71596=CARTESIAN_POINT('Origin',(0.0185921750515698,-0.0326412092571505,
0.073002864439015));
#71597=CARTESIAN_POINT('Ctrl Pts',(0.00212893797309369,-0.033178164828644,
0.0743986820477356));
#71598=CARTESIAN_POINT('Ctrl Pts',(0.00217188403951269,-0.0331276811561084,
0.0743969005188));
#71599=CARTESIAN_POINT('Ctrl Pts',(0.00221405463159051,-0.0330765663526748,
0.0743951511249712));
#71600=CARTESIAN_POINT('Ctrl Pts',(0.00229688110570806,-0.0329730614522356,
0.0743917152665022));
#71601=CARTESIAN_POINT('Ctrl Pts',(0.00233750352844884,-0.0329207133441171,
0.074390030195206));
#71602=CARTESIAN_POINT('Ctrl Pts',(0.00237736575892228,-0.0328677532371618,
0.0743883766059144));
#71603=CARTESIAN_POINT('',(0.00225042224738872,-0.0331951640388701,0.0742689813119258));
#71604=CARTESIAN_POINT('Origin',(0.00812378219310841,-0.0315241814719618,
0.07415));
#71605=CARTESIAN_POINT('',(0.00212893797367636,-0.0332121607144414,0.0743986820498679));
#71606=CARTESIAN_POINT('',(0.00212948283705904,-0.0331951640388587,0.0744114865772719));
#71607=CARTESIAN_POINT('Origin',(0.0185824901785092,-0.0326413645154682,
0.072958564314666));
#71608=CARTESIAN_POINT('Origin',(0.0186512205433514,-0.0326412102439409,
0.0744261714448057));
#71609=CARTESIAN_POINT('Origin',(0.0186452323088342,-0.0326413658176302,
0.0744711213127881));
#71610=CARTESIAN_POINT('Ctrl Pts',(0.00237294324046329,-0.0337436976235975,
0.0742273067962073));
#71611=CARTESIAN_POINT('Ctrl Pts',(0.00237363854950455,-0.0336723290703325,
0.0742790307133109));
#71612=CARTESIAN_POINT('Ctrl Pts',(0.00237526409629952,-0.033601104548885,
0.0743307337562853));
#71613=CARTESIAN_POINT('Ctrl Pts',(0.00238045414521322,-0.0333736987606857,
0.0744958113307069));
#71614=CARTESIAN_POINT('Ctrl Pts',(0.00239510874438618,-0.0331450831799192,
0.0746603190354133));
#71615=CARTESIAN_POINT('Ctrl Pts',(0.00238173582579931,-0.0337436976235975,
0.0744771521292499));
#71616=CARTESIAN_POINT('Ctrl Pts',(0.00238467828163104,-0.0336723290703325,
0.0745287969645084));
#71617=CARTESIAN_POINT('Ctrl Pts',(0.00238854918924797,-0.033601104548885,
0.0745803805193434));
#71618=CARTESIAN_POINT('Ctrl Pts',(0.00240090823048522,-0.0333736987606857,
0.0747450765918053));
#71619=CARTESIAN_POINT('Ctrl Pts',(0.00242269811526736,-0.0331450831799192,
0.0749087920251213));
#71620=CARTESIAN_POINT('Ctrl Pts',(0.00238182375165267,-0.0337436976235975,
0.0744796505825803));
#71621=CARTESIAN_POINT('Ctrl Pts',(0.00238478867895231,-0.0336723290703325,
0.0745312946270204));
#71622=CARTESIAN_POINT('Ctrl Pts',(0.00238868204017745,-0.033601104548885,
0.074582876986974));
#71623=CARTESIAN_POINT('Ctrl Pts',(0.00240111277133794,-0.0333736987606857,
0.0747475692444162));
#71624=CARTESIAN_POINT('Ctrl Pts',(0.00242297400897617,-0.0331450831799192,
0.0749112767550183));
#71625=CARTESIAN_POINT('',(0.0023839040237067,-0.0336938721132548,0.0745132128858211));
#71626=CARTESIAN_POINT('',(0.00240367281197103,-0.0333679869984219,0.0747487267053694));
#71627=CARTESIAN_POINT('Ctrl Pts',(0.00238390402370562,-0.0336938721132476,
0.0745132128858081));
#71628=CARTESIAN_POINT('Ctrl Pts',(0.00238532181398584,-0.0336629187933822,
0.0745356183229366));
#71629=CARTESIAN_POINT('Ctrl Pts',(0.00238687034366562,-0.033631995230096,
0.0745580082925362));
#71630=CARTESIAN_POINT('Ctrl Pts',(0.00238854918924793,-0.033601104548887,
0.0745803805193432));
#71631=CARTESIAN_POINT('Ctrl Pts',(0.00239276198728257,-0.0335235892595373,
0.074636520091747));
#71632=CARTESIAN_POINT('Ctrl Pts',(0.00239780299271234,-0.033445866865335,
0.0746926476830146));
#71633=CARTESIAN_POINT('Ctrl Pts',(0.00240367281094795,-0.0333679869925471,
0.0747487266973178));
#71634=CARTESIAN_POINT('Ctrl Pts',(0.00240367675719604,-0.0333679692464398,
0.0747487710027038));
#71635=CARTESIAN_POINT('Ctrl Pts',(0.00240412689138218,-0.033339189539121,
0.0747487179270901));
#71636=CARTESIAN_POINT('Ctrl Pts',(0.00240446390868399,-0.0333104081088676,
0.0747486749194812));
#71637=CARTESIAN_POINT('Ctrl Pts',(0.00240490930745797,-0.0332532698468693,
0.0747486124976845));
#71638=CARTESIAN_POINT('Ctrl Pts',(0.00240502102613422,-0.0332249172402823,
0.0747485927389032));
#71639=CARTESIAN_POINT('Ctrl Pts',(0.00240502395830143,-0.0331960985318751,
0.0747485854943265));
#71640=CARTESIAN_POINT('Ctrl Pts',(0.00240502397625562,-0.0331956312606631,
0.0747485853800244));
#71641=CARTESIAN_POINT('Ctrl Pts',(0.00240502396467461,-0.0331951640388587,
0.0747485852693819));
#71642=CARTESIAN_POINT('',(0.00239201124142713,-0.0331951640388587,0.074624264438329));
#71643=CARTESIAN_POINT('',(0.00239851760306085,-0.0331951640388687,0.0746864248538654));
#71644=CARTESIAN_POINT('',(0.00237736578028421,-0.0335216366567729,0.0743883766049044));
#71645=CARTESIAN_POINT('Origin',(0.0189232670005926,-0.0326434571526242,
0.0724900041920831));
#71646=CARTESIAN_POINT('',(0.00237872314766524,-0.0336938721132325,0.0743883202978607));
#71647=CARTESIAN_POINT('Origin',(-0.00853246199787757,-0.0336938867896247,
0.074840944499333));
#71648=CARTESIAN_POINT('',(0.00238131358569597,-0.0336938721132536,0.0744507665918509));
#71649=CARTESIAN_POINT('Ctrl Pts',(0.00212379741339946,-0.0335235895815171,
0.0741635145584381));
#71650=CARTESIAN_POINT('Ctrl Pts',(0.00212398346790408,-0.0334144449262748,
0.0742461161618138));
#71651=CARTESIAN_POINT('Ctrl Pts',(0.00212587622312389,-0.0333049234473147,
0.0743288088206783));
#71652=CARTESIAN_POINT('Ctrl Pts',(0.0021294828370589,-0.0331951640388587,
0.0744114865772718));
#71653=CARTESIAN_POINT('Ctrl Pts',(0.00220880789566106,-0.0335235895815171,
0.0742384437943317));
#71654=CARTESIAN_POINT('Ctrl Pts',(0.00221002549861985,-0.0334144449262748,
0.0743198750610488));
#71655=CARTESIAN_POINT('Ctrl Pts',(0.00221292680914344,-0.0333049234473147,
0.0744013747276649));
#71656=CARTESIAN_POINT('Ctrl Pts',(0.00221751755741549,-0.0331951640388587,
0.0744828382450707));
#71657=CARTESIAN_POINT('Ctrl Pts',(0.00229381837792267,-0.0335235895815171,
0.0743133730302253));
#71658=CARTESIAN_POINT('Ctrl Pts',(0.00229606752933562,-0.0334144449262748,
0.0743936339602838));
#71659=CARTESIAN_POINT('Ctrl Pts',(0.00229997739516298,-0.0333049234473147,
0.0744739406346515));
#71660=CARTESIAN_POINT('Ctrl Pts',(0.00230555227777208,-0.0331951640388587,
0.0745541899128695));
#71661=CARTESIAN_POINT('Ctrl Pts',(0.00237882886018428,-0.0335235895815171,
0.0743883022661188));
#71662=CARTESIAN_POINT('Ctrl Pts',(0.00238210956005139,-0.0334144449262748,
0.0744673928595188));
#71663=CARTESIAN_POINT('Ctrl Pts',(0.00238702798118253,-0.0333049234473147,
0.0745465065416382));
#71664=CARTESIAN_POINT('Ctrl Pts',(0.00239358699812867,-0.0331951640388587,
0.0746255415806684));
#71665=CARTESIAN_POINT('',(0.00226074703925309,-0.0331951640388687,0.0745178755078105));
#71666=CARTESIAN_POINT('Ctrl Pts',(0.00212893797680065,-0.0332121607145973,
0.0743986820497332));
#71667=CARTESIAN_POINT('Ctrl Pts',(0.00217181179869377,-0.0332625444109943,
0.0743969035298045));
#71668=CARTESIAN_POINT('Ctrl Pts',(0.00221394683735506,-0.0333135300747218,
0.0743951556565651));
#71669=CARTESIAN_POINT('Ctrl Pts',(0.00229677279440457,-0.0334167203140626,
0.0743917198160283));
#71670=CARTESIAN_POINT('Ctrl Pts',(0.0023374316336624,-0.0334688847587328,
0.0743900331794583));
#71671=CARTESIAN_POINT('Ctrl Pts',(0.00237736578099208,-0.033521636656241,
0.074388376605033));
#71672=CARTESIAN_POINT('Ctrl Pts',(0.00238527708192473,-0.0336938721132474,
0.0745117209813181));
#71673=CARTESIAN_POINT('Ctrl Pts',(0.00238739435486032,-0.0336474569765,
0.0745453103559748));
#71674=CARTESIAN_POINT('Ctrl Pts',(0.00238990468875923,-0.033601104548885,
0.074578872643713));
#71675=CARTESIAN_POINT('Ctrl Pts',(0.00239626027702875,-0.0334837508592656,
0.074663844639805));
#71676=CARTESIAN_POINT('Ctrl Pts',(0.00240513097081255,-0.0333660264659097,
0.0747485909932007));
#71677=CARTESIAN_POINT('Ctrl Pts',(0.00238390402370508,-0.0336938721132474,
0.0745132128857947));
#71678=CARTESIAN_POINT('Ctrl Pts',(0.00238603002925264,-0.0336474569765,
0.0745468102974167));
#71679=CARTESIAN_POINT('Ctrl Pts',(0.00238854918924798,-0.033601104548885,
0.0745803805193434));
#71680=CARTESIAN_POINT('Ctrl Pts',(0.00239492712316441,-0.0334837508592656,
0.0746653726029762));
#71681=CARTESIAN_POINT('Ctrl Pts',(0.00240382074801805,-0.0333660264659097,
0.0747501383729442));
#71682=CARTESIAN_POINT('Ctrl Pts',(0.00215368868249986,-0.0336938721132474,
0.0747633547175056));
#71683=CARTESIAN_POINT('Ctrl Pts',(0.00215727885119442,-0.0336474569765,
0.0747982996559134));
#71684=CARTESIAN_POINT('Ctrl Pts',(0.00216127784851377,-0.033601104548885,
0.0748332001724142));
#71685=CARTESIAN_POINT('Ctrl Pts',(0.00217140239029833,-0.0334837508592656,
0.0749215602560544));
#71686=CARTESIAN_POINT('Ctrl Pts',(0.00218414077860928,-0.0333660264659097,
0.0750095815272931));
#71687=CARTESIAN_POINT('',(0.00215638230256883,-0.0336769361243754,0.0747746107158768));
#71688=CARTESIAN_POINT('',(0.00215506173625341,-0.0336938721132327,0.0747618628178939));
#71689=CARTESIAN_POINT('Ctrl Pts',(0.00215638230256886,-0.0336769361243751,
0.0747746107158772));
#71690=CARTESIAN_POINT('Ctrl Pts',(0.00215615992238297,-0.033679758667006,
0.0747724861421816));
#71691=CARTESIAN_POINT('Ctrl Pts',(0.00215593868522542,-0.0336825812712914,
0.0747703615300778));
#71692=CARTESIAN_POINT('Ctrl Pts',(0.00215549849665084,-0.0336882266005929,
0.0747661122309904));
#71693=CARTESIAN_POINT('Ctrl Pts',(0.00215527954523117,-0.0336910493256095,
0.0747639875440074));
#71694=CARTESIAN_POINT('Ctrl Pts',(0.00215506173625251,-0.0336938721132332,
0.0747618628178946));
#71695=CARTESIAN_POINT('Ctrl Pts',(0.00215638230256887,-0.0336769361243754,
0.0747746107158769));
#71696=CARTESIAN_POINT('Ctrl Pts',(0.0021980683132912,-0.0336279007656795,
0.0747702474203919));
#71697=CARTESIAN_POINT('Ctrl Pts',(0.00224034786837482,-0.0335767878916504,
0.0747658219983228));
#71698=CARTESIAN_POINT('Ctrl Pts',(0.00232320394749111,-0.0334733199151693,
0.0747571494112931));
#71699=CARTESIAN_POINT('Ctrl Pts',(0.00236382979889138,-0.0334209645163038,
0.0747528970832124));
#71700=CARTESIAN_POINT('Ctrl Pts',(0.00240367281091008,-0.0333679869844681,
0.0747487266953188));
#71701=CARTESIAN_POINT('',(0.00226948287999006,-0.0336938721132538,0.0746375378518675));
#71702=CARTESIAN_POINT('Origin',(0.00812378219310841,-0.0315241814719618,
0.07415));
#71703=CARTESIAN_POINT('',(0.00215638230386339,-0.0337108120655394,0.0747746107157469));
#71704=CARTESIAN_POINT('',(0.00215773009560755,-0.0336938721132327,0.0747873557640231));
#71705=CARTESIAN_POINT('Origin',(0.0185450458257195,-0.0345562511617489,
0.0741829112955836));
#71706=CARTESIAN_POINT('Ctrl Pts',(0.00215773009561513,-0.0336938721132297,
0.0747873557640264));
#71707=CARTESIAN_POINT('Ctrl Pts',(0.0021575032128262,-0.0336910493391369,
0.0747852319979679));
#71708=CARTESIAN_POINT('Ctrl Pts',(0.00215727745417631,-0.0336882266073566,
0.0747831080183507));
#71709=CARTESIAN_POINT('Ctrl Pts',(0.00215682818914659,-0.0336825812712765,
0.0747788596641427));
#71710=CARTESIAN_POINT('Ctrl Pts',(0.00215660468275411,-0.0336797586669985,
0.0747767352895666));
#71711=CARTESIAN_POINT('Ctrl Pts',(0.0021563823025688,-0.033676936124375,
0.0747746107158766));
#71712=CARTESIAN_POINT('Origin',(0.0183123534849744,-0.0345562514305373,
0.0719598466703149));
#71713=CARTESIAN_POINT('Ctrl Pts',(0.00238914140683346,-0.034243627687391,
0.0745882009269639));
#71714=CARTESIAN_POINT('Ctrl Pts',(0.00240566842724529,-0.033943005420181,
0.0748044864697307));
#71715=CARTESIAN_POINT('Ctrl Pts',(0.00243844000940833,-0.0336441434784052,
0.0750189126850498));
#71716=CARTESIAN_POINT('Ctrl Pts',(0.00241360232646182,-0.034243627687391,
0.0748370013759405));
#71717=CARTESIAN_POINT('Ctrl Pts',(0.00243951301049845,-0.033943005420181,
0.0750523643599149));
#71718=CARTESIAN_POINT('Ctrl Pts',(0.00248157210737336,-0.0336441434784052,
0.075265163821342));
#71719=CARTESIAN_POINT('Ctrl Pts',(0.0024138469356581,-0.034243627687391,
0.0748394893804303));
#71720=CARTESIAN_POINT('Ctrl Pts',(0.00243985145633099,-0.033943005420181,
0.0750548431388167));
#71721=CARTESIAN_POINT('Ctrl Pts',(0.00248200342835301,-0.0336441434784052,
0.0752676263327049));
#71722=CARTESIAN_POINT('',(0.00241803668792201,-0.0341934961088741,0.0748729061004349));
#71723=CARTESIAN_POINT('',(0.0024525545003163,-0.0338664212873141,0.0751067138871893));
#71724=CARTESIAN_POINT('Origin',(0.0190764587066775,-0.0345610751535256,
0.0732760016444799));
#71725=CARTESIAN_POINT('Origin',(-0.00836090388560083,-0.0336938005063928,
0.0769309530129564));
#71726=CARTESIAN_POINT('',(0.0024331008925787,-0.0336938721132327,0.0749832294616745));
#71727=CARTESIAN_POINT('',(0.00244349750017906,-0.0336938721132427,0.0750448586800035));
#71728=CARTESIAN_POINT('',(0.00240367281090953,-0.0340203938281605,0.0747487266953136));
#71729=CARTESIAN_POINT('Origin',(0.0190479843192207,-0.0345589643246074,
0.0737563366905984));
#71730=CARTESIAN_POINT('',(0.00240502396467459,-0.0341934961088739,0.074748585269382));
#71731=CARTESIAN_POINT('Origin',(-0.00855455086234155,-0.0341934220717637,
0.0758957286238388));
#71732=CARTESIAN_POINT('',(0.0024115303263083,-0.0341934961088841,0.0748107456849185));
#71733=CARTESIAN_POINT('Ctrl Pts',(0.00213648542098265,-0.0340223579322397,
0.0745402273216054));
#71734=CARTESIAN_POINT('Ctrl Pts',(0.00214186767350316,-0.0339125849573575,
0.0746228077596185));
#71735=CARTESIAN_POINT('Ctrl Pts',(0.0021489553671536,-0.0338030433565231,
0.0747052187691935));
#71736=CARTESIAN_POINT('Ctrl Pts',(0.00215773009560691,-0.0336938721132327,
0.0747873557640227));
#71737=CARTESIAN_POINT('Ctrl Pts',(0.00222603299406526,-0.0340223579322397,
0.074609670910117));
#71738=CARTESIAN_POINT('Ctrl Pts',(0.00223237305478783,-0.0339125849573575,
0.0746910162535475));
#71739=CARTESIAN_POINT('Ctrl Pts',(0.00224039232001169,-0.0338030433565231,
0.0747721732120223));
#71740=CARTESIAN_POINT('Ctrl Pts',(0.00225007133424981,-0.0336938721132327,
0.0748530389085596));
#71741=CARTESIAN_POINT('Ctrl Pts',(0.00231558056714786,-0.0340223579322397,
0.0746791144986287));
#71742=CARTESIAN_POINT('Ctrl Pts',(0.0023228784360725,-0.0339125849573575,
0.0747592247474764));
#71743=CARTESIAN_POINT('Ctrl Pts',(0.00233182927286978,-0.0338030433565231,
0.0748391276548511));
#71744=CARTESIAN_POINT('Ctrl Pts',(0.00234241257289271,-0.0336938721132327,
0.0749187220530965));
#71745=CARTESIAN_POINT('Ctrl Pts',(0.00240512814023047,-0.0340223579322397,
0.0747485580871403));
#71746=CARTESIAN_POINT('Ctrl Pts',(0.00241338381735716,-0.0339125849573575,
0.0748274332414054));
#71747=CARTESIAN_POINT('Ctrl Pts',(0.00242326622572788,-0.0338030433565231,
0.0749060820976799));
#71748=CARTESIAN_POINT('Ctrl Pts',(0.00243475381153561,-0.0336938721132327,
0.0749844051976334));
#71749=CARTESIAN_POINT('',(0.00229541549410313,-0.0336938721132427,0.0748852926128588));
#71750=CARTESIAN_POINT('Ctrl Pts',(0.00215638230744163,-0.0337108120662682,
0.0747746107153668));
#71751=CARTESIAN_POINT('Ctrl Pts',(0.00219914793354054,-0.0337611408994438,
0.0747701344160031));
#71752=CARTESIAN_POINT('Ctrl Pts',(0.00224113318184206,-0.0338121088781615,
0.0747657397991719));
#71753=CARTESIAN_POINT('Ctrl Pts',(0.00232358117069541,-0.0339153382773233,
0.0747571099271531));
#71754=CARTESIAN_POINT('Ctrl Pts',(0.00236400903073593,-0.0339675558473108,
0.074752878322926));
#71755=CARTESIAN_POINT('Ctrl Pts',(0.00240367281094967,-0.0340203938281304,
0.0747487266953146));
#71756=CARTESIAN_POINT('Ctrl Pts',(0.00241931371808394,-0.0341934961088741,
0.0748713304821396));
#71757=CARTESIAN_POINT('Ctrl Pts',(0.00243422665749493,-0.0340287516186244,
0.0749892658735396));
#71758=CARTESIAN_POINT('Ctrl Pts',(0.0024540012132723,-0.0338644633283559,
0.0751064841283056));
#71759=CARTESIAN_POINT('Ctrl Pts',(0.00241803668792207,-0.0341934961088741,
0.0748729061004349));
#71760=CARTESIAN_POINT('Ctrl Pts',(0.00243298220199995,-0.0340287516186244,
0.0749908678934274));
#71761=CARTESIAN_POINT('Ctrl Pts',(0.00245279039580763,-0.0338644633283559,
0.0751081111808905));
#71762=CARTESIAN_POINT('Ctrl Pts',(0.00220525882686514,-0.0341934961088741,
0.0751354345048027));
#71763=CARTESIAN_POINT('Ctrl Pts',(0.00222563190886776,-0.0340287516186244,
0.0752577953124335));
#71764=CARTESIAN_POINT('Ctrl Pts',(0.00225104484745915,-0.0338644633283559,
0.0753792095301615));
#71765=CARTESIAN_POINT('',(0.00220737723511777,-0.0341764758832392,0.0751480743277191));
#71766=CARTESIAN_POINT('',(0.00220525882686678,-0.034193496108874,0.0751354345048007));
#71767=CARTESIAN_POINT('Origin',(0.0186196216528808,-0.0345621026454919,
0.0728987275951916));
#71768=CARTESIAN_POINT('Ctrl Pts',(0.00220737723570005,-0.034176475883748,
0.075148074325991));
#71769=CARTESIAN_POINT('Ctrl Pts',(0.00224970356681359,-0.0341260050041583,
0.0751409340258941));
#71770=CARTESIAN_POINT('Ctrl Pts',(0.00229129416008601,-0.0340749269150491,
0.0751339178033822));
#71771=CARTESIAN_POINT('Ctrl Pts',(0.00237303613459714,-0.0339715436310937,
0.075120128256751));
#71772=CARTESIAN_POINT('Ctrl Pts',(0.0024131565058429,-0.033919277824191,
0.0751133601699633));
#71773=CARTESIAN_POINT('Ctrl Pts',(0.00245255449839893,-0.0338664212861448,
0.0751067138851224));
#71774=CARTESIAN_POINT('',(0.00231164775740439,-0.0341934961088841,0.0750041703026279));
#71775=CARTESIAN_POINT('Origin',(0.00812378219310841,-0.0315241814719618,
0.07415));
#71776=CARTESIAN_POINT('',(0.00220737723598346,-0.0342105180190534,0.0751480743284265));
#71777=CARTESIAN_POINT('',(0.00220952263615493,-0.0341934961088739,0.0751607095987538));
#71778=CARTESIAN_POINT('Origin',(0.0186172940355559,-0.0345621701730135,
0.072853459403901));
#71779=CARTESIAN_POINT('Origin',(0.0184492530654878,-0.0345621040853264,
0.0718887970165648));
#71780=CARTESIAN_POINT('Origin',(0.0184618988578972,-0.0345621714960468,
0.0719323247288287));
#71781=CARTESIAN_POINT('Ctrl Pts',(0.0024328513723479,-0.0346945769586966,
0.0749817503506608));
#71782=CARTESIAN_POINT('Ctrl Pts',(0.00245027271645716,-0.0345275153362945,
0.0751009491752261));
#71783=CARTESIAN_POINT('Ctrl Pts',(0.00247144725993594,-0.0343603235965186,
0.0752196309454758));
#71784=CARTESIAN_POINT('Ctrl Pts',(0.00249630716099106,-0.034193496108874,
0.0753374455841857));
#71785=CARTESIAN_POINT('Ctrl Pts',(0.00244679668926106,-0.0346945769586966,
0.0750644156790485));
#71786=CARTESIAN_POINT('Ctrl Pts',(0.00246594949177079,-0.0345275153362945,
0.0751833224133676));
#71787=CARTESIAN_POINT('Ctrl Pts',(0.00248884675552448,-0.0343603235965186,
0.0753016575650486));
#71788=CARTESIAN_POINT('Ctrl Pts',(0.00251541555892339,-0.034193496108874,
0.0754190721577369));
#71789=CARTESIAN_POINT('Ctrl Pts',(0.00246074200617428,-0.0346945769586966,
0.0751470810074338));
#71790=CARTESIAN_POINT('Ctrl Pts',(0.00248162626708448,-0.0345275153362945,
0.0752656956515077));
#71791=CARTESIAN_POINT('Ctrl Pts',(0.00250624625111307,-0.0343603235965186,
0.075383684184621));
#71792=CARTESIAN_POINT('Ctrl Pts',(0.00253452395685577,-0.034193496108874,
0.0755006987312884));
#71793=CARTESIAN_POINT('Ctrl Pts',(0.00247468732308737,-0.0346945769586966,
0.0752297463358237));
#71794=CARTESIAN_POINT('Ctrl Pts',(0.00249730304239805,-0.0345275153362945,
0.0753480688896505));
#71795=CARTESIAN_POINT('Ctrl Pts',(0.00252364574670156,-0.0343603235965186,
0.0754657108041943));
#71796=CARTESIAN_POINT('Ctrl Pts',(0.00255363235478807,-0.034193496108874,
0.0755823253048392));
#71797=CARTESIAN_POINT('',(0.00247468732294121,-0.0346945769586966,0.0752297463349562));
#71798=CARTESIAN_POINT('',(0.00252381793467388,-0.0343667727832779,0.0754609253620189));
#71799=CARTESIAN_POINT('Origin',(0.018954003831437,-0.0345626461565567,
0.0718936746724204));
#71800=CARTESIAN_POINT('Origin',(-0.00823743066395237,-0.0341934771027668,
0.0779800887105191));
#71801=CARTESIAN_POINT('',(0.00249664906299847,-0.034193496108874,0.075338906109001));
#71802=CARTESIAN_POINT('',(0.00251089488590508,-0.034193496108884,0.0753997609077536));
#71803=CARTESIAN_POINT('',(0.00245255450041352,-0.0345211942962698,0.0751067138848273));
#71804=CARTESIAN_POINT('Origin',(0.0190307066060976,-0.0345625596119866,
0.0723683396847151));
#71805=CARTESIAN_POINT('',(0.00245389410775944,-0.0346945769586885,0.0751064878983125));
#71806=CARTESIAN_POINT('Origin',(-0.00845552983703033,-0.0346945685853896,
0.0769468640561198));
#71807=CARTESIAN_POINT('',(0.00246429071536032,-0.0346945769587026,0.0751681171166444));
#71808=CARTESIAN_POINT('Ctrl Pts',(0.00217280268249536,-0.0345231616327841,
0.0749154037263385));
#71809=CARTESIAN_POINT('Ctrl Pts',(0.00218335269526068,-0.0344132092796988,
0.0749974296005833));
#71810=CARTESIAN_POINT('Ctrl Pts',(0.00219559880420149,-0.0343032738558979,
0.0750792330239777));
#71811=CARTESIAN_POINT('Ctrl Pts',(0.0022095226361549,-0.0341934961088739,
0.0751607095987539));
#71812=CARTESIAN_POINT('Ctrl Pts',(0.0022665338036514,-0.0345231616327841,
0.0749790874217822));
#71813=CARTESIAN_POINT('Ctrl Pts',(0.00227796160649894,-0.0344132092796988,
0.0750598213444847));
#71814=CARTESIAN_POINT('Ctrl Pts',(0.00229105873723346,-0.0343032738558979,
0.0751403147266002));
#71815=CARTESIAN_POINT('Ctrl Pts',(0.00230580577542545,-0.0341934961088739,
0.0752204648766023));
#71816=CARTESIAN_POINT('Ctrl Pts',(0.00236026492480743,-0.0345231616327841,
0.0750427711172259));
#71817=CARTESIAN_POINT('Ctrl Pts',(0.0023725705177372,-0.0344132092796988,
0.0751222130883861));
#71818=CARTESIAN_POINT('Ctrl Pts',(0.00238651867026543,-0.0343032738558979,
0.0752013964292226));
#71819=CARTESIAN_POINT('Ctrl Pts',(0.002402088914696,-0.0341934961088739,
0.0752802201544507));
#71820=CARTESIAN_POINT('Ctrl Pts',(0.00245399604596347,-0.0345231616327841,
0.0751064548126695));
#71821=CARTESIAN_POINT('Ctrl Pts',(0.00246717942897545,-0.0344132092796988,
0.0751846048322875));
#71822=CARTESIAN_POINT('Ctrl Pts',(0.0024819786032974,-0.0343032738558979,
0.075262478131845));
#71823=CARTESIAN_POINT('Ctrl Pts',(0.00249837205396655,-0.0341934961088739,
0.0753399754322991));
#71824=CARTESIAN_POINT('',(0.0023530858495867,-0.0341934961088839,0.0752498078538874));
#71825=CARTESIAN_POINT('Ctrl Pts',(0.00220737723938524,-0.0342105180195385,
0.075148074327847));
#71826=CARTESIAN_POINT('Ctrl Pts',(0.00224975115590851,-0.0342610556241365,
0.0751409260142033));
#71827=CARTESIAN_POINT('Ctrl Pts',(0.00229136469440918,-0.0343122189870295,
0.075133905973352));
#71828=CARTESIAN_POINT('Ctrl Pts',(0.00237310749295284,-0.0344158119695179,
0.0751201162836077));
#71829=CARTESIAN_POINT('Ctrl Pts',(0.00241320331961001,-0.034468199045008,
0.0751133522747961));
#71830=CARTESIAN_POINT('Ctrl Pts',(0.00245255450043772,-0.0345211942962506,
0.0751067138848174));
#71831=CARTESIAN_POINT('Ctrl Pts',(0.00247586261179299,-0.0346945769586932,
0.0752280940445576));
#71832=CARTESIAN_POINT('Ctrl Pts',(0.00249815144332193,-0.0345296777077528,
0.0753448607855227));
#71833=CARTESIAN_POINT('Ctrl Pts',(0.00252524730602475,-0.0343648066252516,
0.0754606065328785));
#71834=CARTESIAN_POINT('Ctrl Pts',(0.00247468732293958,-0.0346945769586932,
0.0752297463349473));
#71835=CARTESIAN_POINT('Ctrl Pts',(0.0024970103144032,-0.0345296777077528,
0.0753465373741779));
#71836=CARTESIAN_POINT('Ctrl Pts',(0.00252414131212109,-0.0343648066252516,
0.0754623059871751));
#71837=CARTESIAN_POINT('Ctrl Pts',(0.00227881362528771,-0.0346945769586932,
0.0755051171319187));
#71838=CARTESIAN_POINT('Ctrl Pts',(0.0023068297131307,-0.0345296777077528,
0.0756259577212511));
#71839=CARTESIAN_POINT('Ctrl Pts',(0.00233981631417512,-0.0343648066252516,
0.0757455371231554));
#71840=CARTESIAN_POINT('',(0.0022817215141913,-0.0346775396664978,0.0755175989972332));
#71841=CARTESIAN_POINT('',(0.00227881362529054,-0.0346945769586886,0.0755051171319192));
#71842=CARTESIAN_POINT('Origin',(0.0184108143037993,-0.0345626619277667,
0.0715850084953972));
#71843=CARTESIAN_POINT('Ctrl Pts',(0.00228172151476219,-0.0346775396670097,
0.0755175989955));
#71844=CARTESIAN_POINT('Ctrl Pts',(0.00232354889847931,-0.0346269749928344,
0.0755078073879644));
#71845=CARTESIAN_POINT('Ctrl Pts',(0.00236463290806837,-0.0345757902891101,
0.0754981897641689));
#71846=CARTESIAN_POINT('Ctrl Pts',(0.00244534805337453,-0.0344721681088584,
0.075479294731196));
#71847=CARTESIAN_POINT('Ctrl Pts',(0.00248494754623924,-0.0344197714290507,
0.0754700247352496));
#71848=CARTESIAN_POINT('Ctrl Pts',(0.00252381793443664,-0.0343667727831552,
0.07546092536172));
#71849=CARTESIAN_POINT('',(0.00237675047412587,-0.0346945769587026,0.0753674317334477));
#71850=CARTESIAN_POINT('Origin',(0.00812378219310841,-0.0315241814719618,
0.07415));
#71851=CARTESIAN_POINT('',(0.00228172151550705,-0.0347116136489607,0.0755175989976839));
#71852=CARTESIAN_POINT('',(0.00228465605720542,-0.0346945769586885,0.0755300746244476));
#71853=CARTESIAN_POINT('Origin',(0.0183986768196557,-0.0345626681602985,
0.0715413506044575));
#71854=CARTESIAN_POINT('Origin',(0.0184804353446439,-0.0345626630729688,
0.0718824000672343));
#71855=CARTESIAN_POINT('Origin',(0.0184889314692112,-0.0345626693828237,
0.0719269102778483));
#71856=CARTESIAN_POINT('Ctrl Pts',(0.00248873755723595,-0.0352450361874068,
0.0753011014626653));
#71857=CARTESIAN_POINT('Ctrl Pts',(0.00253215206129927,-0.0349452760959493,
0.0755136306585492));
#71858=CARTESIAN_POINT('Ctrl Pts',(0.00259145179795907,-0.034644428984174,
0.075722285923276));
#71859=CARTESIAN_POINT('Ctrl Pts',(0.00248929764596918,-0.0352450361874068,
0.0753035635604722));
#71860=CARTESIAN_POINT('Ctrl Pts',(0.00253280500957504,-0.0349452760959493,
0.075516071632263));
#71861=CARTESIAN_POINT('Ctrl Pts',(0.00259219575082006,-0.034644428984174,
0.0757246988383471));
#71862=CARTESIAN_POINT('Ctrl Pts',(0.00254475197599172,-0.0352450361874068,
0.0755473356205648));
#71863=CARTESIAN_POINT('Ctrl Pts',(0.00259745335371073,-0.0349452760959493,
0.0757577521979789));
#71864=CARTESIAN_POINT('Ctrl Pts',(0.00266585444992848,-0.034644428984174,
0.07596360132064));
#71865=CARTESIAN_POINT('Ctrl Pts',(0.00254530651929195,-0.0352450361874068,
0.0755497733411657));
#71866=CARTESIAN_POINT('Ctrl Pts',(0.00259809983715208,-0.0349452760959493,
0.075760169003636));
#71867=CARTESIAN_POINT('Ctrl Pts',(0.00266659103691956,-0.034644428984174,
0.0759659903454629));
#71868=CARTESIAN_POINT('',(0.00255362199724152,-0.0351951634053262,0.0755822945559194));
#71869=CARTESIAN_POINT('',(0.00261718186944784,-0.0348678972925388,0.0758099632150931));
#71870=CARTESIAN_POINT('Origin',(0.0185317384632803,-0.0345636767885976,
0.070571876353144));
#71871=CARTESIAN_POINT('Origin',(-0.00796241552129287,-0.0346946199341063,
0.0789991807159483));
#71872=CARTESIAN_POINT('',(0.00258240495244123,-0.0346945769330289,0.0756898906696988));
#71873=CARTESIAN_POINT('',(0.0026004437710606,-0.0346945769458128,0.0757497308912099));
#71874=CARTESIAN_POINT('',(0.00252381793464359,-0.0350221583435275,0.0754609253616882));
#71875=CARTESIAN_POINT('Origin',(0.0187097009618073,-0.0345628458715169,
0.0710185000669408));
#71876=CARTESIAN_POINT('',(0.00252502157108339,-0.035195136029876,0.0754606404896734));
#71877=CARTESIAN_POINT('Origin',(-0.00820389956172542,-0.03519518383668,
0.0779722326526504));
#71878=CARTESIAN_POINT('',(0.00255363235447195,-0.035195137132875,0.0755823253039986));
#71879=CARTESIAN_POINT('Ctrl Pts',(0.00223260586095877,-0.0350241211494342,
0.0752875594153934));
#71880=CARTESIAN_POINT('Ctrl Pts',(0.00224827527548829,-0.0349144232818961,
0.0753687079538924));
#71881=CARTESIAN_POINT('Ctrl Pts',(0.0022656314671941,-0.0348045283579412,
0.0754495811657081));
#71882=CARTESIAN_POINT('Ctrl Pts',(0.00228465605976146,-0.0346945769439158,
0.0755300746352625));
#71883=CARTESIAN_POINT('Ctrl Pts',(0.00233015078822936,-0.0350241211494342,
0.0753452320169192));
#71884=CARTESIAN_POINT('Ctrl Pts',(0.00234661461919822,-0.0349144232818961,
0.0754250369140401));
#71885=CARTESIAN_POINT('Ctrl Pts',(0.00236473792881249,-0.0348045283579412,
0.075504549259088));
#71886=CARTESIAN_POINT('Ctrl Pts',(0.00238450129331217,-0.0346945769439158,
0.0755836663430184));
#71887=CARTESIAN_POINT('Ctrl Pts',(0.00242769571549996,-0.0350241211494342,
0.0754029046184451));
#71888=CARTESIAN_POINT('Ctrl Pts',(0.00244495396290814,-0.0349144232818961,
0.0754813658741877));
#71889=CARTESIAN_POINT('Ctrl Pts',(0.00246384439043087,-0.0348045283579412,
0.0755595173524679));
#71890=CARTESIAN_POINT('Ctrl Pts',(0.00248434652686288,-0.0346945769439158,
0.0756372580507742));
#71891=CARTESIAN_POINT('Ctrl Pts',(0.00252524064277055,-0.0350241211494342,
0.0754605772199709));
#71892=CARTESIAN_POINT('Ctrl Pts',(0.00254329330661806,-0.0349144232818961,
0.0755376948343354));
#71893=CARTESIAN_POINT('Ctrl Pts',(0.00256295085204925,-0.0348045283579412,
0.0756144854458478));
#71894=CARTESIAN_POINT('Ctrl Pts',(0.00258419176041358,-0.0346945769439158,
0.07569084975853));
#71895=CARTESIAN_POINT('',(0.00243353050467004,-0.0346945769458128,0.0756099826468189));
#71896=CARTESIAN_POINT('Ctrl Pts',(0.0022817215187041,-0.034711613649279,
0.0755175989969295));
#71897=CARTESIAN_POINT('Ctrl Pts',(0.00232353229480107,-0.0347621546532343,
0.0755078112903928));
#71898=CARTESIAN_POINT('Ctrl Pts',(0.00236460792446927,-0.0348133084097125,
0.0754981956781862));
#71899=CARTESIAN_POINT('Ctrl Pts',(0.00244532317134808,-0.0349168561544567,
0.0754793006175525));
#71900=CARTESIAN_POINT('Ctrl Pts',(0.00248493077292884,-0.0349692089015914,
0.0754700286638342));
#71901=CARTESIAN_POINT('Ctrl Pts',(0.00252381793468374,-0.0350221583434999,
0.0754609253616993));
#71902=CARTESIAN_POINT('Ctrl Pts',(0.00255440383340984,-0.0351951371254872,
0.0755810822271085));
#71903=CARTESIAN_POINT('Ctrl Pts',(0.00258399056056355,-0.035030733898092,
0.0756962256303476));
#71904=CARTESIAN_POINT('Ctrl Pts',(0.00261831100713141,-0.0348659306897825,
0.0758100477928667));
#71905=CARTESIAN_POINT('Ctrl Pts',(0.00255363235458435,-0.0351951371254872,
0.0755823253039693));
#71906=CARTESIAN_POINT('Ctrl Pts',(0.00258324478157223,-0.035030733898092,
0.075697484657049));
#71907=CARTESIAN_POINT('Ctrl Pts',(0.00261759156523801,-0.0348659306897825,
0.0758113216935779));
#71908=CARTESIAN_POINT('Ctrl Pts',(0.00242433169938697,-0.0351951371254872,
0.0757906662813757));
#71909=CARTESIAN_POINT('Ctrl Pts',(0.00245825144536512,-0.035030733898092,
0.0759084988443757));
#71910=CARTESIAN_POINT('Ctrl Pts',(0.00249701235409287,-0.0348659306897825,
0.076024828780441));
#71911=CARTESIAN_POINT('Origin',(-0.00247467617372032,-0.0308609197410693,
0.0773449024790721));
#71912=CARTESIAN_POINT('',(0.00249726018426095,-0.0351951371254872,0.0756731572726532));
#71913=CARTESIAN_POINT('Origin',(0.0090085778923309,-0.03518404674412,0.0737354131937099));
#71914=CARTESIAN_POINT('Origin',(-0.00307767051212848,-0.0352322613345126,
0.0783566974641126));
#71915=CARTESIAN_POINT('',(0.00269015874208231,-0.0351951142564657,0.0760350864107232));
#71916=CARTESIAN_POINT('',(0.00273355139268732,-0.0351951372916788,0.0761519770024135));
#71917=CARTESIAN_POINT('Origin',(0.00839212773806127,-0.035287512144001,
0.0743597447775152));
#71918=CARTESIAN_POINT('Origin',(0.00690647465570691,-0.0298325076522345,
0.066746395969514));
#71919=CARTESIAN_POINT('Origin',(-0.000254157257254604,-0.033873118223129,
0.0738958328557447));
#71920=CARTESIAN_POINT('Ctrl Pts',(0.00261993952981883,-0.0321934096636942,
0.0724809129192682));
#71921=CARTESIAN_POINT('Ctrl Pts',(0.00259006366587907,-0.0320508460843096,
0.0725794290820573));
#71922=CARTESIAN_POINT('Ctrl Pts',(0.00256285726334741,-0.0319086045660617,
0.0726786736688491));
#71923=CARTESIAN_POINT('Ctrl Pts',(0.00253836131002253,-0.0317669892864235,
0.0727784281659069));
#71924=CARTESIAN_POINT('Ctrl Pts',(0.00259735658310347,-0.0321934096636942,
0.0725616621802282));
#71925=CARTESIAN_POINT('Ctrl Pts',(0.00256892609248277,-0.0320508460843096,
0.0726605825670096));
#71926=CARTESIAN_POINT('Ctrl Pts',(0.002543174834155,-0.0319086045660617,
0.0727601922386784));
#71927=CARTESIAN_POINT('Ctrl Pts',(0.00252014059802141,-0.0317669892864235,
0.0728602721533488));
#71928=CARTESIAN_POINT('Ctrl Pts',(0.0025747736363881,-0.0321934096636942,
0.0726424114411881));
#71929=CARTESIAN_POINT('Ctrl Pts',(0.00254778851908645,-0.0320508460843096,
0.0727417360519618));
#71930=CARTESIAN_POINT('Ctrl Pts',(0.00252349240496258,-0.0319086045660617,
0.0728417108085077));
#71931=CARTESIAN_POINT('Ctrl Pts',(0.00250191988602029,-0.0317669892864235,
0.0729421161407907));
#71932=CARTESIAN_POINT('Ctrl Pts',(0.00255219068967273,-0.0321934096636942,
0.0727231607021481));
#71933=CARTESIAN_POINT('Ctrl Pts',(0.00252665094569015,-0.0320508460843096,
0.0728228895369141));
#71934=CARTESIAN_POINT('Ctrl Pts',(0.00250380997577015,-0.0319086045660617,
0.0729232293783371));
#71935=CARTESIAN_POINT('Ctrl Pts',(0.00248369917401917,-0.0317669892864235,
0.0730239601282326));
#71936=CARTESIAN_POINT('',(0.00255259470305427,-0.0321934096636942,0.0727217160819132));
#71937=CARTESIAN_POINT('',(0.00249861816834072,-0.0318665617511265,0.0729518119164843));
#71938=CARTESIAN_POINT('Origin',(0.0185752685902041,-0.0326371944423118,
0.0774642709158772));
#71939=CARTESIAN_POINT('Origin',(-0.00822206054077306,-0.0316939261509366,
0.0706682537005622));
#71940=CARTESIAN_POINT('',(0.0025849267118823,-0.0320197221621813,0.0726012362592632));
#71941=CARTESIAN_POINT('Ctrl Pts',(0.00258483310894102,-0.0320197392094734,
0.0726013958003824));
#71942=CARTESIAN_POINT('Ctrl Pts',(0.00257695335811615,-0.0319792716576031,
0.0726295797666881));
#71943=CARTESIAN_POINT('Ctrl Pts',(0.00256925259888108,-0.0319386439829669,
0.0726579521091869));
#71944=CARTESIAN_POINT('Ctrl Pts',(0.00256173090911167,-0.03189790993816,
0.0726865448288411));
#71945=CARTESIAN_POINT('Ctrl Pts',(0.00255420936801374,-0.0318571766984903,
0.0727151369833401));
#71946=CARTESIAN_POINT('Ctrl Pts',(0.00254690339562464,-0.0318163871833552,
0.072743803729002));
#71947=CARTESIAN_POINT('Ctrl Pts',(0.00253983470939491,-0.0317755399638303,
0.0727724455944296));
#71948=CARTESIAN_POINT('',(0.00258626132929582,-0.0321934096636184,0.0726013351935164));
#71949=CARTESIAN_POINT('Origin',(0.00035674042977136,-0.0324113908119595,
0.0719996587770169));
#71950=CARTESIAN_POINT('',(0.00256942801618504,-0.0321934096636663,0.0726615256377248));
#71951=CARTESIAN_POINT('Ctrl Pts',(0.00255436214565888,-0.0321934096636618,
0.0727207211778884));
#71952=CARTESIAN_POINT('Ctrl Pts',(0.00253465127678719,-0.0320835708272592,
0.0727975278208948));
#71953=CARTESIAN_POINT('Ctrl Pts',(0.00251654135050567,-0.0319739230346489,
0.0728746978283338));
#71954=CARTESIAN_POINT('Ctrl Pts',(0.00250004795967516,-0.0318646057455573,
0.0729521306882717));
#71955=CARTESIAN_POINT('Ctrl Pts',(0.0024556133303472,-0.0321934096636618,
0.0727763074733133));
#71956=CARTESIAN_POINT('Ctrl Pts',(0.00243666903981085,-0.0320835708272592,
0.0728544759394432));
#71957=CARTESIAN_POINT('Ctrl Pts',(0.00241935343007684,-0.0319739230346489,
0.0729329911157941));
#71958=CARTESIAN_POINT('Ctrl Pts',(0.00240368094564729,-0.0318646057455573,
0.0730117508473781));
#71959=CARTESIAN_POINT('Ctrl Pts',(0.00235686451503552,-0.0321934096636618,
0.0728318937687382));
#71960=CARTESIAN_POINT('Ctrl Pts',(0.00233868680283451,-0.0320835708272592,
0.0729114240579916));
#71961=CARTESIAN_POINT('Ctrl Pts',(0.002322165509648,-0.0319739230346489,
0.0729912844032544));
#71962=CARTESIAN_POINT('Ctrl Pts',(0.00230731393161943,-0.0318646057455573,
0.0730713710064846));
#71963=CARTESIAN_POINT('Ctrl Pts',(0.00225811569972384,-0.0321934096636618,
0.0728874800641631));
#71964=CARTESIAN_POINT('Ctrl Pts',(0.00224070456585816,-0.0320835708272592,
0.07296837217654));
#71965=CARTESIAN_POINT('Ctrl Pts',(0.00222497758921917,-0.0319739230346489,
0.0730495776907147));
#71966=CARTESIAN_POINT('Ctrl Pts',(0.00221094691759156,-0.0318646057455573,
0.073130991165591));
#71967=CARTESIAN_POINT('',(0.00225543231761759,-0.0321763980308446,0.0729000121134659));
#71968=CARTESIAN_POINT('',(0.00225811569971697,-0.0321934096636185,0.072887480064195));
#71969=CARTESIAN_POINT('Origin',(0.018301100644114,-0.032638623085492,0.0769450855961415));
#71970=CARTESIAN_POINT('Ctrl Pts',(0.00225543232071656,-0.0321763980306266,
0.0729000121141224));
#71971=CARTESIAN_POINT('Ctrl Pts',(0.002297409501156,-0.0321259596175108,
0.0729089534635944));
#71972=CARTESIAN_POINT('Ctrl Pts',(0.00233865937247787,-0.0320749164631984,
0.0729177398925782));
#71973=CARTESIAN_POINT('Ctrl Pts',(0.00241973769352951,-0.0319716057793896,
0.0729350099806482));
#71974=CARTESIAN_POINT('Ctrl Pts',(0.00245953455235092,-0.031919378669009,
0.0729434869107129));
#71975=CARTESIAN_POINT('Ctrl Pts',(0.00249861817015242,-0.0318665617525271,
0.0729518119168646));
#71976=CARTESIAN_POINT('',(0.00240535520139562,-0.0321934096636664,0.0728045980730641));
#71977=CARTESIAN_POINT('Origin',(0.00812378219310841,-0.0315241814719618,
0.07415));
#71978=CARTESIAN_POINT('',(0.00225543231725343,-0.032210423332378,0.0729000121133884));
#71979=CARTESIAN_POINT('',(0.00225277570667768,-0.0321934096636183,0.0729125498651181));
#71980=CARTESIAN_POINT('Origin',(0.0183166330047819,-0.0326387230361829,
0.0769024945259561));
#71981=CARTESIAN_POINT('Origin',(0.018556727463541,-0.0326386245551484,
0.0757450017082887));
#71982=CARTESIAN_POINT('Origin',(0.0185535487766797,-0.0326387242491453,
0.0757902245208387));
#71983=CARTESIAN_POINT('Ctrl Pts',(0.00253439533689285,-0.0327445246967097,
0.0727946846966241));
#71984=CARTESIAN_POINT('Ctrl Pts',(0.00248327878458362,-0.032443687833936,
0.0730054918681366));
#71985=CARTESIAN_POINT('Ctrl Pts',(0.00244818630673866,-0.0321434074405927,
0.073219550466375));
#71986=CARTESIAN_POINT('Ctrl Pts',(0.00248077689844309,-0.0327445246967097,
0.0730388671346867));
#71987=CARTESIAN_POINT('Ctrl Pts',(0.00243886983734017,-0.032443687833936,
0.0732516965586647));
#71988=CARTESIAN_POINT('Ctrl Pts',(0.00241311301183042,-0.0321434074405927,
0.0734670779678456));
#71989=CARTESIAN_POINT('',(0.00247390547970712,-0.0326943950436612,0.0730743522308083));
#71990=CARTESIAN_POINT('',(0.00243448329139577,-0.0323666188837389,0.0733073832383745));
#71991=CARTESIAN_POINT('Origin',(0.0190022764167063,-0.0326395579111547,
0.0761437190053379));
#71992=CARTESIAN_POINT('Origin',(-0.00849094901744373,-0.0321933825603011,
0.071689266830627));
#71993=CARTESIAN_POINT('',(0.00245414059759521,-0.0321934096532688,0.0731839310712801));
#71994=CARTESIAN_POINT('',(0.00244498388243575,-0.0321934096584275,0.0732457566720727));
#71995=CARTESIAN_POINT('',(0.00249861816740909,-0.0325210109756238,0.0729518119162755));
#71996=CARTESIAN_POINT('Origin',(0.0188875491908828,-0.0326393129156696,
0.0766106473652476));
#71997=CARTESIAN_POINT('',(0.00249994689401835,-0.0326943950436593,0.0729520949416965));
#71998=CARTESIAN_POINT('Origin',(-0.00831977921037526,-0.0326943765538164,
0.0706474379779526));
#71999=CARTESIAN_POINT('',(0.00248692618687274,-0.0326943950436702,0.0730132235862623));
#72000=CARTESIAN_POINT('Ctrl Pts',(0.00230893750821803,-0.0325229783203769,
0.0726709525732306));
#72001=CARTESIAN_POINT('Ctrl Pts',(0.00228854887178465,-0.032413025309245,
0.0727511100800496));
#72002=CARTESIAN_POINT('Ctrl Pts',(0.00226982148868562,-0.0323031222208069,
0.0728316771945477));
#72003=CARTESIAN_POINT('Ctrl Pts',(0.00225277570575284,-0.0321934096576658,
0.0729125498695059));
#72004=CARTESIAN_POINT('Ctrl Pts',(0.0023726429815818,-0.0325229783203769,
0.0727646689266587));
#72005=CARTESIAN_POINT('Ctrl Pts',(0.00235354622303098,-0.032413025309245,
0.0728439482549205));
#72006=CARTESIAN_POINT('Ctrl Pts',(0.00233609235562436,-0.0323031222208069,
0.0729236105999009));
#72007=CARTESIAN_POINT('Ctrl Pts',(0.00232030013580616,-0.0321934096576658,
0.0730035531308888));
#72008=CARTESIAN_POINT('Ctrl Pts',(0.00243634845494557,-0.0325229783203769,
0.0728583852800867));
#72009=CARTESIAN_POINT('Ctrl Pts',(0.00241854357427731,-0.032413025309245,
0.0729367864297913));
#72010=CARTESIAN_POINT('Ctrl Pts',(0.00240236322256311,-0.0323031222208069,
0.0730155440052541));
#72011=CARTESIAN_POINT('Ctrl Pts',(0.00238782456585947,-0.0321934096576658,
0.0730945563922718));
#72012=CARTESIAN_POINT('Ctrl Pts',(0.00250005392830934,-0.0325229783203769,
0.0729521016335148));
#72013=CARTESIAN_POINT('Ctrl Pts',(0.00248354092552364,-0.032413025309245,
0.0730296246046622));
#72014=CARTESIAN_POINT('Ctrl Pts',(0.00246863408950186,-0.0323031222208069,
0.0731074774106072));
#72015=CARTESIAN_POINT('Ctrl Pts',(0.00245534899591279,-0.0321934096576658,
0.0731855596536547));
#72016=CARTESIAN_POINT('',(0.00235345815208435,-0.0321934096584274,0.0730482404676965));
#72017=CARTESIAN_POINT('Ctrl Pts',(0.00225543232065011,-0.0322104233328924,
0.0729000121141082));
#72018=CARTESIAN_POINT('Ctrl Pts',(0.00229746638087521,-0.0322609421831408,
0.072908965579259));
#72019=CARTESIAN_POINT('Ctrl Pts',(0.00233874403892756,-0.0323120888240825,
0.0729177579269624));
#72020=CARTESIAN_POINT('Ctrl Pts',(0.00241982297379117,-0.0324156524631811,
0.0729350281457774));
#72021=CARTESIAN_POINT('Ctrl Pts',(0.00245959092292148,-0.0324680267167303,
0.0729434989179262));
#72022=CARTESIAN_POINT('Ctrl Pts',(0.00249861816745052,-0.0325210109755912,
0.0729518119162889));
#72023=CARTESIAN_POINT('Origin',(0.0106777517417982,-0.0262834582512102,
0.0667081839996702));
#72024=CARTESIAN_POINT('Origin',(-0.00137820958750585,-0.0342770679433053,
0.0665648411243571));
#72025=CARTESIAN_POINT('Ctrl Pts',(0.00247560655120864,-0.0326943950436604,
0.0730732485793327));
#72026=CARTESIAN_POINT('Ctrl Pts',(0.0024607668985846,-0.0325844576448134,
0.0731510910254874));
#72027=CARTESIAN_POINT('Ctrl Pts',(0.00244753610514621,-0.0324744968375322,
0.0732292458890192));
#72028=CARTESIAN_POINT('Ctrl Pts',(0.00243592974177329,-0.0323646534831894,
0.0733076127995393));
#72029=CARTESIAN_POINT('Ctrl Pts',(0.0023805430241299,-0.0326943950436604,
0.0731349255880212));
#72030=CARTESIAN_POINT('Ctrl Pts',(0.00236655339628062,-0.0325844576448134,
0.0732140781877471));
#72031=CARTESIAN_POINT('Ctrl Pts',(0.00235419978389844,-0.0324744968375322,
0.0732935257176657));
#72032=CARTESIAN_POINT('Ctrl Pts',(0.00234349661112315,-0.0323646534831894,
0.0733731661666505));
#72033=CARTESIAN_POINT('Ctrl Pts',(0.00228547949705116,-0.0326943950436604,
0.0731966025967096));
#72034=CARTESIAN_POINT('Ctrl Pts',(0.00227233989397664,-0.0325844576448134,
0.0732770653500068));
#72035=CARTESIAN_POINT('Ctrl Pts',(0.00226086346265067,-0.0324744968375322,
0.0733578055463122));
#72036=CARTESIAN_POINT('Ctrl Pts',(0.002251063480473,-0.0323646534831894,
0.0734387195337618));
#72037=CARTESIAN_POINT('Ctrl Pts',(0.00219041596997242,-0.0326943950436604,
0.0732582796053981));
#72038=CARTESIAN_POINT('Ctrl Pts',(0.00217812639167266,-0.0325844576448134,
0.0733400525122664));
#72039=CARTESIAN_POINT('Ctrl Pts',(0.00216752714140291,-0.0324744968375322,
0.0734220853749587));
#72040=CARTESIAN_POINT('Ctrl Pts',(0.00215863034982285,-0.0323646534831894,
0.073504272900873));
#72041=CARTESIAN_POINT('',(0.00218852477659689,-0.0326773559991149,0.0732709554164597));
#72042=CARTESIAN_POINT('',(0.00219041596997239,-0.0326943950436586,0.0732582796053982));
#72043=CARTESIAN_POINT('Origin',(0.0186218521183369,-0.0326395662072158,
0.0756540325384767));
#72044=CARTESIAN_POINT('Ctrl Pts',(0.00218852477990817,-0.0326773559987408,
0.0732709554169462));
#72045=CARTESIAN_POINT('Ctrl Pts',(0.00223101472548232,-0.0326267922586254,
0.0732772484138444));
#72046=CARTESIAN_POINT('Ctrl Pts',(0.00227275156745392,-0.0325756109579953,
0.0732834298719168));
#72047=CARTESIAN_POINT('Ctrl Pts',(0.00235475456441007,-0.0324719985462359,
0.0732955749711518));
#72048=CARTESIAN_POINT('Ctrl Pts',(0.00239498783015737,-0.0324196091621769,
0.0733015337412356));
#72049=CARTESIAN_POINT('Ctrl Pts',(0.002434483291444,-0.0323666188837756,
0.0733073832383817));
#72050=CARTESIAN_POINT('',(0.00233216072484976,-0.0326943950436699,0.0731663159181133));
#72051=CARTESIAN_POINT('Origin',(0.00812378219310841,-0.0315241814719618,
0.07415));
#72052=CARTESIAN_POINT('',(0.00218852477663969,-0.032711433838005,0.0732709554164661));
#72053=CARTESIAN_POINT('',(0.0021866606600143,-0.0326943950436593,0.0732836352377341));
#72054=CARTESIAN_POINT('Origin',(0.0186277245646419,-0.0326395663828417,
0.0756091043363607));
#72055=CARTESIAN_POINT('Origin',(0.0186071336100769,-0.0326395680916905,
0.0757534299451567));
#72056=CARTESIAN_POINT('Origin',(0.0185997258295675,-0.0326395677069748,
0.0757981315088539));
#72057=CARTESIAN_POINT('Ctrl Pts',(0.002460316931823,-0.0332451089994433,
0.0731483582305965));
#72058=CARTESIAN_POINT('Ctrl Pts',(0.00242253939441707,-0.0329451141710254,
0.0733619593176228));
#72059=CARTESIAN_POINT('Ctrl Pts',(0.00240095848609075,-0.0326442513127493,
0.0735777991450574));
#72060=CARTESIAN_POINT('Ctrl Pts',(0.00242213832423559,-0.0332451089994433,
0.0733954258203826));
#72061=CARTESIAN_POINT('Ctrl Pts',(0.00239367909343392,-0.0329451141710254,
0.0736104668371525));
#72062=CARTESIAN_POINT('Ctrl Pts',(0.00238149848078103,-0.0326442513127493,
0.0738270406106954));
#72063=CARTESIAN_POINT('Ctrl Pts',(0.00242175653815972,-0.0332451089994433,
0.0733978964962804));
#72064=CARTESIAN_POINT('Ctrl Pts',(0.00239339049042408,-0.0329451141710254,
0.0736129519123477));
#72065=CARTESIAN_POINT('Ctrl Pts',(0.00238130388072793,-0.0326442513127493,
0.0738295330253518));
#72066=CARTESIAN_POINT('',(0.00241751373855127,-0.0331951640388616,0.0734312334700842));
#72067=CARTESIAN_POINT('',(0.00239280147173386,-0.0328677532354992,0.0736662799972576));
#72068=CARTESIAN_POINT('Origin',(0.0191286168676268,-0.0326402808281847,
0.0747621277855758));
#72069=CARTESIAN_POINT('Origin',(-0.00862402338789303,-0.0326944278779084,
0.0727367892861736));
#72070=CARTESIAN_POINT('',(0.00240466836925949,-0.0326943950436593,0.0735418371354143));
#72071=CARTESIAN_POINT('',(0.00239941178496456,-0.0326943950436693,0.0736041156896901));
#72072=CARTESIAN_POINT('',(0.00243448329139616,-0.0330220786163545,0.0733073832383717));
#72073=CARTESIAN_POINT('Origin',(0.019119573466244,-0.0326396682762752,
0.0752428260920572));
#72074=CARTESIAN_POINT('',(0.00243582716738045,-0.0331951640388587,0.0733075822738707));
#72075=CARTESIAN_POINT('Origin',(-0.00847678952003185,-0.033195202656004,
0.0716913624358378));
#72076=CARTESIAN_POINT('',(0.00242667045297585,-0.0331951640388701,0.0733694078719874));
#72077=CARTESIAN_POINT('Ctrl Pts',(0.00222754144166722,-0.0330240426238171,
0.0730389891984906));
#72078=CARTESIAN_POINT('Ctrl Pts',(0.00221223618547105,-0.0329142774063519,
0.0731202156592707));
#72079=CARTESIAN_POINT('Ctrl Pts',(0.00219860247688576,-0.0328043479726691,
0.0732017990168026));
#72080=CARTESIAN_POINT('Ctrl Pts',(0.00218666066001426,-0.0326943950436593,
0.0732836352377341));
#72081=CARTESIAN_POINT('Ctrl Pts',(0.00229700570278015,-0.0330240426238171,
0.0731285204914141));
#72082=CARTESIAN_POINT('Ctrl Pts',(0.00228293382737012,-0.0329142774063519,
0.0732087900143216));
#72083=CARTESIAN_POINT('Ctrl Pts',(0.00227051433187736,-0.0328043479726691,
0.0732893904594863));
#72084=CARTESIAN_POINT('Ctrl Pts',(0.00225976597022969,-0.0326943950436593,
0.073370219009902));
#72085=CARTESIAN_POINT('Ctrl Pts',(0.00236646996389308,-0.0330240426238171,
0.0732180517843375));
#72086=CARTESIAN_POINT('Ctrl Pts',(0.00235363146926918,-0.0329142774063519,
0.0732973643693725));
#72087=CARTESIAN_POINT('Ctrl Pts',(0.00234242618686896,-0.0328043479726691,
0.0733769819021701));
#72088=CARTESIAN_POINT('Ctrl Pts',(0.00233287128044513,-0.0326943950436593,
0.0734568027820699));
#72089=CARTESIAN_POINT('Ctrl Pts',(0.00243593422500602,-0.0330240426238171,
0.073307583077261));
#72090=CARTESIAN_POINT('Ctrl Pts',(0.00242432911116825,-0.0329142774063519,
0.0733859387244234));
#72091=CARTESIAN_POINT('Ctrl Pts',(0.00241433804186056,-0.0328043479726691,
0.0734645733448538));
#72092=CARTESIAN_POINT('Ctrl Pts',(0.00240597659066056,-0.0326943950436593,
0.0735433865542377));
#72093=CARTESIAN_POINT('',(0.0022956645146469,-0.0326943950436693,0.0734127361865842));
#72094=CARTESIAN_POINT('Ctrl Pts',(0.0021885247799137,-0.0327114338383321,
0.0732709554169469));
#72095=CARTESIAN_POINT('Ctrl Pts',(0.00223100765805619,-0.0327619876831129,
0.0732772473671192));
#72096=CARTESIAN_POINT('Ctrl Pts',(0.00227274104798354,-0.0328131562604663,
0.0732834283139248));
#72097=CARTESIAN_POINT('Ctrl Pts',(0.00235474396955514,-0.0329167375858764,
0.0732955734019949));
#72098=CARTESIAN_POINT('Ctrl Pts',(0.00239498082705073,-0.0329691088920619,
0.0733015327040366));
#72099=CARTESIAN_POINT('Ctrl Pts',(0.0024344832914428,-0.0330220786163187,
0.0733073832383814));
#72100=CARTESIAN_POINT('Ctrl Pts',(0.00241914241450137,-0.0331951640388604,
0.0734300249923475));
#72101=CARTESIAN_POINT('Ctrl Pts',(0.00240425739282318,-0.0330306422010619,
0.0735479647622954));
#72102=CARTESIAN_POINT('Ctrl Pts',(0.00239425966501202,-0.0328657861914644,
0.0736664189671357));
#72103=CARTESIAN_POINT('Ctrl Pts',(0.00241751373855174,-0.0331951640388604,
0.0734312334700811));
#72104=CARTESIAN_POINT('Ctrl Pts',(0.00240265370137588,-0.0330306422010619,
0.0735492069118601));
#72105=CARTESIAN_POINT('Ctrl Pts',(0.00239268232841017,-0.0328657861914644,
0.0736676937271233));
#72106=CARTESIAN_POINT('Ctrl Pts',(0.0021461325260133,-0.0331951640388604,
0.0736325983596107));
#72107=CARTESIAN_POINT('Ctrl Pts',(0.00213543557882531,-0.0330306422010619,
0.0737561824339654));
#72108=CARTESIAN_POINT('Ctrl Pts',(0.00212985563186088,-0.0328657861914644,
0.0738801030226711));
#72109=CARTESIAN_POINT('',(0.00214504098399125,-0.0331781648281896,0.0736453679061157));
#72110=CARTESIAN_POINT('',(0.00214613252601325,-0.033195164038858,0.0736325983596112));
#72111=CARTESIAN_POINT('Origin',(0.0186534028072523,-0.0326412086709817,
0.0743239466882793));
#72112=CARTESIAN_POINT('Ctrl Pts',(0.00214504098516957,-0.033178164828644,
0.0736453679047027));
#72113=CARTESIAN_POINT('Ctrl Pts',(0.00218787169502291,-0.0331276811546784,
0.0736489829931305));
#72114=CARTESIAN_POINT('Ctrl Pts',(0.00222992901774062,-0.0330765663497797,
0.0736525327705596));
#72115=CARTESIAN_POINT('Ctrl Pts',(0.00231253300989468,-0.0329730614463142,
0.0736595049148786));
#72116=CARTESIAN_POINT('Ctrl Pts',(0.00235304630866117,-0.0329207133373816,
0.0736629244705147));
#72117=CARTESIAN_POINT('Ctrl Pts',(0.00239280146422714,-0.0328677532289352,
0.0736662799825947));
#72118=CARTESIAN_POINT('',(0.00228182313229225,-0.0331951640388698,0.0735319159148577));
#72119=CARTESIAN_POINT('Origin',(0.00812378219310841,-0.0315241814719618,
0.07415));
#72120=CARTESIAN_POINT('',(0.00214504098548132,-0.0332121607144223,0.0736453679068907));
#72121=CARTESIAN_POINT('',(0.00214397671962883,-0.0331951640388587,0.0736581397562618));
#72122=CARTESIAN_POINT('Origin',(0.018649346519188,-0.0326413645333489,
0.0742787828462342));
#72123=CARTESIAN_POINT('Origin',(0.018533594970632,-0.0326412101255305,
0.0757434317878519));
#72124=CARTESIAN_POINT('Origin',(0.018522020263712,-0.0326413657463797,
0.0757872766267247));
#72125=CARTESIAN_POINT('Ctrl Pts',(0.00240860121255209,-0.0337436976235975,
0.0735059259673862));
#72126=CARTESIAN_POINT('Ctrl Pts',(0.00240280831309068,-0.0336723290703325,
0.0735573291712847));
#72127=CARTESIAN_POINT('Ctrl Pts',(0.00239794093240255,-0.033601104548885,
0.0736088282553585));
#72128=CARTESIAN_POINT('Ctrl Pts',(0.00238240035003915,-0.0333736987606856,
0.0737732546294123));
#72129=CARTESIAN_POINT('Ctrl Pts',(0.00237632111074342,-0.0331450831799191,
0.073938301850032));
#72130=CARTESIAN_POINT('Ctrl Pts',(0.00238601054224536,-0.0337436976235975,
0.0737549031985041));
#72131=CARTESIAN_POINT('Ctrl Pts',(0.00238245698173415,-0.0336723290703325,
0.073806509586315));
#72132=CARTESIAN_POINT('Ctrl Pts',(0.00237983223236211,-0.033601104548885,
0.0738581715427814));
#72133=CARTESIAN_POINT('Ctrl Pts',(0.00237145192755075,-0.0333736987606856,
0.0740231179361216));
#72134=CARTESIAN_POINT('Ctrl Pts',(0.00237255100794119,-0.0331450831799191,
0.0741882734210653));
#72135=CARTESIAN_POINT('Ctrl Pts',(0.00238578463554229,-0.0337436976235975,
0.0737573929708152));
#72136=CARTESIAN_POINT('Ctrl Pts',(0.00238225346842058,-0.0336723290703325,
0.0738090013904653));
#72137=CARTESIAN_POINT('Ctrl Pts',(0.0023796511453617,-0.033601104548885,
0.0738606649756556));
#72138=CARTESIAN_POINT('Ctrl Pts',(0.00237134244332586,-0.0333736987606856,
0.0740256165691887));
#72139=CARTESIAN_POINT('Ctrl Pts',(0.00237251330691316,-0.0331450831799191,
0.0741907731367756));
#72140=CARTESIAN_POINT('',(0.00238364203203872,-0.0336938721132548,0.0737909513524937));
#72141=CARTESIAN_POINT('',(0.00237373722885253,-0.0333679870047995,0.0740270857660023));
#72142=CARTESIAN_POINT('Ctrl Pts',(0.00238364203203947,-0.0336938721132476,
0.0737909513524793));
#72143=CARTESIAN_POINT('Ctrl Pts',(0.00238224049673511,-0.0336629187933822,
0.0738133578122843));
#72144=CARTESIAN_POINT('Ctrl Pts',(0.00238097060850649,-0.033631995230096,
0.0738357653125182));
#72145=CARTESIAN_POINT('Ctrl Pts',(0.00237983223236218,-0.0336011045488869,
0.07385817154278));
#72146=CARTESIAN_POINT('Ctrl Pts',(0.00237697565708572,-0.033523589259537,
0.0739143964414873));
#72147=CARTESIAN_POINT('Ctrl Pts',(0.00237494226013591,-0.033445866866549,
0.0739707132557272));
#72148=CARTESIAN_POINT('Ctrl Pts',(0.0023737372288467,-0.0333679869962413,
0.0740270857541789));
#72149=CARTESIAN_POINT('Ctrl Pts',(0.002373735591128,-0.0333679692470414,
0.0740271302038922));
#72150=CARTESIAN_POINT('Ctrl Pts',(0.00237418882798317,-0.033339189541522,
0.0740271339635706));
#72151=CARTESIAN_POINT('Ctrl Pts',(0.0023745285780814,-0.0333104081130171,
0.0740271335345558));
#72152=CARTESIAN_POINT('Ctrl Pts',(0.00237497828857451,-0.0332532698153858,
0.0740271274282393));
#72153=CARTESIAN_POINT('Ctrl Pts',(0.00237509160253743,-0.0332249170742957,
0.0740271218262043));
#72154=CARTESIAN_POINT('Ctrl Pts',(0.00237509541952204,-0.0331960985387042,
0.0740271150074511));
#72155=CARTESIAN_POINT('Ctrl Pts',(0.00237509545166307,-0.0331956312537763,
0.0740271148962221));
#72156=CARTESIAN_POINT('Ctrl Pts',(0.00237509545404053,-0.0331951640388589,
0.0740271147850021));
#72157=CARTESIAN_POINT('',(0.00237776687175779,-0.0331951640388587,0.0739021433341527));
#72158=CARTESIAN_POINT('',(0.00237643116290913,-0.0331951640388687,0.0739646290595873));
#72159=CARTESIAN_POINT('',(0.00239280147937305,-0.0335216366567733,0.073666279983748));
#72160=CARTESIAN_POINT('Origin',(0.0190461624799162,-0.032643457152522,
0.0738566281064757));
#72161=CARTESIAN_POINT('',(0.00239415520064963,-0.0336938721132326,0.073666394243946));
#72162=CARTESIAN_POINT('Origin',(-0.008487720796425,-0.0336938867896233,
0.0727479146722203));
#72163=CARTESIAN_POINT('',(0.00238889861635418,-0.0336938721132537,0.0737286727982298));
#72164=CARTESIAN_POINT('Ctrl Pts',(0.00216941526218682,-0.0335235895815171,
0.0734114104983307));
#72165=CARTESIAN_POINT('Ctrl Pts',(0.00215924712354743,-0.0334144449262748,
0.0734933840822045));
#72166=CARTESIAN_POINT('Ctrl Pts',(0.00215076081549949,-0.0333049234473147,
0.0735756619098868));
#72167=CARTESIAN_POINT('Ctrl Pts',(0.00214397671962867,-0.0331951640388587,
0.0736581397562617));
#72168=CARTESIAN_POINT('Ctrl Pts',(0.00224436428798135,-0.0335235895815171,
0.0734964035334477));
#72169=CARTESIAN_POINT('Ctrl Pts',(0.00223536624580623,-0.0334144449262748,
0.0735773452964204));
#72170=CARTESIAN_POINT('Ctrl Pts',(0.00222803006187835,-0.0333049234473147,
0.073658565944452));
#72171=CARTESIAN_POINT('Ctrl Pts',(0.00222237452467511,-0.0331951640388587,
0.0737399624710165));
#72172=CARTESIAN_POINT('Ctrl Pts',(0.00231931331377588,-0.0335235895815171,
0.0735813965685646));
#72173=CARTESIAN_POINT('Ctrl Pts',(0.00231148536806503,-0.0334144449262748,
0.0736613065106362));
#72174=CARTESIAN_POINT('Ctrl Pts',(0.00230529930825722,-0.0333049234473147,
0.0737414699790171));
#72175=CARTESIAN_POINT('Ctrl Pts',(0.00230077232972155,-0.0331951640388587,
0.0738217851857713));
#72176=CARTESIAN_POINT('Ctrl Pts',(0.00239426233957041,-0.0335235895815171,
0.0736663896036816));
#72177=CARTESIAN_POINT('Ctrl Pts',(0.00238760449032383,-0.0334144449262748,
0.0737452677248521));
#72178=CARTESIAN_POINT('Ctrl Pts',(0.00238256855463608,-0.0333049234473147,
0.0738243740135823));
#72179=CARTESIAN_POINT('Ctrl Pts',(0.00237917013476799,-0.0331951640388587,
0.0739036079005261));
#72180=CARTESIAN_POINT('',(0.00226087179570331,-0.0331951640388687,0.0737801415452172));
#72181=CARTESIAN_POINT('Ctrl Pts',(0.00214504098859704,-0.0332121607145974,
0.0736453679071492));
#72182=CARTESIAN_POINT('Ctrl Pts',(0.00218779964525095,-0.0332625444109927,
0.0736489769261144));
#72183=CARTESIAN_POINT('Ctrl Pts',(0.00222982150315124,-0.0333135300747189,
0.0736525237560192));
#72184=CARTESIAN_POINT('Ctrl Pts',(0.00231242497779767,-0.0334167203140631,
0.0736594958531316));
#72185=CARTESIAN_POINT('Ctrl Pts',(0.00235297460157892,-0.0334688847587333,
0.0736629184199919));
#72186=CARTESIAN_POINT('Ctrl Pts',(0.00239280148005874,-0.0335216366562418,
0.0736662799839652));
#72187=CARTESIAN_POINT('Ctrl Pts',(0.00238519125082585,-0.0336938721132474,
0.0737896432999643));
#72188=CARTESIAN_POINT('Ctrl Pts',(0.00238308196348132,-0.0336474569765,
0.0738232331770189));
#72189=CARTESIAN_POINT('Ctrl Pts',(0.00238136603258792,-0.033601104548885,
0.0738568454443452));
#72190=CARTESIAN_POINT('Ctrl Pts',(0.00237702169008348,-0.0334837508592655,
0.0739419439772629));
#72191=CARTESIAN_POINT('Ctrl Pts',(0.00237520090126284,-0.0333660264659097,
0.0740271338730523));
#72192=CARTESIAN_POINT('Ctrl Pts',(0.00238364203204049,-0.0336938721132474,
0.0737909513524672));
#72193=CARTESIAN_POINT('Ctrl Pts',(0.00238154040116131,-0.0336474569765,
0.0738245502976135));
#72194=CARTESIAN_POINT('Ctrl Pts',(0.00237983223236211,-0.033601104548885,
0.0738581715427814));
#72195=CARTESIAN_POINT('Ctrl Pts',(0.00237550754169554,-0.0334837508592655,
0.0739432928055301));
#72196=CARTESIAN_POINT('Ctrl Pts',(0.00237370706961516,-0.0333660264659097,
0.0740285048388446));
#72197=CARTESIAN_POINT('Ctrl Pts',(0.00212389092293176,-0.0336938721132474,
0.0740102671080028));
#72198=CARTESIAN_POINT('Ctrl Pts',(0.00212307301994653,-0.0336474569765,
0.0740453864625853));
#72199=CARTESIAN_POINT('Ctrl Pts',(0.00212266628939154,-0.033601104548885,
0.0740805129853544));
#72200=CARTESIAN_POINT('Ctrl Pts',(0.00212163654113961,-0.0334837508592655,
0.0741694452649036));
#72201=CARTESIAN_POINT('Ctrl Pts',(0.00212324249290732,-0.0333660264659097,
0.0742583690055255));
#72202=CARTESIAN_POINT('',(0.00212515255234191,-0.0336769361243753,0.0740217719495674));
#72203=CARTESIAN_POINT('',(0.00212544013436168,-0.0336938721132327,0.0740089590617211));
#72204=CARTESIAN_POINT('Ctrl Pts',(0.00212515255234192,-0.033676936124375,
0.0740217719495677));
#72205=CARTESIAN_POINT('Ctrl Pts',(0.00212519820538143,-0.033679758667006,
0.0740196362571424));
#72206=CARTESIAN_POINT('Ctrl Pts',(0.00212524499724999,-0.0336825812712915,
0.0740175006698712));
#72207=CARTESIAN_POINT('Ctrl Pts',(0.00212534085811385,-0.0336882266020684,
0.0740132297064027));
#72208=CARTESIAN_POINT('Ctrl Pts',(0.00212538992711016,-0.0336910493285604,
0.0740110943302047));
#72209=CARTESIAN_POINT('Ctrl Pts',(0.00212544013436201,-0.0336938721132326,
0.074008959061721));
#72210=CARTESIAN_POINT('Ctrl Pts',(0.00212515255234196,-0.0336769361243753,
0.0740217719495674));
#72211=CARTESIAN_POINT('Ctrl Pts',(0.00216705673264463,-0.0336279007536338,
0.0740226677027089));
#72212=CARTESIAN_POINT('Ctrl Pts',(0.00220955756321641,-0.0335767878672832,
0.0740235762099796));
#72213=CARTESIAN_POINT('Ctrl Pts',(0.00229284726020332,-0.0334733198899511,
0.0740253566291929));
#72214=CARTESIAN_POINT('Ctrl Pts',(0.0023336857126357,-0.0334209645035433,
0.0740262296010973));
#72215=CARTESIAN_POINT('Ctrl Pts',(0.00237373722915698,-0.0333679869844681,
0.0740270857512829));
#72216=CARTESIAN_POINT('',(0.0022545410832102,-0.0336938721132538,0.0738999552071174));
#72217=CARTESIAN_POINT('Origin',(0.00812378219310841,-0.0315241814719618,
0.07415));
#72218=CARTESIAN_POINT('',(0.00212515255364349,-0.0337108120655397,0.0740217719496001));
#72219=CARTESIAN_POINT('',(0.00212489233953393,-0.0336938721132327,0.074034585422462));
#72220=CARTESIAN_POINT('Origin',(0.0184587460170713,-0.0345562512088088,
0.0754887825082202));
#72221=CARTESIAN_POINT('Ctrl Pts',(0.00212489233954153,-0.0336938721132294,
0.0740345854224665));
#72222=CARTESIAN_POINT('Ctrl Pts',(0.00212493342423983,-0.0336910493404263,
0.0740324499679598));
#72223=CARTESIAN_POINT('Ctrl Pts',(0.00212497565100609,-0.0336882266080013,
0.0740303144410065));
#72224=CARTESIAN_POINT('Ctrl Pts',(0.00212506238854535,-0.0336825812712813,
0.0740260432780174));
#72225=CARTESIAN_POINT('Ctrl Pts',(0.0021251068993025,-0.0336797586670009,
0.0740239076419885));
#72226=CARTESIAN_POINT('Ctrl Pts',(0.00212515255234193,-0.033676936124375,
0.0740217719495671));
#72227=CARTESIAN_POINT('Origin',(0.0185065124361043,-0.0345562516912807,
0.0732540829213579));
#72228=CARTESIAN_POINT('Ctrl Pts',(0.00237943962316015,-0.034243627687391,
0.073866004508697));
#72229=CARTESIAN_POINT('Ctrl Pts',(0.00236872855663149,-0.0339430054201809,
0.074082655960267));
#72230=CARTESIAN_POINT('Ctrl Pts',(0.00237436699415386,-0.0336441434784051,
0.074299498729194));
#72231=CARTESIAN_POINT('Ctrl Pts',(0.00237252469634862,-0.034243627687391,
0.0741159088579732));
#72232=CARTESIAN_POINT('Ctrl Pts',(0.00237123892773092,-0.0339430054201809,
0.0743328211103074));
#72233=CARTESIAN_POINT('Ctrl Pts',(0.00238629553146314,-0.0336441434784051,
0.0745492139870331));
#72234=CARTESIAN_POINT('Ctrl Pts',(0.00237245554708051,-0.034243627687391,
0.0741184079014659));
#72235=CARTESIAN_POINT('Ctrl Pts',(0.00237126403144192,-0.0339430054201809,
0.0743353227618078));
#72236=CARTESIAN_POINT('Ctrl Pts',(0.00238641481683623,-0.0336441434784051,
0.0745517111396116));
#72237=CARTESIAN_POINT('',(0.00237242403632307,-0.0341934961088741,0.0741520862358514));
#72238=CARTESIAN_POINT('',(0.0023773657793568,-0.0338664212891033,0.0743883766089048));
#72239=CARTESIAN_POINT('Origin',(0.0190996333364463,-0.0345610818075015,
0.0746556369668814));
#72240=CARTESIAN_POINT('Origin',(-0.00857946260158768,-0.0336938005044531,
0.0748429706856536));
#72241=CARTESIAN_POINT('',(0.00237354227162478,-0.0336938721132327,0.0742634277099163));
#72242=CARTESIAN_POINT('',(0.00237613270965501,-0.0336938721132426,0.0743258740038986));
#72243=CARTESIAN_POINT('',(0.00237373722915707,-0.0340203938281605,0.0740270857512775));
#72244=CARTESIAN_POINT('Origin',(0.0190111828180154,-0.0345589643243929,
0.0751286064196521));
#72245=CARTESIAN_POINT('',(0.00237509545404047,-0.0341934961088739,0.074027114785002));
#72246=CARTESIAN_POINT('Origin',(-0.00864183503513343,-0.0341934220717644,
0.0737916134911796));
#72247=CARTESIAN_POINT('',(0.00237375974519177,-0.034193496108884,0.0740896005104367));
#72248=CARTESIAN_POINT('Ctrl Pts',(0.00213478859230788,-0.0340223579322396,
0.0737867429978597));
#72249=CARTESIAN_POINT('Ctrl Pts',(0.00212977833083434,-0.0339125849573575,
0.0738693468395658));
#72250=CARTESIAN_POINT('Ctrl Pts',(0.00212648129759202,-0.0338030433565231,
0.073951996337279));
#72251=CARTESIAN_POINT('Ctrl Pts',(0.0021248923395334,-0.0336938721132327,
0.0740345854224616));
#72252=CARTESIAN_POINT('Ctrl Pts',(0.00221492646653166,-0.0340223579322397,
0.0738668622898264));
#72253=CARTESIAN_POINT('Ctrl Pts',(0.00221102125905422,-0.0339125849573575,
0.0739483608212386));
#72254=CARTESIAN_POINT('Ctrl Pts',(0.00220880562594467,-0.0338030433565231,
0.0740298829132967));
#72255=CARTESIAN_POINT('Ctrl Pts',(0.00220827315903309,-0.0336938721132327,
0.0741113240618156));
#72256=CARTESIAN_POINT('Ctrl Pts',(0.00229506434075544,-0.0340223579322397,
0.0739469815817931));
#72257=CARTESIAN_POINT('Ctrl Pts',(0.00229226418727411,-0.0339125849573575,
0.0740273748029114));
#72258=CARTESIAN_POINT('Ctrl Pts',(0.00229112995429731,-0.0338030433565231,
0.0741077694893144));
#72259=CARTESIAN_POINT('Ctrl Pts',(0.00229165397853278,-0.0336938721132327,
0.0741880627011696));
#72260=CARTESIAN_POINT('Ctrl Pts',(0.00237520221497922,-0.0340223579322397,
0.0740271008737598));
#72261=CARTESIAN_POINT('Ctrl Pts',(0.00237350711549399,-0.0339125849573575,
0.0741063887845841));
#72262=CARTESIAN_POINT('Ctrl Pts',(0.00237345428264996,-0.0338030433565231,
0.0741856560653321));
#72263=CARTESIAN_POINT('Ctrl Pts',(0.00237503479803247,-0.0336938721132327,
0.0742648013405236));
#72264=CARTESIAN_POINT('',(0.00224921730558935,-0.0336938721132427,0.0741490065661992));
#72265=CARTESIAN_POINT('Ctrl Pts',(0.00212515255724037,-0.0337108120662684,
0.074021771949672));
#72266=CARTESIAN_POINT('Ctrl Pts',(0.00216814199267721,-0.0337611408994435,
0.0740226909014702));
#72267=CARTESIAN_POINT('Ctrl Pts',(0.0022103469662926,-0.0338121088781604,
0.0740235930844369));
#72268=CARTESIAN_POINT('Ctrl Pts',(0.00229322643789414,-0.0339153382773233,
0.0740253647345805));
#72269=CARTESIAN_POINT('Ctrl Pts',(0.00233386587282454,-0.0339675558473115,
0.0740262334522417));
#72270=CARTESIAN_POINT('Ctrl Pts',(0.0023737372291968,-0.0340203938281304,
0.0740270857512837));
#72271=CARTESIAN_POINT('Ctrl Pts',(0.00237388847297717,-0.0341934961088741,
0.0741506830971307));
#72272=CARTESIAN_POINT('Ctrl Pts',(0.00237390259547209,-0.03402875161944,
0.074269557619096));
#72273=CARTESIAN_POINT('Ctrl Pts',(0.0023788298800418,-0.0338644633299819,
0.074388329981364));
#72274=CARTESIAN_POINT('Ctrl Pts',(0.00237242403632317,-0.0341934961088741,
0.0741520862358513));
#72275=CARTESIAN_POINT('Ctrl Pts',(0.00237246716760552,-0.03402875161944,
0.0742709910338906));
#72276=CARTESIAN_POINT('Ctrl Pts',(0.0023774246875083,-0.0338644633299819,
0.074389792447407));
#72277=CARTESIAN_POINT('Ctrl Pts',(0.00212842045843375,-0.0341934961088741,
0.0743858763879789));
#72278=CARTESIAN_POINT('Ctrl Pts',(0.00213329701689356,-0.03402875161944,
0.0745098257677254));
#72279=CARTESIAN_POINT('Ctrl Pts',(0.00214329233029034,-0.0338644633299819,
0.0746334676832399));
#72280=CARTESIAN_POINT('',(0.00212893797252645,-0.0341764758832388,0.0743986820490732));
#72281=CARTESIAN_POINT('',(0.00212842045843431,-0.034193496108874,0.0743858763879783));
#72282=CARTESIAN_POINT('Origin',(0.0186936848809415,-0.034562102674501,
0.0742240717872174));
#72283=CARTESIAN_POINT('Ctrl Pts',(0.00212893797332019,-0.0341764758837474,
0.0743986820474324));
#72284=CARTESIAN_POINT('Ctrl Pts',(0.00217182546541595,-0.0341260050043394,
0.0743969029466841));
#72285=CARTESIAN_POINT('Ctrl Pts',(0.00221396747014351,-0.0340749269154166,
0.0743951547327292));
#72286=CARTESIAN_POINT('Ctrl Pts',(0.00229679317293366,-0.0339715436318644,
0.074391718906788));
#72287=CARTESIAN_POINT('Ctrl Pts',(0.00233744544902731,-0.033919277825295,
0.0743900326042564));
#72288=CARTESIAN_POINT('Ctrl Pts',(0.00237736577692892,-0.0338664212873869,
0.0743883766051632));
#72289=CARTESIAN_POINT('',(0.00225042224738869,-0.0341934961088841,0.0742689813119249));
#72290=CARTESIAN_POINT('Origin',(0.00812378219310841,-0.0315241814719618,
0.07415));
#72291=CARTESIAN_POINT('',(0.00212893797329664,-0.0342105180190537,0.0743986820498836));
#72292=CARTESIAN_POINT('',(0.00212948283705898,-0.0341934961088739,0.0744114865772719));
#72293=CARTESIAN_POINT('Origin',(0.0186970490369613,-0.034562170373609,
0.0741788690574407));
#72294=CARTESIAN_POINT('Origin',(0.0186512375102797,-0.0345621039704051,
0.0732007520833079));
#72295=CARTESIAN_POINT('Origin',(0.0186583280135043,-0.0345621716132366,
0.0732455212001824));
#72296=CARTESIAN_POINT('Ctrl Pts',(0.00237348010070173,-0.0346945769586966,
0.0742619289889591));
#72297=CARTESIAN_POINT('Ctrl Pts',(0.0023758244981894,-0.0345275153362944,
0.0743823713685799));
#72298=CARTESIAN_POINT('Ctrl Pts',(0.00238195730403783,-0.0343603235965185,
0.0745027711716261));
#72299=CARTESIAN_POINT('Ctrl Pts',(0.00239185508771714,-0.034193496108874,
0.0746227725785056));
#72300=CARTESIAN_POINT('Ctrl Pts',(0.00237695474171148,-0.0346945769586966,
0.0743456902881114));
#72301=CARTESIAN_POINT('Ctrl Pts',(0.00238105355314609,-0.0345275153362944,
0.0744660598899851));
#72302=CARTESIAN_POINT('Ctrl Pts',(0.0023889389379296,-0.0343603235965185,
0.0745863317217564));
#72303=CARTESIAN_POINT('Ctrl Pts',(0.00240058228780687,-0.034193496108874,
0.0747061504193534));
#72304=CARTESIAN_POINT('Ctrl Pts',(0.00238042938272128,-0.0346945769586966,
0.074429451587263));
#72305=CARTESIAN_POINT('Ctrl Pts',(0.00238628260810281,-0.0345275153362944,
0.0745497484113905));
#72306=CARTESIAN_POINT('Ctrl Pts',(0.0023959205718214,-0.0343603235965185,
0.0746698922718872));
#72307=CARTESIAN_POINT('Ctrl Pts',(0.00240930948789662,-0.034193496108874,
0.0747895282602017));
#72308=CARTESIAN_POINT('Ctrl Pts',(0.00238390402373097,-0.0346945769586966,
0.0745132128864162));
#72309=CARTESIAN_POINT('Ctrl Pts',(0.00239151166305946,-0.0345275153362944,
0.0746334369327957));
#72310=CARTESIAN_POINT('Ctrl Pts',(0.00240290220571316,-0.0343603235965185,
0.074753452822017));
#72311=CARTESIAN_POINT('Ctrl Pts',(0.00241803668798633,-0.034193496108874,
0.0748729061010489));
#72312=CARTESIAN_POINT('',(0.00238390402370603,-0.0346945769586966,0.0745132128858109));
#72313=CARTESIAN_POINT('',(0.00240367281090493,-0.0343667727831449,0.074748726695533));
#72314=CARTESIAN_POINT('Origin',(0.0191513968172488,-0.0345626457061575,
0.0732688525457317));
#72315=CARTESIAN_POINT('Origin',(-0.00858845504753611,-0.0341934771029168,
0.0758992828933265));
#72316=CARTESIAN_POINT('',(0.00239201124142713,-0.034193496108874,0.074624264438329));
#72317=CARTESIAN_POINT('',(0.00239851760306086,-0.0341934961088839,0.0746864248538655));
#72318=CARTESIAN_POINT('',(0.00237736577990387,-0.0345211942962703,0.0743883766050832));
#72319=CARTESIAN_POINT('Origin',(0.0191680034977935,-0.0345625596118732,
0.0737493887132169));
#72320=CARTESIAN_POINT('',(0.00237872314766526,-0.0346945769586885,0.0743883202978607));
#72321=CARTESIAN_POINT('Origin',(-0.00867533702907217,-0.0346945685853894,
0.0748468710747448));
#72322=CARTESIAN_POINT('',(0.00238131358569564,-0.0346945769587026,0.0744507665918459));
#72323=CARTESIAN_POINT('Ctrl Pts',(0.00212379740940387,-0.0345231616327842,
0.0741635127844013));
#72324=CARTESIAN_POINT('Ctrl Pts',(0.00212398366411236,-0.0344132092796988,
0.0742462141273418));
#72325=CARTESIAN_POINT('Ctrl Pts',(0.00212588052125579,-0.0343032738558979,
0.0743289073507414));
#72326=CARTESIAN_POINT('Ctrl Pts',(0.00212948283705895,-0.0341934961088739,
0.0744114865772719));
#72327=CARTESIAN_POINT('Ctrl Pts',(0.00220880774919815,-0.0345231616327842,
0.0742384419393851));
#72328=CARTESIAN_POINT('Ctrl Pts',(0.00221002679681628,-0.0344132092796988,
0.0743199715344765));
#72329=CARTESIAN_POINT('Ctrl Pts',(0.00221293215690198,-0.0343032738558979,
0.0744014717079772));
#72330=CARTESIAN_POINT('Ctrl Pts',(0.00221751743282267,-0.0341934961088739,
0.0744828381440889));
#72331=CARTESIAN_POINT('Ctrl Pts',(0.00229381808899242,-0.0345231616327842,
0.0743133710943689));
#72332=CARTESIAN_POINT('Ctrl Pts',(0.00229606992952019,-0.0344132092796988,
0.0743937289416112));
#72333=CARTESIAN_POINT('Ctrl Pts',(0.00229998379254817,-0.0343032738558979,
0.0744740360652129));
#72334=CARTESIAN_POINT('Ctrl Pts',(0.00230555202858638,-0.0341934961088739,
0.074554189710906));
#72335=CARTESIAN_POINT('Ctrl Pts',(0.00237882842878669,-0.0345231616327842,
0.0743883002493527));
#72336=CARTESIAN_POINT('Ctrl Pts',(0.00238211306222411,-0.0344132092796988,
0.0744674863487459));
#72337=CARTESIAN_POINT('Ctrl Pts',(0.00238703542819436,-0.0343032738558979,
0.0745466004224487));
#72338=CARTESIAN_POINT('Ctrl Pts',(0.00239358662435009,-0.0341934961088739,
0.074625541277723));
#72339=CARTESIAN_POINT('',(0.00226074703925305,-0.0341934961088839,0.0745178755078104));
#72340=CARTESIAN_POINT('Ctrl Pts',(0.00212893797674334,-0.0342105180195387,
0.0743986820497355));
#72341=CARTESIAN_POINT('Ctrl Pts',(0.00217187368354173,-0.0342610556241366,
0.0743969009626567));
#72342=CARTESIAN_POINT('Ctrl Pts',(0.00221403893128144,-0.0343122189870292,
0.0743951518362646));
#72343=CARTESIAN_POINT('Ctrl Pts',(0.00229686546984916,-0.0344158119695183,
0.0743917159716049));
#72344=CARTESIAN_POINT('Ctrl Pts',(0.00233749288403387,-0.0344681990450091,
0.0743900306386304));
#72345=CARTESIAN_POINT('Ctrl Pts',(0.00237736577992857,-0.0345211942962515,
0.0743883766050772));
#72346=CARTESIAN_POINT('Ctrl Pts',(0.00238527713202041,-0.0346945769586933,
0.0745117209268942));
#72347=CARTESIAN_POINT('Ctrl Pts',(0.00239275545623842,-0.034529677707698,
0.0746303604585962));
#72348=CARTESIAN_POINT('Ctrl Pts',(0.00240513087118744,-0.0343648066251421,
0.074748589528289));
#72349=CARTESIAN_POINT('Ctrl Pts',(0.00238390402370555,-0.0346945769586933,
0.0745132128858019));
#72350=CARTESIAN_POINT('Ctrl Pts',(0.00239141319311831,-0.034529677707698,
0.0746318808055468));
#72351=CARTESIAN_POINT('Ctrl Pts',(0.00240382060020912,-0.0343648066251421,
0.074750136964165));
#72352=CARTESIAN_POINT('Ctrl Pts',(0.00215506173625195,-0.0346945769586933,
0.0747618628178917));
#72353=CARTESIAN_POINT('Ctrl Pts',(0.00216771156707162,-0.034529677707698,
0.0748852618900061));
#72354=CARTESIAN_POINT('Ctrl Pts',(0.00218545078581339,-0.0343648066251421,
0.0750080326900234));
#72355=CARTESIAN_POINT('',(0.00215638230304205,-0.0346775396664975,0.0747746107150898));
#72356=CARTESIAN_POINT('',(0.00215506173625342,-0.0346945769586887,0.0747618628178938));
#72357=CARTESIAN_POINT('Origin',(0.0186511766211248,-0.0345626618038484,
0.0728945410564125));
#72358=CARTESIAN_POINT('Ctrl Pts',(0.00215638230382469,-0.0346775396670097,
0.0747746107134425));
#72359=CARTESIAN_POINT('Ctrl Pts',(0.00219910707997535,-0.0346269749928188,
0.0747701386769084));
#72360=CARTESIAN_POINT('Ctrl Pts',(0.00224107253777998,-0.0345757902890782,
0.0747657460827174));
#72361=CARTESIAN_POINT('Ctrl Pts',(0.0023235193956571,-0.0344721681088003,
0.0747571163328799));
#72362=CARTESIAN_POINT('Ctrl Pts',(0.00236396847327309,-0.0344197714289742,
0.0747528825661073));
#72363=CARTESIAN_POINT('Ctrl Pts',(0.00240367281076893,-0.0343667727830615,
0.0747487266952973));
#72364=CARTESIAN_POINT('',(0.00226948287998973,-0.0346945769587026,0.0746375378518624));
#72365=CARTESIAN_POINT('Origin',(0.00812378219310841,-0.0315241814719618,
0.07415));
#72366=CARTESIAN_POINT('',(0.00215638230429078,-0.0347116136489792,0.0747746107157019));
#72367=CARTESIAN_POINT('',(0.00215773009560744,-0.0346945769586885,0.074787355764023));
#72368=CARTESIAN_POINT('Origin',(0.018644606527977,-0.0345626681934436,
0.0728497064115708));
#72369=CARTESIAN_POINT('Origin',(0.0186829756296675,-0.0345626630859793,
0.0731983135855367));
#72370=CARTESIAN_POINT('Origin',(0.0186858261559396,-0.0345626693552011,
0.0732435377202918));
#72371=CARTESIAN_POINT('Ctrl Pts',(0.00238890029881963,-0.0352450361874068,
0.0745857663183217));
#72372=CARTESIAN_POINT('Ctrl Pts',(0.00240533549520417,-0.0349452760959493,
0.0748020609381946));
#72373=CARTESIAN_POINT('Ctrl Pts',(0.00243801619670002,-0.0346444289841739,
0.0750165031215818));
#72374=CARTESIAN_POINT('Ctrl Pts',(0.0023891473884064,-0.0352450361874068,
0.074588279199484));
#72375=CARTESIAN_POINT('Ctrl Pts',(0.00240567735965917,-0.0349452760959493,
0.0748045645002203));
#72376=CARTESIAN_POINT('Ctrl Pts',(0.00243845186482231,-0.0346444289841739,
0.0750189902521146));
#72377=CARTESIAN_POINT('Ctrl Pts',(0.00241361170392928,-0.0352450361874068,
0.0748370793145684));
#72378=CARTESIAN_POINT('Ctrl Pts',(0.00243952532550101,-0.0349452760959493,
0.075052441928504));
#72379=CARTESIAN_POINT('Ctrl Pts',(0.00248158732247518,-0.0346444289841739,
0.0752652407999173));
#72380=CARTESIAN_POINT('Ctrl Pts',(0.00241385634708451,-0.0352450361874068,
0.0748395673157192));
#72381=CARTESIAN_POINT('Ctrl Pts',(0.00243986380515942,-0.0349452760959493,
0.075054920702787));
#72382=CARTESIAN_POINT('Ctrl Pts',(0.00248201867705171,-0.0346444289841739,
0.0752677033053952));
#72383=CARTESIAN_POINT('',(0.00241803026600223,-0.0351951634053262,0.0748728742967211));
#72384=CARTESIAN_POINT('',(0.00245255450039629,-0.0348678972925388,0.0751067138848245));
#72385=CARTESIAN_POINT('Origin',(0.0188981264262113,-0.0345636767886491,
0.0719045537410315));
#72386=CARTESIAN_POINT('Origin',(-0.0084433345167475,-0.0346946199341098,
0.076944808478318));
#72387=CARTESIAN_POINT('',(0.00243310089014555,-0.0346945769330288,0.0749832294438517));
#72388=CARTESIAN_POINT('',(0.00244349749883294,-0.0346945769458128,0.07504485867081));
#72389=CARTESIAN_POINT('',(0.00240367281090796,-0.0350221583435275,0.0747487266952989));
#72390=CARTESIAN_POINT('Origin',(0.0190187088434312,-0.0345628458713957,
0.0723699603085454));
#72391=CARTESIAN_POINT('',(0.00240490266024603,-0.035195136029876,0.0747485949252347));
#72392=CARTESIAN_POINT('Origin',(-0.00855420375129167,-0.0351951838366786,
0.0758956914862782));
#72393=CARTESIAN_POINT('',(0.00241803668780661,-0.035195137132875,0.0748729061004478));
#72394=CARTESIAN_POINT('Ctrl Pts',(0.00213648554604413,-0.0350241211494342,
0.0745402292404247));
#72395=CARTESIAN_POINT('Ctrl Pts',(0.00214186079383076,-0.0349144232818961,
0.0746227017968508));
#72396=CARTESIAN_POINT('Ctrl Pts',(0.00214894402563534,-0.0348045283579411,
0.0747051126068645));
#72397=CARTESIAN_POINT('Ctrl Pts',(0.00215773009678787,-0.0346945769439157,
0.074787355775073));
#72398=CARTESIAN_POINT('Ctrl Pts',(0.0022260330087906,-0.0350241211494342,
0.0746096726974142));
#72399=CARTESIAN_POINT('Ctrl Pts',(0.00223236481172434,-0.0349144232818961,
0.0746909117742568));
#72400=CARTESIAN_POINT('Ctrl Pts',(0.002240379674316,-0.0348045283579411,
0.0747720685937117));
#72401=CARTESIAN_POINT('Ctrl Pts',(0.0022500711988244,-0.0346945769439157,
0.074853038822183));
#72402=CARTESIAN_POINT('Ctrl Pts',(0.00231558047153708,-0.0350241211494342,
0.0746791161544036));
#72403=CARTESIAN_POINT('Ctrl Pts',(0.00232286882961792,-0.0349144232818961,
0.0747591217516629));
#72404=CARTESIAN_POINT('Ctrl Pts',(0.00233181532299665,-0.0348045283579411,
0.0748390245805589));
#72405=CARTESIAN_POINT('Ctrl Pts',(0.00234241230086092,-0.0346945769439157,
0.074918721869293));
#72406=CARTESIAN_POINT('Ctrl Pts',(0.00240512793428355,-0.0350241211494342,
0.0747485596113931));
#72407=CARTESIAN_POINT('Ctrl Pts',(0.00241337284751149,-0.0349144232818961,
0.0748273317290688));
#72408=CARTESIAN_POINT('Ctrl Pts',(0.00242325097167731,-0.0348045283579411,
0.074905980567406));
#72409=CARTESIAN_POINT('Ctrl Pts',(0.00243475340289745,-0.0346945769439157,
0.074984404916403));
#72410=CARTESIAN_POINT('',(0.00229541549275694,-0.0346945769458128,0.0748852926036652));
#72411=CARTESIAN_POINT('Ctrl Pts',(0.00215638230755627,-0.034711613649279,
0.0747746107153548));
#72412=CARTESIAN_POINT('Ctrl Pts',(0.00219909011810518,-0.0347621546532347,
0.0747701404675735));
#72413=CARTESIAN_POINT('Ctrl Pts',(0.00224104700993601,-0.0348133084097138,
0.0747657488188281));
#72414=CARTESIAN_POINT('Ctrl Pts',(0.00232349397203097,-0.0349168561544564,
0.0747571190542807));
#72415=CARTESIAN_POINT('Ctrl Pts',(0.00236395133978478,-0.034969208901592,
0.0747528843614666));
#72416=CARTESIAN_POINT('Ctrl Pts',(0.00240367281094638,-0.0350221583434999,
0.074748726695315));
#72417=CARTESIAN_POINT('Ctrl Pts',(0.00241895788224886,-0.0351951371254872,
0.0748717695175402));
#72418=CARTESIAN_POINT('Ctrl Pts',(0.00243388001417029,-0.035030733898092,
0.0749897131808378));
#72419=CARTESIAN_POINT('Ctrl Pts',(0.00245366413408612,-0.0348659306897825,
0.0751069393141541));
#72420=CARTESIAN_POINT('Ctrl Pts',(0.00241803668792182,-0.0351951371254872,
0.0748729061004327));
#72421=CARTESIAN_POINT('Ctrl Pts',(0.00243298231798144,-0.035030733898092,
0.0749908688088451));
#72422=CARTESIAN_POINT('Ctrl Pts',(0.00245279070311158,-0.0348659306897825,
0.0751081129997988));
#72423=CARTESIAN_POINT('Ctrl Pts',(0.00226364355862915,-0.0351951371254872,
0.0750633985777853));
#72424=CARTESIAN_POINT('Ctrl Pts',(0.00228252750113895,-0.035030733898092,
0.0751845532672762));
#72425=CARTESIAN_POINT('Ctrl Pts',(0.00230640276147664,-0.0348659306897825,
0.0753048239370764));
#72426=CARTESIAN_POINT('Origin',(-0.00279153162246081,-0.0308609197411044,
0.0759913706608974));
#72427=CARTESIAN_POINT('',(0.0023507247646528,-0.0351951371254872,0.0749559565255237));
#72428=CARTESIAN_POINT('Origin',(0.00905356251905436,-0.0351840467441192,
0.0738495766405217));
#72429=CARTESIAN_POINT('Origin',(-0.00351662015186023,-0.0352322614047276,
0.0769196211525918));
#72430=CARTESIAN_POINT('',(0.00249674051053438,-0.0351951142564656,0.0753392083442391));
#72431=CARTESIAN_POINT('',(0.00252514072129866,-0.0351951372916786,0.0754606157599132));
#72432=CARTESIAN_POINT('Origin',(0.00836370110251291,-0.035287511944211,
0.0743917270355528));
#72433=CARTESIAN_POINT('Origin',(0.00784399112240425,-0.0298325076522344,
0.0666522065087368));
#72434=CARTESIAN_POINT('Origin',(-0.000155814137235747,-0.0338733336719971,
0.0728482042036773));
#72435=CARTESIAN_POINT('Ctrl Pts',(0.00287253105406548,-0.0321934096636942,
0.0718042597714128));
#72436=CARTESIAN_POINT('Ctrl Pts',(0.00283054342099563,-0.0320508460843093,
0.0718982546661998));
#72437=CARTESIAN_POINT('Ctrl Pts',(0.00279111290409766,-0.0319086045660614,
0.071993306813379));
#72438=CARTESIAN_POINT('Ctrl Pts',(0.00275430755500245,-0.0317669892864229,
0.0720892045593931));
#72439=CARTESIAN_POINT('Ctrl Pts',(0.00284000561464614,-0.0321934096636942,
0.0718815419065962));
#72440=CARTESIAN_POINT('Ctrl Pts',(0.00279940129499496,-0.0320508460843093,
0.0719761189912605));
#72441=CARTESIAN_POINT('Ctrl Pts',(0.00276136869078604,-0.0319086045660614,
0.0720717157224417));
#72442=CARTESIAN_POINT('Ctrl Pts',(0.00272597274716384,-0.0317669892864229,
0.0721681195217954));
#72443=CARTESIAN_POINT('Ctrl Pts',(0.00280748017522678,-0.0321934096636942,
0.0719588240417795));
#72444=CARTESIAN_POINT('Ctrl Pts',(0.00276825916899429,-0.0320508460843093,
0.072053983316321));
#72445=CARTESIAN_POINT('Ctrl Pts',(0.00273162447747442,-0.0319086045660614,
0.0721501246315045));
#72446=CARTESIAN_POINT('Ctrl Pts',(0.00269763793932524,-0.0317669892864229,
0.0722470344841978));
#72447=CARTESIAN_POINT('Ctrl Pts',(0.00277495473580743,-0.0321934096636942,
0.0720361061769628));
#72448=CARTESIAN_POINT('Ctrl Pts',(0.00273711704299362,-0.0320508460843093,
0.0721318476413816));
#72449=CARTESIAN_POINT('Ctrl Pts',(0.0027018802641628,-0.0319086045660614,
0.0722285335405672));
#72450=CARTESIAN_POINT('Ctrl Pts',(0.00266930313148663,-0.0317669892864229,
0.0723259494466002));
#72451=CARTESIAN_POINT('',(0.00277553662234814,-0.0321934096636942,0.0720347235842935));
#72452=CARTESIAN_POINT('',(0.00269314705375743,-0.0318665617511262,0.0722562399908496));
#72453=CARTESIAN_POINT('Origin',(0.0180774672077036,-0.0326371944420532,
0.0787480554851963));
#72454=CARTESIAN_POINT('Origin',(-0.00765679016673187,-0.0316939261509361,
0.0686470309856634));
#72455=CARTESIAN_POINT('',(0.00282271380938108,-0.0320197221621828,0.0719192460562448));
#72456=CARTESIAN_POINT('Ctrl Pts',(0.00282260094872311,-0.0320197392094742,
0.0719193926077748));
#72457=CARTESIAN_POINT('Ctrl Pts',(0.00281125094445531,-0.0319792716576039,
0.0719463667404374));
#72458=CARTESIAN_POINT('Ctrl Pts',(0.00280005491057772,-0.0319386439829676,
0.0719735501974854));
#72459=CARTESIAN_POINT('Ctrl Pts',(0.00278900891356809,-0.0318979099381608,
0.0720009747373043));
#72460=CARTESIAN_POINT('Ctrl Pts',(0.00277796313489029,-0.0318571766984908,
0.072028398735058));
#72461=CARTESIAN_POINT('Ctrl Pts',(0.00276712187634602,-0.0318163871833554,
0.0720559237537243));
#72462=CARTESIAN_POINT('Ctrl Pts',(0.00275651915120915,-0.0317755399638303,
0.072083453828186));
#72463=CARTESIAN_POINT('',(0.00282402550318807,-0.0321934096636183,0.071919511482288));
#72464=CARTESIAN_POINT('Origin',(0.000689099354915879,-0.0324111540182647,
0.0710438044112699));
#72465=CARTESIAN_POINT('',(0.00279978106277811,-0.0321934096636662,0.0719771175333007));
#72466=CARTESIAN_POINT('Ctrl Pts',(0.00277741482267836,-0.0321934096636618,
0.0720339580446808));
#72467=CARTESIAN_POINT('Ctrl Pts',(0.00274823295496786,-0.0320835708272592,
0.0721076886174341));
#72468=CARTESIAN_POINT('Ctrl Pts',(0.00272059386429774,-0.0319739230346489,
0.0721819803406944));
#72469=CARTESIAN_POINT('Ctrl Pts',(0.00269452561806012,-0.0318646057455573,
0.0722567354493983));
#72470=CARTESIAN_POINT('Ctrl Pts',(0.0026724778611228,-0.0321934096636618,
0.0720767295172299));
#72471=CARTESIAN_POINT('Ctrl Pts',(0.00264388584535289,-0.0320835708272592,
0.072151907252466));
#72472=CARTESIAN_POINT('Ctrl Pts',(0.00261686621343762,-0.0319739230346489,
0.072227633091841));
#72473=CARTESIAN_POINT('Ctrl Pts',(0.00259144609939487,-0.0318646057455573,
0.0723038074962655));
#72474=CARTESIAN_POINT('Ctrl Pts',(0.00256754089956724,-0.0321934096636618,
0.0721195009897789));
#72475=CARTESIAN_POINT('Ctrl Pts',(0.00253953873573791,-0.0320835708272592,
0.072196125887498));
#72476=CARTESIAN_POINT('Ctrl Pts',(0.00251313856257751,-0.0319739230346489,
0.0722732858429875));
#72477=CARTESIAN_POINT('Ctrl Pts',(0.00248836658072962,-0.0318646057455573,
0.0723508795431327));
#72478=CARTESIAN_POINT('Ctrl Pts',(0.00246260393801168,-0.0321934096636618,
0.0721622724623279));
#72479=CARTESIAN_POINT('Ctrl Pts',(0.00243519162612294,-0.0320835708272592,
0.07224034452253));
#72480=CARTESIAN_POINT('Ctrl Pts',(0.0024094109117174,-0.0319739230346489,
0.0723189385941341));
#72481=CARTESIAN_POINT('Ctrl Pts',(0.00238528706206437,-0.0318646057455573,
0.0723979515899999));
#72482=CARTESIAN_POINT('',(0.00245837103291331,-0.0321763980308256,0.0721743693757221));
#72483=CARTESIAN_POINT('',(0.00246260393800085,-0.0321934096636184,0.0721622724623588));
#72484=CARTESIAN_POINT('Origin',(0.0178705323178745,-0.0326386231243202,
0.0781986017914123));
#72485=CARTESIAN_POINT('Ctrl Pts',(0.00245837103590465,-0.0321763980306268,
0.0721743693767623));
#72486=CARTESIAN_POINT('Ctrl Pts',(0.0024988965654995,-0.0321259596175073,
0.0721885013567844));
#72487=CARTESIAN_POINT('Ctrl Pts',(0.00253871993771195,-0.0320749164631912,
0.072202388481909));
#72488=CARTESIAN_POINT('Ctrl Pts',(0.00261699441599857,-0.0319716057793887,
0.0722296841983239));
#72489=CARTESIAN_POINT('Ctrl Pts',(0.0026554150236457,-0.0319193786690081,
0.0722430821542649));
#72490=CARTESIAN_POINT('Ctrl Pts',(0.00269314705550645,-0.0318665617525265,
0.072256239991455));
#72491=CARTESIAN_POINT('',(0.0026190702801845,-0.0321934096636663,0.0720984980233362));
#72492=CARTESIAN_POINT('Origin',(0.00812378219310841,-0.0315241814719618,
0.07415));
#72493=CARTESIAN_POINT('',(0.00245837103256181,-0.0322104233323781,0.0721743693755995));
#72494=CARTESIAN_POINT('',(0.00245416397318719,-0.0321934096636183,0.0721864753018188));
#72495=CARTESIAN_POINT('Origin',(0.017891280271871,-0.0326387229794279,
0.0781582931490726));
#72496=CARTESIAN_POINT('Origin',(0.0182745539159592,-0.0326386246414647,
0.0770400193105253));
#72497=CARTESIAN_POINT('Origin',(0.0182657321622171,-0.0326387241409828,
0.0770844873325173));
#72498=CARTESIAN_POINT('Ctrl Pts',(0.00274833537119431,-0.0327445246967096,
0.072104835834273));
#72499=CARTESIAN_POINT('Ctrl Pts',(0.00267120074370361,-0.032443687833936,
0.0723075741254835));
#72500=CARTESIAN_POINT('Ctrl Pts',(0.00260955632423863,-0.0321434074405927,
0.0725155465540164));
#72501=CARTESIAN_POINT('Ctrl Pts',(0.00266453555560477,-0.0327445246967096,
0.0723403726486082));
#72502=CARTESIAN_POINT('Ctrl Pts',(0.0025962843442909,-0.032443687833936,
0.0725462715015319));
#72503=CARTESIAN_POINT('Ctrl Pts',(0.00254373617058122,-0.0321434074405927,
0.0727567263777426));
#72504=CARTESIAN_POINT('',(0.00265327085821773,-0.0326943950436612,0.0723747167170185));
#72505=CARTESIAN_POINT('',(0.00258495299593697,-0.0323666188837389,0.0726009692951519));
#72506=CARTESIAN_POINT('Origin',(0.0186666169906941,-0.0326395579111819,
0.0774914347928655));
#72507=CARTESIAN_POINT('Origin',(-0.00805152535827163,-0.0321933825603026,
0.0696262928316853));
#72508=CARTESIAN_POINT('',(0.0026199279576995,-0.0321934096532688,0.0724809542990163));
#72509=CARTESIAN_POINT('',(0.00260309464350963,-0.0321934096584275,0.0725411447457605));
#72510=CARTESIAN_POINT('',(0.00269314705285821,-0.0325210109756238,0.0722562399905266));
#72511=CARTESIAN_POINT('Origin',(0.018494272782392,-0.0326393129154779,
0.0779403021487711));
#72512=CARTESIAN_POINT('',(0.0026944298295701,-0.0326943950436593,0.07225668731781));
#72513=CARTESIAN_POINT('Origin',(-0.00775112945723936,-0.0326943765538138,
0.068614132187655));
#72514=CARTESIAN_POINT('',(0.00267385034390392,-0.0326943950436702,0.0723157020174243));
#72515=CARTESIAN_POINT('Ctrl Pts',(0.00254016309196034,-0.0325229783203769,
0.0719538220169292));
#72516=CARTESIAN_POINT('Ctrl Pts',(0.00250988882649095,-0.032413025309245,
0.0720307920841329));
#72517=CARTESIAN_POINT('Ctrl Pts',(0.00248121137742225,-0.0323031222208069,
0.072108376739389));
#72518=CARTESIAN_POINT('Ctrl Pts',(0.00245416397171971,-0.0321934096576658,
0.0721864753060561));
#72519=CARTESIAN_POINT('Ctrl Pts',(0.00259162045502572,-0.0325229783203769,
0.0720547838018912));
#72520=CARTESIAN_POINT('Ctrl Pts',(0.00256273794555414,-0.032413025309245,
0.0721310445304703));
#72521=CARTESIAN_POINT('Ctrl Pts',(0.00253543736781553,-0.0323031222208069,
0.0722078911644263));
#72522=CARTESIAN_POINT('Ctrl Pts',(0.00250975021845946,-0.0321934096576658,
0.0722852240347048));
#72523=CARTESIAN_POINT('Ctrl Pts',(0.0026430778180911,-0.0325229783203769,
0.0721557455868532));
#72524=CARTESIAN_POINT('Ctrl Pts',(0.00261558706461734,-0.032413025309245,
0.0722312969768077));
#72525=CARTESIAN_POINT('Ctrl Pts',(0.00258966335820881,-0.0323031222208069,
0.0723074055894637));
#72526=CARTESIAN_POINT('Ctrl Pts',(0.0025653364651992,-0.0321934096576658,
0.0723839727633535));
#72527=CARTESIAN_POINT('Ctrl Pts',(0.00269453518115648,-0.0325229783203769,
0.0722567073718152));
#72528=CARTESIAN_POINT('Ctrl Pts',(0.00266843618368053,-0.032413025309245,
0.0723315494231452));
#72529=CARTESIAN_POINT('Ctrl Pts',(0.00264388934860209,-0.0323031222208069,
0.072406920014501));
#72530=CARTESIAN_POINT('Ctrl Pts',(0.00262092271193895,-0.0321934096576658,
0.0724827214920023));
#72531=CARTESIAN_POINT('',(0.00253704596545532,-0.0321934096584274,0.0723337147999117));
#72532=CARTESIAN_POINT('Ctrl Pts',(0.00245837103584071,-0.0322104233328925,
0.0721743693767398));
#72533=CARTESIAN_POINT('Ctrl Pts',(0.00249895147820631,-0.03226094218314,
0.0721885205058314));
#72534=CARTESIAN_POINT('Ctrl Pts',(0.00253880167622704,-0.0323120888240809,
0.0722024169856044));
#72535=CARTESIAN_POINT('Ctrl Pts',(0.00261707674710496,-0.0324156524631811,
0.0722297129086665));
#72536=CARTESIAN_POINT('Ctrl Pts',(0.00265546944481441,-0.0324680267167308,
0.0722431011319038));
#72537=CARTESIAN_POINT('Ctrl Pts',(0.00269314705289765,-0.0325210109755911,
0.0722562399905452));
#72538=CARTESIAN_POINT('Origin',(0.0115903197919812,-0.0262834582512137,
0.0670869622035607));
#72539=CARTESIAN_POINT('Origin',(-0.000352622835556759,-0.0342770775805864,
0.0654337076718416));
#72540=CARTESIAN_POINT('Ctrl Pts',(0.00265509684047048,-0.0326943950436604,
0.0723738349689563));
#72541=CARTESIAN_POINT('Ctrl Pts',(0.00263061795745464,-0.0325844576448134,
0.0724492037025243));
#72542=CARTESIAN_POINT('Ctrl Pts',(0.00260769609100913,-0.0324744968375322,
0.0725250840334893));
#72543=CARTESIAN_POINT('Ctrl Pts',(0.00258635926897814,-0.0323646534831894,
0.0726013783344614));
#72544=CARTESIAN_POINT('Ctrl Pts',(0.00255305273876136,-0.0326943950436604,
0.0724231110167664));
#72545=CARTESIAN_POINT('Ctrl Pts',(0.0025292529720375,-0.0325844576448134,
0.072499886109307));
#72546=CARTESIAN_POINT('Ctrl Pts',(0.00250703935575539,-0.0324744968375322,
0.0725771588535364));
#72547=CARTESIAN_POINT('Ctrl Pts',(0.00248643898570054,-0.0323646534831894,
0.0726548298505402));
#72548=CARTESIAN_POINT('Ctrl Pts',(0.00245100863705224,-0.0326943950436604,
0.0724723870645765));
#72549=CARTESIAN_POINT('Ctrl Pts',(0.00242788798662036,-0.0325844576448134,
0.0725505685160898));
#72550=CARTESIAN_POINT('Ctrl Pts',(0.00240638262050166,-0.0324744968375322,
0.0726292336735836));
#72551=CARTESIAN_POINT('Ctrl Pts',(0.00238651870242293,-0.0323646534831894,
0.0727082813666191));
#72552=CARTESIAN_POINT('Ctrl Pts',(0.00234896453534312,-0.0326943950436604,
0.0725216631123867));
#72553=CARTESIAN_POINT('Ctrl Pts',(0.00232652300120322,-0.0325844576448134,
0.0726012509228725));
#72554=CARTESIAN_POINT('Ctrl Pts',(0.00230572588524793,-0.0324744968375322,
0.0726813084936307));
#72555=CARTESIAN_POINT('Ctrl Pts',(0.00228659841914533,-0.0323646534831894,
0.072761732882698));
#72556=CARTESIAN_POINT('',(0.00234549955420468,-0.0326773559991329,0.0725340019415104));
#72557=CARTESIAN_POINT('',(0.00234896453534291,-0.0326943950436594,0.0725216631123874));
#72558=CARTESIAN_POINT('Origin',(0.018350566223493,-0.0326395671359021,
0.0769579310642256));
#72559=CARTESIAN_POINT('Ctrl Pts',(0.00234549955742792,-0.032677355998741,
0.0725340019424086));
#72560=CARTESIAN_POINT('Ctrl Pts',(0.00238686573544265,-0.0326267922586223,
0.0725455707194201));
#72561=CARTESIAN_POINT('Ctrl Pts',(0.00242749872782376,-0.0325756109579881,
0.0725569344482132));
#72562=CARTESIAN_POINT('Ctrl Pts',(0.00250733292209098,-0.0324719985462362,
0.072579261480482));
#72563=CARTESIAN_POINT('Ctrl Pts',(0.00254650210459833,-0.032419609162177,
0.072590215829177));
#72564=CARTESIAN_POINT('Ctrl Pts',(0.00258495299598395,-0.0323666188837757,
0.0726009692951651));
#72565=CARTESIAN_POINT('',(0.00250111769679032,-0.0326943950436703,0.0724481899147129));
#72566=CARTESIAN_POINT('Origin',(0.00812378219310841,-0.0315241814719618,
0.07415));
#72567=CARTESIAN_POINT('',(0.00234549955424635,-0.032711433837987,0.0725340019415222));
#72568=CARTESIAN_POINT('',(0.00234206093373601,-0.0326943950436593,0.0725463481428483));
#72569=CARTESIAN_POINT('Origin',(0.0183620233690585,-0.0326395665175228,
0.0769140920533534));
#72570=CARTESIAN_POINT('Origin',(0.0183235060544162,-0.0326395680346485,
0.0770546987928396));
#72571=CARTESIAN_POINT('Origin',(0.0183105541251864,-0.0326395676274512,
0.0770981194695469));
#72572=CARTESIAN_POINT('Ctrl Pts',(0.00263051404883578,-0.0332451089994434,
0.0724464360607481));
#72573=CARTESIAN_POINT('Ctrl Pts',(0.00256626308366603,-0.0329451141710254,
0.0726536180584844));
#72574=CARTESIAN_POINT('Ctrl Pts',(0.00251780044374341,-0.0326442513127493,
0.0728650511193878));
#72575=CARTESIAN_POINT('Ctrl Pts',(0.00256167071103577,-0.0332451089994434,
0.0726867704004512));
#72576=CARTESIAN_POINT('Ctrl Pts',(0.00250648410378859,-0.0329451141710254,
0.0728965488671531));
#72577=CARTESIAN_POINT('Ctrl Pts',(0.00246725564756127,-0.0326442513127493,
0.0731098882562337));
#72578=CARTESIAN_POINT('Ctrl Pts',(0.00256098227765777,-0.0332451089994434,
0.0726891737438483));
#72579=CARTESIAN_POINT('Ctrl Pts',(0.00250588631398981,-0.0329451141710254,
0.0728989781752398));
#72580=CARTESIAN_POINT('Ctrl Pts',(0.00246675019959945,-0.0326442513127493,
0.0731123366276022));
#72581=CARTESIAN_POINT('',(0.00255259470306739,-0.0331951640388616,0.0727217160818621));
#72582=CARTESIAN_POINT('',(0.00249861815856648,-0.032867753235499,0.0729518119286545));
#72583=CARTESIAN_POINT('Origin',(0.0189651205048505,-0.0326402808279159,
0.0761365724894495));
#72584=CARTESIAN_POINT('Origin',(-0.0083148397757615,-0.0326944278779092,
0.0706488767437466));
#72585=CARTESIAN_POINT('',(0.00252598830832928,-0.0326943950436593,0.0728298376525857));
#72586=CARTESIAN_POINT('',(0.00251296760118381,-0.0326943950436693,0.0728909662971511));
#72587=CARTESIAN_POINT('',(0.00258495299593777,-0.0330220786163545,0.0726009692951491));
#72588=CARTESIAN_POINT('Origin',(0.0188959009399299,-0.0326396682764628,
0.07661234690804));
#72589=CARTESIAN_POINT('',(0.00258626132929582,-0.0331951640388588,0.0726013351935165));
#72590=CARTESIAN_POINT('Origin',(-0.00803773995683232,-0.0331952026560128,
0.0696301458319343));
#72591=CARTESIAN_POINT('',(0.0025694280161916,-0.0331951640388701,0.0726615256376993));
#72592=CARTESIAN_POINT('Ctrl Pts',(0.0024132816373922,-0.0330240426238172,
0.0723087549312516));
#72593=CARTESIAN_POINT('Ctrl Pts',(0.00238791669273204,-0.032914277406352,
0.0723874226398777));
#72594=CARTESIAN_POINT('Ctrl Pts',(0.00236416538400663,-0.0328043479726691,
0.0724666539314852));
#72595=CARTESIAN_POINT('Ctrl Pts',(0.00234206093373597,-0.0326943950436593,
0.0725463481428483));
#72596=CARTESIAN_POINT('Ctrl Pts',(0.00247097690561098,-0.0330240426238172,
0.0724062864236511));
#72597=CARTESIAN_POINT('Ctrl Pts',(0.00244695555227895,-0.032914277406352,
0.0724841593237477));
#72598=CARTESIAN_POINT('Ctrl Pts',(0.00242453207379845,-0.0328043479726691,
0.0725625676347988));
#72599=CARTESIAN_POINT('Ctrl Pts',(0.00240373796260485,-0.0326943950436593,
0.0726414117010313));
#72600=CARTESIAN_POINT('Ctrl Pts',(0.00252867217382976,-0.0330240426238172,
0.0725038179160505));
#72601=CARTESIAN_POINT('Ctrl Pts',(0.00250599441182586,-0.032914277406352,
0.0725808960076177));
#72602=CARTESIAN_POINT('Ctrl Pts',(0.00248489876359028,-0.0328043479726691,
0.0726584813381124));
#72603=CARTESIAN_POINT('Ctrl Pts',(0.00246541499147372,-0.0326943950436593,
0.0727364752592143));
#72604=CARTESIAN_POINT('Ctrl Pts',(0.00258636744204854,-0.0330240426238172,
0.07260134940845));
#72605=CARTESIAN_POINT('Ctrl Pts',(0.00256503327137277,-0.032914277406352,
0.0726776326914877));
#72606=CARTESIAN_POINT('Ctrl Pts',(0.0025452654533821,-0.0328043479726691,
0.072754395041426));
#72607=CARTESIAN_POINT('Ctrl Pts',(0.0025270920203426,-0.0326943950436593,
0.0728315388173973));
#72608=CARTESIAN_POINT('',(0.00243402462104264,-0.0326943950436693,0.072688092897727));
#72609=CARTESIAN_POINT('Ctrl Pts',(0.00234549955743356,-0.0327114338383322,
0.0725340019424101));
#72610=CARTESIAN_POINT('Ctrl Pts',(0.00238685885493013,-0.0327619876831102,
0.0725455687951641));
#72611=CARTESIAN_POINT('Ctrl Pts',(0.00242748848656163,-0.0328131562604616,
0.0725569315840646));
#72612=CARTESIAN_POINT('Ctrl Pts',(0.0025073226074475,-0.0329167375858765,
0.0725792585958111));
#72613=CARTESIAN_POINT('Ctrl Pts',(0.00254649528670868,-0.0329691088920617,
0.0725902139224345));
#72614=CARTESIAN_POINT('Ctrl Pts',(0.00258495299598281,-0.0330220786163186,
0.0726009692951646));
#72615=CARTESIAN_POINT('Ctrl Pts',(0.00255436199884358,-0.0331951640388604,
0.0727207212605565));
#72616=CARTESIAN_POINT('Ctrl Pts',(0.00252481257727386,-0.0330306422010619,
0.0728358654522929));
#72617=CARTESIAN_POINT('Ctrl Pts',(0.00250004743601074,-0.0328657861914645,
0.0729521325627926));
#72618=CARTESIAN_POINT('Ctrl Pts',(0.00255259470306825,-0.0331951640388604,
0.072721716081859));
#72619=CARTESIAN_POINT('Ctrl Pts',(0.00252306584879114,-0.0330306422010619,
0.0728368968113025));
#72620=CARTESIAN_POINT('Ctrl Pts',(0.00249832276738788,-0.0328657861914645,
0.0729531995782202));
#72621=CARTESIAN_POINT('Ctrl Pts',(0.00225811569971723,-0.0331951640388604,
0.0728874800641939));
#72622=CARTESIAN_POINT('Ctrl Pts',(0.00223201390949691,-0.0330306422010619,
0.0730087489582292));
#72623=CARTESIAN_POINT('Ctrl Pts',(0.00221094659399328,-0.0328657861914645,
0.0731309930432835));
#72624=CARTESIAN_POINT('',(0.00225543231627635,-0.0331781648281893,0.072900012112519));
#72625=CARTESIAN_POINT('',(0.00225811569971698,-0.0331951640388588,0.072887480064195));
#72626=CARTESIAN_POINT('Origin',(0.0185485722983833,-0.0326412091073963,
0.0756422870574227));
#72627=CARTESIAN_POINT('Ctrl Pts',(0.00225543231762155,-0.033178164828644,
0.0729000121112653));
#72628=CARTESIAN_POINT('Ctrl Pts',(0.00229747220381256,-0.0331276811546783,
0.0729089668050028));
#72629=CARTESIAN_POINT('Ctrl Pts',(0.00233875298689534,-0.0330765663497793,
0.072917759771628));
#72630=CARTESIAN_POINT('Ctrl Pts',(0.00241983178050239,-0.0329730614463187,
0.0729350299639476));
#72631=CARTESIAN_POINT('Ctrl Pts',(0.00245959703584213,-0.0329207133373865,
0.072943500218103));
#72632=CARTESIAN_POINT('Ctrl Pts',(0.00249861815295666,-0.032867753228935,
0.0729518119131668));
#72633=CARTESIAN_POINT('',(0.00240535520140218,-0.0331951640388701,0.0728045980730385));
#72634=CARTESIAN_POINT('Origin',(0.00812378219310841,-0.0315241814719618,
0.07415));
#72635=CARTESIAN_POINT('',(0.00225543231765757,-0.0332121607144417,0.0729000121134746));
#72636=CARTESIAN_POINT('',(0.00225277570667803,-0.0331951640388587,0.0729125498651186));
#72637=CARTESIAN_POINT('Origin',(0.0185502083173675,-0.0326413646593987,
0.0755969704929008));
#72638=CARTESIAN_POINT('Origin',(0.0182518005157393,-0.0326412102062352,
0.0770355624861156));
#72639=CARTESIAN_POINT('Origin',(0.0182348218801358,-0.0326413658608145,
0.0770776108576931));
#72640=CARTESIAN_POINT('Ctrl Pts',(0.00253439100278785,-0.0337436976235975,
0.0727947025708106));
#72641=CARTESIAN_POINT('Ctrl Pts',(0.00252220125230878,-0.0336723290703325,
0.0728449744022718));
#72642=CARTESIAN_POINT('Ctrl Pts',(0.00251091770563862,-0.033601104548885,
0.072895457356125));
#72643=CARTESIAN_POINT('Ctrl Pts',(0.00247489157626549,-0.0333736987606857,
0.0730566394276685));
#72644=CARTESIAN_POINT('Ctrl Pts',(0.00244817437173634,-0.0331450831799191,
0.0732196232709377));
#72645=CARTESIAN_POINT('Ctrl Pts',(0.00248077334520411,-0.0337436976235975,
0.0730388851803373));
#72646=CARTESIAN_POINT('Ctrl Pts',(0.00247077981012201,-0.0336723290703325,
0.0730896392571367));
#72647=CARTESIAN_POINT('Ctrl Pts',(0.00246170079762656,-0.033601104548885,
0.0731405648753196));
#72648=CARTESIAN_POINT('Ctrl Pts',(0.00243271330917961,-0.0333736987606857,
0.0733031602863809));
#72649=CARTESIAN_POINT('Ctrl Pts',(0.00241310425202402,-0.0331450831799191,
0.0734671512222955));
#72650=CARTESIAN_POINT('Ctrl Pts',(0.00248023716862828,-0.0337436976235975,
0.0730413270064326));
#72651=CARTESIAN_POINT('Ctrl Pts',(0.00247026559570014,-0.0336723290703325,
0.0730920859056854));
#72652=CARTESIAN_POINT('Ctrl Pts',(0.00246120862854643,-0.033601104548885,
0.0731430159505116));
#72653=CARTESIAN_POINT('Ctrl Pts',(0.00243229152650876,-0.0333736987606857,
0.073305625494968));
#72654=CARTESIAN_POINT('Ctrl Pts',(0.0024127535508269,-0.0331450831799191,
0.0734696265018091));
#72655=CARTESIAN_POINT('',(0.0024739054797044,-0.0336938721132548,0.0730743522308228));
#72656=CARTESIAN_POINT('',(0.00243448329033809,-0.0333679869945434,0.0733073832455932));
#72657=CARTESIAN_POINT('Ctrl Pts',(0.002473905479702,-0.0336938721132646,
0.0730743522308302));
#72658=CARTESIAN_POINT('Ctrl Pts',(0.00246970672186403,-0.0336629187933929,
0.0730964063500471));
#72659=CARTESIAN_POINT('Ctrl Pts',(0.00246563844262391,-0.0336319952301037,
0.0731184780012467));
#72660=CARTESIAN_POINT('Ctrl Pts',(0.00246170079762486,-0.0336011045488947,
0.0731405648753273));
#72661=CARTESIAN_POINT('Ctrl Pts',(0.00245181989893595,-0.0335235892595451,
0.0731959884000984));
#72662=CARTESIAN_POINT('Ctrl Pts',(0.00244274416720702,-0.0334458668660366,
0.0732516062887103));
#72663=CARTESIAN_POINT('Ctrl Pts',(0.00243448329001444,-0.0333679869945382,
0.0733073832455381));
#72664=CARTESIAN_POINT('Ctrl Pts',(0.00243447609490957,-0.0333679692460365,
0.0733074271351641));
#72665=CARTESIAN_POINT('Ctrl Pts',(0.0024349252866878,-0.0333391895375683,
0.0733074876708405));
#72666=CARTESIAN_POINT('Ctrl Pts',(0.00243526241153149,-0.0333104081062018,
0.0733075298271899));
#72667=CARTESIAN_POINT('Ctrl Pts',(0.00243570934097129,-0.0332532698406287,
0.0733075801326614));
#72668=CARTESIAN_POINT('Ctrl Pts',(0.00243582246359359,-0.0332249172150636,
0.0733075887777692));
#72669=CARTESIAN_POINT('Ctrl Pts',(0.00243582710526423,-0.0331960985328845,
0.0733075824901749));
#72670=CARTESIAN_POINT('Ctrl Pts',(0.00243582715108201,-0.0331956312596458,
0.073307582383917));
#72671=CARTESIAN_POINT('Ctrl Pts',(0.00243582716738049,-0.0331951640388591,
0.0733075822738707));
#72672=CARTESIAN_POINT('',(0.00245414059620932,-0.0331951640388587,0.0731839310776592));
#72673=CARTESIAN_POINT('',(0.00244498388180488,-0.0331951640388687,0.073245756675775));
#72674=CARTESIAN_POINT('',(0.0024986181678396,-0.0335216366567738,0.0729518119162085));
#72675=CARTESIAN_POINT('Origin',(0.0189968054966534,-0.0326434571528791,
0.0752278786714746));
#72676=CARTESIAN_POINT('',(0.00249994689401839,-0.0336938721132328,0.0729520949416964));
#72677=CARTESIAN_POINT('Origin',(-0.00818100638126998,-0.033693886789632,
0.0706769977807942));
#72678=CARTESIAN_POINT('',(0.0024869261868714,-0.0336938721132538,0.0730132235862696));
#72679=CARTESIAN_POINT('Ctrl Pts',(0.00230893703444126,-0.0335235895815172,
0.0726709544358767));
#72680=CARTESIAN_POINT('Ctrl Pts',(0.00228857506027835,-0.0334144449262748,
0.0727510072278623));
#72681=CARTESIAN_POINT('Ctrl Pts',(0.00226984352311004,-0.0333049234473147,
0.0728315726538694));
#72682=CARTESIAN_POINT('Ctrl Pts',(0.00225277570667789,-0.0331951640388587,
0.0729125498651184));
#72683=CARTESIAN_POINT('Ctrl Pts',(0.00237264261285953,-0.0335235895815172,
0.0727646708792808));
#72684=CARTESIAN_POINT('Ctrl Pts',(0.00235357083005078,-0.0334144449262748,
0.0728438466385548));
#72685=CARTESIAN_POINT('Ctrl Pts',(0.0023361128476744,-0.0333049234473147,
0.0729235073698635));
#72686=CARTESIAN_POINT('Ctrl Pts',(0.002320300216196,-0.0331951640388587,
0.0730035532337389));
#72687=CARTESIAN_POINT('Ctrl Pts',(0.0024363481912778,-0.0335235895815172,
0.072858387322685));
#72688=CARTESIAN_POINT('Ctrl Pts',(0.0024185665998232,-0.0334144449262748,
0.0729366860492473));
#72689=CARTESIAN_POINT('Ctrl Pts',(0.00240238217223875,-0.0333049234473147,
0.0730154420858577));
#72690=CARTESIAN_POINT('Ctrl Pts',(0.0023878247257141,-0.0331951640388587,
0.0730945566023593));
#72691=CARTESIAN_POINT('Ctrl Pts',(0.00250005376969607,-0.0335235895815172,
0.0729521037660892));
#72692=CARTESIAN_POINT('Ctrl Pts',(0.00248356236959563,-0.0334144449262748,
0.0730295254599398));
#72693=CARTESIAN_POINT('Ctrl Pts',(0.00246865149680311,-0.0333049234473147,
0.0731073768018518));
#72694=CARTESIAN_POINT('Ctrl Pts',(0.00245534923523221,-0.0331951640388587,
0.0731855599709798));
#72695=CARTESIAN_POINT('',(0.00235345815145367,-0.0331951640388687,0.0730482404713989));
#72696=CARTESIAN_POINT('Ctrl Pts',(0.00225543232071546,-0.0332121607145975,
0.0729000121141221));
#72697=CARTESIAN_POINT('Ctrl Pts',(0.00229740148257267,-0.0332625444109919,
0.0729089517555959));
#72698=CARTESIAN_POINT('Ctrl Pts',(0.00233864744991015,-0.0333135300747167,
0.0729177373530184));
#72699=CARTESIAN_POINT('Ctrl Pts',(0.00241972573601266,-0.0334167203140634,
0.072935007433644));
#72700=CARTESIAN_POINT('Ctrl Pts',(0.00245952665252752,-0.0334688847587342,
0.0729434852280108));
#72701=CARTESIAN_POINT('Ctrl Pts',(0.00249861816849204,-0.0335216366562426,
0.0729518119165108));
#72702=CARTESIAN_POINT('Ctrl Pts',(0.00247474426424094,-0.0336938721132388,
0.0730738080292304));
#72703=CARTESIAN_POINT('Ctrl Pts',(0.00246844495551768,-0.0336474569764957,
0.0731068737227775));
#72704=CARTESIAN_POINT('Ctrl Pts',(0.00246253315411867,-0.033601104548885,
0.0731400108920043));
#72705=CARTESIAN_POINT('Ctrl Pts',(0.00244756583218471,-0.0334837508592656,
0.0732239065857737));
#72706=CARTESIAN_POINT('Ctrl Pts',(0.00243509108614637,-0.0333660264659097,
0.0733082089515187));
#72707=CARTESIAN_POINT('Ctrl Pts',(0.00247390547970826,-0.0336938721132388,
0.0730743522308028));
#72708=CARTESIAN_POINT('Ctrl Pts',(0.00246760935637739,-0.0336474569764957,
0.0731074228340341));
#72709=CARTESIAN_POINT('Ctrl Pts',(0.00246170079762656,-0.033601104548885,
0.0731405648753196));
#72710=CARTESIAN_POINT('Ctrl Pts',(0.00244674168533225,-0.0334837508592656,
0.0732244729040216));
#72711=CARTESIAN_POINT('Ctrl Pts',(0.00243427551083811,-0.0333660264659097,
0.073308787356014));
#72712=CARTESIAN_POINT('Ctrl Pts',(0.00218871503290588,-0.0336938721132388,
0.0732593831696475));
#72713=CARTESIAN_POINT('Ctrl Pts',(0.00218350195705983,-0.0336474569764957,
0.0732941230872002));
#72714=CARTESIAN_POINT('Ctrl Pts',(0.00217869591301452,-0.033601104548885,
0.0733289216499863));
#72715=CARTESIAN_POINT('Ctrl Pts',(0.0021665281144706,-0.0334837508592656,
0.0734170236102697));
#72716=CARTESIAN_POINT('Ctrl Pts',(0.00215697630287576,-0.0333660264659097,
0.073505447439764));
#72717=CARTESIAN_POINT('',(0.00218852477495756,-0.0336769361243753,0.073270955416213));
#72718=CARTESIAN_POINT('',(0.00219041596997241,-0.033693872113232,0.0732582796053983));
#72719=CARTESIAN_POINT('Ctrl Pts',(0.00218852477495752,-0.033676936124375,
0.0732709554162133));
#72720=CARTESIAN_POINT('Ctrl Pts',(0.00218883774124687,-0.0336797586670072,
0.0732688422862028));
#72721=CARTESIAN_POINT('Ctrl Pts',(0.00218915182420595,-0.0336825812712939,
0.0732667294032504));
#72722=CARTESIAN_POINT('Ctrl Pts',(0.00218978222305854,-0.0336882266040259,
0.0732625041306933));
#72723=CARTESIAN_POINT('Ctrl Pts',(0.0021900985389585,-0.0336910493324753,
0.0732603917410849));
#72724=CARTESIAN_POINT('Ctrl Pts',(0.00219041596997441,-0.0336938721132317,
0.0732582796053982));
#72725=CARTESIAN_POINT('Ctrl Pts',(0.00218852477495759,-0.0336769361243753,
0.073270955416213));
#72726=CARTESIAN_POINT('Ctrl Pts',(0.00222998626234548,-0.0336279007516223,
0.0732770960927425));
#72727=CARTESIAN_POINT('Ctrl Pts',(0.00227203809666917,-0.0335767878632079,
0.073283324202931));
#72728=CARTESIAN_POINT('Ctrl Pts',(0.0023544478837272,-0.0334733198857318,
0.0732955295500391));
#72729=CARTESIAN_POINT('Ctrl Pts',(0.00239485489871443,-0.0334209645014067,
0.0733015140533508));
#72730=CARTESIAN_POINT('Ctrl Pts',(0.00243448329139574,-0.0333679869844681,
0.0733073832383745));
#72731=CARTESIAN_POINT('',(0.00233216072484841,-0.0336938721132534,0.0731663159181205));
#72732=CARTESIAN_POINT('Origin',(0.00812378219310841,-0.0315241814719618,
0.07415));
#72733=CARTESIAN_POINT('',(0.00218852477624567,-0.0337108120655398,0.073270955416408));
#72734=CARTESIAN_POINT('',(0.00218666066001425,-0.0336938721132327,0.073283635237734));
#72735=CARTESIAN_POINT('Origin',(0.0182094577056769,-0.0345562511818623,
0.076773540193245));
#72736=CARTESIAN_POINT('Ctrl Pts',(0.0021866606600214,-0.0336938721132293,
0.0732836352377395));
#72737=CARTESIAN_POINT('Ctrl Pts',(0.00218696906411422,-0.0336910493409645,
0.0732815217716105));
#72738=CARTESIAN_POINT('Ctrl Pts',(0.00218727861043721,-0.0336882266082704,
0.0732794083761406));
#72739=CARTESIAN_POINT('Ctrl Pts',(0.00218789998272394,-0.0336825812712746,
0.0732751817634371));
#72740=CARTESIAN_POINT('Ctrl Pts',(0.00218821180866932,-0.0336797586669975,
0.0732730685462159));
#72741=CARTESIAN_POINT('Ctrl Pts',(0.0021885247749576,-0.033676936124375,
0.0732709554162127));
#72742=CARTESIAN_POINT('Origin',(0.0185369295380939,-0.034556251520342,
0.0745624488552952));
#72743=CARTESIAN_POINT('Ctrl Pts',(0.00246032955331888,-0.034243627687391,
0.0731482868689784));
#72744=CARTESIAN_POINT('Ctrl Pts',(0.00242254931976735,-0.0339430054201809,
0.0733618875065393));
#72745=CARTESIAN_POINT('Ctrl Pts',(0.00240096569112108,-0.0336441434784052,
0.0735777270890724));
#72746=CARTESIAN_POINT('Ctrl Pts',(0.00242214783259408,-0.034243627687391,
0.0733953539776808));
#72747=CARTESIAN_POINT('Ctrl Pts',(0.00239368588866121,-0.0339430054201809,
0.0736103946625782));
#72748=CARTESIAN_POINT('Ctrl Pts',(0.00238150254761548,-0.0336441434784052,
0.0738269683096698));
#72749=CARTESIAN_POINT('Ctrl Pts',(0.00242176601538683,-0.034243627687391,
0.0733978246487678));
#72750=CARTESIAN_POINT('Ctrl Pts',(0.00239339725435015,-0.0339430054201809,
0.0736128797341386));
#72751=CARTESIAN_POINT('Ctrl Pts',(0.00238130791618042,-0.0336441434784052,
0.0738294607218758));
#72752=CARTESIAN_POINT('',(0.00241751373855154,-0.0341934961088741,0.0734312334700822));
#72753=CARTESIAN_POINT('',(0.00239280147842421,-0.0338664212863773,0.0736662799856491));
#72754=CARTESIAN_POINT('Origin',(0.0189497159229241,-0.0345610720406939,
0.0760272755920783));
#72755=CARTESIAN_POINT('Origin',(-0.00853460080732833,-0.033693800507303,
0.0727439981907874));
#72756=CARTESIAN_POINT('',(0.00240466836925947,-0.0336938721132327,0.0735418371354143));
#72757=CARTESIAN_POINT('',(0.00239941178496455,-0.0336938721132427,0.0736041156896902));
#72758=CARTESIAN_POINT('',(0.00243448329139656,-0.0340203938281605,0.0733073832383692));
#72759=CARTESIAN_POINT('Origin',(0.018802680505642,-0.0345589643240237,
0.0764854429407088));
#72760=CARTESIAN_POINT('',(0.00243582716738048,-0.0341934961088739,0.0733075822738707));
#72761=CARTESIAN_POINT('Origin',(-0.0084647153816561,-0.0341934220717687,
0.0716931503575934));
#72762=CARTESIAN_POINT('',(0.002426670452976,-0.0341934961088841,0.0733694078719864));
#72763=CARTESIAN_POINT('Ctrl Pts',(0.00222754177036901,-0.0340223579322397,
0.073038987454037));
#72764=CARTESIAN_POINT('Ctrl Pts',(0.00221221800971782,-0.0339125849573575,
0.0731203119875072));
#72765=CARTESIAN_POINT('Ctrl Pts',(0.00219858824576653,-0.0338030433565231,
0.0732018965414073));
#72766=CARTESIAN_POINT('Ctrl Pts',(0.00218666066001375,-0.0336938721132326,
0.0732836352377335));
#72767=CARTESIAN_POINT('Ctrl Pts',(0.00229700612358545,-0.0340223579322397,
0.0731285189203635));
#72768=CARTESIAN_POINT('Ctrl Pts',(0.00228291723536276,-0.0339125849573575,
0.0732088853592322));
#72769=CARTESIAN_POINT('Ctrl Pts',(0.00227050164577749,-0.0338030433565231,
0.0732894869327829));
#72770=CARTESIAN_POINT('Ctrl Pts',(0.00225976609503748,-0.0336938721132326,
0.0733702191577206));
#72771=CARTESIAN_POINT('Ctrl Pts',(0.00236647047680189,-0.0340223579322397,
0.0732180503866899));
#72772=CARTESIAN_POINT('Ctrl Pts',(0.00235361646100771,-0.0339125849573575,
0.0732974587309572));
#72773=CARTESIAN_POINT('Ctrl Pts',(0.00234241504578844,-0.0338030433565231,
0.0733770773241585));
#72774=CARTESIAN_POINT('Ctrl Pts',(0.00233287153006121,-0.0336938721132326,
0.0734568030777077));
#72775=CARTESIAN_POINT('Ctrl Pts',(0.00243593483001833,-0.0340223579322397,
0.0733075818530164));
#72776=CARTESIAN_POINT('Ctrl Pts',(0.00242431568665266,-0.0339125849573575,
0.0733860321026821));
#72777=CARTESIAN_POINT('Ctrl Pts',(0.0024143284457994,-0.0338030433565231,
0.0734646677155342));
#72778=CARTESIAN_POINT('Ctrl Pts',(0.00240597696508495,-0.0336938721132326,
0.0735433869976948));
#72779=CARTESIAN_POINT('',(0.00229566451464686,-0.0336938721132427,0.0734127361865842));
#72780=CARTESIAN_POINT('Ctrl Pts',(0.0021885247798043,-0.0337108120662684,
0.0732709554169307));
#72781=CARTESIAN_POINT('Ctrl Pts',(0.00223106005550166,-0.033761140899443,
0.0732772551274719));
#72782=CARTESIAN_POINT('Ctrl Pts',(0.0022728191567851,-0.0338121088781593,
0.073283439882272));
#72783=CARTESIAN_POINT('Ctrl Pts',(0.00235482305235754,-0.033915338277323,
0.0732955851145971));
#72784=CARTESIAN_POINT('Ctrl Pts',(0.00239503315401185,-0.0339675558473116,
0.0733015404539501));
#72785=CARTESIAN_POINT('Ctrl Pts',(0.0024344832914352,-0.0340203938281304,
0.0733073832383803));
#72786=CARTESIAN_POINT('Ctrl Pts',(0.0024191424893604,-0.0341934961088741,
0.0734300249368031));
#72787=CARTESIAN_POINT('Ctrl Pts',(0.00240425757213368,-0.0340287516182428,
0.0735479638684953));
#72788=CARTESIAN_POINT('Ctrl Pts',(0.00239425987930614,-0.0338644633275951,
0.0736664172285476));
#72789=CARTESIAN_POINT('Ctrl Pts',(0.00241751373855163,-0.0341934961088741,
0.0734312334700822));
#72790=CARTESIAN_POINT('Ctrl Pts',(0.00240265380679836,-0.0340287516182428,
0.0735492060749143));
#72791=CARTESIAN_POINT('Ctrl Pts',(0.00239268246983108,-0.0338644633275951,
0.0736676920466647));
#72792=CARTESIAN_POINT('Ctrl Pts',(0.00214613252601321,-0.0341934961088741,
0.0736325983596118));
#72793=CARTESIAN_POINT('Ctrl Pts',(0.00213543565471333,-0.0340287516182428,
0.0737561815572157));
#72794=CARTESIAN_POINT('Ctrl Pts',(0.00212985571099966,-0.0338644633275951,
0.0738801012651471));
#72795=CARTESIAN_POINT('',(0.00214504098444017,-0.0341764758832386,0.0736453679059581));
#72796=CARTESIAN_POINT('',(0.00214613252601315,-0.034193496108874,0.0736325983596118));
#72797=CARTESIAN_POINT('Origin',(0.0186010544269866,-0.0345621026495323,
0.075548247761691));
#72798=CARTESIAN_POINT('Ctrl Pts',(0.00214504098543265,-0.034176475883747,
0.0736453679044303));
#72799=CARTESIAN_POINT('Ctrl Pts',(0.00218781327756581,-0.0341260050040171,
0.0736489780605097));
#72800=CARTESIAN_POINT('Ctrl Pts',(0.00222984208957002,-0.0340749269147647,
0.0736525254254876));
#72801=CARTESIAN_POINT('Ctrl Pts',(0.00231244531064647,-0.0339715436305273,
0.0736594975052568));
#72802=CARTESIAN_POINT('Ctrl Pts',(0.00235298838128689,-0.0339192778237525,
0.0736629195809504));
#72803=CARTESIAN_POINT('Ctrl Pts',(0.00239280147742893,-0.0338664212855041,
0.0736662799837048));
#72804=CARTESIAN_POINT('',(0.00228182313229235,-0.0341934961088841,0.0735319159148571));
#72805=CARTESIAN_POINT('Origin',(0.00812378219310841,-0.0315241814719618,
0.07415));
#72806=CARTESIAN_POINT('',(0.00214504098510271,-0.0342105180190538,0.0736453679068587));
#72807=CARTESIAN_POINT('',(0.0021439767196288,-0.0341934961088739,0.0736581397562618));
#72808=CARTESIAN_POINT('Origin',(0.0186100572327185,-0.0345621703323684,
0.0755038230687897));
#72809=CARTESIAN_POINT('Origin',(0.0186871976013945,-0.0345621039636221,
0.0745276772041862));
#72810=CARTESIAN_POINT('Origin',(0.0186886212027649,-0.034562171586023,
0.074572982011659));
#72811=CARTESIAN_POINT('Ctrl Pts',(0.00240479452811651,-0.0346945769586966,
0.0735403424402366));
#72812=CARTESIAN_POINT('Ctrl Pts',(0.00239202500643369,-0.0345275153362944,
0.0736601289266377));
#72813=CARTESIAN_POINT('Ctrl Pts',(0.00238301935663994,-0.0343603235965185,
0.073780347985663));
#72814=CARTESIAN_POINT('Ctrl Pts',(0.00237779892898214,-0.0341934961088739,
0.0739006436668402));
#72815=CARTESIAN_POINT('Ctrl Pts',(0.00239774369607375,-0.0346945769586966,
0.0736238787445202));
#72816=CARTESIAN_POINT('Ctrl Pts',(0.00238672387573027,-0.0345275153362944,
0.0737438129134213));
#72817=CARTESIAN_POINT('Ctrl Pts',(0.00237947302431693,-0.0343603235965185,
0.0738641246666484));
#72818=CARTESIAN_POINT('Ctrl Pts',(0.00237600729809141,-0.0341934961088739,
0.0739844578567164));
#72819=CARTESIAN_POINT('Ctrl Pts',(0.00239069286403098,-0.0346945769586966,
0.0737074150488039));
#72820=CARTESIAN_POINT('Ctrl Pts',(0.00238142274502685,-0.0345275153362944,
0.073827496900205));
#72821=CARTESIAN_POINT('Ctrl Pts',(0.00237592669199397,-0.0343603235965185,
0.0739479013476339));
#72822=CARTESIAN_POINT('Ctrl Pts',(0.0023742156672008,-0.0341934961088739,
0.074068272046593));
#72823=CARTESIAN_POINT('Ctrl Pts',(0.00238364203198824,-0.0346945769586966,
0.0737909513530872));
#72824=CARTESIAN_POINT('Ctrl Pts',(0.00237612161432341,-0.0345275153362944,
0.0739111808869886));
#72825=CARTESIAN_POINT('Ctrl Pts',(0.0023723803596709,-0.0343603235965185,
0.0740316780286192));
#72826=CARTESIAN_POINT('Ctrl Pts',(0.00237242403630996,-0.0341934961088739,
0.0741520862364687));
#72827=CARTESIAN_POINT('',(0.00238364203203939,-0.0346945769586966,0.0737909513524835));
#72828=CARTESIAN_POINT('',(0.00237373722912618,-0.0343667727831445,0.0740270857514938));
#72829=CARTESIAN_POINT('Origin',(0.0191748778417514,-0.0345626457064276,
0.0746579272563131));
#72830=CARTESIAN_POINT('Origin',(-0.00867591732885543,-0.0341934771028958,
0.0737908895859129));
#72831=CARTESIAN_POINT('',(0.00237776687175778,-0.034193496108874,0.0739021433341527));
#72832=CARTESIAN_POINT('',(0.00237643116290913,-0.0341934961088839,0.0739646290595874));
#72833=CARTESIAN_POINT('',(0.00239280147897343,-0.0345211942962709,0.0736662799838778));
#72834=CARTESIAN_POINT('Origin',(0.0191311264218782,-0.0345625596119205,
0.0751367556212441));
#72835=CARTESIAN_POINT('',(0.00239415520064965,-0.0346945769586885,0.073666394243946));
#72836=CARTESIAN_POINT('Origin',(-0.00863021209177555,-0.0346945685853906,
0.0727358884589146));
#72837=CARTESIAN_POINT('',(0.00238889861635452,-0.0346945769587025,0.0737286727982248));
#72838=CARTESIAN_POINT('Ctrl Pts',(0.00216941548056856,-0.0345231616327842,
0.073411408737782));
#72839=CARTESIAN_POINT('Ctrl Pts',(0.0021592350398722,-0.0344132092796988,
0.0734934812998365));
#72840=CARTESIAN_POINT('Ctrl Pts',(0.00215075273064796,-0.0343032738558979,
0.0735757602017098));
#72841=CARTESIAN_POINT('Ctrl Pts',(0.00214397671962875,-0.0341934961088739,
0.0736581397562618));
#72842=CARTESIAN_POINT('Ctrl Pts',(0.00224436437515982,-0.0345231616327842,
0.0734964016747713));
#72843=CARTESIAN_POINT('Ctrl Pts',(0.00223535544243938,-0.0344132092796988,
0.0735774411718335));
#72844=CARTESIAN_POINT('Ctrl Pts',(0.00222802321261212,-0.0343032738558979,
0.0736586628302974));
#72845=CARTESIAN_POINT('Ctrl Pts',(0.00222237441372113,-0.0341934961088739,
0.0737399623552154));
#72846=CARTESIAN_POINT('Ctrl Pts',(0.00231931326975108,-0.0345231616327842,
0.0735813946117606));
#72847=CARTESIAN_POINT('Ctrl Pts',(0.00231147584500655,-0.0344132092796988,
0.0736614010438304));
#72848=CARTESIAN_POINT('Ctrl Pts',(0.00230529369457628,-0.0343032738558979,
0.073741565458885));
#72849=CARTESIAN_POINT('Ctrl Pts',(0.00230077210781351,-0.0341934961088739,
0.0738217849541689));
#72850=CARTESIAN_POINT('Ctrl Pts',(0.00239426216434234,-0.0345231616327842,
0.0736663875487499));
#72851=CARTESIAN_POINT('Ctrl Pts',(0.00238759624757372,-0.0344132092796988,
0.0737453609158274));
#72852=CARTESIAN_POINT('Ctrl Pts',(0.00238256417654045,-0.0343032738558979,
0.0738244680874726));
#72853=CARTESIAN_POINT('Ctrl Pts',(0.00237916980190589,-0.0341934961088739,
0.0739036075531224));
#72854=CARTESIAN_POINT('',(0.00226087179570329,-0.0341934961088839,0.0737801415452172));
#72855=CARTESIAN_POINT('Ctrl Pts',(0.00214504098853992,-0.0342105180195387,
0.0736453679071444));
#72856=CARTESIAN_POINT('Ctrl Pts',(0.00218786136386767,-0.0342610556241353,
0.0736489821354375));
#72857=CARTESIAN_POINT('Ctrl Pts',(0.00222991334970009,-0.0343122189870262,
0.0736525315082725));
#72858=CARTESIAN_POINT('Ctrl Pts',(0.00231251740430272,-0.0344158119695188,
0.0736595036543358));
#72859=CARTESIAN_POINT('Ctrl Pts',(0.00235303568742227,-0.0344681990450085,
0.0736629235759062));
#72860=CARTESIAN_POINT('Ctrl Pts',(0.00239280147899817,-0.0345211942962524,
0.0736662799838758));
#72861=CARTESIAN_POINT('Ctrl Pts',(0.00238519130502,-0.0346945769586932,
0.0737896432542134));
#72862=CARTESIAN_POINT('Ctrl Pts',(0.00237774118428112,-0.034529677707698,
0.073908284560328));
#72863=CARTESIAN_POINT('Ctrl Pts',(0.00237520098378099,-0.034364806625142,
0.0740271324092652));
#72864=CARTESIAN_POINT('Ctrl Pts',(0.00238364203204002,-0.0346945769586932,
0.0737909513524745));
#72865=CARTESIAN_POINT('Ctrl Pts',(0.0023762189553071,-0.034529677707698,
0.0739096246887117));
#72866=CARTESIAN_POINT('Ctrl Pts',(0.00237370709953858,-0.0343648066251421,
0.0740285034226486));
#72867=CARTESIAN_POINT('Ctrl Pts',(0.0021254401343527,-0.0346945769586932,
0.0740089590617254));
#72868=CARTESIAN_POINT('Ctrl Pts',(0.00212252421275124,-0.034529677707698,
0.0741329705394995));
#72869=CARTESIAN_POINT('Ctrl Pts',(0.00212473629110149,-0.0343648066251421,
0.0742569965687347));
#72870=CARTESIAN_POINT('',(0.00212515255291101,-0.0346775396664972,0.0740217719488452));
#72871=CARTESIAN_POINT('',(0.00212544013436173,-0.0346945769586886,0.0740089590617211));
#72872=CARTESIAN_POINT('Origin',(0.0187255156885455,-0.0345626617235455,
0.0742238730028019));
#72873=CARTESIAN_POINT('Ctrl Pts',(0.00212515255389289,-0.0346775396670097,
0.0740217719473096));
#72874=CARTESIAN_POINT('Ctrl Pts',(0.00216810092722141,-0.0346269749928192,
0.0740226900084676));
#72875=CARTESIAN_POINT('Ctrl Pts',(0.00221028601288986,-0.0345757902890794,
0.0740235917177184));
#72876=CARTESIAN_POINT('Ctrl Pts',(0.00229316434710726,-0.0344721681088162,
0.0740253633473307));
#72877=CARTESIAN_POINT('Ctrl Pts',(0.00233382510333092,-0.0344197714290091,
0.0740262325787656));
#72878=CARTESIAN_POINT('Ctrl Pts',(0.00237373722902026,-0.0343667727830607,
0.0740270857512437));
#72879=CARTESIAN_POINT('',(0.00225454108321056,-0.0346945769587026,0.0738999552071123));
#72880=CARTESIAN_POINT('Origin',(0.00812378219310841,-0.0315241814719618,
0.07415));
#72881=CARTESIAN_POINT('',(0.00212515255407319,-0.0347116136489611,0.0740217719496091));
#72882=CARTESIAN_POINT('',(0.00212489233953384,-0.0346945769586885,0.0740345854224619));
#72883=CARTESIAN_POINT('Origin',(0.0187246164869726,-0.0345626683317801,
0.0741785687284629));
#72884=CARTESIAN_POINT('Origin',(0.0187189911031968,-0.0345626630395094,
0.0745292358347301));
#72885=CARTESIAN_POINT('Origin',(0.0187161510230357,-0.0345626693449426,
0.0745744605800943));
#72886=CARTESIAN_POINT('Ctrl Pts',(0.0023795055537286,-0.0352450361874067,
0.0738635588788241));
#72887=CARTESIAN_POINT('Ctrl Pts',(0.00236870224956947,-0.0349452760959492,
0.0740802078273224));
#72888=CARTESIAN_POINT('Ctrl Pts',(0.00237424852171626,-0.034644428984174,
0.0742970550480364));
#72889=CARTESIAN_POINT('Ctrl Pts',(0.00237943574741855,-0.0352450361874067,
0.0738660829137049));
#72890=CARTESIAN_POINT('Ctrl Pts',(0.00236872763879703,-0.0349452760959492,
0.0740827344949913));
#72891=CARTESIAN_POINT('Ctrl Pts',(0.0023743690343533,-0.034644428984174,
0.0742995771704966));
#72892=CARTESIAN_POINT('Ctrl Pts',(0.0023725242315717,-0.0352450361874067,
0.0741159873573403));
#72893=CARTESIAN_POINT('Ctrl Pts',(0.00237124142370388,-0.0349452760959492,
0.0743328996107243));
#72894=CARTESIAN_POINT('Ctrl Pts',(0.00238630097861556,-0.034644428984174,
0.0745492922655673));
#72895=CARTESIAN_POINT('Ctrl Pts',(0.00237245511641323,-0.0352450361874067,
0.0741184864017767));
#72896=CARTESIAN_POINT('Ctrl Pts',(0.00237126656155295,-0.0349452760959492,
0.0743354012618816));
#72897=CARTESIAN_POINT('Ctrl Pts',(0.00238642029805818,-0.034644428984174,
0.074551789416518));
#72898=CARTESIAN_POINT('',(0.00237242165110434,-0.0351951634053262,0.0741520538780395));
#72899=CARTESIAN_POINT('',(0.00237736577994594,-0.0348678972935461,0.0743883766056446));
#72900=CARTESIAN_POINT('Origin',(0.0190945965440124,-0.0345636767883521,
0.0732726431573248));
#72901=CARTESIAN_POINT('Origin',(-0.00866297998397881,-0.0346946199326802,
0.0748463754880312));
#72902=CARTESIAN_POINT('',(0.00237354227144593,-0.0346945769330288,0.0742634276919279));
#72903=CARTESIAN_POINT('',(0.00237613270947176,-0.0346945769458128,0.0743258739946087));
#72904=CARTESIAN_POINT('',(0.00237373722915741,-0.0350221583435276,0.0740270857512628));
#72905=CARTESIAN_POINT('Origin',(0.0191558972229172,-0.0345628458717777,
0.0737494928402475));
#72906=CARTESIAN_POINT('',(0.00237497389593432,-0.035195136029876,0.0740271091612433));
#72907=CARTESIAN_POINT('Origin',(-0.00864148601942892,-0.0351951838366824,
0.0737916207221787));
#72908=CARTESIAN_POINT('',(0.00237242403620701,-0.035195137132875,0.0741520862358497));
#72909=CARTESIAN_POINT('Ctrl Pts',(0.00213478847589137,-0.0350241211494343,
0.073786744917223));
#72910=CARTESIAN_POINT('Ctrl Pts',(0.0021297847860665,-0.0349144232818962,
0.0738692408500946));
#72911=CARTESIAN_POINT('Ctrl Pts',(0.00212648335117296,-0.0348045283579412,
0.0739518895906026));
#72912=CARTESIAN_POINT('Ctrl Pts',(0.00212489233932004,-0.0346945769439157,
0.0740345854335728));
#72913=CARTESIAN_POINT('Ctrl Pts',(0.00221492625713316,-0.0350241211494343,
0.0738668640648758));
#72914=CARTESIAN_POINT('Ctrl Pts',(0.00221102617571708,-0.0349144232818962,
0.0739482561326685));
#72915=CARTESIAN_POINT('Ctrl Pts',(0.0022088061921152,-0.0348045283579412,
0.0740297775350068));
#72916=CARTESIAN_POINT('Ctrl Pts',(0.00220827303550138,-0.0346945769439157,
0.0741113239591468));
#72917=CARTESIAN_POINT('Ctrl Pts',(0.00229506403837495,-0.0350241211494343,
0.0739469832125286));
#72918=CARTESIAN_POINT('Ctrl Pts',(0.00229226756536765,-0.0349144232818962,
0.0740272714152425));
#72919=CARTESIAN_POINT('Ctrl Pts',(0.00229112903305743,-0.0348045283579412,
0.0741076654794111));
#72920=CARTESIAN_POINT('Ctrl Pts',(0.00229165373168272,-0.0346945769439157,
0.0741880624847209));
#72921=CARTESIAN_POINT('Ctrl Pts',(0.00237520181961674,-0.0350241211494343,
0.0740271023601814));
#72922=CARTESIAN_POINT('Ctrl Pts',(0.00237350895501823,-0.0349144232818962,
0.0741062866978165));
#72923=CARTESIAN_POINT('Ctrl Pts',(0.00237345187399967,-0.0348045283579412,
0.0741855534238153));
#72924=CARTESIAN_POINT('Ctrl Pts',(0.00237503442786406,-0.0346945769439157,
0.0742648010102949));
#72925=CARTESIAN_POINT('',(0.00224921730540605,-0.0346945769458128,0.0741490065569093));
#72926=CARTESIAN_POINT('Ctrl Pts',(0.0021251525573556,-0.0347116136492792,
0.0740217719496746));
#72927=CARTESIAN_POINT('Ctrl Pts',(0.00216808387467062,-0.034762154653234,
0.0740226896591267));
#72928=CARTESIAN_POINT('Ctrl Pts',(0.00221026034341442,-0.0348133084097118,
0.0740235912327669));
#72929=CARTESIAN_POINT('Ctrl Pts',(0.00229313878288501,-0.0349168561544567,
0.0740253628608474));
#72930=CARTESIAN_POINT('Ctrl Pts',(0.00233380787995237,-0.0349692089015909,
0.0740262322125731));
#72931=CARTESIAN_POINT('Ctrl Pts',(0.00237373722919349,-0.0350221583435001,
0.0740270857512836));
#72932=CARTESIAN_POINT('Ctrl Pts',(0.00237348041836607,-0.0351951371254872,
0.0741510740715169));
#72933=CARTESIAN_POINT('Ctrl Pts',(0.00237350262412072,-0.0350307338985332,
0.0742699579525277));
#72934=CARTESIAN_POINT('Ctrl Pts',(0.00237843840996862,-0.0348659306906667,
0.0743887393301731));
#72935=CARTESIAN_POINT('Ctrl Pts',(0.00237242403632317,-0.0351951371254872,
0.0741520862358493));
#72936=CARTESIAN_POINT('Ctrl Pts',(0.00237246716794029,-0.0350307338985332,
0.0742709919568959));
#72937=CARTESIAN_POINT('Ctrl Pts',(0.00237742476444186,-0.0348659306906667,
0.0743897942910266));
#72938=CARTESIAN_POINT('Ctrl Pts',(0.00219537330481443,-0.0351951371254872,
0.0743217260329856));
#72939=CARTESIAN_POINT('Ctrl Pts',(0.00219892363279228,-0.0350307338985332,
0.0744442921668109));
#72940=CARTESIAN_POINT('Ctrl Pts',(0.00220753671758532,-0.0348659306906667,
0.0745666068297094));
#72941=CARTESIAN_POINT('Origin',(-0.00293624707561006,-0.0308609188508701,
0.0746088010768252));
#72942=CARTESIAN_POINT('',(0.00229523390934874,-0.0351951371254872,0.0742260453625317));
#72943=CARTESIAN_POINT('Origin',(0.00908388395447356,-0.0351840467441202,
0.0739684779432064));
#72944=CARTESIAN_POINT('Origin',(-0.00377189715848901,-0.0352322613739614,
0.0754388458336736));
#72945=CARTESIAN_POINT('',(0.00239206408775232,-0.0351951142564655,0.0746245757517679));
#72946=CARTESIAN_POINT('',(0.00240502397038673,-0.0351951372916786,0.0747485853239551));
#72947=CARTESIAN_POINT('Origin',(0.00833153237709209,-0.0352875121341927,
0.0744198901674271));
#72948=CARTESIAN_POINT('Origin',(0.00878592006143388,-0.0298325076522275,
0.066676261730273));
#72949=CARTESIAN_POINT('Origin',(7.23359568405449E-5,-0.0338731629816332,
0.0718204020753387));
#72950=CARTESIAN_POINT('Ctrl Pts',(0.00320793794572019,-0.0321934096636941,
0.0711646003482395));
#72951=CARTESIAN_POINT('Ctrl Pts',(0.00315450071357742,-0.0320508460843131,
0.0712525916193816));
#72952=CARTESIAN_POINT('Ctrl Pts',(0.00310346792512061,-0.0319086045660688,
0.0713419522978032));
#72953=CARTESIAN_POINT('Ctrl Pts',(0.00305493362259791,-0.0317669892864341,
0.0714324809280297));
#72954=CARTESIAN_POINT('Ctrl Pts',(0.00316598295920628,-0.0321934096636941,
0.0712371965722084));
#72955=CARTESIAN_POINT('Ctrl Pts',(0.0031138451649028,-0.0320508460843131,
0.0713259388176304));
#72956=CARTESIAN_POINT('Ctrl Pts',(0.00306413101170198,-0.0319086045660688,
0.0714160149907642));
#72957=CARTESIAN_POINT('Ctrl Pts',(0.00301693157576772,-0.0317669892864341,
0.0715072223292938));
#72958=CARTESIAN_POINT('Ctrl Pts',(0.00312402797269236,-0.0321934096636941,
0.0713097927961771));
#72959=CARTESIAN_POINT('Ctrl Pts',(0.00307318961622818,-0.0320508460843131,
0.0713992860158791));
#72960=CARTESIAN_POINT('Ctrl Pts',(0.00302479409828335,-0.0319086045660688,
0.071490077683725));
#72961=CARTESIAN_POINT('Ctrl Pts',(0.00297892952893754,-0.0317669892864341,
0.0715819637305579));
#72962=CARTESIAN_POINT('Ctrl Pts',(0.00308207298617844,-0.0321934096636941,
0.0713823890201459));
#72963=CARTESIAN_POINT('Ctrl Pts',(0.00303253406755356,-0.0320508460843131,
0.0714726332141279));
#72964=CARTESIAN_POINT('Ctrl Pts',(0.00298545718486472,-0.0319086045660688,
0.0715641403766859));
#72965=CARTESIAN_POINT('Ctrl Pts',(0.00294092748210736,-0.0317669892864341,
0.0716567051318221));
#72966=CARTESIAN_POINT('',(0.00308282356917989,-0.0321934096636941,0.0713810902593544));
#72967=CARTESIAN_POINT('',(0.00297332029942594,-0.0318665617511259,0.0715905337918369));
#72968=CARTESIAN_POINT('Origin',(0.0174226902661654,-0.0326371944421278,
0.0799593259731346));
#72969=CARTESIAN_POINT('Origin',(-0.00684265072727457,-0.0316939261509315,
0.0667125933533414));
#72970=CARTESIAN_POINT('',(0.00314410192199668,-0.0320197221621831,0.071272436175507));
#72971=CARTESIAN_POINT('Ctrl Pts',(0.00314397158350144,-0.0320197392094748,
0.0712725674262431));
#72972=CARTESIAN_POINT('Ctrl Pts',(0.00312933032213814,-0.0319792716576045,
0.0712979063270771));
#72973=CARTESIAN_POINT('Ctrl Pts',(0.00311481558176056,-0.0319386439829683,
0.0713234721993179));
#72974=CARTESIAN_POINT('Ctrl Pts',(0.00310041947948218,-0.0318979099381615,
0.0713492960579256));
#72975=CARTESIAN_POINT('Ctrl Pts',(0.00308602366175272,-0.0318571766984912,
0.071375119406107));
#72976=CARTESIAN_POINT('Ctrl Pts',(0.00307181809017675,-0.0318163871833557,
0.0714010686117907));
#72977=CARTESIAN_POINT('Ctrl Pts',(0.00305784853744171,-0.0317755399638303,
0.0714270527295668));
#72978=CARTESIAN_POINT('',(0.00314537000600163,-0.0321934096636183,0.0712728639074129));
#72979=CARTESIAN_POINT('Origin',(0.00113569280887835,-0.0324113643887189,
0.0701357262204479));
#72980=CARTESIAN_POINT('',(0.00311409678760076,-0.0321934096636663,0.0713269770833937));
#72981=CARTESIAN_POINT('Ctrl Pts',(0.00308478290689466,-0.0321934096636618,
0.071380566157171));
#72982=CARTESIAN_POINT('Ctrl Pts',(0.00304659025583153,-0.0320835708272592,
0.0714500578844942));
#72983=CARTESIAN_POINT('Ctrl Pts',(0.00300985788574346,-0.0319739230346488,
0.0715202996987203));
#72984=CARTESIAN_POINT('Ctrl Pts',(0.00297462589591431,-0.0318646057455572,
0.0715911981234695));
#72985=CARTESIAN_POINT('Ctrl Pts',(0.00297531271766522,-0.0321934096636618,
0.0714098482751716));
#72986=CARTESIAN_POINT('Ctrl Pts',(0.00293752388983048,-0.0320835708272592,
0.0714808496817204));
#72987=CARTESIAN_POINT('Ctrl Pts',(0.00290122635147,-0.0319739230346488,
0.0715525919423959));
#72988=CARTESIAN_POINT('Ctrl Pts',(0.00286645949819773,-0.0318646057455572,
0.0716249797037988));
#72989=CARTESIAN_POINT('Ctrl Pts',(0.00286584252843579,-0.0321934096636618,
0.0714391303931721));
#72990=CARTESIAN_POINT('Ctrl Pts',(0.00282845752382942,-0.0320835708272592,
0.0715116414789465));
#72991=CARTESIAN_POINT('Ctrl Pts',(0.00279259481719655,-0.0319739230346488,
0.0715848841860716));
#72992=CARTESIAN_POINT('Ctrl Pts',(0.00275829310048115,-0.0318646057455572,
0.0716587612841281));
#72993=CARTESIAN_POINT('Ctrl Pts',(0.00275637233920636,-0.0321934096636618,
0.0714684125111727));
#72994=CARTESIAN_POINT('Ctrl Pts',(0.00271939115782836,-0.0320835708272592,
0.0715424332761726));
#72995=CARTESIAN_POINT('Ctrl Pts',(0.00268396328292309,-0.0319739230346488,
0.0716171764297472));
#72996=CARTESIAN_POINT('Ctrl Pts',(0.00265012670276457,-0.0318646057455572,
0.0716925428644575));
#72997=CARTESIAN_POINT('',(0.00275065666655781,-0.0321763980308258,0.0714798835131076));
#72998=CARTESIAN_POINT('',(0.00275637233919176,-0.0321934096636184,0.0714684125112019));
#72999=CARTESIAN_POINT('Origin',(0.0172862519340763,-0.032638623111625,
0.0793882690510444));
#73000=CARTESIAN_POINT('Ctrl Pts',(0.00275065666939444,-0.0321763980306269,
0.0714798835145151));
#73001=CARTESIAN_POINT('Ctrl Pts',(0.00278909143633438,-0.0321259596175033,
0.0714989832553213));
#73002=CARTESIAN_POINT('Ctrl Pts',(0.00282686027106803,-0.0320749164631834,
0.0715177520683285));
#73003=CARTESIAN_POINT('Ctrl Pts',(0.0029010964713076,-0.0319716057793887,
0.0715546429433331));
#73004=CARTESIAN_POINT('Ctrl Pts',(0.00293753491184741,-0.0319193786690067,
0.0715727506313821));
#73005=CARTESIAN_POINT('Ctrl Pts',(0.00297332030108458,-0.031866561752526,
0.0715905337926576));
#73006=CARTESIAN_POINT('',(0.00291959795419583,-0.0321934096636663,0.0714247513852882));
#73007=CARTESIAN_POINT('Origin',(0.00812378219310841,-0.0315241814719618,
0.07415));
#73008=CARTESIAN_POINT('',(0.00275065666622462,-0.0322104233323614,0.0714798835129422));
#73009=CARTESIAN_POINT('',(0.00274496550589061,-0.0321934096636183,0.0714913666959626));
#73010=CARTESIAN_POINT('Origin',(0.0173118880729296,-0.0326387230595964,
0.0793508786892778));
#73011=CARTESIAN_POINT('Origin',(0.0178322963308996,-0.0326386244950934,
0.0782894597796565));
#73012=CARTESIAN_POINT('Origin',(0.0178179710295711,-0.0326387241904305,
0.0783324713134188));
#73013=CARTESIAN_POINT('Ctrl Pts',(0.00304704941301366,-0.0327445246967097,
0.0714472404325372));
#73014=CARTESIAN_POINT('Ctrl Pts',(0.00294511316949499,-0.032443687833936,
0.0716387125394833));
#73015=CARTESIAN_POINT('Ctrl Pts',(0.00285788897772951,-0.0321434074405927,
0.0718373189488763));
#73016=CARTESIAN_POINT('Ctrl Pts',(0.00293438979343578,-0.0327445246967097,
0.07167041706688));
#73017=CARTESIAN_POINT('Ctrl Pts',(0.00284087079428464,-0.032443687833936,
0.0718661382008406));
#73018=CARTESIAN_POINT('Ctrl Pts',(0.00276235998846516,-0.0321434074405927,
0.0720683475449638));
#73019=CARTESIAN_POINT('',(0.00291890946840458,-0.0326943950436612,0.0717030784811042));
#73020=CARTESIAN_POINT('',(0.00282277334565379,-0.0323666188837389,0.0719189844914907));
#73021=CARTESIAN_POINT('Origin',(0.0181646907621997,-0.0326395579109636,
0.0787864541573588));
#73022=CARTESIAN_POINT('Origin',(-0.00735700719535952,-0.0321933825603006,
0.0676346595754701));
#73023=CARTESIAN_POINT('',(0.00287251438693947,-0.0321934096532689,0.0718042993744971));
#73024=CARTESIAN_POINT('',(0.00284826994513973,-0.0321934096584275,0.0718619054278915));
#73025=CARTESIAN_POINT('',(0.00297332029857321,-0.0325210109756239,0.0715905337914046));
#73026=CARTESIAN_POINT('Origin',(0.0179374475416283,-0.0326393129159266,
0.0792101816038873));
#73027=CARTESIAN_POINT('',(0.00297453689523271,-0.0326943950436593,0.0715911383659319));
#73028=CARTESIAN_POINT('Origin',(-0.00693212286675309,-0.0326943765538135,
0.0666681302351314));
#73029=CARTESIAN_POINT('',(0.00294672318182864,-0.0326943950436702,0.0716471084235281));
#73030=CARTESIAN_POINT('Ctrl Pts',(0.00285944568442008,-0.0325229783203769,
0.0712713264993541));
#73031=CARTESIAN_POINT('Ctrl Pts',(0.00281976323316612,-0.032413025309245,
0.071343895263003));
#73032=CARTESIAN_POINT('Ctrl Pts',(0.00278158797863065,-0.032303122220807,
0.0714172739026568));
#73033=CARTESIAN_POINT('Ctrl Pts',(0.00274496550390364,-0.0321934096576658,
0.0714913666999825));
#73034=CARTESIAN_POINT('Ctrl Pts',(0.00289784342383241,-0.0325229783203769,
0.0713779414881895));
#73035=CARTESIAN_POINT('Ctrl Pts',(0.00285963065786802,-0.032413025309245,
0.0714499809398402));
#73036=CARTESIAN_POINT('Ctrl Pts',(0.00282291391621693,-0.032303122220807,
0.0715227999454484));
#73037=CARTESIAN_POINT('Ctrl Pts',(0.00278773693901311,-0.0321934096576658,
0.0715963035694566));
#73038=CARTESIAN_POINT('Ctrl Pts',(0.00293624116324473,-0.0325229783203769,
0.0714845564770249));
#73039=CARTESIAN_POINT('Ctrl Pts',(0.00289949808256992,-0.032413025309245,
0.0715560666166775));
#73040=CARTESIAN_POINT('Ctrl Pts',(0.00286423985380321,-0.032303122220807,
0.0716283259882399));
#73041=CARTESIAN_POINT('Ctrl Pts',(0.00283050837412259,-0.0321934096576658,
0.0717012404389307));
#73042=CARTESIAN_POINT('Ctrl Pts',(0.00297463890265705,-0.0325229783203769,
0.0715911714658602));
#73043=CARTESIAN_POINT('Ctrl Pts',(0.00293936550727183,-0.032413025309245,
0.0716621522935148));
#73044=CARTESIAN_POINT('Ctrl Pts',(0.0029055657913895,-0.032303122220807,
0.0717338520310315));
#73045=CARTESIAN_POINT('Ctrl Pts',(0.00287327980923206,-0.0321934096576658,
0.0718061773084048));
#73046=CARTESIAN_POINT('',(0.00280873994649101,-0.0321934096584275,0.0716478330347288));
#73047=CARTESIAN_POINT('Ctrl Pts',(0.00275065666933405,-0.0322104233328926,
0.071479883514485));
#73048=CARTESIAN_POINT('Ctrl Pts',(0.00278914351602082,-0.0322609421831371,
0.0714990091357568));
#73049=CARTESIAN_POINT('Ctrl Pts',(0.00282693779257923,-0.0323120888240734,
0.0715177905918107));
#73050=CARTESIAN_POINT('Ctrl Pts',(0.0029011745548487,-0.0324156524631814,
0.07155468174611));
#73051=CARTESIAN_POINT('Ctrl Pts',(0.00293758652535974,-0.0324680267167317,
0.0715727762801575));
#73052=CARTESIAN_POINT('Ctrl Pts',(0.00297332029861009,-0.0325210109755912,
0.0715905337914279));
#73053=CARTESIAN_POINT('Origin',(0.0124482184734131,-0.0262834582512208,
0.0675771287327571));
#73054=CARTESIAN_POINT('Origin',(0.000806663783453315,-0.0342770697900545,
0.0644400878420418));
#73055=CARTESIAN_POINT('Ctrl Pts',(0.00292083156457773,-0.0326943950436604,
0.071702432542149));
#73056=CARTESIAN_POINT('Ctrl Pts',(0.00288709949777823,-0.0325844576448134,
0.0717741389531789));
#73057=CARTESIAN_POINT('Ctrl Pts',(0.00285484804985231,-0.0324744968375323,
0.0718465480734288));
#73058=CARTESIAN_POINT('Ctrl Pts',(0.00282411726359269,-0.0323646534831895,
0.0719195665581506));
#73059=CARTESIAN_POINT('Ctrl Pts',(0.00281341618468038,-0.0326943950436604,
0.0717385305163707));
#73060=CARTESIAN_POINT('Ctrl Pts',(0.00278018161562046,-0.0325844576448134,
0.0718117173126535));
#73061=CARTESIAN_POINT('Ctrl Pts',(0.00274845831743698,-0.0324744968375323,
0.0718855966338565));
#73062=CARTESIAN_POINT('Ctrl Pts',(0.0027182856302444,-0.0323646534831895,
0.0719600732608581));
#73063=CARTESIAN_POINT('Ctrl Pts',(0.00270600080478302,-0.0326943950436604,
0.0717746284905924));
#73064=CARTESIAN_POINT('Ctrl Pts',(0.00267326373346269,-0.0325844576448134,
0.0718492956721281));
#73065=CARTESIAN_POINT('Ctrl Pts',(0.00264206858502164,-0.0324744968375323,
0.0719246451942843));
#73066=CARTESIAN_POINT('Ctrl Pts',(0.0026124539968961,-0.0323646534831895,
0.0720005799635657));
#73067=CARTESIAN_POINT('Ctrl Pts',(0.00259858542488566,-0.0326943950436604,
0.0718107264648142));
#73068=CARTESIAN_POINT('Ctrl Pts',(0.00256634585130493,-0.0325844576448134,
0.0718868740316027));
#73069=CARTESIAN_POINT('Ctrl Pts',(0.00253567885260631,-0.0324744968375323,
0.0719636937547119));
#73070=CARTESIAN_POINT('Ctrl Pts',(0.0025066223635478,-0.0323646534831895,
0.0720410866662732));
#73071=CARTESIAN_POINT('',(0.00259360130080664,-0.032677355999133,0.0718225337212939));
#73072=CARTESIAN_POINT('',(0.00259858542488537,-0.0326943950436594,0.0718107264648148));
#73073=CARTESIAN_POINT('Origin',(0.0179179980259199,-0.0326395670272396,
0.0782175454982723));
#73074=CARTESIAN_POINT('Ctrl Pts',(0.00259360130389114,-0.0326773559987412,
0.0718225337225895));
#73075=CARTESIAN_POINT('Ctrl Pts',(0.00263319134500798,-0.0326267922586193,
0.0718391958331907));
#73076=CARTESIAN_POINT('Ctrl Pts',(0.00267207968123486,-0.032575610957982,
0.0718555626199136));
#73077=CARTESIAN_POINT('Ctrl Pts',(0.00274848603988036,-0.0324719985462361,
0.0718877194745789));
#73078=CARTESIAN_POINT('Ctrl Pts',(0.00278597341774083,-0.0324196091621768,
0.0719034966452622));
#73079=CARTESIAN_POINT('Ctrl Pts',(0.00282277334569873,-0.0323666188837757,
0.0719189844915097));
#73080=CARTESIAN_POINT('',(0.00275874744665497,-0.0326943950436703,0.0717569024729695));
#73081=CARTESIAN_POINT('Origin',(0.00812378219310841,-0.0315241814719618,
0.07415));
#73082=CARTESIAN_POINT('',(0.00259360130084671,-0.0327114338380053,0.0718225337213109));
#73083=CARTESIAN_POINT('',(0.00258864240555084,-0.0326943950436593,0.071834351595725));
#73084=CARTESIAN_POINT('Origin',(0.0179348591208374,-0.0326395665215589,
0.078175488213683));
#73085=CARTESIAN_POINT('Origin',(0.0178790229887526,-0.0326395681402186,
0.0783101586361176));
#73086=CARTESIAN_POINT('Origin',(0.0178607309245503,-0.0326395676290809,
0.0783516136817013));
#73087=CARTESIAN_POINT('Ctrl Pts',(0.00288734328600302,-0.0332451089994434,
0.0717713801118816));
#73088=CARTESIAN_POINT('Ctrl Pts',(0.00279763216917186,-0.0329451141710254,
0.071968875636459));
#73089=CARTESIAN_POINT('Ctrl Pts',(0.00272305208243469,-0.0326442513127493,
0.0721725675051566));
#73090=CARTESIAN_POINT('Ctrl Pts',(0.00278892091855253,-0.0332451089994434,
0.0720011909853959));
#73091=CARTESIAN_POINT('Ctrl Pts',(0.00270787726062302,-0.0329451141710254,
0.0722023985702943));
#73092=CARTESIAN_POINT('Ctrl Pts',(0.00264221961700992,-0.0326442513127493,
0.0724091390853039));
#73093=CARTESIAN_POINT('',(0.00277553662236751,-0.0331951640388616,0.0720347235842445));
#73094=CARTESIAN_POINT('',(0.0026931470528567,-0.0328677532092642,0.0722562399905309));
#73095=CARTESIAN_POINT('Origin',(0.0186306846361962,-0.0326401908901966,
0.0774795677200636));
#73096=CARTESIAN_POINT('Origin',(-0.00774627647633802,-0.0326944279134284,
0.0686158263327017));
#73097=CARTESIAN_POINT('',(0.00273558880092205,-0.0326943950436593,0.0721386579186026));
#73098=CARTESIAN_POINT('',(0.00271500931525608,-0.0326943950436693,0.0721976726182163));
#73099=CARTESIAN_POINT('',(0.00282277334565488,-0.0330220786163545,0.0719189844914881));
#73100=CARTESIAN_POINT('Origin',(0.0185023456661935,-0.0326396682763639,
0.0779430350420078));
#73101=CARTESIAN_POINT('',(0.0028240255031881,-0.0331951640388588,0.0719195114822879));
#73102=CARTESIAN_POINT('Origin',(-0.00734381359202158,-0.033195202656006,
0.0676402104103637));
#73103=CARTESIAN_POINT('',(0.0027997810627878,-0.0331951640388701,0.0719771175332762));
#73104=CARTESIAN_POINT('Ctrl Pts',(0.00268907983816847,-0.0330240426238172,
0.0716075581986534));
#73105=CARTESIAN_POINT('Ctrl Pts',(0.00265405522537389,-0.0329142774063519,
0.0716824265183666));
#73106=CARTESIAN_POINT('Ctrl Pts',(0.0026205608888353,-0.0328043479726691,
0.0717580562192506));
#73107=CARTESIAN_POINT('Ctrl Pts',(0.00258864240555083,-0.0326943950436593,
0.0718343515957249));
#73108=CARTESIAN_POINT('Ctrl Pts',(0.00273409622464781,-0.0330240426238172,
0.0717115517606312));
#73109=CARTESIAN_POINT('Ctrl Pts',(0.00270050422448549,-0.0329142774063519,
0.0717857999357634));
#73110=CARTESIAN_POINT('Ctrl Pts',(0.00266843039466803,-0.0328043479726691,
0.0718607795667967));
#73111=CARTESIAN_POINT('Ctrl Pts',(0.00263791846948381,-0.0326943950436593,
0.0719363957308223));
#73112=CARTESIAN_POINT('Ctrl Pts',(0.00277911261112714,-0.0330240426238172,
0.071815545322609));
#73113=CARTESIAN_POINT('Ctrl Pts',(0.00274695322359709,-0.0329142774063519,
0.0718891733531601));
#73114=CARTESIAN_POINT('Ctrl Pts',(0.00271629990050076,-0.0328043479726691,
0.0719635029143427));
#73115=CARTESIAN_POINT('Ctrl Pts',(0.0026871945334168,-0.0326943950436593,
0.0720384398659197));
#73116=CARTESIAN_POINT('Ctrl Pts',(0.00282412899760648,-0.0330240426238172,
0.0719195388845869));
#73117=CARTESIAN_POINT('Ctrl Pts',(0.00279340222270869,-0.0329142774063519,
0.0719925467705569));
#73118=CARTESIAN_POINT('Ctrl Pts',(0.00276416940633348,-0.0328043479726691,
0.0720662262618888));
#73119=CARTESIAN_POINT('Ctrl Pts',(0.00273647059734978,-0.0326943950436593,
0.072140484001017));
#73120=CARTESIAN_POINT('',(0.00266211560324645,-0.0326943950436693,0.0719865047571738));
#73121=CARTESIAN_POINT('Ctrl Pts',(0.00259360130389673,-0.0327114338383323,
0.0718225337225918));
#73122=CARTESIAN_POINT('Ctrl Pts',(0.00263318475991938,-0.0327619876831079,
0.0718391930617494));
#73123=CARTESIAN_POINT('Ctrl Pts',(0.00267206987969294,-0.0328131562604566,
0.0718555584947757));
#73124=CARTESIAN_POINT('Ctrl Pts',(0.00274847616811621,-0.0329167375858769,
0.0718877153198868));
#73125=CARTESIAN_POINT('Ctrl Pts',(0.0027859668925906,-0.032969108892062,
0.0719034938990468));
#73126=CARTESIAN_POINT('Ctrl Pts',(0.00282277334569761,-0.0330220786163187,
0.0719189844915091));
#73127=CARTESIAN_POINT('Ctrl Pts',(0.00277741466668486,-0.0331951640388604,
0.0720339581082862));
#73128=CARTESIAN_POINT('Ctrl Pts',(0.00274827046695098,-0.0330855618127442,
0.072107593513923));
#73129=CARTESIAN_POINT('Ctrl Pts',(0.00272062717571139,-0.0329757224171941,
0.0721818843631614));
#73130=CARTESIAN_POINT('Ctrl Pts',(0.00269452485838531,-0.0328657861694599,
0.0722567372584769));
#73131=CARTESIAN_POINT('Ctrl Pts',(0.00267247775712366,-0.0331951640388604,
0.0720767295596433));
#73132=CARTESIAN_POINT('Ctrl Pts',(0.00264392264767487,-0.0330855618127442,
0.072151810259092));
#73133=CARTESIAN_POINT('Ctrl Pts',(0.00261689874314343,-0.0329757224171941,
0.0722275352685439));
#73134=CARTESIAN_POINT('Ctrl Pts',(0.00259144540587207,-0.0328657861694599,
0.0723038093150394));
#73135=CARTESIAN_POINT('Ctrl Pts',(0.00256754084756247,-0.0331951640388604,
0.0721195010110005));
#73136=CARTESIAN_POINT('Ctrl Pts',(0.00253957482839877,-0.0330855618127442,
0.072196027004261));
#73137=CARTESIAN_POINT('Ctrl Pts',(0.00251317031057548,-0.0329757224171941,
0.0722731861739263));
#73138=CARTESIAN_POINT('Ctrl Pts',(0.00248836595335883,-0.0328657861694599,
0.0723508813716019));
#73139=CARTESIAN_POINT('Ctrl Pts',(0.00246260393800127,-0.0331951640388604,
0.0721622724623576));
#73140=CARTESIAN_POINT('Ctrl Pts',(0.00243522700912267,-0.0330855618127442,
0.07224024374943));
#73141=CARTESIAN_POINT('Ctrl Pts',(0.00240944187800752,-0.0329757224171941,
0.0723188370793087));
#73142=CARTESIAN_POINT('Ctrl Pts',(0.00238528650084559,-0.0328657861694599,
0.0723979534281644));
#73143=CARTESIAN_POINT('',(0.00245837103251906,-0.0331781648278993,0.0721743693755846));
#73144=CARTESIAN_POINT('',(0.00246260393800087,-0.0331951640388588,0.0721622724623588));
#73145=CARTESIAN_POINT('Origin',(0.0182793365849877,-0.0326412091099719,
0.0769370925964116));
#73146=CARTESIAN_POINT('Ctrl Pts',(0.00245837103582962,-0.0331781648273345,
0.0721743693767361));
#73147=CARTESIAN_POINT('Ctrl Pts',(0.00249895721972424,-0.0331276810207545,
0.0721885225080019));
#73148=CARTESIAN_POINT('Ctrl Pts',(0.00253881023828218,-0.0330765665169234,
0.0722024199713469));
#73149=CARTESIAN_POINT('Ctrl Pts',(0.00261708542752709,-0.0329730612715178,
0.0722297159356858));
#73150=CARTESIAN_POINT('Ctrl Pts',(0.0026554751898153,-0.0329207135598908,
0.0722431031352889));
#73151=CARTESIAN_POINT('Ctrl Pts',(0.00269314705289973,-0.0328677532092986,
0.072256239990546));
#73152=CARTESIAN_POINT('',(0.00261907028019419,-0.0331951640388702,0.0720984980233116));
#73153=CARTESIAN_POINT('Origin',(0.00812378219310841,-0.0315241814719618,
0.07415));
#73154=CARTESIAN_POINT('',(0.00245837103295193,-0.0332121607144419,0.0721743693757357));
#73155=CARTESIAN_POINT('',(0.00245416397318748,-0.0331951640388587,0.0721864753018193));
#73156=CARTESIAN_POINT('Origin',(0.0182866392920863,-0.0326413646240691,
0.0768923383319838));
#73157=CARTESIAN_POINT('Origin',(0.0178102809754642,-0.0326412100744096,
0.0782821863608264));
#73158=CARTESIAN_POINT('Origin',(0.0177881662202434,-0.0326413658440793,
0.0783217750389539));
#73159=CARTESIAN_POINT('Ctrl Pts',(0.00274832883103548,-0.0337436976235975,
0.0721048530243088));
#73160=CARTESIAN_POINT('Ctrl Pts',(0.00272993446918561,-0.0336723290703325,
0.0721532006665195));
#73161=CARTESIAN_POINT('Ctrl Pts',(0.00271241270480488,-0.033601104548885,
0.0722018713438128));
#73162=CARTESIAN_POINT('Ctrl Pts',(0.00265646918200321,-0.0333736987606857,
0.0723572671752923));
#73163=CARTESIAN_POINT('Ctrl Pts',(0.00260953535851614,-0.0331450831799192,
0.072515617288641));
#73164=CARTESIAN_POINT('Ctrl Pts',(0.00266452976866446,-0.0337436976235975,
0.0723403901066244));
#73165=CARTESIAN_POINT('Ctrl Pts',(0.00264825386302956,-0.0336723290703325,
0.0723894914503022));
#73166=CARTESIAN_POINT('Ctrl Pts',(0.00263286376886128,-0.033601104548885,
0.0724388776027813));
#73167=CARTESIAN_POINT('Ctrl Pts',(0.00258372624678785,-0.0333736987606857,
0.0725965578048016));
#73168=CARTESIAN_POINT('Ctrl Pts',(0.00254371829863148,-0.0331450831799192,
0.0727567979566642));
#73169=CARTESIAN_POINT('Ctrl Pts',(0.00266369177804075,-0.0337436976235975,
0.0723427454774475));
#73170=CARTESIAN_POINT('Ctrl Pts',(0.002647437056968,-0.0336723290703325,
0.07239185435814));
#73171=CARTESIAN_POINT('Ctrl Pts',(0.00263206827950185,-0.033601104548885,
0.072441247665371));
#73172=CARTESIAN_POINT('Ctrl Pts',(0.0025829988174357,-0.0333736987606857,
0.0725989507110966));
#73173=CARTESIAN_POINT('Ctrl Pts',(0.00254306012803263,-0.0331450831799192,
0.0727592097633445));
#73174=CARTESIAN_POINT('',(0.00265327085821316,-0.0336938721132548,0.0723747167170325));
#73175=CARTESIAN_POINT('',(0.00258495299398426,-0.0333679869945434,0.0726009693021799));
#73176=CARTESIAN_POINT('Ctrl Pts',(0.00265327085821043,-0.0336938721132646,
0.0723747167170381));
#73177=CARTESIAN_POINT('Ctrl Pts',(0.00264634109475723,-0.0336629187933929,
0.072396070689041));
#73178=CARTESIAN_POINT('Ctrl Pts',(0.0026395385836991,-0.0336319952301037,
0.0724174584080862));
#73179=CARTESIAN_POINT('Ctrl Pts',(0.00263286376885911,-0.0336011045488947,
0.0724388776027873));
#73180=CARTESIAN_POINT('Ctrl Pts',(0.00261611437443248,-0.0335235892595451,
0.0724926256915283));
#73181=CARTESIAN_POINT('Ctrl Pts',(0.00260013943773531,-0.0334458668660366,
0.0725466675256716));
#73182=CARTESIAN_POINT('Ctrl Pts',(0.00258495299366919,-0.0333679869945382,
0.0726009693020844));
#73183=CARTESIAN_POINT('Ctrl Pts',(0.0025849403544701,-0.0333679692460736,
0.0726010119438432));
#73184=CARTESIAN_POINT('Ctrl Pts',(0.0025853784171049,-0.0333391895375831,
0.0726011283008377));
#73185=CARTESIAN_POINT('Ctrl Pts',(0.00258570760002757,-0.0333104081062015,
0.0726012123777164));
#73186=CARTESIAN_POINT('Ctrl Pts',(0.00258614470042685,-0.0332532698303069,
0.0726013183016452));
#73187=CARTESIAN_POINT('Ctrl Pts',(0.00258625584754641,-0.0332249171635303,
0.0726013410562512));
#73188=CARTESIAN_POINT('Ctrl Pts',(0.00258626124055257,-0.033196098535,
0.0726013354003529));
#73189=CARTESIAN_POINT('Ctrl Pts',(0.0025862612993336,-0.0331956312575113,
0.0726013353006517));
#73190=CARTESIAN_POINT('Ctrl Pts',(0.00258626132929588,-0.0331951640388587,
0.0726013351935164));
#73191=CARTESIAN_POINT('',(0.00261992795552372,-0.0331951640388587,0.0724809543051726));
#73192=CARTESIAN_POINT('',(0.00260309464241977,-0.0331951640388687,0.0725411447493546));
#73193=CARTESIAN_POINT('',(0.00269314705329479,-0.0335216366567741,0.0722562399905133));
#73194=CARTESIAN_POINT('Origin',(0.0187759744413429,-0.0326434571526037,
0.0765821304451633));
#73195=CARTESIAN_POINT('',(0.00269442982957012,-0.0336938721132328,0.0722566873178099));
#73196=CARTESIAN_POINT('Origin',(-0.00761715546663589,-0.033693886789626,
0.0686608510278571));
#73197=CARTESIAN_POINT('',(0.00267385034390164,-0.0336938721132538,0.0723157020174312));
#73198=CARTESIAN_POINT('Ctrl Pts',(0.00254016238846795,-0.0335235895815171,
0.0719538238055078));
#73199=CARTESIAN_POINT('Ctrl Pts',(0.00250992769927774,-0.0334144449262748,
0.0720306933252545));
#73200=CARTESIAN_POINT('Ctrl Pts',(0.00248124634051988,-0.0333049234473147,
0.0721082757846909));
#73201=CARTESIAN_POINT('Ctrl Pts',(0.00245416397318736,-0.0331951640388587,
0.0721864753018191));
#73202=CARTESIAN_POINT('Ctrl Pts',(0.00259161984448248,-0.0335235895815171,
0.0720547856929032));
#73203=CARTESIAN_POINT('Ctrl Pts',(0.00256277509444792,-0.0334144449262748,
0.0721309467994575));
#73204=CARTESIAN_POINT('Ctrl Pts',(0.00253547063643401,-0.0333049234473147,
0.0722077913167236));
#73205=CARTESIAN_POINT('Ctrl Pts',(0.00250975028532488,-0.0331951640388587,
0.0722852241468193));
#73206=CARTESIAN_POINT('Ctrl Pts',(0.002643077300497,-0.0335235895815171,
0.0721557475802987));
#73207=CARTESIAN_POINT('Ctrl Pts',(0.0026156224896181,-0.0334144449262748,
0.0722312002736604));
#73208=CARTESIAN_POINT('Ctrl Pts',(0.00258969493234813,-0.0333049234473147,
0.0723073068487562));
#73209=CARTESIAN_POINT('Ctrl Pts',(0.0025653365974624,-0.0331951640388587,
0.0723839729918196));
#73210=CARTESIAN_POINT('Ctrl Pts',(0.00269453475651152,-0.0335235895815171,
0.0722567094676941));
#73211=CARTESIAN_POINT('Ctrl Pts',(0.00266846988478829,-0.0334144449262748,
0.0723314537478634));
#73212=CARTESIAN_POINT('Ctrl Pts',(0.00264391922826226,-0.0333049234473147,
0.0724068223807889));
#73213=CARTESIAN_POINT('Ctrl Pts',(0.00262092290959992,-0.0331951640388587,
0.0724827218368198));
#73214=CARTESIAN_POINT('',(0.0025370459643656,-0.0331951640388687,0.0723337148035059));
#73215=CARTESIAN_POINT('Ctrl Pts',(0.0024583710359038,-0.0332121607145976,
0.0721743693767619));
#73216=CARTESIAN_POINT('Ctrl Pts',(0.00249888882421,-0.0332625444109904,
0.0721884986572576));
#73217=CARTESIAN_POINT('Ctrl Pts',(0.00253870842744081,-0.0333135300747139,
0.0722023844680778));
#73218=CARTESIAN_POINT('Ctrl Pts',(0.00261698287199452,-0.0334167203140642,
0.0722296801727295));
#73219=CARTESIAN_POINT('Ctrl Pts',(0.00265540739701302,-0.0334688847587347,
0.072243079494721));
#73220=CARTESIAN_POINT('Ctrl Pts',(0.0026931470539036,-0.0335216366562431,
0.0722562399908959));
#73221=CARTESIAN_POINT('Ctrl Pts',(0.00265417123522845,-0.0336938721132389,
0.0723742819342105));
#73222=CARTESIAN_POINT('Ctrl Pts',(0.00264377736814366,-0.0336474569764957,
0.0724062973821562));
#73223=CARTESIAN_POINT('Ctrl Pts',(0.00263375899449409,-0.033601104548885,
0.0724384323097205));
#73224=CARTESIAN_POINT('Ctrl Pts',(0.00260839477578187,-0.0334837508592655,
0.0725197905580304));
#73225=CARTESIAN_POINT('Ctrl Pts',(0.00258545250874611,-0.0333660264659097,
0.0726018646741827));
#73226=CARTESIAN_POINT('Ctrl Pts',(0.00265327085821957,-0.0336938721132389,
0.0723747167170131));
#73227=CARTESIAN_POINT('Ctrl Pts',(0.0026428795360628,-0.0336474569764957,
0.0724067374351643));
#73228=CARTESIAN_POINT('Ctrl Pts',(0.00263286376886128,-0.033601104548885,
0.0724388776027813));
#73229=CARTESIAN_POINT('Ctrl Pts',(0.00260750614907625,-0.0334837508592655,
0.0725202491176999));
#73230=CARTESIAN_POINT('Ctrl Pts',(0.00258457087118706,-0.0333660264659097,
0.0726023362990952));
#73231=CARTESIAN_POINT('Ctrl Pts',(0.00234713869739755,-0.0336938721132389,
0.0725225447907597));
#73232=CARTESIAN_POINT('Ctrl Pts',(0.00233761266201098,-0.0336474569764957,
0.0725563574020336));
#73233=CARTESIAN_POINT('Ctrl Pts',(0.00232848309866109,-0.033601104548885,
0.0725902792107175));
#73234=CARTESIAN_POINT('Ctrl Pts',(0.00230536914327736,-0.0334837508592655,
0.0726761614311924));
#73235=CARTESIAN_POINT('Ctrl Pts',(0.00228481020609527,-0.0333660264659097,
0.0727626908529466));
#73236=CARTESIAN_POINT('',(0.00234549955260835,-0.0336769361243754,0.0725340019410606));
#73237=CARTESIAN_POINT('',(0.00234896453534305,-0.033693872113232,0.0725216631123868));
#73238=CARTESIAN_POINT('Ctrl Pts',(0.00234549955260829,-0.0336769361243751,
0.0725340019410609));
#73239=CARTESIAN_POINT('Ctrl Pts',(0.00234607489648189,-0.0336797586670061,
0.0725319446987896));
#73240=CARTESIAN_POINT('Ctrl Pts',(0.00234665131725535,-0.0336825812712917,
0.0725298878415841));
#73241=CARTESIAN_POINT('Ctrl Pts',(0.00234780631258848,-0.0336882266054485,
0.0725257748954517));
#73242=CARTESIAN_POINT('Ctrl Pts',(0.0023483848871579,-0.0336910493353204,
0.0725237188065247));
#73243=CARTESIAN_POINT('Ctrl Pts',(0.00234896453534645,-0.0336938721132312,
0.0725216631123867));
#73244=CARTESIAN_POINT('Ctrl Pts',(0.00234549955260836,-0.0336769361243754,
0.0725340019410606));
#73245=CARTESIAN_POINT('Ctrl Pts',(0.00238586447293965,-0.0336279007516211,
0.0725452906988046));
#73246=CARTESIAN_POINT('Ctrl Pts',(0.00242680412680003,-0.0335767878632072,
0.072556740190857));
#73247=CARTESIAN_POINT('Ctrl Pts',(0.00250703435245218,-0.0334733198857316,
0.0725791779802468));
#73248=CARTESIAN_POINT('Ctrl Pts',(0.00254637268890566,-0.0334209645014069,
0.0725901796358093));
#73249=CARTESIAN_POINT('Ctrl Pts',(0.00258495299593697,-0.0333679869844681,
0.0726009692951519));
#73250=CARTESIAN_POINT('',(0.00250111769678811,-0.0336938721132534,0.0724481899147197));
#73251=CARTESIAN_POINT('Origin',(0.00812378219310841,-0.0315241814719618,
0.07415));
#73252=CARTESIAN_POINT('',(0.00234549955386281,-0.0337108120655682,0.0725340019414152));
#73253=CARTESIAN_POINT('',(0.00234206093373597,-0.0336938721132327,0.0725463481428482));
#73254=CARTESIAN_POINT('Origin',(0.0178011120907627,-0.0345562513279639,
0.0780169232437248));
#73255=CARTESIAN_POINT('Ctrl Pts',(0.00234206093374247,-0.0336938721132293,
0.0725463481428547));
#73256=CARTESIAN_POINT('Ctrl Pts',(0.00234263179342879,-0.0336910493414198,
0.0725442899956516));
#73257=CARTESIAN_POINT('Ctrl Pts',(0.00234320377762032,-0.0336882266084981,
0.0725422320612115));
#73258=CARTESIAN_POINT('Ctrl Pts',(0.00234434998528453,-0.0336825812712737,
0.072538116655043));
#73259=CARTESIAN_POINT('Ctrl Pts',(0.00234492420873666,-0.0336797586669971,
0.0725360591833251));
#73260=CARTESIAN_POINT('Ctrl Pts',(0.00234549955260843,-0.0336769361243751,
0.0725340019410604));
#73261=CARTESIAN_POINT('Origin',(0.0184031252217066,-0.0345562515972652,
0.0758643098980786));
#73262=CARTESIAN_POINT('Ctrl Pts',(0.00263053551478968,-0.0342436276873911,
0.0724463668437305));
#73263=CARTESIAN_POINT('Ctrl Pts',(0.00256628193106721,-0.0339430054201811,
0.072653548057629));
#73264=CARTESIAN_POINT('Ctrl Pts',(0.00251781662296948,-0.0336441434784053,
0.0728649805346154));
#73265=CARTESIAN_POINT('Ctrl Pts',(0.00256168914869608,-0.0342436276873911,
0.0726867003159638));
#73266=CARTESIAN_POINT('Ctrl Pts',(0.00250649989130621,-0.0339430054201811,
0.0728964781133647));
#73267=CARTESIAN_POINT('Ctrl Pts',(0.0024672687440488,-0.0336441434784053,
0.0731098170350327));
#73268=CARTESIAN_POINT('Ctrl Pts',(0.00256100068503515,-0.0342436276873911,
0.0726891036506861));
#73269=CARTESIAN_POINT('Ctrl Pts',(0.0025059020709086,-0.0339430054201811,
0.0728989074139221));
#73270=CARTESIAN_POINT('Ctrl Pts',(0.00246676326525959,-0.0336441434784053,
0.0731122654000369));
#73271=CARTESIAN_POINT('',(0.00255259470306785,-0.0341934961088741,0.0727217160818602));
#73272=CARTESIAN_POINT('',(0.00249861816545665,-0.033866421289281,0.0729518119189903));
#73273=CARTESIAN_POINT('Origin',(0.0186290599892738,-0.0345610818076339,
0.0773693346343042));
#73274=CARTESIAN_POINT('Origin',(-0.00822703412941682,-0.0336938005044306,
0.0706672710820475));
#73275=CARTESIAN_POINT('',(0.0025259883083293,-0.0336938721132327,0.0728298376525857));
#73276=CARTESIAN_POINT('',(0.00251296760118384,-0.0336938721132427,0.0728909662971511));
#73277=CARTESIAN_POINT('',(0.00258495299593841,-0.0340203938281605,0.0726009692951467));
#73278=CARTESIAN_POINT('Origin',(0.0184257655862531,-0.0345589643247985,
0.0778054481328131));
#73279=CARTESIAN_POINT('',(0.0025862613292958,-0.0341934961088741,0.0726013351935164));
#73280=CARTESIAN_POINT('Origin',(-0.00802598527630373,-0.0341934220717649,
0.0696334335361931));
#73281=CARTESIAN_POINT('',(0.00256942801619183,-0.0341934961088841,0.0726615256376983));
#73282=CARTESIAN_POINT('Ctrl Pts',(0.00241328218214011,-0.0340223579322397,
0.0723087532417509));
#73283=CARTESIAN_POINT('Ctrl Pts',(0.00238788658717071,-0.0339125849573575,
0.0723875159305114));
#73284=CARTESIAN_POINT('Ctrl Pts',(0.00236413904203001,-0.0338030433565231,
0.0724667489034471));
#73285=CARTESIAN_POINT('Ctrl Pts',(0.00234206093373559,-0.0336938721132327,
0.0725463481428476));
#73286=CARTESIAN_POINT('Ctrl Pts',(0.00247097752000295,-0.0340223579322397,
0.0724062849177297));
#73287=CARTESIAN_POINT('Ctrl Pts',(0.00244692714121859,-0.0339125849573575,
0.0724842518373053));
#73288=CARTESIAN_POINT('Ctrl Pts',(0.00242450739642207,-0.0338030433565231,
0.0725626617573847));
#73289=CARTESIAN_POINT('Ctrl Pts',(0.00240373806790193,-0.0336938721132327,
0.0726414118633269));
#73290=CARTESIAN_POINT('Ctrl Pts',(0.0025286728578658,-0.0340223579322397,
0.0725038165937084));
#73291=CARTESIAN_POINT('Ctrl Pts',(0.00250596769526647,-0.0339125849573575,
0.0725809877440991));
#73292=CARTESIAN_POINT('Ctrl Pts',(0.00248487575081414,-0.0338030433565231,
0.0726585746113223));
#73293=CARTESIAN_POINT('Ctrl Pts',(0.00246541520206826,-0.0336938721132327,
0.0727364755838062));
#73294=CARTESIAN_POINT('Ctrl Pts',(0.00258636819572864,-0.0340223579322397,
0.0726013482696872));
#73295=CARTESIAN_POINT('Ctrl Pts',(0.00256500824931436,-0.0339125849573575,
0.072677723650893));
#73296=CARTESIAN_POINT('Ctrl Pts',(0.0025452441052062,-0.0338030433565231,
0.0727544874652599));
#73297=CARTESIAN_POINT('Ctrl Pts',(0.0025270923362346,-0.0336938721132327,
0.0728315393042854));
#73298=CARTESIAN_POINT('',(0.00243402462104263,-0.0336938721132427,0.072688092897727));
#73299=CARTESIAN_POINT('Ctrl Pts',(0.00234549955732709,-0.0337108120662685,
0.0725340019423802));
#73300=CARTESIAN_POINT('Ctrl Pts',(0.00238690986657648,-0.033761140899441,
0.0725455830614654));
#73301=CARTESIAN_POINT('Ctrl Pts',(0.00242756452955417,-0.0338121088781553,
0.0725569528508209));
#73302=CARTESIAN_POINT('Ctrl Pts',(0.00250739959868047,-0.0339153382773236,
0.0725792801277594));
#73303=CARTESIAN_POINT('Ctrl Pts',(0.00254654622973458,-0.0339675558473117,
0.072590228169545));
#73304=CARTESIAN_POINT('Ctrl Pts',(0.00258495299597539,-0.0340203938281304,
0.0726009692951626));
#73305=CARTESIAN_POINT('Ctrl Pts',(0.00255436207816171,-0.0341934961088741,
0.0727207212159088));
#73306=CARTESIAN_POINT('Ctrl Pts',(0.00252481286551814,-0.0340287516194401,
0.0728358645882933));
#73307=CARTESIAN_POINT('Ctrl Pts',(0.00250004786501172,-0.033864463329982,
0.0729521308642372));
#73308=CARTESIAN_POINT('Ctrl Pts',(0.00255259470306794,-0.0341934961088741,
0.0727217160818602));
#73309=CARTESIAN_POINT('Ctrl Pts',(0.00252306605849399,-0.0340287516194401,
0.0728368959933322));
#73310=CARTESIAN_POINT('Ctrl Pts',(0.00249832311867037,-0.033864463329982,
0.0729531979270476));
#73311=CARTESIAN_POINT('Ctrl Pts',(0.002258115699717,-0.0341934961088741,
0.0728874800641951));
#73312=CARTESIAN_POINT('Ctrl Pts',(0.00223201409486208,-0.0340287516194401,
0.073008748097023));
#73313=CARTESIAN_POINT('Ctrl Pts',(0.00221094689309027,-0.033864463329982,
0.0731309913077608));
#73314=CARTESIAN_POINT('',(0.00225543231674149,-0.0341764758832383,0.0729000121124188));
#73315=CARTESIAN_POINT('',(0.00225811569971695,-0.034193496108874,0.072887480064195));
#73316=CARTESIAN_POINT('Origin',(0.018343191126596,-0.0345621026071988,
0.0768503725182579));
#73317=CARTESIAN_POINT('Ctrl Pts',(0.00225543231791702,-0.0341764758837467,
0.0729000121110281));
#73318=CARTESIAN_POINT('Ctrl Pts',(0.00229741486488263,-0.0341260050044177,
0.0729089545895575));
#73319=CARTESIAN_POINT('Ctrl Pts',(0.00233866766410551,-0.034074926915576,
0.0729177415893458));
#73320=CARTESIAN_POINT('Ctrl Pts',(0.00241974570017303,-0.0339715436321982,
0.0729350116208483));
#73321=CARTESIAN_POINT('Ctrl Pts',(0.00245954017661583,-0.0339192778256753,
0.07294348810656));
#73322=CARTESIAN_POINT('Ctrl Pts',(0.00249861816420593,-0.0338664212878159,
0.0729518119155586));
#73323=CARTESIAN_POINT('',(0.0024053552014024,-0.0341934961088841,0.0728045980730376));
#73324=CARTESIAN_POINT('Origin',(0.00812378219310841,-0.0315241814719618,
0.07415));
#73325=CARTESIAN_POINT('',(0.0022554323172859,-0.034210518019037,0.0729000121133953));
#73326=CARTESIAN_POINT('',(0.00225277570667799,-0.0341934961088739,0.0729125498651185));
#73327=CARTESIAN_POINT('Origin',(0.0183576906715232,-0.0345621703957348,
0.0768074265873306));
#73328=CARTESIAN_POINT('Origin',(0.0185565663266295,-0.0345621038964406,
0.0758486461905739));
#73329=CARTESIAN_POINT('Origin',(0.0185523004742703,-0.0345621716491088,
0.0758937719971404));
#73330=CARTESIAN_POINT('Ctrl Pts',(0.00252630080736586,-0.0346945769586966,
0.0728283705554236));
#73331=CARTESIAN_POINT('Ctrl Pts',(0.00249861874949764,-0.0345275153362944,
0.0729456120441572));
#73332=CARTESIAN_POINT('Ctrl Pts',(0.00247461666853867,-0.0343603235965185,
0.0730637544327854));
#73333=CARTESIAN_POINT('Ctrl Pts',(0.00245436035880645,-0.034193496108874,
0.073182447253507));
#73334=CARTESIAN_POINT('Ctrl Pts',(0.00250883569810389,-0.0346945769586966,
0.0729103644474174));
#73335=CARTESIAN_POINT('Ctrl Pts',(0.00248287103513205,-0.0345275153362944,
0.0730279717498572));
#73336=CARTESIAN_POINT('Ctrl Pts',(0.00246059829778009,-0.0343603235965185,
0.073146426036321));
#73337=CARTESIAN_POINT('Ctrl Pts',(0.0024420781520247,-0.034193496108874,
0.073265375992569));
#73338=CARTESIAN_POINT('Ctrl Pts',(0.00249137058884199,-0.0346945769586966,
0.0729923583394103));
#73339=CARTESIAN_POINT('Ctrl Pts',(0.00246712332076652,-0.0345275153362944,
0.0731103314555584));
#73340=CARTESIAN_POINT('Ctrl Pts',(0.00244657992702156,-0.0343603235965185,
0.0732290976398585));
#73341=CARTESIAN_POINT('Ctrl Pts',(0.00242979594524296,-0.034193496108874,
0.0733483047316324));
#73342=CARTESIAN_POINT('Ctrl Pts',(0.00247390547957996,-0.0346945769586966,
0.0730743522314051));
#73343=CARTESIAN_POINT('Ctrl Pts',(0.00245137560640087,-0.0345275153362944,
0.0731926911612572));
#73344=CARTESIAN_POINT('Ctrl Pts',(0.00243256155626293,-0.0343603235965185,
0.0733117692433922));
#73345=CARTESIAN_POINT('Ctrl Pts',(0.00241751373846119,-0.034193496108874,
0.0734312334706929));
#73346=CARTESIAN_POINT('',(0.00247390547970629,-0.0346945769586966,0.0730743522308127));
#73347=CARTESIAN_POINT('',(0.00243448329133996,-0.034366772783144,0.0733073832385791));
#73348=CARTESIAN_POINT('Origin',(0.0190240764866805,-0.0345626457061231,
0.0760389916498902));
#73349=CARTESIAN_POINT('Origin',(-0.0084984381877856,-0.0341934771028977,
0.0716881604615297));
#73350=CARTESIAN_POINT('',(0.00245414059620934,-0.0341934961088739,0.0731839310776592));
#73351=CARTESIAN_POINT('',(0.00244498388180492,-0.0341934961088839,0.073245756675775));
#73352=CARTESIAN_POINT('',(0.00249861816742679,-0.0345211942962711,0.072951811916287));
#73353=CARTESIAN_POINT('Origin',(0.0189206569525864,-0.0345625596115329,
0.0765085608031198));
#73354=CARTESIAN_POINT('',(0.00249994689401839,-0.0346945769586885,0.0729520949416963));
#73355=CARTESIAN_POINT('Origin',(-0.00832086656064614,-0.0346945685853893,
0.0706472063572769));
#73356=CARTESIAN_POINT('',(0.00248692618687234,-0.0346945769587026,0.0730132235862645));
#73357=CARTESIAN_POINT('Ctrl Pts',(0.00230893747175623,-0.0345231616327841,
0.0726709527165808));
#73358=CARTESIAN_POINT('Ctrl Pts',(0.00228855088728632,-0.0344132092796988,
0.0727511021644182));
#73359=CARTESIAN_POINT('Ctrl Pts',(0.00226982318277795,-0.0343032738558979,
0.0728316691573314));
#73360=CARTESIAN_POINT('Ctrl Pts',(0.00225277570667794,-0.0341934961088739,
0.0729125498651185));
#73361=CARTESIAN_POINT('Ctrl Pts',(0.00237264293230449,-0.0345231616327841,
0.072764669046187));
#73362=CARTESIAN_POINT('Ctrl Pts',(0.00235354809549615,-0.0344132092796988,
0.0728439404039408));
#73363=CARTESIAN_POINT('Ctrl Pts',(0.00233609390940038,-0.0343032738558979,
0.0729236026332944));
#73364=CARTESIAN_POINT('Ctrl Pts',(0.00232030012063065,-0.0341934961088739,
0.0730035531049446));
#73365=CARTESIAN_POINT('Ctrl Pts',(0.00243634839285275,-0.0345231616327841,
0.0728583853757931));
#73366=CARTESIAN_POINT('Ctrl Pts',(0.00241854530370599,-0.0344132092796988,
0.0729367786434633));
#73367=CARTESIAN_POINT('Ctrl Pts',(0.00240236463602281,-0.0343032738558979,
0.0730155361092575));
#73368=CARTESIAN_POINT('Ctrl Pts',(0.00238782453458337,-0.0341934961088739,
0.0730945563447708));
#73369=CARTESIAN_POINT('Ctrl Pts',(0.002500053853401,-0.0345231616327841,
0.0729521017053992));
#73370=CARTESIAN_POINT('Ctrl Pts',(0.00248354251191583,-0.0344132092796988,
0.0730296168829859));
#73371=CARTESIAN_POINT('Ctrl Pts',(0.00246863536264524,-0.0343032738558979,
0.0731074695852204));
#73372=CARTESIAN_POINT('Ctrl Pts',(0.00245534894853608,-0.0341934961088739,
0.073185559584597));
#73373=CARTESIAN_POINT('',(0.00235345815145366,-0.0341934961088839,0.0730482404713988));
#73374=CARTESIAN_POINT('Ctrl Pts',(0.00225543232065939,-0.0342105180195389,
0.0729000121141101));
#73375=CARTESIAN_POINT('Ctrl Pts',(0.00229746206161806,-0.0342610556241343,
0.0729089646592356));
#73376=CARTESIAN_POINT('Ctrl Pts',(0.00233873760060634,-0.0343122189870239,
0.0729177565555677));
#73377=CARTESIAN_POINT('Ctrl Pts',(0.00241981645595705,-0.0344158119695192,
0.0729350267574461));
#73378=CARTESIAN_POINT('Ctrl Pts',(0.00245958661048381,-0.03446819904501,
0.0729434979993555));
#73379=CARTESIAN_POINT('Ctrl Pts',(0.00249861816745104,-0.0345211942962529,
0.072951811916289));
#73380=CARTESIAN_POINT('Ctrl Pts',(0.0024756064843927,-0.0346945769586932,
0.0730732486226806));
#73381=CARTESIAN_POINT('Ctrl Pts',(0.00245334541155146,-0.034529677707698,
0.0731900206589373));
#73382=CARTESIAN_POINT('Ctrl Pts',(0.00243592965608153,-0.0343648066251421,
0.073307612985545));
#73383=CARTESIAN_POINT('Ctrl Pts',(0.00247390547970809,-0.0346945769586932,
0.0730743522308038));
#73384=CARTESIAN_POINT('Ctrl Pts',(0.00245166722318391,-0.034529677707698,
0.0731911594341289));
#73385=CARTESIAN_POINT('Ctrl Pts',(0.00243427571802203,-0.0343648066251421,
0.0733087859547356));
#73386=CARTESIAN_POINT('Ctrl Pts',(0.00219041596997284,-0.0346945769586932,
0.0732582796053955));
#73387=CARTESIAN_POINT('Ctrl Pts',(0.0021719802817755,-0.034529677707698,
0.0733809477537435));
#73388=CARTESIAN_POINT('Ctrl Pts',(0.0021586303339369,-0.0343648066251421,
0.0735042730476258));
#73389=CARTESIAN_POINT('',(0.00218852477561365,-0.0346775396664969,0.0732709554155673));
#73390=CARTESIAN_POINT('',(0.00219041596997232,-0.0346945769586887,0.0732582796053988));
#73391=CARTESIAN_POINT('Origin',(0.0186326590362704,-0.0345626618789612,
0.0755520402302187));
#73392=CARTESIAN_POINT('Ctrl Pts',(0.00218852477677931,-0.0346775396670097,
0.0732709554141674));
#73393=CARTESIAN_POINT('Ctrl Pts',(0.00223101942578306,-0.0346269749928186,
0.0732772490946446));
#73394=CARTESIAN_POINT('Ctrl Pts',(0.00227275885531511,-0.0345757902890784,
0.0732834308868437));
#73395=CARTESIAN_POINT('Ctrl Pts',(0.00235476162507108,-0.0344721681087817,
0.0732955759562511));
#73396=CARTESIAN_POINT('Ctrl Pts',(0.00239499281551225,-0.034419771428957,
0.073301534477595));
#73397=CARTESIAN_POINT('Ctrl Pts',(0.00243448329126564,-0.0343667727830599,
0.0733073832383186));
#73398=CARTESIAN_POINT('',(0.00233216072484931,-0.0346945769587026,0.0731663159181158));
#73399=CARTESIAN_POINT('Origin',(0.00812378219310841,-0.0315241814719618,
0.07415));
#73400=CARTESIAN_POINT('',(0.00218852477667093,-0.0347116136489613,0.0732709554164708));
#73401=CARTESIAN_POINT('',(0.00218666066001419,-0.0346945769586885,0.0732836352377339));
#73402=CARTESIAN_POINT('Origin',(0.0186374449334779,-0.0345626683579165,
0.0755069803020974));
#73403=CARTESIAN_POINT('Origin',(0.0185879136793979,-0.0345626628398701,
0.0758541774810751));
#73404=CARTESIAN_POINT('Origin',(0.0185794279522539,-0.0345626695130172,
0.07589868918301));
#73405=CARTESIAN_POINT('Ctrl Pts',(0.00246070148270513,-0.0352450361874068,
0.0731458687869191));
#73406=CARTESIAN_POINT('Ctrl Pts',(0.00242283005256249,-0.0349452760959492,
0.073359455380705));
#73407=CARTESIAN_POINT('Ctrl Pts',(0.00240115442733529,-0.034644428984174,
0.073575287828537));
#73408=CARTESIAN_POINT('Ctrl Pts',(0.00246031588138545,-0.0352450361874068,
0.0731483641699803));
#73409=CARTESIAN_POINT('Ctrl Pts',(0.00242253856615933,-0.0349452760959492,
0.0733619653069586));
#73410=CARTESIAN_POINT('Ctrl Pts',(0.00240095788393081,-0.034644428984174,
0.0735778051675469));
#73411=CARTESIAN_POINT('Ctrl Pts',(0.00242213753290251,-0.0352450361874068,
0.0733954317998048));
#73412=CARTESIAN_POINT('Ctrl Pts',(0.00239367852624155,-0.0349452760959492,
0.0736104728568243));
#73413=CARTESIAN_POINT('Ctrl Pts',(0.00238149814091364,-0.034644428984174,
0.0738270466536636));
#73414=CARTESIAN_POINT('Ctrl Pts',(0.00242175574941768,-0.0352450361874068,
0.0733979024761031));
#73415=CARTESIAN_POINT('Ctrl Pts',(0.00239338992584237,-0.0349452760959492,
0.0736129579323229));
#73416=CARTESIAN_POINT('Ctrl Pts',(0.00238130354348347,-0.034644428984174,
0.0738295390685247));
#73417=CARTESIAN_POINT('',(0.00241751542765013,-0.0351951634053263,0.0734312010684742));
#73418=CARTESIAN_POINT('',(0.0023928014789834,-0.0348678972934074,0.0736662799844453));
#73419=CARTESIAN_POINT('Origin',(0.0191180503661572,-0.0345636767881002,
0.0746545690151686));
#73420=CARTESIAN_POINT('Origin',(-0.00861789031430973,-0.0346946199326795,
0.0727369448443345));
#73421=CARTESIAN_POINT('',(0.00240466837133796,-0.0346945769330289,0.0735418371175442));
#73422=CARTESIAN_POINT('',(0.00239941178594709,-0.0346945769458128,0.0736041156804507));
#73423=CARTESIAN_POINT('',(0.00243448329139868,-0.0350221583435276,0.0733073832383547));
#73424=CARTESIAN_POINT('Origin',(0.0191191025579792,-0.0345628458719109,
0.0751353416087238));
#73425=CARTESIAN_POINT('',(0.0024357072726396,-0.035195136029876,0.0733075614591906));
#73426=CARTESIAN_POINT('Origin',(-0.0084643700309076,-0.0351951838366836,
0.0716932013219096));
#73427=CARTESIAN_POINT('',(0.00241751373843655,-0.035195137132875,0.073431233470066));
#73428=CARTESIAN_POINT('Ctrl Pts',(0.00222754141431054,-0.0350241211494343,
0.0730389893436746));
#73429=CARTESIAN_POINT('Ctrl Pts',(0.00221223769805176,-0.0349144232818962,
0.0731202076428497));
#73430=CARTESIAN_POINT('Ctrl Pts',(0.00219860366206057,-0.0348045283579413,
0.0732017908938422));
#73431=CARTESIAN_POINT('Ctrl Pts',(0.00218666065840955,-0.0346945769439158,
0.0732836352487303));
#73432=CARTESIAN_POINT('Ctrl Pts',(0.00229700569336549,-0.0350241211494343,
0.0731285206551714));
#73433=CARTESIAN_POINT('Ctrl Pts',(0.00228293523421331,-0.0349144232818962,
0.073208782112384));
#73434=CARTESIAN_POINT('Ctrl Pts',(0.00227051541488546,-0.0348045283579413,
0.0732893824563923));
#73435=CARTESIAN_POINT('Ctrl Pts',(0.00225976598534772,-0.0346945769439158,
0.0733702190403788));
#73436=CARTESIAN_POINT('Ctrl Pts',(0.00236646997242043,-0.0350241211494343,
0.0732180519666682));
#73437=CARTESIAN_POINT('Ctrl Pts',(0.00235363277037486,-0.0349144232818962,
0.0732973565819183));
#73438=CARTESIAN_POINT('Ctrl Pts',(0.00234242716771034,-0.0348045283579413,
0.0733769740189424));
#73439=CARTESIAN_POINT('Ctrl Pts',(0.00233287131228588,-0.0346945769439158,
0.0734568028320273));
#73440=CARTESIAN_POINT('Ctrl Pts',(0.00243593425147538,-0.0350241211494343,
0.073307583278165));
#73441=CARTESIAN_POINT('Ctrl Pts',(0.0024243303065364,-0.0349144232818962,
0.0733859310514526));
#73442=CARTESIAN_POINT('Ctrl Pts',(0.00241433892053522,-0.0348045283579413,
0.0734645655814925));
#73443=CARTESIAN_POINT('Ctrl Pts',(0.00240597663922405,-0.0346945769439158,
0.0735433866236757));
#73444=CARTESIAN_POINT('',(0.00229566451562936,-0.0346945769458128,0.0734127361773446));
#73445=CARTESIAN_POINT('Ctrl Pts',(0.0021885247799184,-0.0347116136492793,
0.0732709554169476));
#73446=CARTESIAN_POINT('Ctrl Pts',(0.00223100255147917,-0.0347621546532328,
0.0732772466108068));
#73447=CARTESIAN_POINT('Ctrl Pts',(0.00227273344902875,-0.0348133084097092,
0.0732834271884774));
#73448=CARTESIAN_POINT('Ctrl Pts',(0.00235473632337568,-0.0349168561544568,
0.0732955722695532));
#73449=CARTESIAN_POINT('Ctrl Pts',(0.00239497577380308,-0.0349692089015917,
0.0733015319556226));
#73450=CARTESIAN_POINT('Ctrl Pts',(0.00243448329143193,-0.0350221583435,
0.0733073832383798));
#73451=CARTESIAN_POINT('Ctrl Pts',(0.00241868864853549,-0.0351951371254872,
0.0734303616867431));
#73452=CARTESIAN_POINT('Ctrl Pts',(0.00240381057796537,-0.0350307338985332,
0.0735483109159624));
#73453=CARTESIAN_POINT('Ctrl Pts',(0.00239382018952007,-0.0348659306906665,
0.0736667742849673));
#73454=CARTESIAN_POINT('Ctrl Pts',(0.00241751373855187,-0.0351951371254872,
0.0734312334700801));
#73455=CARTESIAN_POINT('Ctrl Pts',(0.00240265369155523,-0.0350307338985332,
0.073549206989826));
#73456=CARTESIAN_POINT('Ctrl Pts',(0.00239268231523604,-0.0348659306906665,
0.0736676938836678));
#73457=CARTESIAN_POINT('Ctrl Pts',(0.00222059760062791,-0.0351951371254872,
0.0735773452660617));
#73458=CARTESIAN_POINT('Ctrl Pts',(0.00220875832333139,-0.0350307338985332,
0.0736993899033987));
#73459=CARTESIAN_POINT('Ctrl Pts',(0.00220197339916482,-0.0348659306906665,
0.0738218195844148));
#73460=CARTESIAN_POINT('Origin',(-0.00290653846384609,-0.030860918850895,
0.073218994061773));
#73461=CARTESIAN_POINT('',(0.00233166274228548,-0.0351951371254872,0.0734949349187452));
#73462=CARTESIAN_POINT('Origin',(0.00909906401176292,-0.0351840467441185,
0.0740902419571476));
#73463=CARTESIAN_POINT('Origin',(-0.00383964241854335,-0.0352322613866184,
0.0739377587820059));
#73464=CARTESIAN_POINT('',(0.00237778028345409,-0.0351951142564653,0.0739024588161934));
#73465=CARTESIAN_POINT('',(0.00237509545286777,-0.0351951372916786,0.0740271148398609));
#73466=CARTESIAN_POINT('Origin',(0.00829604622235164,-0.0352875119212674,
0.0744437979227203));
#73467=CARTESIAN_POINT('Origin',(0.00971740669074562,-0.0298325076522173,
0.0668181822689157));
#73468=CARTESIAN_POINT('Origin',(0.000427998268266064,-0.0338732996266689,
0.0708299719531315));
#73469=CARTESIAN_POINT('Ctrl Pts',(0.00362087063773921,-0.0321934096636942,
0.0705720224609657));
#73470=CARTESIAN_POINT('Ctrl Pts',(0.00355682654359785,-0.0320508460843192,
0.0706526224335524));
#73471=CARTESIAN_POINT('Ctrl Pts',(0.00349499630114318,-0.0319086045660808,
0.0707348823719354));
#73472=CARTESIAN_POINT('Ctrl Pts',(0.00343549846013825,-0.031766989286452,
0.0708186141957953));
#73473=CARTESIAN_POINT('Ctrl Pts',(0.00357014775933072,-0.0321934096636942,
0.0706387878879011));
#73474=CARTESIAN_POINT('Ctrl Pts',(0.00350729873453828,-0.0320508460843192,
0.0707202957758575));
#73475=CARTESIAN_POINT('Ctrl Pts',(0.00344668705424083,-0.0319086045660808,
0.0708034308358836));
#73476=CARTESIAN_POINT('Ctrl Pts',(0.00338842848929625,-0.031766989286452,
0.0708880033193749));
#73477=CARTESIAN_POINT('Ctrl Pts',(0.00351942488092221,-0.0321934096636942,
0.0707055533148366));
#73478=CARTESIAN_POINT('Ctrl Pts',(0.0034577709254787,-0.0320508460843192,
0.0707879691181626));
#73479=CARTESIAN_POINT('Ctrl Pts',(0.00339837780733849,-0.0319086045660808,
0.0708719792998318));
#73480=CARTESIAN_POINT('Ctrl Pts',(0.00334135851845424,-0.031766989286452,
0.0709573924429544));
#73481=CARTESIAN_POINT('Ctrl Pts',(0.00346870200251372,-0.0321934096636942,
0.070772318741772));
#73482=CARTESIAN_POINT('Ctrl Pts',(0.00340824311641913,-0.0320508460843192,
0.0708556424604677));
#73483=CARTESIAN_POINT('Ctrl Pts',(0.00335006856043615,-0.0319086045660808,
0.0709405277637799));
#73484=CARTESIAN_POINT('Ctrl Pts',(0.00329428854761224,-0.031766989286452,
0.0710267815665341));
#73485=CARTESIAN_POINT('',(0.00346960944483376,-0.0321934096636942,0.0707711242950919));
#73486=CARTESIAN_POINT('',(0.00333471940589462,-0.0318665617511257,0.0709651919038781));
#73487=CARTESIAN_POINT('Origin',(0.0166212639895788,-0.0326371944420649,
0.0810789799200326));
#73488=CARTESIAN_POINT('Origin',(-0.00579248170359597,-0.0316939261509038,
0.0648954480805042));
#73489=CARTESIAN_POINT('',(0.00354402256720402,-0.0320197221621841,0.0706710071952549));
#73490=CARTESIAN_POINT('Ctrl Pts',(0.00354387680638793,-0.0320197392094754,
0.0706711210752944));
#73491=CARTESIAN_POINT('Ctrl Pts',(0.00352617518936717,-0.0319792716576052,
0.0706944251346968));
#73492=CARTESIAN_POINT('Ctrl Pts',(0.00350857064861603,-0.0319386439829691,
0.0707179702330528));
#73493=CARTESIAN_POINT('Ctrl Pts',(0.00349105147620165,-0.0318979099381623,
0.0707417861527729));
#73494=CARTESIAN_POINT('Ctrl Pts',(0.00347353265006574,-0.0318571766984918,
0.0707656016017551));
#73495=CARTESIAN_POINT('Ctrl Pts',(0.00345618679580781,-0.0318163871833561,
0.0707895657599812));
#73496=CARTESIAN_POINT('Ctrl Pts',(0.00343907072366616,-0.0317755399638303,
0.0708135941360121));
#73497=CARTESIAN_POINT('',(0.00354522704296514,-0.0321934096636184,0.0706715904874358));
#73498=CARTESIAN_POINT('Origin',(0.00174950357711688,-0.0324018949057924,
0.0693329757938452));
#73499=CARTESIAN_POINT('',(0.00350741824390944,-0.0321934096636663,0.0707213573912738));
#73500=CARTESIAN_POINT('Ctrl Pts',(0.00347161902000672,-0.0321934096636618,
0.070770849895742));
#73501=CARTESIAN_POINT('Ctrl Pts',(0.00342501790651343,-0.0320835708272592,
0.070835006851583));
#73502=CARTESIAN_POINT('Ctrl Pts',(0.00337977154842656,-0.0319739230346488,
0.0709000910014041));
#73503=CARTESIAN_POINT('Ctrl Pts',(0.00333593144453206,-0.0318646057455572,
0.0709660146316876));
#73504=CARTESIAN_POINT('Ctrl Pts',(0.0033593420133819,-0.0321934096636618,
0.070786180862701));
#73505=CARTESIAN_POINT('Ctrl Pts',(0.00331295232587124,-0.0320835708272592,
0.070851886205967));
#73506=CARTESIAN_POINT('Ctrl Pts',(0.00326794931492861,-0.0319739230346488,
0.0709185134696356));
#73507=CARTESIAN_POINT('Ctrl Pts',(0.00322438401647163,-0.0318646057455572,
0.0709859729897772));
#73508=CARTESIAN_POINT('Ctrl Pts',(0.00324706500675709,-0.0321934096636618,
0.07080151182966));
#73509=CARTESIAN_POINT('Ctrl Pts',(0.00320088674522905,-0.0320835708272592,
0.0708687655603509));
#73510=CARTESIAN_POINT('Ctrl Pts',(0.00315612708143066,-0.0319739230346488,
0.0709369359378671));
#73511=CARTESIAN_POINT('Ctrl Pts',(0.00311283658841121,-0.0318646057455572,
0.0710059313478667));
#73512=CARTESIAN_POINT('Ctrl Pts',(0.00313478800013228,-0.0321934096636618,
0.070816842796619));
#73513=CARTESIAN_POINT('Ctrl Pts',(0.00308882116458686,-0.0320835708272592,
0.0708856449147348));
#73514=CARTESIAN_POINT('Ctrl Pts',(0.00304430484793271,-0.0319739230346488,
0.0709553584060986));
#73515=CARTESIAN_POINT('Ctrl Pts',(0.00300128916035079,-0.0318646057455572,
0.0710258897059563));
#73516=CARTESIAN_POINT('',(0.00312767969950581,-0.0321763980308448,0.0708275069825419));
#73517=CARTESIAN_POINT('',(0.00313478800011415,-0.0321934096636184,0.0708168427966462));
#73518=CARTESIAN_POINT('Origin',(0.016557473997587,-0.032638623064701,0.0804953256685402));
#73519=CARTESIAN_POINT('Ctrl Pts',(0.0031276797021428,-0.0321763980306271,
0.0708275069842942));
#73520=CARTESIAN_POINT('Ctrl Pts',(0.00316341756719317,-0.032125959617499,
0.0708512732715633));
#73521=CARTESIAN_POINT('Ctrl Pts',(0.00319853622736263,-0.0320749164631742,
0.0708746277770612));
#73522=CARTESIAN_POINT('Ctrl Pts',(0.00326756340033043,-0.0319716057793889,
0.070920532019517));
#73523=CARTESIAN_POINT('Ctrl Pts',(0.00330144501778713,-0.0319193786690074,
0.0709430638706159));
#73524=CARTESIAN_POINT('Ctrl Pts',(0.00333471940743654,-0.0318665617525257,
0.070965191904901));
#73525=CARTESIAN_POINT('',(0.00330219872248395,-0.0321934096636663,0.0707939835458791));
#73526=CARTESIAN_POINT('Origin',(0.00812378219310841,-0.0315241814719618,
0.07415));
#73527=CARTESIAN_POINT('',(0.00312767969919601,-0.0322104233323785,0.070827506982336));
#73528=CARTESIAN_POINT('',(0.00312059419090078,-0.0321934096636183,0.0708381863255016));
#73529=CARTESIAN_POINT('Origin',(0.0165875939923736,-0.0326387231199789,
0.0804614432059535));
#73530=CARTESIAN_POINT('Origin',(0.0172369298668578,-0.0326386244598137,
0.0794736183952894));
#73531=CARTESIAN_POINT('Origin',(0.01721732674277,-0.032638724241897,0.0795144951905481));
#73532=CARTESIAN_POINT('Ctrl Pts',(0.00342582656346833,-0.0327445246967098,
0.0708322691637306));
#73533=CARTESIAN_POINT('Ctrl Pts',(0.00330069629937572,-0.032443687833936,
0.0710094554569059));
#73534=CARTESIAN_POINT('Ctrl Pts',(0.00318926791291908,-0.0321434074405927,
0.071195563705441));
#73535=CARTESIAN_POINT('Ctrl Pts',(0.00328608384940243,-0.0327445246967098,
0.0710395659892381));
#73536=CARTESIAN_POINT('Ctrl Pts',(0.00316877191289618,-0.032443687833936,
0.0712220227650352));
#73537=CARTESIAN_POINT('Ctrl Pts',(0.00306553663727474,-0.0321434074405927,
0.0714127976149198));
#73538=CARTESIAN_POINT('',(0.00326663203070031,-0.0326943950436612,0.071070029659263));
#73539=CARTESIAN_POINT('',(0.00314419377156412,-0.0323666188837389,0.0712721841351429));
#73540=CARTESIAN_POINT('Origin',(0.0175044134070871,-0.0326395579110853,
0.0800083538704801));
#73541=CARTESIAN_POINT('Origin',(-0.00641834808919296,-0.0321933825603042,
0.065745777979453));
#73542=CARTESIAN_POINT('',(0.00320791644643815,-0.0321934096532688,0.0711646375500956));
#73543=CARTESIAN_POINT('',(0.00317664322635874,-0.0321934096584274,0.071218750728266));
#73544=CARTESIAN_POINT('',(0.00333471940510188,-0.0325210109756239,0.070965191903343));
#73545=CARTESIAN_POINT('Origin',(0.017225854936219,-0.0326393129159402,
0.0804002589717525));
#73546=CARTESIAN_POINT('',(0.00333585063525292,-0.0326943950436595,0.0709659441906129));
#73547=CARTESIAN_POINT('Origin',(-0.00587567575929243,-0.0326943765538164,
0.0648401219455952));
#73548=CARTESIAN_POINT('',(0.00330124133298662,-0.0326943950436703,0.071017986924948));
#73549=CARTESIAN_POINT('Ctrl Pts',(0.00326175000838405,-0.0325229783203769,
0.0706342293825203));
#73550=CARTESIAN_POINT('Ctrl Pts',(0.00321328518730691,-0.032413025309245,
0.0707012523898611));
#73551=CARTESIAN_POINT('Ctrl Pts',(0.00316621417387347,-0.0323031222208069,
0.0707692677889311));
#73552=CARTESIAN_POINT('Ctrl Pts',(0.00312059418842563,-0.0321934096576658,
0.0708381863292408));
#73553=CARTESIAN_POINT('Ctrl Pts',(0.00328648256885509,-0.0325229783203769,
0.0707448161931664));
#73554=CARTESIAN_POINT('Ctrl Pts',(0.00323954218454434,-0.032413025309245,
0.070811498262702));
#73555=CARTESIAN_POINT('Ctrl Pts',(0.00319398832393011,-0.0323031222208069,
0.0708791412407439));
#73556=CARTESIAN_POINT('Ctrl Pts',(0.00314987628082275,-0.0321934096576658,
0.0709476564224224));
#73557=CARTESIAN_POINT('Ctrl Pts',(0.00331121512932613,-0.0325229783203769,
0.0708554030038125));
#73558=CARTESIAN_POINT('Ctrl Pts',(0.00326579918178176,-0.032413025309245,
0.0709217441355429));
#73559=CARTESIAN_POINT('Ctrl Pts',(0.00322176247398675,-0.0323031222208069,
0.0709890146925567));
#73560=CARTESIAN_POINT('Ctrl Pts',(0.00317915837321986,-0.0321934096576658,
0.071057126515604));
#73561=CARTESIAN_POINT('Ctrl Pts',(0.00333594768979717,-0.0325229783203769,
0.0709659898144587));
#73562=CARTESIAN_POINT('Ctrl Pts',(0.00329205617901919,-0.032413025309245,
0.0710319900083838));
#73563=CARTESIAN_POINT('Ctrl Pts',(0.00324953662404339,-0.0323031222208069,
0.0710988881443695));
#73564=CARTESIAN_POINT('Ctrl Pts',(0.00320844046561698,-0.0321934096576658,
0.0711665966087856));
#73565=CARTESIAN_POINT('',(0.00316425531880832,-0.0321934096584275,0.0710014119373104));
#73566=CARTESIAN_POINT('Ctrl Pts',(0.00312767970208687,-0.0322104233328928,
0.0708275069842569));
#73567=CARTESIAN_POINT('Ctrl Pts',(0.00316346599253226,-0.0322609421831346,
0.0708513054752362));
#73568=CARTESIAN_POINT('Ctrl Pts',(0.00319860830931172,-0.0323120888240686,
0.0708746757127897));
#73569=CARTESIAN_POINT('Ctrl Pts',(0.00326763600488211,-0.0324156524631813,
0.0709205803027851));
#73570=CARTESIAN_POINT('Ctrl Pts',(0.0033014930096676,-0.0324680267167311,
0.0709430957860314));
#73571=CARTESIAN_POINT('Ctrl Pts',(0.00333471940513553,-0.0325210109755913,
0.0709651919033707));
#73572=CARTESIAN_POINT('Origin',(0.0132379182114124,-0.0262834582512268,
0.0681709533682772));
#73573=CARTESIAN_POINT('Origin',(0.00208133209419324,-0.0342770788205475,
0.0635995452934657));
#73574=CARTESIAN_POINT('Ctrl Pts',(0.00326861992818894,-0.0326943950436604,
0.071069629716258));
#73575=CARTESIAN_POINT('Ctrl Pts',(0.00322616665244976,-0.0325844576448134,
0.0711365429518124));
#73576=CARTESIAN_POINT('Ctrl Pts',(0.00318509424764331,-0.0324744968375322,
0.0712043389262659));
#73577=CARTESIAN_POINT('Ctrl Pts',(0.00314545414001204,-0.0323646534831894,
0.0712729300496142));
#73578=CARTESIAN_POINT('Ctrl Pts',(0.00315752727481116,-0.0326943950436604,
0.0710919803302739));
#73579=CARTESIAN_POINT('Ctrl Pts',(0.00311538203242263,-0.0325844576448134,
0.0711604246308018));
#73580=CARTESIAN_POINT('Ctrl Pts',(0.0030746493477007,-0.0324744968375322,
0.0712297454079498));
#73581=CARTESIAN_POINT('Ctrl Pts',(0.00303538018467171,-0.0323646534831894,
0.0712998531240512));
#73582=CARTESIAN_POINT('Ctrl Pts',(0.00304643462143338,-0.0326943950436604,
0.0711143309442899));
#73583=CARTESIAN_POINT('Ctrl Pts',(0.00300459741239551,-0.0325844576448134,
0.0711843063097911));
#73584=CARTESIAN_POINT('Ctrl Pts',(0.0029642044477581,-0.0324744968375322,
0.0712551518896336));
#73585=CARTESIAN_POINT('Ctrl Pts',(0.00292530622933137,-0.0323646534831894,
0.0713267761984882));
#73586=CARTESIAN_POINT('Ctrl Pts',(0.0029353419680556,-0.0326943950436604,
0.0711366815583059));
#73587=CARTESIAN_POINT('Ctrl Pts',(0.00289381279236838,-0.0325844576448134,
0.0712081879887805));
#73588=CARTESIAN_POINT('Ctrl Pts',(0.00285375954781549,-0.0324744968375322,
0.0712805583713175));
#73589=CARTESIAN_POINT('Ctrl Pts',(0.00281523227399103,-0.0323646534831894,
0.0713536992729253));
#73590=CARTESIAN_POINT('',(0.00292891730365027,-0.032677355999133,0.0711477710346538));
#73591=CARTESIAN_POINT('',(0.00293534196805522,-0.0326943950436594,0.0711366815583065));
#73592=CARTESIAN_POINT('Origin',(0.0173309690388185,-0.0326395670637737,
0.0794130124607109));
#73593=CARTESIAN_POINT('Ctrl Pts',(0.00292891730654715,-0.0326773559987413,
0.0711477710363262));
#73594=CARTESIAN_POINT('Ctrl Pts',(0.00296610685216895,-0.0326267922586144,
0.0711692637090808));
#73595=CARTESIAN_POINT('Ctrl Pts',(0.00300263723995047,-0.0325756109579706,
0.0711903754397316));
#73596=CARTESIAN_POINT('Ctrl Pts',(0.00307441078905216,-0.0324719985462362,
0.0712318549839823));
#73597=CARTESIAN_POINT('Ctrl Pts',(0.0031096251639229,-0.0324196091621772,
0.0712522061612474));
#73598=CARTESIAN_POINT('Ctrl Pts',(0.00314419377160632,-0.0323666188837756,
0.0712721841351673));
#73599=CARTESIAN_POINT('',(0.00310098699938777,-0.0326943950436702,0.0711033556087947));
#73600=CARTESIAN_POINT('Origin',(0.00812378219310841,-0.0315241814719618,
0.07415));
#73601=CARTESIAN_POINT('',(0.00292891730368791,-0.0327114338379873,0.0711477710346757));
#73602=CARTESIAN_POINT('',(0.00292251633834769,-0.0326943950436593,0.0711588742072384));
#73603=CARTESIAN_POINT('Origin',(0.0173529681295403,-0.0326395666107975,
0.0793734000170662));
#73604=CARTESIAN_POINT('Origin',(0.0172806936696031,-0.0326395680226932,
0.0795000104820588));
#73605=CARTESIAN_POINT('Origin',(0.0172573503043656,-0.0326395676472844,
0.0795388459199229));
#73606=CARTESIAN_POINT('Ctrl Pts',(0.00322675429283235,-0.0332451089994435,
0.071133836419569));
#73607=CARTESIAN_POINT('Ctrl Pts',(0.003112997822243,-0.0329451141710254,
0.0713185308485872));
#73608=CARTESIAN_POINT('Ctrl Pts',(0.00301347646121109,-0.0326442513127493,
0.0715112691826301));
#73609=CARTESIAN_POINT('Ctrl Pts',(0.00310030507526074,-0.0332451089994435,
0.0713494995721371));
#73610=CARTESIAN_POINT('Ctrl Pts',(0.00299468247354755,-0.0329451141710254,
0.0715389631114226));
#73611=CARTESIAN_POINT('Ctrl Pts',(0.00290363110281041,-0.0326442513127493,
0.0717358443309388));
#73612=CARTESIAN_POINT('Ctrl Pts',(0.00309904058308502,-0.0332451089994435,
0.0713516562036627));
#73613=CARTESIAN_POINT('Ctrl Pts',(0.0029934993200606,-0.0329451141710254,
0.071541167434051));
#73614=CARTESIAN_POINT('Ctrl Pts',(0.0029025326492264,-0.0326442513127493,
0.0717380900824218));
#73615=CARTESIAN_POINT('',(0.0030828235692053,-0.0331951640388616,0.0713810902593082));
#73616=CARTESIAN_POINT('',(0.00297332028693037,-0.0328677532354987,0.071590533801195));
#73617=CARTESIAN_POINT('Origin',(0.0181304794375318,-0.0326402808280178,
0.0787702918631664));
#73618=CARTESIAN_POINT('Origin',(-0.00692769621469471,-0.0326944278779092,
0.0666707517731004));
#73619=CARTESIAN_POINT('',(0.00303016432206029,-0.0326943950436593,0.0714791982507606));
#73620=CARTESIAN_POINT('',(0.00300235060865649,-0.0326943950436694,0.0715351683083562));
#73621=CARTESIAN_POINT('',(0.00314419377156557,-0.0330220786163545,0.0712721841351405));
#73622=CARTESIAN_POINT('Origin',(0.0179451142460192,-0.0326396682765936,
0.0792139047477438));
#73623=CARTESIAN_POINT('',(0.00314537000600169,-0.033195164038859,0.0712728639074128));
#73624=CARTESIAN_POINT('Origin',(-0.00640595420462623,-0.0331952026560018,
0.0657529386041598));
#73625=CARTESIAN_POINT('',(0.0031140967876135,-0.0331951640388702,0.0713269770833705));
#73626=CARTESIAN_POINT('Ctrl Pts',(0.00305058654161593,-0.0330240426238172,
0.0709464572920434));
#73627=CARTESIAN_POINT('Ctrl Pts',(0.0030064546197534,-0.0329142774063519,
0.0710163455047177));
#73628=CARTESIAN_POINT('Ctrl Pts',(0.00296374548109739,-0.0328043479726691,
0.0710871808893163));
#73629=CARTESIAN_POINT('Ctrl Pts',(0.00292251633834767,-0.0326943950436593,
0.0711588742072383));
#73630=CARTESIAN_POINT('Ctrl Pts',(0.00308221411104959,-0.0330240426238172,
0.0710552728830045));
#73631=CARTESIAN_POINT('Ctrl Pts',(0.00303958122996644,-0.0329142774063519,
0.0711247253950967));
#73632=CARTESIAN_POINT('Ctrl Pts',(0.00299836287226821,-0.0328043479726691,
0.0711950938725401));
#73633=CARTESIAN_POINT('Ctrl Pts',(0.00295861432438048,-0.0326943950436593,
0.0712662896222814));
#73634=CARTESIAN_POINT('Ctrl Pts',(0.00311384168048324,-0.0330240426238172,
0.0711640884739656));
#73635=CARTESIAN_POINT('Ctrl Pts',(0.00307270784017947,-0.0329142774063519,
0.0712331052854756));
#73636=CARTESIAN_POINT('Ctrl Pts',(0.00303298026343902,-0.0328043479726691,
0.071303006855764));
#73637=CARTESIAN_POINT('Ctrl Pts',(0.00299471231041328,-0.0326943950436593,
0.0713737050373245));
#73638=CARTESIAN_POINT('Ctrl Pts',(0.00314546924991689,-0.0330240426238172,
0.0712729040649268));
#73639=CARTESIAN_POINT('Ctrl Pts',(0.00310583445039251,-0.0329142774063519,
0.0713414851758545));
#73640=CARTESIAN_POINT('Ctrl Pts',(0.00306759765460984,-0.0328043479726691,
0.0714109198389878));
#73641=CARTESIAN_POINT('Ctrl Pts',(0.00303081029644609,-0.0326943950436593,
0.0714811204523675));
#73642=CARTESIAN_POINT('',(0.00297634033021399,-0.0326943950436693,0.0713190362290095));
#73643=CARTESIAN_POINT('Ctrl Pts',(0.00292891730655267,-0.0327114338383325,
0.0711477710363293));
#73644=CARTESIAN_POINT('Ctrl Pts',(0.00296610066635426,-0.0327619876831058,
0.0711692601341597));
#73645=CARTESIAN_POINT('Ctrl Pts',(0.0030026280327023,-0.0328131562604518,
0.0711903701186562));
#73646=CARTESIAN_POINT('Ctrl Pts',(0.00307440151585102,-0.032916737585877,
0.0712318496247912));
#73647=CARTESIAN_POINT('Ctrl Pts',(0.00310961903441792,-0.0329691088920623,
0.0712522026188688));
#73648=CARTESIAN_POINT('Ctrl Pts',(0.00314419377160533,-0.0330220786163187,
0.0712721841351665));
#73649=CARTESIAN_POINT('Ctrl Pts',(0.00308478274413301,-0.0331951640388604,
0.0713805662007306));
#73650=CARTESIAN_POINT('Ctrl Pts',(0.00302752647592885,-0.0330306422010619,
0.0714847442836322));
#73651=CARTESIAN_POINT('Ctrl Pts',(0.00297462492252726,-0.0328657861914645,
0.071591199808869));
#73652=CARTESIAN_POINT('Ctrl Pts',(0.00308282356920689,-0.0331951640388604,
0.0713810902593056));
#73653=CARTESIAN_POINT('Ctrl Pts',(0.00302557813557777,-0.0330306422010619,
0.0714853088468927));
#73654=CARTESIAN_POINT('Ctrl Pts',(0.0029726890815944,-0.0328657861914645,
0.0715918043943996));
#73655=CARTESIAN_POINT('Ctrl Pts',(0.00275637233919229,-0.0331951640388604,
0.0714684125112009));
#73656=CARTESIAN_POINT('Ctrl Pts',(0.00270093223713529,-0.0330306422010619,
0.0715793802686675));
#73657=CARTESIAN_POINT('Ctrl Pts',(0.00265012592236956,-0.0328657861914645,
0.0716925446026832));
#73658=CARTESIAN_POINT('',(0.00275065666549445,-0.033178164828189,0.071479883511857));
#73659=CARTESIAN_POINT('',(0.00275637233919176,-0.0331951640388588,0.0714684125112019));
#73660=CARTESIAN_POINT('Origin',(0.0178499416008269,-0.0326412092185282,
0.0781879441317988));
#73661=CARTESIAN_POINT('Ctrl Pts',(0.00275065666710743,-0.033178164828644,
0.0714798835109781));
#73662=CARTESIAN_POINT('Ctrl Pts',(0.00278914885119287,-0.033127681154678,
0.0714990117710988));
#73663=CARTESIAN_POINT('Ctrl Pts',(0.00282694600068731,-0.0330765663497788,
0.0715177946037952));
#73664=CARTESIAN_POINT('Ctrl Pts',(0.00290118263271588,-0.0329730614463246,
0.0715546856972969));
#73665=CARTESIAN_POINT('Ctrl Pts',(0.00293759212287904,-0.0329207133374027,
0.0715727790597024));
#73666=CARTESIAN_POINT('Ctrl Pts',(0.00297332028534813,-0.0328677532289348,
0.0715905337847994));
#73667=CARTESIAN_POINT('',(0.00291959795420853,-0.0331951640388701,0.0714247513852651));
#73668=CARTESIAN_POINT('Origin',(0.00812378219310841,-0.0315241814719618,
0.07415));
#73669=CARTESIAN_POINT('',(0.00275065666659455,-0.033212160714442,0.0714798835131262));
#73670=CARTESIAN_POINT('',(0.00274496550589083,-0.0331951640388587,0.0714913666959631));
#73671=CARTESIAN_POINT('Origin',(0.0178627958923643,-0.0326413646727927,
0.0781444579374741));
#73672=CARTESIAN_POINT('Origin',(0.0172159996961188,-0.0326412100651403,
0.079463643032878));
#73673=CARTESIAN_POINT('Origin',(0.0171890976271707,-0.0326413658901262,
0.0795001477874614));
#73674=CARTESIAN_POINT('Ctrl Pts',(0.00304704076994315,-0.0337436976235975,
0.0714472566673252));
#73675=CARTESIAN_POINT('Ctrl Pts',(0.00302273188679711,-0.0336723290703325,
0.0714929176490864));
#73676=CARTESIAN_POINT('Ctrl Pts',(0.00299924823339709,-0.033601104548885,
0.0715390084841644));
#73677=CARTESIAN_POINT('Ctrl Pts',(0.00292426957994049,-0.0333736987606857,
0.0716861673904885));
#73678=CARTESIAN_POINT('Ctrl Pts',(0.00285785931192881,-0.0331450831799192,
0.0718373864980354));
#73679=CARTESIAN_POINT('Ctrl Pts',(0.00293438186405758,-0.0337436976235975,
0.0716704336619386));
#73680=CARTESIAN_POINT('Ctrl Pts',(0.0029120802686245,-0.0336723290703325,
0.0717171079149733));
#73681=CARTESIAN_POINT('Ctrl Pts',(0.00289062180376203,-0.033601104548885,
0.0717641757526222));
#73682=CARTESIAN_POINT('Ctrl Pts',(0.00282210917613855,-0.0333736987606857,
0.0719144540346219));
#73683=CARTESIAN_POINT('Ctrl Pts',(0.00276233328622339,-0.0331450831799192,
0.0720684163195151));
#73684=CARTESIAN_POINT('Ctrl Pts',(0.00293325527499873,-0.0337436976235975,
0.0716726654318848));
#73685=CARTESIAN_POINT('Ctrl Pts',(0.00291097375244277,-0.0336723290703325,
0.0717193498176322));
#73686=CARTESIAN_POINT('Ctrl Pts',(0.00288953553946568,-0.033601104548885,
0.0717664274253068));
#73687=CARTESIAN_POINT('Ctrl Pts',(0.00282108757210053,-0.0333736987606857,
0.0719167369010632));
#73688=CARTESIAN_POINT('Ctrl Pts',(0.00276137802596633,-0.0331450831799192,
0.0720707266177299));
#73689=CARTESIAN_POINT('',(0.00291890946839834,-0.0336938721132548,0.0717030784811175));
#73690=CARTESIAN_POINT('',(0.00282277333995648,-0.0333679870047996,0.0719189845050616));
#73691=CARTESIAN_POINT('Ctrl Pts',(0.002918909468406,-0.0336938721132481,
0.071703078481101));
#73692=CARTESIAN_POINT('Ctrl Pts',(0.0029093579858429,-0.0336629187933826,
0.0717233955410027));
#73693=CARTESIAN_POINT('Ctrl Pts',(0.00289992852262783,-0.0336319952300965,
0.0717437620307916));
#73694=CARTESIAN_POINT('Ctrl Pts',(0.00289062180376428,-0.0336011045488875,
0.0717641757526174));
#73695=CARTESIAN_POINT('Ctrl Pts',(0.00286726806155567,-0.0335235892595377,
0.071815400765861));
#73696=CARTESIAN_POINT('Ctrl Pts',(0.00284464585483451,-0.0334458668665494,
0.0718670142721589));
#73697=CARTESIAN_POINT('Ctrl Pts',(0.00282277334430087,-0.0333679869962417,
0.0719189844940655));
#73698=CARTESIAN_POINT('Ctrl Pts',(0.00282275545855579,-0.0333679692470412,
0.0719190252194836));
#73699=CARTESIAN_POINT('Ctrl Pts',(0.00282317548349692,-0.0333391895414745,
0.0719191955627592));
#73700=CARTESIAN_POINT('Ctrl Pts',(0.00282349153308067,-0.0333104081129247,
0.0719193202342241));
#73701=CARTESIAN_POINT('Ctrl Pts',(0.00282391191135071,-0.0332532697957439,
0.0719194801062434));
#73702=CARTESIAN_POINT('Ctrl Pts',(0.00282401933036336,-0.0332249169766573,
0.0719195166106337));
#73703=CARTESIAN_POINT('Ctrl Pts',(0.00282402538918768,-0.0331960985427074,
0.0719195116764479));
#73704=CARTESIAN_POINT('Ctrl Pts',(0.00282402546003503,-0.0331956312497407,
0.071919511584822));
#73705=CARTESIAN_POINT('Ctrl Pts',(0.00282402550318796,-0.0331951640388588,
0.0719195114822884));
#73706=CARTESIAN_POINT('',(0.00287251438400792,-0.0331951640388587,0.071804299380333));
#73707=CARTESIAN_POINT('',(0.00284826994360801,-0.0331951640388687,0.0718619054313205));
#73708=CARTESIAN_POINT('',(0.0029733202990091,-0.0335216366567745,0.0715905337914453));
#73709=CARTESIAN_POINT('Origin',(0.0183871519506845,-0.032643457152678,
0.0778980260693054));
#73710=CARTESIAN_POINT('',(0.00297453689523276,-0.0336938721132329,0.0715911383659318));
#73711=CARTESIAN_POINT('Origin',(-0.0068050609203762,-0.0336938867896239,
0.0667312724711584));
#73712=CARTESIAN_POINT('',(0.00294672318182555,-0.0336938721132539,0.0716471084235347));
#73713=CARTESIAN_POINT('Ctrl Pts',(0.00285944476230661,-0.0335235895815172,
0.0712713281856582));
#73714=CARTESIAN_POINT('Ctrl Pts',(0.00281981417719894,-0.0334144449262748,
0.0713438021549198));
#73715=CARTESIAN_POINT('Ctrl Pts',(0.00278163531901257,-0.0333049234473147,
0.0714171781260547));
#73716=CARTESIAN_POINT('Ctrl Pts',(0.00274496550589072,-0.0331951640388587,
0.071491366695963));
#73717=CARTESIAN_POINT('Ctrl Pts',(0.00289784258109682,-0.0335235895815172,
0.0713779432877689));
#73718=CARTESIAN_POINT('Ctrl Pts',(0.00285967976277552,-0.0334144449262748,
0.0714498886354565));
#73719=CARTESIAN_POINT('Ctrl Pts',(0.00282295943673785,-0.0333049234473147,
0.071522705054738));
#73720=CARTESIAN_POINT('Ctrl Pts',(0.00278773699129957,-0.0331951640388587,
0.0715963036890676));
#73721=CARTESIAN_POINT('Ctrl Pts',(0.00293624039988703,-0.0335235895815172,
0.0714845583898797));
#73722=CARTESIAN_POINT('Ctrl Pts',(0.00289954534835211,-0.0334144449262748,
0.0715559751159933));
#73723=CARTESIAN_POINT('Ctrl Pts',(0.00286428355446313,-0.0333049234473147,
0.0716282319834214));
#73724=CARTESIAN_POINT('Ctrl Pts',(0.00283050847670842,-0.0331951640388587,
0.0717012406821722));
#73725=CARTESIAN_POINT('Ctrl Pts',(0.00297463821867724,-0.0335235895815172,
0.0715911734919904));
#73726=CARTESIAN_POINT('Ctrl Pts',(0.00293941093392869,-0.0334144449262748,
0.07166206159653));
#73727=CARTESIAN_POINT('Ctrl Pts',(0.00290560767218842,-0.0333049234473147,
0.0717337589121048));
#73728=CARTESIAN_POINT('Ctrl Pts',(0.00287327996211727,-0.0331951640388587,
0.0718061776752768));
#73729=CARTESIAN_POINT('',(0.00280873994495937,-0.0331951640388687,0.071647833038158));
#73730=CARTESIAN_POINT('Ctrl Pts',(0.00275065666939384,-0.0332121607145978,
0.0714798835145147));
#73731=CARTESIAN_POINT('Ctrl Pts',(0.00278908409442409,-0.0332625444109897,
0.0714989796068384));
#73732=CARTESIAN_POINT('Ctrl Pts',(0.002826849354618,-0.0333135300747116,
0.0715177466435245));
#73733=CARTESIAN_POINT('Ctrl Pts',(0.00290108552287232,-0.0334167203140644,
0.0715546375026344));
#73734=CARTESIAN_POINT('Ctrl Pts',(0.00293752767868182,-0.0334688847587355,
0.0715727470369388));
#73735=CARTESIAN_POINT('Ctrl Pts',(0.00297332029956439,-0.0335216366562437,
0.0715905337919021));
#73736=CARTESIAN_POINT('Ctrl Pts',(0.00292083142185517,-0.033693872113248,
0.0717024325901044));
#73737=CARTESIAN_POINT('Ctrl Pts',(0.00290650499761469,-0.0336474569765003,
0.0717328871874937));
#73738=CARTESIAN_POINT('Ctrl Pts',(0.00289253606454429,-0.033601104548885,
0.0717635074069987));
#73739=CARTESIAN_POINT('Ctrl Pts',(0.00285716993767254,-0.0334837508592655,
0.0718410307627479));
#73740=CARTESIAN_POINT('Ctrl Pts',(0.00282411651876059,-0.0333660264659096,
0.0719195680476179));
#73741=CARTESIAN_POINT('Ctrl Pts',(0.00291890946840991,-0.033693872113248,
0.0717030784810931));
#73742=CARTESIAN_POINT('Ctrl Pts',(0.00290458682478371,-0.0336474569765003,
0.0717335443283136));
#73743=CARTESIAN_POINT('Ctrl Pts',(0.00289062180376203,-0.033601104548885,
0.0717641757526222));
#73744=CARTESIAN_POINT('Ctrl Pts',(0.00285526558129819,-0.0334837508592655,
0.0718417274763579));
#73745=CARTESIAN_POINT('Ctrl Pts',(0.00282222290304712,-0.0333660264659096,
0.0719202928232692));
#73746=CARTESIAN_POINT('Ctrl Pts',(0.00259666348057398,-0.033693872113248,
0.0718113723527249));
#73747=CARTESIAN_POINT('Ctrl Pts',(0.00258297471691422,-0.0336474569765003,
0.071843724412645));
#73748=CARTESIAN_POINT('Ctrl Pts',(0.00256966561292629,-0.033601104548885,
0.0718762345000432));
#73749=CARTESIAN_POINT('Ctrl Pts',(0.00253597002158697,-0.0334837508592655,
0.0719585425667899));
#73750=CARTESIAN_POINT('Ctrl Pts',(0.00250472818553856,-0.0333660264659096,
0.0720418129601336));
#73751=CARTESIAN_POINT('',(0.00259360129927857,-0.0336769361243753,0.0718225337206482));
#73752=CARTESIAN_POINT('',(0.00259858542488537,-0.0336938721132327,0.0718107264648148));
#73753=CARTESIAN_POINT('Ctrl Pts',(0.00259360129927847,-0.033676936124375,
0.0718225337206485));
#73754=CARTESIAN_POINT('Ctrl Pts',(0.00259442994721403,-0.0336797586669862,
0.071820564810069));
#73755=CARTESIAN_POINT('Ctrl Pts',(0.00259525961529622,-0.0336825812712519,
0.0718185964164901));
#73756=CARTESIAN_POINT('Ctrl Pts',(0.0025969209922326,-0.0336882266062521,
0.0718146606608783));
#73757=CARTESIAN_POINT('Ctrl Pts',(0.00259775270108091,-0.0336910493369274,
0.0718126932988885));
#73758=CARTESIAN_POINT('Ctrl Pts',(0.00259858542488982,-0.0336938721132311,
0.0718107264648143));
#73759=CARTESIAN_POINT('Ctrl Pts',(0.00259360129927861,-0.0336769361243753,
0.0718225337206483));
#73760=CARTESIAN_POINT('Ctrl Pts',(0.00263223409018507,-0.033627899461326,
0.0718387929569804));
#73761=CARTESIAN_POINT('Ctrl Pts',(0.00267141690363832,-0.0335767852527761,
0.0718552836792171));
#73762=CARTESIAN_POINT('Ctrl Pts',(0.00274820223265939,-0.0334733171841367,
0.0718876000297085));
#73763=CARTESIAN_POINT('Ctrl Pts',(0.00278585051157554,-0.0334209631343279,
0.07190344491821));
#73764=CARTESIAN_POINT('Ctrl Pts',(0.00282277334565376,-0.0333679869844681,
0.0719189844914907));
#73765=CARTESIAN_POINT('',(0.00275874744665185,-0.0336938721132538,0.0717569024729762));
#73766=CARTESIAN_POINT('Origin',(0.00812378219310841,-0.0315241814719618,
0.07415));
#73767=CARTESIAN_POINT('',(0.00259360130047952,-0.033710812065584,0.0718225337211568));
#73768=CARTESIAN_POINT('',(0.00258864240555081,-0.0336938721132327,0.0718343515957249));
#73769=CARTESIAN_POINT('Origin',(0.0172401493584967,-0.0345562513266994,
0.0791993224028963));
#73770=CARTESIAN_POINT('Ctrl Pts',(0.00258864240555639,-0.0336938721132293,
0.071834351595732));
#73771=CARTESIAN_POINT('Ctrl Pts',(0.00258946671812912,-0.0336910493412779,
0.0718323812252257));
#73772=CARTESIAN_POINT('Ctrl Pts',(0.00259029211961167,-0.0336882266084272,
0.0718304112068913));
#73773=CARTESIAN_POINT('Ctrl Pts',(0.00259194508622508,-0.0336825812712832,
0.0718264719098986));
#73774=CARTESIAN_POINT('Ctrl Pts',(0.00259277265133854,-0.0336797586670018,
0.0718245026312384));
#73775=CARTESIAN_POINT('Ctrl Pts',(0.0025936012992787,-0.033676936124375,
0.071822533720648));
#73776=CARTESIAN_POINT('Origin',(0.0181072094118419,-0.0345562516517652,
0.0771391352255455));
#73777=CARTESIAN_POINT('Ctrl Pts',(0.00288737325788412,-0.0342436276873911,
0.0717713141310582));
#73778=CARTESIAN_POINT('Ctrl Pts',(0.00279765964138925,-0.0339430054201811,
0.071968808549787));
#73779=CARTESIAN_POINT('Ctrl Pts',(0.00272307698070054,-0.0336441434784053,
0.072172499504761));
#73780=CARTESIAN_POINT('Ctrl Pts',(0.00278894799474185,-0.0342436276873911,
0.0720011237643971));
#73781=CARTESIAN_POINT('Ctrl Pts',(0.00270790179145247,-0.0339430054201811,
0.0722023303531213));
#73782=CARTESIAN_POINT('Ctrl Pts',(0.00264224153661118,-0.0336441434784053,
0.0724090700671285));
#73783=CARTESIAN_POINT('Ctrl Pts',(0.00278796374211043,-0.0342436276873911,
0.0720034218607305));
#73784=CARTESIAN_POINT('Ctrl Pts',(0.0027070042129531,-0.0339430054201811,
0.0722046655711546));
#73785=CARTESIAN_POINT('Ctrl Pts',(0.00264143318217029,-0.0336441434784053,
0.0724114357727522));
#73786=CARTESIAN_POINT('',(0.00277553662236825,-0.0341934961088741,0.0720347235842427));
#73787=CARTESIAN_POINT('',(0.00269314705195942,-0.0338664212862887,0.0722562399920861));
#73788=CARTESIAN_POINT('Origin',(0.0181427398522205,-0.034561072040627,
0.0786605977649371));
#73789=CARTESIAN_POINT('Origin',(-0.00766158860517668,-0.0336938005073027,
0.0686453988303866));
#73790=CARTESIAN_POINT('',(0.00273558880092204,-0.0336938721132327,0.0721386579186026));
#73791=CARTESIAN_POINT('',(0.00271500931525608,-0.0336938721132427,0.0721976726182162));
#73792=CARTESIAN_POINT('',(0.00282277334565588,-0.0340203938281605,0.0719189844914858));
#73793=CARTESIAN_POINT('Origin',(0.017886382235818,-0.0345589643246135,
0.0790678047230892));
#73794=CARTESIAN_POINT('',(0.00282402550318816,-0.0341934961088741,0.0719195114822878));
#73795=CARTESIAN_POINT('Origin',(-0.00733256363980539,-0.0341934220717646,
0.0676449453940501));
#73796=CARTESIAN_POINT('',(0.00279978106278821,-0.0341934961088841,0.0719771175332752));
#73797=CARTESIAN_POINT('Ctrl Pts',(0.00268908059037142,-0.0340223579322397,
0.0716075565907498));
#73798=CARTESIAN_POINT('Ctrl Pts',(0.00265401366478708,-0.0339125849573575,
0.0716825153001484));
#73799=CARTESIAN_POINT('Ctrl Pts',(0.0026205228514299,-0.0338030433565231,
0.0717581471408051));
#73800=CARTESIAN_POINT('Ctrl Pts',(0.00258864240555047,-0.0336938721132327,
0.0718343515957243));
#73801=CARTESIAN_POINT('Ctrl Pts',(0.00273409702293709,-0.0340223579322397,
0.0717115503435881));
#73802=CARTESIAN_POINT('Ctrl Pts',(0.00270046444243147,-0.0339125849573575,
0.0717858881589738));
#73803=CARTESIAN_POINT('Ctrl Pts',(0.00266839411519205,-0.0338030433565231,
0.0718608698543025));
#73804=CARTESIAN_POINT('Ctrl Pts',(0.00263791855360951,-0.0336938721132327,
0.0719363959050354));
#73805=CARTESIAN_POINT('Ctrl Pts',(0.00277911345550275,-0.0340223579322397,
0.0718155440964263));
#73806=CARTESIAN_POINT('Ctrl Pts',(0.00274691522007587,-0.0339125849573575,
0.0718892610177992));
#73807=CARTESIAN_POINT('Ctrl Pts',(0.00271626537895419,-0.0338030433565231,
0.0719635925677999));
#73808=CARTESIAN_POINT('Ctrl Pts',(0.00268719470166855,-0.0336938721132327,
0.0720384402143466));
#73809=CARTESIAN_POINT('Ctrl Pts',(0.00282412988806841,-0.0340223579322397,
0.0719195378492646));
#73810=CARTESIAN_POINT('Ctrl Pts',(0.00279336599772027,-0.0339125849573575,
0.0719926338766246));
#73811=CARTESIAN_POINT('Ctrl Pts',(0.00276413664271634,-0.0338030433565231,
0.0720663152812973));
#73812=CARTESIAN_POINT('Ctrl Pts',(0.00273647084972759,-0.0336938721132327,
0.0721404845236578));
#73813=CARTESIAN_POINT('',(0.00266211560324642,-0.0336938721132427,0.0719865047571738));
#73814=CARTESIAN_POINT('Ctrl Pts',(0.0025936013037948,-0.0337108120662688,
0.0718225337225488));
#73815=CARTESIAN_POINT('Ctrl Pts',(0.0026332335812827,-0.0337611408994398,
0.0718392136090115));
#73816=CARTESIAN_POINT('Ctrl Pts',(0.00267214265763427,-0.033812108878153,
0.0718555891245521));
#73817=CARTESIAN_POINT('Ctrl Pts',(0.00274854985358115,-0.0339153382773235,
0.0718877463316092));
#73818=CARTESIAN_POINT('Ctrl Pts',(0.00278601564827816,-0.0339675558473108,
0.0719035144186683));
#73819=CARTESIAN_POINT('Ctrl Pts',(0.00282277334569056,-0.0340203938281304,
0.0719189844915061));
#73820=CARTESIAN_POINT('Ctrl Pts',(0.00277741475298016,-0.0341934961088741,
0.0720339580731138));
#73821=CARTESIAN_POINT('Ctrl Pts',(0.00273366725318469,-0.0340287516182428,
0.0721444900080067));
#73822=CARTESIAN_POINT('Ctrl Pts',(0.0026945255035161,-0.0338644633275951,
0.0722567356128313));
#73823=CARTESIAN_POINT('Ctrl Pts',(0.00277553662236835,-0.0341934961088741,
0.0720347235842427));
#73824=CARTESIAN_POINT('Ctrl Pts',(0.00273180494891239,-0.0340287516182428,
0.0721452943480065));
#73825=CARTESIAN_POINT('Ctrl Pts',(0.0026926806168867,-0.0338644633275951,
0.0722575780944087));
#73826=CARTESIAN_POINT('Ctrl Pts',(0.00246260393800087,-0.0341934961088741,
0.0721622724623588));
#73827=CARTESIAN_POINT('Ctrl Pts',(0.00242150923711545,-0.0340287516182428,
0.0722793128628397));
#73828=CARTESIAN_POINT('Ctrl Pts',(0.00238528701941142,-0.0338644633275951,
0.0723979517297015));
#73829=CARTESIAN_POINT('',(0.00245837103217539,-0.0341764758832382,0.0721743693745735));
#73830=CARTESIAN_POINT('',(0.00246260393800085,-0.034193496108874,0.0721622724623588));
#73831=CARTESIAN_POINT('Origin',(0.0179241615674465,-0.034562102639047,
0.0781099108692202));
#73832=CARTESIAN_POINT('Ctrl Pts',(0.00245837103351531,-0.0341764758837464,
0.0721743693733416));
#73833=CARTESIAN_POINT('Ctrl Pts',(0.00249890174612151,-0.0341260050040274,
0.0721885031462305));
#73834=CARTESIAN_POINT('Ctrl Pts',(0.00253872795190624,-0.0340749269147865,
0.0722023912047264));
#73835=CARTESIAN_POINT('Ctrl Pts',(0.00261700215513479,-0.0339715436305901,
0.0722296868295073));
#73836=CARTESIAN_POINT('Ctrl Pts',(0.0026554204551241,-0.0339192778237013,
0.0722430840460927));
#73837=CARTESIAN_POINT('Ctrl Pts',(0.00269314705147574,-0.0338664212854263,
0.0722562399900086));
#73838=CARTESIAN_POINT('',(0.00261907028019455,-0.0341934961088841,0.0720984980233107));
#73839=CARTESIAN_POINT('Origin',(0.00812378219310841,-0.0315241814719618,
0.07415));
#73840=CARTESIAN_POINT('',(0.00245837103259312,-0.0342105180190372,0.0721743693756105));
#73841=CARTESIAN_POINT('',(0.00245416397318747,-0.0341934961088739,0.0721864753018193));
#73842=CARTESIAN_POINT('Origin',(0.0179439291967614,-0.0345621704431894,
0.0780691208298281));
#73843=CARTESIAN_POINT('Origin',(0.0182614037932373,-0.0345621038666668,
0.0771428264373991));
#73844=CARTESIAN_POINT('Origin',(0.0182515158399669,-0.0345621716292033,
0.0771870617550893));
#73845=CARTESIAN_POINT('Ctrl Pts',(0.00273608271184164,-0.0346945769586965,
0.0721372415564544));
#73846=CARTESIAN_POINT('Ctrl Pts',(0.00269392468037706,-0.0345275153362944,
0.0722500890792067));
#73847=CARTESIAN_POINT('Ctrl Pts',(0.00265530469540775,-0.0343603235965186,
0.0723642916213943));
#73848=CARTESIAN_POINT('Ctrl Pts',(0.00262033195770613,-0.034193496108874,
0.0724795097249739));
#73849=CARTESIAN_POINT('Ctrl Pts',(0.00270847876056665,-0.0346945769586965,
0.0722163999435012));
#73850=CARTESIAN_POINT('Ctrl Pts',(0.00266797873321206,-0.0345275153362944,
0.072329825642065));
#73851=CARTESIAN_POINT('Ctrl Pts',(0.00263103536429461,-0.0343603235965186,
0.0724445543669067));
#73852=CARTESIAN_POINT('Ctrl Pts',(0.00259775287277131,-0.034193496108874,
0.0725602451774675));
#73853=CARTESIAN_POINT('Ctrl Pts',(0.00268087480929167,-0.0346945769586965,
0.0722955583305481));
#73854=CARTESIAN_POINT('Ctrl Pts',(0.00264203278604706,-0.0345275153362944,
0.0724095622049234));
#73855=CARTESIAN_POINT('Ctrl Pts',(0.00260676603318147,-0.0343603235965186,
0.0725248171124188));
#73856=CARTESIAN_POINT('Ctrl Pts',(0.00257517378783649,-0.034193496108874,
0.0726409806299595));
#73857=CARTESIAN_POINT('Ctrl Pts',(0.00265327085801668,-0.0346945769586965,
0.0723747167175948));
#73858=CARTESIAN_POINT('Ctrl Pts',(0.00261608683888205,-0.0345275153362944,
0.0724892987677815));
#73859=CARTESIAN_POINT('Ctrl Pts',(0.00258249670206834,-0.0343603235965186,
0.0726050798579316));
#73860=CARTESIAN_POINT('Ctrl Pts',(0.00255259470290167,-0.034193496108874,
0.0727217160824547));
#73861=CARTESIAN_POINT('',(0.00265327085821636,-0.0346945769586966,0.0723747167170228));
#73862=CARTESIAN_POINT('',(0.00258495299585706,-0.0343667727831436,0.0726009692953471));
#73863=CARTESIAN_POINT('Origin',(0.0187013709783458,-0.0345626457062745,
0.0773902655172281));
#73864=CARTESIAN_POINT('Origin',(-0.00805881704567561,-0.0341934771029153,
0.0696242573967093));
#73865=CARTESIAN_POINT('',(0.0026199279555237,-0.034193496108874,0.0724809543051726));
#73866=CARTESIAN_POINT('',(0.00260309464241975,-0.0341934961088841,0.0725411447493545));
#73867=CARTESIAN_POINT('',(0.00269314705287547,-0.0345211942962717,0.0722562399905395));
#73868=CARTESIAN_POINT('Origin',(0.018539914317741,-0.0345625596119444,
0.0778431700731569));
#73869=CARTESIAN_POINT('',(0.00269442982957011,-0.0346945769586887,0.0722566873178099));
#73870=CARTESIAN_POINT('Origin',(-0.00775217934461158,-0.0346945685853861,
0.0686137665159061));
#73871=CARTESIAN_POINT('',(0.00267385034390324,-0.0346945769587026,0.0723157020174264));
#73872=CARTESIAN_POINT('Ctrl Pts',(0.00254016303781951,-0.0345231616327842,
0.0719538221545793));
#73873=CARTESIAN_POINT('Ctrl Pts',(0.00250989181819146,-0.0344132092796988,
0.072030784483528));
#73874=CARTESIAN_POINT('Ctrl Pts',(0.00248121406548646,-0.034303273855898,
0.0721083689778747));
#73875=CARTESIAN_POINT('Ctrl Pts',(0.0024541639731874,-0.0341934961088739,
0.0721864753018193));
#73876=CARTESIAN_POINT('Ctrl Pts',(0.00259162039115611,-0.0345231616327842,
0.072054783914301));
#73877=CARTESIAN_POINT('Ctrl Pts',(0.00256274078724304,-0.0344132092796988,
0.07213103697608));
#73878=CARTESIAN_POINT('Ctrl Pts',(0.0025354399078201,-0.034303273855898,
0.0722078834553787));
#73879=CARTESIAN_POINT('Ctrl Pts',(0.00250975020665528,-0.0341934961088739,
0.0722852240070632));
#73880=CARTESIAN_POINT('Ctrl Pts',(0.00264307774449271,-0.0345231616327842,
0.0721557456740226));
#73881=CARTESIAN_POINT('Ctrl Pts',(0.00261558975629461,-0.0344132092796988,
0.0722312894686321));
#73882=CARTESIAN_POINT('Ctrl Pts',(0.00258966575015374,-0.034303273855898,
0.0723073979328828));
#73883=CARTESIAN_POINT('Ctrl Pts',(0.00256533644012315,-0.0341934961088739,
0.0723839727123072));
#73884=CARTESIAN_POINT('Ctrl Pts',(0.00269453509782931,-0.0345231616327842,
0.0722567074337443));
#73885=CARTESIAN_POINT('Ctrl Pts',(0.00266843872534619,-0.0344132092796988,
0.0723315419611842));
#73886=CARTESIAN_POINT('Ctrl Pts',(0.00264389159248737,-0.034303273855898,
0.0724069124103868));
#73887=CARTESIAN_POINT('Ctrl Pts',(0.00262092267359103,-0.0341934961088739,
0.0724827214175512));
#73888=CARTESIAN_POINT('',(0.00253704596436558,-0.0341934961088839,0.0723337148035059));
#73889=CARTESIAN_POINT('Ctrl Pts',(0.00245837103584969,-0.0342105180195391,
0.072174369376743));
#73890=CARTESIAN_POINT('Ctrl Pts',(0.00249894730831671,-0.0342610556241328,
0.072188519051716));
#73891=CARTESIAN_POINT('Ctrl Pts',(0.00253879546055414,-0.0343122189870209,
0.0722024148180876));
#73892=CARTESIAN_POINT('Ctrl Pts',(0.0026170704546704,-0.03441581196952,
0.0722297107143816));
#73893=CARTESIAN_POINT('Ctrl Pts',(0.00265546528150917,-0.0344681990450108,
0.0722430996800844));
#73894=CARTESIAN_POINT('Ctrl Pts',(0.00269314705289859,-0.0345211942962537,
0.0722562399905454));
#73895=CARTESIAN_POINT('Ctrl Pts',(0.00265509676874847,-0.0346945769586931,
0.072373835003588));
#73896=CARTESIAN_POINT('Ctrl Pts',(0.0026183758142217,-0.034529677707698,
0.072486896205219));
#73897=CARTESIAN_POINT('Ctrl Pts',(0.0025863591606494,-0.0343648066251421,
0.0726013785082602));
#73898=CARTESIAN_POINT('Ctrl Pts',(0.00265327085821918,-0.0346945769586931,
0.0723747167170142));
#73899=CARTESIAN_POINT('Ctrl Pts',(0.00261656813249361,-0.034529677707698,
0.0724878156680534));
#73900=CARTESIAN_POINT('Ctrl Pts',(0.00258457125236397,-0.0343648066251421,
0.0726023349348334));
#73901=CARTESIAN_POINT('Ctrl Pts',(0.00234896453534388,-0.0346945769586931,
0.072521663112384));
#73902=CARTESIAN_POINT('Ctrl Pts',(0.00231529982236665,-0.034529677707698,
0.0726410533813284));
#73903=CARTESIAN_POINT('Ctrl Pts',(0.00228659838499166,-0.0343648066251421,
0.0727617330263024));
#73904=CARTESIAN_POINT('',(0.00234549955334111,-0.0346775396664966,0.0725340019405017));
#73905=CARTESIAN_POINT('',(0.00234896453534292,-0.0346945769586885,0.0725216631123873));
#73906=CARTESIAN_POINT('Origin',(0.0183740712136008,-0.0345626618126048,
0.0768580961612871));
#73907=CARTESIAN_POINT('Ctrl Pts',(0.00234549955467211,-0.0346775396670096,
0.0725340019392594));
#73908=CARTESIAN_POINT('Ctrl Pts',(0.00238687031335062,-0.0346269749928187,
0.072545571983955));
#73909=CARTESIAN_POINT('Ctrl Pts',(0.00242750583100824,-0.0345757902890786,
0.0725569363685466));
#73910=CARTESIAN_POINT('Ctrl Pts',(0.00250733980358265,-0.0344721681088186,
0.0725792633427411));
#73911=CARTESIAN_POINT('Ctrl Pts',(0.0025465069583118,-0.0344197714290122,
0.0725902171845494));
#73912=CARTESIAN_POINT('Ctrl Pts',(0.00258495299581539,-0.0343667727830592,
0.0726009692950803));
#73913=CARTESIAN_POINT('',(0.00250111769678964,-0.0346945769587026,0.0724481899147151));
#73914=CARTESIAN_POINT('Origin',(0.00812378219310841,-0.0315241814719618,
0.07415));
#73915=CARTESIAN_POINT('',(0.0023454995542768,-0.0347116136489615,0.0725340019415307));
#73916=CARTESIAN_POINT('',(0.00234206093373591,-0.0346945769586885,0.0725463481428481));
#73917=CARTESIAN_POINT('Origin',(0.018384466689097,-0.034562668345578,0.0768139913977689));
#73918=CARTESIAN_POINT('Origin',(0.0182918108157433,-0.0345626629385285,
0.0771522428356373));
#73919=CARTESIAN_POINT('Origin',(0.0182778130545486,-0.0345626694088764,
0.0771953402433519));
#73920=CARTESIAN_POINT('Ctrl Pts',(0.0026312075774452,-0.0352450361874068,
0.0724440144440831));
#73921=CARTESIAN_POINT('Ctrl Pts',(0.0025668652763957,-0.0349452760959493,
0.0726511702949823));
#73922=CARTESIAN_POINT('Ctrl Pts',(0.00251830959135272,-0.034644428984174,
0.072862584163298));
#73923=CARTESIAN_POINT('Ctrl Pts',(0.00263051226227906,-0.0352450361874068,
0.0724464418216433));
#73924=CARTESIAN_POINT('Ctrl Pts',(0.0025662615112765,-0.0349452760959493,
0.0726536238967844));
#73925=CARTESIAN_POINT('Ctrl Pts',(0.00251779909151362,-0.034644428984174,
0.0728650570189173));
#73926=CARTESIAN_POINT('Ctrl Pts',(0.00256166917652225,-0.0352450361874068,
0.0726867762335436));
#73927=CARTESIAN_POINT('Ctrl Pts',(0.00250648278660377,-0.0349452760959493,
0.07289655476827));
#73928=CARTESIAN_POINT('Ctrl Pts',(0.0024672545529891,-0.034644428984174,
0.0731098942089546));
#73929=CARTESIAN_POINT('Ctrl Pts',(0.00256098074566468,-0.0352450361874068,
0.0726891795776626));
#73930=CARTESIAN_POINT('Ctrl Pts',(0.00250588499935705,-0.0349452760959493,
0.0728989840769848));
#73931=CARTESIAN_POINT('Ctrl Pts',(0.00246674910760385,-0.034644428984174,
0.073112342580855));
#73932=CARTESIAN_POINT('',(0.00255260043984588,-0.0351951634053264,0.0727216841474485));
#73933=CARTESIAN_POINT('',(0.00249861816740813,-0.0348678972925388,0.07295181191628));
#73934=CARTESIAN_POINT('Origin',(0.018968118011654,-0.0345636767880447,
0.076028537518523));
#73935=CARTESIAN_POINT('Origin',(-0.00830877103174432,-0.0346946199341129,
0.070649785006046));
#73936=CARTESIAN_POINT('',(0.00252598831263244,-0.0346945769330288,0.0728298376351159));
#73937=CARTESIAN_POINT('',(0.00251296760331662,-0.0346945769458128,0.0728909662881075));
#73938=CARTESIAN_POINT('',(0.00258495299594239,-0.0350221583435276,0.0726009692951326));
#73939=CARTESIAN_POINT('Origin',(0.0189089051229494,-0.0345628458717638,
0.0765056509510742));
#73940=CARTESIAN_POINT('',(0.00258614498873088,-0.035195136029876,0.0726012995161749));
#73941=CARTESIAN_POINT('Origin',(-0.0080256490247682,-0.0351951838366814,
0.0696335273409525));
#73942=CARTESIAN_POINT('',(0.00255259470295588,-0.035195137132875,0.0727217160818296));
#73943=CARTESIAN_POINT('Ctrl Pts',(0.00241328159205483,-0.0350241211494343,
0.0723087550718622));
#73944=CARTESIAN_POINT('Ctrl Pts',(0.00238791919810954,-0.0349144232818962,
0.0723874148762453));
#73945=CARTESIAN_POINT('Ctrl Pts',(0.00236416757791286,-0.0348045283579412,
0.0724666460211186));
#73946=CARTESIAN_POINT('Ctrl Pts',(0.00234206093076571,-0.0346945769439157,
0.0725463481535567));
#73947=CARTESIAN_POINT('Ctrl Pts',(0.00247097687574631,-0.0350241211494343,
0.0724062865849373));
#73948=CARTESIAN_POINT('Ctrl Pts',(0.00244695793840415,-0.0349144232818962,
0.0724841516604435));
#73949=CARTESIAN_POINT('Ctrl Pts',(0.00242453415132036,-0.0348045283579412,
0.0725625598305485));
#73950=CARTESIAN_POINT('Ctrl Pts',(0.0024037379737839,-0.0346945769439157,
0.0726414117331626));
#73951=CARTESIAN_POINT('Ctrl Pts',(0.00252867215943778,-0.0350241211494343,
0.0725038180980124));
#73952=CARTESIAN_POINT('Ctrl Pts',(0.00250599667869876,-0.0349144232818962,
0.0725808884446417));
#73953=CARTESIAN_POINT('Ctrl Pts',(0.00248490072472786,-0.0348045283579412,
0.0726584736399783));
#73954=CARTESIAN_POINT('Ctrl Pts',(0.0024654150168021,-0.0346945769439157,
0.0727364753127685));
#73955=CARTESIAN_POINT('Ctrl Pts',(0.00258636744312925,-0.0350241211494343,
0.0726013496110874));
#73956=CARTESIAN_POINT('Ctrl Pts',(0.00256503541899336,-0.0349144232818962,
0.0726776252288399));
#73957=CARTESIAN_POINT('Ctrl Pts',(0.00254526729813537,-0.0348045283579412,
0.0727543874494082));
#73958=CARTESIAN_POINT('Ctrl Pts',(0.00252709205982029,-0.0346945769439157,
0.0728315388923744));
#73959=CARTESIAN_POINT('',(0.00243402462317538,-0.0346945769458128,0.0726880928886834));
#73960=CARTESIAN_POINT('Ctrl Pts',(0.00234549955743811,-0.0347116136492794,
0.0725340019424112));
#73961=CARTESIAN_POINT('Ctrl Pts',(0.00238685388341253,-0.034762154653232,
0.0725455674047919));
#73962=CARTESIAN_POINT('Ctrl Pts',(0.00242748108858528,-0.0348133084097077,
0.0725569295150907));
#73963=CARTESIAN_POINT('Ctrl Pts',(0.00250731516349295,-0.0349168561544568,
0.0725792565139786));
#73964=CARTESIAN_POINT('Ctrl Pts',(0.00254649036710825,-0.0349692089015911,
0.072590212546582));
#73965=CARTESIAN_POINT('Ctrl Pts',(0.00258495299597225,-0.0350221583435,
0.0726009692951616));
#73966=CARTESIAN_POINT('Ctrl Pts',(0.00255386961196152,-0.0351951371254874,
0.0727209984280599));
#73967=CARTESIAN_POINT('Ctrl Pts',(0.00252432590104789,-0.0350307338980917,
0.0728361528759925));
#73968=CARTESIAN_POINT('Ctrl Pts',(0.00249956689264955,-0.0348659306897818,
0.0729524299985762));
#73969=CARTESIAN_POINT('Ctrl Pts',(0.00255259470306853,-0.0351951371254874,
0.072721716081858));
#73970=CARTESIAN_POINT('Ctrl Pts',(0.0025230658291969,-0.0350307338980917,
0.0728368968877321));
#73971=CARTESIAN_POINT('Ctrl Pts',(0.00249832273456456,-0.0348659306897818,
0.0729531997325036));
#73972=CARTESIAN_POINT('Ctrl Pts',(0.00233891864385632,-0.0351951371254874,
0.0728419956063795));
#73973=CARTESIAN_POINT('Ctrl Pts',(0.00231187647368822,-0.0350307338980917,
0.0729615940307128));
#73974=CARTESIAN_POINT('Ctrl Pts',(0.00228980054282336,-0.0348659306897818,
0.0730822079409672));
#73975=CARTESIAN_POINT('Origin',(-0.00270287367950345,-0.0308609197411111,
0.0718438681262935));
#73976=CARTESIAN_POINT('',(0.00245943675900611,-0.0351951371254874,0.0727741552426069));
#73977=CARTESIAN_POINT('Origin',(0.00909886329211686,-0.0351840467441176,
0.0742129483911409));
#73978=CARTESIAN_POINT('Origin',(-0.00371869835454763,-0.0352322613820738,
0.072440018805345));
#73979=CARTESIAN_POINT('',(0.00245411436176611,-0.0351951142564653,0.0731842457529613));
#73980=CARTESIAN_POINT('',(0.00243582715934136,-0.0351951372916786,0.0733075823281499));
#73981=CARTESIAN_POINT('Origin',(0.00825783852632709,-0.035287511665086,
0.0744630656346189));
#73982=CARTESIAN_POINT('Origin',(0.0106237609097371,-0.0298325076522142,
0.0670757299530051));
#73983=CARTESIAN_POINT('Origin',(0.000904856559393061,-0.0338733559830917,
0.0698917526735384));
#73984=CARTESIAN_POINT('Ctrl Pts',(0.00410481693489538,-0.0321934096636942,
0.0700358714168625));
#73985=CARTESIAN_POINT('Ctrl Pts',(0.00403117599237873,-0.0320508460843247,
0.0701078089811792));
#73986=CARTESIAN_POINT('Ctrl Pts',(0.00395952339578597,-0.0319086045660919,
0.0701816708911563));
#73987=CARTESIAN_POINT('Ctrl Pts',(0.00389000033279445,-0.0317669892864685,
0.0702572854077693));
#73988=CARTESIAN_POINT('Ctrl Pts',(0.00404612609468526,-0.0321934096636942,
0.0700957531160981));
#73989=CARTESIAN_POINT('Ctrl Pts',(0.00397355700606964,-0.0320508460843247,
0.0701687412185063));
#73990=CARTESIAN_POINT('Ctrl Pts',(0.0039030036810822,-0.0319086045660919,
0.0702436240758665));
#73991=CARTESIAN_POINT('Ctrl Pts',(0.00383460475949915,-0.0317669892864685,
0.0703202279457344));
#73992=CARTESIAN_POINT('Ctrl Pts',(0.00398743525447512,-0.0321934096636942,
0.0701556348153335));
#73993=CARTESIAN_POINT('Ctrl Pts',(0.00391593801976054,-0.0320508460843247,
0.0702296734558335));
#73994=CARTESIAN_POINT('Ctrl Pts',(0.00384648396637842,-0.0319086045660919,
0.0703055772605765));
#73995=CARTESIAN_POINT('Ctrl Pts',(0.00377920918620383,-0.0317669892864685,
0.0703831704836995));
#73996=CARTESIAN_POINT('Ctrl Pts',(0.00392874441426499,-0.0321934096636942,
0.0702155165145691));
#73997=CARTESIAN_POINT('Ctrl Pts',(0.00385831903345145,-0.0320508460843247,
0.0702906056931606));
#73998=CARTESIAN_POINT('Ctrl Pts',(0.00378996425167463,-0.0319086045660919,
0.0703675304452866));
#73999=CARTESIAN_POINT('Ctrl Pts',(0.00372381361290853,-0.0317669892864685,
0.0704461130216646));
#74000=CARTESIAN_POINT('',(0.00392979440499592,-0.0321934096636942,0.0702144452191382));
#74001=CARTESIAN_POINT('',(0.00377164489336527,-0.0318665617511256,0.0703900763421073));
#74002=CARTESIAN_POINT('Origin',(0.0156858273485652,-0.0326371944421723,
0.0820893597144095));
#74003=CARTESIAN_POINT('Origin',(-0.00452284489056498,-0.0316939261509002,
0.063224252635214));
#74004=CARTESIAN_POINT('',(0.00401616875752808,-0.0320197221621845,0.0701244440097831));
#74005=CARTESIAN_POINT('Ctrl Pts',(0.00401600987312598,-0.0320197392094761,
0.0701245387231699));
#74006=CARTESIAN_POINT('Ctrl Pts',(0.00399552706552251,-0.0319792716576057,
0.0701454404222029));
#74007=CARTESIAN_POINT('Ctrl Pts',(0.00397511035852195,-0.0319386439829698,
0.0701665934264079));
#74008=CARTESIAN_POINT('Ctrl Pts',(0.00395474440378606,-0.031897909938163,
0.0701880258159594));
#74009=CARTESIAN_POINT('Ctrl Pts',(0.00393437885159715,-0.0318571766984924,
0.0702094577818851));
#74010=CARTESIAN_POINT('Ctrl Pts',(0.00391416626914079,-0.0318163871833565,
0.0702310589635628));
#74011=CARTESIAN_POINT('Ctrl Pts',(0.00389417360827464,-0.0317755399638303,
0.0702527526560048));
#74012=CARTESIAN_POINT('',(0.00401729062974265,-0.0321934096636183,0.070125173663373));
#74013=CARTESIAN_POINT('Origin',(0.00239233619437014,-0.0324040108403075,
0.068561306614717));
#74014=CARTESIAN_POINT('',(0.00397354251737928,-0.0321934096636663,0.0701698094412656));
#74015=CARTESIAN_POINT('Ctrl Pts',(0.00393182252542624,-0.0321934096636618,
0.0702144248500637));
#74016=CARTESIAN_POINT('Ctrl Pts',(0.00387754787690073,-0.0320835708272592,
0.0702722352409033));
#74017=CARTESIAN_POINT('Ctrl Pts',(0.00382450109291094,-0.0319739230346488,
0.0703311353103973));
#74018=CARTESIAN_POINT('Ctrl Pts',(0.00377274425957832,-0.0318646057455573,
0.0703910444911847));
#74019=CARTESIAN_POINT('Ctrl Pts',(0.00381850937687154,-0.0321934096636618,
0.0702155628874739));
#74020=CARTESIAN_POINT('Ctrl Pts',(0.00376425042276885,-0.0320835708272592,
0.0702749359549432));
#74021=CARTESIAN_POINT('Ctrl Pts',(0.00371125166361012,-0.0319739230346488,
0.0703353974698556));
#74022=CARTESIAN_POINT('Ctrl Pts',(0.00365957497074976,-0.0318646057455573,
0.0703968648718049));
#74023=CARTESIAN_POINT('Ctrl Pts',(0.00370519622831685,-0.0321934096636618,
0.0702167009248841));
#74024=CARTESIAN_POINT('Ctrl Pts',(0.00365095296863698,-0.0320835708272592,
0.070277636668983));
#74025=CARTESIAN_POINT('Ctrl Pts',(0.0035980022343093,-0.0319739230346488,
0.0703396596293139));
#74026=CARTESIAN_POINT('Ctrl Pts',(0.0035464056819212,-0.0318646057455573,
0.070402685252425));
#74027=CARTESIAN_POINT('Ctrl Pts',(0.00359188307976215,-0.0321934096636618,
0.0702178389622942));
#74028=CARTESIAN_POINT('Ctrl Pts',(0.0035376555145051,-0.0320835708272592,
0.0702803373830229));
#74029=CARTESIAN_POINT('Ctrl Pts',(0.00348475280500847,-0.0319739230346488,
0.0703439217887722));
#74030=CARTESIAN_POINT('Ctrl Pts',(0.00343323639309263,-0.0318646057455573,
0.0704085056330452));
#74031=CARTESIAN_POINT('',(0.00358349425330485,-0.0321763980308449,0.0702275281516227));
#74032=CARTESIAN_POINT('',(0.00359188307974073,-0.0321934096636184,0.0702178389623189));
#74033=CARTESIAN_POINT('Origin',(0.0156956915595299,-0.0326386231130585,
0.0815023127650536));
#74034=CARTESIAN_POINT('Ctrl Pts',(0.00358349425570071,-0.0321763980306272,
0.0702275281536921));
#74035=CARTESIAN_POINT('Ctrl Pts',(0.00361597161137929,-0.0321259596174965,
0.0702555861788765));
#74036=CARTESIAN_POINT('Ctrl Pts',(0.00364788625473379,-0.0320749164631678,
0.0702831580623622));
#74037=CARTESIAN_POINT('Ctrl Pts',(0.00371061580068031,-0.0319716057793885,
0.070337351734944));
#74038=CARTESIAN_POINT('Ctrl Pts',(0.00374140626170689,-0.0319193786690071,
0.0703639524083413));
#74039=CARTESIAN_POINT('Ctrl Pts',(0.00377164489476594,-0.0318665617525255,
0.0703900763433163));
#74040=CARTESIAN_POINT('',(0.00376083874237832,-0.0321934096636663,0.0702161420907385));
#74041=CARTESIAN_POINT('Origin',(0.00812378219310841,-0.0315241814719618,
0.07415));
#74042=CARTESIAN_POINT('',(0.00358349425302338,-0.0322104233323617,0.0702275281513797));
#74043=CARTESIAN_POINT('',(0.00357512613946538,-0.0321934096636183,0.0702372352350691));
#74044=CARTESIAN_POINT('Origin',(0.0157298205001204,-0.0326387232157297,
0.0814724724679504));
#74045=CARTESIAN_POINT('Origin',(0.0164978436301158,-0.0326386244487335,
0.0805738203269208));
#74046=CARTESIAN_POINT('Origin',(0.0164732718154305,-0.0326387242180456,
0.0806119178557787));
#74047=CARTESIAN_POINT('Ctrl Pts',(0.00387869328062491,-0.0327445246967096,
0.0702696204921284));
#74048=CARTESIAN_POINT('Ctrl Pts',(0.0037323423749724,-0.032443687833936,
0.0704297266378436));
#74049=CARTESIAN_POINT('Ctrl Pts',(0.00359846708604318,-0.0321434074405928,
0.0706004016872655));
#74050=CARTESIAN_POINT('Ctrl Pts',(0.00371407129815008,-0.0327445246967096,
0.0704577683140293));
#74051=CARTESIAN_POINT('Ctrl Pts',(0.00357481650360626,-0.032443687833936,
0.070624083279314));
#74052=CARTESIAN_POINT('Ctrl Pts',(0.00344848484014925,-0.0321434074405928,
0.0708004150016139));
#74053=CARTESIAN_POINT('',(0.00369095475257805,-0.0326943950436612,0.0704855538095802));
#74054=CARTESIAN_POINT('',(0.00354414528154417,-0.0323666188837389,0.0706707686541077));
#74055=CARTESIAN_POINT('Origin',(0.0166961978936742,-0.0326395579112711,
0.0811378638432646));
#74056=CARTESIAN_POINT('Origin',(-0.00525035045722684,-0.0321933825603105,
0.0639894352154793));
#74057=CARTESIAN_POINT('',(0.00362084464535784,-0.0321934096532689,0.0705720566748985));
#74058=CARTESIAN_POINT('',(0.00358303584436114,-0.0321934096584275,0.0706218235806995));
#74059=CARTESIAN_POINT('',(0.00377164489264482,-0.0325210109756239,0.0703900763414779));
#74060=CARTESIAN_POINT('Origin',(0.0163707172064862,-0.0326393129158769,
0.081491766021844));
#74061=CARTESIAN_POINT('',(0.00377267291611207,-0.0326943950436593,0.0703909644774707));
#74062=CARTESIAN_POINT('Origin',(-0.00459844862906292,-0.0326943765538128,
0.063158935663208));
#74063=CARTESIAN_POINT('',(0.00373181383435506,-0.0326943950436702,0.0704382591435355));
#74064=CARTESIAN_POINT('Ctrl Pts',(0.00374073148433831,-0.0325229783203769,
0.0700525780685438));
#74065=CARTESIAN_POINT('Ctrl Pts',(0.00368424861261789,-0.032413025309245,
0.0701129983267132));
#74066=CARTESIAN_POINT('Ctrl Pts',(0.00362902417828721,-0.032303122220807,
0.0701745778417256));
#74067=CARTESIAN_POINT('Ctrl Pts',(0.00357512613654111,-0.0321934096576658,
0.0702372352384686));
#74068=CARTESIAN_POINT('Ctrl Pts',(0.00375140881861494,-0.0325229783203769,
0.0701653926809355));
#74069=CARTESIAN_POINT('Ctrl Pts',(0.00369648109385924,-0.032413025309245,
0.0702256657522854));
#74070=CARTESIAN_POINT('Ctrl Pts',(0.00364280852587634,-0.032303122220807,
0.0702870659325893));
#74071=CARTESIAN_POINT('Ctrl Pts',(0.0035904570901365,-0.0321934096576658,
0.070349512146594));
#74072=CARTESIAN_POINT('Ctrl Pts',(0.00376208615289156,-0.0325229783203769,
0.0702782072933271));
#74073=CARTESIAN_POINT('Ctrl Pts',(0.00370871357510059,-0.032413025309245,
0.0703383331778576));
#74074=CARTESIAN_POINT('Ctrl Pts',(0.00365659287346548,-0.032303122220807,
0.070399554023453));
#74075=CARTESIAN_POINT('Ctrl Pts',(0.00360578804373189,-0.0321934096576658,
0.0704617890547194));
#74076=CARTESIAN_POINT('Ctrl Pts',(0.00377276348716819,-0.0325229783203769,
0.0703910219057188));
#74077=CARTESIAN_POINT('Ctrl Pts',(0.00372094605634195,-0.032413025309245,
0.0704510006034297));
#74078=CARTESIAN_POINT('Ctrl Pts',(0.00367037722105461,-0.032303122220807,
0.0705120421143167));
#74079=CARTESIAN_POINT('Ctrl Pts',(0.00362111899732728,-0.0321934096576658,
0.0705740659628447));
#74080=CARTESIAN_POINT('',(0.00359798539261125,-0.0321934096584275,0.0704046459545161));
#74081=CARTESIAN_POINT('Ctrl Pts',(0.00358349425565004,-0.0322104233328929,
0.0702275281536483));
#74082=CARTESIAN_POINT('Ctrl Pts',(0.00361601561867657,-0.0322609421831325,
0.0702556241979155));
#74083=CARTESIAN_POINT('Ctrl Pts',(0.00364795176034818,-0.0323120888240634,
0.0702832146543609));
#74084=CARTESIAN_POINT('Ctrl Pts',(0.00371068178122496,-0.0324156524631812,
0.0703374087372471));
#74085=CARTESIAN_POINT('Ctrl Pts',(0.00374144987509459,-0.032468026716731,
0.0703639900870716));
#74086=CARTESIAN_POINT('Ctrl Pts',(0.00377164489267473,-0.0325210109755913,
0.0703900763415096));
#74087=CARTESIAN_POINT('Origin',(0.0139469649693696,-0.0262834582512307,
0.0688590711408863));
#74088=CARTESIAN_POINT('Origin',(0.00345130090604331,-0.0342770954208307,
0.0629253641850408));
#74089=CARTESIAN_POINT('Ctrl Pts',(0.00369297710105128,-0.0326943950436604,
0.0704854061698654));
#74090=CARTESIAN_POINT('Ctrl Pts',(0.00364247212989119,-0.0325844576448134,
0.0705464709682477));
#74091=CARTESIAN_POINT('Ctrl Pts',(0.00359322650456347,-0.0324744968375322,
0.0706085846138884));
#74092=CARTESIAN_POINT('Ctrl Pts',(0.00354530222373777,-0.0323646534831894,
0.0706716666528736));
#74093=CARTESIAN_POINT('Ctrl Pts',(0.00357995917170039,-0.0326943950436604,
0.070493656941141));
#74094=CARTESIAN_POINT('Ctrl Pts',(0.00352956791163207,-0.0325844576448134,
0.070556279338408));
#74095=CARTESIAN_POINT('Ctrl Pts',(0.00348046821914228,-0.0324744968375322,
0.0706199483414351));
#74096=CARTESIAN_POINT('Ctrl Pts',(0.00343272187843611,-0.0323646534831894,
0.0706845815060732));
#74097=CARTESIAN_POINT('Ctrl Pts',(0.00346694124234949,-0.0326943950436604,
0.0705019077124166));
#74098=CARTESIAN_POINT('Ctrl Pts',(0.00341666369337294,-0.0325844576448134,
0.0705660877085682));
#74099=CARTESIAN_POINT('Ctrl Pts',(0.0033677099337211,-0.0324744968375322,
0.0706313120689818));
#74100=CARTESIAN_POINT('Ctrl Pts',(0.00332014153313445,-0.0323646534831894,
0.0706974963592727));
#74101=CARTESIAN_POINT('Ctrl Pts',(0.0033539233129986,-0.0326943950436604,
0.0705101584836922));
#74102=CARTESIAN_POINT('Ctrl Pts',(0.00330375947511382,-0.0325844576448134,
0.0705758960787284));
#74103=CARTESIAN_POINT('Ctrl Pts',(0.00325495164829991,-0.0324744968375322,
0.0706426757965286));
#74104=CARTESIAN_POINT('Ctrl Pts',(0.0032075611878328,-0.0323646534831894,
0.0707104112124722));
#74105=CARTESIAN_POINT('',(0.0033461594290625,-0.0326773559991151,0.0705203552922419));
#74106=CARTESIAN_POINT('',(0.00335392331299816,-0.0326943950436594,0.0705101584836928));
#74107=CARTESIAN_POINT('Origin',(0.0165987371531689,-0.0326395670956439,
0.0805254785140288));
#74108=CARTESIAN_POINT('Ctrl Pts',(0.00334615943172621,-0.0326773559987414,
0.0705203552942646));
#74109=CARTESIAN_POINT('Ctrl Pts',(0.00338036198050024,-0.0326267922586118,
0.070546339576884));
#74110=CARTESIAN_POINT('Ctrl Pts',(0.00341395831379564,-0.032575610957966,
0.0705718633068576));
#74111=CARTESIAN_POINT('Ctrl Pts',(0.00347996714161408,-0.0324719985462366,
0.0706220113835035));
#74112=CARTESIAN_POINT('Ctrl Pts',(0.00351235316176784,-0.032419609162177,
0.0706466156171281));
#74113=CARTESIAN_POINT('Ctrl Pts',(0.00354414528158299,-0.0323666188837756,
0.0706707686541372));
#74114=CARTESIAN_POINT('',(0.0035224390327981,-0.0326943950436703,0.0704978561466466));
#74115=CARTESIAN_POINT('Origin',(0.00812378219310841,-0.0315241814719618,
0.07415));
#74116=CARTESIAN_POINT('',(0.0033461594290972,-0.0327114338379875,0.0705203552922685));
#74117=CARTESIAN_POINT('',(0.00333841734075972,-0.0326943950436593,0.0705305686593156));
#74118=CARTESIAN_POINT('Origin',(0.0166255274977898,-0.0326395666325422,
0.0804889356024141));
#74119=CARTESIAN_POINT('Origin',(0.0165379545151668,-0.0326395680308184,
0.0806054893179686));
#74120=CARTESIAN_POINT('Origin',(0.0165099277966083,-0.0326395676864378,
0.0806410927357026));
#74121=CARTESIAN_POINT('Ctrl Pts',(0.00364339435499156,-0.0332451089994433,
0.070543859428689));
#74122=CARTESIAN_POINT('Ctrl Pts',(0.00350738653814015,-0.0329451141710254,
0.070712840020671));
#74123=CARTESIAN_POINT('Ctrl Pts',(0.00338449341412824,-0.0326442513127494,
0.0708915852213949));
#74124=CARTESIAN_POINT('Ctrl Pts',(0.00349091246699706,-0.0332451089994433,
0.0707419737235636));
#74125=CARTESIAN_POINT('Ctrl Pts',(0.00336237665302521,-0.0329451141710254,
0.0709167052640417));
#74126=CARTESIAN_POINT('Ctrl Pts',(0.00324736748967208,-0.0326442513127494,
0.0711006222536213));
#74127=CARTESIAN_POINT('Ctrl Pts',(0.00348938764811711,-0.0332451089994433,
0.0707439548665123));
#74128=CARTESIAN_POINT('Ctrl Pts',(0.00336092655417406,-0.0329451141710254,
0.0709187439164753));
#74129=CARTESIAN_POINT('Ctrl Pts',(0.00324599623042752,-0.0326442513127494,
0.0711027126239436));
#74130=CARTESIAN_POINT('',(0.00346960944486475,-0.0331951640388616,0.0707711242950492));
#74131=CARTESIAN_POINT('',(0.00333471939232407,-0.0328677532354985,0.0709651919115967));
#74132=CARTESIAN_POINT('Origin',(0.0174724975217998,-0.0326402808279898,
0.079988031204783));
#74133=CARTESIAN_POINT('Origin',(-0.0058716122919306,-0.0326944278779021,
0.0648432771865053));
#74134=CARTESIAN_POINT('',(0.00340506923980481,-0.0326943950436593,0.0708618587219638));
#74135=CARTESIAN_POINT('',(0.00337045993753886,-0.0326943950436694,0.0709139014562983));
#74136=CARTESIAN_POINT('',(0.00354414528154591,-0.0330220786163545,0.0706707686541055));
#74137=CARTESIAN_POINT('Origin',(0.0172329945527583,-0.0326396682765297,
0.0804049136502552));
#74138=CARTESIAN_POINT('',(0.0035452270429651,-0.0331951640388587,0.0706715904874359));
#74139=CARTESIAN_POINT('Origin',(-0.00523895195084356,-0.0331952026560205,
0.0639980929800267));
#74140=CARTESIAN_POINT('',(0.00350741824392492,-0.0331951640388701,0.0707213573912525));
#74141=CARTESIAN_POINT('Ctrl Pts',(0.0034921005710676,-0.0330240426238172,
0.0703358781676416));
#74142=CARTESIAN_POINT('Ctrl Pts',(0.00343955732690801,-0.032914277406352,
0.070399684094414));
#74143=CARTESIAN_POINT('Ctrl Pts',(0.0033883069347644,-0.0328043479726691,
0.070464608046397));
#74144=CARTESIAN_POINT('Ctrl Pts',(0.00333841734075968,-0.0326943950436593,
0.0705305686593156));
#74145=CARTESIAN_POINT('Ctrl Pts',(0.0035098405377922,-0.0330240426238172,
0.0704477997007132));
#74146=CARTESIAN_POINT('Ctrl Pts',(0.00345883912179054,-0.032914277406352,
0.0705113612421608));
#74147=CARTESIAN_POINT('Ctrl Pts',(0.0034091262743351,-0.0328043479726691,
0.0705760088130891));
#74148=CARTESIAN_POINT('Ctrl Pts',(0.00336076796208867,-0.0326943950436593,
0.0706416613490422));
#74149=CARTESIAN_POINT('Ctrl Pts',(0.0035275805045168,-0.0330240426238172,
0.0705597212337848));
#74150=CARTESIAN_POINT('Ctrl Pts',(0.00347812091667307,-0.032914277406352,
0.0706230383899076));
#74151=CARTESIAN_POINT('Ctrl Pts',(0.0034299456139058,-0.0328043479726691,
0.0706874095797811));
#74152=CARTESIAN_POINT('Ctrl Pts',(0.00338311858341766,-0.0326943950436593,
0.0707527540387689));
#74153=CARTESIAN_POINT('Ctrl Pts',(0.0035453204712414,-0.0330240426238172,
0.0706716427668565));
#74154=CARTESIAN_POINT('Ctrl Pts',(0.00349740271155559,-0.032914277406352,
0.0707347155376544));
#74155=CARTESIAN_POINT('Ctrl Pts',(0.0034507649534765,-0.0328043479726691,
0.0707988103464731));
#74156=CARTESIAN_POINT('Ctrl Pts',(0.00340546920474664,-0.0326943950436593,
0.0708638467284955));
#74157=CARTESIAN_POINT('',(0.00337174329029227,-0.0326943950436693,0.0706962136906497));
#74158=CARTESIAN_POINT('Ctrl Pts',(0.00334615943173144,-0.0327114338383327,
0.0705203552942685));
#74159=CARTESIAN_POINT('Ctrl Pts',(0.00338035629151675,-0.0327619876831051,
0.0705463352548623));
#74160=CARTESIAN_POINT('Ctrl Pts',(0.00341394984605243,-0.0328131562604493,
0.070571856873763));
#74161=CARTESIAN_POINT('Ctrl Pts',(0.00347995861321972,-0.0329167375858768,
0.0706220049043311));
#74162=CARTESIAN_POINT('Ctrl Pts',(0.00351234752457318,-0.0329691088920619,
0.0706466113344513));
#74163=CARTESIAN_POINT('Ctrl Pts',(0.00354414528158209,-0.0330220786163187,
0.0706707686541364));
#74164=CARTESIAN_POINT('Ctrl Pts',(0.00347161885306906,-0.0331951640388604,
0.0707708499185587));
#74165=CARTESIAN_POINT('Ctrl Pts',(0.00340175709164472,-0.0330306422010619,
0.0708670304129244));
#74166=CARTESIAN_POINT('Ctrl Pts',(0.00333593026758393,-0.0328657861914645,
0.0709660161817996));
#74167=CARTESIAN_POINT('Ctrl Pts',(0.00346960944486666,-0.0331951640388604,
0.0707711242950467));
#74168=CARTESIAN_POINT('Ctrl Pts',(0.00339975335600029,-0.0330306422010619,
0.0708673463326386));
#74169=CARTESIAN_POINT('Ctrl Pts',(0.00333393391667554,-0.0328657861914645,
0.0709663733747889));
#74170=CARTESIAN_POINT('Ctrl Pts',(0.00313478800011482,-0.0331951640388604,
0.0708168427966452));
#74171=CARTESIAN_POINT('Ctrl Pts',(0.00306587711195702,-0.0330306422010619,
0.0709199870529398));
#74172=CARTESIAN_POINT('Ctrl Pts',(0.00300128816825202,-0.0328657861914645,
0.0710258913326662));
#74173=CARTESIAN_POINT('',(0.00312767969860762,-0.0331781648281888,0.0708275069811679));
#74174=CARTESIAN_POINT('',(0.00313478800011414,-0.0331951640388588,0.0708168427966462));
#74175=CARTESIAN_POINT('Origin',(0.0172671593927324,-0.0326412091979399,
0.0793751147514508));
#74176=CARTESIAN_POINT('Ctrl Pts',(0.00312767970031722,-0.033178164828644,
0.0708275069804985));
#74177=CARTESIAN_POINT('Ctrl Pts',(0.00316347095534084,-0.0331276811546778,
0.0708513087584733));
#74178=CARTESIAN_POINT('Ctrl Pts',(0.00319861594986478,-0.0330765663497786,
0.0708746807218895));
#74179=CARTESIAN_POINT('Ctrl Pts',(0.00326764352385894,-0.0329730614462931,
0.0709205852352549));
#74180=CARTESIAN_POINT('Ctrl Pts',(0.00330149821473158,-0.0329207133373202,
0.0709430992452487));
#74181=CARTESIAN_POINT('Ctrl Pts',(0.00333471939280908,-0.0328677532289346,
0.0709651918951324));
#74182=CARTESIAN_POINT('',(0.00330219872249944,-0.0331951640388701,0.0707939835458577));
#74183=CARTESIAN_POINT('Origin',(0.00812378219310841,-0.0315241814719618,
0.07415));
#74184=CARTESIAN_POINT('',(0.00312767969954,-0.0332121607144422,0.0708275069825649));
#74185=CARTESIAN_POINT('',(0.00312059419090093,-0.0331951640388587,0.0708381863255022));
#74186=CARTESIAN_POINT('Origin',(0.0172853622406674,-0.0326413648569167,
0.0793335826227612));
#74187=CARTESIAN_POINT('Origin',(0.0164783289049674,-0.0326412101666988,
0.0805613003101866));
#74188=CARTESIAN_POINT('Origin',(0.0164470635230991,-0.0326413658922313,
0.0805941455259154));
#74189=CARTESIAN_POINT('Ctrl Pts',(0.00342581595379246,-0.0337436976235975,
0.0708322841872385));
#74190=CARTESIAN_POINT('Ctrl Pts',(0.0033959759149589,-0.0336723290703325,
0.0708745384075912));
#74191=CARTESIAN_POINT('Ctrl Pts',(0.00336690072378216,-0.033601104548885,
0.0709173225204514));
#74192=CARTESIAN_POINT('Ctrl Pts',(0.00327406939782573,-0.0333736987606858,
0.0710539237177589));
#74193=CARTESIAN_POINT('Ctrl Pts',(0.00318923001488756,-0.0331450831799193,
0.071195627003844));
#74194=CARTESIAN_POINT('Ctrl Pts',(0.00328607390263732,-0.0337436976235975,
0.0710395814596252));
#74195=CARTESIAN_POINT('Ctrl Pts',(0.00325809832688837,-0.0336723290703325,
0.0710830925411644));
#74196=CARTESIAN_POINT('Ctrl Pts',(0.00323090990414125,-0.033601104548885,
0.0711270997760665));
#74197=CARTESIAN_POINT('Ctrl Pts',(0.00314410265603281,-0.0333736987606858,
0.0712676061597666));
#74198=CARTESIAN_POINT('Ctrl Pts',(0.00306550152585123,-0.0331450831799193,
0.0714128625004848));
#74199=CARTESIAN_POINT('Ctrl Pts',(0.00328467648212577,-0.0337436976235975,
0.0710416544323491));
#74200=CARTESIAN_POINT('Ctrl Pts',(0.00325671955100766,-0.0336723290703325,
0.0710851780825002));
#74201=CARTESIAN_POINT('Ctrl Pts',(0.00322954999594483,-0.033601104548885,
0.0711291975486227));
#74202=CARTESIAN_POINT('Ctrl Pts',(0.00314280298861488,-0.0333736987606858,
0.0712697429841868));
#74203=CARTESIAN_POINT('Ctrl Pts',(0.00306426424096087,-0.0331450831799193,
0.0714150348554512));
#74204=CARTESIAN_POINT('',(0.00326663203069243,-0.0336938721132548,0.0710700296592754));
#74205=CARTESIAN_POINT('',(0.00314419376792775,-0.0333679869945434,0.0712721841414624));
#74206=CARTESIAN_POINT('Ctrl Pts',(0.00326663203069023,-0.0336938721132646,
0.0710700296592773));
#74207=CARTESIAN_POINT('Ctrl Pts',(0.00325460946161088,-0.0336629187933929,
0.0710889893948913));
#74208=CARTESIAN_POINT('Ctrl Pts',(0.00324270175451054,-0.0336319952301037,
0.0711080134637059));
#74209=CARTESIAN_POINT('Ctrl Pts',(0.00323090990413955,-0.0336011045488947,
0.0711270997760688));
#74210=CARTESIAN_POINT('Ctrl Pts',(0.0032013201166146,-0.0335235892595451,
0.071174993864756));
#74211=CARTESIAN_POINT('Ctrl Pts',(0.00317240740429413,-0.0334458668660366,
0.0712233650700992));
#74212=CARTESIAN_POINT('Ctrl Pts',(0.00314419376764526,-0.0333679869945382,
0.0712721841412908));
#74213=CARTESIAN_POINT('Ctrl Pts',(0.00314417092095408,-0.0333679692460735,
0.071272222300142));
#74214=CARTESIAN_POINT('Ctrl Pts',(0.00314456628424068,-0.033339189537642,
0.0712724439433076));
#74215=CARTESIAN_POINT('Ctrl Pts',(0.00314486421620311,-0.0333104081062908,
0.0712726072432279));
#74216=CARTESIAN_POINT('Ctrl Pts',(0.00314526124204551,-0.0332532698353254,
0.0712728185417925));
#74217=CARTESIAN_POINT('Ctrl Pts',(0.00314536323838122,-0.0332249171884949,
0.0712728682228483));
#74218=CARTESIAN_POINT('Ctrl Pts',(0.00314536986861459,-0.0331960985339516,
0.071272864085671));
#74219=CARTESIAN_POINT('Ctrl Pts',(0.00314536995033752,-0.0331956312585707,
0.0712728640037306));
#74220=CARTESIAN_POINT('Ctrl Pts',(0.00314537000600209,-0.0331951640388598,
0.0712728639074122));
#74221=CARTESIAN_POINT('',(0.00320791644279702,-0.0331951640388587,0.0711646375555192));
#74222=CARTESIAN_POINT('',(0.00317664322440935,-0.0331951640388689,0.071218750731476));
#74223=CARTESIAN_POINT('',(0.00333471940553021,-0.0335216366567748,0.0709651919034373));
#74224=CARTESIAN_POINT('Origin',(0.0178364699876207,-0.0326434571528789,
0.0791548130834105));
#74225=CARTESIAN_POINT('',(0.00333585063525283,-0.0336938721132327,0.070965944190613));
#74226=CARTESIAN_POINT('Origin',(-0.00575752938773102,-0.0336938867896278,
0.0649186911191892));
#74227=CARTESIAN_POINT('',(0.00330124133298263,-0.0336938721132538,0.0710179869249542));
#74228=CARTESIAN_POINT('Ctrl Pts',(0.00326174888219176,-0.0335235895815171,
0.070634230939956));
#74229=CARTESIAN_POINT('Ctrl Pts',(0.00321334739916796,-0.0334144449262748,
0.0707011664009435));
#74230=CARTESIAN_POINT('Ctrl Pts',(0.00316627314495361,-0.0333049234473147,
0.0707691787008793));
#74231=CARTESIAN_POINT('Ctrl Pts',(0.00312059419090086,-0.0331951640388587,
0.070838186325502));
#74232=CARTESIAN_POINT('Ctrl Pts',(0.00328648150721761,-0.0335235895815171,
0.070744817872933));
#74233=CARTESIAN_POINT('Ctrl Pts',(0.00323960247105187,-0.0334144449262748,
0.0708114128406429));
#74234=CARTESIAN_POINT('Ctrl Pts',(0.00319404537846771,-0.0333049234473147,
0.0708790528035093));
#74235=CARTESIAN_POINT('Ctrl Pts',(0.00314987631770572,-0.0331951640388587,
0.0709476565476434));
#74236=CARTESIAN_POINT('Ctrl Pts',(0.00331121413224346,-0.0335235895815172,
0.0708554048059099));
#74237=CARTESIAN_POINT('Ctrl Pts',(0.00326585754293578,-0.0334144449262748,
0.0709216592803423));
#74238=CARTESIAN_POINT('Ctrl Pts',(0.00322181761198181,-0.0333049234473147,
0.0709889269061394));
#74239=CARTESIAN_POINT('Ctrl Pts',(0.00317915844451057,-0.0331951640388587,
0.0710571267697849));
#74240=CARTESIAN_POINT('Ctrl Pts',(0.00333594675726931,-0.0335235895815172,
0.0709659917388869));
#74241=CARTESIAN_POINT('Ctrl Pts',(0.00329211261481969,-0.0334144449262748,
0.0710319057200417));
#74242=CARTESIAN_POINT('Ctrl Pts',(0.00324958984549591,-0.0333049234473147,
0.0710988010087694));
#74243=CARTESIAN_POINT('Ctrl Pts',(0.00320844057131542,-0.0331951640388587,
0.0711665969919264));
#74244=CARTESIAN_POINT('',(0.00316425531685898,-0.0331951640388687,0.0710014119405206));
#74245=CARTESIAN_POINT('Ctrl Pts',(0.00312767970214249,-0.0332121607145979,
0.0708275069842939));
#74246=CARTESIAN_POINT('Ctrl Pts',(0.00316341074044679,-0.0332625444109863,
0.0708512687316609));
#74247=CARTESIAN_POINT('Ctrl Pts',(0.00319852607688945,-0.0333135300747045,
0.0708746210268322));
#74248=CARTESIAN_POINT('Ctrl Pts',(0.00326755322012772,-0.0334167203140649,
0.0709205252495173));
#74249=CARTESIAN_POINT('Ctrl Pts',(0.00330143829216079,-0.0334688847587354,
0.0709430593979601));
#74250=CARTESIAN_POINT('Ctrl Pts',(0.00333471940602311,-0.033521636656244,
0.0709651919039611));
#74251=CARTESIAN_POINT('Ctrl Pts',(0.00326761224679909,-0.033693872113239,
0.0710698324506134));
#74252=CARTESIAN_POINT('Ctrl Pts',(0.00324958300402455,-0.0336474569764958,
0.0710982572247573));
#74253=CARTESIAN_POINT('Ctrl Pts',(0.00323188774449564,-0.033601104548885,
0.0711268911062677));
#74254=CARTESIAN_POINT('Ctrl Pts',(0.00318708741576369,-0.0334837508592656,
0.07119938551091));
#74255=CARTESIAN_POINT('Ctrl Pts',(0.00314445491954967,-0.0333660264659097,
0.0712731756079792));
#74256=CARTESIAN_POINT('Ctrl Pts',(0.00326663203070348,-0.033693872113239,
0.0710700296592581));
#74257=CARTESIAN_POINT('Ctrl Pts',(0.00324860394225659,-0.0336474569764958,
0.071098460170932));
#74258=CARTESIAN_POINT('Ctrl Pts',(0.00323090990414125,-0.033601104548885,
0.0711270997760665));
#74259=CARTESIAN_POINT('Ctrl Pts',(0.00318611266774766,-0.0334837508592656,
0.0711996086716091));
#74260=CARTESIAN_POINT('Ctrl Pts',(0.00314348369190948,-0.0333660264659097,
0.0712734131615827));
#74261=CARTESIAN_POINT('Ctrl Pts',(0.00293335422767099,-0.033693872113239,
0.0711370814696989));
#74262=CARTESIAN_POINT('Ctrl Pts',(0.00291571861572076,-0.0336474569764958,
0.0711674627669472));
#74263=CARTESIAN_POINT('Ctrl Pts',(0.00289843986361754,-0.033601104548885,
0.0711980484295541));
#74264=CARTESIAN_POINT('Ctrl Pts',(0.0028546940359264,-0.0334837508592655,
0.0712754842951902));
#74265=CARTESIAN_POINT('Ctrl Pts',(0.00281326200342863,-0.0333660264659097,
0.0713541824362755));
#74266=CARTESIAN_POINT('',(0.00292891730221443,-0.0336769361243753,0.0711477710338222));
#74267=CARTESIAN_POINT('',(0.00293534196805525,-0.0336938721132327,0.0711366815583065));
#74268=CARTESIAN_POINT('Ctrl Pts',(0.00292891730221426,-0.033676936124375,
0.0711477710338225));
#74269=CARTESIAN_POINT('Ctrl Pts',(0.0029299861859421,-0.0336797586669841,
0.0711459215058175));
#74270=CARTESIAN_POINT('Ctrl Pts',(0.00293105601697502,-0.0336825812712478,
0.0711440726185949));
#74271=CARTESIAN_POINT('Ctrl Pts',(0.0029331975748887,-0.033688226607443,
0.0711403761225528));
#74272=CARTESIAN_POINT('Ctrl Pts',(0.00293426930175874,-0.0336910493393091,
0.0711385285137804));
#74273=CARTESIAN_POINT('Ctrl Pts',(0.00293534196806087,-0.0336938721132307,
0.0711366815583066));
#74274=CARTESIAN_POINT('Ctrl Pts',(0.00292891730221448,-0.0336769361243754,
0.0711477710338222));
#74275=CARTESIAN_POINT('Ctrl Pts',(0.0029652049241925,-0.0336279031301482,
0.0711687424646687));
#74276=CARTESIAN_POINT('Ctrl Pts',(0.0030020146345147,-0.0335767851899347,
0.0711900156220816));
#74277=CARTESIAN_POINT('Ctrl Pts',(0.00307414236519179,-0.0334733198857316,
0.0712316998558108));
#74278=CARTESIAN_POINT('Ctrl Pts',(0.00310950881498663,-0.0334209645014074,
0.0712521389205869));
#74279=CARTESIAN_POINT('Ctrl Pts',(0.0031441937715641,-0.0333679869844682,
0.0712721841351429));
#74280=CARTESIAN_POINT('',(0.00310098699938384,-0.0336938721132538,0.071103355608801));
#74281=CARTESIAN_POINT('Origin',(0.00812378219310841,-0.0315241814719618,
0.07415));
#74282=CARTESIAN_POINT('',(0.00292891730334296,-0.0337108120655685,0.0711477710344767));
#74283=CARTESIAN_POINT('',(0.00292251633834766,-0.0336938721132327,0.0711588742072383));
#74284=CARTESIAN_POINT('Origin',(0.0165354160029626,-0.0345562514102215,
0.0803020907901988));
#74285=CARTESIAN_POINT('Ctrl Pts',(0.00292251633835219,-0.0336938721132294,
0.0711588742072459));
#74286=CARTESIAN_POINT('Ctrl Pts',(0.00292358110397635,-0.0336910493410251,
0.0711570226872939));
#74287=CARTESIAN_POINT('Ctrl Pts',(0.00292464690564218,-0.0336882266083007,
0.0711551716534623));
#74288=CARTESIAN_POINT('Ctrl Pts',(0.00292678056290971,-0.0336825812712639,
0.0711514705907239));
#74289=CARTESIAN_POINT('Ctrl Pts',(0.0029278484184837,-0.0336797586669922,
0.0711496205618321));
#74290=CARTESIAN_POINT('Ctrl Pts',(0.00292891730221458,-0.033676936124375,
0.0711477710338219));
#74291=CARTESIAN_POINT('Origin',(0.0176538489882102,-0.0345562515768689,
0.078366820253175));
#74292=CARTESIAN_POINT('Ctrl Pts',(0.00322679229796606,-0.0342436276873911,
0.0711337747154972));
#74293=CARTESIAN_POINT('Ctrl Pts',(0.00311303348602325,-0.0339430054201811,
0.0713184677340956));
#74294=CARTESIAN_POINT('Ctrl Pts',(0.00301350968585616,-0.0336441434784053,
0.0715112048390181));
#74295=CARTESIAN_POINT('Ctrl Pts',(0.00310034036297127,-0.0342436276873911,
0.0713494362747424));
#74296=CARTESIAN_POINT('Ctrl Pts',(0.00299471536082295,-0.0339430054201811,
0.0715388985066906));
#74297=CARTESIAN_POINT('Ctrl Pts',(0.00290366149984018,-0.0336441434784053,
0.0717357786042467));
#74298=CARTESIAN_POINT('Ctrl Pts',(0.00309907584362133,-0.0342436276873911,
0.0713515928903348));
#74299=CARTESIAN_POINT('Ctrl Pts',(0.00299353217957095,-0.0339430054201811,
0.0715411028144165));
#74300=CARTESIAN_POINT('Ctrl Pts',(0.00290256301798002,-0.0336441434784053,
0.071738024341899));
#74301=CARTESIAN_POINT('',(0.00308282356920625,-0.0341934961088741,0.0713810902593065));
#74302=CARTESIAN_POINT('',(0.0029733202979627,-0.0338664212863039,0.0715905337923547));
#74303=CARTESIAN_POINT('Origin',(0.0174984095754237,-0.0345610720405512,
0.0798807387145763));
#74304=CARTESIAN_POINT('Origin',(-0.00684720665499033,-0.0336938005073043,
0.0667103724431221));
#74305=CARTESIAN_POINT('',(0.00303016432206031,-0.0336938721132327,0.0714791982507606));
#74306=CARTESIAN_POINT('',(0.00300235060865654,-0.0336938721132428,0.0715351683083563));
#74307=CARTESIAN_POINT('',(0.00314419377156682,-0.0340203938281605,0.0712721841351383));
#74308=CARTESIAN_POINT('Origin',(0.0171930368507349,-0.0345589643244692,
0.0802526045951889));
#74309=CARTESIAN_POINT('',(0.00314537000600162,-0.034193496108874,0.0712728639074129));
#74310=CARTESIAN_POINT('Origin',(-0.0063953862268463,-0.0341934220717719,
0.0657590459209844));
#74311=CARTESIAN_POINT('',(0.00311409678761393,-0.0341934961088841,0.0713269770833697));
#74312=CARTESIAN_POINT('Ctrl Pts',(0.00305058748941132,-0.0340223579322397,
0.0709464557910948));
#74313=CARTESIAN_POINT('Ctrl Pts',(0.00300640225957646,-0.0339125849573575,
0.071016428377506));
#74314=CARTESIAN_POINT('Ctrl Pts',(0.00296369634813591,-0.0338030433565231,
0.0710872663265762));
#74315=CARTESIAN_POINT('Ctrl Pts',(0.00292251633834744,-0.0336938721132327,
0.0711588742072376));
#74316=CARTESIAN_POINT('Ctrl Pts',(0.00308221508064672,-0.0340223579322397,
0.0710552715771874));
#74317=CARTESIAN_POINT('Ctrl Pts',(0.00303953070430557,-0.0339125849573575,
0.0711248079366273));
#74318=CARTESIAN_POINT('Ctrl Pts',(0.00299831556284169,-0.0338030433565231,
0.071195178901078));
#74319=CARTESIAN_POINT('Ctrl Pts',(0.00295861438600814,-0.0336938721132327,
0.0712662898056645));
#74320=CARTESIAN_POINT('Ctrl Pts',(0.00311384267188213,-0.0340223579322397,
0.0711640873632801));
#74321=CARTESIAN_POINT('Ctrl Pts',(0.00307265914903468,-0.0339125849573575,
0.0712331874957486));
#74322=CARTESIAN_POINT('Ctrl Pts',(0.00303293477754747,-0.0338030433565231,
0.0713030914755798));
#74323=CARTESIAN_POINT('Ctrl Pts',(0.00299471243366884,-0.0336938721132327,
0.0713737054040914));
#74324=CARTESIAN_POINT('Ctrl Pts',(0.00314547026311753,-0.0340223579322397,
0.0712729031493728));
#74325=CARTESIAN_POINT('Ctrl Pts',(0.00310578759376378,-0.0339125849573575,
0.0713415670548699));
#74326=CARTESIAN_POINT('Ctrl Pts',(0.00306755399225326,-0.0338030433565231,
0.0714110040500815));
#74327=CARTESIAN_POINT('Ctrl Pts',(0.00303081048132955,-0.0336938721132327,
0.0714811210025183));
#74328=CARTESIAN_POINT('',(0.00297634033021399,-0.0336938721132427,0.0713190362290094));
#74329=CARTESIAN_POINT('Ctrl Pts',(0.00292891730645694,-0.0337108120662688,
0.071147771036274));
#74330=CARTESIAN_POINT('Ctrl Pts',(0.00296614652749129,-0.033761140899437,
0.0711692866383397));
#74331=CARTESIAN_POINT('Ctrl Pts',(0.00300269639783767,-0.0338121088781463,
0.0711904096284017));
#74332=CARTESIAN_POINT('Ctrl Pts',(0.00307447073348461,-0.0339153382773235,
0.0712318896272146));
#74333=CARTESIAN_POINT('Ctrl Pts',(0.00310966483386169,-0.0339675558473108,
0.0712522290873949));
#74334=CARTESIAN_POINT('Ctrl Pts',(0.00314419377159869,-0.0340203938281304,
0.0712721841351628));
#74335=CARTESIAN_POINT('Ctrl Pts',(0.00308478283418244,-0.0341934961088741,
0.0713805661766441));
#74336=CARTESIAN_POINT('Ctrl Pts',(0.00302752697167734,-0.0340287516182428,
0.0714847435186065));
#74337=CARTESIAN_POINT('Ctrl Pts',(0.00297462576178992,-0.0338644633275951,
0.0715911982712576));
#74338=CARTESIAN_POINT('Ctrl Pts',(0.00308282356920633,-0.0341934961088741,
0.0713810902593065));
#74339=CARTESIAN_POINT('Ctrl Pts',(0.0030255785416974,-0.0340287516182428,
0.0714853081075287));
#74340=CARTESIAN_POINT('Ctrl Pts',(0.00297268983170229,-0.0338644633275951,
0.0715918028840092));
#74341=CARTESIAN_POINT('Ctrl Pts',(0.00275637233919177,-0.0341934961088741,
0.071468412511202));
#74342=CARTESIAN_POINT('Ctrl Pts',(0.00270093263044727,-0.0340287516182428,
0.0715793794814226));
#74343=CARTESIAN_POINT('Ctrl Pts',(0.00265012664293871,-0.0338644633275951,
0.0716925429977116));
#74344=CARTESIAN_POINT('',(0.0027506566659699,-0.034176475883238,0.0714798835118756));
#74345=CARTESIAN_POINT('',(0.00275637233919176,-0.034193496108874,0.0714684125112019));
#74346=CARTESIAN_POINT('Origin',(0.0173505741629366,-0.034562102665955,
0.0793069990404853));
#74347=CARTESIAN_POINT('Ctrl Pts',(0.00275065666745294,-0.0341764758837462,
0.071479883510822));
#74348=CARTESIAN_POINT('Ctrl Pts',(0.00278909635182647,-0.0341260050040262,
0.0714989856799601));
#74349=CARTESIAN_POINT('Ctrl Pts',(0.00282686788080487,-0.0340749269147838,
0.0715177557741188));
#74350=CARTESIAN_POINT('Ctrl Pts',(0.00290110381968543,-0.0339715436305319,
0.0715546465237605));
#74351=CARTESIAN_POINT('Ctrl Pts',(0.0029375400635527,-0.0339192778234585,
0.0715727531891187));
#74352=CARTESIAN_POINT('Ctrl Pts',(0.00297332029732877,-0.0338664212853344,
0.0715905337907483));
#74353=CARTESIAN_POINT('',(0.00291959795420901,-0.0341934961088841,0.0714247513852643));
#74354=CARTESIAN_POINT('Origin',(0.00812378219310841,-0.0315241814719618,
0.07415));
#74355=CARTESIAN_POINT('',(0.00275065666625436,-0.0342105180190544,0.071479883512957));
#74356=CARTESIAN_POINT('',(0.00274496550589082,-0.0341934961088739,0.0714913666959631));
#74357=CARTESIAN_POINT('Origin',(0.0173752979548923,-0.0345621706502888,
0.0792690082965156));
#74358=CARTESIAN_POINT('Origin',(0.0178063648150556,-0.0345621037473414,
0.0783898080859335));
#74359=CARTESIAN_POINT('Origin',(0.0177910107596772,-0.0345621716267852,
0.0784324551737312));
#74360=CARTESIAN_POINT('Ctrl Pts',(0.0030308318555927,-0.0346945769586965,
0.0714778549605037));
#74361=CARTESIAN_POINT('Ctrl Pts',(0.00297486270787194,-0.0345275153362944,
0.071584528844429));
#74362=CARTESIAN_POINT('Ctrl Pts',(0.0029222338791257,-0.0343603235965185,
0.0716929904978644));
#74363=CARTESIAN_POINT('Ctrl Pts',(0.00287309625441993,-0.034193496108874,
0.0718029168259806));
#74364=CARTESIAN_POINT('Ctrl Pts',(0.00299352439310611,-0.0346945769586965,
0.0715529294675527));
#74365=CARTESIAN_POINT('Ctrl Pts',(0.00293912771099369,-0.0345275153362944,
0.0716603847712169));
#74366=CARTESIAN_POINT('Ctrl Pts',(0.00288809632950747,-0.0343603235965185,
0.0717695785939104));
#74367=CARTESIAN_POINT('Ctrl Pts',(0.00284057637698957,-0.034193496108874,
0.071880185745591));
#74368=CARTESIAN_POINT('Ctrl Pts',(0.00295621693061952,-0.0346945769586965,
0.0716280039746005));
#74369=CARTESIAN_POINT('Ctrl Pts',(0.00290339271411542,-0.0345275153362944,
0.0717362406980053));
#74370=CARTESIAN_POINT('Ctrl Pts',(0.0028539587798892,-0.0343603235965185,
0.0718461666899566));
#74371=CARTESIAN_POINT('Ctrl Pts',(0.00280805649955915,-0.034193496108874,
0.0719574546651999));
#74372=CARTESIAN_POINT('Ctrl Pts',(0.00291890946813294,-0.0346945769586965,
0.0717030784816508));
#74373=CARTESIAN_POINT('Ctrl Pts',(0.00286765771723718,-0.0345275153362944,
0.0718120966247927));
#74374=CARTESIAN_POINT('Ctrl Pts',(0.00281982123027101,-0.0343603235965185,
0.0719227547860021));
#74375=CARTESIAN_POINT('Ctrl Pts',(0.00277553662212886,-0.034193496108874,
0.0720347235848117));
#74376=CARTESIAN_POINT('',(0.0029189094684027,-0.0346945769586966,0.0717030784811083));
#74377=CARTESIAN_POINT('',(0.00282277334555112,-0.0343667727831433,0.0719189844916737));
#74378=CARTESIAN_POINT('Origin',(0.0182118505758894,-0.034562645706894,
0.078690438462228));
#74379=CARTESIAN_POINT('Origin',(-0.0073639863885442,-0.0341934771029151,
0.0676317265628182));
#74380=CARTESIAN_POINT('',(0.00287251438400795,-0.034193496108874,0.071804299380333));
#74381=CARTESIAN_POINT('',(0.00284826994360806,-0.0341934961088841,0.0718619054313204));
#74382=CARTESIAN_POINT('',(0.00297332029858978,-0.034521194296272,0.0715905337914187));
#74383=CARTESIAN_POINT('Origin',(0.0179949030575089,-0.0345625596118343,
0.0791195358443171));
#74384=CARTESIAN_POINT('',(0.00297453689523274,-0.0346945769586886,0.0715911383659319));
#74385=CARTESIAN_POINT('Origin',(-0.00693311847756907,-0.0346945685853897,
0.0666676355251271));
#74386=CARTESIAN_POINT('',(0.00294672318182772,-0.0346945769587026,0.0716471084235301));
#74387=CARTESIAN_POINT('Ctrl Pts',(0.00285944561345406,-0.0345231616327842,
0.0712713266291331));
#74388=CARTESIAN_POINT('Ctrl Pts',(0.00281976715388458,-0.0344132092796988,
0.0713438880972906));
#74389=CARTESIAN_POINT('Ctrl Pts',(0.00278159161827437,-0.0343032738558979,
0.0714172665392481));
#74390=CARTESIAN_POINT('Ctrl Pts',(0.00274496550589077,-0.0341934961088739,
0.0714913666959631));
#74391=CARTESIAN_POINT('Ctrl Pts',(0.00289784334637777,-0.0345231616327842,
0.0713779415917079));
#74392=CARTESIAN_POINT('Ctrl Pts',(0.00285963442396553,-0.0344132092796988,
0.0714499738011767));
#74393=CARTESIAN_POINT('Ctrl Pts',(0.00282291740239268,-0.0343032738558979,
0.0715227926155359));
#74394=CARTESIAN_POINT('Ctrl Pts',(0.00278773693076643,-0.0341934961088739,
0.0715963035405536));
#74395=CARTESIAN_POINT('Ctrl Pts',(0.00293624107930148,-0.0345231616327842,
0.0714845565542826));
#74396=CARTESIAN_POINT('Ctrl Pts',(0.00289950169404647,-0.0344132092796988,
0.0715560595050627));
#74397=CARTESIAN_POINT('Ctrl Pts',(0.002864243186511,-0.0343032738558979,
0.0716283186918237));
#74398=CARTESIAN_POINT('Ctrl Pts',(0.00283050835564208,-0.0341934961088739,
0.071701240385144));
#74399=CARTESIAN_POINT('Ctrl Pts',(0.00297463881222519,-0.0345231616327842,
0.0715911715168574));
#74400=CARTESIAN_POINT('Ctrl Pts',(0.00293936896412741,-0.0344132092796988,
0.0716621452089488));
#74401=CARTESIAN_POINT('Ctrl Pts',(0.00290556897062931,-0.0343032738558979,
0.0717338447681115));
#74402=CARTESIAN_POINT('Ctrl Pts',(0.00287327978051774,-0.0341934961088739,
0.0718061772297345));
#74403=CARTESIAN_POINT('',(0.00280873994495938,-0.0341934961088839,0.0716478330381581));
#74404=CARTESIAN_POINT('Ctrl Pts',(0.00275065666934253,-0.0342105180195392,
0.0714798835144891));
#74405=CARTESIAN_POINT('Ctrl Pts',(0.00278913956126267,-0.034261055624132,
0.0714990071704826));
#74406=CARTESIAN_POINT('Ctrl Pts',(0.00282693189758478,-0.0343122189870191,
0.0715177876623571));
#74407=CARTESIAN_POINT('Ctrl Pts',(0.00290116858704878,-0.0344158119695203,
0.0715546787804765));
#74408=CARTESIAN_POINT('Ctrl Pts',(0.00293758257684465,-0.0344681990450117,
0.0715727743179857));
#74409=CARTESIAN_POINT('Ctrl Pts',(0.0029733202986113,-0.0345211942962542,
0.0715905337914284));
#74410=CARTESIAN_POINT('Ctrl Pts',(0.00292083148908078,-0.0346945769586932,
0.0717024325675185));
#74411=CARTESIAN_POINT('Ctrl Pts',(0.00287022976425739,-0.034529677707698,
0.0718099998918345));
#74412=CARTESIAN_POINT('Ctrl Pts',(0.00282411713433537,-0.034364806625142,
0.0719195667170019));
#74413=CARTESIAN_POINT('Ctrl Pts',(0.00291890946840661,-0.0346945769586932,
0.0717030784811002));
#74414=CARTESIAN_POINT('Ctrl Pts',(0.00286832109738949,-0.034529677707698,
0.0718106855418335));
#74415=CARTESIAN_POINT('Ctrl Pts',(0.00282222345220572,-0.034364806625142,
0.0719202915175391));
#74416=CARTESIAN_POINT('Ctrl Pts',(0.00259858542488672,-0.0346945769586932,
0.0718107264648117));
#74417=CARTESIAN_POINT('Ctrl Pts',(0.00255022259976356,-0.034529677707698,
0.0719249559984909));
#74418=CARTESIAN_POINT('Ctrl Pts',(0.00250662231166498,-0.034364806625142,
0.0720410868044649));
#74419=CARTESIAN_POINT('',(0.00259360130007642,-0.0346775396664965,0.071822533720185));
#74420=CARTESIAN_POINT('',(0.00259858542488539,-0.0346945769586885,0.0718107264648148));
#74421=CARTESIAN_POINT('Origin',(0.0179538301029704,-0.0345626618414984,
0.0781214438937064));
#74422=CARTESIAN_POINT('Ctrl Pts',(0.00259360130155185,-0.0346775396670097,
0.07182253371912));
#74423=CARTESIAN_POINT('Ctrl Pts',(0.00263319572832671,-0.0346269749928193,
0.0718391976615173));
#74424=CARTESIAN_POINT('Ctrl Pts',(0.00267208648772173,-0.0345757902890796,
0.0718555654153675));
#74425=CARTESIAN_POINT('Ctrl Pts',(0.00274849263373398,-0.0344721681087812,
0.0718877221846446));
#74426=CARTESIAN_POINT('Ctrl Pts',(0.00278597806337797,-0.0344197714289114,
0.071903498598308));
#74427=CARTESIAN_POINT('Ctrl Pts',(0.0028227733455425,-0.0343667727830586,
0.0719189844914046));
#74428=CARTESIAN_POINT('',(0.00275874744665404,-0.0346945769587026,0.0717569024729716));
#74429=CARTESIAN_POINT('Origin',(0.00812378219310841,-0.0315241814719618,
0.07415));
#74430=CARTESIAN_POINT('',(0.00259360130087575,-0.03471161364898,0.0718225337213232));
#74431=CARTESIAN_POINT('',(0.00258864240555078,-0.0346945769586885,0.0718343515957248));
#74432=CARTESIAN_POINT('Origin',(0.0179696711837717,-0.0345626685633996,
0.0780789899898139));
#74433=CARTESIAN_POINT('Origin',(0.0178353519249934,-0.0345626628434408,
0.0784029612363081));
#74434=CARTESIAN_POINT('Origin',(0.0178160631121034,-0.0345626694948275,
0.0784439642081316));
#74435=CARTESIAN_POINT('Ctrl Pts',(0.00288833485497925,-0.0352450361874068,
0.0717690645125704));
#74436=CARTESIAN_POINT('Ctrl Pts',(0.00279853639954668,-0.0349452760959493,
0.0719665226490653));
#74437=CARTESIAN_POINT('Ctrl Pts',(0.00272386640684683,-0.0346444289841741,
0.0721701838148685));
#74438=CARTESIAN_POINT('Ctrl Pts',(0.00288734079150217,-0.0352450361874068,
0.0717713856034353));
#74439=CARTESIAN_POINT('Ctrl Pts',(0.00279762987744806,-0.0349452760959493,
0.0719688812316495));
#74440=CARTESIAN_POINT('Ctrl Pts',(0.00272305000146052,-0.0346444289841741,
0.0721725731886873));
#74441=CARTESIAN_POINT('Ctrl Pts',(0.00278891866505875,-0.0352450361874068,
0.072001196580167));
#74442=CARTESIAN_POINT('Ctrl Pts',(0.00270787521421854,-0.0349452760959493,
0.0722024042597919));
#74443=CARTESIAN_POINT('Ctrl Pts',(0.00264221778499502,-0.0346444289841741,
0.0724091448538994));
#74444=CARTESIAN_POINT('Ctrl Pts',(0.00278793444379431,-0.0352450361874068,
0.0720034946899342));
#74445=CARTESIAN_POINT('Ctrl Pts',(0.00270697766758624,-0.0349452760959493,
0.0722047394900734));
#74446=CARTESIAN_POINT('Ctrl Pts',(0.00264140946283037,-0.0346444289841741,
0.0724115105705516));
#74447=CARTESIAN_POINT('',(0.00277554631635331,-0.0351951634053266,0.072034692620652));
#74448=CARTESIAN_POINT('',(0.00269314705285671,-0.0348678972925388,0.072256239990531));
#74449=CARTESIAN_POINT('Origin',(0.0186471640029153,-0.0345636767884868,
0.0773728803636752));
#74450=CARTESIAN_POINT('Origin',(-0.00774050194262602,-0.0346946199341123,
0.0686178395383498));
#74451=CARTESIAN_POINT('',(0.00273558880738216,-0.0346945769330288,0.0721386579018089));
#74452=CARTESIAN_POINT('',(0.0027150093185055,-0.0346945769458129,0.0721976726095114));
#74453=CARTESIAN_POINT('',(0.00282277334566154,-0.0350221583435276,0.0719189844914724));
#74454=CARTESIAN_POINT('Origin',(0.018528619856001,-0.0345628458719578,
0.0778388102710214));
#74455=CARTESIAN_POINT('',(0.00282391455155809,-0.035195136029876,0.0719194615049381));
#74456=CARTESIAN_POINT('Origin',(-0.00733224189768627,-0.0351951838366883,
0.0676450808400573));
#74457=CARTESIAN_POINT('',(0.00277553662226091,-0.035195137132875,0.0720347235841983));
#74458=CARTESIAN_POINT('Ctrl Pts',(0.0026890797755654,-0.0350241211494343,
0.0716075583324728));
#74459=CARTESIAN_POINT('Ctrl Pts',(0.00265405868403688,-0.0349144232818962,
0.0716824191299597));
#74460=CARTESIAN_POINT('Ctrl Pts',(0.00262056405687373,-0.0348045283579412,
0.071758048646229));
#74461=CARTESIAN_POINT('Ctrl Pts',(0.00258864240126185,-0.0346945769439158,
0.0718343516059767));
#74462=CARTESIAN_POINT('Ctrl Pts',(0.0027340961748041,-0.0350241211494343,
0.0717115519169025));
#74463=CARTESIAN_POINT('Ctrl Pts',(0.00270050755226207,-0.0349144232818962,
0.0717857926319474));
#74464=CARTESIAN_POINT('Ctrl Pts',(0.00266843343393998,-0.0348045283579412,
0.0718607720844678));
#74465=CARTESIAN_POINT('Ctrl Pts',(0.0026379184765476,-0.0346945769439158,
0.0719363957641014));
#74466=CARTESIAN_POINT('Ctrl Pts',(0.0027791125740428,-0.0350241211494343,
0.0718155455013322));
#74467=CARTESIAN_POINT('Ctrl Pts',(0.00274695642048726,-0.0349144232818962,
0.071889166133935));
#74468=CARTESIAN_POINT('Ctrl Pts',(0.00271630281100623,-0.0348045283579412,
0.0719634955227065));
#74469=CARTESIAN_POINT('Ctrl Pts',(0.00268719455183335,-0.0346945769439158,
0.0720384399222262));
#74470=CARTESIAN_POINT('Ctrl Pts',(0.0028241289732815,-0.0350241211494343,
0.0719195390857619));
#74471=CARTESIAN_POINT('Ctrl Pts',(0.00279340528871245,-0.0349144232818962,
0.0719925396359226));
#74472=CARTESIAN_POINT('Ctrl Pts',(0.00276417218807248,-0.0348045283579412,
0.0720662189609453));
#74473=CARTESIAN_POINT('Ctrl Pts',(0.0027364706271191,-0.0346945769439158,
0.0721404840803509));
#74474=CARTESIAN_POINT('',(0.00266211560649583,-0.0346945769458128,0.0719865047484688));
#74475=CARTESIAN_POINT('Ctrl Pts',(0.00259360130390104,-0.0347116136492796,
0.0718225337225936));
#74476=CARTESIAN_POINT('Ctrl Pts',(0.00263318000186453,-0.034762154653231,
0.0718391910592448));
#74477=CARTESIAN_POINT('Ctrl Pts',(0.00267206279936505,-0.0348133084097055,
0.0718555555149049));
#74478=CARTESIAN_POINT('Ctrl Pts',(0.00274846904378221,-0.0349168561544571,
0.0718877123214953));
#74479=CARTESIAN_POINT('Ctrl Pts',(0.00278596218422295,-0.0349692089015917,
0.071903491917454));
#74480=CARTESIAN_POINT('Ctrl Pts',(0.00282277334568756,-0.0350221583435,
0.0719189844915049));
#74481=CARTESIAN_POINT('Ctrl Pts',(0.00277689142409584,-0.0351951371254876,
0.0720341713778109));
#74482=CARTESIAN_POINT('Ctrl Pts',(0.00273314799484822,-0.0350307338980915,
0.0721447149897066));
#74483=CARTESIAN_POINT('Ctrl Pts',(0.00269401083086319,-0.0348659306897811,
0.0722569721058663));
#74484=CARTESIAN_POINT('Ctrl Pts',(0.0027755366223692,-0.0351951371254876,
0.0720347235842403));
#74485=CARTESIAN_POINT('Ctrl Pts',(0.00273180460964304,-0.0350307338980915,
0.0721452952058117));
#74486=CARTESIAN_POINT('Ctrl Pts',(0.00269268001009425,-0.0348659306897811,
0.0722575798358558));
#74487=CARTESIAN_POINT('Ctrl Pts',(0.00254847044096598,-0.0351951371254876,
0.0721272739573489));
#74488=CARTESIAN_POINT('Ctrl Pts',(0.00250665184913576,-0.0350307338980915,
0.0722425400297545));
#74489=CARTESIAN_POINT('Ctrl Pts',(0.00246963306219441,-0.0348659306897811,
0.0723594360155021));
#74490=CARTESIAN_POINT('Origin',(-0.0023284672996302,-0.030860919741036,
0.070505112876027));
#74491=CARTESIAN_POINT('',(0.00267654088693848,-0.0351951371254876,0.0720750734601824));
#74492=CARTESIAN_POINT('Origin',(0.00908328496106734,-0.0351840467441164,
0.0743346620914201));
#74493=CARTESIAN_POINT('Origin',(-0.00341101805982505,-0.0352322613913528,
0.0709692410551445));
#74494=CARTESIAN_POINT('',(0.00261986248867378,-0.0351951142564652,0.0724812632111186));
#74495=CARTESIAN_POINT('',(0.00258626131451716,-0.0351951372916786,0.07260133524636));
#74496=CARTESIAN_POINT('Origin',(0.00821759083541753,-0.0352875121537596,
0.0744774156840959));
#74497=CARTESIAN_POINT('Origin',(0.0114906889709513,-0.029832507652212,
0.0674448431017022));
#74498=CARTESIAN_POINT('Origin',(0.00149551904094535,-0.0338734032822288,
0.0690206808999644));
#74499=CARTESIAN_POINT('Ctrl Pts',(0.00465214471498694,-0.0321934096636941,
0.069564602638177));
#74500=CARTESIAN_POINT('Ctrl Pts',(0.00457006828575119,-0.0320508460843319,
0.0696267432958608));
#74501=CARTESIAN_POINT('Ctrl Pts',(0.00448972333927352,-0.0319086045661065,
0.0696910423309887));
#74502=CARTESIAN_POINT('Ctrl Pts',(0.00441127147453155,-0.0317669892864902,
0.0697573470542575));
#74503=CARTESIAN_POINT('Ctrl Pts',(0.00458641150258548,-0.0321934096636941,
0.0696166562395441));
#74504=CARTESIAN_POINT('Ctrl Pts',(0.00450526680802655,-0.0320508460843319,
0.0696799734904281));
#74505=CARTESIAN_POINT('Ctrl Pts',(0.00442588450643241,-0.0319086045661065,
0.0697454231977286));
#74506=CARTESIAN_POINT('Ctrl Pts',(0.0043484239200655,-0.0317669892864902,
0.0698128503651842));
#74507=CARTESIAN_POINT('Ctrl Pts',(0.00452067829018401,-0.0321934096636941,
0.0696687098409112));
#74508=CARTESIAN_POINT('Ctrl Pts',(0.00444046533030192,-0.0320508460843319,
0.0697332036849953));
#74509=CARTESIAN_POINT('Ctrl Pts',(0.00436204567359129,-0.0319086045661065,
0.0697998040644686));
#74510=CARTESIAN_POINT('Ctrl Pts',(0.00428557636559944,-0.0317669892864902,
0.069868353676111));
#74511=CARTESIAN_POINT('Ctrl Pts',(0.00445494507778255,-0.0321934096636941,
0.0697207634422783));
#74512=CARTESIAN_POINT('Ctrl Pts',(0.00437566385257729,-0.0320508460843319,
0.0697864338795626));
#74513=CARTESIAN_POINT('Ctrl Pts',(0.00429820684075017,-0.0319086045661065,
0.0698541849312086));
#74514=CARTESIAN_POINT('Ctrl Pts',(0.00422272881113338,-0.0317669892864902,
0.0699238569870377));
#74515=CARTESIAN_POINT('',(0.00445612105794349,-0.0321934096636941,0.0697198321930652));
#74516=CARTESIAN_POINT('',(0.0042772061858937,-0.0318665617511257,0.0698742570224911));
#74517=CARTESIAN_POINT('Origin',(0.0146311327386297,-0.0326371944421084,
0.0829745310635062));
#74518=CARTESIAN_POINT('Origin',(-0.00305376322288012,-0.0316939261508759,
0.0617253627574423));
#74519=CARTESIAN_POINT('',(0.00455309446550072,-0.0320197221621846,0.0696413662470279));
#74520=CARTESIAN_POINT('Ctrl Pts',(0.00455292496321436,-0.0320197392094765,
0.0696414403000754));
#74521=CARTESIAN_POINT('Ctrl Pts',(0.00452998399114003,-0.0319792716576063,
0.069659610006459));
#74522=CARTESIAN_POINT('Ctrl Pts',(0.00450707710155583,-0.0319386439829706,
0.0696780373210006));
#74523=CARTESIAN_POINT('Ctrl Pts',(0.00448418554777068,-0.0318979099381638,
0.0696967481787971));
#74524=CARTESIAN_POINT('Ctrl Pts',(0.0044612944464526,-0.031857176698493,
0.0697154586667608));
#74525=CARTESIAN_POINT('Ctrl Pts',(0.00443853390029749,-0.0318163871833569,
0.0697343562083512));
#74526=CARTESIAN_POINT('Ctrl Pts',(0.00441597994691168,-0.0317755399638302,
0.0697533730947152));
#74527=CARTESIAN_POINT('',(0.00455411604157367,-0.0321934096636183,0.0696422307549535));
#74528=CARTESIAN_POINT('Origin',(0.0031040652733624,-0.0324113879591786,
0.0678450009147852));
#74529=CARTESIAN_POINT('',(0.00450511854976857,-0.0321934096636662,0.0696810314740193));
#74530=CARTESIAN_POINT('Ctrl Pts',(0.00445813573896037,-0.0321934096636618,
0.0697200661754986));
#74531=CARTESIAN_POINT('Ctrl Pts',(0.00439704349903201,-0.0320835708272592,
0.069770618296939));
#74532=CARTESIAN_POINT('Ctrl Pts',(0.00433703286861146,-0.0319739230346488,
0.0698224053968247));
#74533=CARTESIAN_POINT('Ctrl Pts',(0.00427817554202042,-0.0318646057455573,
0.0698753553245471));
#74534=CARTESIAN_POINT('Ctrl Pts',(0.00434557346451849,-0.0321934096636618,
0.0697069933358301));
#74535=CARTESIAN_POINT('Ctrl Pts',(0.00428430093994273,-0.0320835708272592,
0.069759097778761));
#74536=CARTESIAN_POINT('Ctrl Pts',(0.00422414225465977,-0.0319739230346488,
0.0698124400307091));
#74537=CARTESIAN_POINT('Ctrl Pts',(0.00416516913971261,-0.0318646057455573,
0.0698669459368185));
#74538=CARTESIAN_POINT('Ctrl Pts',(0.00423301119007662,-0.0321934096636618,
0.0696939204961617));
#74539=CARTESIAN_POINT('Ctrl Pts',(0.00417155838085345,-0.0320835708272592,
0.069747577260583));
#74540=CARTESIAN_POINT('Ctrl Pts',(0.00411125164070808,-0.0319739230346488,
0.0698024746645934));
#74541=CARTESIAN_POINT('Ctrl Pts',(0.0040521627374048,-0.0318646057455573,
0.0698585365490899));
#74542=CARTESIAN_POINT('Ctrl Pts',(0.00412044891563474,-0.0321934096636618,
0.0696808476564932));
#74543=CARTESIAN_POINT('Ctrl Pts',(0.00405881582176417,-0.0320835708272592,
0.0697360567424051));
#74544=CARTESIAN_POINT('Ctrl Pts',(0.00399836102675639,-0.0319739230346488,
0.0697925092984778));
#74545=CARTESIAN_POINT('Ctrl Pts',(0.00393915633509698,-0.0318646057455573,
0.0698501271613613));
#74546=CARTESIAN_POINT('',(0.00411091186015112,-0.032176398030845,0.0696894090449235));
#74547=CARTESIAN_POINT('',(0.00412044891561043,-0.0321934096636184,0.069680847656515));
#74548=CARTESIAN_POINT('Origin',(0.0147144957395131,-0.0326386230867408,
0.0823933495046793));
#74549=CARTESIAN_POINT('Ctrl Pts',(0.00411091186226809,-0.0321763980306273,
0.0696894090472774));
#74550=CARTESIAN_POINT('Ctrl Pts',(0.00413961652127484,-0.0321259596174931,
0.0697213163185597));
#74551=CARTESIAN_POINT('Ctrl Pts',(0.00416782383482309,-0.0320749164631609,
0.0697526707549605));
#74552=CARTESIAN_POINT('Ctrl Pts',(0.00422326647133633,-0.0319716057793885,
0.0698142991910765));
#74553=CARTESIAN_POINT('Ctrl Pts',(0.00425048019196887,-0.0319193786690077,
0.0698445491782618));
#74554=CARTESIAN_POINT('Ctrl Pts',(0.00427720618713083,-0.0318665617525256,
0.069874257023867));
#74555=CARTESIAN_POINT('',(0.00428828498678695,-0.0321934096636663,0.0697003399248001));
#74556=CARTESIAN_POINT('Origin',(0.00812378219310841,-0.0315241814719618,
0.07415));
#74557=CARTESIAN_POINT('',(0.00411091185990249,-0.0322104233323619,0.0696894090446472));
#74558=CARTESIAN_POINT('',(0.00410139311123134,-0.0321934096636183,0.0696979907823519));
#74559=CARTESIAN_POINT('Origin',(0.0147520956102168,-0.0326387231234825,
0.0823680219401029));
#74560=CARTESIAN_POINT('Origin',(0.0156266935458865,-0.0326386244938891,
0.0815727147650413));
#74561=CARTESIAN_POINT('Origin',(0.0155975407542225,-0.0326387243547428,
0.0816074322076005));
#74562=CARTESIAN_POINT('Ctrl Pts',(0.0043985075858247,-0.0327445246967097,
0.0697681677233916));
#74563=CARTESIAN_POINT('Ctrl Pts',(0.00423324407982012,-0.032443687833936,
0.0699086687520859));
#74564=CARTESIAN_POINT('Ctrl Pts',(0.00407903318169789,-0.0321434074405927,
0.0700612189549092));
#74565=CARTESIAN_POINT('Ctrl Pts',(0.00421160252194496,-0.0327445246967097,
0.0699341993381404));
#74566=CARTESIAN_POINT('Ctrl Pts',(0.00405260100066022,-0.032443687833936,
0.0700817496065585));
#74567=CARTESIAN_POINT('Ctrl Pts',(0.00390516527516717,-0.0321434074405927,
0.0702408573446777));
#74568=CARTESIAN_POINT('',(0.00418518581123572,-0.0326943950436612,0.0699588684653545));
#74569=CARTESIAN_POINT('',(0.00401632040136206,-0.0323666188837389,0.0701242227297893));
#74570=CARTESIAN_POINT('Origin',(0.0157527902649768,-0.0326395579109763,
0.0821571710290731));
#74571=CARTESIAN_POINT('Origin',(-0.00387143505510243,-0.0321933825603063,
0.0623933310808583));
#74572=CARTESIAN_POINT('',(0.00410478685933017,-0.0321934096532688,0.070035902103298));
#74573=CARTESIAN_POINT('',(0.00406103874479378,-0.0321934096584274,0.0700805378828959));
#74574=CARTESIAN_POINT('',(0.00427720618525688,-0.0325210109756239,0.0698742570217772));
#74575=CARTESIAN_POINT('Origin',(0.0153855203852089,-0.0326393129158089,
0.0824674890361115));
#74576=CARTESIAN_POINT('',(0.00427811478949626,-0.0326943950436593,0.0698752670000577));
#74577=CARTESIAN_POINT('Origin',(-0.00312058435812075,-0.0326943765538058,
0.0616510851198891));
#74578=CARTESIAN_POINT('',(0.00423165030037599,-0.0326943950436702,0.069917067732716));
#74579=CARTESIAN_POINT('Ctrl Pts',(0.00428883628827747,-0.0325229783203769,
0.0695355455461076));
#74580=CARTESIAN_POINT('Ctrl Pts',(0.00422522613454202,-0.032413025309245,
0.0695884101915409));
#74581=CARTESIAN_POINT('Ctrl Pts',(0.00416271920163296,-0.032303122220807,
0.069642582676758));
#74582=CARTESIAN_POINT('Ctrl Pts',(0.00410139310790405,-0.0321934096576658,
0.0696979907853581));
#74583=CARTESIAN_POINT('Ctrl Pts',(0.00428529000841981,-0.0325229783203769,
0.0696488088064151));
#74584=CARTESIAN_POINT('Ctrl Pts',(0.00422324118625079,-0.032413025309245,
0.0697017223372388));
#74585=CARTESIAN_POINT('Ctrl Pts',(0.00416229635935874,-0.032303122220807,
0.0697559114022826));
#74586=CARTESIAN_POINT('Ctrl Pts',(0.00410253114440126,-0.0321934096576658,
0.0698113038345151));
#74587=CARTESIAN_POINT('Ctrl Pts',(0.00428174372856215,-0.0325229783203769,
0.0697620720667227));
#74588=CARTESIAN_POINT('Ctrl Pts',(0.00422125623795956,-0.032413025309245,
0.0698150344829366));
#74589=CARTESIAN_POINT('Ctrl Pts',(0.00416187351708452,-0.032303122220807,
0.0698692401278072));
#74590=CARTESIAN_POINT('Ctrl Pts',(0.00410366918089846,-0.0321934096576658,
0.0699246168836721));
#74591=CARTESIAN_POINT('Ctrl Pts',(0.00427819744870449,-0.0325229783203769,
0.0698753353270303));
#74592=CARTESIAN_POINT('Ctrl Pts',(0.00421927128966834,-0.032413025309245,
0.0699283466286345));
#74593=CARTESIAN_POINT('Ctrl Pts',(0.0041614506748103,-0.032303122220807,
0.0699825688533318));
#74594=CARTESIAN_POINT('Ctrl Pts',(0.00410480721739566,-0.0321934096576658,
0.0700379299328292));
#74595=CARTESIAN_POINT('',(0.00410308998553813,-0.0321934096584275,0.0698669464423854));
#74596=CARTESIAN_POINT('Ctrl Pts',(0.00411091186222349,-0.0322104233328931,
0.0696894090472278));
#74597=CARTESIAN_POINT('Ctrl Pts',(0.00413965541650832,-0.0322609421831288,
0.0697213595533796));
#74598=CARTESIAN_POINT('Ctrl Pts',(0.00416788173104027,-0.0323120888240559,
0.0697527351107362));
#74599=CARTESIAN_POINT('Ctrl Pts',(0.00422332478732175,-0.0324156524631813,
0.0698143640134545));
#74600=CARTESIAN_POINT('Ctrl Pts',(0.00425051873905522,-0.032468026716731,
0.0698445920260914));
#74601=CARTESIAN_POINT('Ctrl Pts',(0.00427720618528259,-0.0325210109755912,
0.0698742570218124));
#74602=CARTESIAN_POINT('Origin',(0.0145641766563385,-0.0262834582512374,
0.0696306300222498));
#74603=CARTESIAN_POINT('Origin',(0.00489496422593971,-0.0342770941894682,
0.0624282604882694));
#74604=CARTESIAN_POINT('Ctrl Pts',(0.00418721071705005,-0.0326943950436604,
0.0699589754572965));
#74605=CARTESIAN_POINT('Ctrl Pts',(0.00412945054403444,-0.0325844576448134,
0.0700132287901579));
#74606=CARTESIAN_POINT('Ctrl Pts',(0.00407280833111478,-0.0324744968375322,
0.0700686805376889));
#74607=CARTESIAN_POINT('Ctrl Pts',(0.00401735567163183,-0.0323646534831895,
0.070125258650873));
#74608=CARTESIAN_POINT('Ctrl Pts',(0.00407404987198554,-0.0326943950436604,
0.0699529962662399));
#74609=CARTESIAN_POINT('Ctrl Pts',(0.00401620729451098,-0.0325844576448134,
0.0700088091676323));
#74610=CARTESIAN_POINT('Ctrl Pts',(0.00395951492573464,-0.0324744968375322,
0.0700658222983268));
#74611=CARTESIAN_POINT('Ctrl Pts',(0.00390404439566649,-0.0323646534831895,
0.0701239616078851));
#74612=CARTESIAN_POINT('Ctrl Pts',(0.00396088902692103,-0.0326943950436604,
0.0699470170751833));
#74613=CARTESIAN_POINT('Ctrl Pts',(0.00390296404498751,-0.0325844576448134,
0.0700043895451067));
#74614=CARTESIAN_POINT('Ctrl Pts',(0.00384622152035449,-0.0324744968375322,
0.0700629640589646));
#74615=CARTESIAN_POINT('Ctrl Pts',(0.00379073311970116,-0.0323646534831895,
0.0701226645648972));
#74616=CARTESIAN_POINT('Ctrl Pts',(0.00384772818185653,-0.0326943950436604,
0.0699410378841267));
#74617=CARTESIAN_POINT('Ctrl Pts',(0.00378972079546405,-0.0325844576448134,
0.0699999699225811));
#74618=CARTESIAN_POINT('Ctrl Pts',(0.00373292811497434,-0.0324744968375322,
0.0700601058196024));
#74619=CARTESIAN_POINT('Ctrl Pts',(0.00367742184373582,-0.0323646534831895,
0.0701213675219093));
#74620=CARTESIAN_POINT('',(0.00383874751947724,-0.0326773559991152,0.069950181215116));
#74621=CARTESIAN_POINT('',(0.003847728181856,-0.0326943950436594,0.0699410378841272));
#74622=CARTESIAN_POINT('Origin',(0.0157328504357829,-0.0326395670218336,
0.0815373995020848));
#74623=CARTESIAN_POINT('Ctrl Pts',(0.00383874752186574,-0.0326773559987415,
0.0699501812174572));
#74624=CARTESIAN_POINT('Ctrl Pts',(0.00386942367916692,-0.0326267922586078,
0.0699802473222834));
#74625=CARTESIAN_POINT('Ctrl Pts',(0.00389955612373196,-0.0325756109579571,
0.0700097805271131));
#74626=CARTESIAN_POINT('Ctrl Pts',(0.00395875923161915,-0.0324719985462364,
0.0700678062710256));
#74627=CARTESIAN_POINT('Ctrl Pts',(0.00398780615017079,-0.0324196091621775,
0.0700962755375468));
#74628=CARTESIAN_POINT('Ctrl Pts',(0.00401632040139686,-0.0323666188837757,
0.0701242227298235));
#74629=CARTESIAN_POINT('',(0.00401645699655587,-0.0326943950436702,0.0699499531747509));
#74630=CARTESIAN_POINT('Origin',(0.00812378219310841,-0.0315241814719618,
0.07415));
#74631=CARTESIAN_POINT('',(0.00383874751950847,-0.0327114338379877,0.0699501812151468));
#74632=CARTESIAN_POINT('',(0.00382978640553166,-0.0326943950436593,0.0699593437057789));
#74633=CARTESIAN_POINT('Origin',(0.0157640093170233,-0.0326395666891383,
0.0815045024555703));
#74634=CARTESIAN_POINT('Origin',(0.0156625188665274,-0.0326395680025381,
0.0816091612983061));
#74635=CARTESIAN_POINT('Origin',(0.0156302508924236,-0.0326395677096589,
0.081640971233586));
#74636=CARTESIAN_POINT('Ctrl Pts',(0.00413069280981186,-0.0332451089994432,
0.0700107534288225));
#74637=CARTESIAN_POINT('Ctrl Pts',(0.00397457857121719,-0.0329451141710253,
0.0701613552588885));
#74638=CARTESIAN_POINT('Ctrl Pts',(0.00383025178220369,-0.0326442513127493,
0.0703232884077009));
#74639=CARTESIAN_POINT('Ctrl Pts',(0.00395458298185639,-0.0332451089994432,
0.0701881944852257));
#74640=CARTESIAN_POINT('Ctrl Pts',(0.00380516104219571,-0.0329451141710253,
0.0703454384061234));
#74641=CARTESIAN_POINT('Ctrl Pts',(0.00366800784943576,-0.0326442513127493,
0.0705134906849743));
#74642=CARTESIAN_POINT('Ctrl Pts',(0.00395282188357683,-0.0332451089994432,
0.0701899688957897));
#74643=CARTESIAN_POINT('Ctrl Pts',(0.00380346686690549,-0.0329451141710253,
0.0703472792375957));
#74644=CARTESIAN_POINT('Ctrl Pts',(0.00366638541010808,-0.0326442513127493,
0.070515392707747));
#74645=CARTESIAN_POINT('',(0.00392979440503199,-0.0331951640388616,0.0702144452190998));
#74646=CARTESIAN_POINT('',(0.00377164487893352,-0.0328677532354985,0.0703900763480648));
#74647=CARTESIAN_POINT('Origin',(0.0166670807805257,-0.0326402808279353,
0.0811137013066832));
#74648=CARTESIAN_POINT('Origin',(-0.00459481279605483,-0.0326944278779134,
0.0631625754702518));
#74649=CARTESIAN_POINT('',(0.00385439107964536,-0.0326943950436593,0.070296375145362));
#74650=CARTESIAN_POINT('',(0.00381353199788872,-0.0326943950436693,0.0703436698114264));
#74651=CARTESIAN_POINT('',(0.00401632040136406,-0.0330220786163545,0.0701242227297873));
#74652=CARTESIAN_POINT('Origin',(0.0163772171391324,-0.0326396682765136,
0.0814972788281632));
#74653=CARTESIAN_POINT('',(0.00401729062974261,-0.0331951640388587,0.070125173663373));
#74654=CARTESIAN_POINT('Origin',(-0.0038612114645624,-0.0331952026559987,
0.0624033491204828));
#74655=CARTESIAN_POINT('',(0.00397354251739729,-0.0331951640388701,0.0701698094412464));
#74656=CARTESIAN_POINT('Ctrl Pts',(0.00400665898653133,-0.0330240426238172,
0.0697854500229821));
#74657=CARTESIAN_POINT('Ctrl Pts',(0.0039465330584229,-0.032914277406352,
0.0698421674062715));
#74658=CARTESIAN_POINT('Ctrl Pts',(0.0038875496620913,-0.0328043479726691,
0.0699001560361325));
#74659=CARTESIAN_POINT('Ctrl Pts',(0.00382978640553166,-0.0326943950436593,
0.0699593437057788));
#74660=CARTESIAN_POINT('Ctrl Pts',(0.00401023158067429,-0.0330240426238172,
0.069898712428729));
#74661=CARTESIAN_POINT('Ctrl Pts',(0.00395166595255125,-0.032914277406352,
0.0699553805960535));
#74662=CARTESIAN_POINT('Ctrl Pts',(0.00389424261664,-0.0328043479726691,
0.0700132877296544));
#74663=CARTESIAN_POINT('Ctrl Pts',(0.00383803717950686,-0.0326943950436593,
0.0700723616721085));
#74664=CARTESIAN_POINT('Ctrl Pts',(0.00401380417481726,-0.0330240426238172,
0.0700119748344759));
#74665=CARTESIAN_POINT('Ctrl Pts',(0.00395679884667959,-0.032914277406352,
0.0700685937858354));
#74666=CARTESIAN_POINT('Ctrl Pts',(0.00390093557118869,-0.0328043479726691,
0.0701264194231762));
#74667=CARTESIAN_POINT('Ctrl Pts',(0.00384628795348206,-0.0326943950436593,
0.0701853796384381));
#74668=CARTESIAN_POINT('Ctrl Pts',(0.00401737676896022,-0.0330240426238172,
0.0701252372402228));
#74669=CARTESIAN_POINT('Ctrl Pts',(0.00396193174080793,-0.032914277406352,
0.0701818069756174));
#74670=CARTESIAN_POINT('Ctrl Pts',(0.00390762852573739,-0.0328043479726691,
0.0702395511166981));
#74671=CARTESIAN_POINT('Ctrl Pts',(0.00385453872745727,-0.0326943950436593,
0.0702983976047677));
#74672=CARTESIAN_POINT('',(0.00384208874259851,-0.0326943950436694,0.0701278594255804));
#74673=CARTESIAN_POINT('Ctrl Pts',(0.00383874752187065,-0.0327114338383328,
0.0699501812174619));
#74674=CARTESIAN_POINT('Ctrl Pts',(0.00386941857673141,-0.032761987683102,
0.0699802423213192));
#74675=CARTESIAN_POINT('Ctrl Pts',(0.00389954852903165,-0.0328131562604436,
0.0700097730834474));
#74676=CARTESIAN_POINT('Ctrl Pts',(0.00395875158252924,-0.0329167375858768,
0.0700677987740519));
#74677=CARTESIAN_POINT('Ctrl Pts',(0.00398780109418897,-0.0329691088920616,
0.0700962705821124));
#74678=CARTESIAN_POINT('Ctrl Pts',(0.00401632040139609,-0.0330220786163187,
0.0701242227298225));
#74679=CARTESIAN_POINT('Ctrl Pts',(0.00393182235694514,-0.0331951640388604,
0.0702144248517776));
#74680=CARTESIAN_POINT('Ctrl Pts',(0.00385045686401168,-0.0330306422010619,
0.0703010909337557));
#74681=CARTESIAN_POINT('Ctrl Pts',(0.00377274289763015,-0.0328657861914645,
0.0703910458815629));
#74682=CARTESIAN_POINT('Ctrl Pts',(0.00392979440503419,-0.0331951640388604,
0.0702144452190975));
#74683=CARTESIAN_POINT('Ctrl Pts',(0.003848429333182,-0.0330306422010619,
0.0703011532276811));
#74684=CARTESIAN_POINT('Ctrl Pts',(0.00377071752039264,-0.0328657861914645,
0.0703911500488642));
#74685=CARTESIAN_POINT('Ctrl Pts',(0.00359188307974148,-0.0331951640388604,
0.070217838962318));
#74686=CARTESIAN_POINT('Ctrl Pts',(0.00351058817135452,-0.0330306422010619,
0.0703115330709035));
#74687=CARTESIAN_POINT('Ctrl Pts',(0.00343323520493602,-0.0328657861914645,
0.0704085071225851));
#74688=CARTESIAN_POINT('',(0.00358349425258602,-0.0331781648281888,0.0702275281501469));
#74689=CARTESIAN_POINT('',(0.00359188307974073,-0.0331951640388588,0.0702178389623189));
#74690=CARTESIAN_POINT('Origin',(0.0165401803771366,-0.0326412093141841,
0.0804798821977587));
#74691=CARTESIAN_POINT('Ctrl Pts',(0.00358349425436534,-0.033178164828644,
0.0702275281496977));
#74692=CARTESIAN_POINT('Ctrl Pts',(0.0036160201308545,-0.0331276811546779,
0.0702556280772692));
#74693=CARTESIAN_POINT('Ctrl Pts',(0.00364795871284956,-0.0330765663497788,
0.0702832205815802));
#74694=CARTESIAN_POINT('Ctrl Pts',(0.00371068862268351,-0.0329730614463369,
0.0703374145731777));
#74695=CARTESIAN_POINT('Ctrl Pts',(0.00374145460550374,-0.0329207133374194,
0.0703639941713307));
#74696=CARTESIAN_POINT('Ctrl Pts',(0.00377164488147798,-0.0328677532289346,
0.0703900763317915));
#74697=CARTESIAN_POINT('',(0.00376083874239636,-0.0331951640388701,0.0702161420907193));
#74698=CARTESIAN_POINT('Origin',(0.00812378219310841,-0.0315241814719618,
0.07415));
#74699=CARTESIAN_POINT('',(0.00358349425333596,-0.0332121607144232,0.0702275281516499));
#74700=CARTESIAN_POINT('',(0.00357512613946546,-0.0331951640388587,0.0702372352350697));
#74701=CARTESIAN_POINT('Origin',(0.0165634452037064,-0.0326413648504218,
0.08044095890546));
#74702=CARTESIAN_POINT('Origin',(0.0156089014564926,-0.0326412100340455,
0.0815578475744207));
#74703=CARTESIAN_POINT('Origin',(0.0155737662735942,-0.0326413659626031,
0.0815865150718522));
#74704=CARTESIAN_POINT('Ctrl Pts',(0.00387868087166481,-0.0337436976235975,
0.0702696340674263));
#74705=CARTESIAN_POINT('Ctrl Pts',(0.0038437802723817,-0.0336723290703325,
0.0703078151520742));
#74706=CARTESIAN_POINT('Ctrl Pts',(0.00380957207656177,-0.033601104548885,
0.0703466178116988));
#74707=CARTESIAN_POINT('Ctrl Pts',(0.00370035208357056,-0.0333736987606857,
0.0704705070175065));
#74708=CARTESIAN_POINT('Ctrl Pts',(0.00359842155345539,-0.0331450831799191,
0.0706004597366589));
#74709=CARTESIAN_POINT('Ctrl Pts',(0.00371405949086468,-0.0337436976235975,
0.0704577824157674));
#74710=CARTESIAN_POINT('Ctrl Pts',(0.00368085112634121,-0.0336723290703325,
0.0704974441300632));
#74711=CARTESIAN_POINT('Ctrl Pts',(0.00364836152337774,-0.033601104548885,
0.0705376967418353));
#74712=CARTESIAN_POINT('Ctrl Pts',(0.00354462865694311,-0.0333736987606857,
0.0706662153576305));
#74713=CARTESIAN_POINT('Ctrl Pts',(0.00344844187327208,-0.0331450831799191,
0.0708004749749087));
#74714=CARTESIAN_POINT('Ctrl Pts',(0.00371241327705668,-0.0337436976235975,
0.0704596638992509));
#74715=CARTESIAN_POINT('Ctrl Pts',(0.00367922183488081,-0.0336723290703325,
0.0704993404198431));
#74716=CARTESIAN_POINT('Ctrl Pts',(0.0036467494178459,-0.033601104548885,
0.0705396075311367));
#74717=CARTESIAN_POINT('Ctrl Pts',(0.00354307142267684,-0.0333736987606857,
0.0706681724410318));
#74718=CARTESIAN_POINT('Ctrl Pts',(0.00344694207647024,-0.0331450831799191,
0.0708024751272912));
#74719=CARTESIAN_POINT('',(0.00369095475256867,-0.0336938721132548,0.0704855538095916));
#74720=CARTESIAN_POINT('',(0.00354414527714575,-0.0333679869945434,0.0706707686599204));
#74721=CARTESIAN_POINT('Ctrl Pts',(0.0036909547525674,-0.0336938721132646,
0.0704855538095919));
#74722=CARTESIAN_POINT('Ctrl Pts',(0.00367665070006428,-0.0336629187933929,
0.070502857214569));
#74723=CARTESIAN_POINT('Ctrl Pts',(0.00366245254073096,-0.0336319952301037,
0.0705202388414836));
#74724=CARTESIAN_POINT('Ctrl Pts',(0.00364836152337687,-0.0336011045488947,
0.0705376967418361));
#74725=CARTESIAN_POINT('Ctrl Pts',(0.00361300233916066,-0.0335235892595451,
0.0705815045875778));
#74726=CARTESIAN_POINT('Ctrl Pts',(0.00357825509263566,-0.0334458668660366,
0.0706258706477928));
#74727=CARTESIAN_POINT('Ctrl Pts',(0.00354414527688669,-0.0333679869945382,
0.0706707686597147));
#74728=CARTESIAN_POINT('Ctrl Pts',(0.00354411782777536,-0.0333679692460734,
0.0706708036542234));
#74729=CARTESIAN_POINT('Ctrl Pts',(0.00354448229424894,-0.03333918953762,
0.0706710731018273));
#74730=CARTESIAN_POINT('Ctrl Pts',(0.00354475741002288,-0.0333104081062542,
0.0706712724548537));
#74731=CARTESIAN_POINT('Ctrl Pts',(0.0035451248223397,-0.0332532698548129,
0.0706715318477102));
#74732=CARTESIAN_POINT('Ctrl Pts',(0.00354521978741927,-0.0332249172858275,
0.0706715939211706));
#74733=CARTESIAN_POINT('Ctrl Pts',(0.0035452268843479,-0.0331960985300325,
0.0706715906470329));
#74734=CARTESIAN_POINT('Ctrl Pts',(0.00354522697566713,-0.0331956312625235,
0.0706715905760188));
#74735=CARTESIAN_POINT('Ctrl Pts',(0.00354522704296523,-0.033195164038859,
0.0706715904874357));
#74736=CARTESIAN_POINT('',(0.00362084464106437,-0.0331951640388587,0.0705720566798239));
#74737=CARTESIAN_POINT('',(0.00358303584202474,-0.0331951640388687,0.0706218235836399));
#74738=CARTESIAN_POINT('',(0.00377164489305891,-0.0335216366567749,0.0703900763416243));
#74739=CARTESIAN_POINT('Origin',(0.0171326131364008,-0.0326434571527407,
0.0803326712051912));
#74740=CARTESIAN_POINT('',(0.00377267291611205,-0.0336938721132326,0.0703909644774707));
#74741=CARTESIAN_POINT('Origin',(-0.00449108115158622,-0.033693886789624,
0.0632516928999231));
#74742=CARTESIAN_POINT('',(0.00373181383435036,-0.0336938721132537,0.0704382591435412));
#74743=CARTESIAN_POINT('Ctrl Pts',(0.00374073017182796,-0.0335235895815172,
0.0700525794725493));
#74744=CARTESIAN_POINT('Ctrl Pts',(0.00368432111118894,-0.0334144449262748,
0.0701129208130575));
#74745=CARTESIAN_POINT('Ctrl Pts',(0.00362909385005637,-0.0333049234473147,
0.0701744968471957));
#74746=CARTESIAN_POINT('Ctrl Pts',(0.00357512613946542,-0.0331951640388587,
0.0702372352350695));
#74747=CARTESIAN_POINT('Ctrl Pts',(0.00375140755481824,-0.0335235895815172,
0.070165394214398));
#74748=CARTESIAN_POINT('Ctrl Pts',(0.00369655161121256,-0.0334144449262748,
0.0702255885597076));
#74749=CARTESIAN_POINT('Ctrl Pts',(0.00364287621464645,-0.0333049234473147,
0.0702869853435383));
#74750=CARTESIAN_POINT('Ctrl Pts',(0.00359045711103427,-0.0331951640388587,
0.0703495122754503));
#74751=CARTESIAN_POINT('Ctrl Pts',(0.00376208493780853,-0.0335235895815172,
0.0702782089562468));
#74752=CARTESIAN_POINT('Ctrl Pts',(0.00370878211123618,-0.0334144449262748,
0.0703382563063576));
#74753=CARTESIAN_POINT('Ctrl Pts',(0.00365665857923653,-0.0333049234473147,
0.070399473839881));
#74754=CARTESIAN_POINT('Ctrl Pts',(0.00360578808260313,-0.0331951640388587,
0.0704617893158311));
#74755=CARTESIAN_POINT('Ctrl Pts',(0.00377276232079881,-0.0335235895815172,
0.0703910236980955));
#74756=CARTESIAN_POINT('Ctrl Pts',(0.0037210126112598,-0.0334144449262748,
0.0704509240530077));
#74757=CARTESIAN_POINT('Ctrl Pts',(0.00367044094382661,-0.0333049234473147,
0.0705119623362236));
#74758=CARTESIAN_POINT('Ctrl Pts',(0.00362111905417199,-0.0331951640388587,
0.0705740663562119));
#74759=CARTESIAN_POINT('',(0.00359798539027491,-0.0331951640388687,0.0704046459574569));
#74760=CARTESIAN_POINT('Ctrl Pts',(0.00358349425570064,-0.0332121607145981,
0.070227528153692));
#74761=CARTESIAN_POINT('Ctrl Pts',(0.00361596540746101,-0.0332625444109836,
0.0702555808191513));
#74762=CARTESIAN_POINT('Ctrl Pts',(0.00364787703032069,-0.0333135300746987,
0.0702831500931627));
#74763=CARTESIAN_POINT('Ctrl Pts',(0.00371060654925751,-0.0334167203140654,
0.0703373437424101));
#74764=CARTESIAN_POINT('Ctrl Pts',(0.0037414001496865,-0.0334688847587355,
0.0703639471280091));
#74765=CARTESIAN_POINT('Ctrl Pts',(0.00377164489348147,-0.0335216366562442,
0.0703900763422066));
#74766=CARTESIAN_POINT('Ctrl Pts',(0.00369195195617788,-0.033693872113239,
0.0704854810096331));
#74767=CARTESIAN_POINT('Ctrl Pts',(0.00367050231051092,-0.0336474569764958,
0.070511421982647));
#74768=CARTESIAN_POINT('Ctrl Pts',(0.0036493578064295,-0.033601104548885,
0.0705376122733537));
#74769=CARTESIAN_POINT('Ctrl Pts',(0.00359582478352168,-0.0334837508592656,
0.0706039200678976));
#74770=CARTESIAN_POINT('Ctrl Pts',(0.0035442801058033,-0.0333660264659097,
0.070671785039406));
#74771=CARTESIAN_POINT('Ctrl Pts',(0.00369095475258184,-0.0336938721132391,
0.0704855538095758));
#74772=CARTESIAN_POINT('Ctrl Pts',(0.0036695055330371,-0.0336474569764958,
0.0705115006195533));
#74773=CARTESIAN_POINT('Ctrl Pts',(0.00364836152337774,-0.033601104548885,
0.0705376967418353));
#74774=CARTESIAN_POINT('Ctrl Pts',(0.00359482975223288,-0.0334837508592656,
0.0706040193005872));
#74775=CARTESIAN_POINT('Ctrl Pts',(0.00354328676322187,-0.0333660264659097,
0.0706718989927277));
#74776=CARTESIAN_POINT('Ctrl Pts',(0.0033519011243526,-0.0336938721132391,
0.0705103061117345));
#74777=CARTESIAN_POINT('Ctrl Pts',(0.00333059678824609,-0.0336474569764958,
0.070538237515108));
#74778=CARTESIAN_POINT('Ctrl Pts',(0.00330962088426888,-0.033601104548885,
0.0705664163987568));
#74779=CARTESIAN_POINT('Ctrl Pts',(0.00325651471806131,-0.0334837508592656,
0.0706377588534238));
#74780=CARTESIAN_POINT('Ctrl Pts',(0.0032055458970172,-0.0333660264659097,
0.0707106436255546));
#74781=CARTESIAN_POINT('',(0.00334615942774154,-0.0336769361243753,0.0705203552912374));
#74782=CARTESIAN_POINT('',(0.00335392331299817,-0.0336938721132327,0.0705101584836928));
#74783=CARTESIAN_POINT('Ctrl Pts',(0.00334615942774136,-0.033676936124375,
0.0705203552912377));
#74784=CARTESIAN_POINT('Ctrl Pts',(0.0033474516903319,-0.0336797586669944,
0.0705186543139611));
#74785=CARTESIAN_POINT('Ctrl Pts',(0.00334874481244644,-0.0336825812712685,
0.070516954091143));
#74786=CARTESIAN_POINT('Ctrl Pts',(0.00335133277778879,-0.0336882266084466,
0.0705135551508626));
#74787=CARTESIAN_POINT('Ctrl Pts',(0.00335262762101661,-0.0336910493413165,
0.0705118564334281));
#74788=CARTESIAN_POINT('Ctrl Pts',(0.00335392331300474,-0.0336938721132303,
0.0705101584836938));
#74789=CARTESIAN_POINT('Ctrl Pts',(0.00334615942774159,-0.0336769361243753,
0.0705203552912374));
#74790=CARTESIAN_POINT('Ctrl Pts',(0.00337953499220296,-0.033627899459312,
0.0705457112992143));
#74791=CARTESIAN_POINT('Ctrl Pts',(0.00341338573099195,-0.0335767852487023,
0.0705714283055508));
#74792=CARTESIAN_POINT('Ctrl Pts',(0.00347972195807058,-0.0334733171799194,
0.0706218251132185));
#74793=CARTESIAN_POINT('Ctrl Pts',(0.00351224698220595,-0.0334209631321932,
0.0706465349506327));
#74794=CARTESIAN_POINT('Ctrl Pts',(0.00354414528154423,-0.033367986984468,
0.0706707686541077));
#74795=CARTESIAN_POINT('',(0.00352243903279342,-0.0336938721132538,0.0704978561466522));
#74796=CARTESIAN_POINT('Origin',(0.00812378219310841,-0.0315241814719618,
0.07415));
#74797=CARTESIAN_POINT('',(0.00334615942877989,-0.0337108120655687,0.0705203552920277));
#74798=CARTESIAN_POINT('',(0.0033384173407597,-0.0336938721132327,0.0705305686593155));
#74799=CARTESIAN_POINT('Origin',(0.0156980260465387,-0.0345562514985363,
0.0813078369163719));
#74800=CARTESIAN_POINT('Ctrl Pts',(0.00333841734076304,-0.0336938721132296,
0.0705305686593232));
#74801=CARTESIAN_POINT('Ctrl Pts',(0.00333970576774112,-0.0336910493402228,
0.0705288651891934));
#74802=CARTESIAN_POINT('Ctrl Pts',(0.00334099516111529,-0.0336882266078996,
0.0705271623319283));
#74803=CARTESIAN_POINT('Ctrl Pts',(0.00334357585981417,-0.03368258127131,
0.0705237578716093));
#74804=CARTESIAN_POINT('Ctrl Pts',(0.00334486716514167,-0.0336797586670152,
0.0705220562685262));
#74805=CARTESIAN_POINT('Ctrl Pts',(0.00334615942774173,-0.033676936124375,
0.0705203552912372));
#74806=CARTESIAN_POINT('Origin',(0.0170501938751676,-0.0345562516464922,
0.0795280033588314));
#74807=CARTESIAN_POINT('Ctrl Pts',(0.00364343979401434,-0.034243627687391,
0.0705438029744785));
#74808=CARTESIAN_POINT('Ctrl Pts',(0.00350742983104413,-0.0339430054201809,
0.0707127818737128));
#74809=CARTESIAN_POINT('Ctrl Pts',(0.00338453444117993,-0.0336441434784052,
0.0708915255493037));
#74810=CARTESIAN_POINT('Ctrl Pts',(0.00349095540972062,-0.034243627687391,
0.0707419153480107));
#74811=CARTESIAN_POINT('Ctrl Pts',(0.00336241737809453,-0.0339430054201809,
0.0709166452906058));
#74812=CARTESIAN_POINT('Ctrl Pts',(0.00324740588475092,-0.0336441434784052,
0.0711005608549621));
#74813=CARTESIAN_POINT('Ctrl Pts',(0.00348943056587769,-0.034243627687391,
0.0707438964717461));
#74814=CARTESIAN_POINT('Ctrl Pts',(0.00336096725356504,-0.0339430054201809,
0.0709186839247747));
#74815=CARTESIAN_POINT('Ctrl Pts',(0.00324603459918663,-0.0336441434784052,
0.0711026512080186));
#74816=CARTESIAN_POINT('',(0.00346960944486587,-0.0341934961088741,0.0707711242950476));
#74817=CARTESIAN_POINT('',(0.00333471940384579,-0.0338664212862863,0.0709651919046286));
#74818=CARTESIAN_POINT('Origin',(0.0167062358242239,-0.0345610720407109,
0.0810105024913875));
#74819=CARTESIAN_POINT('Origin',(-0.00579672281994097,-0.0336938005072901,
0.0648926728744124));
#74820=CARTESIAN_POINT('',(0.00340506923980481,-0.0336938721132327,0.0708618587219638));
#74821=CARTESIAN_POINT('',(0.00337045993753882,-0.0336938721132427,0.0709139014562984));
#74822=CARTESIAN_POINT('',(0.00354414528154742,-0.0340203938281605,0.0706707686541035));
#74823=CARTESIAN_POINT('Origin',(0.0163566639023995,-0.0345589643241676,
0.081341162747349));
#74824=CARTESIAN_POINT('',(0.00354522704296507,-0.0341934961088739,0.0706715904874359));
#74825=CARTESIAN_POINT('Origin',(-0.00522923290532131,-0.0341934220717675,
0.0640054768600253));
#74826=CARTESIAN_POINT('',(0.00350741824392547,-0.0341934961088841,0.0707213573912518));
#74827=CARTESIAN_POINT('Ctrl Pts',(0.00349210169950806,-0.0340223579322397,
0.0703358767973186));
#74828=CARTESIAN_POINT('Ctrl Pts',(0.00343949499289216,-0.0339125849573575,
0.0703997597512552));
#74829=CARTESIAN_POINT('Ctrl Pts',(0.00338824748110293,-0.0338030433565231,
0.0704646866519656));
#74830=CARTESIAN_POINT('Ctrl Pts',(0.00333841734075952,-0.0336938721132327,
0.0705305686593148));
#74831=CARTESIAN_POINT('Ctrl Pts',(0.00350984166340604,-0.0340223579322397,
0.0704477985267156));
#74832=CARTESIAN_POINT('Ctrl Pts',(0.00345877864934265,-0.0339125849573575,
0.0705114368002823));
#74833=CARTESIAN_POINT('Ctrl Pts',(0.00340906868105594,-0.0338030433565231,
0.070576087241708));
#74834=CARTESIAN_POINT('Ctrl Pts',(0.00336076800024638,-0.0336938721132327,
0.0706416615387033));
#74835=CARTESIAN_POINT('Ctrl Pts',(0.00352758162730401,-0.0340223579322397,
0.0705597202561127));
#74836=CARTESIAN_POINT('Ctrl Pts',(0.00347806230579314,-0.0339125849573575,
0.0706231138493094));
#74837=CARTESIAN_POINT('Ctrl Pts',(0.00342988988100896,-0.0338030433565231,
0.0706874878314505));
#74838=CARTESIAN_POINT('Ctrl Pts',(0.00338311865973323,-0.0336938721132327,
0.0707527544180917));
#74839=CARTESIAN_POINT('Ctrl Pts',(0.00354532159120199,-0.0340223579322397,
0.0706716419855097));
#74840=CARTESIAN_POINT('Ctrl Pts',(0.00349734596224362,-0.0339125849573575,
0.0707347908983365));
#74841=CARTESIAN_POINT('Ctrl Pts',(0.00345071108096197,-0.0338030433565231,
0.0707988884211929));
#74842=CARTESIAN_POINT('Ctrl Pts',(0.00340546931922008,-0.0336938721132327,
0.0708638472974802));
#74843=CARTESIAN_POINT('',(0.00337174329029226,-0.0336938721132427,0.0706962136906497));
#74844=CARTESIAN_POINT('Ctrl Pts',(0.00334615943164338,-0.033710812066269,
0.0705203552942016));
#74845=CARTESIAN_POINT('Ctrl Pts',(0.00338039846916955,-0.0337611408994349,
0.0705463672979728));
#74846=CARTESIAN_POINT('Ctrl Pts',(0.00341401272022329,-0.0338121088781425,
0.0705719046403851));
#74847=CARTESIAN_POINT('Ctrl Pts',(0.00348002227141877,-0.0339153382773237,
0.0706220532665934));
#74848=CARTESIAN_POINT('Ctrl Pts',(0.00351238964548876,-0.0339675558473105,
0.0706466433344575));
#74849=CARTESIAN_POINT('Ctrl Pts',(0.00354414528157595,-0.0340203938281304,
0.0706707686541318));
#74850=CARTESIAN_POINT('Ctrl Pts',(0.00347161894542728,-0.0341934961088741,
0.0707708499059484));
#74851=CARTESIAN_POINT('Ctrl Pts',(0.00340175767936725,-0.0340287516182428,
0.0708670297160649));
#74852=CARTESIAN_POINT('Ctrl Pts',(0.00333593129294256,-0.0338644633275951,
0.0709660147615001));
#74853=CARTESIAN_POINT('Ctrl Pts',(0.00346960944486598,-0.0341934961088741,
0.0707711242950476));
#74854=CARTESIAN_POINT('Ctrl Pts',(0.0033997538515844,-0.0340287516182428,
0.0708673456500051));
#74855=CARTESIAN_POINT('Ctrl Pts',(0.00333393485017068,-0.0338644633275951,
0.0709663719703218));
#74856=CARTESIAN_POINT('Ctrl Pts',(0.00313478800011416,-0.0341934961088741,
0.0708168427966462));
#74857=CARTESIAN_POINT('Ctrl Pts',(0.00306587760083556,-0.0340287516182428,
0.0709199863211976));
#74858=CARTESIAN_POINT('Ctrl Pts',(0.00300128908429549,-0.0338644633275951,
0.0710258898306616));
#74859=CARTESIAN_POINT('',(0.00312767969907691,-0.0341764758832379,0.070827506981246));
#74860=CARTESIAN_POINT('',(0.00313478800011417,-0.034193496108874,0.0708168427966462));
#74861=CARTESIAN_POINT('Origin',(0.0166314748765275,-0.0345621026256374,
0.0804227582310192));
#74862=CARTESIAN_POINT('Ctrl Pts',(0.0031276797006797,-0.034176475883746,
0.0708275069803871));
#74863=CARTESIAN_POINT('Ctrl Pts',(0.0031634221400341,-0.0341260050040264,
0.0708512762931555));
#74864=CARTESIAN_POINT('Ctrl Pts',(0.00319854331262926,-0.0340749269147844,
0.0708746324073788));
#74865=CARTESIAN_POINT('Ctrl Pts',(0.00326757024200344,-0.0339715436305533,
0.0709205364926982));
#74866=CARTESIAN_POINT('Ctrl Pts',(0.00330144980820865,-0.0339192778236031,
0.070943067053803));
#74867=CARTESIAN_POINT('Ctrl Pts',(0.0033347194038929,-0.0338664212854243,
0.0709651919024983));
#74868=CARTESIAN_POINT('',(0.00330219872250002,-0.0341934961088841,0.070793983545857));
#74869=CARTESIAN_POINT('Origin',(0.00812378219310841,-0.0315241814719618,
0.07415));
#74870=CARTESIAN_POINT('',(0.00312767969922361,-0.0342105180190374,0.0708275069823544));
#74871=CARTESIAN_POINT('',(0.00312059419090093,-0.0341934961088739,0.0708381863255021));
#74872=CARTESIAN_POINT('Origin',(0.0166607652514386,-0.0345621705449535,
0.0803881656872907));
#74873=CARTESIAN_POINT('Origin',(0.017198625998726,-0.0345621038351193,
0.0795699252462993));
#74874=CARTESIAN_POINT('Origin',(0.0171780478231302,-0.0345621716956665,
0.0796103116433129));
#74875=CARTESIAN_POINT('Ctrl Pts',(0.00340589986854741,-0.0346945769586965,
0.070860609688088));
#74876=CARTESIAN_POINT('Ctrl Pts',(0.00333700227146439,-0.0345275153362944,
0.0709594276223129));
#74877=CARTESIAN_POINT('Ctrl Pts',(0.0032711945870095,-0.0343603235965185,
0.0710604378819296));
#74878=CARTESIAN_POINT('Ctrl Pts',(0.00320866700499458,-0.034193496108874,
0.0711633388307211));
#74879=CARTESIAN_POINT('Ctrl Pts',(0.00335947725581904,-0.0346945769586965,
0.0709304163453157));
#74880=CARTESIAN_POINT('Ctrl Pts',(0.00329204178712072,-0.0345275153362944,
0.0710302066197508));
#74881=CARTESIAN_POINT('Ctrl Pts',(0.00322772718843645,-0.0343603235965185,
0.0711321434884827));
#74882=CARTESIAN_POINT('Ctrl Pts',(0.00316671919296221,-0.034193496108874,
0.0712359226404277));
#74883=CARTESIAN_POINT('Ctrl Pts',(0.00331305464309072,-0.0346945769586965,
0.0710002230025449));
#74884=CARTESIAN_POINT('Ctrl Pts',(0.00324708130277711,-0.0345275153362944,
0.0711009856171904));
#74885=CARTESIAN_POINT('Ctrl Pts',(0.00318425978986348,-0.0343603235965185,
0.0712038490950376));
#74886=CARTESIAN_POINT('Ctrl Pts',(0.00312477138092993,-0.034193496108874,
0.0713085064501362));
#74887=CARTESIAN_POINT('Ctrl Pts',(0.00326663203036231,-0.0346945769586965,
0.0710700296597711));
#74888=CARTESIAN_POINT('Ctrl Pts',(0.00320212081843338,-0.0345275153362944,
0.0711717646146266));
#74889=CARTESIAN_POINT('Ctrl Pts',(0.00314079239129035,-0.0343603235965185,
0.0712755547015891));
#74890=CARTESIAN_POINT('Ctrl Pts',(0.00308282356889745,-0.034193496108874,
0.071381090259841));
#74891=CARTESIAN_POINT('',(0.00326663203069789,-0.0346945769586966,0.0710700296592668));
#74892=CARTESIAN_POINT('',(0.00314419377144035,-0.034366772783143,0.0712721841353108));
#74893=CARTESIAN_POINT('Origin',(0.0175632353100188,-0.0345626457064379,
0.0799190059793397));
#74894=CARTESIAN_POINT('Origin',(-0.00642490442479576,-0.034193477102909,
0.0657419929855118));
#74895=CARTESIAN_POINT('',(0.00320791644279703,-0.034193496108874,0.0711646375555192));
#74896=CARTESIAN_POINT('',(0.00317664322440932,-0.0341934961088841,0.0712187507314761));
#74897=CARTESIAN_POINT('',(0.00333471940511753,-0.0345211942962721,0.0709651919033584));
#74898=CARTESIAN_POINT('Origin',(0.0172942183244265,-0.034562559611922,
0.0803175290668221));
#74899=CARTESIAN_POINT('',(0.00333585063525286,-0.0346945769586885,0.0709659441906129));
#74900=CARTESIAN_POINT('Origin',(-0.0058766013599473,-0.0346945685853852,
0.064839506119231));
#74901=CARTESIAN_POINT('',(0.00330124133298537,-0.0346945769587026,0.0710179869249498));
#74902=CARTESIAN_POINT('Ctrl Pts',(0.00326174992171197,-0.0345231616327842,
0.0706342295023815));
#74903=CARTESIAN_POINT('Ctrl Pts',(0.00321328997521123,-0.0344132092796988,
0.0707012457720489));
#74904=CARTESIAN_POINT('Ctrl Pts',(0.00316621870769734,-0.034303273855898,
0.0707692609397534));
#74905=CARTESIAN_POINT('Ctrl Pts',(0.00312059419090085,-0.0341934961088739,
0.0708381863255021));
#74906=CARTESIAN_POINT('Ctrl Pts',(0.00328648247903689,-0.0345231616327842,
0.0707448162861609));
#74907=CARTESIAN_POINT('Ctrl Pts',(0.00323954681565681,-0.0344132092796988,
0.0708114916523462));
#74908=CARTESIAN_POINT('Ctrl Pts',(0.00319399270129795,-0.034303273855898,
0.0708791344055637));
#74909=CARTESIAN_POINT('Ctrl Pts',(0.0031498762762636,-0.0341934961088739,
0.0709476563927137));
#74910=CARTESIAN_POINT('Ctrl Pts',(0.00331121503636181,-0.0345231616327842,
0.0708554030699402));
#74911=CARTESIAN_POINT('Ctrl Pts',(0.00326580365610239,-0.0344132092796988,
0.0709217375326434));
#74912=CARTESIAN_POINT('Ctrl Pts',(0.00322176669489857,-0.034303273855898,
0.0709890078713739));
#74913=CARTESIAN_POINT('Ctrl Pts',(0.00317915836162634,-0.0341934961088739,
0.0710571264599253));
#74914=CARTESIAN_POINT('Ctrl Pts',(0.00333594759368673,-0.0345231616327842,
0.0709659898537196));
#74915=CARTESIAN_POINT('Ctrl Pts',(0.00329206049654798,-0.0344132092796988,
0.0710319834129407));
#74916=CARTESIAN_POINT('Ctrl Pts',(0.00324954068849918,-0.034303273855898,
0.0710988813371842));
#74917=CARTESIAN_POINT('Ctrl Pts',(0.00320844044698908,-0.0341934961088739,
0.0711665965271368));
#74918=CARTESIAN_POINT('',(0.00316425531685898,-0.0341934961088839,0.0710014119405207));
#74919=CARTESIAN_POINT('Ctrl Pts',(0.00312767970209473,-0.0342105180195393,
0.0708275069842621));
#74920=CARTESIAN_POINT('Ctrl Pts',(0.00316346231527264,-0.0342610556241295,
0.0708513030297961));
#74921=CARTESIAN_POINT('Ctrl Pts',(0.00319860282795846,-0.0343122189870136,
0.0708746720675967));
#74922=CARTESIAN_POINT('Ctrl Pts',(0.00326763045583263,-0.0344158119695204,
0.070920576612573));
#74923=CARTESIAN_POINT('Ctrl Pts',(0.0033014893382135,-0.0344681990450117,
0.0709430933444522));
#74924=CARTESIAN_POINT('Ctrl Pts',(0.0033347194051368,-0.0345211942962544,
0.0709651919033716));
#74925=CARTESIAN_POINT('Ctrl Pts',(0.00326861985010767,-0.0346945769586932,
0.0710696297319652));
#74926=CARTESIAN_POINT('Ctrl Pts',(0.00320493537441614,-0.034529677707698,
0.071170006778004));
#74927=CARTESIAN_POINT('Ctrl Pts',(0.00314545399186463,-0.0343648066251421,
0.0712729301910127));
#74928=CARTESIAN_POINT('Ctrl Pts',(0.00326663203070282,-0.0346945769586932,
0.0710700296592592));
#74929=CARTESIAN_POINT('Ctrl Pts',(0.00320295582322511,-0.034529677707698,
0.0711704478020577));
#74930=CARTESIAN_POINT('Ctrl Pts',(0.00314348440038918,-0.0343648066251421,
0.0712734119349765));
#74931=CARTESIAN_POINT('Ctrl Pts',(0.00293534196805695,-0.0346945769586932,
0.0711366815583036));
#74932=CARTESIAN_POINT('Ctrl Pts',(0.00287304374143061,-0.034529677707698,
0.0712439488887339));
#74933=CARTESIAN_POINT('Ctrl Pts',(0.00281523220519733,-0.0343648066251421,
0.0713536994035245));
#74934=CARTESIAN_POINT('',(0.00292891730306486,-0.0346775396664965,0.0711477710334621));
#74935=CARTESIAN_POINT('',(0.00293534196805525,-0.0346945769586886,0.0711366815583065));
#74936=CARTESIAN_POINT('Origin',(0.0173785634158705,-0.0345626618297238,
0.07932215959235));
#74937=CARTESIAN_POINT('Ctrl Pts',(0.00292891730466133,-0.0346775396670097,
0.0711477710325909));
#74938=CARTESIAN_POINT('Ctrl Pts',(0.00296611097177062,-0.0346269749928187,
0.0711692660723642));
#74939=CARTESIAN_POINT('Ctrl Pts',(0.00300264364239575,-0.0345757902890786,
0.0711903790662173));
#74940=CARTESIAN_POINT('Ctrl Pts',(0.00307441699124798,-0.0344721681087842,
0.0712318584991063));
#74941=CARTESIAN_POINT('Ctrl Pts',(0.0031096295281245,-0.0344197714289452,
0.0712522086811331));
#74942=CARTESIAN_POINT('Ctrl Pts',(0.00314419377146478,-0.0343667727830583,
0.0712721841350437));
#74943=CARTESIAN_POINT('',(0.00310098699938657,-0.0346945769587026,0.0711033556087966));
#74944=CARTESIAN_POINT('Origin',(0.00812378219310841,-0.0315241814719618,
0.07415));
#74945=CARTESIAN_POINT('',(0.0029289173037152,-0.0347116136489618,0.0711477710346915));
#74946=CARTESIAN_POINT('',(0.00292251633834764,-0.0346945769586885,0.0711588742072382));
#74947=CARTESIAN_POINT('Origin',(0.0173996004797876,-0.0345626684329631,
0.0792820256874896));
#74948=CARTESIAN_POINT('Origin',(0.0172257359434592,-0.0345626628847385,
0.0795866077582412));
#74949=CARTESIAN_POINT('Origin',(0.0172014601357675,-0.0345626695489208,
0.0796248698269157));
#74950=CARTESIAN_POINT('Ctrl Pts',(0.00322802826454031,-0.0352450361874068,
0.0711316633559964));
#74951=CARTESIAN_POINT('Ctrl Pts',(0.00311418983000982,-0.0349452760959493,
0.0713163097453188));
#74952=CARTESIAN_POINT('Ctrl Pts',(0.00301458312004364,-0.034644428984174,
0.0715090063503637));
#74953=CARTESIAN_POINT('Ctrl Pts',(0.00322675112972715,-0.0352450361874068,
0.0711338415551767));
#74954=CARTESIAN_POINT('Ctrl Pts',(0.0031129948473268,-0.0349452760959493,
0.0713185361124289));
#74955=CARTESIAN_POINT('Ctrl Pts',(0.00301347368431078,-0.034644428984174,
0.0715112745605292));
#74956=CARTESIAN_POINT('Ctrl Pts',(0.00310030213832565,-0.0352450361874068,
0.0713495048403541));
#74957=CARTESIAN_POINT('Ctrl Pts',(0.00299467973019645,-0.0349452760959493,
0.0715389684995745));
#74958=CARTESIAN_POINT('Ctrl Pts',(0.00290362856224478,-0.034644428984174,
0.0717358498244349));
#74959=CARTESIAN_POINT('Ctrl Pts',(0.00309903764841163,-0.0352450361874068,
0.071351661473206));
#74960=CARTESIAN_POINT('Ctrl Pts',(0.00299349657902514,-0.0349452760959493,
0.0715411728234459));
#74961=CARTESIAN_POINT('Ctrl Pts',(0.00290253011102412,-0.034644428984174,
0.0717380955770739));
#74962=CARTESIAN_POINT('',(0.00308283706751842,-0.0351951634053268,0.0713810607548514));
#74963=CARTESIAN_POINT('',(0.00297332029856974,-0.0348678972925434,0.0715905337914116));
#74964=CARTESIAN_POINT('Origin',(0.0181602499772387,-0.0345636767877706,
0.0786663964587444));
#74965=CARTESIAN_POINT('Origin',(-0.00692204325513113,-0.0346946199340719,
0.0666731392099248));
#74966=CARTESIAN_POINT('',(0.00303016433057554,-0.0346945769330288,0.0714791982349079));
#74967=CARTESIAN_POINT('',(0.00300235061297133,-0.0346945769458129,0.0715351683001273));
#74968=CARTESIAN_POINT('',(0.00314419377157413,-0.0350221583435276,0.0712721841351256));
#74969=CARTESIAN_POINT('Origin',(0.0179842440841164,-0.0345628458719571,
0.0791137948493126));
#74970=CARTESIAN_POINT('',(0.00314526619307874,-0.0351951360298761,0.0712728004182273));
#74971=CARTESIAN_POINT('Origin',(-0.00639508383650517,-0.0351951838366808,
0.0657592203489523));
#74972=CARTESIAN_POINT('',(0.00308282356910537,-0.0351951371328751,0.071381090259249));
#74973=CARTESIAN_POINT('Ctrl Pts',(0.00305058646273447,-0.0350241211494343,
0.0709464574169615));
#74974=CARTESIAN_POINT('Ctrl Pts',(0.00300645897715671,-0.0349144232818962,
0.0710163386080562));
#74975=CARTESIAN_POINT('Ctrl Pts',(0.00296374957330617,-0.0348045283579412,
0.0710871737730708));
#74976=CARTESIAN_POINT('Ctrl Pts',(0.00292251633280762,-0.0346945769439157,
0.0711588742168717));
#74977=CARTESIAN_POINT('Ctrl Pts',(0.00308221404201289,-0.0350241211494343,
0.0710552730317966));
#74978=CARTESIAN_POINT('Ctrl Pts',(0.00303958544691334,-0.0349144232818962,
0.0711247185659545));
#74979=CARTESIAN_POINT('Ctrl Pts',(0.00299836682535904,-0.0348045283579412,
0.0711950868301334));
#74980=CARTESIAN_POINT('Ctrl Pts',(0.00295861432721755,-0.0346945769439157,
0.0712662896561834));
#74981=CARTESIAN_POINT('Ctrl Pts',(0.00311384162129132,-0.0350241211494343,
0.0711640886466316));
#74982=CARTESIAN_POINT('Ctrl Pts',(0.00307271191666998,-0.0349144232818962,
0.0712330985238528));
#74983=CARTESIAN_POINT('Ctrl Pts',(0.0030329840774119,-0.0348045283579412,
0.0713029998871961));
#74984=CARTESIAN_POINT('Ctrl Pts',(0.00299471232162748,-0.0346945769439157,
0.0713737050954951));
#74985=CARTESIAN_POINT('Ctrl Pts',(0.00314546920056974,-0.0350241211494343,
0.0712729042614667));
#74986=CARTESIAN_POINT('Ctrl Pts',(0.00310583838642662,-0.0349144232818962,
0.0713414784817511));
#74987=CARTESIAN_POINT('Ctrl Pts',(0.00306760132946477,-0.0348045283579412,
0.0714109129442587));
#74988=CARTESIAN_POINT('Ctrl Pts',(0.00303081031603742,-0.0346945769439157,
0.0714811205348068));
#74989=CARTESIAN_POINT('',(0.00297634033452877,-0.0346945769458128,0.0713190362207805));
#74990=CARTESIAN_POINT('Ctrl Pts',(0.00292891730655676,-0.0347116136492798,
0.0711477710363316));
#74991=CARTESIAN_POINT('Ctrl Pts',(0.00296609619679808,-0.0347621546532283,
0.0711692575511029));
#74992=CARTESIAN_POINT('Ctrl Pts',(0.00300262138168077,-0.0348133084096993,
0.0711903662748816));
#74993=CARTESIAN_POINT('Ctrl Pts',(0.00307439482349242,-0.034916856154457,
0.0712318457571271));
#74994=CARTESIAN_POINT('Ctrl Pts',(0.00310961461153599,-0.0349692089015911,
0.0712522000627862));
#74995=CARTESIAN_POINT('Ctrl Pts',(0.00314419377159582,-0.0350221583435,
0.0712721841351612));
#74996=CARTESIAN_POINT('Ctrl Pts',(0.00308423689773535,-0.0351951371254879,
0.0713807122088686));
#74997=CARTESIAN_POINT('Ctrl Pts',(0.00302698361016444,-0.0350307338980929,
0.0714849016459314));
#74998=CARTESIAN_POINT('Ctrl Pts',(0.00297408550704852,-0.0348659306897834,
0.0715913683938852));
#74999=CARTESIAN_POINT('Ctrl Pts',(0.00308282356920761,-0.0351951371254879,
0.0713810902593042));
#75000=CARTESIAN_POINT('Ctrl Pts',(0.00302557809759226,-0.0350307338980929,
0.0714853089160476));
#75001=CARTESIAN_POINT('Ctrl Pts',(0.00297268901143414,-0.0348659306897834,
0.071591804535672));
#75002=CARTESIAN_POINT('Ctrl Pts',(0.00284594823493688,-0.0351951371254879,
0.071444451906329));
#75003=CARTESIAN_POINT('Ctrl Pts',(0.0027900127256193,-0.0350307338980929,
0.0715535678119876));
#75004=CARTESIAN_POINT('Ctrl Pts',(0.0027386348909858,-0.0348659306897834,
0.0716649023537017));
#75005=CARTESIAN_POINT('Origin',(-0.00178922270627967,-0.0308609197384417,
0.0692238396757387));
#75006=CARTESIAN_POINT('',(0.00297955126429345,-0.0351951371254879,0.071408714508792));
#75007=CARTESIAN_POINT('Origin',(0.00905257469815753,-0.0351840467441159,
0.0744534635602127));
#75008=CARTESIAN_POINT('Origin',(-0.00292136006055052,-0.0352322614082497,
0.0695486482211981));
#75009=CARTESIAN_POINT('',(0.00287241071720265,-0.0351951142564652,0.0718045976452916));
#75010=CARTESIAN_POINT('',(0.00282402548190293,-0.0351951372916786,0.0719195115328626));
#75011=CARTESIAN_POINT('Origin',(0.00817580825674042,-0.0352875120661354,
0.0744865877874527));
#75012=CARTESIAN_POINT('Origin',(0.0123045189010117,-0.0298325076521961,
0.0679197005801442));
#75013=CARTESIAN_POINT('Origin',(0.00219055981987634,-0.0338732045131652,
0.0682298561825369));
#75014=CARTESIAN_POINT('Ctrl Pts',(0.00525422229196418,-0.0321934096636942,
0.0691656483150708));
#75015=CARTESIAN_POINT('Ctrl Pts',(0.00516500477033232,-0.0320508460843443,
0.0692170120708283));
#75016=CARTESIAN_POINT('Ctrl Pts',(0.00507723456177527,-0.0319086045661309,
0.0692707341969115));
#75017=CARTESIAN_POINT('Ctrl Pts',(0.00499109112805847,-0.0317669892865267,
0.0693266834617408));
#75018=CARTESIAN_POINT('Ctrl Pts',(0.0051824833593981,-0.0321934096636942,
0.0692090529021806));
#75019=CARTESIAN_POINT('Ctrl Pts',(0.00509404275920641,-0.0320508460843443,
0.0692617007506693));
#75020=CARTESIAN_POINT('Ctrl Pts',(0.0050070833873262,-0.0319086045661309,
0.0693166851269273));
#75021=CARTESIAN_POINT('Ctrl Pts',(0.00492178273589887,-0.0317669892865267,
0.0693738722252596));
#75022=CARTESIAN_POINT('Ctrl Pts',(0.00511074442683202,-0.0321934096636942,
0.0692524574892904));
#75023=CARTESIAN_POINT('Ctrl Pts',(0.00502308074808051,-0.0320508460843443,
0.0693063894305101));
#75024=CARTESIAN_POINT('Ctrl Pts',(0.00493693221287711,-0.0319086045661309,
0.0693626360569431));
#75025=CARTESIAN_POINT('Ctrl Pts',(0.00485247434373929,-0.0317669892865268,
0.0694210609887785));
#75026=CARTESIAN_POINT('Ctrl Pts',(0.00503900549426594,-0.0321934096636942,
0.0692958620764002));
#75027=CARTESIAN_POINT('Ctrl Pts',(0.0049521187369546,-0.0320508460843443,
0.0693510781103512));
#75028=CARTESIAN_POINT('Ctrl Pts',(0.00486678103842803,-0.0319086045661309,
0.069408586986959));
#75029=CARTESIAN_POINT('Ctrl Pts',(0.0047831659515797,-0.0317669892865268,
0.0694682497522974));
#75030=CARTESIAN_POINT('',(0.00504028891794717,-0.0321934096636942,0.0692950855597615));
#75031=CARTESIAN_POINT('',(0.00484343027988913,-0.0318665617511257,0.0694258687238353));
#75032=CARTESIAN_POINT('Origin',(0.0134738133231417,-0.0326371944421483,
0.0837205342863425));
#75033=CARTESIAN_POINT('Origin',(-0.00140840499145849,-0.0316939261509243,
0.0604224168376222));
#75034=CARTESIAN_POINT('',(0.00514633205196241,-0.0320197221621856,0.0692293923318842));
#75035=CARTESIAN_POINT('Ctrl Pts',(0.00514615460494484,-0.032019739209477,
0.0692294445567315));
#75036=CARTESIAN_POINT('Ctrl Pts',(0.00512111726123343,-0.0319792716576067,
0.0692445957233421));
#75037=CARTESIAN_POINT('Ctrl Pts',(0.00509608144439834,-0.0319386439829713,
0.069260006738462));
#75038=CARTESIAN_POINT('Ctrl Pts',(0.00507102530504198,-0.0318979099381645,
0.0692757009830988));
#75039=CARTESIAN_POINT('Ctrl Pts',(0.0050459696609371,-0.0318571766984935,
0.0692913949175282));
#75040=CARTESIAN_POINT('Ctrl Pts',(0.00502102009849267,-0.0318163871833572,
0.0693072907935115));
#75041=CARTESIAN_POINT('Ctrl Pts',(0.00499626054190498,-0.0317755399638303,
0.0693233309661393));
#75042=CARTESIAN_POINT('',(0.00514723722102942,-0.0321934096636183,0.0692303780603392));
#75043=CARTESIAN_POINT('Origin',(0.00393412247364323,-0.0324113231919104,
0.067265984065929));
#75044=CARTESIAN_POINT('',(0.00509376306949829,-0.0321934096636663,0.0692627318100604));
#75045=CARTESIAN_POINT('Ctrl Pts',(0.00504225838682757,-0.0321934096636618,
0.0692955702036599));
#75046=CARTESIAN_POINT('Ctrl Pts',(0.00497531201661472,-0.0320835708272592,
0.0693380668185477));
#75047=CARTESIAN_POINT('Ctrl Pts',(0.00490928394325373,-0.0319739230346488,
0.069381924235324));
#75048=CARTESIAN_POINT('Ctrl Pts',(0.00484425433860424,-0.0318646057455572,
0.0694270798579903));
#75049=CARTESIAN_POINT('Ctrl Pts',(0.00493222216080788,-0.0321934096636618,
0.0692684926534038));
#75050=CARTESIAN_POINT('Ctrl Pts',(0.00486490237007399,-0.0320835708272592,
0.0693125067536056));
#75051=CARTESIAN_POINT('Ctrl Pts',(0.00479853249707075,-0.0319739230346488,
0.069357888503411));
#75052=CARTESIAN_POINT('Ctrl Pts',(0.00473319300128829,-0.0318646057455572,
0.069404573322981));
#75053=CARTESIAN_POINT('Ctrl Pts',(0.00482218593478819,-0.0321934096636618,
0.0692414151031477));
#75054=CARTESIAN_POINT('Ctrl Pts',(0.00475449272353326,-0.0320835708272592,
0.0692869466886635));
#75055=CARTESIAN_POINT('Ctrl Pts',(0.00468778105088776,-0.0319739230346488,
0.0693338527714981));
#75056=CARTESIAN_POINT('Ctrl Pts',(0.00462213166397235,-0.0318646057455572,
0.0693820667879717));
#75057=CARTESIAN_POINT('Ctrl Pts',(0.00471214970876851,-0.0321934096636618,
0.0692143375528915));
#75058=CARTESIAN_POINT('Ctrl Pts',(0.00464408307699253,-0.0320835708272592,
0.0692613866237214));
#75059=CARTESIAN_POINT('Ctrl Pts',(0.00457702960470477,-0.0319739230346488,
0.0693098170395851));
#75060=CARTESIAN_POINT('Ctrl Pts',(0.0045110703266564,-0.0318646057455572,
0.0693595602529624));
#75061=CARTESIAN_POINT('',(0.00470161482932084,-0.0321763980308261,0.0692216361222138));
#75062=CARTESIAN_POINT('',(0.00471214970874164,-0.0321934096636185,0.0692143375529101));
#75063=CARTESIAN_POINT('Origin',(0.01362936035573,-0.0326386230750649,0.0831543836591411));
#75064=CARTESIAN_POINT('Ctrl Pts',(0.0047016148311254,-0.0321763980306274,
0.069221636124815));
#75065=CARTESIAN_POINT('Ctrl Pts',(0.00472609410383957,-0.0321259596174904,
0.0692568894454666));
#75066=CARTESIAN_POINT('Ctrl Pts',(0.00475014924139586,-0.0320749164631554,
0.0692915319565902));
#75067=CARTESIAN_POINT('Ctrl Pts',(0.00479743060497968,-0.0319716057793888,
0.0693596232389876));
#75068=CARTESIAN_POINT('Ctrl Pts',(0.00482063840858775,-0.0319193786690074,
0.0693930454795933));
#75069=CARTESIAN_POINT('Ctrl Pts',(0.00484343028094309,-0.0318665617525257,
0.0694258687253562));
#75070=CARTESIAN_POINT('',(0.00487621931335441,-0.0321934096636664,0.0692547115563458));
#75071=CARTESIAN_POINT('Origin',(0.00812378219310841,-0.0315241814719618,
0.07415));
#75072=CARTESIAN_POINT('',(0.00470161482910887,-0.032210423332379,0.0692216361219087));
#75073=CARTESIAN_POINT('',(0.00469109556167723,-0.0321934096636183,0.0692289571744985));
#75074=CARTESIAN_POINT('Origin',(0.0136698375773385,-0.0326387233381217,
0.0831339680613262));
#75075=CARTESIAN_POINT('Origin',(0.014637217912418,-0.0326386244463913,
0.0824545485597093));
#75076=CARTESIAN_POINT('Origin',(0.0146039435917886,-0.0326387242889573,
0.0824853382453447));
#75077=CARTESIAN_POINT('Ctrl Pts',(0.00497707169695243,-0.0327445246967096,
0.0693358190672367));
#75078=CARTESIAN_POINT('Ctrl Pts',(0.00479550189480918,-0.0324436878339359,
0.0694544991937564));
#75079=CARTESIAN_POINT('Ctrl Pts',(0.00462338738547849,-0.0321434074405927,
0.0695865187421534));
#75080=CARTESIAN_POINT('Ctrl Pts',(0.00477083115617685,-0.0327445246967096,
0.0694771160570865));
#75081=CARTESIAN_POINT('Ctrl Pts',(0.0045945904571248,-0.0324436878339359,
0.0696035746727626));
#75082=CARTESIAN_POINT('Ctrl Pts',(0.00442837581906062,-0.0321434074405927,
0.0697429492026246));
#75083=CARTESIAN_POINT('',(0.00474153088763896,-0.0326943950436612,0.0694982797690907));
#75084=CARTESIAN_POINT('',(0.00455327264731455,-0.0323666188837389,0.0696411657179049));
#75085=CARTESIAN_POINT('Origin',(0.0146890686202625,-0.0326395579112807,
0.0830502003442997));
#75086=CARTESIAN_POINT('Origin',(-0.00230334794594286,-0.0321933825602924,
0.0609826366339883));
#75087=CARTESIAN_POINT('',(0.00465211103054775,-0.0321934096532689,0.0695646293131717));
#75088=CARTESIAN_POINT('',(0.00460311353637187,-0.0321934096584275,0.0696034300336581));
#75089=CARTESIAN_POINT('',(0.0048434302793459,-0.0325210109756239,0.0694258687230481));
#75090=CARTESIAN_POINT('Origin',(0.0142858016141189,-0.0326393129159858,
0.0833120402794587));
#75091=CARTESIAN_POINT('',(0.00484420513512571,-0.0326943950436593,0.0694269846156556));
#75092=CARTESIAN_POINT('Origin',(-0.0014653897014078,-0.0326943765538158,
0.0603403499416489));
#75093=CARTESIAN_POINT('',(0.00479286801139234,-0.0326943950436702,0.0694626321923832));
#75094=CARTESIAN_POINT('Ctrl Pts',(0.00489742048002139,-0.0325229783203769,
0.0690912857269507));
#75095=CARTESIAN_POINT('Ctrl Pts',(0.00482768621439418,-0.032413025309245,
0.0691357610526098));
#75096=CARTESIAN_POINT('Ctrl Pts',(0.00475888255457854,-0.0323031222208069,
0.0691816721755787));
#75097=CARTESIAN_POINT('Ctrl Pts',(0.00469109555799938,-0.0321934096576658,
0.069228957177064));
#75098=CARTESIAN_POINT('Ctrl Pts',(0.00487970651298126,-0.0325229783203769,
0.0692032114058989));
#75099=CARTESIAN_POINT('Ctrl Pts',(0.0048115151403907,-0.032413025309245,
0.0692479309182062));
#75100=CARTESIAN_POINT('Ctrl Pts',(0.00474425919091624,-0.0323031222208069,
0.0692940542740633));
#75101=CARTESIAN_POINT('Ctrl Pts',(0.00467802272988302,-0.0321934096576658,
0.0693415193527775));
#75102=CARTESIAN_POINT('Ctrl Pts',(0.00486199254594113,-0.0325229783203769,
0.0693151370848471));
#75103=CARTESIAN_POINT('Ctrl Pts',(0.00479534406638722,-0.032413025309245,
0.0693601007838027));
#75104=CARTESIAN_POINT('Ctrl Pts',(0.00472963582725395,-0.0323031222208069,
0.0694064363725479));
#75105=CARTESIAN_POINT('Ctrl Pts',(0.00466494990176666,-0.0321934096576658,
0.0694540815284909));
#75106=CARTESIAN_POINT('Ctrl Pts',(0.004844278578901,-0.0325229783203769,
0.0694270627637952));
#75107=CARTESIAN_POINT('Ctrl Pts',(0.00477917299238373,-0.032413025309245,
0.0694722706493991));
#75108=CARTESIAN_POINT('Ctrl Pts',(0.00471501246359166,-0.0323031222208069,
0.0695188184710325));
#75109=CARTESIAN_POINT('Ctrl Pts',(0.0046518770736503,-0.0321934096576658,
0.0695666437042044));
#75110=CARTESIAN_POINT('',(0.00467160329642365,-0.0321934096584275,0.0693967932434306));
#75111=CARTESIAN_POINT('Ctrl Pts',(0.00470161483108758,-0.0322104233328934,
0.0692216361247604));
#75112=CARTESIAN_POINT('Ctrl Pts',(0.00472612727361019,-0.0322609421831263,
0.0692569372142288));
#75113=CARTESIAN_POINT('Ctrl Pts',(0.00475019861516221,-0.0323120888240518,
0.0692916030612151));
#75114=CARTESIAN_POINT('Ctrl Pts',(0.00479748033672828,-0.0324156524631818,
0.0693596948591533));
#75115=CARTESIAN_POINT('Ctrl Pts',(0.00482067128146181,-0.0324680267167314,
0.069393092820786));
#75116=CARTESIAN_POINT('Ctrl Pts',(0.00484343027936698,-0.0325210109755913,
0.0694258687230862));
#75117=CARTESIAN_POINT('Origin',(0.0150798194753273,-0.0262834582512383,
0.0704734620679012));
#75118=CARTESIAN_POINT('Origin',(0.00638952005960307,-0.0342770595364488,
0.0621161235546925));
#75119=CARTESIAN_POINT('Ctrl Pts',(0.00474352641682006,-0.0326943950436604,
0.0694986397053626));
#75120=CARTESIAN_POINT('Ctrl Pts',(0.00467942195438166,-0.0325844576448134,
0.0695452259652344));
#75121=CARTESIAN_POINT('Ctrl Pts',(0.00461627643540422,-0.0324744968375322,
0.0695931413074722));
#75122=CARTESIAN_POINT('Ctrl Pts',(0.00455416991882988,-0.0323646534831895,
0.0696423232242119));
#75123=CARTESIAN_POINT('Ctrl Pts',(0.00463200727016761,-0.0326943950436604,
0.0694785248473886));
#75124=CARTESIAN_POINT('Ctrl Pts',(0.00456762558728707,-0.0325844576448134,
0.0695266480501104));
#75125=CARTESIAN_POINT('Ctrl Pts',(0.00450423461474615,-0.0324744968375322,
0.0695761061773433));
#75126=CARTESIAN_POINT('Ctrl Pts',(0.0044419146987117,-0.0323646534831895,
0.0696268347401793));
#75127=CARTESIAN_POINT('Ctrl Pts',(0.00452048812351516,-0.0326943950436604,
0.0694584099894146));
#75128=CARTESIAN_POINT('Ctrl Pts',(0.00445582922019247,-0.0325844576448134,
0.0695080701349864));
#75129=CARTESIAN_POINT('Ctrl Pts',(0.00439219279408808,-0.0324744968375322,
0.0695590710472144));
#75130=CARTESIAN_POINT('Ctrl Pts',(0.00432965947859353,-0.0323646534831895,
0.0696113462561468));
#75131=CARTESIAN_POINT('Ctrl Pts',(0.00440896897686272,-0.0326943950436604,
0.0694382951314406));
#75132=CARTESIAN_POINT('Ctrl Pts',(0.00434403285309788,-0.0325844576448134,
0.0694894922198624));
#75133=CARTESIAN_POINT('Ctrl Pts',(0.00428015097343002,-0.0324744968375322,
0.0695420359170855));
#75134=CARTESIAN_POINT('Ctrl Pts',(0.00421740425847536,-0.0323646534831895,
0.0695958577721142));
#75135=CARTESIAN_POINT('',(0.00439891316645083,-0.0326773559991153,0.0694462407890779));
#75136=CARTESIAN_POINT('',(0.00440896897686215,-0.0326943950436594,0.069438295131441));
#75137=CARTESIAN_POINT('Origin',(0.0147469639985691,-0.0326395670261279,
0.0824328167942656));
#75138=CARTESIAN_POINT('Ctrl Pts',(0.00439891316852646,-0.0326773559987416,
0.0694462407917005));
#75139=CARTESIAN_POINT('Ctrl Pts',(0.00442557915302754,-0.0326267922586054,
0.0694799145582994));
#75140=CARTESIAN_POINT('Ctrl Pts',(0.00445177250220936,-0.0325756109579523,
0.0695129914817018));
#75141=CARTESIAN_POINT('Ctrl Pts',(0.00450323622179075,-0.0324719985462366,
0.0695779797922375));
#75142=CARTESIAN_POINT('Ctrl Pts',(0.00452848595148346,-0.0324196091621776,
0.0696098651143161));
#75143=CARTESIAN_POINT('Ctrl Pts',(0.00455327264734479,-0.0323666188837757,
0.0696411657179432));
#75144=CARTESIAN_POINT('',(0.00457524993226056,-0.0326943950436703,0.0694682874502759));
#75145=CARTESIAN_POINT('Origin',(0.00812378219310841,-0.0315241814719618,
0.07415));
#75146=CARTESIAN_POINT('',(0.00439891316647808,-0.032711433838006,0.0694462407891124));
#75147=CARTESIAN_POINT('',(0.0043888743489824,-0.0326943950436593,0.0694542079053788));
#75148=CARTESIAN_POINT('Origin',(0.0147820001238029,-0.0326395667286811,
0.0824040842777885));
#75149=CARTESIAN_POINT('Origin',(0.0146681926336194,-0.032639567897862,
0.0824951977524825));
#75150=CARTESIAN_POINT('Origin',(0.0146321924657103,-0.0326395677254717,
0.0825227126084884));
#75151=CARTESIAN_POINT('Ctrl Pts',(0.00468096466956283,-0.0332451089994433,
0.0695429258200494));
#75152=CARTESIAN_POINT('Ctrl Pts',(0.00450720602402564,-0.0329451141710254,
0.0696727738073743));
#75153=CARTESIAN_POINT('Ctrl Pts',(0.00434372168968992,-0.0326442513127493,
0.0698153411217842));
#75154=CARTESIAN_POINT('Ctrl Pts',(0.00448400425883616,-0.0332451089994433,
0.0696968952865237));
#75155=CARTESIAN_POINT('Ctrl Pts',(0.00431605266673542,-0.0329451141710254,
0.0698341717572756));
#75156=CARTESIAN_POINT('Ctrl Pts',(0.00415891843234981,-0.0326442513127493,
0.0699837090405706));
#75157=CARTESIAN_POINT('Ctrl Pts',(0.00448203465472889,-0.0332451089994433,
0.0696984349811885));
#75158=CARTESIAN_POINT('Ctrl Pts',(0.00431414113316252,-0.0329451141710254,
0.0698357857367745));
#75159=CARTESIAN_POINT('Ctrl Pts',(0.0041570703997764,-0.0326442513127493,
0.0699853927197585));
#75160=CARTESIAN_POINT('',(0.0044561210579841,-0.0331951640388616,0.0697198321930316));
#75161=CARTESIAN_POINT('',(0.00427720617082845,-0.0328677532354985,0.0698742570265934));
#75162=CARTESIAN_POINT('Origin',(0.0157269311170673,-0.0326402808279943,
0.0821295496793115));
#75163=CARTESIAN_POINT('Origin',(-0.0031174335433749,-0.0326944278779242,
0.0616551520620115));
#75164=CARTESIAN_POINT('',(0.00437104376775591,-0.0326943950436593,0.0697916655347617));
#75165=CARTESIAN_POINT('',(0.00432457927863608,-0.0326943950436693,0.0698334662674197));
#75166=CARTESIAN_POINT('',(0.00455327264731677,-0.0330220786163545,0.0696411657179031));
#75167=CARTESIAN_POINT('Origin',(0.0153912781259877,-0.0326396682765248,
0.0824737730299198));
#75168=CARTESIAN_POINT('',(0.00455411604157358,-0.0331951640388587,0.0696422307549535));
#75169=CARTESIAN_POINT('Origin',(-0.00229446032951578,-0.0331952026560113,
0.0609938568475875));
#75170=CARTESIAN_POINT('',(0.00450511854978884,-0.0331951640388701,0.0696810314740025));
#75171=CARTESIAN_POINT('Ctrl Pts',(0.00458614689441293,-0.0330240426238172,
0.069303853438716));
#75172=CARTESIAN_POINT('Ctrl Pts',(0.00451938650415942,-0.0329142774063519,
0.0693525878115066));
#75173=CARTESIAN_POINT('Ctrl Pts',(0.00445360030703494,-0.0328043479726691,
0.0694027266039119));
#75174=CARTESIAN_POINT('Ctrl Pts',(0.0043888743489824,-0.0326943950436593,
0.0694542079053788));
#75175=CARTESIAN_POINT('Ctrl Pts',(0.00457549577403047,-0.0330240426238172,
0.0694166705013398));
#75176=CARTESIAN_POINT('Ctrl Pts',(0.00451028954872694,-0.0329142774063519,
0.0694655516036906));
#75177=CARTESIAN_POINT('Ctrl Pts',(0.00444606132467023,-0.0328043479726691,
0.0695158050698752));
#75178=CARTESIAN_POINT('Ctrl Pts',(0.00438289515596947,-0.0326943950436593,
0.0695673687874687));
#75179=CARTESIAN_POINT('Ctrl Pts',(0.00456484465364802,-0.0330240426238172,
0.0695294875639636));
#75180=CARTESIAN_POINT('Ctrl Pts',(0.00450119259329447,-0.0329142774063519,
0.0695785153958745));
#75181=CARTESIAN_POINT('Ctrl Pts',(0.00443852234230552,-0.0328043479726691,
0.0696288835358384));
#75182=CARTESIAN_POINT('Ctrl Pts',(0.00437691596295654,-0.0326943950436593,
0.0696805296695587));
#75183=CARTESIAN_POINT('Ctrl Pts',(0.00455419353326556,-0.0330240426238172,
0.0696423046265874));
#75184=CARTESIAN_POINT('Ctrl Pts',(0.00449209563786199,-0.0329142774063519,
0.0696914791880584));
#75185=CARTESIAN_POINT('Ctrl Pts',(0.00443098335994081,-0.0328043479726691,
0.0697419620018017));
#75186=CARTESIAN_POINT('Ctrl Pts',(0.0043709367699436,-0.0326943950436593,
0.0697936905516486));
#75187=CARTESIAN_POINT('',(0.00437995905837915,-0.0326943950436693,0.0696229367200802));
#75188=CARTESIAN_POINT('Ctrl Pts',(0.00439891316853094,-0.0327114338383331,
0.069446240791706));
#75189=CARTESIAN_POINT('Ctrl Pts',(0.00442557471761049,-0.0327619876830991,
0.0694799089572611));
#75190=CARTESIAN_POINT('Ctrl Pts',(0.00445176590032874,-0.0328131562604373,
0.0695129831448564));
#75191=CARTESIAN_POINT('Ctrl Pts',(0.00450322957263624,-0.0329167375858768,
0.0695779713956947));
#75192=CARTESIAN_POINT('Ctrl Pts',(0.00452848155645018,-0.0329691088920615,
0.0696098595642743));
#75193=CARTESIAN_POINT('Ctrl Pts',(0.00455327264734411,-0.0330220786163186,
0.0696411657179421));
#75194=CARTESIAN_POINT('Ctrl Pts',(0.00445813557159303,-0.0331951640388604,
0.0697200661560827));
#75195=CARTESIAN_POINT('Ctrl Pts',(0.00436654952957937,-0.0330306422010619,
0.0697958510497885));
#75196=CARTESIAN_POINT('Ctrl Pts',(0.00427817401655101,-0.0328657861914645,
0.0698753565332643));
#75197=CARTESIAN_POINT('Ctrl Pts',(0.00445612105798658,-0.0331951640388604,
0.0697198321930296));
#75198=CARTESIAN_POINT('Ctrl Pts',(0.0043645301789368,-0.0330306422010619,
0.0697956587355127));
#75199=CARTESIAN_POINT('Ctrl Pts',(0.0042761515543933,-0.0328657861914645,
0.0698752060320969));
#75200=CARTESIAN_POINT('Ctrl Pts',(0.00412044891561131,-0.0331951640388604,
0.0696808476565142));
#75201=CARTESIAN_POINT('Ctrl Pts',(0.00402805205626363,-0.0330306422010619,
0.069763614005328));
#75202=CARTESIAN_POINT('Ctrl Pts',(0.00393915496962046,-0.0328657861914645,
0.0698501284902403));
#75203=CARTESIAN_POINT('',(0.00411091185962303,-0.0331781648281887,0.0696894090433693));
#75204=CARTESIAN_POINT('',(0.00412044891561044,-0.0331951640388588,0.069680847656515));
#75205=CARTESIAN_POINT('Origin',(0.015680470248199,-0.0326412091686146,
0.0814848236176645));
#75206=CARTESIAN_POINT('Ctrl Pts',(0.00411091186144395,-0.033178164828644,
0.0696894090431472));
#75207=CARTESIAN_POINT('Ctrl Pts',(0.00413965940689649,-0.033127681154678,
0.0697213639676716));
#75208=CARTESIAN_POINT('Ctrl Pts',(0.00416788788584545,-0.0330765663497789,
0.0697527418626016));
#75209=CARTESIAN_POINT('Ctrl Pts',(0.00422333084341036,-0.0329730614463125,
0.0698143706608437));
#75210=CARTESIAN_POINT('Ctrl Pts',(0.00425052292029112,-0.032920713337378,
0.0698445966710455));
#75211=CARTESIAN_POINT('Ctrl Pts',(0.00427720617539217,-0.0328677532289346,
0.0698742570107675));
#75212=CARTESIAN_POINT('',(0.00428828498680727,-0.0331951640388702,0.0697003399247833));
#75213=CARTESIAN_POINT('Origin',(0.00812378219310841,-0.0315241814719618,
0.07415));
#75214=CARTESIAN_POINT('',(0.00411091186017873,-0.0332121607144234,0.0696894090449544));
#75215=CARTESIAN_POINT('',(0.00410139311123134,-0.0331951640388587,0.0696979907823525));
#75216=CARTESIAN_POINT('Origin',(0.0157084293955862,-0.0326413649983711,
0.0814491230060563));
#75217=CARTESIAN_POINT('Origin',(0.0146214296216661,-0.0326412100335714,
0.0824375687480616));
#75218=CARTESIAN_POINT('Origin',(0.0145829785968182,-0.0326413660078431,
0.0824616066048647));
#75219=CARTESIAN_POINT('Ctrl Pts',(0.00439849357327689,-0.0337436976235975,
0.0697681796363892));
#75220=CARTESIAN_POINT('Ctrl Pts',(0.00435908281684353,-0.0336723290703325,
0.0698016854468189));
#75221=CARTESIAN_POINT('Ctrl Pts',(0.00432028110006349,-0.033601104548885,
0.0698358947120861));
#75222=CARTESIAN_POINT('Ctrl Pts',(0.00419639490457184,-0.0333736987606857,
0.0699451181196106));
#75223=CARTESIAN_POINT('Ctrl Pts',(0.00407898073262994,-0.0331450831799191,
0.0700612708398194));
#75224=CARTESIAN_POINT('Ctrl Pts',(0.00421158904034702,-0.0337436976235975,
0.0699342118488369));
#75225=CARTESIAN_POINT('Ctrl Pts',(0.00417367160279528,-0.0336723290703325,
0.069969398706962));
#75226=CARTESIAN_POINT('Ctrl Pts',(0.00413639320006255,-0.033601104548885,
0.0700052618878707));
#75227=CARTESIAN_POINT('Ctrl Pts',(0.00401737064457243,-0.0333736987606857,
0.0701197659204165));
#75228=CARTESIAN_POINT('Ctrl Pts',(0.00390511513044965,-0.0331450831799191,
0.0702409114598875));
#75229=CARTESIAN_POINT('Ctrl Pts',(0.00420971999501772,-0.0337436976235975,
0.0699358721709613));
#75230=CARTESIAN_POINT('Ctrl Pts',(0.0041718174906548,-0.0336723290703325,
0.0699710758395633));
#75231=CARTESIAN_POINT('Ctrl Pts',(0.00413455432106253,-0.033601104548885,
0.0700069555596285));
#75232=CARTESIAN_POINT('Ctrl Pts',(0.00401558040197243,-0.0333736987606857,
0.0701215123984247));
#75233=CARTESIAN_POINT('Ctrl Pts',(0.00390337647442785,-0.0331450831799191,
0.0702427078660882));
#75234=CARTESIAN_POINT('',(0.00418518581122499,-0.0336938721132548,0.0699588684653646));
#75235=CARTESIAN_POINT('',(0.00401632039107351,-0.0333679870047996,0.0701242227403068));
#75236=CARTESIAN_POINT('Ctrl Pts',(0.00418518581124073,-0.0336938721132494,
0.0699588684653497));
#75237=CARTESIAN_POINT('Ctrl Pts',(0.00416882585876012,-0.0336629187933839,
0.0699742426546625));
#75238=CARTESIAN_POINT('Ctrl Pts',(0.00415256116064488,-0.0336319952300977,
0.0699897077210402));
#75239=CARTESIAN_POINT('Ctrl Pts',(0.00413639320006895,-0.0336011045488887,
0.0700052618878647));
#75240=CARTESIAN_POINT('Ctrl Pts',(0.00409582225461918,-0.0335235892595388,
0.0700442926147639));
#75241=CARTESIAN_POINT('Ctrl Pts',(0.00405578845983254,-0.0334458668665506,
0.0700839538495439));
#75242=CARTESIAN_POINT('Ctrl Pts',(0.00401632039915872,-0.033367986996243,
0.0701242227316827));
#75243=CARTESIAN_POINT('Ctrl Pts',(0.00401628877738654,-0.033367969247041,
0.0701242540130376));
#75244=CARTESIAN_POINT('Ctrl Pts',(0.00401661659916247,-0.0333391895417412,
0.0701245670156927));
#75245=CARTESIAN_POINT('Ctrl Pts',(0.00401686455999755,-0.0333104081134104,
0.0701247992779087));
#75246=CARTESIAN_POINT('Ctrl Pts',(0.00401719656448682,-0.0332532698872406,
0.0701251026742335));
#75247=CARTESIAN_POINT('Ctrl Pts',(0.00401728300028147,-0.0332249174314659,
0.070125176161426));
#75248=CARTESIAN_POINT('Ctrl Pts',(0.00401729045242689,-0.033196098524122,
0.070125173801778));
#75249=CARTESIAN_POINT('Ctrl Pts',(0.00401729055187332,-0.0331956312684894,
0.0701251737428223));
#75250=CARTESIAN_POINT('Ctrl Pts',(0.00401729062974416,-0.0331951640388587,
0.0701251736633715));
#75251=CARTESIAN_POINT('',(0.00410478685445198,-0.0331951640388587,0.0700359021076475));
#75252=CARTESIAN_POINT('',(0.00406103874210729,-0.0331951640388687,0.0700805378855203));
#75253=CARTESIAN_POINT('',(0.00427720618565027,-0.0335216366567749,0.0698742570219735));
#75254=CARTESIAN_POINT('Origin',(0.0162866816396492,-0.0326434571525472,
0.081413024908701));
#75255=CARTESIAN_POINT('',(0.00427811478949624,-0.0336938721132326,0.0698752670000577));
#75256=CARTESIAN_POINT('Origin',(-0.00302568927549291,-0.0336938867896202,
0.0617565678363322));
#75257=CARTESIAN_POINT('',(0.00423165030037061,-0.0336938721132537,0.0699170677327212));
#75258=CARTESIAN_POINT('Ctrl Pts',(0.00428883481014811,-0.0335235895815172,
0.069535546774541));
#75259=CARTESIAN_POINT('Ctrl Pts',(0.00422530777647728,-0.0334144449262749,
0.069588342375584));
#75260=CARTESIAN_POINT('Ctrl Pts',(0.00416279847532571,-0.0333049234473147,
0.0696425110530825));
#75261=CARTESIAN_POINT('Ctrl Pts',(0.00410139311123132,-0.0331951640388587,
0.0696979907823524));
#75262=CARTESIAN_POINT('Ctrl Pts',(0.00428528856239471,-0.0335235895815172,
0.0696488101693902));
#75263=CARTESIAN_POINT('Ctrl Pts',(0.00422332082234909,-0.0334144449262749,
0.0697016545915155));
#75264=CARTESIAN_POINT('Ctrl Pts',(0.004162373614869,-0.0333049234473147,
0.0697558399323529));
#75265=CARTESIAN_POINT('Ctrl Pts',(0.00410253114898426,-0.0331951640388587,
0.0698113039649746));
#75266=CARTESIAN_POINT('Ctrl Pts',(0.00428174231464131,-0.0335235895815172,
0.0697620735642394));
#75267=CARTESIAN_POINT('Ctrl Pts',(0.00422133386822089,-0.0334144449262749,
0.069814966807447));
#75268=CARTESIAN_POINT('Ctrl Pts',(0.00416194875441229,-0.0333049234473147,
0.0698691688116234));
#75269=CARTESIAN_POINT('Ctrl Pts',(0.0041036691867372,-0.0331951640388587,
0.0699246171475968));
#75270=CARTESIAN_POINT('Ctrl Pts',(0.00427819606688791,-0.0335235895815172,
0.0698753369590886));
#75271=CARTESIAN_POINT('Ctrl Pts',(0.0042193469140927,-0.0334144449262749,
0.0699282790233785));
#75272=CARTESIAN_POINT('Ctrl Pts',(0.00416152389395558,-0.0333049234473147,
0.0699824976908938));
#75273=CARTESIAN_POINT('Ctrl Pts',(0.00410480722449014,-0.0331951640388587,
0.070037930330219));
#75274=CARTESIAN_POINT('',(0.00410308998285166,-0.0331951640388687,0.06986694644501));
#75275=CARTESIAN_POINT('Ctrl Pts',(0.00411091186226826,-0.0332121607145984,
0.0696894090472775));
#75276=CARTESIAN_POINT('Ctrl Pts',(0.00413961103802514,-0.033262544410982,
0.0697213102235373));
#75277=CARTESIAN_POINT('Ctrl Pts',(0.00416781568194698,-0.0333135300746948,
0.0697526616924685));
#75278=CARTESIAN_POINT('Ctrl Pts',(0.00422325829459368,-0.0334167203140651,
0.0698142901020552));
#75279=CARTESIAN_POINT('Ctrl Pts',(0.00425047478994511,-0.0334688847587358,
0.0698445431735279));
#75280=CARTESIAN_POINT('Ctrl Pts',(0.00427720618599561,-0.0335216366562442,
0.069874257022605));
#75281=CARTESIAN_POINT('Ctrl Pts',(0.00418721056670061,-0.0336938721132493,
0.0699589754493442));
#75282=CARTESIAN_POINT('Ctrl Pts',(0.00416267910927351,-0.0336474569765009,
0.0699820175093691));
#75283=CARTESIAN_POINT('Ctrl Pts',(0.00413841906916301,-0.033601104548885,
0.0700053451622198));
#75284=CARTESIAN_POINT('Ctrl Pts',(0.00407699822534293,-0.0334837508592656,
0.0700644054158677));
#75285=CARTESIAN_POINT('Ctrl Pts',(0.00401735443079853,-0.0333660264659097,
0.0701252597615537));
#75286=CARTESIAN_POINT('Ctrl Pts',(0.00418518581124541,-0.0336938721132493,
0.0699588684653455));
#75287=CARTESIAN_POINT('Ctrl Pts',(0.00416065372760546,-0.0336474569765009,
0.0699819223769358));
#75288=CARTESIAN_POINT('Ctrl Pts',(0.00413639320006256,-0.033601104548885,
0.0700052618878707));
#75289=CARTESIAN_POINT('Ctrl Pts',(0.00407497112217571,-0.0334837508592656,
0.0700643521634612));
#75290=CARTESIAN_POINT('Ctrl Pts',(0.00401532698371886,-0.0333660264659097,
0.0701252365544743));
#75291=CARTESIAN_POINT('Ctrl Pts',(0.00384570343603074,-0.0336938721132493,
0.0699409309006279));
#75292=CARTESIAN_POINT('Ctrl Pts',(0.00382106635787218,-0.0336474569765009,
0.0699659719152129));
#75293=CARTESIAN_POINT('Ctrl Pts',(0.00379672410455441,-0.033601104548885,
0.0699912996220781));
#75294=CARTESIAN_POINT('Ctrl Pts',(0.00373509511579557,-0.0334837508592656,
0.0700554235526489));
#75295=CARTESIAN_POINT('Ctrl Pts',(0.00367539331496028,-0.0333660264659097,
0.0701213455194301));
#75296=CARTESIAN_POINT('',(0.003838747518292,-0.0336769361243754,0.0699501812139545));
#75297=CARTESIAN_POINT('',(0.00384772818185602,-0.0336938721132328,0.0699410378841272));
#75298=CARTESIAN_POINT('Ctrl Pts',(0.00383874751829182,-0.033676936124375,
0.0699501812139546));
#75299=CARTESIAN_POINT('Ctrl Pts',(0.00384024277999362,-0.0336797586670049,
0.0699486556128355));
#75300=CARTESIAN_POINT('Ctrl Pts',(0.00384173879988311,-0.0336825812712892,
0.0699471308679525));
#75301=CARTESIAN_POINT('Ctrl Pts',(0.00384473235897705,-0.033688226609326,
0.0699440830869327));
#75302=CARTESIAN_POINT('Ctrl Pts',(0.00384622989819641,-0.033691049343075,
0.0699425600508077));
#75303=CARTESIAN_POINT('Ctrl Pts',(0.00384772818186329,-0.03369387211323,
0.0699410378841292));
#75304=CARTESIAN_POINT('Ctrl Pts',(0.003838747518292,-0.0336769361243754,
0.0699501812139545));
#75305=CARTESIAN_POINT('Ctrl Pts',(0.00386867971389577,-0.0336279031321641,
0.0699795181521461));
#75306=CARTESIAN_POINT('Ctrl Pts',(0.00389904255917442,-0.0335767851940115,
0.0700092771757418));
#75307=CARTESIAN_POINT('Ctrl Pts',(0.00395853781724498,-0.0334733198899499,
0.0700675892598876));
#75308=CARTESIAN_POINT('Ctrl Pts',(0.00398771017746988,-0.0334209645035421,
0.0700961814734416));
#75309=CARTESIAN_POINT('Ctrl Pts',(0.00401632040136205,-0.0333679869844681,
0.0701242227297893));
#75310=CARTESIAN_POINT('',(0.0040164569965505,-0.0336938721132538,0.0699499531747559));
#75311=CARTESIAN_POINT('Origin',(0.00812378219310841,-0.0315241814719618,
0.07415));
#75312=CARTESIAN_POINT('',(0.00383874751922387,-0.0337108120655845,0.0699501812148682));
#75313=CARTESIAN_POINT('',(0.00382978640553166,-0.0336938721132327,0.0699593437057788));
#75314=CARTESIAN_POINT('Origin',(0.0147411860276537,-0.0345562514810309,
0.0822006996781526));
#75315=CARTESIAN_POINT('Ctrl Pts',(0.00382978640553377,-0.0336938721132299,
0.0699593437057861));
#75316=CARTESIAN_POINT('Ctrl Pts',(0.00383127817504152,-0.0336910493388199,
0.0699578151499866));
#75317=CARTESIAN_POINT('Ctrl Pts',(0.00383277082540093,-0.0336882266071981,
0.0699562873244816));
#75318=CARTESIAN_POINT('Ctrl Pts',(0.00383575786619216,-0.033682581271266,
0.0699532331570176));
#75319=CARTESIAN_POINT('Ctrl Pts',(0.00383725225659651,-0.0336797586669932,
0.0699517068150672));
#75320=CARTESIAN_POINT('Ctrl Pts',(0.00383874751829216,-0.0336769361243751,
0.0699501812139543));
#75321=CARTESIAN_POINT('Origin',(0.0163057639141442,-0.0345562517080938,
0.0806043721342636));
#75322=CARTESIAN_POINT('Ctrl Pts',(0.00413074496612322,-0.034243627687391,
0.0700107031147898));
#75323=CARTESIAN_POINT('Ctrl Pts',(0.00397462881049004,-0.0339430054201809,
0.0701613029964762));
#75324=CARTESIAN_POINT('Ctrl Pts',(0.00383029996464101,-0.0336441434784052,
0.0703232343481949));
#75325=CARTESIAN_POINT('Ctrl Pts',(0.00395463290236064,-0.034243627687391,
0.0701881419521319));
#75326=CARTESIAN_POINT('Ctrl Pts',(0.00380520896280041,-0.0339430054201809,
0.0703453840098006));
#75327=CARTESIAN_POINT('Ctrl Pts',(0.0036680536370505,-0.0336441434784052,
0.0705134345826412));
#75328=CARTESIAN_POINT('Ctrl Pts',(0.00395287178172302,-0.034243627687391,
0.0701899163405053));
#75329=CARTESIAN_POINT('Ctrl Pts',(0.00380351476432351,-0.0339430054201809,
0.0703472248199339));
#75330=CARTESIAN_POINT('Ctrl Pts',(0.00366643117377459,-0.0336441434784052,
0.0705153365849856));
#75331=CARTESIAN_POINT('',(0.00392979440503335,-0.0341934961088741,0.0702144452190983));
#75332=CARTESIAN_POINT('',(0.00377164489123366,-0.0338664212864733,0.070390076342541));
#75333=CARTESIAN_POINT('Origin',(0.0157787116534421,-0.0345610720404402,
0.0820320720457151));
#75334=CARTESIAN_POINT('Origin',(-0.0045267054850951,-0.0336938005073093,
0.0632209686267812));
#75335=CARTESIAN_POINT('',(0.00385439107964538,-0.0336938721132327,0.070296375145362));
#75336=CARTESIAN_POINT('',(0.00381353199788871,-0.0336938721132427,0.0703436698114264));
#75337=CARTESIAN_POINT('',(0.00401632040136582,-0.0340203938281605,0.0701242227297855));
#75338=CARTESIAN_POINT('Origin',(0.015390453490231,-0.0345589643244941,
0.0823163119673952));
#75339=CARTESIAN_POINT('',(0.00401729062974263,-0.0341934961088739,0.070125173663373));
#75340=CARTESIAN_POINT('Origin',(-0.0038524944108664,-0.0341934220717632,
0.0624118928000223));
#75341=CARTESIAN_POINT('',(0.003973542517398,-0.034193496108884,0.0701698094412456));
#75342=CARTESIAN_POINT('Ctrl Pts',(0.00400666027782073,-0.0340223579322397,
0.0697854488048955));
#75343=CARTESIAN_POINT('Ctrl Pts',(0.00394646173361285,-0.0339125849573575,
0.0698422346540121));
#75344=CARTESIAN_POINT('Ctrl Pts',(0.00388748082534962,-0.0338030433565231,
0.069900226570353));
#75345=CARTESIAN_POINT('Ctrl Pts',(0.00382978640553159,-0.0336938721132327,
0.0699593437057781));
#75346=CARTESIAN_POINT('Ctrl Pts',(0.00401023284455326,-0.0340223579322397,
0.0698987114050655));
#75347=CARTESIAN_POINT('Ctrl Pts',(0.00395159648700299,-0.0339125849573575,
0.0699554479791692));
#75348=CARTESIAN_POINT('Ctrl Pts',(0.00389417564778862,-0.0338030433565231,
0.0700133583214883));
#75349=CARTESIAN_POINT('Ctrl Pts',(0.00383803719359283,-0.0336938721132327,
0.0700723618650565));
#75350=CARTESIAN_POINT('Ctrl Pts',(0.00401380541128579,-0.0340223579322397,
0.0700119740052354));
#75351=CARTESIAN_POINT('Ctrl Pts',(0.00395673124039312,-0.0339125849573575,
0.0700686613043262));
#75352=CARTESIAN_POINT('Ctrl Pts',(0.00390087047022762,-0.0338030433565231,
0.0701264900726237));
#75353=CARTESIAN_POINT('Ctrl Pts',(0.00384628798165408,-0.0336938721132327,
0.0701853800243348));
#75354=CARTESIAN_POINT('Ctrl Pts',(0.00401737797801833,-0.0340223579322397,
0.0701252366054053));
#75355=CARTESIAN_POINT('Ctrl Pts',(0.00396186599378326,-0.0339125849573575,
0.0701818746294833));
#75356=CARTESIAN_POINT('Ctrl Pts',(0.00390756529266662,-0.0338030433565231,
0.070239621823759));
#75357=CARTESIAN_POINT('Ctrl Pts',(0.00385453876971533,-0.0336938721132327,
0.0702983981836132));
#75358=CARTESIAN_POINT('',(0.00384208874259852,-0.0336938721132427,0.0701278594255804));
#75359=CARTESIAN_POINT('Ctrl Pts',(0.00383874752179171,-0.0337108120662692,
0.0699501812173845));
#75360=CARTESIAN_POINT('Ctrl Pts',(0.0038694564057343,-0.0337611408994321,
0.069980279398022));
#75361=CARTESIAN_POINT('Ctrl Pts',(0.00389960492067525,-0.0338121088781361,
0.0700098283536383));
#75362=CARTESIAN_POINT('Ctrl Pts',(0.00395880867736566,-0.0339153382773237,
0.0700678547334513));
#75363=CARTESIAN_POINT('Ctrl Pts',(0.0039878388723051,-0.0339675558473117,
0.0700963076089405));
#75364=CARTESIAN_POINT('Ctrl Pts',(0.0040163204013906,-0.0340203938281304,
0.0701242227298172));
#75365=CARTESIAN_POINT('Ctrl Pts',(0.00393182245015566,-0.0341934961088741,
0.0702144248508423));
#75366=CARTESIAN_POINT('Ctrl Pts',(0.00385045753443956,-0.0340287516182428,
0.0703010903160523));
#75367=CARTESIAN_POINT('Ctrl Pts',(0.00377274409291432,-0.0338644633275951,
0.0703910446009745));
#75368=CARTESIAN_POINT('Ctrl Pts',(0.00392979440503345,-0.0341934961088741,
0.0702144452190984));
#75369=CARTESIAN_POINT('Ctrl Pts',(0.003848429910415,-0.0340287516182428,
0.0703011526125435));
#75370=CARTESIAN_POINT('Ctrl Pts',(0.00377071862255335,-0.0338644633275951,
0.0703911487724697));
#75371=CARTESIAN_POINT('Ctrl Pts',(0.00359188307974076,-0.0341934961088741,
0.0702178389623189));
#75372=CARTESIAN_POINT('Ctrl Pts',(0.00351058874808976,-0.0340287516182428,
0.0703115324062039));
#75373=CARTESIAN_POINT('Ctrl Pts',(0.00343323630200735,-0.0338644633275951,
0.0704085057472349));
#75374=CARTESIAN_POINT('',(0.00358349425304188,-0.0341764758832377,0.0702275281502832));
#75375=CARTESIAN_POINT('',(0.00359188307974075,-0.034193496108874,0.0702178389623189));
#75376=CARTESIAN_POINT('Origin',(0.0157782040706306,-0.0345621026475542,
0.0814395923005888));
#75377=CARTESIAN_POINT('Ctrl Pts',(0.00358349425473896,-0.0341764758837459,
0.0702275281496326));
#75378=CARTESIAN_POINT('Ctrl Pts',(0.00361597576944247,-0.0341260050040449,
0.0702555897497597));
#75379=CARTESIAN_POINT('Ctrl Pts',(0.00364789270377078,-0.0340749269148221,
0.070283163544164));
#75380=CARTESIAN_POINT('Ctrl Pts',(0.00371062202772195,-0.0339715436306273,
0.0703373570303035));
#75381=CARTESIAN_POINT('Ctrl Pts',(0.00374141061532904,-0.0339192778237161,
0.0703639561667697));
#75382=CARTESIAN_POINT('Ctrl Pts',(0.00377164489147254,-0.0338664212855619,
0.0703900763404203));
#75383=CARTESIAN_POINT('',(0.00376083874239706,-0.0341934961088841,0.0702161420907186));
#75384=CARTESIAN_POINT('Origin',(0.00812378219310841,-0.0315241814719618,
0.07415));
#75385=CARTESIAN_POINT('',(0.0035834942530485,-0.0342105180190376,0.0702275281514014));
#75386=CARTESIAN_POINT('',(0.00357512613946545,-0.0341934961088739,0.0702372352350696));
#75387=CARTESIAN_POINT('Origin',(0.0158115988130717,-0.0345621706866152,
0.0814089435689751));
#75388=CARTESIAN_POINT('Origin',(0.0164477712777528,-0.0345621037838267,
0.0806645670300262));
#75389=CARTESIAN_POINT('Origin',(0.0164222936593224,-0.034562171692472,
0.0807020557971328));
#75390=CARTESIAN_POINT('Ctrl Pts',(0.00385537170408677,-0.0346945769586966,
0.0702952400658775));
#75391=CARTESIAN_POINT('Ctrl Pts',(0.00377463221390489,-0.0345275153362944,
0.0703846436325484));
#75392=CARTESIAN_POINT('Ctrl Pts',(0.00369668350023679,-0.0343603235965185,
0.0704766095062116));
#75393=CARTESIAN_POINT('Ctrl Pts',(0.00362175205823326,-0.0341934961088739,
0.070570862266246));
#75394=CARTESIAN_POINT('Ctrl Pts',(0.00380056605345085,-0.0346945769586966,
0.070358677980599));
#75395=CARTESIAN_POINT('Ctrl Pts',(0.00372115529579197,-0.0345275153362944,
0.0704492294735654));
#75396=CARTESIAN_POINT('Ctrl Pts',(0.00364457175955056,-0.0343603235965185,
0.0705423017830219));
#75397=CARTESIAN_POINT('Ctrl Pts',(0.00357103785365299,-0.0341934961088739,
0.0706376162760104));
#75398=CARTESIAN_POINT('Ctrl Pts',(0.00374576040281499,-0.0346945769586966,
0.0704221158953208));
#75399=CARTESIAN_POINT('Ctrl Pts',(0.00366767837767903,-0.0345275153362944,
0.0705138153145834));
#75400=CARTESIAN_POINT('Ctrl Pts',(0.00359246001886427,-0.0343603235965185,
0.0706079940598334));
#75401=CARTESIAN_POINT('Ctrl Pts',(0.00352032364907269,-0.0341934961088739,
0.0707043702857762));
#75402=CARTESIAN_POINT('Ctrl Pts',(0.00369095475217901,-0.0346945769586966,
0.0704855538100419));
#75403=CARTESIAN_POINT('Ctrl Pts',(0.00361420145956612,-0.0345275153362944,
0.0705784011555995));
#75404=CARTESIAN_POINT('Ctrl Pts',(0.00354034827817808,-0.0343603235965185,
0.0706736863366425));
#75405=CARTESIAN_POINT('Ctrl Pts',(0.00346960944449247,-0.0341934961088739,
0.0707711242955393));
#75406=CARTESIAN_POINT('',(0.0036909547525752,-0.0346945769586966,0.0704855538095837));
#75407=CARTESIAN_POINT('',(0.00354414528140131,-0.0343667727831428,0.070670768654258));
#75408=CARTESIAN_POINT('Origin',(0.016765754229002,-0.0345626457063744,
0.0810565928262449));
#75409=CARTESIAN_POINT('Origin',(-0.00525638033940051,-0.034193477102889,
0.0639848578490789));
#75410=CARTESIAN_POINT('',(0.00362084464106437,-0.034193496108874,0.0705720566798239));
#75411=CARTESIAN_POINT('',(0.00358303584202472,-0.0341934961088839,0.0706218235836399));
#75412=CARTESIAN_POINT('',(0.00377164489265938,-0.0345211942962721,0.0703900763414942));
#75413=CARTESIAN_POINT('Origin',(0.0164489103351654,-0.0345625596120514,
0.08141825667154));
#75414=CARTESIAN_POINT('',(0.00377267291611208,-0.0346945769586885,0.0703909644774707));
#75415=CARTESIAN_POINT('Origin',(-0.00459928980844164,-0.0346945685853842,
0.0631582087556491));
#75416=CARTESIAN_POINT('',(0.00373181383435364,-0.0346945769587026,0.0704382591435372));
#75417=CARTESIAN_POINT('Ctrl Pts',(0.00374073138332709,-0.0345231616327842,
0.0700525781765969));
#75418=CARTESIAN_POINT('Ctrl Pts',(0.00368425419219998,-0.0344132092796988,
0.0701129923611679));
#75419=CARTESIAN_POINT('Ctrl Pts',(0.00362902953479011,-0.0343032738558979,
0.0701745716147944));
#75420=CARTESIAN_POINT('Ctrl Pts',(0.00357512613946539,-0.0341934961088739,
0.0702372352350696));
#75421=CARTESIAN_POINT('Ctrl Pts',(0.0037514087178497,-0.0345231616327842,
0.0701653927619394));
#75422=CARTESIAN_POINT('Ctrl Pts',(0.0036964865169513,-0.0344132092796988,
0.0702256597744864));
#75423=CARTESIAN_POINT('Ctrl Pts',(0.00364281372540257,-0.0343032738558979,
0.0702870596999361));
#75424=CARTESIAN_POINT('Ctrl Pts',(0.00359045708933678,-0.0341934961088739,
0.070349512116548));
#75425=CARTESIAN_POINT('Ctrl Pts',(0.00376208605237231,-0.0345231616327842,
0.0702782073472817));
#75426=CARTESIAN_POINT('Ctrl Pts',(0.00370871884170262,-0.0344132092796988,
0.0703383271878048));
#75427=CARTESIAN_POINT('Ctrl Pts',(0.00365659791601503,-0.0343032738558979,
0.0703995477850777));
#75428=CARTESIAN_POINT('Ctrl Pts',(0.00360578803920817,-0.0341934961088739,
0.0704617889980265));
#75429=CARTESIAN_POINT('Ctrl Pts',(0.00377276338689492,-0.0345231616327842,
0.0703910219326241));
#75430=CARTESIAN_POINT('Ctrl Pts',(0.00372095116645394,-0.0344132092796988,
0.0704509946011233));
#75431=CARTESIAN_POINT('Ctrl Pts',(0.00367038210662749,-0.0343032738558979,
0.0705120358702194));
#75432=CARTESIAN_POINT('Ctrl Pts',(0.00362111898907955,-0.0341934961088739,
0.0705740658795049));
#75433=CARTESIAN_POINT('',(0.00359798539027491,-0.0341934961088839,0.0704046459574568));
#75434=CARTESIAN_POINT('Ctrl Pts',(0.00358349425565724,-0.0342105180195395,
0.0702275281536545));
#75435=CARTESIAN_POINT('Ctrl Pts',(0.00361601227690777,-0.0342610556241267,
0.0702556213108751));
#75436=CARTESIAN_POINT('Ctrl Pts',(0.00364794677908014,-0.0343122189870072,
0.0702832103509149));
#75437=CARTESIAN_POINT('Ctrl Pts',(0.00371067673843757,-0.0344158119695202,
0.070337404380653));
#75438=CARTESIAN_POINT('Ctrl Pts',(0.00374144653860155,-0.0344681990450108,
0.0703639872045892));
#75439=CARTESIAN_POINT('Ctrl Pts',(0.00377164489267596,-0.0345211942962546,
0.0703900763415107));
#75440=CARTESIAN_POINT('Ctrl Pts',(0.00369297702161709,-0.0346945769586932,
0.0704854061756626));
#75441=CARTESIAN_POINT('Ctrl Pts',(0.00361721413728232,-0.034529677707698,
0.0705770099374461));
#75442=CARTESIAN_POINT('Ctrl Pts',(0.00354530205903659,-0.0343648066251421,
0.0706716667745894));
#75443=CARTESIAN_POINT('Ctrl Pts',(0.00369095475258102,-0.0346945769586932,
0.0704855538095767));
#75444=CARTESIAN_POINT('Ctrl Pts',(0.00361519492047297,-0.034529677707698,
0.0705771993803416));
#75445=CARTESIAN_POINT('Ctrl Pts',(0.00354328761984949,-0.0343648066251421,
0.0706718978645897));
#75446=CARTESIAN_POINT('Ctrl Pts',(0.00335392331300024,-0.0346945769586932,
0.0705101584836901));
#75447=CARTESIAN_POINT('Ctrl Pts',(0.00327867216511978,-0.034529677707698,
0.0706087719409925));
#75448=CARTESIAN_POINT('Ctrl Pts',(0.00320756110321309,-0.0343648066251421,
0.0707104113334196));
#75449=CARTESIAN_POINT('',(0.00334615942863117,-0.0346775396664963,0.0705203552909863));
#75450=CARTESIAN_POINT('',(0.00335392331299816,-0.0346945769586886,0.0705101584836928));
#75451=CARTESIAN_POINT('Origin',(0.016657343190845,-0.0345626618351403,
0.0804413072159766));
#75452=CARTESIAN_POINT('Ctrl Pts',(0.00334615943032344,-0.0346775396670097,
0.0705203552903225));
#75453=CARTESIAN_POINT('Ctrl Pts',(0.00338036577141767,-0.0346269749928192,
0.0705463424378536));
#75454=CARTESIAN_POINT('Ctrl Pts',(0.00341396421123299,-0.0345757902890796,
0.070571867707184));
#75455=CARTESIAN_POINT('Ctrl Pts',(0.00347997285435171,-0.0344721681087691,
0.0706220156482585));
#75456=CARTESIAN_POINT('Ctrl Pts',(0.00351235717575486,-0.0344197714289052,
0.0706466186641413));
#75457=CARTESIAN_POINT('Ctrl Pts',(0.00354414528145819,-0.034366772783058,
0.0706707686539969));
#75458=CARTESIAN_POINT('',(0.00352243903279668,-0.0346945769587026,0.0704978561466482));
#75459=CARTESIAN_POINT('Origin',(0.00812378219310841,-0.0315241814719618,
0.07415));
#75460=CARTESIAN_POINT('',(0.00334615942912236,-0.034711613648962,0.0705203552922876));
#75461=CARTESIAN_POINT('',(0.00333841734075968,-0.0346945769586885,0.0705305686593154));
#75462=CARTESIAN_POINT('Origin',(0.0166832442648657,-0.0345626685577737,
0.0804041264557915));
#75463=CARTESIAN_POINT('Origin',(0.0164725764164216,-0.0345626627644068,
0.0806845157712007));
#75464=CARTESIAN_POINT('Origin',(0.0164436967321114,-0.0345626695232125,
0.0807194335678264));
#75465=CARTESIAN_POINT('Ctrl Pts',(0.00364493063813646,-0.0352450361874068,
0.0705418631713652));
#75466=CARTESIAN_POINT('Ctrl Pts',(0.00350884752462439,-0.0349452760959492,
0.070710785829653));
#75467=CARTESIAN_POINT('Ctrl Pts',(0.00338587495471023,-0.034644428984174,
0.0708894789333667));
#75468=CARTESIAN_POINT('Ctrl Pts',(0.00364339057316616,-0.0352450361874068,
0.0705438641273586));
#75469=CARTESIAN_POINT('Ctrl Pts',(0.00350738292694774,-0.0349452760959492,
0.0707128448701498));
#75470=CARTESIAN_POINT('Ctrl Pts',(0.00338448998509506,-0.034644428984174,
0.0708915902088497));
#75471=CARTESIAN_POINT('Ctrl Pts',(0.00349090889293795,-0.0352450361874068,
0.0707419785821436));
#75472=CARTESIAN_POINT('Ctrl Pts',(0.00336237325599172,-0.0349452760959492,
0.0709167102658732));
#75473=CARTESIAN_POINT('Ctrl Pts',(0.00324736428062184,-0.034644428984174,
0.0711006273853824));
#75474=CARTESIAN_POINT('Ctrl Pts',(0.00348938407613567,-0.0352450361874068,
0.0707439597266914));
#75475=CARTESIAN_POINT('Ctrl Pts',(0.00336092315928216,-0.0349452760959492,
0.0709187489198304));
#75476=CARTESIAN_POINT('Ctrl Pts',(0.00324599302357711,-0.034644428984174,
0.0711027177571476));
#75477=CARTESIAN_POINT('',(0.00346962653462896,-0.0351951634053271,0.0707710967150308));
#75478=CARTESIAN_POINT('',(0.00333471940509753,-0.0348678972925434,0.0709651919033495));
#75479=CARTESIAN_POINT('Origin',(0.017515054857925,-0.0345636767888727,
0.0798886862858971));
#75480=CARTESIAN_POINT('Origin',(-0.00586630416223851,-0.0346946199341124,
0.0648463558596404));
#75481=CARTESIAN_POINT('',(0.0034050692502411,-0.0346945769330288,0.0708618587073022));
#75482=CARTESIAN_POINT('',(0.00337045994285098,-0.0346945769458128,0.070913901448675));
#75483=CARTESIAN_POINT('',(0.00354414528155627,-0.0350221583435276,0.0706707686540918));
#75484=CARTESIAN_POINT('Origin',(0.0172843629381708,-0.0345628458716402,
0.0803104974173432));
#75485=CARTESIAN_POINT('',(0.00354513200593994,-0.035195136029876,0.0706715144876764));
#75486=CARTESIAN_POINT('Origin',(-0.00522895466634155,-0.0351951838366816,
0.0640056876872522));
#75487=CARTESIAN_POINT('',(0.00346960944477295,-0.035195137132875,0.070771124294978));
#75488=CARTESIAN_POINT('Ctrl Pts',(0.00349210047715177,-0.0350241211494343,
0.0703358782816882));
#75489=CARTESIAN_POINT('Ctrl Pts',(0.00343956251433281,-0.0349144232818962,
0.070399677798262));
#75490=CARTESIAN_POINT('Ctrl Pts',(0.00338831188660698,-0.0348045283579412,
0.0704646014991549));
#75491=CARTESIAN_POINT('Ctrl Pts',(0.00333841733405596,-0.0346945769439157,
0.0705305686681786));
#75492=CARTESIAN_POINT('Ctrl Pts',(0.00350984045065131,-0.0350241211494343,
0.0704477998396794));
#75493=CARTESIAN_POINT('Ctrl Pts',(0.00345884416140406,-0.0349144232818962,
0.0705113549953919));
#75494=CARTESIAN_POINT('Ctrl Pts',(0.00340913107890226,-0.0348045283579412,
0.0705760023216674));
#75495=CARTESIAN_POINT('Ctrl Pts',(0.00336076796065435,-0.0346945769439157,
0.0706416613830324));
#75496=CARTESIAN_POINT('Ctrl Pts',(0.00352758042415085,-0.0350241211494343,
0.0705597213976706));
#75497=CARTESIAN_POINT('Ctrl Pts',(0.0034781258084753,-0.0349144232818962,
0.0706230321925219));
#75498=CARTESIAN_POINT('Ctrl Pts',(0.00342995027119753,-0.0348045283579412,
0.0706874031441799));
#75499=CARTESIAN_POINT('Ctrl Pts',(0.00338311858725274,-0.0346945769439157,
0.0707527540978863));
#75500=CARTESIAN_POINT('Ctrl Pts',(0.00354532039765039,-0.0350241211494343,
0.0706716429556618));
#75501=CARTESIAN_POINT('Ctrl Pts',(0.00349740745554654,-0.0349144232818962,
0.0707347093896518));
#75502=CARTESIAN_POINT('Ctrl Pts',(0.00345076946349281,-0.0348045283579412,
0.0707988039666924));
#75503=CARTESIAN_POINT('Ctrl Pts',(0.00340546921385113,-0.0346945769439157,
0.0708638468127401));
#75504=CARTESIAN_POINT('',(0.0033717432956044,-0.0346945769458128,0.0706962136830263));
#75505=CARTESIAN_POINT('Ctrl Pts',(0.00334615943173523,-0.0347116136492799,
0.0705203552942714));
#75506=CARTESIAN_POINT('Ctrl Pts',(0.00338035218094575,-0.0347621546532253,
0.0705463321319886));
#75507=CARTESIAN_POINT('Ctrl Pts',(0.00341394372922662,-0.0348133084096931,
0.0705718522267019));
#75508=CARTESIAN_POINT('Ctrl Pts',(0.00347995245837948,-0.0349168561544571,
0.0706220002283899));
#75509=CARTESIAN_POINT('Ctrl Pts',(0.00351234345693012,-0.0349692089015923,
0.0706466082441908));
#75510=CARTESIAN_POINT('Ctrl Pts',(0.00354414528157333,-0.0350221583435,
0.0706707686541298));
#75511=CARTESIAN_POINT('Ctrl Pts',(0.00347105901116135,-0.0351951371254883,
0.0707709263626847));
#75512=CARTESIAN_POINT('Ctrl Pts',(0.00340119878381317,-0.0350307338980928,
0.0708671184952531));
#75513=CARTESIAN_POINT('Ctrl Pts',(0.00333537397625194,-0.034865930689783,
0.0709661158307866));
#75514=CARTESIAN_POINT('Ctrl Pts',(0.0034696094448677,-0.0351951371254883,
0.0707711242950452));
#75515=CARTESIAN_POINT('Ctrl Pts',(0.00339975330964688,-0.0350307338980928,
0.0708673463964872));
#75516=CARTESIAN_POINT('Ctrl Pts',(0.0033339338293622,-0.034865930689783,
0.0709663735061541));
#75517=CARTESIAN_POINT('Ctrl Pts',(0.00322666062325334,-0.0351951371254883,
0.0708042979649621));
#75518=CARTESIAN_POINT('Ctrl Pts',(0.00315749033284418,-0.0350307338980928,
0.0709055428808597));
#75519=CARTESIAN_POINT('Ctrl Pts',(0.003092563709662,-0.034865930689783,
0.0710095601663106));
#75520=CARTESIAN_POINT('Origin',(-0.0010936440991894,-0.0308609197384602,
0.068020254962796));
#75521=CARTESIAN_POINT('',(0.00336368923641043,-0.0351951371254883,0.0707855872671623));
#75522=CARTESIAN_POINT('Origin',(0.00900721682260279,-0.0351840467441148,
0.0745674792273879));
#75523=CARTESIAN_POINT('Origin',(-0.00225761982641391,-0.0352322614444702,
0.0682005758416904));
#75524=CARTESIAN_POINT('',(0.00320777621092359,-0.0351951142564653,0.0711649204756739));
#75525=CARTESIAN_POINT('',(0.00314536997854559,-0.0351951372916787,0.071272863954921));
#75526=CARTESIAN_POINT('Origin',(0.00813327152284308,-0.0352875127175844,
0.0744904946253621));
#75527=CARTESIAN_POINT('Origin',(0.01305241611569,-0.0298325076522079,0.0684928136022584));
#75528=CARTESIAN_POINT('Origin',(0.00297934781069869,-0.0338732790727179,
0.067533109811178));
#75529=CARTESIAN_POINT('Ctrl Pts',(0.00590155454277438,-0.0321934096636941,
0.0688453001955434));
#75530=CARTESIAN_POINT('Ctrl Pts',(0.00580660294236103,-0.0320508460843585,
0.0688850770122644));
#75531=CARTESIAN_POINT('Ctrl Pts',(0.00571279166034753,-0.0319086045661596,
0.068927374999284));
#75532=CARTESIAN_POINT('Ctrl Pts',(0.00562031519106785,-0.0317669892865695,
0.0689720864523457));
#75533=CARTESIAN_POINT('Ctrl Pts',(0.00582494125586505,-0.0321934096636941,
0.0688793712521285));
#75534=CARTESIAN_POINT('Ctrl Pts',(0.00573059951114002,-0.0320508460843585,
0.0689205194102022));
#75535=CARTESIAN_POINT('Ctrl Pts',(0.00563743447021791,-0.0319086045661596,
0.0689641713189593));
#75536=CARTESIAN_POINT('Ctrl Pts',(0.00554563899596201,-0.0317669892865695,
0.0690102164734667));
#75537=CARTESIAN_POINT('Ctrl Pts',(0.00574832796895574,-0.0321934096636941,
0.0689134423087136));
#75538=CARTESIAN_POINT('Ctrl Pts',(0.00565459607991902,-0.0320508460843585,
0.0689559618081398));
#75539=CARTESIAN_POINT('Ctrl Pts',(0.00556207728008829,-0.0319086045661596,
0.0690009676386347));
#75540=CARTESIAN_POINT('Ctrl Pts',(0.00547096280085618,-0.0317669892865695,
0.0690483464945876));
#75541=CARTESIAN_POINT('Ctrl Pts',(0.00567171468204641,-0.0321934096636941,
0.0689475133652987));
#75542=CARTESIAN_POINT('Ctrl Pts',(0.00557859264869801,-0.0320508460843585,
0.0689914042060775));
#75543=CARTESIAN_POINT('Ctrl Pts',(0.00548672008995868,-0.0319086045661596,
0.0690377639583101));
#75544=CARTESIAN_POINT('Ctrl Pts',(0.00539628660575034,-0.0317669892865695,
0.0690864765157086));
#75545=CARTESIAN_POINT('',(0.00567308530888974,-0.0321934096636941,0.0689469038273657));
#75546=CARTESIAN_POINT('',(0.00546138748314337,-0.0318665617511259,0.069051982797464));
#75547=CARTESIAN_POINT('Origin',(0.0122321207203587,-0.0326371944422025,
0.0843156044656728));
#75548=CARTESIAN_POINT('Origin',(0.000387281604560991,-0.0316939261509096,
0.0593359630523767));
#75549=CARTESIAN_POINT('',(0.00578652580579316,-0.0320197221621852,0.0688950193390954));
#75550=CARTESIAN_POINT('Ctrl Pts',(0.00578634321248903,-0.0320197392094773,
0.0688950489121256));
#75551=CARTESIAN_POINT('Ctrl Pts',(0.00575960435100756,-0.031979271657607,
0.0689069425960148));
#75552=CARTESIAN_POINT('Ctrl Pts',(0.00573283443670875,-0.0319386439829719,
0.0689190942707985));
#75553=CARTESIAN_POINT('Ctrl Pts',(0.00570600886206676,-0.031897909938165,
0.0689315243946623));
#75554=CARTESIAN_POINT('Ctrl Pts',(0.00567918381765027,-0.0318571766984939,
0.0689439542728364));
#75555=CARTESIAN_POINT('Ctrl Pts',(0.00565243870842038,-0.0318163871833576,
0.0689565977957526));
#75556=CARTESIAN_POINT('Ctrl Pts',(0.00562586402162872,-0.0317755399638302,
0.0689694082915398));
#75557=CARTESIAN_POINT('',(0.0057873002927968,-0.0321934096636183,0.068896110742553));
#75558=CARTESIAN_POINT('Origin',(0.00482998040805077,-0.032411314875615,
0.0667952183655116));
#75559=CARTESIAN_POINT('',(0.00573019280085328,-0.0321934096636663,0.0689215072849694));
#75560=CARTESIAN_POINT('Ctrl Pts',(0.0056749785059328,-0.0321934096636618,
0.0689476314896054));
#75561=CARTESIAN_POINT('Ctrl Pts',(0.00560323378968558,-0.0320835708272592,
0.0689814024009375));
#75562=CARTESIAN_POINT('Ctrl Pts',(0.00553222957554433,-0.0319739230346488,
0.0690166384769426));
#75563=CARTESIAN_POINT('Ctrl Pts',(0.00546205324854853,-0.0318646057455572,
0.0690532876634087));
#75564=CARTESIAN_POINT('Ctrl Pts',(0.00556920366535213,-0.0321934096636618,
0.0689069762579045));
#75565=CARTESIAN_POINT('Ctrl Pts',(0.00549689828177492,-0.0320835708272592,
0.0689422058867243));
#75566=CARTESIAN_POINT('Ctrl Pts',(0.00542536391359611,-0.0319739230346488,
0.0689789114370829));
#75567=CARTESIAN_POINT('Ctrl Pts',(0.0053546884798588,-0.0318646057455572,
0.0690170389226206));
#75568=CARTESIAN_POINT('Ctrl Pts',(0.00546342882477146,-0.0321934096636618,
0.0688663210262035));
#75569=CARTESIAN_POINT('Ctrl Pts',(0.00539056277386426,-0.0320835708272592,
0.068903009372511));
#75570=CARTESIAN_POINT('Ctrl Pts',(0.00531849825164789,-0.0319739230346488,
0.0689411843972231));
#75571=CARTESIAN_POINT('Ctrl Pts',(0.00524732371116907,-0.0318646057455572,
0.0689807901818324));
#75572=CARTESIAN_POINT('Ctrl Pts',(0.00535765398419079,-0.0321934096636618,
0.0688256657945026));
#75573=CARTESIAN_POINT('Ctrl Pts',(0.0052842272659536,-0.0320835708272592,
0.0688638128582977));
#75574=CARTESIAN_POINT('Ctrl Pts',(0.00521163258969967,-0.0319739230346488,
0.0689034573573634));
#75575=CARTESIAN_POINT('Ctrl Pts',(0.00513995894247935,-0.0318646057455572,
0.0689445414410442));
#75576=CARTESIAN_POINT('',(0.00534628742212121,-0.0321763980308452,0.0688315864419187));
#75577=CARTESIAN_POINT('',(0.00535765398416181,-0.0321934096636184,0.0688256657945176));
#75578=CARTESIAN_POINT('Origin',(0.0124573985862644,-0.032638623105711,
0.0837734131738772));
#75579=CARTESIAN_POINT('Ctrl Pts',(0.0053462874235849,-0.0321763980306276,
0.0688315864447262));
#75580=CARTESIAN_POINT('Ctrl Pts',(0.00536615525725229,-0.0321259596174872,
0.0688696298488218));
#75581=CARTESIAN_POINT('Ctrl Pts',(0.00538567885492711,-0.0320749164631493,
0.0689070141015737));
#75582=CARTESIAN_POINT('Ctrl Pts',(0.005424053290234,-0.0319716057793892,
0.0689804943900522));
#75583=CARTESIAN_POINT('Ctrl Pts',(0.00544288917589063,-0.0319193786690081,
0.0690165617953779));
#75584=CARTESIAN_POINT('Ctrl Pts',(0.00546138748399746,-0.031866561752526,
0.0690519827991057));
#75585=CARTESIAN_POINT('',(0.00551536964653578,-0.0321934096636663,0.0688862848109516));
#75586=CARTESIAN_POINT('Origin',(0.00812378219310841,-0.0315241814719618,
0.07415));
#75587=CARTESIAN_POINT('',(0.00534628742194917,-0.0322104233323791,0.0688315864415895));
#75588=CARTESIAN_POINT('',(0.00533493353088838,-0.0321934096636183,0.0688375313516916));
#75589=CARTESIAN_POINT('Origin',(0.0125001154882419,-0.0326387233587389,
0.0837582318680157));
#75590=CARTESIAN_POINT('Origin',(0.0135450215143358,-0.0326386243771962,
0.0832054147042603));
#75591=CARTESIAN_POINT('Origin',(0.0135081509368146,-0.0326387244007988,
0.0832317913507903));
#75592=CARTESIAN_POINT('Ctrl Pts',(0.0056052613123584,-0.0327445246967097,
0.0689793929202437));
#75593=CARTESIAN_POINT('Ctrl Pts',(0.00541024867832073,-0.032443687833936,
0.0690743804880976));
#75594=CARTESIAN_POINT('Ctrl Pts',(0.00522294490640992,-0.0321434074405927,
0.0691837873549253));
#75595=CARTESIAN_POINT('Ctrl Pts',(0.00538293783121712,-0.0327445246967097,
0.0690937269472576));
#75596=CARTESIAN_POINT('Ctrl Pts',(0.00519223737550286,-0.032443687833936,
0.0691970995822799));
#75597=CARTESIAN_POINT('Ctrl Pts',(0.00500986512900158,-0.0321434074405927,
0.0693145428842906));
#75598=CARTESIAN_POINT('',(0.00535121608758842,-0.0326943950436612,0.0691110514796713));
#75599=CARTESIAN_POINT('',(0.00514653396172323,-0.0323666188837389,0.0692292157160962));
#75600=CARTESIAN_POINT('Origin',(0.0135218084878484,-0.0326395579110189,
0.0838028681836174));
#75601=CARTESIAN_POINT('Origin',(-0.000570818722665324,-0.0321933825603095,
0.0597795993160227));
#75602=CARTESIAN_POINT('',(0.00525418552987477,-0.0321934096532689,0.0691656705579445));
#75603=CARTESIAN_POINT('',(0.00520071137581225,-0.0321934096584275,0.0691980243087788));
#75604=CARTESIAN_POINT('',(0.00546138748270218,-0.0325210109756239,0.0690519827966157));
#75605=CARTESIAN_POINT('Origin',(0.0130889041165304,-0.0326393129159009,
0.0840121006749662));
#75606=CARTESIAN_POINT('',(0.00546201637008394,-0.0326943950436593,0.0690531870052572));
#75607=CARTESIAN_POINT('Origin',(0.000341031935603809,-0.0326943765538163,
0.0592474012077398));
#75608=CARTESIAN_POINT('',(0.00540661622884618,-0.0326943950436702,0.0690821192424742));
#75609=CARTESIAN_POINT('Ctrl Pts',(0.00555688632331576,-0.0325229783203769,
0.0687268048538092));
#75610=CARTESIAN_POINT('Ctrl Pts',(0.00548212769682297,-0.032413025309245,
0.06876218945724));
#75611=CARTESIAN_POINT('Ctrl Pts',(0.00540811238491736,-0.0323031222208069,
0.0687991151721256));
#75612=CARTESIAN_POINT('Ctrl Pts',(0.00533493352691798,-0.0321934096576658,
0.0688375313537759));
#75613=CARTESIAN_POINT('Ctrl Pts',(0.0055252840289352,-0.0325229783203769,
0.0688356278165799));
#75614=CARTESIAN_POINT('Ctrl Pts',(0.00545202552460439,-0.032413025309245,
0.0688714480569477));
#75615=CARTESIAN_POINT('Ctrl Pts',(0.00537951911904752,-0.0323031222208069,
0.0689087783107434));
#75616=CARTESIAN_POINT('Ctrl Pts',(0.00530785600049679,-0.0321934096576658,
0.0689475674832935));
#75617=CARTESIAN_POINT('Ctrl Pts',(0.00549368173455463,-0.0325229783203769,
0.0689444507793506));
#75618=CARTESIAN_POINT('Ctrl Pts',(0.00542192335238582,-0.032413025309245,
0.0689807066566553));
#75619=CARTESIAN_POINT('Ctrl Pts',(0.00535092585317768,-0.032303122220807,
0.0690184414493611));
#75620=CARTESIAN_POINT('Ctrl Pts',(0.00528077847407559,-0.0321934096576658,
0.0690576036128112));
#75621=CARTESIAN_POINT('Ctrl Pts',(0.00546207944017407,-0.0325229783203769,
0.0690532737421213));
#75622=CARTESIAN_POINT('Ctrl Pts',(0.00539182118016725,-0.032413025309245,
0.0690899652563629));
#75623=CARTESIAN_POINT('Ctrl Pts',(0.00532233258730784,-0.032303122220807,
0.0691281045879789));
#75624=CARTESIAN_POINT('Ctrl Pts',(0.0052537009476544,-0.0321934096576658,
0.0691676397423288));
#75625=CARTESIAN_POINT('',(0.00529455953074173,-0.0321934096584275,0.069001600954455));
#75626=CARTESIAN_POINT('Ctrl Pts',(0.00534628742355425,-0.0322104233328935,
0.0688315864446675));
#75627=CARTESIAN_POINT('Ctrl Pts',(0.00536618217845319,-0.0322609421831227,
0.0688696813981825));
#75628=CARTESIAN_POINT('Ctrl Pts',(0.00538571892758863,-0.0323120888240435,
0.068907090833681));
#75629=CARTESIAN_POINT('Ctrl Pts',(0.00542409365344589,-0.0324156524631814,
0.0689805716785123));
#75630=CARTESIAN_POINT('Ctrl Pts',(0.00544291585612749,-0.0324680267167309,
0.0690166128833349));
#75631=CARTESIAN_POINT('Ctrl Pts',(0.0054613874827183,-0.0325210109755912,
0.0690519827966562));
#75632=CARTESIAN_POINT('Origin',(0.0154857614310304,-0.0262834582512449,
0.0713742753129969));
#75633=CARTESIAN_POINT('Origin',(0.00791146188208468,-0.034277077895491,
0.0619935970171797));
#75634=CARTESIAN_POINT('Ctrl Pts',(0.00535315076944912,-0.0326943950436604,
0.0691116586838633));
#75635=CARTESIAN_POINT('Ctrl Pts',(0.0052837129832547,-0.0325844576448134,
0.069149843177598));
#75636=CARTESIAN_POINT('Ctrl Pts',(0.00521506000077505,-0.0324744968375322,
0.069189466460972));
#75637=CARTESIAN_POINT('Ctrl Pts',(0.00514727908397632,-0.0323646534831894,
0.0692304765530607));
#75638=CARTESIAN_POINT('Ctrl Pts',(0.00524503204476973,-0.0326943950436604,
0.0690777253822981));
#75639=CARTESIAN_POINT('Ctrl Pts',(0.00517512659408197,-0.0325844576448134,
0.069117399954695));
#75640=CARTESIAN_POINT('Ctrl Pts',(0.00510603673128137,-0.0324744968375322,
0.0691585230942548));
#75641=CARTESIAN_POINT('Ctrl Pts',(0.00503785025158459,-0.0323646534831894,
0.069201040890629));
#75642=CARTESIAN_POINT('Ctrl Pts',(0.00513691332009035,-0.0326943950436604,
0.0690437920807329));
#75643=CARTESIAN_POINT('Ctrl Pts',(0.00506654020490923,-0.0325844576448134,
0.069084956731792));
#75644=CARTESIAN_POINT('Ctrl Pts',(0.00499701346178769,-0.0324744968375322,
0.0691275797275376));
#75645=CARTESIAN_POINT('Ctrl Pts',(0.00492842141919285,-0.0323646534831894,
0.0691716052281974));
#75646=CARTESIAN_POINT('Ctrl Pts',(0.00502879459541097,-0.0326943950436604,
0.0690098587791677));
#75647=CARTESIAN_POINT('Ctrl Pts',(0.0049579538157365,-0.0325844576448134,
0.069052513508889));
#75648=CARTESIAN_POINT('Ctrl Pts',(0.00488799019229401,-0.0324744968375322,
0.0690966363608204));
#75649=CARTESIAN_POINT('Ctrl Pts',(0.00481899258680112,-0.0323646534831894,
0.0691421695657657));
#75650=CARTESIAN_POINT('',(0.00501782222310387,-0.0326773559991334,0.0690164814556856));
#75651=CARTESIAN_POINT('',(0.00502879459541033,-0.0326943950436594,0.0690098587791681));
#75652=CARTESIAN_POINT('Origin',(0.0136566259742715,-0.0326395670209633,
0.0831976090128865));
#75653=CARTESIAN_POINT('Ctrl Pts',(0.00501782222483375,-0.0326773559987417,
0.0690164814585482));
#75654=CARTESIAN_POINT('Ctrl Pts',(0.00504005749802945,-0.0326267922586026,
0.0690532318315055));
#75655=CARTESIAN_POINT('Ctrl Pts',(0.00506189866706431,-0.0325756109579462,
0.0690893308306403));
#75656=CARTESIAN_POINT('Ctrl Pts',(0.00510481138473952,-0.0324719985462365,
0.0691602568033186));
#75657=CARTESIAN_POINT('Ctrl Pts',(0.00512586572225259,-0.0324196091621774,
0.069195055330378));
#75658=CARTESIAN_POINT('Ctrl Pts',(0.00514653396174843,-0.0323666188837756,
0.069229215716138));
#75659=CARTESIAN_POINT('',(0.00519000534150938,-0.0326943950436702,0.0690604551294297));
#75660=CARTESIAN_POINT('Origin',(0.00812378219310841,-0.0315241814719618,
0.07415));
#75661=CARTESIAN_POINT('',(0.00501782222312663,-0.0327114338379879,0.0690164814557234));
#75662=CARTESIAN_POINT('',(0.00500686402026083,-0.0326943950436593,0.069023127551441));
#75663=CARTESIAN_POINT('Origin',(0.0136949868758667,-0.0326395667777739,
0.083173494238871));
#75664=CARTESIAN_POINT('Origin',(0.0135706575092932,-0.0326395679847929,
0.0832496254823012));
#75665=CARTESIAN_POINT('Origin',(0.0135314925742125,-0.0326395677859133,
0.0832724112383833));
#75666=CARTESIAN_POINT('Ctrl Pts',(0.00528553181829957,-0.0332451089994433,
0.0691477545232268));
#75667=CARTESIAN_POINT('Ctrl Pts',(0.00509686904345838,-0.0329451141710254,
0.069254800887483));
#75668=CARTESIAN_POINT('Ctrl Pts',(0.00491680540941372,-0.0326442513127493,
0.0693757539957767));
#75669=CARTESIAN_POINT('Ctrl Pts',(0.00507082700813731,-0.0332451089994433,
0.0692758242093091));
#75670=CARTESIAN_POINT('Ctrl Pts',(0.00488699446053337,-0.0329451141710254,
0.0693909682979662));
#75671=CARTESIAN_POINT('Ctrl Pts',(0.00471235728526579,-0.0326442513127493,
0.0695196322934187));
#75672=CARTESIAN_POINT('',(0.00504028891799165,-0.0331951640388616,0.0692950855597332));
#75673=CARTESIAN_POINT('',(0.00484343027934221,-0.0328677532092642,0.0694258687230506));
#75674=CARTESIAN_POINT('Origin',(0.014666974025928,-0.0326401908899162,
0.0830194791727825));
#75675=CARTESIAN_POINT('Origin',(-0.00146245926292119,-0.0326944279134284,
0.0603445729840615));
#75676=CARTESIAN_POINT('',(0.00494687938261152,-0.0326943950436593,0.0693556894622211));
#75677=CARTESIAN_POINT('',(0.00489554225887862,-0.0326943950436693,0.0693913370389483));
#75678=CARTESIAN_POINT('',(0.00514653396172563,-0.0330220786163545,0.0692292157160947));
#75679=CARTESIAN_POINT('Origin',(0.0142907263605349,-0.032639668276516,
0.0833189963584933));
#75680=CARTESIAN_POINT('',(0.00514723722102947,-0.0331951640388587,0.0692303780603392));
#75681=CARTESIAN_POINT('Origin',(-0.000563407297126675,-0.0331952026560132,
0.0597918448727092));
#75682=CARTESIAN_POINT('',(0.00509376306952056,-0.0331951640388701,0.0692627318100462));
#75683=CARTESIAN_POINT('Ctrl Pts',(0.00522142542423587,-0.0330240426238172,
0.0688986834806688));
#75684=CARTESIAN_POINT('Ctrl Pts',(0.00514908342307229,-0.032914277406352,
0.0689386662727892));
#75685=CARTESIAN_POINT('Ctrl Pts',(0.00507753191278236,-0.0328043479726691,
0.0689801645090312));
#75686=CARTESIAN_POINT('Ctrl Pts',(0.00500686402026084,-0.0326943950436593,
0.069023127551441));
#75687=CARTESIAN_POINT('Ctrl Pts',(0.00519671856385909,-0.0330240426238172,
0.0690092760076984));
#75688=CARTESIAN_POINT('Ctrl Pts',(0.00512590008250043,-0.032914277406352,
0.0690495991608912));
#75689=CARTESIAN_POINT('Ctrl Pts',(0.00505587988775971,-0.0328043479726691,
0.0690914064324779));
#75690=CARTESIAN_POINT('Ctrl Pts',(0.00498674915570538,-0.0326943950436593,
0.0691346467345818));
#75691=CARTESIAN_POINT('Ctrl Pts',(0.00517201170348231,-0.0330240426238172,
0.069119868534728));
#75692=CARTESIAN_POINT('Ctrl Pts',(0.00510271674192856,-0.032914277406352,
0.0691605320489933));
#75693=CARTESIAN_POINT('Ctrl Pts',(0.00503422786273706,-0.0328043479726691,
0.0692026483559246));
#75694=CARTESIAN_POINT('Ctrl Pts',(0.00496663429114993,-0.0326943950436593,
0.0692461659177226));
#75695=CARTESIAN_POINT('Ctrl Pts',(0.00514730484310553,-0.0330240426238172,
0.0692304610617576));
#75696=CARTESIAN_POINT('Ctrl Pts',(0.00507953340135669,-0.032914277406352,
0.0692714649370953));
#75697=CARTESIAN_POINT('Ctrl Pts',(0.0050125758377144,-0.0328043479726691,
0.0693138902793714));
#75698=CARTESIAN_POINT('Ctrl Pts',(0.00494651942659447,-0.0326943950436593,
0.0693576851008633));
#75699=CARTESIAN_POINT('',(0.00497687170144618,-0.0326943950436694,0.0691894085068411));
#75700=CARTESIAN_POINT('Ctrl Pts',(0.00501782222483762,-0.0327114338383332,
0.0690164814585545));
#75701=CARTESIAN_POINT('Ctrl Pts',(0.00504005379958046,-0.0327619876830956,
0.0690532257187232));
#75702=CARTESIAN_POINT('Ctrl Pts',(0.00506189316211955,-0.0328131562604296,
0.0690893217320889));
#75703=CARTESIAN_POINT('Ctrl Pts',(0.00510480584038152,-0.0329167375858771,
0.0691602476396251));
#75704=CARTESIAN_POINT('Ctrl Pts',(0.00512586205748005,-0.0329691088920615,
0.069195049273256));
#75705=CARTESIAN_POINT('Ctrl Pts',(0.00514653396174787,-0.0330220786163186,
0.0692292157161368));
#75706=CARTESIAN_POINT('Ctrl Pts',(0.00504225822323976,-0.0331951640388604,
0.069295570163427));
#75707=CARTESIAN_POINT('Ctrl Pts',(0.00497539826488769,-0.0330855618127442,
0.0693380119271814));
#75708=CARTESIAN_POINT('Ctrl Pts',(0.00490936730693175,-0.0329757224171941,
0.0693818661678264));
#75709=CARTESIAN_POINT('Ctrl Pts',(0.00484425266066457,-0.0328657861694599,
0.0694270808750398));
#75710=CARTESIAN_POINT('Ctrl Pts',(0.00493222205174072,-0.0331951640388604,
0.0692684926265878));
#75711=CARTESIAN_POINT('Ctrl Pts',(0.00486498915505268,-0.0330855618127442,
0.0693124499161797));
#75712=CARTESIAN_POINT('Ctrl Pts',(0.00479861631324684,-0.0329757224171941,
0.0693578284831826));
#75713=CARTESIAN_POINT('Ctrl Pts',(0.00473319137116802,-0.0328657861694599,
0.0694045743867574));
#75714=CARTESIAN_POINT('Ctrl Pts',(0.00482218588024168,-0.0331951640388604,
0.0692414150897486));
#75715=CARTESIAN_POINT('Ctrl Pts',(0.00475458004521767,-0.0330855618127442,
0.069286887905178));
#75716=CARTESIAN_POINT('Ctrl Pts',(0.00468786531956193,-0.0329757224171941,
0.0693337907985387));
#75717=CARTESIAN_POINT('Ctrl Pts',(0.00462213008167146,-0.0328657861694599,
0.069382067898475));
#75718=CARTESIAN_POINT('Ctrl Pts',(0.00471214970874264,-0.0331951640388604,
0.0692143375529094));
#75719=CARTESIAN_POINT('Ctrl Pts',(0.00464417093538266,-0.0330855618127442,
0.0692613258941764));
#75720=CARTESIAN_POINT('Ctrl Pts',(0.00457711432587703,-0.0329757224171941,
0.0693097531138949));
#75721=CARTESIAN_POINT('Ctrl Pts',(0.00451106879217491,-0.0328657861694599,
0.0693595614101926));
#75722=CARTESIAN_POINT('',(0.00470161482908265,-0.0331781648279162,0.0692216361218709));
#75723=CARTESIAN_POINT('',(0.00471214970874164,-0.0331951640388588,0.0692143375529101));
#75724=CARTESIAN_POINT('Origin',(0.0147015863296263,-0.0326412091934606,
0.0823740905285352));
#75725=CARTESIAN_POINT('Ctrl Pts',(0.00470161483108013,-0.0331781648273352,
0.0692216361247498));
#75726=CARTESIAN_POINT('Ctrl Pts',(0.00472613074176301,-0.0331276810207405,
0.0692569422088178));
#75727=CARTESIAN_POINT('Ctrl Pts',(0.00475020378706199,-0.0330765665168933,
0.0692916105094203));
#75728=CARTESIAN_POINT('Ctrl Pts',(0.0047974855800995,-0.0329730612715184,
0.0693597024102866));
#75729=CARTESIAN_POINT('Ctrl Pts',(0.00482067475170455,-0.0329207135598913,
0.0693930978183848));
#75730=CARTESIAN_POINT('Ctrl Pts',(0.0048434302793682,-0.0328677532092986,
0.0694258687230881));
#75731=CARTESIAN_POINT('',(0.00487621931337665,-0.0331951640388701,0.0692547115563316));
#75732=CARTESIAN_POINT('Origin',(0.00812378219310841,-0.0315241814719618,
0.07415));
#75733=CARTESIAN_POINT('',(0.00470161482934441,-0.0332121607144427,0.069221636122248));
#75734=CARTESIAN_POINT('',(0.00469109556167718,-0.0331951640388587,0.069228957174499));
#75735=CARTESIAN_POINT('Origin',(0.014733799291535,-0.0326413651105875,
0.082342175563266));
#75736=CARTESIAN_POINT('Origin',(0.0135314857625357,-0.0326412100173772,
0.0831865897364757));
#75737=CARTESIAN_POINT('Origin',(0.0134903253941661,-0.0326413661000901,
0.0832056188927701));
#75738=CARTESIAN_POINT('Ctrl Pts',(0.00497705630180331,-0.0337436976235975,
0.0693358291300589));
#75739=CARTESIAN_POINT('Ctrl Pts',(0.0049337569193915,-0.0336723290703325,
0.0693641312596247));
#75740=CARTESIAN_POINT('Ctrl Pts',(0.00489097360790398,-0.033601104548885,
0.0693932076299855));
#75741=CARTESIAN_POINT('Ctrl Pts',(0.00475437496922083,-0.0333736987606857,
0.0694860427208433));
#75742=CARTESIAN_POINT('Ctrl Pts',(0.00462332884708358,-0.0331450831799191,
0.0695865636443243));
#75743=CARTESIAN_POINT('Ctrl Pts',(0.00477081621287937,-0.0337436976235975,
0.06947712677944));
#75744=CARTESIAN_POINT('Ctrl Pts',(0.00472878768294034,-0.0336723290703325,
0.0695072838636221));
#75745=CARTESIAN_POINT('Ctrl Pts',(0.00468730838311847,-0.033601104548885,
0.069538192029881));
#75746=CARTESIAN_POINT('Ctrl Pts',(0.00455487319537358,-0.0333736987606857,
0.0696368756821829));
#75747=CARTESIAN_POINT('Ctrl Pts',(0.00442831928731498,-0.0331450831799191,
0.0697429966063202));
#75748=CARTESIAN_POINT('Ctrl Pts',(0.00476875381199013,-0.0337436976235975,
0.0694785397559338));
#75749=CARTESIAN_POINT('Ctrl Pts',(0.00472673799057583,-0.0336723290703325,
0.0695087153896621));
#75750=CARTESIAN_POINT('Ctrl Pts',(0.00468527173087061,-0.033601104548885,
0.06953964187388));
#75751=CARTESIAN_POINT('Ctrl Pts',(0.00455287817763511,-0.0333736987606857,
0.0696383840117963));
#75752=CARTESIAN_POINT('Ctrl Pts',(0.0044263691917173,-0.0331450831799191,
0.0697445609359402));
#75753=CARTESIAN_POINT('',(0.00474153088762703,-0.0336938721132548,0.0694982797690993));
#75754=CARTESIAN_POINT('',(0.00455327264161155,-0.0333679869945434,0.069641165722439));
#75755=CARTESIAN_POINT('Ctrl Pts',(0.00474153088762864,-0.0336938721132646,
0.0694982797690973));
#75756=CARTESIAN_POINT('Ctrl Pts',(0.00472337304140678,-0.0336629187933929,
0.0695114822825854));
#75757=CARTESIAN_POINT('Ctrl Pts',(0.00470529830852139,-0.0336319952301037,
0.0695247868950853));
#75758=CARTESIAN_POINT('Ctrl Pts',(0.00468730838312026,-0.0336011045488947,
0.0695381920298795));
#75759=CARTESIAN_POINT('Ctrl Pts',(0.00464216550448278,-0.0335235892595451,
0.0695718301000573));
#75760=CARTESIAN_POINT('Ctrl Pts',(0.00459747651609426,-0.0334458668660366,
0.0696061610300895));
#75761=CARTESIAN_POINT('Ctrl Pts',(0.00455327264141187,-0.0333679869945382,
0.0696411657221753));
#75762=CARTESIAN_POINT('Ctrl Pts',(0.0045532373518823,-0.0333679692460362,
0.0696411927909531));
#75763=CARTESIAN_POINT('Ctrl Pts',(0.00455352335907653,-0.0333391895375493,
0.0696415444124923));
#75764=CARTESIAN_POINT('Ctrl Pts',(0.00455374025450246,-0.0333104081061546,
0.0696418059209864));
#75765=CARTESIAN_POINT('Ctrl Pts',(0.00455403161565926,-0.033253269824495,
0.0696421485364477));
#75766=CARTESIAN_POINT('Ctrl Pts',(0.00455410816086979,-0.0332249171348981,
0.0696422322757971));
#75767=CARTESIAN_POINT('Ctrl Pts',(0.0045541158481945,-0.0331960985361085,
0.0696422308701326));
#75768=CARTESIAN_POINT('Ctrl Pts',(0.00455411595436276,-0.0331956312563914,
0.0696422308240151));
#75769=CARTESIAN_POINT('Ctrl Pts',(0.00455411604157513,-0.0331951640388587,
0.0696422307549524));
#75770=CARTESIAN_POINT('',(0.00465211102516163,-0.0331951640388587,0.0695646293168766));
#75771=CARTESIAN_POINT('',(0.00460311353337761,-0.0331951640388687,0.069603430035925));
#75772=CARTESIAN_POINT('',(0.00484343027971246,-0.0335216366567749,0.0694258687232914));
#75773=CARTESIAN_POINT('Origin',(0.0153120163414045,-0.0326434571528763,
0.0823788363706307));
#75774=CARTESIAN_POINT('',(0.0048442051351257,-0.0336938721132327,0.0694269846156556));
#75775=CARTESIAN_POINT('Origin',(-0.00138446321486033,-0.0336938867896402,
0.060456894283551));
#75776=CARTESIAN_POINT('',(0.00479286801138636,-0.0336938721132538,0.0694626321923875));
#75777=CARTESIAN_POINT('Ctrl Pts',(0.00489741885958399,-0.0335235895815172,
0.0690912867604388));
#75778=CARTESIAN_POINT('Ctrl Pts',(0.00482777571215158,-0.0334144449262748,
0.0691357040038496));
#75779=CARTESIAN_POINT('Ctrl Pts',(0.00475897018000144,-0.0333049234473147,
0.0691816110523054));
#75780=CARTESIAN_POINT('Ctrl Pts',(0.00469109556167717,-0.0331951640388587,
0.0692289571744989));
#75781=CARTESIAN_POINT('Ctrl Pts',(0.00487970490753242,-0.0335235895815172,
0.0692032125768915));
#75782=CARTESIAN_POINT('Ctrl Pts',(0.00481160263932514,-0.0334144449262748,
0.0692478736877279));
#75783=CARTESIAN_POINT('Ctrl Pts',(0.00474434479480116,-0.0333049234473147,
0.0692939930503782));
#75784=CARTESIAN_POINT('Ctrl Pts',(0.00467802271807902,-0.0331951640388587,
0.0693415194827825));
#75785=CARTESIAN_POINT('Ctrl Pts',(0.00486199095548085,-0.0335235895815172,
0.0693151383933442));
#75786=CARTESIAN_POINT('Ctrl Pts',(0.0047954295664987,-0.0334144449262748,
0.0693600433716061));
#75787=CARTESIAN_POINT('Ctrl Pts',(0.00472971940960087,-0.0333049234473147,
0.069406375048451));
#75788=CARTESIAN_POINT('Ctrl Pts',(0.00466494987448086,-0.0331951640388587,
0.0694540817910662));
#75789=CARTESIAN_POINT('Ctrl Pts',(0.00484427700342929,-0.0335235895815172,
0.0694270642097969));
#75790=CARTESIAN_POINT('Ctrl Pts',(0.00477925649367226,-0.0334144449262748,
0.0694722130554844));
#75791=CARTESIAN_POINT('Ctrl Pts',(0.00471509402440059,-0.0333049234473147,
0.0695187570465238));
#75792=CARTESIAN_POINT('Ctrl Pts',(0.00465187703088271,-0.0331951640388587,
0.0695666440993499));
#75793=CARTESIAN_POINT('',(0.0046716032934294,-0.0331951640388687,0.0693967932456978));
#75794=CARTESIAN_POINT('Ctrl Pts',(0.00470161483112568,-0.0332121607145986,
0.0692216361248153));
#75795=CARTESIAN_POINT('Ctrl Pts',(0.00472608942773211,-0.0332625444109771,
0.0692568827112666));
#75796=CARTESIAN_POINT('Ctrl Pts',(0.00475014228863203,-0.033313530074685,
0.0692915219437223));
#75797=CARTESIAN_POINT('Ctrl Pts',(0.0047974236318699,-0.0334167203140656,
0.0693596131968189));
#75798=CARTESIAN_POINT('Ctrl Pts',(0.00482063380175359,-0.0334688847587368,
0.0693930388451559));
#75799=CARTESIAN_POINT('Ctrl Pts',(0.00484343027997499,-0.0335216366562442,
0.0694258687239619));
#75800=CARTESIAN_POINT('Ctrl Pts',(0.00474251486686462,-0.0336938721132391,
0.0694984572507384));
#75801=CARTESIAN_POINT('Ctrl Pts',(0.00471528784360763,-0.0336474569764958,
0.0695182489304224));
#75802=CARTESIAN_POINT('Ctrl Pts',(0.00468829437256328,-0.033601104548885,
0.0695383579806518));
#75803=CARTESIAN_POINT('Ctrl Pts',(0.00461995311006718,-0.0334837508592656,
0.0695892694724721));
#75804=CARTESIAN_POINT('Ctrl Pts',(0.00455315047107649,-0.0333660264659097,
0.0696421837010198));
#75805=CARTESIAN_POINT('Ctrl Pts',(0.00474153088764373,-0.0336938721132391,
0.0694982797690873));
#75806=CARTESIAN_POINT('Ctrl Pts',(0.00471430282552774,-0.0336474569764958,
0.0695180772083282));
#75807=CARTESIAN_POINT('Ctrl Pts',(0.00468730838311847,-0.033601104548885,
0.069538192029881));
#75808=CARTESIAN_POINT('Ctrl Pts',(0.0046189646613497,-0.0334837508592656,
0.0695891181333652));
#75809=CARTESIAN_POINT('Ctrl Pts',(0.00455215999714016,-0.0333660264659097,
0.0696420470400339));
#75810=CARTESIAN_POINT('Ctrl Pts',(0.00440697360539036,-0.0336938721132391,
0.0694379352236103));
#75811=CARTESIAN_POINT('Ctrl Pts',(0.00437939232662525,-0.0336474569764958,
0.0694596909376421));
#75812=CARTESIAN_POINT('Ctrl Pts',(0.00435206761584843,-0.033601104548885,
0.0694817680346504));
#75813=CARTESIAN_POINT('Ctrl Pts',(0.00428288773050648,-0.0334837508592656,
0.0695376621684326));
#75814=CARTESIAN_POINT('Ctrl Pts',(0.00421539448294333,-0.0333660264659097,
0.0695955817010667));
#75815=CARTESIAN_POINT('',(0.00439891316541995,-0.0336769361243754,0.0694462407877776));
#75816=CARTESIAN_POINT('',(0.00440896897686215,-0.0336938721132327,0.069438295131441));
#75817=CARTESIAN_POINT('Ctrl Pts',(0.00439891316541972,-0.0336769361243751,
0.0694462407877777));
#75818=CARTESIAN_POINT('Ctrl Pts',(0.00440058784506195,-0.0336797586670119,
0.06944491462246));
#75819=CARTESIAN_POINT('Ctrl Pts',(0.00440226316959848,-0.0336825812713033,
0.0694435894016527));
#75820=CARTESIAN_POINT('Ctrl Pts',(0.0044056151122592,-0.033688226610054,
0.0694409408454027));
#75821=CARTESIAN_POINT('Ctrl Pts',(0.00440729173041062,-0.0336910493445311,
0.0694396175099648));
#75822=CARTESIAN_POINT('Ctrl Pts',(0.00440896897686973,-0.0336938721132297,
0.0694382951314443));
#75823=CARTESIAN_POINT('Ctrl Pts',(0.00439891316541994,-0.0336769361243754,
0.0694462407877776));
#75824=CARTESIAN_POINT('Ctrl Pts',(0.00442493244446343,-0.0336279031301501,
0.0694790978956615));
#75825=CARTESIAN_POINT('Ctrl Pts',(0.00445132607601624,-0.0335767851899374,
0.069512427735351));
#75826=CARTESIAN_POINT('Ctrl Pts',(0.00450304375408568,-0.0334733198857323,
0.0695777367442975));
#75827=CARTESIAN_POINT('Ctrl Pts',(0.00452840252591669,-0.0334209645014072,
0.0696097597646312));
#75828=CARTESIAN_POINT('Ctrl Pts',(0.00455327264731456,-0.0333679869844681,
0.0696411657179049));
#75829=CARTESIAN_POINT('',(0.00457524993225459,-0.0336938721132538,0.0694682874502802));
#75830=CARTESIAN_POINT('Origin',(0.00812378219310841,-0.0315241814719618,
0.07415));
#75831=CARTESIAN_POINT('',(0.00439891316623064,-0.0337108120655408,0.0694462407888005));
#75832=CARTESIAN_POINT('',(0.00438887434898242,-0.0336938721132327,0.0694542079053787));
#75833=CARTESIAN_POINT('Origin',(0.0136799853731458,-0.0345562515490529,
0.0829665979872995));
#75834=CARTESIAN_POINT('Ctrl Pts',(0.00438887434898348,-0.0336938721132302,
0.0694542079053855));
#75835=CARTESIAN_POINT('Ctrl Pts',(0.00439054593505895,-0.0336910493375117,
0.0694528783703849));
#75836=CARTESIAN_POINT('Ctrl Pts',(0.00439221830234833,-0.0336882266065441,
0.0694515496712456));
#75837=CARTESIAN_POINT('Ctrl Pts',(0.00439556457770277,-0.0336825812713071,
0.0694488939626126));
#75838=CARTESIAN_POINT('Ctrl Pts',(0.00439723848577676,-0.0336797586670138,
0.0694475669530962));
#75839=CARTESIAN_POINT('Ctrl Pts',(0.00439891316542014,-0.0336769361243751,
0.0694462407877774));
#75840=CARTESIAN_POINT('Origin',(0.0154322992487056,-0.0345562517336882,
0.0815789516969124));
#75841=CARTESIAN_POINT('Ctrl Pts',(0.00468102272062642,-0.034243627687391,
0.0695428824396771));
#75842=CARTESIAN_POINT('Ctrl Pts',(0.00450726241736391,-0.0339430054201809,
0.0696727282537171));
#75843=CARTESIAN_POINT('Ctrl Pts',(0.00434377626764699,-0.0336441434784052,
0.0698152935274142));
#75844=CARTESIAN_POINT('Ctrl Pts',(0.00448406036984477,-0.034243627687391,
0.0696968494243672));
#75845=CARTESIAN_POINT('Ctrl Pts',(0.00431610702713881,-0.0339430054201809,
0.0698341237959283));
#75846=CARTESIAN_POINT('Ctrl Pts',(0.00415897089040231,-0.0336441434784052,
0.0699836591193309));
#75847=CARTESIAN_POINT('Ctrl Pts',(0.00448209074633695,-0.034243627687391,
0.0696983890942141));
#75848=CARTESIAN_POINT('Ctrl Pts',(0.00431419547323655,-0.0339430054201809,
0.0698357377513504));
#75849=CARTESIAN_POINT('Ctrl Pts',(0.00415712283662986,-0.0336441434784052,
0.06998534277525));
#75850=CARTESIAN_POINT('',(0.00445612105798559,-0.0341934961088741,0.0697198321930303));
#75851=CARTESIAN_POINT('',(0.0042772061819807,-0.0338664212894524,0.0698742570236255));
#75852=CARTESIAN_POINT('Origin',(0.0147304530405027,-0.0345610818077101,
0.0829293437895861));
#75853=CARTESIAN_POINT('Origin',(-0.00305720950804172,-0.0336938005044372,
0.0617216445300011));
#75854=CARTESIAN_POINT('',(0.00437104376775592,-0.0336938721132327,0.0697916655347617));
#75855=CARTESIAN_POINT('',(0.00432457927863607,-0.0336938721132426,0.0698334662674197));
#75856=CARTESIAN_POINT('',(0.00455327264731872,-0.0340203938281605,0.0696411657179016));
#75857=CARTESIAN_POINT('Origin',(0.0143096433318419,-0.0345589643242961,
0.0831626735693432));
#75858=CARTESIAN_POINT('',(0.00455411604157358,-0.034193496108874,0.0696422307549535));
#75859=CARTESIAN_POINT('Origin',(-0.00228688298184838,-0.0341934220717671,
0.0610034258243513));
#75860=CARTESIAN_POINT('',(0.00450511854978958,-0.034193496108884,0.0696810314740019));
#75861=CARTESIAN_POINT('Ctrl Pts',(0.00458614832818682,-0.0340223579322397,
0.069303852392076));
#75862=CARTESIAN_POINT('Ctrl Pts',(0.00451930731339,-0.0339125849573575,
0.0693526455896097));
#75863=CARTESIAN_POINT('Ctrl Pts',(0.0044535231728096,-0.0338030433565231,
0.0694027879544177));
#75864=CARTESIAN_POINT('Ctrl Pts',(0.00438887434898245,-0.0336938721132327,
0.069454207905378));
#75865=CARTESIAN_POINT('Ctrl Pts',(0.0045754971562424,-0.0340223579322397,
0.0694166696441543));
#75866=CARTESIAN_POINT('Ctrl Pts',(0.00451021218559149,-0.0339125849573575,
0.0694656097491285));
#75867=CARTESIAN_POINT('Ctrl Pts',(0.00444598603638544,-0.0338030433565231,
0.0695158667116488));
#75868=CARTESIAN_POINT('Ctrl Pts',(0.0043828951457616,-0.0336938721132327,
0.0695673689806607));
#75869=CARTESIAN_POINT('Ctrl Pts',(0.00456484598429799,-0.0340223579322397,
0.0695294868962326));
#75870=CARTESIAN_POINT('Ctrl Pts',(0.00450111705779298,-0.0339125849573575,
0.0695785739086474));
#75871=CARTESIAN_POINT('Ctrl Pts',(0.00443844889996129,-0.0338030433565231,
0.06962894546888));
#75872=CARTESIAN_POINT('Ctrl Pts',(0.00437691594254075,-0.0336938721132327,
0.0696805300559434));
#75873=CARTESIAN_POINT('Ctrl Pts',(0.00455419481235357,-0.0340223579322397,
0.0696423041483109));
#75874=CARTESIAN_POINT('Ctrl Pts',(0.00449202192999447,-0.0339125849573575,
0.0696915380681663));
#75875=CARTESIAN_POINT('Ctrl Pts',(0.00443091176353713,-0.0338030433565231,
0.0697420242261112));
#75876=CARTESIAN_POINT('Ctrl Pts',(0.00437093673931991,-0.0336938721132327,
0.0697936911312261));
#75877=CARTESIAN_POINT('',(0.00437995905837917,-0.0336938721132427,0.0696229367200802));
#75878=CARTESIAN_POINT('Ctrl Pts',(0.00439891316846227,-0.0337108120662694,
0.0694462407916194));
#75879=CARTESIAN_POINT('Ctrl Pts',(0.00442560760137709,-0.0337611408994287,
0.0694799504828339));
#75880=CARTESIAN_POINT('Ctrl Pts',(0.00445181492011522,-0.033812108878129,
0.0695130450469718));
#75881=CARTESIAN_POINT('Ctrl Pts',(0.00450327920369031,-0.0339153382773236,
0.0695780340697179));
#75882=CARTESIAN_POINT('Ctrl Pts',(0.0045285143959822,-0.033967555847311,
0.0696099010339878));
#75883=CARTESIAN_POINT('Ctrl Pts',(0.00455327264733931,-0.0340203938281304,
0.0696411657179362));
#75884=CARTESIAN_POINT('Ctrl Pts',(0.00445813566200616,-0.0341934961088741,
0.0697200661665839));
#75885=CARTESIAN_POINT('Ctrl Pts',(0.00436655027062025,-0.03402875161944,
0.0697958505202239));
#75886=CARTESIAN_POINT('Ctrl Pts',(0.00427817536200608,-0.033864463329982,
0.0698753554112645));
#75887=CARTESIAN_POINT('Ctrl Pts',(0.00445612105798569,-0.0341934961088741,
0.0697198321930303));
#75888=CARTESIAN_POINT('Ctrl Pts',(0.00436453082938092,-0.03402875161944,
0.069795658197021));
#75889=CARTESIAN_POINT('Ctrl Pts',(0.00427615280912178,-0.033864463329982,
0.0698752049027488));
#75890=CARTESIAN_POINT('Ctrl Pts',(0.00412044891561043,-0.0341934961088741,
0.069680847656515));
#75891=CARTESIAN_POINT('Ctrl Pts',(0.00402805271243154,-0.03402875161944,
0.0697636134175524));
#75892=CARTESIAN_POINT('Ctrl Pts',(0.00393915623170969,-0.033864463329982,
0.0698501272619776));
#75893=CARTESIAN_POINT('',(0.00411091186005815,-0.0341764758832377,0.0696894090435617));
#75894=CARTESIAN_POINT('',(0.00412044891561043,-0.034193496108874,0.069680847656515));
#75895=CARTESIAN_POINT('Origin',(0.0148042182940886,-0.0345621027386101,
0.0823414650918333));
#75896=CARTESIAN_POINT('Ctrl Pts',(0.00411091186182281,-0.0341764758837459,
0.0696894090431294));
#75897=CARTESIAN_POINT('Ctrl Pts',(0.00413962019877557,-0.0341260050044363,
0.0697213203821793));
#75898=CARTESIAN_POINT('Ctrl Pts',(0.00416782954551442,-0.0340749269156142,
0.0697526770013249));
#75899=CARTESIAN_POINT('Ctrl Pts',(0.00422327198472234,-0.0339715436322714,
0.0698143052241697));
#75900=CARTESIAN_POINT('Ctrl Pts',(0.00425048403929732,-0.0339192778254715,
0.0698445534516979));
#75901=CARTESIAN_POINT('Ctrl Pts',(0.00427720618315993,-0.0338664212876715,
0.0698742570193955));
#75902=CARTESIAN_POINT('',(0.00428828498680801,-0.0341934961088841,0.0697003399247827));
#75903=CARTESIAN_POINT('Origin',(0.00812378219310841,-0.0315241814719618,
0.07415));
#75904=CARTESIAN_POINT('',(0.00411091185992463,-0.0342105180190378,0.0696894090446719));
#75905=CARTESIAN_POINT('',(0.00410139311123135,-0.0341934961088739,0.0696979907823524));
#75906=CARTESIAN_POINT('Origin',(0.0148411909658773,-0.0345621707841575,
0.082315243466159));
#75907=CARTESIAN_POINT('Origin',(0.0155656421348607,-0.0345621036641094,
0.0816564701496351));
#75908=CARTESIAN_POINT('Origin',(0.0155356672756884,-0.0345621718092742,
0.0816904701435844));
#75909=CARTESIAN_POINT('Ctrl Pts',(0.00437215892286278,-0.0346945769586965,
0.0697906623105502));
#75910=CARTESIAN_POINT('Ctrl Pts',(0.00428085084957366,-0.0345275153362944,
0.0698692415620135));
#75911=CARTESIAN_POINT('Ctrl Pts',(0.00419199040447123,-0.0343603235965185,
0.0699507126929578));
#75912=CARTESIAN_POINT('Ctrl Pts',(0.00410583681608137,-0.034193496108874,
0.0700348308419054));
#75913=CARTESIAN_POINT('Ctrl Pts',(0.00430983455216918,-0.0346945769586965,
0.0698467310289543));
#75914=CARTESIAN_POINT('Ctrl Pts',(0.00421970086063573,-0.0345275153362944,
0.0699266156893151));
#75915=CARTESIAN_POINT('Ctrl Pts',(0.00413205615495252,-0.0343603235965185,
0.0700093556335772));
#75916=CARTESIAN_POINT('Ctrl Pts',(0.00404715601225469,-0.034193496108874,
0.0700947023011167));
#75917=CARTESIAN_POINT('Ctrl Pts',(0.00424751018147558,-0.0346945769586965,
0.0699027997473563));
#75918=CARTESIAN_POINT('Ctrl Pts',(0.00415855087169777,-0.0345275153362944,
0.0699839898166162));
#75919=CARTESIAN_POINT('Ctrl Pts',(0.00407212190543375,-0.0343603235965185,
0.0700679985741978));
#75920=CARTESIAN_POINT('Ctrl Pts',(0.00398847520842793,-0.034193496108874,
0.0701545737603309));
#75921=CARTESIAN_POINT('Ctrl Pts',(0.004185185810782,-0.0346945769586965,
0.0699588684657625));
#75922=CARTESIAN_POINT('Ctrl Pts',(0.00409740088275988,-0.0345275153362944,
0.0700413639439183));
#75923=CARTESIAN_POINT('Ctrl Pts',(0.0040121876559151,-0.0343603235965185,
0.0701266415148161));
#75924=CARTESIAN_POINT('Ctrl Pts',(0.00392979440460133,-0.034193496108874,
0.0702144452195393));
#75925=CARTESIAN_POINT('',(0.00418518581123245,-0.0346945769586966,0.0699588684653575));
#75926=CARTESIAN_POINT('',(0.00401632040120248,-0.0343667727831428,0.0701242227299197));
#75927=CARTESIAN_POINT('Origin',(0.0158319840860491,-0.0345626457065531,
0.082085258578487));
#75928=CARTESIAN_POINT('Origin',(-0.00387684372025463,-0.0341934771028963,
0.0623880340926365));
#75929=CARTESIAN_POINT('',(0.00410478685445196,-0.034193496108874,0.0700359021076476));
#75930=CARTESIAN_POINT('',(0.0040610387421073,-0.034193496108884,0.0700805378855203));
#75931=CARTESIAN_POINT('',(0.00427720618527019,-0.034521194296272,0.0698742570217944));
#75932=CARTESIAN_POINT('Origin',(0.0154723101030635,-0.0345625596116798,
0.0824043595268634));
#75933=CARTESIAN_POINT('',(0.00427811478949626,-0.0346945769586885,0.0698752670000577));
#75934=CARTESIAN_POINT('Origin',(-0.00312132793923013,-0.0346945685853823,
0.0616502586418894));
#75935=CARTESIAN_POINT('',(0.00423165030037435,-0.0346945769587026,0.0699170677327176));
#75936=CARTESIAN_POINT('Ctrl Pts',(0.00428883617452006,-0.0345231616327841,
0.0695355456406487));
#75937=CARTESIAN_POINT('Ctrl Pts',(0.0042252324178085,-0.0344132092796988,
0.0695884049723428));
#75938=CARTESIAN_POINT('Ctrl Pts',(0.00416272529633964,-0.0343032738558979,
0.069642577170276));
#75939=CARTESIAN_POINT('Ctrl Pts',(0.00410139311123132,-0.034193496108874,
0.0696979907823524));
#75940=CARTESIAN_POINT('Ctrl Pts',(0.00428528989829662,-0.0345231616327841,
0.0696488088741512));
#75941=CARTESIAN_POINT('Ctrl Pts',(0.00422324731579701,-0.0344132092796988,
0.0697017170862703));
#75942=CARTESIAN_POINT('Ctrl Pts',(0.00416230229904373,-0.0343032738558979,
0.0697559058704493));
#75943=CARTESIAN_POINT('Ctrl Pts',(0.00410253114737363,-0.034193496108874,
0.0698113038046059));
#75944=CARTESIAN_POINT('Ctrl Pts',(0.00428174362207317,-0.0345231616327841,
0.0697620721076537));
#75945=CARTESIAN_POINT('Ctrl Pts',(0.00422126221378552,-0.0344132092796988,
0.0698150292001977));
#75946=CARTESIAN_POINT('Ctrl Pts',(0.00416187930174781,-0.0343032738558979,
0.0698692345706226));
#75947=CARTESIAN_POINT('Ctrl Pts',(0.00410366918351593,-0.034193496108874,
0.0699246168268594));
#75948=CARTESIAN_POINT('Ctrl Pts',(0.00427819734584973,-0.0345231616327841,
0.0698753353411561));
#75949=CARTESIAN_POINT('Ctrl Pts',(0.00421927711177403,-0.0344132092796988,
0.0699283413141251));
#75950=CARTESIAN_POINT('Ctrl Pts',(0.0041614563044519,-0.0343032738558979,
0.0699825632707959));
#75951=CARTESIAN_POINT('Ctrl Pts',(0.00410480721965824,-0.034193496108874,
0.0700379298491129));
#75952=CARTESIAN_POINT('',(0.00410308998285166,-0.0341934961088839,0.06986694644501));
#75953=CARTESIAN_POINT('Ctrl Pts',(0.00411091186222982,-0.0342105180195396,
0.0696894090472348));
#75954=CARTESIAN_POINT('Ctrl Pts',(0.00413965246293281,-0.0342610556241236,
0.0697213562702702));
#75955=CARTESIAN_POINT('Ctrl Pts',(0.00416787732841666,-0.0343122189870013,
0.0697527302169068));
#75956=CARTESIAN_POINT('Ctrl Pts',(0.00422332033032435,-0.0344158119695205,
0.0698143590591847));
#75957=CARTESIAN_POINT('Ctrl Pts',(0.00425051986541438,-0.0344682069747753,
0.0698445932781199));
#75958=CARTESIAN_POINT('Ctrl Pts',(0.00427721020851433,-0.034521202284613,
0.0698742614939208));
#75959=CARTESIAN_POINT('Ctrl Pts',(0.00418721063751565,-0.0346945769586932,
0.0699589754530923));
#75960=CARTESIAN_POINT('Ctrl Pts',(0.00410056417048217,-0.034529677707698,
0.0700403612845754));
#75961=CARTESIAN_POINT('Ctrl Pts',(0.00401735549297437,-0.034364806625142,
0.0701252587509863));
#75962=CARTESIAN_POINT('Ctrl Pts',(0.00418518581123912,-0.0346945769586932,
0.0699588684653514));
#75963=CARTESIAN_POINT('Ctrl Pts',(0.00409853713230981,-0.034529677707698,
0.0700402961586851));
#75964=CARTESIAN_POINT('Ctrl Pts',(0.00401532797498495,-0.034364806625142,
0.0701252355425959));
#75965=CARTESIAN_POINT('Ctrl Pts',(0.00384772818185842,-0.0346945769586932,
0.0699410378841248));
#75966=CARTESIAN_POINT('Ctrl Pts',(0.00376071086827876,-0.034529677707698,
0.0700294422751687));
#75967=CARTESIAN_POINT('Ctrl Pts',(0.00367742174462465,-0.034364806625142,
0.0701213676312973));
#75968=CARTESIAN_POINT('',(0.00383874751920677,-0.0346775396664962,0.0699501812138163));
#75969=CARTESIAN_POINT('',(0.00384772818185601,-0.0346945769586886,0.0699410378841272));
#75970=CARTESIAN_POINT('Origin',(0.0158015436411093,-0.0345626618350802,
0.0814612371772208));
#75971=CARTESIAN_POINT('Ctrl Pts',(0.00383874752096816,-0.0346775396670097,
0.0699501812133703));
#75972=CARTESIAN_POINT('Ctrl Pts',(0.00386942708161475,-0.0346269749928192,
0.0699802506358189));
#75973=CARTESIAN_POINT('Ctrl Pts',(0.00389956142315404,-0.0345757902890796,
0.0700097856318815));
#75974=CARTESIAN_POINT('Ctrl Pts',(0.00395876436476409,-0.0344721681088223,
0.0700678112181175));
#75975=CARTESIAN_POINT('Ctrl Pts',(0.0039878097505526,-0.0344197714290205,
0.0700962790635588));
#75976=CARTESIAN_POINT('Ctrl Pts',(0.00401632040129074,-0.0343667727830579,
0.0701242227296687));
#75977=CARTESIAN_POINT('',(0.00401645699655423,-0.0346945769587026,0.0699499531747524));
#75978=CARTESIAN_POINT('Origin',(0.00812378219310841,-0.0315241814719618,
0.07415));
#75979=CARTESIAN_POINT('',(0.00383874751953099,-0.0347116136489621,0.0699501812151688));
#75980=CARTESIAN_POINT('',(0.00382978640553166,-0.0346945769586885,0.0699593437057787));
#75981=CARTESIAN_POINT('Origin',(0.0158319003503651,-0.0345626685753207,
0.0814275957869821));
#75982=CARTESIAN_POINT('Origin',(0.0155877516718174,-0.0345626627740259,
0.0816793705041721));
#75983=CARTESIAN_POINT('Origin',(0.0155547234227488,-0.0345626695951028,
0.0817103933327597));
#75984=CARTESIAN_POINT('Ctrl Pts',(0.0041324671762908,-0.0352450361874068,
0.070008965459918));
#75985=CARTESIAN_POINT('Ctrl Pts',(0.00397628549578934,-0.0349452760959493,
0.0701595003759405));
#75986=CARTESIAN_POINT('Ctrl Pts',(0.00383188641681499,-0.034644428984174,
0.0703213718813314));
#75987=CARTESIAN_POINT('Ctrl Pts',(0.00413068846890791,-0.0352450361874068,
0.0700107576164531));
#75988=CARTESIAN_POINT('Ctrl Pts',(0.00397457438069932,-0.0349452760959493,
0.0701613596175253));
#75989=CARTESIAN_POINT('Ctrl Pts',(0.00383024775511567,-0.034644428984174,
0.0703232929260563));
#75990=CARTESIAN_POINT('Ctrl Pts',(0.00395457882703833,-0.0352450361874068,
0.070188198857546));
#75991=CARTESIAN_POINT('Ctrl Pts',(0.00380515704505319,-0.0349452760959493,
0.0703454429427528));
#75992=CARTESIAN_POINT('Ctrl Pts',(0.0036680040225097,-0.034644428984174,
0.0705134953740692));
#75993=CARTESIAN_POINT('Ctrl Pts',(0.00395281773061963,-0.0352450361874068,
0.0701899732699569));
#75994=CARTESIAN_POINT('Ctrl Pts',(0.00380346287169672,-0.0349452760959493,
0.0703472837760051));
#75995=CARTESIAN_POINT('Ctrl Pts',(0.00366638158518364,-0.034644428984174,
0.0705153973985493));
#75996=CARTESIAN_POINT('',(0.00392981481673165,-0.0351951634053275,0.0702144199984733));
#75997=CARTESIAN_POINT('',(0.00377164489264186,-0.0348678972925388,0.0703900763414813));
#75998=CARTESIAN_POINT('Origin',(0.0167217537595203,-0.0345636767885282,
0.0810204736003928));
#75999=CARTESIAN_POINT('Origin',(-0.00458993218393289,-0.034694619934112,
0.0631662949218706));
#76000=CARTESIAN_POINT('',(0.00385439109183824,-0.0346945769330288,0.0702963751321229));
#76001=CARTESIAN_POINT('',(0.00381353200411445,-0.0346945769458128,0.0703436698045289));
#76002=CARTESIAN_POINT('',(0.00401632040137605,-0.0350221583435276,0.0701242227297751));
#76003=CARTESIAN_POINT('Origin',(0.0164400139611837,-0.0345628458716476,
0.0814100452612684));
#76004=CARTESIAN_POINT('',(0.00401720586740456,-0.035195136029876,0.0701250863516008));
#76005=CARTESIAN_POINT('Origin',(-0.00385224485374814,-0.0351951838366788,
0.0624121369015669));
#76006=CARTESIAN_POINT('',(0.00392979440494988,-0.0351951371328751,0.0702144452190176));
#76007=CARTESIAN_POINT('Ctrl Pts',(0.00400665887906221,-0.0350241211494343,
0.0697854501243585));
#76008=CARTESIAN_POINT('Ctrl Pts',(0.00394653899406037,-0.0349144232818962,
0.0698421618099233));
#76009=CARTESIAN_POINT('Ctrl Pts',(0.00388755539547412,-0.0348045283579412,
0.0699001501611477));
#76010=CARTESIAN_POINT('Ctrl Pts',(0.00382978639776993,-0.0346945769439158,
0.0699593437137317));
#76011=CARTESIAN_POINT('Ctrl Pts',(0.00401023147680345,-0.0350241211494343,
0.0698987125556777));
#76012=CARTESIAN_POINT('Ctrl Pts',(0.00395167173535362,-0.0349144232818962,
0.0699553750301733));
#76013=CARTESIAN_POINT('Ctrl Pts',(0.00389424819691255,-0.0348045283579412,
0.0700132818915915));
#76014=CARTESIAN_POINT('Ctrl Pts',(0.00383803717382372,-0.0346945769439158,
0.070072361705651));
#76015=CARTESIAN_POINT('Ctrl Pts',(0.00401380407454468,-0.0350241211494343,
0.0700119749869968));
#76016=CARTESIAN_POINT('Ctrl Pts',(0.00395680447664688,-0.0349144232818962,
0.0700685882504234));
#76017=CARTESIAN_POINT('Ctrl Pts',(0.00390094099835097,-0.0348045283579412,
0.0701264136220353));
#76018=CARTESIAN_POINT('Ctrl Pts',(0.00384628794987751,-0.0346945769439158,
0.0701853796975702));
#76019=CARTESIAN_POINT('Ctrl Pts',(0.00401737667228592,-0.0350241211494343,
0.070125237418316));
#76020=CARTESIAN_POINT('Ctrl Pts',(0.00396193721794013,-0.0349144232818962,
0.0701818014706735));
#76021=CARTESIAN_POINT('Ctrl Pts',(0.00390763379978939,-0.0348045283579412,
0.070239545352479));
#76022=CARTESIAN_POINT('Ctrl Pts',(0.00385453872593129,-0.0346945769439158,
0.0702983976894894));
#76023=CARTESIAN_POINT('',(0.00384208874882424,-0.0346945769458128,0.0701278594186829));
#76024=CARTESIAN_POINT('Ctrl Pts',(0.00383874752187396,-0.03471161364928,
0.0699501812174652));
#76025=CARTESIAN_POINT('Ctrl Pts',(0.00386941488997327,-0.0347621546532222,
0.0699802387078791));
#76026=CARTESIAN_POINT('Ctrl Pts',(0.00389954304286951,-0.0348133084096866,
0.0700097677063879));
#76027=CARTESIAN_POINT('Ctrl Pts',(0.00395874606227251,-0.034916856154457,
0.0700677933635758));
#76028=CARTESIAN_POINT('Ctrl Pts',(0.00398779744593243,-0.0349692089015913,
0.0700962670064083));
#76029=CARTESIAN_POINT('Ctrl Pts',(0.00401632040138823,-0.0350221583435,
0.070124222729815));
#76030=CARTESIAN_POINT('Ctrl Pts',(0.00393125734856887,-0.0351951371254888,
0.070214430526322));
#76031=CARTESIAN_POINT('Ctrl Pts',(0.00384989191896045,-0.0350307338980916,
0.0703011083470038));
#76032=CARTESIAN_POINT('Ctrl Pts',(0.00377217850349031,-0.0348659306897799,
0.070391075022998));
#76033=CARTESIAN_POINT('Ctrl Pts',(0.00392979440503568,-0.0351951371254888,
0.0702144452190959));
#76034=CARTESIAN_POINT('Ctrl Pts',(0.00384842927919115,-0.0350307338980916,
0.0703011532852173));
#76035=CARTESIAN_POINT('Ctrl Pts',(0.00377071741730197,-0.0348659306897799,
0.0703911501682518));
#76036=CARTESIAN_POINT('Ctrl Pts',(0.00368460354412518,-0.0351951371254888,
0.0702169077433135));
#76037=CARTESIAN_POINT('Ctrl Pts',(0.0036032893294238,-0.0350307338980916,
0.0703086849766463));
#76038=CARTESIAN_POINT('Ctrl Pts',(0.00352583784932513,-0.0348659306897799,
0.070403744591106));
#76039=CARTESIAN_POINT('Origin',(-0.000252701167597929,-0.0308609197411073,
0.0669133399892798));
#76040=CARTESIAN_POINT('',(0.00382289671799627,-0.0351951371254888,0.0702155188241323));
#76041=CARTESIAN_POINT('Origin',(0.00894792665521693,-0.0351840467441147,
0.0746749109977826));
#76042=CARTESIAN_POINT('Origin',(-0.0014300780706032,-0.0352322613594373,
0.066946369667333));
#76043=CARTESIAN_POINT('',(0.00362067005566337,-0.0351951142564653,0.0705723197933546));
#76044=CARTESIAN_POINT('',(0.00354522700977118,-0.0351951372916786,0.0706715905311282));
#76045=CARTESIAN_POINT('Origin',(0.00809048848650377,-0.0352875122426966,
0.0744889700069903));
#76046=CARTESIAN_POINT('Origin',(0.0137225858292214,-0.0298325076521994,
0.0691551438332945));
#76047=CARTESIAN_POINT('Origin',(0.00384922868754202,-0.0338732835503703,
0.0669405297094214));
#76048=CARTESIAN_POINT('Ctrl Pts',(0.00658393265112485,-0.0321934096636942,
0.0686086103608062));
#76049=CARTESIAN_POINT('Ctrl Pts',(0.00648474441538785,-0.0320508460843686,
0.0686361729343328));
#76050=CARTESIAN_POINT('Ctrl Pts',(0.00638637151987351,-0.0319086045661796,
0.068666379717769));
#76051=CARTESIAN_POINT('Ctrl Pts',(0.00628902042419258,-0.0317669892865994,
0.0686991482327426));
#76052=CARTESIAN_POINT('Ctrl Pts',(0.00650365324717335,-0.0321934096636942,
0.0686328105659513));
#76053=CARTESIAN_POINT('Ctrl Pts',(0.00640489818358434,-0.0320508460843686,
0.0686618101025796));
#76054=CARTESIAN_POINT('Ctrl Pts',(0.00630699674196796,-0.0319086045661796,
0.0686934411271617));
#76055=CARTESIAN_POINT('Ctrl Pts',(0.00621015411434681,-0.0317669892865994,
0.068727618178255));
#76056=CARTESIAN_POINT('Ctrl Pts',(0.00642337384322185,-0.0321934096636942,
0.0686570107710964));
#76057=CARTESIAN_POINT('Ctrl Pts',(0.00632505195178082,-0.0320508460843686,
0.0686874472708264));
#76058=CARTESIAN_POINT('Ctrl Pts',(0.0062276219640624,-0.0319086045661796,
0.0687205025365546));
#76059=CARTESIAN_POINT('Ctrl Pts',(0.00613128780450104,-0.0317669892865994,
0.0687560881237672));
#76060=CARTESIAN_POINT('Ctrl Pts',(0.00634309443927034,-0.0321934096636942,
0.0686812109762414));
#76061=CARTESIAN_POINT('Ctrl Pts',(0.0062452057199773,-0.0320508460843686,
0.0687130844390733));
#76062=CARTESIAN_POINT('Ctrl Pts',(0.00614824718615683,-0.0319086045661796,
0.0687475639459472));
#76063=CARTESIAN_POINT('Ctrl Pts',(0.00605242149465527,-0.0317669892865994,
0.0687845580692796));
#76064=CARTESIAN_POINT('',(0.00634453065367179,-0.0321934096636942,0.0686807780297913));
#76065=CARTESIAN_POINT('',(0.00612133224141135,-0.0318665617511261,0.0687584956477846));
#76066=CARTESIAN_POINT('Origin',(0.0109256371654381,-0.0326371944421567,
0.0847503569909728));
#76067=CARTESIAN_POINT('Origin',(0.00230497730286294,-0.0316939261509612,
0.058483135554525));
#76068=CARTESIAN_POINT('',(0.00646357948906075,-0.0320197221621857,0.0686435205305022));
#76069=CARTESIAN_POINT('Ctrl Pts',(0.00646339462907598,-0.0320197392094775,
0.068643526985331));
#76070=CARTESIAN_POINT('Ctrl Pts',(0.00643537593764299,-0.0319792716576073,
0.0686519756159989));
#76071=CARTESIAN_POINT('Ctrl Pts',(0.00640729410342048,-0.0319386439829724,
0.0686606763112761));
#76072=CARTESIAN_POINT('Ctrl Pts',(0.00637912214882976,-0.0318979099381656,
0.0686696462838884));
#76073=CARTESIAN_POINT('Ctrl Pts',(0.00635095075107656,-0.0318571766984944,
0.0686786160792031));
#76074=CARTESIAN_POINT('Ctrl Pts',(0.00632283188141053,-0.0318163871833579,
0.0686878078531429));
#76075=CARTESIAN_POINT('Ctrl Pts',(0.00629486116310049,-0.0317755399638302,
0.0686971866429181));
#76076=CARTESIAN_POINT('',(0.00646421107987872,-0.0321934096636183,0.0686447003968781));
#76077=CARTESIAN_POINT('Origin',(0.00577732083413186,-0.032411512718906,
0.0664390070771916));
#76078=CARTESIAN_POINT('',(0.00640437086678525,-0.0321934096636663,0.0686627392133447));
#76079=CARTESIAN_POINT('Ctrl Pts',(0.00634631772202925,-0.0321934096636618,
0.0686817372347041));
#76080=CARTESIAN_POINT('Ctrl Pts',(0.00627090611678108,-0.0320835708272592,
0.0687062498550351));
#76081=CARTESIAN_POINT('Ctrl Pts',(0.00619604554073242,-0.0319739230346489,
0.0687323088963013));
#76082=CARTESIAN_POINT('Ctrl Pts',(0.00612182921398835,-0.0318646057455573,
0.0687598736670035));
#76083=CARTESIAN_POINT('Ctrl Pts',(0.00624647239931037,-0.0321934096636618,
0.0686281454788485));
#76084=CARTESIAN_POINT('Ctrl Pts',(0.00617032172198197,-0.0320835708272592,
0.0686540350439947));
#76085=CARTESIAN_POINT('Ctrl Pts',(0.00609475099834633,-0.0319739230346489,
0.0686814855264505));
#76086=CARTESIAN_POINT('Ctrl Pts',(0.00601985422046366,-0.0318646057455573,
0.0687104543847327));
#76087=CARTESIAN_POINT('Ctrl Pts',(0.00614662707659148,-0.0321934096636618,
0.0685745537229929));
#76088=CARTESIAN_POINT('Ctrl Pts',(0.00606973732718286,-0.0320835708272592,
0.0686018202329543));
#76089=CARTESIAN_POINT('Ctrl Pts',(0.00599345645596023,-0.0319739230346489,
0.0686306621565996));
#76090=CARTESIAN_POINT('Ctrl Pts',(0.00591787922693896,-0.0318646057455573,
0.0686610351024619));
#76091=CARTESIAN_POINT('Ctrl Pts',(0.00604678175387259,-0.0321934096636618,
0.0685209619671374));
#76092=CARTESIAN_POINT('Ctrl Pts',(0.00596915293238375,-0.0320835708272592,
0.0685496054219139));
#76093=CARTESIAN_POINT('Ctrl Pts',(0.00589216191357413,-0.0319739230346489,
0.0685798387867487));
#76094=CARTESIAN_POINT('Ctrl Pts',(0.00581590423341427,-0.0318646057455573,
0.0686116158201911));
#76095=CARTESIAN_POINT('',(0.00603476276665501,-0.0321763980308453,0.0685254113205008));
#76096=CARTESIAN_POINT('',(0.00604678175384193,-0.0321934096636184,0.0685209619671487));
#76097=CARTESIAN_POINT('Origin',(0.0112170931696844,-0.032638623146326,
0.0842406758194546));
#76098=CARTESIAN_POINT('Ctrl Pts',(0.00603476276775469,-0.0321763980306276,
0.0685254113234703));
#76099=CARTESIAN_POINT('Ctrl Pts',(0.00604970583476894,-0.0321259596174849,
0.0685656448438009));
#76100=CARTESIAN_POINT('Ctrl Pts',(0.00606438999376357,-0.0320749164631446,
0.0686051812661828));
#76101=CARTESIAN_POINT('Ctrl Pts',(0.00609325231302661,-0.0319716057793892,
0.0686828917326989));
#76102=CARTESIAN_POINT('Ctrl Pts',(0.00610741922756306,-0.0319193786690082,
0.0687210354982171));
#76103=CARTESIAN_POINT('Ctrl Pts',(0.00612133224205194,-0.0318665617525264,
0.068758495649521));
#76104=CARTESIAN_POINT('',(0.00619565620376686,-0.0321934096636664,0.06860086999848));
#76105=CARTESIAN_POINT('Origin',(0.00812378219310841,-0.0315241814719618,
0.07415));
#76106=CARTESIAN_POINT('',(0.00603476276652569,-0.0322104233323623,0.0685254113201528));
#76107=CARTESIAN_POINT('',(0.00602275330948016,-0.0321934096636183,0.0685298863329836));
#76108=CARTESIAN_POINT('Origin',(0.011261375913722,-0.0326387234006215,
0.0842309679557854));
#76109=CARTESIAN_POINT('Origin',(0.0123673288377802,-0.0326386243116258,
0.0838134712769871));
#76110=CARTESIAN_POINT('Origin',(0.0123274431598962,-0.0326387243621781,
0.0838350188156792));
#76111=CARTESIAN_POINT('Ctrl Pts',(0.00627316950654523,-0.0327445246967097,
0.0687045103356693));
#76112=CARTESIAN_POINT('Ctrl Pts',(0.00606778950634687,-0.032443687833936,
0.0687743073341694));
#76113=CARTESIAN_POINT('Ctrl Pts',(0.00586825036422881,-0.0321434074405927,
0.0688593761077817));
#76114=CARTESIAN_POINT('Ctrl Pts',(0.00603826925914547,-0.0327445246967097,
0.0687900782839417));
#76115=CARTESIAN_POINT('Ctrl Pts',(0.00583611650687456,-0.032443687833936,
0.0688687346901042));
#76116=CARTESIAN_POINT('Ctrl Pts',(0.00564046277120741,-0.0321434074405927,
0.0689623946132334));
#76117=CARTESIAN_POINT('',(0.00600462631127269,-0.0326943950436611,0.0688032904185394));
#76118=CARTESIAN_POINT('',(0.0057867482592627,-0.0323666188837389,0.0688948694219787));
#76119=CARTESIAN_POINT('Origin',(0.0122694182553645,-0.0326395579111418,
0.0844033045251258));
#76120=CARTESIAN_POINT('Origin',(0.00129882962827823,-0.0321933825602991,
0.0588031917507565));
#76121=CARTESIAN_POINT('',(0.00590151528279517,-0.0321934096532688,0.0688453176555126));
#76122=CARTESIAN_POINT('',(0.00584440778819952,-0.0321934096584275,0.0688707141987171));
#76123=CARTESIAN_POINT('',(0.00612133224107911,-0.0325210109756238,0.0687584956468886));
#76124=CARTESIAN_POINT('Origin',(0.0118137036797941,-0.0326393129158326,
0.0845566298508461));
#76125=CARTESIAN_POINT('',(0.00612180524213315,-0.0326943950436593,0.0687597691804743));
#76126=CARTESIAN_POINT('Origin',(0.00227019204011562,-0.0326943765538122,
0.0583894754321644));
#76127=CARTESIAN_POINT('',(0.00606321577671292,-0.0326943950436702,0.0687815297995169));
#76128=CARTESIAN_POINT('Ctrl Pts',(0.006256833647866,-0.0325229783203769,
0.068447851007783));
#76129=CARTESIAN_POINT('Ctrl Pts',(0.00617822964870606,-0.032413025309245,
0.0684735868526517));
#76130=CARTESIAN_POINT('Ctrl Pts',(0.00610016995039386,-0.0323031222208069,
0.0685009448188719));
#76131=CARTESIAN_POINT('Ctrl Pts',(0.00602275330527986,-0.0321934096576658,
0.0685298863345538));
#76132=CARTESIAN_POINT('Ctrl Pts',(0.00621184141320569,-0.0325229783203769,
0.0685518550512456));
#76133=CARTESIAN_POINT('Ctrl Pts',(0.00613467110751046,-0.032413025309245,
0.0685782111130852));
#76134=CARTESIAN_POINT('Ctrl Pts',(0.00605805771520003,-0.0323031222208069,
0.0686061595444171));
#76135=CARTESIAN_POINT('Ctrl Pts',(0.00598209810932082,-0.0321934096576658,
0.0686356610823807));
#76136=CARTESIAN_POINT('Ctrl Pts',(0.00616684917854538,-0.0325229783203769,
0.0686558590947081));
#76137=CARTESIAN_POINT('Ctrl Pts',(0.00609111256631486,-0.032413025309245,
0.0686828353735186));
#76138=CARTESIAN_POINT('Ctrl Pts',(0.00601594548000621,-0.0323031222208069,
0.0687113742699624));
#76139=CARTESIAN_POINT('Ctrl Pts',(0.00594144291336179,-0.0321934096576658,
0.0687414358302075));
#76140=CARTESIAN_POINT('Ctrl Pts',(0.00612185694388507,-0.0325229783203769,
0.0687598631381707));
#76141=CARTESIAN_POINT('Ctrl Pts',(0.00604755402511927,-0.032413025309245,
0.0687874596339521));
#76142=CARTESIAN_POINT('Ctrl Pts',(0.00597383324481239,-0.0323031222208069,
0.0688165889955077));
#76143=CARTESIAN_POINT('Ctrl Pts',(0.00590078771740276,-0.0321934096576658,
0.0688472105780344));
#76144=CARTESIAN_POINT('',(0.00596213429654121,-0.0321934096584274,0.0686876019939325));
#76145=CARTESIAN_POINT('Ctrl Pts',(0.00603476276773177,-0.0322104233328937,
0.0685254113234084));
#76146=CARTESIAN_POINT('Ctrl Pts',(0.00604972608283879,-0.0322609421831202,
0.0685656993607969));
#76147=CARTESIAN_POINT('Ctrl Pts',(0.00606442013335418,-0.0323120888240375,
0.0686052624156628));
#76148=CARTESIAN_POINT('Ctrl Pts',(0.00609328267115004,-0.0324156524631816,
0.0686829734705684));
#76149=CARTESIAN_POINT('Ctrl Pts',(0.00610743929439966,-0.0324680267167313,
0.068721089527251));
#76150=CARTESIAN_POINT('Ctrl Pts',(0.00612133224109001,-0.0325210109755912,
0.0687584956469308));
#76151=CARTESIAN_POINT('Origin',(0.0157756005763264,-0.0262834582512467,
0.0723188633945439));
#76152=CARTESIAN_POINT('Origin',(0.00943677067931257,-0.0342770989687757,
0.0620627815514928));
#76153=CARTESIAN_POINT('Ctrl Pts',(0.0060064696347242,-0.0326943950436604,
0.0688041353146785));
#76154=CARTESIAN_POINT('Ctrl Pts',(0.00593279360014221,-0.0325844576448134,
0.0688333158499997));
#76155=CARTESIAN_POINT('Ctrl Pts',(0.00585971585270536,-0.0324744968375322,
0.0688640221916614));
#76156=CARTESIAN_POINT('Ctrl Pts',(0.00578732948123054,-0.0323646534831894,
0.0688962137054484));
#76157=CARTESIAN_POINT('Ctrl Pts',(0.0059034564288931,-0.0326943950436604,
0.0687569187179587));
#76158=CARTESIAN_POINT('Ctrl Pts',(0.00582912966111497,-0.0325844576448134,
0.0687875189683235));
#76159=CARTESIAN_POINT('Ctrl Pts',(0.00575543049646335,-0.0324744968375322,
0.0688196585837337));
#76160=CARTESIAN_POINT('Ctrl Pts',(0.0056824527946217,-0.0323646534831894,
0.0688532950825982));
#76161=CARTESIAN_POINT('Ctrl Pts',(0.00580044322306199,-0.0326943950436604,
0.0687097021212388));
#76162=CARTESIAN_POINT('Ctrl Pts',(0.00572546572208774,-0.0325844576448134,
0.0687417220866473));
#76163=CARTESIAN_POINT('Ctrl Pts',(0.00565114514022135,-0.0324744968375322,
0.068775294975806));
#76164=CARTESIAN_POINT('Ctrl Pts',(0.00557757610801285,-0.0323646534831894,
0.068810376459748));
#76165=CARTESIAN_POINT('Ctrl Pts',(0.00569743001723089,-0.0326943950436604,
0.0686624855245189));
#76166=CARTESIAN_POINT('Ctrl Pts',(0.0056218017830605,-0.0325844576448134,
0.0686959252049712));
#76167=CARTESIAN_POINT('Ctrl Pts',(0.00554685978397934,-0.0324744968375322,
0.0687309313678783));
#76168=CARTESIAN_POINT('Ctrl Pts',(0.00547269942140401,-0.0323646534831894,
0.0687674578368979));
#76169=CARTESIAN_POINT('',(0.00568571412389441,-0.0326773559991155,0.0686676807763526));
#76170=CARTESIAN_POINT('',(0.00569743001723023,-0.0326943950436594,0.0686624855245192));
#76171=CARTESIAN_POINT('Origin',(0.0124790316359852,-0.0326395670859815,
0.0838197150605463));
#76172=CARTESIAN_POINT('Ctrl Pts',(0.0056857141252513,-0.0326773559987418,
0.0686676807794101));
#76173=CARTESIAN_POINT('Ctrl Pts',(0.00570316802359972,-0.0326267922586007,
0.0687069281833901));
#76174=CARTESIAN_POINT('Ctrl Pts',(0.00572031256420384,-0.0325756109579419,
0.068745479955476));
#76175=CARTESIAN_POINT('Ctrl Pts',(0.00575399752078182,-0.0324719985462368,
0.0688212250453391));
#76176=CARTESIAN_POINT('Ctrl Pts',(0.00577052442663532,-0.0324196091621779,
0.0688583879838198));
#76177=CARTESIAN_POINT('Ctrl Pts',(0.00578674825928252,-0.0323666188837756,
0.0688948694220232));
#76178=CARTESIAN_POINT('',(0.00585102816426146,-0.0326943950436702,0.0687328879715393));
#76179=CARTESIAN_POINT('Origin',(0.00812378219310841,-0.0315241814719618,
0.07415));
#76180=CARTESIAN_POINT('',(0.00568571412391236,-0.0327114338379881,0.0686676807763931));
#76181=CARTESIAN_POINT('',(0.00567400935308163,-0.0326943950436593,0.0686729010386623));
#76182=CARTESIAN_POINT('Origin',(0.0125201122070344,-0.0326395669401792,
0.0838005981465262));
#76183=CARTESIAN_POINT('Origin',(0.0123872216574439,-0.0326395679064938,
0.0838605466837996));
#76184=CARTESIAN_POINT('Origin',(0.0123455098264391,-0.0326395678140561,
0.0838782439513655));
#76185=CARTESIAN_POINT('Ctrl Pts',(0.00593485987093565,-0.0332451089994433,
0.0688314716257697));
#76186=CARTESIAN_POINT('Ctrl Pts',(0.00573426829145138,-0.0329451141710254,
0.0689140281818464));
#76187=CARTESIAN_POINT('Ctrl Pts',(0.00554046506877148,-0.0326442513127493,
0.0690114595812519));
#76188=CARTESIAN_POINT('Ctrl Pts',(0.00570579668445249,-0.0332451089994433,
0.068931621796005));
#76189=CARTESIAN_POINT('Ctrl Pts',(0.00550898233043731,-0.0329451141710254,
0.0690228176115056));
#76190=CARTESIAN_POINT('Ctrl Pts',(0.00531959634686495,-0.0326442513127493,
0.0691285792110471));
#76191=CARTESIAN_POINT('Ctrl Pts',(0.00570350605258766,-0.0332451089994433,
0.0689326232977073));
#76192=CARTESIAN_POINT('Ctrl Pts',(0.00550672947082717,-0.0329451141710254,
0.0690239055058022));
#76193=CARTESIAN_POINT('Ctrl Pts',(0.00531738765964588,-0.0326442513127493,
0.0691297504073451));
#76194=CARTESIAN_POINT('',(0.00567308530893743,-0.0331951640388616,0.0689469038273432));
#76195=CARTESIAN_POINT('',(0.00546138746752985,-0.0328677532354987,0.0690519827976921));
#76196=CARTESIAN_POINT('Origin',(0.0135036309031346,-0.0326402808279522,
0.0837696837008342));
#76197=CARTESIAN_POINT('Origin',(0.00034307225992035,-0.0326944278779019,
0.0592521240019454));
#76198=CARTESIAN_POINT('',(0.00557281665257838,-0.0326943950436593,0.0689953225308435));
#76199=CARTESIAN_POINT('',(0.00551741651134116,-0.0326943950436694,0.0690242547680603));
#76200=CARTESIAN_POINT('',(0.00578674825926528,-0.0330220786163545,0.0688948694219775));
#76201=CARTESIAN_POINT('Origin',(0.0130929182019664,-0.032639668276383,
0.0840196191375121));
#76202=CARTESIAN_POINT('',(0.00578730029279678,-0.0331951640388587,0.068896110742553));
#76203=CARTESIAN_POINT('Origin',(0.00130464766631461,-0.0331952026560022,
0.0588162697243794));
#76204=CARTESIAN_POINT('',(0.0057301928008771,-0.0331951640388701,0.0689215072849581));
#76205=CARTESIAN_POINT('Ctrl Pts',(0.00590247585408771,-0.0330240426238172,
0.0685763299211161));
#76206=CARTESIAN_POINT('Ctrl Pts',(0.00582569311858744,-0.0329142774063519,
0.06860693058005));
#76207=CARTESIAN_POINT('Ctrl Pts',(0.00574950470519212,-0.0328043479726691,
0.0686391338081532));
#76208=CARTESIAN_POINT('Ctrl Pts',(0.00567400935308162,-0.0326943950436593,
0.0686729010386623));
#76209=CARTESIAN_POINT('Ctrl Pts',(0.00586410289566394,-0.0330240426238172,
0.0686829538023354));
#76210=CARTESIAN_POINT('Ctrl Pts',(0.00578878900800608,-0.0329142774063519,
0.0687140830861565));
#76211=CARTESIAN_POINT('Ctrl Pts',(0.00571408110288044,-0.0328043479726691,
0.0687467848374978));
#76212=CARTESIAN_POINT('Ctrl Pts',(0.00564007604041373,-0.0326943950436593,
0.0687810197987173));
#76213=CARTESIAN_POINT('Ctrl Pts',(0.00582572993724016,-0.0330240426238172,
0.0687895776835547));
#76214=CARTESIAN_POINT('Ctrl Pts',(0.00575188489742471,-0.0329142774063519,
0.068821235592263));
#76215=CARTESIAN_POINT('Ctrl Pts',(0.00567865750056877,-0.0328043479726691,
0.0688544358668425));
#76216=CARTESIAN_POINT('Ctrl Pts',(0.00560614272774585,-0.0326943950436593,
0.0688891385587724));
#76217=CARTESIAN_POINT('Ctrl Pts',(0.00578735697881639,-0.0330240426238172,
0.068896201564774));
#76218=CARTESIAN_POINT('Ctrl Pts',(0.00571498078684335,-0.0329142774063519,
0.0689283880983696));
#76219=CARTESIAN_POINT('Ctrl Pts',(0.00564323389825709,-0.0328043479726691,
0.0689620868961871));
#76220=CARTESIAN_POINT('Ctrl Pts',(0.00557220941507797,-0.0326943950436593,
0.0689972573188274));
#76221=CARTESIAN_POINT('',(0.00562341300284001,-0.0326943950436694,0.0688341117847629));
#76222=CARTESIAN_POINT('Ctrl Pts',(0.00568571412525445,-0.0327114338383335,
0.068667680779417));
#76223=CARTESIAN_POINT('Ctrl Pts',(0.00570316512044694,-0.0327619876830919,
0.068706921655266));
#76224=CARTESIAN_POINT('Ctrl Pts',(0.00572030824301397,-0.0328131562604212,
0.0687454702387077));
#76225=CARTESIAN_POINT('Ctrl Pts',(0.00575399316865828,-0.0329167375858774,
0.0688212152590123));
#76226=CARTESIAN_POINT('Ctrl Pts',(0.00577052154991993,-0.0329691088920632,
0.0688583815151439));
#76227=CARTESIAN_POINT('Ctrl Pts',(0.00578674825928208,-0.0330220786163186,
0.0688948694220221));
#76228=CARTESIAN_POINT('Ctrl Pts',(0.00567497834865205,-0.0331951640388604,
0.0689476314291769));
#76229=CARTESIAN_POINT('Ctrl Pts',(0.00556742271389869,-0.033030642201062,
0.068998258878634));
#76230=CARTESIAN_POINT('Ctrl Pts',(0.00546205147040875,-0.0328657861914645,
0.0690532884547829));
#76231=CARTESIAN_POINT('Ctrl Pts',(0.00567308530894032,-0.0331951640388604,
0.0689469038273419));
#76232=CARTESIAN_POINT('Ctrl Pts',(0.00556551463148551,-0.033030642201062,
0.0689975704141814));
#76233=CARTESIAN_POINT('Ctrl Pts',(0.00546012997573719,-0.0328657861914645,
0.0690526397160007));
#76234=CARTESIAN_POINT('Ctrl Pts',(0.00535765398416284,-0.0331951640388604,
0.0688256657945171));
#76235=CARTESIAN_POINT('Ctrl Pts',(0.00524757678810997,-0.033030642201062,
0.0688828537217605));
#76236=CARTESIAN_POINT('Ctrl Pts',(0.00513995728942306,-0.0328657861914645,
0.0689445423885937));
#76237=CARTESIAN_POINT('',(0.00534628742199613,-0.0331781648281888,0.0688315864402821));
#76238=CARTESIAN_POINT('',(0.00535765398416181,-0.0331951640388588,0.0688256657945176));
#76239=CARTESIAN_POINT('Origin',(0.0136189663352319,-0.0326412092601028,
0.0831336584167454));
#76240=CARTESIAN_POINT('Ctrl Pts',(0.00534628742381383,-0.033178164828644,
0.0688315864405209));
#76241=CARTESIAN_POINT('Ctrl Pts',(0.00536618494568857,-0.0331276811546781,
0.0688696866661652));
#76242=CARTESIAN_POINT('Ctrl Pts',(0.00538572320991325,-0.033076566349779,
0.0689070989040707));
#76243=CARTESIAN_POINT('Ctrl Pts',(0.00542409786612605,-0.0329730614463308,
0.0689805796231364));
#76244=CARTESIAN_POINT('Ctrl Pts',(0.00544291875083521,-0.032920713337418,
0.0690166184221636));
#76245=CARTESIAN_POINT('Ctrl Pts',(0.00546138747588533,-0.0328677532289347,
0.0690519827834986));
#76246=CARTESIAN_POINT('',(0.00551536964655962,-0.0331951640388701,0.0688862848109404));
#76247=CARTESIAN_POINT('Origin',(0.00812378219310841,-0.0315241814719618,
0.07415));
#76248=CARTESIAN_POINT('',(0.00534628742214034,-0.0332121607144428,0.0688315864419558));
#76249=CARTESIAN_POINT('',(0.00533493353088822,-0.0331951640388587,0.0688375313516922));
#76250=CARTESIAN_POINT('Origin',(0.0136549253353356,-0.0326413651674531,
0.0831060325170448));
#76251=CARTESIAN_POINT('Origin',(0.0123562593090519,-0.0326412099775407,
0.0837930984558483));
#76252=CARTESIAN_POINT('Origin',(0.01231303860202,-0.0326413661134083,0.0838068188101578));
#76253=CARTESIAN_POINT('Ctrl Pts',(0.00557414628843926,-0.0336938721132646,
0.0689946281401935));
#76254=CARTESIAN_POINT('Ctrl Pts',(0.00546622319260924,-0.0335278710435224,
0.069048002485935));
#76255=CARTESIAN_POINT('Ctrl Pts',(0.00536001186947911,-0.0333620469224384,
0.0691047424949314));
#76256=CARTESIAN_POINT('Ctrl Pts',(0.00525546893502409,-0.0331951640388587,
0.0691648940520025));
#76257=CARTESIAN_POINT('Ctrl Pts',(0.00549983622149611,-0.0336938721132646,
0.0690334359200156));
#76258=CARTESIAN_POINT('Ctrl Pts',(0.00539272553180373,-0.0335278710435224,
0.0690883658805011));
#76259=CARTESIAN_POINT('Ctrl Pts',(0.00528737511268256,-0.0333620469224384,
0.0691466354801345));
#76260=CARTESIAN_POINT('Ctrl Pts',(0.00518374226268052,-0.0331951640388587,
0.0692082912212457));
#76261=CARTESIAN_POINT('Ctrl Pts',(0.00542552615455296,-0.0336938721132646,
0.0690722436998376));
#76262=CARTESIAN_POINT('Ctrl Pts',(0.00531922787099822,-0.0335278710435224,
0.0691287292750671));
#76263=CARTESIAN_POINT('Ctrl Pts',(0.005214738355886,-0.0333620469224384,
0.0691885284653376));
#76264=CARTESIAN_POINT('Ctrl Pts',(0.00511201559033694,-0.0331951640388587,
0.069251688390489));
#76265=CARTESIAN_POINT('Ctrl Pts',(0.00535121608760981,-0.0336938721132646,
0.0691110514796596));
#76266=CARTESIAN_POINT('Ctrl Pts',(0.00524573021019271,-0.0335278710435224,
0.0691690926696332));
#76267=CARTESIAN_POINT('Ctrl Pts',(0.00514210159908944,-0.0333620469224384,
0.0692304214505407));
#76268=CARTESIAN_POINT('Ctrl Pts',(0.00504028891799337,-0.0331951640388587,
0.0692950855597323));
#76269=CARTESIAN_POINT('',(0.00535121608757554,-0.0336938721132548,0.0691110514796784));
#76270=CARTESIAN_POINT('',(0.00514653394508866,-0.0333679846208662,0.069229215691045));
#76271=CARTESIAN_POINT('Ctrl Pts',(0.00535121608758644,-0.033693872113239,
0.0691110514796663));
#76272=CARTESIAN_POINT('Ctrl Pts',(0.00533154670769848,-0.0336629187933851,
0.0691218741058165));
#76273=CARTESIAN_POINT('Ctrl Pts',(0.00531194698936719,-0.033631995230099,
0.0691328084427585));
#76274=CARTESIAN_POINT('Ctrl Pts',(0.00524341592934891,-0.0335235892595403,
0.069171568059534));
#76275=CARTESIAN_POINT('Ctrl Pts',(0.00519477652140877,-0.0334458668645711,
0.0692000272619926));
#76276=CARTESIAN_POINT('Ctrl Pts',(0.00514653395765004,-0.0333679869902153,
0.0692292157118869));
#76277=CARTESIAN_POINT('Ctrl Pts',(0.00514653356476184,-0.0333679128829488,
0.0692292150600056));
#76278=CARTESIAN_POINT('Ctrl Pts',(0.0051467682263833,-0.0333391359256866,
0.0692296029078199));
#76279=CARTESIAN_POINT('Ctrl Pts',(0.00514694409275441,-0.0333103578181726,
0.0692298935790735));
#76280=CARTESIAN_POINT('Ctrl Pts',(0.00514706131756792,-0.0332815781851601,
0.0692300873277904));
#76281=CARTESIAN_POINT('Ctrl Pts',(0.00514717864297711,-0.0332527738550986,
0.0692302812427714));
#76282=CARTESIAN_POINT('Ctrl Pts',(0.00514723722102821,-0.0332239691713941,
0.06923037806034));
#76283=CARTESIAN_POINT('Ctrl Pts',(0.00514723722102868,-0.0331951640388599,
0.0692303780603397));
#76284=CARTESIAN_POINT('',(0.00525418552406561,-0.0331951640388587,0.0691656705609461));
#76285=CARTESIAN_POINT('',(0.00520071137255754,-0.0331951640388687,0.0691980243106526));
#76286=CARTESIAN_POINT('',(0.00546138748282756,-0.0335216366559765,0.0690519827968478));
#76287=CARTESIAN_POINT('Origin',(0.0142239882975866,-0.0326434571528019,
0.0832148741677039));
#76288=CARTESIAN_POINT('',(0.00546201637008394,-0.0336938721132327,0.0690531870052572));
#76289=CARTESIAN_POINT('Origin',(0.000406713303217545,-0.0336938867896339,
0.0593731693981297));
#76290=CARTESIAN_POINT('',(0.00540661622883974,-0.0336938721132538,0.0690821192424778));
#76291=CARTESIAN_POINT('Ctrl Pts',(0.00555688458612558,-0.0335235895815172,
0.0687268056760533));
#76292=CARTESIAN_POINT('Ctrl Pts',(0.00548222363896938,-0.0334144449262748,
0.0687621440753697));
#76293=CARTESIAN_POINT('Ctrl Pts',(0.0054082069801651,-0.0333049234473147,
0.0687990655132052));
#76294=CARTESIAN_POINT('Ctrl Pts',(0.00533493353088825,-0.0331951640388587,
0.0688375313516921));
#76295=CARTESIAN_POINT('Ctrl Pts',(0.0055252822893815,-0.0335235895815172,
0.0688356287771228));
#76296=CARTESIAN_POINT('Ctrl Pts',(0.0054521195064645,-0.0334144449262748,
0.0688714022442731));
#76297=CARTESIAN_POINT('Ctrl Pts',(0.00537961172128263,-0.0333049234473147,
0.0689087282988371));
#76298=CARTESIAN_POINT('Ctrl Pts',(0.00530785597249189,-0.0331951640388587,
0.0689475676107942));
#76299=CARTESIAN_POINT('Ctrl Pts',(0.00549367999263743,-0.0335235895815172,
0.0689444518781923));
#76300=CARTESIAN_POINT('Ctrl Pts',(0.00542201537395962,-0.0334144449262748,
0.0689806604131765));
#76301=CARTESIAN_POINT('Ctrl Pts',(0.00535101646240017,-0.0333049234473147,
0.0690183910844689));
#76302=CARTESIAN_POINT('Ctrl Pts',(0.00528077841409552,-0.0331951640388587,
0.0690576038698963));
#76303=CARTESIAN_POINT('Ctrl Pts',(0.00546207769589335,-0.0335235895815172,
0.0690532749792618));
#76304=CARTESIAN_POINT('Ctrl Pts',(0.00539191124145473,-0.0334144449262748,
0.0690899185820799));
#76305=CARTESIAN_POINT('Ctrl Pts',(0.0053224212035177,-0.0333049234473147,
0.0691280538701008));
#76306=CARTESIAN_POINT('Ctrl Pts',(0.00525370085569916,-0.0331951640388587,
0.0691676401289984));
#76307=CARTESIAN_POINT('',(0.00529455952748692,-0.0331951640388687,0.0690016009563292));
#76308=CARTESIAN_POINT('Ctrl Pts',(0.00534628742358526,-0.0332121607145988,
0.0688315864447267));
#76309=CARTESIAN_POINT('Ctrl Pts',(0.00536615146201264,-0.0332625444109202,
0.0688696225816059));
#76310=CARTESIAN_POINT('Ctrl Pts',(0.00538567321188656,-0.0333135300745695,
0.068907003296159));
#76311=CARTESIAN_POINT('Ctrl Pts',(0.00542404666424387,-0.0334167177151536,
0.068980481702462));
#76312=CARTESIAN_POINT('Ctrl Pts',(0.00544288636915261,-0.0334688874167339,
0.0690165564209686));
#76313=CARTESIAN_POINT('Ctrl Pts',(0.00546138748300939,-0.0335216366556671,
0.0690519827972136));
#76314=CARTESIAN_POINT('Ctrl Pts',(0.00535121608759359,-0.033693872113239,
0.0691110514796686));
#76315=CARTESIAN_POINT('Ctrl Pts',(0.00532172144980367,-0.0336474569764958,
0.0691272802291192));
#76316=CARTESIAN_POINT('Ctrl Pts',(0.00529241881100787,-0.033601104548885,
0.0691438531385406));
#76317=CARTESIAN_POINT('Ctrl Pts',(0.00521823126667602,-0.0334837508592656,
0.0691858119348449));
#76318=CARTESIAN_POINT('Ctrl Pts',(0.00514531962617555,-0.0333660264659097,
0.0692299506366928));
#76319=CARTESIAN_POINT('Ctrl Pts',(0.00502686006645084,-0.033693872113239,
0.0690092516229594));
#76320=CARTESIAN_POINT('Ctrl Pts',(0.00499676956031882,-0.0336474569764958,
0.0690273789358345));
#76321=CARTESIAN_POINT('Ctrl Pts',(0.00496689331909221,-0.033601104548885,
0.0690458572539809));
#76322=CARTESIAN_POINT('Ctrl Pts',(0.00489125354528501,-0.0334837508592655,
0.0690926401070958));
#76323=CARTESIAN_POINT('Ctrl Pts',(0.00481703325982658,-0.0333660264659097,
0.0691416437799547));
#76324=CARTESIAN_POINT('',(0.00501782222224344,-0.0336769361243753,0.069016481454267));
#76325=CARTESIAN_POINT('',(0.00502879459541034,-0.0336938721132327,0.0690098587791681));
#76326=CARTESIAN_POINT('Ctrl Pts',(0.00501782222224317,-0.033676936124375,
0.0690164814542672));
#76327=CARTESIAN_POINT('Ctrl Pts',(0.005019649909106,-0.0336797586669845,
0.0690153756391845));
#76328=CARTESIAN_POINT('Ctrl Pts',(0.00502147811739939,-0.0336825812712485,
0.0690142708419912));
#76329=CARTESIAN_POINT('Ctrl Pts',(0.00502513558148546,-0.0336882266105785,
0.0690120632799841));
#76330=CARTESIAN_POINT('Ctrl Pts',(0.00502696483725222,-0.03369104934558,
0.0690109605152117));
#76331=CARTESIAN_POINT('Ctrl Pts',(0.00502879459541793,-0.0336938721132295,
0.0690098587791725));
#76332=CARTESIAN_POINT('Ctrl Pts',(0.00501782222224345,-0.0336769361243754,
0.0690164814542671));
#76333=CARTESIAN_POINT('Ctrl Pts',(0.00503951824392448,-0.0336279031301476,
0.0690523405544207));
#76334=CARTESIAN_POINT('Ctrl Pts',(0.00506152641722645,-0.0335767851899352,
0.0690887155775568));
#76335=CARTESIAN_POINT('Ctrl Pts',(0.00510465089668413,-0.0334733198857318,
0.0691599915492846));
#76336=CARTESIAN_POINT('Ctrl Pts',(0.00512579615833764,-0.0334209645014078,
0.0691949403554103));
#76337=CARTESIAN_POINT('Ctrl Pts',(0.00514653396172319,-0.0333679869844681,
0.0692292157160962));
#76338=CARTESIAN_POINT('',(0.00519000534150295,-0.0336938721132538,0.0690604551294333));
#76339=CARTESIAN_POINT('Origin',(0.00812378219310841,-0.0315241814719618,
0.07415));
#76340=CARTESIAN_POINT('',(0.00501782222292022,-0.0337108120655555,0.0690164814553829));
#76341=CARTESIAN_POINT('',(0.00500686402026081,-0.0336938721132327,0.069023127551441));
#76342=CARTESIAN_POINT('Origin',(0.0125311601701808,-0.0345562516250795,
0.083593453341771));
#76343=CARTESIAN_POINT('Ctrl Pts',(0.00500686402026099,-0.0336938721132306,
0.0690231275514468));
#76344=CARTESIAN_POINT('Ctrl Pts',(0.0050086890615784,-0.0336910493355375,
0.0690220180047386));
#76345=CARTESIAN_POINT('Ctrl Pts',(0.00501051477127385,-0.0336882266055569,
0.0690209093863788));
#76346=CARTESIAN_POINT('Ctrl Pts',(0.00501416750820236,-0.0336825812712406,
0.0690186940186733));
#76347=CARTESIAN_POINT('Ctrl Pts',(0.00501599453538342,-0.0336797586669805,
0.069017587269348));
#76348=CARTESIAN_POINT('Ctrl Pts',(0.0050178222222437,-0.033676936124375,
0.0690164814542668));
#76349=CARTESIAN_POINT('Origin',(0.0144435748101146,-0.0345562517443326,
0.082436372141593));
#76350=CARTESIAN_POINT('Ctrl Pts',(0.00528559484861555,-0.034243627687391,
0.0691477187606492));
#76351=CARTESIAN_POINT('Ctrl Pts',(0.00509693070150552,-0.033943005420181,
0.0692547627609895));
#76352=CARTESIAN_POINT('Ctrl Pts',(0.00491686552216361,-0.0336441434784052,
0.0693757136171344));
#76353=CARTESIAN_POINT('Ctrl Pts',(0.00507088842474626,-0.034243627687391,
0.0692757857413635));
#76354=CARTESIAN_POINT('Ctrl Pts',(0.0048870544034395,-0.033943005420181,
0.0693909275279737));
#76355=CARTESIAN_POINT('Ctrl Pts',(0.00471241558646132,-0.0336441434784052,
0.0695195893405603));
#76356=CARTESIAN_POINT('Ctrl Pts',(0.00506874136050757,-0.034243627687391,
0.0692770664111706));
#76357=CARTESIAN_POINT('Ctrl Pts',(0.00488495564045884,-0.033943005420181,
0.0693922891756435));
#76358=CARTESIAN_POINT('Ctrl Pts',(0.0047103710871043,-0.0336441434784052,
0.0695210280977945));
#76359=CARTESIAN_POINT('',(0.00504028891799333,-0.0341934961088741,0.0692950855597322));
#76360=CARTESIAN_POINT('',(0.00484343027595112,-0.03386642128919,0.069425868724495));
#76361=CARTESIAN_POINT('Origin',(0.0135780139220781,-0.034561081807594,
0.0836881514620321));
#76362=CARTESIAN_POINT('Origin',(-0.00141135814116461,-0.0336938005044317,
0.0604182960296151));
#76363=CARTESIAN_POINT('',(0.00494687938261151,-0.0336938721132327,0.0693556894622211));
#76364=CARTESIAN_POINT('',(0.00489554225887861,-0.0336938721132427,0.0693913370389483));
#76365=CARTESIAN_POINT('',(0.00514653396172778,-0.0340203938281605,0.0692292157160934));
#76366=CARTESIAN_POINT('Origin',(0.01313127844728,-0.0345589643244171,0.0838668999249553));
#76367=CARTESIAN_POINT('',(0.00514723722102949,-0.034193496108874,0.0692303780603392));
#76368=CARTESIAN_POINT('Origin',(-0.000557089076279621,-0.0341934220717597,
0.0598022881300443));
#76369=CARTESIAN_POINT('',(0.00509376306952142,-0.0341934961088841,0.0692627318100457));
#76370=CARTESIAN_POINT('Ctrl Pts',(0.00522142697788282,-0.0340223579322396,
0.0688986826219814));
#76371=CARTESIAN_POINT('Ctrl Pts',(0.00514899761522924,-0.0339125849573574,
0.0689387136700595));
#76372=CARTESIAN_POINT('Ctrl Pts',(0.00507744769752613,-0.0338030433565231,
0.068980215708288));
#76373=CARTESIAN_POINT('Ctrl Pts',(0.00500686402026092,-0.0336938721132326,
0.0690231275514403));
#76374=CARTESIAN_POINT('Ctrl Pts',(0.00519672004260572,-0.0340223579322396,
0.0690092753305091));
#76375=CARTESIAN_POINT('Ctrl Pts',(0.00512581604184064,-0.0339125849573574,
0.0690496471516631));
#76376=CARTESIAN_POINT('Ctrl Pts',(0.00505579746738269,-0.0338030433565231,
0.0690914581520635));
#76377=CARTESIAN_POINT('Ctrl Pts',(0.00498674912136458,-0.0336938721132326,
0.069134646924971));
#76378=CARTESIAN_POINT('Ctrl Pts',(0.00517201310732862,-0.0340223579322397,
0.0691198680390369));
#76379=CARTESIAN_POINT('Ctrl Pts',(0.00510263446845203,-0.0339125849573575,
0.0691605806332668));
#76380=CARTESIAN_POINT('Ctrl Pts',(0.00503414723723926,-0.0338030433565231,
0.0692027005958391));
#76381=CARTESIAN_POINT('Ctrl Pts',(0.00496663422246824,-0.0336938721132327,
0.0692461662985017));
#76382=CARTESIAN_POINT('Ctrl Pts',(0.00514730617205152,-0.0340223579322397,
0.0692304607475647));
#76383=CARTESIAN_POINT('Ctrl Pts',(0.00507945289506342,-0.0339125849573575,
0.0692715141148704));
#76384=CARTESIAN_POINT('Ctrl Pts',(0.00501249700709583,-0.0338030433565231,
0.0693139430396147));
#76385=CARTESIAN_POINT('Ctrl Pts',(0.00494651932357189,-0.0336938721132327,
0.0693576856720325));
#76386=CARTESIAN_POINT('',(0.00497687170144616,-0.0336938721132427,0.0691894085068411));
#76387=CARTESIAN_POINT('Ctrl Pts',(0.00501782222478039,-0.0337108120662696,
0.0690164814584599));
#76388=CARTESIAN_POINT('Ctrl Pts',(0.00504008121951515,-0.0337611408994269,
0.0690532710382845));
#76389=CARTESIAN_POINT('Ctrl Pts',(0.00506193403697947,-0.0338121088781246,
0.0690893892898982));
#76390=CARTESIAN_POINT('Ctrl Pts',(0.0051048472249419,-0.0339153382773238,
0.0691603160398654));
#76391=CARTESIAN_POINT('Ctrl Pts',(0.0051258894405293,-0.0339675558473111,
0.0691950945318533));
#76392=CARTESIAN_POINT('Ctrl Pts',(0.0051465339617439,-0.0340203938281304,
0.0692292157161303));
#76393=CARTESIAN_POINT('Ctrl Pts',(0.00504225831159741,-0.0341934961088741,
0.0692955701851708));
#76394=CARTESIAN_POINT('Ctrl Pts',(0.00494189680028251,-0.03402875161944,
0.0693592782632969));
#76395=CARTESIAN_POINT('Ctrl Pts',(0.00484425414914076,-0.033864463329982,
0.0694270799214622));
#76396=CARTESIAN_POINT('Ctrl Pts',(0.00504028891799343,-0.0341934961088741,
0.0692950855597323));
#76397=CARTESIAN_POINT('Ctrl Pts',(0.00493991738742946,-0.03402875161944,
0.0693588343535194));
#76398=CARTESIAN_POINT('Ctrl Pts',(0.00484226640840904,-0.033864463329982,
0.069426677106658));
#76399=CARTESIAN_POINT('Ctrl Pts',(0.00471214970874164,-0.0341934961088741,
0.0692143375529102));
#76400=CARTESIAN_POINT('Ctrl Pts',(0.00461010877676299,-0.03402875161944,
0.0692848703662873));
#76401=CARTESIAN_POINT('Ctrl Pts',(0.00451107021147381,-0.033864463329982,
0.0693595603398275));
#76402=CARTESIAN_POINT('',(0.00470161482939921,-0.0341764758832377,0.0692216361208511));
#76403=CARTESIAN_POINT('',(0.00471214970874166,-0.034193496108874,0.0692143375529101));
#76404=CARTESIAN_POINT('Origin',(0.0137248784044839,-0.0345621026793295,
0.0831141536822559));
#76405=CARTESIAN_POINT('Ctrl Pts',(0.00470161483120347,-0.034176475883746,
0.069221636120644));
#76406=CARTESIAN_POINT('Ctrl Pts',(0.0047260972430818,-0.0341260050043381,
0.0692568939380233));
#76407=CARTESIAN_POINT('Ctrl Pts',(0.00475015412427072,-0.0340749269154154,
0.0692915388695708));
#76408=CARTESIAN_POINT('Ctrl Pts',(0.00479743531893986,-0.0339715436318372,
0.0693596299158009));
#76409=CARTESIAN_POINT('Ctrl Pts',(0.00482064169003878,-0.0339192778253278,
0.0693930502016218));
#76410=CARTESIAN_POINT('Ctrl Pts',(0.00484343027765033,-0.0338664212874711,
0.0694258687205468));
#76411=CARTESIAN_POINT('',(0.0048762193133775,-0.0341934961088841,0.0692547115563312));
#76412=CARTESIAN_POINT('Origin',(0.00812378219310841,-0.0315241814719618,
0.07415));
#76413=CARTESIAN_POINT('',(0.00470161482912772,-0.034210518019055,0.0692216361219359));
#76414=CARTESIAN_POINT('',(0.00469109556167716,-0.0341934961088739,0.069228957174499));
#76415=CARTESIAN_POINT('Origin',(0.0137648456250437,-0.034562170836886,
0.0830927724808212));
#76416=CARTESIAN_POINT('Origin',(0.014566150630993,-0.034562103658163,0.0825299917182353));
#76417=CARTESIAN_POINT('Origin',(0.0145321507033199,-0.0345621718255471,
0.0825599665698366));
#76418=CARTESIAN_POINT('Ctrl Pts',(0.00494811148172171,-0.0346945769586965,
0.0693548339147276));
#76419=CARTESIAN_POINT('Ctrl Pts',(0.00484767480818592,-0.0345275153362944,
0.0694213496092468));
#76420=CARTESIAN_POINT('Ctrl Pts',(0.00474930401395107,-0.0343603235965185,
0.0694910411490686));
#76421=CARTESIAN_POINT('Ctrl Pts',(0.00465328697272945,-0.034193496108874,
0.0695636980934709));
#76422=CARTESIAN_POINT('Ctrl Pts',(0.004879251283527,-0.0346945769586965,
0.0694026491996313));
#76423=CARTESIAN_POINT('Ctrl Pts',(0.00477981612027772,-0.0345275153362944,
0.0694706071985718));
#76424=CARTESIAN_POINT('Ctrl Pts',(0.00468249245451773,-0.0343603235965185,
0.0695417099192921));
#76425=CARTESIAN_POINT('Ctrl Pts',(0.00458756500098687,-0.034193496108874,
0.0696157427934518));
#76426=CARTESIAN_POINT('Ctrl Pts',(0.00481039108533224,-0.0346945769586965,
0.0694504644845362));
#76427=CARTESIAN_POINT('Ctrl Pts',(0.00471195743236938,-0.0345275153362944,
0.0695198647878973));
#76428=CARTESIAN_POINT('Ctrl Pts',(0.00461568089508422,-0.0343603235965185,
0.0695923786895156));
#76429=CARTESIAN_POINT('Ctrl Pts',(0.00452184302924412,-0.034193496108874,
0.0696677874934326));
#76430=CARTESIAN_POINT('Ctrl Pts',(0.00474153088713759,-0.0346945769586965,
0.0694982797694387));
#76431=CARTESIAN_POINT('Ctrl Pts',(0.00464409874446132,-0.0345275153362944,
0.0695691223772218));
#76432=CARTESIAN_POINT('Ctrl Pts',(0.00454886933565105,-0.0343603235965185,
0.0696430474597389));
#76433=CARTESIAN_POINT('Ctrl Pts',(0.00445612105750169,-0.034193496108874,
0.0697198321934136));
#76434=CARTESIAN_POINT('',(0.00474153088763531,-0.0346945769586966,0.0694982797690933));
#76435=CARTESIAN_POINT('',(0.00455327264714076,-0.0343667727831427,0.0696411657180134));
#76436=CARTESIAN_POINT('Origin',(0.0147766509948415,-0.0345626457065548,
0.0829887805624754));
#76437=CARTESIAN_POINT('Origin',(-0.00230804983714372,-0.0341934771028877,
0.0609767033420708));
#76438=CARTESIAN_POINT('',(0.0046521110251616,-0.034193496108874,0.0695646293168766));
#76439=CARTESIAN_POINT('',(0.00460311353337759,-0.034193496108884,0.0696034300359251));
#76440=CARTESIAN_POINT('',(0.00484343027935788,-0.0345211942962721,0.069425868723066));
#76441=CARTESIAN_POINT('Origin',(0.0143798191940824,-0.0345625596120614,
0.0832602862009375));
#76442=CARTESIAN_POINT('',(0.00484420513512573,-0.0346945769586885,0.0694269846156556));
#76443=CARTESIAN_POINT('Origin',(-0.00146602387291882,-0.0346945685853955,
0.0603394368119114));
#76444=CARTESIAN_POINT('',(0.00479286801139052,-0.0346945769587026,0.0694626321923844));
#76445=CARTESIAN_POINT('Ctrl Pts',(0.00489742035531189,-0.0345231616327842,
0.0690912858064888));
#76446=CARTESIAN_POINT('Ctrl Pts',(0.00482769310225423,-0.0344132092796988,
0.0691357566620687));
#76447=CARTESIAN_POINT('Ctrl Pts',(0.00475888929137185,-0.0343032738558979,
0.0691816674763862));
#76448=CARTESIAN_POINT('Ctrl Pts',(0.00469109556167711,-0.0341934961088739,
0.069228957174499));
#76449=CARTESIAN_POINT('Ctrl Pts',(0.00487970639523689,-0.0345231616327842,
0.0692032114592987));
#76450=CARTESIAN_POINT('Ctrl Pts',(0.0048115218797245,-0.0344132092796988,
0.069247926476879));
#76451=CARTESIAN_POINT('Ctrl Pts',(0.00474426577708761,-0.0343032738558979,
0.0692940495302901));
#76452=CARTESIAN_POINT('Ctrl Pts',(0.00467802273658055,-0.0341934961088739,
0.0693415193234766));
#76453=CARTESIAN_POINT('Ctrl Pts',(0.00486199243516188,-0.0345231616327842,
0.0693151371121086));
#76454=CARTESIAN_POINT('Ctrl Pts',(0.00479535065719477,-0.0344132092796988,
0.0693600962916893));
#76455=CARTESIAN_POINT('Ctrl Pts',(0.00472964226280337,-0.0343032738558979,
0.0694064315841939));
#76456=CARTESIAN_POINT('Ctrl Pts',(0.004664949911484,-0.0341934961088739,
0.0694540814724543));
#76457=CARTESIAN_POINT('Ctrl Pts',(0.00484427847508689,-0.0345231616327842,
0.0694270627649186));
#76458=CARTESIAN_POINT('Ctrl Pts',(0.00477917943466504,-0.0344132092796988,
0.0694722661064996));
#76459=CARTESIAN_POINT('Ctrl Pts',(0.00471501874851913,-0.0343032738558979,
0.0695188136380977));
#76460=CARTESIAN_POINT('Ctrl Pts',(0.00465187708638745,-0.0341934961088739,
0.0695666436214319));
#76461=CARTESIAN_POINT('',(0.00467160329342937,-0.0341934961088839,0.0693967932456977));
#76462=CARTESIAN_POINT('Ctrl Pts',(0.00470161483109297,-0.0342105180195399,
0.0692216361247682));
#76463=CARTESIAN_POINT('Ctrl Pts',(0.00472612475480663,-0.0342610556241199,
0.0692569335868257));
#76464=CARTESIAN_POINT('Ctrl Pts',(0.00475019486061234,-0.0343122189869934,
0.0692915976541774));
#76465=CARTESIAN_POINT('Ctrl Pts',(0.00479747653581031,-0.0344158119695211,
0.0693596893853396));
#76466=CARTESIAN_POINT('Ctrl Pts',(0.00482066876663529,-0.0344681990450118,
0.0693930891991104));
#76467=CARTESIAN_POINT('Ctrl Pts',(0.00484343027936789,-0.0345211942962545,
0.0694258687230875));
#76468=CARTESIAN_POINT('Ctrl Pts',(0.0047435263384397,-0.0346945769586932,
0.0694986396912232));
#76469=CARTESIAN_POINT('Ctrl Pts',(0.00464736275525272,-0.034529677707698,
0.0695685240892262));
#76470=CARTESIAN_POINT('Ctrl Pts',(0.0045541697290336,-0.0343648066251421,
0.0696423233011442));
#76471=CARTESIAN_POINT('Ctrl Pts',(0.00474153088764269,-0.0346945769586932,
0.0694982797690881));
#76472=CARTESIAN_POINT('Ctrl Pts',(0.00464535986332024,-0.034529677707698,
0.0695682054216243));
#76473=CARTESIAN_POINT('Ctrl Pts',(0.00455216110741178,-0.0343648066251421,
0.069642046160373));
#76474=CARTESIAN_POINT('Ctrl Pts',(0.00440896897686485,-0.0346945769586932,
0.0694382951314389));
#76475=CARTESIAN_POINT('Ctrl Pts',(0.00431155781260277,-0.034529677707698,
0.0695150962661672));
#76476=CARTESIAN_POINT('Ctrl Pts',(0.00421740414643578,-0.0343648066251421,
0.0695958578682178));
#76477=CARTESIAN_POINT('',(0.00439891316634542,-0.0346775396664962,0.0694462407877545));
#76478=CARTESIAN_POINT('',(0.00440896897686213,-0.0346945769586886,0.0694382951314411));
#76479=CARTESIAN_POINT('Origin',(0.014824661290163,-0.0345626618061633,
0.0823658646068263));
#76480=CARTESIAN_POINT('Ctrl Pts',(0.00439891316814823,-0.0346775396670097,
0.0694462407875334));
#76481=CARTESIAN_POINT('Ctrl Pts',(0.00442558211322793,-0.0346269749930482,
0.0694799182719924));
#76482=CARTESIAN_POINT('Ctrl Pts',(0.00445177711982146,-0.0345757902895592,
0.0695129972101099));
#76483=CARTESIAN_POINT('Ctrl Pts',(0.00450323940186589,-0.0344721707114263,
0.069577983711416));
#76484=CARTESIAN_POINT('Ctrl Pts',(0.00452849032766865,-0.0344197687642437,
0.0696098706373707));
#76485=CARTESIAN_POINT('Ctrl Pts',(0.00455327264725885,-0.0343667727830579,
0.0696411657177762));
#76486=CARTESIAN_POINT('',(0.00457524993225872,-0.0346945769587026,0.0694682874502772));
#76487=CARTESIAN_POINT('Origin',(0.00812378219310841,-0.0315241814719618,
0.07415));
#76488=CARTESIAN_POINT('',(0.00439891316649769,-0.0347116136489807,0.0694462407891372));
#76489=CARTESIAN_POINT('',(0.00438887434898241,-0.0346945769586885,0.0694542079053786));
#76490=CARTESIAN_POINT('Origin',(0.0148589946893147,-0.0345626686843321,
0.0823362930815001));
#76491=CARTESIAN_POINT('Origin',(0.0145852157278249,-0.0345626627999594,
0.0825554825893273));
#76492=CARTESIAN_POINT('Origin',(0.0145485596705449,-0.0345626696657839,
0.0825821210917095));
#76493=CARTESIAN_POINT('Ctrl Pts',(0.00468294913655636,-0.0352450361874068,
0.0695413743369022));
#76494=CARTESIAN_POINT('Ctrl Pts',(0.00450913196746544,-0.0349452760959492,
0.0696711474851085));
#76495=CARTESIAN_POINT('Ctrl Pts',(0.00434558363916616,-0.034644428984174,
0.0698136445818391));
#76496=CARTESIAN_POINT('Ctrl Pts',(0.00468095983803887,-0.0352450361874068,
0.0695429294305999));
#76497=CARTESIAN_POINT('Ctrl Pts',(0.00450720132026919,-0.0349452760959492,
0.0696727776064309));
#76498=CARTESIAN_POINT('Ctrl Pts',(0.00434371712805659,-0.034644428984174,
0.0698153450997831));
#76499=CARTESIAN_POINT('Ctrl Pts',(0.004483999588783,-0.0352450361874068,
0.0696968991036301));
#76500=CARTESIAN_POINT('Ctrl Pts',(0.0043160481325211,-0.0349452760959492,
0.0698341757571574));
#76501=CARTESIAN_POINT('Ctrl Pts',(0.00415891404790077,-0.034644428984174,
0.0699837132130496));
#76502=CARTESIAN_POINT('Ctrl Pts',(0.00448202998629044,-0.0352450361874068,
0.0696984388003605));
#76503=CARTESIAN_POINT('Ctrl Pts',(0.00431413660064362,-0.0349452760959492,
0.0698357897386648));
#76504=CARTESIAN_POINT('Ctrl Pts',(0.00415706601709922,-0.034644428984174,
0.0699853968941822));
#76505=CARTESIAN_POINT('',(0.00445614446971457,-0.035195163405328,0.0697198097295415));
#76506=CARTESIAN_POINT('',(0.0042772061852535,-0.0348678972925388,0.0698742570217802));
#76507=CARTESIAN_POINT('Origin',(0.0157928575127484,-0.034563676789046,
0.0820439094430579));
#76508=CARTESIAN_POINT('Origin',(-0.00311305772362403,-0.0346946199341114,
0.0616594540075098));
#76509=CARTESIAN_POINT('',(0.00437104378151317,-0.0346945769330288,0.0697916655231541));
#76510=CARTESIAN_POINT('',(0.00432457928567719,-0.0346945769458128,0.069833466261357));
#76511=CARTESIAN_POINT('',(0.00455327264733022,-0.0350221583435276,0.0696411657178925));
#76512=CARTESIAN_POINT('Origin',(0.0154645130411218,-0.0345628458717289,
0.0823950978543954));
#76513=CARTESIAN_POINT('',(0.00455404289067444,-0.035195136029876,0.0696421335081262));
#76514=CARTESIAN_POINT('Origin',(-0.00228666599125885,-0.0351951838366893,
0.0610036992822474));
#76515=CARTESIAN_POINT('',(0.00445612105791295,-0.035195137132875,0.0697198321929397));
#76516=CARTESIAN_POINT('Ctrl Pts',(0.00458614677508542,-0.0350241211494343,
0.0693038535258235));
#76517=CARTESIAN_POINT('Ctrl Pts',(0.00451939309440105,-0.0349144232818962,
0.0693525830032198));
#76518=CARTESIAN_POINT('Ctrl Pts',(0.00445360673153917,-0.0348045283579412,
0.0694027214938365));
#76519=CARTESIAN_POINT('Ctrl Pts',(0.00438887434028513,-0.0346945769439157,
0.0694542079122961));
#76520=CARTESIAN_POINT('Ctrl Pts',(0.0045754956550678,-0.0350241211494343,
0.069416670614269));
#76521=CARTESIAN_POINT('Ctrl Pts',(0.00451029598351996,-0.0349144232818962,
0.0694655468064763));
#76522=CARTESIAN_POINT('Ctrl Pts',(0.00444606759264397,-0.0348045283579412,
0.0695157999772407));
#76523=CARTESIAN_POINT('Ctrl Pts',(0.00438289514612716,-0.0346945769439157,
0.0695673688200344));
#76524=CARTESIAN_POINT('Ctrl Pts',(0.00456484453505019,-0.0350241211494343,
0.0695294877027144));
#76525=CARTESIAN_POINT('Ctrl Pts',(0.00450119887263888,-0.0349144232818962,
0.0695785106097329));
#76526=CARTESIAN_POINT('Ctrl Pts',(0.00443852845374877,-0.0348045283579412,
0.069628878460645));
#76527=CARTESIAN_POINT('Ctrl Pts',(0.0043769159519692,-0.0346945769439157,
0.0696805297277726));
#76528=CARTESIAN_POINT('Ctrl Pts',(0.00455419341503258,-0.0350241211494343,
0.0696423047911598));
#76529=CARTESIAN_POINT('Ctrl Pts',(0.00449210176175779,-0.0349144232818962,
0.0696914744129894));
#76530=CARTESIAN_POINT('Ctrl Pts',(0.00443098931485357,-0.0348045283579412,
0.0697419569440492));
#76531=CARTESIAN_POINT('Ctrl Pts',(0.00437093675781124,-0.0346945769439157,
0.0697936906355109));
#76532=CARTESIAN_POINT('',(0.00437995906542026,-0.0346945769458128,0.0696229367140174));
#76533=CARTESIAN_POINT('Ctrl Pts',(0.00439891316853388,-0.0347116136492803,
0.0694462407917096));
#76534=CARTESIAN_POINT('Ctrl Pts',(0.00442557151280757,-0.0347621546532191,
0.0694799049102405));
#76535=CARTESIAN_POINT('Ctrl Pts',(0.00445176113135062,-0.0348133084096798,
0.0695129771225977));
#76536=CARTESIAN_POINT('Ctrl Pts',(0.00450322477402094,-0.0349168561544572,
0.0695779653360103));
#76537=CARTESIAN_POINT('Ctrl Pts',(0.00452847838511639,-0.0349692089015925,
0.0696098555595186));
#76538=CARTESIAN_POINT('Ctrl Pts',(0.00455327264733732,-0.0350221583435,
0.0696411657179335));
#76539=CARTESIAN_POINT('Ctrl Pts',(0.00445757430726783,-0.0351951371254893,
0.0697200009715545));
#76540=CARTESIAN_POINT('Ctrl Pts',(0.00436598685682996,-0.0350307338980916,
0.0697957975193377));
#76541=CARTESIAN_POINT('Ctrl Pts',(0.00427761042043704,-0.0348659306897796,
0.0698753147075681));
#76542=CARTESIAN_POINT('Ctrl Pts',(0.00445612105798853,-0.0351951371254893,
0.069719832193028));
#76543=CARTESIAN_POINT('Ctrl Pts',(0.00436453011816052,-0.0350307338980916,
0.0697956587858282));
#76544=CARTESIAN_POINT('Ctrl Pts',(0.0042761514371521,-0.0348659306897796,
0.0698752061376226));
#76545=CARTESIAN_POINT('Ctrl Pts',(0.00421255496412829,-0.0351951371254893,
0.0696915447360682));
#76546=CARTESIAN_POINT('Ctrl Pts',(0.00412037919887578,-0.0350307338980916,
0.0697724069050406));
#76547=CARTESIAN_POINT('Ctrl Pts',(0.00403162431796947,-0.0348659306897796,
0.0698570097016025));
#76548=CARTESIAN_POINT('Origin',(0.000720343904793222,-0.0308609197410131,
0.0659205514694643));
#76549=CARTESIAN_POINT('',(0.0043499317327492,-0.0351951371254893,0.0697074994995907));
#76550=CARTESIAN_POINT('Origin',(0.00887563923730569,-0.0351840467441134,
0.0747740646081582));
#76551=CARTESIAN_POINT('Origin',(-0.000451870359554896,-0.035232261333163,
0.0658057740145225));
#76552=CARTESIAN_POINT('',(0.00410458066883951,-0.0351951142564652,0.0700361412650968));
#76553=CARTESIAN_POINT('',(0.00401729059133434,-0.0351951372916786,0.0701251737025606));
#76554=CARTESIAN_POINT('Origin',(0.00804826481983064,-0.0352875123221079,
0.0744821219329415));
#76555=CARTESIAN_POINT('Origin',(0.0143044590648397,-0.0298325076521956,
0.0698962459298664));
#76556=CARTESIAN_POINT('Origin',(0.00478655016906604,-0.0338732271129292,
0.0664614842499923));
#76557=CARTESIAN_POINT('Ctrl Pts',(0.00729059510661384,-0.0321934096636941,
0.0684593115509448));
#76558=CARTESIAN_POINT('Ctrl Pts',(0.00718873449328596,-0.0320508460843821,
0.0684742252030288));
#76559=CARTESIAN_POINT('Ctrl Pts',(0.00708735138360126,-0.0319086045662065,
0.0684918644038634));
#76560=CARTESIAN_POINT('Ctrl Pts',(0.00698666094645583,-0.0317669892866397,
0.0685121732016937));
#76561=CARTESIAN_POINT('Ctrl Pts',(0.00720791563977711,-0.0321934096636941,
0.0684732592529581));
#76562=CARTESIAN_POINT('Ctrl Pts',(0.00710630468367337,-0.0320508460843821,
0.0684896528281265));
#76563=CARTESIAN_POINT('Ctrl Pts',(0.0070052108055836,-0.0319086045662065,
0.0685087641283815));
#76564=CARTESIAN_POINT('Ctrl Pts',(0.00690484829068893,-0.0317669892866397,
0.0685305340835495));
#76565=CARTESIAN_POINT('Ctrl Pts',(0.00712523617294039,-0.0321934096636941,
0.0684872069549715));
#76566=CARTESIAN_POINT('Ctrl Pts',(0.00702387487406078,-0.0320508460843821,
0.0685050804532242));
#76567=CARTESIAN_POINT('Ctrl Pts',(0.00692307022756595,-0.0319086045662065,
0.0685256638528998));
#76568=CARTESIAN_POINT('Ctrl Pts',(0.00682303563492204,-0.0317669892866397,
0.0685488949654052));
#76569=CARTESIAN_POINT('Ctrl Pts',(0.00704255670610367,-0.0321934096636941,
0.0685011546569848));
#76570=CARTESIAN_POINT('Ctrl Pts',(0.00694144506444819,-0.0320508460843821,
0.0685205080783219));
#76571=CARTESIAN_POINT('Ctrl Pts',(0.00684092964954828,-0.0319086045662065,
0.068542563577418));
#76572=CARTESIAN_POINT('Ctrl Pts',(0.00674122297915514,-0.0317669892866397,
0.0685672558472609));
#76573=CARTESIAN_POINT('',(0.00704403585810413,-0.0321934096636941,0.068500905129842));
#76574=CARTESIAN_POINT('',(0.00681285683162341,-0.0318665617511264,0.0685500357424682));
#76575=CARTESIAN_POINT('Origin',(0.00957496668345433,-0.0326371944421322,
0.0850179355532371));
#76576=CARTESIAN_POINT('Origin',(0.00431443910331527,-0.0316939261509309,
0.0578773838241723));
#76577=CARTESIAN_POINT('',(0.00716681556072824,-0.0320197221621859,0.0684788621925544));
#76578=CARTESIAN_POINT('Ctrl Pts',(0.00716663134941515,-0.0320197392094778,
0.0684788454273853));
#76579=CARTESIAN_POINT('Ctrl Pts',(0.00713777469953208,-0.0319792716576075,
0.0684837157648794));
#76580=CARTESIAN_POINT('Ctrl Pts',(0.00710882381268693,-0.0319386439829729,
0.0684888282654879));
#76581=CARTESIAN_POINT('Ctrl Pts',(0.00707974976670056,-0.0318979099381661,
0.0684941966250222));
#76582=CARTESIAN_POINT('Ctrl Pts',(0.00705067629538211,-0.0318571766984948,
0.0684995648784473));
#76583=CARTESIAN_POINT('Ctrl Pts',(0.00702162711665199,-0.0318163871833584,
0.0685051599436445));
#76584=CARTESIAN_POINT('Ctrl Pts',(0.0069927014817602,-0.0317755399638303,
0.0685109591182903));
#76585=CARTESIAN_POINT('',(0.0071672942947959,-0.0321934096636183,0.068480111914651));
#76586=CARTESIAN_POINT('Origin',(0.00676376797449013,-0.0324103422814711,
0.0662141487655565));
#76587=CARTESIAN_POINT('',(0.00710566507646001,-0.0321934096636663,0.0684905085222565));
#76588=CARTESIAN_POINT('Ctrl Pts',(0.00704568861464045,-0.0321934096636618,
0.0685020807501934));
#76589=CARTESIAN_POINT('Ctrl Pts',(0.0069677994064548,-0.0320835708272592,
0.0685169485008574));
#76590=CARTESIAN_POINT('Ctrl Pts',(0.00689026306450258,-0.0319739230346488,
0.0685334195407371));
#76591=CARTESIAN_POINT('Ctrl Pts',(0.00681317717381767,-0.0318646057455572,
0.068551465182775));
#76592=CARTESIAN_POINT('Ctrl Pts',(0.0069533474301673,-0.0321934096636618,
0.0684363976441872));
#76593=CARTESIAN_POINT('Ctrl Pts',(0.0068745524007594,-0.0320835708272592,
0.0684525388517516));
#76594=CARTESIAN_POINT('Ctrl Pts',(0.00679613711712243,-0.0319739230346488,
0.0684703013557981));
#76595=CARTESIAN_POINT('Ctrl Pts',(0.00671820016202277,-0.0318646057455572,
0.0684896547306246));
#76596=CARTESIAN_POINT('Ctrl Pts',(0.00686100624569415,-0.0321934096636618,
0.068370714538181));
#76597=CARTESIAN_POINT('Ctrl Pts',(0.00678130539506401,-0.0320835708272592,
0.0683881292026458));
#76598=CARTESIAN_POINT('Ctrl Pts',(0.00670201116974227,-0.0319739230346488,
0.068407183170859));
#76599=CARTESIAN_POINT('Ctrl Pts',(0.00662322315022787,-0.0318646057455572,
0.0684278442784741));
#76600=CARTESIAN_POINT('Ctrl Pts',(0.006768665061221,-0.0321934096636618,
0.0683050314321747));
#76601=CARTESIAN_POINT('Ctrl Pts',(0.00668805838936861,-0.0320835708272592,
0.06832371955354));
#76602=CARTESIAN_POINT('Ctrl Pts',(0.00660788522236212,-0.0319739230346488,
0.06834406498592));
#76603=CARTESIAN_POINT('Ctrl Pts',(0.00652824613843297,-0.0318646057455572,
0.0683660338263237));
#76604=CARTESIAN_POINT('',(0.00675618319546388,-0.0321763980308454,0.0683079393225251));
#76605=CARTESIAN_POINT('',(0.00676866506118924,-0.0321934096636184,0.0683050314321821));
#76606=CARTESIAN_POINT('Origin',(0.00992800456953099,-0.0326386231073049,
0.0845488027386375));
#76607=CARTESIAN_POINT('Ctrl Pts',(0.00675618319618208,-0.0321763980306277,
0.0683079393256096));
#76608=CARTESIAN_POINT('Ctrl Pts',(0.00676596583544919,-0.0321259596174836,
0.0683497284555247));
#76609=CARTESIAN_POINT('Ctrl Pts',(0.00677557897780387,-0.0320749164631413,
0.0683907935345376));
#76610=CARTESIAN_POINT('Ctrl Pts',(0.00679447400500781,-0.03197160577939,
0.0684715086386123));
#76611=CARTESIAN_POINT('Ctrl Pts',(0.00680374852771889,-0.0319193786690096,
0.0685111272143545));
#76612=CARTESIAN_POINT('Ctrl Pts',(0.00681285683204034,-0.0318665617525269,
0.0685500357442718));
#76613=CARTESIAN_POINT('',(0.00690635045965669,-0.0321934096636663,0.0684029682810221));
#76614=CARTESIAN_POINT('Origin',(0.00812378219310841,-0.0315241814719618,
0.07415));
#76615=CARTESIAN_POINT('',(0.00675618319537921,-0.0322104233323793,0.0683079393221637));
#76616=CARTESIAN_POINT('',(0.00674370756866053,-0.0321934096636183,0.0683108738640975));
#76617=CARTESIAN_POINT('Origin',(0.00997315455773778,-0.0326387235070079,
0.0845447211264128));
#76618=CARTESIAN_POINT('Origin',(0.0111227131009451,-0.0326386242831274,
0.084269129501095));
#76619=CARTESIAN_POINT('Origin',(0.0110804413412371,-0.0326387243911324,
0.084285507925658));
#76620=CARTESIAN_POINT('Ctrl Pts',(0.00697026296830151,-0.0327445246967097,
0.0685155063760795));
#76621=CARTESIAN_POINT('Ctrl Pts',(0.00675775456723365,-0.032443687833936,
0.0685590120648648));
#76622=CARTESIAN_POINT('Ctrl Pts',(0.00654912690637849,-0.0321434074405927,
0.0686184011598839));
#76623=CARTESIAN_POINT('Ctrl Pts',(0.00672649047186738,-0.0327445246967097,
0.06857095878795));
#76624=CARTESIAN_POINT('Ctrl Pts',(0.00651607349270334,-0.032443687833936,
0.0686236585067403));
#76625=CARTESIAN_POINT('Ctrl Pts',(0.00631022384415969,-0.0321434074405927,
0.0686920579780508));
#76626=CARTESIAN_POINT('',(0.00669145688913583,-0.0326943950436612,0.0685798501614767));
#76627=CARTESIAN_POINT('',(0.00646381897801533,-0.0323666188837389,0.0686433996763394));
#76628=CARTESIAN_POINT('Origin',(0.0109516488654873,-0.0326395579113589,
0.0848420401288825));
#76629=CARTESIAN_POINT('Origin',(0.0032761114381671,-0.032193382560307,
0.0580688125701116));
#76630=CARTESIAN_POINT('',(0.00658389151240922,-0.0321934096532689,0.0686086227625171));
#76631=CARTESIAN_POINT('',(0.00652405129658461,-0.0321934096584275,0.0686266615794344));
#76632=CARTESIAN_POINT('',(0.00681285683140512,-0.0325210109756239,0.0685500357415387));
#76633=CARTESIAN_POINT('Origin',(0.0104803109773102,-0.0326393129157746,
0.0849370402584136));
#76634=CARTESIAN_POINT('',(0.00681316648662225,-0.0326943950436593,0.0685513585156833));
#76635=CARTESIAN_POINT('Origin',(0.00429166690332564,-0.0326943765538226,
0.0577801024812186));
#76636=CARTESIAN_POINT('',(0.00675231168788904,-0.0326943950436702,0.0685656043385901));
#76637=CARTESIAN_POINT('Ctrl Pts',(0.00698622386623576,-0.0325229783203769,
0.0682588234576625));
#76638=CARTESIAN_POINT('Ctrl Pts',(0.00690501412643116,-0.032413025309245,
0.0682745046743217));
#76639=CARTESIAN_POINT('Ctrl Pts',(0.00682414108978533,-0.032303122220807,
0.0682918634404063));
#76640=CARTESIAN_POINT('Ctrl Pts',(0.0067437075642966,-0.0321934096576658,
0.0683108738651289));
#76641=CARTESIAN_POINT('Ctrl Pts',(0.00692855124571332,-0.0325229783203769,
0.0683563683759227));
#76642=CARTESIAN_POINT('Ctrl Pts',(0.00684868616047378,-0.032413025309245,
0.0683728446083945));
#76643=CARTESIAN_POINT('Ctrl Pts',(0.00676917402037314,-0.032303122220807,
0.0683909704538051));
#76644=CARTESIAN_POINT('Ctrl Pts',(0.00669011585552622,-0.0321934096576658,
0.068410719100305));
#76645=CARTESIAN_POINT('Ctrl Pts',(0.00687087862519088,-0.0325229783203769,
0.0684539132941828));
#76646=CARTESIAN_POINT('Ctrl Pts',(0.00679235819451639,-0.032413025309245,
0.0684711845424674));
#76647=CARTESIAN_POINT('Ctrl Pts',(0.00671420695096094,-0.032303122220807,
0.0684900774672039));
#76648=CARTESIAN_POINT('Ctrl Pts',(0.00663652414675584,-0.0321934096576658,
0.0685105643354812));
#76649=CARTESIAN_POINT('Ctrl Pts',(0.00681320600466844,-0.0325229783203769,
0.068551458212443));
#76650=CARTESIAN_POINT('Ctrl Pts',(0.006736030228559,-0.032413025309245,
0.0685695244765402));
#76651=CARTESIAN_POINT('Ctrl Pts',(0.00665923988154875,-0.032303122220807,
0.0685891844806027));
#76652=CARTESIAN_POINT('Ctrl Pts',(0.00658293243798545,-0.0321934096576658,
0.0686104095706573));
#76653=CARTESIAN_POINT('',(0.00666379954097551,-0.0321934096584275,0.0684597483130441));
#76654=CARTESIAN_POINT('Ctrl Pts',(0.0067561831961672,-0.0322104233328939,
0.0683079393255456));
#76655=CARTESIAN_POINT('Ctrl Pts',(0.00676597909106434,-0.0322609421831152,
0.0683497850803887));
#76656=CARTESIAN_POINT('Ctrl Pts',(0.0067755987090056,-0.0323120888240273,
0.0683908778216115));
#76657=CARTESIAN_POINT('Ctrl Pts',(0.00679449387927703,-0.0324156524631819,
0.068471593536837));
#76658=CARTESIAN_POINT('Ctrl Pts',(0.00680376166468919,-0.0324680267167316,
0.0685111833323961));
#76659=CARTESIAN_POINT('Ctrl Pts',(0.00681285683141068,-0.0325210109755913,
0.0685500357415819));
#76660=CARTESIAN_POINT('Origin',(0.0159447659747408,-0.0262834582512507,
0.0732923295942242));
#76661=CARTESIAN_POINT('Origin',(0.0109413105581775,-0.0342770797690015,
0.0623227055287267));
#76662=CARTESIAN_POINT('Ctrl Pts',(0.00669317978386622,-0.0326943950436604,
0.068580919425046));
#76663=CARTESIAN_POINT('Ctrl Pts',(0.00661642741597393,-0.0325844576448134,
0.0686006358074801));
#76664=CARTESIAN_POINT('Ctrl Pts',(0.00654007738331149,-0.0324744968375322,
0.0686219409500783));
#76665=CARTESIAN_POINT('Ctrl Pts',(0.00646422713348024,-0.0323646534831894,
0.0686448062061611));
#76666=CARTESIAN_POINT('Ctrl Pts',(0.00659689667667646,-0.0326943950436604,
0.0685211641671075));
#76667=CARTESIAN_POINT('Ctrl Pts',(0.00651932076933648,-0.0325844576448134,
0.0685422075112125));
#76668=CARTESIAN_POINT('Ctrl Pts',(0.00644217458268614,-0.0324744968375322,
0.0685648567415387));
#76669=CARTESIAN_POINT('Ctrl Pts',(0.00636555656065241,-0.0323646534831894,
0.0685890814752131));
#76670=CARTESIAN_POINT('Ctrl Pts',(0.00650061356948669,-0.0326943950436604,
0.0684614089091691));
#76671=CARTESIAN_POINT('Ctrl Pts',(0.00642221412269904,-0.0325844576448134,
0.0684837792149449));
#76672=CARTESIAN_POINT('Ctrl Pts',(0.00634427178206078,-0.0324744968375322,
0.0685077725329991));
#76673=CARTESIAN_POINT('Ctrl Pts',(0.00626688598782457,-0.0323646534831894,
0.068533356744265));
#76674=CARTESIAN_POINT('Ctrl Pts',(0.00640433046229693,-0.0326943950436604,
0.0684016536512307));
#76675=CARTESIAN_POINT('Ctrl Pts',(0.00632510747606159,-0.0325844576448134,
0.0684253509186773));
#76676=CARTESIAN_POINT('Ctrl Pts',(0.00624636898143543,-0.0324744968375322,
0.0684506883244595));
#76677=CARTESIAN_POINT('Ctrl Pts',(0.00616821541499673,-0.0323646534831894,
0.068477632013317));
#76678=CARTESIAN_POINT('',(0.0063920558145679,-0.0326773559991157,0.0684053395461553));
#76679=CARTESIAN_POINT('',(0.00640433046229621,-0.0326943950436594,0.0684016536512309));
#76680=CARTESIAN_POINT('Origin',(0.0112327526299647,-0.0326395670494284,
0.0842893241052763));
#76681=CARTESIAN_POINT('Ctrl Pts',(0.00639205581553023,-0.0326773559987419,
0.0684053395493593));
#76682=CARTESIAN_POINT('Ctrl Pts',(0.0064044530806279,-0.0326267922585978,
0.068446465029357));
#76683=CARTESIAN_POINT('Ctrl Pts',(0.00641663061315396,-0.0325756109579362,
0.0684868615899192));
#76684=CARTESIAN_POINT('Ctrl Pts',(0.00644055657674764,-0.0324719985462367,
0.0685662312516508));
#76685=CARTESIAN_POINT('Ctrl Pts',(0.00645229541176373,-0.0324196091621771,
0.0686051725198134));
#76686=CARTESIAN_POINT('Ctrl Pts',(0.00646381897802939,-0.0323666188837756,
0.0686433996763861));
#76687=CARTESIAN_POINT('',(0.00654789367572602,-0.0326943950436703,0.0684907519063639));
#76688=CARTESIAN_POINT('Origin',(0.00812378219310841,-0.0315241814719618,
0.07415));
#76689=CARTESIAN_POINT('',(0.00639205581458065,-0.0327114338379882,0.0684053395461977));
#76690=CARTESIAN_POINT('',(0.00637978906701307,-0.0326943950436593,0.0684090516483641));
#76691=CARTESIAN_POINT('Origin',(0.0112759051401613,-0.0326395669585225,
0.0842755065717678));
#76692=CARTESIAN_POINT('Origin',(0.0111365488380453,-0.0326395678495505,
0.0843183266738395));
#76693=CARTESIAN_POINT('Origin',(0.011092948081802,-0.0326395679003803,
0.0843306565853654));
#76694=CARTESIAN_POINT('Ctrl Pts',(0.00661870853619124,-0.0332451089994433,
0.0685990650979088));
#76695=CARTESIAN_POINT('Ctrl Pts',(0.00640935160109997,-0.0329451141710254,
0.0686558298795999));
#76696=CARTESIAN_POINT('Ctrl Pts',(0.0062048651823789,-0.0326442513127493,
0.0687282030187462));
#76697=CARTESIAN_POINT('Ctrl Pts',(0.00637889943667374,-0.0332451089994433,
0.0686697163242861));
#76698=CARTESIAN_POINT('Ctrl Pts',(0.00617220715618131,-0.0329451141710254,
0.0687355256541421));
#76699=CARTESIAN_POINT('Ctrl Pts',(0.00597105909439879,-0.0326442513127493,
0.0688167169341688));
#76700=CARTESIAN_POINT('',(0.00634453065372195,-0.0331951640388616,0.068680778029775));
#76701=CARTESIAN_POINT('',(0.00612133224107488,-0.0328677532092642,0.0687584956468902));
#76702=CARTESIAN_POINT('Origin',(0.0122556578473816,-0.032640190890057,
0.0843680538129557));
#76703=CARTESIAN_POINT('Origin',(0.00227198026462762,-0.0326944279134336,
0.0583942945404394));
#76704=CARTESIAN_POINT('',(0.00623898417299244,-0.0326943950436593,0.0687162479424096));
#76705=CARTESIAN_POINT('',(0.00618039470757279,-0.0326943950436693,0.068738008561452));
#76706=CARTESIAN_POINT('',(0.00646381897801807,-0.0330220786163545,0.0686433996763386));
#76707=CARTESIAN_POINT('Origin',(0.011816743799778,-0.0326396682763674,
0.0845645921266418));
#76708=CARTESIAN_POINT('',(0.0064642110798787,-0.0331951640388587,0.0686447003968781));
#76709=CARTESIAN_POINT('Origin',(0.00328024443866656,-0.0331952026560115,
0.0580825166274355));
#76710=CARTESIAN_POINT('',(0.00640437086681032,-0.0331951640388701,0.0686627392133366));
#76711=CARTESIAN_POINT('Ctrl Pts',(0.00661855761185007,-0.0330240426238172,
0.0683418764682563));
#76712=CARTESIAN_POINT('Ctrl Pts',(0.00653854505161971,-0.0329142774063519,
0.0683626124033324));
#76713=CARTESIAN_POINT('Ctrl Pts',(0.006458921271911,-0.032804347972669,
0.0683850127591524));
#76714=CARTESIAN_POINT('Ctrl Pts',(0.00637978906701304,-0.0326943950436592,
0.0684090516483641));
#76715=CARTESIAN_POINT('Ctrl Pts',(0.00656712371985652,-0.0330240426238172,
0.0684428501813645));
#76716=CARTESIAN_POINT('Ctrl Pts',(0.00648850217089816,-0.0329142774063519,
0.0684642946684124));
#76717=CARTESIAN_POINT('Ctrl Pts',(0.00641028474367978,-0.032804347972669,
0.0684873751733547));
#76718=CARTESIAN_POINT('Ctrl Pts',(0.00633257245484427,-0.0326943950436592,
0.0685120648879004));
#76719=CARTESIAN_POINT('Ctrl Pts',(0.00651568982786298,-0.0330240426238172,
0.0685438238944727));
#76720=CARTESIAN_POINT('Ctrl Pts',(0.0064384592901766,-0.0329142774063519,
0.0685659769334924));
#76721=CARTESIAN_POINT('Ctrl Pts',(0.00636164821544856,-0.032804347972669,
0.0685897375875569));
#76722=CARTESIAN_POINT('Ctrl Pts',(0.0062853558426755,-0.0326943950436592,
0.0686150781274367));
#76723=CARTESIAN_POINT('Ctrl Pts',(0.00646425593586943,-0.0330240426238172,
0.0686447976075808));
#76724=CARTESIAN_POINT('Ctrl Pts',(0.00638841640945504,-0.0329142774063519,
0.0686676591985724));
#76725=CARTESIAN_POINT('Ctrl Pts',(0.00631301168721734,-0.032804347972669,
0.0686921000017591));
#76726=CARTESIAN_POINT('Ctrl Pts',(0.00623813923050673,-0.0326943950436592,
0.068718091366973));
#76727=CARTESIAN_POINT('',(0.00630938662001275,-0.0326943950436693,0.0685626497953969));
#76728=CARTESIAN_POINT('Ctrl Pts',(0.0063920558155326,-0.0327114338383336,
0.0684053395493668));
#76729=CARTESIAN_POINT('Ctrl Pts',(0.00640445101855673,-0.0327619876830886,
0.0684464581888426));
#76730=CARTESIAN_POINT('Ctrl Pts',(0.00641662754386919,-0.0328131562604148,
0.0684868514081724));
#76731=CARTESIAN_POINT('Ctrl Pts',(0.00644055348549382,-0.0329167375858771,
0.0685662209970261));
#76732=CARTESIAN_POINT('Ctrl Pts',(0.00645229336847186,-0.0329691088920623,
0.0686051657415956));
#76733=CARTESIAN_POINT('Ctrl Pts',(0.00646381897802911,-0.0330220786163187,
0.0686433996763849));
#76734=CARTESIAN_POINT('Ctrl Pts',(0.00634631757358637,-0.0331951640388604,
0.0686817371550525));
#76735=CARTESIAN_POINT('Ctrl Pts',(0.00627100330633363,-0.0330855618127442,
0.0687062181372552));
#76736=CARTESIAN_POINT('Ctrl Pts',(0.00619614072618659,-0.032975722417194,
0.0687322733848046));
#76737=CARTESIAN_POINT('Ctrl Pts',(0.00612182733583426,-0.0328657861694598,
0.0687598742348139));
#76738=CARTESIAN_POINT('Ctrl Pts',(0.00624647230033861,-0.0331951640388604,
0.0686281454257511));
#76739=CARTESIAN_POINT('Ctrl Pts',(0.00617041991534398,-0.0330855618127442,
0.0686540015747676));
#76740=CARTESIAN_POINT('Ctrl Pts',(0.00609484710770694,-0.032975722417194,
0.0686814482361032));
#76741=CARTESIAN_POINT('Ctrl Pts',(0.00601985237700612,-0.0328657861694598,
0.0687104550096942));
#76742=CARTESIAN_POINT('Ctrl Pts',(0.00614662702709085,-0.0331951640388604,
0.0685745536964497));
#76743=CARTESIAN_POINT('Ctrl Pts',(0.00606983652435434,-0.0330855618127442,
0.0686017850122799));
#76744=CARTESIAN_POINT('Ctrl Pts',(0.0059935534892273,-0.032975722417194,
0.0686306230874018));
#76745=CARTESIAN_POINT('Ctrl Pts',(0.00591787741817799,-0.0328657861694598,
0.0686610357845745));
#76746=CARTESIAN_POINT('Ctrl Pts',(0.00604678175384308,-0.0331951640388604,
0.0685209619671483));
#76747=CARTESIAN_POINT('Ctrl Pts',(0.00596925313336469,-0.0330855618127442,
0.0685495684497923));
#76748=CARTESIAN_POINT('Ctrl Pts',(0.00589225987074765,-0.032975722417194,
0.0685797979387003));
#76749=CARTESIAN_POINT('Ctrl Pts',(0.00581590245934985,-0.0328657861694598,
0.0686116165594547));
#76750=CARTESIAN_POINT('',(0.00603476276650962,-0.0331781648279164,0.0685254113201094));
#76751=CARTESIAN_POINT('',(0.00604678175384198,-0.0331951640388587,0.0685209619671487));
#76752=CARTESIAN_POINT('Origin',(0.0124496843299243,-0.0326412092132826,
0.083751548933787));
#76753=CARTESIAN_POINT('Ctrl Pts',(0.00603476276772703,-0.0331781648273353,
0.0685254113233959));
#76754=CARTESIAN_POINT('Ctrl Pts',(0.00604972819993293,-0.0331276810207345,
0.0685657050609758));
#76755=CARTESIAN_POINT('Ctrl Pts',(0.00606442329048319,-0.0330765665168813,
0.0686052709160877));
#76756=CARTESIAN_POINT('Ctrl Pts',(0.00609328587190068,-0.0329730612715184,
0.0686829820884425));
#76757=CARTESIAN_POINT('Ctrl Pts',(0.00610744141276619,-0.0329207135598909,
0.0687210952308556));
#76758=CARTESIAN_POINT('Ctrl Pts',(0.00612133224109073,-0.0328677532092985,
0.0687584956469329));
#76759=CARTESIAN_POINT('',(0.00619565620379196,-0.0331951640388701,0.0686008699984719));
#76760=CARTESIAN_POINT('Origin',(0.00812378219310841,-0.0315241814719618,
0.07415));
#76761=CARTESIAN_POINT('',(0.00603476276666942,-0.0332121607144237,0.0685254113205401));
#76762=CARTESIAN_POINT('',(0.00602275330947992,-0.0331951640388587,0.0685298863329841));
#76763=CARTESIAN_POINT('Origin',(0.012488821924199,-0.0326413652568557,
0.0837286474373116));
#76764=CARTESIAN_POINT('Origin',(0.011114284309464,-0.0326412100054318,
0.0842475298356103));
#76765=CARTESIAN_POINT('Origin',(0.0110696848207288,-0.0326413661676127,
0.084255724981764));
#76766=CARTESIAN_POINT('Ctrl Pts',(0.0062731520925408,-0.0337436976235975,
0.0687045162537317));
#76767=CARTESIAN_POINT('Ctrl Pts',(0.00622417458644122,-0.0336723290703325,
0.0687211611013268));
#76768=CARTESIAN_POINT('Ctrl Pts',(0.00617550439209288,-0.033601104548885,
0.0687386842071387));
#76769=CARTESIAN_POINT('Ctrl Pts',(0.00602011010256092,-0.0333736987606857,
0.0687946320128644));
#76770=CARTESIAN_POINT('Ctrl Pts',(0.0058681824982094,-0.0331450831799192,
0.0688594050413615));
#76771=CARTESIAN_POINT('Ctrl Pts',(0.00603825211877815,-0.0337436976235975,
0.0687900849531859));
#76772=CARTESIAN_POINT('Ctrl Pts',(0.00599004423052975,-0.0336723290703325,
0.0688088425267451));
#76773=CARTESIAN_POINT('Ctrl Pts',(0.00594218153080748,-0.033601104548885,
0.0688284641737325));
#76774=CARTESIAN_POINT('Ctrl Pts',(0.00578936541166089,-0.0333736987606857,
0.0688911122057338));
#76775=CARTESIAN_POINT('Ctrl Pts',(0.00564039622669078,-0.0331450831799192,
0.0689624264687813));
#76776=CARTESIAN_POINT('Ctrl Pts',(0.00603590311904052,-0.0337436976235975,
0.0687909406401804));
#76777=CARTESIAN_POINT('Ctrl Pts',(0.00598770292697063,-0.0336723290703325,
0.0688097193409994));
#76778=CARTESIAN_POINT('Ctrl Pts',(0.00593984830219463,-0.033601104548885,
0.0688293619733985));
#76779=CARTESIAN_POINT('Ctrl Pts',(0.0057870579647519,-0.0333736987606857,
0.0688920770076626));
#76780=CARTESIAN_POINT('Ctrl Pts',(0.0056381183639756,-0.0331450831799192,
0.0689634566830555));
#76781=CARTESIAN_POINT('',(0.00600462631125898,-0.0336938721132548,0.0688032904185449));
#76782=CARTESIAN_POINT('',(0.00578674824582927,-0.0333679870047996,0.0688948694279671));
#76783=CARTESIAN_POINT('Ctrl Pts',(0.00600462631128152,-0.0336938721132513,
0.0688032904185359));
#76784=CARTESIAN_POINT('Ctrl Pts',(0.00598375559559105,-0.0336629187933857,
0.0688115624780597));
#76785=CARTESIAN_POINT('Ctrl Pts',(0.00596293999109099,-0.0336319952300996,
0.0688199540984121));
#76786=CARTESIAN_POINT('Ctrl Pts',(0.00594218153081813,-0.0336011045488905,
0.0688284641737283));
#76787=CARTESIAN_POINT('Ctrl Pts',(0.00589009145084816,-0.0335235892595407,
0.0688498188646805));
#76788=CARTESIAN_POINT('Ctrl Pts',(0.00583826869550219,-0.0334458668665523,
0.0688719575253822));
#76789=CARTESIAN_POINT('Ctrl Pts',(0.00578674825651963,-0.0333679869962447,
0.0688948694229269));
#76790=CARTESIAN_POINT('Ctrl Pts',(0.00578670733990235,-0.0333679692470408,
0.0688948868668454));
#76791=CARTESIAN_POINT('Ctrl Pts',(0.00578689691692108,-0.0333391895417259,
0.0688952985685979));
#76792=CARTESIAN_POINT('Ctrl Pts',(0.00578704196364883,-0.0333104081133762,
0.0688956058010175));
#76793=CARTESIAN_POINT('Ctrl Pts',(0.00578723896601389,-0.0332532698772281,
0.0688960101108606));
#76794=CARTESIAN_POINT('Ctrl Pts',(0.0057872922798601,-0.033224917381766,
0.0688961102564426));
#76795=CARTESIAN_POINT('Ctrl Pts',(0.00578730007695781,-0.0331960985261731,
0.0688961108059752));
#76796=CARTESIAN_POINT('Ctrl Pts',(0.00578730019114828,-0.0331956312664165,
0.0688961107877576));
#76797=CARTESIAN_POINT('Ctrl Pts',(0.0057873002927981,-0.0331951640388587,
0.0688961107425525));
#76798=CARTESIAN_POINT('',(0.00590151527665438,-0.0331951640388587,0.0688453176577636));
#76799=CARTESIAN_POINT('',(0.00584440778473558,-0.0331951640388687,0.0688707142001683));
#76800=CARTESIAN_POINT('',(0.00612133224137555,-0.0335216366567747,0.0687584956472138));
#76801=CARTESIAN_POINT('Origin',(0.0130397563591545,-0.0326434571527544,
0.0839079534837288));
#76802=CARTESIAN_POINT('',(0.00612180524213312,-0.0336938721132327,0.0687597691804743));
#76803=CARTESIAN_POINT('Origin',(0.00231959251784929,-0.0336938867896205,
0.0585224839769945));
#76804=CARTESIAN_POINT('',(0.00606321577670605,-0.0336938721132538,0.0687815297995196));
#76805=CARTESIAN_POINT('Ctrl Pts',(0.00625683182131963,-0.0335235895815172,
0.0684478516058156));
#76806=CARTESIAN_POINT('Ctrl Pts',(0.00617833052217658,-0.0334144449262749,
0.0684735538533703));
#76807=CARTESIAN_POINT('Ctrl Pts',(0.0061002700236429,-0.0333049234473147,
0.068500907407455));
#76808=CARTESIAN_POINT('Ctrl Pts',(0.00602275330948,-0.0331951640388587,
0.0685298863329839));
#76809=CARTESIAN_POINT('Ctrl Pts',(0.00621183956698099,-0.0335235895815172,
0.0685518557861903));
#76810=CARTESIAN_POINT('Ctrl Pts',(0.00613477009014618,-0.0334144449262749,
0.0685781774407076));
#76811=CARTESIAN_POINT('Ctrl Pts',(0.0060581558553928,-0.0333049234473147,
0.0686061215330071));
#76812=CARTESIAN_POINT('Ctrl Pts',(0.00598209806555667,-0.0331951640388587,
0.0686356612053659));
#76813=CARTESIAN_POINT('Ctrl Pts',(0.00616684731264234,-0.0335235895815172,
0.0686558599665651));
#76814=CARTESIAN_POINT('Ctrl Pts',(0.00609120965811578,-0.0334144449262749,
0.0686828010280449));
#76815=CARTESIAN_POINT('Ctrl Pts',(0.00601604168714269,-0.0333049234473147,
0.0687113356585592));
#76816=CARTESIAN_POINT('Ctrl Pts',(0.00594144282163335,-0.0331951640388587,
0.0687414360777479));
#76817=CARTESIAN_POINT('Ctrl Pts',(0.0061218550583037,-0.0335235895815172,
0.0687598641469398));
#76818=CARTESIAN_POINT('Ctrl Pts',(0.00604764922608538,-0.0334144449262749,
0.0687874246153822));
#76819=CARTESIAN_POINT('Ctrl Pts',(0.00597392751889259,-0.0333049234473147,
0.0688165497841113));
#76820=CARTESIAN_POINT('Ctrl Pts',(0.00590078757771002,-0.0331951640388587,
0.0688472109501299));
#76821=CARTESIAN_POINT('',(0.00596213429307715,-0.0331951640388687,0.0686876019953839));
#76822=CARTESIAN_POINT('Ctrl Pts',(0.00603476276775504,-0.0332121607145989,
0.068525411323471));
#76823=CARTESIAN_POINT('Ctrl Pts',(0.00604970298029355,-0.0332625444109694,
0.0685656371582569));
#76824=CARTESIAN_POINT('Ctrl Pts',(0.00606438574952495,-0.0333135300746684,
0.0686051698387849));
#76825=CARTESIAN_POINT('Ctrl Pts',(0.00609324805637579,-0.0334167203140655,
0.0686828802718817));
#76826=CARTESIAN_POINT('Ctrl Pts',(0.00610741641537851,-0.0334688847587357,
0.0687210279265394));
#76827=CARTESIAN_POINT('Ctrl Pts',(0.00612133224146106,-0.0335216366562436,
0.0687584956479298));
#76828=CARTESIAN_POINT('Ctrl Pts',(0.00600646949786311,-0.0336938721132512,
0.0688041352519375));
#76829=CARTESIAN_POINT('Ctrl Pts',(0.00597517837754259,-0.0336474569765019,
0.0688165285857433));
#76830=CARTESIAN_POINT('Ctrl Pts',(0.00594403448092964,-0.033601104548885,
0.0688292873724213));
#76831=CARTESIAN_POINT('Ctrl Pts',(0.00586518529514674,-0.0334837508592655,
0.0688615896868568));
#76832=CARTESIAN_POINT('Ctrl Pts',(0.00578732791866564,-0.0333660264659096,
0.0688962142813527));
#76833=CARTESIAN_POINT('Ctrl Pts',(0.0060046263112863,-0.0336938721132512,
0.0688032904185342));
#76834=CARTESIAN_POINT('Ctrl Pts',(0.00597333024587553,-0.0336474569765019,
0.0688156945411226));
#76835=CARTESIAN_POINT('Ctrl Pts',(0.00594218153080748,-0.033601104548885,
0.0688284641737325));
#76836=CARTESIAN_POINT('Ctrl Pts',(0.00586332014580413,-0.0334837508592655,
0.0688607939475741));
#76837=CARTESIAN_POINT('Ctrl Pts',(0.0057854513891387,-0.0333660264659097,
0.068895446350906));
#76838=CARTESIAN_POINT('Ctrl Pts',(0.00569558683942607,-0.0336938721132512,
0.0686616406951254));
#76839=CARTESIAN_POINT('Ctrl Pts',(0.00566346165117972,-0.0336474569765019,
0.068675853728293));
#76840=CARTESIAN_POINT('Ctrl Pts',(0.00563150504567037,-0.033601104548885,
0.0686904418534641));
#76841=CARTESIAN_POINT('Ctrl Pts',(0.00555059826781557,-0.0334837508592655,
0.0687273756323722));
#76842=CARTESIAN_POINT('Ctrl Pts',(0.0054708214427003,-0.0333660264659097,
0.068766690628262));
#76843=CARTESIAN_POINT('',(0.00568571412321803,-0.0336769361243754,0.068667680774838));
#76844=CARTESIAN_POINT('',(0.0056974300172302,-0.0336938721132327,0.0686624855245192));
#76845=CARTESIAN_POINT('Ctrl Pts',(0.00568571412321775,-0.0336769361243751,
0.0686676807748381));
#76846=CARTESIAN_POINT('Ctrl Pts',(0.00568766599362715,-0.0336797586670183,
0.0686668127493317));
#76847=CARTESIAN_POINT('Ctrl Pts',(0.00568961825378007,-0.033682581271316,
0.0686659457990411));
#76848=CARTESIAN_POINT('Ctrl Pts',(0.00569352355871244,-0.033688226610875,
0.0686642140460501));
#76849=CARTESIAN_POINT('Ctrl Pts',(0.00569547660353143,-0.033691049346173,
0.0686633492433572));
#76850=CARTESIAN_POINT('Ctrl Pts',(0.0056974300172374,-0.0336938721132294,
0.0686624855245247));
#76851=CARTESIAN_POINT('Ctrl Pts',(0.00568571412321801,-0.0336769361243754,
0.068667680774838));
#76852=CARTESIAN_POINT('Ctrl Pts',(0.00570274472761296,-0.0336279031321627,
0.0687059763462553));
#76853=CARTESIAN_POINT('Ctrl Pts',(0.00572002035994807,-0.0335767851940105,
0.0687448228954735));
#76854=CARTESIAN_POINT('Ctrl Pts',(0.0057538715420316,-0.0334733198899491,
0.0688209417654192));
#76855=CARTESIAN_POINT('Ctrl Pts',(0.0057704698207817,-0.0334209645035413,
0.0688582651953198));
#76856=CARTESIAN_POINT('Ctrl Pts',(0.00578674825926269,-0.0333679869844681,
0.0688948694219787));
#76857=CARTESIAN_POINT('',(0.00585102816425459,-0.0336938721132538,0.0687328879715421));
#76858=CARTESIAN_POINT('Origin',(0.00812378219310841,-0.0315241814719618,
0.07415));
#76859=CARTESIAN_POINT('',(0.00568571412375028,-0.0337108120655693,0.0686676807760293));
#76860=CARTESIAN_POINT('',(0.00567400935308169,-0.0336938721132327,0.0686729010386622));
#76861=CARTESIAN_POINT('Origin',(0.0113128278435283,-0.0345562516955559,
0.0840713794002105));
#76862=CARTESIAN_POINT('Ctrl Pts',(0.00567400935308121,-0.033693872113231,
0.0686729010386669));
#76863=CARTESIAN_POINT('Ctrl Pts',(0.0056759590678808,-0.0336910493335091,
0.0686720289787689));
#76864=CARTESIAN_POINT('Ctrl Pts',(0.00567790932733335,-0.0336882266045427,
0.0686711579246108));
#76865=CARTESIAN_POINT('Ctrl Pts',(0.00568181091981302,-0.0336825812712757,
0.0686694178353954));
#76866=CARTESIAN_POINT('Ctrl Pts',(0.00568376225282281,-0.0336797586669981,
0.0686685488003381));
#76867=CARTESIAN_POINT('Ctrl Pts',(0.00568571412321826,-0.0336769361243751,
0.0686676807748379));
#76868=CARTESIAN_POINT('Origin',(0.0133551836121441,-0.0345562518084255,
0.0831631116134414));
#76869=CARTESIAN_POINT('Ctrl Pts',(0.00593492688647828,-0.0342436276873911,
0.0688314440449839));
#76870=CARTESIAN_POINT('Ctrl Pts',(0.00573433424182315,-0.033943005420181,
0.0689139980837942));
#76871=CARTESIAN_POINT('Ctrl Pts',(0.00554052976830017,-0.0336441434784052,
0.0690114270551327));
#76872=CARTESIAN_POINT('Ctrl Pts',(0.00570586243808517,-0.0342436276873911,
0.0689315913289329));
#76873=CARTESIAN_POINT('Ctrl Pts',(0.00550904691051073,-0.033943005420181,
0.069022784675835));
#76874=CARTESIAN_POINT('Ctrl Pts',(0.00531965957175876,-0.0336441434784052,
0.0691285439039623));
#76875=CARTESIAN_POINT('',(0.0056730853089392,-0.0341934961088741,0.0689469038273424));
#76876=CARTESIAN_POINT('',(0.0054613874790652,-0.0338664212895199,0.0690519827975974));
#76877=CARTESIAN_POINT('Origin',(0.0123395583110997,-0.0345610818075423,
0.0842965367884047));
#76878=CARTESIAN_POINT('Origin',(0.000384867417876509,-0.0336938005044518,
0.0593315050317913));
#76879=CARTESIAN_POINT('',(0.00557281665257841,-0.0336938721132327,0.0689953225308435));
#76880=CARTESIAN_POINT('',(0.00551741651134117,-0.0336938721132427,0.0690242547680603));
#76881=CARTESIAN_POINT('',(0.00578674825926758,-0.0340203938281605,0.0688948694219765));
#76882=CARTESIAN_POINT('Origin',(0.0118739423558916,-0.0345589643244194,
0.0844178849644761));
#76883=CARTESIAN_POINT('',(0.00578730029279683,-0.034193496108874,0.068896110742553));
#76884=CARTESIAN_POINT('Origin',(0.00130960736199823,-0.0341934220717618,
0.0588274224331425));
#76885=CARTESIAN_POINT('',(0.00573019280087801,-0.0341934961088841,0.0689215072849577));
#76886=CARTESIAN_POINT('Ctrl Pts',(0.00590247750310578,-0.0340223579322397,
0.0685763292639232));
#76887=CARTESIAN_POINT('Ctrl Pts',(0.00582560204691174,-0.0339125849573575,
0.0686069668490042));
#76888=CARTESIAN_POINT('Ctrl Pts',(0.00574941473702995,-0.0338030433565231,
0.0686391740487182));
#76889=CARTESIAN_POINT('Ctrl Pts',(0.00567400935308184,-0.0336938721132327,
0.0686729010386616));
#76890=CARTESIAN_POINT('Ctrl Pts',(0.00586410444762454,-0.0340223579322397,
0.068682953315822));
#76891=CARTESIAN_POINT('Ctrl Pts',(0.00578869961519338,-0.0339125849573575,
0.0687141201654192));
#76892=CARTESIAN_POINT('Ctrl Pts',(0.00571399285022984,-0.0338030433565231,
0.0687468258192468));
#76893=CARTESIAN_POINT('Ctrl Pts',(0.00564007598248167,-0.0336938721132327,
0.0687810199833012));
#76894=CARTESIAN_POINT('Ctrl Pts',(0.0058257313921433,-0.0340223579322397,
0.0687895773677208));
#76895=CARTESIAN_POINT('Ctrl Pts',(0.00575179718347503,-0.0339125849573575,
0.0688212734818342));
#76896=CARTESIAN_POINT('Ctrl Pts',(0.00567857096342973,-0.0338030433565231,
0.0688544775897753));
#76897=CARTESIAN_POINT('Ctrl Pts',(0.00560614261188149,-0.0336938721132327,
0.0688891389279408));
#76898=CARTESIAN_POINT('Ctrl Pts',(0.00578735833666206,-0.0340223579322397,
0.0688962014196196));
#76899=CARTESIAN_POINT('Ctrl Pts',(0.00571489475175667,-0.0339125849573575,
0.0689284267982492));
#76900=CARTESIAN_POINT('Ctrl Pts',(0.00564314907662961,-0.0338030433565231,
0.0689621293603038));
#76901=CARTESIAN_POINT('Ctrl Pts',(0.00557220924128132,-0.0336938721132327,
0.0689972578725805));
#76902=CARTESIAN_POINT('',(0.00562341300284005,-0.0336938721132427,0.0688341117847629));
#76903=CARTESIAN_POINT('Ctrl Pts',(0.00568571412520953,-0.0337108120662699,
0.0686676807793159));
#76904=CARTESIAN_POINT('Ctrl Pts',(0.00570318664412029,-0.0337611408994238,
0.0687069700540986));
#76905=CARTESIAN_POINT('Ctrl Pts',(0.00572034032832543,-0.0338121088781185,
0.0687455423867835));
#76906=CARTESIAN_POINT('Ctrl Pts',(0.00575402565406572,-0.0339153382773242,
0.068821288306757));
#76907=CARTESIAN_POINT('Ctrl Pts',(0.0057705430446389,-0.0339675558473115,
0.0688584298488686));
#76908=CARTESIAN_POINT('Ctrl Pts',(0.00578674825927892,-0.0340203938281304,
0.0688948694220151));
#76909=CARTESIAN_POINT('Ctrl Pts',(0.00567497843361324,-0.0341934961088741,
0.0689476314618332));
#76910=CARTESIAN_POINT('Ctrl Pts',(0.00560324085231802,-0.0340836138583034,
0.0689813990154933));
#76911=CARTESIAN_POINT('Ctrl Pts',(0.0055322364407307,-0.0339738896647348,
0.0690166348255629));
#76912=CARTESIAN_POINT('Ctrl Pts',(0.00546205305262393,-0.033864463329982,
0.069053287702634));
#76913=CARTESIAN_POINT('Ctrl Pts',(0.00556920361712944,-0.0341934961088741,
0.0689069762393947));
#76914=CARTESIAN_POINT('Ctrl Pts',(0.00549690542439284,-0.0340836138583034,
0.0689422023651342));
#76915=CARTESIAN_POINT('Ctrl Pts',(0.00542537085244468,-0.0339738896647348,
0.0689789076481103));
#76916=CARTESIAN_POINT('Ctrl Pts',(0.00535468830752193,-0.033864463329982,
0.0690170389726853));
#76917=CARTESIAN_POINT('Ctrl Pts',(0.00546342880064564,-0.0341934961088741,
0.0688663210169561));
#76918=CARTESIAN_POINT('Ctrl Pts',(0.00539056999646766,-0.0340836138583034,
0.0689030057147751));
#76919=CARTESIAN_POINT('Ctrl Pts',(0.00531850526415866,-0.0339738896647348,
0.0689411804706578));
#76920=CARTESIAN_POINT('Ctrl Pts',(0.00524732356241992,-0.033864463329982,
0.0689807902427367));
#76921=CARTESIAN_POINT('Ctrl Pts',(0.00535765398416183,-0.0341934961088741,
0.0688256657945176));
#76922=CARTESIAN_POINT('Ctrl Pts',(0.00528423456854248,-0.0340836138583034,
0.068863809064416));
#76923=CARTESIAN_POINT('Ctrl Pts',(0.00521163967587265,-0.0339738896647348,
0.0689034532932052));
#76924=CARTESIAN_POINT('Ctrl Pts',(0.00513995881731792,-0.033864463329982,
0.0689445415127881));
#76925=CARTESIAN_POINT('',(0.00534628742210696,-0.03417647588326,0.0688315864418915));
#76926=CARTESIAN_POINT('',(0.00535765398416182,-0.034193496108874,0.0688256657945176));
#76927=CARTESIAN_POINT('Origin',(0.0125572058492587,-0.0345621026014781,
0.0837454721759852));
#76928=CARTESIAN_POINT('Ctrl Pts',(0.00534628742358402,-0.0341764758830167,
0.0688315864447245));
#76929=CARTESIAN_POINT('Ctrl Pts',(0.005366157861692,-0.0341260048546759,
0.0688696348358654));
#76930=CARTESIAN_POINT('Ctrl Pts',(0.00538568272774161,-0.0340749271290188,
0.0689070215173464));
#76931=CARTESIAN_POINT('Ctrl Pts',(0.00542405717566493,-0.0339715434429171,
0.0689805018299831));
#76932=CARTESIAN_POINT('Ctrl Pts',(0.00544289174144717,-0.0339192781035154,
0.069016566707967));
#76933=CARTESIAN_POINT('Ctrl Pts',(0.0054613874812267,-0.033866421287732,
0.0690519827938002));
#76934=CARTESIAN_POINT('',(0.00551536964656051,-0.0341934961088841,0.06888628481094));
#76935=CARTESIAN_POINT('Origin',(0.00812378219310841,-0.0315241814719618,
0.07415));
#76936=CARTESIAN_POINT('',(0.00534628742196449,-0.034210518019038,0.0688315864416189));
#76937=CARTESIAN_POINT('',(0.00533493353088824,-0.0341934961088739,0.0688375313516922));
#76938=CARTESIAN_POINT('Origin',(0.0125995375225319,-0.0345621708608686,
0.0837292687609065));
#76939=CARTESIAN_POINT('Origin',(0.0134650591095609,-0.0345621036373532,
0.0832713557882409));
#76940=CARTESIAN_POINT('Origin',(0.0134275703865789,-0.0345621717810568,
0.0832968329301066));
#76941=CARTESIAN_POINT('Ctrl Pts',(0.00557414626475439,-0.0346945769586966,
0.0689946281525624));
#76942=CARTESIAN_POINT('Ctrl Pts',(0.00546616493731153,-0.0345275153362944,
0.0690480312979003));
#76943=CARTESIAN_POINT('Ctrl Pts',(0.00535983516013318,-0.0343603235965185,
0.069104844169385));
#76944=CARTESIAN_POINT('Ctrl Pts',(0.00525546891217763,-0.034193496108874,
0.0691648940658255));
#76945=CARTESIAN_POINT('Ctrl Pts',(0.00549983620543779,-0.0346945769586966,
0.0690334359284018));
#76946=CARTESIAN_POINT('Ctrl Pts',(0.00539266772239766,-0.0345275153362944,
0.0690883955276842));
#76947=CARTESIAN_POINT('Ctrl Pts',(0.00528719994890919,-0.0343603235965185,
0.0691467396924839));
#76948=CARTESIAN_POINT('Ctrl Pts',(0.00518374224719534,-0.034193496108874,
0.0692082912306149));
#76949=CARTESIAN_POINT('Ctrl Pts',(0.0054255261461213,-0.0346945769586966,
0.0690722437042413));
#76950=CARTESIAN_POINT('Ctrl Pts',(0.00531917050748389,-0.0345275153362944,
0.0691287597574667));
#76951=CARTESIAN_POINT('Ctrl Pts',(0.00521456473768522,-0.0343603235965185,
0.0691886352155814));
#76952=CARTESIAN_POINT('Ctrl Pts',(0.00511201558221298,-0.034193496108874,
0.0692516883954046));
#76953=CARTESIAN_POINT('Ctrl Pts',(0.00535121608680457,-0.0346945769586966,
0.0691110514800807));
#76954=CARTESIAN_POINT('Ctrl Pts',(0.00524567329256993,-0.0345275153362944,
0.0691691239872521));
#76955=CARTESIAN_POINT('Ctrl Pts',(0.00514192952646121,-0.0343603235965185,
0.0692305307386816));
#76956=CARTESIAN_POINT('Ctrl Pts',(0.00504028891723077,-0.034193496108874,
0.0692950855601937));
#76957=CARTESIAN_POINT('',(0.00535121608758449,-0.0346945769586966,0.0691110514796735));
#76958=CARTESIAN_POINT('',(0.00514653396144725,-0.0343667727832754,0.0692292157162159));
#76959=CARTESIAN_POINT('Origin',(0.0136163976382128,-0.0345626461564186,
0.0837529099911741));
#76960=CARTESIAN_POINT('Origin',(-0.000574742401596686,-0.0341934771027763,
0.059773124973944));
#76961=CARTESIAN_POINT('',(0.00525418552406562,-0.0341934961088739,0.0691656705609461));
#76962=CARTESIAN_POINT('',(0.00520071137255756,-0.0341934961088839,0.0691980243106526));
#76963=CARTESIAN_POINT('',(0.00546138748271273,-0.034521194296272,0.0690519827966342));
#76964=CARTESIAN_POINT('Origin',(0.0131886668458207,-0.034562559611912,
0.0839725382199522));
#76965=CARTESIAN_POINT('',(0.00546201637008398,-0.0346945769586886,0.0690531870052571));
#76966=CARTESIAN_POINT('Origin',(0.000340517204970014,-0.0346945685853854,
0.0592464157979725));
#76967=CARTESIAN_POINT('',(0.00540661622884424,-0.0346945769587026,0.0690821192424753));
#76968=CARTESIAN_POINT('Ctrl Pts',(0.00555688618962087,-0.0345231616327842,
0.0687268049170898));
#76969=CARTESIAN_POINT('Ctrl Pts',(0.0054821350806509,-0.0344132092796988,
0.0687621859645974));
#76970=CARTESIAN_POINT('Ctrl Pts',(0.00540811965755405,-0.0343032738558979,
0.0687991113543318));
#76971=CARTESIAN_POINT('Ctrl Pts',(0.0053349335308882,-0.0341934961088739,
0.0688375313516922));
#76972=CARTESIAN_POINT('Ctrl Pts',(0.0055252839054265,-0.0345231616327842,
0.0688356278548013));
#76973=CARTESIAN_POINT('Ctrl Pts',(0.00545203276744245,-0.0344132092796988,
0.0688714444953041));
#76974=CARTESIAN_POINT('Ctrl Pts',(0.00537952624783742,-0.0343032738558979,
0.0689087744298423));
#76975=CARTESIAN_POINT('Ctrl Pts',(0.00530785601081389,-0.0341934961088739,
0.0689475674550632));
#76976=CARTESIAN_POINT('Ctrl Pts',(0.00549368162123214,-0.0345231616327842,
0.0689444507925129));
#76977=CARTESIAN_POINT('Ctrl Pts',(0.005421930454234,-0.0344132092796988,
0.0689807030260108));
#76978=CARTESIAN_POINT('Ctrl Pts',(0.00535093283812078,-0.0343032738558979,
0.0690184375053529));
#76979=CARTESIAN_POINT('Ctrl Pts',(0.00528077849073958,-0.0341934961088739,
0.0690576035584343));
#76980=CARTESIAN_POINT('Ctrl Pts',(0.00546207933703777,-0.0345231616327842,
0.0690532737302244));
#76981=CARTESIAN_POINT('Ctrl Pts',(0.00539182814102554,-0.0344132092796988,
0.0690899615567174));
#76982=CARTESIAN_POINT('Ctrl Pts',(0.00532233942840415,-0.0343032738558979,
0.0691281005808634));
#76983=CARTESIAN_POINT('Ctrl Pts',(0.00525370097066527,-0.0341934961088739,
0.0691676396618053));
#76984=CARTESIAN_POINT('',(0.00529455952748693,-0.0341934961088839,0.0690016009563292));
#76985=CARTESIAN_POINT('Ctrl Pts',(0.00534628742355866,-0.03421051801954,
0.0688315864446759));
#76986=CARTESIAN_POINT('Ctrl Pts',(0.00536618013406737,-0.0342610556239182,
0.0688696774835435));
#76987=CARTESIAN_POINT('Ctrl Pts',(0.00538571588016893,-0.0343122189865703,
0.0689070849984284));
#76988=CARTESIAN_POINT('Ctrl Pts',(0.00542408960451617,-0.0344158093671077,
0.0689805639255444));
#76989=CARTESIAN_POINT('Ctrl Pts',(0.00544291474401996,-0.0344682017099466,
0.0690166107538446));
#76990=CARTESIAN_POINT('Ctrl Pts',(0.00546138748271902,-0.0345211942962543,
0.0690519827966574));
#76991=CARTESIAN_POINT('Ctrl Pts',(0.00535315069336335,-0.0346945769586932,
0.0691116586599817));
#76992=CARTESIAN_POINT('Ctrl Pts',(0.00524898655120909,-0.0345296777077528,
0.0691689395057838));
#76993=CARTESIAN_POINT('Ctrl Pts',(0.00514727888600538,-0.0343648066252516,
0.0692304766055316));
#76994=CARTESIAN_POINT('Ctrl Pts',(0.00535121608759247,-0.0346945769586932,
0.0691110514796692));
#76995=CARTESIAN_POINT('Ctrl Pts',(0.00524703939241488,-0.0345296777077528,
0.0691683723220768));
#76996=CARTESIAN_POINT('Ctrl Pts',(0.0051453208380107,-0.0343648066252516,
0.0692299499030813));
#76997=CARTESIAN_POINT('Ctrl Pts',(0.00502879459541324,-0.0346945769586932,
0.0690098587791664));
#76998=CARTESIAN_POINT('Ctrl Pts',(0.00492252581275511,-0.0345296777077528,
0.0690738454577844));
#76999=CARTESIAN_POINT('Ctrl Pts',(0.00481899246366886,-0.0343648066252516,
0.0691421696470237));
#77000=CARTESIAN_POINT('',(0.00501782222316508,-0.0346775396664962,0.0690164814543596));
#77001=CARTESIAN_POINT('',(0.00502879459541034,-0.0346945769586886,0.0690098587791681));
#77002=CARTESIAN_POINT('Origin',(0.0137421018776223,-0.0345626618292509,
0.0831409227960663));
#77003=CARTESIAN_POINT('Ctrl Pts',(0.00501782222498079,-0.0346775396670097,
0.0690164814543668));
#77004=CARTESIAN_POINT('Ctrl Pts',(0.00504005996953166,-0.0346269749928338,
0.0690532358870802));
#77005=CARTESIAN_POINT('Ctrl Pts',(0.005061902530474,-0.0345757902891088,
0.0690893370929175));
#77006=CARTESIAN_POINT('Ctrl Pts',(0.00510481512632278,-0.0344721681088299,
0.0691602628715452));
#77007=CARTESIAN_POINT('Ctrl Pts',(0.00512586833264621,-0.0344197714289979,
0.0691950596410056));
#77008=CARTESIAN_POINT('Ctrl Pts',(0.0051465339616478,-0.034366772783151,
0.0692292157159015));
#77009=CARTESIAN_POINT('',(0.00519000534150742,-0.0346945769587026,0.0690604551294308));
#77010=CARTESIAN_POINT('Origin',(0.00812378219310841,-0.0315241814719618,
0.07415));
#77011=CARTESIAN_POINT('',(0.00501782222314295,-0.0347116136489808,0.0690164814557504));
#77012=CARTESIAN_POINT('',(0.00500686402026083,-0.0346945769586885,0.0690231275514409));
#77013=CARTESIAN_POINT('Origin',(0.0137798706785429,-0.0345626688067305,
0.0831158875518691));
#77014=CARTESIAN_POINT('Origin',(0.0134807789049568,-0.0345626626943302,
0.0832990351857672));
#77015=CARTESIAN_POINT('Origin',(0.0134410735156174,-0.0345626697525361,
0.0833208694376766));
#77016=CARTESIAN_POINT('Ctrl Pts',(0.00528769508957777,-0.0352450361874068,
0.0691464639936529));
#77017=CARTESIAN_POINT('Ctrl Pts',(0.00509898363248728,-0.0349452760959493,
0.069253428773973));
#77018=CARTESIAN_POINT('Ctrl Pts',(0.00491886530969939,-0.034644428984174,
0.0693743041977043));
#77019=CARTESIAN_POINT('Ctrl Pts',(0.00528552657235165,-0.0352450361874068,
0.0691477574997566));
#77020=CARTESIAN_POINT('Ctrl Pts',(0.0050968639006444,-0.0349452760959493,
0.0692548040670459));
#77021=CARTESIAN_POINT('Ctrl Pts',(0.00491680038517477,-0.034644428984174,
0.0693757573706836));
#77022=CARTESIAN_POINT('Ctrl Pts',(0.00507082189649861,-0.0352450361874068,
0.0692758274110036));
#77023=CARTESIAN_POINT('Ctrl Pts',(0.00488698946075453,-0.0349452760959493,
0.0693909716980202));
#77024=CARTESIAN_POINT('Ctrl Pts',(0.00471235241243916,-0.034644428984174,
0.0695196358834792));
#77025=CARTESIAN_POINT('Ctrl Pts',(0.00506867484974007,-0.0352450361874068,
0.069277108110116));
#77026=CARTESIAN_POINT('Ctrl Pts',(0.00488489071635562,-0.0349452760959493,
0.0693923333743298));
#77027=CARTESIAN_POINT('Ctrl Pts',(0.00471030793271181,-0.034644428984174,
0.0695210746686072));
#77028=CARTESIAN_POINT('',(0.00504031496053605,-0.0351951634053284,0.0692950662076422));
#77029=CARTESIAN_POINT('',(0.00484343027934216,-0.0348678972925388,0.0694258687230507));
#77030=CARTESIAN_POINT('Origin',(0.0147430153683402,-0.0345636767881302,
0.0829428536169149));
#77031=CARTESIAN_POINT('Origin',(-0.00145897125933837,-0.0346946199341064,
0.0603495961363917));
#77032=CARTESIAN_POINT('',(0.00494687939771636,-0.0346945769330288,0.0693556894524282));
#77033=CARTESIAN_POINT('',(0.00489554226662406,-0.0346945769458128,0.0693913370338159));
#77034=CARTESIAN_POINT('',(0.00514653396174029,-0.0350221583435276,0.0692292157160859));
#77035=CARTESIAN_POINT('Origin',(0.0143732444102733,-0.0345628458718996,
0.0832501203288295));
#77036=CARTESIAN_POINT('',(0.00514717683520144,-0.0351951360298761,0.0692302724120965));
#77037=CARTESIAN_POINT('Origin',(-0.000556908188897693,-0.0351951838366778,
0.0598025866993451));
#77038=CARTESIAN_POINT('',(0.00504028891793258,-0.0351951371328751,0.0692950855596333));
#77039=CARTESIAN_POINT('Ctrl Pts',(0.00522142529493176,-0.0350241211494343,
0.068898683552134));
#77040=CARTESIAN_POINT('Ctrl Pts',(0.00514909056398597,-0.0349144232818962,
0.0689386623283936));
#77041=CARTESIAN_POINT('Ctrl Pts',(0.00507753892708967,-0.0348045283579412,
0.0689801602444542));
#77042=CARTESIAN_POINT('Ctrl Pts',(0.00500686401076511,-0.0346945769439157,
0.0690231275572138));
#77043=CARTESIAN_POINT('Ctrl Pts',(0.00519671843168066,-0.0350241211494343,
0.0690092761048272));
#77044=CARTESIAN_POINT('Ctrl Pts',(0.00512590706780351,-0.0349144232818962,
0.069049595207998));
#77045=CARTESIAN_POINT('Ctrl Pts',(0.0050558867445849,-0.0348045283579412,
0.0690914021655859));
#77046=CARTESIAN_POINT('Ctrl Pts',(0.00498674914185908,-0.0346945769439157,
0.0691346467656571));
#77047=CARTESIAN_POINT('Ctrl Pts',(0.00517201156842956,-0.0350241211494342,
0.0691198686575205));
#77048=CARTESIAN_POINT('Ctrl Pts',(0.00510272357162104,-0.0349144232818962,
0.0691605280876023));
#77049=CARTESIAN_POINT('Ctrl Pts',(0.00503423456208013,-0.0348045283579412,
0.0692026440867175));
#77050=CARTESIAN_POINT('Ctrl Pts',(0.00496663427295305,-0.0346945769439157,
0.0692461659741004));
#77051=CARTESIAN_POINT('Ctrl Pts',(0.00514730470517846,-0.0350241211494342,
0.0692304612102137));
#77052=CARTESIAN_POINT('Ctrl Pts',(0.00507954007543858,-0.0349144232818962,
0.0692714609672067));
#77053=CARTESIAN_POINT('Ctrl Pts',(0.00501258237957536,-0.0348045283579412,
0.0693138860078492));
#77054=CARTESIAN_POINT('Ctrl Pts',(0.00494651940404702,-0.0346945769439157,
0.0693576851825436));
#77055=CARTESIAN_POINT('',(0.00497687170919161,-0.0346945769458128,0.0691894085017085));
#77056=CARTESIAN_POINT('Ctrl Pts',(0.00501782222484005,-0.0347116136492805,
0.0690164814585585));
#77057=CARTESIAN_POINT('Ctrl Pts',(0.00504005112727424,-0.034762154653215,
0.069053221301946));
#77058=CARTESIAN_POINT('Ctrl Pts',(0.0050618891855351,-0.0348133084096714,
0.0690893151596056));
#77059=CARTESIAN_POINT('Ctrl Pts',(0.0051048018390844,-0.034916856154457,
0.0691602410262969));
#77060=CARTESIAN_POINT('Ctrl Pts',(0.00512585941308189,-0.0349692089015918,
0.069195044902605));
#77061=CARTESIAN_POINT('Ctrl Pts',(0.00514653396174227,-0.0350221583435,
0.0692292157161274));
#77062=CARTESIAN_POINT('Ctrl Pts',(0.00504170955441301,-0.0351951371254899,
0.0692954351478188));
#77063=CARTESIAN_POINT('Ctrl Pts',(0.00494134447195073,-0.0350307338980918,
0.0693591550658663));
#77064=CARTESIAN_POINT('Ctrl Pts',(0.00484369876383043,-0.0348659306897793,
0.069426968732773));
#77065=CARTESIAN_POINT('Ctrl Pts',(0.00504028891799687,-0.0351951371254899,
0.06929508555973));
#77066=CARTESIAN_POINT('Ctrl Pts',(0.0049399166080202,-0.0350307338980918,
0.0693588348485441));
#77067=CARTESIAN_POINT('Ctrl Pts',(0.00484226489248684,-0.0348659306897793,
0.0694266781598411));
#77068=CARTESIAN_POINT('Ctrl Pts',(0.00480218877398651,-0.0351951371254899,
0.0692364942316872));
#77069=CARTESIAN_POINT('Ctrl Pts',(0.00470060512506399,-0.0350307338980918,
0.0693051660915897));
#77070=CARTESIAN_POINT('Ctrl Pts',(0.00460194656084147,-0.0348659306897793,
0.0693779778336128));
#77071=CARTESIAN_POINT('Origin',(0.00181014562194367,-0.0308609197410754,
0.0650575462689631));
#77072=CARTESIAN_POINT('',(0.00493648262365106,-0.0351951371254899,0.0692695410617617));
#77073=CARTESIAN_POINT('Origin',(0.00879149458470891,-0.0351840467441126,
0.0748633763469272));
#77074=CARTESIAN_POINT('Origin',(0.000661576364853088,-0.0352322614578571,
0.0647967767776562));
#77075=CARTESIAN_POINT('',(0.00465187649100793,-0.0351951142564654,0.0695648407465883));
#77076=CARTESIAN_POINT('',(0.00455411599855671,-0.0351951372916786,0.0696422307890182));
#77077=CARTESIAN_POINT('Origin',(0.0080072158301023,-0.0352875118963586,
0.0744700109874943));
#77078=CARTESIAN_POINT('Origin',(0.0147888593340341,-0.0298325076521914,
0.0707044322691962));
#77079=CARTESIAN_POINT('Origin',(0.00577656859764103,-0.0338731362290147,
0.0661036106639049));
#77080=CARTESIAN_POINT('Ctrl Pts',(0.00801039742017867,-0.0321934096636942,
0.0683997582973775));
#77081=CARTESIAN_POINT('Ctrl Pts',(0.0079074708319817,-0.0320508460843967,
0.0684017878308188));
#77082=CARTESIAN_POINT('Ctrl Pts',(0.00780467638033086,-0.0319086045662354,
0.06840658126832));
#77083=CARTESIAN_POINT('Ctrl Pts',(0.00770223455006554,-0.0317669892866828,
0.0684141100671357));
#77084=CARTESIAN_POINT('Ctrl Pts',(0.00792662179503905,-0.0321934096636942,
0.0684032335326665));
#77085=CARTESIAN_POINT('Ctrl Pts',(0.00782375741189882,-0.0320508460843967,
0.0684067626099037));
#77086=CARTESIAN_POINT('Ctrl Pts',(0.00772106540818489,-0.0319086045662354,
0.0684130527892125));
#77087=CARTESIAN_POINT('Ctrl Pts',(0.00761876578283156,-0.0317669892866828,
0.0684220723232597));
#77088=CARTESIAN_POINT('Ctrl Pts',(0.00784284616989943,-0.0321934096636942,
0.0684067087679555));
#77089=CARTESIAN_POINT('Ctrl Pts',(0.00774004399181596,-0.0320508460843967,
0.0684117373889885));
#77090=CARTESIAN_POINT('Ctrl Pts',(0.00763745443603893,-0.0319086045662354,
0.0684195243101051));
#77091=CARTESIAN_POINT('Ctrl Pts',(0.00753529701559759,-0.0317669892866828,
0.0684300345793837));
#77092=CARTESIAN_POINT('Ctrl Pts',(0.0077590705447598,-0.0321934096636942,
0.0684101840032445));
#77093=CARTESIAN_POINT('Ctrl Pts',(0.00765633057173309,-0.0320508460843967,
0.0684167121680733));
#77094=CARTESIAN_POINT('Ctrl Pts',(0.00755384346389296,-0.0319086045662354,
0.0684259958309976));
#77095=CARTESIAN_POINT('Ctrl Pts',(0.00745182824836361,-0.0317669892866828,
0.0684379968355076));
#77096=CARTESIAN_POINT('',(0.00776056930724865,-0.0321934096636942,0.0684101218306007));
#77097=CARTESIAN_POINT('',(0.00752505549789501,-0.0318665617511268,0.0684298906187498));
#77098=CARTESIAN_POINT('Origin',(0.00820141015539198,-0.0326371944420527,
0.0851141202804744));
#77099=CARTESIAN_POINT('Origin',(0.00638397650341509,-0.0316939261509635,
0.0575282609788763));
#77100=CARTESIAN_POINT('',(0.00788514356785206,-0.0320197221621866,0.0684036410856033));
#77101=CARTESIAN_POINT('Ctrl Pts',(0.00788496291033336,-0.0320197392094778,
0.0684036013648333));
#77102=CARTESIAN_POINT('Ctrl Pts',(0.00785572338860702,-0.0319792716576076,
0.0684048166010218));
#77103=CARTESIAN_POINT('Ctrl Pts',(0.00782636002191936,-0.0319386439829735,
0.0684062602797732));
#77104=CARTESIAN_POINT('Ctrl Pts',(0.00779684239961052,-0.0318979099381666,
0.0684079423639928));
#77105=CARTESIAN_POINT('Ctrl Pts',(0.00776732536073717,-0.0318571766984953,
0.0684096244149649));
#77106=CARTESIAN_POINT('Ctrl Pts',(0.0077378039958447,-0.0318163871833588,
0.0684115345338993));
#77107=CARTESIAN_POINT('Ctrl Pts',(0.00770837961891253,-0.0317755399638303,
0.068413662636967));
#77108=CARTESIAN_POINT('',(0.00788546189524767,-0.0321934096636183,0.0684049409545569));
#77109=CARTESIAN_POINT('Origin',(0.00776873771683435,-0.0324113708469043,
0.0660987583219195));
#77110=CARTESIAN_POINT('',(0.00782301560125816,-0.0321934096636663,0.0684075313925888));
#77111=CARTESIAN_POINT('Ctrl Pts',(0.007762061687006,-0.0321934096636618,
0.0684114953261555));
#77112=CARTESIAN_POINT('Ctrl Pts',(0.00768292323522471,-0.0320835708272592,
0.0684164837338431));
#77113=CARTESIAN_POINT('Ctrl Pts',(0.00760393392179947,-0.0319739230346488,
0.0684231070141982));
#77114=CARTESIAN_POINT('Ctrl Pts',(0.00752519415771869,-0.0318646057455573,
0.0684313489370169));
#77115=CARTESIAN_POINT('Ctrl Pts',(0.00767868091641969,-0.0321934096636618,
0.0683347567318175));
#77116=CARTESIAN_POINT('Ctrl Pts',(0.00759848417961592,-0.0320835708272592,
0.0683408950253147));
#77117=CARTESIAN_POINT('Ctrl Pts',(0.00751846099184358,-0.0319739230346488,
0.0683486894256524));
#77118=CARTESIAN_POINT('Ctrl Pts',(0.00743871297186613,-0.0318646057455573,
0.068358122102741));
#77119=CARTESIAN_POINT('Ctrl Pts',(0.00759530014583338,-0.0321934096636618,
0.0682580181374796));
#77120=CARTESIAN_POINT('Ctrl Pts',(0.00751404512400712,-0.0320835708272592,
0.0682653063167864));
#77121=CARTESIAN_POINT('Ctrl Pts',(0.00743298806188769,-0.0319739230346488,
0.0682742718371066));
#77122=CARTESIAN_POINT('Ctrl Pts',(0.00735223178601357,-0.0318646057455573,
0.0682848952684651));
#77123=CARTESIAN_POINT('Ctrl Pts',(0.00751191937524706,-0.0321934096636618,
0.0681812795431417));
#77124=CARTESIAN_POINT('Ctrl Pts',(0.00742960606839833,-0.0320835708272592,
0.068189717608258));
#77125=CARTESIAN_POINT('Ctrl Pts',(0.0073475151319318,-0.0319739230346488,
0.0681998542485608));
#77126=CARTESIAN_POINT('Ctrl Pts',(0.00726575060016101,-0.0318646057455573,
0.0682116684341893));
#77127=CARTESIAN_POINT('',(0.00749917147742976,-0.0321763980308455,0.0681826001113111));
#77128=CARTESIAN_POINT('',(0.0075119193752146,-0.0321934096636184,0.068181279543145));
#77129=CARTESIAN_POINT('Origin',(0.00861046215821728,-0.0326386231061021,
0.0846929340187781));
#77130=CARTESIAN_POINT('Ctrl Pts',(0.00749917147775506,-0.0321763980306277,
0.0681826001144621));
#77131=CARTESIAN_POINT('Ctrl Pts',(0.00750363941120969,-0.0321259596174824,
0.0682252858144191));
#77132=CARTESIAN_POINT('Ctrl Pts',(0.00750802993192638,-0.0320749164631392,
0.0682672319292351));
#77133=CARTESIAN_POINT('Ctrl Pts',(0.00751665968120572,-0.0319716057793906,
0.0683496787454615));
#77134=CARTESIAN_POINT('Ctrl Pts',(0.00752089554732806,-0.03191937866901,
0.0683901473228217));
#77135=CARTESIAN_POINT('Ctrl Pts',(0.00752505549808159,-0.0318665617525276,
0.0684298906205918));
#77136=CARTESIAN_POINT('',(0.00763624434124162,-0.0321934096636663,0.0682957006868829));
#77137=CARTESIAN_POINT('Origin',(0.00812378219310841,-0.0315241814719618,
0.07415));
#77138=CARTESIAN_POINT('',(0.00749917147739109,-0.0322104233323794,0.068182600110942));
#77139=CARTESIAN_POINT('',(0.00748642642908507,-0.0321934096636183,0.0681839479024995));
#77140=CARTESIAN_POINT('Origin',(0.00865576766829494,-0.0326387235197539,
0.0846945433864166));
#77141=CARTESIAN_POINT('Origin',(0.00983080235707136,-0.0326386242537259,
0.0845652026842633));
#77142=CARTESIAN_POINT('Origin',(0.00978681119076951,-0.0326387243745439,
0.0845761540139851));
#77143=CARTESIAN_POINT('Ctrl Pts',(0.00768554811731203,-0.0327445246967097,
0.0684153617468221));
#77144=CARTESIAN_POINT('Ctrl Pts',(0.0074692626998059,-0.032443687833936,
0.0684318900151914));
#77145=CARTESIAN_POINT('Ctrl Pts',(0.00725483670305344,-0.0321434074405927,
0.0684646628301117));
#77146=CARTESIAN_POINT('Ctrl Pts',(0.00743674780973492,-0.0327445246967097,
0.0684398241046301));
#77147=CARTESIAN_POINT('Ctrl Pts',(0.00722138500513619,-0.032443687833936,
0.0684657360300016));
#77148=CARTESIAN_POINT('Ctrl Pts',(0.00700858581564219,-0.0321434074405927,
0.0685077963489708));
#77149=CARTESIAN_POINT('',(0.0074008760926723,-0.0326943950436611,0.0684442544948138));
#77150=CARTESIAN_POINT('',(0.00716706830828393,-0.0323666188837389,0.0684787723072879));
#77151=CARTESIAN_POINT('Origin',(0.00958928232954848,-0.0326395579112405,
0.0851121558730604));
#77152=CARTESIAN_POINT('Origin',(0.00532984421989297,-0.0321933825603065,
0.057588043245766));
#77153=CARTESIAN_POINT('',(0.00729055273794418,-0.0321934096532689,0.0684593186988152));
#77154=CARTESIAN_POINT('',(0.00722892351684091,-0.0321934096584275,0.0684697153065266));
#77155=CARTESIAN_POINT('',(0.00752505549779406,-0.0325210109756239,0.0684298906178012));
#77156=CARTESIAN_POINT('Origin',(0.00910975440756268,-0.0326393129158705,
0.0851473325956557));
#77157=CARTESIAN_POINT('',(0.00752519692372645,-0.0326943950436593,0.0684312417715662));
#77158=CARTESIAN_POINT('Origin',(0.00637357625577623,-0.032694376553807,
0.0574288926357137));
#77159=CARTESIAN_POINT('',(0.00746303650820937,-0.0326943950436702,0.0684377481331999));
#77160=CARTESIAN_POINT('Ctrl Pts',(0.0077335540589646,-0.0325229783203769,
0.0681627032808331));
#77161=CARTESIAN_POINT('Ctrl Pts',(0.00765101930462442,-0.032413025309245,
0.0681680825671286));
#77162=CARTESIAN_POINT('Ctrl Pts',(0.00756860834574407,-0.032303122220807,
0.0681751683749668));
#77163=CARTESIAN_POINT('Ctrl Pts',(0.00748642642462623,-0.0321934096576658,
0.0681839479029759));
#77164=CARTESIAN_POINT('Ctrl Pts',(0.00766411058425769,-0.0325229783203769,
0.0682522507322593));
#77165=CARTESIAN_POINT('Ctrl Pts',(0.00758281023957715,-0.032413025309245,
0.068258587295335));
#77166=CARTESIAN_POINT('Ctrl Pts',(0.00750165330563394,-0.032303122220807,
0.0682666046994141));
#77167=CARTESIAN_POINT('Ctrl Pts',(0.007420743376306,-0.0321934096576658,
0.0682762890064978));
#77168=CARTESIAN_POINT('Ctrl Pts',(0.00759466710955079,-0.0325229783203769,
0.0683417981836855));
#77169=CARTESIAN_POINT('Ctrl Pts',(0.00751460117452988,-0.032413025309245,
0.0683490920235413));
#77170=CARTESIAN_POINT('Ctrl Pts',(0.00743469826552381,-0.032303122220807,
0.0683580410238614));
#77171=CARTESIAN_POINT('Ctrl Pts',(0.00735506032798578,-0.0321934096576658,
0.0683686301100198));
#77172=CARTESIAN_POINT('Ctrl Pts',(0.00752522363484389,-0.0325229783203769,
0.0684313456351116));
#77173=CARTESIAN_POINT('Ctrl Pts',(0.00744639210948262,-0.032413025309245,
0.0684395967517477));
#77174=CARTESIAN_POINT('Ctrl Pts',(0.00736774322541367,-0.032303122220807,
0.0684494773483087));
#77175=CARTESIAN_POINT('Ctrl Pts',(0.00728937727966555,-0.0321934096576658,
0.0684609712135418));
#77176=CARTESIAN_POINT('',(0.00738848958398549,-0.0321934096584275,0.0683216333004508));
#77177=CARTESIAN_POINT('Ctrl Pts',(0.00749917147774838,-0.0322104233328942,
0.0681826001143968));
#77178=CARTESIAN_POINT('Ctrl Pts',(0.00750364546532274,-0.0322609421831134,
0.0682253436541457));
#77179=CARTESIAN_POINT('Ctrl Pts',(0.00750803894356958,-0.0323120888240227,
0.0682673180246502));
#77180=CARTESIAN_POINT('Ctrl Pts',(0.00751666875819141,-0.0324156524631819,
0.0683497654651452));
#77181=CARTESIAN_POINT('Ctrl Pts',(0.00752090154725391,-0.0324680267167318,
0.0683902046448552));
#77182=CARTESIAN_POINT('Ctrl Pts',(0.00752505549779413,-0.0325210109755912,
0.0684298906178448));
#77183=CARTESIAN_POINT('Origin',(0.0159905897868985,-0.0262834582512493,
0.0742793217685553));
#77184=CARTESIAN_POINT('Origin',(0.0124014873473407,-0.0342770978491508,
0.0627690532049329));
#77185=CARTESIAN_POINT('Ctrl Pts',(0.00740245138760245,-0.0326943950436603,
0.068445531262888));
#77186=CARTESIAN_POINT('Ctrl Pts',(0.00732383311709117,-0.0325844576448133,
0.0684554725533059));
#77187=CARTESIAN_POINT('Ctrl Pts',(0.00724541488482755,-0.0324744968375322,
0.068467040502015));
#77188=CARTESIAN_POINT('Ctrl Pts',(0.00716729696039047,-0.0323646534831894,
0.068480218901646));
#77189=CARTESIAN_POINT('Ctrl Pts',(0.00731441682117113,-0.0326943950436603,
0.0683741797198448));
#77190=CARTESIAN_POINT('Ctrl Pts',(0.00723481519266967,-0.0325844576448133,
0.0683853342915824));
#77191=CARTESIAN_POINT('Ctrl Pts',(0.00715543862546899,-0.0324744968375322,
0.0683981359449325));
#77192=CARTESIAN_POINT('Ctrl Pts',(0.00707638859522006,-0.0323646534831894,
0.0684125668748955));
#77193=CARTESIAN_POINT('Ctrl Pts',(0.00722638225473981,-0.0326943950436603,
0.0683028281768015));
#77194=CARTESIAN_POINT('Ctrl Pts',(0.00714579726824817,-0.0325844576448133,
0.0683151960298589));
#77195=CARTESIAN_POINT('Ctrl Pts',(0.00706546236611043,-0.0324744968375322,
0.0683292313878501));
#77196=CARTESIAN_POINT('Ctrl Pts',(0.00698548023004965,-0.0323646534831894,
0.068344914848145));
#77197=CARTESIAN_POINT('Ctrl Pts',(0.00713834768830848,-0.0326943950436603,
0.0682314766337582));
#77198=CARTESIAN_POINT('Ctrl Pts',(0.00705677934382667,-0.0325844576448133,
0.0682450577681354));
#77199=CARTESIAN_POINT('Ctrl Pts',(0.00697548610675187,-0.0324744968375322,
0.0682603268307676));
#77200=CARTESIAN_POINT('Ctrl Pts',(0.00689457186487923,-0.0323646534831894,
0.0682772628213945));
#77201=CARTESIAN_POINT('',(0.00712570786471424,-0.0326773559991336,0.0682335950430089));
#77202=CARTESIAN_POINT('',(0.0071383476883078,-0.0326943950436594,0.0682314766337583));
#77203=CARTESIAN_POINT('Origin',(0.00993744315770636,-0.0326395670738684,
0.0845990298098265));
#77204=CARTESIAN_POINT('Ctrl Pts',(0.00712570786526682,-0.0326773559987419,
0.068233595046309));
#77205=CARTESIAN_POINT('Ctrl Pts',(0.00713285298483651,-0.0326267922585964,
0.0682759500289366));
#77206=CARTESIAN_POINT('Ctrl Pts',(0.00713987146232143,-0.0325756109579333,
0.0683175543000823));
#77207=CARTESIAN_POINT('Ctrl Pts',(0.0071536611061937,-0.0324719985462369,
0.0683992968267055));
#77208=CARTESIAN_POINT('Ctrl Pts',(0.00716042674193148,-0.0324196091621777,
0.068439402297488));
#77209=CARTESIAN_POINT('Ctrl Pts',(0.0071670683082921,-0.0323666188837756,
0.0684787723073359));
#77210=CARTESIAN_POINT('',(0.00726961189050005,-0.0326943950436702,0.0683378655642961));
#77211=CARTESIAN_POINT('Origin',(0.00812378219310841,-0.0315241814719618,
0.07415));
#77212=CARTESIAN_POINT('',(0.00712570786472155,-0.0327114338379883,0.0682335950430528));
#77213=CARTESIAN_POINT('',(0.00711307259435397,-0.0326943950436593,0.0682357404430475));
#77214=CARTESIAN_POINT('Origin',(0.0099819871076458,-0.0326395670367085,
0.0845907295957668));
#77215=CARTESIAN_POINT('Origin',(0.00983836293701956,-0.0326395678116252,
0.084615746030193));
#77216=CARTESIAN_POINT('Origin',(0.00979356073219717,-0.0326395679143015,
0.0846225142356918));
#77217=CARTESIAN_POINT('Ctrl Pts',(0.00732629311210369,-0.0332451089994433,
0.0684542001294218));
#77218=CARTESIAN_POINT('Ctrl Pts',(0.00711147250533561,-0.0329451141710254,
0.0684842779222104));
#77219=CARTESIAN_POINT('Ctrl Pts',(0.00689952776355092,-0.0326442513127493,
0.0685304514334594));
#77220=CARTESIAN_POINT('Ctrl Pts',(0.00707952003230626,-0.0332451089994433,
0.0684942381998959));
#77221=CARTESIAN_POINT('Ctrl Pts',(0.006866209486072,-0.0329451141710254,
0.0685336231916627));
#77222=CARTESIAN_POINT('Ctrl Pts',(0.00665647157117369,-0.0326442513127493,
0.0685889637171875));
#77223=CARTESIAN_POINT('Ctrl Pts',(0.00707705230150829,-0.0332451089994433,
0.0684946385806006));
#77224=CARTESIAN_POINT('Ctrl Pts',(0.00686375685587936,-0.0329451141710254,
0.0685341166443573));
#77225=CARTESIAN_POINT('Ctrl Pts',(0.00665404100924992,-0.0326442513127493,
0.0685895488400247));
#77226=CARTESIAN_POINT('',(0.00704403585815591,-0.0331951640388616,0.0685009051298321));
#77227=CARTESIAN_POINT('',(0.00681285681644229,-0.032867753235499,0.0685500357388078));
#77228=CARTESIAN_POINT('Origin',(0.0109422950086399,-0.0326402808281317,
0.0848053776164348));
#77229=CARTESIAN_POINT('Origin',(0.00429246866519795,-0.0326944278779127,
0.0577851842994068));
#77230=CARTESIAN_POINT('',(0.00693487608410739,-0.0326943950436593,0.0685228668698901));
#77231=CARTESIAN_POINT('',(0.00687402128537481,-0.0326943950436693,0.0685371126927966));
#77232=CARTESIAN_POINT('',(0.00716706830828674,-0.0330220786163545,0.0684787723072874));
#77233=CARTESIAN_POINT('Origin',(0.0104823291870166,-0.0326396682763501,
0.0849453207766407));
#77234=CARTESIAN_POINT('',(0.00716729429479589,-0.0331951640388587,0.068480111914651));
#77235=CARTESIAN_POINT('Origin',(0.00533222690299956,-0.0331952026559981,
0.0576021572729662));
#77236=CARTESIAN_POINT('',(0.0071056650764859,-0.0331951640388701,0.0684905085222516));
#77237=CARTESIAN_POINT('Ctrl Pts',(0.00735837766043643,-0.0330240426238172,
0.068199020593097));
#77238=CARTESIAN_POINT('Ctrl Pts',(0.00727639712134802,-0.032914277406352,
0.068209564786232));
#77239=CARTESIAN_POINT('Ctrl Pts',(0.00719459368989688,-0.0328043479726691,
0.0682218090027762));
#77240=CARTESIAN_POINT('Ctrl Pts',(0.007113072594354,-0.0326943950436593,
0.0682357404430475));
#77241=CARTESIAN_POINT('Ctrl Pts',(0.00729469397807497,-0.0330240426238172,
0.0682927517223196));
#77242=CARTESIAN_POINT('Ctrl Pts',(0.00721400467660942,-0.032914277406352,
0.0683041732202231));
#77243=CARTESIAN_POINT('Ctrl Pts',(0.00713351126285038,-0.0328043479726691,
0.0683172684854157));
#77244=CARTESIAN_POINT('Ctrl Pts',(0.00705331731686408,-0.0326943950436593,
0.0683320235817404));
#77245=CARTESIAN_POINT('Ctrl Pts',(0.00723101029571351,-0.0330240426238172,
0.0683864828515421));
#77246=CARTESIAN_POINT('Ctrl Pts',(0.00715161223187082,-0.0329142774063519,
0.0683987816542143));
#77247=CARTESIAN_POINT('Ctrl Pts',(0.00707242883580387,-0.0328043479726691,
0.0684127279680553));
#77248=CARTESIAN_POINT('Ctrl Pts',(0.00699356203937417,-0.0326943950436593,
0.0684283067204333));
#77249=CARTESIAN_POINT('Ctrl Pts',(0.00716732661335206,-0.0330240426238172,
0.0684802139807647));
#77250=CARTESIAN_POINT('Ctrl Pts',(0.00708921978713222,-0.0329142774063519,
0.0684933900882054));
#77251=CARTESIAN_POINT('Ctrl Pts',(0.00701134640875737,-0.0328043479726691,
0.0685081874506948));
#77252=CARTESIAN_POINT('Ctrl Pts',(0.00693380676188425,-0.0326943950436593,
0.0685245898591262));
#77253=CARTESIAN_POINT('',(0.00702397433924068,-0.0326943950436693,0.0683793036564788));
#77254=CARTESIAN_POINT('Ctrl Pts',(0.00712570786526824,-0.0327114338383338,
0.0682335950463169));
#77255=CARTESIAN_POINT('Ctrl Pts',(0.00713285179636839,-0.0327619876830847,
0.0682759429839112));
#77256=CARTESIAN_POINT('Ctrl Pts',(0.00713986969334866,-0.0328131562604072,
0.0683175438139299));
#77257=CARTESIAN_POINT('Ctrl Pts',(0.00715365932456068,-0.0329167375858778,
0.0683992862655054));
#77258=CARTESIAN_POINT('Ctrl Pts',(0.00716042556428761,-0.0329691088920624,
0.0684393953166267));
#77259=CARTESIAN_POINT('Ctrl Pts',(0.00716706830829191,-0.0330220786163187,
0.0684787723073348));
#77260=CARTESIAN_POINT('Ctrl Pts',(0.00704568847732885,-0.0331951640388604,
0.0685020806525492));
#77261=CARTESIAN_POINT('Ctrl Pts',(0.00692892136592929,-0.0330306422010619,
0.0685243695489135));
#77262=CARTESIAN_POINT('Ctrl Pts',(0.00681317525473458,-0.0328657861914645,
0.0685514655070815));
#77263=CARTESIAN_POINT('Ctrl Pts',(0.007044035858159,-0.0331951640388604,
0.0685009051298316));
#77264=CARTESIAN_POINT('Ctrl Pts',(0.00692724444358094,-0.0330306422010619,
0.0685232281930377));
#77265=CARTESIAN_POINT('Ctrl Pts',(0.00681147546212611,-0.0328657861914645,
0.068550359293328));
#77266=CARTESIAN_POINT('Ctrl Pts',(0.0067686650611903,-0.0331951640388604,
0.0683050314321819));
#77267=CARTESIAN_POINT('Ctrl Pts',(0.00664782408349586,-0.0330306422010619,
0.0683330476100639));
#77268=CARTESIAN_POINT('Ctrl Pts',(0.00652824430166454,-0.0328657861914645,
0.0683660343330059));
#77269=CARTESIAN_POINT('',(0.00675618319574967,-0.0331781648281891,0.0683079393209088));
#77270=CARTESIAN_POINT('',(0.00676866506118923,-0.0331951640388588,0.0683050314321821));
#77271=CARTESIAN_POINT('Origin',(0.0112121800492513,-0.0326412092471448,
0.0842180170307076));
#77272=CARTESIAN_POINT('Ctrl Pts',(0.00675618319744972,-0.033178164828644,
0.0683079393215935));
#77273=CARTESIAN_POINT('Ctrl Pts',(0.00676598046126932,-0.0331276811546782,
0.0683497908710576));
#77274=CARTESIAN_POINT('Ctrl Pts',(0.00677560084977164,-0.0330765663497795,
0.0683908867034381));
#77275=CARTESIAN_POINT('Ctrl Pts',(0.00679449598386189,-0.0329730614463221,
0.0684716022795236));
#77276=CARTESIAN_POINT('Ctrl Pts',(0.00680376309100563,-0.0329207133374056,
0.0685111894171055));
#77277=CARTESIAN_POINT('Ctrl Pts',(0.00681285682806447,-0.032867753228935,
0.0685500357271382));
#77278=CARTESIAN_POINT('',(0.00690635045968257,-0.0331951640388701,0.0684029682810171));
#77279=CARTESIAN_POINT('Origin',(0.00812378219310841,-0.0315241814719618,
0.07415));
#77280=CARTESIAN_POINT('',(0.00675618319547328,-0.033212160714443,0.068307939322566));
#77281=CARTESIAN_POINT('',(0.00674370756866027,-0.0331951640388587,0.0683108738640981));
#77282=CARTESIAN_POINT('Origin',(0.0112538793822697,-0.0326413652941119,
0.0842002015163731));
#77283=CARTESIAN_POINT('Origin',(0.00982514711364439,-0.0326412099009382,
0.0845427171574036));
#77284=CARTESIAN_POINT('Origin',(0.00977987220206338,-0.0326413661470917,
0.0845452574844475));
#77285=CARTESIAN_POINT('Ctrl Pts',(0.0069702449498819,-0.0337436976235975,
0.0685155100649225));
#77286=CARTESIAN_POINT('Ctrl Pts',(0.00691956749347552,-0.0336723290703325,
0.0685258851537115));
#77287=CARTESIAN_POINT('Ctrl Pts',(0.00686908485063321,-0.033601104548885,
0.0685371700917642));
#77288=CARTESIAN_POINT('Ctrl Pts',(0.0067079037720858,-0.0333736987606857,
0.0685732006635465));
#77289=CARTESIAN_POINT('Ctrl Pts',(0.00654905594916388,-0.0331450831799191,
0.068618421359446));
#77290=CARTESIAN_POINT('Ctrl Pts',(0.00672647263077907,-0.0337436976235975,
0.0685709632563478));
#77291=CARTESIAN_POINT('Ctrl Pts',(0.00667629392878052,-0.0336723290703325,
0.0685835308703194));
#77292=CARTESIAN_POINT('Ctrl Pts',(0.00662634939627669,-0.033601104548885,
0.0685969990078362));
#77293=CARTESIAN_POINT('Ctrl Pts',(0.00646688639744637,-0.0333736987606857,
0.0686400001030398));
#77294=CARTESIAN_POINT('Ctrl Pts',(0.00631015383180769,-0.0331450831799191,
0.0686920812421688));
#77295=CARTESIAN_POINT('Ctrl Pts',(0.00672403490758804,-0.0337436976235975,
0.0685715177882619));
#77296=CARTESIAN_POINT('Ctrl Pts',(0.00667386119313358,-0.0336723290703325,
0.0685841073274855));
#77297=CARTESIAN_POINT('Ctrl Pts',(0.00662392204173313,-0.033601104548885,
0.0685975972969969));
#77298=CARTESIAN_POINT('Ctrl Pts',(0.00646447622369998,-0.0333736987606857,
0.0686406680974347));
#77299=CARTESIAN_POINT('Ctrl Pts',(0.00630776481063412,-0.0331450831799191,
0.0686928178409961));
#77300=CARTESIAN_POINT('',(0.0066914568891216,-0.0336938721132548,0.0685798501614804));
#77301=CARTESIAN_POINT('',(0.00646381896393862,-0.0333679870047995,0.0686433996805959));
#77302=CARTESIAN_POINT('Ctrl Pts',(0.00669145688914577,-0.0336938721132519,
0.0685798501614743));
#77303=CARTESIAN_POINT('Ctrl Pts',(0.00666971398131391,-0.0336629187933865,
0.0685854411990537));
#77304=CARTESIAN_POINT('Ctrl Pts',(0.00664801076515907,-0.0336319952301003,
0.0685911577619526));
#77305=CARTESIAN_POINT('Ctrl Pts',(0.00662634939628842,-0.0336011045488913,
0.0685969990078332));
#77306=CARTESIAN_POINT('Ctrl Pts',(0.00657199360968862,-0.0335235892595416,
0.0686116566925097));
#77307=CARTESIAN_POINT('Ctrl Pts',(0.0065178047823149,-0.033445866866553,
0.0686271256697595));
#77308=CARTESIAN_POINT('Ctrl Pts',(0.00646381897517569,-0.0333679869962453,
0.0686433996769363));
#77309=CARTESIAN_POINT('Ctrl Pts',(0.00646377619489206,-0.0333679692470407,
0.0686434118550933));
#77310=CARTESIAN_POINT('Ctrl Pts',(0.00646391267711552,-0.0333391895417761,
0.0686438440707583));
#77311=CARTESIAN_POINT('Ctrl Pts',(0.00646401807368413,-0.0333104081135165,
0.0686441670597292));
#77312=CARTESIAN_POINT('Ctrl Pts',(0.0064641628490814,-0.0332532699115172,
0.0686445928721591));
#77313=CARTESIAN_POINT('Ctrl Pts',(0.00646420318974104,-0.0332249175515492,
0.068644698910686));
#77314=CARTESIAN_POINT('Ctrl Pts',(0.00646421085788016,-0.0331960985192758,
0.0686447004327229));
#77315=CARTESIAN_POINT('Ctrl Pts',(0.0064642109733624,-0.0331956312733899,
0.0686447004289874));
#77316=CARTESIAN_POINT('Ctrl Pts',(0.00646421107987799,-0.0331951640388603,
0.0686447003968783));
#77317=CARTESIAN_POINT('',(0.00658389150603356,-0.0331951640388587,0.0686086227639818));
#77318=CARTESIAN_POINT('',(0.00652405129296613,-0.0331951640388687,0.0686266615804399));
#77319=CARTESIAN_POINT('',(0.00681285683165936,-0.0335216366567744,0.0685500357418976));
#77320=CARTESIAN_POINT('Origin',(0.0117779965714527,-0.0326434571527492,
0.0844471440443612));
#77321=CARTESIAN_POINT('',(0.00681316648662222,-0.0336938721132326,0.0685513585156833));
#77322=CARTESIAN_POINT('Origin',(0.00432400742965567,-0.0336938867896239,
0.0579182537421924));
#77323=CARTESIAN_POINT('',(0.00675231168788191,-0.0336938721132537,0.0685656043385918));
#77324=CARTESIAN_POINT('Ctrl Pts',(0.00698622197913881,-0.0335235895815172,
0.0682588238220527));
#77325=CARTESIAN_POINT('Ctrl Pts',(0.00690511834039081,-0.0334144449262748,
0.0682744845780479));
#77326=CARTESIAN_POINT('Ctrl Pts',(0.00682424506282069,-0.0333049234473147,
0.0682918388664937));
#77327=CARTESIAN_POINT('Ctrl Pts',(0.00674370756866033,-0.0331951640388587,
0.0683108738640979));
#77328=CARTESIAN_POINT('Ctrl Pts',(0.00692854932193361,-0.0335235895815172,
0.0683563688736789));
#77329=CARTESIAN_POINT('Ctrl Pts',(0.00684878858286978,-0.0334144449262748,
0.0683728236073476));
#77330=CARTESIAN_POINT('Ctrl Pts',(0.00676927615079407,-0.0333049234473147,
0.0683909450423542));
#77331=CARTESIAN_POINT('Ctrl Pts',(0.00669011579669301,-0.0331951640388587,
0.0684107192168355));
#77332=CARTESIAN_POINT('Ctrl Pts',(0.00687087666472841,-0.0335235895815172,
0.0684539139253052));
#77333=CARTESIAN_POINT('Ctrl Pts',(0.00679245882534875,-0.0334144449262748,
0.0684711626366474));
#77334=CARTESIAN_POINT('Ctrl Pts',(0.00671430723876745,-0.0333049234473147,
0.0684900512182147));
#77335=CARTESIAN_POINT('Ctrl Pts',(0.00663652402472568,-0.0331951640388587,
0.068510564569573));
#77336=CARTESIAN_POINT('Ctrl Pts',(0.00681320400752322,-0.0335235895815172,
0.0685514589769314));
#77337=CARTESIAN_POINT('Ctrl Pts',(0.00673612906782772,-0.0334144449262748,
0.0685695016659471));
#77338=CARTESIAN_POINT('Ctrl Pts',(0.00665933832674083,-0.0333049234473147,
0.0685891573940752));
#77339=CARTESIAN_POINT('Ctrl Pts',(0.00658293225275836,-0.0331951640388587,
0.0686104099223105));
#77340=CARTESIAN_POINT('',(0.00666379953735691,-0.0331951640388687,0.0684597483140499));
#77341=CARTESIAN_POINT('Ctrl Pts',(0.00675618319618243,-0.0332121607145991,
0.0683079393256107));
#77342=CARTESIAN_POINT('Ctrl Pts',(0.00676596396673557,-0.0332625444109669,
0.0683497204728199));
#77343=CARTESIAN_POINT('Ctrl Pts',(0.00677557619926364,-0.0333135300746636,
0.0683907816652977));
#77344=CARTESIAN_POINT('Ctrl Pts',(0.00679447121834327,-0.0334167203140648,
0.0684714967346675));
#77345=CARTESIAN_POINT('Ctrl Pts',(0.00680374668669211,-0.0334688847587346,
0.0685111193499218));
#77346=CARTESIAN_POINT('Ctrl Pts',(0.00681285683165345,-0.0335216366562431,
0.0685500357426192));
#77347=CARTESIAN_POINT('Ctrl Pts',(0.00669317965594853,-0.0336938721132518,
0.0685809193456466));
#77348=CARTESIAN_POINT('Ctrl Pts',(0.00666058197885721,-0.0336474569765022,
0.068589293137022));
#77349=CARTESIAN_POINT('Ctrl Pts',(0.00662808456118034,-0.033601104548885,
0.068598047951588));
#77350=CARTESIAN_POINT('Ctrl Pts',(0.00654580857125863,-0.0334837508592655,
0.068620213129208));
#77351=CARTESIAN_POINT('Ctrl Pts',(0.00646422551105693,-0.0333660264659096,
0.0686448065816831));
#77352=CARTESIAN_POINT('Ctrl Pts',(0.0066914568891505,-0.0336938721132518,
0.068579850161473));
#77353=CARTESIAN_POINT('Ctrl Pts',(0.00665885295376941,-0.0336474569765022,
0.0685882340367742));
#77354=CARTESIAN_POINT('Ctrl Pts',(0.00662634939627669,-0.033601104548885,
0.0685969990078362));
#77355=CARTESIAN_POINT('Ctrl Pts',(0.00654405786175287,-0.0334837508592655,
0.0686191898993688));
#77356=CARTESIAN_POINT('Ctrl Pts',(0.00646246002573164,-0.0333660264659096,
0.0686438095150837));
#77357=CARTESIAN_POINT('Ctrl Pts',(0.00640260770369985,-0.0336938721132518,
0.0684005844721348));
#77358=CARTESIAN_POINT('Ctrl Pts',(0.00636895446675226,-0.0336474569765022,
0.068410659077569));
#77359=CARTESIAN_POINT('Ctrl Pts',(0.00633542147172276,-0.033601104548885,
0.0684211269463137));
#77360=CARTESIAN_POINT('Ctrl Pts',(0.00625052363803872,-0.0334837508592655,
0.0684476291832578));
#77361=CARTESIAN_POINT('Ctrl Pts',(0.00616644840145523,-0.0333660264659096,
0.0684766354812069));
#77362=CARTESIAN_POINT('',(0.00639205581408608,-0.0336769361243753,0.0684053395445685));
#77363=CARTESIAN_POINT('',(0.00640433046229623,-0.0336938721132327,0.0684016536512309));
#77364=CARTESIAN_POINT('Ctrl Pts',(0.00639205581408579,-0.033676936124375,
0.0684053395445686));
#77365=CARTESIAN_POINT('Ctrl Pts',(0.00639410108586206,-0.0336797586670244,
0.0684047229979311));
#77366=CARTESIAN_POINT('Ctrl Pts',(0.00639614660954832,-0.0336825812713284,
0.0684041075668789));
#77367=CARTESIAN_POINT('Ctrl Pts',(0.00640023816625122,-0.033688226610976,
0.0684028789337534));
#77368=CARTESIAN_POINT('Ctrl Pts',(0.0064022841993198,-0.0336910493463751,
0.0684022657316887));
#77369=CARTESIAN_POINT('Ctrl Pts',(0.00640433046230283,-0.0336938721132293,
0.0684016536512373));
#77370=CARTESIAN_POINT('Ctrl Pts',(0.00639205581408608,-0.0336769361243753,
0.0684053395445686));
#77371=CARTESIAN_POINT('Ctrl Pts',(0.00640415332488983,-0.0336278994613247,
0.0684454706488616));
#77372=CARTESIAN_POINT('Ctrl Pts',(0.00641642307030404,-0.0335767852527761,
0.0684861731074774));
#77373=CARTESIAN_POINT('Ctrl Pts',(0.00644046770507109,-0.0334733171841366,
0.0685659364374034));
#77374=CARTESIAN_POINT('Ctrl Pts',(0.00645225692480437,-0.0334209631343272,
0.0686050448469222));
#77375=CARTESIAN_POINT('Ctrl Pts',(0.00646381897801536,-0.0333679869844681,
0.0686433996763394));
#77376=CARTESIAN_POINT('',(0.00654789367571891,-0.0336938721132538,0.0684907519063656));
#77377=CARTESIAN_POINT('Origin',(0.00812378219310841,-0.0315241814719618,
0.07415));
#77378=CARTESIAN_POINT('',(0.0063920558144654,-0.033710812065585,0.0684053395458166));
#77379=CARTESIAN_POINT('',(0.00637978906701309,-0.0336938721132327,0.068409051648364));
#77380=CARTESIAN_POINT('Origin',(0.0100442027223466,-0.0345562517227294,
0.0843928399467902));
#77381=CARTESIAN_POINT('Ctrl Pts',(0.00637978906701234,-0.0336938721132314,
0.0684090516483674));
#77382=CARTESIAN_POINT('Ctrl Pts',(0.00638183270751947,-0.0336910493311555,
0.0684084308284648));
#77383=CARTESIAN_POINT('Ctrl Pts',(0.00638387675977588,-0.0336882266033658,
0.0684078110754133));
#77384=CARTESIAN_POINT('Ctrl Pts',(0.00638796567720988,-0.0336825812712471,
0.0684065737067743));
#77385=CARTESIAN_POINT('Ctrl Pts',(0.00639001054233957,-0.0336797586669837,
0.068405956091197));
#77386=CARTESIAN_POINT('Ctrl Pts',(0.00639205581408636,-0.033676936124375,
0.0684053395445684));
#77387=CARTESIAN_POINT('Origin',(0.0121842899637513,-0.0345562518086802,
0.0837477087828097));
#77388=CARTESIAN_POINT('Ctrl Pts',(0.00661877848008525,-0.034243627687391,
0.0685990461338805));
#77389=CARTESIAN_POINT('Ctrl Pts',(0.0064094208037195,-0.033943005420181,
0.0686558082846532));
#77390=CARTESIAN_POINT('Ctrl Pts',(0.00620493344833617,-0.0336441434784053,
0.0687281788581062));
#77391=CARTESIAN_POINT('Ctrl Pts',(0.00637896849035594,-0.034243627687391,
0.0686696943385713));
#77392=CARTESIAN_POINT('Ctrl Pts',(0.00617227535495563,-0.033943005420181,
0.0687355010722084));
#77393=CARTESIAN_POINT('Ctrl Pts',(0.00597112624589656,-0.0336441434784053,
0.0688166898296711));
#77394=CARTESIAN_POINT('Ctrl Pts',(0.00637657039045866,-0.034243627687391,
0.0686704008206182));
#77395=CARTESIAN_POINT('Ctrl Pts',(0.00616990390046798,-0.033943005420181,
0.0687362980000839));
#77396=CARTESIAN_POINT('Ctrl Pts',(0.00596878817387217,-0.0336441434784053,
0.0688175749393868));
#77397=CARTESIAN_POINT('',(0.00634453065372381,-0.034193496108874,0.0686807780297744));
#77398=CARTESIAN_POINT('',(0.0061213322399811,-0.0338664212864867,0.0687584956471367));
#77399=CARTESIAN_POINT('Origin',(0.0110346308465843,-0.0345610720405585,
0.0847449027782907));
#77400=CARTESIAN_POINT('Origin',(0.00230317710792826,-0.033693800507297,
0.05847839760108));
#77401=CARTESIAN_POINT('',(0.00623898417299239,-0.0336938721132327,0.0687162479424096));
#77402=CARTESIAN_POINT('',(0.00618039470757276,-0.0336938721132427,0.0687380085614519));
#77403=CARTESIAN_POINT('',(0.00646381897802044,-0.0340203938281605,0.0686433996763379));
#77404=CARTESIAN_POINT('Origin',(0.0105574639983245,-0.0345589643244318,
0.0848069393239999));
#77405=CARTESIAN_POINT('',(0.00646421107987864,-0.034193496108874,0.0686447003968781));
#77406=CARTESIAN_POINT('Origin',(0.00328376725328437,-0.0341934220717591,
0.0580942029998901));
#77407=CARTESIAN_POINT('',(0.00640437086681123,-0.0341934961088841,0.0686627392133364));
#77408=CARTESIAN_POINT('Ctrl Pts',(0.00661855933023323,-0.0340223579322397,
0.0683418760229223));
#77409=CARTESIAN_POINT('Ctrl Pts',(0.00653845015236607,-0.0339125849573575,
0.0683626369719874));
#77410=CARTESIAN_POINT('Ctrl Pts',(0.00645882696969454,-0.0338030433565231,
0.0683850414064078));
#77411=CARTESIAN_POINT('Ctrl Pts',(0.00637978906701337,-0.0336938721132327,
0.0684090516483634));
#77412=CARTESIAN_POINT('Ctrl Pts',(0.00656712532055574,-0.0340223579322397,
0.0684428498931996));
#77413=CARTESIAN_POINT('Ctrl Pts',(0.00648840883571061,-0.0339125849573575,
0.0684643202514037));
#77414=CARTESIAN_POINT('Ctrl Pts',(0.0064101920505526,-0.0338030433565231,
0.0684874047709601));
#77415=CARTESIAN_POINT('Ctrl Pts',(0.00633257237423454,-0.0336938721132327,
0.0685120650637679));
#77416=CARTESIAN_POINT('Ctrl Pts',(0.00651569131087825,-0.0340223579322397,
0.0685438237634769));
#77417=CARTESIAN_POINT('Ctrl Pts',(0.00643836751905516,-0.0339125849573575,
0.06856600353082));
#77418=CARTESIAN_POINT('Ctrl Pts',(0.00636155713141065,-0.0338030433565231,
0.0685897681355124));
#77419=CARTESIAN_POINT('Ctrl Pts',(0.00628535568145572,-0.0336938721132327,
0.0686150784791725));
#77420=CARTESIAN_POINT('Ctrl Pts',(0.00646425730120076,-0.0340223579322397,
0.0686447976337542));
#77421=CARTESIAN_POINT('Ctrl Pts',(0.0063883262023997,-0.0339125849573575,
0.0686676868102363));
#77422=CARTESIAN_POINT('Ctrl Pts',(0.00631292221226871,-0.0338030433565231,
0.0686921315000647));
#77423=CARTESIAN_POINT('Ctrl Pts',(0.00623813898867689,-0.0336938721132327,
0.068718091894577));
#77424=CARTESIAN_POINT('',(0.00630938662001274,-0.0336938721132427,0.0685626497953968));
#77425=CARTESIAN_POINT('Ctrl Pts',(0.00639205581550063,-0.03371081206627,
0.068405339549261));
#77426=CARTESIAN_POINT('Ctrl Pts',(0.00640446630652668,-0.0337611408994182,
0.0684465089036657));
#77427=CARTESIAN_POINT('Ctrl Pts',(0.00641665033362538,-0.0338121088781064,
0.0684869270086906));
#77428=CARTESIAN_POINT('Ctrl Pts',(0.00644057655943417,-0.0339153382773244,
0.068566297540269));
#77429=CARTESIAN_POINT('Ctrl Pts',(0.00645231039752609,-0.0339675637691194,
0.068605222232122));
#77430=CARTESIAN_POINT('Ctrl Pts',(0.00646382071677454,-0.0340204018098272,
0.0686434054443299));
#77431=CARTESIAN_POINT('Ctrl Pts',(0.00634631765569402,-0.0341934961088741,
0.0686817371991245));
#77432=CARTESIAN_POINT('Ctrl Pts',(0.00623326563024816,-0.0340287516182428,
0.0687184848781279));
#77433=CARTESIAN_POINT('Ctrl Pts',(0.00612182901504797,-0.0338644633275951,
0.0687598736829219));
#77434=CARTESIAN_POINT('Ctrl Pts',(0.00634453065372386,-0.0341934961088741,
0.0686807780297745));
#77435=CARTESIAN_POINT('Ctrl Pts',(0.00623145879820733,-0.0340287516182428,
0.0687175626536358));
#77436=CARTESIAN_POINT('Ctrl Pts',(0.0061200038968399,-0.0338644633275951,
0.0687589891913109));
#77437=CARTESIAN_POINT('Ctrl Pts',(0.00604678175384191,-0.0341934961088741,
0.0685209619671487));
#77438=CARTESIAN_POINT('Ctrl Pts',(0.00593040582713559,-0.0340287516182428,
0.068563902314945));
#77439=CARTESIAN_POINT('Ctrl Pts',(0.00581590409858431,-0.0338644633275951,
0.0686116158763756));
#77440=CARTESIAN_POINT('',(0.00603476276706981,-0.0341764758832379,0.0685254113192004));
#77441=CARTESIAN_POINT('',(0.00604678175384194,-0.034193496108874,0.0685209619671487));
#77442=CARTESIAN_POINT('Origin',(0.0113196153181899,-0.0345621026496214,
0.0842254642322378));
#77443=CARTESIAN_POINT('Ctrl Pts',(0.00603476276886755,-0.0341764758837464,
0.0685254113194495));
#77444=CARTESIAN_POINT('Ctrl Pts',(0.00604970775821637,-0.0341260050040501,
0.0685656499761387));
#77445=CARTESIAN_POINT('Ctrl Pts',(0.00606439300421029,-0.034074926914832,
0.0686051891767446));
#77446=CARTESIAN_POINT('Ctrl Pts',(0.00609325521875247,-0.0339715436306764,
0.0686828993729217));
#77447=CARTESIAN_POINT('Ctrl Pts',(0.00610742123204215,-0.0339192778236902,
0.068721040889147));
#77448=CARTESIAN_POINT('Ctrl Pts',(0.0061213322405873,-0.0338664212854632,
0.0687584956454671));
#77449=CARTESIAN_POINT('',(0.00619565620379288,-0.0341934961088841,0.0686008699984716));
#77450=CARTESIAN_POINT('Origin',(0.00812378219310841,-0.0315241814719618,
0.07415));
#77451=CARTESIAN_POINT('',(0.00603476276653722,-0.0342105180190382,0.0685254113201839));
#77452=CARTESIAN_POINT('',(0.00602275330947995,-0.0341934961088739,0.0685298863329841));
#77453=CARTESIAN_POINT('Origin',(0.0113636440338325,-0.0345621709122607,
0.0842146942021983));
#77454=CARTESIAN_POINT('Origin',(0.012279732518218,-0.0345621036048912,
0.0838688707717797));
#77455=CARTESIAN_POINT('Origin',(0.0122393463298125,-0.0345621718614647,
0.0838894481597944));
#77456=CARTESIAN_POINT('Ctrl Pts',(0.00624039032944951,-0.0346945769586966,
0.0687157256841039));
#77457=CARTESIAN_POINT('Ctrl Pts',(0.00612656727813833,-0.0345275153362944,
0.0687551740807572));
#77458=CARTESIAN_POINT('Ctrl Pts',(0.00601395540212098,-0.0343603235965185,
0.0687982123109832));
#77459=CARTESIAN_POINT('Ctrl Pts',(0.00590288586550722,-0.0341934961088739,
0.0688447081367231));
#77460=CARTESIAN_POINT('Ctrl Pts',(0.00616180232339275,-0.0346945769586966,
0.0687449139289149));
#77461=CARTESIAN_POINT('Ctrl Pts',(0.00604859063155547,-0.0345275153362944,
0.06878600838282));
#77462=CARTESIAN_POINT('Ctrl Pts',(0.00593664204012637,-0.0343603235965185,
0.0688306738693598));
#77463=CARTESIAN_POINT('Ctrl Pts',(0.00582628567998455,-0.0341934961088739,
0.0688787733669295));
#77464=CARTESIAN_POINT('Ctrl Pts',(0.00608321431733598,-0.0346945769586966,
0.0687741021737259));
#77465=CARTESIAN_POINT('Ctrl Pts',(0.0059706139849726,-0.0345275153362944,
0.0688168426848828));
#77466=CARTESIAN_POINT('Ctrl Pts',(0.00585932867813176,-0.0343603235965185,
0.0688631354277364));
#77467=CARTESIAN_POINT('Ctrl Pts',(0.00574968549446188,-0.0341934961088739,
0.068912838597136));
#77468=CARTESIAN_POINT('Ctrl Pts',(0.00600462631127922,-0.0346945769586966,
0.068803290418537));
#77469=CARTESIAN_POINT('Ctrl Pts',(0.00589263733838974,-0.0345275153362944,
0.0688476769869456));
#77470=CARTESIAN_POINT('Ctrl Pts',(0.00578201531613716,-0.0343603235965185,
0.068895596986113));
#77471=CARTESIAN_POINT('Ctrl Pts',(0.00567308530893922,-0.0341934961088739,
0.0689469038273425));
#77472=CARTESIAN_POINT('',(0.00600462631126852,-0.0346945769586966,0.0688032904185411));
#77473=CARTESIAN_POINT('',(0.0057867482589667,-0.0343667727832908,0.0688948694220707));
#77474=CARTESIAN_POINT('Origin',(0.0123695229635273,-0.0345626461566603,
0.084365595431727));
#77475=CARTESIAN_POINT('Origin',(0.00129574829283271,-0.0341934771027846,
0.0587962767159609));
#77476=CARTESIAN_POINT('',(0.00590151527665439,-0.0341934961088739,0.0688453176577636));
#77477=CARTESIAN_POINT('',(0.00584440778473561,-0.034193496108884,0.0688707142001683));
#77478=CARTESIAN_POINT('',(0.00612133224108813,-0.0345211942962717,0.0687584956469073));
#77479=CARTESIAN_POINT('Origin',(0.011917638240633,-0.0345625596118878,
0.0845298829433527));
#77480=CARTESIAN_POINT('',(0.00612180524213312,-0.0346945769586885,0.0687597691804744));
#77481=CARTESIAN_POINT('Origin',(0.00226980493413639,-0.0346945685853964,
0.0583884332561724));
#77482=CARTESIAN_POINT('',(0.00606321577671083,-0.0346945769587026,0.0687815297995178));
#77483=CARTESIAN_POINT('Ctrl Pts',(0.00625683350729417,-0.0345231616327842,
0.0684478510538082));
#77484=CARTESIAN_POINT('Ctrl Pts',(0.00617823741205449,-0.0344132092796988,
0.0684735843129886));
#77485=CARTESIAN_POINT('Ctrl Pts',(0.00610017764418005,-0.0343032738558979,
0.0685009419426854));
#77486=CARTESIAN_POINT('Ctrl Pts',(0.00602275330947989,-0.0341934961088739,
0.0685298863329841));
#77487=CARTESIAN_POINT('Ctrl Pts',(0.00621184128588049,-0.0345231616327842,
0.0685518550736859));
#77488=CARTESIAN_POINT('Ctrl Pts',(0.00613467873962887,-0.0344132092796988,
0.0685782084872945));
#77489=CARTESIAN_POINT('Ctrl Pts',(0.00605806527418315,-0.0343032738558979,
0.0686061565875924));
#77490=CARTESIAN_POINT('Ctrl Pts',(0.00598209812309473,-0.0341934961088739,
0.068635661055666));
#77491=CARTESIAN_POINT('Ctrl Pts',(0.00616684906446681,-0.0345231616327842,
0.0686558590935636));
#77492=CARTESIAN_POINT('Ctrl Pts',(0.00609112006720326,-0.0344132092796988,
0.0686828326616004));
#77493=CARTESIAN_POINT('Ctrl Pts',(0.00601595290418624,-0.0343032738558979,
0.0687113712324993));
#77494=CARTESIAN_POINT('Ctrl Pts',(0.00594144293670958,-0.0341934961088739,
0.068741435778348));
#77495=CARTESIAN_POINT('Ctrl Pts',(0.00612185684305314,-0.0345231616327842,
0.0687598631134413));
#77496=CARTESIAN_POINT('Ctrl Pts',(0.00604756139477765,-0.0344132092796988,
0.0687874568359063));
#77497=CARTESIAN_POINT('Ctrl Pts',(0.00597384053418934,-0.0343032738558979,
0.0688165858774063));
#77498=CARTESIAN_POINT('Ctrl Pts',(0.00590078775032442,-0.0341934961088739,
0.0688472105010299));
#77499=CARTESIAN_POINT('',(0.00596213429307717,-0.0341934961088839,0.0686876019953838));
#77500=CARTESIAN_POINT('Ctrl Pts',(0.0060347627677351,-0.0342105180195403,
0.0685254113234173));
#77501=CARTESIAN_POINT('Ctrl Pts',(0.00604972454526662,-0.0342610556241142,
0.0685656952209547));
#77502=CARTESIAN_POINT('Ctrl Pts',(0.00606441784143634,-0.0343122189869805,
0.0686052562447796));
#77503=CARTESIAN_POINT('Ctrl Pts',(0.00609328035092692,-0.0344158119695204,
0.0686829672234745));
#77504=CARTESIAN_POINT('Ctrl Pts',(0.00610743775925481,-0.0344681990450104,
0.0687210853939441));
#77505=CARTESIAN_POINT('Ctrl Pts',(0.00612133224109043,-0.0345211942962538,
0.0687584956469318));
#77506=CARTESIAN_POINT('Ctrl Pts',(0.00600646956223161,-0.0346945769586932,
0.0688041352814491));
#77507=CARTESIAN_POINT('Ctrl Pts',(0.0059328008443355,-0.0345846629175836,
0.0688333129197011));
#77508=CARTESIAN_POINT('Ctrl Pts',(0.00585972292521789,-0.0344746925049831,
0.0688640189803979));
#77509=CARTESIAN_POINT('Ctrl Pts',(0.00578732927824432,-0.0343648066252516,
0.0688962137326933));
#77510=CARTESIAN_POINT('Ctrl Pts',(0.00590345638056552,-0.0346945769586932,
0.0687569186958054));
#77511=CARTESIAN_POINT('Ctrl Pts',(0.00582913699425355,-0.0345846629175836,
0.0687875159077689));
#77512=CARTESIAN_POINT('Ctrl Pts',(0.0057554376517857,-0.0344746925049831,
0.0688196552401995));
#77513=CARTESIAN_POINT('Ctrl Pts',(0.00568245261518233,-0.0343648066252516,
0.0688532951224898));
#77514=CARTESIAN_POINT('Ctrl Pts',(0.00580044319889943,-0.0346945769586932,
0.0687097021101616));
#77515=CARTESIAN_POINT('Ctrl Pts',(0.00572547314417161,-0.0345846629175836,
0.0687417188958366));
#77516=CARTESIAN_POINT('Ctrl Pts',(0.0056511523783535,-0.0344746925049831,
0.068775291500001));
#77517=CARTESIAN_POINT('Ctrl Pts',(0.00557757595212033,-0.0343648066252516,
0.0688103765122862));
#77518=CARTESIAN_POINT('Ctrl Pts',(0.00569743001723334,-0.0346945769586932,
0.0686624855245178));
#77519=CARTESIAN_POINT('Ctrl Pts',(0.00562180929408966,-0.0345846629175836,
0.0686959218839044));
#77520=CARTESIAN_POINT('Ctrl Pts',(0.00554686710492131,-0.0344746925049831,
0.0687309277598026));
#77521=CARTESIAN_POINT('Ctrl Pts',(0.00547269928905834,-0.0343648066252516,
0.0687674579020826));
#77522=CARTESIAN_POINT('',(0.00568571412388135,-0.0346775396663606,0.0686676807763232));
#77523=CARTESIAN_POINT('',(0.00569743001723021,-0.0346945769586886,0.0686624855245192));
#77524=CARTESIAN_POINT('Origin',(0.0125709383820059,-0.0345626618064187,
0.0837741889178235));
#77525=CARTESIAN_POINT('Ctrl Pts',(0.00568571412524865,-0.0346775396659408,
0.0686676807794041));
#77526=CARTESIAN_POINT('Ctrl Pts',(0.00570317000872294,-0.0346269748528332,
0.0687069326472027));
#77527=CARTESIAN_POINT('Ctrl Pts',(0.00572031551976361,-0.0345757904815517,
0.068745486601444));
#77528=CARTESIAN_POINT('Ctrl Pts',(0.00575400050052634,-0.0344721679344607,
0.0688212317456897));
#77529=CARTESIAN_POINT('Ctrl Pts',(0.00577052639654102,-0.0344197716860284,
0.068858392413414));
#77530=CARTESIAN_POINT('Ctrl Pts',(0.00578674825918659,-0.034366772783177,
0.0688948694218075));
#77531=CARTESIAN_POINT('',(0.00585102816425936,-0.0346945769587026,0.0687328879715402));
#77532=CARTESIAN_POINT('Origin',(0.00812378219310841,-0.0315241814719618,
0.07415));
#77533=CARTESIAN_POINT('',(0.00568571412392511,-0.0347116136489625,0.0686676807764219));
#77534=CARTESIAN_POINT('',(0.0056740093530817,-0.0346945769586885,0.0686729010386621));
#77535=CARTESIAN_POINT('Origin',(0.0126115469653707,-0.034562668844092,
0.0837540846355363));
#77536=CARTESIAN_POINT('Origin',(0.0122918590496367,-0.0345626626357112,
0.0838983018354193));
#77537=CARTESIAN_POINT('Origin',(0.0122497303169883,-0.0345626697496677,
0.0839149876111518));
#77538=CARTESIAN_POINT('Ctrl Pts',(0.00593716783041815,-0.0352450361874068,
0.0688304624021912));
#77539=CARTESIAN_POINT('Ctrl Pts',(0.00573653817773724,-0.0349452760959493,
0.0689129319161419));
#77540=CARTESIAN_POINT('Ctrl Pts',(0.00554269043400859,-0.034644428984174,
0.0690102793892341));
#77541=CARTESIAN_POINT('Ctrl Pts',(0.00593485429329546,-0.0352450361874068,
0.0688314739213368));
#77542=CARTESIAN_POINT('Ctrl Pts',(0.00573426279068515,-0.0349452760959493,
0.0689140306917719));
#77543=CARTESIAN_POINT('Ctrl Pts',(0.00554045966116219,-0.034644428984174,
0.0690114622998426));
#77544=CARTESIAN_POINT('Ctrl Pts',(0.00570579121184181,-0.0352450361874068,
0.0689316243317951));
#77545=CARTESIAN_POINT('Ctrl Pts',(0.00550897694394346,-0.0349452760959493,
0.0690228203581108));
#77546=CARTESIAN_POINT('Ctrl Pts',(0.00531959106250815,-0.034644428984174,
0.0691285821620719));
#77547=CARTESIAN_POINT('Ctrl Pts',(0.00570350058102728,-0.0352450361874068,
0.0689326258358997));
#77548=CARTESIAN_POINT('Ctrl Pts',(0.00550672408547605,-0.0349452760959493,
0.0690239082547742));
#77549=CARTESIAN_POINT('Ctrl Pts',(0.00531738237652162,-0.034644428984174,
0.0691297533606941));
#77550=CARTESIAN_POINT('',(0.00567311357158921,-0.035195163405329,0.0689468878918456));
#77551=CARTESIAN_POINT('',(0.00546138748269816,-0.0348678972925388,0.0690519827966178));
#77552=CARTESIAN_POINT('Origin',(0.0135887839607815,-0.0345636767887483,
0.0837031292376524));
#77553=CARTESIAN_POINT('Origin',(0.000346240795818812,-0.0346946199341177,
0.0592573789986556));
#77554=CARTESIAN_POINT('',(0.00557281666879287,-0.0346945769330288,0.0689953225230199));
#77555=CARTESIAN_POINT('',(0.00551741651966883,-0.0346945769458128,0.0690242547639391));
#77556=CARTESIAN_POINT('',(0.00578674825928095,-0.0350221583435276,0.0688948694219706));
#77557=CARTESIAN_POINT('Origin',(0.01318341802763,-0.0345628458718028,0.0839616284697936));
#77558=CARTESIAN_POINT('',(0.00578725362435978,-0.035195136029876,0.0688959983590295));
#77559=CARTESIAN_POINT('Origin',(0.00130974932011656,-0.0351951838366708,
0.0588277413573055));
#77560=CARTESIAN_POINT('',(0.00567308530889138,-0.035195137132875,0.0689469038272366));
#77561=CARTESIAN_POINT('Ctrl Pts',(0.00590247571684632,-0.0350241211494343,
0.0685763299758115));
#77562=CARTESIAN_POINT('Ctrl Pts',(0.0058257006975568,-0.0349144232818962,
0.0686069275617508));
#77563=CARTESIAN_POINT('Ctrl Pts',(0.00574951219868282,-0.0348045283579412,
0.0686391304563295));
#77564=CARTESIAN_POINT('Ctrl Pts',(0.00567400934293733,-0.0346945769439158,
0.0686729010431994));
#77565=CARTESIAN_POINT('Ctrl Pts',(0.00586410275235436,-0.0350241211494343,
0.0686829538821318));
#77566=CARTESIAN_POINT('Ctrl Pts',(0.0057887964336569,-0.0349144232818962,
0.0687140800399236));
#77567=CARTESIAN_POINT('Ctrl Pts',(0.00571408844042096,-0.0348045283579412,
0.0687467814636396));
#77568=CARTESIAN_POINT('Ctrl Pts',(0.00564007602278193,-0.0346945769439158,
0.0687810198278122));
#77569=CARTESIAN_POINT('Ctrl Pts',(0.0058257297878624,-0.0350241211494343,
0.0687895777884522));
#77570=CARTESIAN_POINT('Ctrl Pts',(0.005751892169757,-0.0349144232818962,
0.0688212325180963));
#77571=CARTESIAN_POINT('Ctrl Pts',(0.00567866468215911,-0.0348045283579412,
0.0688544324709497));
#77572=CARTESIAN_POINT('Ctrl Pts',(0.00560614270262652,-0.0346945769439158,
0.068889138612425));
#77573=CARTESIAN_POINT('Ctrl Pts',(0.00578735682337044,-0.0350241211494343,
0.0688962016947726));
#77574=CARTESIAN_POINT('Ctrl Pts',(0.0057149879058571,-0.0349144232818962,
0.068928384996269));
#77575=CARTESIAN_POINT('Ctrl Pts',(0.00564324092389725,-0.0348045283579412,
0.0689620834782598));
#77576=CARTESIAN_POINT('Ctrl Pts',(0.00557220938247111,-0.0346945769439158,
0.0689972573970378));
#77577=CARTESIAN_POINT('',(0.00562341301116769,-0.0346945769458128,0.0688341117806416));
#77578=CARTESIAN_POINT('Ctrl Pts',(0.00568571412525632,-0.0347116136492807,
0.0686676807794213));
#77579=CARTESIAN_POINT('Ctrl Pts',(0.00570316302278226,-0.034762154653213,
0.0687069169383889));
#77580=CARTESIAN_POINT('Ctrl Pts',(0.00572030512153781,-0.0348133084096664,
0.0687454632196547));
#77581=CARTESIAN_POINT('Ctrl Pts',(0.00575399002778241,-0.0349168561544574,
0.0688212081963366));
#77582=CARTESIAN_POINT('Ctrl Pts',(0.00577051947416102,-0.0349692089015921,
0.0688583768475247));
#77583=CARTESIAN_POINT('Ctrl Pts',(0.00578674825927763,-0.0350221583435,
0.0688948694220121));
#77584=CARTESIAN_POINT('Ctrl Pts',(0.00567445092821152,-0.0351951371254906,
0.0689474287117786));
#77585=CARTESIAN_POINT('Ctrl Pts',(0.00556689103103042,-0.0350307338980921,
0.0689980670989182));
#77586=CARTESIAN_POINT('Ctrl Pts',(0.00546151598233047,-0.0348659306897792,
0.0690531077824641));
#77587=CARTESIAN_POINT('Ctrl Pts',(0.00567308530894344,-0.0351951371254906,
0.0689469038273406));
#77588=CARTESIAN_POINT('Ctrl Pts',(0.00556551456010591,-0.0350307338980921,
0.0689975704478017));
#77589=CARTESIAN_POINT('Ctrl Pts',(0.00546012983593585,-0.0348659306897792,
0.0690526397890546));
#77590=CARTESIAN_POINT('Ctrl Pts',(0.00544420609628805,-0.0351951371254906,
0.0688589326484588));
#77591=CARTESIAN_POINT('Ctrl Pts',(0.00533481659852212,-0.0350307338980921,
0.068914331203038));
#77592=CARTESIAN_POINT('Ctrl Pts',(0.00522781025547691,-0.0348659306897792,
0.0689742036058547));
#77593=CARTESIAN_POINT('Origin',(0.00299951715930774,-0.0308609197411333,
0.0643379344954456));
#77594=CARTESIAN_POINT('',(0.00557329913276375,-0.0351951371254906,0.0689085503768337));
#77595=CARTESIAN_POINT('Origin',(0.00869681970877851,-0.0351840467441122,
0.0749414377145248));
#77596=CARTESIAN_POINT('Origin',(0.00189259307280093,-0.0352322614929444,
0.0639351132346021));
#77597=CARTESIAN_POINT('',(0.00525392634011456,-0.0351951142564654,0.0691658509285475));
#77598=CARTESIAN_POINT('',(0.00514723717408231,-0.0351951372916787,0.0692303780887438));
#77599=CARTESIAN_POINT('Origin',(0.00796802316457458,-0.0352875118755706,
0.0744528703542965));
#77600=CARTESIAN_POINT('Origin',(0.0151681473551898,-0.0298325076521879,
0.0715669572699247));
#77601=CARTESIAN_POINT('Origin',(0.00680340913363432,-0.0338732635903356,
0.0658731868073005));
#77602=CARTESIAN_POINT('Ctrl Pts',(0.00873198787934537,-0.0321934096636942,
0.0684308897904884));
#77603=CARTESIAN_POINT('Ctrl Pts',(0.00862961853006105,-0.0320508460844117,
0.068420003198335));
#77604=CARTESIAN_POINT('Ctrl Pts',(0.00852703386635374,-0.0319086045662657,
0.0684118752771323));
#77605=CARTESIAN_POINT('Ctrl Pts',(0.0084244562118284,-0.031766989286728,
0.0684065053432813));
#77606=CARTESIAN_POINT('Ctrl Pts',(0.00864843728755645,-0.0321934096636942,
0.0684238377525166));
#77607=CARTESIAN_POINT('Ctrl Pts',(0.00854594171015065,-0.0320508460844117,
0.068414446676169));
#77608=CARTESIAN_POINT('Ctrl Pts',(0.00844327109505708,-0.0319086045662657,
0.0684078165346489));
#77609=CARTESIAN_POINT('Ctrl Pts',(0.00834064768544859,-0.031766989286728,
0.068403943404138));
#77610=CARTESIAN_POINT('Ctrl Pts',(0.00856488669576753,-0.0321934096636942,
0.0684167857145446));
#77611=CARTESIAN_POINT('Ctrl Pts',(0.00846226489024025,-0.0320508460844117,
0.068408890154003));
#77612=CARTESIAN_POINT('Ctrl Pts',(0.00835950832376042,-0.0319086045662657,
0.0684037577921656));
#77613=CARTESIAN_POINT('Ctrl Pts',(0.00825683915906878,-0.031766989286728,
0.0684013814649947));
#77614=CARTESIAN_POINT('Ctrl Pts',(0.00848133610397861,-0.0321934096636942,
0.0684097336765728));
#77615=CARTESIAN_POINT('Ctrl Pts',(0.00837858807032984,-0.0320508460844117,
0.068403333631837));
#77616=CARTESIAN_POINT('Ctrl Pts',(0.00827574555246378,-0.0319086045662657,
0.0683996990496821));
#77617=CARTESIAN_POINT('Ctrl Pts',(0.00817303063268897,-0.031766989286728,
0.0683988195258514));
#77618=CARTESIAN_POINT('',(0.00848283084057609,-0.0321934096636942,0.0684098598389279));
#77619=CARTESIAN_POINT('',(0.00824669644181227,-0.0318665617511272,0.0683999550370014));
#77620=CARTESIAN_POINT('Origin',(0.00682662938771915,-0.0326371944421028,
0.0850373942807947));
#77621=CARTESIAN_POINT('Origin',(0.00848095171668544,-0.0316939261509279,
0.0574412728810131));
#77622=CARTESIAN_POINT('',(0.00860723504865228,-0.032019722162187,0.0684190434914406));
#77623=CARTESIAN_POINT('Ctrl Pts',(0.00860706079400472,-0.0320197392094779,
0.0684189814414899));
#77624=CARTESIAN_POINT('Ctrl Pts',(0.00857789952515948,-0.0319792716576076,
0.0684165224113723));
#77625=CARTESIAN_POINT('Ctrl Pts',(0.00854858675646262,-0.0319386439829738,
0.0684142745005901));
#77626=CARTESIAN_POINT('Ctrl Pts',(0.00851909106836822,-0.031897909938167,
0.0684122437820222));
#77627=CARTESIAN_POINT('Ctrl Pts',(0.00848959596327579,-0.0318571766984958,
0.0684102131035927));
#77628=CARTESIAN_POINT('Ctrl Pts',(0.0084600679817806,-0.0318163871833592,
0.0684084081525476));
#77629=CARTESIAN_POINT('Ctrl Pts',(0.00843060890280958,-0.0317755399638303,
0.0684068316225805));
#77630=CARTESIAN_POINT('',(0.0086073879491624,-0.0321934096636184,0.0684203730075413));
#77631=CARTESIAN_POINT('Origin',(0.00878062777302303,-0.0324113749715919,
0.0661177156651816));
#77632=CARTESIAN_POINT('',(0.00854510939487925,-0.0321934096636663,0.0684151164232446));
#77633=CARTESIAN_POINT('Ctrl Pts',(0.00848413930783408,-0.0321934096636618,
0.0684114095488407));
#77634=CARTESIAN_POINT('Ctrl Pts',(0.00840499967311677,-0.0320835708272592,
0.0684064399433827));
#77635=CARTESIAN_POINT('Ctrl Pts',(0.00832580309687715,-0.0319739230346488,
0.0684031110111253));
#77636=CARTESIAN_POINT('Ctrl Pts',(0.00824665123251692,-0.0318646057455573,
0.0684014192346785));
#77637=CARTESIAN_POINT('Ctrl Pts',(0.00841103391569604,-0.0321934096636618,
0.0683248256796451));
#77638=CARTESIAN_POINT('Ctrl Pts',(0.008330700221943,-0.0320835708272592,
0.0683208642545198));
#77639=CARTESIAN_POINT('Ctrl Pts',(0.00825033114351001,-0.0319739230346488,
0.068318567628799));
#77640=CARTESIAN_POINT('Ctrl Pts',(0.00817002973256898,-0.0318646057455573,
0.0683179308491973));
#77641=CARTESIAN_POINT('Ctrl Pts',(0.00833792852355801,-0.0321934096636618,
0.0682382418104496));
#77642=CARTESIAN_POINT('Ctrl Pts',(0.00825640077076924,-0.0320835708272592,
0.0682352885656568));
#77643=CARTESIAN_POINT('Ctrl Pts',(0.00817485919014287,-0.0319739230346488,
0.0682340242464728));
#77644=CARTESIAN_POINT('Ctrl Pts',(0.00809340823262104,-0.0318646057455573,
0.0682344424637161));
#77645=CARTESIAN_POINT('Ctrl Pts',(0.00826482313141997,-0.0321934096636618,
0.0681516579412541));
#77646=CARTESIAN_POINT('Ctrl Pts',(0.00818210131959548,-0.0320835708272592,
0.0681497128767939));
#77647=CARTESIAN_POINT('Ctrl Pts',(0.00809938723677573,-0.0319739230346488,
0.0681494808641465));
#77648=CARTESIAN_POINT('Ctrl Pts',(0.00801678673267309,-0.0318646057455573,
0.0681509540782349));
#77649=CARTESIAN_POINT('',(0.00825201024350632,-0.0321763980308456,0.0681513703610936));
#77650=CARTESIAN_POINT('',(0.00826482313138734,-0.0321934096636185,0.0681516579412533));
#77651=CARTESIAN_POINT('Origin',(0.00728524449179297,-0.0326386231366924,
0.0846707968808568));
#77652=CARTESIAN_POINT('Ctrl Pts',(0.00825201024343353,-0.0321763980306277,
0.0681513703642613));
#77653=CARTESIAN_POINT('Ctrl Pts',(0.00825109300909574,-0.0321259596174814,
0.0681942794552726));
#77654=CARTESIAN_POINT('Ctrl Pts',(0.00825019166703981,-0.0320749164631369,
0.068236445090604));
#77655=CARTESIAN_POINT('Ctrl Pts',(0.00824842004209381,-0.031971605779391,
0.0683193233834387));
#77656=CARTESIAN_POINT('Ctrl Pts',(0.00824755044948827,-0.0319193786690104,
0.0683600037487772));
#77657=CARTESIAN_POINT('Ctrl Pts',(0.00824669644176559,-0.0318665617525284,
0.0683999550388528));
#77658=CARTESIAN_POINT('',(0.00837382698599171,-0.0321934096636664,0.0682807588901006));
#77659=CARTESIAN_POINT('Origin',(0.00812378219310841,-0.0315241814719618,
0.07415));
#77660=CARTESIAN_POINT('',(0.00825201024351424,-0.0322104233323795,0.0681513703607228));
#77661=CARTESIAN_POINT('',(0.00823919677064607,-0.0321934096636183,0.0681511101464259));
#77662=CARTESIAN_POINT('Origin',(0.00732999092986969,-0.0326387236409409,
0.084678071674358));
#77663=CARTESIAN_POINT('Origin',(0.00851197086234812,-0.0326386241790837,
0.0846970221127516));
#77664=CARTESIAN_POINT('Origin',(0.00846695424061251,-0.0326387244629747,
0.0847023730764388));
#77665=CARTESIAN_POINT('Ctrl Pts',(0.00840774447948624,-0.0327445246967098,
0.0684056557885242));
#77666=CARTESIAN_POINT('Ctrl Pts',(0.00819109299577849,-0.032443687833936,
0.0683949459758117));
#77667=CARTESIAN_POINT('Ctrl Pts',(0.00797425028918936,-0.0321434074405927,
0.0684005856637645));
#77668=CARTESIAN_POINT('Ctrl Pts',(0.0081578400902427,-0.0327445246967098,
0.068398742306274));
#77669=CARTESIAN_POINT('Ctrl Pts',(0.00794092786028926,-0.032443687833936,
0.0683974577916846));
#77670=CARTESIAN_POINT('Ctrl Pts',(0.00772453510018328,-0.0321434074405927,
0.0684125156419567));
#77671=CARTESIAN_POINT('',(0.00812169595725582,-0.0326943950436612,0.0683986418432147));
#77672=CARTESIAN_POINT('',(0.0078854055880294,-0.0323666188837389,0.0684035835867776));
#77673=CARTESIAN_POINT('Origin',(0.00820380398097328,-0.0326395579111606,
0.0852093918711237));
#77674=CARTESIAN_POINT('Origin',(0.0074276388939793,-0.0321933825602993,
0.0573684659390598));
#77675=CARTESIAN_POINT('',(0.00801035448973432,-0.0321934096532689,0.0683997600786812));
#77676=CARTESIAN_POINT('',(0.00794790819298478,-0.0321934096584275,0.0684023505164726));
#77677=CARTESIAN_POINT('',(0.00824669644183017,-0.0325210109756238,0.0683999550360487));
#77678=CARTESIAN_POINT('Origin',(0.00772364846753187,-0.0326393129157461,
0.0851841904293704));
#77679=CARTESIAN_POINT('',(0.00824666740810641,-0.0326943950436594,0.0684013132609321));
#77680=CARTESIAN_POINT('Origin',(0.00848308765021364,-0.032694376553819,
0.0573413845913037));
#77681=CARTESIAN_POINT('',(0.00818418168269111,-0.0326943950436703,0.0683999775520834));
#77682=CARTESIAN_POINT('Ctrl Pts',(0.00848703838247985,-0.0325229783203769,
0.0681610063499027));
#77683=CARTESIAN_POINT('Ctrl Pts',(0.0084044802359839,-0.032413025309245,
0.0681559988712761));
#77684=CARTESIAN_POINT('Ctrl Pts',(0.00832183102492051,-0.0323031222208069,
0.0681526999734455));
#77685=CARTESIAN_POINT('Ctrl Pts',(0.00823919676616269,-0.0321934096576658,
0.0681511101463396));
#77686=CARTESIAN_POINT('Ctrl Pts',(0.00840691921866812,-0.0325229783203769,
0.0682411441176928));
#77687=CARTESIAN_POINT('Ctrl Pts',(0.00832546576954866,-0.032413025309245,
0.0682372410799873));
#77688=CARTESIAN_POINT('Ctrl Pts',(0.00824394393509196,-0.0323031222208069,
0.0682350236034833));
#77689=CARTESIAN_POINT('Ctrl Pts',(0.00816245823920177,-0.0321934096576658,
0.068234490843843));
#77690=CARTESIAN_POINT('Ctrl Pts',(0.00832680005485639,-0.0325229783203769,
0.068321281885483));
#77691=CARTESIAN_POINT('Ctrl Pts',(0.00824645130311342,-0.032413025309245,
0.0683184832886985));
#77692=CARTESIAN_POINT('Ctrl Pts',(0.00816605684526341,-0.0323031222208069,
0.0683173472335212));
#77693=CARTESIAN_POINT('Ctrl Pts',(0.00808571971224084,-0.0321934096576658,
0.0683178715413464));
#77694=CARTESIAN_POINT('Ctrl Pts',(0.00824668089104465,-0.0325229783203769,
0.0684014196532732));
#77695=CARTESIAN_POINT('Ctrl Pts',(0.00816743683667817,-0.032413025309245,
0.0683997254974097));
#77696=CARTESIAN_POINT('Ctrl Pts',(0.00808816975543486,-0.0323031222208069,
0.068399670863559));
#77697=CARTESIAN_POINT('Ctrl Pts',(0.00800898118527992,-0.0321934096576658,
0.0684012522388497));
#77698=CARTESIAN_POINT('',(0.00812477563068398,-0.0321934096584275,0.0682754351124071));
#77699=CARTESIAN_POINT('Ctrl Pts',(0.00825201024343501,-0.0322104233328944,
0.068151370364196));
#77700=CARTESIAN_POINT('Ctrl Pts',(0.00825109176623048,-0.0322609421831085,
0.0681943375976923));
#77701=CARTESIAN_POINT('Ctrl Pts',(0.008250189817007,-0.0323120888240131,
0.06823653163658));
#77702=CARTESIAN_POINT('Ctrl Pts',(0.00824841817864644,-0.032415652463182,
0.0683194105569602));
#77703=CARTESIAN_POINT('Ctrl Pts',(0.00824754921774712,-0.0324680267167319,
0.0683600613707999));
#77704=CARTESIAN_POINT('Ctrl Pts',(0.00824669644182473,-0.0325210109755912,
0.0683999550360919));
#77705=CARTESIAN_POINT('Origin',(0.0159123493438964,-0.0262834582512498,
0.0752642744613413));
#77706=CARTESIAN_POINT('Origin',(0.0137941110260438,-0.0342770758373598,
0.0633949811933364));
#77707=CARTESIAN_POINT('Ctrl Pts',(0.00812309880904369,-0.0326943950436605,
0.0684001059803989));
#77708=CARTESIAN_POINT('Ctrl Pts',(0.00804385449300363,-0.0325844576448134,
0.068400115398712));
#77709=CARTESIAN_POINT('Ctrl Pts',(0.00796460476350637,-0.0324744968375322,
0.0684017637200703));
#77710=CARTESIAN_POINT('Ctrl Pts',(0.00788545113079718,-0.0323646534831894,
0.068405047432015));
#77711=CARTESIAN_POINT('Ctrl Pts',(0.00804470114107275,-0.0326943950436605,
0.0683182834087079));
#77712=CARTESIAN_POINT('Ctrl Pts',(0.00796432915664294,-0.0325844576448134,
0.0683193732938186));
#77713=CARTESIAN_POINT('Ctrl Pts',(0.00788397402477391,-0.0324744968375322,
0.0683221254804718));
#77714=CARTESIAN_POINT('Ctrl Pts',(0.00780373865250897,-0.0323646534831894,
0.0683265350223373));
#77715=CARTESIAN_POINT('Ctrl Pts',(0.0079663034731018,-0.0326943950436605,
0.0682364608370169));
#77716=CARTESIAN_POINT('Ctrl Pts',(0.00788480382028225,-0.0325844576448134,
0.0682386311889251));
#77717=CARTESIAN_POINT('Ctrl Pts',(0.00780334328604146,-0.0324744968375322,
0.0682424872408734));
#77718=CARTESIAN_POINT('Ctrl Pts',(0.00772202617422075,-0.0323646534831894,
0.0682480226126596));
#77719=CARTESIAN_POINT('Ctrl Pts',(0.00788790580513086,-0.0326943950436605,
0.0681546382653259));
#77720=CARTESIAN_POINT('Ctrl Pts',(0.00780527848392157,-0.0325844576448134,
0.0681578890840317));
#77721=CARTESIAN_POINT('Ctrl Pts',(0.007722712547309,-0.0324744968375322,
0.0681628490012749));
#77722=CARTESIAN_POINT('Ctrl Pts',(0.00764031369593254,-0.0323646534831894,
0.0681695102029818));
#77723=CARTESIAN_POINT('',(0.00787510014324013,-0.0326773559991159,0.0681551557803234));
#77724=CARTESIAN_POINT('',(0.00788790580513014,-0.0326943950436595,0.0681546382653259));
#77725=CARTESIAN_POINT('Origin',(0.00861353130803579,-0.0326395669917778,
0.084743947908737));
#77726=CARTESIAN_POINT('Ctrl Pts',(0.00787510014337409,-0.032677355998742,
0.0681551557836675));
#77727=CARTESIAN_POINT('Ctrl Pts',(0.00787688043461156,-0.0326267922585957,
0.0681980723055467));
#77728=CARTESIAN_POINT('Ctrl Pts',(0.00787862917147246,-0.0325756109579314,
0.0682402281630666));
#77729=CARTESIAN_POINT('Ctrl Pts',(0.00788206502470259,-0.0324719985462369,
0.0683230544261068));
#77730=CARTESIAN_POINT('Ctrl Pts',(0.00788375076304503,-0.0324196091621773,
0.0683636916122777));
#77731=CARTESIAN_POINT('Ctrl Pts',(0.00788540558803144,-0.0323666188837756,
0.0684035835868263));
#77732=CARTESIAN_POINT('',(0.00800480088120298,-0.0326943950436704,0.0682766400542803));
#77733=CARTESIAN_POINT('Origin',(0.00812378219310841,-0.0315241814719618,
0.07415));
#77734=CARTESIAN_POINT('',(0.00787510014324197,-0.0327114338379884,0.0681551557803679));
#77735=CARTESIAN_POINT('',(0.00786229561583587,-0.0326943950436593,0.0681557006439515));
#77736=CARTESIAN_POINT('Origin',(0.00865876418508889,-0.0326395670442531,
0.0847412958988538));
#77737=CARTESIAN_POINT('Origin',(0.0085131371617776,-0.0326395678070698,
0.0847481145319865));
#77738=CARTESIAN_POINT('Origin',(0.00846784000449152,-0.0326395679529206,
0.0847492139789644));
#77739=CARTESIAN_POINT('Ctrl Pts',(0.00804645456722067,-0.0332451089994434,
0.0683991613273998));
#77740=CARTESIAN_POINT('Ctrl Pts',(0.00782955813807205,-0.0329451141710254,
0.0684020777865259));
#77741=CARTESIAN_POINT('Ctrl Pts',(0.00761349756841127,-0.0326442513127493,
0.0684213234860225));
#77742=CARTESIAN_POINT('Ctrl Pts',(0.00779660926602679,-0.0332451089994434,
0.0684079548176817));
#77743=CARTESIAN_POINT('Ctrl Pts',(0.00758004448879027,-0.0329451141710254,
0.0684202943465118));
#77744=CARTESIAN_POINT('Ctrl Pts',(0.00736502441298541,-0.0326442513127493,
0.0684489113643881));
#77745=CARTESIAN_POINT('Ctrl Pts',(0.00779411081301486,-0.0332451089994434,
0.0684080427525845));
#77746=CARTESIAN_POINT('Ctrl Pts',(0.00757754935229745,-0.0329451141710254,
0.0684204765121117));
#77747=CARTESIAN_POINT('Ctrl Pts',(0.00736253968143116,-0.0326442513127493,
0.0684491872431718));
#77748=CARTESIAN_POINT('',(0.0077605693073013,-0.0331951640388616,0.0684101218305974));
#77749=CARTESIAN_POINT('',(0.00752505548329177,-0.0328677532354991,0.0684298906132163));
#77750=CARTESIAN_POINT('Origin',(0.00958459726176004,-0.0326402808280928,
0.0850746101061591));
#77751=CARTESIAN_POINT('Origin',(0.00637373518186439,-0.0326944278779095,
0.05743403482466));
#77752=CARTESIAN_POINT('',(0.00764951775477939,-0.0326943950436593,0.0684182290483187));
#77753=CARTESIAN_POINT('',(0.00758735733926293,-0.0326943950436694,0.0684247354099524));
#77754=CARTESIAN_POINT('',(0.0078854055880323,-0.0330220786163545,0.0684035835867775));
#77755=CARTESIAN_POINT('Origin',(0.00911071887922066,-0.0326396682763578,
0.0851558007694508));
#77756=CARTESIAN_POINT('',(0.00788546189524771,-0.0331951640388588,0.0684049409545569));
#77757=CARTESIAN_POINT('Origin',(0.0074282336680204,-0.0331952026560223,
0.0573827673067081));
#77758=CARTESIAN_POINT('',(0.00782301560128451,-0.0331951640388702,0.0684075313925871));
#77759=CARTESIAN_POINT('Ctrl Pts',(0.00811026859573352,-0.0330240426238172,
0.0681500152181272));
#77760=CARTESIAN_POINT('Ctrl Pts',(0.00802761295986126,-0.032914277406352,
0.0681502013810968));
#77761=CARTESIAN_POINT('Ctrl Pts',(0.00794491996564863,-0.0328043479726691,
0.068152096359756));
#77762=CARTESIAN_POINT('Ctrl Pts',(0.00786229561583584,-0.0326943950436593,
0.0681557006439515));
#77763=CARTESIAN_POINT('Ctrl Pts',(0.00803533945271779,-0.0330240426238172,
0.0682350255675641));
#77764=CARTESIAN_POINT('Ctrl Pts',(0.00795385491723059,-0.032914277406352,
0.0682362439524786));
#77765=CARTESIAN_POINT('Ctrl Pts',(0.00787235494615025,-0.0328043479726691,
0.0682391474577668));
#77766=CARTESIAN_POINT('Ctrl Pts',(0.00779094404944688,-0.0326943950436593,
0.0682437352391871));
#77767=CARTESIAN_POINT('Ctrl Pts',(0.00796041030970206,-0.0330240426238172,
0.068320035917001));
#77768=CARTESIAN_POINT('Ctrl Pts',(0.00788009687459993,-0.032914277406352,
0.0683222865238605));
#77769=CARTESIAN_POINT('Ctrl Pts',(0.00779978992665187,-0.0328043479726691,
0.0683261985557777));
#77770=CARTESIAN_POINT('Ctrl Pts',(0.00771959248305792,-0.0326943950436593,
0.0683317698344226));
#77771=CARTESIAN_POINT('Ctrl Pts',(0.00788548116668633,-0.0330240426238172,
0.0684050462664379));
#77772=CARTESIAN_POINT('Ctrl Pts',(0.00780633883196926,-0.032914277406352,
0.0684083290952423));
#77773=CARTESIAN_POINT('Ctrl Pts',(0.00772722490715349,-0.0328043479726691,
0.0684132496537885));
#77774=CARTESIAN_POINT('Ctrl Pts',(0.00764824091666895,-0.0326943950436593,
0.0684198044296582));
#77775=CARTESIAN_POINT('',(0.00775590668531764,-0.0326943950436693,0.0682869648461451));
#77776=CARTESIAN_POINT('Ctrl Pts',(0.00787510014337457,-0.0327114338383341,
0.0681551557836757));
#77777=CARTESIAN_POINT('Ctrl Pts',(0.00787688013849059,-0.0327619876830805,
0.0681980651671147));
#77778=CARTESIAN_POINT('Ctrl Pts',(0.00787862873071166,-0.0328131562603977,
0.0682402175378805));
#77779=CARTESIAN_POINT('Ctrl Pts',(0.0078820645807877,-0.0329167375858776,
0.0683230437248869));
#77780=CARTESIAN_POINT('Ctrl Pts',(0.00788375046962117,-0.0329691088920625,
0.0683636845388643));
#77781=CARTESIAN_POINT('Ctrl Pts',(0.00788540558803146,-0.0330220786163187,
0.0684035835868251));
#77782=CARTESIAN_POINT('Ctrl Pts',(0.00776206156301519,-0.0331951640388604,
0.0684114952120716));
#77783=CARTESIAN_POINT('Ctrl Pts',(0.0076434216557117,-0.0330306422010619,
0.068418973554185));
#77784=CARTESIAN_POINT('Ctrl Pts',(0.00752519221312171,-0.0328657861914644,
0.0684313490182411));
#77785=CARTESIAN_POINT('Ctrl Pts',(0.00776056930730447,-0.0331951640388604,
0.0684101218305973));
#77786=CARTESIAN_POINT('Ctrl Pts',(0.00764190100621953,-0.0330306422010619,
0.0684176310241408));
#77787=CARTESIAN_POINT('Ctrl Pts',(0.00752364446923242,-0.0328657861914644,
0.0684300384868095));
#77788=CARTESIAN_POINT('Ctrl Pts',(0.0075119193752158,-0.0331951640388604,
0.0681812795431449));
#77789=CARTESIAN_POINT('Ctrl Pts',(0.00738851990655781,-0.0330306422010619,
0.0681939294146148));
#77790=CARTESIAN_POINT('Ctrl Pts',(0.00726574871437195,-0.0328657861914644,
0.0682116687066678));
#77791=CARTESIAN_POINT('',(0.00749917147791584,-0.0331781648281892,0.0681826001097433));
#77792=CARTESIAN_POINT('',(0.00751191937521466,-0.0331951640388588,0.068181279543145));
#77793=CARTESIAN_POINT('Origin',(0.00992597004207064,-0.0326412092057475,
0.0845257066684922));
#77794=CARTESIAN_POINT('Ctrl Pts',(0.00749917147951614,-0.033178164828644,
0.0681826001106365));
#77795=CARTESIAN_POINT('Ctrl Pts',(0.0075036460989602,-0.0331276811546782,
0.0682253495708871));
#77796=CARTESIAN_POINT('Ctrl Pts',(0.00750803995426746,-0.0330765663497791,
0.068267327104754));
#77797=CARTESIAN_POINT('Ctrl Pts',(0.00751666975043236,-0.032973061446316,
0.0683497744026723));
#77798=CARTESIAN_POINT('Ctrl Pts',(0.0075209021997093,-0.0329207133373781,
0.0683902108603701));
#77799=CARTESIAN_POINT('Ctrl Pts',(0.00752505549628465,-0.0328677532289351,
0.0684298906030954));
#77800=CARTESIAN_POINT('',(0.00763624434126798,-0.0331951640388702,0.0682957006868812));
#77801=CARTESIAN_POINT('Origin',(0.00812378219310841,-0.0315241814719618,
0.07415));
#77802=CARTESIAN_POINT('',(0.007499171477434,-0.033212160714424,0.068182600111353));
#77803=CARTESIAN_POINT('',(0.00748642642908472,-0.0331951640388587,0.0681839479025));
#77804=CARTESIAN_POINT('Origin',(0.00996957324839171,-0.0326413653794834,
0.0845132577386242));
#77805=CARTESIAN_POINT('Origin',(0.00850917857750277,-0.0326412099826809,
0.0846740047827594));
#77806=CARTESIAN_POINT('Origin',(0.00846394233505875,-0.0326413662553115,
0.0846708507653181));
#77807=CARTESIAN_POINT('Ctrl Pts',(0.00768552977863837,-0.0337436976235975,
0.0684153631482707));
#77808=CARTESIAN_POINT('Ctrl Pts',(0.00763395158568592,-0.0336723290703325,
0.0684193048569054));
#77809=CARTESIAN_POINT('Ctrl Pts',(0.00758245263578412,-0.033601104548885,
0.0684241736569848));
#77810=CARTESIAN_POINT('Ctrl Pts',(0.00741802669011486,-0.0333736987606857,
0.068439718771183));
#77811=CARTESIAN_POINT('Ctrl Pts',(0.00725476377368111,-0.0331450831799191,
0.0684646739770972));
#77812=CARTESIAN_POINT('Ctrl Pts',(0.00743672954929019,-0.0337436976235975,
0.0684398263017117));
#77813=CARTESIAN_POINT('Ctrl Pts',(0.00738537138164728,-0.0336723290703325,
0.068446005757316));
#77814=CARTESIAN_POINT('Ctrl Pts',(0.00733413267147486,-0.033601104548885,
0.0684531079847882));
#77815=CARTESIAN_POINT('Ctrl Pts',(0.00717053761971092,-0.0333736987606857,
0.068475783990235));
#77816=CARTESIAN_POINT('Ctrl Pts',(0.00700851343959128,-0.0331450831799191,
0.0685078106547699));
#77817=CARTESIAN_POINT('Ctrl Pts',(0.00743424154699671,-0.0337436976235975,
0.0684400709332462));
#77818=CARTESIAN_POINT('Ctrl Pts',(0.0073828855796069,-0.0336723290703325,
0.0684462727663201));
#77819=CARTESIAN_POINT('Ctrl Pts',(0.00733164947183177,-0.033601104548885,
0.0684533973280662));
#77820=CARTESIAN_POINT('Ctrl Pts',(0.00716806272900688,-0.0333736987606857,
0.0684761446424256));
#77821=CARTESIAN_POINT('Ctrl Pts',(0.00700605093625038,-0.0331450831799191,
0.0685082420215466));
#77822=CARTESIAN_POINT('',(0.00740087609265772,-0.0336938721132548,0.0684442544948156));
#77823=CARTESIAN_POINT('',(0.00716706829378607,-0.0333679870047996,0.0684787723097453));
#77824=CARTESIAN_POINT('Ctrl Pts',(0.00740087609268289,-0.0336938721132527,
0.0684442544948124));
#77825=CARTESIAN_POINT('Ctrl Pts',(0.00737860389135478,-0.0336629187933872,
0.0684470763364449));
#77826=CARTESIAN_POINT('Ctrl Pts',(0.00735635533622876,-0.033631995230101,
0.0684500276882784));
#77827=CARTESIAN_POINT('Ctrl Pts',(0.00733413267148733,-0.033601104548892,
0.0684531079847866));
#77828=CARTESIAN_POINT('Ctrl Pts',(0.00727836840148316,-0.0335235892595422,
0.0684608375027439));
#77829=CARTESIAN_POINT('Ctrl Pts',(0.00722266809226004,-0.0334458668665538,
0.0684693928415299));
#77830=CARTESIAN_POINT('Ctrl Pts',(0.0071670683053924,-0.0333679869962462,
0.068478772307524));
#77831=CARTESIAN_POINT('Ctrl Pts',(0.00716702433611697,-0.0333679692470407,
0.0684787790278612));
#77832=CARTESIAN_POINT('Ctrl Pts',(0.00716710557115595,-0.0333391895416172,
0.0684792249411365));
#77833=CARTESIAN_POINT('Ctrl Pts',(0.00716716965538581,-0.0333104081131861,
0.0684795585929379));
#77834=CARTESIAN_POINT('Ctrl Pts',(0.00716725992084898,-0.0332532698396013,
0.0684799991934275));
#77835=CARTESIAN_POINT('Ctrl Pts',(0.00716728665582308,-0.0332249171946172,
0.068480109450876));
#77836=CARTESIAN_POINT('Ctrl Pts',(0.00716729406987529,-0.0331960985338305,
0.0684801119224179));
#77837=CARTESIAN_POINT('Ctrl Pts',(0.00716729418510157,-0.033195631258691,
0.0684801119331561));
#77838=CARTESIAN_POINT('Ctrl Pts',(0.00716729429479814,-0.0331951640388587,
0.0684801119146507));
#77839=CARTESIAN_POINT('',(0.00729055273143395,-0.0331951640388587,0.0684593186994703));
#77840=CARTESIAN_POINT('',(0.00722892351312492,-0.0331951640388687,0.0684697153070706));
#77841=CARTESIAN_POINT('',(0.00752505549800226,-0.033521636656774,0.068429890618188));
#77842=CARTESIAN_POINT('Origin',(0.0104586076404711,-0.0326434571524804,
0.0848239424923361));
#77843=CARTESIAN_POINT('',(0.00752519692372646,-0.0336938721132327,0.0684312417715662));
#77844=CARTESIAN_POINT('Origin',(0.00638834720438303,-0.0336938867896287,
0.0575700078327438));
#77845=CARTESIAN_POINT('',(0.00746303650820209,-0.0336938721132538,0.0684377481332009));
#77846=CARTESIAN_POINT('Ctrl Pts',(0.00773355214107778,-0.0335235895815172,
0.0681627034058339));
#77847=CARTESIAN_POINT('Ctrl Pts',(0.00765112521555684,-0.0334144449262748,
0.0681680756907924));
#77848=CARTESIAN_POINT('Ctrl Pts',(0.00756871457884892,-0.0333049234473147,
0.0681751570261036));
#77849=CARTESIAN_POINT('Ctrl Pts',(0.00748642642908477,-0.0331951640388587,
0.0681839479024999));
#77850=CARTESIAN_POINT('Ctrl Pts',(0.00766410861326214,-0.0335235895815172,
0.0682522509849771));
#77851=CARTESIAN_POINT('Ctrl Pts',(0.00758291448647106,-0.0334144449262748,
0.0682585792968177));
#77852=CARTESIAN_POINT('Ctrl Pts',(0.00750175781562528,-0.0333049234473147,
0.068266592288676));
#77853=CARTESIAN_POINT('Ctrl Pts',(0.00742074330333155,-0.0331951640388587,
0.0682762891147356));
#77854=CARTESIAN_POINT('Ctrl Pts',(0.00759466508544649,-0.0335235895815172,
0.0683417985641202));
#77855=CARTESIAN_POINT('Ctrl Pts',(0.00751470375738527,-0.0334144449262748,
0.0683490829028429));
#77856=CARTESIAN_POINT('Ctrl Pts',(0.00743480105240163,-0.0333049234473147,
0.0683580275512484));
#77857=CARTESIAN_POINT('Ctrl Pts',(0.00735506017757833,-0.0331951640388587,
0.0683686303269713));
#77858=CARTESIAN_POINT('Ctrl Pts',(0.00752522155763084,-0.0335235895815172,
0.0684313461432633));
#77859=CARTESIAN_POINT('Ctrl Pts',(0.00744649302829949,-0.0334144449262748,
0.0684395865088681));
#77860=CARTESIAN_POINT('Ctrl Pts',(0.00736784428917799,-0.0333049234473147,
0.0684494628138208));
#77861=CARTESIAN_POINT('Ctrl Pts',(0.00728937705182512,-0.0331951640388587,
0.068460971539207));
#77862=CARTESIAN_POINT('',(0.00738848958026934,-0.0331951640388687,0.0683216333009952));
#77863=CARTESIAN_POINT('Ctrl Pts',(0.00749917147775533,-0.0332121607145994,
0.0681826001144633));
#77864=CARTESIAN_POINT('Ctrl Pts',(0.00750363855772909,-0.0332625444109625,
0.0682252776604436));
#77865=CARTESIAN_POINT('Ctrl Pts',(0.007508028662905,-0.0333135300746545,
0.0682672198053353));
#77866=CARTESIAN_POINT('Ctrl Pts',(0.00751665840847482,-0.0334167203140651,
0.0683496665861217));
#77867=CARTESIAN_POINT('Ctrl Pts',(0.00752089470649319,-0.0334688847587347,
0.0683901392896609));
#77868=CARTESIAN_POINT('Ctrl Pts',(0.00752505549790497,-0.0335216366562424,
0.0684298906189037));
#77869=CARTESIAN_POINT('Ctrl Pts',(0.00740245127064529,-0.0336938721132526,
0.0684455311680823));
#77870=CARTESIAN_POINT('Ctrl Pts',(0.00736906112162373,-0.0336474569765026,
0.068449753357335));
#77871=CARTESIAN_POINT('Ctrl Pts',(0.00733572268657267,-0.033601104548885,
0.0684543661311333));
#77872=CARTESIAN_POINT('Ctrl Pts',(0.0072513174340225,-0.0334837508592655,
0.0684660446138457));
#77873=CARTESIAN_POINT('Ctrl Pts',(0.00716729530369496,-0.0333660264659096,
0.0684802190708632));
#77874=CARTESIAN_POINT('Ctrl Pts',(0.00740087609268784,-0.0336938721132526,
0.0684442544948119));
#77875=CARTESIAN_POINT('Ctrl Pts',(0.00736747847087398,-0.0336474569765026,
0.0684484859041039));
#77876=CARTESIAN_POINT('Ctrl Pts',(0.00733413267147486,-0.033601104548885,
0.0684531079847882));
#77877=CARTESIAN_POINT('Ctrl Pts',(0.00724970877408859,-0.0334837508592655,
0.0684648100303961));
#77878=CARTESIAN_POINT('Ctrl Pts',(0.00716566870532982,-0.0333660264659096,
0.0684790085924473));
#77879=CARTESIAN_POINT('Ctrl Pts',(0.00713677251785141,-0.0336938721132526,
0.0682301999665531));
#77880=CARTESIAN_POINT('Ctrl Pts',(0.00710212196385264,-0.0336474569765026,
0.0682359772617078));
#77881=CARTESIAN_POINT('Ctrl Pts',(0.00706754141466618,-0.033601104548885,
0.0682421597894828));
#77882=CARTESIAN_POINT('Ctrl Pts',(0.00697999141470561,-0.0334837508592655,
0.0682578125283545));
#77883=CARTESIAN_POINT('Ctrl Pts',(0.00689294368335894,-0.0333660264659096,
0.0682760526817168));
#77884=CARTESIAN_POINT('',(0.00712570786443446,-0.0336769361243754,0.068233595041375));
#77885=CARTESIAN_POINT('',(0.00713834768830781,-0.0336938721132328,0.0682314766337583));
#77886=CARTESIAN_POINT('Ctrl Pts',(0.00712570786443419,-0.0336769361243751,
0.0682335950413751));
#77887=CARTESIAN_POINT('Ctrl Pts',(0.00712781428237837,-0.033679758666975,
0.0682332396969235));
#77888=CARTESIAN_POINT('Ctrl Pts',(0.00712992081042633,-0.0336825812712295,
0.0682328854908329));
#77889=CARTESIAN_POINT('Ctrl Pts',(0.00713413409255186,-0.0336882266108864,
0.0682321793538773));
#77890=CARTESIAN_POINT('Ctrl Pts',(0.00713624084656904,-0.0336910493461957,
0.0682318274230456));
#77891=CARTESIAN_POINT('Ctrl Pts',(0.00713834768831345,-0.0336938721132294,
0.0682314766337654));
#77892=CARTESIAN_POINT('Ctrl Pts',(0.00712570786443447,-0.0336769361243754,
0.0682335950413751));
#77893=CARTESIAN_POINT('Ctrl Pts',(0.0071326800361329,-0.033627900766312,
0.068274924820154));
#77894=CARTESIAN_POINT('Ctrl Pts',(0.00713975148078475,-0.0335767878929294,
0.0683168430711277));
#77895=CARTESIAN_POINT('Ctrl Pts',(0.00715360953070402,-0.0334733199164922,
0.0683989910964836));
#77896=CARTESIAN_POINT('Ctrl Pts',(0.00716040438618989,-0.0334209645169725,
0.0684392697766759));
#77897=CARTESIAN_POINT('Ctrl Pts',(0.00716706830828396,-0.0333679869844681,
0.0684787723072879));
#77898=CARTESIAN_POINT('',(0.00726961189049276,-0.0336938721132538,0.068337865564297));
#77899=CARTESIAN_POINT('Origin',(0.00812378219310841,-0.0315241814719618,
0.07415));
#77900=CARTESIAN_POINT('',(0.00712570786465501,-0.0337108120655413,0.0682335950426601));
#77901=CARTESIAN_POINT('',(0.00711307259435403,-0.0336938721132327,0.0682357404430475));
#77902=CARTESIAN_POINT('Origin',(0.00874529130525542,-0.0345562517440147,
0.0845527643280791));
#77903=CARTESIAN_POINT('Ctrl Pts',(0.00711307259435331,-0.033693872113232,
0.0682357404430494));
#77904=CARTESIAN_POINT('Ctrl Pts',(0.00711517793149364,-0.0336910493284972,
0.0682353806542312));
#77905=CARTESIAN_POINT('Ctrl Pts',(0.00711728354044955,-0.0336882266020367,
0.0682350219759683));
#77906=CARTESIAN_POINT('Ctrl Pts',(0.00712149529799299,-0.0336825812712153,
0.0682343068417588));
#77907=CARTESIAN_POINT('Ctrl Pts',(0.00712360144649586,-0.0336797586669679,
0.0682339503858257));
#77908=CARTESIAN_POINT('Ctrl Pts',(0.00712570786443473,-0.0336769361243751,
0.068233595041375));
#77909=CARTESIAN_POINT('Origin',(0.0109493597483956,-0.0345562517879156,
0.0841809445835711));
#77910=CARTESIAN_POINT('Ctrl Pts',(0.00732636488129234,-0.034243627687391,
0.0684541900812249));
#77911=CARTESIAN_POINT('Ctrl Pts',(0.00711154386883641,-0.0339430054201809,
0.0684842651709342));
#77912=CARTESIAN_POINT('Ctrl Pts',(0.00689959851934188,-0.0336441434784052,
0.0685304360193264));
#77913=CARTESIAN_POINT('Ctrl Pts',(0.00707959129702041,-0.034243627687391,
0.0684942250422663));
#77914=CARTESIAN_POINT('Ctrl Pts',(0.00686628022801189,-0.0339430054201809,
0.0685336073511379));
#77915=CARTESIAN_POINT('Ctrl Pts',(0.00665654159025616,-0.0336441434784052,
0.0685889452427313));
#77916=CARTESIAN_POINT('Ctrl Pts',(0.00707712356117769,-0.034243627687391,
0.0684946253918768));
#77917=CARTESIAN_POINT('Ctrl Pts',(0.00686382759160364,-0.0339430054201809,
0.06853410077294));
#77918=CARTESIAN_POINT('Ctrl Pts',(0.00665411102096531,-0.0336441434784052,
0.0685895303349653));
#77919=CARTESIAN_POINT('',(0.00704403585815788,-0.0341934961088741,0.0685009051298317));
#77920=CARTESIAN_POINT('',(0.00681285682892965,-0.0338664212873204,0.0685500357415913));
#77921=CARTESIAN_POINT('Origin',(0.00968378016107057,-0.0345610751536084,
0.0850261850981422));
#77922=CARTESIAN_POINT('Origin',(0.00431323542083257,-0.0336938005063867,
0.0578724600114735));
#77923=CARTESIAN_POINT('',(0.00693487608410741,-0.0336938721132327,0.0685228668698901));
#77924=CARTESIAN_POINT('',(0.00687402128537482,-0.0336938721132427,0.0685371126927967));
#77925=CARTESIAN_POINT('',(0.00716706830828924,-0.0340203938281605,0.068478772307287));
#77926=CARTESIAN_POINT('Origin',(0.00920260502512305,-0.0345589643243972,
0.0850279273847569));
#77927=CARTESIAN_POINT('',(0.00716729429479592,-0.034193496108874,0.068480111914651));
#77928=CARTESIAN_POINT('Origin',(0.00533425715374061,-0.0341934220717661,
0.057614193034139));
#77929=CARTESIAN_POINT('',(0.00710566507648691,-0.0341934961088841,0.0684905085222514));
#77930=CARTESIAN_POINT('Ctrl Pts',(0.00735837942108477,-0.0340223579322397,
0.0681990203666452));
#77931=CARTESIAN_POINT('Ctrl Pts',(0.00727629989113435,-0.0339125849573575,
0.0682095772671256));
#77932=CARTESIAN_POINT('Ctrl Pts',(0.0071944965408284,-0.0338030433565231,
0.0682218256049378));
#77933=CARTESIAN_POINT('Ctrl Pts',(0.00711307259435439,-0.0336938721132327,
0.0682357404430468));
#77934=CARTESIAN_POINT('Ctrl Pts',(0.00729469560226883,-0.0340223579322397,
0.0682927516370478));
#77935=CARTESIAN_POINT('Ctrl Pts',(0.00721390887099868,-0.0339125849573575,
0.0683041869034841));
#77936=CARTESIAN_POINT('Ctrl Pts',(0.00713341559107257,-0.0338030433565231,
0.0683172862321059));
#77937=CARTESIAN_POINT('Ctrl Pts',(0.00705331721484792,-0.0336938721132327,
0.0683320237461181));
#77938=CARTESIAN_POINT('Ctrl Pts',(0.00723101178345289,-0.0340223579322397,
0.0683864829074505));
#77939=CARTESIAN_POINT('Ctrl Pts',(0.00715151785086301,-0.0339125849573575,
0.0683987965398426));
#77940=CARTESIAN_POINT('Ctrl Pts',(0.00707233464131675,-0.0338030433565231,
0.068412746859274));
#77941=CARTESIAN_POINT('Ctrl Pts',(0.00699356183534144,-0.0336938721132327,
0.0684283070491894));
#77942=CARTESIAN_POINT('Ctrl Pts',(0.00716732796463695,-0.0340223579322397,
0.0684802141778531));
#77943=CARTESIAN_POINT('Ctrl Pts',(0.00708912683072734,-0.0339125849573575,
0.0684934061762011));
#77944=CARTESIAN_POINT('Ctrl Pts',(0.00701125369156093,-0.0338030433565231,
0.0685082074864422));
#77945=CARTESIAN_POINT('Ctrl Pts',(0.00693380645583497,-0.0336938721132327,
0.0685245903522606));
#77946=CARTESIAN_POINT('',(0.00702397433924072,-0.0336938721132427,0.0683793036564788));
#77947=CARTESIAN_POINT('Ctrl Pts',(0.00712570786524982,-0.0337108120662702,
0.0682335950462078));
#77948=CARTESIAN_POINT('Ctrl Pts',(0.00713286060753573,-0.0337611408994164,
0.0682759952149251));
#77949=CARTESIAN_POINT('Ctrl Pts',(0.00713988282814399,-0.0338121088781025,
0.0683176216746322));
#77950=CARTESIAN_POINT('Ctrl Pts',(0.00715367262314392,-0.0339153382773243,
0.068399365097113));
#77951=CARTESIAN_POINT('Ctrl Pts',(0.00716043436360203,-0.0339675558473115,
0.0684394474773785));
#77952=CARTESIAN_POINT('Ctrl Pts',(0.00716706830829067,-0.0340203938281304,
0.0684787723073271));
#77953=CARTESIAN_POINT('Ctrl Pts',(0.00704568855271773,-0.0341934961088741,
0.0685020807061749));
#77954=CARTESIAN_POINT('Ctrl Pts',(0.0069289222710861,-0.0340287516186244,
0.0685243694428034));
#77955=CARTESIAN_POINT('Ctrl Pts',(0.00681317697440068,-0.0338644633283558,
0.0685514651731272));
#77956=CARTESIAN_POINT('Ctrl Pts',(0.00704403585815796,-0.0341934961088741,
0.0685009051298318));
#77957=CARTESIAN_POINT('Ctrl Pts',(0.00692724527241162,-0.0340287516186244,
0.0685232280346182));
#77958=CARTESIAN_POINT('Ctrl Pts',(0.00681147710457479,-0.0338644633283559,
0.0685503589084114));
#77959=CARTESIAN_POINT('Ctrl Pts',(0.00676866506118924,-0.0341934961088741,
0.0683050314321821));
#77960=CARTESIAN_POINT('Ctrl Pts',(0.006647824941065,-0.0340287516186244,
0.0683330474112423));
#77961=CARTESIAN_POINT('Ctrl Pts',(0.00652824599817819,-0.0338644633283559,
0.0683660338650138));
#77962=CARTESIAN_POINT('',(0.00675618319603834,-0.034176475883238,0.068307939321287));
#77963=CARTESIAN_POINT('',(0.00676866506118928,-0.034193496108874,0.0683050314321821));
#77964=CARTESIAN_POINT('Origin',(0.0100316246976099,-0.0345621026625278,
0.084546560318849));
#77965=CARTESIAN_POINT('Ctrl Pts',(0.00675618319779017,-0.0341764758837466,
0.0683079393217599));
#77966=CARTESIAN_POINT('Ctrl Pts',(0.00676596710045816,-0.0341260050041473,
0.0683497337883827));
#77967=CARTESIAN_POINT('Ctrl Pts',(0.00677558097301842,-0.0340749269150289,
0.0683908017598703));
#77968=CARTESIAN_POINT('Ctrl Pts',(0.0067944759301737,-0.0339715436310858,
0.0684715165824595));
#77969=CARTESIAN_POINT('Ctrl Pts',(0.00680374984062147,-0.0339192778243037,
0.0685111328135425));
#77970=CARTESIAN_POINT('Ctrl Pts',(0.00681285683097385,-0.0338664212861684,
0.0685500357395477));
#77971=CARTESIAN_POINT('',(0.00690635045968359,-0.0341934961088841,0.0684029682810169));
#77972=CARTESIAN_POINT('Origin',(0.00812378219310841,-0.0315241814719618,
0.07415));
#77973=CARTESIAN_POINT('',(0.00675618319538678,-0.0342105180190554,0.068307939322196));
#77974=CARTESIAN_POINT('',(0.00674370756866026,-0.0341934961088739,0.068310873864098));
#77975=CARTESIAN_POINT('Origin',(0.0100766559208261,-0.03456217101078,0.0845413933107676));
#77976=CARTESIAN_POINT('Origin',(0.0110288640294853,-0.0345621035739969,
0.0843131131097792));
#77977=CARTESIAN_POINT('Origin',(0.0109862174074218,-0.0345621718861817,
0.0843284667798951));
#77978=CARTESIAN_POINT('Ctrl Pts',(0.00693633660892827,-0.0346945769586966,
0.0685225249678815));
#77979=CARTESIAN_POINT('Ctrl Pts',(0.00681846689126245,-0.0345275153362944,
0.0685473964910694));
#77980=CARTESIAN_POINT('Ctrl Pts',(0.00670134887296188,-0.0343603235965185,
0.0685759813414362));
#77981=CARTESIAN_POINT('Ctrl Pts',(0.00658532768063191,-0.0341934961088739,
0.068608189829528));
#77982=CARTESIAN_POINT('Ctrl Pts',(0.00685471003537714,-0.0346945769586966,
0.0685416333658137));
#77983=CARTESIAN_POINT('Ctrl Pts',(0.00673724055075659,-0.0345275153362944,
0.0685682145902662));
#77984=CARTESIAN_POINT('Ctrl Pts',(0.00662057663755315,-0.0343603235965185,
0.0685984969971529));
#77985=CARTESIAN_POINT('Ctrl Pts',(0.00650506200471142,-0.0341934961088739,
0.0686323858963626));
#77986=CARTESIAN_POINT('Ctrl Pts',(0.00677308346182602,-0.0346945769586966,
0.0685607417637437));
#77987=CARTESIAN_POINT('Ctrl Pts',(0.00665601421025059,-0.0345275153362944,
0.0685890326894601));
#77988=CARTESIAN_POINT('Ctrl Pts',(0.0065398044021443,-0.0343603235965185,
0.0686210126528679));
#77989=CARTESIAN_POINT('Ctrl Pts',(0.00642479632879096,-0.0341934961088739,
0.0686565819631985));
#77990=CARTESIAN_POINT('Ctrl Pts',(0.00669145688827487,-0.0346945769586966,
0.0685798501616782));
#77991=CARTESIAN_POINT('Ctrl Pts',(0.00657478786974487,-0.0345275153362944,
0.0686098507886597));
#77992=CARTESIAN_POINT('Ctrl Pts',(0.00645903216673571,-0.0343603235965185,
0.0686435283085863));
#77993=CARTESIAN_POINT('Ctrl Pts',(0.00634453065287045,-0.0341934961088739,
0.0686807780300318));
#77994=CARTESIAN_POINT('',(0.00669145688913151,-0.0346945769586966,0.0685798501614778));
#77995=CARTESIAN_POINT('',(0.00646381897772016,-0.034366772783276,0.068643399676385));
#77996=CARTESIAN_POINT('Origin',(0.0110556904213785,-0.0345626461564986,
0.0848171748300519));
#77997=CARTESIAN_POINT('Origin',(0.00327392128255998,-0.0341934771027958,
0.0580615658089922));
#77998=CARTESIAN_POINT('',(0.00658389150603352,-0.0341934961088739,0.0686086227639818));
#77999=CARTESIAN_POINT('',(0.00652405129296608,-0.034193496108884,0.06862666158044));
#78000=CARTESIAN_POINT('',(0.00681285683141268,-0.0345211942962713,0.0685500357415574));
#78001=CARTESIAN_POINT('Origin',(0.0105867782592795,-0.0345625596118762,
0.0849235307122997));
#78002=CARTESIAN_POINT('',(0.00681316648662224,-0.0346945769586886,0.0685513585156833));
#78003=CARTESIAN_POINT('Origin',(0.0042914133953859,-0.0346945685853918,
0.0577790200246689));
#78004=CARTESIAN_POINT('',(0.00675231168788688,-0.0346945769587026,0.0685656043385906));
#78005=CARTESIAN_POINT('Ctrl Pts',(0.00698622372100385,-0.0345231616327842,
0.0682588234857065));
#78006=CARTESIAN_POINT('Ctrl Pts',(0.00690502214686742,-0.0344132092796988,
0.0682745031276902));
#78007=CARTESIAN_POINT('Ctrl Pts',(0.00682414908338544,-0.0343032738558979,
0.0682918615511867));
#78008=CARTESIAN_POINT('Ctrl Pts',(0.00674370756866024,-0.0341934961088739,
0.068310873864098));
#78009=CARTESIAN_POINT('Ctrl Pts',(0.0069285511165796,-0.0345231616327842,
0.0683563683822279));
#78010=CARTESIAN_POINT('Ctrl Pts',(0.00684869406150948,-0.0344132092796988,
0.0683728429598671));
#78011=CARTESIAN_POINT('Ctrl Pts',(0.00676918189033981,-0.0343032738558979,
0.0683909684676876));
#78012=CARTESIAN_POINT('Ctrl Pts',(0.00669011587253975,-0.0341934961088739,
0.0684107190755274));
#78013=CARTESIAN_POINT('Ctrl Pts',(0.00687087851215535,-0.0345231616327842,
0.0684539132787493));
#78014=CARTESIAN_POINT('Ctrl Pts',(0.00679236597615154,-0.0344132092796988,
0.068471182792044));
#78015=CARTESIAN_POINT('Ctrl Pts',(0.00671421469729419,-0.0343032738558979,
0.0684900753841886));
#78016=CARTESIAN_POINT('Ctrl Pts',(0.00663652417641926,-0.0341934961088739,
0.0685105642869568));
#78017=CARTESIAN_POINT('Ctrl Pts',(0.00681320590773109,-0.0345231616327842,
0.0685514581752708));
#78018=CARTESIAN_POINT('Ctrl Pts',(0.00673603789079361,-0.0344132092796988,
0.0685695226242208));
#78019=CARTESIAN_POINT('Ctrl Pts',(0.00665924750424856,-0.0343032738558979,
0.0685891823006895));
#78020=CARTESIAN_POINT('Ctrl Pts',(0.00658293248029878,-0.0341934961088739,
0.0686104094983862));
#78021=CARTESIAN_POINT('',(0.00666379953735689,-0.0341934961088839,0.0684597483140499));
#78022=CARTESIAN_POINT('Ctrl Pts',(0.00675618319616943,-0.0342105180195406,
0.0683079393255548));
#78023=CARTESIAN_POINT('Ctrl Pts',(0.00676597808447636,-0.0342610556241096,
0.0683497807804818));
#78024=CARTESIAN_POINT('Ctrl Pts',(0.00677559720857732,-0.0343122189869719,
0.0683908714121353));
#78025=CARTESIAN_POINT('Ctrl Pts',(0.00679449236031797,-0.0344158119695203,
0.0684715870482019));
#78026=CARTESIAN_POINT('Ctrl Pts',(0.00680376065969012,-0.0344681990450108,
0.0685111790392771));
#78027=CARTESIAN_POINT('Ctrl Pts',(0.00681285683141085,-0.0345211942962532,
0.0685500357415825));
#78028=CARTESIAN_POINT('Ctrl Pts',(0.00669317971611005,-0.0346945769586932,
0.068580919382993));
#78029=CARTESIAN_POINT('Ctrl Pts',(0.00657804291494672,-0.0345296777077528,
0.0686104960769332));
#78030=CARTESIAN_POINT('Ctrl Pts',(0.00646422692867993,-0.0343648066252516,
0.0686448062077502));
#78031=CARTESIAN_POINT('Ctrl Pts',(0.00669145688914032,-0.0346945769586932,
0.0685798501614757));
#78032=CARTESIAN_POINT('Ctrl Pts',(0.00657629798257868,-0.0345296777077528,
0.0686094624736444));
#78033=CARTESIAN_POINT('Ctrl Pts',(0.0064624613819365,-0.0343648066252516,
0.0686438091058911));
#78034=CARTESIAN_POINT('Ctrl Pts',(0.00640433046229951,-0.0346945769586932,
0.06840165365123));
#78035=CARTESIAN_POINT('Ctrl Pts',(0.00628548746897756,-0.0345296777077528,
0.0684372020991076));
#78036=CARTESIAN_POINT('Ctrl Pts',(0.00616821527552477,-0.0343648066252516,
0.0684776320614004));
#78037=CARTESIAN_POINT('',(0.00639205581495692,-0.0346775396664964,0.0684053395448861));
#78038=CARTESIAN_POINT('',(0.00640433046229623,-0.0346945769586887,0.0684016536512309));
#78039=CARTESIAN_POINT('Origin',(0.0113296404334329,-0.0345626618229783,
0.0842556756019206));
#78040=CARTESIAN_POINT('Ctrl Pts',(0.00639205581671261,-0.0346775396670097,
0.068405339545346));
#78041=CARTESIAN_POINT('Ctrl Pts',(0.0064044544659018,-0.0346269749928334,
0.0684464695721525));
#78042=CARTESIAN_POINT('Ctrl Pts',(0.00641663279782036,-0.0345757902891081,
0.0684868686162392));
#78043=CARTESIAN_POINT('Ctrl Pts',(0.00644055869167247,-0.0344721681088438,
0.0685662380597165));
#78044=CARTESIAN_POINT('Ctrl Pts',(0.00645229686813701,-0.0344197714290001,
0.0686051773441915));
#78045=CARTESIAN_POINT('Ctrl Pts',(0.0064638189779905,-0.0343667727831519,
0.0686433996761315));
#78046=CARTESIAN_POINT('',(0.00654789367572387,-0.0346945769587026,0.0684907519063644));
#78047=CARTESIAN_POINT('Origin',(0.00812378219310841,-0.0315241814719618,
0.07415));
#78048=CARTESIAN_POINT('',(0.00639205581458973,-0.0347116136489626,0.0684053395462279));
#78049=CARTESIAN_POINT('',(0.00637978906701314,-0.0346945769586885,0.0684090516483639));
#78050=CARTESIAN_POINT('Origin',(0.0113724486185158,-0.0345626688543831,
0.0842408196828196));
#78051=CARTESIAN_POINT('Origin',(0.0110372063907197,-0.0345626626523952,
0.0843438322450094));
#78052=CARTESIAN_POINT('Origin',(0.010993318521225,-0.0345626697901873,
0.0843551060349324));
#78053=CARTESIAN_POINT('Ctrl Pts',(0.00662110080507579,-0.0352450361874068,
0.0685983601615324));
#78054=CARTESIAN_POINT('Ctrl Pts',(0.0064117172727439,-0.0349452760959493,
0.0686550347200684));
#78055=CARTESIAN_POINT('Ctrl Pts',(0.0062071975366287,-0.0346444289841739,
0.0687273198965322));
#78056=CARTESIAN_POINT('Ctrl Pts',(0.00661870271482155,-0.0352450361874068,
0.0685990666763112));
#78057=CARTESIAN_POINT('Ctrl Pts',(0.00640934582913179,-0.0349452760959493,
0.0686558316803052));
#78058=CARTESIAN_POINT('Ctrl Pts',(0.00620485947668039,-0.0346444289841739,
0.0687282050381468));
#78059=CARTESIAN_POINT('Ctrl Pts',(0.00637889368574284,-0.0352450361874068,
0.0686697181552573));
#78060=CARTESIAN_POINT('Ctrl Pts',(0.00617220146430665,-0.0349452760959493,
0.0687355277051972));
#78061=CARTESIAN_POINT('Ctrl Pts',(0.00597105347828606,-0.0346444289841739,
0.0688167192009672));
#78062=CARTESIAN_POINT('',(0.00634456095533437,-0.0351951633467146,0.0686807659675127));
#78063=CARTESIAN_POINT('',(0.00612133224107484,-0.0348678972925388,0.0687584956468902));
#78064=CARTESIAN_POINT('Origin',(0.0123492203897781,-0.0345631633298062,
0.0843130374478586));
#78065=CARTESIAN_POINT('Origin',(0.00227410942706091,-0.0346946199341028,
0.0584000273317687));
#78066=CARTESIAN_POINT('',(0.00623898419006084,-0.0346945769330288,0.0687162479366787));
#78067=CARTESIAN_POINT('',(0.00618039471635125,-0.0346945769458128,0.068738008558407));
#78068=CARTESIAN_POINT('',(0.00646381897803458,-0.0350221583435275,0.0686433996763336));
#78069=CARTESIAN_POINT('Origin',(0.0119137981656891,-0.0345628458714449,
0.0845184013684698));
#78070=CARTESIAN_POINT('',(0.00646417886482151,-0.035195136029876,0.0686445830504279));
#78071=CARTESIAN_POINT('Origin',(0.00328386838325173,-0.035195183836688,
0.0580945371203709));
#78072=CARTESIAN_POINT('',(0.00634453065880707,-0.035195137132875,0.0686807780281208));
#78073=CARTESIAN_POINT('Ctrl Pts',(0.00661855746883567,-0.0350241211494342,
0.0683418765053196));
#78074=CARTESIAN_POINT('Ctrl Pts',(0.00653855294911979,-0.0349144232818961,
0.0683626103587302));
#78075=CARTESIAN_POINT('Ctrl Pts',(0.00645892912640817,-0.0348045283579412,
0.0683850103729423));
#78076=CARTESIAN_POINT('Ctrl Pts',(0.00637978905638008,-0.0346945769439157,
0.068409051651594));
#78077=CARTESIAN_POINT('Ctrl Pts',(0.00656712356767582,-0.0350241211494342,
0.0684428502425703));
#78078=CARTESIAN_POINT('Ctrl Pts',(0.00648850991978973,-0.0349144232818961,
0.0684642925768807));
#78079=CARTESIAN_POINT('Ctrl Pts',(0.00641029244621817,-0.0348045283579412,
0.0684873727457379));
#78080=CARTESIAN_POINT('Ctrl Pts',(0.00633257243370495,-0.0346945769439157,
0.0685120649145559));
#78081=CARTESIAN_POINT('Ctrl Pts',(0.00651568966651597,-0.0350241211494342,
0.068543823979821));
#78082=CARTESIAN_POINT('Ctrl Pts',(0.00643846689045967,-0.0349144232818961,
0.0685659747950312));
#78083=CARTESIAN_POINT('Ctrl Pts',(0.00636165576602818,-0.0348045283579412,
0.0685897351185336));
#78084=CARTESIAN_POINT('Ctrl Pts',(0.00628535581102983,-0.0346945769439157,
0.0686150781775178));
#78085=CARTESIAN_POINT('Ctrl Pts',(0.00646425576535612,-0.0350241211494342,
0.0686447977170718));
#78086=CARTESIAN_POINT('Ctrl Pts',(0.0063884238611296,-0.0349144232818961,
0.0686676570131817));
#78087=CARTESIAN_POINT('Ctrl Pts',(0.00631301908583818,-0.0348045283579412,
0.0686920974913292));
#78088=CARTESIAN_POINT('Ctrl Pts',(0.0062381391883547,-0.0346945769439157,
0.0687180914404797));
#78089=CARTESIAN_POINT('',(0.00630938662879126,-0.0346945769458128,0.0685626497923518));
#78090=CARTESIAN_POINT('Ctrl Pts',(0.00639205581553391,-0.0347116136492808,
0.0684053395493713));
#78091=CARTESIAN_POINT('Ctrl Pts',(0.0064044495286139,-0.0347621546532085,
0.0684464532462514));
#78092=CARTESIAN_POINT('Ctrl Pts',(0.00641662532672676,-0.0348133084096574,
0.0684868440532401));
#78093=CARTESIAN_POINT('Ctrl Pts',(0.00644055125457274,-0.0349168561544573,
0.0685662135963857));
#78094=CARTESIAN_POINT('Ctrl Pts',(0.00645229189408879,-0.0349692089015913,
0.0686051608506207));
#78095=CARTESIAN_POINT('Ctrl Pts',(0.00646381897802599,-0.0350221583434999,
0.0686433996763744));
#78096=CARTESIAN_POINT('Ctrl Pts',(0.00634581971921704,-0.0351951371254913,
0.068681469932819));
#78097=CARTESIAN_POINT('Ctrl Pts',(0.00627050925695388,-0.0350856248736006,
0.068705955338248));
#78098=CARTESIAN_POINT('Ctrl Pts',(0.00619564299169479,-0.0349758427080694,
0.068732017228011));
#78099=CARTESIAN_POINT('Ctrl Pts',(0.0061213187293352,-0.034865930689779,
0.0687596278671616));
#78100=CARTESIAN_POINT('Ctrl Pts',(0.00627337379092395,-0.0351951371254913,
0.0686425847412442));
#78101=CARTESIAN_POINT('Ctrl Pts',(0.00619752781697544,-0.0350856248736006,
0.0686680678437292));
#78102=CARTESIAN_POINT('Ctrl Pts',(0.00612214621905836,-0.0349758427080694,
0.0686951393165914));
#78103=CARTESIAN_POINT('Ctrl Pts',(0.00604732753873635,-0.034865930689779,
0.0687237701711421));
#78104=CARTESIAN_POINT('Ctrl Pts',(0.00620092786263085,-0.0351951371254913,
0.0686036995496694));
#78105=CARTESIAN_POINT('Ctrl Pts',(0.00612454637699699,-0.0350856248736006,
0.0686301803492104));
#78106=CARTESIAN_POINT('Ctrl Pts',(0.00604864944642193,-0.0349758427080694,
0.0686582614051718));
#78107=CARTESIAN_POINT('Ctrl Pts',(0.00597333634813751,-0.034865930689779,
0.0686879124751227));
#78108=CARTESIAN_POINT('Ctrl Pts',(0.00612848193433776,-0.0351951371254913,
0.0685648143580946));
#78109=CARTESIAN_POINT('Ctrl Pts',(0.00605156493701854,-0.0350856248736006,
0.0685922928546916));
#78110=CARTESIAN_POINT('Ctrl Pts',(0.0059751526737855,-0.0349758427080694,
0.0686213834937522));
#78111=CARTESIAN_POINT('Ctrl Pts',(0.00589934515753867,-0.034865930689779,
0.0686520547791032));
#78112=CARTESIAN_POINT('Origin',(0.00426970141720928,-0.0308609197410927,
0.0637730648563144));
#78113=CARTESIAN_POINT('',(0.00625033828332303,-0.0351951371254913,0.0686302204835531));
#78114=CARTESIAN_POINT('Origin',(0.00859310768890597,-0.0351840467441098,
0.0750070176365937));
#78115=CARTESIAN_POINT('Origin',(0.00322208857129343,-0.0352322615287784,
0.0632348972788652));
#78116=CARTESIAN_POINT('',(0.00590123553039178,-0.0351951142564656,0.0688454641187499));
#78117=CARTESIAN_POINT('',(0.00578730024265978,-0.0351951372916786,0.0688961107648497));
#78118=CARTESIAN_POINT('Origin',(0.00793123669642114,-0.0352875104107299,
0.0744308068679663));
#78119=CARTESIAN_POINT('Origin',(0.0154363415296375,-0.0298325076521851,
0.0724702183975427));
#78120=CARTESIAN_POINT('Origin',(0.00785119176127153,-0.0338732556787189,
0.0657729478221477));
#78121=CARTESIAN_POINT('Ctrl Pts',(0.0094439865715157,-0.0321934096636941,
0.068552215068034));
#78122=CARTESIAN_POINT('Ctrl Pts',(0.00934378888693288,-0.0320508460844246,
0.0685285840383499));
#78123=CARTESIAN_POINT('Ctrl Pts',(0.00924303183259509,-0.0319086045662913,
0.0685076629406188));
#78124=CARTESIAN_POINT('Ctrl Pts',(0.00914193606469694,-0.0317669892867664,
0.0684894789611682));
#78125=CARTESIAN_POINT('Ctrl Pts',(0.00936197865582068,-0.0321934096636941,
0.0685347469716528));
#78126=CARTESIAN_POINT('Ctrl Pts',(0.00926146830063105,-0.0320508460844246,
0.0685125838446069));
#78127=CARTESIAN_POINT('Ctrl Pts',(0.00916043825108861,-0.0319086045662913,
0.068493137943553));
#78128=CARTESIAN_POINT('Ctrl Pts',(0.00905910948969717,-0.0317669892867664,
0.0684764332300684));
#78129=CARTESIAN_POINT('Ctrl Pts',(0.00927997074012567,-0.0321934096636941,
0.0685172788752715));
#78130=CARTESIAN_POINT('Ctrl Pts',(0.00917914771432923,-0.0320508460844246,
0.0684965836508641));
#78131=CARTESIAN_POINT('Ctrl Pts',(0.00907784466958213,-0.0319086045662913,
0.0684786129464871));
#78132=CARTESIAN_POINT('Ctrl Pts',(0.00897628291469741,-0.0317669892867664,
0.0684633874989687));
#78133=CARTESIAN_POINT('Ctrl Pts',(0.00919796282443065,-0.0321934096636941,
0.0684998107788903));
#78134=CARTESIAN_POINT('Ctrl Pts',(0.00909682712802741,-0.0320508460844246,
0.0684805834571211));
#78135=CARTESIAN_POINT('Ctrl Pts',(0.00899525108807564,-0.0319086045662913,
0.0684640879494213));
#78136=CARTESIAN_POINT('Ctrl Pts',(0.00889345633969765,-0.0317669892867663,
0.0684503417678689));
#78137=CARTESIAN_POINT('',(0.00919942996224764,-0.0321934096636941,0.0685001232865888));
#78138=CARTESIAN_POINT('',(0.00896639895460232,-0.0318665617511278,0.06846070109923));
#78139=CARTESIAN_POINT('Origin',(0.00547230549469594,-0.032637194442216,
0.0847889675687293));
#78140=CARTESIAN_POINT('Origin',(0.0105722941342516,-0.0316939261508945,
0.0576177913948755));
#78141=CARTESIAN_POINT('',(0.00932170218911971,-0.0320197221621871,0.0685248265049253));
#78142=CARTESIAN_POINT('Ctrl Pts',(0.0093215370854431,-0.0320197392094776,
0.0685247431043587));
#78143=CARTESIAN_POINT('Ctrl Pts',(0.0092929139601089,-0.0319792716576074,
0.0685186485883089));
#78144=CARTESIAN_POINT('Ctrl Pts',(0.00926411406927588,-0.031938643982974,
0.0685127445388893));
#78145=CARTESIAN_POINT('Ctrl Pts',(0.00923510548001692,-0.0318979099381672,
0.0685070330431788));
#78146=CARTESIAN_POINT('Ctrl Pts',(0.00920609746413207,-0.0318571766984959,
0.0685013216603598));
#78147=CARTESIAN_POINT('Ctrl Pts',(0.00917702853994146,-0.0318163871833594,
0.0684958301044913));
#78148=CARTESIAN_POINT('Ctrl Pts',(0.00914799934620503,-0.0317755399638303,
0.0684905738043085));
#78149=CARTESIAN_POINT('',(0.00932168725141204,-0.0321934096636183,0.06852616470091));
#78150=CARTESIAN_POINT('Origin',(0.00978186381970738,-0.0324111717947839,
0.0662648353462695));
#78151=CARTESIAN_POINT('',(0.00926055860683984,-0.0321934096636663,0.0685131439937594));
#78152=CARTESIAN_POINT('Ctrl Pts',(0.00920053388169604,-0.0321934096636617,
0.0685018247710085));
#78153=CARTESIAN_POINT('Ctrl Pts',(0.00912264114335793,-0.0320835708272592,
0.0684869755260517));
#78154=CARTESIAN_POINT('Ctrl Pts',(0.009044486281621,-0.0319739230346488,
0.068473746880432));
#78155=CARTESIAN_POINT('Ctrl Pts',(0.00896617058916533,-0.0318646057455573,
0.0684621480850449));
#78156=CARTESIAN_POINT('Ctrl Pts',(0.00913885678371131,-0.0321934096636617,
0.0684067611062953));
#78157=CARTESIAN_POINT('Ctrl Pts',(0.00905965304334853,-0.0320835708272592,
0.068392762436588));
#78158=CARTESIAN_POINT('Ctrl Pts',(0.00898020554263194,-0.0319739230346488,
0.0683804110039684));
#78159=CARTESIAN_POINT('Ctrl Pts',(0.00890061714194762,-0.0318646057455573,
0.068369714810071));
#78160=CARTESIAN_POINT('Ctrl Pts',(0.00907717968572658,-0.0321934096636617,
0.068311697441582));
#78161=CARTESIAN_POINT('Ctrl Pts',(0.00899666494333912,-0.0320835708272592,
0.0682985493471242));
#78162=CARTESIAN_POINT('Ctrl Pts',(0.00891592480364289,-0.0319739230346488,
0.0682870751275048));
#78163=CARTESIAN_POINT('Ctrl Pts',(0.00883506369472991,-0.0318646057455573,
0.0682772815350971));
#78164=CARTESIAN_POINT('Ctrl Pts',(0.00901550258774186,-0.0321934096636617,
0.0682166337768687));
#78165=CARTESIAN_POINT('Ctrl Pts',(0.00893367684332971,-0.0320835708272592,
0.0682043362576605));
#78166=CARTESIAN_POINT('Ctrl Pts',(0.00885164406465383,-0.0319739230346488,
0.0681937392510411));
#78167=CARTESIAN_POINT('Ctrl Pts',(0.0087695102475122,-0.0318646057455573,
0.0681848482601232));
#78168=CARTESIAN_POINT('',(0.00900282677662865,-0.0321763980308457,0.0682147425836894));
#78169=CARTESIAN_POINT('',(0.00901550258770958,-0.0321934096636184,0.0682166337768639));
#78170=CARTESIAN_POINT('Origin',(0.00597325106342534,-0.0326386231399442,
0.0844827409580259));
#78171=CARTESIAN_POINT('Ctrl Pts',(0.00900282677615878,-0.0321763980306278,
0.0682147425868238));
#78172=CARTESIAN_POINT('Ctrl Pts',(0.00899653883936201,-0.0321259596174822,
0.0682571983668901));
#78173=CARTESIAN_POINT('Ctrl Pts',(0.00899035984923604,-0.032074916463138,
0.0682989185454781));
#78174=CARTESIAN_POINT('Ctrl Pts',(0.00897821478964855,-0.0319716057793914,
0.0683809212747366));
#78175=CARTESIAN_POINT('Ctrl Pts',(0.00897225345231002,-0.0319193786690108,
0.0684211718743905));
#78176=CARTESIAN_POINT('Ctrl Pts',(0.00896639895432312,-0.0318665617525293,
0.0684607011010613));
#78177=CARTESIAN_POINT('',(0.00910746627498862,-0.0321934096636663,0.0683583785317363));
#78178=CARTESIAN_POINT('Origin',(0.00812378219310841,-0.0315241814719618,
0.07415));
#78179=CARTESIAN_POINT('',(0.00900282677668285,-0.0322104233323627,0.0682147425833225));
#78180=CARTESIAN_POINT('',(0.00899014695537404,-0.0321934096636183,0.0682128784669062));
#78181=CARTESIAN_POINT('Origin',(0.00601673289315573,-0.0326387236839092,
0.0844955662196018));
#78182=CARTESIAN_POINT('Origin',(0.00718701739197183,-0.0326386240897199,
0.0846625085056469));
#78183=CARTESIAN_POINT('Origin',(0.00714168519673485,-0.0326387244881,0.0846621754870935));
#78184=CARTESIAN_POINT('Ctrl Pts',(0.00912546258677331,-0.0327445246967097,
0.0684865415699463));
#78185=CARTESIAN_POINT('Ctrl Pts',(0.00891186176018342,-0.032443687833936,
0.0684487625762962));
#78186=CARTESIAN_POINT('Ctrl Pts',(0.00869602208277616,-0.0321434074405928,
0.0684271801960333));
#78187=CARTESIAN_POINT('Ctrl Pts',(0.0088783952573674,-0.0327445246967097,
0.0684483612773827));
#78188=CARTESIAN_POINT('Ctrl Pts',(0.00866335443750278,-0.032443687833936,
0.0684199005803948));
#78189=CARTESIAN_POINT('Ctrl Pts',(0.00844678074987853,-0.0321434074405928,
0.068407718490676));
#78190=CARTESIAN_POINT('',(0.00884254872302497,-0.0326943950436612,0.068443731545443));
#78191=CARTESIAN_POINT('',(0.00860750220923627,-0.0323666188837389,0.0684190192858466));
#78192=CARTESIAN_POINT('Origin',(0.00681706364081476,-0.0326395579111504,
0.0851322146524214));
#78193=CARTESIAN_POINT('Origin',(0.00953641204844979,-0.0321933825603182,
0.057413543452628));
#78194=CARTESIAN_POINT('',(0.00873194506416534,-0.0321934096532689,0.0684308861771334));
#78195=CARTESIAN_POINT('',(0.00866966650717283,-0.0321934096584275,0.0684256295922533));
#78196=CARTESIAN_POINT('',(0.00896639895473841,-0.0325210109756238,0.068460701098288));
#78197=CARTESIAN_POINT('Origin',(0.00634385287505525,-0.0326393129158472,
0.0850470324884165));
#78198=CARTESIAN_POINT('',(0.00896619991923769,-0.0326943950436593,0.0684620449742721));
#78199=CARTESIAN_POINT('Origin',(0.01058693251845,-0.0326943765538216,0.0575189584561217));
#78200=CARTESIAN_POINT('',(0.00890437432114132,-0.0326943950436702,0.0684528882598675));
#78201=CARTESIAN_POINT('Ctrl Pts',(0.00923479393888999,-0.0325229783203769,
0.0682537594264856));
#78202=CARTESIAN_POINT('Ctrl Pts',(0.00915351439152637,-0.032413025309245,
0.0682384441538662));
#78203=CARTESIAN_POINT('Ctrl Pts',(0.00907193035571066,-0.032303122220807,
0.0682248125759562));
#78204=CARTESIAN_POINT('Ctrl Pts',(0.00899014695093679,-0.0321934096576658,
0.0682128784662587));
#78205=CARTESIAN_POINT('Ctrl Pts',(0.0091452626130476,-0.0325229783203769,
0.0683232236901697));
#78206=CARTESIAN_POINT('Ctrl Pts',(0.00906494062903978,-0.032413025309245,
0.0683091426049192));
#78207=CARTESIAN_POINT('Ctrl Pts',(0.00898433954209778,-0.032303122220807,
0.0682967252187612));
#78208=CARTESIAN_POINT('Ctrl Pts',(0.00890356315774672,-0.0321934096576658,
0.0682859837943346));
#78209=CARTESIAN_POINT('Ctrl Pts',(0.00905573128720521,-0.0325229783203769,
0.0683926879538539));
#78210=CARTESIAN_POINT('Ctrl Pts',(0.00897636686655319,-0.032413025309245,
0.0683798410559721));
#78211=CARTESIAN_POINT('Ctrl Pts',(0.0088967487284849,-0.032303122220807,
0.0683686378615661));
#78212=CARTESIAN_POINT('Ctrl Pts',(0.00881697936455664,-0.0321934096576658,
0.0683590891224106));
#78213=CARTESIAN_POINT('Ctrl Pts',(0.00896619996136282,-0.0325229783203769,
0.068462152217538));
#78214=CARTESIAN_POINT('Ctrl Pts',(0.0088877931040666,-0.032413025309245,
0.0684505395070251));
#78215=CARTESIAN_POINT('Ctrl Pts',(0.00880915791487202,-0.032303122220807,
0.0684405505043711));
#78216=CARTESIAN_POINT('Ctrl Pts',(0.00873039557136657,-0.0321934096576658,
0.0684321944504865));
#78217=CARTESIAN_POINT('',(0.00886104601027864,-0.0321934096584275,0.0683218823219358));
#78218=CARTESIAN_POINT('Ctrl Pts',(0.00900282677616828,-0.0322104233328946,
0.0682147425867594));
#78219=CARTESIAN_POINT('Ctrl Pts',(0.00899653031911972,-0.0322609421831059,
0.0682572558950655));
#78220=CARTESIAN_POINT('Ctrl Pts',(0.00899034716670475,-0.0323120888240066,
0.0682990041771383));
#78221=CARTESIAN_POINT('Ctrl Pts',(0.00897820201515553,-0.0324156524631819,
0.0683810075273171));
#78222=CARTESIAN_POINT('Ctrl Pts',(0.00897224500832695,-0.0324680267167319,
0.0684212288876685));
#78223=CARTESIAN_POINT('Ctrl Pts',(0.00896639895472762,-0.0325210109755912,
0.0684607010983302));
#78224=CARTESIAN_POINT('Origin',(0.0157112785443541,-0.0262834582511764,
0.0762316543803413));
#78225=CARTESIAN_POINT('Origin',(0.0150973441873914,-0.0342770700395395,
0.0641904785327736));
#78226=CARTESIAN_POINT('Ctrl Pts',(0.00884375700785978,-0.0326943950436604,
0.0684453599614188));
#78227=CARTESIAN_POINT('Ctrl Pts',(0.0087651363764932,-0.0325844576448134,
0.0684354373590949));
#78228=CARTESIAN_POINT('Ctrl Pts',(0.00868630496533801,-0.0324744968375323,
0.06842714005809));
#78229=CARTESIAN_POINT('Ctrl Pts',(0.00860736392442869,-0.0323646534831895,
0.0684204772962495));
#78230=CARTESIAN_POINT('Ctrl Pts',(0.00877623261640564,-0.0326943950436604,
0.0683543567519142));
#78231=CARTESIAN_POINT('Ctrl Pts',(0.00869635779025389,-0.0325844576448134,
0.0683453647622587));
#78232=CARTESIAN_POINT('Ctrl Pts',(0.00861629134214797,-0.0324744968375323,
0.0683380240785876));
#78233=CARTESIAN_POINT('Ctrl Pts',(0.00853613598761797,-0.0323646534831895,
0.0683323426912462));
#78234=CARTESIAN_POINT('Ctrl Pts',(0.00870870822495149,-0.0326943950436604,
0.0682633535424095));
#78235=CARTESIAN_POINT('Ctrl Pts',(0.00862757920401458,-0.0325844576448134,
0.0682552921654225));
#78236=CARTESIAN_POINT('Ctrl Pts',(0.00854627771895792,-0.0324744968375323,
0.0682489080990851));
#78237=CARTESIAN_POINT('Ctrl Pts',(0.00846490805080725,-0.0323646534831895,
0.0682442080862429));
#78238=CARTESIAN_POINT('Ctrl Pts',(0.00864118383349735,-0.0326943950436604,
0.0681723503329048));
#78239=CARTESIAN_POINT('Ctrl Pts',(0.00855880061777527,-0.0325844576448134,
0.0681652195685863));
#78240=CARTESIAN_POINT('Ctrl Pts',(0.00847626409576787,-0.0324744968375323,
0.0681597921195827));
#78241=CARTESIAN_POINT('Ctrl Pts',(0.00839368011399654,-0.0323646534831895,
0.0681560734812396));
#78242=CARTESIAN_POINT('',(0.00862841428624813,-0.032677355999116,0.0681712587921285));
#78243=CARTESIAN_POINT('',(0.00864118383349658,-0.0326943950436595,0.0681723503329048));
#78244=CARTESIAN_POINT('Origin',(0.00728189562577048,-0.0326395670678001,
0.0847217934799203));
#78245=CARTESIAN_POINT('Ctrl Pts',(0.00862841428596128,-0.032677355998742,
0.0681712587954638));
#78246=CARTESIAN_POINT('Ctrl Pts',(0.00862480167261006,-0.032626792258595,
0.0682140600374077));
#78247=CARTESIAN_POINT('Ctrl Pts',(0.00862125309022181,-0.0325756109579303,
0.0682561026582453));
#78248=CARTESIAN_POINT('Ctrl Pts',(0.00861428096735214,-0.0324719985462367,
0.0683387064380571));
#78249=CARTESIAN_POINT('Ctrl Pts',(0.00861086022319848,-0.032419609162177,
0.0683792344669148));
#78250=CARTESIAN_POINT('Ctrl Pts',(0.00860750220923214,-0.0323666188837756,
0.0684190192858952));
#78251=CARTESIAN_POINT('',(0.00874186627827078,-0.0326943950436703,0.0683080409391839));
#78252=CARTESIAN_POINT('Origin',(0.00812378219310841,-0.0315241814719618,
0.07415));
#78253=CARTESIAN_POINT('',(0.00862841428624429,-0.0327114338379885,0.068171258792173));
#78254=CARTESIAN_POINT('',(0.00861564243684584,-0.0326943950436593,0.0681701945265212));
#78255=CARTESIAN_POINT('Origin',(0.00732710419379926,-0.0326395671577066,
0.0847248312028982));
#78256=CARTESIAN_POINT('Origin',(0.00718177098644518,-0.0326395677642361,
0.0847133440405204));
#78257=CARTESIAN_POINT('Origin',(0.00713669334567575,-0.0326395680194222,
0.0847087577456239));
#78258=CARTESIAN_POINT('Ctrl Pts',(0.00876783552519102,-0.0332451089994433,
0.0684348166866291));
#78259=CARTESIAN_POINT('Ctrl Pts',(0.00855228385991727,-0.0329451141710254,
0.0684105258177901));
#78260=CARTESIAN_POINT('Ctrl Pts',(0.00833551486663236,-0.0326442513127494,
0.0684025401893565));
#78261=CARTESIAN_POINT('Ctrl Pts',(0.00851885821225085,-0.0332451089994433,
0.0684122269181242));
#78262=CARTESIAN_POINT('Ctrl Pts',(0.0083024545599187,-0.0329451141710254,
0.0683973263822767));
#78263=CARTESIAN_POINT('Ctrl Pts',(0.0080855433182496,-0.0326442513127494,
0.0683987685850377));
#78264=CARTESIAN_POINT('Ctrl Pts',(0.00851636843912145,-0.0332451089994433,
0.0684120010204392));
#78265=CARTESIAN_POINT('Ctrl Pts',(0.00829995626691872,-0.0329451141710254,
0.0683971943879216));
#78266=CARTESIAN_POINT('Ctrl Pts',(0.00808304360276577,-0.0326442513127494,
0.0683987308689945));
#78267=CARTESIAN_POINT('',(0.00848283084062868,-0.0331951640388616,0.0684098598389312));
#78268=CARTESIAN_POINT('',(0.00824669642355681,-0.0328677532457581,0.0683999550269371));
#78269=CARTESIAN_POINT('Origin',(0.00820381225447208,-0.0326403163409033,
0.0851715565180648));
#78270=CARTESIAN_POINT('Origin',(0.00848245237122557,-0.0326944278639109,
0.0573464992760607));
#78271=CARTESIAN_POINT('',(0.00837163885895575,-0.0326943950436593,0.0684039846786494));
#78272=CARTESIAN_POINT('',(0.00830915313354108,-0.0326943950436694,0.0684026489698008));
#78273=CARTESIAN_POINT('',(0.00860750220923909,-0.0330220786163545,0.0684190192858468));
#78274=CARTESIAN_POINT('Origin',(0.00772354399028894,-0.0326396682763611,
0.0851927127086911));
#78275=CARTESIAN_POINT('',(0.00860738794916238,-0.0331951640388587,0.0684203730075413));
#78276=CARTESIAN_POINT('Origin',(0.00953520974333515,-0.0331952026559975,
0.0574278065989809));
#78277=CARTESIAN_POINT('',(0.00854510939490553,-0.0331951640388701,0.0684151164232462));
#78278=CARTESIAN_POINT('Ctrl Pts',(0.00886237264853371,-0.0330240426238172,
0.0681956331873849));
#78279=CARTESIAN_POINT('Ctrl Pts',(0.00878034544463144,-0.0329142774063519,
0.0681854583842876));
#78280=CARTESIAN_POINT('Ctrl Pts',(0.00869806700557452,-0.0328043479726691,
0.0681769742401163));
#78281=CARTESIAN_POINT('Ctrl Pts',(0.00861564243684584,-0.0326943950436593,
0.0681701945265212));
#78282=CARTESIAN_POINT('Ctrl Pts',(0.00877737972220961,-0.0330240426238172,
0.0682705820930427));
#78283=CARTESIAN_POINT('Ctrl Pts',(0.00869638501250196,-0.0329142774063519,
0.0682615781503101));
#78284=CARTESIAN_POINT('Ctrl Pts',(0.00861516378733005,-0.0328043479726691,
0.068254244105681));
#78285=CARTESIAN_POINT('Ctrl Pts',(0.00853381983838319,-0.0326943950436593,
0.0682485922201432));
#78286=CARTESIAN_POINT('Ctrl Pts',(0.00869238679588551,-0.0330240426238172,
0.0683455309987005));
#78287=CARTESIAN_POINT('Ctrl Pts',(0.00861242458037248,-0.0329142774063519,
0.0683376979163326));
#78288=CARTESIAN_POINT('Ctrl Pts',(0.00853226056908557,-0.0328043479726691,
0.0683315139712456));
#78289=CARTESIAN_POINT('Ctrl Pts',(0.00845199723992054,-0.0326943950436593,
0.0683269899137652));
#78290=CARTESIAN_POINT('Ctrl Pts',(0.00860739386956141,-0.0330240426238172,
0.0684204799043583));
#78291=CARTESIAN_POINT('Ctrl Pts',(0.00852846414824299,-0.0329142774063519,
0.0684138176823551));
#78292=CARTESIAN_POINT('Ctrl Pts',(0.00844935735084109,-0.0328043479726691,
0.0684087838368103));
#78293=CARTESIAN_POINT('Ctrl Pts',(0.00837017464145789,-0.0326943950436593,
0.0684053876073873));
#78294=CARTESIAN_POINT('',(0.0084936406479108,-0.0326943950436694,0.0682870896025953));
#78295=CARTESIAN_POINT('Ctrl Pts',(0.00862841428596059,-0.0327114338383342,
0.0681712587954722));
#78296=CARTESIAN_POINT('Ctrl Pts',(0.008624802273507,-0.0327619876830778,
0.0682140529181476));
#78297=CARTESIAN_POINT('Ctrl Pts',(0.00862125398462585,-0.0328131562603919,
0.0682560920615946));
#78298=CARTESIAN_POINT('Ctrl Pts',(0.0086142818681561,-0.0329167375858774,
0.0683386957655818));
#78299=CARTESIAN_POINT('Ctrl Pts',(0.0086108608186221,-0.0329691088920621,
0.0683792274125011));
#78300=CARTESIAN_POINT('Ctrl Pts',(0.0086075022092323,-0.0330220786163186,
0.068419019285894));
#78301=CARTESIAN_POINT('Ctrl Pts',(0.00848413919911251,-0.0331951640388604,
0.068411409420108));
#78302=CARTESIAN_POINT('Ctrl Pts',(0.00836549752124305,-0.0330306422053994,
0.0684039592702446));
#78303=CARTESIAN_POINT('Ctrl Pts',(0.00824664929933022,-0.0328657862001532,
0.0684014190716655));
#78304=CARTESIAN_POINT('Ctrl Pts',(0.00848283084063181,-0.0331951640388604,
0.0684098598389315));
#78305=CARTESIAN_POINT('Ctrl Pts',(0.00836415712616587,-0.0330306422053994,
0.0684024367385402));
#78306=CARTESIAN_POINT('Ctrl Pts',(0.0082452780130147,-0.0328657862001532,
0.0683999248904258));
#78307=CARTESIAN_POINT('Ctrl Pts',(0.00826482313138845,-0.0331951640388604,
0.0681516579412534));
#78308=CARTESIAN_POINT('Ctrl Pts',(0.00814081125837241,-0.0330306422053994,
0.0681487420103583));
#78309=CARTESIAN_POINT('Ctrl Pts',(0.00801678483414019,-0.0328657862001532,
0.0681509541120963));
#78310=CARTESIAN_POINT('',(0.00825201024418503,-0.0331781648281895,0.0681513703595991));
#78311=CARTESIAN_POINT('',(0.00826482313138731,-0.0331951640388588,0.0681516579412533));
#78312=CARTESIAN_POINT('Origin',(0.00861133834247988,-0.0326412092360721,
0.0846697652686003));
#78313=CARTESIAN_POINT('Ctrl Pts',(0.00825201024566016,-0.033178164828644,
0.0681513703606867));
#78314=CARTESIAN_POINT('Ctrl Pts',(0.00825109165333182,-0.0331276811560401,
0.0681943435460393));
#78315=CARTESIAN_POINT('Ctrl Pts',(0.00825018968174488,-0.0330765663525361,
0.0682365407694903));
#78316=CARTESIAN_POINT('Ctrl Pts',(0.00824841804298898,-0.0329730614519476,
0.068319419543932));
#78317=CARTESIAN_POINT('Ctrl Pts',(0.00824754908615228,-0.0329207133437511,
0.0683600676141577));
#78318=CARTESIAN_POINT('Ctrl Pts',(0.00824669644230155,-0.0328677532367531,
0.0683999550153815));
#78319=CARTESIAN_POINT('',(0.00837382698601799,-0.0331951640388701,0.0682807588901023));
#78320=CARTESIAN_POINT('Origin',(0.00812378219310841,-0.0315241814719618,
0.07415));
#78321=CARTESIAN_POINT('',(0.00825201024350532,-0.033212160714424,0.0681513703611358));
#78322=CARTESIAN_POINT('',(0.00823919677064574,-0.0331951640388587,0.0681511101464263));
#78323=CARTESIAN_POINT('Origin',(0.00865615796368383,-0.0326413654336508,
0.0846628791406934));
#78324=CARTESIAN_POINT('Origin',(0.0071871319098763,-0.0326412098688358,
0.0846393229117763));
#78325=CARTESIAN_POINT('Origin',(0.00714264784117156,-0.0326413662714906,
0.0846305242971188));
#78326=CARTESIAN_POINT('Ctrl Pts',(0.00840772610977036,-0.0337436976235975,
0.0684056548804768));
#78327=CARTESIAN_POINT('Ctrl Pts',(0.00835606059918607,-0.0336723290703325,
0.0684031010458575));
#78328=CARTESIAN_POINT('Ctrl Pts',(0.00830435751142873,-0.033601104548885,
0.0684014769240775));
#78329=CARTESIAN_POINT('Ctrl Pts',(0.00813927979402415,-0.0333736987606857,
0.0683962914249547));
#78330=CARTESIAN_POINT('Ctrl Pts',(0.00797417653779931,-0.0331450831799192,
0.0684005875823786));
#78331=CARTESIAN_POINT('Ctrl Pts',(0.00815782169841966,-0.0337436976235975,
0.0683987421973904));
#78332=CARTESIAN_POINT('Ctrl Pts',(0.00810609401411603,-0.0336723290703325,
0.0683984360409208));
#78333=CARTESIAN_POINT('Ctrl Pts',(0.008054369191343,-0.033601104548885,
0.0683990603519785));
#78334=CARTESIAN_POINT('Ctrl Pts',(0.00788922207833876,-0.0333736987606857,
0.0684010536535167));
#78335=CARTESIAN_POINT('Ctrl Pts',(0.00772446150184724,-0.0331450831799192,
0.0684125207638257));
#78336=CARTESIAN_POINT('Ctrl Pts',(0.00815532265430615,-0.0337436976235975,
0.0683986730705595));
#78337=CARTESIAN_POINT('Ctrl Pts',(0.00810359434826533,-0.0336723290703325,
0.0683983893908714));
#78338=CARTESIAN_POINT('Ctrl Pts',(0.00805186930814214,-0.033601104548885,
0.0683990361862575));
#78339=CARTESIAN_POINT('Ctrl Pts',(0.0078867215011819,-0.0333736987606857,
0.0684011012758023));
#78340=CARTESIAN_POINT('Ctrl Pts',(0.00772196435148772,-0.0331450831799192,
0.0684126400956403));
#78341=CARTESIAN_POINT('',(0.00812169595724109,-0.0336938721132548,0.0683986418432147));
#78342=CARTESIAN_POINT('',(0.00788540557795273,-0.0333679869984219,0.068403583587206));
#78343=CARTESIAN_POINT('Ctrl Pts',(0.00812169595725132,-0.0336938721132646,
0.0683986418432142));
#78344=CARTESIAN_POINT('Ctrl Pts',(0.00809924570835516,-0.033662918793393,
0.0683986499867719));
#78345=CARTESIAN_POINT('Ctrl Pts',(0.00807680268726717,-0.0336319952301037,
0.0683987895829587));
#78346=CARTESIAN_POINT('Ctrl Pts',(0.0080543691913531,-0.0336011045488947,
0.0683990603519784));
#78347=CARTESIAN_POINT('Ctrl Pts',(0.00799807587379437,-0.0335235892595451,
0.068399739804101));
#78348=CARTESIAN_POINT('Ctrl Pts',(0.00794174250742213,-0.0334458668673266,
0.0684012465815856));
#78349=CARTESIAN_POINT('Ctrl Pts',(0.00788540557794386,-0.0333679869984148,
0.0684035835867571));
#78350=CARTESIAN_POINT('Ctrl Pts',(0.00788536112028597,-0.0333679692463166,
0.0684035847431947));
#78351=CARTESIAN_POINT('Ctrl Pts',(0.00788538582701036,-0.0333391895391197,
0.0684040373217868));
#78352=CARTESIAN_POINT('Ctrl Pts',(0.00788540758825821,-0.0333104081089681,
0.0684043763745313));
#78353=CARTESIAN_POINT('Ctrl Pts',(0.00788544192004787,-0.0332532698661692,
0.0684048248137598));
#78354=CARTESIAN_POINT('Ctrl Pts',(0.00788545462428967,-0.0332249173360562,
0.0684049375528162));
#78355=CARTESIAN_POINT('Ctrl Pts',(0.00788546167119418,-0.0331960985279258,
0.0684049409340705));
#78356=CARTESIAN_POINT('Ctrl Pts',(0.00788546178409538,-0.0331956312646462,
0.0684049409591678));
#78357=CARTESIAN_POINT('Ctrl Pts',(0.00788546189524772,-0.0331951640388588,
0.0684049409545569));
#78358=CARTESIAN_POINT('',(0.00801035448319217,-0.0331951640388587,0.0683997600785164));
#78359=CARTESIAN_POINT('',(0.00794790818922994,-0.0331951640388687,0.0684023505165466));
#78360=CARTESIAN_POINT('',(0.00824669644198909,-0.0335216366567736,0.0683999550364575));
#78361=CARTESIAN_POINT('Origin',(0.00910239711679951,-0.0326434571526194,
0.0850324064906018));
#78362=CARTESIAN_POINT('',(0.00824666740810635,-0.0336938721132327,0.0684013132609321));
#78363=CARTESIAN_POINT('Origin',(0.00848005542000744,-0.0336938867896227,
0.0574832383406437));
#78364=CARTESIAN_POINT('',(0.00818418168268372,-0.0336938721132538,0.0683999775520834));
#78365=CARTESIAN_POINT('Ctrl Pts',(0.00848703646404946,-0.0335235895815171,
0.0681610062335428));
#78366=CARTESIAN_POINT('Ctrl Pts',(0.00840458617361054,-0.0334144449262748,
0.0681560053233215));
#78367=CARTESIAN_POINT('Ctrl Pts',(0.00832193784273545,-0.0333049234473147,
0.0681527020286099));
#78368=CARTESIAN_POINT('Ctrl Pts',(0.00823919677064589,-0.0331951640388587,
0.0681511101464262));
#78369=CARTESIAN_POINT('Ctrl Pts',(0.00840691723154057,-0.0335235895815171,
0.0682411441213866));
#78370=CARTESIAN_POINT('Ctrl Pts',(0.00832557019690479,-0.0334144449262748,
0.068237246210141));
#78371=CARTESIAN_POINT('Ctrl Pts',(0.00824404917646885,-0.0333049234473147,
0.0682350243891827));
#78372=CARTESIAN_POINT('Ctrl Pts',(0.00816245815323709,-0.0331951640388587,
0.0682344909420812));
#78373=CARTESIAN_POINT('Ctrl Pts',(0.00832679799903168,-0.0335235895815171,
0.0683212820092303));
#78374=CARTESIAN_POINT('Ctrl Pts',(0.00824655422019905,-0.0334144449262748,
0.0683184870969605));
#78375=CARTESIAN_POINT('Ctrl Pts',(0.00816616051020225,-0.0333049234473147,
0.0683173467497555));
#78376=CARTESIAN_POINT('Ctrl Pts',(0.00808571953582829,-0.0331951640388587,
0.0683178717377361));
#78377=CARTESIAN_POINT('Ctrl Pts',(0.00824667876652278,-0.0335235895815171,
0.0684014198970741));
#78378=CARTESIAN_POINT('Ctrl Pts',(0.00816753824349331,-0.0334144449262748,
0.06839972798378));
#78379=CARTESIAN_POINT('Ctrl Pts',(0.00808827184393565,-0.0333049234473147,
0.0683996691103284));
#78380=CARTESIAN_POINT('Ctrl Pts',(0.0080089809184195,-0.0331951640388587,
0.0684012525333911));
#78381=CARTESIAN_POINT('',(0.00812477562692895,-0.0331951640388687,0.0682754351124813));
#78382=CARTESIAN_POINT('Ctrl Pts',(0.00825201024343362,-0.0332121607145995,
0.0681513703642628));
#78383=CARTESIAN_POINT('Ctrl Pts',(0.00825109318430936,-0.033262544410958,
0.0681942712586196));
#78384=CARTESIAN_POINT('Ctrl Pts',(0.00825019192755287,-0.0333135300746445,
0.0682364329032445));
#78385=CARTESIAN_POINT('Ctrl Pts',(0.00824842030336822,-0.0334167203140643,
0.0683193111604632));
#78386=CARTESIAN_POINT('Ctrl Pts',(0.00824755062210575,-0.0334688847587333,
0.068359995673575));
#78387=CARTESIAN_POINT('Ctrl Pts',(0.00824669644180204,-0.0335216366562416,
0.0683999550371558));
#78388=CARTESIAN_POINT('Ctrl Pts',(0.00812309870278496,-0.0336938721132533,
0.0684001058694834));
#78389=CARTESIAN_POINT('Ctrl Pts',(0.0080894426644167,-0.0336474569765029,
0.068400109870179));
#78390=CARTESIAN_POINT('Ctrl Pts',(0.00805578897901491,-0.033601104548885,
0.0684005078570237));
#78391=CARTESIAN_POINT('Ctrl Pts',(0.00797058558505805,-0.0334837508592655,
0.0684015154682114));
#78392=CARTESIAN_POINT('Ctrl Pts',(0.00788544946376104,-0.0333660264659096,
0.0684050473901492));
#78393=CARTESIAN_POINT('Ctrl Pts',(0.00812169595727198,-0.0336938721132533,
0.0683986418432148));
#78394=CARTESIAN_POINT('Ctrl Pts',(0.00808803134947216,-0.0336474569765029,
0.0683986540546454));
#78395=CARTESIAN_POINT('Ctrl Pts',(0.008054369191343,-0.033601104548885,
0.0683990603519785));
#78396=CARTESIAN_POINT('Ctrl Pts',(0.00796914434638846,-0.0334837508592655,
0.0684000890034121));
#78397=CARTESIAN_POINT('Ctrl Pts',(0.00788398740697958,-0.0333660264659096,
0.068403642591994));
#78398=CARTESIAN_POINT('Ctrl Pts',(0.00788650306420541,-0.0336938721132533,
0.0681531742438294));
#78399=CARTESIAN_POINT('Ctrl Pts',(0.00785140165309137,-0.0336474569765029,
0.0681545631173086));
#78400=CARTESIAN_POINT('Ctrl Pts',(0.00781631890566614,-0.033601104548885,
0.0681563628019574));
#78401=CARTESIAN_POINT('Ctrl Pts',(0.00772749745522845,-0.0334837508592655,
0.068160919189714));
#78402=CARTESIAN_POINT('Ctrl Pts',(0.00763885002384193,-0.0333660264659096,
0.0681681055403747));
#78403=CARTESIAN_POINT('',(0.00787510014316679,-0.0336769361243754,0.0681551557786681));
#78404=CARTESIAN_POINT('',(0.00788790580513013,-0.0336938721132327,0.0681546382653259));
#78405=CARTESIAN_POINT('Ctrl Pts',(0.00787510014316647,-0.0336769361243751,
0.0681551557786681));
#78406=CARTESIAN_POINT('Ctrl Pts',(0.00787723448785643,-0.0336797586669899,
0.0681550672403853));
#78407=CARTESIAN_POINT('Ctrl Pts',(0.00787936879910747,-0.0336825812712593,
0.068154979845287));
#78408=CARTESIAN_POINT('Ctrl Pts',(0.00788363736050296,-0.0336882266106913,
0.0681548073407118));
#78409=CARTESIAN_POINT('Ctrl Pts',(0.00788577161061702,-0.0336910493458056,
0.0681547222312585));
#78410=CARTESIAN_POINT('Ctrl Pts',(0.00788790580513471,-0.0336938721132295,
0.0681546382653335));
#78411=CARTESIAN_POINT('Ctrl Pts',(0.00787510014316678,-0.0336769361243754,
0.0681551557786681));
#78412=CARTESIAN_POINT('Ctrl Pts',(0.00787683730438134,-0.0336279018392284,
0.0681970325883166));
#78413=CARTESIAN_POINT('Ctrl Pts',(0.00787859945683888,-0.0335767825782273,
0.0682395118483854));
#78414=CARTESIAN_POINT('Ctrl Pts',(0.007882052262458,-0.0334733171828138,
0.0683227467735353));
#78415=CARTESIAN_POINT('Ctrl Pts',(0.00788374523620226,-0.0334209631336572,
0.068363558379654));
#78416=CARTESIAN_POINT('Ctrl Pts',(0.00788540558802949,-0.0333679869844681,
0.0684035835867776));
#78417=CARTESIAN_POINT('',(0.00800480088119561,-0.0336938721132538,0.0682766400542803));
#78418=CARTESIAN_POINT('Origin',(0.00812378219310841,-0.0315241814719618,
0.07415));
#78419=CARTESIAN_POINT('',(0.00787510014322512,-0.0337108120655559,0.06815515577997));
#78420=CARTESIAN_POINT('',(0.00786229561583594,-0.0336938721132327,0.0681557006439514));
#78421=CARTESIAN_POINT('Origin',(0.0074365782648503,-0.0345562518650087,
0.0845486310755648));
#78422=CARTESIAN_POINT('Ctrl Pts',(0.00786229561583568,-0.0336938721132325,
0.068155700643952));
#78423=CARTESIAN_POINT('Ctrl Pts',(0.00786442944729637,-0.0336910493258036,
0.0681556075607988));
#78424=CARTESIAN_POINT('Ctrl Pts',(0.00786656340618438,-0.0336882266006898,
0.0681555156136469));
#78425=CARTESIAN_POINT('Ctrl Pts',(0.00787083158178454,-0.0336825812712704,
0.0681553339917212));
#78426=CARTESIAN_POINT('Ctrl Pts',(0.00787296579847292,-0.0336797586669955,
0.068155244316951));
#78427=CARTESIAN_POINT('Ctrl Pts',(0.00787510014316708,-0.0336769361243751,
0.068155155778668));
#78428=CARTESIAN_POINT('Origin',(0.00966986852248645,-0.0345562518009696,
0.0844559863629194));
#78429=CARTESIAN_POINT('Ctrl Pts',(0.00804652702986067,-0.034243627687391,
0.0683991603535004));
#78430=CARTESIAN_POINT('Ctrl Pts',(0.00782963053700891,-0.033943005420181,
0.0684020740800157));
#78431=CARTESIAN_POINT('Ctrl Pts',(0.00761356969817478,-0.0336441434784052,
0.0684213170614867));
#78432=CARTESIAN_POINT('Ctrl Pts',(0.0077966816178855,-0.034243627687391,
0.0684079506956411));
#78433=CARTESIAN_POINT('Ctrl Pts',(0.00758011665825297,-0.033943005420181,
0.0684202874972104));
#78434=CARTESIAN_POINT('Ctrl Pts',(0.00736509619540987,-0.0336441434784052,
0.0684489018113266));
#78435=CARTESIAN_POINT('Ctrl Pts',(0.00779418316376575,-0.034243627687391,
0.0684080385990625));
#78436=CARTESIAN_POINT('Ctrl Pts',(0.00757762151946541,-0.033943005420181,
0.0684204696313823));
#78437=CARTESIAN_POINT('Ctrl Pts',(0.00736261146038223,-0.0336441434784052,
0.0684491776588249));
#78438=CARTESIAN_POINT('',(0.00776056930730323,-0.0341934961088741,0.0684101218305973));
#78439=CARTESIAN_POINT('',(0.00752505549616061,-0.0338664212871963,0.0684298906172921));
#78440=CARTESIAN_POINT('Origin',(0.00830833166368909,-0.0345610751537998,
0.0851359427198085));
#78441=CARTESIAN_POINT('Origin',(0.00638339852864064,-0.0336938005063805,
0.0575232252220561));
#78442=CARTESIAN_POINT('',(0.00764951775477944,-0.0336938721132327,0.0684182290483187));
#78443=CARTESIAN_POINT('',(0.00758735733926295,-0.0336938721132427,0.0684247354099524));
#78444=CARTESIAN_POINT('',(0.00788540558803474,-0.0340203938281605,0.0684035835867774));
#78445=CARTESIAN_POINT('Origin',(0.00783073237135354,-0.0345589643243248,
0.0850773640322105));
#78446=CARTESIAN_POINT('',(0.00788546189524766,-0.034193496108874,0.0684049409545569));
#78447=CARTESIAN_POINT('Origin',(0.00742873964645005,-0.0341934220717729,
0.0573949626134628));
#78448=CARTESIAN_POINT('',(0.00782301560128544,-0.0341934961088841,0.068407531392587));
#78449=CARTESIAN_POINT('Ctrl Pts',(0.0081102703708805,-0.0340223579322396,
0.0681500152141289));
#78450=CARTESIAN_POINT('Ctrl Pts',(0.0080275149320661,-0.0339125849573575,
0.0681502015773978));
#78451=CARTESIAN_POINT('Ctrl Pts',(0.007944821501827,-0.0338030433565231,
0.0681521006549977));
#78452=CARTESIAN_POINT('Ctrl Pts',(0.00786229561583637,-0.0336938721132327,
0.0681557006439509));
#78453=CARTESIAN_POINT('Ctrl Pts',(0.00803534107479174,-0.0340223579322397,
0.0682350256865303));
#78454=CARTESIAN_POINT('Ctrl Pts',(0.00795375815210837,-0.0339125849573575,
0.068236245520216));
#78455=CARTESIAN_POINT('Ctrl Pts',(0.00787225780452297,-0.0338030433565231,
0.0682391530736658));
#78456=CARTESIAN_POINT('Ctrl Pts',(0.00779094392763323,-0.0336938721132327,
0.0682437353894825));
#78457=CARTESIAN_POINT('Ctrl Pts',(0.00796041177870297,-0.0340223579322397,
0.0683200361589317));
#78458=CARTESIAN_POINT('Ctrl Pts',(0.00788000137215064,-0.0339125849573575,
0.0683222894630343));
#78459=CARTESIAN_POINT('Ctrl Pts',(0.00779969410721894,-0.0338030433565231,
0.0683262054923338));
#78460=CARTESIAN_POINT('Ctrl Pts',(0.00771959223943009,-0.0336938721132327,
0.0683317701350142));
#78461=CARTESIAN_POINT('Ctrl Pts',(0.00788548248261421,-0.0340223579322397,
0.0684050466313331));
#78462=CARTESIAN_POINT('Ctrl Pts',(0.00780624459219291,-0.0339125849573575,
0.0684083334058526));
#78463=CARTESIAN_POINT('Ctrl Pts',(0.00772713040991491,-0.0338030433565231,
0.0684132579110019));
#78464=CARTESIAN_POINT('Ctrl Pts',(0.00764824055122694,-0.0336938721132327,
0.0684198048805459));
#78465=CARTESIAN_POINT('',(0.00775590668531769,-0.0336938721132427,0.0682869648461451));
#78466=CARTESIAN_POINT('Ctrl Pts',(0.00787510014336996,-0.0337108120662704,
0.0681551557835653));
#78467=CARTESIAN_POINT('Ctrl Pts',(0.00787688233389737,-0.0337611408994119,
0.0681981180906034));
#78468=CARTESIAN_POINT('Ctrl Pts',(0.00787863200340158,-0.0338121088780922,
0.0682402964308537));
#78469=CARTESIAN_POINT('Ctrl Pts',(0.00788206789428731,-0.0339153382773239,
0.0683231236016381));
#78470=CARTESIAN_POINT('Ctrl Pts',(0.00788375266207461,-0.033967555847311,
0.0683637373911592));
#78471=CARTESIAN_POINT('Ctrl Pts',(0.0078854055880311,-0.0340203938281304,
0.0684035835868175));
#78472=CARTESIAN_POINT('Ctrl Pts',(0.00776206163108845,-0.0341934961088741,
0.0684114952747232));
#78473=CARTESIAN_POINT('Ctrl Pts',(0.00764342256703021,-0.0340287516186244,
0.0684189735623579));
#78474=CARTESIAN_POINT('Ctrl Pts',(0.00752519396108338,-0.0338644633283559,
0.0684313489024514));
#78475=CARTESIAN_POINT('Ctrl Pts',(0.00776056930730329,-0.0341934961088741,
0.0684101218305973));
#78476=CARTESIAN_POINT('Ctrl Pts',(0.00764190184836983,-0.0340287516186244,
0.0684176309708505));
#78477=CARTESIAN_POINT('Ctrl Pts',(0.00752364614697278,-0.0338644633283559,
0.0684300383107814));
#78478=CARTESIAN_POINT('Ctrl Pts',(0.00751191937521459,-0.0341934961088741,
0.0681812795431451));
#78479=CARTESIAN_POINT('Ctrl Pts',(0.00738852078228368,-0.0340287516186244,
0.0681939293248429));
#78480=CARTESIAN_POINT('Ctrl Pts',(0.00726575045616308,-0.0338644633283559,
0.0682116684549956));
#78481=CARTESIAN_POINT('',(0.00749917147815481,-0.0341764758832383,0.0681826001101547));
#78482=CARTESIAN_POINT('',(0.00751191937521463,-0.034193496108874,0.068181279543145));
#78483=CARTESIAN_POINT('Origin',(0.00871354627553403,-0.0345621026663571,
0.084703696538433));
#78484=CARTESIAN_POINT('Ctrl Pts',(0.00749917147983292,-0.034176475883747,
0.0681826001108439));
#78485=CARTESIAN_POINT('Ctrl Pts',(0.00750363999786195,-0.0341260050041165,
0.0682252912637987));
#78486=CARTESIAN_POINT('Ctrl Pts',(0.00750803088050584,-0.0340749269149653,
0.0682672403398259));
#78487=CARTESIAN_POINT('Ctrl Pts',(0.00751666059557544,-0.0339715436309371,
0.0683496868680737));
#78488=CARTESIAN_POINT('Ctrl Pts',(0.00752089614811635,-0.0339192778242717,
0.0683901530424331));
#78489=CARTESIAN_POINT('Ctrl Pts',(0.00752505549761581,-0.0338664212861681,
0.0684298906157721));
#78490=CARTESIAN_POINT('',(0.00763624434126893,-0.0341934961088841,0.0682957006868812));
#78491=CARTESIAN_POINT('Origin',(0.00812378219310841,-0.0315241814719618,
0.07415));
#78492=CARTESIAN_POINT('',(0.0074991714773945,-0.0342105180190384,0.0681826001109751));
#78493=CARTESIAN_POINT('',(0.00748642642908479,-0.0341934961088739,0.0681839479025));
#78494=CARTESIAN_POINT('Origin',(0.00875886989547323,-0.0345621710737136,
0.0847042138250342));
#78495=CARTESIAN_POINT('Origin',(0.00973218070959005,-0.034562103557307,
0.0845970769388304));
#78496=CARTESIAN_POINT('Origin',(0.00968794611505139,-0.0345621719168675,
0.0846069645717558));
#78497=CARTESIAN_POINT('Ctrl Pts',(0.00765100961461013,-0.0346945769586965,
0.0684180728946081));
#78498=CARTESIAN_POINT('Ctrl Pts',(0.00753095210644929,-0.0345275153362944,
0.0684279753055526));
#78499=CARTESIAN_POINT('Ctrl Pts',(0.00741117496697709,-0.0343603235965185,
0.0684416559758941));
#78500=CARTESIAN_POINT('Ctrl Pts',(0.00729203184244175,-0.034193496108874,
0.0684590691792403));
#78501=CARTESIAN_POINT('Ctrl Pts',(0.00756763177367103,-0.0346945769586965,
0.0684268000947073));
#78502=CARTESIAN_POINT('Ctrl Pts',(0.00744775706021046,-0.0345275153362944,
0.0684384488879129));
#78503=CARTESIAN_POINT('Ctrl Pts',(0.00732821768483326,-0.0343603235965185,
0.0684538706434943));
#78504=CARTESIAN_POINT('Ctrl Pts',(0.00720936651405417,-0.034193496108874,
0.0684730144961536));
#78505=CARTESIAN_POINT('Ctrl Pts',(0.00748425393273184,-0.0346945769586965,
0.0684355272948049));
#78506=CARTESIAN_POINT('Ctrl Pts',(0.0073645620139717,-0.0345275153362944,
0.0684489224702714));
#78507=CARTESIAN_POINT('Ctrl Pts',(0.00724526040268954,-0.0343603235965185,
0.0684660853110933));
#78508=CARTESIAN_POINT('Ctrl Pts',(0.00712670118566658,-0.034193496108874,
0.0684869598130667));
#78509=CARTESIAN_POINT('Ctrl Pts',(0.00740087609179284,-0.0346945769586965,
0.0684442544949057));
#78510=CARTESIAN_POINT('Ctrl Pts',(0.00728136696773278,-0.0345275153362944,
0.0684593960526336));
#78511=CARTESIAN_POINT('Ctrl Pts',(0.0071623031205456,-0.0343603235965185,
0.068478299978695));
#78512=CARTESIAN_POINT('Ctrl Pts',(0.00704403585727901,-0.034193496108874,
0.0685009051299801));
#78513=CARTESIAN_POINT('',(0.00740087609266788,-0.0346945769586966,0.0684442544948143));
#78514=CARTESIAN_POINT('',(0.00716706830798636,-0.0343667727832763,0.0684787723072952));
#78515=CARTESIAN_POINT('Origin',(0.00969561993458519,-0.0345626461566601,
0.0851005265089994));
#78516=CARTESIAN_POINT('Origin',(0.00532857933020388,-0.034193477102778,
0.0575805791713511));
#78517=CARTESIAN_POINT('',(0.007290552731434,-0.034193496108874,0.0684593186994703));
#78518=CARTESIAN_POINT('',(0.00722892351312495,-0.0341934961088839,0.0684697153070706));
#78519=CARTESIAN_POINT('',(0.00752505549780014,-0.0345211942962709,0.0684298906178197));
#78520=CARTESIAN_POINT('Origin',(0.00921707535829783,-0.0345625596120209,
0.0851472734654589));
#78521=CARTESIAN_POINT('',(0.00752519692372647,-0.0346945769586885,0.0684312417715662));
#78522=CARTESIAN_POINT('Origin',(0.00637346058295795,-0.0346945685853895,
0.057427786922971));
#78523=CARTESIAN_POINT('',(0.00746303650820717,-0.0346945769587026,0.0684377481332003));
#78524=CARTESIAN_POINT('Ctrl Pts',(0.00773355391136304,-0.0345231616327841,
0.0681627032904536));
#78525=CARTESIAN_POINT('Ctrl Pts',(0.00765102745566147,-0.0344132092796988,
0.06816808203792));
#78526=CARTESIAN_POINT('Ctrl Pts',(0.0075686165130943,-0.0343032738558979,
0.068175167502508));
#78527=CARTESIAN_POINT('Ctrl Pts',(0.00748642642908473,-0.0341934961088739,
0.0681839479025));
#78528=CARTESIAN_POINT('Ctrl Pts',(0.00766411045535195,-0.0345231616327841,
0.0682522507223301));
#78529=CARTESIAN_POINT('Ctrl Pts',(0.00758281828492609,-0.0344132092796988,
0.068258586650069));
#78530=CARTESIAN_POINT('Ctrl Pts',(0.00750166136247011,-0.0343032738558979,
0.0682666037153261));
#78531=CARTESIAN_POINT('Ctrl Pts',(0.00742074339629089,-0.0341934961088739,
0.0682762889840479));
#78532=CARTESIAN_POINT('Ctrl Pts',(0.00759466699934085,-0.0345231616327841,
0.0683417981542066));
#78533=CARTESIAN_POINT('Ctrl Pts',(0.00751460911419072,-0.0344132092796988,
0.0683490912622181));
#78534=CARTESIAN_POINT('Ctrl Pts',(0.00743470621184593,-0.0343032738558979,
0.0683580399281443));
#78535=CARTESIAN_POINT('Ctrl Pts',(0.00735506036349704,-0.0341934961088739,
0.0683686300655959));
#78536=CARTESIAN_POINT('Ctrl Pts',(0.00752522354332976,-0.0345231616327841,
0.0684313455860831));
#78537=CARTESIAN_POINT('Ctrl Pts',(0.00744639994345534,-0.0344132092796988,
0.0684395958743671));
#78538=CARTESIAN_POINT('Ctrl Pts',(0.00736775106122175,-0.0343032738558979,
0.0684494761409624));
#78539=CARTESIAN_POINT('Ctrl Pts',(0.0072893773307032,-0.0341934961088739,
0.0684609711471438));
#78540=CARTESIAN_POINT('',(0.00738848958026939,-0.0341934961088839,0.0683216333009951));
#78541=CARTESIAN_POINT('Ctrl Pts',(0.00749917147774936,-0.0342105180195407,
0.0681826001144063));
#78542=CARTESIAN_POINT('Ctrl Pts',(0.00750364500559306,-0.0342610556241064,
0.0682253392619848));
#78543=CARTESIAN_POINT('Ctrl Pts',(0.00750803825829279,-0.034312218986965,
0.0682673114776594));
#78544=CARTESIAN_POINT('Ctrl Pts',(0.00751666806445142,-0.03441581196952,
0.0683497588372985));
#78545=CARTESIAN_POINT('Ctrl Pts',(0.00752090108824999,-0.0344681990450097,
0.0683902002596279));
#78546=CARTESIAN_POINT('Ctrl Pts',(0.00752505549779421,-0.0345211942962525,
0.0684298906178449));
#78547=CARTESIAN_POINT('Ctrl Pts',(0.00740245132565116,-0.0346945769586932,
0.0684455312126745));
#78548=CARTESIAN_POINT('Ctrl Pts',(0.00728451546986506,-0.0345296777077528,
0.0684604442179569));
#78549=CARTESIAN_POINT('Ctrl Pts',(0.00716729675700591,-0.0343648066252516,
0.0684802188775543));
#78550=CARTESIAN_POINT('Ctrl Pts',(0.00740087609267687,-0.0346945769586932,
0.0684442544948132));
#78551=CARTESIAN_POINT('Ctrl Pts',(0.00728291384165238,-0.0345296777077528,
0.0684592000669228));
#78552=CARTESIAN_POINT('Ctrl Pts',(0.00716567010212613,-0.0343648066252516,
0.0684790083564589));
#78553=CARTESIAN_POINT('Ctrl Pts',(0.00713834768831118,-0.0346945769586932,
0.0682314766337577));
#78554=CARTESIAN_POINT('Ctrl Pts',(0.00701598640556762,-0.0345296777077528,
0.0682518497948666));
#78555=CARTESIAN_POINT('Ctrl Pts',(0.00689457172048071,-0.0343648066252516,
0.0682772628516183));
#78556=CARTESIAN_POINT('',(0.00712570786525928,-0.0346775396664966,0.0682335950417985));
#78557=CARTESIAN_POINT('',(0.00713834768830782,-0.0346945769586886,0.0682314766337583));
#78558=CARTESIAN_POINT('Origin',(0.0100377842878865,-0.034562661826208,
0.0845777899648913));
#78559=CARTESIAN_POINT('Ctrl Pts',(0.00712570786694295,-0.0346775396670097,
0.0682335950424754));
#78560=CARTESIAN_POINT('Ctrl Pts',(0.00713285378982359,-0.0346269749928344,
0.0682759547095296));
#78561=CARTESIAN_POINT('Ctrl Pts',(0.00713987274912904,-0.0345757902891101,
0.0683175615448052));
#78562=CARTESIAN_POINT('Ctrl Pts',(0.00715366235116246,-0.0344721681088617,
0.068399303846144));
#78563=CARTESIAN_POINT('Ctrl Pts',(0.00716042758215949,-0.0344197714290521,
0.0684394072663182));
#78564=CARTESIAN_POINT('Ctrl Pts',(0.00716706830828532,-0.0343667727831525,
0.068478772307078));
#78565=CARTESIAN_POINT('',(0.00726961189049784,-0.0346945769587026,0.0683378655642963));
#78566=CARTESIAN_POINT('Origin',(0.00812378219310841,-0.0315241814719618,
0.07415));
#78567=CARTESIAN_POINT('',(0.0071257078647268,-0.0347116136489812,0.0682335950430839));
#78568=CARTESIAN_POINT('',(0.00711307259435407,-0.0346945769586886,0.0682357404430474));
#78569=CARTESIAN_POINT('Origin',(0.0100821166646013,-0.0345626689394674,
0.0845684159877676));
#78570=CARTESIAN_POINT('Origin',(0.00973660713539254,-0.0345626626257731,
0.0846285994614035));
#78571=CARTESIAN_POINT('Origin',(0.00969165239065285,-0.0345626697747338,
0.0846342838689481));
#78572=CARTESIAN_POINT('Ctrl Pts',(0.00732877954649289,-0.0352450361874068,
0.0684537965786412));
#78573=CARTESIAN_POINT('Ctrl Pts',(0.00711394370916413,-0.0349452760959493,
0.0684837805954732));
#78574=CARTESIAN_POINT('Ctrl Pts',(0.0069019767166667,-0.034644428984174,
0.0685298617451737));
#78575=CARTESIAN_POINT('Ctrl Pts',(0.00732628713881102,-0.0352450361874068,
0.0684542009657669));
#78576=CARTESIAN_POINT('Ctrl Pts',(0.00711146655319298,-0.0349452760959493,
0.068484278985297));
#78577=CARTESIAN_POINT('Ctrl Pts',(0.00689952184974562,-0.034644428984174,
0.0685304527218228));
#78578=CARTESIAN_POINT('Ctrl Pts',(0.0070795141010024,-0.0352450361874068,
0.0684942392950365));
#78579=CARTESIAN_POINT('Ctrl Pts',(0.00686620358575187,-0.0349452760959493,
0.0685336245124117));
#78580=CARTESIAN_POINT('Ctrl Pts',(0.00665646571894468,-0.034644428984174,
0.0685889652613342));
#78581=CARTESIAN_POINT('Ctrl Pts',(0.00707704637062432,-0.0352450361874068,
0.0684946396783292));
#78582=CARTESIAN_POINT('Ctrl Pts',(0.00686375095607746,-0.0349452760959493,
0.0685341179676828));
#78583=CARTESIAN_POINT('Ctrl Pts',(0.00665403515763668,-0.034644428984174,
0.0685895503867294));
#78584=CARTESIAN_POINT('',(0.00704406719588301,-0.0351951634053301,0.0685008967236133));
#78585=CARTESIAN_POINT('',(0.00681285683139752,-0.0348678972925434,0.0685500357415405));
#78586=CARTESIAN_POINT('Origin',(0.0110413242494258,-0.0345636767881713,
0.0847620907885232));
#78587=CARTESIAN_POINT('Origin',(0.00429423075620386,-0.0346946199341032,
0.0577910621877315));
#78588=CARTESIAN_POINT('',(0.00693487610176077,-0.0346945769330288,0.0685228668663425));
#78589=CARTESIAN_POINT('',(0.00687402129446573,-0.0346945769458128,0.068537112690876));
#78590=CARTESIAN_POINT('',(0.0071670683083037,-0.0350221583435276,0.0684787723072845));
#78591=CARTESIAN_POINT('Origin',(0.0105844074873605,-0.0345628458714861,
0.0849116583843685));
#78592=CARTESIAN_POINT('',(0.00716727704116918,-0.035195136029876,0.0684799914558962));
#78593=CARTESIAN_POINT('Origin',(0.0053343155728567,-0.0351951838366754,
0.0576145372036346));
#78594=CARTESIAN_POINT('',(0.0070440358581378,-0.035195137132875,0.0685009051297173));
#78595=CARTESIAN_POINT('Ctrl Pts',(0.00735837751390443,-0.0350241211494342,
0.0681990206119436));
#78596=CARTESIAN_POINT('Ctrl Pts',(0.00727640521283051,-0.0349144232818962,
0.0682095637475715));
#78597=CARTESIAN_POINT('Ctrl Pts',(0.00719460178153038,-0.0348045283579412,
0.0682218076198117));
#78598=CARTESIAN_POINT('Ctrl Pts',(0.00711307258340003,-0.0346945769439158,
0.0682357404449193));
#78599=CARTESIAN_POINT('Ctrl Pts',(0.00729469381942308,-0.0350241211494342,
0.0682927517639695));
#78600=CARTESIAN_POINT('Ctrl Pts',(0.00721401262653705,-0.0349144232818962,
0.0683041721163775));
#78601=CARTESIAN_POINT('Ctrl Pts',(0.00713351920891297,-0.0348045283579412,
0.0683172670423256));
#78602=CARTESIAN_POINT('Ctrl Pts',(0.0070533172925506,-0.0346945769439158,
0.0683320236055363));
#78603=CARTESIAN_POINT('Ctrl Pts',(0.00723101012494173,-0.0350241211494342,
0.0683864829159954));
#78604=CARTESIAN_POINT('Ctrl Pts',(0.0071516200402436,-0.0349144232818962,
0.0683987804851836));
#78605=CARTESIAN_POINT('Ctrl Pts',(0.00707243663629556,-0.0348045283579412,
0.0684127264648395));
#78606=CARTESIAN_POINT('Ctrl Pts',(0.00699356200170117,-0.0346945769439158,
0.0684283067661533));
#78607=CARTESIAN_POINT('Ctrl Pts',(0.00716732643046039,-0.0350241211494342,
0.0684802140680213));
#78608=CARTESIAN_POINT('Ctrl Pts',(0.00708922745395014,-0.0349144232818962,
0.0684933888539896));
#78609=CARTESIAN_POINT('Ctrl Pts',(0.00701135406367814,-0.0348045283579412,
0.0685081858873534));
#78610=CARTESIAN_POINT('Ctrl Pts',(0.00693380671085173,-0.0346945769439158,
0.0685245899267703));
#78611=CARTESIAN_POINT('',(0.00702397434833165,-0.0346945769458128,0.068379303654558));
#78612=CARTESIAN_POINT('Ctrl Pts',(0.00712570786526901,-0.0347116136492811,
0.0682335950463216));
#78613=CARTESIAN_POINT('Ctrl Pts',(0.00713285093764519,-0.0347621546532048,
0.0682759378935546));
#78614=CARTESIAN_POINT('Ctrl Pts',(0.00713986841550647,-0.0348133084096492,
0.0683175362391114));
#78615=CARTESIAN_POINT('Ctrl Pts',(0.00715365803877717,-0.0349168561544575,
0.0683992786436124));
#78616=CARTESIAN_POINT('Ctrl Pts',(0.00716042471453214,-0.0349692089015917,
0.0684393902794295));
#78617=CARTESIAN_POINT('Ctrl Pts',(0.00716706830829008,-0.0350221583435,
0.068478772307324));
#78618=CARTESIAN_POINT('Ctrl Pts',(0.00704522804053917,-0.0351951371254919,
0.0685017531397606));
#78619=CARTESIAN_POINT('Ctrl Pts',(0.00692845408053324,-0.035030733898094,
0.0685240515701573));
#78620=CARTESIAN_POINT('Ctrl Pts',(0.00681270152137923,-0.0348659306897816,
0.0685511573404456));
#78621=CARTESIAN_POINT('Ctrl Pts',(0.00704403585816338,-0.035195137125492,
0.0685009051298308));
#78622=CARTESIAN_POINT('Ctrl Pts',(0.00692724436608421,-0.035030733898094,
0.0685232282078501));
#78623=CARTESIAN_POINT('Ctrl Pts',(0.00681147530855085,-0.0348659306897816,
0.0685503593293192));
#78624=CARTESIAN_POINT('Ctrl Pts',(0.0068442248494029,-0.035195137125492,
0.0683587777817316));
#78625=CARTESIAN_POINT('Ctrl Pts',(0.00672449496357548,-0.035030733898094,
0.0683852318269914));
#78626=CARTESIAN_POINT('Ctrl Pts',(0.00660596076046755,-0.0348659306897816,
0.068416611832798));
#78627=CARTESIAN_POINT('Origin',(0.00560066682560257,-0.0308609197383906,
0.0633718456812268));
#78628=CARTESIAN_POINT('',(0.00695692276348074,-0.035195137125492,0.0684389408106035));
#78629=CARTESIAN_POINT('Origin',(0.00848199412557994,-0.0351840467441107,
0.0750590818785555));
#78630=CARTESIAN_POINT('Origin',(0.00462868883488077,-0.0352322614588957,
0.0627063745744573));
#78631=CARTESIAN_POINT('',(0.00658359560922478,-0.0351951142564657,0.0686087330085759));
#78632=CARTESIAN_POINT('',(0.00646421102734251,-0.0351951372916786,0.0686447004127151));
#78633=CARTESIAN_POINT('Origin',(0.00789759517336728,-0.0352875118894279,
0.0744046163418812));
#78634=CARTESIAN_POINT('Origin',(0.0155892122750297,-0.0298325076521865,
0.073399970684482));
#78635=CARTESIAN_POINT('Origin',(0.00890344754906864,-0.0338731501726093,
0.0658046183588913));
#78636=CARTESIAN_POINT('Ctrl Pts',(0.0101351648519866,-0.0321934096636942,
0.0687618207579114));
#78637=CARTESIAN_POINT('Ctrl Pts',(0.0100387190094497,-0.0320508460844432,
0.0687258179661549));
#78638=CARTESIAN_POINT('Ctrl Pts',(0.0099413785634212,-0.0319086045663286,
0.0686924336301076));
#78639=CARTESIAN_POINT('Ctrl Pts',(0.00984335902280536,-0.031766989286822,
0.0686617223772792));
#78640=CARTESIAN_POINT('Ctrl Pts',(0.0100559929262052,-0.0321934096636942,
0.0687342120854356));
#78641=CARTESIAN_POINT('Ctrl Pts',(0.00995905290157842,-0.0320508460844432,
0.0686996264334484));
#78642=CARTESIAN_POINT('Ctrl Pts',(0.00986125672182438,-0.0319086045663286,
0.0686676714463398));
#78643=CARTESIAN_POINT('Ctrl Pts',(0.00976282062375176,-0.031766989286822,
0.0686383985931954));
#78644=CARTESIAN_POINT('Ctrl Pts',(0.00997682100042376,-0.0321934096636942,
0.06870660341296));
#78645=CARTESIAN_POINT('Ctrl Pts',(0.00987938679370717,-0.0320508460844432,
0.0686734349007418));
#78646=CARTESIAN_POINT('Ctrl Pts',(0.00978113488022756,-0.0319086045663286,
0.068642909262572));
#78647=CARTESIAN_POINT('Ctrl Pts',(0.00968228222469816,-0.031766989286822,
0.0686150748091116));
#78648=CARTESIAN_POINT('Ctrl Pts',(0.00989764907464233,-0.0321934096636942,
0.0686789947404844));
#78649=CARTESIAN_POINT('Ctrl Pts',(0.00979972068583591,-0.0320508460844432,
0.0686472433680353));
#78650=CARTESIAN_POINT('Ctrl Pts',(0.00970101303863074,-0.0319086045663286,
0.0686181470788042));
#78651=CARTESIAN_POINT('Ctrl Pts',(0.00960174382564456,-0.031766989286822,
0.0685917510250278));
#78652=CARTESIAN_POINT('',(0.00989906547603906,-0.0321934096636942,0.0686794886650928));
#78653=CARTESIAN_POINT('',(0.00967281289770884,-0.0318665617511283,0.0686111708037462));
#78654=CARTESIAN_POINT('Origin',(0.00415979697328217,-0.0326371944421585,
0.0843727579835789));
#78655=CARTESIAN_POINT('Origin',(0.0126250220541809,-0.0316939261509442,
0.0580550327220509));
#78656=CARTESIAN_POINT('',(0.0100172774156477,-0.032019722162186,0.0687193218647438));
#78657=CARTESIAN_POINT('Ctrl Pts',(0.0100171240667253,-0.0320197392094775,
0.0687192184288374));
#78658=CARTESIAN_POINT('Ctrl Pts',(0.00998949048868716,-0.0319792716576073,
0.0687095845410141));
#78659=CARTESIAN_POINT('Ctrl Pts',(0.00996165766720061,-0.0319386439829743,
0.0687001174633433));
#78660=CARTESIAN_POINT('Ctrl Pts',(0.00993359365955867,-0.0318979099381674,
0.0686908152641895));
#78661=CARTESIAN_POINT('Ctrl Pts',(0.00990553020662064,-0.0318571766984962,
0.0686815132488999));
#78662=CARTESIAN_POINT('Ctrl Pts',(0.00987737877403414,-0.0318163871833598,
0.0686724216933247));
#78663=CARTESIAN_POINT('Ctrl Pts',(0.00984923727325862,-0.0317755399638303,
0.0686635685179199));
#78664=CARTESIAN_POINT('',(0.0100170948752984,-0.0321934096636184,0.0687206476364617));
#78665=CARTESIAN_POINT('Origin',(0.0107576046418906,-0.0324114026571386,
0.0665332235056358));
#78666=CARTESIAN_POINT('',(0.00995808017567875,-0.0321934096636663,0.0687000681507873));
#78667=CARTESIAN_POINT('Ctrl Pts',(0.00989994743820871,-0.0321934096636618,
0.0686813150905937));
#78668=CARTESIAN_POINT('Ctrl Pts',(0.00982453001126425,-0.0320835708272592,
0.0686568203876015));
#78669=CARTESIAN_POINT('Ctrl Pts',(0.00974864941288699,-0.0319739230346488,
0.0686339006522635));
#78670=CARTESIAN_POINT('Ctrl Pts',(0.0096724049775894,-0.0318646057455573,
0.0686125777578681));
#78671=CARTESIAN_POINT('Ctrl Pts',(0.00985067131905665,-0.0321934096636618,
0.0685792708411436));
#78672=CARTESIAN_POINT('Ctrl Pts',(0.00977384662238364,-0.0320835708272592,
0.0685554556942381));
#78673=CARTESIAN_POINT('Ctrl Pts',(0.00969657363392936,-0.0319739230346488,
0.0685332442441905));
#78674=CARTESIAN_POINT('Ctrl Pts',(0.00961895340012431,-0.0318646057455573,
0.0685126573213648));
#78675=CARTESIAN_POINT('Ctrl Pts',(0.00980139519990459,-0.0321934096636618,
0.0684772265916935));
#78676=CARTESIAN_POINT('Ctrl Pts',(0.00972316323350302,-0.0320835708272592,
0.0684540910008747));
#78677=CARTESIAN_POINT('Ctrl Pts',(0.00964449785497172,-0.0319739230346488,
0.0684325878361175));
#78678=CARTESIAN_POINT('Ctrl Pts',(0.00956550182265921,-0.0318646057455573,
0.0684127368848614));
#78679=CARTESIAN_POINT('Ctrl Pts',(0.00975211908075253,-0.0321934096636618,
0.0683751823422434));
#78680=CARTESIAN_POINT('Ctrl Pts',(0.00967247984462241,-0.0320835708272592,
0.0683527263075112));
#78681=CARTESIAN_POINT('Ctrl Pts',(0.00959242207601408,-0.0319739230346488,
0.0683319314280444));
#78682=CARTESIAN_POINT('Ctrl Pts',(0.00951205024519412,-0.0318646057455573,
0.0683128164483581));
#78683=CARTESIAN_POINT('',(0.00973978025155323,-0.0321763980308458,0.0683717173612915));
#78684=CARTESIAN_POINT('',(0.00975211908072106,-0.0321934096636184,0.0683751823422345));
#78685=CARTESIAN_POINT('Origin',(0.00469517298259082,-0.0326386230618203,
0.0841317309506976));
#78686=CARTESIAN_POINT('Ctrl Pts',(0.00973978025069336,-0.0321763980306277,
0.0683717173643431));
#78687=CARTESIAN_POINT('Ctrl Pts',(0.00972822077595706,-0.0321259596174817,
0.0684130502804517));
#78688=CARTESIAN_POINT('Ctrl Pts',(0.00971686158412674,-0.0320749164631385,
0.0684536670501569));
#78689=CARTESIAN_POINT('Ctrl Pts',(0.00969453462474263,-0.031971605779392,
0.0685335009838122));
#78690=CARTESIAN_POINT('Ctrl Pts',(0.00968357555652206,-0.0319193786690118,
0.0685726870417803));
#78691=CARTESIAN_POINT('Ctrl Pts',(0.00967281289720152,-0.0318665617525302,
0.0686111708055284));
#78692=CARTESIAN_POINT('',(0.00982559227839006,-0.0321934096636663,0.0685273355036737));
#78693=CARTESIAN_POINT('Origin',(0.00812378219310841,-0.0315241814719618,
0.07415));
#78694=CARTESIAN_POINT('',(0.00973978025165294,-0.0322104233323627,0.0683717173609343));
#78695=CARTESIAN_POINT('',(0.00972743405025982,-0.0321934096636183,0.0683682787406278));
#78696=CARTESIAN_POINT('Origin',(0.00473670438611051,-0.0326387237043649,
0.0841499047667895));
#78697=CARTESIAN_POINT('Origin',(0.00587683744484425,-0.0326386241300037,
0.0844622064349481));
#78698=CARTESIAN_POINT('Origin',(0.00583190441155826,-0.0326387244927525,
0.0844561943596892));
#78699=CARTESIAN_POINT('Ctrl Pts',(0.00982738359587753,-0.0327445246967097,
0.0686567434739962));
#78700=CARTESIAN_POINT('Ctrl Pts',(0.00962020203903971,-0.032443687833936,
0.0685924910967068));
#78701=CARTESIAN_POINT('Ctrl Pts',(0.00940876931146334,-0.0321434074405927,
0.0685440270152576));
#78702=CARTESIAN_POINT('Ctrl Pts',(0.00958704972568487,-0.0327445246967097,
0.0685878984971409));
#78703=CARTESIAN_POINT('Ctrl Pts',(0.00937727163809743,-0.032443687833936,
0.0685327104599476));
#78704=CARTESIAN_POINT('Ctrl Pts',(0.00916393251938352,-0.0321434074405927,
0.06849348054907));
#78705=CARTESIAN_POINT('',(0.00955206611124706,-0.0326943950436612,0.0685788125099592));
#78706=CARTESIAN_POINT('',(0.00932197027682842,-0.0323666188837389,0.0685248359742998));
#78707=CARTESIAN_POINT('Origin',(0.00545093103263963,-0.0326395579112774,
0.0848818413481453));
#78708=CARTESIAN_POINT('Origin',(0.0116229071770842,-0.0321933825602941,
0.0577225648590064));
#78709=CARTESIAN_POINT('',(0.00944394454682107,-0.0321934096532688,0.0685522061170054));
#78710=CARTESIAN_POINT('',(0.00938281589963273,-0.0321934096584275,0.0685391854089375));
#78711=CARTESIAN_POINT('',(0.00967281289796098,-0.0325210109756238,0.0686111708028298));
#78712=CARTESIAN_POINT('Origin',(0.0049921278315033,-0.0326393129156624,
0.0847380218359002));
#78713=CARTESIAN_POINT('',(0.00967244699959204,-0.0326943950436593,0.0686124791361874));
#78714=CARTESIAN_POINT('Origin',(0.0126519322500182,-0.0326943765538051,
0.0579588138369248));
#78715=CARTESIAN_POINT('',(0.00961225655542955,-0.0326943950436702,0.0685956458230833));
#78716=CARTESIAN_POINT('Ctrl Pts',(0.00996502817638299,-0.0325229783203769,
0.0684394997391562));
#78717=CARTESIAN_POINT('Ctrl Pts',(0.00988630905516765,-0.032413025309245,
0.0684141182035422));
#78718=CARTESIAN_POINT('Ctrl Pts',(0.00980707682358036,-0.0323031222208069,
0.0683903689236795));
#78719=CARTESIAN_POINT('Ctrl Pts',(0.00972743404593875,-0.0321934096576658,
0.0683682787394293));
#78720=CARTESIAN_POINT('Ctrl Pts',(0.00986749665100188,-0.0325229783203769,
0.0684971950058001));
#78721=CARTESIAN_POINT('Ctrl Pts',(0.00978957285777552,-0.032413025309245,
0.0684731579401305));
#78722=CARTESIAN_POINT('Ctrl Pts',(0.00971116364563802,-0.0323031222208069,
0.0684507364739161));
#78723=CARTESIAN_POINT('Ctrl Pts',(0.00963237046466076,-0.0321934096576658,
0.0684299557833831));
#78724=CARTESIAN_POINT('Ctrl Pts',(0.00976996512562077,-0.0325229783203769,
0.068554890272444));
#78725=CARTESIAN_POINT('Ctrl Pts',(0.00969283666038338,-0.032413025309245,
0.0685321976767189));
#78726=CARTESIAN_POINT('Ctrl Pts',(0.00961525046769568,-0.0323031222208069,
0.0685111040241527));
#78727=CARTESIAN_POINT('Ctrl Pts',(0.00953730688338278,-0.0321934096576658,
0.0684916328273369));
#78728=CARTESIAN_POINT('Ctrl Pts',(0.00967243360023966,-0.0325229783203769,
0.0686125855390879));
#78729=CARTESIAN_POINT('Ctrl Pts',(0.00959610046299125,-0.032413025309245,
0.0685912374133073));
#78730=CARTESIAN_POINT('Ctrl Pts',(0.00951933728975334,-0.0323031222208069,
0.0685714715743892));
#78731=CARTESIAN_POINT('Ctrl Pts',(0.00944224330210479,-0.0321934096576658,
0.0685533098712907));
#78732=CARTESIAN_POINT('',(0.00958568929905662,-0.0321934096584275,0.0684602424287965));
#78733=CARTESIAN_POINT('Ctrl Pts',(0.00973978025071093,-0.0322104233328948,
0.0683717173642805));
#78734=CARTESIAN_POINT('Ctrl Pts',(0.00972820511270824,-0.0322609421831021,
0.0684131062871274));
#78735=CARTESIAN_POINT('Ctrl Pts',(0.00971683826910974,-0.032312088823999,
0.0684537504170378));
#78736=CARTESIAN_POINT('Ctrl Pts',(0.00969451114066534,-0.0324156524631821,
0.0685335849551975));
#78737=CARTESIAN_POINT('Ctrl Pts',(0.0096835600334637,-0.0324680267167318,
0.0685727425471806));
#78738=CARTESIAN_POINT('Ctrl Pts',(0.009672812897945,-0.0325210109755912,
0.0686111708028703));
#78739=CARTESIAN_POINT('Origin',(0.015390548394678,-0.0262834582511949,
0.0771662053661228));
#78740=CARTESIAN_POINT('Origin',(0.0162906581482553,-0.0342770845939972,
0.0651430105617909));
#78741=CARTESIAN_POINT('Ctrl Pts',(0.00955306077375524,-0.0326943950436604,
0.0685805795236342));
#78742=CARTESIAN_POINT('Ctrl Pts',(0.00947630372138444,-0.0325844576448134,
0.0685608813860393));
#78743=CARTESIAN_POINT('Ctrl Pts',(0.00939913384701679,-0.0324744968375322,
0.0685427693160645));
#78744=CARTESIAN_POINT('Ctrl Pts',(0.0093216503452795,-0.0323646534831894,
0.068526265156173));
#78745=CARTESIAN_POINT('Ctrl Pts',(0.0094974745588082,-0.0326943950436604,
0.0684818308512924));
#78746=CARTESIAN_POINT('Ctrl Pts',(0.00941935656465779,-0.0325844576448134,
0.0684628987959191));
#78747=CARTESIAN_POINT('Ctrl Pts',(0.00934084149603092,-0.0324744968375322,
0.0684455810088901));
#78748=CARTESIAN_POINT('Ctrl Pts',(0.00926203025705925,-0.0323646534831894,
0.0684298982912141));
#78749=CARTESIAN_POINT('Ctrl Pts',(0.00944188834386116,-0.0326943950436604,
0.0683830821789505));
#78750=CARTESIAN_POINT('Ctrl Pts',(0.00936240940793115,-0.0325844576448134,
0.0683649162057989));
#78751=CARTESIAN_POINT('Ctrl Pts',(0.00928254914504506,-0.0324744968375322,
0.0683483927017157));
#78752=CARTESIAN_POINT('Ctrl Pts',(0.009202410168839,-0.0323646534831894,
0.0683335314262551));
#78753=CARTESIAN_POINT('Ctrl Pts',(0.00938630212891412,-0.0326943950436604,
0.0682843335066087));
#78754=CARTESIAN_POINT('Ctrl Pts',(0.0093054622512045,-0.0325844576448134,
0.0682669336156788));
#78755=CARTESIAN_POINT('Ctrl Pts',(0.00922425679405919,-0.0324744968375322,
0.0682512043945413));
#78756=CARTESIAN_POINT('Ctrl Pts',(0.00914279008061875,-0.0323646534831894,
0.0682371645612962));
#78757=CARTESIAN_POINT('',(0.00937377007969489,-0.032677355999134,0.0682816501243087));
#78758=CARTESIAN_POINT('',(0.00938630212891341,-0.0326943950436594,0.0682843335066086));
#78759=CARTESIAN_POINT('Origin',(0.00596353707384605,-0.0326395670796928,
0.084532915372086));
#78760=CARTESIAN_POINT('Ctrl Pts',(0.00937377007899148,-0.032677355998742,
0.0682816501275826));
#78761=CARTESIAN_POINT('Ctrl Pts',(0.00936482153412216,-0.0326267922585947,
0.0683236610884369));
#78762=CARTESIAN_POINT('Ctrl Pts',(0.00935603159574872,-0.0325756109579294,
0.0683649274353469));
#78763=CARTESIAN_POINT('Ctrl Pts',(0.00933876145132211,-0.032471998546237,
0.0684460060209773));
#78764=CARTESIAN_POINT('Ctrl Pts',(0.00933028817185125,-0.0324196091621783,
0.0684857857412956));
#78765=CARTESIAN_POINT('Ctrl Pts',(0.00932197027681829,-0.0323666188837756,
0.0685248359743474));
#78766=CARTESIAN_POINT('',(0.00946918412009023,-0.0326943950436702,0.0684315730082939));
#78767=CARTESIAN_POINT('Origin',(0.00812378219310841,-0.0315241814719618,
0.07415));
#78768=CARTESIAN_POINT('',(0.00937377007968546,-0.0327114338379885,0.0682816501243525));
#78769=CARTESIAN_POINT('',(0.00936123232798897,-0.0326943950436593,0.0682789935135703));
#78770=CARTESIAN_POINT('Origin',(0.0060080083695752,-0.0326395672210718,
0.0845415952384133));
#78771=CARTESIAN_POINT('Origin',(0.00586526092940993,-0.0326395677385031,
0.0845119835878526));
#78772=CARTESIAN_POINT('Origin',(0.00582111352953083,-0.0326395679977111,
0.0845017838739028));
#78773=CARTESIAN_POINT('Ctrl Pts',(0.00947905937737567,-0.0332451089994433,
0.0685606039007953));
#78774=CARTESIAN_POINT('Ctrl Pts',(0.00926825185450242,-0.0329451141710254,
0.0685094887855036));
#78775=CARTESIAN_POINT('Ctrl Pts',(0.00905419301410892,-0.0326442513127493,
0.0684743977672704));
#78776=CARTESIAN_POINT('Ctrl Pts',(0.00923487657364615,-0.0332451089994433,
0.0685069871276474));
#78777=CARTESIAN_POINT('Ctrl Pts',(0.00902204686108887,-0.0329451141710254,
0.0684650815174738));
#78778=CARTESIAN_POINT('Ctrl Pts',(0.00880666527341307,-0.0326442513127493,
0.0684393261607204));
#78779=CARTESIAN_POINT('Ctrl Pts',(0.00923243474560885,-0.0332451089994433,
0.0685064509599159));
#78780=CARTESIAN_POINT('Ctrl Pts',(0.00901958481115473,-0.0329451141710254,
0.0684646374447935));
#78781=CARTESIAN_POINT('Ctrl Pts',(0.00880418999600611,-0.0326442513127493,
0.0684389754446548));
#78782=CARTESIAN_POINT('',(0.00919942996229942,-0.0331951640388616,0.0685001232865986));
#78783=CARTESIAN_POINT('',(0.00896639894183233,-0.0328677532354997,0.0684607010902404));
#78784=CARTESIAN_POINT('Origin',(0.00682186301550851,-0.0326402808281147,
0.0850946833251804));
#78785=CARTESIAN_POINT('Origin',(0.0105858075905475,-0.0326944278779061,
0.0575239786106484));
#78786=CARTESIAN_POINT('',(0.00908985111544921,-0.0326943950436593,0.0684803584031009));
#78787=CARTESIAN_POINT('',(0.00902802551735345,-0.0326943950436694,0.0684712016886965));
#78788=CARTESIAN_POINT('',(0.00932197027683122,-0.0330220786163545,0.0685248359743003));
#78789=CARTESIAN_POINT('Origin',(0.00634268109692061,-0.0326396682763936,
0.085055474472575));
#78790=CARTESIAN_POINT('',(0.00932168725141204,-0.0331951640388587,0.06852616470091));
#78791=CARTESIAN_POINT('Origin',(0.0116199269105786,-0.0331952026560299,
0.057736564890264));
#78792=CARTESIAN_POINT('',(0.00926055860686573,-0.0331951640388701,0.0685131439937643));
#78793=CARTESIAN_POINT('Ctrl Pts',(0.00960282868863939,-0.0330240426238172,
0.0683351550782438));
#78794=CARTESIAN_POINT('Ctrl Pts',(0.00952272353471329,-0.032914277406352,
0.0683147797718027));
#78795=CARTESIAN_POINT('Ctrl Pts',(0.00944215723094673,-0.0328043479726691,
0.0682960503048226));
#78796=CARTESIAN_POINT('Ctrl Pts',(0.00936123232798902,-0.0326943950436593,
0.0682789935135703));
#78797=CARTESIAN_POINT('Ctrl Pts',(0.00950911236822733,-0.0330240426238172,
0.068398860551108));
#78798=CARTESIAN_POINT('Ctrl Pts',(0.00942988481925516,-0.032914277406352,
0.068379776278284));
#78799=CARTESIAN_POINT('Ctrl Pts',(0.00935022324723181,-0.0328043479726691,
0.0683623203460024));
#78800=CARTESIAN_POINT('Ctrl Pts',(0.00927022908870884,-0.0326943950436593,
0.0683465179271179));
#78801=CARTESIAN_POINT('Ctrl Pts',(0.00941539604781526,-0.0330240426238172,
0.0684625660239722));
#78802=CARTESIAN_POINT('Ctrl Pts',(0.00933704610379704,-0.032914277406352,
0.0684447727847653));
#78803=CARTESIAN_POINT('Ctrl Pts',(0.00925828926351689,-0.0328043479726691,
0.0684285903871823));
#78804=CARTESIAN_POINT('Ctrl Pts',(0.00917922584942867,-0.0326943950436593,
0.0684140423406654));
#78805=CARTESIAN_POINT('Ctrl Pts',(0.0093216797274032,-0.0330240426238172,
0.0685262714968365));
#78806=CARTESIAN_POINT('Ctrl Pts',(0.00924420738833892,-0.032914277406352,
0.0685097692912466));
#78807=CARTESIAN_POINT('Ctrl Pts',(0.00916635527980197,-0.0328043479726691,
0.0684948604283621));
#78808=CARTESIAN_POINT('Ctrl Pts',(0.0090882226101485,-0.0326943950436593,
0.068481566754213));
#78809=CARTESIAN_POINT('',(0.00922554172172909,-0.0326943950436694,0.0683796759583456));
#78810=CARTESIAN_POINT('Ctrl Pts',(0.00937377007898977,-0.0327114338383345,
0.068281650127591));
#78811=CARTESIAN_POINT('Ctrl Pts',(0.00936482302256169,-0.032761987683073,
0.0683236541006224));
#78812=CARTESIAN_POINT('Ctrl Pts',(0.00935603381121453,-0.0328131562603818,
0.0683649170343438));
#78813=CARTESIAN_POINT('Ctrl Pts',(0.00933876368263874,-0.0329167375858778,
0.068445995545559));
#78814=CARTESIAN_POINT('Ctrl Pts',(0.00933028964673212,-0.0329691088920621,
0.0684857788171354));
#78815=CARTESIAN_POINT('Ctrl Pts',(0.00932197027681863,-0.0330220786163186,
0.0685248359743463));
#78816=CARTESIAN_POINT('Ctrl Pts',(0.00920053378997214,-0.0331951640388604,
0.0685018246296733));
#78817=CARTESIAN_POINT('Ctrl Pts',(0.00908376138546374,-0.033030642201062,
0.068479563480757));
#78818=CARTESIAN_POINT('Ctrl Pts',(0.00896616868546174,-0.0328657861914645,
0.0684621476801156));
#78819=CARTESIAN_POINT('Ctrl Pts',(0.00919942996230253,-0.0331951640388604,
0.0685001232865992));
#78820=CARTESIAN_POINT('Ctrl Pts',(0.00908262238361688,-0.033030642201062,
0.0684778849586123));
#78821=CARTESIAN_POINT('Ctrl Pts',(0.00896499548270671,-0.0328657861914645,
0.0684604934131856));
#78822=CARTESIAN_POINT('Ctrl Pts',(0.00901550258771073,-0.0331951640388604,
0.0682166337768641));
#78823=CARTESIAN_POINT('Ctrl Pts',(0.00889283404516787,-0.033030642201062,
0.0681981980294236));
#78824=CARTESIAN_POINT('Ctrl Pts',(0.00876950835320592,-0.0328657861914645,
0.0681848480550647));
#78825=CARTESIAN_POINT('',(0.00900282677748922,-0.0331781648281898,0.0682147425822916));
#78826=CARTESIAN_POINT('',(0.00901550258770959,-0.0331951640388588,0.0682166337768639));
#78827=CARTESIAN_POINT('Origin',(0.00728901762487964,-0.0326412092428282,
0.0846479206670505));
#78828=CARTESIAN_POINT('Ctrl Pts',(0.00900282677881569,-0.033178164828644,
0.0682147425835564));
#78829=CARTESIAN_POINT('Ctrl Pts',(0.00899652946141545,-0.0331276811546773,
0.068257261783508));
#78830=CARTESIAN_POINT('Ctrl Pts',(0.00899034588751766,-0.0330765663497778,
0.068299013223338));
#78831=CARTESIAN_POINT('Ctrl Pts',(0.00897820075354882,-0.032973061446299,
0.0683810164308291));
#78832=CARTESIAN_POINT('Ctrl Pts',(0.00897224409454443,-0.0329207133373404,
0.0684212350701986));
#78833=CARTESIAN_POINT('Ctrl Pts',(0.00896639895693368,-0.0328677532289356,
0.0684607010836685));
#78834=CARTESIAN_POINT('',(0.00910746627501451,-0.0331951640388702,0.0683583785317412));
#78835=CARTESIAN_POINT('Origin',(0.00812378219310841,-0.0315241814719618,
0.07415));
#78836=CARTESIAN_POINT('',(0.00900282677662223,-0.0332121607144241,0.0682147425837313));
#78837=CARTESIAN_POINT('',(0.00899014695537356,-0.0331951640388587,0.0682128784669066));
#78838=CARTESIAN_POINT('Origin',(0.00733434671698646,-0.032641365580181,
0.0846467061318248));
#78839=CARTESIAN_POINT('Origin',(0.00587985698336055,-0.0326412098755649,
0.084439217681164));
#78840=CARTESIAN_POINT('Origin',(0.00583682644230013,-0.0326413663090767,
0.0844249134056763));
#78841=CARTESIAN_POINT('Ctrl Pts',(0.00912544447571675,-0.0337436976235975,
0.068486538366723));
#78842=CARTESIAN_POINT('Ctrl Pts',(0.00907450644346596,-0.0336723290703325,
0.0684775292643472));
#78843=CARTESIAN_POINT('Ctrl Pts',(0.00902341460643292,-0.033601104548885,
0.0684694378340787));
#78844=CARTESIAN_POINT('Ctrl Pts',(0.00886028849150909,-0.0333736987606857,
0.0684436035000535));
#78845=CARTESIAN_POINT('Ctrl Pts',(0.00869594867247166,-0.0331450831799191,
0.0684271728560183));
#78846=CARTESIAN_POINT('Ctrl Pts',(0.00887837702421617,-0.0337436976235975,
0.068448358864251));
#78847=CARTESIAN_POINT('Ctrl Pts',(0.00882709559973389,-0.0336723290703325,
0.068441571923978));
#78848=CARTESIAN_POINT('Ctrl Pts',(0.00877570039571424,-0.033601104548885,
0.0684357084728629));
#78849=CARTESIAN_POINT('Ctrl Pts',(0.00861160569009581,-0.0333736987606857,
0.0684169876349365));
#78850=CARTESIAN_POINT('Ctrl Pts',(0.00844670708994683,-0.0331450831799191,
0.06840771434784));
#78851=CARTESIAN_POINT('Ctrl Pts',(0.00887590634970116,-0.0337436976235975,
0.0684479770692262));
#78852=CARTESIAN_POINT('Ctrl Pts',(0.00882462149129657,-0.0336723290703325,
0.0684412123505743));
#78853=CARTESIAN_POINT('Ctrl Pts',(0.00877322325360705,-0.033601104548885,
0.0684353711792508));
#78854=CARTESIAN_POINT('Ctrl Pts',(0.00860911886208168,-0.0333736987606857,
0.0684167214762853));
#78855=CARTESIAN_POINT('Ctrl Pts',(0.00844421467412158,-0.0331450831799191,
0.0684075197627583));
#78856=CARTESIAN_POINT('',(0.00884254872301036,-0.0336938721132548,0.0684437315454411));
#78857=CARTESIAN_POINT('',(0.00860750220198468,-0.0333679869945434,0.0684190192852437));
#78858=CARTESIAN_POINT('Ctrl Pts',(0.0088425487230217,-0.0336938721132647,
0.068443731545442));
#78859=CARTESIAN_POINT('Ctrl Pts',(0.00882027448038528,-0.033662918793393,
0.0684409258624969));
#78860=CARTESIAN_POINT('Ctrl Pts',(0.00879799093318047,-0.0336319952301038,
0.0684382515015221));
#78861=CARTESIAN_POINT('Ctrl Pts',(0.00877570039572543,-0.0336011045488948,
0.0684357084728643));
#78862=CARTESIAN_POINT('Ctrl Pts',(0.00871976580985809,-0.0335235892595452,
0.0684293271437862));
#78863=CARTESIAN_POINT('Ctrl Pts',(0.0086636878005343,-0.0334458668660367,
0.0684237615970615));
#78864=CARTESIAN_POINT('Ctrl Pts',(0.00860750220201912,-0.0333679869945383,
0.0684190192849199));
#78865=CARTESIAN_POINT('Ctrl Pts',(0.00860745794719471,-0.0333679692459108,
0.0684190148598652));
#78866=CARTESIAN_POINT('Ctrl Pts',(0.00860742573596226,-0.0333391895377652,
0.0684194669663275));
#78867=CARTESIAN_POINT('Ctrl Pts',(0.00860740483103624,-0.0333104081066984,
0.0684198060729485));
#78868=CARTESIAN_POINT('Ctrl Pts',(0.00860738268779856,-0.0332532699288407,
0.0684202552784963));
#78869=CARTESIAN_POINT('Ctrl Pts',(0.00860738115929402,-0.0332249176525949,
0.0684203687210718));
#78870=CARTESIAN_POINT('Ctrl Pts',(0.00860738772962057,-0.0331960985150662,
0.0684203729591516));
#78871=CARTESIAN_POINT('Ctrl Pts',(0.00860738783830507,-0.0331956312776463,
0.0684203729981844));
#78872=CARTESIAN_POINT('Ctrl Pts',(0.00860738794916192,-0.0331951640388598,
0.0684203730075412));
#78873=CARTESIAN_POINT('',(0.00873194505769415,-0.0331951640388587,0.0684308861761511));
#78874=CARTESIAN_POINT('',(0.00866966650343826,-0.0331951640388687,0.0684256295918562));
#78875=CARTESIAN_POINT('',(0.0089663989548458,-0.0335216366567732,0.0684607010987125));
#78876=CARTESIAN_POINT('Origin',(0.00773075325147134,-0.0326434571526403,
0.0850692484370686));
#78877=CARTESIAN_POINT('',(0.00896619991923771,-0.0336938721132327,0.0684620449742721));
#78878=CARTESIAN_POINT('Origin',(0.0105661453900854,-0.0336938867896312,
0.0576593136321265));
#78879=CARTESIAN_POINT('',(0.00890437432113403,-0.0336938721132538,0.0684528882598666));
#78880=CARTESIAN_POINT('Ctrl Pts',(0.00923479205017076,-0.0335235895815172,
0.0682537590706003));
#78881=CARTESIAN_POINT('Ctrl Pts',(0.00915361868514744,-0.0334144449262748,
0.0682384638325407));
#78882=CARTESIAN_POINT('Ctrl Pts',(0.00907203607365478,-0.0333049234473147,
0.0682248280027372));
#78883=CARTESIAN_POINT('Ctrl Pts',(0.00899014695537373,-0.0331951640388587,
0.0682128784669064));
#78884=CARTESIAN_POINT('Ctrl Pts',(0.00914526064112622,-0.0335235895815172,
0.0683232234447813));
#78885=CARTESIAN_POINT('Ctrl Pts',(0.00906504358997627,-0.0334144449262748,
0.0683091607828383));
#78886=CARTESIAN_POINT('Ctrl Pts',(0.0089844438551407,-0.0333049234473147,
0.0682967391885072));
#78887=CARTESIAN_POINT('Ctrl Pts',(0.00890356306014734,-0.0331951640388587,
0.0682859838810239));
#78888=CARTESIAN_POINT('Ctrl Pts',(0.00905572923208167,-0.0335235895815172,
0.0683926878189622));
#78889=CARTESIAN_POINT('Ctrl Pts',(0.00897646849480509,-0.0334144449262748,
0.0683798577331359));
#78890=CARTESIAN_POINT('Ctrl Pts',(0.00889685163662663,-0.0333049234473147,
0.0683686503742772));
#78891=CARTESIAN_POINT('Ctrl Pts',(0.00881697916492096,-0.0331951640388587,
0.0683590892951414));
#78892=CARTESIAN_POINT('Ctrl Pts',(0.00896619782303712,-0.0335235895815172,
0.0684621521931432));
#78893=CARTESIAN_POINT('Ctrl Pts',(0.00888789339963391,-0.0334144449262748,
0.0684505546834335));
#78894=CARTESIAN_POINT('Ctrl Pts',(0.00880925941811255,-0.0333049234473147,
0.0684405615600472));
#78895=CARTESIAN_POINT('Ctrl Pts',(0.00873039526969457,-0.0331951640388587,
0.0684321947092588));
#78896=CARTESIAN_POINT('',(0.00886104600654386,-0.0331951640388687,0.0683218823215388));
#78897=CARTESIAN_POINT('Ctrl Pts',(0.00900282677615849,-0.0332121607145997,
0.0682147425868254));
#78898=CARTESIAN_POINT('Ctrl Pts',(0.00899654004050732,-0.0332625444109542,
0.0682571902568275));
#78899=CARTESIAN_POINT('Ctrl Pts',(0.00899036163517683,-0.0333135300746364,
0.0682989064868647));
#78900=CARTESIAN_POINT('Ctrl Pts',(0.00897821658080767,-0.0334167203140643,
0.0683809091808895));
#78901=CARTESIAN_POINT('Ctrl Pts',(0.00897225463565744,-0.0334688847587331,
0.0684211638844984));
#78902=CARTESIAN_POINT('Ctrl Pts',(0.00896639895457182,-0.0335216366562408,
0.0684607010993822));
#78903=CARTESIAN_POINT('Ctrl Pts',(0.00884314451846207,-0.0336938721132389,
0.0684445345041274));
#78904=CARTESIAN_POINT('Ctrl Pts',(0.00880974853564058,-0.0336474569764957,
0.0684403238377273));
#78905=CARTESIAN_POINT('Ctrl Pts',(0.0087763055499666,-0.033601104548885,
0.0684365044019894));
#78906=CARTESIAN_POINT('Ctrl Pts',(0.0086916355992645,-0.0334837508592656,
0.0684268344688444));
#78907=CARTESIAN_POINT('Ctrl Pts',(0.0086067162891965,-0.0333660264659097,
0.0684196777282104));
#78908=CARTESIAN_POINT('Ctrl Pts',(0.00884254872303063,-0.0336938721132389,
0.0684437315454438));
#78909=CARTESIAN_POINT('Ctrl Pts',(0.00880914804022551,-0.0336474569764957,
0.0684395243664322));
#78910=CARTESIAN_POINT('Ctrl Pts',(0.00877570039571424,-0.033601104548885,
0.0684357084728629));
#78911=CARTESIAN_POINT('Ctrl Pts',(0.00869101864990724,-0.0334837508592656,
0.0684260475076745));
#78912=CARTESIAN_POINT('Ctrl Pts',(0.00860608781565303,-0.0333660264659097,
0.0684189000805725));
#78913=CARTESIAN_POINT('Ctrl Pts',(0.00863997564415778,-0.0336938721132389,
0.0681707220456216));
#78914=CARTESIAN_POINT('Ctrl Pts',(0.00860497694615604,-0.0336474569764957,
0.0681677005940614));
#78915=CARTESIAN_POINT('Ctrl Pts',(0.00856994527638209,-0.033601104548885,
0.0681650890534824));
#78916=CARTESIAN_POINT('Ctrl Pts',(0.00848125314280023,-0.0334837508592656,
0.0681584772331672));
#78917=CARTESIAN_POINT('Ctrl Pts',(0.00839240403432243,-0.0333660264659097,
0.0681544964480833));
#78918=CARTESIAN_POINT('',(0.00862841428638208,-0.0336769361243754,0.0681712587904779));
#78919=CARTESIAN_POINT('',(0.00864118383349715,-0.033693872113232,0.0681723503329048));
#78920=CARTESIAN_POINT('Ctrl Pts',(0.00862841428638182,-0.0336769361243751,
0.0681712587904778));
#78921=CARTESIAN_POINT('Ctrl Pts',(0.00863054289791591,-0.0336797586669902,
0.0681714384546674));
#78922=CARTESIAN_POINT('Ctrl Pts',(0.00863267133299573,-0.0336825812712599,
0.0681716192488361));
#78923=CARTESIAN_POINT('Ctrl Pts',(0.00863692785609007,-0.033688226610724,
0.0681719830971155));
#78924=CARTESIAN_POINT('Ctrl Pts',(0.00863905594407222,-0.0336910493458711,
0.0681721661512459));
#78925=CARTESIAN_POINT('Ctrl Pts',(0.0086411838335001,-0.0336938721132293,
0.0681723503329129));
#78926=CARTESIAN_POINT('Ctrl Pts',(0.00862841428638209,-0.0336769361243754,
0.0681712587904779));
#78927=CARTESIAN_POINT('Ctrl Pts',(0.00862488911540854,-0.0336279007516212,
0.068213024039362));
#78928=CARTESIAN_POINT('Ctrl Pts',(0.00862131375149712,-0.0335767878632074,
0.0682553839602703));
#78929=CARTESIAN_POINT('Ctrl Pts',(0.00861430704219723,-0.0334733198857322,
0.0683383975105235));
#78930=CARTESIAN_POINT('Ctrl Pts',(0.0086108715253995,-0.0334209645014077,
0.0683791005615683));
#78931=CARTESIAN_POINT('Ctrl Pts',(0.00860750220923624,-0.0333679869844681,
0.0684190192858466));
#78932=CARTESIAN_POINT('',(0.00874186627826375,-0.0336938721132534,0.068308040939183));
#78933=CARTESIAN_POINT('Origin',(0.00812378219310841,-0.0315241814719618,
0.07415));
#78934=CARTESIAN_POINT('',(0.00862841428627746,-0.033710812065556,0.0681712587917762));
#78935=CARTESIAN_POINT('',(0.00861564243684592,-0.0336938721132327,0.0681701945265211));
#78936=CARTESIAN_POINT('Origin',(0.00613870297800496,-0.0345562519032924,
0.0843805051160357));
#78937=CARTESIAN_POINT('Ctrl Pts',(0.00861564243684644,-0.0336938721132331,
0.0681701945265203));
#78938=CARTESIAN_POINT('Ctrl Pts',(0.00861777111120703,-0.0336910493226405,
0.0681703696175487));
#78939=CARTESIAN_POINT('Ctrl Pts',(0.00861989976603181,-0.0336882265991082,
0.0681705458512997));
#78940=CARTESIAN_POINT('Ctrl Pts',(0.00862415704786373,-0.0336825812712695,
0.0681709006056672));
#78941=CARTESIAN_POINT('Ctrl Pts',(0.00862628567484466,-0.033679758666995,
0.068171079126288));
#78942=CARTESIAN_POINT('Ctrl Pts',(0.00862841428638236,-0.0336769361243751,
0.0681712587904779));
#78943=CARTESIAN_POINT('Origin',(0.008365994683725,-0.0345562518554779,
0.0845684961448049));
#78944=CARTESIAN_POINT('Ctrl Pts',(0.00876790753850355,-0.0342436276873911,
0.0684348248023863));
#78945=CARTESIAN_POINT('Ctrl Pts',(0.00855235615251585,-0.033943005420181,
0.0684105312144997));
#78946=CARTESIAN_POINT('Ctrl Pts',(0.00833558723283896,-0.0336441434784052,
0.0684025428557366));
#78947=CARTESIAN_POINT('Ctrl Pts',(0.00851893051022238,-0.0342436276873911,
0.0684122318966795));
#78948=CARTESIAN_POINT('Ctrl Pts',(0.00830252701874881,-0.033943005420181,
0.0683973286322161));
#78949=CARTESIAN_POINT('Ctrl Pts',(0.0080856157319643,-0.0336441434784052,
0.0683987681040282));
#78950=CARTESIAN_POINT('Ctrl Pts',(0.00851644073993956,-0.0342436276873911,
0.0684120059676224));
#78951=CARTESIAN_POINT('Ctrl Pts',(0.00830002872741114,-0.033943005420181,
0.0683971966063933));
#78952=CARTESIAN_POINT('Ctrl Pts',(0.00808311601695554,-0.0336441434784052,
0.0683987303565111));
#78953=CARTESIAN_POINT('',(0.00848283084063066,-0.0341934961088741,0.0684098598389313));
#78954=CARTESIAN_POINT('',(0.00824669644070164,-0.0338664212863613,0.0683999550358944));
#78955=CARTESIAN_POINT('Origin',(0.00692997697895972,-0.034561072040625,
0.0850724463328746));
#78956=CARTESIAN_POINT('Origin',(0.00848102226634798,-0.0336938005072915,
0.0574362049537827));
#78957=CARTESIAN_POINT('',(0.00837163885895573,-0.0336938721132327,0.0684039846786494));
#78958=CARTESIAN_POINT('',(0.00830915313354104,-0.0336938721132427,0.0684026489698008));
#78959=CARTESIAN_POINT('',(0.00860750220924159,-0.0340203938281605,0.0684190192858471));
#78960=CARTESIAN_POINT('Origin',(0.00646348128806438,-0.0345589643244434,
0.0849544696214529));
#78961=CARTESIAN_POINT('',(0.00860738794916238,-0.034193496108874,0.0684203730075413));
#78962=CARTESIAN_POINT('Origin',(0.00953418318736831,-0.0341934220717554,
0.0574399691515785));
#78963=CARTESIAN_POINT('',(0.00854510939490652,-0.0341934961088841,0.0684151164232464));
#78964=CARTESIAN_POINT('Ctrl Pts',(0.00886237441018436,-0.0340223579322396,
0.0681956334059029));
#78965=CARTESIAN_POINT('Ctrl Pts',(0.00878024816521174,-0.0339125849573574,
0.0681854462929001));
#78966=CARTESIAN_POINT('Ctrl Pts',(0.00869796877983302,-0.0338030433565231,
0.0681769661606995));
#78967=CARTESIAN_POINT('Ctrl Pts',(0.00861564243684641,-0.0336938721132327,
0.0681701945265206));
#78968=CARTESIAN_POINT('Ctrl Pts',(0.00877738131658268,-0.0340223579322397,
0.0682705824143705));
#78969=CARTESIAN_POINT('Ctrl Pts',(0.00869628881391204,-0.0339125849573575,
0.0682615675777997));
#78970=CARTESIAN_POINT('Ctrl Pts',(0.00861506670783471,-0.0338030433565231,
0.0682542375022226));
#78971=CARTESIAN_POINT('Ctrl Pts',(0.00853381969869298,-0.0336938721132327,
0.0682485923539863));
#78972=CARTESIAN_POINT('Ctrl Pts',(0.00869238822298099,-0.0340223579322397,
0.0683455314228382));
#78973=CARTESIAN_POINT('Ctrl Pts',(0.00861232946261234,-0.0339125849573575,
0.0683376888626994));
#78974=CARTESIAN_POINT('Ctrl Pts',(0.0085321646358364,-0.0338030433565231,
0.0683315088437457));
#78975=CARTESIAN_POINT('Ctrl Pts',(0.00845199696053956,-0.0336938721132327,
0.0683269901814519));
#78976=CARTESIAN_POINT('Ctrl Pts',(0.0086073951293793,-0.0340223579322397,
0.0684204804313058));
#78977=CARTESIAN_POINT('Ctrl Pts',(0.00852837011131264,-0.0339125849573575,
0.0684138101475991));
#78978=CARTESIAN_POINT('Ctrl Pts',(0.00844926256383809,-0.0338030433565231,
0.0684087801852688));
#78979=CARTESIAN_POINT('Ctrl Pts',(0.00837017422238613,-0.0336938721132327,
0.0684053880089176));
#78980=CARTESIAN_POINT('',(0.00849364064791083,-0.0336938721132427,0.0682870896025953));
#78981=CARTESIAN_POINT('Ctrl Pts',(0.00862841428596992,-0.0337108120662706,
0.068171258795362));
#78982=CARTESIAN_POINT('Ctrl Pts',(0.0086247978185304,-0.0337611408994095,
0.0682141056994763));
#78983=CARTESIAN_POINT('Ctrl Pts',(0.00862124734359817,-0.0338121088780875,
0.0682561707426506));
#78984=CARTESIAN_POINT('Ctrl Pts',(0.00861427514431629,-0.0339153382773245,
0.0683387754277732));
#78985=CARTESIAN_POINT('Ctrl Pts',(0.00861085636963837,-0.0339675558473123,
0.0683792801228283));
#78986=CARTESIAN_POINT('Ctrl Pts',(0.00860750220923303,-0.0340203938281304,
0.0684190192858864));
#78987=CARTESIAN_POINT('Ctrl Pts',(0.00848413925925491,-0.0341934961088741,
0.06841140949134));
#78988=CARTESIAN_POINT('Ctrl Pts',(0.00836549842141796,-0.0340287516182428,
0.068403959392891));
#78989=CARTESIAN_POINT('Ctrl Pts',(0.00824665104168689,-0.0338644633275951,
0.0684014191762442));
#78990=CARTESIAN_POINT('Ctrl Pts',(0.00848283084063074,-0.0341934961088741,
0.0684098598389314));
#78991=CARTESIAN_POINT('Ctrl Pts',(0.00836415796495106,-0.0340287516182428,
0.0684024367910067));
#78992=CARTESIAN_POINT('Ctrl Pts',(0.0082452796927717,-0.033864463327595,
0.0683999249259183));
#78993=CARTESIAN_POINT('Ctrl Pts',(0.00826482313138735,-0.0341934961088741,
0.0681516579412533));
#78994=CARTESIAN_POINT('Ctrl Pts',(0.0081408121348877,-0.0340287516182428,
0.0681487420309681));
#78995=CARTESIAN_POINT('Ctrl Pts',(0.00801678658662852,-0.033864463327595,
0.0681509540808397));
#78996=CARTESIAN_POINT('',(0.00825201024437053,-0.0341764758832384,0.0681513703600372));
#78997=CARTESIAN_POINT('',(0.00826482313138735,-0.034193496108874,0.0681516579412533));
#78998=CARTESIAN_POINT('Origin',(0.00738616690623692,-0.0345621026576131,
0.0846943946009223));
#78999=CARTESIAN_POINT('Ctrl Pts',(0.0082520102459485,-0.0341764758837473,
0.0681513703609318));
#79000=CARTESIAN_POINT('Ctrl Pts',(0.0082510929081322,-0.0341260050040342,
0.0681942849352783));
#79001=CARTESIAN_POINT('Ctrl Pts',(0.00825019155400999,-0.0340749269147992,
0.0682364535538986));
#79002=CARTESIAN_POINT('Ctrl Pts',(0.00824841993121393,-0.0339715436305663,
0.0683193315568962));
#79003=CARTESIAN_POINT('Ctrl Pts',(0.00824755032866946,-0.0339192778235215,
0.0683600094991655));
#79004=CARTESIAN_POINT('Ctrl Pts',(0.00824669644189481,-0.0338664212853738,
0.0683999550346134));
#79005=CARTESIAN_POINT('',(0.00837382698601901,-0.0341934961088841,0.0682807588901023));
#79006=CARTESIAN_POINT('Origin',(0.00812378219310841,-0.0315241814719618,
0.07415));
#79007=CARTESIAN_POINT('',(0.00825201024351351,-0.0342105180190385,0.0681513703607559));
#79008=CARTESIAN_POINT('',(0.00823919677064574,-0.0341934961088739,0.0681511101464263));
#79009=CARTESIAN_POINT('Origin',(0.00743106824044017,-0.0345621711153071,
0.0847005881547815));
#79010=CARTESIAN_POINT('Origin',(0.00841013196553991,-0.0345621034777229,
0.0847162844815517));
#79011=CARTESIAN_POINT('Origin',(0.00836500708698931,-0.0345621719574124,
0.0847205499687025));
#79012=CARTESIAN_POINT('Ctrl Pts',(0.00837313852628012,-0.0346945769586966,
0.0684040167358742));
#79013=CARTESIAN_POINT('Ctrl Pts',(0.00825278660624681,-0.0345275153362944,
0.0683987938676391));
#79014=CARTESIAN_POINT('Ctrl Pts',(0.00813223930264381,-0.0343603235965185,
0.0683973546056114));
#79015=CARTESIAN_POINT('Ctrl Pts',(0.00801185320414964,-0.034193496108874,
0.0683996979075932));
#79016=CARTESIAN_POINT('Ctrl Pts',(0.00828932433605479,-0.0346945769586966,
0.0684022251049759));
#79017=CARTESIAN_POINT('Ctrl Pts',(0.00816893488959499,-0.0345275153362944,
0.0683987577585124));
#79018=CARTESIAN_POINT('Ctrl Pts',(0.00804840525940311,-0.0343603235965185,
0.0683990756524959));
#79019=CARTESIAN_POINT('Ctrl Pts',(0.00792809190464829,-0.034193496108874,
0.0684031725486176));
#79020=CARTESIAN_POINT('Ctrl Pts',(0.00820551014582946,-0.0346945769586966,
0.0684004334740784));
#79021=CARTESIAN_POINT('Ctrl Pts',(0.00808508317294308,-0.0345275153362944,
0.0683987216493865));
#79022=CARTESIAN_POINT('Ctrl Pts',(0.00796457121616235,-0.0343603235965185,
0.0684007966993806));
#79023=CARTESIAN_POINT('Ctrl Pts',(0.00784433060514703,-0.034193496108874,
0.0684066471896415));
#79024=CARTESIAN_POINT('Ctrl Pts',(0.00812169595560415,-0.0346945769586966,
0.0683986418431793));
#79025=CARTESIAN_POINT('Ctrl Pts',(0.00800123145629136,-0.0345275153362944,
0.0683986855402592));
#79026=CARTESIAN_POINT('Ctrl Pts',(0.00788073717292172,-0.0343603235965185,
0.0684025177462647));
#79027=CARTESIAN_POINT('Ctrl Pts',(0.0077605693056456,-0.034193496108874,
0.0684101218306662));
#79028=CARTESIAN_POINT('',(0.00812169595725133,-0.0346945769586966,0.0683986418432147));
#79029=CARTESIAN_POINT('',(0.0078854055874641,-0.0343667727836481,0.0684035835867093));
#79030=CARTESIAN_POINT('Origin',(0.00831075887806156,-0.0345626474182898,
0.0852111818206586));
#79031=CARTESIAN_POINT('Origin',(0.00742731571724248,-0.0341934771023922,
0.0573609022276176));
#79032=CARTESIAN_POINT('',(0.00801035448319213,-0.034193496108874,0.0683997600785164));
#79033=CARTESIAN_POINT('',(0.0079479081892299,-0.0341934961088839,0.0684023505165466));
#79034=CARTESIAN_POINT('',(0.00824669644183473,-0.0345211942962704,0.0683999550360667));
#79035=CARTESIAN_POINT('Origin',(0.00783013057141495,-0.0345625596119596,
0.0851975826479658));
#79036=CARTESIAN_POINT('',(0.00824666740810637,-0.0346945769586885,0.0684013132609321));
#79037=CARTESIAN_POINT('Origin',(0.00848311153581144,-0.034694568585393,
0.0573402731026649));
#79038=CARTESIAN_POINT('',(0.00818418168268885,-0.0346945769587026,0.0683999775520834));
#79039=CARTESIAN_POINT('Ctrl Pts',(0.00848703823483649,-0.0345231616327842,
0.0681610063409479));
#79040=CARTESIAN_POINT('Ctrl Pts',(0.00840448838907507,-0.0344132092796988,
0.0681559993678363));
#79041=CARTESIAN_POINT('Ctrl Pts',(0.00832183923721686,-0.0343032738558979,
0.0681527001315066));
#79042=CARTESIAN_POINT('Ctrl Pts',(0.0082391967706457,-0.0341934961088739,
0.0681511101464262));
#79043=CARTESIAN_POINT('Ctrl Pts',(0.00840691909202334,-0.0345231616327842,
0.0682411440916858));
#79044=CARTESIAN_POINT('Ctrl Pts',(0.00832547383233092,-0.0344132092796988,
0.0682372414481591));
#79045=CARTESIAN_POINT('Ctrl Pts',(0.00824395205173651,-0.0343032738558979,
0.0682350236369445));
#79046=CARTESIAN_POINT('Ctrl Pts',(0.00816245826184278,-0.0341934961088739,
0.0682344908240748));
#79047=CARTESIAN_POINT('Ctrl Pts',(0.00832679994921019,-0.0345231616327842,
0.0683212818424236));
#79048=CARTESIAN_POINT('Ctrl Pts',(0.00824645927558676,-0.0344132092796988,
0.0683184835284819));
#79049=CARTESIAN_POINT('Ctrl Pts',(0.00816606486625616,-0.0343032738558979,
0.0683173471423824));
#79050=CARTESIAN_POINT('Ctrl Pts',(0.00808571975303985,-0.0341934961088739,
0.0683178715017235));
#79051=CARTESIAN_POINT('Ctrl Pts',(0.00824668080639703,-0.0345231616327842,
0.0684014195931615));
#79052=CARTESIAN_POINT('Ctrl Pts',(0.0081674447188426,-0.0344132092796988,
0.0683997256088047));
#79053=CARTESIAN_POINT('Ctrl Pts',(0.00808817768077582,-0.0343032738558979,
0.0683996706478203));
#79054=CARTESIAN_POINT('Ctrl Pts',(0.00800898124423693,-0.0341934961088739,
0.0684012521793721));
#79055=CARTESIAN_POINT('',(0.00812477562692893,-0.0341934961088839,0.0682754351124813));
#79056=CARTESIAN_POINT('Ctrl Pts',(0.0082520102434348,-0.0342105180195408,
0.0681513703642054));
#79057=CARTESIAN_POINT('Ctrl Pts',(0.0082510918606096,-0.0342610556241025,
0.0681943331825463));
#79058=CARTESIAN_POINT('Ctrl Pts',(0.00825018995768933,-0.034312218986956,
0.0682365250553266));
#79059=CARTESIAN_POINT('Ctrl Pts',(0.00824841832106623,-0.0344158119695194,
0.0683194038944269));
#79060=CARTESIAN_POINT('Ctrl Pts',(0.0082475493119773,-0.0344681990450092,
0.0683600569626224));
#79061=CARTESIAN_POINT('Ctrl Pts',(0.00824669644182474,-0.0345211942962516,
0.0683999550360913));
#79062=CARTESIAN_POINT('Ctrl Pts',(0.00812309875368016,-0.0346945769586932,
0.068400105922614));
#79063=CARTESIAN_POINT('Ctrl Pts',(0.008004223762275,-0.0345296777079064,
0.0684001200522406));
#79064=CARTESIAN_POINT('Ctrl Pts',(0.00788545093205472,-0.0343648066255586,
0.0684050473824189));
#79065=CARTESIAN_POINT('Ctrl Pts',(0.00812169595726038,-0.0346945769586932,
0.0683986418432148));
#79066=CARTESIAN_POINT('Ctrl Pts',(0.00800279069704963,-0.0345296777079064,
0.0683986849746647));
#79067=CARTESIAN_POINT('Ctrl Pts',(0.00788398882256008,-0.0343648066255586,
0.0684036425329222));
#79068=CARTESIAN_POINT('Ctrl Pts',(0.00788790580513354,-0.0346945769586932,
0.0681546382653258));
#79069=CARTESIAN_POINT('Ctrl Pts',(0.0077639559436077,-0.0345296777079064,
0.0681595148427402));
#79070=CARTESIAN_POINT('Ctrl Pts',(0.00764031354911486,-0.0343648066255586,
0.0681695102148508));
#79071=CARTESIAN_POINT('',(0.0078751001439325,-0.0346775396664968,0.0681551557791907));
#79072=CARTESIAN_POINT('',(0.00788790580513014,-0.0346945769586886,0.0681546382653259));
#79073=CARTESIAN_POINT('Origin',(0.0087157432631322,-0.0345626617603281,
0.0847354518265223));
#79074=CARTESIAN_POINT('Ctrl Pts',(0.00787510014551747,-0.0346775396670097,
0.0681551557800743));
#79075=CARTESIAN_POINT('Ctrl Pts',(0.00787688064661579,-0.0346269749928753,
0.0681980770500881));
#79076=CARTESIAN_POINT('Ctrl Pts',(0.00787862954012581,-0.0345757902891929,
0.0682402355118727));
#79077=CARTESIAN_POINT('Ctrl Pts',(0.00788206538008038,-0.0344721681090186,
0.0683230615461074));
#79078=CARTESIAN_POINT('Ctrl Pts',(0.00788375097388189,-0.0344197714292427,
0.068363696647088));
#79079=CARTESIAN_POINT('Ctrl Pts',(0.00788540558804893,-0.0343667727834134,
0.0684035835863732));
#79080=CARTESIAN_POINT('',(0.00800480088120074,-0.0346945769587026,0.0682766400542803));
#79081=CARTESIAN_POINT('Origin',(0.00812378219310841,-0.0315241814719618,
0.07415));
#79082=CARTESIAN_POINT('',(0.00787510014324329,-0.0347116136489629,0.0681551557803994));
#79083=CARTESIAN_POINT('',(0.00786229561583599,-0.0346945769586885,0.0681557006439514));
#79084=CARTESIAN_POINT('Origin',(0.00876090076159747,-0.0345626690069087,
0.0847317081345435));
#79085=CARTESIAN_POINT('Origin',(0.00841057271511297,-0.0345626625822889,
0.0847481130835297));
#79086=CARTESIAN_POINT('Origin',(0.00836526010754044,-0.0345626698054885,
0.0847481183952486));
#79087=CARTESIAN_POINT('Ctrl Pts',(0.00804897197365624,-0.0352450361874068,
0.0683990725915997));
#79088=CARTESIAN_POINT('Ctrl Pts',(0.00783207218728833,-0.0349452760959492,
0.0684018941053252));
#79089=CARTESIAN_POINT('Ctrl Pts',(0.00761600111833985,-0.0346444289841739,
0.068421045382818));
#79090=CARTESIAN_POINT('Ctrl Pts',(0.00804644853620733,-0.0352450361874068,
0.0683991614084979));
#79091=CARTESIAN_POINT('Ctrl Pts',(0.00782955209962371,-0.0349452760959492,
0.0684020780952285));
#79092=CARTESIAN_POINT('Ctrl Pts',(0.00761349153976328,-0.0346444289841739,
0.0684213240230304));
#79093=CARTESIAN_POINT('Ctrl Pts',(0.00779660324423548,-0.0352450361874068,
0.0684079551607973));
#79094=CARTESIAN_POINT('Ctrl Pts',(0.00758003846946215,-0.0349452760959492,
0.06842029491734));
#79095=CARTESIAN_POINT('Ctrl Pts',(0.00736501841337003,-0.0346444289841739,
0.0684489121628801));
#79096=CARTESIAN_POINT('Ctrl Pts',(0.00779410479131576,-0.0352450361874068,
0.0684080430983203));
#79097=CARTESIAN_POINT('Ctrl Pts',(0.00757754333316053,-0.0349452760959492,
0.0684204770855611));
#79098=CARTESIAN_POINT('Ctrl Pts',(0.0073625336821061,-0.0346444289841739,
0.0684491880442786));
#79099=CARTESIAN_POINT('',(0.00776060145150039,-0.0351951634053307,0.0684101174183231));
#79100=CARTESIAN_POINT('',(0.00752505549724609,-0.0348678972935789,0.0684298906178893));
#79101=CARTESIAN_POINT('Origin',(0.00968827090518434,-0.0345636767883711,
0.0850440762627313));
#79102=CARTESIAN_POINT('Origin',(0.0063747315425424,-0.0346946199326766,
0.0574400884190866));
#79103=CARTESIAN_POINT('',(0.00764951777273953,-0.0346945769330288,0.0684182290470105));
#79104=CARTESIAN_POINT('',(0.0075873573485229,-0.0346945769458128,0.0684247354091863));
#79105=CARTESIAN_POINT('',(0.00788540558804949,-0.0350221583435275,0.0684035835867768));
#79106=CARTESIAN_POINT('Origin',(0.00921621127826716,-0.0345628458713778,
0.0851351976181047));
#79107=CARTESIAN_POINT('',(0.00788545987515186,-0.035195136029876,0.0684048192832028));
#79108=CARTESIAN_POINT('Origin',(0.00742875437489389,-0.0351951838366844,
0.0573953113939836));
#79109=CARTESIAN_POINT('',(0.00776056930729773,-0.035195137132875,0.0684101218304813));
#79110=CARTESIAN_POINT('Ctrl Pts',(0.00811026844799484,-0.0350241211494342,
0.06815001521846));
#79111=CARTESIAN_POINT('Ctrl Pts',(0.00802762111771867,-0.0349144232818961,
0.068150201364758));
#79112=CARTESIAN_POINT('Ctrl Pts',(0.00794492816680862,-0.0348045283579411,
0.0681520960018471));
#79113=CARTESIAN_POINT('Ctrl Pts',(0.00786229560473368,-0.0346945769439157,
0.0681557006444357));
#79114=CARTESIAN_POINT('Ctrl Pts',(0.00803533929009677,-0.0350241211494342,
0.0682350255890013));
#79115=CARTESIAN_POINT('Ctrl Pts',(0.0079538629428192,-0.0349144232818961,
0.0682362438537273));
#79116=CARTESIAN_POINT('Ctrl Pts',(0.00787236301042293,-0.0348045283579411,
0.0682391470219615));
#79117=CARTESIAN_POINT('Ctrl Pts',(0.00779094402234273,-0.0346945769439157,
0.068243735259748));
#79118=CARTESIAN_POINT('Ctrl Pts',(0.00796041013219871,-0.0350241211494342,
0.0683200359595427));
#79119=CARTESIAN_POINT('Ctrl Pts',(0.00788010476791974,-0.0349144232818961,
0.0683222863426966));
#79120=CARTESIAN_POINT('Ctrl Pts',(0.00779979785403725,-0.0348045283579411,
0.068326198042076));
#79121=CARTESIAN_POINT('Ctrl Pts',(0.00771959243995177,-0.0346945769439157,
0.0683317698750604));
#79122=CARTESIAN_POINT('Ctrl Pts',(0.00788548097430065,-0.0350241211494342,
0.0684050463300841));
#79123=CARTESIAN_POINT('Ctrl Pts',(0.00780634659302027,-0.0349144232818961,
0.0684083288316659));
#79124=CARTESIAN_POINT('Ctrl Pts',(0.00772723269765157,-0.0348045283579411,
0.0684132490621905));
#79125=CARTESIAN_POINT('Ctrl Pts',(0.00764824085756082,-0.0346945769439157,
0.0684198044903728));
#79126=CARTESIAN_POINT('',(0.00775590669457766,-0.0346945769458128,0.0682869648453788));
#79127=CARTESIAN_POINT('Ctrl Pts',(0.00787510014337482,-0.0347116136492813,
0.0681551557836804));
#79128=CARTESIAN_POINT('Ctrl Pts',(0.0078768799245296,-0.0347621546532016,
0.0681980600092714));
#79129=CARTESIAN_POINT('Ctrl Pts',(0.00787862841232228,-0.0348133084096431,
0.0682402098626383));
#79130=CARTESIAN_POINT('Ctrl Pts',(0.00788206426041952,-0.0349168561544575,
0.0683230360019436));
#79131=CARTESIAN_POINT('Ctrl Pts',(0.00788375025789453,-0.0349692089015915,
0.0683636794348842));
#79132=CARTESIAN_POINT('Ctrl Pts',(0.00788540558803104,-0.0350221583435,
0.0684035835868141));
#79133=CARTESIAN_POINT('Ctrl Pts',(0.00776164580514364,-0.0351951371254927,
0.0684111125737866));
#79134=CARTESIAN_POINT('Ctrl Pts',(0.00764299790862322,-0.0350307338985342,
0.0684185995163758));
#79135=CARTESIAN_POINT('Ctrl Pts',(0.00752476083944801,-0.0348659306906632,
0.0684309839069909));
#79136=CARTESIAN_POINT('Ctrl Pts',(0.00776056930730941,-0.0351951371254927,
0.068410121830597));
#79137=CARTESIAN_POINT('Ctrl Pts',(0.00764190092779522,-0.0350307338985342,
0.0684176310291034));
#79138=CARTESIAN_POINT('Ctrl Pts',(0.0075236443129899,-0.0348659306906632,
0.0684300385032024));
#79139=CARTESIAN_POINT('Ctrl Pts',(0.00758014714814886,-0.0351951371254927,
0.0682440722392592));
#79140=CARTESIAN_POINT('Ctrl Pts',(0.00745804579752596,-0.0350307338985342,
0.0682553115526956));
#79141=CARTESIAN_POINT('Ctrl Pts',(0.00733651331474012,-0.0348659306906632,
0.0682715878427632));
#79142=CARTESIAN_POINT('Origin',(0.00697142147160639,-0.0308609188509344,
0.0631406035306795));
#79143=CARTESIAN_POINT('',(0.00768190931389185,-0.0351951371254927,0.068337727952692));
#79144=CARTESIAN_POINT('Origin',(0.00836523134608927,-0.0351840467441094,
0.0750968093562229));
#79145=CARTESIAN_POINT('Origin',(0.00609052858765088,-0.0352322613840174,
0.062358635348931));
#79146=CARTESIAN_POINT('',(0.00729024535054908,-0.0351951142564659,0.0684593909890488));
#79147=CARTESIAN_POINT('',(0.00716729424068905,-0.0351951372916786,0.0684801119237786));
#79148=CARTESIAN_POINT('Origin',(0.0078674724186718,-0.0352875123591893,
0.0743743206838547));
#79149=CARTESIAN_POINT('Origin',(0.0156243487284059,-0.0298325076521828,
0.0743415513817782));
#79150=CARTESIAN_POINT('Origin',(0.00994290486824038,-0.0338733259208977,
0.0659684674412729));
#79151=CARTESIAN_POINT('Ctrl Pts',(0.0107946224263853,-0.0321934096636941,
0.0690564012531785));
#79152=CARTESIAN_POINT('Ctrl Pts',(0.01070344943444,-0.0320508460844559,
0.0690085944848839));
#79153=CARTESIAN_POINT('Ctrl Pts',(0.0106110607136982,-0.0319086045663538,
0.0689632734014443));
#79154=CARTESIAN_POINT('Ctrl Pts',(0.0105176632270694,-0.0317669892868597,
0.0689205192100429));
#79155=CARTESIAN_POINT('Ctrl Pts',(0.0107195350790821,-0.0321934096636941,
0.069019087409866));
#79156=CARTESIAN_POINT('Ctrl Pts',(0.0106276941871107,-0.0320508460844559,
0.0689726246693307));
#79157=CARTESIAN_POINT('Ctrl Pts',(0.0105346741813155,-0.0319086045663538,
0.068928664545405));
#79158=CARTESIAN_POINT('Ctrl Pts',(0.0104406831426264,-0.0317669892868597,
0.0688872852029833));
#79159=CARTESIAN_POINT('Ctrl Pts',(0.0106444477317788,-0.0321934096636941,
0.0689817735665535));
#79160=CARTESIAN_POINT('Ctrl Pts',(0.0105519389397814,-0.0320508460844559,
0.0689366548537775));
#79161=CARTESIAN_POINT('Ctrl Pts',(0.0104582876489329,-0.0319086045663538,
0.0688940556893655));
#79162=CARTESIAN_POINT('Ctrl Pts',(0.0103637030581834,-0.0317669892868597,
0.0688540511959236));
#79163=CARTESIAN_POINT('Ctrl Pts',(0.0105693603844755,-0.0321934096636941,
0.0689444597232408));
#79164=CARTESIAN_POINT('Ctrl Pts',(0.010476183692452,-0.0320508460844559,
0.0689006850382243));
#79165=CARTESIAN_POINT('Ctrl Pts',(0.0103819011165501,-0.0319086045663538,
0.0688594468333262));
#79166=CARTESIAN_POINT('Ctrl Pts',(0.0102867229737405,-0.0317669892868597,
0.0688208171888639));
#79167=CARTESIAN_POINT('',(0.0105707037119558,-0.0321934096636941,0.0689451272752735));
#79168=CARTESIAN_POINT('',(0.010354797701258,-0.0318665617511289,0.0688489911534236));
#79169=CARTESIAN_POINT('Origin',(0.00290980286696623,-0.0326371944420151,
0.0837953293979655));
#79170=CARTESIAN_POINT('Origin',(0.0146067627215476,-0.0316939261508845,
0.0587461012863982));
#79171=CARTESIAN_POINT('',(0.0106829910913967,-0.0320197221621863,0.0689994622628841));
#79172=CARTESIAN_POINT('Ctrl Pts',(0.0106828519156328,-0.0320197392094772,
0.0689993404228847));
#79173=CARTESIAN_POINT('Ctrl Pts',(0.010656643682924,-0.031979271657607,
0.0689863190954539));
#79174=CARTESIAN_POINT('Ctrl Pts',(0.0106302168710053,-0.0319386439829744,
0.0689734382910022));
#79175=CARTESIAN_POINT('Ctrl Pts',(0.0106035400311454,-0.0318979099381675,
0.0689606920896429));
#79176=CARTESIAN_POINT('Ctrl Pts',(0.0105768637185712,-0.0318571766984964,
0.0689479461402207));
#79177=CARTESIAN_POINT('Ctrl Pts',(0.0105500737424975,-0.0318163871833599,
0.0689353979642012));
#79178=CARTESIAN_POINT('Ctrl Pts',(0.0105232637429612,-0.0317755399638303,
0.0689230875334388));
#79179=CARTESIAN_POINT('',(0.0106826438271765,-0.0321934096636183,0.0690007547021243));
#79180=CARTESIAN_POINT('Origin',(0.0116881152669688,-0.0324103521494481,
0.0669303005759181));
#79181=CARTESIAN_POINT('',(0.0106266737695762,-0.0321934096636662,0.0689729409887089));
#79182=CARTESIAN_POINT('Ctrl Pts',(0.0105713498077764,-0.0321934096636618,
0.0689470498380344));
#79183=CARTESIAN_POINT('Ctrl Pts',(0.0104995970701007,-0.0320835708272592,
0.0689132959731054));
#79184=CARTESIAN_POINT('Ctrl Pts',(0.0104271874174485,-0.0319739230346488,
0.0688810466059669));
#79185=CARTESIAN_POINT('Ctrl Pts',(0.0103542166595999,-0.0318646057455573,
0.0688503358873456));
#79186=CARTESIAN_POINT('Ctrl Pts',(0.0105352517812921,-0.0321934096636618,
0.0688396343026195));
#79187=CARTESIAN_POINT('Ctrl Pts',(0.0104620176996683,-0.0320835708272592,
0.0688063782576089));
#79188=CARTESIAN_POINT('Ctrl Pts',(0.0103881378646649,-0.0319739230346488,
0.068774657077969));
#79189=CARTESIAN_POINT('Ctrl Pts',(0.0103137099151944,-0.0318646057455573,
0.068744504094286));
#79190=CARTESIAN_POINT('Ctrl Pts',(0.0104991537548079,-0.0321934096636618,
0.0687322187672045));
#79191=CARTESIAN_POINT('Ctrl Pts',(0.0104244383292359,-0.0320835708272592,
0.0686994605421124));
#79192=CARTESIAN_POINT('Ctrl Pts',(0.0103490883118814,-0.0319739230346488,
0.0686682675499711));
#79193=CARTESIAN_POINT('Ctrl Pts',(0.0102732031707889,-0.0318646057455573,
0.0686386723012265));
#79194=CARTESIAN_POINT('Ctrl Pts',(0.0104630557283236,-0.0321934096636618,
0.0686248032317896));
#79195=CARTESIAN_POINT('Ctrl Pts',(0.0103868589588035,-0.0320835708272592,
0.0685925428266158));
#79196=CARTESIAN_POINT('Ctrl Pts',(0.0103100387590979,-0.0319739230346488,
0.0685618780219732));
#79197=CARTESIAN_POINT('Ctrl Pts',(0.0102326964263834,-0.0318646057455573,
0.0685328405081669));
#79198=CARTESIAN_POINT('',(0.0104512484717458,-0.0321763980308269,0.0686198191078848));
#79199=CARTESIAN_POINT('',(0.0104630557282936,-0.0321934096636184,0.0686248032317769));
#79200=CARTESIAN_POINT('Origin',(0.00347116593862575,-0.0326386230878191,
0.083623303336139));
#79201=CARTESIAN_POINT('Ctrl Pts',(0.0104512484705094,-0.0321763980306278,
0.0686198191108053));
#79202=CARTESIAN_POINT('Ctrl Pts',(0.0104345997576559,-0.0321259596174827,
0.0686593773181772));
#79203=CARTESIAN_POINT('Ctrl Pts',(0.010418239505362,-0.0320749164631402,
0.0686982501282784));
#79204=CARTESIAN_POINT('Ctrl Pts',(0.0103860827556678,-0.0319716057793924,
0.0687746562375072));
#79205=CARTESIAN_POINT('Ctrl Pts',(0.010370298787618,-0.031919378669013,
0.0688121597662465));
#79206=CARTESIAN_POINT('Ctrl Pts',(0.0103547977005306,-0.0318665617525313,
0.0688489911551285));
#79207=CARTESIAN_POINT('',(0.0105168797201347,-0.0321934096636663,0.0687849652535352));
#79208=CARTESIAN_POINT('Origin',(0.00812378219310841,-0.0315241814719618,
0.07415));
#79209=CARTESIAN_POINT('',(0.0104512484718894,-0.0322104233323627,0.068619819107543));
#79210=CARTESIAN_POINT('',(0.0104394305973831,-0.0321934096636183,0.0686148602124426));
#79211=CARTESIAN_POINT('Origin',(0.00351009208260348,-0.0326387237493397,
0.0836465390198752));
#79212=CARTESIAN_POINT('Origin',(0.00460209302538108,-0.0326386240213093,
0.0840992745560143));
#79213=CARTESIAN_POINT('Origin',(0.00455826793499113,-0.0326387245235589,
0.0840876784787476));
#79214=CARTESIAN_POINT('Ctrl Pts',(0.0105024377931778,-0.0327445246967096,
0.0689135773149736));
#79215=CARTESIAN_POINT('Ctrl Pts',(0.0103049428830077,-0.032443687833936,
0.068823864852417));
#79216=CARTESIAN_POINT('Ctrl Pts',(0.01010125152568,-0.0321434074405927,
0.0687492833772971));
#79217=CARTESIAN_POINT('Ctrl Pts',(0.0102726275908998,-0.0327445246967096,
0.0688151533802376));
#79218=CARTESIAN_POINT('Ctrl Pts',(0.0100714205613462,-0.032443687833936,
0.0687341083511532));
#79219=CARTESIAN_POINT('Ctrl Pts',(0.00986468049688743,-0.0321434074405927,
0.0686684492982461));
#79220=CARTESIAN_POINT('',(0.0102390586088646,-0.0326943950436612,0.0688017544292594));
#79221=CARTESIAN_POINT('',(0.0100175422025775,-0.0323666188837389,0.0687193648597483));
#79222=CARTESIAN_POINT('Origin',(0.0041269508842937,-0.0326395579111481,
0.0844622204949339));
#79223=CARTESIAN_POINT('Origin',(0.0136542190453974,-0.0321933825603012,
0.0582906567238054));
#79224=CARTESIAN_POINT('',(0.0101351242805322,-0.0321934096532688,0.0687618066103723));
#79225=CARTESIAN_POINT('',(0.0100761095784306,-0.0321934096584275,0.0687412271234611));
#79226=CARTESIAN_POINT('',(0.0103547977016218,-0.0325210109756239,0.0688489911525471));
#79227=CARTESIAN_POINT('Origin',(0.00368979084779726,-0.0326393129157865,
0.0842620317531794));
#79228=CARTESIAN_POINT('',(0.0103542707108206,-0.0326943950436593,0.0688502433100797));
#79229=CARTESIAN_POINT('Origin',(0.0146455201351887,-0.0326943765538048,
0.0586540138571446));
#79230=CARTESIAN_POINT('',(0.0102966646598526,-0.0326943950436702,0.0688259988696796));
#79231=CARTESIAN_POINT('Ctrl Pts',(0.0106662248648126,-0.0325229783203769,
0.0687152980522278));
#79232=CARTESIAN_POINT('Ctrl Pts',(0.0105913076173117,-0.032413025309245,
0.068680250535598));
#79233=CARTESIAN_POINT('Ctrl Pts',(0.010515676729576,-0.0323031222208069,
0.0686467580941132));
#79234=CARTESIAN_POINT('Ctrl Pts',(0.0104394305932463,-0.0321934096576658,
0.068614860210712));
#79235=CARTESIAN_POINT('Ctrl Pts',(0.0105622312703106,-0.0325229783203769,
0.068760314433011));
#79236=CARTESIAN_POINT('Ctrl Pts',(0.0104879345726343,-0.032413025309245,
0.0687267004658072));
#79237=CARTESIAN_POINT('Ctrl Pts',(0.0104129537954161,-0.0323031222208069,
0.0686946285194523));
#79238=CARTESIAN_POINT('Ctrl Pts',(0.0103373864333454,-0.0321934096576658,
0.0686641362867163));
#79239=CARTESIAN_POINT('Ctrl Pts',(0.0104582376758086,-0.0325229783203769,
0.0688053308137942));
#79240=CARTESIAN_POINT('Ctrl Pts',(0.010384561527957,-0.032413025309245,
0.0687731503960163));
#79241=CARTESIAN_POINT('Ctrl Pts',(0.0103102308612563,-0.0323031222208069,
0.0687424989447914));
#79242=CARTESIAN_POINT('Ctrl Pts',(0.0102353422734446,-0.0321934096576658,
0.0687134123627207));
#79243=CARTESIAN_POINT('Ctrl Pts',(0.0103542440813066,-0.0325229783203769,
0.0688503471945773));
#79244=CARTESIAN_POINT('Ctrl Pts',(0.0102811884832796,-0.032413025309245,
0.0688196003262255));
#79245=CARTESIAN_POINT('Ctrl Pts',(0.0102075079270964,-0.0323031222208069,
0.0687903693701304));
#79246=CARTESIAN_POINT('Ctrl Pts',(0.0101332981135437,-0.0321934096576658,
0.0687626884387251));
#79247=CARTESIAN_POINT('',(0.0102872774394729,-0.0321934096584275,0.0686883334114516));
#79248=CARTESIAN_POINT('Ctrl Pts',(0.0104512484705346,-0.0322104233328949,
0.0686198191107456));
#79249=CARTESIAN_POINT('Ctrl Pts',(0.0104345771984191,-0.0322609421830998,
0.0686594309200968));
#79250=CARTESIAN_POINT('Ctrl Pts',(0.0104182059255511,-0.0323120888239943,
0.0686983299156378));
#79251=CARTESIAN_POINT('Ctrl Pts',(0.0103860489323641,-0.0324156524631822,
0.0687747366034181));
#79252=CARTESIAN_POINT('Ctrl Pts',(0.0103702764302917,-0.0324680267167324,
0.0688122128884162));
#79253=CARTESIAN_POINT('Ctrl Pts',(0.0103547977016009,-0.0325210109755913,
0.0688489911525853));
#79254=CARTESIAN_POINT('Origin',(0.0149552170010535,-0.026283458251215,
0.078053188991479));
#79255=CARTESIAN_POINT('Origin',(0.0173551804691235,-0.0342770991216957,
0.0662375992804839));
#79256=CARTESIAN_POINT('Ctrl Pts',(0.0102398239626242,-0.0326943950436604,
0.0688036321737721));
#79257=CARTESIAN_POINT('Ctrl Pts',(0.0101661409938175,-0.0325844576448134,
0.0687744691523033));
#79258=CARTESIAN_POINT('Ctrl Pts',(0.0100918496712552,-0.0324744968375322,
0.0687468279515219));
#79259=CARTESIAN_POINT('Ctrl Pts',(0.0100170456697988,-0.0323646534831894,
0.0687207426740401));
#79260=CARTESIAN_POINT('Ctrl Pts',(0.0101970525519996,-0.0326943950436604,
0.0686986953641456));
#79261=CARTESIAN_POINT('Ctrl Pts',(0.0101219233572837,-0.0325844576448134,
0.0686701218128773));
#79262=CARTESIAN_POINT('Ctrl Pts',(0.0100461978976708,-0.0324744968375322,
0.0686431000343372));
#79263=CARTESIAN_POINT('Ctrl Pts',(0.00996997367457563,-0.0323646534831894,
0.0686176633121527));
#79264=CARTESIAN_POINT('Ctrl Pts',(0.010154281141375,-0.0326943950436604,
0.0685937585545191));
#79265=CARTESIAN_POINT('Ctrl Pts',(0.0100777057207499,-0.0325844576448134,
0.0685657744734514));
#79266=CARTESIAN_POINT('Ctrl Pts',(0.0100005461240864,-0.0324744968375322,
0.0685393721171524));
#79267=CARTESIAN_POINT('Ctrl Pts',(0.00992290167935243,-0.0323646534831894,
0.0685145839502653));
#79268=CARTESIAN_POINT('Ctrl Pts',(0.0101115097307504,-0.0326943950436604,
0.0684888217448926));
#79269=CARTESIAN_POINT('Ctrl Pts',(0.0100334880842161,-0.0325844576448134,
0.0684614271340255));
#79270=CARTESIAN_POINT('Ctrl Pts',(0.00995489435050194,-0.0324744968375322,
0.0684356441999677));
#79271=CARTESIAN_POINT('Ctrl Pts',(0.00987582968412923,-0.0323646534831894,
0.0684115045883779));
#79272=CARTESIAN_POINT('',(0.0100994128174638,-0.0326773559991341,0.068484588839611));
#79273=CARTESIAN_POINT('',(0.0101115097307497,-0.0326943950436594,0.0684888217448924));
#79274=CARTESIAN_POINT('Origin',(0.0046792468833737,-0.0326395670827019,
0.084180292496662));
#79275=CARTESIAN_POINT('Ctrl Pts',(0.0100994128163548,-0.032677355998742,
0.0684845888427716));
#79276=CARTESIAN_POINT('Ctrl Pts',(0.0100852694638655,-0.0326267922585946,
0.0685251469845875));
#79277=CARTESIAN_POINT('Ctrl Pts',(0.0100713767920861,-0.0325756109579296,
0.0685649862626271));
#79278=CARTESIAN_POINT('Ctrl Pts',(0.0100440809865966,-0.0324719985462368,
0.068643260996348));
#79279=CARTESIAN_POINT('Ctrl Pts',(0.0100306888004874,-0.0324196091621778,
0.0686816650581751));
#79280=CARTESIAN_POINT('Ctrl Pts',(0.0100175422025614,-0.0323666188837757,
0.0687193648597944));
#79281=CARTESIAN_POINT('',(0.0101752841698171,-0.0326943950436702,0.0686452880870859));
#79282=CARTESIAN_POINT('Origin',(0.00812378219310841,-0.0315241814719618,
0.07415));
#79283=CARTESIAN_POINT('',(0.0100994128174488,-0.0327114338379886,0.0684845888396533));
#79284=CARTESIAN_POINT('',(0.0100873068912882,-0.0326943950436593,0.0684803817800796));
#79285=CARTESIAN_POINT('Origin',(0.00472227965081183,-0.0326395672612986,
0.0841944774514547));
#79286=CARTESIAN_POINT('Origin',(0.00458436906086605,-0.0326395676967327,
0.0841472085234683));
#79287=CARTESIAN_POINT('Origin',(0.00454184827979971,-0.0326395680217033,
0.0841315559643501));
#79288=CARTESIAN_POINT('Ctrl Pts',(0.0101689096987611,-0.0332451089994433,
0.0687745392303894));
#79289=CARTESIAN_POINT('Ctrl Pts',(0.00996617087885437,-0.0329451141710254,
0.0686974059845477));
#79290=CARTESIAN_POINT('Ctrl Pts',(0.00975819802713791,-0.0326442513127493,
0.0686357629828349));
#79291=CARTESIAN_POINT('Ctrl Pts',(0.00993337231292476,-0.0332451089994433,
0.0686907410211401));
#79292=CARTESIAN_POINT('Ctrl Pts',(0.00972747299184772,-0.0329451141710254,
0.0686224912131459));
#79293=CARTESIAN_POINT('Ctrl Pts',(0.00951701775446562,-0.0326442513127493,
0.0685699444742397));
#79294=CARTESIAN_POINT('Ctrl Pts',(0.0099310169390664,-0.0332451089994433,
0.0686899030390476));
#79295=CARTESIAN_POINT('Ctrl Pts',(0.00972508601297765,-0.0329451141710254,
0.0686217420654319));
#79296=CARTESIAN_POINT('Ctrl Pts',(0.0095146059517389,-0.0326442513127493,
0.0685692862891537));
#79297=CARTESIAN_POINT('',(0.00989906547608922,-0.0331951640388616,0.0686794886651091));
#79298=CARTESIAN_POINT('',(0.0096728128861654,-0.0328677532355001,0.068611170793228));
#79299=CARTESIAN_POINT('Origin',(0.00546039648536102,-0.0326402808281567,
0.0848452074883621));
#79300=CARTESIAN_POINT('Origin',(0.0126501866039726,-0.0326944278779143,
0.0579636533031569));
#79301=CARTESIAN_POINT('',(0.00979282788793583,-0.0326943950436593,0.0686461457624153));
#79302=CARTESIAN_POINT('',(0.00973263744377394,-0.0326943950436694,0.0686293124493114));
#79303=CARTESIAN_POINT('',(0.0100175422025802,-0.0330220786163545,0.0687193648597492));
#79304=CARTESIAN_POINT('Origin',(0.00498990723212481,-0.0326396682762087,
0.0847462503893336));
#79305=CARTESIAN_POINT('',(0.0100170948752985,-0.0331951640388587,0.0687206476364617));
#79306=CARTESIAN_POINT('Origin',(0.0136495077187538,-0.0331952026560047,
0.0583041728748783));
#79307=CARTESIAN_POINT('',(0.00995808017570384,-0.0331951640388701,0.0687000681507954));
#79308=CARTESIAN_POINT('Ctrl Pts',(0.010319959281971,-0.0330240426238172,
0.0685663805471387));
#79309=CARTESIAN_POINT('Ctrl Pts',(0.0102430394841509,-0.0329142774063519,
0.068536126068108));
#79310=CARTESIAN_POINT('Ctrl Pts',(0.0101654558944131,-0.032804347972669,
0.0685074466532019));
#79311=CARTESIAN_POINT('Ctrl Pts',(0.0100873068912882,-0.0326943950436593,
0.0684803817800796));
#79312=CARTESIAN_POINT('Ctrl Pts',(0.0102189975298273,-0.0330240426238172,
0.0686178379138465));
#79313=CARTESIAN_POINT('Ctrl Pts',(0.0101427866073661,-0.0329142774063519,
0.0685889742813138));
#79314=CARTESIAN_POINT('Ctrl Pts',(0.0100659409990697,-0.032804347972669,
0.0685616717518596));
#79315=CARTESIAN_POINT('Ctrl Pts',(0.00998855818663668,-0.0326943950436593,
0.068535968013214));
#79316=CARTESIAN_POINT('Ctrl Pts',(0.0101180357776836,-0.0330240426238172,
0.0686692952805543));
#79317=CARTESIAN_POINT('Ctrl Pts',(0.0100425337305813,-0.0329142774063519,
0.0686418224945197));
#79318=CARTESIAN_POINT('Ctrl Pts',(0.00996642610372621,-0.032804347972669,
0.0686158968505174));
#79319=CARTESIAN_POINT('Ctrl Pts',(0.00988980948198516,-0.0326943950436593,
0.0685915542463484));
#79320=CARTESIAN_POINT('Ctrl Pts',(0.0100170740255399,-0.0330240426238172,
0.0687207526472621));
#79321=CARTESIAN_POINT('Ctrl Pts',(0.00994228085379651,-0.0329142774063519,
0.0686946707077255));
#79322=CARTESIAN_POINT('Ctrl Pts',(0.00986691120838275,-0.032804347972669,
0.0686701219491752));
#79323=CARTESIAN_POINT('Ctrl Pts',(0.00979106077733364,-0.0326943950436593,
0.0686471404794828));
#79324=CARTESIAN_POINT('',(0.00994006738962203,-0.0326943950436693,0.0685632637712575));
#79325=CARTESIAN_POINT('Ctrl Pts',(0.010099412816352,-0.0327114338383347,
0.06848458884278));
#79326=CARTESIAN_POINT('Ctrl Pts',(0.0100852718163742,-0.032761987683071,
0.0685251402384234));
#79327=CARTESIAN_POINT('Ctrl Pts',(0.0100713802936745,-0.0328131562603779,
0.0685649762213077));
#79328=CARTESIAN_POINT('Ctrl Pts',(0.0100440845132367,-0.0329167375858778,
0.0686432508831895));
#79329=CARTESIAN_POINT('Ctrl Pts',(0.0100306911315659,-0.0329691088920621,
0.0686816583734653));
#79330=CARTESIAN_POINT('Ctrl Pts',(0.0100175422025619,-0.0330220786163186,
0.0687193648597932));
#79331=CARTESIAN_POINT('Ctrl Pts',(0.00989994736492207,-0.0331951640388604,
0.0686813149388771));
#79332=CARTESIAN_POINT('Ctrl Pts',(0.00978688580747801,-0.033030642201062,
0.0686445938627211));
#79333=CARTESIAN_POINT('Ctrl Pts',(0.00967240313964828,-0.0328657861914645,
0.0686125771175346));
#79334=CARTESIAN_POINT('Ctrl Pts',(0.00989906547609221,-0.0331951640388604,
0.0686794886651103));
#79335=CARTESIAN_POINT('Ctrl Pts',(0.00978596616160892,-0.033030642201062,
0.0686427858214403));
#79336=CARTESIAN_POINT('Ctrl Pts',(0.00967144652257091,-0.0328657861914645,
0.0686107888536987));
#79337=CARTESIAN_POINT('Ctrl Pts',(0.00975211908072219,-0.0331951640388604,
0.0683751823422348));
#79338=CARTESIAN_POINT('Ctrl Pts',(0.0096327284281165,-0.0330306422010619,
0.0683415175210759));
#79339=CARTESIAN_POINT('Ctrl Pts',(0.00951204839152569,-0.0328657861914645,
0.0683128160074971));
#79340=CARTESIAN_POINT('',(0.00973978025258226,-0.0331781648281902,0.0683717173600123));
#79341=CARTESIAN_POINT('',(0.00975211908072106,-0.0331951640388588,0.0683751823422345));
#79342=CARTESIAN_POINT('Origin',(0.00597986164658149,-0.0326412092584411,
0.0844605176198909));
#79343=CARTESIAN_POINT('Ctrl Pts',(0.00973978025373896,-0.033178164828644,
0.0683717173614345));
#79344=CARTESIAN_POINT('Ctrl Pts',(0.00972820352374881,-0.0331276811546772,
0.068413112021642));
#79345=CARTESIAN_POINT('Ctrl Pts',(0.00971683586621816,-0.0330765663497772,
0.0684537592315872));
#79346=CARTESIAN_POINT('Ctrl Pts',(0.00969450877310779,-0.0329730614463314,
0.0685335936303563));
#79347=CARTESIAN_POINT('Ctrl Pts',(0.00968355835202192,-0.0329207133373986,
0.0685727485663901));
#79348=CARTESIAN_POINT('Ctrl Pts',(0.0096728129019712,-0.0328677532289359,
0.0686111707886005));
#79349=CARTESIAN_POINT('',(0.00982559227841514,-0.0331951640388701,0.0685273355036818));
#79350=CARTESIAN_POINT('Origin',(0.00812378219310841,-0.0315241814719618,
0.07415));
#79351=CARTESIAN_POINT('',(0.00973978025154155,-0.0332121607144241,0.0683717173613322));
#79352=CARTESIAN_POINT('',(0.0097274340502593,-0.0331951640388587,0.0683682787406282));
#79353=CARTESIAN_POINT('Origin',(0.00602498555138481,-0.0326413655988795,
0.0844649937999266));
#79354=CARTESIAN_POINT('Origin',(0.00460796994952319,-0.032641209838483,
0.0840768460134683));
#79355=CARTESIAN_POINT('Origin',(0.00456707180094442,-0.0326413663911616,
0.0840572609498495));
#79356=CARTESIAN_POINT('Ctrl Pts',(0.00982736602910231,-0.0337436976235975,
0.0686567380261141));
#79357=CARTESIAN_POINT('Ctrl Pts',(0.00977795879838256,-0.0336723290703325,
0.068641415734908));
#79358=CARTESIAN_POINT('Ctrl Pts',(0.00972828396086462,-0.033601104548885,
0.0686269846028399));
#79359=CARTESIAN_POINT('Ctrl Pts',(0.00956968204470073,-0.0333736987606857,
0.0685809088567926));
#79360=CARTESIAN_POINT('Ctrl Pts',(0.00940869739996884,-0.0331450831799192,
0.0685440105323699));
#79361=CARTESIAN_POINT('Ctrl Pts',(0.009587031938753,-0.0337436976235975,
0.0685878938178176));
#79362=CARTESIAN_POINT('Ctrl Pts',(0.0095370055127902,-0.0336723290703325,
0.0685747331278437));
#79363=CARTESIAN_POINT('Ctrl Pts',(0.00948675046059336,-0.033601104548885,
0.0685624743846825));
#79364=CARTESIAN_POINT('Ctrl Pts',(0.00932629603389381,-0.0333736987606857,
0.0685233346460888));
#79365=CARTESIAN_POINT('Ctrl Pts',(0.0091638599595174,-0.0331450831799192,
0.0684934672068642));
#79366=CARTESIAN_POINT('Ctrl Pts',(0.0095846285978495,-0.0337436976235975,
0.0685872053757347));
#79367=CARTESIAN_POINT('Ctrl Pts',(0.00953459597993428,-0.0336723290703325,
0.0685740663017731));
#79368=CARTESIAN_POINT('Ctrl Pts',(0.00948433512559065,-0.033601104548885,
0.0685618292825009));
#79369=CARTESIAN_POINT('Ctrl Pts',(0.00932386217378574,-0.0333736987606857,
0.0685227589039818));
#79370=CARTESIAN_POINT('Ctrl Pts',(0.00916141158511288,-0.0331450831799192,
0.068492961773609));
#79371=CARTESIAN_POINT('',(0.00955206611123276,-0.0336938721132548,0.0685788125099555));
#79372=CARTESIAN_POINT('',(0.00932197026244842,-0.0333679870047996,0.0685248359712446));
#79373=CARTESIAN_POINT('Ctrl Pts',(0.00955206611125787,-0.0336938721132548,
0.0685788125099619));
#79374=CARTESIAN_POINT('Ctrl Pts',(0.00953031915298532,-0.0336629187933894,
0.0685732372478075));
#79375=CARTESIAN_POINT('Ctrl Pts',(0.00950854650451064,-0.0336319952301032,
0.0685677911059402));
#79376=CARTESIAN_POINT('Ctrl Pts',(0.00948675046060606,-0.0336011045488942,
0.0685624743846858));
#79377=CARTESIAN_POINT('Ctrl Pts',(0.009432056728263,-0.0335235892595445,
0.0685491329117786));
#79378=CARTESIAN_POINT('Ctrl Pts',(0.00937711846022698,-0.0334458668665561,
0.0685365828131935));
#79379=CARTESIAN_POINT('Ctrl Pts',(0.00932197027405363,-0.0333679869962484,
0.068524835973455));
#79380=CARTESIAN_POINT('Ctrl Pts',(0.00932192691853327,-0.0333679692468933,
0.0685248260356988));
#79381=CARTESIAN_POINT('Ctrl Pts',(0.00932183829732831,-0.0333391895415735,
0.0685252705399856));
#79382=CARTESIAN_POINT('Ctrl Pts',(0.0093217750559261,-0.0333104081132863,
0.0685256043525627));
#79383=CARTESIAN_POINT('Ctrl Pts',(0.00932169678684232,-0.033253269890485,
0.0685260472410793));
#79384=CARTESIAN_POINT('Ctrl Pts',(0.00932168105404384,-0.033224917447262,
0.0685261595976384));
#79385=CARTESIAN_POINT('Ctrl Pts',(0.0093216870395485,-0.0331960985234834,
0.0685261646253599));
#79386=CARTESIAN_POINT('Ctrl Pts',(0.00932168714260407,-0.0331956312691392,
0.0685261646777334));
#79387=CARTESIAN_POINT('Ctrl Pts',(0.00932168725141207,-0.033195164038861,
0.06852616470091));
#79388=CARTESIAN_POINT('',(0.00944394454052274,-0.0331951640388587,0.0685522061152209));
#79389=CARTESIAN_POINT('',(0.00938281589597739,-0.0331951640388687,0.0685391854080754));
#79390=CARTESIAN_POINT('',(0.00967281289801524,-0.0335216366567727,0.0686111708032634));
#79391=CARTESIAN_POINT('Origin',(0.00636530768705754,-0.0326434571528351,
0.0849338873136656));
#79392=CARTESIAN_POINT('',(0.00967244699959201,-0.0336938721132327,0.0686124791361874));
#79393=CARTESIAN_POINT('Origin',(0.012613717613471,-0.0336938867896221,
0.0580954568811573));
#79394=CARTESIAN_POINT('',(0.00961225655542239,-0.0336938721132538,0.0685956458230815));
#79395=CARTESIAN_POINT('Ctrl Pts',(0.00996502634716105,-0.0335235895815172,
0.0684394991493578));
#79396=CARTESIAN_POINT('Ctrl Pts',(0.0098864100600104,-0.0334144449262749,
0.0684141507985011));
#79397=CARTESIAN_POINT('Ctrl Pts',(0.00980717977441849,-0.0333049234473147,
0.0683903974787876));
#79398=CARTESIAN_POINT('Ctrl Pts',(0.00972743405025945,-0.0331951640388587,
0.068368278740628));
#79399=CARTESIAN_POINT('Ctrl Pts',(0.00986749472538496,-0.0335235895815172,
0.0684971945151993));
#79400=CARTESIAN_POINT('Ctrl Pts',(0.00978967272853683,-0.0334144449262749,
0.0684731888791384));
#79401=CARTESIAN_POINT('Ctrl Pts',(0.00971126538526795,-0.0333049234473147,
0.0684507634073975));
#79402=CARTESIAN_POINT('Ctrl Pts',(0.0096323703569659,-0.0331951640388587,
0.0684299558571563));
#79403=CARTESIAN_POINT('Ctrl Pts',(0.00976996310360887,-0.0335235895815172,
0.0685548898810407));
#79404=CARTESIAN_POINT('Ctrl Pts',(0.00969293539706327,-0.0334144449262749,
0.0685322269597758));
#79405=CARTESIAN_POINT('Ctrl Pts',(0.00961535099611742,-0.0333049234473147,
0.0685111293360074));
#79406=CARTESIAN_POINT('Ctrl Pts',(0.00953730666367236,-0.0331951640388587,
0.0684916329736847));
#79407=CARTESIAN_POINT('Ctrl Pts',(0.00967243148183278,-0.0335235895815172,
0.0686125852468822));
#79408=CARTESIAN_POINT('Ctrl Pts',(0.00959619806558971,-0.0334144449262749,
0.0685912650404131));
#79409=CARTESIAN_POINT('Ctrl Pts',(0.00951943660696689,-0.0333049234473147,
0.0685714952646172));
#79410=CARTESIAN_POINT('Ctrl Pts',(0.00944224297037881,-0.0331951640388587,
0.068553310090213));
#79411=CARTESIAN_POINT('',(0.00958568929540102,-0.0331951640388687,0.0684602424279345));
#79412=CARTESIAN_POINT('Ctrl Pts',(0.00973978025069291,-0.0332121607145999,
0.0683717173643448));
#79413=CARTESIAN_POINT('Ctrl Pts',(0.00972822298409216,-0.0332625444109513,
0.0684130423848801));
#79414=CARTESIAN_POINT('Ctrl Pts',(0.00971686486733106,-0.0333135300746303,
0.0684536553104628));
#79415=CARTESIAN_POINT('Ctrl Pts',(0.00969453791753884,-0.0334167203140639,
0.0685334892098206));
#79416=CARTESIAN_POINT('Ctrl Pts',(0.0096835777319374,-0.0334688847587326,
0.0685726792632041));
#79417=CARTESIAN_POINT('Ctrl Pts',(0.00967281289765872,-0.0335216366562399,
0.0686111708038939));
#79418=CARTESIAN_POINT('Ctrl Pts',(0.0095530606999123,-0.0336938721132547,
0.0685805793924302));
#79419=CARTESIAN_POINT('Ctrl Pts',(0.00952046103296096,-0.0336474569765037,
0.0685722133510435));
#79420=CARTESIAN_POINT('Ctrl Pts',(0.00948776566468227,-0.033601104548885,
0.0685642295031653));
#79421=CARTESIAN_POINT('Ctrl Pts',(0.00940498850935112,-0.0334837508592655,
0.068544016235943));
#79422=CARTESIAN_POINT('Ctrl Pts',(0.00932164874262919,-0.0333660264659096,
0.0685262647036357));
#79423=CARTESIAN_POINT('Ctrl Pts',(0.00955206611126368,-0.0336938721132547,
0.0685788125099635));
#79424=CARTESIAN_POINT('Ctrl Pts',(0.00951945610216294,-0.0336474569765037,
0.0685704522902343));
#79425=CARTESIAN_POINT('Ctrl Pts',(0.00948675046059336,-0.033601104548885,
0.0685624743846825));
#79426=CARTESIAN_POINT('Ctrl Pts',(0.00940394729565166,-0.0334837508592655,
0.0685422761620644));
#79427=CARTESIAN_POINT('Ctrl Pts',(0.0093205819765435,-0.0333660264659096,
0.0685245404384735));
#79428=CARTESIAN_POINT('Ctrl Pts',(0.00938530754500726,-0.0336938721132547,
0.0682825666325416));
#79429=CARTESIAN_POINT('Ctrl Pts',(0.00935096351048089,-0.0336474569765037,
0.0682751825060373));
#79430=CARTESIAN_POINT('Ctrl Pts',(0.00931653538870579,-0.033601104548885,
0.0682682009257848));
#79431=CARTESIAN_POINT('Ctrl Pts',(0.00922937129990751,-0.0334837508592655,
0.0682505251697544));
#79432=CARTESIAN_POINT('Ctrl Pts',(0.00914172171785406,-0.0333660264659096,
0.0682354400282854));
#79433=CARTESIAN_POINT('',(0.00937377008003389,-0.0336769361243754,0.0682816501226887));
#79434=CARTESIAN_POINT('',(0.00938630212891338,-0.0336938721132327,0.0682843335066086));
#79435=CARTESIAN_POINT('Ctrl Pts',(0.00937377008003363,-0.0336769361243751,
0.0682816501226887));
#79436=CARTESIAN_POINT('Ctrl Pts',(0.00937585938891902,-0.033679758666967,
0.0682820951559353));
#79437=CARTESIAN_POINT('Ctrl Pts',(0.00937794838111765,-0.0336825812712137,
0.0682825412881353));
#79438=CARTESIAN_POINT('Ctrl Pts',(0.00938212573710684,-0.033688226609505,
0.0682834357509796));
#79439=CARTESIAN_POINT('Ctrl Pts',(0.00938421410081141,-0.033691049343433,
0.0682838840816254));
#79440=CARTESIAN_POINT('Ctrl Pts',(0.00938630212891564,-0.0336938721132299,
0.0682843335066159));
#79441=CARTESIAN_POINT('Ctrl Pts',(0.00937377008003389,-0.0336769361243754,
0.0682816501226887));
#79442=CARTESIAN_POINT('Ctrl Pts',(0.00936503832843738,-0.0336279018525336,
0.0683226432986591));
#79443=CARTESIAN_POINT('Ctrl Pts',(0.00935618095953362,-0.0335767826051515,
0.0683642262133951));
#79444=CARTESIAN_POINT('Ctrl Pts',(0.00933882560463971,-0.0334733172106813,
0.0684457048387705));
#79445=CARTESIAN_POINT('Ctrl Pts',(0.00933031595447219,-0.0334209631477606,
0.0684856553095198));
#79446=CARTESIAN_POINT('Ctrl Pts',(0.00932197027682847,-0.0333679869844681,
0.0685248359742998));
#79447=CARTESIAN_POINT('',(0.00946918412008307,-0.0336938721132538,0.0684315730082921));
#79448=CARTESIAN_POINT('Origin',(0.00812378219310841,-0.0315241814719618,
0.07415));
#79449=CARTESIAN_POINT('',(0.00937377007976809,-0.0337108120655697,0.0682816501239629));
#79450=CARTESIAN_POINT('',(0.00936123232798906,-0.0336938721132327,0.0682789935135702));
#79451=CARTESIAN_POINT('Origin',(0.00487213367656529,-0.034556251928565,
0.0840510377659916));
#79452=CARTESIAN_POINT('Ctrl Pts',(0.00936123232799071,-0.0336938721132336,
0.0682789935135684));
#79453=CARTESIAN_POINT('Ctrl Pts',(0.00936332227440066,-0.0336910493199299,
0.0682794340180156));
#79454=CARTESIAN_POINT('Ctrl Pts',(0.00936541205519568,-0.0336882265977529,
0.0682798756530937));
#79455=CARTESIAN_POINT('Ctrl Pts',(0.00936959130360236,-0.0336825812712303,
0.0682807611888089));
#79456=CARTESIAN_POINT('Ctrl Pts',(0.0093716807711426,-0.0336797586669754,
0.0682812050894407));
#79457=CARTESIAN_POINT('Ctrl Pts',(0.00937377008003416,-0.0336769361243751,
0.0682816501226888));
#79458=CARTESIAN_POINT('Origin',(0.00705830094378643,-0.034556251861001,
0.0845167005544149));
#79459=CARTESIAN_POINT('Ctrl Pts',(0.00947912980566762,-0.0342436276873911,
0.0685606209782186));
#79460=CARTESIAN_POINT('Ctrl Pts',(0.00926832290066522,-0.0339430054201811,
0.0685095032003237));
#79461=CARTESIAN_POINT('Ctrl Pts',(0.00905426447550039,-0.0336441434784052,
0.0684744094825159));
#79462=CARTESIAN_POINT('Ctrl Pts',(0.0092349476775481,-0.0342436276873911,
0.0685070011282839));
#79463=CARTESIAN_POINT('Ctrl Pts',(0.00902211846656726,-0.0339430054201811,
0.0684650928311712));
#79464=CARTESIAN_POINT('Ctrl Pts',(0.00880673717641047,-0.0336441434784052,
0.0684393347593488));
#79465=CARTESIAN_POINT('Ctrl Pts',(0.0092325058562669,-0.0342436276873911,
0.0685064649297845));
#79466=CARTESIAN_POINT('Ctrl Pts',(0.00901965642222629,-0.0339430054201811,
0.0684646487274797));
#79467=CARTESIAN_POINT('Ctrl Pts',(0.00880426190341958,-0.0336441434784052,
0.0684389840121171));
#79468=CARTESIAN_POINT('',(0.00919942996230135,-0.0341934961088741,0.068500123286599));
#79469=CARTESIAN_POINT('',(0.00896639895363432,-0.0338664212862939,0.0684607010976068));
#79470=CARTESIAN_POINT('Origin',(0.00557044497237628,-0.0345610720406228,
0.0848366961130874));
#79471=CARTESIAN_POINT('Origin',(0.0105729984233713,-0.0336938005072981,
0.0576127721447583));
#79472=CARTESIAN_POINT('',(0.00908985111544924,-0.0336938721132327,0.0684803584031009));
#79473=CARTESIAN_POINT('',(0.00902802551735347,-0.0336938721132427,0.0684712016886965));
#79474=CARTESIAN_POINT('',(0.00932197027683366,-0.0340203938281605,0.0685248359743009));
#79475=CARTESIAN_POINT('Origin',(0.00512241414220757,-0.0345589643243073,
0.0846611822701679));
#79476=CARTESIAN_POINT('',(0.00932168725141203,-0.034193496108874,0.06852616470091));
#79477=CARTESIAN_POINT('Origin',(0.0116173839760832,-0.0341934220717635,
0.0577485028575781));
#79478=CARTESIAN_POINT('',(0.0092605586068667,-0.0341934961088841,0.0685131439937645));
#79479=CARTESIAN_POINT('Ctrl Pts',(0.0096028304090113,-0.0340223579322397,
0.0683351555158321));
#79480=CARTESIAN_POINT('Ctrl Pts',(0.00952262853782355,-0.0339125849573575,
0.0683147555834151));
#79481=CARTESIAN_POINT('Ctrl Pts',(0.00944206079236394,-0.0338030433565231,
0.0682960299781646));
#79482=CARTESIAN_POINT('Ctrl Pts',(0.00936123232798963,-0.0336938721132327,
0.0682789935135698));
#79483=CARTESIAN_POINT('Ctrl Pts',(0.00950911390975521,-0.0340223579322397,
0.06839886106973));
#79484=CARTESIAN_POINT('Ctrl Pts',(0.00942979070430676,-0.0339125849573575,
0.0683797537322607));
#79485=CARTESIAN_POINT('Ctrl Pts',(0.00935012776087007,-0.0338030433565231,
0.0683623016273272));
#79486=CARTESIAN_POINT('Ctrl Pts',(0.00927022893334515,-0.0336938721132327,
0.0683465180423977));
#79487=CARTESIAN_POINT('Ctrl Pts',(0.00941539741049911,-0.0340223579322397,
0.0684625666236279));
#79488=CARTESIAN_POINT('Ctrl Pts',(0.00933695287078998,-0.0339125849573575,
0.0684447518811061));
#79489=CARTESIAN_POINT('Ctrl Pts',(0.0092581947293762,-0.0338030433565231,
0.0684285732764898));
#79490=CARTESIAN_POINT('Ctrl Pts',(0.00917922553870066,-0.0336938721132327,
0.0684140425712256));
#79491=CARTESIAN_POINT('Ctrl Pts',(0.00932168091124302,-0.0340223579322397,
0.0685262721775258));
#79492=CARTESIAN_POINT('Ctrl Pts',(0.0092441150372732,-0.0339125849573575,
0.0685097500299517));
#79493=CARTESIAN_POINT('Ctrl Pts',(0.00916626169788233,-0.0338030433565231,
0.0684948449256524));
#79494=CARTESIAN_POINT('Ctrl Pts',(0.00908822214405618,-0.0336938721132327,
0.0684815671000535));
#79495=CARTESIAN_POINT('',(0.00922554172172915,-0.0336938721132427,0.0683796759583456));
#79496=CARTESIAN_POINT('Ctrl Pts',(0.00937377007901281,-0.0337108120662708,
0.0682816501274828));
#79497=CARTESIAN_POINT('Ctrl Pts',(0.00936481198745918,-0.0337611408994052,
0.0683237059073984));
#79498=CARTESIAN_POINT('Ctrl Pts',(0.00935601736120198,-0.0338121088780783,
0.0683649942626355));
#79499=CARTESIAN_POINT('Ctrl Pts',(0.00933874702749835,-0.0339153382773248,
0.0684460737368694));
#79500=CARTESIAN_POINT('Ctrl Pts',(0.00933027862647408,-0.0339675558473126,
0.0684858305542207));
#79501=CARTESIAN_POINT('Ctrl Pts',(0.00932197027682019,-0.0340203938281304,
0.0685248359743387));
#79502=CARTESIAN_POINT('Ctrl Pts',(0.00920053384070664,-0.0341934961088741,
0.0685018247078726));
#79503=CARTESIAN_POINT('Ctrl Pts',(0.00908376226624132,-0.0340287516182428,
0.0684795637158362));
#79504=CARTESIAN_POINT('Ctrl Pts',(0.00896617040716373,-0.0338644633275951,
0.068462148003154));
#79505=CARTESIAN_POINT('Ctrl Pts',(0.00919942996230142,-0.0341934961088741,
0.0685001232865991));
#79506=CARTESIAN_POINT('Ctrl Pts',(0.00908262321229166,-0.0340287516182428,
0.0684778851163791));
#79507=CARTESIAN_POINT('Ctrl Pts',(0.00896499715096946,-0.0338644633275951,
0.0684604936598445));
#79508=CARTESIAN_POINT('Ctrl Pts',(0.00901550258770956,-0.0341934961088741,
0.0682166337768639));
#79509=CARTESIAN_POINT('Ctrl Pts',(0.00889283491542242,-0.0340287516182428,
0.0681981981602134));
#79510=CARTESIAN_POINT('Ctrl Pts',(0.0087695101022927,-0.0338644633275951,
0.0681848482444032));
#79511=CARTESIAN_POINT('',(0.00900282677761839,-0.0341764758832387,0.0682147425827495));
#79512=CARTESIAN_POINT('',(0.00901550258770958,-0.0341934961088741,0.0682166337768639));
#79513=CARTESIAN_POINT('Origin',(0.00607042016919592,-0.0345621026741051,
0.0845188009261542));
#79514=CARTESIAN_POINT('Ctrl Pts',(0.00900282677907111,-0.0341764758837478,
0.0682147425838354));
#79515=CARTESIAN_POINT('Ctrl Pts',(0.00899653805236467,-0.0341260050040109,
0.0682572037910506));
#79516=CARTESIAN_POINT('Ctrl Pts',(0.00899035867635939,-0.034074926914751,
0.0682989269279109));
#79517=CARTESIAN_POINT('Ctrl Pts',(0.00897821365523165,-0.0339715436305192,
0.0683809293698836));
#79518=CARTESIAN_POINT('Ctrl Pts',(0.00897225261175909,-0.0339192778237909,
0.0684211775640896));
#79519=CARTESIAN_POINT('Ctrl Pts',(0.00896639895499798,-0.0338664212855148,
0.0684607010967668));
#79520=CARTESIAN_POINT('',(0.00910746627501547,-0.0341934961088841,0.0683583785317415));
#79521=CARTESIAN_POINT('Origin',(0.00812378219310841,-0.0315241814719618,
0.07415));
#79522=CARTESIAN_POINT('',(0.00900282677667802,-0.0342105180190385,0.0682147425833554));
#79523=CARTESIAN_POINT('',(0.00899014695537364,-0.0341934961088739,0.0682128784669065));
#79524=CARTESIAN_POINT('Origin',(0.00611419109639066,-0.0345621711952478,
0.0845305732891805));
#79525=CARTESIAN_POINT('Origin',(0.00708356742671601,-0.0345621034907608,
0.0846688553305032));
#79526=CARTESIAN_POINT('Origin',(0.00703826376628337,-0.0345621719649244,
0.0846674314698193));
#79527=CARTESIAN_POINT('Ctrl Pts',(0.00909133493960705,-0.0346945769586965,
0.068480578165699));
#79528=CARTESIAN_POINT('Ctrl Pts',(0.00897258662937496,-0.0345275153362944,
0.0684603123860367));
#79529=CARTESIAN_POINT('Ctrl Pts',(0.00885317026463046,-0.0343603235965185,
0.0684437758896621));
#79530=CARTESIAN_POINT('Ctrl Pts',(0.00873343975286591,-0.034193496108874,
0.0684310123350075));
#79531=CARTESIAN_POINT('Ctrl Pts',(0.00900840620054512,-0.0346945769586965,
0.0684682959589172));
#79532=CARTESIAN_POINT('Ctrl Pts',(0.00888940063457446,-0.0345275153362944,
0.0684497671548973));
#79533=CARTESIAN_POINT('Ctrl Pts',(0.00876978157383706,-0.0343603235965185,
0.0684349761738923));
#79534=CARTESIAN_POINT('Ctrl Pts',(0.00864990344858244,-0.034193496108874,
0.0684239615029649));
#79535=CARTESIAN_POINT('Ctrl Pts',(0.00892547746148334,-0.0346945769586965,
0.0684560137521339));
#79536=CARTESIAN_POINT('Ctrl Pts',(0.00880621463977408,-0.0345275153362944,
0.0684392219237586));
#79537=CARTESIAN_POINT('Ctrl Pts',(0.00868639288304374,-0.0343603235965185,
0.0684261764581236));
#79538=CARTESIAN_POINT('Ctrl Pts',(0.008566367144299,-0.034193496108874,
0.0684169106709219));
#79539=CARTESIAN_POINT('Ctrl Pts',(0.00884254872242126,-0.0346945769586965,
0.0684437315453535));
#79540=CARTESIAN_POINT('Ctrl Pts',(0.00872302864497345,-0.0345275153362944,
0.0684286766926186));
#79541=CARTESIAN_POINT('Ctrl Pts',(0.00860300419225025,-0.0343603235965185,
0.0684173767423528));
#79542=CARTESIAN_POINT('Ctrl Pts',(0.00848283084001552,-0.034193496108874,
0.0684098598388795));
#79543=CARTESIAN_POINT('',(0.00884254872302055,-0.0346945769586966,0.0684437315454424));
#79544=CARTESIAN_POINT('',(0.00860750220904207,-0.0343667727831449,0.068419019285803));
#79545=CARTESIAN_POINT('Origin',(0.00692295317821726,-0.0345626457063574,
0.0851473958191031));
#79546=CARTESIAN_POINT('Origin',(0.00953704488077846,-0.034193477102925,
0.0574059994983898));
#79547=CARTESIAN_POINT('',(0.00873194505769415,-0.034193496108874,0.0684308861761511));
#79548=CARTESIAN_POINT('',(0.00866966650343826,-0.034193496108884,0.0684256295918562));
#79549=CARTESIAN_POINT('',(0.00896639895474167,-0.0345211942962698,0.0684607010983054));
#79550=CARTESIAN_POINT('Origin',(0.00644781684592441,-0.0345625596119992,
0.0850736648505043));
#79551=CARTESIAN_POINT('',(0.00896619991923768,-0.0346945769586885,0.0684620449742721));
#79552=CARTESIAN_POINT('Origin',(0.0105870954200286,-0.0346945685853848,
0.0575178587106754));
#79553=CARTESIAN_POINT('',(0.00890437432113911,-0.0346945769587026,0.0684528882598673));
#79554=CARTESIAN_POINT('Ctrl Pts',(0.00923479379353328,-0.0345231616327842,
0.0682537593990969));
#79555=CARTESIAN_POINT('Ctrl Pts',(0.00915352241809257,-0.0344132092796988,
0.0682384456683642));
#79556=CARTESIAN_POINT('Ctrl Pts',(0.00907193848344034,-0.0343032738558979,
0.0682248137620447));
#79557=CARTESIAN_POINT('Ctrl Pts',(0.00899014695537362,-0.0341934961088739,
0.0682128784669065));
#79558=CARTESIAN_POINT('Ctrl Pts',(0.00914526249066111,-0.0345231616327842,
0.068323223648495));
#79559=CARTESIAN_POINT('Ctrl Pts',(0.00906494858210052,-0.0344132092796988,
0.0683091439807224));
#79560=CARTESIAN_POINT('Ctrl Pts',(0.00898434759054642,-0.0343032738558979,
0.0682967262692438));
#79561=CARTESIAN_POINT('Ctrl Pts',(0.00890356318268683,-0.0341934961088739,
0.0682859837775601));
#79562=CARTESIAN_POINT('Ctrl Pts',(0.00905573118778895,-0.0345231616327842,
0.0683926878978931));
#79563=CARTESIAN_POINT('Ctrl Pts',(0.00897637474610847,-0.0344132092796988,
0.0683798422930806));
#79564=CARTESIAN_POINT('Ctrl Pts',(0.00889675669765251,-0.0343032738558979,
0.068368638776443));
#79565=CARTESIAN_POINT('Ctrl Pts',(0.00881697941000005,-0.0341934961088739,
0.0683590890882136));
#79566=CARTESIAN_POINT('Ctrl Pts',(0.00896619988491678,-0.0345231616327842,
0.0684621521472912));
#79567=CARTESIAN_POINT('Ctrl Pts',(0.00888780091011641,-0.0344132092796988,
0.0684505406054388));
#79568=CARTESIAN_POINT('Ctrl Pts',(0.0088091658047586,-0.0343032738558979,
0.0684405512836422));
#79569=CARTESIAN_POINT('Ctrl Pts',(0.00873039563731326,-0.0341934961088739,
0.0684321943988672));
#79570=CARTESIAN_POINT('',(0.00886104600654389,-0.0341934961088839,0.0683218823215388));
#79571=CARTESIAN_POINT('Ctrl Pts',(0.00900282677616696,-0.0342105180195411,
0.0682147425867688));
#79572=CARTESIAN_POINT('Ctrl Pts',(0.00899653096611941,-0.0342610556240986,
0.0682572515265621));
#79573=CARTESIAN_POINT('Ctrl Pts',(0.00899034813112771,-0.0343122189869487,
0.0682989976654116));
#79574=CARTESIAN_POINT('Ctrl Pts',(0.00897820299148925,-0.034415811969519,
0.0683810009351696));
#79575=CARTESIAN_POINT('Ctrl Pts',(0.00897224565430533,-0.0344681990450086,
0.0684212245260606));
#79576=CARTESIAN_POINT('Ctrl Pts',(0.00896639895472783,-0.0345211942962507,
0.0684607010983291));
#79577=CARTESIAN_POINT('Ctrl Pts',(0.00884375696040208,-0.0346945769586932,
0.0684453598974565));
#79578=CARTESIAN_POINT('Ctrl Pts',(0.00872581756275587,-0.034529677707698,
0.0684304749285805));
#79579=CARTESIAN_POINT('Ctrl Pts',(0.00860736373340941,-0.0343648066251421,
0.0684204772224062));
#79580=CARTESIAN_POINT('Ctrl Pts',(0.00884254872302953,-0.0346945769586932,
0.0684437315454436));
#79581=CARTESIAN_POINT('Ctrl Pts',(0.00872457566035763,-0.034529677707698,
0.0684288715560203));
#79582=CARTESIAN_POINT('Ctrl Pts',(0.00860608922717556,-0.0343648066251421,
0.0684189001993606));
#79583=CARTESIAN_POINT('Ctrl Pts',(0.00864118383350006,-0.0346945769586932,
0.0681723503329051));
#79584=CARTESIAN_POINT('Ctrl Pts',(0.00851760015628211,-0.034529677707698,
0.0681616534200916));
#79585=CARTESIAN_POINT('Ctrl Pts',(0.00839367996653584,-0.0343648066251421,
0.0681560734745996));
#79586=CARTESIAN_POINT('',(0.00862841428707689,-0.034677539666497,0.0681712587910915));
#79587=CARTESIAN_POINT('',(0.0086411838334966,-0.0346945769586886,0.0681723503329048));
#79588=CARTESIAN_POINT('Origin',(0.00738436647832412,-0.0345626618200292,
0.0847261748801848));
#79589=CARTESIAN_POINT('Ctrl Pts',(0.00862841428853804,-0.0346775396670096,
0.0681712587921676));
#79590=CARTESIAN_POINT('Ctrl Pts',(0.00862480128828991,-0.0346269749928196,
0.0682140647711545));
#79591=CARTESIAN_POINT('Ctrl Pts',(0.00862125253491084,-0.0345757902890802,
0.0682561099954001));
#79592=CARTESIAN_POINT('Ctrl Pts',(0.00861428042754002,-0.0344721681087925,
0.0683387135466323));
#79593=CARTESIAN_POINT('Ctrl Pts',(0.00861085980132514,-0.0344197714289547,
0.0683792394886702));
#79594=CARTESIAN_POINT('Ctrl Pts',(0.00860750220928402,-0.0343667727830614,
0.0684190192857122));
#79595=CARTESIAN_POINT('',(0.00874186627826858,-0.0346945769587026,0.0683080409391836));
#79596=CARTESIAN_POINT('Origin',(0.00812378219310841,-0.0315241814719618,
0.07415));
#79597=CARTESIAN_POINT('',(0.00862841428624165,-0.0347116136489629,0.0681712587922044));
#79598=CARTESIAN_POINT('',(0.00861564243684597,-0.0346945769586885,0.0681701945265211));
#79599=CARTESIAN_POINT('Origin',(0.00742963708757855,-0.034562669108892,
0.0847281199836829));
#79600=CARTESIAN_POINT('Origin',(0.00708001546907962,-0.0345626625512408,
0.0847004881000318));
#79601=CARTESIAN_POINT('Origin',(0.00703505963744553,-0.0345626698804197,
0.0846948142349712));
#79602=CARTESIAN_POINT('Ctrl Pts',(0.00877034420266972,-0.0352450361874068,
0.068435044165226));
#79603=CARTESIAN_POINT('Ctrl Pts',(0.00855480110646341,-0.0349452760959493,
0.0684106586788882));
#79604=CARTESIAN_POINT('Ctrl Pts',(0.00833803353089584,-0.034644428984174,
0.0684025780570867));
#79605=CARTESIAN_POINT('Ctrl Pts',(0.00876782953156976,-0.0352450361874068,
0.0684348160112013));
#79606=CARTESIAN_POINT('Ctrl Pts',(0.0085522778303932,-0.0349452760959493,
0.0684105253672403));
#79607=CARTESIAN_POINT('Ctrl Pts',(0.00833550881821709,-0.034644428984174,
0.06840253996654));
#79608=CARTESIAN_POINT('Ctrl Pts',(0.00851885219493944,-0.0352450361874068,
0.0684122265038036));
#79609=CARTESIAN_POINT('Ctrl Pts',(0.00830244851651108,-0.0349452760959493,
0.0683973261941819));
#79610=CARTESIAN_POINT('Ctrl Pts',(0.0080855372658654,-0.034644428984174,
0.068398768625282));
#79611=CARTESIAN_POINT('Ctrl Pts',(0.00851636242157314,-0.0352450361874068,
0.0684120006087297));
#79612=CARTESIAN_POINT('Ctrl Pts',(0.00829995022337226,-0.0349452760959493,
0.0683971942024513));
#79613=CARTESIAN_POINT('Ctrl Pts',(0.00808303755034189,-0.034644428984174,
0.0683987309118695));
#79614=CARTESIAN_POINT('',(0.00848286328436634,-0.0351951634053313,0.0684098594901857));
#79615=CARTESIAN_POINT('',(0.00824669644126924,-0.0348678972934172,0.0683999550361109));
#79616=CARTESIAN_POINT('Origin',(0.00831054463921628,-0.0345636767887066,
0.0851542556470295));
#79617=CARTESIAN_POINT('Origin',(0.00848283195180577,-0.0346946199326463,
0.0573526369146102));
#79618=CARTESIAN_POINT('',(0.00837163887693946,-0.0346945769330288,0.0684039846796013));
#79619=CARTESIAN_POINT('',(0.00830915314282402,-0.0346945769458128,0.0684026489702012));
#79620=CARTESIAN_POINT('',(0.00860750220925616,-0.0350221583435276,0.0684190192858483));
#79621=CARTESIAN_POINT('Origin',(0.00783078680931817,-0.0345628458717247,
0.085185493723715));
#79622=CARTESIAN_POINT('',(0.00860740119445584,-0.0351951360298762,0.0684202520424167));
#79623=CARTESIAN_POINT('Origin',(0.00953415430134055,-0.0351951838366932,
0.0574403170438433));
#79624=CARTESIAN_POINT('',(0.00848283084063969,-0.035195137132875,0.0684098598388155));
#79625=CARTESIAN_POINT('Ctrl Pts',(0.00886237250191847,-0.0350241211494343,
0.0681956331691984));
#79626=CARTESIAN_POINT('Ctrl Pts',(0.00878035354020962,-0.0349144232818962,
0.0681854593905283));
#79627=CARTESIAN_POINT('Ctrl Pts',(0.00869807518692388,-0.0348045283579412,
0.0681769749129075));
#79628=CARTESIAN_POINT('Ctrl Pts',(0.00861564242577058,-0.0346945769439158,
0.06817019452561));
#79629=CARTESIAN_POINT('Ctrl Pts',(0.00877737955818422,-0.0350241211494343,
0.0682705820939291));
#79630=CARTESIAN_POINT('Ctrl Pts',(0.00869639298718329,-0.0349144232818962,
0.0682615790582105));
#79631=CARTESIAN_POINT('Ctrl Pts',(0.00861517184263443,-0.0348045283579412,
0.0682542446840336));
#79632=CARTESIAN_POINT('Ctrl Pts',(0.00853381980891576,-0.0346945769439158,
0.068248592237145));
#79633=CARTESIAN_POINT('Ctrl Pts',(0.00869238661444998,-0.0350241211494343,
0.0683455310186597));
#79634=CARTESIAN_POINT('Ctrl Pts',(0.00861243243415695,-0.0349144232818962,
0.0683376987258926));
#79635=CARTESIAN_POINT('Ctrl Pts',(0.00853226849834498,-0.0348045283579412,
0.0683315144551596));
#79636=CARTESIAN_POINT('Ctrl Pts',(0.00845199719206094,-0.0346945769439158,
0.06832698994868));
#79637=CARTESIAN_POINT('Ctrl Pts',(0.00860739367071574,-0.0350241211494343,
0.0684204799433904));
#79638=CARTESIAN_POINT('Ctrl Pts',(0.00852847188113062,-0.0349144232818962,
0.0684138183935748));
#79639=CARTESIAN_POINT('Ctrl Pts',(0.00844936515405553,-0.0348045283579412,
0.0684087842262857));
#79640=CARTESIAN_POINT('Ctrl Pts',(0.00837017457520612,-0.0346945769439158,
0.068405387660215));
#79641=CARTESIAN_POINT('',(0.00849364065719382,-0.0346945769458128,0.0682870896029957));
#79642=CARTESIAN_POINT('Ctrl Pts',(0.00862841428596019,-0.0347116136492814,
0.0681712587954768));
#79643=CARTESIAN_POINT('Ctrl Pts',(0.00862480270768245,-0.0347621546531972,
0.0682140477741575));
#79644=CARTESIAN_POINT('Ctrl Pts',(0.00862125463071028,-0.0348133084096332,
0.0682560844069658));
#79645=CARTESIAN_POINT('Ctrl Pts',(0.00861428251825559,-0.0349168561544578,
0.0683386880633838));
#79646=CARTESIAN_POINT('Ctrl Pts',(0.00861086124826331,-0.0349692089015921,
0.0683792223222317));
#79647=CARTESIAN_POINT('Ctrl Pts',(0.00860750220923327,-0.0350221583435,
0.0684190192858831));
#79648=CARTESIAN_POINT('Ctrl Pts',(0.00848377467691702,-0.0351951371254934,
0.06841097769077));
#79649=CARTESIAN_POINT('Ctrl Pts',(0.00836512399177465,-0.0350307338985347,
0.068403535072054));
#79650=CARTESIAN_POINT('Ctrl Pts',(0.00824626708148386,-0.0348659306906634,
0.0684010027738433));
#79651=CARTESIAN_POINT('Ctrl Pts',(0.00848283084063733,-0.0351951371254934,
0.0684098598389319));
#79652=CARTESIAN_POINT('Ctrl Pts',(0.00836415704460963,-0.0350307338985347,
0.0684024367334387));
#79653=CARTESIAN_POINT('Ctrl Pts',(0.00824527784968418,-0.0348659306906634,
0.0683999248869747));
#79654=CARTESIAN_POINT('Ctrl Pts',(0.00832464289630539,-0.0351951371254934,
0.0682225067056039));
#79655=CARTESIAN_POINT('Ctrl Pts',(0.0082020956918058,-0.0350307338985347,
0.0682183540366006));
#79656=CARTESIAN_POINT('Ctrl Pts',(0.00807948156888189,-0.0348659306906634,
0.068219269924209));
#79657=CARTESIAN_POINT('Origin',(0.00836035143919025,-0.0308609188508941,
0.0630829868146784));
#79658=CARTESIAN_POINT('',(0.00841386446357033,-0.0351951371254934,0.0683281780970498));
#79659=CARTESIAN_POINT('Origin',(0.00824466076921519,-0.03518404674411,
0.0751196050847292));
#79660=CARTESIAN_POINT('Origin',(0.00758442489567276,-0.0352322614919394,
0.0621970607340446));
#79661=CARTESIAN_POINT('',(0.00801004046581113,-0.0351951142564661,0.0683997932730299));
#79662=CARTESIAN_POINT('',(0.00788546184042353,-0.0351951372916786,0.0684049409568311));
#79663=CARTESIAN_POINT('Origin',(0.00784137974656666,-0.0352875121444807,
0.0743403964868405));
#79664=CARTESIAN_POINT('Origin',(0.015541196766919,-0.0298325076521634,
0.0752801111993773));
#79665=CARTESIAN_POINT('Origin',(0.0109540556667107,-0.0338732909226762,
0.0662609219776647));
#79666=CARTESIAN_POINT('Ctrl Pts',(0.0114119592548226,-0.0321934096636941,
0.0694313108434516));
#79667=CARTESIAN_POINT('Ctrl Pts',(0.0113274969660167,-0.0320508460844714,
0.0693724540399162));
#79668=CARTESIAN_POINT('Ctrl Pts',(0.0112415169958787,-0.0319086045663848,
0.0693159109496467));
#79669=CARTESIAN_POINT('Ctrl Pts',(0.0111542144973951,-0.0317669892869059,
0.069261788078814));
#79670=CARTESIAN_POINT('Ctrl Pts',(0.0113421406583195,-0.0321934096636941,
0.0693848802909014));
#79671=CARTESIAN_POINT('Ctrl Pts',(0.0112568472847337,-0.0320508460844714,
0.069327273206995));
#79672=CARTESIAN_POINT('Ctrl Pts',(0.011170070433957,-0.0319086045663848,
0.0692720012236699));
#79673=CARTESIAN_POINT('Ctrl Pts',(0.0110820067494801,-0.0317669892869059,
0.0692191679689228));
#79674=CARTESIAN_POINT('Ctrl Pts',(0.0112723220618163,-0.0321934096636941,
0.0693384497383512));
#79675=CARTESIAN_POINT('Ctrl Pts',(0.0111861976034507,-0.0320508460844714,
0.0692820923740737));
#79676=CARTESIAN_POINT('Ctrl Pts',(0.0110986238720354,-0.0319086045663848,
0.0692280914976931));
#79677=CARTESIAN_POINT('Ctrl Pts',(0.0110097990015652,-0.0317669892869059,
0.0691765478590318));
#79678=CARTESIAN_POINT('Ctrl Pts',(0.0112025034653132,-0.0321934096636941,
0.0692920191858011));
#79679=CARTESIAN_POINT('Ctrl Pts',(0.0111155479221677,-0.0320508460844714,
0.0692369115411526));
#79680=CARTESIAN_POINT('Ctrl Pts',(0.0110271773101137,-0.0319086045663848,
0.0691841817717163));
#79681=CARTESIAN_POINT('Ctrl Pts',(0.0109375912536502,-0.0317669892869059,
0.0691339277491406));
#79682=CARTESIAN_POINT('',(0.0112037525338003,-0.0321934096636941,0.0692928498375633));
#79683=CARTESIAN_POINT('',(0.0110015980574996,-0.0318665617511295,0.0691704115792809));
#79684=CARTESIAN_POINT('Origin',(0.00174203632914428,-0.0326371944419843,
0.0830657882059943));
#79685=CARTESIAN_POINT('Origin',(0.0164862628977425,-0.0316939261508995,
0.0596800985292627));
#79686=CARTESIAN_POINT('',(0.0113083445140224,-0.0320197221621859,0.069360829717921));
#79687=CARTESIAN_POINT('Ctrl Pts',(0.011308221706302,-0.0320197392094768,
0.0693606913953178));
#79688=CARTESIAN_POINT('Ctrl Pts',(0.0112838521384082,-0.0319792716576065,
0.0693444879823917));
#79689=CARTESIAN_POINT('Ctrl Pts',(0.011259248102668,-0.0319386439829744,
0.06932839658914));
#79690=CARTESIAN_POINT('Ctrl Pts',(0.0112343791402907,-0.0318979099381675,
0.0693124074007847));
#79691=CARTESIAN_POINT('Ctrl Pts',(0.0112095106694653,-0.0318571766984965,
0.0692964185284665));
#79692=CARTESIAN_POINT('Ctrl Pts',(0.0111845046438307,-0.0318163871833603,
0.0692806116242346));
#79693=CARTESIAN_POINT('Ctrl Pts',(0.011159448955242,-0.0317755399638303,
0.0692650380809617));
#79694=CARTESIAN_POINT('',(0.0113078380024955,-0.0321934096636183,0.0693620684421445));
#79695=CARTESIAN_POINT('Origin',(0.0125300026055346,-0.0324016312812858,
0.0674874531578453));
#79696=CARTESIAN_POINT('',(0.0112557952681579,-0.0321934096636663,0.0693274591398639));
#79697=CARTESIAN_POINT('Ctrl Pts',(0.0112041525739548,-0.0321934096636618,
0.0692948382176211));
#79698=CARTESIAN_POINT('Ctrl Pts',(0.011137196109084,-0.0320835708272592,
0.0692523575093689));
#79699=CARTESIAN_POINT('Ctrl Pts',(0.0110693993456345,-0.0319739230346488,
0.0692112871022145));
#79700=CARTESIAN_POINT('Ctrl Pts',(0.0110008530576767,-0.0318646057455572,
0.0691716728857455));
#79701=CARTESIAN_POINT('Ctrl Pts',(0.0111818019275799,-0.0321934096636618,
0.0691837454034018));
#79702=CARTESIAN_POINT('Ctrl Pts',(0.0111133134062204,-0.0320835708272592,
0.0691415729279822));
#79703=CARTESIAN_POINT('Ctrl Pts',(0.0110439918537996,-0.0319739230346488,
0.0691008422807022));
#79704=CARTESIAN_POINT('Ctrl Pts',(0.0109739299618877,-0.0318646057455572,
0.0690615987667271));
#79705=CARTESIAN_POINT('Ctrl Pts',(0.011159451281205,-0.0321934096636618,
0.0690726525891825));
#79706=CARTESIAN_POINT('Ctrl Pts',(0.0110894307033567,-0.0320835708272592,
0.0690307883465955));
#79707=CARTESIAN_POINT('Ctrl Pts',(0.0110185843619647,-0.0319739230346488,
0.06899039745919));
#79708=CARTESIAN_POINT('Ctrl Pts',(0.0109470068660988,-0.0318646057455572,
0.0689515246477087));
#79709=CARTESIAN_POINT('Ctrl Pts',(0.0111371006348302,-0.0321934096636618,
0.0689615597749632));
#79710=CARTESIAN_POINT('Ctrl Pts',(0.0110655480004931,-0.0320835708272592,
0.0689200037652088));
#79711=CARTESIAN_POINT('Ctrl Pts',(0.0109931768701297,-0.0319739230346488,
0.0688799526376777));
#79712=CARTESIAN_POINT('Ctrl Pts',(0.0109200837703098,-0.0318646057455572,
0.0688414505286903));
#79713=CARTESIAN_POINT('',(0.0111260111583635,-0.0321763980308461,0.0689551351107169));
#79714=CARTESIAN_POINT('',(0.0111371006348019,-0.0321934096636184,0.0689615597749468));
#79715=CARTESIAN_POINT('Origin',(0.00232053340556324,-0.0326386231341034,
0.0829654760549868));
#79716=CARTESIAN_POINT('Ctrl Pts',(0.01112601115677,-0.0321763980306278,
0.0689551351134602));
#79717=CARTESIAN_POINT('Ctrl Pts',(0.0111045357659456,-0.032125959617482,
0.0689922947555354));
#79718=CARTESIAN_POINT('Ctrl Pts',(0.0110834324641401,-0.0320749164631395,
0.0690288105585962));
#79719=CARTESIAN_POINT('Ctrl Pts',(0.0110419530552891,-0.0319716057793937,
0.0691005838734109));
#79720=CARTESIAN_POINT('Ctrl Pts',(0.0110215931100143,-0.031919378669013,
0.069135813419871));
#79721=CARTESIAN_POINT('Ctrl Pts',(0.0110015980565636,-0.0318665617525324,
0.0691704115808816));
#79722=CARTESIAN_POINT('',(0.0111704265843111,-0.0321934096636663,0.0691272048062651));
#79723=CARTESIAN_POINT('Origin',(0.00812378219310841,-0.0315241814719618,
0.07415));
#79724=CARTESIAN_POINT('',(0.0111260111585486,-0.0322104233323797,0.0689551351103958));
#79725=CARTESIAN_POINT('',(0.0111149079858696,-0.0321934096636183,0.0689487341452394));
#79726=CARTESIAN_POINT('Origin',(0.00235624051314064,-0.0326387238286708,
0.0829934069770395));
#79727=CARTESIAN_POINT('Origin',(0.0033828877309766,-0.0326386239491269,
0.0835794368688629));
#79728=CARTESIAN_POINT('Origin',(0.0033408619234511,-0.0326387246148537,
0.0835624393439663));
#79729=CARTESIAN_POINT('Ctrl Pts',(0.0111399791707251,-0.0327445246967096,
0.0692529926697814));
#79730=CARTESIAN_POINT('Ctrl Pts',(0.0109552855199338,-0.032443687833936,
0.0691392349410836));
#79731=CARTESIAN_POINT('Ctrl Pts',(0.010762547867239,-0.0321434074405927,
0.0690397122667085));
#79732=CARTESIAN_POINT('Ctrl Pts',(0.0109243168805336,-0.0327445246967096,
0.0691265419814108));
#79733=CARTESIAN_POINT('Ctrl Pts',(0.0107348540640651,-0.032443687833936,
0.0690209180889579));
#79734=CARTESIAN_POINT('Ctrl Pts',(0.0105379734681785,-0.0321434074405927,
0.0689298653765085));
#79735=CARTESIAN_POINT('',(0.0108926919338008,-0.0326943950436612,0.0691090413760972));
#79736=CARTESIAN_POINT('',(0.0106832484016998,-0.0323666188837389,0.0689995381054628));
#79737=CARTESIAN_POINT('Origin',(0.00286600315301682,-0.0326395579112592,
0.0838799697641049));
#79738=CARTESIAN_POINT('Origin',(0.0155983125060639,-0.0321933825603078,
0.0591088598334281));
#79739=CARTESIAN_POINT('',(0.0107945839480072,-0.0321934096532689,0.0690563821322444));
#79740=CARTESIAN_POINT('',(0.0107386138880983,-0.0321934096584275,0.0690285684172921));
#79741=CARTESIAN_POINT('',(0.0110015980579694,-0.0325210109756238,0.069170411578458));
#79742=CARTESIAN_POINT('Origin',(0.00245738055630698,-0.03263931291576,
0.0836265688898258));
#79743=CARTESIAN_POINT('',(0.0110009182856955,-0.0326943950436593,0.0691715878128933));
#79744=CARTESIAN_POINT('Origin',(0.0165362565107906,-0.0326943765538283,
0.0595935949407701));
#79745=CARTESIAN_POINT('',(0.0109468051097582,-0.0326943950436702,0.0691403145945052));
#79746=CARTESIAN_POINT('Ctrl Pts',(0.0113273257135278,-0.0325229783203769,
0.0690768048615494));
#79747=CARTESIAN_POINT('Ctrl Pts',(0.0112573918294877,-0.032413025309245,
0.0690326440841773));
#79748=CARTESIAN_POINT('Ctrl Pts',(0.0111865550298829,-0.032303122220807,
0.0689899366768802));
#79749=CARTESIAN_POINT('Ctrl Pts',(0.0111149079819824,-0.0321934096576658,
0.068948734143004));
#79750=CARTESIAN_POINT('Ctrl Pts',(0.0112185100910129,-0.0325229783203769,
0.0691084324212555));
#79751=CARTESIAN_POINT('Ctrl Pts',(0.0111490121921917,-0.032413025309245,
0.0690657716648601));
#79752=CARTESIAN_POINT('Ctrl Pts',(0.011078642341541,-0.032303122220807,
0.0690245550321178));
#79753=CARTESIAN_POINT('Ctrl Pts',(0.0110074925408185,-0.0321934096576658,
0.0689848321379043));
#79754=CARTESIAN_POINT('Ctrl Pts',(0.011109694468498,-0.0325229783203769,
0.0691400599809615));
#79755=CARTESIAN_POINT('Ctrl Pts',(0.0110406325548958,-0.032413025309245,
0.0690988992455428));
#79756=CARTESIAN_POINT('Ctrl Pts',(0.010970729653199,-0.032303122220807,
0.0690591733873553));
#79757=CARTESIAN_POINT('Ctrl Pts',(0.0109000770996546,-0.0321934096576658,
0.0690209301328046));
#79758=CARTESIAN_POINT('Ctrl Pts',(0.0110008788459832,-0.0325229783203769,
0.0691716875406675));
#79759=CARTESIAN_POINT('Ctrl Pts',(0.0109322529175998,-0.032413025309245,
0.0691320268262256));
#79760=CARTESIAN_POINT('Ctrl Pts',(0.010862816964857,-0.032303122220807,
0.0690937917425929));
#79761=CARTESIAN_POINT('Ctrl Pts',(0.0107926616584907,-0.0321934096576658,
0.0690570281277049));
#79762=CARTESIAN_POINT('',(0.0109547459674448,-0.0321934096584275,0.0690025581388497));
#79763=CARTESIAN_POINT('Ctrl Pts',(0.0111260111568023,-0.0322104233328951,
0.0689551351134042));
#79764=CARTESIAN_POINT('Ctrl Pts',(0.0111045066664953,-0.0322609421830959,
0.0689923451073623));
#79765=CARTESIAN_POINT('Ctrl Pts',(0.011083389149112,-0.0323120888239857,
0.0690288855081357));
#79766=CARTESIAN_POINT('Ctrl Pts',(0.0110419094261723,-0.0324156524631821,
0.0691006593664293));
#79767=CARTESIAN_POINT('Ctrl Pts',(0.0110215642710091,-0.0324680267167318,
0.0691358633210402));
#79768=CARTESIAN_POINT('Ctrl Pts',(0.011001598057944,-0.0325210109755912,
0.0691704115784933));
#79769=CARTESIAN_POINT('Origin',(0.0144121497996153,-0.0262834582512331,
0.0788786169947828));
#79770=CARTESIAN_POINT('Origin',(0.0182740287853487,-0.0342770848922325,
0.0674570010021419));
#79771=CARTESIAN_POINT('Ctrl Pts',(0.0108932159087258,-0.0326943950436604,
0.0691110002382951));
#79772=CARTESIAN_POINT('Ctrl Pts',(0.0108237690479174,-0.0325844576448134,
0.0690728322512219));
#79773=CARTESIAN_POINT('Ctrl Pts',(0.0107535278956968,-0.0324744968375322,
0.0690360978378822));
#79774=CARTESIAN_POINT('Ctrl Pts',(0.01068258309831,-0.0323646534831895,
0.0690008428232186));
#79775=CARTESIAN_POINT('Ctrl Pts',(0.0108639338331196,-0.0326943950436604,
0.0690015302075579));
#79776=CARTESIAN_POINT('Ctrl Pts',(0.0107929782701189,-0.0325844576448134,
0.0689637657823671));
#79777=CARTESIAN_POINT('Ctrl Pts',(0.0107212366552543,-0.0324744968375322,
0.0689274661619053));
#79778=CARTESIAN_POINT('Ctrl Pts',(0.0106488015495679,-0.0323646534831895,
0.0688926765875164));
#79779=CARTESIAN_POINT('Ctrl Pts',(0.0108346517575133,-0.0326943950436604,
0.0688920601768208));
#79780=CARTESIAN_POINT('Ctrl Pts',(0.0107621874923204,-0.0325844576448134,
0.0688546993135122));
#79781=CARTESIAN_POINT('Ctrl Pts',(0.0106889454148117,-0.0324744968375322,
0.0688188344859283));
#79782=CARTESIAN_POINT('Ctrl Pts',(0.0106150200008259,-0.0323646534831895,
0.0687845103518142));
#79783=CARTESIAN_POINT('Ctrl Pts',(0.0108053696819071,-0.0326943950436604,
0.0687825901460836));
#79784=CARTESIAN_POINT('Ctrl Pts',(0.010731396714522,-0.0325844576448134,
0.0687456328446574));
#79785=CARTESIAN_POINT('Ctrl Pts',(0.0106566541743692,-0.0324744968375322,
0.0687102028099514));
#79786=CARTESIAN_POINT('Ctrl Pts',(0.0105812384520838,-0.0323646534831895,
0.0686763441161119));
#79787=CARTESIAN_POINT('',(0.0107938986801022,-0.0326773559991343,0.0687768744732653));
#79788=CARTESIAN_POINT('',(0.0108053696819065,-0.0326943950436595,0.0687825901460834));
#79789=CARTESIAN_POINT('Origin',(0.00344927916746203,-0.0326395670565505,
0.0836694858002616));
#79790=CARTESIAN_POINT('Ctrl Pts',(0.0107938986786049,-0.0326773559987421,
0.0687768744762628));
#79791=CARTESIAN_POINT('Ctrl Pts',(0.0107747835676132,-0.0326267922585945,
0.0688153401729154));
#79792=CARTESIAN_POINT('Ctrl Pts',(0.0107560072581608,-0.0325756109579297,
0.0688531240928712));
#79793=CARTESIAN_POINT('Ctrl Pts',(0.0107191162627669,-0.032471998546237,
0.0689273605353723));
#79794=CARTESIAN_POINT('Ctrl Pts',(0.010701016372794,-0.0324196091621769,
0.0689637832837125));
#79795=CARTESIAN_POINT('Ctrl Pts',(0.0106832484016781,-0.0323666188837756,
0.0689995381055065));
#79796=CARTESIAN_POINT('',(0.0108490308078636,-0.0326943950436702,0.0689458157611003));
#79797=CARTESIAN_POINT('Origin',(0.00812378219310841,-0.0315241814719618,
0.07415));
#79798=CARTESIAN_POINT('',(0.0107938986800819,-0.0327114338380068,0.0687768744733054));
#79799=CARTESIAN_POINT('',(0.0107824154971443,-0.0326943950436593,0.0687711833127829));
#79800=CARTESIAN_POINT('Origin',(0.00349019476756723,-0.0326395672881448,
0.0836889521683736));
#79801=CARTESIAN_POINT('Origin',(0.00335929596177808,-0.0326395676539919,
0.0836247712427188));
#79802=CARTESIAN_POINT('Origin',(0.00331907223276828,-0.0326395680355474,
0.0836039130573845));
#79803=CARTESIAN_POINT('Ctrl Pts',(0.0108265071376824,-0.0332451089994433,
0.0690732487874648));
#79804=CARTESIAN_POINT('Ctrl Pts',(0.0106350343330425,-0.0329451141710254,
0.0689713138484372));
#79805=CARTESIAN_POINT('Ctrl Pts',(0.0104364273261115,-0.0326442513127493,
0.0688840910102056));
#79806=CARTESIAN_POINT('Ctrl Pts',(0.0106033297350171,-0.0332451089994433,
0.0689605906899326));
#79807=CARTESIAN_POINT('Ctrl Pts',(0.0104076079607119,-0.0329451141710254,
0.0688670730243603));
#79808=CARTESIAN_POINT('Ctrl Pts',(0.0102053980784369,-0.0326442513127493,
0.0687885635967636));
#79809=CARTESIAN_POINT('Ctrl Pts',(0.0106010979609905,-0.0332451089994433,
0.0689594641089573));
#79810=CARTESIAN_POINT('Ctrl Pts',(0.0104053336969887,-0.0329451141710254,
0.0688660306161196));
#79811=CARTESIAN_POINT('Ctrl Pts',(0.0102030877859601,-0.0326442513127493,
0.0687876083226291));
#79812=CARTESIAN_POINT('',(0.0105707037120035,-0.0331951640388616,0.0689451272752959));
#79813=CARTESIAN_POINT('',(0.0103547976911229,-0.0328677532355004,0.0688489911415425));
#79814=CARTESIAN_POINT('Origin',(0.00414093313941138,-0.032640280828004,
0.0844270618394905));
#79815=CARTESIAN_POINT('Origin',(0.0146431817190043,-0.0326944278779173,
0.0586585963809617));
#79816=CARTESIAN_POINT('',(0.0104694828127754,-0.0326943950436593,0.0688987321908995));
#79817=CARTESIAN_POINT('',(0.010411876761808,-0.0326943950436693,0.0688744877504997));
#79818=CARTESIAN_POINT('',(0.0106832484017023,-0.0330220786163545,0.0689995381054641));
#79819=CARTESIAN_POINT('Origin',(0.00368655644724267,-0.0326396682762806,
0.0842699171074804));
#79820=CARTESIAN_POINT('',(0.0106826438271766,-0.0331951640388587,0.0690007547021243));
#79821=CARTESIAN_POINT('Origin',(0.0155919445563444,-0.0331952026560276,
0.0591216790399452));
#79822=CARTESIAN_POINT('',(0.0106266737696,-0.0331951640388701,0.0689729409887201));
#79823=CARTESIAN_POINT('Ctrl Pts',(0.0110024548506785,-0.0330240426238172,
0.0688856630302979));
#79824=CARTESIAN_POINT('Ctrl Pts',(0.0109299334801259,-0.032914277406352,
0.068846006509885));
#79825=CARTESIAN_POINT('Ctrl Pts',(0.0108565561439731,-0.0328043479726691,
0.0688078294385581));
#79826=CARTESIAN_POINT('Ctrl Pts',(0.0107824154971443,-0.0326943950436593,
0.0687711833127828));
#79827=CARTESIAN_POINT('Ctrl Pts',(0.0108958398939461,-0.0330240426238172,
0.0689240607774371));
#79828=CARTESIAN_POINT('Ctrl Pts',(0.0108238474897694,-0.032914277406352,
0.0688858729819231));
#79829=CARTESIAN_POINT('Ctrl Pts',(0.010751029746348,-0.0328043479726691,
0.0688491544324955));
#79830=CARTESIAN_POINT('Ctrl Pts',(0.0106774786531833,-0.0326943950436593,
0.0688139547374019));
#79831=CARTESIAN_POINT('Ctrl Pts',(0.0107892249372137,-0.0330240426238172,
0.0689624585245763));
#79832=CARTESIAN_POINT('Ctrl Pts',(0.010717761499413,-0.032914277406352,
0.0689257394539612));
#79833=CARTESIAN_POINT('Ctrl Pts',(0.0106455033487229,-0.0328043479726691,
0.0688904794264329));
#79834=CARTESIAN_POINT('Ctrl Pts',(0.0105725418092224,-0.0326943950436593,
0.0688567261620209));
#79835=CARTESIAN_POINT('Ctrl Pts',(0.0106826099804813,-0.0330240426238172,
0.0690008562717155));
#79836=CARTESIAN_POINT('Ctrl Pts',(0.0106116755090565,-0.032914277406352,
0.0689656059259994));
#79837=CARTESIAN_POINT('Ctrl Pts',(0.0105399769510978,-0.0328043479726691,
0.0689318044203703));
#79838=CARTESIAN_POINT('Ctrl Pts',(0.0104676049652615,-0.0326943950436593,
0.06889949758664));
#79839=CARTESIAN_POINT('',(0.0106259491549698,-0.0326943950436694,0.0688349577518512));
#79840=CARTESIAN_POINT('Ctrl Pts',(0.0107938986786009,-0.0327114338383348,
0.0687768744762708));
#79841=CARTESIAN_POINT('Ctrl Pts',(0.010774786747092,-0.0327619876830663,
0.0688153337747907));
#79842=CARTESIAN_POINT('Ctrl Pts',(0.010756011990653,-0.0328131562603672,
0.0688531145695884));
#79843=CARTESIAN_POINT('Ctrl Pts',(0.0107191210291131,-0.0329167375858782,
0.0689273509439647));
#79844=CARTESIAN_POINT('Ctrl Pts',(0.0107010195233077,-0.0329691088920629,
0.068963776943875));
#79845=CARTESIAN_POINT('Ctrl Pts',(0.0106832484016786,-0.0330220786163187,
0.0689995381055054));
#79846=CARTESIAN_POINT('Ctrl Pts',(0.0105713497540828,-0.0331951640388604,
0.0689470496783287));
#79847=CARTESIAN_POINT('Ctrl Pts',(0.0104637820920036,-0.0330306422010619,
0.0688964477882399));
#79848=CARTESIAN_POINT('Ctrl Pts',(0.0103542149164065,-0.0328657861914644,
0.0688503350217061));
#79849=CARTESIAN_POINT('Ctrl Pts',(0.0105707037120064,-0.0331951640388604,
0.0689451272752974));
#79850=CARTESIAN_POINT('Ctrl Pts',(0.010463096305477,-0.0330306422010619,
0.0688945387417142));
#79851=CARTESIAN_POINT('Ctrl Pts',(0.0103534899714295,-0.0328657861914644,
0.0688484409629531));
#79852=CARTESIAN_POINT('Ctrl Pts',(0.0104630557282946,-0.0331951640388604,
0.0686248032317774));
#79853=CARTESIAN_POINT('Ctrl Pts',(0.0103488258275382,-0.0330306422010619,
0.06857644025124));
#79854=CARTESIAN_POINT('Ctrl Pts',(0.0102326946425863,-0.0328657861914644,
0.0685328398384559));
#79855=CARTESIAN_POINT('',(0.0104512484729271,-0.0331781648281907,0.0686198191067445));
#79856=CARTESIAN_POINT('',(0.0104630557282936,-0.0331951640388588,0.0686248032317769));
#79857=CARTESIAN_POINT('Origin',(0.00470451661030899,-0.032641209230929,
0.0841105116536204));
#79858=CARTESIAN_POINT('Ctrl Pts',(0.0104512484738955,-0.033178164828644,
0.0686198191083014));
#79859=CARTESIAN_POINT('Ctrl Pts',(0.0104345749032635,-0.0331276811546787,
0.0686594364102444));
#79860=CARTESIAN_POINT('Ctrl Pts',(0.0104182024368507,-0.0330765663497806,
0.0686983383595207));
#79861=CARTESIAN_POINT('Ctrl Pts',(0.0103860454961961,-0.0329730614463516,
0.068774744913422));
#79862=CARTESIAN_POINT('Ctrl Pts',(0.0103702740077172,-0.0329207133374511,
0.0688122186493851));
#79863=CARTESIAN_POINT('Ctrl Pts',(0.010354797707384,-0.0328677532289362,
0.0688489911389325));
#79864=CARTESIAN_POINT('',(0.0105168797201585,-0.0331951640388701,0.0687849652535464));
#79865=CARTESIAN_POINT('Origin',(0.00812378219310841,-0.0315241814719618,
0.07415));
#79866=CARTESIAN_POINT('',(0.010451248471729,-0.0332121607144433,0.0686198191079238));
#79867=CARTESIAN_POINT('',(0.0104394305973826,-0.0331951640388587,0.0686148602124429));
#79868=CARTESIAN_POINT('Origin',(0.00474872370061134,-0.032641365599196,
0.0841206079314246));
#79869=CARTESIAN_POINT('Origin',(0.00339152961651254,-0.032641209865241,
0.0835579214911582));
#79870=CARTESIAN_POINT('Origin',(0.00335340817838117,-0.0326413662232479,
0.0835333653520963));
#79871=CARTESIAN_POINT('Ctrl Pts',(0.0105024210477226,-0.0337436976235975,
0.0689135697083491));
#79872=CARTESIAN_POINT('Ctrl Pts',(0.0104553238000768,-0.0336723290703325,
0.0688921758699981));
#79873=CARTESIAN_POINT('Ctrl Pts',(0.010407849363936,-0.033601104548885,
0.0688716326237038));
#79874=CARTESIAN_POINT('Ctrl Pts',(0.0102562728934941,-0.0333736987606857,
0.0688060421076739));
#79875=CARTESIAN_POINT('Ctrl Pts',(0.0101011822470827,-0.0331450831799191,
0.0687492580114819));
#79876=CARTESIAN_POINT('Ctrl Pts',(0.010272610530698,-0.0337436976235975,
0.0688151465085186));
#79877=CARTESIAN_POINT('Ctrl Pts',(0.0102246280498765,-0.0336723290703325,
0.0687958196207865));
#79878=CARTESIAN_POINT('Ctrl Pts',(0.0101763057016965,-0.033601104548885,
0.0687773589132818));
#79879=CARTESIAN_POINT('Ctrl Pts',(0.0100220220160757,-0.0333736987606857,
0.0687184175310795));
#79880=CARTESIAN_POINT('Ctrl Pts',(0.00986461018139935,-0.0331450831799191,
0.0686684269670849));
#79881=CARTESIAN_POINT('Ctrl Pts',(0.0102703124255278,-0.0337436976235975,
0.0688141622765203));
#79882=CARTESIAN_POINT('Ctrl Pts',(0.0102223210923745,-0.0336723290703325,
0.0687948560582944));
#79883=CARTESIAN_POINT('Ctrl Pts',(0.0101739902650741,-0.033601104548885,
0.0687764161761776));
#79884=CARTESIAN_POINT('Ctrl Pts',(0.0100196795073015,-0.0333736987606857,
0.0687175412853135));
#79885=CARTESIAN_POINT('Ctrl Pts',(0.00986224446074252,-0.0331450831799191,
0.0686676186566409));
#79886=CARTESIAN_POINT('',(0.0102390586088509,-0.0336938721132548,0.068801754429254));
#79887=CARTESIAN_POINT('',(0.0100175421957065,-0.0333679869945434,0.0687193648573588));
#79888=CARTESIAN_POINT('Ctrl Pts',(0.0102390586088633,-0.0336938721132647,
0.0688017544292584));
#79889=CARTESIAN_POINT('Ctrl Pts',(0.0102181818974938,-0.0336629187933931,
0.0687934975131143));
#79890=CARTESIAN_POINT('Ctrl Pts',(0.0101972635154301,-0.0336319952301038,
0.0687853654792674));
#79891=CARTESIAN_POINT('Ctrl Pts',(0.0101763057017087,-0.0336011045488948,
0.0687773589132866));
#79892=CARTESIAN_POINT('Ctrl Pts',(0.0101237153757214,-0.0335235892595452,
0.068757267699548));
#79893=CARTESIAN_POINT('Ctrl Pts',(0.0100707832553676,-0.0334458668660367,
0.0687379309708968));
#79894=CARTESIAN_POINT('Ctrl Pts',(0.0100175421958193,-0.0333679869945383,
0.0687193648570566));
#79895=CARTESIAN_POINT('Ctrl Pts',(0.0100175004318051,-0.0333679692459107,
0.0687193495652948));
#79896=CARTESIAN_POINT('Ctrl Pts',(0.0100173567982299,-0.033339189537294,
0.0687197794573971));
#79897=CARTESIAN_POINT('Ctrl Pts',(0.0100172522176963,-0.0333104081058071,
0.0687201027115236));
#79898=CARTESIAN_POINT('Ctrl Pts',(0.0100171190569288,-0.0332532697893318,
0.0687205322986892));
#79899=CARTESIAN_POINT('Ctrl Pts',(0.0100170893695625,-0.0332249169603541,
0.068720641797861));
#79900=CARTESIAN_POINT('Ctrl Pts',(0.0100170946743579,-0.0331960985432907,
0.0687206475348756));
#79901=CARTESIAN_POINT('Ctrl Pts',(0.0100170947702574,-0.0331956312491536,
0.0687206475998321));
#79902=CARTESIAN_POINT('Ctrl Pts',(0.0100170948752981,-0.0331951640388592,
0.0687206476364617));
#79903=CARTESIAN_POINT('',(0.0101351242745059,-0.0331951640388587,0.0687618066078137));
#79904=CARTESIAN_POINT('',(0.0100761095749122,-0.0331951640388687,0.0687412271221477));
#79905=CARTESIAN_POINT('',(0.0103547977016224,-0.0335216366567721,0.068848991152983));
#79906=CARTESIAN_POINT('Origin',(0.00502759431603476,-0.0326434571528016,
0.0846284578461628));
#79907=CARTESIAN_POINT('',(0.0103542707108206,-0.0336938721132327,0.0688502433100797));
#79908=CARTESIAN_POINT('Origin',(0.0145904810943599,-0.0336938867896154,
0.0587847899417411));
#79909=CARTESIAN_POINT('',(0.0102966646598458,-0.0336938721132538,0.0688259988696769));
#79910=CARTESIAN_POINT('Ctrl Pts',(0.0106662231239361,-0.0335235895815172,
0.0687152972378179));
#79911=CARTESIAN_POINT('Ctrl Pts',(0.0105914037404695,-0.0334144449262749,
0.0686802955327995));
#79912=CARTESIAN_POINT('Ctrl Pts',(0.010515775289712,-0.0333049234473147,
0.0686467993272172));
#79913=CARTESIAN_POINT('Ctrl Pts',(0.0104394305973828,-0.0331951640388587,
0.0686148602124428));
#79914=CARTESIAN_POINT('Ctrl Pts',(0.0105622294213664,-0.0335235895815172,
0.0687603137049349));
#79915=CARTESIAN_POINT('Ctrl Pts',(0.010488029778199,-0.0334144449262748,
0.0687267436779772));
#79916=CARTESIAN_POINT('Ctrl Pts',(0.0104130513571384,-0.0333049234473147,
0.068694667991912));
#79917=CARTESIAN_POINT('Ctrl Pts',(0.0103373863172536,-0.0331951640388587,
0.0686641363464102));
#79918=CARTESIAN_POINT('Ctrl Pts',(0.0104582357187967,-0.0335235895815172,
0.068805330172052));
#79919=CARTESIAN_POINT('Ctrl Pts',(0.0103846558159284,-0.0334144449262748,
0.0687731918231549));
#79920=CARTESIAN_POINT('Ctrl Pts',(0.0103103274245648,-0.0333049234473147,
0.0687425366566068));
#79921=CARTESIAN_POINT('Ctrl Pts',(0.0102353420371244,-0.0331951640388587,
0.0687134124803776));
#79922=CARTESIAN_POINT('Ctrl Pts',(0.010354242016227,-0.0335235895815172,
0.0688503466391691));
#79923=CARTESIAN_POINT('Ctrl Pts',(0.0102812818536578,-0.0334144449262748,
0.0688196399683326));
#79924=CARTESIAN_POINT('Ctrl Pts',(0.0102076034919911,-0.0333049234473147,
0.0687904053213016));
#79925=CARTESIAN_POINT('Ctrl Pts',(0.0101332977569952,-0.0331951640388587,
0.0687626886143449));
#79926=CARTESIAN_POINT('',(0.0102872774359542,-0.0331951640388687,0.0686883334101383));
#79927=CARTESIAN_POINT('Ctrl Pts',(0.0104512484705087,-0.0332121607146001,
0.0686198191108072));
#79928=CARTESIAN_POINT('Ctrl Pts',(0.0104346029379576,-0.0332625444109475,
0.068659369761615));
#79929=CARTESIAN_POINT('Ctrl Pts',(0.010418244234053,-0.0333135300746226,
0.0686982388926455));
#79930=CARTESIAN_POINT('Ctrl Pts',(0.0103860874981719,-0.0334167203140633,
0.0687746449690538));
#79931=CARTESIAN_POINT('Ctrl Pts',(0.0103703019207934,-0.033468884758732,
0.068812152321659));
#79932=CARTESIAN_POINT('Ctrl Pts',(0.010354797701189,-0.0335216366562388,
0.0688489911535642));
#79933=CARTESIAN_POINT('Ctrl Pts',(0.010239435998588,-0.033693872113239,
0.0688026803298203));
#79934=CARTESIAN_POINT('Ctrl Pts',(0.0102081363621296,-0.0336474569764958,
0.0687902967060484));
#79935=CARTESIAN_POINT('Ctrl Pts',(0.0101766939043906,-0.033601104548885,
0.0687782803325739));
#79936=CARTESIAN_POINT('Ctrl Pts',(0.0100970888304696,-0.0334837508592656,
0.0687478576376741));
#79937=CARTESIAN_POINT('Ctrl Pts',(0.0100166172257038,-0.0333660264659097,
0.0687198071655686));
#79938=CARTESIAN_POINT('Ctrl Pts',(0.01023905860887,-0.033693872113239,
0.0688017544292617));
#79939=CARTESIAN_POINT('Ctrl Pts',(0.0102077535528084,-0.0336474569764958,
0.0687893730144771));
#79940=CARTESIAN_POINT('Ctrl Pts',(0.0101763057016965,-0.033601104548885,
0.0687773589132818));
#79941=CARTESIAN_POINT('Ctrl Pts',(0.0100966869729955,-0.0334837508592656,
0.0687469419712704));
#79942=CARTESIAN_POINT('Ctrl Pts',(0.0100162018899158,-0.0333660264659097,
0.0687188976541466));
#79943=CARTESIAN_POINT('Ctrl Pts',(0.0101107444374813,-0.033693872113239,
0.0684869441487776));
#79944=CARTESIAN_POINT('Ctrl Pts',(0.0100775966923829,-0.0336474569764958,
0.0684753137994173));
#79945=CARTESIAN_POINT('Ctrl Pts',(0.0100443150706655,-0.033601104548885,
0.0684640722831846));
#79946=CARTESIAN_POINT('Ctrl Pts',(0.00996005365640166,-0.0334837508592656,
0.06843561134867));
#79947=CARTESIAN_POINT('Ctrl Pts',(0.00987498588704208,-0.0333660264659097,
0.0684096597525077));
#79948=CARTESIAN_POINT('',(0.0100994128180023,-0.0336769361243753,0.068484588838047));
#79949=CARTESIAN_POINT('',(0.0101115097307497,-0.0336938721132327,0.0684888217448924));
#79950=CARTESIAN_POINT('Ctrl Pts',(0.010099412818002,-0.033676936124375,
0.0684845888380469));
#79951=CARTESIAN_POINT('Ctrl Pts',(0.0101014298746358,-0.0336797586670073,
0.0684852922219222));
#79952=CARTESIAN_POINT('Ctrl Pts',(0.0101034464793446,-0.0336825812712942,
0.0684859966563938));
#79953=CARTESIAN_POINT('Ctrl Pts',(0.0101074787891163,-0.0336882266087494,
0.0684874076274563));
#79954=CARTESIAN_POINT('Ctrl Pts',(0.0101094944941804,-0.033691049341922,
0.0684881141640662));
#79955=CARTESIAN_POINT('Ctrl Pts',(0.0101115097307509,-0.0336938721132301,
0.0684888217448993));
#79956=CARTESIAN_POINT('Ctrl Pts',(0.0100994128180023,-0.0336769361243754,
0.0684845888380471));
#79957=CARTESIAN_POINT('Ctrl Pts',(0.0100856121074421,-0.0336279018378428,
0.0685241644037756));
#79958=CARTESIAN_POINT('Ctrl Pts',(0.0100716128563743,-0.0335767825754274,
0.0685643093135892));
#79959=CARTESIAN_POINT('Ctrl Pts',(0.0100441823742831,-0.0334733171799184,
0.0686429702522584));
#79960=CARTESIAN_POINT('Ctrl Pts',(0.0100307327075941,-0.0334209631321928,
0.0686815391480939));
#79961=CARTESIAN_POINT('Ctrl Pts',(0.0100175422025775,-0.0333679869844681,
0.0687193648597483));
#79962=CARTESIAN_POINT('',(0.0101752841698103,-0.0336938721132538,0.0686452880870832));
#79963=CARTESIAN_POINT('Origin',(0.00812378219310841,-0.0315241814719618,
0.07415));
#79964=CARTESIAN_POINT('',(0.0100994128175795,-0.0337108120655561,0.0684845888392771));
#79965=CARTESIAN_POINT('',(0.0100873068912882,-0.0336938721132327,0.0684803817800796));
#79966=CARTESIAN_POINT('Origin',(0.00365684478420917,-0.0345562519868347,
0.0835654253639754));
#79967=CARTESIAN_POINT('Ctrl Pts',(0.0100873068912913,-0.0336938721132343,
0.0684803817800769));
#79968=CARTESIAN_POINT('Ctrl Pts',(0.0100893251502616,-0.0336910493167714,
0.0684810807515388));
#79969=CARTESIAN_POINT('Ctrl Pts',(0.0100913430998275,-0.0336882265961736,
0.068481780822788));
#79970=CARTESIAN_POINT('Ctrl Pts',(0.0100953784054197,-0.0336825812712429,
0.0684831831741107));
#79971=CARTESIAN_POINT('Ctrl Pts',(0.0100973957613872,-0.0336797586669816,
0.0684838854541783));
#79972=CARTESIAN_POINT('Ctrl Pts',(0.0100994128180026,-0.033676936124375,
0.0684845888380471));
#79973=CARTESIAN_POINT('Origin',(0.00576741051423809,-0.0345562518742467,
0.0843014157688912));
#79974=CARTESIAN_POINT('Ctrl Pts',(0.0101689774313362,-0.034243627687391,
0.0687745650001576));
#79975=CARTESIAN_POINT('Ctrl Pts',(0.0099662395581409,-0.033943005420181,
0.0686974291901479));
#79976=CARTESIAN_POINT('Ctrl Pts',(0.00975826745672531,-0.0336441434784052,
0.0686357835621895));
#79977=CARTESIAN_POINT('Ctrl Pts',(0.0099334411014061,-0.034243627687391,
0.0686907638230592));
#79978=CARTESIAN_POINT('Ctrl Pts',(0.00972754261471318,-0.033943005420181,
0.0686225114121775));
#79979=CARTESIAN_POINT('Ctrl Pts',(0.00951708801279247,-0.0336441434784052,
0.0685699620169003));
#79980=CARTESIAN_POINT('Ctrl Pts',(0.0099310857381068,-0.034243627687391,
0.0686899258112882));
#79981=CARTESIAN_POINT('Ctrl Pts',(0.0097251556452789,-0.033943005420181,
0.0686217622343978));
#79982=CARTESIAN_POINT('Ctrl Pts',(0.00951467621835315,-0.0336441434784052,
0.0685693038014475));
#79983=CARTESIAN_POINT('',(0.00989906547609107,-0.034193496108874,0.0686794886651097));
#79984=CARTESIAN_POINT('',(0.00967281289662403,-0.0338664212864422,0.0686111708017387));
#79985=CARTESIAN_POINT('Origin',(0.00425118061923489,-0.0345610720404941,
0.0844324103120104));
#79986=CARTESIAN_POINT('Origin',(0.0126263498928281,-0.0336938005073008,
0.0580501413238942));
#79987=CARTESIAN_POINT('',(0.0097928278879358,-0.0336938721132327,0.0686461457624153));
#79988=CARTESIAN_POINT('',(0.0097326374437739,-0.0336938721132427,0.0686293124493113));
#79989=CARTESIAN_POINT('',(0.0100175422025825,-0.0340203938281605,0.06871936485975));
#79990=CARTESIAN_POINT('Origin',(0.00382868036302869,-0.0345589643244605,
0.0842021272954969));
#79991=CARTESIAN_POINT('',(0.0100170948752984,-0.034193496108874,0.0687206476364617));
#79992=CARTESIAN_POINT('Origin',(0.0136454885882588,-0.0341934220717668,
0.058315697980597));
#79993=CARTESIAN_POINT('',(0.00995808017570475,-0.0341934961088841,0.0687000681507957));
#79994=CARTESIAN_POINT('Ctrl Pts',(0.0103199609339328,-0.0340223579322396,
0.0685663811968963));
#79995=CARTESIAN_POINT('Ctrl Pts',(0.0102429482679489,-0.0339125849573575,
0.0685360901641857));
#79996=CARTESIAN_POINT('Ctrl Pts',(0.0101653627638831,-0.0338030433565231,
0.0685074143998663));
#79997=CARTESIAN_POINT('Ctrl Pts',(0.0100873068912889,-0.0336938721132327,
0.0684803817800792));
#79998=CARTESIAN_POINT('Ctrl Pts',(0.0102189989941991,-0.0340223579322396,
0.0686178386215836));
#79999=CARTESIAN_POINT('Ctrl Pts',(0.0101426960603082,-0.0339125849573575,
0.0685889401173418));
#80000=CARTESIAN_POINT('Ctrl Pts',(0.0100658486117185,-0.0338030433565231,
0.0685616412131723));
#80001=CARTESIAN_POINT('Ctrl Pts',(0.00998855801804967,-0.0336938721132327,
0.0685359681081126));
#80002=CARTESIAN_POINT('Ctrl Pts',(0.0101180370544654,-0.0340223579322396,
0.068669296046271));
#80003=CARTESIAN_POINT('Ctrl Pts',(0.0100424438526675,-0.0339125849573575,
0.0686417900704979));
#80004=CARTESIAN_POINT('Ctrl Pts',(0.00996633445955384,-0.0338030433565231,
0.0686158680264783));
#80005=CARTESIAN_POINT('Ctrl Pts',(0.00988980914481046,-0.0336938721132327,
0.068591554436146));
#80006=CARTESIAN_POINT('Ctrl Pts',(0.0100170751147317,-0.0340223579322396,
0.0687207534709584));
#80007=CARTESIAN_POINT('Ctrl Pts',(0.00994219164502685,-0.0339125849573575,
0.068694640023654));
#80008=CARTESIAN_POINT('Ctrl Pts',(0.0098668203073892,-0.0338030433565231,
0.0686700948397844));
#80009=CARTESIAN_POINT('Ctrl Pts',(0.00979106027157125,-0.0336938721132327,
0.0686471407641794));
#80010=CARTESIAN_POINT('',(0.00994006738962203,-0.0336938721132427,0.0685632637712574));
#80011=CARTESIAN_POINT('Ctrl Pts',(0.0100994128163883,-0.0337108120662709,
0.0684845888426755));
#80012=CARTESIAN_POINT('Ctrl Pts',(0.0100852543751759,-0.0337611408994033,
0.0685251902536224));
#80013=CARTESIAN_POINT('Ctrl Pts',(0.0100713542941038,-0.0338121088780741,
0.0685650507788977));
#80014=CARTESIAN_POINT('Ctrl Pts',(0.0100440581894573,-0.0339153382773246,
0.0686433263704953));
#80015=CARTESIAN_POINT('Ctrl Pts',(0.01003067371383,-0.0339675558473111,
0.0686817083213825));
#80016=CARTESIAN_POINT('Ctrl Pts',(0.0100175422025644,-0.0340203938281304,
0.068719364859786));
#80017=CARTESIAN_POINT('Ctrl Pts',(0.00989994740545553,-0.0341934961088741,
0.0686813150228184));
#80018=CARTESIAN_POINT('Ctrl Pts',(0.00978688665184713,-0.0340287516182428,
0.0686445942063371));
#80019=CARTESIAN_POINT('Ctrl Pts',(0.00967240480728664,-0.0338644633275951,
0.0686125776538122));
#80020=CARTESIAN_POINT('Ctrl Pts',(0.00989906547609109,-0.0341934961088741,
0.0686794886651098));
#80021=CARTESIAN_POINT('Ctrl Pts',(0.00978596696397589,-0.0340287516182428,
0.0686427860818234));
#80022=CARTESIAN_POINT('Ctrl Pts',(0.0096714481467643,-0.0338644633275951,
0.068610789307501));
#80023=CARTESIAN_POINT('Ctrl Pts',(0.00975211908072102,-0.0341934961088741,
0.0683751823422345));
#80024=CARTESIAN_POINT('Ctrl Pts',(0.0096327292751165,-0.0340287516182428,
0.0683415177599062));
#80025=CARTESIAN_POINT('Ctrl Pts',(0.00951205010308995,-0.0338644633275951,
0.0683128164145612));
#80026=CARTESIAN_POINT('',(0.00973978025265297,-0.0341764758832392,0.0683717173604828));
#80027=CARTESIAN_POINT('',(0.00975211908072106,-0.034193496108874,0.0683751823422345));
#80028=CARTESIAN_POINT('Origin',(0.00478705626700944,-0.0345621026283397,
0.0841796852961523));
#80029=CARTESIAN_POINT('Ctrl Pts',(0.00973978025395748,-0.0341764758837484,
0.0683717173617427));
#80030=CARTESIAN_POINT('Ctrl Pts',(0.00972821931534931,-0.0341260050040601,
0.0684130555631635));
#80031=CARTESIAN_POINT('Ctrl Pts',(0.0097168593699231,-0.0340749269148501,
0.068453675219413));
#80032=CARTESIAN_POINT('Ctrl Pts',(0.00969453248471447,-0.0339715436306823,
0.0685335088728231));
#80033=CARTESIAN_POINT('Ctrl Pts',(0.00968357400950415,-0.0339192778238538,
0.0685726925812178));
#80034=CARTESIAN_POINT('Ctrl Pts',(0.00967281289844593,-0.0338664212856951,
0.0686111708012219));
#80035=CARTESIAN_POINT('',(0.00982559227841607,-0.0341934961088841,0.0685273355036821));
#80036=CARTESIAN_POINT('Origin',(0.00812378219310841,-0.0315241814719618,
0.07415));
#80037=CARTESIAN_POINT('',(0.00973978025164394,-0.0342105180190556,0.0683717173609663));
#80038=CARTESIAN_POINT('',(0.00972743405025934,-0.0341934961088739,0.0683682787406281));
#80039=CARTESIAN_POINT('Origin',(0.00482900654019169,-0.0345621712168763,
0.0841968505876941));
#80040=CARTESIAN_POINT('Origin',(0.00577340770126758,-0.0345621034657148,
0.084455537330222));
#80041=CARTESIAN_POINT('Origin',(0.00572863976026522,-0.0345621719545859,
0.0844484466111688));
#80042=CARTESIAN_POINT('Ctrl Pts',(0.00979427246813991,-0.0346945769586966,
0.0686465497645994));
#80043=CARTESIAN_POINT('Ctrl Pts',(0.00967900049949819,-0.0345275153362944,
0.068611560676961));
#80044=CARTESIAN_POINT('Ctrl Pts',(0.00956259834102009,-0.0343603235965185,
0.0685801877366656));
#80045=CARTESIAN_POINT('Ctrl Pts',(0.00944541163767919,-0.034193496108874,
0.068552518614256));
#80046=CARTESIAN_POINT('Ctrl Pts',(0.00971353701564637,-0.0346945769586966,
0.0686239706796645));
#80047=CARTESIAN_POINT('Ctrl Pts',(0.00959779211903051,-0.0345275153362944,
0.0685906726284033));
#80048=CARTESIAN_POINT('Ctrl Pts',(0.00948097009179245,-0.0343603235965185,
0.0685610060350233));
#80049=CARTESIAN_POINT('Ctrl Pts',(0.00936341774568531,-0.034193496108874,
0.0685350535049942));
#80050=CARTESIAN_POINT('Ctrl Pts',(0.00963280156315282,-0.0346945769586966,
0.0686013915947291));
#80051=CARTESIAN_POINT('Ctrl Pts',(0.00951658373856283,-0.0345275153362944,
0.0685697845798461));
#80052=CARTESIAN_POINT('Ctrl Pts',(0.00939934184256478,-0.0343603235965185,
0.0685418243333825));
#80053=CARTESIAN_POINT('Ctrl Pts',(0.00928142385369134,-0.034193496108874,
0.0685175883957352));
#80054=CARTESIAN_POINT('Ctrl Pts',(0.00955206611065928,-0.0346945769586966,
0.0685788125097948));
#80055=CARTESIAN_POINT('Ctrl Pts',(0.00943537535809516,-0.0345275153362944,
0.068548896531288));
#80056=CARTESIAN_POINT('Ctrl Pts',(0.00931771359333718,-0.0343603235965185,
0.0685226426317385));
#80057=CARTESIAN_POINT('Ctrl Pts',(0.00919942996169755,-0.034193496108874,
0.0685001232864705));
#80058=CARTESIAN_POINT('',(0.00955206611124268,-0.0346945769586966,0.068578812509958));
#80059=CARTESIAN_POINT('',(0.00932197027664225,-0.0343667727831454,0.068524835974231));
#80060=CARTESIAN_POINT('Origin',(0.00555408289492608,-0.034562645706327,
0.0849101742849005));
#80061=CARTESIAN_POINT('Origin',(0.011624481658412,-0.0341934771028874,
0.0577151599463111));
#80062=CARTESIAN_POINT('',(0.00944394454052274,-0.034193496108874,0.0685522061152209));
#80063=CARTESIAN_POINT('',(0.00938281589597739,-0.034193496108884,0.0685391854080754));
#80064=CARTESIAN_POINT('',(0.00967281289796297,-0.0345211942962692,0.0686111708028464));
#80065=CARTESIAN_POINT('Origin',(0.00509193409485608,-0.0345625596120452,
0.0847774743351235));
#80066=CARTESIAN_POINT('',(0.00967244699959198,-0.0346945769586885,0.0686124791361874));
#80067=CARTESIAN_POINT('Origin',(0.0126522315959922,-0.0346945685853837,
0.0579577431490891));
#80068=CARTESIAN_POINT('',(0.00961225655542733,-0.0346945769587026,0.0685956458230828));
#80069=CARTESIAN_POINT('Ctrl Pts',(0.00996502803560501,-0.0345231616327842,
0.0684394996937654));
#80070=CARTESIAN_POINT('Ctrl Pts',(0.00988631682862492,-0.0344132092796988,
0.0684141207120934));
#80071=CARTESIAN_POINT('Ctrl Pts',(0.00980708473856406,-0.0343032738558979,
0.06839037111909));
#80072=CARTESIAN_POINT('Ctrl Pts',(0.00972743405025934,-0.0341934961088739,
0.0683682787406281));
#80073=CARTESIAN_POINT('Ctrl Pts',(0.00986749653480353,-0.0345231616327842,
0.0684971949491148));
#80074=CARTESIAN_POINT('Ctrl Pts',(0.00978958057569002,-0.0344132092796988,
0.068473160301868));
#80075=CARTESIAN_POINT('Ctrl Pts',(0.00971117149896178,-0.0343032738558979,
0.0684507385248535));
#80076=CARTESIAN_POINT('Ctrl Pts',(0.0096323704915066,-0.0341934961088739,
0.0684299557698666));
#80077=CARTESIAN_POINT('Ctrl Pts',(0.00976996503400206,-0.0345231616327842,
0.0685548902044643));
#80078=CARTESIAN_POINT('Ctrl Pts',(0.00969284432275511,-0.0344132092796988,
0.0685321998916426));
#80079=CARTESIAN_POINT('Ctrl Pts',(0.0096152582593595,-0.0343032738558979,
0.0685111059306169));
#80080=CARTESIAN_POINT('Ctrl Pts',(0.00953730693275385,-0.0341934961088739,
0.0684916327991051));
#80081=CARTESIAN_POINT('Ctrl Pts',(0.00967243353320058,-0.0345231616327842,
0.0686125854598137));
#80082=CARTESIAN_POINT('Ctrl Pts',(0.00959610806982021,-0.0344132092796988,
0.0685912394814172));
#80083=CARTESIAN_POINT('Ctrl Pts',(0.00951934501975722,-0.0343032738558979,
0.0685714733363804));
#80084=CARTESIAN_POINT('Ctrl Pts',(0.00944224337400111,-0.0341934961088739,
0.0685533098283437));
#80085=CARTESIAN_POINT('',(0.00958568929540103,-0.0341934961088839,0.0684602424279345));
#80086=CARTESIAN_POINT('Ctrl Pts',(0.00973978025070836,-0.0342105180195413,
0.0683717173642896));
#80087=CARTESIAN_POINT('Ctrl Pts',(0.00972820630212458,-0.0342610556240955,
0.068413102034162));
#80088=CARTESIAN_POINT('Ctrl Pts',(0.0097168400420636,-0.0343122189869412,
0.0684537440775323));
#80089=CARTESIAN_POINT('Ctrl Pts',(0.00969451293551567,-0.0344158119695182,
0.0685335785373973));
#80090=CARTESIAN_POINT('Ctrl Pts',(0.00968356122100284,-0.034468199045008,
0.0685727383009274));
#80091=CARTESIAN_POINT('Ctrl Pts',(0.00967281289794548,-0.0345211942962497,
0.0686111708028684));
#80092=CARTESIAN_POINT('Ctrl Pts',(0.00955306073468827,-0.0346945769586932,
0.0685805794542282));
#80093=CARTESIAN_POINT('Ctrl Pts',(0.00943791690570001,-0.034529677707698,
0.068551030131706));
#80094=CARTESIAN_POINT('Ctrl Pts',(0.00932165016502144,-0.0343648066251421,
0.0685262650589709));
#80095=CARTESIAN_POINT('Ctrl Pts',(0.00955206611125146,-0.0346945769586932,
0.0685788125099604));
#80096=CARTESIAN_POINT('Ctrl Pts',(0.00943688575194071,-0.034529677707698,
0.0685492837505741));
#80097=CARTESIAN_POINT('Ctrl Pts',(0.00932058336204766,-0.0343648066251421,
0.0685245407332356));
#80098=CARTESIAN_POINT('Ctrl Pts',(0.0093863021289167,-0.0346945769586932,
0.0682843335066093));
#80099=CARTESIAN_POINT('Ctrl Pts',(0.00926503362457833,-0.034529677707698,
0.0682582318002669));
#80100=CARTESIAN_POINT('Ctrl Pts',(0.009142789935153,-0.0343648066251421,
0.0682371645362269));
#80101=CARTESIAN_POINT('',(0.00937377008064706,-0.0346775396664974,0.0682816501233835));
#80102=CARTESIAN_POINT('',(0.00938630212891341,-0.0346945769586885,0.0682843335066086));
#80103=CARTESIAN_POINT('Origin',(0.00606465087396489,-0.0345626617849754,
0.0845501050758799));
#80104=CARTESIAN_POINT('Ctrl Pts',(0.00937377008196102,-0.0346775396670097,
0.0682816501246353));
#80105=CARTESIAN_POINT('Ctrl Pts',(0.00936482055953663,-0.0346269749928194,
0.0683236657366887));
#80106=CARTESIAN_POINT('Ctrl Pts',(0.00935603012522731,-0.03457579028908,
0.0683649346450465));
#80107=CARTESIAN_POINT('Ctrl Pts',(0.00933876002482597,-0.0344721681087937,
0.0684460130058423));
#80108=CARTESIAN_POINT('Ctrl Pts',(0.00933028712391344,-0.0344197714289673,
0.06848579067057));
#80109=CARTESIAN_POINT('Ctrl Pts',(0.00932197027689282,-0.0343667727830624,
0.0685248359741716));
#80110=CARTESIAN_POINT('',(0.00946918412008804,-0.0346945769587026,0.0684315730082934));
#80111=CARTESIAN_POINT('Origin',(0.00812378219310841,-0.0315241814719618,
0.07415));
#80112=CARTESIAN_POINT('',(0.00937377007967882,-0.034711613648963,0.0682816501243834));
#80113=CARTESIAN_POINT('',(0.00936123232798914,-0.0346945769586885,0.0682789935135702));
#80114=CARTESIAN_POINT('Origin',(0.00610932057602584,-0.034562669183425,
0.084557708751051));
#80115=CARTESIAN_POINT('Origin',(0.00576591901831826,-0.0345626625264326,
0.0844864758811781));
#80116=CARTESIAN_POINT('Origin',(0.0057220288670672,-0.0345626698720476,
0.0844752120881819));
#80117=CARTESIAN_POINT('Ctrl Pts',(0.00948151976255504,-0.0352450361874068,
0.068561144006316));
#80118=CARTESIAN_POINT('Ctrl Pts',(0.00927073259989667,-0.0349452760959493,
0.0685099360936015));
#80119=CARTESIAN_POINT('Ctrl Pts',(0.00905668707186739,-0.034644428984174,
0.0684747510087387));
#80120=CARTESIAN_POINT('Ctrl Pts',(0.00947905351566946,-0.0352450361874068,
0.0685606024794936));
#80121=CARTESIAN_POINT('Ctrl Pts',(0.00926824592899184,-0.0349452760959493,
0.0685094875828067));
#80122=CARTESIAN_POINT('Ctrl Pts',(0.00905418704131359,-0.034644428984174,
0.0684743967881435));
#80123=CARTESIAN_POINT('Ctrl Pts',(0.00923487065571117,-0.0352450361874068,
0.0685069859624248));
#80124=CARTESIAN_POINT('Ctrl Pts',(0.00902204088890987,-0.0349452760959493,
0.0684650805734222));
#80125=CARTESIAN_POINT('Ctrl Pts',(0.00880665926370981,-0.034644428984174,
0.0684393254420825));
#80126=CARTESIAN_POINT('Ctrl Pts',(0.00923242882711158,-0.0352450361874068,
0.0685064497972541));
#80127=CARTESIAN_POINT('Ctrl Pts',(0.00901957883850905,-0.0349452760959493,
0.0684646365033283));
#80128=CARTESIAN_POINT('Ctrl Pts',(0.00880418398593377,-0.034644428984174,
0.0684389747286218));
#80129=CARTESIAN_POINT('',(0.00919946219391866,-0.0351951634053319,0.0685001270068821));
#80130=CARTESIAN_POINT('',(0.00896639895473392,-0.0348678972925388,0.0684607010982874));
#80131=CARTESIAN_POINT('Origin',(0.00692987301931678,-0.0345636767880432,
0.0850908913454142));
#80132=CARTESIAN_POINT('Origin',(0.0105852836484402,-0.0346946199340767,
0.0575300926224854));
#80133=CARTESIAN_POINT('',(0.00908985113317312,-0.0346945769330288,0.0684803584062982));
#80134=CARTESIAN_POINT('',(0.00902802552651304,-0.0346945769458128,0.0684712016902573));
#80135=CARTESIAN_POINT('',(0.00932197027684797,-0.0350221583435276,0.0685248359743039));
#80136=CARTESIAN_POINT('Origin',(0.0064499830532711,-0.0345628458717242,
0.0850617534996283));
#80137=CARTESIAN_POINT('',(0.00932171555320903,-0.035195136029876,0.0685260463497064));
#80138=CARTESIAN_POINT('Origin',(0.0116173115732708,-0.035195183836691,
0.0577488443566961));
#80139=CARTESIAN_POINT('',(0.00919942996232486,-0.0351951371328749,0.0685001232864853));
#80140=CARTESIAN_POINT('Ctrl Pts',(0.00960282854545952,-0.0350241211494342,
0.0683351550418249));
#80141=CARTESIAN_POINT('Ctrl Pts',(0.00952273144033991,-0.0349144232818961,
0.0683147817847539));
#80142=CARTESIAN_POINT('Ctrl Pts',(0.0094421652634605,-0.0348045283579412,
0.0682960519977036));
#80143=CARTESIAN_POINT('Ctrl Pts',(0.00936123231711517,-0.0346945769439157,
0.0682789935112782));
#80144=CARTESIAN_POINT('Ctrl Pts',(0.00950911220538419,-0.0350241211494342,
0.0683988605314295));
#80145=CARTESIAN_POINT('Ctrl Pts',(0.00942989261726361,-0.0349144232818961,
0.0683797781785178));
#80146=CARTESIAN_POINT('Ctrl Pts',(0.00935023116653086,-0.0348045283579412,
0.0683623219293919));
#80147=CARTESIAN_POINT('Ctrl Pts',(0.00927022905734283,-0.0346945769439157,
0.0683465179402924));
#80148=CARTESIAN_POINT('Ctrl Pts',(0.00941539586530886,-0.0350241211494342,
0.0684625660210341));
#80149=CARTESIAN_POINT('Ctrl Pts',(0.00933705379418732,-0.0349144232818961,
0.0684447745722818));
#80150=CARTESIAN_POINT('Ctrl Pts',(0.00925829706960123,-0.0348045283579412,
0.0684285918610801));
#80151=CARTESIAN_POINT('Ctrl Pts',(0.00917922579757049,-0.0346945769439157,
0.0684140423693066));
#80152=CARTESIAN_POINT('Ctrl Pts',(0.00932167952523353,-0.0350241211494342,
0.0685262715106388));
#80153=CARTESIAN_POINT('Ctrl Pts',(0.00924421497111102,-0.0349144232818961,
0.0685097709660457));
#80154=CARTESIAN_POINT('Ctrl Pts',(0.00916636297267159,-0.0348045283579412,
0.0684948617927684));
#80155=CARTESIAN_POINT('Ctrl Pts',(0.00908822253779814,-0.0346945769439157,
0.0684815667983207));
#80156=CARTESIAN_POINT('',(0.00922554173088876,-0.0346945769458128,0.0683796759599063));
#80157=CARTESIAN_POINT('Ctrl Pts',(0.00937377007898878,-0.0347116136492817,
0.0682816501275956));
#80158=CARTESIAN_POINT('Ctrl Pts',(0.00936482409802611,-0.0347621546531941,
0.0683236490516123));
#80159=CARTESIAN_POINT('Ctrl Pts',(0.00935603541158321,-0.0348133084096261,
0.0683649095210523));
#80160=CARTESIAN_POINT('Ctrl Pts',(0.00933876529295336,-0.0349168561544579,
0.0684459879855739));
#80161=CARTESIAN_POINT('Ctrl Pts',(0.00933029071096543,-0.0349692089015914,
0.0684857738208522));
#80162=CARTESIAN_POINT('Ctrl Pts',(0.0093219702768209,-0.0350221583434999,
0.0685248359743356));
#80163=CARTESIAN_POINT('Ctrl Pts',(0.00920022625217223,-0.0351951371254941,
0.0685013506178967));
#80164=CARTESIAN_POINT('Ctrl Pts',(0.0090834439702777,-0.0350307338980939,
0.068479095812359));
#80165=CARTESIAN_POINT('Ctrl Pts',(0.00896584166303073,-0.0348659306897793,
0.068461686761144));
#80166=CARTESIAN_POINT('Ctrl Pts',(0.00919942996230845,-0.0351951371254941,
0.0685001232866004));
#80167=CARTESIAN_POINT('Ctrl Pts',(0.00908262230610942,-0.0350307338980939,
0.068477884943856));
#80168=CARTESIAN_POINT('Ctrl Pts',(0.00896499532666516,-0.0348659306897793,
0.0684604933901143));
#80169=CARTESIAN_POINT('Ctrl Pts',(0.00906597095118402,-0.0351951371254941,
0.0682944212821137));
#80170=CARTESIAN_POINT('Ctrl Pts',(0.00894491053510396,-0.0350307338980939,
0.0682749421206894));
#80171=CARTESIAN_POINT('Ctrl Pts',(0.00882314846967821,-0.0348659306897793,
0.0682604831617183));
#80172=CARTESIAN_POINT('Origin',(0.00974555209516449,-0.0308609197410205,
0.0631999048410406));
#80173=CARTESIAN_POINT('',(0.00914124484255691,-0.0351951371254941,0.0684104418506048));
#80174=CARTESIAN_POINT('Origin',(0.00812218386499098,-0.0351840467441105,
0.0751271095618081));
#80175=CARTESIAN_POINT('Origin',(0.00908679811530163,-0.0352322614053928,
0.06222345922568));
#80176=CARTESIAN_POINT('',(0.00873162935605851,-0.0351951142564663,0.0684308797521022));
#80177=CARTESIAN_POINT('',(0.00860738789448549,-0.0351951372916787,0.0684203730029262));
#80178=CARTESIAN_POINT('Origin',(0.00781973432811109,-0.0352875126913164,
0.0743035585178548));
#80179=CARTESIAN_POINT('Origin',(0.0153410677464602,-0.0298325076523007,
0.0762008484880468));
#80180=CARTESIAN_POINT('Origin',(0.0119206263900213,-0.0338732385636012,
0.066677789022853));
#80181=CARTESIAN_POINT('Ctrl Pts',(0.0119774395667351,-0.0321934096636942,
0.0698806369805316));
#80182=CARTESIAN_POINT('Ctrl Pts',(0.0119010200018148,-0.0320508460844833,
0.0698116583487073));
#80183=CARTESIAN_POINT('Ctrl Pts',(0.0118228047377682,-0.0319086045664086,
0.0697447849699195));
#80184=CARTESIAN_POINT('Ctrl Pts',(0.0117429740399792,-0.0317669892869414,
0.0696801469696607));
#80185=CARTESIAN_POINT('Ctrl Pts',(0.0119139908020065,-0.0321934096636942,
0.0698258219562938));
#80186=CARTESIAN_POINT('Ctrl Pts',(0.011836590074256,-0.0320508460844833,
0.069757979027143));
#80187=CARTESIAN_POINT('Ctrl Pts',(0.0117574249012691,-0.0319086045664086,
0.0696922668566142));
#80188=CARTESIAN_POINT('Ctrl Pts',(0.0116766773879117,-0.0317669892869414,
0.0696288129015313));
#80189=CARTESIAN_POINT('Ctrl Pts',(0.0118505420372779,-0.0321934096636942,
0.0697710069320561));
#80190=CARTESIAN_POINT('Ctrl Pts',(0.0117721601466973,-0.0320508460844833,
0.0697042997055786));
#80191=CARTESIAN_POINT('Ctrl Pts',(0.0116920450647701,-0.0319086045664086,
0.0696397487433092));
#80192=CARTESIAN_POINT('Ctrl Pts',(0.0116103807358444,-0.0317669892869414,
0.0695774788334018));
#80193=CARTESIAN_POINT('Ctrl Pts',(0.0117870932725493,-0.0321934096636942,
0.0697161919078182));
#80194=CARTESIAN_POINT('Ctrl Pts',(0.0117077302191384,-0.0320508460844833,
0.0696506203840143));
#80195=CARTESIAN_POINT('Ctrl Pts',(0.011626665228271,-0.0319086045664086,
0.069587230630004));
#80196=CARTESIAN_POINT('Ctrl Pts',(0.0115440840837769,-0.0317669892869414,
0.0695261447652723));
#80197=CARTESIAN_POINT('',(0.011788228383487,-0.0321934096636942,0.0697171725594356));
#80198=CARTESIAN_POINT('',(0.0116030135384361,-0.0318665617511301,0.069570363089195));
#80199=CARTESIAN_POINT('Origin',(0.000674913735238927,-0.0326371944422868,
0.0821956397080663));
#80200=CARTESIAN_POINT('Origin',(0.018233881790812,-0.031693926150954,0.0608422947860181));
#80201=CARTESIAN_POINT('',(0.0118834754864822,-0.0320197221621852,0.0697977252492182));
#80202=CARTESIAN_POINT('Ctrl Pts',(0.0118833709835563,-0.0320197392094763,
0.0697975726254411));
#80203=CARTESIAN_POINT('Ctrl Pts',(0.0118612244031211,-0.0319792716576062,
0.069778442664521));
#80204=CARTESIAN_POINT('Ctrl Pts',(0.0118388311639004,-0.0319386439829743,
0.0697593944533535));
#80205=CARTESIAN_POINT('Ctrl Pts',(0.0118161622773984,-0.0318979099381674,
0.0697404144370541));
#80206=CARTESIAN_POINT('Ctrl Pts',(0.0117934938389622,-0.0318571766984966,
0.0697214347959076));
#80207=CARTESIAN_POINT('Ctrl Pts',(0.0117706661237289,-0.0318163871833605,
0.0697026184477855));
#80208=CARTESIAN_POINT('Ctrl Pts',(0.0117477598892644,-0.0317755399638303,
0.0696840273960825));
#80209=CARTESIAN_POINT('',(0.0118828177156378,-0.0321934096636183,0.0697988907230038));
#80210=CARTESIAN_POINT('Origin',(0.013336754182227,-0.0324029947590523,
0.0680846214846591));
#80211=CARTESIAN_POINT('',(0.0118355230495724,-0.0321934096636663,0.0697580316412297));
#80212=CARTESIAN_POINT('Ctrl Pts',(0.0117883760591032,-0.0321934096636618,
0.0697191953988487));
#80213=CARTESIAN_POINT('Ctrl Pts',(0.0117272718104862,-0.0320835708272592,
0.0696686577934193));
#80214=CARTESIAN_POINT('Ctrl Pts',(0.0116651571316989,-0.0319739230346488,
0.0696194140511041));
#80215=CARTESIAN_POINT('Ctrl Pts',(0.0116021163295406,-0.0318646057455573,
0.0695715210766456));
#80216=CARTESIAN_POINT('Ctrl Pts',(0.0117801252758827,-0.0321934096636618,
0.069606177305869));
#80217=CARTESIAN_POINT('Ctrl Pts',(0.0117174624196823,-0.0320835708272592,
0.0695557534851704));
#80218=CARTESIAN_POINT('Ctrl Pts',(0.0116537923921365,-0.0319739230346488,
0.0695066557168894));
#80219=CARTESIAN_POINT('Ctrl Pts',(0.0115892014756718,-0.0318646057455573,
0.0694589405662804));
#80220=CARTESIAN_POINT('Ctrl Pts',(0.0117718744926621,-0.0321934096636618,
0.0694931592128893));
#80221=CARTESIAN_POINT('Ctrl Pts',(0.0117076530288784,-0.0320835708272592,
0.0694428491769216));
#80222=CARTESIAN_POINT('Ctrl Pts',(0.0116424276525741,-0.0319739230346488,
0.0693938973826746));
#80223=CARTESIAN_POINT('Ctrl Pts',(0.0115762866218029,-0.0318646057455573,
0.0693463600559153));
#80224=CARTESIAN_POINT('Ctrl Pts',(0.0117636237094416,-0.0321934096636618,
0.0693801411199095));
#80225=CARTESIAN_POINT('Ctrl Pts',(0.0116978436380745,-0.0320835708272592,
0.0693299448686727));
#80226=CARTESIAN_POINT('Ctrl Pts',(0.0116310629130117,-0.0319739230346488,
0.0692811390484598));
#80227=CARTESIAN_POINT('Ctrl Pts',(0.0115633717679341,-0.0318646057455573,
0.0692337795455501));
#80228=CARTESIAN_POINT('',(0.0117534269007546,-0.0321763980308461,0.0693723772361148));
#80229=CARTESIAN_POINT('',(0.0117636237094156,-0.0321934096636185,0.0693801411198898));
#80230=CARTESIAN_POINT('Origin',(0.00126142167047686,-0.0326386230766307,
0.0821686235382898));
#80231=CARTESIAN_POINT('Ctrl Pts',(0.0117534268988288,-0.0321763980306276,
0.0693723772386375));
#80232=CARTESIAN_POINT('Ctrl Pts',(0.0117274635097776,-0.0321259596174846,
0.0694065522856601));
#80233=CARTESIAN_POINT('Ctrl Pts',(0.0117019499701367,-0.0320749164631432,
0.0694401352056522));
#80234=CARTESIAN_POINT('Ctrl Pts',(0.0116518020571826,-0.0319716057793938,
0.0695061438180066));
#80235=CARTESIAN_POINT('Ctrl Pts',(0.011627187223183,-0.0319193786690137,
0.0695385437911935));
#80236=CARTESIAN_POINT('Ctrl Pts',(0.0116030135373063,-0.0318665617525335,
0.069570363090666));
#80237=CARTESIAN_POINT('',(0.0117759260464613,-0.0321934096636664,0.0695486568396727));
#80238=CARTESIAN_POINT('Origin',(0.00812378219310841,-0.0315241814719618,
0.07415));
#80239=CARTESIAN_POINT('',(0.0117534269009785,-0.0322104233323795,0.0693723772358195));
#80240=CARTESIAN_POINT('',(0.0117432135337924,-0.0321934096636183,0.0693646351476514));
#80241=CARTESIAN_POINT('Origin',(0.00129334652218236,-0.0326387238943641,
0.0822008092625748));
#80242=CARTESIAN_POINT('Origin',(0.00223844929347,-0.0326386239132421,0.0829108912217361));
#80243=CARTESIAN_POINT('Origin',(0.00219888526709953,-0.032638724647286,
0.0828887605941058));
#80244=CARTESIAN_POINT('Ctrl Pts',(0.0117299533201467,-0.0327445246967097,
0.0696696367555168));
#80245=CARTESIAN_POINT('Ctrl Pts',(0.0115609736579378,-0.032443687833936,
0.0695336277880152));
#80246=CARTESIAN_POINT('Ctrl Pts',(0.0113822292977948,-0.0321434074405927,
0.0694107334464117));
#80247=CARTESIAN_POINT('Ctrl Pts',(0.0115318400651885,-0.0327445246967097,
0.0695171535164056));
#80248=CARTESIAN_POINT('Ctrl Pts',(0.0113571094036004,-0.032443687833936,
0.0693886165124647));
#80249=CARTESIAN_POINT('Ctrl Pts',(0.0111731932008937,-0.0321434074405927,
0.0692736060961405));
#80250=CARTESIAN_POINT('',(0.0115026578980598,-0.0326943950436612,0.0694958272517568));
#80251=CARTESIAN_POINT('',(0.0113085902897616,-0.0323666188837389,0.069360937211991));
#80252=CARTESIAN_POINT('Origin',(0.00168797373835554,-0.0326395579111556,
0.0831442715978149));
#80253=CARTESIAN_POINT('Origin',(0.0174245285709706,-0.0321933825603032,
0.0601642709255512));
#80254=CARTESIAN_POINT('',(0.011411923476348,-0.0321934096532689,0.0694312870506711));
#80255=CARTESIAN_POINT('',(0.0113598807399114,-0.0321934096584275,0.0693966777465776));
#80256=CARTESIAN_POINT('',(0.0116030135390043,-0.032521010975624,0.0695703630884385));
#80257=CARTESIAN_POINT('Origin',(0.00131433280402838,-0.0326393129156693,
0.0828416548734633));
#80258=CARTESIAN_POINT('',(0.0116021917056727,-0.0326943950436593,0.0695714448498568));
#80259=CARTESIAN_POINT('Origin',(0.0182943225340461,-0.0326943765538181,
0.0607627388341716));
#80260=CARTESIAN_POINT('',(0.0115524248018762,-0.0326943950436702,0.0695336360508168));
#80261=CARTESIAN_POINT('Ctrl Pts',(0.0119379047672226,-0.032522978320377,
0.0695183189887841));
#80262=CARTESIAN_POINT('Ctrl Pts',(0.0118740571457712,-0.032413025309245,
0.0694657413925093));
#80263=CARTESIAN_POINT('Ctrl Pts',(0.0118091315729429,-0.032303122220807,
0.069414492540725));
#80264=CARTESIAN_POINT('Ctrl Pts',(0.0117432135302167,-0.0321934096576658,
0.0693646351449463));
#80265=CARTESIAN_POINT('Ctrl Pts',(0.011825983204065,-0.032522978320377,
0.0695360589419031));
#80266=CARTESIAN_POINT('Ctrl Pts',(0.0117623801274794,-0.032413025309245,
0.0694850241819289));
#80267=CARTESIAN_POINT('Ctrl Pts',(0.0116977309779776,-0.032303122220807,
0.0694353128737191));
#80268=CARTESIAN_POINT('Ctrl Pts',(0.0116321208134636,-0.0321934096576658,
0.0693869857717991));
#80269=CARTESIAN_POINT('Ctrl Pts',(0.0117140616409074,-0.032522978320377,
0.0695537988950221));
#80270=CARTESIAN_POINT('Ctrl Pts',(0.0116507031091875,-0.032413025309245,
0.0695043069713484));
#80271=CARTESIAN_POINT('Ctrl Pts',(0.0115863303830124,-0.032303122220807,
0.0694561332067131));
#80272=CARTESIAN_POINT('Ctrl Pts',(0.0115210280967104,-0.0321934096576658,
0.0694093363986518));
#80273=CARTESIAN_POINT('Ctrl Pts',(0.0116021400777498,-0.032522978320377,
0.069571538848141));
#80274=CARTESIAN_POINT('Ctrl Pts',(0.0115390260908957,-0.032413025309245,
0.069523589760768));
#80275=CARTESIAN_POINT('Ctrl Pts',(0.0114749297880471,-0.032303122220807,
0.0694769535397072));
#80276=CARTESIAN_POINT('Ctrl Pts',(0.0114099353799573,-0.0321934096576658,
0.0694316870255046));
#80277=CARTESIAN_POINT('',(0.0115775685055598,-0.0321934096584275,0.0693979610993311));
#80278=CARTESIAN_POINT('Ctrl Pts',(0.0117534268988682,-0.0322104233328948,
0.0693723772385859));
#80279=CARTESIAN_POINT('Ctrl Pts',(0.0117274283290297,-0.0322609421830896,
0.0694065985933172));
#80280=CARTESIAN_POINT('Ctrl Pts',(0.0117018976029963,-0.0323120888239738,
0.0694402041353746));
#80281=CARTESIAN_POINT('Ctrl Pts',(0.0116517493103102,-0.0324156524631823,
0.069506213247562));
#80282=CARTESIAN_POINT('Ctrl Pts',(0.0116271523573068,-0.0324680267167318,
0.0695385896843918));
#80283=CARTESIAN_POINT('Ctrl Pts',(0.0116030135389745,-0.0325210109755913,
0.0695703630884703));
#80284=CARTESIAN_POINT('Origin',(0.0137699112845517,-0.0262834582512301,
0.0796294718833777));
#80285=CARTESIAN_POINT('Origin',(0.0190328750298983,-0.0342770935979982,
0.0687819385306052));
#80286=CARTESIAN_POINT('Ctrl Pts',(0.0115029322307526,-0.0326943950436604,
0.0694978363392128));
#80287=CARTESIAN_POINT('Ctrl Pts',(0.011438816696423,-0.0325844576448134,
0.069451265318492));
#80288=CARTESIAN_POINT('Ctrl Pts',(0.0113737334594747,-0.0324744968375322,
0.0694060170162363));
#80289=CARTESIAN_POINT('Ctrl Pts',(0.0113077667079925,-0.0323646534831894,
0.0693621482570324));
#80290=CARTESIAN_POINT('Ctrl Pts',(0.0114876012859894,-0.0326943950436604,
0.0693855594951439));
#80291=CARTESIAN_POINT('Ctrl Pts',(0.0114219383663192,-0.0325844576448134,
0.0693391997635751));
#80292=CARTESIAN_POINT('Ctrl Pts',(0.0113553120043256,-0.0324744968375322,
0.0692941947678907));
#80293=CARTESIAN_POINT('Ctrl Pts',(0.0112878083609354,-0.0323646534831894,
0.0692506009936677));
#80294=CARTESIAN_POINT('Ctrl Pts',(0.0114722703412261,-0.0326943950436604,
0.069273282651075));
#80295=CARTESIAN_POINT('Ctrl Pts',(0.0114050600362155,-0.0325844576448134,
0.0692271342086583));
#80296=CARTESIAN_POINT('Ctrl Pts',(0.0113368905491766,-0.0324744968375322,
0.0691823725195451));
#80297=CARTESIAN_POINT('Ctrl Pts',(0.0112678500138783,-0.0323646534831894,
0.069139053730303));
#80298=CARTESIAN_POINT('Ctrl Pts',(0.0114569393964629,-0.0326943950436604,
0.0691610058070061));
#80299=CARTESIAN_POINT('Ctrl Pts',(0.0113881817061117,-0.0325844576448134,
0.0691150686537415));
#80300=CARTESIAN_POINT('Ctrl Pts',(0.0113184690940275,-0.0324744968375322,
0.0690705502711994));
#80301=CARTESIAN_POINT('Ctrl Pts',(0.0112478916668211,-0.0323646534831894,
0.0690275064669383));
#80302=CARTESIAN_POINT('',(0.0114462752106906,-0.0326773559991343,0.0691538975062259));
#80303=CARTESIAN_POINT('',(0.0114569393964622,-0.0326943950436595,0.0691610058070057));
#80304=CARTESIAN_POINT('Origin',(0.00229303105636561,-0.032639567058775,
0.0830085512661952));
#80305=CARTESIAN_POINT('Ctrl Pts',(0.0114462752088285,-0.032677355998742,
0.0691538975090129));
#80306=CARTESIAN_POINT('Ctrl Pts',(0.0114224897960546,-0.0326267922585966,
0.0691896641334863));
#80307=CARTESIAN_POINT('Ctrl Pts',(0.0113991259625462,-0.0325756109579332,
0.0692247968203686));
#80308=CARTESIAN_POINT('Ctrl Pts',(0.0113532215702813,-0.032471998546237,
0.0692938242186076));
#80309=CARTESIAN_POINT('Ctrl Pts',(0.0113306994225228,-0.0324196091621781,
0.0693276912449599));
#80310=CARTESIAN_POINT('Ctrl Pts',(0.0113085902897346,-0.0323666188837756,
0.0693609372120315));
#80311=CARTESIAN_POINT('',(0.011479798647271,-0.0326943950436703,0.0693284165293912));
#80312=CARTESIAN_POINT('Origin',(0.00812378219310841,-0.0315241814719618,
0.07415));
#80313=CARTESIAN_POINT('',(0.0114462752106653,-0.0327114338379885,0.0691538975062631));
#80314=CARTESIAN_POINT('',(0.0114355958676051,-0.0326943950436593,0.0691468119977928));
#80315=CARTESIAN_POINT('Origin',(0.0023311841216073,-0.0326395674607007,
0.0830329919927061));
#80316=CARTESIAN_POINT('Origin',(0.00220936153178273,-0.0326395675911541,
0.0829529113907568));
#80317=CARTESIAN_POINT('Origin',(0.00217206945053782,-0.0326395680949288,
0.0829271762291045));
#80318=CARTESIAN_POINT('Ctrl Pts',(0.0114414809896982,-0.0332451089994433,
0.0694520217438662));
#80319=CARTESIAN_POINT('Ctrl Pts',(0.0112642938408344,-0.0329451141710254,
0.0693268926865341));
#80320=CARTESIAN_POINT('Ctrl Pts',(0.0110781848298304,-0.0326442513127493,
0.0692154655680471));
#80321=CARTESIAN_POINT('Ctrl Pts',(0.0112341832111637,-0.0332451089994433,
0.0693122804435478));
#80322=CARTESIAN_POINT('Ctrl Pts',(0.0110517256329297,-0.0329451141710254,
0.0691949697498483));
#80323=CARTESIAN_POINT('Ctrl Pts',(0.0108609500763995,-0.0326442513127493,
0.0690917357741336));
#80324=CARTESIAN_POINT('Ctrl Pts',(0.0112321102333783,-0.0332451089994433,
0.0693108830305446));
#80325=CARTESIAN_POINT('Ctrl Pts',(0.0110495999508507,-0.0329451141710254,
0.0691936505204814));
#80326=CARTESIAN_POINT('Ctrl Pts',(0.0108587777288652,-0.0326442513127493,
0.0690904984761945));
#80327=CARTESIAN_POINT('',(0.0112037525338448,-0.0331951640388616,0.0692928498375915));
#80328=CARTESIAN_POINT('',(0.0110015980489326,-0.0328677532355008,0.0691704115662241));
#80329=CARTESIAN_POINT('Origin',(0.0028842817016618,-0.0326402808280941,
0.0838468407867844));
#80330=CARTESIAN_POINT('Origin',(0.0165333618382668,-0.0326944278779039,
0.059597848045385));
#80331=CARTESIAN_POINT('',(0.0111091446375892,-0.0326943950436593,0.0692341342496886));
#80332=CARTESIAN_POINT('',(0.0110550314616524,-0.0326943950436693,0.0692028610313009));
#80333=CARTESIAN_POINT('',(0.011308590289764,-0.0330220786163545,0.0693609372119926));
#80334=CARTESIAN_POINT('Origin',(0.0024531833626679,-0.0326396682763794,
0.0836339866880716));
#80335=CARTESIAN_POINT('',(0.0113078380024956,-0.0331951640388587,0.0693620684421445));
#80336=CARTESIAN_POINT('Origin',(0.0174166038075984,-0.0331952026560207,
0.0601761906990763));
#80337=CARTESIAN_POINT('',(0.0112557952681802,-0.0331951640388701,0.069327459139878));
#80338=CARTESIAN_POINT('Ctrl Pts',(0.0116395520319408,-0.0330240426238172,
0.0692879672522316));
#80339=CARTESIAN_POINT('Ctrl Pts',(0.0115725727939913,-0.032914277406352,
0.0692395340974531));
#80340=CARTESIAN_POINT('Ctrl Pts',(0.0115045589158483,-0.0328043479726691,
0.0691924614449262));
#80341=CARTESIAN_POINT('Ctrl Pts',(0.0114355958676054,-0.0326943950436593,
0.0691468119977927));
#80342=CARTESIAN_POINT('Ctrl Pts',(0.011528965252176,-0.0330240426238172,
0.0693126998243922));
#80343=CARTESIAN_POINT('Ctrl Pts',(0.0114623267295038,-0.032914277406352,
0.0692657901102445));
#80344=CARTESIAN_POINT('Ctrl Pts',(0.0113946852302704,-0.0328043479726691,
0.0692202346143025));
#80345=CARTESIAN_POINT('Ctrl Pts',(0.0113261258010506,-0.0326943950436593,
0.0691760940829798));
#80346=CARTESIAN_POINT('Ctrl Pts',(0.0114183784724112,-0.0330240426238172,
0.0693374323965528));
#80347=CARTESIAN_POINT('Ctrl Pts',(0.0113520806650162,-0.032914277406352,
0.0692920461230358));
#80348=CARTESIAN_POINT('Ctrl Pts',(0.0112848115446925,-0.0328043479726691,
0.0692480077836788));
#80349=CARTESIAN_POINT('Ctrl Pts',(0.0112166557344957,-0.0326943950436593,
0.0692053761681669));
#80350=CARTESIAN_POINT('Ctrl Pts',(0.0113077916926463,-0.0330240426238172,
0.0693621649687135));
#80351=CARTESIAN_POINT('Ctrl Pts',(0.0112418346005287,-0.032914277406352,
0.0693183021358272));
#80352=CARTESIAN_POINT('Ctrl Pts',(0.0111749378591146,-0.0328043479726691,
0.0692757809530551));
#80353=CARTESIAN_POINT('Ctrl Pts',(0.0111071856679408,-0.0326943950436593,
0.069234658253354));
#80354=CARTESIAN_POINT('',(0.0112723702526072,-0.0326943950436693,0.0691904731237507));
#80355=CARTESIAN_POINT('Ctrl Pts',(0.0114462752088236,-0.0327114338383348,
0.0691538975090203));
#80356=CARTESIAN_POINT('Ctrl Pts',(0.0114224937523609,-0.0327619876830622,
0.0691896581843056));
#80357=CARTESIAN_POINT('Ctrl Pts',(0.011399131851307,-0.0328131562603595,
0.0692247879653157));
#80358=CARTESIAN_POINT('Ctrl Pts',(0.0113532275011655,-0.0329167375858782,
0.0692938153002127));
#80359=CARTESIAN_POINT('Ctrl Pts',(0.0113307033427855,-0.0329691088920628,
0.0693276853499788));
#80360=CARTESIAN_POINT('Ctrl Pts',(0.0113085902897355,-0.0330220786163187,
0.0693609372120307));
#80361=CARTESIAN_POINT('Ctrl Pts',(0.011204152540701,-0.0331951640388604,
0.0692948380524451));
#80362=CARTESIAN_POINT('Ctrl Pts',(0.0111037751802755,-0.0330306422010619,
0.0692311533704583));
#80363=CARTESIAN_POINT('Ctrl Pts',(0.0110008514367224,-0.0328657861914645,
0.0691716718084518));
#80364=CARTESIAN_POINT('Ctrl Pts',(0.0112037525338475,-0.0331951640388604,
0.0692928498375933));
#80365=CARTESIAN_POINT('Ctrl Pts',(0.0111033340683546,-0.0330306422010619,
0.0692291734254917));
#80366=CARTESIAN_POINT('Ctrl Pts',(0.0110003695966612,-0.0328657861914645,
0.0691697018252196));
#80367=CARTESIAN_POINT('Ctrl Pts',(0.0111371006348029,-0.0331951640388604,
0.0689615597749474));
#80368=CARTESIAN_POINT('Ctrl Pts',(0.0110298329596683,-0.0330306422010619,
0.0688992613481253));
#80369=CARTESIAN_POINT('Ctrl Pts',(0.0109200820845154,-0.0328657861914645,
0.0688414496406912));
#80370=CARTESIAN_POINT('',(0.0111260111596784,-0.0331781648281912,0.0689551351097334));
#80371=CARTESIAN_POINT('',(0.0111371006348019,-0.0331951640388588,0.0689615597749468));
#80372=CARTESIAN_POINT('Origin',(0.00348309549379353,-0.0326412092206366,
0.0836034223100902));
#80373=CARTESIAN_POINT('Ctrl Pts',(0.0111260111604432,-0.033178164828644,
0.0689551351114003));
#80374=CARTESIAN_POINT('Ctrl Pts',(0.0111045037013377,-0.0331276811546776,
0.0689923502665628));
#80375=CARTESIAN_POINT('Ctrl Pts',(0.0110833846296175,-0.0330765663497784,
0.0690288934481934));
#80376=CARTESIAN_POINT('Ctrl Pts',(0.0110419049755672,-0.0329730614463203,
0.0691006671802621));
#80377=CARTESIAN_POINT('Ctrl Pts',(0.0110215611454689,-0.0329207133373788,
0.0691358687330006));
#80378=CARTESIAN_POINT('Ctrl Pts',(0.0110015980653927,-0.0328677532289366,
0.0691704115656726));
#80379=CARTESIAN_POINT('',(0.0111704265843334,-0.0331951640388702,0.0691272048062792));
#80380=CARTESIAN_POINT('Origin',(0.00812378219310841,-0.0315241814719618,
0.07415));
#80381=CARTESIAN_POINT('',(0.0111260111583418,-0.0332121607144241,0.0689551351107534));
#80382=CARTESIAN_POINT('',(0.0111149079858691,-0.0331951640388587,0.0689487341452396));
#80383=CARTESIAN_POINT('Origin',(0.00352568836954617,-0.0326413657536576,
0.0836189795529282));
#80384=CARTESIAN_POINT('Origin',(0.00224971951351425,-0.0326412097728248,
0.0828906286422365));
#80385=CARTESIAN_POINT('Origin',(0.00221497665047648,-0.0326413663048814,
0.0828614882365986));
#80386=CARTESIAN_POINT('Ctrl Pts',(0.0111399635106757,-0.0337436976235975,
0.0692529830243751));
#80387=CARTESIAN_POINT('Ctrl Pts',(0.0110959189978337,-0.0336723290703325,
0.0692258550324901));
#80388=CARTESIAN_POINT('Ctrl Pts',(0.0110513936632877,-0.033601104548885,
0.0691995236512357));
#80389=CARTESIAN_POINT('Ctrl Pts',(0.0109092330900541,-0.0333736987606857,
0.069115452766843));
#80390=CARTESIAN_POINT('Ctrl Pts',(0.0107624823141038,-0.0331450831799192,
0.0690396784179996));
#80391=CARTESIAN_POINT('Ctrl Pts',(0.0109243008161114,-0.0337436976235975,
0.0691265330256671));
#80392=CARTESIAN_POINT('Ctrl Pts',(0.010879118992817,-0.0336723290703325,
0.0691013447367416));
#80393=CARTESIAN_POINT('Ctrl Pts',(0.0108334914209511,-0.033601104548885,
0.0690769732012787));
#80394=CARTESIAN_POINT('Ctrl Pts',(0.0106878116222958,-0.0333736987606857,
0.0689991597162749));
#80395=CARTESIAN_POINT('Ctrl Pts',(0.0105379065059857,-0.0331450831799192,
0.0689298344085676));
#80396=CARTESIAN_POINT('Ctrl Pts',(0.0109221441891658,-0.0337436976235975,
0.06912526852568));
#80397=CARTESIAN_POINT('Ctrl Pts',(0.0108769509927668,-0.0336723290703325,
0.0691000996337841));
#80398=CARTESIAN_POINT('Ctrl Pts',(0.0108313123985277,-0.033601104548885,
0.0690757476967791));
#80399=CARTESIAN_POINT('Ctrl Pts',(0.0106855974076183,-0.0333736987606857,
0.0689979967857692));
#80400=CARTESIAN_POINT('Ctrl Pts',(0.0105356607479045,-0.0331450831799192,
0.0689287359684733));
#80401=CARTESIAN_POINT('',(0.0108926919337879,-0.0336938721132548,0.0691090413760902));
#80402=CARTESIAN_POINT('',(0.0106832483951838,-0.0333679869945434,0.0689995381022298));
#80403=CARTESIAN_POINT('Ctrl Pts',(0.0108926919338001,-0.0336938721132647,
0.0691090413760963));
#80404=CARTESIAN_POINT('Ctrl Pts',(0.010873014707535,-0.0336629187933931,
0.0690982330224601));
#80405=CARTESIAN_POINT('Ctrl Pts',(0.0108532804872594,-0.0336319952301038,
0.0690875433436641));
#80406=CARTESIAN_POINT('Ctrl Pts',(0.0108334914209631,-0.0336011045488948,
0.0690769732012853));
#80407=CARTESIAN_POINT('Ctrl Pts',(0.0107838338821881,-0.0335235892595452,
0.0690504490971577));
#80408=CARTESIAN_POINT('Ctrl Pts',(0.0107337426821419,-0.0334458668660368,
0.0690246306905843));
#80409=CARTESIAN_POINT('Ctrl Pts',(0.0106832483953328,-0.0333679869945383,
0.0689995381019455));
#80410=CARTESIAN_POINT('Ctrl Pts',(0.0106832088772076,-0.0333679692459107,
0.0689995176963455));
#80411=CARTESIAN_POINT('Ctrl Pts',(0.0106830124964596,-0.0333391895374034,
0.0689999261965583));
#80412=CARTESIAN_POINT('Ctrl Pts',(0.0106828682260881,-0.0333104081060166,
0.0690002337943113));
#80413=CARTESIAN_POINT('Ctrl Pts',(0.0106826822739281,-0.0332532698340219,
0.0690006433042667));
#80414=CARTESIAN_POINT('Ctrl Pts',(0.0106826390953484,-0.0332249171825216,
0.0690007482188445));
#80415=CARTESIAN_POINT('Ctrl Pts',(0.010682643640639,-0.0331960985342078,
0.069000754576199));
#80416=CARTESIAN_POINT('Ctrl Pts',(0.0106826437275517,-0.0331956312583094,
0.0690007546526169));
#80417=CARTESIAN_POINT('Ctrl Pts',(0.0106826438271752,-0.0331951640388587,
0.0690007547021237));
#80418=CARTESIAN_POINT('',(0.0107945839423478,-0.0331951640388587,0.0690563821289519));
#80419=CARTESIAN_POINT('',(0.0107386138847722,-0.0331951640388687,0.0690285684155481));
#80420=CARTESIAN_POINT('',(0.0110015980579165,-0.0335216366567716,0.0691704115788894));
#80421=CARTESIAN_POINT('Origin',(0.00373870967775345,-0.0326434571529732,
0.0841577768371651));
#80422=CARTESIAN_POINT('',(0.0110009182856956,-0.0336938721132327,0.0691715878128933));
#80423=CARTESIAN_POINT('Origin',(0.0164652605990008,-0.0336938867896302,
0.0597164414344764));
#80424=CARTESIAN_POINT('',(0.0109468051097517,-0.0336938721132538,0.0691403145945018));
#80425=CARTESIAN_POINT('Ctrl Pts',(0.0113273240884512,-0.0335235895815172,
0.0690768038353716));
#80426=CARTESIAN_POINT('Ctrl Pts',(0.011257481555041,-0.0334144449262749,
0.0690327007739887));
#80427=CARTESIAN_POINT('Ctrl Pts',(0.0111866476449646,-0.0333049234473147,
0.0689899899377093));
#80428=CARTESIAN_POINT('Ctrl Pts',(0.0111149079858693,-0.0331951640388587,
0.0689487341452395));
#80429=CARTESIAN_POINT('Ctrl Pts',(0.0112185083479003,-0.0335235895815172,
0.0691084314671863));
#80430=CARTESIAN_POINT('Ctrl Pts',(0.0111491012311111,-0.0334144449262749,
0.0690658264687105));
#80431=CARTESIAN_POINT('Ctrl Pts',(0.0110787341867489,-0.0333049234473147,
0.0690246064210513));
#80432=CARTESIAN_POINT('Ctrl Pts',(0.0110074924181604,-0.0331951640388587,
0.0689848321825771));
#80433=CARTESIAN_POINT('Ctrl Pts',(0.0111096926073494,-0.0335235895815172,
0.0691400590990009));
#80434=CARTESIAN_POINT('Ctrl Pts',(0.0110407209071812,-0.0334144449262749,
0.0690989521634323));
#80435=CARTESIAN_POINT('Ctrl Pts',(0.0109708207285332,-0.0333049234473147,
0.0690592229043934));
#80436=CARTESIAN_POINT('Ctrl Pts',(0.0109000768504515,-0.0331951640388587,
0.0690209302199148));
#80437=CARTESIAN_POINT('Ctrl Pts',(0.0110008768667985,-0.0335235895815172,
0.0691716867308156));
#80438=CARTESIAN_POINT('Ctrl Pts',(0.0109323405832513,-0.0334144449262749,
0.0691320778581541));
#80439=CARTESIAN_POINT('Ctrl Pts',(0.0108629072703175,-0.0333049234473147,
0.0690938393877355));
#80440=CARTESIAN_POINT('Ctrl Pts',(0.0107926612827427,-0.0331951640388587,
0.0690570282572524));
#80441=CARTESIAN_POINT('',(0.0109547459641184,-0.0331951640388687,0.0690025581371058));
#80442=CARTESIAN_POINT('Ctrl Pts',(0.0111260111567689,-0.0332121607146002,
0.0689551351134619));
#80443=CARTESIAN_POINT('Ctrl Pts',(0.01110453986826,-0.0332625444109438,
0.0689922876571531));
#80444=CARTESIAN_POINT('Ctrl Pts',(0.0110834385637455,-0.0333135300746151,
0.0690288000042159));
#80445=CARTESIAN_POINT('Ctrl Pts',(0.0110419591727085,-0.0334167203140627,
0.0691005732882063));
#80446=CARTESIAN_POINT('Ctrl Pts',(0.0110215971515384,-0.0334688847587306,
0.0691358064266762));
#80447=CARTESIAN_POINT('Ctrl Pts',(0.0110015980574129,-0.0335216366562379,
0.0691704115794121));
#80448=CARTESIAN_POINT('Ctrl Pts',(0.0108929503015822,-0.033693872113239,
0.0691100072751299));
#80449=CARTESIAN_POINT('Ctrl Pts',(0.0108634495517166,-0.0336474569764958,
0.0690937984152836));
#80450=CARTESIAN_POINT('Ctrl Pts',(0.0108337610780916,-0.033601104548885,
0.0690779360096034));
#80451=CARTESIAN_POINT('Ctrl Pts',(0.0107585966886809,-0.0334837508592656,
0.0690377760454171));
#80452=CARTESIAN_POINT('Ctrl Pts',(0.0106822752829264,-0.0333660264659097,
0.0689998609932269));
#80453=CARTESIAN_POINT('Ctrl Pts',(0.0108926919338059,-0.033693872113239,
0.0691090413761001));
#80454=CARTESIAN_POINT('Ctrl Pts',(0.0108631855302128,-0.0336474569764958,
0.0690928340285662));
#80455=CARTESIAN_POINT('Ctrl Pts',(0.0108334914209511,-0.033601104548885,
0.0690769732012787));
#80456=CARTESIAN_POINT('Ctrl Pts',(0.0107583127634042,-0.0334837508592656,
0.0690368172332199));
#80457=CARTESIAN_POINT('Ctrl Pts',(0.0106819772141925,-0.0333660264659097,
0.0689989065981968));
#80458=CARTESIAN_POINT('Ctrl Pts',(0.0108048457483965,-0.033693872113239,
0.0687806314386948));
#80459=CARTESIAN_POINT('Ctrl Pts',(0.0107734170524618,-0.0336474569764958,
0.0687649382840344));
#80460=CARTESIAN_POINT('Ctrl Pts',(0.010741806801852,-0.033601104548885,
0.0687496141172468));
#80461=CARTESIAN_POINT('Ctrl Pts',(0.0106617769149603,-0.0334837508592656,
0.0687108168501874));
#80462=CARTESIAN_POINT('Ctrl Pts',(0.0105806325278338,-0.0333660264659097,
0.0686744080715062));
#80463=CARTESIAN_POINT('',(0.0107938986808316,-0.0336769361243753,0.0687768744717819));
#80464=CARTESIAN_POINT('',(0.0108053696819065,-0.0336938721132327,0.0687825901460834));
#80465=CARTESIAN_POINT('Ctrl Pts',(0.0107938986808316,-0.0336769361243753,
0.0687768744717819));
#80466=CARTESIAN_POINT('Ctrl Pts',(0.0107958116749797,-0.0336797586669839,
0.0687778251134874));
#80467=CARTESIAN_POINT('Ctrl Pts',(0.0107977240890918,-0.0336825812712471,
0.0687787767408637));
#80468=CARTESIAN_POINT('Ctrl Pts',(0.0108015477607022,-0.0336882266077742,
0.0687806819681071));
#80469=CARTESIAN_POINT('Ctrl Pts',(0.0108034590181517,-0.0336910493399714,
0.0687816355679669));
#80470=CARTESIAN_POINT('Ctrl Pts',(0.0108053696819068,-0.0336938721132305,
0.0687825901460893));
#80471=CARTESIAN_POINT('Ctrl Pts',(0.0107938986808316,-0.0336769361243754,
0.068776874471782));
#80472=CARTESIAN_POINT('Ctrl Pts',(0.0107752466593742,-0.0336279018378449,
0.0688144082846725));
#80473=CARTESIAN_POINT('Ctrl Pts',(0.0107563263052245,-0.0335767825754299,
0.0688524820684775));
#80474=CARTESIAN_POINT('Ctrl Pts',(0.0107192532908787,-0.0334733171799203,
0.0689270847911321));
#80475=CARTESIAN_POINT('Ctrl Pts',(0.0107010757143986,-0.0334209631321945,
0.0689636638694876));
#80476=CARTESIAN_POINT('Ctrl Pts',(0.0106832484016998,-0.0333679869844681,
0.0689995381054628));
#80477=CARTESIAN_POINT('',(0.0108490308078572,-0.0336938721132538,0.0689458157610968));
#80478=CARTESIAN_POINT('Origin',(0.00812378219310841,-0.0315241814719618,
0.07415));
#80479=CARTESIAN_POINT('',(0.0107938986802588,-0.0337108120655415,0.0687768744729486));
#80480=CARTESIAN_POINT('',(0.0107824154971444,-0.0336938721132327,0.0687711833127828));
#80481=CARTESIAN_POINT('Origin',(0.00251200221662774,-0.0345562520221669,
0.0829313261019018));
#80482=CARTESIAN_POINT('Ctrl Pts',(0.0107824154971489,-0.0336938721132347,
0.0687711833127797));
#80483=CARTESIAN_POINT('Ctrl Pts',(0.0107843302391102,-0.0336910493139422,
0.0687721297285144));
#80484=CARTESIAN_POINT('Ctrl Pts',(0.0107862445333863,-0.0336882265947589,
0.0687730771951645));
#80485=CARTESIAN_POINT('Ctrl Pts',(0.0107900722571568,-0.0336825812713119,
0.0687749742459279));
#80486=CARTESIAN_POINT('Ctrl Pts',(0.0107919856866616,-0.0336797586670162,
0.0687759238300656));
#80487=CARTESIAN_POINT('Ctrl Pts',(0.0107938986808319,-0.033676936124375,
0.0687768744717821));
#80488=CARTESIAN_POINT('Origin',(0.00451368155345254,-0.0345562519193588,
0.0839260370577549));
#80489=CARTESIAN_POINT('Ctrl Pts',(0.0108265711063576,-0.034243627687391,
0.0690732828431734));
#80490=CARTESIAN_POINT('Ctrl Pts',(0.0106350995623394,-0.033943005420181,
0.0689713454788514));
#80491=CARTESIAN_POINT('Ctrl Pts',(0.0104364936289488,-0.0336441434784052,
0.0688841201291205));
#80492=CARTESIAN_POINT('Ctrl Pts',(0.0106033951232425,-0.034243627687391,
0.0689606219335347));
#80493=CARTESIAN_POINT('Ctrl Pts',(0.0104076745029704,-0.033943005420181,
0.0688671017901755));
#80494=CARTESIAN_POINT('Ctrl Pts',(0.0102054655840775,-0.0336441434784052,
0.0687885898067987));
#80495=CARTESIAN_POINT('Ctrl Pts',(0.0106011633634114,-0.034243627687391,
0.0689594953244383));
#80496=CARTESIAN_POINT('Ctrl Pts',(0.0104054002523767,-0.033943005420181,
0.0688660593532888));
#80497=CARTESIAN_POINT('Ctrl Pts',(0.0102031553036288,-0.0336441434784052,
0.0687876345035754));
#80498=CARTESIAN_POINT('',(0.0105707037120053,-0.0341934961088741,0.0689451272752967));
#80499=CARTESIAN_POINT('',(0.0103547976992636,-0.0338664212891259,0.0688489911502866));
#80500=CARTESIAN_POINT('Origin',(0.00299297806214719,-0.0345610818078395,
0.0838659572887302));
#80501=CARTESIAN_POINT('Origin',(0.0146086594711115,-0.0336938005044541,
0.0587413997481238));
#80502=CARTESIAN_POINT('',(0.0104694828127754,-0.0336938721132327,0.0688987321908995));
#80503=CARTESIAN_POINT('',(0.010411876761808,-0.0336938721132427,0.0688744877504997));
#80504=CARTESIAN_POINT('',(0.0106832484017046,-0.0340203938281605,0.0689995381054652));
#80505=CARTESIAN_POINT('Origin',(0.00260268290546713,-0.034558964324509,
0.0835845442688159));
#80506=CARTESIAN_POINT('',(0.0106826438271766,-0.034193496108874,0.0690007547021244));
#80507=CARTESIAN_POINT('Origin',(0.0155865124599212,-0.0341934220717751,
0.0591326094498503));
#80508=CARTESIAN_POINT('',(0.0106266737696009,-0.034193496108884,0.0689729409887205));
#80509=CARTESIAN_POINT('Ctrl Pts',(0.0110024564081781,-0.0340223579322397,
0.0688856638819777));
#80510=CARTESIAN_POINT('Ctrl Pts',(0.0109298474831456,-0.0339125849573575,
0.0688459594566543));
#80511=CARTESIAN_POINT('Ctrl Pts',(0.0108564677902201,-0.0338030433565231,
0.0688077857671993));
#80512=CARTESIAN_POINT('Ctrl Pts',(0.0107824154971451,-0.0336938721132326,
0.0687711833127826));
#80513=CARTESIAN_POINT('Ctrl Pts',(0.0108958412580681,-0.0340223579322397,
0.068924061663128));
#80514=CARTESIAN_POINT('Ctrl Pts',(0.0108237619385833,-0.0339125849573575,
0.0688858277387887));
#80515=CARTESIAN_POINT('Ctrl Pts',(0.0107509419150112,-0.0338030433565231,
0.0688491125554094));
#80516=CARTESIAN_POINT('Ctrl Pts',(0.0106774784740318,-0.0336938721132326,
0.0688139548104227));
#80517=CARTESIAN_POINT('Ctrl Pts',(0.0107892261079581,-0.0340223579322397,
0.0689624594442784));
#80518=CARTESIAN_POINT('Ctrl Pts',(0.010717676394021,-0.0339125849573575,
0.068925696020923));
#80519=CARTESIAN_POINT('Ctrl Pts',(0.0106454160398023,-0.0338030433565231,
0.0688904393436196));
#80520=CARTESIAN_POINT('Ctrl Pts',(0.0105725414509186,-0.0336938721132326,
0.0688567263080628));
#80521=CARTESIAN_POINT('Ctrl Pts',(0.0106826109578481,-0.0340223579322397,
0.0690008572254287));
#80522=CARTESIAN_POINT('Ctrl Pts',(0.0106115908494587,-0.0339125849573575,
0.0689655643030574));
#80523=CARTESIAN_POINT('Ctrl Pts',(0.0105398901645934,-0.0338030433565231,
0.0689317661318297));
#80524=CARTESIAN_POINT('Ctrl Pts',(0.0104676044278054,-0.0336938721132326,
0.0688994978057029));
#80525=CARTESIAN_POINT('',(0.0106259491549699,-0.0336938721132427,0.0688349577518512));
#80526=CARTESIAN_POINT('Ctrl Pts',(0.0107938986786503,-0.0337108120662711,
0.0687768744761719));
#80527=CARTESIAN_POINT('Ctrl Pts',(0.010774763174856,-0.0337611408993995,
0.0688153812096439));
#80528=CARTESIAN_POINT('Ctrl Pts',(0.0107559768515518,-0.0338121088780665,
0.0688531852806615));
#80529=CARTESIAN_POINT('Ctrl Pts',(0.0107190854518366,-0.0339153382773247,
0.068927422536786));
#80530=CARTESIAN_POINT('Ctrl Pts',(0.0107009959827818,-0.0339675558473121,
0.0689638243149171));
#80531=CARTESIAN_POINT('Ctrl Pts',(0.0106832484016821,-0.0340203938281304,
0.0689995381054985));
#80532=CARTESIAN_POINT('Ctrl Pts',(0.0105713497830771,-0.0341934961088741,
0.0689470497646084));
#80533=CARTESIAN_POINT('Ctrl Pts',(0.0104637828866879,-0.03402875161944,
0.0688964482332763));
#80534=CARTESIAN_POINT('Ctrl Pts',(0.0103542165044892,-0.033864463329982,
0.0688503357613862));
#80535=CARTESIAN_POINT('Ctrl Pts',(0.0105707037120054,-0.0341934961088741,
0.0689451272752969));
#80536=CARTESIAN_POINT('Ctrl Pts',(0.0104630970696646,-0.03402875161944,
0.0688945391009751));
#80537=CARTESIAN_POINT('Ctrl Pts',(0.0103534915275316,-0.033864463329982,
0.0688484416174124));
#80538=CARTESIAN_POINT('Ctrl Pts',(0.0104630557282936,-0.0341934961088741,
0.068624803231777));
#80539=CARTESIAN_POINT('Ctrl Pts',(0.0103488266387562,-0.03402875161944,
0.0685764405946958));
#80540=CARTESIAN_POINT('Ctrl Pts',(0.010232696291323,-0.033864463329982,
0.0685328404574597));
#80541=CARTESIAN_POINT('',(0.0104512484729383,-0.0341764758832396,0.0686198191072201));
#80542=CARTESIAN_POINT('',(0.0104630557282936,-0.034193496108874,0.068624803231777));
#80543=CARTESIAN_POINT('Origin',(0.00355631448922339,-0.0345621026280434,
0.0836823955081816));
#80544=CARTESIAN_POINT('Ctrl Pts',(0.0104512484740739,-0.0341764758837489,
0.0686198191086342));
#80545=CARTESIAN_POINT('Ctrl Pts',(0.0104345976465681,-0.0341260050043703,
0.068659382375928));
#80546=CARTESIAN_POINT('Ctrl Pts',(0.0104182362849394,-0.0340749269154777,
0.0686982579551276));
#80547=CARTESIAN_POINT('Ctrl Pts',(0.0103860796441643,-0.0339715436320037,
0.0687746637951318));
#80548=CARTESIAN_POINT('Ctrl Pts',(0.0103702965590176,-0.0339192778255033,
0.068812165066936));
#80549=CARTESIAN_POINT('Ctrl Pts',(0.0103547977028726,-0.0338664212876329,
0.0688489911496625));
#80550=CARTESIAN_POINT('',(0.0105168797201595,-0.0341934961088841,0.0687849652535469));
#80551=CARTESIAN_POINT('Origin',(0.00812378219310841,-0.0315241814719618,
0.07415));
#80552=CARTESIAN_POINT('',(0.0104512484718765,-0.0342105180190387,0.0686198191075735));
#80553=CARTESIAN_POINT('',(0.0104394305973826,-0.0341934961088739,0.0686148602124429));
#80554=CARTESIAN_POINT('Origin',(0.00359578260681611,-0.0345621712411221,
0.0837046830863977));
#80555=CARTESIAN_POINT('Origin',(0.00450031454071362,-0.0345621033373562,
0.0840796952059308));
#80556=CARTESIAN_POINT('Origin',(0.00445678854298556,-0.0345621719856087,
0.0840670494826787));
#80557=CARTESIAN_POINT('Ctrl Pts',(0.010470865367133,-0.0346945769586966,
0.0688993140613139));
#80558=CARTESIAN_POINT('Ctrl Pts',(0.0103608876478873,-0.0345275153362944,
0.0688501534645131));
#80559=CARTESIAN_POINT('Ctrl Pts',(0.01024933542725,-0.0343603235965185,
0.0688044388503067));
#80560=CARTESIAN_POINT('Ctrl Pts',(0.0101365406366484,-0.034193496108874,
0.0687623005187312));
#80561=CARTESIAN_POINT('Ctrl Pts',(0.0103935964475227,-0.0346945769586966,
0.0688667941838835));
#80562=CARTESIAN_POINT('Ctrl Pts',(0.0102829375864239,-0.0345275153362944,
0.0688192520155407));
#80563=CARTESIAN_POINT('Ctrl Pts',(0.0101707549458408,-0.0343603235965185,
0.0687751776696851));
#80564=CARTESIAN_POINT('Ctrl Pts',(0.0100573822496017,-0.034193496108874,
0.0687346965674563));
#80565=CARTESIAN_POINT('Ctrl Pts',(0.0103163275279121,-0.0346945769586966,
0.0688342743064553));
#80566=CARTESIAN_POINT('Ctrl Pts',(0.0102049875249603,-0.0345275153362944,
0.068788350566571));
#80567=CARTESIAN_POINT('Ctrl Pts',(0.0100921744644315,-0.0343603235965185,
0.0687459164890658));
#80568=CARTESIAN_POINT('Ctrl Pts',(0.00997822386255483,-0.034193496108874,
0.0687070926161821));
#80569=CARTESIAN_POINT('Ctrl Pts',(0.0102390586083021,-0.0346945769586966,
0.0688017544290226));
#80570=CARTESIAN_POINT('Ctrl Pts',(0.0101270374634973,-0.0345275153362944,
0.0687574491175959));
#80571=CARTESIAN_POINT('Ctrl Pts',(0.0100135939830225,-0.0343603235965185,
0.068716655308442));
#80572=CARTESIAN_POINT('Ctrl Pts',(0.00989906547550811,-0.034193496108874,
0.0686794886649065));
#80573=CARTESIAN_POINT('',(0.0102390586088605,-0.0346945769586966,0.0688017544292578));
#80574=CARTESIAN_POINT('',(0.0100175422024024,-0.034366772783146,0.0687193648596557));
#80575=CARTESIAN_POINT('Origin',(0.00422573830431933,-0.0345626457063142,
0.0845032583751714));
#80576=CARTESIAN_POINT('Origin',(0.0136567081479814,-0.0341934771029089,
0.058283507172973));
#80577=CARTESIAN_POINT('',(0.0101351242745058,-0.034193496108874,0.0687618066078136));
#80578=CARTESIAN_POINT('',(0.0100761095749121,-0.034193496108884,0.0687412271221477));
#80579=CARTESIAN_POINT('',(0.0103547977016228,-0.0345211942962687,0.0688489911525628));
#80580=CARTESIAN_POINT('Origin',(0.00378386539959845,-0.0345625596121401,
0.0843136821996429));
#80581=CARTESIAN_POINT('',(0.0103542707108205,-0.0346945769586885,0.0688502433100797));
#80582=CARTESIAN_POINT('Origin',(0.0146459511829038,-0.0346945685853839,
0.0586529890756434));
#80583=CARTESIAN_POINT('',(0.0102966646598505,-0.0346945769587026,0.0688259988696787));
#80584=CARTESIAN_POINT('Ctrl Pts',(0.0106662247308337,-0.0345231616327842,
0.0687152979895507));
#80585=CARTESIAN_POINT('Ctrl Pts',(0.0105913150150681,-0.0344132092796988,
0.068680253998641));
#80586=CARTESIAN_POINT('Ctrl Pts',(0.0105156843069898,-0.034303273855898,
0.0686467612642227));
#80587=CARTESIAN_POINT('Ctrl Pts',(0.0104394305973826,-0.034193496108874,
0.0686148602124428));
#80588=CARTESIAN_POINT('Ctrl Pts',(0.0105622311621331,-0.0345231616327842,
0.0687603143622092));
#80589=CARTESIAN_POINT('Ctrl Pts',(0.0104879419336865,-0.0344132092796988,
0.0687267037762327));
#80590=CARTESIAN_POINT('Ctrl Pts',(0.0104129613297634,-0.034303273855898,
0.0686946315384999));
#80591=CARTESIAN_POINT('Ctrl Pts',(0.0103373864616736,-0.034193496108874,
0.0686641362766711));
#80592=CARTESIAN_POINT('Ctrl Pts',(0.0104582375934324,-0.0345231616327842,
0.0688053307348676));
#80593=CARTESIAN_POINT('Ctrl Pts',(0.010384568852305,-0.0344132092796988,
0.0687731535538245));
#80594=CARTESIAN_POINT('Ctrl Pts',(0.0103102383525372,-0.034303273855898,
0.0687425018127771));
#80595=CARTESIAN_POINT('Ctrl Pts',(0.0102353423259647,-0.034193496108874,
0.0687134123408994));
#80596=CARTESIAN_POINT('Ctrl Pts',(0.0103542440247318,-0.0345231616327842,
0.068850347107526));
#80597=CARTESIAN_POINT('Ctrl Pts',(0.0102811957709235,-0.0344132092796988,
0.0688196033314162));
#80598=CARTESIAN_POINT('Ctrl Pts',(0.0102075153753109,-0.034303273855898,
0.0687903720870543));
#80599=CARTESIAN_POINT('Ctrl Pts',(0.0101332981902558,-0.034193496108874,
0.0687626884051277));
#80600=CARTESIAN_POINT('',(0.0102872774359542,-0.0341934961088839,0.0686883334101383));
#80601=CARTESIAN_POINT('Ctrl Pts',(0.0104512484705309,-0.0342105180195415,
0.0686198191107543));
#80602=CARTESIAN_POINT('Ctrl Pts',(0.0104345789114949,-0.0342610556240919,
0.0686594268497396));
#80603=CARTESIAN_POINT('Ctrl Pts',(0.0104182084790762,-0.0343122189869339,
0.0686983238483292));
#80604=CARTESIAN_POINT('Ctrl Pts',(0.0103860515174253,-0.0344158119695181,
0.0687747304611784));
#80605=CARTESIAN_POINT('Ctrl Pts',(0.010370278140664,-0.0344681990450068,
0.0688122088244829));
#80606=CARTESIAN_POINT('Ctrl Pts',(0.010354797701602,-0.0345211942962487,
0.0688489911525828));
#80607=CARTESIAN_POINT('Ctrl Pts',(0.0102398239325642,-0.0346945769586932,
0.0688036321000172));
#80608=CARTESIAN_POINT('Ctrl Pts',(0.0101292915592006,-0.034529677707698,
0.068759884434317));
#80609=CARTESIAN_POINT('Ctrl Pts',(0.0100170455031449,-0.034364806625142,
0.0687207425550122));
#80610=CARTESIAN_POINT('Ctrl Pts',(0.0102390586088688,-0.0346945769586932,
0.0688017544292611));
#80611=CARTESIAN_POINT('Ctrl Pts',(0.010128487415991,-0.034529677707698,
0.0687580225860868));
#80612=CARTESIAN_POINT('Ctrl Pts',(0.0100162032275512,-0.034364806625142,
0.0687188981202339));
#80613=CARTESIAN_POINT('Ctrl Pts',(0.0101115097307529,-0.0346945769586932,
0.0684888217448935));
#80614=CARTESIAN_POINT('Ctrl Pts',(0.00999446887604978,-0.034529677707698,
0.0684477268845236));
#80615=CARTESIAN_POINT('Ctrl Pts',(0.00987582954295247,-0.034364806625142,
0.0684115045452745));
#80616=CARTESIAN_POINT('',(0.0100994128185244,-0.0346775396664979,0.0684845888388123));
#80617=CARTESIAN_POINT('',(0.0101115097307497,-0.0346945769586887,0.0684888217448924));
#80618=CARTESIAN_POINT('Origin',(0.0047774089511205,-0.0345626617882452,
0.0842100195120109));
#80619=CARTESIAN_POINT('Ctrl Pts',(0.0100994128196703,-0.0346775396670096,
0.0684845888402199));
#80620=CARTESIAN_POINT('Ctrl Pts',(0.0100852679143845,-0.0346269749928194,
0.0685251514740384));
#80621=CARTESIAN_POINT('Ctrl Pts',(0.0100713744295451,-0.03457579028908,
0.0685649932311711));
#80622=CARTESIAN_POINT('Ctrl Pts',(0.0100440786959155,-0.0344721681088028,
0.0686432677473408));
#80623=CARTESIAN_POINT('Ctrl Pts',(0.0100306871430088,-0.0344197714289582,
0.0686816698172453));
#80624=CARTESIAN_POINT('Ctrl Pts',(0.0100175422026577,-0.0343667727830634,
0.0687193648596285));
#80625=CARTESIAN_POINT('',(0.0101752841698151,-0.0346945769587026,0.0686452880870851));
#80626=CARTESIAN_POINT('Origin',(0.00812378219310841,-0.0315241814719618,
0.07415));
#80627=CARTESIAN_POINT('',(0.0100994128174384,-0.0347116136489814,0.0684845888396831));
#80628=CARTESIAN_POINT('',(0.0100873068912883,-0.0346945769586885,0.0684803817800795));
#80629=CARTESIAN_POINT('Origin',(0.00482077341001143,-0.0345626692432209,
0.0842231616457031));
#80630=CARTESIAN_POINT('Origin',(0.00448900754622532,-0.0345626624903524,
0.0841094508668875));
#80631=CARTESIAN_POINT('Origin',(0.00444687538083543,-0.0345626699464334,
0.0840927749539778));
#80632=CARTESIAN_POINT('Ctrl Pts',(0.0101712829898971,-0.0352450361874068,
0.0687753834450469));
#80633=CARTESIAN_POINT('Ctrl Pts',(0.00996857600025991,-0.0349452760959493,
0.0686981606853295));
#80634=CARTESIAN_POINT('Ctrl Pts',(0.00976062814561051,-0.034644428984174,
0.0686364260272122));
#80635=CARTESIAN_POINT('Ctrl Pts',(0.0101689040614125,-0.0352450361874068,
0.0687745370856283));
#80636=CARTESIAN_POINT('Ctrl Pts',(0.0099661651508061,-0.0349452760959493,
0.068697404048671));
#80637=CARTESIAN_POINT('Ctrl Pts',(0.00975819222415695,-0.034644428984174,
0.0686357612628389));
#80638=CARTESIAN_POINT('Ctrl Pts',(0.00993336658769556,-0.0352450361874068,
0.0686907391233917));
#80639=CARTESIAN_POINT('Ctrl Pts',(0.00972746718508211,-0.0349452760959493,
0.068622489528026));
#80640=CARTESIAN_POINT('Ctrl Pts',(0.00951701188221981,-0.034644428984174,
0.0685699430080529));
#80641=CARTESIAN_POINT('Ctrl Pts',(0.00993101121295839,-0.0352450361874068,
0.0686899011437694));
#80642=CARTESIAN_POINT('Ctrl Pts',(0.00972508020542487,-0.0349452760959493,
0.0686217403828196));
#80643=CARTESIAN_POINT('Ctrl Pts',(0.00951460007880043,-0.034644428984174,
0.068569284825505));
#80644=CARTESIAN_POINT('',(0.0098990969872778,-0.0351951634053324,0.0686794963957505));
#80645=CARTESIAN_POINT('',(0.00967281289795655,-0.0348678972925388,0.0686111708028286));
#80646=CARTESIAN_POINT('Origin',(0.00556803005911865,-0.0345636767881918,
0.084854982652011));
#80647=CARTESIAN_POINT('Origin',(0.0126488990635694,-0.0346946199341088,
0.0579696530374064));
#80648=CARTESIAN_POINT('',(0.00979282790512056,-0.0346945769330288,0.0686461457678075));
#80649=CARTESIAN_POINT('',(0.00973263745266564,-0.0346945769458128,0.0686293124520078));
#80650=CARTESIAN_POINT('',(0.0100175422025963,-0.0350221583435276,0.0687193648597549));
#80651=CARTESIAN_POINT('Origin',(0.00509557610916057,-0.0345628458717967,
0.0847659284061648));
#80652=CARTESIAN_POINT('',(0.0100171377872637,-0.035195136029876,0.0687205337656475));
#80653=CARTESIAN_POINT('Origin',(0.0136453737232144,-0.0351951838366821,
0.0583160276328767));
#80654=CARTESIAN_POINT('',(0.00989906547612863,-0.0351951371328749,0.0686794886649999));
#80655=CARTESIAN_POINT('Ctrl Pts',(0.0103199591444846,-0.0350241211494343,
0.0685663804930619));
#80656=CARTESIAN_POINT('Ctrl Pts',(0.0102430470751497,-0.0349144232818962,
0.0685361290560242));
#80657=CARTESIAN_POINT('Ctrl Pts',(0.0101654636514139,-0.0348045283579412,
0.0685074493394749));
#80658=CARTESIAN_POINT('Ctrl Pts',(0.0100873068807874,-0.0346945769439157,
0.0684803817764428));
#80659=CARTESIAN_POINT('Ctrl Pts',(0.0102189973707346,-0.0350241211494343,
0.0686178378739136));
#80660=CARTESIAN_POINT('Ctrl Pts',(0.0101427941057225,-0.0349144232818962,
0.0685889771439134));
#80661=CARTESIAN_POINT('Ctrl Pts',(0.0100659486574713,-0.0348045283579412,
0.0685616743153149));
#80662=CARTESIAN_POINT('Ctrl Pts',(0.00998855815386677,-0.0346945769439157,
0.0685359680223534));
#80663=CARTESIAN_POINT('Ctrl Pts',(0.0101180355969845,-0.0350241211494343,
0.0686692952547653));
#80664=CARTESIAN_POINT('Ctrl Pts',(0.0100425411362953,-0.0349144232818962,
0.0686418252318026));
#80665=CARTESIAN_POINT('Ctrl Pts',(0.0099664336635288,-0.0348045283579412,
0.0686158992911549));
#80666=CARTESIAN_POINT('Ctrl Pts',(0.00988980942694615,-0.0346945769439157,
0.068591554268264));
#80667=CARTESIAN_POINT('Ctrl Pts',(0.0100170738232344,-0.0350241211494343,
0.068720752635617));
#80668=CARTESIAN_POINT('Ctrl Pts',(0.00994228816686812,-0.0349144232818962,
0.0686946733196917));
#80669=CARTESIAN_POINT('Ctrl Pts',(0.00986691866958626,-0.0348045283579412,
0.068670124266995));
#80670=CARTESIAN_POINT('Ctrl Pts',(0.00979106070002554,-0.0346945769439157,
0.0686471405141747));
#80671=CARTESIAN_POINT('',(0.00994006739851381,-0.0346945769458128,0.0685632637739539));
#80672=CARTESIAN_POINT('Ctrl Pts',(0.0100994128163504,-0.0347116136492819,
0.0684845888427845));
#80673=CARTESIAN_POINT('Ctrl Pts',(0.0100852735162157,-0.034762154653018,
0.0685251353638779));
#80674=CARTESIAN_POINT('Ctrl Pts',(0.0100713828231747,-0.0348133084092587,
0.0685649689675707));
#80675=CARTESIAN_POINT('Ctrl Pts',(0.0100440877442627,-0.0349168535524575,
0.068643241617724));
#80676=CARTESIAN_POINT('Ctrl Pts',(0.0100306921521641,-0.0349692115648189,
0.0686816554467496));
#80677=CARTESIAN_POINT('Ctrl Pts',(0.0100175422025655,-0.0350221583435,
0.0687193648597829));
#80678=CARTESIAN_POINT('Ctrl Pts',(0.00989970166157871,-0.0351951371254949,
0.0686808061201181));
#80679=CARTESIAN_POINT('Ctrl Pts',(0.00978662950959834,-0.0350307338980944,
0.0686440900993564));
#80680=CARTESIAN_POINT('Ctrl Pts',(0.00967213646435204,-0.0348659306897796,
0.0686120788462681));
#80681=CARTESIAN_POINT('Ctrl Pts',(0.00989906547609839,-0.0351951371254948,
0.0686794886651122));
#80682=CARTESIAN_POINT('Ctrl Pts',(0.00978596608656237,-0.0350307338980944,
0.0686427857970862));
#80683=CARTESIAN_POINT('Ctrl Pts',(0.00967144637065151,-0.0348659306897796,
0.0686107888112521));
#80684=CARTESIAN_POINT('Ctrl Pts',(0.00979244012651159,-0.0351951371254948,
0.0684586818329578));
#80685=CARTESIAN_POINT('Ctrl Pts',(0.00967477569425959,-0.0350307338980944,
0.0684241833771355));
#80686=CARTESIAN_POINT('Ctrl Pts',(0.00955578594716994,-0.0348659306897796,
0.0683945775979893));
#80687=CARTESIAN_POINT('Origin',(0.0111051747892662,-0.0308609197409787,
0.0634895112778859));
#80688=CARTESIAN_POINT('',(0.00985257922775907,-0.0351951371254948,0.068583221864822));
#80689=CARTESIAN_POINT('Origin',(0.00799973216735054,-0.0351840467441115,
0.0751192044374587));
#80690=CARTESIAN_POINT('Origin',(0.0105739807007534,-0.03523226137531,0.0624382776241762));
#80691=CARTESIAN_POINT('',(0.0094436321334361,-0.0351951142564665,0.0685521601739209));
#80692=CARTESIAN_POINT('',(0.00932168719774462,-0.0351951372916786,0.0685261646894785));
#80693=CARTESIAN_POINT('Origin',(0.00780291615939653,-0.0352875117313075,
0.0742641367432437));
#80694=CARTESIAN_POINT('Origin',(0.0150271178216191,-0.029832507652297,
0.0770892426711197));
#80695=CARTESIAN_POINT('Origin',(0.0128271015320566,-0.0338732790926143,
0.0672126203309357));
#80696=CARTESIAN_POINT('Ctrl Pts',(0.012482145399802,-0.0321934096636941,
0.0703972935228224));
#80697=CARTESIAN_POINT('Ctrl Pts',(0.0124149737409575,-0.0320508460844994,
0.0703192808969426));
#80698=CARTESIAN_POINT('Ctrl Pts',(0.0123457566844405,-0.0319086045664406,
0.070243131862772));
#80699=CARTESIAN_POINT('Ctrl Pts',(0.0122746567651399,-0.0317669892869893,
0.0701689981129682));
#80700=CARTESIAN_POINT('Ctrl Pts',(0.0124260670917702,-0.0321934096636941,
0.0703349584925741));
#80701=CARTESIAN_POINT('Ctrl Pts',(0.0123577796655692,-0.0320508460844994,
0.0702579496417028));
#80702=CARTESIAN_POINT('Ctrl Pts',(0.0122874746524418,-0.0319086045664406,
0.0701828336041581));
#80703=CARTESIAN_POINT('Ctrl Pts',(0.0122153167467269,-0.0317669892869893,
0.0701097596555202));
#80704=CARTESIAN_POINT('Ctrl Pts',(0.0123699887837384,-0.0321934096636941,
0.0702726234623258));
#80705=CARTESIAN_POINT('Ctrl Pts',(0.0123005855901808,-0.0320508460844994,
0.0701966183864629));
#80706=CARTESIAN_POINT('Ctrl Pts',(0.012229192620443,-0.0319086045664406,
0.0701225353455443));
#80707=CARTESIAN_POINT('Ctrl Pts',(0.012155976728314,-0.0317669892869893,
0.0700505211980724));
#80708=CARTESIAN_POINT('Ctrl Pts',(0.0123139104757066,-0.0321934096636941,
0.0702102884320775));
#80709=CARTESIAN_POINT('Ctrl Pts',(0.0122433915147925,-0.0320508460844994,
0.0701352871312231));
#80710=CARTESIAN_POINT('Ctrl Pts',(0.0121709105884443,-0.0319086045664406,
0.0700622370869305));
#80711=CARTESIAN_POINT('Ctrl Pts',(0.0120966367099011,-0.0317669892869893,
0.0699912827406245));
#80712=CARTESIAN_POINT('',(0.0123149137277173,-0.0321934096636941,0.0702114036180884));
#80713=CARTESIAN_POINT('',(0.012149559462665,-0.0318665617511309,0.0700425382089351));
#80714=CARTESIAN_POINT('Origin',(-0.000274735752390532,-0.0326371944420916,
0.0811986066656033));
#80715=CARTESIAN_POINT('Origin',(0.0198220583471527,-0.0316939261509129,
0.062214361471898));
#80716=CARTESIAN_POINT('',(0.0123993138497735,-0.0320197221621844,0.0703032587532579));
#80717=CARTESIAN_POINT('Ctrl Pts',(0.0123992292997157,-0.0320197392094758,
0.070303094235275));
#80718=CARTESIAN_POINT('Ctrl Pts',(0.0123796549715422,-0.0319792716576056,
0.0702813394172722));
#80719=CARTESIAN_POINT('Ctrl Pts',(0.0123598256836007,-0.0319386439829741,
0.0702596347898578));
#80720=CARTESIAN_POINT('Ctrl Pts',(0.0123397143748557,-0.0318979099381672,
0.0702379632718098));
#80721=CARTESIAN_POINT('Ctrl Pts',(0.0123196034636246,-0.0318571766984966,
0.0702162921821141));
#80722=CARTESIAN_POINT('Ctrl Pts',(0.0122993140654981,-0.0318163871833606,
0.070194763135152));
#80723=CARTESIAN_POINT('Ctrl Pts',(0.0122789185301591,-0.0317755399638303,
0.07017344776701));
#80724=CARTESIAN_POINT('',(0.0123985151930508,-0.0321934096636182,0.0703043325963879));
#80725=CARTESIAN_POINT('Origin',(0.0140999142739366,-0.0324111592547179,
0.068745425676449));
#80726=CARTESIAN_POINT('',(0.012356714460394,-0.0321934096636662,0.0702578681072482));
#80727=CARTESIAN_POINT('Ctrl Pts',(0.0123148067098626,-0.0321934096636618,
0.070213429015471));
#80728=CARTESIAN_POINT('Ctrl Pts',(0.012260518328002,-0.0320835708272592,
0.0701556315210916));
#80729=CARTESIAN_POINT('Ctrl Pts',(0.0122050653194668,-0.0319739230346488,
0.0700989910468487));
#80730=CARTESIAN_POINT('Ctrl Pts',(0.0121485241942168,-0.0318646057455573,
0.0700435746152177));
#80731=CARTESIAN_POINT('Ctrl Pts',(0.0123207859095765,-0.0321934096636618,
0.0701002680065709));
#80732=CARTESIAN_POINT('Ctrl Pts',(0.0122649369492106,-0.0320835708272592,
0.0700423880543674));
#80733=CARTESIAN_POINT('Ctrl Pts',(0.0122079225609088,-0.0319739230346488,
0.0699856974662205));
#80734=CARTESIAN_POINT('Ctrl Pts',(0.0121498212572286,-0.0318646057455573,
0.0699302631754066));
#80735=CARTESIAN_POINT('Ctrl Pts',(0.0123267651092905,-0.0321934096636618,
0.0699871069976707));
#80736=CARTESIAN_POINT('Ctrl Pts',(0.0122693555704193,-0.0320835708272592,
0.0699291445876432));
#80737=CARTESIAN_POINT('Ctrl Pts',(0.0122107798023508,-0.0319739230346488,
0.0698724038855923));
#80738=CARTESIAN_POINT('Ctrl Pts',(0.0121511183202404,-0.0318646057455573,
0.0698169517355954));
#80739=CARTESIAN_POINT('Ctrl Pts',(0.0123327443090045,-0.0321934096636618,
0.0698739459887705));
#80740=CARTESIAN_POINT('Ctrl Pts',(0.012273774191628,-0.0320835708272592,
0.0698159011209191));
#80741=CARTESIAN_POINT('Ctrl Pts',(0.0122136370437928,-0.0319739230346488,
0.0697591103049642));
#80742=CARTESIAN_POINT('Ctrl Pts',(0.0121524153832521,-0.0318646057455573,
0.0697036402957843));
#80743=CARTESIAN_POINT('',(0.0123236009778616,-0.0321763980308462,0.069864965326513));
#80744=CARTESIAN_POINT('',(0.0123327443089812,-0.0321934096636184,0.0698739459887476));
#80745=CARTESIAN_POINT('Origin',(0.0003105334440736,-0.032638623101237,
0.0812453123874431));
#80746=CARTESIAN_POINT('Ctrl Pts',(0.0123236009756338,-0.0321763980306277,
0.0698649653287753));
#80747=CARTESIAN_POINT('Ctrl Pts',(0.012293559046511,-0.0321259596174869,
0.0698956168198389));
#80748=CARTESIAN_POINT('Ctrl Pts',(0.0122640376327977,-0.0320749164631494,
0.0699257372340511));
#80749=CARTESIAN_POINT('Ctrl Pts',(0.0122060120782834,-0.031971605779395,
0.0699849401486972));
#80750=CARTESIAN_POINT('Ctrl Pts',(0.0121775305461949,-0.0319193786690147,
0.0700139995816793));
#80751=CARTESIAN_POINT('Ctrl Pts',(0.0121495594613591,-0.0318665617525348,
0.0700425382102534));
#80752=CARTESIAN_POINT('',(0.0123238290183593,-0.0321934096636663,0.070042674803428));
#80753=CARTESIAN_POINT('Origin',(0.00812378219310841,-0.0315241814719618,
0.07415));
#80754=CARTESIAN_POINT('',(0.0123236009781209,-0.032210423332362,0.0698649653262478));
#80755=CARTESIAN_POINT('',(0.0123144384873291,-0.0321934096636183,0.0698560042124233));
#80756=CARTESIAN_POINT('Origin',(0.000338172652233866,-0.0326387239418652,
0.0812812454835279));
#80757=CARTESIAN_POINT('Origin',(0.00118682613749727,-0.0326386238749014,
0.0821041810387247));
#80758=CARTESIAN_POINT('Origin',(0.0011503477403256,-0.0326387246157369,
0.0820772662926032));
#80759=CARTESIAN_POINT('Ctrl Pts',(0.0122630559966726,-0.0327445246967097,
0.0701569388460572));
#80760=CARTESIAN_POINT('Ctrl Pts',(0.0121124552332627,-0.032443687833936,
0.070000823582417));
#80761=CARTESIAN_POINT('Ctrl Pts',(0.0119505230710078,-0.0321434074405927,
0.0698564956907656));
#80762=CARTESIAN_POINT('Ctrl Pts',(0.0120856161413255,-0.0327445246967097,
0.069980827807975));
#80763=CARTESIAN_POINT('Ctrl Pts',(0.0119283732415301,-0.032443687833936,
0.0698314047978827));
#80764=CARTESIAN_POINT('Ctrl Pts',(0.0117603219003864,-0.0321434074405927,
0.0696942504606531));
#80765=CARTESIAN_POINT('',(0.0120593369740092,-0.0326943950436612,0.0699560122119241));
#80766=CARTESIAN_POINT('',(0.0118837058516271,-0.0323666188837389,0.0697978626995335));
#80767=CARTESIAN_POINT('Origin',(0.000611440867388505,-0.0326395579112146,
0.0822667283954489));
#80768=CARTESIAN_POINT('Origin',(0.0191040660565653,-0.0321933825603054,
0.0614402451953115));
#80769=CARTESIAN_POINT('',(0.0119774070524119,-0.0321934096532689,0.0698806088911313));
#80770=CARTESIAN_POINT('',(0.01193011238449,-0.0321934096584275,0.0698397498072968));
#80771=CARTESIAN_POINT('',(0.0121495594633223,-0.0325210109756239,0.0700425382082568));
#80772=CARTESIAN_POINT('Origin',(0.000278674135473845,-0.0326393129159324,
0.0819196682680485));
#80773=CARTESIAN_POINT('',(0.0121486085297355,-0.0326943950436593,0.0700435084366343));
#80774=CARTESIAN_POINT('Origin',(0.0198919937411281,-0.0326943765538128,
0.0621430083161342));
#80775=CARTESIAN_POINT('',(0.0121039727518823,-0.0326943950436702,0.0699997603242893));
#80776=CARTESIAN_POINT('Ctrl Pts',(0.0124883328294781,-0.0325229783203769,
0.0700328774923979));
#80777=CARTESIAN_POINT('Ctrl Pts',(0.0124315783857464,-0.032413025309245,
0.0699727122573219));
#80778=CARTESIAN_POINT('Ctrl Pts',(0.0123735879547627,-0.032303122220807,
0.0699137301860576));
#80779=CARTESIAN_POINT('Ctrl Pts',(0.0123144384841223,-0.0321934096576658,
0.0698560042092912));
#80780=CARTESIAN_POINT('Ctrl Pts',(0.0123750703955872,-0.0325229783203769,
0.0700364500692717));
#80781=CARTESIAN_POINT('Ctrl Pts',(0.0123183651997495,-0.032413025309245,
0.0699778461543701));
#80782=CARTESIAN_POINT('Ctrl Pts',(0.012260456307104,-0.032303122220807,
0.0699204241477193));
#80783=CARTESIAN_POINT('Ctrl Pts',(0.0122014204902863,-0.0321934096576658,
0.0698642549853593));
#80784=CARTESIAN_POINT('Ctrl Pts',(0.0122618079616962,-0.0325229783203769,
0.0700400226461456));
#80785=CARTESIAN_POINT('Ctrl Pts',(0.0122051520137526,-0.032413025309245,
0.0699829800514183));
#80786=CARTESIAN_POINT('Ctrl Pts',(0.0121473246594452,-0.032303122220807,
0.069927118109381));
#80787=CARTESIAN_POINT('Ctrl Pts',(0.0120884024964504,-0.0321934096576658,
0.0698725057614275));
#80788=CARTESIAN_POINT('Ctrl Pts',(0.0121485455278052,-0.0325229783203769,
0.0700435952230195));
#80789=CARTESIAN_POINT('Ctrl Pts',(0.0120919388277557,-0.032413025309245,
0.0699881139484665));
#80790=CARTESIAN_POINT('Ctrl Pts',(0.0120341930117865,-0.032303122220807,
0.0699338120710428));
#80791=CARTESIAN_POINT('Ctrl Pts',(0.0119753845026145,-0.0321934096576658,
0.0698807565374957));
#80792=CARTESIAN_POINT('',(0.0121459227703356,-0.0321934096584275,0.0698683065520066));
#80793=CARTESIAN_POINT('Ctrl Pts',(0.01232360097568,-0.0322104233328938,
0.0698649653287282));
#80794=CARTESIAN_POINT('Ctrl Pts',(0.0122935183392906,-0.0322609421830787,
0.0698956583530241));
#80795=CARTESIAN_POINT('Ctrl Pts',(0.0122639770394119,-0.0323120888239514,
0.0699257990568896));
#80796=CARTESIAN_POINT('Ctrl Pts',(0.0122059510455046,-0.0324156524631821,
0.0699850024198442));
#80797=CARTESIAN_POINT('Ctrl Pts',(0.012177490203303,-0.032468026716732,
0.0700140407431437));
#80798=CARTESIAN_POINT('Ctrl Pts',(0.0121495594632888,-0.0325210109755912,
0.0700425382082847));
#80799=CARTESIAN_POINT('Origin',(0.0130386299408862,-0.0262834582512054,
0.0802939122271317));
#80800=CARTESIAN_POINT('Origin',(0.0196196688966671,-0.0342770993098472,
0.0701915402537489));
#80801=CARTESIAN_POINT('Ctrl Pts',(0.0120593573380794,-0.0326943950436604,
0.069958039840129));
#80802=CARTESIAN_POINT('Ctrl Pts',(0.0120015842705057,-0.0325844576448134,
0.0699038002385773));
#80803=CARTESIAN_POINT('Ctrl Pts',(0.0119426853503551,-0.0324744968375322,
0.0698507516401625));
#80804=CARTESIAN_POINT('Ctrl Pts',(0.0118827369798552,-0.0323646534831894,
0.0697989609729569));
#80805=CARTESIAN_POINT('Ctrl Pts',(0.0120582193023163,-0.0326943950436604,
0.0698447268556302));
#80806=CARTESIAN_POINT('Ctrl Pts',(0.011998884569445,-0.0325844576448134,
0.0697905029383443));
#80807=CARTESIAN_POINT('Ctrl Pts',(0.0119384241978517,-0.0324744968375322,
0.0697375023231039));
#80808=CARTESIAN_POINT('Ctrl Pts',(0.0118769165895386,-0.0323646534831894,
0.0696857918489081));
#80809=CARTESIAN_POINT('Ctrl Pts',(0.0120570812665532,-0.0326943950436604,
0.0697314138711315));
#80810=CARTESIAN_POINT('Ctrl Pts',(0.0119961848683844,-0.0325844576448134,
0.0696772056381113));
#80811=CARTESIAN_POINT('Ctrl Pts',(0.0119341630453483,-0.0324744968375322,
0.0696242530060453));
#80812=CARTESIAN_POINT('Ctrl Pts',(0.0118710961992221,-0.0323646534831894,
0.0695726227248592));
#80813=CARTESIAN_POINT('Ctrl Pts',(0.0120559432307901,-0.0326943950436604,
0.0696181008866328));
#80814=CARTESIAN_POINT('Ctrl Pts',(0.0119934851673237,-0.0325844576448134,
0.0695639083378783));
#80815=CARTESIAN_POINT('Ctrl Pts',(0.011929901892845,-0.0324744968375322,
0.0695110036889868));
#80816=CARTESIAN_POINT('Ctrl Pts',(0.0118652758089055,-0.0323646534831894,
0.0694594536008104));
#80817=CARTESIAN_POINT('',(0.0120462540416307,-0.0326773559991344,0.0696097120600405));
#80818=CARTESIAN_POINT('',(0.0120559432307895,-0.0326943950436595,0.0696181008866323));
#80819=CARTESIAN_POINT('Origin',(0.00122873732670427,-0.0326395670818651,
0.0822079120823499));
#80820=CARTESIAN_POINT('Ctrl Pts',(0.012046254039433,-0.0326773559987419,
0.0696097120625729));
#80821=CARTESIAN_POINT('Ctrl Pts',(0.0120181734350441,-0.0326267922585961,
0.069642215553835));
#80822=CARTESIAN_POINT('Ctrl Pts',(0.0119905905390908,-0.0325756109579332,
0.0696741429441854));
#80823=CARTESIAN_POINT('Ctrl Pts',(0.0119363966896439,-0.0324719985462367,
0.0697368726948545));
#80824=CARTESIAN_POINT('Ctrl Pts',(0.0119098074718235,-0.0324196091621777,
0.0697676498959831));
#80825=CARTESIAN_POINT('Ctrl Pts',(0.0118837058515953,-0.0323666188837757,
0.0697978626995705));
#80826=CARTESIAN_POINT('',(0.0120576401024093,-0.0326943950436703,0.0697870565492882));
#80827=CARTESIAN_POINT('Origin',(0.00812378219310841,-0.0315241814719618,
0.07415));
#80828=CARTESIAN_POINT('',(0.0120462540416011,-0.032711433837988,0.069609712060074));
#80829=CARTESIAN_POINT('',(0.0120365469580376,-0.0326943950436593,0.0696013439463572));
#80830=CARTESIAN_POINT('Origin',(0.00126352644271611,-0.0326395674874853,
0.0822369417702879));
#80831=CARTESIAN_POINT('Origin',(0.00115270127190298,-0.0326395675869598,
0.0821422241959825));
#80832=CARTESIAN_POINT('Origin',(0.0011189287679231,-0.032639568138318,
0.0821120180695751));
#80833=CARTESIAN_POINT('Ctrl Pts',(0.0120041327497945,-0.0332451089994434,
0.0699048846238029));
#80834=CARTESIAN_POINT('Ctrl Pts',(0.0118440256038911,-0.0329451141710254,
0.069758534808149));
#80835=CARTESIAN_POINT('Ctrl Pts',(0.0116733496390936,-0.0326442513127493,
0.0696246606816282));
#80836=CARTESIAN_POINT('Ctrl Pts',(0.011815983805192,-0.0332451089994434,
0.0697402639244818));
#80837=CARTESIAN_POINT('Ctrl Pts',(0.0116496678880329,-0.0329451141710254,
0.0696010102623728));
#80838=CARTESIAN_POINT('Ctrl Pts',(0.0114733353017379,-0.0326442513127493,
0.0694746798000061));
#80839=CARTESIAN_POINT('Ctrl Pts',(0.011814102315746,-0.0332451089994434,
0.0697386177174885));
#80840=CARTESIAN_POINT('Ctrl Pts',(0.0116477243108743,-0.0329451141710254,
0.069599435016915));
#80841=CARTESIAN_POINT('Ctrl Pts',(0.0114713351583643,-0.0326442513127493,
0.06947317999119));
#80842=CARTESIAN_POINT('',(0.0117882283835276,-0.0331951640388616,0.0697171725594692));
#80843=CARTESIAN_POINT('',(0.0116030135315722,-0.0328677532355012,0.0695703630751684));
#80844=CARTESIAN_POINT('Origin',(0.00171026031731824,-0.0326402808279703,
0.0831136947616987));
#80845=CARTESIAN_POINT('Origin',(0.0182909184960013,-0.0326944278779088,
0.0607665962590047));
#80846=CARTESIAN_POINT('',(0.0117017255132845,-0.0326943950436593,0.069647062447956));
#80847=CARTESIAN_POINT('',(0.0116519586094886,-0.0326943950436694,0.0696092536489164));
#80848=CARTESIAN_POINT('',(0.0118837058516293,-0.0330220786163545,0.0697978626995353));
#80849=CARTESIAN_POINT('Origin',(0.00130923900946434,-0.0326396682765535,
0.0828484881322693));
#80850=CARTESIAN_POINT('',(0.0118828177156378,-0.0331951640388588,0.0697988907230038));
#80851=CARTESIAN_POINT('Origin',(0.0190947098355173,-0.0331952026560135,
0.0614510777399818));
#80852=CARTESIAN_POINT('',(0.0118355230495927,-0.0331951640388701,0.0697580316412465));
#80853=CARTESIAN_POINT('Ctrl Pts',(0.012221203422627,-0.0330240426238172,
0.0697669486350351));
#80854=CARTESIAN_POINT('Ctrl Pts',(0.0121608226198746,-0.032914277406352,
0.0697105026656744));
#80855=CARTESIAN_POINT('Ctrl Pts',(0.0120992448192292,-0.0328043479726691,
0.0696552767957977));
#80856=CARTESIAN_POINT('Ctrl Pts',(0.0120365469580396,-0.0326943950436593,
0.0696013439463569));
#80857=CARTESIAN_POINT('Ctrl Pts',(0.0121083888394075,-0.0330240426238172,
0.0697776259847796));
#80858=CARTESIAN_POINT('Ctrl Pts',(0.0120481551275503,-0.032914277406352,
0.0697227341462127));
#80859=CARTESIAN_POINT('Ctrl Pts',(0.0119867566193549,-0.0328043479726691,
0.069669060141141));
#80860=CARTESIAN_POINT('Ctrl Pts',(0.0119242700772341,-0.0326943950436593,
0.0696166748961364));
#80861=CARTESIAN_POINT('Ctrl Pts',(0.011995574256188,-0.0330240426238172,
0.0697883033345242));
#80862=CARTESIAN_POINT('Ctrl Pts',(0.011935487635226,-0.032914277406352,
0.069734965626751));
#80863=CARTESIAN_POINT('Ctrl Pts',(0.0118742684194807,-0.0328043479726691,
0.0696828434864842));
#80864=CARTESIAN_POINT('Ctrl Pts',(0.0118119931964286,-0.0326943950436593,
0.0696320058459159));
#80865=CARTESIAN_POINT('Ctrl Pts',(0.0118827596729685,-0.0330240426238172,
0.0697989806842687));
#80866=CARTESIAN_POINT('Ctrl Pts',(0.0118228201429016,-0.032914277406352,
0.0697471971072893));
#80867=CARTESIAN_POINT('Ctrl Pts',(0.0117617802196065,-0.0328043479726691,
0.0696966268318275));
#80868=CARTESIAN_POINT('Ctrl Pts',(0.0116997163156231,-0.0326943950436593,
0.0696473367956954));
#80869=CARTESIAN_POINT('',(0.011869136235671,-0.0326943950436694,0.0696242031971666));
#80870=CARTESIAN_POINT('Ctrl Pts',(0.0120462540394279,-0.0327114338383338,
0.0696097120625789));
#80871=CARTESIAN_POINT('Ctrl Pts',(0.0120181781057898,-0.0327619876830519,
0.069642210147415));
#80872=CARTESIAN_POINT('Ctrl Pts',(0.0119905974912604,-0.0328131562603384,
0.0696741348970017));
#80873=CARTESIAN_POINT('Ctrl Pts',(0.0119364036915331,-0.0329167375858776,
0.0697368645901201));
#80874=CARTESIAN_POINT('Ctrl Pts',(0.0119098121000111,-0.0329691088920627,
0.0697676445388245));
#80875=CARTESIAN_POINT('Ctrl Pts',(0.0118837058515961,-0.0330220786163186,
0.0697978626995695));
#80876=CARTESIAN_POINT('Ctrl Pts',(0.0117883760468137,-0.0331951640388604,
0.0697191952308074));
#80877=CARTESIAN_POINT('Ctrl Pts',(0.0116967719989783,-0.0330306422010619,
0.0696434321024011));
#80878=CARTESIAN_POINT('Ctrl Pts',(0.0116021148563886,-0.0328657861914645,
0.0695715198046872));
#80879=CARTESIAN_POINT('Ctrl Pts',(0.01178822838353,-0.0331951640388604,
0.0697171725594713));
#80880=CARTESIAN_POINT('Ctrl Pts',(0.0116965825182616,-0.0330306422010619,
0.0696414124839086));
#80881=CARTESIAN_POINT('Ctrl Pts',(0.0116018837201488,-0.0328657861914645,
0.0695695049647883));
#80882=CARTESIAN_POINT('Ctrl Pts',(0.0117636237094165,-0.0331951640388604,
0.0693801411198905));
#80883=CARTESIAN_POINT('Ctrl Pts',(0.0116650099352193,-0.0330306422010619,
0.0693048897301902));
#80884=CARTESIAN_POINT('Ctrl Pts',(0.0115633702067286,-0.0328657861914645,
0.0692337784532672));
#80885=CARTESIAN_POINT('',(0.0117534269021824,-0.0331781648281916,0.0693723772353038));
#80886=CARTESIAN_POINT('',(0.0117636237094156,-0.0331951640388588,0.0693801411198898));
#80887=CARTESIAN_POINT('Origin',(0.00233486059486569,-0.0326412092479985,
0.0829472470704646));
#80888=CARTESIAN_POINT('Ctrl Pts',(0.0117534269027313,-0.033178164828644,
0.0693723772370544));
#80889=CARTESIAN_POINT('Ctrl Pts',(0.0117274247406303,-0.0331276811546768,
0.0694066033402079));
#80890=CARTESIAN_POINT('Ctrl Pts',(0.0117018921239798,-0.033076566349777,
0.0694402114463882));
#80891=CARTESIAN_POINT('Ctrl Pts',(0.0116517439154597,-0.0329730614463061,
0.0695062204419807));
#80892=CARTESIAN_POINT('Ctrl Pts',(0.0116271485781008,-0.0329207133373501,
0.0695385946619604));
#80893=CARTESIAN_POINT('Ctrl Pts',(0.0116030135479716,-0.0328677532289369,
0.0695703630766842));
#80894=CARTESIAN_POINT('',(0.0117759260464816,-0.0331951640388701,0.0695486568396894));
#80895=CARTESIAN_POINT('Origin',(0.00812378219310841,-0.0315241814719618,
0.07415));
#80896=CARTESIAN_POINT('',(0.0117534269007285,-0.0332121607144239,0.0693723772361483));
#80897=CARTESIAN_POINT('',(0.0117432135337918,-0.0331951640388587,0.0693646351476515));
#80898=CARTESIAN_POINT('Origin',(0.00237516798546861,-0.0326413658408602,
0.0829680195320731));
#80899=CARTESIAN_POINT('Origin',(0.00120054720875783,-0.0326412098231721,
0.0820854907417792));
#80900=CARTESIAN_POINT('Origin',(0.00116973075216782,-0.0326413664870062,
0.0820522257248164));
#80901=CARTESIAN_POINT('Ctrl Pts',(0.0117299389924713,-0.0337436976235975,
0.069669625223443));
#80902=CARTESIAN_POINT('Ctrl Pts',(0.0116896418227116,-0.0336723290703325,
0.0696371909026615));
#80903=CARTESIAN_POINT('Ctrl Pts',(0.0116487677808844,-0.033601104548885,
0.0696054866480589));
#80904=CARTESIAN_POINT('Ctrl Pts',(0.0115182650620217,-0.0333736987606857,
0.0695042612433717));
#80905=CARTESIAN_POINT('Ctrl Pts',(0.0113821685039338,-0.0331450831799191,
0.0694106916486237));
#80906=CARTESIAN_POINT('Ctrl Pts',(0.0115318252498913,-0.0337436976235975,
0.0695171426178747));
#80907=CARTESIAN_POINT('Ctrl Pts',(0.0114901566284677,-0.0336723290703325,
0.0694864901621189));
#80908=CARTESIAN_POINT('Ctrl Pts',(0.0114479434069807,-0.033601104548885,
0.0694565921523709));
#80909=CARTESIAN_POINT('Ctrl Pts',(0.0113131649527408,-0.0333736987606857,
0.0693611337297076));
#80910=CARTESIAN_POINT('Ctrl Pts',(0.01117313064803,-0.0331450831799191,
0.0692735669798031));
#80911=CARTESIAN_POINT('Ctrl Pts',(0.0115298441124655,-0.0337436976235975,
0.069515617791819));
#80912=CARTESIAN_POINT('Ctrl Pts',(0.0114881617765253,-0.0336723290703325,
0.0694849831547135));
#80913=CARTESIAN_POINT('Ctrl Pts',(0.0114459351632417,-0.033601104548885,
0.069455103207414));
#80914=CARTESIAN_POINT('Ctrl Pts',(0.011311113951648,-0.0333736987606857,
0.0693597024545709));
#80915=CARTESIAN_POINT('Ctrl Pts',(0.011171040269471,-0.0331450831799191,
0.0692721957331149));
#80916=CARTESIAN_POINT('',(0.0115026578980479,-0.0336938721132548,0.0694958272517481));
#80917=CARTESIAN_POINT('',(0.0113085902837036,-0.0333679869945434,0.0693609372079656));
#80918=CARTESIAN_POINT('Ctrl Pts',(0.0115026578980595,-0.0336938721132648,
0.069495827251756));
#80919=CARTESIAN_POINT('Ctrl Pts',(0.0114844904785115,-0.0336629187933931,
0.0694826379148211));
#80920=CARTESIAN_POINT('Ctrl Pts',(0.0114662516404663,-0.0336319952301039,
0.0694695591736962));
#80921=CARTESIAN_POINT('Ctrl Pts',(0.011447943406992,-0.0336011045488949,
0.0694565921523791));
#80922=CARTESIAN_POINT('Ctrl Pts',(0.0114020017844801,-0.0335235892595453,
0.0694240534588295));
#80923=CARTESIAN_POINT('Ctrl Pts',(0.0113555414728891,-0.0334458668660368,
0.0693921605460286));
#80924=CARTESIAN_POINT('Ctrl Pts',(0.0113085902838861,-0.0333679869945384,
0.0693609372077037));
#80925=CARTESIAN_POINT('Ctrl Pts',(0.0113085536348728,-0.0333679692459108,
0.0693609120100735));
#80926=CARTESIAN_POINT('Ctrl Pts',(0.0113083076039904,-0.0333391895374089,
0.0693612926761041));
#80927=CARTESIAN_POINT('Ctrl Pts',(0.0113081259190156,-0.033310408106043,
0.0693615797664861));
#80928=CARTESIAN_POINT('Ctrl Pts',(0.0113078901079837,-0.0332532698453461,
0.0693619627412726));
#80929=CARTESIAN_POINT('Ctrl Pts',(0.0113078341202312,-0.0332249172387362,
0.0693620614167115));
#80930=CARTESIAN_POINT('Ctrl Pts',(0.0113078378332342,-0.0331960985319339,
0.0693620682938483));
#80931=CARTESIAN_POINT('Ctrl Pts',(0.0113078379098615,-0.0331956312606037,
0.0693620683805414));
#80932=CARTESIAN_POINT('Ctrl Pts',(0.011307838002495,-0.0331951640388587,
0.0693620684421443));
#80933=CARTESIAN_POINT('',(0.0114119234711446,-0.0331951640388587,0.0694312870466964));
#80934=CARTESIAN_POINT('',(0.0113598807368301,-0.0331951640388687,0.0693966777444304));
#80935=CARTESIAN_POINT('',(0.0116030135388988,-0.0335216366567709,0.0695703630888588));
#80936=CARTESIAN_POINT('Origin',(0.0025189802526022,-0.0326434571526564,
0.0835292672104726));
#80937=CARTESIAN_POINT('',(0.0116021917056727,-0.0336938721132328,0.0695714448498568));
#80938=CARTESIAN_POINT('Origin',(0.0182084903229778,-0.0336938867896242,
0.0608757189737409));
#80939=CARTESIAN_POINT('',(0.0115524248018703,-0.0336938721132538,0.0695336360508124));
#80940=CARTESIAN_POINT('Ctrl Pts',(0.0119379032835746,-0.0335235895815171,
0.0695183177670219));
#80941=CARTESIAN_POINT('Ctrl Pts',(0.0118741390586945,-0.0334144449262748,
0.0694658088808983));
#80942=CARTESIAN_POINT('Ctrl Pts',(0.0118092167823753,-0.0333049234473147,
0.0694145569893242));
#80943=CARTESIAN_POINT('Ctrl Pts',(0.011743213533793,-0.0331951640388587,
0.0693646351476513));
#80944=CARTESIAN_POINT('Ctrl Pts',(0.011825981594274,-0.0335235895815171,
0.0695360577768871));
#80945=CARTESIAN_POINT('Ctrl Pts',(0.0117624615955566,-0.0334144449262748,
0.0694850897131702));
#80946=CARTESIAN_POINT('Ctrl Pts',(0.0116978156582176,-0.0333049234473147,
0.0694353753686924));
#80947=CARTESIAN_POINT('Ctrl Pts',(0.0116321206861739,-0.0331951640388587,
0.0693869858007465));
#80948=CARTESIAN_POINT('Ctrl Pts',(0.0117140599049735,-0.0335235895815171,
0.0695537977867523));
#80949=CARTESIAN_POINT('Ctrl Pts',(0.0116507841324187,-0.0334144449262748,
0.0695043705454422));
#80950=CARTESIAN_POINT('Ctrl Pts',(0.01158641453406,-0.0333049234473147,
0.0694561937480607));
#80951=CARTESIAN_POINT('Ctrl Pts',(0.0115210278385547,-0.0331951640388587,
0.0694093364538417));
#80952=CARTESIAN_POINT('Ctrl Pts',(0.0116021382156729,-0.0335235895815171,
0.0695715377966175));
#80953=CARTESIAN_POINT('Ctrl Pts',(0.0115391066692808,-0.0334144449262748,
0.0695236513777141));
#80954=CARTESIAN_POINT('Ctrl Pts',(0.0114750134099023,-0.0333049234473147,
0.0694770121274289));
#80955=CARTESIAN_POINT('Ctrl Pts',(0.0114099349909356,-0.0331951640388587,
0.0694316871069369));
#80956=CARTESIAN_POINT('',(0.0115775685024782,-0.0331951640388687,0.069397961097184));
#80957=CARTESIAN_POINT('Ctrl Pts',(0.0117534268988279,-0.0332121607145998,
0.069372377238639));
#80958=CARTESIAN_POINT('Ctrl Pts',(0.0117274684694097,-0.0332625444109364,
0.0694065457574039));
#80959=CARTESIAN_POINT('Ctrl Pts',(0.0117019573444652,-0.0333135300745996,
0.0694401254989722));
#80960=CARTESIAN_POINT('Ctrl Pts',(0.0116518094530428,-0.0334167203140615,
0.069506134082985));
#80961=CARTESIAN_POINT('Ctrl Pts',(0.0116271921093181,-0.0334688847587301,
0.0695385373596798));
#80962=CARTESIAN_POINT('Ctrl Pts',(0.0116030135383331,-0.0335216366562365,
0.0695703630893147));
#80963=CARTESIAN_POINT('Ctrl Pts',(0.011502793169285,-0.0336938721132391,
0.0694968179164566));
#80964=CARTESIAN_POINT('Ctrl Pts',(0.0114755565504605,-0.0336474569764958,
0.0694770394439383));
#80965=CARTESIAN_POINT('Ctrl Pts',(0.0114480902659135,-0.033601104548885,
0.0694575811656658));
#80966=CARTESIAN_POINT('Ctrl Pts',(0.0113785519483352,-0.0334837508592656,
0.0694083172788185));
#80967=CARTESIAN_POINT('Ctrl Pts',(0.0113075843757529,-0.0333660264659097,
0.0693611355895662));
#80968=CARTESIAN_POINT('Ctrl Pts',(0.0115026578980645,-0.0336938721132391,
0.0694958272517603));
#80969=CARTESIAN_POINT('Ctrl Pts',(0.0114754154805508,-0.0336474569764958,
0.0694760495710293));
#80970=CARTESIAN_POINT('Ctrl Pts',(0.0114479434069807,-0.033601104548885,
0.0694565921523709));
#80971=CARTESIAN_POINT('Ctrl Pts',(0.0113783904329272,-0.0334837508592656,
0.0694073304418688));
#80972=CARTESIAN_POINT('Ctrl Pts',(0.0113074082747952,-0.0333660264659097,
0.0693601513623077));
#80973=CARTESIAN_POINT('Ctrl Pts',(0.0114566650854551,-0.0336938721132391,
0.069158996878329));
#80974=CARTESIAN_POINT('Ctrl Pts',(0.0114274510879935,-0.0336474569764958,
0.0691394884087922));
#80975=CARTESIAN_POINT('Ctrl Pts',(0.0113980107210265,-0.033601104548885,
0.0691203232627141));
#80976=CARTESIAN_POINT('Ctrl Pts',(0.0113234744806307,-0.0334837508592656,
0.0690718015191877));
#80977=CARTESIAN_POINT('Ctrl Pts',(0.0112475331711956,-0.0333660264659097,
0.069025509746177));
#80978=CARTESIAN_POINT('',(0.0114462752115993,-0.0336769361243754,0.0691538975048465));
#80979=CARTESIAN_POINT('',(0.0114569393964622,-0.0336938721132327,0.0691610058070057));
#80980=CARTESIAN_POINT('Ctrl Pts',(0.0114462752115991,-0.0336769361243751,
0.0691538975048463));
#80981=CARTESIAN_POINT('Ctrl Pts',(0.0114480539742393,-0.0336797586670174,
0.0691550804122145));
#80982=CARTESIAN_POINT('Ctrl Pts',(0.0114498320378798,-0.0336825812713142,
0.0691562642247834));
#80983=CARTESIAN_POINT('Ctrl Pts',(0.011453386769613,-0.0336882266065813,
0.0691586336613392));
#80984=CARTESIAN_POINT('Ctrl Pts',(0.0114551634377228,-0.0336910493375859,
0.0691598192853521));
#80985=CARTESIAN_POINT('Ctrl Pts',(0.0114569393964618,-0.033693872113231,
0.0691610058070105));
#80986=CARTESIAN_POINT('Ctrl Pts',(0.0114462752115993,-0.0336769361243754,
0.0691538975048466));
#80987=CARTESIAN_POINT('Ctrl Pts',(0.0114230655246271,-0.0336279007642973,
0.0691887983983469));
#80988=CARTESIAN_POINT('Ctrl Pts',(0.0113995253676171,-0.0335767878888534,
0.0692241962265806));
#80989=CARTESIAN_POINT('Ctrl Pts',(0.0113533932582843,-0.0334733199122758,
0.0692935660477545));
#80990=CARTESIAN_POINT('Ctrl Pts',(0.011330773841734,-0.0334209645148407,
0.0693275793392299));
#80991=CARTESIAN_POINT('Ctrl Pts',(0.0113085902897616,-0.0333679869844681,
0.069360937211991));
#80992=CARTESIAN_POINT('',(0.0114797986472651,-0.0336938721132538,0.069328416529387));
#80993=CARTESIAN_POINT('Origin',(0.00812378219310841,-0.0315241814719618,
0.07415));
#80994=CARTESIAN_POINT('',(0.0114462752108855,-0.0337108120655561,0.0691538975059313));
#80995=CARTESIAN_POINT('',(0.0114355958676053,-0.0336938721132327,0.0691468119977928));
#80996=CARTESIAN_POINT('Origin',(0.00145566079514954,-0.0345562520628783,
0.0821587400759693));
#80997=CARTESIAN_POINT('Ctrl Pts',(0.0114355958676116,-0.0336938721132354,
0.0691468119977896));
#80998=CARTESIAN_POINT('Ctrl Pts',(0.0114373768958059,-0.033691049310948,
0.0691479909328059));
#80999=CARTESIAN_POINT('Ctrl Pts',(0.0114391573452941,-0.0336882265932618,
0.0691491708524663));
#81000=CARTESIAN_POINT('Ctrl Pts',(0.011442717121866,-0.0336825812713166,
0.0691515326847868));
#81001=CARTESIAN_POINT('Ctrl Pts',(0.0114444964489586,-0.0336797586670186,
0.069152714597478));
#81002=CARTESIAN_POINT('Ctrl Pts',(0.0114462752115996,-0.0336769361243751,
0.0691538975048466));
#81003=CARTESIAN_POINT('Origin',(0.00331688607508279,-0.034556251966675,
0.0833964844080882));
#81004=CARTESIAN_POINT('Ctrl Pts',(0.0114415401856491,-0.0342436276873911,
0.0694520635484362));
#81005=CARTESIAN_POINT('Ctrl Pts',(0.0112643545914368,-0.033943005420181,
0.0693269322429318));
#81006=CARTESIAN_POINT('Ctrl Pts',(0.0110782469602823,-0.0336441434784052,
0.0692155027672996));
#81007=CARTESIAN_POINT('Ctrl Pts',(0.0112342441679217,-0.0342436276873911,
0.0693123196361024));
#81008=CARTESIAN_POINT('Ctrl Pts',(0.01105178804517,-0.033943005420181,
0.0691950066287928));
#81009=CARTESIAN_POINT('Ctrl Pts',(0.0108610137647496,-0.0336441434784052,
0.0690917702381949));
#81010=CARTESIAN_POINT('Ctrl Pts',(0.0112321712077444,-0.0342436276873911,
0.069310922196979));
#81011=CARTESIAN_POINT('Ctrl Pts',(0.0110496623797073,-0.033943005420181,
0.0691936873726515));
#81012=CARTESIAN_POINT('Ctrl Pts',(0.0108588414327943,-0.0336441434784052,
0.0690905329129039));
#81013=CARTESIAN_POINT('',(0.0112037525338465,-0.0341934961088741,0.0692928498375926));
#81014=CARTESIAN_POINT('',(0.0110015980565918,-0.0338664212864015,0.0691704115772006));
#81015=CARTESIAN_POINT('Origin',(0.00181571405895566,-0.0345610720403922,
0.0831462926353022));
#81016=CARTESIAN_POINT('Origin',(0.0164887661466842,-0.0336938005072906,
0.0596756914227284));
#81017=CARTESIAN_POINT('',(0.0111091446375892,-0.0336938721132327,0.0692341342496886));
#81018=CARTESIAN_POINT('',(0.0110550314616524,-0.0336938721132427,0.069202861031301));
#81019=CARTESIAN_POINT('',(0.0113085902897661,-0.0340203938281605,0.0693609372119939));
#81020=CARTESIAN_POINT('Origin',(0.00146375648181164,-0.0345589643247137,
0.0828181728425343));
#81021=CARTESIAN_POINT('',(0.0113078380024956,-0.034193496108874,0.0693620684421446));
#81022=CARTESIAN_POINT('Origin',(0.0174098449021397,-0.03419342207177,0.0601863542975626));
#81023=CARTESIAN_POINT('',(0.011255795268181,-0.0341934961088841,0.0693274591398785));
#81024=CARTESIAN_POINT('Ctrl Pts',(0.0116395534704149,-0.0340223579322396,
0.0692879682924021));
#81025=CARTESIAN_POINT('Ctrl Pts',(0.0115724933724561,-0.0339125849573575,
0.0692394766369716));
#81026=CARTESIAN_POINT('Ctrl Pts',(0.0115044767322633,-0.0338030433565231,
0.0691924070442675));
#81027=CARTESIAN_POINT('Ctrl Pts',(0.0114355958676059,-0.0336938721132327,
0.0691468119977926));
#81028=CARTESIAN_POINT('Ctrl Pts',(0.0115289664945347,-0.0340223579322396,
0.069312700874069));
#81029=CARTESIAN_POINT('Ctrl Pts',(0.0114622475233824,-0.0339125849573575,
0.0692657345014588));
#81030=CARTESIAN_POINT('Ctrl Pts',(0.0113946033401003,-0.0338030433565231,
0.0692201820592443));
#81031=CARTESIAN_POINT('Ctrl Pts',(0.0113261256141595,-0.0336938721132327,
0.0691760941329712));
#81032=CARTESIAN_POINT('Ctrl Pts',(0.0114183795186545,-0.0340223579322396,
0.0693374334557359));
#81033=CARTESIAN_POINT('Ctrl Pts',(0.0113520016743087,-0.0339125849573575,
0.0692919923659461));
#81034=CARTESIAN_POINT('Ctrl Pts',(0.0112847299479373,-0.0338030433565231,
0.0692479570742211));
#81035=CARTESIAN_POINT('Ctrl Pts',(0.0112166553607131,-0.0336938721132327,
0.0692053762681498));
#81036=CARTESIAN_POINT('Ctrl Pts',(0.0113077925427743,-0.0340223579322396,
0.0693621660374028));
#81037=CARTESIAN_POINT('Ctrl Pts',(0.0112417558252349,-0.0339125849573575,
0.0693182502304333));
#81038=CARTESIAN_POINT('Ctrl Pts',(0.0111748565557743,-0.0338030433565231,
0.0692757320891979));
#81039=CARTESIAN_POINT('Ctrl Pts',(0.0111071851072667,-0.0336938721132327,
0.0692346584033284));
#81040=CARTESIAN_POINT('',(0.0112723702526072,-0.0336938721132427,0.0691904731237507));
#81041=CARTESIAN_POINT('Ctrl Pts',(0.0114462752088848,-0.0337108120662714,
0.0691538975089284));
#81042=CARTESIAN_POINT('Ctrl Pts',(0.0114224644208348,-0.0337611408993968,
0.0691897022907372));
#81043=CARTESIAN_POINT('Ctrl Pts',(0.0113990881268399,-0.0338121088780606,
0.0692248537147147));
#81044=CARTESIAN_POINT('Ctrl Pts',(0.0113531832314666,-0.0339153382773249,
0.0692938818694883));
#81045=CARTESIAN_POINT('Ctrl Pts',(0.011330674050718,-0.0339675558473115,
0.0693277293970754));
#81046=CARTESIAN_POINT('Ctrl Pts',(0.0113085902897396,-0.0340203938281304,
0.0693609372120242));
#81047=CARTESIAN_POINT('Ctrl Pts',(0.0112041525590857,-0.0341934961088741,
0.0692948381438295));
#81048=CARTESIAN_POINT('Ctrl Pts',(0.0111037759126635,-0.0340287516182428,
0.0692311539132652));
#81049=CARTESIAN_POINT('Ctrl Pts',(0.011000852918602,-0.0338644633275951,
0.069171672742606));
#81050=CARTESIAN_POINT('Ctrl Pts',(0.0112037525338465,-0.0341934961088741,
0.0692928498375927));
#81051=CARTESIAN_POINT('Ctrl Pts',(0.0111033347807592,-0.0340287516182428,
0.0692291738772351));
#81052=CARTESIAN_POINT('Ctrl Pts',(0.0110003710569715,-0.0338644633275951,
0.0691697026686855));
#81053=CARTESIAN_POINT('Ctrl Pts',(0.0111371006348019,-0.0341934961088741,
0.0689615597749468));
#81054=CARTESIAN_POINT('Ctrl Pts',(0.0110298337206636,-0.0340287516182428,
0.0688992617900928));
#81055=CARTESIAN_POINT('Ctrl Pts',(0.0109200836410751,-0.0338644633275951,
0.0688414504606155));
#81056=CARTESIAN_POINT('',(0.0111260111596299,-0.0341764758832402,0.0689551351102066));
#81057=CARTESIAN_POINT('',(0.0111371006348019,-0.034193496108874,0.0689615597749468));
#81058=CARTESIAN_POINT('Origin',(0.0023976043209724,-0.0345621026484597,
0.0830347742799198));
#81059=CARTESIAN_POINT('Ctrl Pts',(0.0111260111605787,-0.0341764758837497,
0.0689551351117523));
#81060=CARTESIAN_POINT('Ctrl Pts',(0.0111045330374642,-0.03412600500405,
0.0689922995090502));
#81061=CARTESIAN_POINT('Ctrl Pts',(0.0110834282878793,-0.0340749269148291,
0.0690288179205656));
#81062=CARTESIAN_POINT('Ctrl Pts',(0.0110419490205638,-0.0339715436306513,
0.0691005909823929));
#81063=CARTESIAN_POINT('Ctrl Pts',(0.0110215902339459,-0.0339192778237239,
0.069135818400637));
#81064=CARTESIAN_POINT('Ctrl Pts',(0.0110015980587762,-0.033866421285529,
0.0691704115771299));
#81065=CARTESIAN_POINT('',(0.0111704265843342,-0.0341934961088841,0.0691272048062798));
#81066=CARTESIAN_POINT('Origin',(0.00812378219310841,-0.0315241814719618,
0.07415));
#81067=CARTESIAN_POINT('',(0.011126011158532,-0.0342105180190558,0.0689551351104245));
#81068=CARTESIAN_POINT('',(0.0111149079858692,-0.0341934961088739,0.0689487341452396));
#81069=CARTESIAN_POINT('Origin',(0.0024339678015844,-0.0345621713328949,
0.0830618326692768));
#81070=CARTESIAN_POINT('Origin',(0.00328436615201417,-0.034562103451728,
0.0835472554685422));
#81071=CARTESIAN_POINT('Origin',(0.00324276790918069,-0.0345621719436217,
0.0835292544665853));
#81072=CARTESIAN_POINT('Ctrl Pts',(0.0111104433623922,-0.0346945769586966,
0.0692348848118891));
#81073=CARTESIAN_POINT('Ctrl Pts',(0.0110074943068725,-0.0345275153362944,
0.0691723279979046));
#81074=CARTESIAN_POINT('Ctrl Pts',(0.0109025512692336,-0.0343603235965186,
0.0691129926565617));
#81075=CARTESIAN_POINT('Ctrl Pts',(0.0107959272325995,-0.034193496108874,
0.0690570496624815));
#81076=CARTESIAN_POINT('Ctrl Pts',(0.0110378595526856,-0.0346945769586966,
0.0691929369998567));
#81077=CARTESIAN_POINT('Ctrl Pts',(0.0109340318834479,-0.0345275153362944,
0.0691319004828274));
#81078=CARTESIAN_POINT('Ctrl Pts',(0.0108282578167764,-0.0343603235965186,
0.0690741134632593));
#81079=CARTESIAN_POINT('Ctrl Pts',(0.0107208527255505,-0.034193496108874,
0.069019742199995));
#81080=CARTESIAN_POINT('Ctrl Pts',(0.0109652757429788,-0.0346945769586966,
0.069150989187823));
#81081=CARTESIAN_POINT('Ctrl Pts',(0.0108605694600231,-0.0345275153362944,
0.0690914729677503));
#81082=CARTESIAN_POINT('Ctrl Pts',(0.0107539643643192,-0.0343603235965186,
0.0690352342699574));
#81083=CARTESIAN_POINT('Ctrl Pts',(0.0106457782185016,-0.034193496108874,
0.0689824347375092));
#81084=CARTESIAN_POINT('Ctrl Pts',(0.0108926919332724,-0.0346945769586966,
0.0691090413757918));
#81085=CARTESIAN_POINT('Ctrl Pts',(0.0107871070365987,-0.0345275153362944,
0.0690510454526731));
#81086=CARTESIAN_POINT('Ctrl Pts',(0.010679670911862,-0.0343603235965186,
0.0689963550766543));
#81087=CARTESIAN_POINT('Ctrl Pts',(0.0105707037114525,-0.034193496108874,
0.0689451272750221));
#81088=CARTESIAN_POINT('',(0.0108926919337969,-0.0346945769586966,0.0691090413760951));
#81089=CARTESIAN_POINT('',(0.0106832484015388,-0.0343667727831467,0.0689995381053479));
#81090=CARTESIAN_POINT('Origin',(0.00295886819440771,-0.0345626457066113,
0.0839330653948164));
#81091=CARTESIAN_POINT('Origin',(0.0156016783748921,-0.0341934771029074,
0.0591020787832341));
#81092=CARTESIAN_POINT('',(0.0107945839423478,-0.034193496108874,0.0690563821289519));
#81093=CARTESIAN_POINT('',(0.0107386138847722,-0.0341934961088839,0.0690285684155482));
#81094=CARTESIAN_POINT('',(0.0110015980579696,-0.0345211942962679,0.0691704115784725));
#81095=CARTESIAN_POINT('Origin',(0.00254423978503176,-0.0345625596119848,
0.0836896027246084));
#81096=CARTESIAN_POINT('',(0.0110009182856956,-0.0346945769586886,0.0691715878128933));
#81097=CARTESIAN_POINT('Origin',(0.0165368126483697,-0.0346945685853955,
0.0595926322947342));
#81098=CARTESIAN_POINT('',(0.0109468051097562,-0.0346945769587026,0.0691403145945042));
#81099=CARTESIAN_POINT('Ctrl Pts',(0.011327325588461,-0.0345231616327842,
0.0690768047825745));
#81100=CARTESIAN_POINT('Ctrl Pts',(0.0112573987348763,-0.0344132092796988,
0.0690326484470979));
#81101=CARTESIAN_POINT('Ctrl Pts',(0.0111865621502266,-0.0343032738558979,
0.0689899407716941));
#81102=CARTESIAN_POINT('Ctrl Pts',(0.0111149079858692,-0.0341934961088739,
0.0689487341452396));
#81103=CARTESIAN_POINT('Ctrl Pts',(0.0112185099925623,-0.0345231616327842,
0.0691084323374537));
#81104=CARTESIAN_POINT('Ctrl Pts',(0.0111490190802936,-0.0344132092796988,
0.0690657758717664));
#81105=CARTESIAN_POINT('Ctrl Pts',(0.0110786494380908,-0.0343032738558979,
0.0690245589716633));
#81106=CARTESIAN_POINT('Ctrl Pts',(0.0110074925701824,-0.0341934961088739,
0.0689848321314887));
#81107=CARTESIAN_POINT('Ctrl Pts',(0.0111096943966636,-0.0345231616327842,
0.0691400598923328));
#81108=CARTESIAN_POINT('Ctrl Pts',(0.0110406394257109,-0.0344132092796988,
0.0690989032964349));
#81109=CARTESIAN_POINT('Ctrl Pts',(0.010970736725955,-0.0343032738558979,
0.0690591771716325));
#81110=CARTESIAN_POINT('Ctrl Pts',(0.0109000771544955,-0.0341934961088739,
0.0690209301177378));
#81111=CARTESIAN_POINT('Ctrl Pts',(0.0110008788007649,-0.0345231616327842,
0.0691716874472119));
#81112=CARTESIAN_POINT('Ctrl Pts',(0.0109322597711282,-0.0344132092796988,
0.0691320307211034));
#81113=CARTESIAN_POINT('Ctrl Pts',(0.0108628240138192,-0.0343032738558979,
0.0690937953716017));
#81114=CARTESIAN_POINT('Ctrl Pts',(0.0107926617388087,-0.0341934961088739,
0.069057028103987));
#81115=CARTESIAN_POINT('',(0.0109547459641185,-0.0341934961088839,0.0690025581371058));
#81116=CARTESIAN_POINT('Ctrl Pts',(0.0111260111567977,-0.0342105180195417,
0.0689551351134124));
#81117=CARTESIAN_POINT('Ctrl Pts',(0.0111045088762136,-0.0342610556240891,
0.0689923412838073));
#81118=CARTESIAN_POINT('Ctrl Pts',(0.0110833924429362,-0.0343122189869276,
0.0690288798087129));
#81119=CARTESIAN_POINT('Ctrl Pts',(0.0110419127606765,-0.0344158119695171,
0.0691006535966165));
#81120=CARTESIAN_POINT('Ctrl Pts',(0.0110215664772404,-0.0344681990450065,
0.0691358595035188));
#81121=CARTESIAN_POINT('Ctrl Pts',(0.0110015980579457,-0.0345211942962475,
0.06917041157849));
#81122=CARTESIAN_POINT('Ctrl Pts',(0.0108932158881468,-0.0346945769586932,
0.0691110001613542));
#81123=CARTESIAN_POINT('Ctrl Pts',(0.0107890381319647,-0.034529677707698,
0.0690537440792977));
#81124=CARTESIAN_POINT('Ctrl Pts',(0.0106825829478883,-0.034364806625142,
0.069000842684242));
#81125=CARTESIAN_POINT('Ctrl Pts',(0.0108926919338048,-0.0346945769586932,
0.0691090413760995));
#81126=CARTESIAN_POINT('Ctrl Pts',(0.0107884736811236,-0.034529677707698,
0.0690517961264283));
#81127=CARTESIAN_POINT('Ctrl Pts',(0.0106819784828642,-0.034364806625142,
0.0689989072282593));
#81128=CARTESIAN_POINT('Ctrl Pts',(0.0108053696819096,-0.0346945769586932,
0.0687825901460849));
#81129=CARTESIAN_POINT('Ctrl Pts',(0.0106944022810373,-0.034529677707698,
0.0687271502221844));
#81130=CARTESIAN_POINT('Ctrl Pts',(0.0105812383174226,-0.034364806625142,
0.0686763440556544));
#81131=CARTESIAN_POINT('',(0.0107938986812547,-0.0346775396664983,0.0687768744726056));
#81132=CARTESIAN_POINT('',(0.0108053696819065,-0.0346945769586886,0.0687825901460834));
#81133=CARTESIAN_POINT('Origin',(0.00354294131826202,-0.034562661799158,
0.0837112814624101));
#81134=CARTESIAN_POINT('Ctrl Pts',(0.0107938986822142,-0.0346775396670097,
0.0687768744741467));
#81135=CARTESIAN_POINT('Ctrl Pts',(0.0107747814676729,-0.034626974992819,
0.0688153444327645));
#81136=CARTESIAN_POINT('Ctrl Pts',(0.0107560040408587,-0.034575790289079,
0.068853130710362));
#81137=CARTESIAN_POINT('Ctrl Pts',(0.0107191131440188,-0.034472168108786,
0.0689273669460453));
#81138=CARTESIAN_POINT('Ctrl Pts',(0.0107010141319057,-0.0344197714289279,
0.0689637877975386));
#81139=CARTESIAN_POINT('Ctrl Pts',(0.0106832484017948,-0.0343667727830644,
0.0689995381053532));
#81140=CARTESIAN_POINT('',(0.0108490308078617,-0.0346945769587026,0.0689458157610992));
#81141=CARTESIAN_POINT('Origin',(0.00812378219310841,-0.0315241814719618,
0.07415));
#81142=CARTESIAN_POINT('',(0.0107938986800678,-0.0347116136489631,0.0687768744733336));
#81143=CARTESIAN_POINT('',(0.0107824154971444,-0.0346945769586886,0.0687711833127828));
#81144=CARTESIAN_POINT('Origin',(0.00358431661738086,-0.0345626693127164,
0.0837297549436195));
#81145=CARTESIAN_POINT('Origin',(0.00326941861635258,-0.0345626624503165,
0.0835753595068454));
#81146=CARTESIAN_POINT('Origin',(0.00322970878627792,-0.0345626699997882,
0.0835535346774191));
#81147=CARTESIAN_POINT('Ctrl Pts',(0.010828755906556,-0.0352450361874068,
0.06907438379749));
#81148=CARTESIAN_POINT('Ctrl Pts',(0.010637325900258,-0.0349452760959493,
0.0689723640398209));
#81149=CARTESIAN_POINT('Ctrl Pts',(0.0104387551808783,-0.034644428984174,
0.0688850534008862));
#81150=CARTESIAN_POINT('Ctrl Pts',(0.0108265018135958,-0.0352450361874068,
0.0690732459530688));
#81151=CARTESIAN_POINT('Ctrl Pts',(0.0106350288927912,-0.0349452760959493,
0.0689713112099108));
#81152=CARTESIAN_POINT('Ctrl Pts',(0.0104364217844615,-0.034644428984174,
0.068884088576466));
#81153=CARTESIAN_POINT('Ctrl Pts',(0.010603324292784,-0.0352450361874068,
0.0689605880895869));
#81154=CARTESIAN_POINT('Ctrl Pts',(0.010407602410936,-0.0349452760959493,
0.0688670706247474));
#81155=CARTESIAN_POINT('Ctrl Pts',(0.0102053924362575,-0.034644428984174,
0.0687885614061507));
#81156=CARTESIAN_POINT('Ctrl Pts',(0.0106010925175759,-0.0352450361874068,
0.0689594615109521));
#81157=CARTESIAN_POINT('Ctrl Pts',(0.0104053281461174,-0.0349452760959493,
0.0688660282188958));
#81158=CARTESIAN_POINT('Ctrl Pts',(0.0102030821427755,-0.034644428984174,
0.0687876061344475));
#81159=CARTESIAN_POINT('',(0.0105707340058111,-0.035195163405333,0.0689451388943784));
#81160=CARTESIAN_POINT('',(0.0103547977016177,-0.0348678972925388,0.0688489911525454));
#81161=CARTESIAN_POINT('Origin',(0.00424649283679008,-0.0345636767883801,
0.0844502499871526));
#81162=CARTESIAN_POINT('Origin',(0.0146411541169871,-0.0346946199340748,
0.0586643881659914));
#81163=CARTESIAN_POINT('',(0.0104694828291501,-0.0346945769330288,0.0688987321984019));
#81164=CARTESIAN_POINT('',(0.0104118767702916,-0.0346945769458128,0.0688744877542892));
#81165=CARTESIAN_POINT('',(0.0106832484017177,-0.0350221583435276,0.0689995381054717));
#81166=CARTESIAN_POINT('Origin',(0.0037889257843654,-0.034562845871725,
0.0843026837793098));
#81167=CARTESIAN_POINT('',(0.0106827006725637,-0.0351951360298761,0.06900064710751));
#81168=CARTESIAN_POINT('Origin',(0.0155863574445573,-0.0351951838366672,
0.059132922238279));
#81169=CARTESIAN_POINT('',(0.0105707037120564,-0.0351951371328749,0.0689451272751924));
#81170=CARTESIAN_POINT('Ctrl Pts',(0.011002454721054,-0.0350241211494343,
0.0688856629594157));
#81171=CARTESIAN_POINT('Ctrl Pts',(0.0109299406367822,-0.0349144232818962,
0.0688460104256449));
#81172=CARTESIAN_POINT('Ctrl Pts',(0.0108565635031284,-0.0348045283579413,
0.0688078330758591));
#81173=CARTESIAN_POINT('Ctrl Pts',(0.0107824154871822,-0.0346945769439158,
0.0687711833078586));
#81174=CARTESIAN_POINT('Ctrl Pts',(0.0108958397411129,-0.0350241211494343,
0.0689240607178794));
#81175=CARTESIAN_POINT('Ctrl Pts',(0.0108238545702202,-0.0349144232818962,
0.0688858767617434));
#81176=CARTESIAN_POINT('Ctrl Pts',(0.0107510370230749,-0.0348045283579413,
0.0688491579355894));
#81177=CARTESIAN_POINT('Ctrl Pts',(0.0106774786195265,-0.0346945769439158,
0.0688139547423621));
#81178=CARTESIAN_POINT('Ctrl Pts',(0.0107892247611718,-0.0350241211494343,
0.068962458476343));
#81179=CARTESIAN_POINT('Ctrl Pts',(0.0107177685036583,-0.0349144232818962,
0.0689257430978419));
#81180=CARTESIAN_POINT('Ctrl Pts',(0.0106455105430213,-0.0348045283579413,
0.0688904827953198));
#81181=CARTESIAN_POINT('Ctrl Pts',(0.0105725417518708,-0.0346945769439158,
0.0688567261768656));
#81182=CARTESIAN_POINT('Ctrl Pts',(0.0106826097812307,-0.0350241211494343,
0.0690008562348067));
#81183=CARTESIAN_POINT('Ctrl Pts',(0.0106116824370963,-0.0349144232818962,
0.0689656094339404));
#81184=CARTESIAN_POINT('Ctrl Pts',(0.0105399840629677,-0.0348045283579413,
0.0689318076550501));
#81185=CARTESIAN_POINT('Ctrl Pts',(0.0104676048842151,-0.0346945769439158,
0.068899497611369));
#81186=CARTESIAN_POINT('',(0.0106259491634536,-0.0346945769458128,0.0688349577556408));
#81187=CARTESIAN_POINT('Ctrl Pts',(0.0107938986785989,-0.034711613649282,
0.068776874476275));
#81188=CARTESIAN_POINT('Ctrl Pts',(0.0107747890444062,-0.0347621546531884,
0.0688153291518623));
#81189=CARTESIAN_POINT('Ctrl Pts',(0.0107560154092216,-0.0348133084096149,
0.0688531076903387));
#81190=CARTESIAN_POINT('Ctrl Pts',(0.0107191244689285,-0.0349168561544585,
0.0689273440219596));
#81191=CARTESIAN_POINT('Ctrl Pts',(0.0107010217966311,-0.0349692089015926,
0.0689637723692235));
#81192=CARTESIAN_POINT('Ctrl Pts',(0.0106832484016836,-0.0350221583435,
0.0689995381054956));
#81193=CARTESIAN_POINT('Ctrl Pts',(0.0105711697600845,-0.0351951371254955,
0.0689465140769634));
#81194=CARTESIAN_POINT('Ctrl Pts',(0.0104635909534011,-0.0350307338980949,
0.068895915874558));
#81195=CARTESIAN_POINT('Ctrl Pts',(0.0103540127938739,-0.0348659306897799,
0.0688498072561803));
#81196=CARTESIAN_POINT('Ctrl Pts',(0.0105707037120127,-0.0351951371254955,
0.0689451272753003));
#81197=CARTESIAN_POINT('Ctrl Pts',(0.010463096234075,-0.0350307338980949,
0.0688945387081464));
#81198=CARTESIAN_POINT('Ctrl Pts',(0.0103534898260282,-0.0348659306897799,
0.0688484409018007));
#81199=CARTESIAN_POINT('Ctrl Pts',(0.0104925935694216,-0.0351951371254955,
0.0687126978711248));
#81200=CARTESIAN_POINT('Ctrl Pts',(0.0103801807593836,-0.0350307338980949,
0.0686637241821611));
#81201=CARTESIAN_POINT('Ctrl Pts',(0.0102658398700227,-0.0348659306897799,
0.0686194384836624));
#81202=CARTESIAN_POINT('Origin',(0.0124177791409169,-0.0308609197410729,
0.0639472399902608));
#81203=CARTESIAN_POINT('',(0.0105366494509915,-0.0351951371254955,0.0688437932956629));
#81204=CARTESIAN_POINT('Origin',(0.00787923681271507,-0.035184046744108,
0.0750960143801669));
#81205=CARTESIAN_POINT('Origin',(0.0120225865149937,-0.0352322613456278,
0.0628375482580576));
#81206=CARTESIAN_POINT('',(0.0101348200888148,-0.0351951142564667,0.0687617218737844));
#81207=CARTESIAN_POINT('',(0.010017094823487,-0.0351951372916786,0.0687206476183941));
#81208=CARTESIAN_POINT('Origin',(0.00779116391085792,-0.0352875111809641,
0.0742229691622023));
#81209=CARTESIAN_POINT('Origin',(0.0146042981700701,-0.0298325076522842,
0.0779312832414659));
#81210=CARTESIAN_POINT('Origin',(0.0136596643096826,-0.0338732158687684,
0.0678567639966745));
#81211=CARTESIAN_POINT('Ctrl Pts',(0.0129181172415396,-0.0321934096636941,
0.0709731324880165));
#81212=CARTESIAN_POINT('Ctrl Pts',(0.0128612528259533,-0.0320508460845115,
0.0708873161737934));
#81213=CARTESIAN_POINT('Ctrl Pts',(0.0128021255712917,-0.0319086045664646,
0.0708030923999977));
#81214=CARTESIAN_POINT('Ctrl Pts',(0.012740877718676,-0.0317669892870252,
0.0707206320341683));
#81215=CARTESIAN_POINT('Ctrl Pts',(0.0128702937786217,-0.0321934096636941,
0.070904260512422));
#81216=CARTESIAN_POINT('Ctrl Pts',(0.0128121965874705,-0.0320508460845115,
0.0708193002154108));
#81217=CARTESIAN_POINT('Ctrl Pts',(0.0127518604862539,-0.0319086045664646,
0.0707359649356342));
#81218=CARTESIAN_POINT('Ctrl Pts',(0.0126894301614559,-0.0317669892870252,
0.0706544234132635));
#81219=CARTESIAN_POINT('Ctrl Pts',(0.012822470315704,-0.0321934096636941,
0.0708353885368273));
#81220=CARTESIAN_POINT('Ctrl Pts',(0.0127631403489876,-0.0320508460845115,
0.0707512842570281));
#81221=CARTESIAN_POINT('Ctrl Pts',(0.0127015954012161,-0.0319086045664646,
0.0706688374712705));
#81222=CARTESIAN_POINT('Ctrl Pts',(0.0126379826042359,-0.0317669892870252,
0.0705882147923585));
#81223=CARTESIAN_POINT('Ctrl Pts',(0.0127746468527862,-0.0321934096636941,
0.0707665165612328));
#81224=CARTESIAN_POINT('Ctrl Pts',(0.0127140841105046,-0.0320508460845115,
0.0706832682986455));
#81225=CARTESIAN_POINT('Ctrl Pts',(0.0126513303161783,-0.0319086045664646,
0.0706017100069068));
#81226=CARTESIAN_POINT('Ctrl Pts',(0.0125865350470158,-0.0317669892870252,
0.0705220061714537));
#81227=CARTESIAN_POINT('',(0.0127755024239863,-0.0321934096636941,0.0707677486944873));
#81228=CARTESIAN_POINT('',(0.0126326164744703,-0.0318665617511315,0.0705794904547992));
#81229=CARTESIAN_POINT('Origin',(-0.00109193559559531,-0.0326371944421813,
0.0800904128854678));
#81230=CARTESIAN_POINT('Origin',(0.0212257461308028,-0.0316939261508822,
0.0637746603378429));
#81231=CARTESIAN_POINT('',(0.0128477245247605,-0.0320197221621845,0.0708694576646901));
#81232=CARTESIAN_POINT('Ctrl Pts',(0.0128476612609758,-0.0320197392094754,
0.0708692838470487));
#81233=CARTESIAN_POINT('Ctrl Pts',(0.0128309678839123,-0.031979271657605,
0.0708452472584388));
#81234=CARTESIAN_POINT('Ctrl Pts',(0.0128140152669662,-0.0319386439829738,
0.0708212285097176));
#81235=CARTESIAN_POINT('Ctrl Pts',(0.0127967787033311,-0.0318979099381669,
0.0707972072627064));
#81236=CARTESIAN_POINT('Ctrl Pts',(0.0127795424803885,-0.0318571766984965,
0.0707731864904916));
#81237=CARTESIAN_POINT('Ctrl Pts',(0.0127621113752979,-0.0318163871833607,
0.0707492842706211));
#81238=CARTESIAN_POINT('Ctrl Pts',(0.0127445481888604,-0.0317755399638303,
0.0707255807421288));
#81239=CARTESIAN_POINT('',(0.0128467975774529,-0.0321934096636184,0.0708704229420174));
#81240=CARTESIAN_POINT('Origin',(0.0147312197857156,-0.0324113359903585,
0.0695363024491413));
#81241=CARTESIAN_POINT('',(0.0128111500007296,-0.0321934096636663,0.0708190858182624));
#81242=CARTESIAN_POINT('Ctrl Pts',(0.0127751424003961,-0.0321934096636617,
0.0707697447081129));
#81243=CARTESIAN_POINT('Ctrl Pts',(0.0127285260455041,-0.0320835708272592,
0.0707055988257963));
#81244=CARTESIAN_POINT('Ctrl Pts',(0.0126806092342916,-0.0319739230346488,
0.07064245487374));
#81245=CARTESIAN_POINT('Ctrl Pts',(0.0126314594732712,-0.0318646057455572,
0.0705803889351675));
#81246=CARTESIAN_POINT('Ctrl Pts',(0.0127952572874932,-0.0321934096636617,
0.0706582254000018));
#81247=CARTESIAN_POINT('Ctrl Pts',(0.0127471029944293,-0.0320835708272592,
0.0705938021177154));
#81248=CARTESIAN_POINT('Ctrl Pts',(0.0126976433963337,-0.0319739230346488,
0.0705304127541433));
#81249=CARTESIAN_POINT('Ctrl Pts',(0.0126469479977051,-0.0318646057455572,
0.0704681335550053));
#81250=CARTESIAN_POINT('Ctrl Pts',(0.0128153721745904,-0.0321934096636617,
0.0705467060918906));
#81251=CARTESIAN_POINT('Ctrl Pts',(0.0127656799433545,-0.0320835708272592,
0.0704820054096346));
#81252=CARTESIAN_POINT('Ctrl Pts',(0.0127146775583757,-0.0319739230346488,
0.0704183706345465));
#81253=CARTESIAN_POINT('Ctrl Pts',(0.0126624365221389,-0.0318646057455573,
0.070355878174843));
#81254=CARTESIAN_POINT('Ctrl Pts',(0.0128354870616876,-0.0321934096636617,
0.0704351867837794));
#81255=CARTESIAN_POINT('Ctrl Pts',(0.0127842568922798,-0.0320835708272592,
0.0703702087015537));
#81256=CARTESIAN_POINT('Ctrl Pts',(0.0127317117204177,-0.0319739230346488,
0.0703063285149497));
#81257=CARTESIAN_POINT('Ctrl Pts',(0.0126779250465728,-0.0318646057455573,
0.0702436227946807));
#81258=CARTESIAN_POINT('',(0.0128275414038829,-0.0321763980308272,0.0704251309734677));
#81259=CARTESIAN_POINT('',(0.0128354870616674,-0.0321934096636184,0.0704351867837538));
#81260=CARTESIAN_POINT('Origin',(-0.00051713526300068,-0.0326386231325254,
0.080210103995993));
#81261=CARTESIAN_POINT('Ctrl Pts',(0.0128275414013882,-0.0321763980306274,
0.0704251309754336));
#81262=CARTESIAN_POINT('Ctrl Pts',(0.0127938947113604,-0.0321259596174857,
0.0704517755182162));
#81263=CARTESIAN_POINT('Ctrl Pts',(0.0127608309939017,-0.0320749164631472,
0.0704779584097262));
#81264=CARTESIAN_POINT('Ctrl Pts',(0.0126958428954888,-0.0319716057793956,
0.0705294219613292));
#81265=CARTESIAN_POINT('Ctrl Pts',(0.0126639438360868,-0.0319193786690155,
0.0705546825694891));
#81266=CARTESIAN_POINT('Ctrl Pts',(0.0126326164730091,-0.0318665617525358,
0.0705794904559439));
#81267=CARTESIAN_POINT('',(0.0128054947428368,-0.0321934096636663,0.0706014677391306));
#81268=CARTESIAN_POINT('Origin',(0.00812378219310841,-0.0315241814719618,
0.07415));
#81269=CARTESIAN_POINT('',(0.0128275414041736,-0.0322104233323615,0.070425130973237));
#81270=CARTESIAN_POINT('',(0.0128195742877292,-0.0321934096636183,0.070415092155874));
#81271=CARTESIAN_POINT('Origin',(-0.000494217309984561,-0.0326387239311533,
0.0802492176941288));
#81272=CARTESIAN_POINT('Origin',(0.000244603150060192,-0.032638623943266,
0.0811720287119732));
#81273=CARTESIAN_POINT('Origin',(0.000211785609694622,-0.0326387246802686,
0.0811407543132531));
#81274=CARTESIAN_POINT('Ctrl Pts',(0.012730879852634,-0.0327445246967096,
0.0707072138963343));
#81275=CARTESIAN_POINT('Ctrl Pts',(0.0126010330520267,-0.0324436878339359,
0.0705334543675219));
#81276=CARTESIAN_POINT('Ctrl Pts',(0.012458466854592,-0.0321434074405927,
0.0703699690628913));
#81277=CARTESIAN_POINT('Ctrl Pts',(0.0125769117294142,-0.0327445246967096,
0.0705102524355553));
#81278=CARTESIAN_POINT('Ctrl Pts',(0.0124396364058737,-0.0324436878339359,
0.0703422999094418));
#81279=CARTESIAN_POINT('Ctrl Pts',(0.0122901001963318,-0.0321434074405927,
0.0701851646571368));
#81280=CARTESIAN_POINT('',(0.0125539500000773,-0.0326943950436612,0.0704823388648763));
#81281=CARTESIAN_POINT('',(0.0123995251713282,-0.0323666188837389,0.0703034239921451));
#81282=CARTESIAN_POINT('Origin',(-0.000346617892861598,-0.0326395579109293,
0.0812611795379471));
#81283=CARTESIAN_POINT('Origin',(0.0206104378674234,-0.0321933825603114,
0.062916659848448));
#81284=CARTESIAN_POINT('',(0.0124821166624009,-0.0321934096532689,0.0703972615797893));
#81285=CARTESIAN_POINT('',(0.0124403159281592,-0.0321934096584275,0.0703507970883738));
#81286=CARTESIAN_POINT('',(0.0126326164752063,-0.0325210109756239,0.0705794904542097));
#81287=CARTESIAN_POINT('Origin',(-0.000633262491841339,-0.0326393129156863,
0.0808751493528338));
#81288=CARTESIAN_POINT('',(0.012631551438155,-0.0326943950436593,0.0705803338484653));
#81289=CARTESIAN_POINT('Origin',(0.021304072888729,-0.0326943765538186,
0.0637126349329132));
#81290=CARTESIAN_POINT('',(0.0125927507191262,-0.0326943950436702,0.0705313363566808));
#81291=CARTESIAN_POINT('Ctrl Pts',(0.0129699293209419,-0.0325229783203769,
0.0706123654774067));
#81292=CARTESIAN_POINT('Ctrl Pts',(0.0129211631064109,-0.032413025309245,
0.0705455614452278));
#81293=CARTESIAN_POINT('Ctrl Pts',(0.0128710223610104,-0.0323031222208069,
0.0704797763369814));
#81294=CARTESIAN_POINT('Ctrl Pts',(0.0128195742849418,-0.0321934096576658,
0.0704150921523647));
#81295=CARTESIAN_POINT('Ctrl Pts',(0.0128571122325598,-0.0325229783203769,
0.0706017143363639));
#81296=CARTESIAN_POINT('Ctrl Pts',(0.0128081991922824,-0.032413025309245,
0.0705364654852812));
#81297=CARTESIAN_POINT('Ctrl Pts',(0.0127579438143233,-0.0323031222208069,
0.0704722383595365));
#81298=CARTESIAN_POINT('Ctrl Pts',(0.0127064133752996,-0.0321934096576658,
0.0704091129579808));
#81299=CARTESIAN_POINT('Ctrl Pts',(0.0127442951441776,-0.0325229783203769,
0.0705910631953211));
#81300=CARTESIAN_POINT('Ctrl Pts',(0.0126952352781539,-0.032413025309245,
0.0705273695253346));
#81301=CARTESIAN_POINT('Ctrl Pts',(0.0126448652676362,-0.0323031222208069,
0.0704647003820916));
#81302=CARTESIAN_POINT('Ctrl Pts',(0.0125932524656573,-0.0321934096576658,
0.0704031337635969));
#81303=CARTESIAN_POINT('Ctrl Pts',(0.0126314780557955,-0.0325229783203769,
0.0705804120542783));
#81304=CARTESIAN_POINT('Ctrl Pts',(0.0125822713640254,-0.032413025309245,
0.070518273565388));
#81305=CARTESIAN_POINT('Ctrl Pts',(0.0125317867209491,-0.0323031222208069,
0.0704571624046467));
#81306=CARTESIAN_POINT('Ctrl Pts',(0.0124800915560151,-0.0321934096576658,
0.0703971545692129));
#81307=CARTESIAN_POINT('',(0.0126508454754985,-0.0321934096584275,0.0704061768681168));
#81308=CARTESIAN_POINT('Ctrl Pts',(0.0128275414014406,-0.0322104233328928,
0.0704251309753922));
#81309=CARTESIAN_POINT('Ctrl Pts',(0.0127938491196484,-0.0322609421830675,
0.0704518116219258));
#81310=CARTESIAN_POINT('Ctrl Pts',(0.0127607631298716,-0.0323120888239297,
0.0704780121506965));
#81311=CARTESIAN_POINT('Ctrl Pts',(0.0126957745393272,-0.0324156524631819,
0.0705294760920144));
#81312=CARTESIAN_POINT('Ctrl Pts',(0.0126638986524107,-0.032468026716732,
0.0705547183500784));
#81313=CARTESIAN_POINT('Ctrl Pts',(0.0126326164751696,-0.0325210109755912,
0.0705794904542332));
#81314=CARTESIAN_POINT('Origin',(0.0122298385122406,-0.0262834582511817,
0.0808614594048683));
#81315=CARTESIAN_POINT('Origin',(0.0200250990363695,-0.0342770846373871,
0.0716635617413367));
#81316=CARTESIAN_POINT('Ctrl Pts',(0.0125537160743714,-0.0326943950436604,
0.0704843530569219));
#81317=CARTESIAN_POINT('Ctrl Pts',(0.0125031965893412,-0.0325844576448134,
0.0704233002654571));
#81318=CARTESIAN_POINT('Ctrl Pts',(0.0124514108571436,-0.0324744968375322,
0.0703632879789696));
#81319=CARTESIAN_POINT('Ctrl Pts',(0.0123984262892402,-0.0323646534831894,
0.0703043921735224));
#81320=CARTESIAN_POINT('Ctrl Pts',(0.0125667888951122,-0.0326943950436604,
0.0703717909454488));
#81321=CARTESIAN_POINT('Ctrl Pts',(0.012514718093222,-0.0325844576448134,
0.0703105579860131));
#81322=CARTESIAN_POINT('Ctrl Pts',(0.0124613772082064,-0.0324744968375322,
0.0702503976025801));
#81323=CARTESIAN_POINT('Ctrl Pts',(0.0124068356466964,-0.0323646534831894,
0.0701913859334797));
#81324=CARTESIAN_POINT('Ctrl Pts',(0.0125798617158531,-0.0326943950436604,
0.0702592288339757));
#81325=CARTESIAN_POINT('Ctrl Pts',(0.0125262395971029,-0.0325844576448134,
0.0701978157065692));
#81326=CARTESIAN_POINT('Ctrl Pts',(0.0124713435592691,-0.0324744968375322,
0.0701375072261906));
#81327=CARTESIAN_POINT('Ctrl Pts',(0.0124152450041526,-0.0323646534831894,
0.0700783796934372));
#81328=CARTESIAN_POINT('Ctrl Pts',(0.0125929345365939,-0.0326943950436604,
0.0701466667225027));
#81329=CARTESIAN_POINT('Ctrl Pts',(0.0125377611009837,-0.0325844576448134,
0.0700850734271252));
#81330=CARTESIAN_POINT('Ctrl Pts',(0.0124813099103318,-0.0324744968375322,
0.0700246168498011));
#81331=CARTESIAN_POINT('Ctrl Pts',(0.0124236543616088,-0.0323646534831894,
0.0699653734533945));
#81332=CARTESIAN_POINT('',(0.0125843731483486,-0.0326773559991344,0.070137129666905));
#81333=CARTESIAN_POINT('',(0.0125929345365934,-0.0326943950436594,0.0701466667225021));
#81334=CARTESIAN_POINT('Origin',(0.000273182598529205,-0.0326395671180591,
0.081280194740831));
#81335=CARTESIAN_POINT('Ctrl Pts',(0.0125843731458498,-0.0326773559987417,
0.0701371296691427));
#81336=CARTESIAN_POINT('Ctrl Pts',(0.0125524401977528,-0.0326267922585975,
0.0701658574277184));
#81337=CARTESIAN_POINT('Ctrl Pts',(0.012521073238102,-0.0325756109579366,
0.0701940760075177));
#81338=CARTESIAN_POINT('Ctrl Pts',(0.012459444600851,-0.032471998546237,
0.0702495188249775));
#81339=CARTESIAN_POINT('Ctrl Pts',(0.0124292076408168,-0.0324196091621768,
0.0702767208260358));
#81340=CARTESIAN_POINT('Ctrl Pts',(0.012399525171292,-0.0323666188837756,
0.0703034239921777));
#81341=CARTESIAN_POINT('',(0.0125734422683454,-0.0326943950436702,0.0703145027936992));
#81342=CARTESIAN_POINT('Origin',(0.00812378219310841,-0.0315241814719618,
0.07415));
#81343=CARTESIAN_POINT('',(0.0125843731483153,-0.0327114338380057,0.0701371296669343));
#81344=CARTESIAN_POINT('',(0.0125757914107548,-0.0326943950436593,0.070127610918123));
#81345=CARTESIAN_POINT('Origin',(0.000304059173981302,-0.032639567556057,
0.0813133555451849));
#81346=CARTESIAN_POINT('Origin',(0.000205979022221549,-0.032639567528189,
0.0812054949052792));
#81347=CARTESIAN_POINT('Origin',(0.000176258798741688,-0.0326395682305313,
0.0811712942880879));
#81348=CARTESIAN_POINT('Ctrl Pts',(0.0125055890636029,-0.0332451089994434,
0.0704246955091312));
#81349=CARTESIAN_POINT('Ctrl Pts',(0.012365086905994,-0.0329451141710254,
0.0702594329591735));
#81350=CARTESIAN_POINT('Ctrl Pts',(0.0122125356493249,-0.0326442513127493,
0.0701052230995668));
#81351=CARTESIAN_POINT('Ctrl Pts',(0.0123395561741835,-0.0332451089994434,
0.0702377915775753));
#81352=CARTESIAN_POINT('Ctrl Pts',(0.0121920048194651,-0.0329451141710254,
0.0700787910604944));
#81353=CARTESIAN_POINT('Ctrl Pts',(0.0120328960736271,-0.0326442513127493,
0.0699313564183334));
#81354=CARTESIAN_POINT('',(0.0123149137277534,-0.0331951640388616,0.0702114036181268));
#81355=CARTESIAN_POINT('',(0.0121495594633191,-0.0328677532092642,0.0700425382082537));
#81356=CARTESIAN_POINT('Origin',(0.000637477768746615,-0.0326401908898243,
0.0822392685832872));
#81357=CARTESIAN_POINT('Origin',(0.0198883945788821,-0.0326944279134316,
0.0621466781364469));
#81358=CARTESIAN_POINT('',(0.0122378800854608,-0.0326943950436593,0.0701310046613436));
#81359=CARTESIAN_POINT('',(0.0121932443076082,-0.0326943950436694,0.070087256548999));
#81360=CARTESIAN_POINT('',(0.0123995251713301,-0.0330220786163546,0.0703034239921472));
#81361=CARTESIAN_POINT('Origin',(0.000272764073846864,-0.0326396682762954,
0.0819258092225879));
#81362=CARTESIAN_POINT('',(0.0123985151930507,-0.0331951640388588,0.0703043325963879));
#81363=CARTESIAN_POINT('Origin',(0.0205997976903381,-0.0331952026560079,
0.0629262342684439));
#81364=CARTESIAN_POINT('',(0.0123567144604121,-0.0331951640388701,0.0702578681072674));
#81365=CARTESIAN_POINT('Ctrl Pts',(0.0127382360328429,-0.0330240426238172,
0.0703150533561725));
#81366=CARTESIAN_POINT('Ctrl Pts',(0.0126854059066167,-0.032914277406352,
0.0702514847588856));
#81367=CARTESIAN_POINT('Ctrl Pts',(0.0126312353021698,-0.0328043479726692,
0.0701889766166173));
#81368=CARTESIAN_POINT('Ctrl Pts',(0.0125757914107584,-0.0326943950436594,
0.0701276109181229));
#81369=CARTESIAN_POINT('Ctrl Pts',(0.0126249727995383,-0.0330240426238172,
0.070311507095317));
#81370=CARTESIAN_POINT('Ctrl Pts',(0.0125720938201138,-0.032914277406352,
0.0702494988094159));
#81371=CARTESIAN_POINT('Ctrl Pts',(0.0125179065941085,-0.0328043479726692,
0.0701885527663376));
#81372=CARTESIAN_POINT('Ctrl Pts',(0.0124624783891836,-0.0326943950436594,
0.0701287489542584));
#81373=CARTESIAN_POINT('Ctrl Pts',(0.0125117095662337,-0.0330240426238172,
0.0703079608344614));
#81374=CARTESIAN_POINT('Ctrl Pts',(0.012458781733611,-0.032914277406352,
0.0702475128599461));
#81375=CARTESIAN_POINT('Ctrl Pts',(0.0124045778860471,-0.0328043479726691,
0.0701881289160579));
#81376=CARTESIAN_POINT('Ctrl Pts',(0.0123491653676087,-0.0326943950436594,
0.0701298869903938));
#81377=CARTESIAN_POINT('Ctrl Pts',(0.012398446332929,-0.0330240426238172,
0.0703044145736059));
#81378=CARTESIAN_POINT('Ctrl Pts',(0.0123454696471081,-0.032914277406352,
0.0702455269104764));
#81379=CARTESIAN_POINT('Ctrl Pts',(0.0122912491779858,-0.0328043479726691,
0.0701877050657782));
#81380=CARTESIAN_POINT('Ctrl Pts',(0.0122358523460338,-0.0326943950436594,
0.0701310250265293));
#81381=CARTESIAN_POINT('',(0.0124068357481178,-0.0326943950436693,0.0701293077897432));
#81382=CARTESIAN_POINT('Ctrl Pts',(0.0125843731458447,-0.0327114338383328,
0.0701371296691474));
#81383=CARTESIAN_POINT('Ctrl Pts',(0.0125524455092796,-0.032761987683039,
0.0701658526493228));
#81384=CARTESIAN_POINT('Ctrl Pts',(0.0125210811440439,-0.0328131562603137,
0.0701940688951149));
#81385=CARTESIAN_POINT('Ctrl Pts',(0.0124594525633205,-0.0329167375858776,
0.070249511661721));
#81386=CARTESIAN_POINT('Ctrl Pts',(0.01242921290394,-0.0329691088920628,
0.0702767160911853));
#81387=CARTESIAN_POINT('Ctrl Pts',(0.0123995251712929,-0.0330220786163187,
0.070303423992177));
#81388=CARTESIAN_POINT('Ctrl Pts',(0.0123148067187297,-0.0331951640388604,
0.0702134288472416));
#81389=CARTESIAN_POINT('Ctrl Pts',(0.0122605884084061,-0.0330855618127442,
0.0701557059560538));
#81390=CARTESIAN_POINT('Ctrl Pts',(0.012205137979225,-0.032975722417194,
0.0700990620531625));
#81391=CARTESIAN_POINT('Ctrl Pts',(0.0121485228807675,-0.0328657861694598,
0.0700435731575748));
#81392=CARTESIAN_POINT('Ctrl Pts',(0.0123207859154805,-0.0331951640388604,
0.0701002678944106));
#81393=CARTESIAN_POINT('Ctrl Pts',(0.0122650090417729,-0.0330855618127442,
0.0700424626518737));
#81394=CARTESIAN_POINT('Ctrl Pts',(0.0122079972235993,-0.032975722417194,
0.0699857685511122));
#81395=CARTESIAN_POINT('Ctrl Pts',(0.0121498199068405,-0.0328657861694598,
0.0699302617734918));
#81396=CARTESIAN_POINT('Ctrl Pts',(0.0123267651122312,-0.0331951640388604,
0.0699871069415795));
#81397=CARTESIAN_POINT('Ctrl Pts',(0.0122694296751397,-0.0330855618127442,
0.0699292193476936));
#81398=CARTESIAN_POINT('Ctrl Pts',(0.0122108564679736,-0.032975722417194,
0.0698724750490619));
#81399=CARTESIAN_POINT('Ctrl Pts',(0.0121511169329135,-0.0328657861694598,
0.0698169503894089));
#81400=CARTESIAN_POINT('Ctrl Pts',(0.012332744308982,-0.0331951640388604,
0.0698739459887484));
#81401=CARTESIAN_POINT('Ctrl Pts',(0.0122738503085065,-0.0330855618127442,
0.0698159760435136));
#81402=CARTESIAN_POINT('Ctrl Pts',(0.0122137157123479,-0.032975722417194,
0.0697591815470117));
#81403=CARTESIAN_POINT('Ctrl Pts',(0.0121524139589865,-0.0328657861694598,
0.069703639005326));
#81404=CARTESIAN_POINT('',(0.0123236009781538,-0.0331781648279009,0.0698649653262148));
#81405=CARTESIAN_POINT('',(0.0123327443089812,-0.0331951640388588,0.0698739459887476));
#81406=CARTESIAN_POINT('Origin',(0.00127792040768298,-0.0326412092999731,
0.0821523339323979));
#81407=CARTESIAN_POINT('Ctrl Pts',(0.0123236009756894,-0.0331781648273353,
0.0698649653287185));
#81408=CARTESIAN_POINT('Ctrl Pts',(0.0122935140830046,-0.0331276810207345,
0.0698956626956716));
#81409=CARTESIAN_POINT('Ctrl Pts',(0.0122639706921897,-0.0330765665168817,
0.0699258055328992));
#81410=CARTESIAN_POINT('Ctrl Pts',(0.0122059446106328,-0.0329730612715187,
0.0699850089852818));
#81411=CARTESIAN_POINT('Ctrl Pts',(0.0121774859444844,-0.0329207135598912,
0.0700140450883752));
#81412=CARTESIAN_POINT('Ctrl Pts',(0.0121495594632872,-0.0328677532092985,
0.0700425382082862));
#81413=CARTESIAN_POINT('',(0.0123238290183773,-0.0331951640388702,0.0700426748034472));
#81414=CARTESIAN_POINT('Origin',(0.00812378219310841,-0.0315241814719618,
0.07415));
#81415=CARTESIAN_POINT('',(0.0123236009778316,-0.0332121607144425,0.0698649653265427));
#81416=CARTESIAN_POINT('',(0.0123144384873285,-0.0331951640388587,0.0698560042124233));
#81417=CARTESIAN_POINT('Origin',(0.00131530656577935,-0.0326413659023442,
0.0821779943499873));
#81418=CARTESIAN_POINT('Origin',(0.000260558269677515,-0.0326412097716166,
0.0811552055021783));
#81419=CARTESIAN_POINT('Origin',(0.000234154020173135,-0.03264136646171,
0.0811183405156123));
#81420=CARTESIAN_POINT('Ctrl Pts',(0.0122630432273274,-0.0337436976235975,
0.0701569256091833));
#81421=CARTESIAN_POINT('Ctrl Pts',(0.0122271289110894,-0.0336723290703325,
0.0701196964681194));
#81422=CARTESIAN_POINT('Ctrl Pts',(0.0121905507700376,-0.033601104548885,
0.0700831193352028));
#81423=CARTESIAN_POINT('Ctrl Pts',(0.0120737640113806,-0.0333736987606857,
0.0699663357953221));
#81424=CARTESIAN_POINT('Ctrl Pts',(0.0119504679951764,-0.0331450831799192,
0.0698564466030744));
#81425=CARTESIAN_POINT('Ctrl Pts',(0.0120856028087995,-0.0337436976235975,
0.069980815138533));
#81426=CARTESIAN_POINT('Ctrl Pts',(0.0120481045282982,-0.0336723290703325,
0.0699451819234852));
#81427=CARTESIAN_POINT('Ctrl Pts',(0.01200997138491,-0.033601104548885,
0.069910228948926));
#81428=CARTESIAN_POINT('Ctrl Pts',(0.0118882198118214,-0.0333736987606857,
0.0697986310249529));
#81429=CARTESIAN_POINT('Ctrl Pts',(0.0117602647433478,-0.0331450831799192,
0.0696942038128069));
#81430=CARTESIAN_POINT('Ctrl Pts',(0.0120838284046142,-0.0337436976235975,
0.0699790540338265));
#81431=CARTESIAN_POINT('Ctrl Pts',(0.0120463142844703,-0.0336723290703325,
0.0699434367780388));
#81432=CARTESIAN_POINT('Ctrl Pts',(0.0120081655910587,-0.033601104548885,
0.0699085000450632));
#81433=CARTESIAN_POINT('Ctrl Pts',(0.0118863643698258,-0.0333736987606857,
0.0697969539772491));
#81434=CARTESIAN_POINT('Ctrl Pts',(0.0117583627108295,-0.0331450831799192,
0.0696925813849042));
#81435=CARTESIAN_POINT('',(0.0120593369739985,-0.0336938721132548,0.069956012211914));
#81436=CARTESIAN_POINT('',(0.0118837058461226,-0.0333679869945434,0.0697978626947793));
#81437=CARTESIAN_POINT('Ctrl Pts',(0.0120593369740092,-0.0336938721132648,
0.0699560122119234));
#81438=CARTESIAN_POINT('Ctrl Pts',(0.0120429658722373,-0.0336629187933931,
0.0699406498954123));
#81439=CARTESIAN_POINT('Ctrl Pts',(0.0120265100537939,-0.0336319952301039,
0.0699253883515189));
#81440=CARTESIAN_POINT('Ctrl Pts',(0.0120099713849204,-0.0336011045488949,
0.0699102289489357));
#81441=CARTESIAN_POINT('Ctrl Pts',(0.0119684702055025,-0.0335235892595452,
0.069872188820599));
#81442=CARTESIAN_POINT('Ctrl Pts',(0.0119263734892345,-0.0334458668660368,
0.0698347243718573));
#81443=CARTESIAN_POINT('Ctrl Pts',(0.0118837058463353,-0.0333679869945384,
0.0697978626945436));
#81444=CARTESIAN_POINT('Ctrl Pts',(0.0118836726444111,-0.0333679692459107,
0.0697978331022651));
#81445=CARTESIAN_POINT('Ctrl Pts',(0.0118833808434531,-0.0333391895375576,
0.069798179930783));
#81446=CARTESIAN_POINT('Ctrl Pts',(0.0118831646091521,-0.0333104081063368,
0.0697984419862041));
#81447=CARTESIAN_POINT('Ctrl Pts',(0.0118828826583311,-0.0332532698941694,
0.0697987923858657));
#81448=CARTESIAN_POINT('Ctrl Pts',(0.0118828147431512,-0.0332249174808968,
0.0697988832651797));
#81449=CARTESIAN_POINT('Ctrl Pts',(0.0118828175663909,-0.0331960985220354,
0.0697988905547451));
#81450=CARTESIAN_POINT('Ctrl Pts',(0.0118828176314533,-0.033195631270599,
0.0697988906502747));
#81451=CARTESIAN_POINT('Ctrl Pts',(0.0118828177156373,-0.0331951640388596,
0.0697988907230034));
#81452=CARTESIAN_POINT('',(0.0119774070477464,-0.0331951640388587,0.069880608886537));
#81453=CARTESIAN_POINT('',(0.0119301123817021,-0.0331951640388687,0.0698397498047804));
#81454=CARTESIAN_POINT('',(0.0121495594631661,-0.0335216366567703,0.0700425382086595));
#81455=CARTESIAN_POINT('Origin',(0.00138764190188798,-0.0326434571528776,
0.0827528409360664));
#81456=CARTESIAN_POINT('',(0.0121486085297355,-0.0336938721132327,0.0700435084366343));
#81457=CARTESIAN_POINT('Origin',(0.0197926776181876,-0.0336938867896162,
0.0622443393975074));
#81458=CARTESIAN_POINT('',(0.012103972751877,-0.0336938721132538,0.0699997603242842));
#81459=CARTESIAN_POINT('Ctrl Pts',(0.0124883315106566,-0.0335235895815172,
0.0700328760943192));
#81460=CARTESIAN_POINT('Ctrl Pts',(0.0124316511942238,-0.0334144449262749,
0.0699727894799563));
#81461=CARTESIAN_POINT('Ctrl Pts',(0.012373664414742,-0.0333049234473147,
0.069913804806034));
#81462=CARTESIAN_POINT('Ctrl Pts',(0.0123144384873313,-0.0331951640388587,
0.0698560042124231));
#81463=CARTESIAN_POINT('Ctrl Pts',(0.0123750689445051,-0.0335235895815172,
0.070036448711682));
#81464=CARTESIAN_POINT('Ctrl Pts',(0.0123184378121842,-0.0334144449262749,
0.0699779213795356));
#81465=CARTESIAN_POINT('Ctrl Pts',(0.0122605324869179,-0.0333049234473147,
0.0699204967631495));
#81466=CARTESIAN_POINT('Ctrl Pts',(0.0122014203603723,-0.0331951640388587,
0.0698642549981249));
#81467=CARTESIAN_POINT('Ctrl Pts',(0.0122618063783537,-0.0335235895815173,
0.0700400213290447));
#81468=CARTESIAN_POINT('Ctrl Pts',(0.0122052244301446,-0.0334144449262749,
0.0699830532791149));
#81469=CARTESIAN_POINT('Ctrl Pts',(0.0121474005590938,-0.0333049234473147,
0.0699271887202649));
#81470=CARTESIAN_POINT('Ctrl Pts',(0.0120884022334132,-0.0331951640388587,
0.0698725057838268));
#81471=CARTESIAN_POINT('Ctrl Pts',(0.0121485438122022,-0.0335235895815173,
0.0700435939464075));
#81472=CARTESIAN_POINT('Ctrl Pts',(0.012092011048105,-0.0334144449262749,
0.0699881851786942));
#81473=CARTESIAN_POINT('Ctrl Pts',(0.0120342686312697,-0.0333049234473147,
0.0699338806773804));
#81474=CARTESIAN_POINT('Ctrl Pts',(0.0119753841064541,-0.0331951640388587,
0.0698807565695286));
#81475=CARTESIAN_POINT('',(0.0121459227675475,-0.0331951640388687,0.0698683065494902));
#81476=CARTESIAN_POINT('Ctrl Pts',(0.0123236009756333,-0.0332121607145988,
0.0698649653287758));
#81477=CARTESIAN_POINT('Ctrl Pts',(0.0122935647852482,-0.0332625444109243,
0.0698956109646606));
#81478=CARTESIAN_POINT('Ctrl Pts',(0.0122640461655568,-0.0333135300745759,
0.0699257285281495));
#81479=CARTESIAN_POINT('Ctrl Pts',(0.0122060206359464,-0.0334167203140609,
0.0699849314173864));
#81480=CARTESIAN_POINT('Ctrl Pts',(0.012177536199884,-0.0334688847587289,
0.0700139938132749));
#81481=CARTESIAN_POINT('Ctrl Pts',(0.0121495594625472,-0.0335216366562355,
0.0700425382090413));
#81482=CARTESIAN_POINT('Ctrl Pts',(0.0120593470153702,-0.033693872113239,
0.0699570120189169));
#81483=CARTESIAN_POINT('Ctrl Pts',(0.012034804065336,-0.0336474569764958,
0.0699339758520533));
#81484=CARTESIAN_POINT('Ctrl Pts',(0.0120099931295819,-0.033601104548885,
0.0699112285698606));
#81485=CARTESIAN_POINT('Ctrl Pts',(0.0119471775446443,-0.0334837508592656,
0.0698536376812768));
#81486=CARTESIAN_POINT('Ctrl Pts',(0.0118826830062478,-0.0333660264659097,
0.0697979334383868));
#81487=CARTESIAN_POINT('Ctrl Pts',(0.0120593369740134,-0.0336938721132391,
0.0699560122119281));
#81488=CARTESIAN_POINT('Ctrl Pts',(0.0120347881717771,-0.0336474569764958,
0.0699329761038399));
#81489=CARTESIAN_POINT('Ctrl Pts',(0.01200997138491,-0.033601104548885,
0.069910228948926));
#81490=CARTESIAN_POINT('Ctrl Pts',(0.0119471409862994,-0.0334837508592656,
0.0698526383825828));
#81491=CARTESIAN_POINT('Ctrl Pts',(0.0118826316502837,-0.0333660264659097,
0.0697969349007517));
#81492=CARTESIAN_POINT('Ctrl Pts',(0.0120559228683337,-0.0336938721132391,
0.0696160734186727));
#81493=CARTESIAN_POINT('Ctrl Pts',(0.0120293842915368,-0.0336474569764958,
0.0695930572944779));
#81494=CARTESIAN_POINT('Ctrl Pts',(0.0120025781003864,-0.033601104548885,
0.0695703534149116));
#81495=CARTESIAN_POINT('Ctrl Pts',(0.0119347109875234,-0.0334837508592656,
0.0695128724117991));
#81496=CARTESIAN_POINT('Ctrl Pts',(0.0118651703955946,-0.0333660264659097,
0.0694574276933728));
#81497=CARTESIAN_POINT('',(0.0120462540427042,-0.0336769361243753,0.0696097120587865));
#81498=CARTESIAN_POINT('',(0.0120559432307895,-0.0336938721132327,0.0696181008866323));
#81499=CARTESIAN_POINT('Ctrl Pts',(0.0120462540427042,-0.0336769361243753,
0.0696097120587865));
#81500=CARTESIAN_POINT('Ctrl Pts',(0.0120478705216501,-0.033679758666993,
0.069611108576638));
#81501=CARTESIAN_POINT('Ctrl Pts',(0.0120494861936565,-0.0336825812712652,
0.0696125059049446));
#81502=CARTESIAN_POINT('Ctrl Pts',(0.0120527159254343,-0.0336882266053286,
0.0696153021832117));
#81503=CARTESIAN_POINT('Ctrl Pts',(0.0120543299851789,-0.0336910493350804,
0.069616701133161));
#81504=CARTESIAN_POINT('Ctrl Pts',(0.0120559432307888,-0.0336938721132314,
0.0696181008866358));
#81505=CARTESIAN_POINT('Ctrl Pts',(0.0120462540427042,-0.0336769361243754,
0.0696097120587866));
#81506=CARTESIAN_POINT('Ctrl Pts',(0.0120188537291051,-0.0336279018378417,
0.0696414281088157));
#81507=CARTESIAN_POINT('Ctrl Pts',(0.0119910592276754,-0.0335767825754279,
0.0696736004339502));
#81508=CARTESIAN_POINT('Ctrl Pts',(0.0119365979875693,-0.0334733171799195,
0.0697366396911326));
#81509=CARTESIAN_POINT('Ctrl Pts',(0.0119098946462121,-0.0334209631321942,
0.0697675489910333));
#81510=CARTESIAN_POINT('Ctrl Pts',(0.0118837058516271,-0.033367986984468,
0.0697978626995336));
#81511=CARTESIAN_POINT('',(0.012057640102404,-0.0336938721132538,0.0697870565492832));
#81512=CARTESIAN_POINT('Origin',(0.00812378219310841,-0.0315241814719618,
0.07415));
#81513=CARTESIAN_POINT('',(0.0120462540418611,-0.0337108120655557,0.0696097120597726));
#81514=CARTESIAN_POINT('',(0.0120365469580377,-0.0336938721132327,0.0696013439463572));
#81515=CARTESIAN_POINT('Origin',(0.000504479743886488,-0.034556252137451,
0.0812598512727581));
#81516=CARTESIAN_POINT('Ctrl Pts',(0.0120365469580457,-0.0336938721132359,
0.0696013439463543));
#81517=CARTESIAN_POINT('Ctrl Pts',(0.0120381661841294,-0.0336910493082178,
0.0696027368084859));
#81518=CARTESIAN_POINT('Ctrl Pts',(0.01203978471031,-0.0336882265918966,
0.0696041305729465));
#81519=CARTESIAN_POINT('Ctrl Pts',(0.0120430204001186,-0.0336825812713121,
0.06960691993915));
#81520=CARTESIAN_POINT('Ctrl Pts',(0.012044637563745,-0.0336797586670163,
0.0696083155409235));
#81521=CARTESIAN_POINT('Ctrl Pts',(0.0120462540427044,-0.033676936124375,
0.0696097120587867));
#81522=CARTESIAN_POINT('Origin',(0.00219589820400869,-0.0345562520449254,
0.0827211093173939));
#81523=CARTESIAN_POINT('Ctrl Pts',(0.0120041862394658,-0.0342436276873911,
0.0699049335179514));
#81524=CARTESIAN_POINT('Ctrl Pts',(0.0118440809177256,-0.0339430054201811,
0.0697585816667022));
#81525=CARTESIAN_POINT('Ctrl Pts',(0.0116734066173258,-0.0336441434784053,
0.0696247053745641));
#81526=CARTESIAN_POINT('Ctrl Pts',(0.0118160393691582,-0.0342436276873911,
0.0697403104478991));
#81527=CARTESIAN_POINT('Ctrl Pts',(0.0116497251859766,-0.0339430054201811,
0.0696010546728438));
#81528=CARTESIAN_POINT('Ctrl Pts',(0.011473394168394,-0.0336441434784053,
0.069474721974575));
#81529=CARTESIAN_POINT('Ctrl Pts',(0.0118141579004551,-0.0342436276873911,
0.0697386642171985));
#81530=CARTESIAN_POINT('Ctrl Pts',(0.0116477816286591,-0.0339430054201811,
0.0695994794029052));
#81531=CARTESIAN_POINT('Ctrl Pts',(0.0114713940439047,-0.0336441434784053,
0.069473222140575));
#81532=CARTESIAN_POINT('',(0.0117882283835291,-0.0341934961088741,0.0697171725594705));
#81533=CARTESIAN_POINT('',(0.011603013537796,-0.0338664212864857,0.0695703630870027));
#81534=CARTESIAN_POINT('Origin',(0.000737920614214256,-0.0345610720403814,
0.0822847436040769));
#81535=CARTESIAN_POINT('Origin',(0.0182369173441908,-0.0336938005072859,
0.0608382359259433));
#81536=CARTESIAN_POINT('',(0.0117017255132845,-0.0336938721132327,0.069647062447956));
#81537=CARTESIAN_POINT('',(0.0116519586094886,-0.0336938721132427,0.0696092536489164));
#81538=CARTESIAN_POINT('',(0.0118837058516312,-0.0340203938281605,0.069797862699537));
#81539=CARTESIAN_POINT('Origin',(0.000429862642817593,-0.0345589643244208,
0.0819150991526489));
#81540=CARTESIAN_POINT('',(0.0118828177156378,-0.034193496108874,0.0697988907230037));
#81541=CARTESIAN_POINT('Origin',(0.0190867304027485,-0.0341934220717863,
0.0614603140868351));
#81542=CARTESIAN_POINT('',(0.0118355230495935,-0.0341934961088841,0.0697580316412471));
#81543=CARTESIAN_POINT('Ctrl Pts',(0.0122212047193902,-0.0340223579322397,
0.0697669498472922));
#81544=CARTESIAN_POINT('Ctrl Pts',(0.0121607510263096,-0.0339125849573575,
0.0697104357041282));
#81545=CARTESIAN_POINT('Ctrl Pts',(0.0120991701018965,-0.0338030433565231,
0.0696552125237701));
#81546=CARTESIAN_POINT('Ctrl Pts',(0.0120365469580398,-0.0336938721132326,
0.0696013439463569));
#81547=CARTESIAN_POINT('Ctrl Pts',(0.0121083899404104,-0.0340223579322397,
0.0697776271818883));
#81548=CARTESIAN_POINT('Ctrl Pts',(0.0120480835156215,-0.0339125849573575,
0.0697226690487597));
#81549=CARTESIAN_POINT('Ctrl Pts',(0.0119866819618085,-0.0338030433565231,
0.0696689977369353));
#81550=CARTESIAN_POINT('Ctrl Pts',(0.011924269885551,-0.0336938721132326,
0.06961667492231));
#81551=CARTESIAN_POINT('Ctrl Pts',(0.0119955751614305,-0.0340223579322397,
0.0697883045164844));
#81552=CARTESIAN_POINT('Ctrl Pts',(0.0119354160049335,-0.0339125849573575,
0.0697349023933912));
#81553=CARTESIAN_POINT('Ctrl Pts',(0.0118741938217205,-0.0338030433565231,
0.0696827829501006));
#81554=CARTESIAN_POINT('Ctrl Pts',(0.0118119928130621,-0.0336938721132326,
0.0696320058982631));
#81555=CARTESIAN_POINT('Ctrl Pts',(0.0118827603824507,-0.0340223579322397,
0.0697989818510805));
#81556=CARTESIAN_POINT('Ctrl Pts',(0.0118227484942454,-0.0339125849573575,
0.0697471357380227));
#81557=CARTESIAN_POINT('Ctrl Pts',(0.0117617056816325,-0.0338030433565231,
0.0696965681632658));
#81558=CARTESIAN_POINT('Ctrl Pts',(0.0116997157405733,-0.0336938721132326,
0.0696473368742162));
#81559=CARTESIAN_POINT('',(0.0118691362356711,-0.0336938721132427,0.0696242031971666));
#81560=CARTESIAN_POINT('Ctrl Pts',(0.0120462540395,-0.0337108120662705,
0.0696097120624956));
#81561=CARTESIAN_POINT('Ctrl Pts',(0.0120181434775496,-0.033761140899387,
0.0696422502298396));
#81562=CARTESIAN_POINT('Ctrl Pts',(0.0119905458709879,-0.0338121088780417,
0.0696741946478196));
#81563=CARTESIAN_POINT('Ctrl Pts',(0.0119363514275711,-0.0339153382773249,
0.0697369250860129));
#81564=CARTESIAN_POINT('Ctrl Pts',(0.0119097775183549,-0.0339675558473121,
0.0697676845673276));
#81565=CARTESIAN_POINT('Ctrl Pts',(0.0118837058516012,-0.0340203938281304,
0.0697978626995637));
#81566=CARTESIAN_POINT('Ctrl Pts',(0.0117883760535999,-0.0341934961088741,
0.0697191953237756));
#81567=CARTESIAN_POINT('Ctrl Pts',(0.0116967726575594,-0.0340287516182428,
0.0696434327327204));
#81568=CARTESIAN_POINT('Ctrl Pts',(0.0116021162095027,-0.0338644633275951,
0.0695715209172042));
#81569=CARTESIAN_POINT('Ctrl Pts',(0.0117882283835291,-0.0341934961088741,
0.0697171725594706));
#81570=CARTESIAN_POINT('Ctrl Pts',(0.0116965831684302,-0.0340287516182428,
0.0696414130213777));
#81571=CARTESIAN_POINT('Ctrl Pts',(0.0116018850632298,-0.0338644633275951,
0.0695695059846287));
#81572=CARTESIAN_POINT('Ctrl Pts',(0.0117636237094156,-0.0341934961088741,
0.0693801411198898));
#81573=CARTESIAN_POINT('Ctrl Pts',(0.0116650106348207,-0.0340287516182428,
0.0693048902640504));
#81574=CARTESIAN_POINT('Ctrl Pts',(0.0115633716482505,-0.0338644633275951,
0.0692337794618147));
#81575=CARTESIAN_POINT('',(0.011753426902075,-0.0341764758832406,0.0693723772357672));
#81576=CARTESIAN_POINT('',(0.0117636237094156,-0.034193496108874,0.0693801411198898));
#81577=CARTESIAN_POINT('Origin',(0.00132919932341822,-0.0345621026952721,
0.0822470348610732));
#81578=CARTESIAN_POINT('Ctrl Pts',(0.011753426902822,-0.0341764758837503,
0.0693723772374202));
#81579=CARTESIAN_POINT('Ctrl Pts',(0.0117274602070376,-0.0341260050040526,
0.0694065566597228));
#81580=CARTESIAN_POINT('Ctrl Pts',(0.0117019449041078,-0.0340749269148332,
0.0694401419861458));
#81581=CARTESIAN_POINT('Ctrl Pts',(0.0116517971633035,-0.0339715436306987,
0.069506150365217));
#81582=CARTESIAN_POINT('Ctrl Pts',(0.0116271837455901,-0.033919277823838,
0.0695385483721489));
#81583=CARTESIAN_POINT('Ctrl Pts',(0.0116030135399985,-0.0338664212855889,
0.069570363087186));
#81584=CARTESIAN_POINT('',(0.0117759260464824,-0.0341934961088841,0.0695486568396901));
#81585=CARTESIAN_POINT('Origin',(0.00812378219310841,-0.0315241814719618,
0.07415));
#81586=CARTESIAN_POINT('',(0.0117534269009585,-0.0342105180190554,0.0693723772358458));
#81587=CARTESIAN_POINT('',(0.0117432135337919,-0.0341934961088739,0.0693646351476515));
#81588=CARTESIAN_POINT('Origin',(0.00136188502771765,-0.0345621713746481,
0.0822784370868789));
#81589=CARTESIAN_POINT('Origin',(0.00214473761887886,-0.034562103232909,
0.082866615634891));
#81590=CARTESIAN_POINT('Origin',(0.00210572411884494,-0.0345621720636347,
0.082843542882067));
#81591=CARTESIAN_POINT('Ctrl Pts',(0.0117029199268719,-0.0346945769586965,
0.0696479698651322));
#81592=CARTESIAN_POINT('Ctrl Pts',(0.0116086231031826,-0.0345275153362944,
0.06957300339229));
#81593=CARTESIAN_POINT('Ctrl Pts',(0.0115119442629357,-0.0343603235965186,
0.0695009830775888));
#81594=CARTESIAN_POINT('Ctrl Pts',(0.0114131725050209,-0.034193496108874,
0.0694321176754391));
#81595=CARTESIAN_POINT('Ctrl Pts',(0.0116361659168294,-0.0346945769586965,
0.0695972556603406));
#81596=CARTESIAN_POINT('Ctrl Pts',(0.0115408068638159,-0.0345275153362944,
0.0695236873769656));
#81597=CARTESIAN_POINT('Ctrl Pts',(0.0114431094912697,-0.0343603235965186,
0.0694530990195095));
#81598=CARTESIAN_POINT('Ctrl Pts',(0.0113433658475022,-0.034193496108874,
0.0693856950625174));
#81599=CARTESIAN_POINT('Ctrl Pts',(0.0115694119067865,-0.0346945769586965,
0.0695465414555489));
#81600=CARTESIAN_POINT('Ctrl Pts',(0.0114729906244489,-0.0345275153362944,
0.06947437136164));
#81601=CARTESIAN_POINT('Ctrl Pts',(0.0113742747196035,-0.0343603235965186,
0.069405214961429));
#81602=CARTESIAN_POINT('Ctrl Pts',(0.0112735591899837,-0.034193496108874,
0.0693392724495953));
#81603=CARTESIAN_POINT('Ctrl Pts',(0.0115026578967444,-0.0346945769586965,
0.0694958272507573));
#81604=CARTESIAN_POINT('Ctrl Pts',(0.0114051743850824,-0.0345275153362944,
0.0694250553463166));
#81605=CARTESIAN_POINT('Ctrl Pts',(0.0113054399479375,-0.0343603235965186,
0.0693573309033509));
#81606=CARTESIAN_POINT('Ctrl Pts',(0.011203752532465,-0.034193496108874,
0.0692928498366739));
#81607=CARTESIAN_POINT('',(0.0115026578980562,-0.0346945769586966,0.0694958272517541));
#81608=CARTESIAN_POINT('',(0.0113085902893507,-0.0343667727836511,0.0693609372115995));
#81609=CARTESIAN_POINT('Origin',(0.00177344996204906,-0.0345626474179267,
0.0832085862090796));
#81610=CARTESIAN_POINT('Origin',(0.0174287120583264,-0.0341934771024118,
0.0601579612037074));
#81611=CARTESIAN_POINT('',(0.0114119234711446,-0.034193496108874,0.0694312870466964));
#81612=CARTESIAN_POINT('',(0.0113598807368301,-0.034193496108884,0.0693966777444305));
#81613=CARTESIAN_POINT('',(0.0116030135390037,-0.0345211942962673,0.0695703630884519));
#81614=CARTESIAN_POINT('Origin',(0.00139260688655039,-0.0345625596123107,
0.0829150780159028));
#81615=CARTESIAN_POINT('',(0.0116021917056726,-0.0346945769586885,0.0695714448498568));
#81616=CARTESIAN_POINT('Origin',(0.0182949952110115,-0.0346945685853857,
0.0607618536886375));
#81617=CARTESIAN_POINT('',(0.0115524248018744,-0.0346945769587026,0.0695336360508154));
#81618=CARTESIAN_POINT('Ctrl Pts',(0.0119379046530404,-0.0345231616327842,
0.0695183188947568));
#81619=CARTESIAN_POINT('Ctrl Pts',(0.01187406344989,-0.0344132092796988,
0.0694657465865016));
#81620=CARTESIAN_POINT('Ctrl Pts',(0.0118091381239245,-0.0343032738558979,
0.0694144974956657));
#81621=CARTESIAN_POINT('Ctrl Pts',(0.011743213533793,-0.0341934961088739,
0.0693646351476512));
#81622=CARTESIAN_POINT('Ctrl Pts',(0.011825983116894,-0.0345231616327842,
0.0695360588464229));
#81623=CARTESIAN_POINT('Ctrl Pts',(0.0117623864340015,-0.0344132092796988,
0.0694850292189705));
#81624=CARTESIAN_POINT('Ctrl Pts',(0.0116977375248132,-0.0343032738558979,
0.0694353176716336));
#81625=CARTESIAN_POINT('Ctrl Pts',(0.0116321208434002,-0.0341934961088739,
0.0693869857691142));
#81626=CARTESIAN_POINT('Ctrl Pts',(0.0117140615807476,-0.0345231616327842,
0.069553798798089));
#81627=CARTESIAN_POINT('Ctrl Pts',(0.0116507094181129,-0.0344132092796988,
0.0695043118514394));
#81628=CARTESIAN_POINT('Ctrl Pts',(0.011586336925702,-0.0343032738558979,
0.0694561378476015));
#81629=CARTESIAN_POINT('Ctrl Pts',(0.0115210281530074,-0.0341934961088739,
0.0694093363905773));
#81630=CARTESIAN_POINT('Ctrl Pts',(0.0116021400446012,-0.0345231616327842,
0.0695715387497551));
#81631=CARTESIAN_POINT('Ctrl Pts',(0.0115390324022244,-0.0344132092796988,
0.0695235944839084));
#81632=CARTESIAN_POINT('Ctrl Pts',(0.0114749363265907,-0.0343032738558979,
0.0694769580235694));
#81633=CARTESIAN_POINT('Ctrl Pts',(0.0114099354626146,-0.0341934961088739,
0.0694316870120403));
#81634=CARTESIAN_POINT('',(0.0115775685024782,-0.0341934961088839,0.069397961097184));
#81635=CARTESIAN_POINT('Ctrl Pts',(0.0117534268988626,-0.034210518019541,
0.0693723772385932));
#81636=CARTESIAN_POINT('Ctrl Pts',(0.0117274310005431,-0.034261055624081,
0.0694065950768619));
#81637=CARTESIAN_POINT('Ctrl Pts',(0.0117019015851772,-0.034312218986911,
0.069440198893716));
#81638=CARTESIAN_POINT('Ctrl Pts',(0.0116517533416707,-0.0344158119695163,
0.0695062079411695));
#81639=CARTESIAN_POINT('Ctrl Pts',(0.0116271550246041,-0.0344681990450054,
0.0695385861734861));
#81640=CARTESIAN_POINT('Ctrl Pts',(0.0116030135389773,-0.0345211942962463,
0.0695703630884668));
#81641=CARTESIAN_POINT('Ctrl Pts',(0.0115029322199276,-0.0346945769586932,
0.0694978362599221));
#81642=CARTESIAN_POINT('Ctrl Pts',(0.0114067520264886,-0.0345296777079064,
0.0694279747242158));
#81643=CARTESIAN_POINT('Ctrl Pts',(0.0113077665763584,-0.0343648066255586,
0.0693621481000903));
#81644=CARTESIAN_POINT('Ctrl Pts',(0.0115026578980635,-0.0346945769586932,
0.0694958272517595));
#81645=CARTESIAN_POINT('Ctrl Pts',(0.0114064361698022,-0.0345296777079064,
0.0694259713874637));
#81646=CARTESIAN_POINT('Ctrl Pts',(0.0113074094547454,-0.0343648066255586,
0.0693601521465749));
#81647=CARTESIAN_POINT('Ctrl Pts',(0.0114569393964651,-0.0346945769586932,
0.0691610058070076));
#81648=CARTESIAN_POINT('Ctrl Pts',(0.0113537954717544,-0.0345296777079064,
0.0690920951403816));
#81649=CARTESIAN_POINT('Ctrl Pts',(0.0112478915410667,-0.0343648066255586,
0.0690275063902431));
#81650=CARTESIAN_POINT('',(0.0114462752119167,-0.0346775396664988,0.0691538975057157));
#81651=CARTESIAN_POINT('',(0.0114569393964623,-0.0346945769586886,0.0691610058070057));
#81652=CARTESIAN_POINT('Origin',(0.00238071619513352,-0.0345626617890403,
0.0830617564758974));
#81653=CARTESIAN_POINT('Ctrl Pts',(0.0114462752126745,-0.0346775396670097,
0.0691538975073658));
#81654=CARTESIAN_POINT('Ctrl Pts',(0.0114224871787978,-0.0346269749928753,
0.0691896680965144));
#81655=CARTESIAN_POINT('Ctrl Pts',(0.0113991219412728,-0.0345757902891938,
0.0692248029823673));
#81656=CARTESIAN_POINT('Ctrl Pts',(0.011353217672773,-0.0344721681090558,
0.0692938301876703));
#81657=CARTESIAN_POINT('Ctrl Pts',(0.0113306966337414,-0.0344197714293279,
0.0693276954420808));
#81658=CARTESIAN_POINT('Ctrl Pts',(0.0113085902900172,-0.0343667727834186,
0.069360937211672));
#81659=CARTESIAN_POINT('',(0.0114797986472692,-0.0346945769587026,0.0693284165293899));
#81660=CARTESIAN_POINT('Origin',(0.00812378219310841,-0.0315241814719618,
0.07415));
#81661=CARTESIAN_POINT('',(0.0114462752106478,-0.034711613648963,0.0691538975062894));
#81662=CARTESIAN_POINT('',(0.0114355958676054,-0.0346945769586885,0.0691468119977928));
#81663=CARTESIAN_POINT('Origin',(0.00241945019131871,-0.0345626692919776,
0.0830852695700954));
#81664=CARTESIAN_POINT('Origin',(0.00212638595541208,-0.0345626624076629,
0.0828926245201263));
#81665=CARTESIAN_POINT('Origin',(0.00208972466723691,-0.0345626700069096,
0.082865994882105));
#81666=CARTESIAN_POINT('Ctrl Pts',(0.011443569771881,-0.0352450361874068,
0.0694534296494727));
#81667=CARTESIAN_POINT('Ctrl Pts',(0.0112664357144761,-0.0349452760959493,
0.0693282218063741));
#81668=CARTESIAN_POINT('Ctrl Pts',(0.0110803737092312,-0.034644428984174,
0.0692167121275547));
#81669=CARTESIAN_POINT('Ctrl Pts',(0.0114414760628377,-0.0352450361874068,
0.0694520182645352));
#81670=CARTESIAN_POINT('Ctrl Pts',(0.0112642887741763,-0.0349452760959493,
0.0693268893869689));
#81671=CARTESIAN_POINT('Ctrl Pts',(0.0110781796369064,-0.034644428984174,
0.0692154624589451));
#81672=CARTESIAN_POINT('Ctrl Pts',(0.011234178137754,-0.0352450361874068,
0.069312277181614));
#81673=CARTESIAN_POINT('Ctrl Pts',(0.0110517204276667,-0.0349452760959493,
0.0691949666735857));
#81674=CARTESIAN_POINT('Ctrl Pts',(0.010860944753267,-0.034644428984174,
0.0690917328936418));
#81675=CARTESIAN_POINT('Ctrl Pts',(0.0112321051585031,-0.0352450361874068,
0.0693108797707847));
#81676=CARTESIAN_POINT('Ctrl Pts',(0.0110495947442016,-0.0349452760959493,
0.069193647446452));
#81677=CARTESIAN_POINT('Ctrl Pts',(0.0108587724044306,-0.034644428984174,
0.0690904955979887));
#81678=CARTESIAN_POINT('',(0.0112037811325199,-0.0351951634053335,0.0692928651618755));
#81679=CARTESIAN_POINT('',(0.0110015980579655,-0.0348678972925388,0.0691704115784557));
#81680=CARTESIAN_POINT('Origin',(0.00298610278410784,-0.0345636767883213,
0.0838830762270324));
#81681=CARTESIAN_POINT('Origin',(0.0165306241745782,-0.0346946199340667,
0.0596033399503948));
#81682=CARTESIAN_POINT('',(0.0111091446528959,-0.0346945769330288,0.069234134259183));
#81683=CARTESIAN_POINT('',(0.0110550314695942,-0.0346945769458128,0.0692028610361239));
#81684=CARTESIAN_POINT('',(0.0113085902897783,-0.0350221583435276,0.069360937212002));
#81685=CARTESIAN_POINT('Origin',(0.00255063873445146,-0.0345628458716655,
0.0836793252647309));
#81686=CARTESIAN_POINT('',(0.0113079078848194,-0.0351951360298761,0.0693619688205612));
#81687=CARTESIAN_POINT('Origin',(0.0174096517011827,-0.035195183836678,
0.0601866450520421));
#81688=CARTESIAN_POINT('',(0.0112037525339102,-0.0351951371328748,0.0692928498374955));
#81689=CARTESIAN_POINT('Ctrl Pts',(0.0116395519122222,-0.0350241211494342,
0.0692879671656622));
#81690=CARTESIAN_POINT('Ctrl Pts',(0.0115725794034403,-0.0349144232818962,
0.069239538879303));
#81691=CARTESIAN_POINT('Ctrl Pts',(0.0115045657610997,-0.0348045283579412,
0.0691924659758927));
#81692=CARTESIAN_POINT('Ctrl Pts',(0.011435595858339,-0.0346945769439158,
0.0691468119916587));
#81693=CARTESIAN_POINT('Ctrl Pts',(0.0115289651080124,-0.0350241211494342,
0.0693126997461491));
#81694=CARTESIAN_POINT('Ctrl Pts',(0.0114623332803859,-0.0349144232818962,
0.0692657947476756));
#81695=CARTESIAN_POINT('Ctrl Pts',(0.0113946920105639,-0.0348045283579412,
0.0692202390017892));
#81696=CARTESIAN_POINT('Ctrl Pts',(0.0113261257670373,-0.0346945769439158,
0.0691760940836826));
#81697=CARTESIAN_POINT('Ctrl Pts',(0.0114183783038026,-0.0350241211494342,
0.0693374323266359));
#81698=CARTESIAN_POINT('Ctrl Pts',(0.0113520871573316,-0.0349144232818962,
0.0692920506160481));
#81699=CARTESIAN_POINT('Ctrl Pts',(0.0112848182600282,-0.0348045283579412,
0.0692480120276857));
#81700=CARTESIAN_POINT('Ctrl Pts',(0.0112166556757357,-0.0346945769439157,
0.0692053761757064));
#81701=CARTESIAN_POINT('Ctrl Pts',(0.0113077914995927,-0.0350241211494342,
0.0693621649071228));
#81702=CARTESIAN_POINT('Ctrl Pts',(0.0112418410342772,-0.0349144232818962,
0.0693183064844206));
#81703=CARTESIAN_POINT('Ctrl Pts',(0.0111749445094924,-0.0348045283579412,
0.0692757850535821));
#81704=CARTESIAN_POINT('Ctrl Pts',(0.011107185584434,-0.0346945769439157,
0.0692346582677302));
#81705=CARTESIAN_POINT('',(0.0112723702605491,-0.0346945769458128,0.0691904731285738));
#81706=CARTESIAN_POINT('Ctrl Pts',(0.011446275208821,-0.034711613649282,
0.0691538975090242));
#81707=CARTESIAN_POINT('Ctrl Pts',(0.0114224966109672,-0.034762154653183,
0.0691896538857593));
#81708=CARTESIAN_POINT('Ctrl Pts',(0.0113991361051192,-0.0348133084096039,
0.069224781568769));
#81709=CARTESIAN_POINT('Ctrl Pts',(0.0113532317814142,-0.0349168561544586,
0.0692938088639129));
#81710=CARTESIAN_POINT('Ctrl Pts',(0.0113307061715391,-0.0349692089015924,
0.0693276810963227));
#81711=CARTESIAN_POINT('Ctrl Pts',(0.0113085902897415,-0.0350221583435,
0.0693609372120215));
#81712=CARTESIAN_POINT('Ctrl Pts',(0.0112040410946606,-0.0351951371254961,
0.0692942841152269));
#81713=CARTESIAN_POINT('Ctrl Pts',(0.01110365221532,-0.0350307338980954,
0.0692306016950558));
#81714=CARTESIAN_POINT('Ctrl Pts',(0.0110007170545465,-0.0348659306897802,
0.0691711228718443));
#81715=CARTESIAN_POINT('Ctrl Pts',(0.0112037525338538,-0.0351951371254961,
0.0692928498375973));
#81716=CARTESIAN_POINT('Ctrl Pts',(0.0111033340017231,-0.0350307338980954,
0.0692291733832398));
#81717=CARTESIAN_POINT('Ctrl Pts',(0.0110003694600711,-0.0348659306897802,
0.069169701746326));
#81718=CARTESIAN_POINT('Ctrl Pts',(0.0111553894418679,-0.0351951371254961,
0.0690524634119508));
#81719=CARTESIAN_POINT('Ctrl Pts',(0.0110500010712104,-0.0350307338980954,
0.0689897868341761));
#81720=CARTESIAN_POINT('Ctrl Pts',(0.0109421122637075,-0.0348659306897802,
0.0689315196282454));
#81721=CARTESIAN_POINT('Origin',(0.0136626645957855,-0.0308609197410717,
0.0645658723227696));
#81722=CARTESIAN_POINT('',(0.01118266731619,-0.0351951371254961,0.0691880467760055));
#81723=CARTESIAN_POINT('Origin',(0.00776259808483813,-0.0351840467441113,
0.0750579051108912));
#81724=CARTESIAN_POINT('Origin',(0.0134096467068773,-0.0352322613132216,
0.0634154466215648));
#81725=CARTESIAN_POINT('',(0.0107942927752421,-0.035195114256467,0.0690562599384998));
#81726=CARTESIAN_POINT('',(0.0106826437780381,-0.0351951372916787,0.0690007546777055));
#81727=CARTESIAN_POINT('Origin',(0.00778461305072263,-0.0352875117104394,
0.0741807531841194));
#81728=CARTESIAN_POINT('Origin',(0.0140792769102759,-0.0298325076522913,
0.0787136907162318));
#81729=CARTESIAN_POINT('Origin',(0.0144049968005323,-0.0338731295099351,
0.0686001892186881));
#81730=CARTESIAN_POINT('Ctrl Pts',(0.0132784795555664,-0.0321934096636942,
0.0715990725516433));
#81731=CARTESIAN_POINT('Ctrl Pts',(0.0132328191690395,-0.032050846084523,
0.0715068059236173));
#81732=CARTESIAN_POINT('Ctrl Pts',(0.0131847141883583,-0.0319086045664877,
0.0714158356694231));
#81733=CARTESIAN_POINT('Ctrl Pts',(0.013134284317649,-0.0317669892870596,
0.0713263491367977));
#81734=CARTESIAN_POINT('Ctrl Pts',(0.0132396651423412,-0.0321934096636942,
0.0715247497828995));
#81735=CARTESIAN_POINT('Ctrl Pts',(0.0131926744136476,-0.032050846084523,
0.0714331779143863));
#81736=CARTESIAN_POINT('Ctrl Pts',(0.0131432587606993,-0.0319086045664877,
0.0713429376395227));
#81737=CARTESIAN_POINT('Ctrl Pts',(0.0130915405803324,-0.0317669892870596,
0.0712542145019387));
#81738=CARTESIAN_POINT('Ctrl Pts',(0.0132008507291159,-0.0321934096636942,
0.0714504270141559));
#81739=CARTESIAN_POINT('Ctrl Pts',(0.0131525296582558,-0.032050846084523,
0.0713595499051552));
#81740=CARTESIAN_POINT('Ctrl Pts',(0.0131018033330405,-0.0319086045664877,
0.0712700396096223));
#81741=CARTESIAN_POINT('Ctrl Pts',(0.0130487968430159,-0.0317669892870596,
0.0711820798670797));
#81742=CARTESIAN_POINT('Ctrl Pts',(0.0131620363158906,-0.0321934096636942,
0.0713761042454123));
#81743=CARTESIAN_POINT('Ctrl Pts',(0.0131123849028638,-0.032050846084523,
0.0712859218959241));
#81744=CARTESIAN_POINT('Ctrl Pts',(0.0130603479053815,-0.0319086045664877,
0.0711971415797219));
#81745=CARTESIAN_POINT('Ctrl Pts',(0.0130060531056993,-0.0317669892870596,
0.0711099452322206));
#81746=CARTESIAN_POINT('',(0.0131627307134113,-0.0321934096636942,0.0713774338944332));
#81747=CARTESIAN_POINT('',(0.0130445664762117,-0.0318665617511322,0.0711727517691103));
#81748=CARTESIAN_POINT('Origin',(-0.00176379806423547,-0.0326371944423759,
0.0788885352453787));
#81749=CARTESIAN_POINT('Origin',(0.0224228080824538,-0.0316939261509285,
0.0654985844740454));
#81750=CARTESIAN_POINT('',(0.013221635807231,-0.0320197221621834,0.0714873926884516));
#81751=CARTESIAN_POINT('Ctrl Pts',(0.0132215948274271,-0.0320197392094745,
0.0714872123123591));
#81752=CARTESIAN_POINT('Ctrl Pts',(0.0132080456660022,-0.0319792716576044,
0.0714612730245034));
#81753=CARTESIAN_POINT('Ctrl Pts',(0.0131942370729477,-0.0319386439829733,
0.0714353189444909));
#81754=CARTESIAN_POINT('Ctrl Pts',(0.0131801470853275,-0.0318979099381666,
0.0714093267979314));
#81755=CARTESIAN_POINT('Ctrl Pts',(0.0131660573762056,-0.0318571766984964,
0.0713833351651248));
#81756=CARTESIAN_POINT('Ctrl Pts',(0.0131517594630909,-0.0318163871833608,
0.0713574367246318));
#81757=CARTESIAN_POINT('Ctrl Pts',(0.0131373056074969,-0.0317755399638303,
0.0713317188545931));
#81758=CARTESIAN_POINT('',(0.0132205951878513,-0.0321934096636183,0.0714882341769757));
#81759=CARTESIAN_POINT('Origin',(0.0152562378528542,-0.0324111610893099,
0.0704014176396957));
#81760=CARTESIAN_POINT('',(0.0131916629506413,-0.0321934096636663,0.0714328340357144));
#81761=CARTESIAN_POINT('Ctrl Pts',(0.0131621233618727,-0.0321934096636618,
0.0713793690459745));
#81762=CARTESIAN_POINT('Ctrl Pts',(0.0131239142017133,-0.0320835708272592,
0.0713098863946038));
#81763=CARTESIAN_POINT('Ctrl Pts',(0.0130842892645605,-0.0319739230346488,
0.0712412347825782));
#81764=CARTESIAN_POINT('Ctrl Pts',(0.0130433059888615,-0.0318646057455572,
0.071173498153992));
#81765=CARTESIAN_POINT('Ctrl Pts',(0.0131960567125676,-0.0321934096636618,
0.0712712501647596));
#81766=CARTESIAN_POINT('Ctrl Pts',(0.0131563565087732,-0.0320835708272592,
0.0712012995460367));
#81767=CARTESIAN_POINT('Ctrl Pts',(0.0131152317082915,-0.0319739230346488,
0.0711322110951696));
#81768=CARTESIAN_POINT('Ctrl Pts',(0.0130727417114348,-0.0318646057455572,
0.0710640691678818));
#81769=CARTESIAN_POINT('Ctrl Pts',(0.0132299900632624,-0.0321934096636618,
0.0711631312835448));
#81770=CARTESIAN_POINT('Ctrl Pts',(0.0131887988158331,-0.0320835708272592,
0.0710927126974697));
#81771=CARTESIAN_POINT('Ctrl Pts',(0.0131461741520224,-0.0319739230346488,
0.0710231874077611));
#81772=CARTESIAN_POINT('Ctrl Pts',(0.013102177434008,-0.0318646057455572,
0.0709546401817716));
#81773=CARTESIAN_POINT('Ctrl Pts',(0.0132639234139572,-0.0321934096636618,
0.07105501240233));
#81774=CARTESIAN_POINT('Ctrl Pts',(0.013221241122893,-0.0320835708272592,
0.0709841258489027));
#81775=CARTESIAN_POINT('Ctrl Pts',(0.0131771165957533,-0.0319739230346488,
0.0709141637203525));
#81776=CARTESIAN_POINT('Ctrl Pts',(0.0131316131565813,-0.0318646057455572,
0.0708452111956613));
#81777=CARTESIAN_POINT('',(0.013257300737261,-0.0321763980308463,0.0710440400301001));
#81778=CARTESIAN_POINT('',(0.0132639234139403,-0.0321934096636184,0.071055012402302));
#81779=CARTESIAN_POINT('Origin',(-0.00120853150640208,-0.0326386231565666,
0.0790793241204305));
#81780=CARTESIAN_POINT('Ctrl Pts',(0.0132573007345385,-0.0321763980306274,
0.0710440400317385));
#81781=CARTESIAN_POINT('Ctrl Pts',(0.0132205799120103,-0.0321259596174894,
0.0710662574258813));
#81782=CARTESIAN_POINT('Ctrl Pts',(0.0131844953253848,-0.0320749164631545,
0.0710880898748471));
#81783=CARTESIAN_POINT('Ctrl Pts',(0.0131135695842014,-0.0319716057793966,
0.0711310024524596));
#81784=CARTESIAN_POINT('Ctrl Pts',(0.0130787560647087,-0.0319193786690175,
0.0711520658609163));
#81785=CARTESIAN_POINT('Ctrl Pts',(0.013044566474618,-0.0318665617525371,
0.0711727517700634));
#81786=CARTESIAN_POINT('',(0.0132133270636858,-0.0321934096636663,0.0712162231483776));
#81787=CARTESIAN_POINT('Origin',(0.00812378219310841,-0.0315241814719618,
0.07415));
#81788=CARTESIAN_POINT('',(0.0132573007375785,-0.0322104233323779,0.0710440400299074));
#81789=CARTESIAN_POINT('',(0.0132506546416669,-0.0321934096636183,0.0710330818271523));
#81790=CARTESIAN_POINT('Origin',(-0.00119069648195176,-0.0326387240834481,
0.0791210015576047));
#81791=CARTESIAN_POINT('Origin',(-0.000573360558493453,-0.0326386239212449,
0.080129134790157));
#81792=CARTESIAN_POINT('Origin',(-0.000601999677916885,-0.0326387246941709,
0.0800939939734251));
#81793=CARTESIAN_POINT('Ctrl Pts',(0.013126047026358,-0.0327445246967098,
0.0713117837400871));
#81794=CARTESIAN_POINT('Ctrl Pts',(0.0130190019501655,-0.0324436878339361,
0.0711231202376705));
#81795=CARTESIAN_POINT('Ctrl Pts',(0.0128980500716496,-0.0321434074405927,
0.0709430557809763));
#81796=CARTESIAN_POINT('Ctrl Pts',(0.0129979788045448,-0.0327445246967098,
0.0710970780565069));
#81797=CARTESIAN_POINT('Ctrl Pts',(0.0128828359711157,-0.0324436878339361,
0.0709132447260388));
#81798=CARTESIAN_POINT('Ctrl Pts',(0.0127541731685286,-0.0321434074405927,
0.0707386066754554));
#81799=CARTESIAN_POINT('',(0.0129786966333756,-0.0326943950436612,0.0710665067248839));
#81800=CARTESIAN_POINT('',(0.0128479134700578,-0.0323666188837389,0.0708696480862338));
#81801=CARTESIAN_POINT('Origin',(-0.00117109338435085,-0.0326395579111445,
0.0801434831307089));
#81802=CARTESIAN_POINT('Origin',(0.0219198877202798,-0.0321933825602988,
0.0645702310453205));
#81803=CARTESIAN_POINT('',(0.0129180927342665,-0.0321934096532689,0.0709730971951112));
#81804=CARTESIAN_POINT('',(0.0128824451562546,-0.0321934096584275,0.0709217600689009));
#81805=CARTESIAN_POINT('',(0.0130445664770146,-0.0325210109756239,0.0711727517686187));
#81806=CARTESIAN_POINT('Origin',(-0.00140709529368095,-0.0326393129158039,
0.0797245708145731));
#81807=CARTESIAN_POINT('',(0.0130434041327693,-0.0326943950436595,0.0711734550279211));
#81808=CARTESIAN_POINT('Origin',(0.0225082911806531,-0.0326943765538162,
0.0654468653035667));
#81809=CARTESIAN_POINT('',(0.0130110503830824,-0.0326943950436703,0.0711199808764126));
#81810=CARTESIAN_POINT('Ctrl Pts',(0.0133750991772516,-0.032522978320377,
0.0712476440721177));
#81811=CARTESIAN_POINT('Ctrl Pts',(0.0133350902642561,-0.032413025309245,
0.07117525478233));
#81812=CARTESIAN_POINT('Ctrl Pts',(0.0132935899539462,-0.032303122220807,
0.0711037041075568));
#81813=CARTESIAN_POINT('Ctrl Pts',(0.0132506546393428,-0.0321934096576658,
0.0710330818233217));
#81814=CARTESIAN_POINT('Ctrl Pts',(0.0132645066272558,-0.032522978320377,
0.0712229371880149));
#81815=CARTESIAN_POINT('Ctrl Pts',(0.0132241571304032,-0.032413025309245,
0.0711520724141105));
#81816=CARTESIAN_POINT('Ctrl Pts',(0.013182347824462,-0.032303122220807,
0.0710820530694124));
#81817=CARTESIAN_POINT('Ctrl Pts',(0.0131391354290384,-0.0321934096576658,
0.0710129669539527));
#81818=CARTESIAN_POINT('Ctrl Pts',(0.01315391407726,-0.032522978320377,
0.0711982303039122));
#81819=CARTESIAN_POINT('Ctrl Pts',(0.0131132239965503,-0.032413025309245,
0.0711288900458909));
#81820=CARTESIAN_POINT('Ctrl Pts',(0.0130711056949777,-0.032303122220807,
0.071060402031268));
#81821=CARTESIAN_POINT('Ctrl Pts',(0.013027616218734,-0.0321934096576658,
0.0709928520845838));
#81822=CARTESIAN_POINT('Ctrl Pts',(0.0130433215272641,-0.032522978320377,
0.0711735234198095));
#81823=CARTESIAN_POINT('Ctrl Pts',(0.0130022908626975,-0.032413025309245,
0.0711057076776714));
#81824=CARTESIAN_POINT('Ctrl Pts',(0.0129598635654934,-0.032303122220807,
0.0710387509931235));
#81825=CARTESIAN_POINT('Ctrl Pts',(0.0129160970084296,-0.0321934096576658,
0.0709727372152148));
#81826=CARTESIAN_POINT('',(0.0130843736883616,-0.0321934096584275,0.0710030895114684));
#81827=CARTESIAN_POINT('Ctrl Pts',(0.0132573007345965,-0.0322104233328919,
0.0710440400317035));
#81828=CARTESIAN_POINT('Ctrl Pts',(0.0132205301548116,-0.0322609421830587,
0.0710662875307434));
#81829=CARTESIAN_POINT('Ctrl Pts',(0.0131844212609603,-0.032312088823912,
0.0710881346864311));
#81830=CARTESIAN_POINT('Ctrl Pts',(0.0131134949826744,-0.0324156524631815,
0.0711310475890096));
#81831=CARTESIAN_POINT('Ctrl Pts',(0.0130787067528211,-0.0324680267167321,
0.0711520956963494));
#81832=CARTESIAN_POINT('Ctrl Pts',(0.0130445664769752,-0.0325210109755913,
0.0711727517686373));
#81833=CARTESIAN_POINT('Origin',(0.011356292122591,-0.0262834582511563,
0.0813231628585625));
#81834=CARTESIAN_POINT('Origin',(0.0202428260747771,-0.0342770653632561,
0.0731747792278278));
#81835=CARTESIAN_POINT('Ctrl Pts',(0.0129782121070416,-0.0326943950436604,
0.0710684757157585));
#81836=CARTESIAN_POINT('Ctrl Pts',(0.0129357429270127,-0.0325844576448134,
0.0710015725733731));
#81837=CARTESIAN_POINT('Ctrl Pts',(0.0128918870747002,-0.0324744968375322,
0.0709355430284206));
#81838=CARTESIAN_POINT('Ctrl Pts',(0.0128467019076805,-0.0323646534831894,
0.0708704709067663));
#81839=CARTESIAN_POINT('Ctrl Pts',(0.013005289618094,-0.0326943950436604,
0.0709584396490503));
#81840=CARTESIAN_POINT('Ctrl Pts',(0.0129613039348363,-0.0325844576448134,
0.070891163327814));
#81841=CARTESIAN_POINT('Ctrl Pts',(0.0129159237540192,-0.0324744968375322,
0.0708247919413732));
#81842=CARTESIAN_POINT('Ctrl Pts',(0.0128692083923189,-0.0323646534831894,
0.0707594097266419));
#81843=CARTESIAN_POINT('Ctrl Pts',(0.0130323671291464,-0.0326943950436604,
0.0708484035823421));
#81844=CARTESIAN_POINT('Ctrl Pts',(0.0129868649426599,-0.0325844576448134,
0.0707807540822548));
#81845=CARTESIAN_POINT('Ctrl Pts',(0.0129399604333382,-0.0324744968375322,
0.0707140408543257));
#81846=CARTESIAN_POINT('Ctrl Pts',(0.0128917148769573,-0.0323646534831894,
0.0706483485465175));
#81847=CARTESIAN_POINT('Ctrl Pts',(0.0130594446401988,-0.0326943950436604,
0.0707383675156339));
#81848=CARTESIAN_POINT('Ctrl Pts',(0.0130124259504834,-0.0325844576448134,
0.0706703448366956));
#81849=CARTESIAN_POINT('Ctrl Pts',(0.0129639971126573,-0.0324744968375322,
0.0706032897672782));
#81850=CARTESIAN_POINT('Ctrl Pts',(0.0129142213615957,-0.0323646534831894,
0.0705372873663931));
#81851=CARTESIAN_POINT('',(0.0130521460710747,-0.0326773559991345,0.0707278326360949));
#81852=CARTESIAN_POINT('',(0.0130594446401983,-0.0326943950436595,0.0707383675156333));
#81853=CARTESIAN_POINT('Origin',(-0.000558563097022123,-0.0326395669463386,
0.0802400300320104));
#81854=CARTESIAN_POINT('Ctrl Pts',(0.0130521460683142,-0.0326773559987418,
0.0707278326380026));
#81855=CARTESIAN_POINT('Ctrl Pts',(0.0130168643781785,-0.032626792258602,
0.070752331609977));
#81856=CARTESIAN_POINT('Ctrl Pts',(0.0129822080305232,-0.0325756109579454,
0.0707763963553641));
#81857=CARTESIAN_POINT('Ctrl Pts',(0.012914116525888,-0.0324719985462361,
0.0708236778732658));
#81858=CARTESIAN_POINT('Ctrl Pts',(0.0128807086785635,-0.0324196091621767,
0.0708468756824462));
#81859=CARTESIAN_POINT('Ctrl Pts',(0.0128479134700177,-0.0323666188837756,
0.0708696480862616));
#81860=CARTESIAN_POINT('',(0.0130190706367969,-0.0326943950436703,0.0709024371202686));
#81861=CARTESIAN_POINT('Origin',(0.00812378219310841,-0.0315241814719618,
0.07415));
#81862=CARTESIAN_POINT('',(0.0130521460710381,-0.0327114338379869,0.0707278326361197));
#81863=CARTESIAN_POINT('',(0.0130448250186083,-0.0326943950436593,0.0707173133685686));
#81864=CARTESIAN_POINT('Origin',(-0.000532086577476713,-0.0326395676484836,
0.0802767990880925));
#81865=CARTESIAN_POINT('Origin',(-0.000615874592565635,-0.0326395675647529,
0.0801574963132246));
#81866=CARTESIAN_POINT('Origin',(-0.000641074086288608,-0.0326395682454631,
0.0801198404787709));
#81867=CARTESIAN_POINT('Ctrl Pts',(0.012937941665499,-0.0332451089994434,
0.0710032566716696));
#81868=CARTESIAN_POINT('Ctrl Pts',(0.0128192602991421,-0.0329451141710254,
0.070821687676544));
#81869=CARTESIAN_POINT('Ctrl Pts',(0.0126872395750486,-0.0326442513127493,
0.0706495740654579));
#81870=CARTESIAN_POINT('Ctrl Pts',(0.012796643269112,-0.0332451089994434,
0.0707970170945306));
#81871=CARTESIAN_POINT('Ctrl Pts',(0.0126701834498412,-0.0329451141710254,
0.0706207772556143));
#81872=CARTESIAN_POINT('Ctrl Pts',(0.012530807784429,-0.0326442513127493,
0.0704545635660392));
#81873=CARTESIAN_POINT('Ctrl Pts',(0.0127952302851482,-0.0332451089994434,
0.0707949546987592));
#81874=CARTESIAN_POINT('Ctrl Pts',(0.0126686926813482,-0.0329451141710254,
0.070618768151405));
#81875=CARTESIAN_POINT('Ctrl Pts',(0.0125292434665228,-0.0326442513127493,
0.070452613461045));
#81876=CARTESIAN_POINT('',(0.0127755024240173,-0.0331951640388616,0.07076774869453));
#81877=CARTESIAN_POINT('',(0.0126326164713081,-0.0328677532355019,0.0705794904395078));
#81878=CARTESIAN_POINT('Origin',(-0.000317427338547305,-0.0326402808280624,
0.0812371057761744));
#81879=CARTESIAN_POINT('Origin',(0.0212998163304004,-0.0326944278779125,
0.0637155244168665));
#81880=CARTESIAN_POINT('',(0.0127091528762318,-0.0326943950436593,0.0706783288320532));
#81881=CARTESIAN_POINT('',(0.0126703521572034,-0.0326943950436693,0.0706293313402693));
#81882=CARTESIAN_POINT('',(0.0128479134700594,-0.0330220786163545,0.0708696480862361));
#81883=CARTESIAN_POINT('Origin',(-0.000639895617482721,-0.0326396682763836,
0.0808805011570728));
#81884=CARTESIAN_POINT('',(0.012846797577453,-0.0331951640388588,0.0708704229420175));
#81885=CARTESIAN_POINT('Origin',(0.021908131514598,-0.0331952026560088,
0.0645783964944561));
#81886=CARTESIAN_POINT('',(0.0128111500007451,-0.0331951640388702,0.0708190858182837));
#81887=CARTESIAN_POINT('Ctrl Pts',(0.013182495949465,-0.0330240426238172,
0.0709236374767695));
#81888=CARTESIAN_POINT('Ctrl Pts',(0.0131380496624148,-0.032914277406352,
0.0708539487663096));
#81889=CARTESIAN_POINT('Ctrl Pts',(0.0130921405569585,-0.0328043479726691,
0.070785144142394));
#81890=CARTESIAN_POINT('Ctrl Pts',(0.0130448250186134,-0.0326943950436593,
0.0707173133685692));
#81891=CARTESIAN_POINT('Ctrl Pts',(0.0130705702949247,-0.0330240426238172,
0.0709059235319659));
#81892=CARTESIAN_POINT('Ctrl Pts',(0.0130258799810269,-0.032914277406352,
0.0708377767064413));
#81893=CARTESIAN_POINT('Ctrl Pts',(0.0129797586021355,-0.0328043479726691,
0.0707705197808633));
#81894=CARTESIAN_POINT('Ctrl Pts',(0.0129322628703094,-0.0326943950436593,
0.0707042405435509));
#81895=CARTESIAN_POINT('Ctrl Pts',(0.0129586446403843,-0.0330240426238172,
0.0708882095871624));
#81896=CARTESIAN_POINT('Ctrl Pts',(0.0129137102996391,-0.032914277406352,
0.0708216046465729));
#81897=CARTESIAN_POINT('Ctrl Pts',(0.0128673766473124,-0.0328043479726691,
0.0707558954193326));
#81898=CARTESIAN_POINT('Ctrl Pts',(0.0128197007220053,-0.0326943950436593,
0.0706911677185326));
#81899=CARTESIAN_POINT('Ctrl Pts',(0.012846718985844,-0.0330240426238172,
0.0708704956423588));
#81900=CARTESIAN_POINT('Ctrl Pts',(0.0128015406182512,-0.032914277406352,
0.0708054325867045));
#81901=CARTESIAN_POINT('Ctrl Pts',(0.0127549946924894,-0.0328043479726691,
0.0707412710578018));
#81902=CARTESIAN_POINT('Ctrl Pts',(0.0127071385737012,-0.0326943950436593,
0.0706780948935143));
#81903=CARTESIAN_POINT('',(0.01287698894743,-0.0326943950436694,0.0706978211003209));
#81904=CARTESIAN_POINT('Ctrl Pts',(0.0130521460683091,-0.0327114338383318,
0.0707278326380061));
#81905=CARTESIAN_POINT('Ctrl Pts',(0.013016870246718,-0.0327619876830289,
0.0707523275349686));
#81906=CARTESIAN_POINT('Ctrl Pts',(0.0129822167655523,-0.0328131562602937,
0.0707763902899169));
#81907=CARTESIAN_POINT('Ctrl Pts',(0.0129141253233661,-0.0329167375858772,
0.0708236717644552));
#81908=CARTESIAN_POINT('Ctrl Pts',(0.0128807144936195,-0.032969108892063,
0.0708468716445758));
#81909=CARTESIAN_POINT('Ctrl Pts',(0.0128479134700188,-0.0330220786163187,
0.0708696480862609));
#81910=CARTESIAN_POINT('Ctrl Pts',(0.0127751424302828,-0.0331951640388604,
0.0707697445422947));
#81911=CARTESIAN_POINT('Ctrl Pts',(0.0127052578159129,-0.0330306422010619,
0.0706735806515658));
#81912=CARTESIAN_POINT('Ctrl Pts',(0.0126314583627242,-0.0328657861914644,
0.0705803873368121));
#81913=CARTESIAN_POINT('Ctrl Pts',(0.0127755024240191,-0.0331951640388604,
0.0707677486945326));
#81914=CARTESIAN_POINT('Ctrl Pts',(0.0127055765467763,-0.0330306422010619,
0.070671577361164));
#81915=CARTESIAN_POINT('Ctrl Pts',(0.0126317355583615,-0.0328657861914644,
0.0705783783155682));
#81916=CARTESIAN_POINT('Ctrl Pts',(0.0128354870616681,-0.0331951640388604,
0.0704351867837546));
#81917=CARTESIAN_POINT('Ctrl Pts',(0.0127586856801389,-0.0330306422010619,
0.0703377753064612));
#81918=CARTESIAN_POINT('Ctrl Pts',(0.0126779238060552,-0.0328657861914644,
0.0702436213484575));
#81919=CARTESIAN_POINT('',(0.012827541405468,-0.0331781648281926,0.0704251309730369));
#81920=CARTESIAN_POINT('',(0.0128354870616674,-0.0331951640388588,0.0704351867837537));
#81921=CARTESIAN_POINT('Origin',(0.000328943744506286,-0.0326412092589798,
0.0812312191671869));
#81922=CARTESIAN_POINT('Ctrl Pts',(0.0128275414055619,-0.033178164828644,
0.0704251309748706));
#81923=CARTESIAN_POINT('Ctrl Pts',(0.0127938444634669,-0.0331276811546771,
0.070451815327297));
#81924=CARTESIAN_POINT('Ctrl Pts',(0.0127607560047859,-0.0330765663497773,
0.0704780178694669));
#81925=CARTESIAN_POINT('Ctrl Pts',(0.0126957675247983,-0.0329730614463247,
0.0705294817187533));
#81926=CARTESIAN_POINT('Ctrl Pts',(0.0126638937540996,-0.0329207133374092,
0.0705547222313894));
#81927=CARTESIAN_POINT('Ctrl Pts',(0.0126326164868155,-0.0328677532289375,
0.0705794904450544));
#81928=CARTESIAN_POINT('',(0.0128054947428523,-0.0331951640388702,0.0706014677391519));
#81929=CARTESIAN_POINT('Origin',(0.00812378219310841,-0.0315241814719618,
0.07415));
#81930=CARTESIAN_POINT('',(0.0128275414038497,-0.0332121607144228,0.0704251309734935));
#81931=CARTESIAN_POINT('',(0.0128195742877286,-0.0331951640388587,0.070415092155874));
#81932=CARTESIAN_POINT('Origin',(0.00036281909636309,-0.0326413659571202,
0.0812613627328244));
#81933=CARTESIAN_POINT('Origin',(-0.0005554229849607,-0.0326412097086312,
0.0801144440300772));
#81934=CARTESIAN_POINT('Origin',(-0.000576998278988514,-0.032641366643145,
0.0800745605478936));
#81935=CARTESIAN_POINT('Ctrl Pts',(0.0127100841162299,-0.0336938721132648,
0.0706795048005746));
#81936=CARTESIAN_POINT('Ctrl Pts',(0.0126374324053212,-0.0335278710435225,
0.0705834946745518));
#81937=CARTESIAN_POINT('Ctrl Pts',(0.0125617954005258,-0.0333620469224385,
0.0704897966634334));
#81938=CARTESIAN_POINT('Ctrl Pts',(0.0124831199004146,-0.0331951640388588,
0.0703983767496028));
#81939=CARTESIAN_POINT('Ctrl Pts',(0.0126580394108509,-0.0336938721132648,
0.0706137828220148));
#81940=CARTESIAN_POINT('Ctrl Pts',(0.0125840118691422,-0.0335278710435225,
0.0705188622053191));
#81941=CARTESIAN_POINT('Ctrl Pts',(0.0125070336842901,-0.0333620469224385,
0.0704262964659372));
#81942=CARTESIAN_POINT('Ctrl Pts',(0.0124270511761946,-0.0331951640388588,
0.0703360523724446));
#81943=CARTESIAN_POINT('Ctrl Pts',(0.0126059947054719,-0.0336938721132648,
0.070548060843455));
#81944=CARTESIAN_POINT('Ctrl Pts',(0.0125305913329632,-0.0335278710435225,
0.0704542297360864));
#81945=CARTESIAN_POINT('Ctrl Pts',(0.0124522719680544,-0.0333620469224385,
0.0703627962684409));
#81946=CARTESIAN_POINT('Ctrl Pts',(0.0123709824519747,-0.0331951640388588,
0.0702737279952865));
#81947=CARTESIAN_POINT('Ctrl Pts',(0.0125539500000929,-0.0336938721132648,
0.0704823388648952));
#81948=CARTESIAN_POINT('Ctrl Pts',(0.0124771707967842,-0.0335278710435225,
0.0703895972668538));
#81949=CARTESIAN_POINT('Ctrl Pts',(0.0123975102518187,-0.0333620469224385,
0.0702992960709447));
#81950=CARTESIAN_POINT('Ctrl Pts',(0.0123149137277548,-0.0331951640388588,
0.0702114036181283));
#81951=CARTESIAN_POINT('',(0.0125539500000679,-0.0336938721132548,0.0704823388648649));
#81952=CARTESIAN_POINT('',(0.0123995251928226,-0.0333679846208724,0.0703034239711086));
#81953=CARTESIAN_POINT('Ctrl Pts',(0.0125539500000827,-0.0336938721132391,
0.0704823388648661));
#81954=CARTESIAN_POINT('Ctrl Pts',(0.0125396333981384,-0.0336629187933924,
0.0704650458416958));
#81955=CARTESIAN_POINT('Ctrl Pts',(0.0125252201173784,-0.0336319952301063,
0.0704478421786947));
#81956=CARTESIAN_POINT('Ctrl Pts',(0.0124743055998606,-0.0335235892595475,
0.0703877878201039));
#81957=CARTESIAN_POINT('Ctrl Pts',(0.0124372363719196,-0.0334458668645783,
0.0703453426725633));
#81958=CARTESIAN_POINT('Ctrl Pts',(0.0123995251747037,-0.0333679869902226,
0.0703034239873527));
#81959=CARTESIAN_POINT('Ctrl Pts',(0.0123995257414162,-0.0333679128829522,
0.0703034234792778));
#81960=CARTESIAN_POINT('Ctrl Pts',(0.0123991887346561,-0.0333391359256882,
0.0703037266598301));
#81961=CARTESIAN_POINT('Ctrl Pts',(0.0123989361660613,-0.0333103578181722,
0.0703039538774858));
#81962=CARTESIAN_POINT('Ctrl Pts',(0.0123987678149064,-0.0332815781851602,
0.0703041053308148));
#81963=CARTESIAN_POINT('Ctrl Pts',(0.0123985993192564,-0.0332527738506924,
0.0703042569141356));
#81964=CARTESIAN_POINT('Ctrl Pts',(0.0123985151930517,-0.0332239691459984,
0.0703043325963891));
#81965=CARTESIAN_POINT('Ctrl Pts',(0.0123985151930517,-0.0331951640388606,
0.0703043325963891));
#81966=CARTESIAN_POINT('',(0.0124821166583467,-0.0331951640388587,0.0703972615746475));
#81967=CARTESIAN_POINT('',(0.0124403159257087,-0.0331951640388687,0.0703507970855277));
#81968=CARTESIAN_POINT('',(0.0126326164750483,-0.0335216366556738,0.0705794904543482));
#81969=CARTESIAN_POINT('Origin',(0.000362536508306777,-0.0326434571528194,
0.0818407427209279));
#81970=CARTESIAN_POINT('',(0.012631551438155,-0.0336938721132328,0.0705803338484653));
#81971=CARTESIAN_POINT('Origin',(0.0211928399800403,-0.0336938867896311,
0.0638007196656732));
#81972=CARTESIAN_POINT('',(0.0125927507191215,-0.0336938721132538,0.0705313363566751));
#81973=CARTESIAN_POINT('Ctrl Pts',(0.0129699281877454,-0.0335235895815172,
0.0706123639250602));
#81974=CARTESIAN_POINT('Ctrl Pts',(0.0129212256622093,-0.0334144449262749,
0.0705456471842605));
#81975=CARTESIAN_POINT('Ctrl Pts',(0.0128710888657169,-0.0333049234473147,
0.0704798599515335));
#81976=CARTESIAN_POINT('Ctrl Pts',(0.012819574287733,-0.0331951640388587,
0.0704150921558742));
#81977=CARTESIAN_POINT('Ctrl Pts',(0.0128571109630711,-0.0335235895815172,
0.0706017128076103));
#81978=CARTESIAN_POINT('Ctrl Pts',(0.0128082618039332,-0.0334144449262749,
0.070536549218025));
#81979=CARTESIAN_POINT('Ctrl Pts',(0.01275801029231,-0.0333049234473147,
0.0704723199502347));
#81980=CARTESIAN_POINT('Ctrl Pts',(0.01270641324481,-0.0331951640388587,
0.0704091129543632));
#81981=CARTESIAN_POINT('Ctrl Pts',(0.0127442937383968,-0.0335235895815172,
0.0705910616901604));
#81982=CARTESIAN_POINT('Ctrl Pts',(0.0126952979456571,-0.0334144449262749,
0.0705274512517894));
#81983=CARTESIAN_POINT('Ctrl Pts',(0.012644931718903,-0.0333049234473147,
0.0704647799489359));
#81984=CARTESIAN_POINT('Ctrl Pts',(0.012593252201887,-0.0331951640388587,
0.0704031337528521));
#81985=CARTESIAN_POINT('Ctrl Pts',(0.0126314765137225,-0.0335235895815172,
0.0705804105727106));
#81986=CARTESIAN_POINT('Ctrl Pts',(0.012582334087381,-0.0334144449262749,
0.0705183532855539));
#81987=CARTESIAN_POINT('Ctrl Pts',(0.0125318531454961,-0.0333049234473147,
0.0704572399476371));
#81988=CARTESIAN_POINT('Ctrl Pts',(0.0124800911589639,-0.0331951640388587,
0.0703971545513411));
#81989=CARTESIAN_POINT('',(0.0126508454730476,-0.0331951640388687,0.0704061768652707));
#81990=CARTESIAN_POINT('Ctrl Pts',(0.0128275414013884,-0.0332121607145979,
0.0704251309754337));
#81991=CARTESIAN_POINT('Ctrl Pts',(0.0127939011387833,-0.0332625444107923,
0.070451770428392));
#81992=CARTESIAN_POINT('Ctrl Pts',(0.0127608405506896,-0.0333135300743102,
0.0704779508417744));
#81993=CARTESIAN_POINT('Ctrl Pts',(0.0126958524803037,-0.0334167203135638,
0.070529414371183));
#81994=CARTESIAN_POINT('Ctrl Pts',(0.0126639501685649,-0.0334688847580745,
0.0705546775548508));
#81995=CARTESIAN_POINT('Ctrl Pts',(0.0126326164748062,-0.0335216366554488,
0.0705794904545209));
#81996=CARTESIAN_POINT('Ctrl Pts',(0.012553950000081,-0.0336938721132391,
0.0704823388648808));
#81997=CARTESIAN_POINT('Ctrl Pts',(0.0125324819623981,-0.0336474569764958,
0.0704564076226211));
#81998=CARTESIAN_POINT('Ctrl Pts',(0.0125107118377876,-0.033601104548885,
0.0704307294676731));
#81999=CARTESIAN_POINT('Ctrl Pts',(0.0124555948875392,-0.0334837508592656,
0.070365718283123));
#82000=CARTESIAN_POINT('Ctrl Pts',(0.0123985757244046,-0.0333660264659097,
0.070302368876206));
#82001=CARTESIAN_POINT('Ctrl Pts',(0.0125931684438169,-0.0336938721132391,
0.0701446526896404));
#82002=CARTESIAN_POINT('Ctrl Pts',(0.0125697238168942,-0.0336474569764958,
0.0701184918888154));
#82003=CARTESIAN_POINT('Ctrl Pts',(0.0125459745512081,-0.033601104548885,
0.0700926073295044));
#82004=CARTESIAN_POINT('Ctrl Pts',(0.0124858468707896,-0.0334837508592656,
0.0700270735765623));
#82005=CARTESIAN_POINT('Ctrl Pts',(0.0124238036930434,-0.0333660264659097,
0.0699633503090509));
#82006=CARTESIAN_POINT('',(0.0125843731495699,-0.0336769361243754,0.0701371296657961));
#82007=CARTESIAN_POINT('',(0.0125929345365934,-0.0336938721132327,0.070146666722502));
#82008=CARTESIAN_POINT('Ctrl Pts',(0.0125843731495697,-0.0336769361243751,
0.0701371296657959));
#82009=CARTESIAN_POINT('Ctrl Pts',(0.0125858018519977,-0.0336797586669916,
0.0701387177702196));
#82010=CARTESIAN_POINT('Ctrl Pts',(0.0125872296522721,-0.0336825812712627,
0.0701403065775715));
#82011=CARTESIAN_POINT('Ctrl Pts',(0.0125900834494012,-0.0336882266040365,
0.0701434855983503));
#82012=CARTESIAN_POINT('Ctrl Pts',(0.0125915094462306,-0.0336910493324964,
0.0701450758117581));
#82013=CARTESIAN_POINT('Ctrl Pts',(0.0125929345365926,-0.0336938721132319,
0.0701466667225041));
#82014=CARTESIAN_POINT('Ctrl Pts',(0.0125843731495699,-0.0336769361243754,
0.0701371296657961));
#82015=CARTESIAN_POINT('Ctrl Pts',(0.0125532146497868,-0.0336279031428258,
0.0701651607093637));
#82016=CARTESIAN_POINT('Ctrl Pts',(0.0125216078565492,-0.0335767852155843,
0.0701935950500561));
#82017=CARTESIAN_POINT('Ctrl Pts',(0.0124596750994393,-0.0334733199122746,
0.0702493114621073));
#82018=CARTESIAN_POINT('Ctrl Pts',(0.0124293075518341,-0.0334209645148378,
0.070276630943336));
#82019=CARTESIAN_POINT('Ctrl Pts',(0.0123995251713282,-0.0333679869844681,
0.0703034239921451));
#82020=CARTESIAN_POINT('',(0.0125734422683407,-0.0336938721132538,0.0703145027936935));
#82021=CARTESIAN_POINT('Origin',(0.00812378219310841,-0.0315241814719618,
0.07415));
#82022=CARTESIAN_POINT('',(0.012584373148611,-0.033710812065555,0.0701371296666677));
#82023=CARTESIAN_POINT('',(0.0125757914107549,-0.0336938721132327,0.070127610918123));
#82024=CARTESIAN_POINT('Origin',(-0.000326540335926023,-0.0345562521474037,
0.0802488360553175));
#82025=CARTESIAN_POINT('Ctrl Pts',(0.0125757914107646,-0.0336938721132364,
0.0701276109181209));
#82026=CARTESIAN_POINT('Ctrl Pts',(0.0125772232981681,-0.033691049305624,
0.070129195741416));
#82027=CARTESIAN_POINT('Ctrl Pts',(0.0125786543761196,-0.0336882265905996,
0.07013078137002));
#82028=CARTESIAN_POINT('Ctrl Pts',(0.0125815149506136,-0.0336825812712941,
0.0701339542799855));
#82029=CARTESIAN_POINT('Ctrl Pts',(0.0125829444471341,-0.0336797586670073,
0.0701355415613637));
#82030=CARTESIAN_POINT('Ctrl Pts',(0.0125843731495701,-0.0336769361243751,
0.0701371296657963));
#82031=CARTESIAN_POINT('Origin',(0.00116839656982703,-0.0345562520431624,
0.0819105626205519));
#82032=CARTESIAN_POINT('Ctrl Pts',(0.0125056360034304,-0.0342436276873911,
0.0704247507217681));
#82033=CARTESIAN_POINT('Ctrl Pts',(0.0123651359107284,-0.033943005420181,
0.0702594863808946));
#82034=CARTESIAN_POINT('Ctrl Pts',(0.0122125865767564,-0.0336441434784052,
0.0701052745813516));
#82035=CARTESIAN_POINT('Ctrl Pts',(0.0123396054690808,-0.0342436276873911,
0.070237844698153));
#82036=CARTESIAN_POINT('Ctrl Pts',(0.0121920560994895,-0.033943005420181,
0.0700788423021119));
#82037=CARTESIAN_POINT('Ctrl Pts',(0.0120329491902269,-0.0336441434784052,
0.0699314056382915));
#82038=CARTESIAN_POINT('Ctrl Pts',(0.0123379451637373,-0.0342436276873911,
0.0702359756379168));
#82039=CARTESIAN_POINT('Ctrl Pts',(0.0121903253013771,-0.033943005420181,
0.0700770358613241));
#82040=CARTESIAN_POINT('Ctrl Pts',(0.0120311528163616,-0.0336441434784052,
0.0699296669488608));
#82041=CARTESIAN_POINT('',(0.0123149137277548,-0.0341934961088741,0.0702114036181282));
#82042=CARTESIAN_POINT('',(0.0121495594626338,-0.0338664212862451,0.0700425382074119));
#82043=CARTESIAN_POINT('Origin',(-0.000223393381571894,-0.0345610720405284,
0.0812949048066704));
#82044=CARTESIAN_POINT('Origin',(0.0198255785810367,-0.0336938005073078,
0.0622107149897495));
#82045=CARTESIAN_POINT('',(0.0122378800854608,-0.0336938721132327,0.0701310046613436));
#82046=CARTESIAN_POINT('',(0.0121932443076082,-0.0336938721132427,0.070087256548999));
#82047=CARTESIAN_POINT('',(0.0123995251713318,-0.0340203938281605,0.0703034239921491));
#82048=CARTESIAN_POINT('Origin',(-0.000482693489046462,-0.0345589643244883,
0.0808895652102122));
#82049=CARTESIAN_POINT('',(0.0123985151930508,-0.034193496108874,0.0703043325963879));
#82050=CARTESIAN_POINT('Origin',(0.0205907235866023,-0.0341934220717551,
0.0629343977337704));
#82051=CARTESIAN_POINT('',(0.0123567144604128,-0.0341934961088841,0.0702578681072681));
#82052=CARTESIAN_POINT('Ctrl Pts',(0.0127382371674446,-0.0340223579322397,
0.070315054721398));
#82053=CARTESIAN_POINT('Ctrl Pts',(0.0126853432700955,-0.0339125849573575,
0.0702514093522981));
#82054=CARTESIAN_POINT('Ctrl Pts',(0.0126311692294267,-0.0338030433565231,
0.0701889034868289));
#82055=CARTESIAN_POINT('Ctrl Pts',(0.0125757914107587,-0.0336938721132327,
0.070127610918123));
#82056=CARTESIAN_POINT('Ctrl Pts',(0.0126249737418219,-0.0340223579322397,
0.0703115084209783));
#82057=CARTESIAN_POINT('Ctrl Pts',(0.0125720309317409,-0.0339125849573575,
0.0702494252499211));
#82058=CARTESIAN_POINT('Ctrl Pts',(0.01251784034658,-0.0338030433565231,
0.0701884814971361));
#82059=CARTESIAN_POINT('Ctrl Pts',(0.0124624781957316,-0.0336938721132327,
0.0701287489562014));
#82060=CARTESIAN_POINT('Ctrl Pts',(0.0125117103161992,-0.0340223579322397,
0.0703079621205585));
#82061=CARTESIAN_POINT('Ctrl Pts',(0.0124587185933862,-0.0339125849573575,
0.0702474411475441));
#82062=CARTESIAN_POINT('Ctrl Pts',(0.0124045114637332,-0.0338030433565231,
0.0701880595074433));
#82063=CARTESIAN_POINT('Ctrl Pts',(0.0123491649807044,-0.0336938721132327,
0.0701298869942798));
#82064=CARTESIAN_POINT('Ctrl Pts',(0.0123984468905764,-0.0340223579322397,
0.0703044158201387));
#82065=CARTESIAN_POINT('Ctrl Pts',(0.0123454062550316,-0.0339125849573575,
0.0702454570451671));
#82066=CARTESIAN_POINT('Ctrl Pts',(0.0122911825808865,-0.0338030433565231,
0.0701876375177504));
#82067=CARTESIAN_POINT('Ctrl Pts',(0.0122358517656772,-0.0336938721132327,
0.0701310250323582));
#82068=CARTESIAN_POINT('',(0.0124068357481178,-0.0336938721132427,0.0701293077897433));
#82069=CARTESIAN_POINT('Ctrl Pts',(0.0125843731459267,-0.0337108120662694,
0.0701371296690737));
#82070=CARTESIAN_POINT('Ctrl Pts',(0.0125524061304323,-0.0337611408993759,
0.0701658880756172));
#82071=CARTESIAN_POINT('Ctrl Pts',(0.0125210224420479,-0.0338121088780195,
0.0701941217050455));
#82072=CARTESIAN_POINT('Ctrl Pts',(0.0124593931293299,-0.0339153382773244,
0.070249565130174));
#82073=CARTESIAN_POINT('Ctrl Pts',(0.0124291735780691,-0.0339675558473119,
0.0702767514698207));
#82074=CARTESIAN_POINT('Ctrl Pts',(0.0123995251712986,-0.0340203938281304,
0.0703034239921718));
#82075=CARTESIAN_POINT('Ctrl Pts',(0.0123148067138119,-0.0341934961088741,
0.0702134289403001));
#82076=CARTESIAN_POINT('Ctrl Pts',(0.0122334212084299,-0.0340287516182428,
0.0701267828100733));
#82077=CARTESIAN_POINT('Ctrl Pts',(0.0121485240951087,-0.033864463327595,
0.0700435744419888));
#82078=CARTESIAN_POINT('Ctrl Pts',(0.0123149137277548,-0.0341934961088741,
0.0702114036181283));
#82079=CARTESIAN_POINT('Ctrl Pts',(0.0122334863504325,-0.0340287516182428,
0.0701247552754726));
#82080=CARTESIAN_POINT('Ctrl Pts',(0.0121485473095084,-0.033864463327595,
0.0700415464274487));
#82081=CARTESIAN_POINT('Ctrl Pts',(0.0123327443089812,-0.0341934961088741,
0.0698739459887476));
#82082=CARTESIAN_POINT('Ctrl Pts',(0.0122443402610246,-0.0340287516182428,
0.0697869290128721));
#82083=CARTESIAN_POINT('Ctrl Pts',(0.0121524152750071,-0.033864463327595,
0.0697036401977087));
#82084=CARTESIAN_POINT('',(0.0123236009792153,-0.0341764758832411,0.0698649653263334));
#82085=CARTESIAN_POINT('',(0.0123327443089812,-0.034193496108874,0.0698739459887476));
#82086=CARTESIAN_POINT('Origin',(0.000367949148720214,-0.0345621026500832,
0.0813316002940054));
#82087=CARTESIAN_POINT('Ctrl Pts',(0.0123236009797485,-0.0341764758837509,
0.0698649653280674));
#82088=CARTESIAN_POINT('Ctrl Pts',(0.012293555221579,-0.0341260050040218,
0.0698956207454876));
#82089=CARTESIAN_POINT('Ctrl Pts',(0.0122640317568554,-0.0340749269147712,
0.0699257433261768));
#82090=CARTESIAN_POINT('Ctrl Pts',(0.0122060064023127,-0.0339715436305228,
0.0699849460310153));
#82091=CARTESIAN_POINT('Ctrl Pts',(0.0121775265216962,-0.0339192778235013,
0.0700140036908399));
#82092=CARTESIAN_POINT('Ctrl Pts',(0.0121495594643107,-0.0338664212852959,
0.070042538207297));
#82093=CARTESIAN_POINT('',(0.012323829018378,-0.0341934961088841,0.0700426748034479));
#82094=CARTESIAN_POINT('Origin',(0.00812378219310841,-0.0315241814719618,
0.07415));
#82095=CARTESIAN_POINT('',(0.0123236009780977,-0.0342105180190549,0.0698649653262714));
#82096=CARTESIAN_POINT('',(0.0123144384873286,-0.0341934961088739,0.0698560042124233));
#82097=CARTESIAN_POINT('Origin',(0.000396441343576246,-0.0345621714110604,
0.0813668513846585));
#82098=CARTESIAN_POINT('Origin',(0.00109940268487801,-0.0345621032237729,
0.082048509369557));
#82099=CARTESIAN_POINT('Origin',(0.00106358853260313,-0.0345621720573663,
0.0820207289396908));
#82100=CARTESIAN_POINT('Ctrl Pts',(0.012238951351207,-0.0346945769586966,
0.0701320546229771));
#82101=CARTESIAN_POINT('Ctrl Pts',(0.0121547938765877,-0.0345275153362944,
0.0700458607573369));
#82102=CARTESIAN_POINT('Ctrl Pts',(0.0120679039167965,-0.0343603235965185,
0.0699622912726633));
#82103=CARTESIAN_POINT('Ctrl Pts',(0.0119785421272265,-0.034193496108874,
0.0698815895109745));
#82104=CARTESIAN_POINT('Ctrl Pts',(0.0121790798919958,-0.0346945769586966,
0.0700733738191504));
#82105=CARTESIAN_POINT('Ctrl Pts',(0.0120936933244458,-0.0345275153362944,
0.0699884339851946));
#82106=CARTESIAN_POINT('Ctrl Pts',(0.0120056133919598,-0.0343603235965185,
0.0699061575104035));
#82107=CARTESIAN_POINT('Ctrl Pts',(0.011915104212505,-0.034193496108874,
0.0698267838603386));
#82108=CARTESIAN_POINT('Ctrl Pts',(0.0121192084327849,-0.0346945769586966,
0.0700146930153222));
#82109=CARTESIAN_POINT('Ctrl Pts',(0.0120325927723039,-0.0345275153362944,
0.0699310072130522));
#82110=CARTESIAN_POINT('Ctrl Pts',(0.011943322867123,-0.0343603235965185,
0.0698500237481442));
#82111=CARTESIAN_POINT('Ctrl Pts',(0.0118516662977839,-0.034193496108874,
0.0697719782097026));
#82112=CARTESIAN_POINT('Ctrl Pts',(0.0120593369735733,-0.0346945769586966,
0.0699560122114968));
#82113=CARTESIAN_POINT('Ctrl Pts',(0.011971492220162,-0.0345275153362944,
0.0698735804409099));
#82114=CARTESIAN_POINT('Ctrl Pts',(0.0118810323422863,-0.0343603235965185,
0.0697938899858841));
#82115=CARTESIAN_POINT('Ctrl Pts',(0.0117882283830619,-0.034193496108874,
0.069717172559067));
#82116=CARTESIAN_POINT('',(0.0120593369740059,-0.0346945769586966,0.069956012211921));
#82117=CARTESIAN_POINT('',(0.0118837058515021,-0.034366772783148,0.0697978626993801));
#82118=CARTESIAN_POINT('Origin',(0.000688184036314178,-0.0345626457063121,
0.0823412505265048));
#82119=CARTESIAN_POINT('Origin',(0.0191090129876251,-0.0341934771028923,
0.0614345146097458));
#82120=CARTESIAN_POINT('',(0.0119774070477464,-0.034193496108874,0.069880608886537));
#82121=CARTESIAN_POINT('',(0.0119301123817021,-0.0341934961088841,0.0698397498047804));
#82122=CARTESIAN_POINT('',(0.0121495594633213,-0.0345211942962664,0.070042538208269));
#82123=CARTESIAN_POINT('Origin',(0.000347128644582184,-0.0345625596120204,
0.0820023227910331));
#82124=CARTESIAN_POINT('',(0.0121486085297354,-0.0346945769586887,0.0700435084366343));
#82125=CARTESIAN_POINT('Origin',(0.0198927720703194,-0.0346945685853879,
0.0621422144752763));
#82126=CARTESIAN_POINT('',(0.0121039727518807,-0.0346945769587026,0.0699997603242877));
#82127=CARTESIAN_POINT('Ctrl Pts',(0.0124883327279811,-0.0345231616327842,
0.0700328773848013));
#82128=CARTESIAN_POINT('Ctrl Pts',(0.0124315839891756,-0.0344132092796988,
0.0699727182004737));
#82129=CARTESIAN_POINT('Ctrl Pts',(0.0123735938330692,-0.0343032738558979,
0.0699137359229829));
#82130=CARTESIAN_POINT('Ctrl Pts',(0.0123144384873313,-0.0341934961088739,
0.0698560042124231));
#82131=CARTESIAN_POINT('Ctrl Pts',(0.0123750703210705,-0.0345231616327842,
0.0700364499636191));
#82132=CARTESIAN_POINT('Ctrl Pts',(0.0123183708252341,-0.0344132092796988,
0.0699778519421101));
#82133=CARTESIAN_POINT('Ctrl Pts',(0.0122604622009777,-0.0343032738558979,
0.069920429728337));
#82134=CARTESIAN_POINT('Ctrl Pts',(0.0122014205203234,-0.0341934961088739,
0.0698642549864478));
#82135=CARTESIAN_POINT('Ctrl Pts',(0.0122618079141598,-0.0345231616327842,
0.0700400225424369));
#82136=CARTESIAN_POINT('Ctrl Pts',(0.0122051576612927,-0.0344132092796988,
0.0699829856837465));
#82137=CARTESIAN_POINT('Ctrl Pts',(0.0121473305688863,-0.0343032738558979,
0.0699271235336912));
#82138=CARTESIAN_POINT('Ctrl Pts',(0.0120884025533155,-0.0341934961088739,
0.0698725057604725));
#82139=CARTESIAN_POINT('Ctrl Pts',(0.0121485455072491,-0.0345231616327842,
0.0700435951212548));
#82140=CARTESIAN_POINT('Ctrl Pts',(0.0120919444973512,-0.0344132092796988,
0.0699881194253828));
#82141=CARTESIAN_POINT('Ctrl Pts',(0.0120341989367948,-0.0343032738558979,
0.0699338173390453));
#82142=CARTESIAN_POINT('Ctrl Pts',(0.0119753845863076,-0.0341934961088739,
0.0698807565344973));
#82143=CARTESIAN_POINT('',(0.0121459227675475,-0.0341934961088839,0.0698683065494902));
#82144=CARTESIAN_POINT('Ctrl Pts',(0.0123236009756735,-0.03421051801954,
0.0698649653287348));
#82145=CARTESIAN_POINT('Ctrl Pts',(0.012293521430468,-0.0342610556240684,
0.0698956551991256));
#82146=CARTESIAN_POINT('Ctrl Pts',(0.0122639816471471,-0.0343122189868869,
0.0699257943556619));
#82147=CARTESIAN_POINT('Ctrl Pts',(0.0122059557101443,-0.0344158119695154,
0.0699849976605572));
#82148=CARTESIAN_POINT('Ctrl Pts',(0.0121774932896023,-0.034468199045003,
0.0700140375942222));
#82149=CARTESIAN_POINT('Ctrl Pts',(0.0121495594632927,-0.034521194296245,
0.0700425382082808));
#82150=CARTESIAN_POINT('Ctrl Pts',(0.0120593573372814,-0.0346945769586932,
0.0699580397604875));
#82151=CARTESIAN_POINT('Ctrl Pts',(0.0119726915254654,-0.034529677707698,
0.0698766745291053));
#82152=CARTESIAN_POINT('Ctrl Pts',(0.0118827368687214,-0.034364806625142,
0.0697989608009381));
#82153=CARTESIAN_POINT('Ctrl Pts',(0.0120593369740125,-0.0346945769586932,
0.0699560122119273));
#82154=CARTESIAN_POINT('Ctrl Pts',(0.0119726292440646,-0.034529677707698,
0.0698746474015413));
#82155=CARTESIAN_POINT('Ctrl Pts',(0.0118826327224075,-0.034364806625142,
0.0697969358265254));
#82156=CARTESIAN_POINT('Ctrl Pts',(0.0120559432307921,-0.0346945769586932,
0.0696181008866346));
#82157=CARTESIAN_POINT('Ctrl Pts',(0.0119622494232922,-0.034529677707698,
0.0695368062394883));
#82158=CARTESIAN_POINT('Ctrl Pts',(0.0118652756935101,-0.034364806625142,
0.0694594535087634));
#82159=CARTESIAN_POINT('',(0.0120462540429111,-0.0346775396664993,0.0696097120596878));
#82160=CARTESIAN_POINT('',(0.0120559432307895,-0.0346945769586886,0.0696181008866323));
#82161=CARTESIAN_POINT('Origin',(0.00130906264192214,-0.034562661834901,
0.0822716875907431));
#82162=CARTESIAN_POINT('Ctrl Pts',(0.0120462540434552,-0.0346775396670097,
0.0696097120614208));
#82163=CARTESIAN_POINT('Ctrl Pts',(0.0120181703416947,-0.0346269749928187,
0.0696422191576203));
#82164=CARTESIAN_POINT('Ctrl Pts',(0.0119905857771611,-0.0345757902890786,
0.0696741485536673));
#82165=CARTESIAN_POINT('Ctrl Pts',(0.0119363920746166,-0.0344721681088032,
0.0697368781285126));
#82166=CARTESIAN_POINT('Ctrl Pts',(0.0119098041788283,-0.0344197714289985,
0.069767653710673));
#82167=CARTESIAN_POINT('Ctrl Pts',(0.0118837058517475,-0.0343667727830668,
0.0697978626994496));
#82168=CARTESIAN_POINT('',(0.0120576401024077,-0.0346945769587026,0.0697870565492867));
#82169=CARTESIAN_POINT('Origin',(0.00812378219310841,-0.0315241814719618,
0.07415));
#82170=CARTESIAN_POINT('',(0.0120462540415805,-0.0347116136489625,0.0696097120600979));
#82171=CARTESIAN_POINT('',(0.0120365469580378,-0.0346945769586885,0.0696013439463572));
#82172=CARTESIAN_POINT('Origin',(0.00134454427527055,-0.034562669423854,
0.0822998697148694));
#82173=CARTESIAN_POINT('Origin',(0.00107793587347129,-0.0345626624041072,
0.0820720131763714));
#82174=CARTESIAN_POINT('Origin',(0.00104490125481206,-0.0345626700230594,
0.0820409986768044));
#82175=CARTESIAN_POINT('Ctrl Pts',(0.0120060286039437,-0.0352450361874068,
0.0699065432214784));
#82176=CARTESIAN_POINT('Ctrl Pts',(0.011845984005332,-0.0349452760959493,
0.0697601218954314));
#82177=CARTESIAN_POINT('Ctrl Pts',(0.0116753650231926,-0.034644428984174,
0.0696261717509751));
#82178=CARTESIAN_POINT('Ctrl Pts',(0.0120041282978596,-0.0352450361874068,
0.0699048805544081));
#82179=CARTESIAN_POINT('Ctrl Pts',(0.0118440209907302,-0.0349452760959493,
0.0697585308995812));
#82180=CARTESIAN_POINT('Ctrl Pts',(0.0116733448767912,-0.034644428984174,
0.0696246569461966));
#82181=CARTESIAN_POINT('Ctrl Pts',(0.0118159791806163,-0.0352450361874068,
0.0697402600524025));
#82182=CARTESIAN_POINT('Ctrl Pts',(0.0116496631093728,-0.0349452760959493,
0.0696010065579749));
#82183=CARTESIAN_POINT('Ctrl Pts',(0.0114733303816012,-0.034644428984174,
0.0694746762750623));
#82184=CARTESIAN_POINT('Ctrl Pts',(0.0118140976894439,-0.0352450361874068,
0.0697386138473825));
#82185=CARTESIAN_POINT('Ctrl Pts',(0.0116477195305592,-0.0349452760959493,
0.069599431314559));
#82186=CARTESIAN_POINT('Ctrl Pts',(0.0114713302366493,-0.034644428984174,
0.069473176468351));
#82187=CARTESIAN_POINT('',(0.0117882548360518,-0.0351951634053341,0.0697171913472817));
#82188=CARTESIAN_POINT('',(0.0116030135390007,-0.0348678972925388,0.0695703630884358));
#82189=CARTESIAN_POINT('Origin',(0.00180673700457118,-0.0345636767884998,
0.0831624060402997));
#82190=CARTESIAN_POINT('Origin',(0.0182875125888102,-0.0346946199340978,
0.0607717005939312));
#82191=CARTESIAN_POINT('',(0.0117017255272817,-0.0346945769330288,0.0696470624592927));
#82192=CARTESIAN_POINT('',(0.0116519586167633,-0.0346945769458128,0.0696092536546967));
#82193=CARTESIAN_POINT('',(0.0118837058516422,-0.0350221583435276,0.0697978626995465));
#82194=CARTESIAN_POINT('Origin',(0.00140024348590816,-0.0345628458718178,
0.0829056835978697));
#82195=CARTESIAN_POINT('',(0.0118828995328131,-0.0351951360298762,0.0697988006455434));
#82196=CARTESIAN_POINT('Origin',(0.0190865024647824,-0.0351951838366724,
0.061460578494381));
#82197=CARTESIAN_POINT('',(0.0117882283836044,-0.0351951371328748,0.0697171725593821));
#82198=CARTESIAN_POINT('Ctrl Pts',(0.0122212033147025,-0.0350241211494343,
0.0697669485341435));
#82199=CARTESIAN_POINT('Ctrl Pts',(0.0121608285778814,-0.0349144232818962,
0.0697105082382016));
#82200=CARTESIAN_POINT('Ctrl Pts',(0.012099251042623,-0.0348045283579412,
0.0696552821489737));
#82201=CARTESIAN_POINT('Ctrl Pts',(0.012036546949615,-0.0346945769439158,
0.06960134393911));
#82202=CARTESIAN_POINT('Ctrl Pts',(0.0121083887061872,-0.0350241211494343,
0.0697776258890849));
#82203=CARTESIAN_POINT('Ctrl Pts',(0.0120481610455526,-0.0349144232818962,
0.0697227395681195));
#82204=CARTESIAN_POINT('Ctrl Pts',(0.0119867627962859,-0.0348045283579412,
0.0696690653438272));
#82205=CARTESIAN_POINT('Ctrl Pts',(0.011924270043401,-0.0346945769439158,
0.0696166748925707));
#82206=CARTESIAN_POINT('Ctrl Pts',(0.0119955740976719,-0.0350241211494343,
0.0697883032440263));
#82207=CARTESIAN_POINT('Ctrl Pts',(0.0119354935132237,-0.0349144232818962,
0.0697349708980374));
#82208=CARTESIAN_POINT('Ctrl Pts',(0.0118742745499488,-0.0348045283579412,
0.0696828485386806));
#82209=CARTESIAN_POINT('Ctrl Pts',(0.011811993137187,-0.0346945769439158,
0.0696320058460315));
#82210=CARTESIAN_POINT('Ctrl Pts',(0.0118827594891566,-0.0350241211494343,
0.0697989805989677));
#82211=CARTESIAN_POINT('Ctrl Pts',(0.0118228259808948,-0.0349144232818962,
0.0697472022279553));
#82212=CARTESIAN_POINT('Ctrl Pts',(0.0117617863036118,-0.0348045283579412,
0.0696966317335341));
#82213=CARTESIAN_POINT('Ctrl Pts',(0.011699716230973,-0.0346945769439158,
0.0696473367994923));
#82214=CARTESIAN_POINT('',(0.0118691362429459,-0.0346945769458128,0.0696242032029469));
#82215=CARTESIAN_POINT('Ctrl Pts',(0.0120462540394248,-0.034711613649281,
0.0696097120625826));
#82216=CARTESIAN_POINT('Ctrl Pts',(0.0120181814806057,-0.0347621546531728,
0.0696422062410426));
#82217=CARTESIAN_POINT('Ctrl Pts',(0.0119906025132298,-0.0348133084095833,
0.069674129084038));
#82218=CARTESIAN_POINT('Ctrl Pts',(0.0119364087447131,-0.0349168561544578,
0.0697368587410297));
#82219=CARTESIAN_POINT('Ctrl Pts',(0.0119098154395837,-0.0349692089015919,
0.0697676406732463));
#82220=CARTESIAN_POINT('Ctrl Pts',(0.0118837058516033,-0.0350221583435,
0.0697978626995612));
#82221=CARTESIAN_POINT('Ctrl Pts',(0.0117883349063016,-0.0351951371254968,
0.0697186316936575));
#82222=CARTESIAN_POINT('Ctrl Pts',(0.0116967191469006,-0.0350307338980959,
0.0696428693655287));
#82223=CARTESIAN_POINT('Ctrl Pts',(0.0116020503338566,-0.0348659306897807,
0.0695709583540564));
#82224=CARTESIAN_POINT('Ctrl Pts',(0.0117882283835361,-0.0351951371254968,
0.0697171725594763));
#82225=CARTESIAN_POINT('Ctrl Pts',(0.0116965824574513,-0.0350307338980959,
0.0696414124336389));
#82226=CARTESIAN_POINT('Ctrl Pts',(0.011601883594524,-0.0348659306897807,
0.0695695048693978));
#82227=CARTESIAN_POINT('Ctrl Pts',(0.011770375057007,-0.0351951371254967,
0.0694726201498912));
#82228=CARTESIAN_POINT('Ctrl Pts',(0.0116736731632914,-0.0350307338980959,
0.0693972291303782));
#82229=CARTESIAN_POINT('Ctrl Pts',(0.0115739379085905,-0.0348659306897807,
0.0693258993256601));
#82230=CARTESIAN_POINT('Origin',(0.0148201985662875,-0.0308609197410856,
0.0653356520739864));
#82231=CARTESIAN_POINT('',(0.0117804447357082,-0.0351951371254968,0.0696105532228179));
#82232=CARTESIAN_POINT('Origin',(0.00765165544607738,-0.0351840467441093,
0.0750054776357416));
#82233=CARTESIAN_POINT('Origin',(0.0147132492090122,-0.0352322613180634,
0.0641627590476698));
#82234=CARTESIAN_POINT('',(0.0114116499145033,-0.0351951142564672,0.069431129326838));
#82235=CARTESIAN_POINT('',(0.0113078379568051,-0.0351951372916787,0.0693620684117596));
#82236=CARTESIAN_POINT('Origin',(0.00778340221991616,-0.0352875121180037,
0.074138041142237));
#82237=CARTESIAN_POINT('Origin',(0.0134603339411495,-0.029832507652317,
0.0794241260621529));
#82238=CARTESIAN_POINT('Origin',(0.0150506355830869,-0.0338732794983985,
0.069431195039007));
#82239=CARTESIAN_POINT('Ctrl Pts',(0.0135575492129203,-0.0321934096636942,
0.0722652422649808));
#82240=CARTESIAN_POINT('Ctrl Pts',(0.0135238129470215,-0.0320508460845295,
0.0721679804229908));
#82241=CARTESIAN_POINT('Ctrl Pts',(0.0134874888845993,-0.0319086045665006,
0.0720716983436474));
#82242=CARTESIAN_POINT('Ctrl Pts',(0.0134486723049796,-0.0317669892870789,
0.0719765969003001));
#82243=CARTESIAN_POINT('Ctrl Pts',(0.0135283559758708,-0.0321934096636942,
0.0721866408175494));
#82244=CARTESIAN_POINT('Ctrl Pts',(0.0134932127814944,-0.0320508460845295,
0.0720899015206002));
#82245=CARTESIAN_POINT('Ctrl Pts',(0.0134554968911776,-0.0319086045665006,
0.071994179393689));
#82246=CARTESIAN_POINT('Ctrl Pts',(0.0134153064818377,-0.0317669892870789,
0.0718996738577699));
#82247=CARTESIAN_POINT('Ctrl Pts',(0.0134991627388212,-0.0321934096636942,
0.0721080393701181));
#82248=CARTESIAN_POINT('Ctrl Pts',(0.0134626126159674,-0.0320508460845295,
0.0720118226182097));
#82249=CARTESIAN_POINT('Ctrl Pts',(0.0134235048977559,-0.0319086045665006,
0.0719166604437308));
#82250=CARTESIAN_POINT('Ctrl Pts',(0.013381940658696,-0.0317669892870789,
0.0718227508152399));
#82251=CARTESIAN_POINT('Ctrl Pts',(0.0134699695017717,-0.0321934096636942,
0.0720294379226868));
#82252=CARTESIAN_POINT('Ctrl Pts',(0.0134320124504403,-0.0320508460845295,
0.0719337437158192));
#82253=CARTESIAN_POINT('Ctrl Pts',(0.0133915129043343,-0.0319086045665006,
0.0718391414937724));
#82254=CARTESIAN_POINT('Ctrl Pts',(0.0133485748355541,-0.0317669892870789,
0.0717458277727096));
#82255=CARTESIAN_POINT('',(0.0134704917745492,-0.0321934096636942,0.0720308441181146));
#82256=CARTESIAN_POINT('',(0.0133789127702746,-0.0318665617511327,0.0718129660665446));
#82257=CARTESIAN_POINT('Origin',(-0.00227972748522134,-0.0326371944424414,
0.0776119280737242));
#82258=CARTESIAN_POINT('Origin',(0.0233943658975282,-0.0316939261509014,
0.0673589466646818));
#82259=CARTESIAN_POINT('',(0.0135151508928967,-0.0320197221621821,0.0721473186200811));
#82260=CARTESIAN_POINT('Ctrl Pts',(0.0135151328433497,-0.032019739209474,
0.072147134530176));
#82261=CARTESIAN_POINT('Ctrl Pts',(0.0135049415759329,-0.0319792716576038,
0.0721197016211392));
#82262=CARTESIAN_POINT('Ctrl Pts',(0.0134944947765313,-0.0319386439829729,
0.0720922215211813));
#82263=CARTESIAN_POINT('Ctrl Pts',(0.0134837735724475,-0.0318979099381661,
0.0720646683867518));
#82264=CARTESIAN_POINT('Ctrl Pts',(0.0134730525802759,-0.0318571766984961,
0.0720371157969292));
#82265=CARTESIAN_POINT('Ctrl Pts',(0.0134621133457679,-0.0318163871833608,
0.0720096295696911));
#82266=CARTESIAN_POINT('Ctrl Pts',(0.0134509967669547,-0.0317755399638303,
0.07198230294428));
#82267=CARTESIAN_POINT('',(0.0135140130126341,-0.0321934096636183,0.0721480230490248));
#82268=CARTESIAN_POINT('Origin',(0.0156707126887725,-0.032411291842895,
0.0713245685473849));
#82269=CARTESIAN_POINT('',(0.0134922523936017,-0.0321934096636663,0.0720894335835798));
#82270=CARTESIAN_POINT('Ctrl Pts',(0.0134696466733588,-0.0321934096636618,
0.0720326878890758));
#82271=CARTESIAN_POINT('Ctrl Pts',(0.0134404472892126,-0.0320835708272592,
0.07195896425157));
#82272=CARTESIAN_POINT('Ctrl Pts',(0.0134097391350493,-0.0319739230346488,
0.0718858876565074));
#82273=CARTESIAN_POINT('Ctrl Pts',(0.0133775686754118,-0.0318646057455572,
0.0718135485850041));
#82274=CARTESIAN_POINT('Ctrl Pts',(0.0135168633384403,-0.0321934096636618,
0.0719296745341005));
#82275=CARTESIAN_POINT('Ctrl Pts',(0.0134862433198451,-0.0320835708272592,
0.0718552997419847));
#82276=CARTESIAN_POINT('Ctrl Pts',(0.0134541018796477,-0.0319739230346488,
0.0717816017699644));
#82277=CARTESIAN_POINT('Ctrl Pts',(0.0134204873771956,-0.0318646057455572,
0.071708671753426));
#82278=CARTESIAN_POINT('Ctrl Pts',(0.0135640800035218,-0.0321934096636618,
0.0718266611791252));
#82279=CARTESIAN_POINT('Ctrl Pts',(0.0135320393504776,-0.0320835708272592,
0.0717516352323994));
#82280=CARTESIAN_POINT('Ctrl Pts',(0.013498464624246,-0.0319739230346488,
0.0716773158834214));
#82281=CARTESIAN_POINT('Ctrl Pts',(0.0134634060789795,-0.0318646057455572,
0.0716037949218479));
#82282=CARTESIAN_POINT('Ctrl Pts',(0.0136112966686033,-0.0321934096636618,
0.0717236478241499));
#82283=CARTESIAN_POINT('Ctrl Pts',(0.01357783538111,-0.0320835708272592,
0.0716479707228141));
#82284=CARTESIAN_POINT('Ctrl Pts',(0.0135428273688444,-0.0319739230346488,
0.0715730299968783));
#82285=CARTESIAN_POINT('Ctrl Pts',(0.0135063247807634,-0.0318646057455572,
0.0714989180902697));
#82286=CARTESIAN_POINT('',(0.0136061014165828,-0.032176398030847,0.0717119319308681));
#82287=CARTESIAN_POINT('',(0.0136112966685892,-0.0321934096636184,0.0717236478241218));
#82288=CARTESIAN_POINT('Origin',(-0.00175275152612349,-0.0326386231579772,
0.0778708058591182));
#82289=CARTESIAN_POINT('Ctrl Pts',(0.0136061014136762,-0.0321763980306286,
0.0717119319321528));
#82290=CARTESIAN_POINT('Ctrl Pts',(0.0135668855679636,-0.0321259596175053,
0.0717293717960751));
#82291=CARTESIAN_POINT('Ctrl Pts',(0.0135283491876663,-0.0320749164631853,
0.0717465094917317));
#82292=CARTESIAN_POINT('Ctrl Pts',(0.0134526043450023,-0.0319716057793979,
0.0717801943383765));
#82293=CARTESIAN_POINT('Ctrl Pts',(0.0134154253954175,-0.0319193786690191,
0.0717967283645963));
#82294=CARTESIAN_POINT('Ctrl Pts',(0.0133789127685737,-0.0318665617525381,
0.071812966067291));
#82295=CARTESIAN_POINT('',(0.0135408942215792,-0.0321934096636663,0.0718772459711283));
#82296=CARTESIAN_POINT('Origin',(0.00812378219310841,-0.0315241814719618,
0.07415));
#82297=CARTESIAN_POINT('',(0.0136061014169218,-0.0322104233323605,0.071711931930717));
#82298=CARTESIAN_POINT('',(0.0136008811544457,-0.0321934096636183,0.0717002271599731));
#82299=CARTESIAN_POINT('Origin',(-0.00174028061319681,-0.0326387240308083,
0.0779143900164998));
#82300=CARTESIAN_POINT('Origin',(-0.00125416538273813,-0.0326386238850291,
0.078991946492578));
#82301=CARTESIAN_POINT('Origin',(-0.00127817429069414,-0.0326387246683772,
0.0789534933216108));
#82302=CARTESIAN_POINT('Ctrl Pts',(0.0134423254954534,-0.0327445246967097,
0.0719611139497267));
#82303=CARTESIAN_POINT('Ctrl Pts',(0.0133597703084729,-0.032443687833936,
0.0717605218098416));
#82304=CARTESIAN_POINT('Ctrl Pts',(0.0132623402322532,-0.0321434074405927,
0.0715667179251309));
#82305=CARTESIAN_POINT('Ctrl Pts',(0.0133421768874091,-0.0327445246967097,
0.0717320500802344));
#82306=CARTESIAN_POINT('Ctrl Pts',(0.0132509824153575,-0.032443687833936,
0.0715352351068499));
#82307=CARTESIAN_POINT('Ctrl Pts',(0.0131452221089815,-0.0321434074405927,
0.0713458484043696));
#82308=CARTESIAN_POINT('',(0.0133268783657655,-0.0326943950436612,0.0716993031158297));
#82309=CARTESIAN_POINT('',(0.0132217993964906,-0.0323666188837389,0.0714876052895898));
#82310=CARTESIAN_POINT('Origin',(-0.00184898313512725,-0.0326395579109298,
0.0789312659146129));
#82311=CARTESIAN_POINT('Origin',(0.0230117647175438,-0.032193382560301,
0.0663748808834647));
#82312=CARTESIAN_POINT('',(0.013278459664916,-0.0321934096532689,0.0715990344654563));
#82313=CARTESIAN_POINT('',(0.0132495274267339,-0.0321934096584275,0.0715436343215988));
#82314=CARTESIAN_POINT('',(0.0133789127711315,-0.0325210109756239,0.0718129660661585));
#82315=CARTESIAN_POINT('Origin',(-0.00203062046382032,-0.0326393129156523,
0.0784860779647287));
#82316=CARTESIAN_POINT('',(0.0133776714505554,-0.0326943950436593,0.0718135180996885));
#82317=CARTESIAN_POINT('Origin',(0.0234856570143876,-0.0326943765538184,
0.0673183490763511));
#82318=CARTESIAN_POINT('',(0.0133522749081705,-0.0326943950436702,0.0717564106077691));
#82319=CARTESIAN_POINT('Ctrl Pts',(0.0136974526277365,-0.0325229783203769,
0.071928694553595));
#82320=CARTESIAN_POINT('Ctrl Pts',(0.0136668319807345,-0.032413025309245,
0.0718518616285417));
#82321=CARTESIAN_POINT('Ctrl Pts',(0.0136346265902,-0.032303122220807,0.0717756737841252));
#82322=CARTESIAN_POINT('Ctrl Pts',(0.0136008811526212,-0.0321934096576658,
0.0717002271558818));
#82323=CARTESIAN_POINT('Ctrl Pts',(0.0135908287267053,-0.0325229783203769,
0.0718903215687538));
#82324=CARTESIAN_POINT('Ctrl Pts',(0.0135596791089464,-0.032413025309245,
0.0718149584518445));
#82325=CARTESIAN_POINT('Ctrl Pts',(0.0135269752327534,-0.032303122220807,
0.0717402511350864));
#82326=CARTESIAN_POINT('Ctrl Pts',(0.0134927623662196,-0.0321934096576658,
0.0716662938350337));
#82327=CARTESIAN_POINT('Ctrl Pts',(0.0134842048256741,-0.0325229783203769,
0.0718519485839126));
#82328=CARTESIAN_POINT('Ctrl Pts',(0.0134525262371584,-0.032413025309245,
0.0717780552751473));
#82329=CARTESIAN_POINT('Ctrl Pts',(0.0134193238753068,-0.032303122220807,
0.0717048284860477));
#82330=CARTESIAN_POINT('Ctrl Pts',(0.013384643579818,-0.0321934096576658,
0.0716323605141857));
#82331=CARTESIAN_POINT('Ctrl Pts',(0.0133775809246429,-0.0325229783203769,
0.0718135755990713));
#82332=CARTESIAN_POINT('Ctrl Pts',(0.0133453733653703,-0.032413025309245,
0.0717411520984501));
#82333=CARTESIAN_POINT('Ctrl Pts',(0.0133116725178602,-0.032303122220807,
0.0716694058370089));
#82334=CARTESIAN_POINT('Ctrl Pts',(0.0132765247934164,-0.0321934096576658,
0.0715984271933376));
#82335=CARTESIAN_POINT('',(0.0134396704100311,-0.0321934096584275,0.0716496308130976));
#82336=CARTESIAN_POINT('Ctrl Pts',(0.0136061014137376,-0.0322104233328912,
0.0717119319321256));
#82337=CARTESIAN_POINT('Ctrl Pts',(0.0135668324299691,-0.0322609421830511,
0.0717293954273236));
#82338=CARTESIAN_POINT('Ctrl Pts',(0.0135282700908689,-0.032312088823898,
0.0717465446672346));
#82339=CARTESIAN_POINT('Ctrl Pts',(0.0134525246746201,-0.0324156524631812,
0.0717802297689611));
#82340=CARTESIAN_POINT('Ctrl Pts',(0.0134153727329965,-0.0324680267167319,
0.0717967517843503));
#82341=CARTESIAN_POINT('Ctrl Pts',(0.0133789127710902,-0.0325210109755913,
0.071812966066172));
#82342=CARTESIAN_POINT('Origin',(0.0104317671203413,-0.0262834582511411,
0.0816717412489181));
#82343=CARTESIAN_POINT('Origin',(0.0202695860884835,-0.0342770968612105,
0.0747014319232182));
#82344=CARTESIAN_POINT('Ctrl Pts',(0.0133261508800732,-0.0326943950436604,
0.0717011958533709));
#82345=CARTESIAN_POINT('Ctrl Pts',(0.0132924017693845,-0.0325844576448134,
0.0716294974625865));
#82346=CARTESIAN_POINT('Ctrl Pts',(0.0132571674299463,-0.0324744968375322,
0.071558491984537));
#82347=CARTESIAN_POINT('Ctrl Pts',(0.0132204942608865,-0.0323646534831894,
0.0714882697729062));
#82348=CARTESIAN_POINT('Ctrl Pts',(0.0133668060529127,-0.0326943950436604,
0.0715954211659316));
#82349=CARTESIAN_POINT('Ctrl Pts',(0.0133315991687882,-0.0325844576448134,
0.0715231624706695));
#82350=CARTESIAN_POINT('Ctrl Pts',(0.01329489536473,-0.0324744968375322,
0.0714516267976334));
#82351=CARTESIAN_POINT('Ctrl Pts',(0.0132567429319998,-0.0323646534831894,
0.071380905153855));
#82352=CARTESIAN_POINT('Ctrl Pts',(0.0134074612257521,-0.0326943950436604,
0.0714896464784924));
#82353=CARTESIAN_POINT('Ctrl Pts',(0.0133707965681918,-0.0325844576448134,
0.0714168274787526));
#82354=CARTESIAN_POINT('Ctrl Pts',(0.0133326232995138,-0.0324744968375322,
0.0713447616107299));
#82355=CARTESIAN_POINT('Ctrl Pts',(0.013292991603113,-0.0323646534831894,
0.0712735405348038));
#82356=CARTESIAN_POINT('Ctrl Pts',(0.0134481163985916,-0.0326943950436604,
0.0713838717910531));
#82357=CARTESIAN_POINT('Ctrl Pts',(0.0134099939675955,-0.0325844576448134,
0.0713104924868356));
#82358=CARTESIAN_POINT('Ctrl Pts',(0.0133703512342975,-0.0324744968375322,
0.0712378964238264));
#82359=CARTESIAN_POINT('Ctrl Pts',(0.0133292402742263,-0.0323646534831894,
0.0711661759157526));
#82360=CARTESIAN_POINT('',(0.0134421957513835,-0.0326773559991349,0.0713725052289173));
#82361=CARTESIAN_POINT('',(0.0134481163985908,-0.0326943950436594,0.0713838717910534));
#82362=CARTESIAN_POINT('Origin',(-0.0012533835582576,-0.0326395670550634,
0.0791038218523109));
#82363=CARTESIAN_POINT('Ctrl Pts',(0.0134421957484051,-0.0326773559987424,
0.0713725052304646));
#82364=CARTESIAN_POINT('Ctrl Pts',(0.0134041217295636,-0.0326267922586104,
0.0713923890524141));
#82365=CARTESIAN_POINT('Ctrl Pts',(0.0133667225452122,-0.0325756109579621,
0.071411920447978));
#82366=CARTESIAN_POINT('Ctrl Pts',(0.013293242016891,-0.0324719985462366,
0.0714502950085406));
#82367=CARTESIAN_POINT('Ctrl Pts',(0.0132571901439852,-0.0324196091621778,
0.071469122782535));
#82368=CARTESIAN_POINT('Ctrl Pts',(0.0132217993964473,-0.0323666188837757,
0.0714876052896124));
#82369=CARTESIAN_POINT('',(0.0133874973821882,-0.0326943950436703,0.0715415874534516));
#82370=CARTESIAN_POINT('Origin',(0.00812378219310841,-0.0315241814719618,
0.07415));
#82371=CARTESIAN_POINT('',(0.0134421957513442,-0.0327114338380046,0.0713725052289375));
#82372=CARTESIAN_POINT('',(0.0134362508414151,-0.0326943950436593,0.0713611513377796));
#82373=CARTESIAN_POINT('Origin',(-0.00123172383876959,-0.0326395677682108,
0.0791436191567031));
#82374=CARTESIAN_POINT('Origin',(-0.00129989860108158,-0.0326395675544282,
0.0790147558839406));
#82375=CARTESIAN_POINT('Origin',(-0.00132017994648858,-0.0326395682222787,
0.0789742386681461));
#82376=CARTESIAN_POINT('Ctrl Pts',(0.013294372096676,-0.0332451089994434,
0.071631443856269));
#82377=CARTESIAN_POINT('Ctrl Pts',(0.0131993831976154,-0.0329451141710254,
0.0714364318674927));
#82378=CARTESIAN_POINT('Ctrl Pts',(0.0130899750517819,-0.0326442513127494,
0.0712491288393898));
#82379=CARTESIAN_POINT('Ctrl Pts',(0.0131800365534401,-0.0332451089994434,
0.0714091211548799));
#82380=CARTESIAN_POINT('Ctrl Pts',(0.0130766626165102,-0.0329451141710254,
0.0712184214016686));
#82381=CARTESIAN_POINT('Ctrl Pts',(0.0129592180690264,-0.0326442513127494,
0.0710360499538552));
#82382=CARTESIAN_POINT('Ctrl Pts',(0.0131788931980078,-0.0332451089994434,
0.0714068979278661));
#82383=CARTESIAN_POINT('Ctrl Pts',(0.0130754354106992,-0.0329451141710254,
0.0712162412970104));
#82384=CARTESIAN_POINT('Ctrl Pts',(0.0129579104991988,-0.0326442513127494,
0.0710339191649999));
#82385=CARTESIAN_POINT('',(0.0131627307134367,-0.0331951640388616,0.0713774338944794));
#82386=CARTESIAN_POINT('',(0.0130445664749898,-0.0328677532355023,0.0711727517535438));
#82387=CARTESIAN_POINT('Origin',(-0.00113911576405468,-0.0326402808282269,
0.0801232577444776));
#82388=CARTESIAN_POINT('Origin',(0.022503705724796,-0.0326944278779141,
0.0654491979966907));
#82389=CARTESIAN_POINT('',(0.0131081116321623,-0.0326943950436593,0.0712804033309572));
#82390=CARTESIAN_POINT('',(0.0130757578824758,-0.0326943950436694,0.0712269291794491));
#82391=CARTESIAN_POINT('',(0.0132217993964919,-0.0330220786163545,0.0714876052895923));
#82392=CARTESIAN_POINT('Origin',(-0.00141434687361303,-0.0326396682762052,
0.079729049067357));
#82393=CARTESIAN_POINT('',(0.0132205951878513,-0.0331951640388588,0.0714882341769756));
#82394=CARTESIAN_POINT('Origin',(0.0229990778064989,-0.0331952026560082,
0.0663815084928096));
#82395=CARTESIAN_POINT('',(0.013191662950654,-0.0331951640388702,0.0714328340357375));
#82396=CARTESIAN_POINT('Ctrl Pts',(0.01354697692822,-0.0330240426238172,
0.0715831032616936));
#82397=CARTESIAN_POINT('Ctrl Pts',(0.0135116154248435,-0.032914277406352,
0.0715083934706549));
#82398=CARTESIAN_POINT('Ctrl Pts',(0.0134746918323956,-0.0328043479726691,
0.0714343774551129));
#82399=CARTESIAN_POINT('Ctrl Pts',(0.0134362508414215,-0.0326943950436593,
0.0713611513377811));
#82400=CARTESIAN_POINT('Ctrl Pts',(0.0134381539868773,-0.0330240426238172,
0.0715515009924333));
#82401=CARTESIAN_POINT('Ctrl Pts',(0.0134023571314531,-0.032914277406352,
0.0714782903434326));
#82402=CARTESIAN_POINT('Ctrl Pts',(0.0133650289613723,-0.0328043479726691,
0.0714057832172486));
#82403=CARTESIAN_POINT('Ctrl Pts',(0.0133262147387084,-0.0326943950436593,
0.0713340738178687));
#82404=CARTESIAN_POINT('Ctrl Pts',(0.0133293310455345,-0.0330240426238172,
0.071519898723173));
#82405=CARTESIAN_POINT('Ctrl Pts',(0.0132930988380627,-0.032914277406352,
0.0714481872162104));
#82406=CARTESIAN_POINT('Ctrl Pts',(0.0132553660903489,-0.0328043479726691,
0.0713771889793842));
#82407=CARTESIAN_POINT('Ctrl Pts',(0.0132161786359954,-0.0326943950436593,
0.0713069962979563));
#82408=CARTESIAN_POINT('Ctrl Pts',(0.0132205081041918,-0.0330240426238172,
0.0714882964539127));
#82409=CARTESIAN_POINT('Ctrl Pts',(0.0131838405446724,-0.032914277406352,
0.0714180840889881));
#82410=CARTESIAN_POINT('Ctrl Pts',(0.0131457032193256,-0.0328043479726691,
0.0713485947415199));
#82411=CARTESIAN_POINT('Ctrl Pts',(0.0131061425332823,-0.0326943950436593,
0.0712799187780439));
#82412=CARTESIAN_POINT('',(0.0132721812367987,-0.0326943950436693,0.0713207773343784));
#82413=CARTESIAN_POINT('Ctrl Pts',(0.0134421957483998,-0.032711433838331,
0.0713725052304673));
#82414=CARTESIAN_POINT('Ctrl Pts',(0.0134041280627768,-0.032761987682735,
0.0713923857449491));
#82415=CARTESIAN_POINT('Ctrl Pts',(0.0133667319719703,-0.0328131562596795,
0.0714119155249218));
#82416=CARTESIAN_POINT('Ctrl Pts',(0.0132932515104146,-0.0329167375861618,
0.0714502900506167));
#82417=CARTESIAN_POINT('Ctrl Pts',(0.0132571964188637,-0.0329691088926659,
0.0714691195055349));
#82418=CARTESIAN_POINT('Ctrl Pts',(0.0132217993964484,-0.0330220786163186,
0.0714876052896119));
#82419=CARTESIAN_POINT('Ctrl Pts',(0.0131621234123062,-0.0331951640388604,
0.0713793688852099));
#82420=CARTESIAN_POINT('Ctrl Pts',(0.0131048423903713,-0.033030642201062,
0.0712752044107868));
#82421=CARTESIAN_POINT('Ctrl Pts',(0.0130433050873985,-0.0328657861914645,
0.071173496429052));
#82422=CARTESIAN_POINT('Ctrl Pts',(0.0131627307134382,-0.0331951640388604,
0.0713774338944822));
#82423=CARTESIAN_POINT('Ctrl Pts',(0.0131054096868106,-0.033030642201062,
0.0712732568644976));
#82424=CARTESIAN_POINT('Ctrl Pts',(0.0130438318943943,-0.0328657861914645,
0.0711715379913659));
#82425=CARTESIAN_POINT('Ctrl Pts',(0.0132639234139576,-0.0331951640388604,
0.07105501240225));
#82426=CARTESIAN_POINT('Ctrl Pts',(0.0131999365296955,-0.033030642201062,
0.0709487432780609));
#82427=CARTESIAN_POINT('Ctrl Pts',(0.0131316121071198,-0.0328657861914645,
0.0708452096053105));
#82428=CARTESIAN_POINT('',(0.0132573007388876,-0.033178164828193,0.071044040029871));
#82429=CARTESIAN_POINT('',(0.0132639234139403,-0.0331951640388588,0.071055012402302));
#82430=CARTESIAN_POINT('Origin',(-0.000497103510496023,-0.0326412092060213,
0.0801984292855081));
#82431=CARTESIAN_POINT('Ctrl Pts',(0.01325730073875,-0.033178164828644,
0.0710440400317029));
#82432=CARTESIAN_POINT('Ctrl Pts',(0.0132205250709329,-0.033127681154677,
0.0710662906233262));
#82433=CARTESIAN_POINT('Ctrl Pts',(0.0131844134752943,-0.0330765663497778,
0.0710881394671044));
#82434=CARTESIAN_POINT('Ctrl Pts',(0.0131134873182336,-0.0329730614463164,
0.0711310522922301));
#82435=CARTESIAN_POINT('Ctrl Pts',(0.0130787014066564,-0.0329207133373767,
0.0711520989331467));
#82436=CARTESIAN_POINT('Ctrl Pts',(0.0130445664896799,-0.0328677532289379,
0.0711727517609904));
#82437=CARTESIAN_POINT('',(0.0132133270636985,-0.0331951640388702,0.0712162231484007));
#82438=CARTESIAN_POINT('Origin',(0.00812378219310841,-0.0315241814719618,
0.07415));
#82439=CARTESIAN_POINT('',(0.013257300737225,-0.0332121607144415,0.0710440400301211));
#82440=CARTESIAN_POINT('',(0.0132506546416663,-0.0331951640388587,0.0710330818271522));
#82441=CARTESIAN_POINT('Origin',(-0.000467273682971033,-0.0326413661553068,
0.0802325807301716));
#82442=CARTESIAN_POINT('Origin',(-0.00123452790923341,-0.0326412096447147,
0.0789796196542873));
#82443=CARTESIAN_POINT('Origin',(-0.00125093443179604,-0.0326413665784978,
0.0789373466122632));
#82444=CARTESIAN_POINT('Ctrl Pts',(0.0131260379500619,-0.0337436976235975,
0.0713117677434667));
#82445=CARTESIAN_POINT('Ctrl Pts',(0.0131005104590007,-0.0336723290703325,
0.0712667766970761));
#82446=CARTESIAN_POINT('Ctrl Pts',(0.0130741778505704,-0.033601104548885,
0.0712222520882799));
#82447=CARTESIAN_POINT('Ctrl Pts',(0.0129901030480482,-0.0333736987606857,
0.0710800938322218));
#82448=CARTESIAN_POINT('Ctrl Pts',(0.0128980089337392,-0.0331450831799192,
0.070942994538663));
#82449=CARTESIAN_POINT('Ctrl Pts',(0.0129979690416467,-0.0337436976235975,
0.0710970624694343));
#82450=CARTESIAN_POINT('Ctrl Pts',(0.0129705104588115,-0.0336723290703325,
0.0710532232942153));
#82451=CARTESIAN_POINT('Ctrl Pts',(0.0129422677895439,-0.033601104548885,
0.0710098851044995));
#82452=CARTESIAN_POINT('Ctrl Pts',(0.0128520945411301,-0.0333736987606857,
0.0708715148495486));
#82453=CARTESIAN_POINT('Ctrl Pts',(0.012754129408031,-0.0331450831799192,
0.0707385472787596));
#82454=CARTESIAN_POINT('Ctrl Pts',(0.0129966883525625,-0.0337436976235975,
0.0710949154166939));
#82455=CARTESIAN_POINT('Ctrl Pts',(0.0129692104588095,-0.0336723290703325,
0.0710510877601868));
#82456=CARTESIAN_POINT('Ctrl Pts',(0.0129409486889336,-0.033601104548885,
0.0710077614346617));
#82457=CARTESIAN_POINT('Ctrl Pts',(0.0128507144560609,-0.0333736987606857,
0.0708694290597219));
#82458=CARTESIAN_POINT('Ctrl Pts',(0.012752690612774,-0.0331450831799192,
0.0707365028061606));
#82459=CARTESIAN_POINT('',(0.0129786966333677,-0.0336938721132548,0.0710665067248715));
#82460=CARTESIAN_POINT('',(0.0128479134659113,-0.0333679869945434,0.070869648080258));
#82461=CARTESIAN_POINT('Ctrl Pts',(0.0129786966333755,-0.0336938721132648,
0.0710665067248828));
#82462=CARTESIAN_POINT('Ctrl Pts',(0.0129666603126299,-0.0336629187933932,
0.0710475557163417));
#82463=CARTESIAN_POINT('Ctrl Pts',(0.0129545168756118,-0.033631995230104,
0.0710286812462819));
#82464=CARTESIAN_POINT('Ctrl Pts',(0.0129422677895513,-0.033601104548895,
0.0710098851045111));
#82465=CARTESIAN_POINT('Ctrl Pts',(0.0129115306412241,-0.0335235892595454,
0.0709627191531304));
#82466=CARTESIAN_POINT('Ctrl Pts',(0.0128800735002384,-0.0334458668660369,
0.0709159626913196));
#82467=CARTESIAN_POINT('Ctrl Pts',(0.012847913466173,-0.0333679869945385,
0.0708696480800845));
#82468=CARTESIAN_POINT('Ctrl Pts',(0.0128478886666482,-0.0333679692459107,
0.0708696111605181));
#82469=CARTESIAN_POINT('Ctrl Pts',(0.01284751978041,-0.0333391895371493,
0.0708698745248455));
#82470=CARTESIAN_POINT('Ctrl Pts',(0.0128472451689676,-0.0333104081054902,
0.0708700745720281));
#82471=CARTESIAN_POINT('Ctrl Pts',(0.0128468849339141,-0.0332532696730203,
0.0708703438459546));
#82472=CARTESIAN_POINT('Ctrl Pts',(0.0128467965568541,-0.0332249163812529,
0.0708704149850103));
#82473=CARTESIAN_POINT('Ctrl Pts',(0.0128467974744775,-0.0331960985669457,
0.0708704227415418));
#82474=CARTESIAN_POINT('Ctrl Pts',(0.0128467975140083,-0.0331956312253307,
0.070870422850649));
#82475=CARTESIAN_POINT('Ctrl Pts',(0.0128467975774544,-0.0331951640388588,
0.0708704229420197));
#82476=CARTESIAN_POINT('',(0.0129180927308873,-0.0331951640388587,0.0709730971895031));
#82477=CARTESIAN_POINT('',(0.0128824451541801,-0.0331951640388687,0.0709217600657703));
#82478=CARTESIAN_POINT('',(0.0130445664767656,-0.033521636656769,0.071172751768968));
#82479=CARTESIAN_POINT('Origin',(-0.000540169405658373,-0.0326434571528753,
0.0808073568996008));
#82480=CARTESIAN_POINT('',(0.0130434041327693,-0.0336938721132327,0.0711734550279212));
#82481=CARTESIAN_POINT('Origin',(0.0223868954136058,-0.0336938867896333,
0.0655203142496365));
#82482=CARTESIAN_POINT('',(0.0130110503830785,-0.0336938721132538,0.0711199808764064));
#82483=CARTESIAN_POINT('Ctrl Pts',(0.0133750982475513,-0.0335235895815173,
0.0712476423899846));
#82484=CARTESIAN_POINT('Ctrl Pts',(0.0133351415808332,-0.0334144449262749,
0.0711753476856053));
#82485=CARTESIAN_POINT('Ctrl Pts',(0.0132936454545612,-0.0333049234473147,
0.071103795398033));
#82486=CARTESIAN_POINT('Ctrl Pts',(0.0132506546416721,-0.0331951640388587,
0.0710330818271533));
#82487=CARTESIAN_POINT('Ctrl Pts',(0.0132645055593811,-0.0335235895815173,
0.0712229355122069));
#82488=CARTESIAN_POINT('Ctrl Pts',(0.0132242087538469,-0.0334144449262749,
0.0711521633339172));
#82489=CARTESIAN_POINT('Ctrl Pts',(0.0131824035522238,-0.0333049234473147,
0.0710821423486446));
#82490=CARTESIAN_POINT('Ctrl Pts',(0.0131391353000311,-0.0331951640388587,
0.0710129669340089));
#82491=CARTESIAN_POINT('Ctrl Pts',(0.0131539128712108,-0.0335235895815172,
0.0711982286344292));
#82492=CARTESIAN_POINT('Ctrl Pts',(0.0131132759268607,-0.0334144449262749,
0.0711289789822291));
#82493=CARTESIAN_POINT('Ctrl Pts',(0.0130711616498865,-0.0333049234473147,
0.0710604892992561));
#82494=CARTESIAN_POINT('Ctrl Pts',(0.0130276159583901,-0.0331951640388587,
0.0709928520408646));
#82495=CARTESIAN_POINT('Ctrl Pts',(0.0130433201830405,-0.0335235895815172,
0.0711735217566515));
#82496=CARTESIAN_POINT('Ctrl Pts',(0.0130023430998744,-0.0334144449262749,
0.071105794630541));
#82497=CARTESIAN_POINT('Ctrl Pts',(0.0129599197475492,-0.0333049234473147,
0.0710388362498676));
#82498=CARTESIAN_POINT('Ctrl Pts',(0.0129160966167491,-0.0331951640388587,
0.0709727371477202));
#82499=CARTESIAN_POINT('',(0.0130843736862868,-0.0331951640388687,0.0710030895083376));
#82500=CARTESIAN_POINT('Ctrl Pts',(0.0132573007345394,-0.0332121607145969,
0.071044040031738));
#82501=CARTESIAN_POINT('Ctrl Pts',(0.0132205869265907,-0.0332625444109045,
0.0710662531818125));
#82502=CARTESIAN_POINT('Ctrl Pts',(0.0131845057551647,-0.0333135300745367,
0.0710880835644541));
#82503=CARTESIAN_POINT('Ctrl Pts',(0.0131135800443987,-0.0334167203140589,
0.0711309961236631));
#82504=CARTESIAN_POINT('Ctrl Pts',(0.0130787629753201,-0.0334688847587269,
0.0711520616797525));
#82505=CARTESIAN_POINT('Ctrl Pts',(0.0130445664760702,-0.0335216366562331,
0.0711727517691849));
#82506=CARTESIAN_POINT('Ctrl Pts',(0.0129784577173806,-0.0336938721132391,
0.0710674776182864));
#82507=CARTESIAN_POINT('Ctrl Pts',(0.012960414690991,-0.0336474569764958,
0.0710390615914907));
#82508=CARTESIAN_POINT('Ctrl Pts',(0.0129420402554495,-0.033601104548885,
0.0710108587281842));
#82509=CARTESIAN_POINT('Ctrl Pts',(0.0128955204092062,-0.0334837508592656,
0.0709394555625372));
#82510=CARTESIAN_POINT('Ctrl Pts',(0.0128469051672095,-0.0333660264659097,
0.070869462231394));
#82511=CARTESIAN_POINT('Ctrl Pts',(0.0129786966333786,-0.033693872113239,
0.0710665067248888));
#82512=CARTESIAN_POINT('Ctrl Pts',(0.0129606479240279,-0.0336474569764958,
0.0710380892996385));
#82513=CARTESIAN_POINT('Ctrl Pts',(0.0129422677895439,-0.033601104548885,
0.0710098851044995));
#82514=CARTESIAN_POINT('Ctrl Pts',(0.0128957335148884,-0.0334837508592656,
0.0709384785669586));
#82515=CARTESIAN_POINT('Ctrl Pts',(0.0128471037508992,-0.0333660264659097,
0.070868482292946));
#82516=CARTESIAN_POINT('Ctrl Pts',(0.0130599291282446,-0.033693872113239,
0.070736398680371));
#82517=CARTESIAN_POINT('Ctrl Pts',(0.0130399481869677,-0.0336474569764958,
0.0707075057743724));
#82518=CARTESIAN_POINT('Ctrl Pts',(0.013019630386853,-0.033601104548885,
0.0706788487502797));
#82519=CARTESIAN_POINT('Ctrl Pts',(0.0129681903883177,-0.0334837508592656,
0.0706062957539401));
#82520=CARTESIAN_POINT('Ctrl Pts',(0.0129146230827298,-0.0333660264659097,
0.0705352988913386));
#82521=CARTESIAN_POINT('',(0.0130521460724243,-0.0336769361243753,0.0707278326351485));
#82522=CARTESIAN_POINT('',(0.0130594446401983,-0.0336938721132327,0.0707383675156333));
#82523=CARTESIAN_POINT('Ctrl Pts',(0.0130521460724241,-0.033676936124375,
0.0707278326351483));
#82524=CARTESIAN_POINT('Ctrl Pts',(0.0130533644668488,-0.0336797586670023,
0.0707295872807962));
#82525=CARTESIAN_POINT('Ctrl Pts',(0.0130545818781333,-0.0336825812712842,
0.0707313425107595));
#82526=CARTESIAN_POINT('Ctrl Pts',(0.0130570147345841,-0.0336882266024761,
0.0707348541386481));
#82527=CARTESIAN_POINT('Ctrl Pts',(0.0130582301797444,-0.0336910493293757,
0.0707366105365684));
#82528=CARTESIAN_POINT('Ctrl Pts',(0.013059444640198,-0.0336938721132324,
0.0707383675156339));
#82529=CARTESIAN_POINT('Ctrl Pts',(0.0130521460724243,-0.0336769361243753,
0.0707278326351486));
#82530=CARTESIAN_POINT('Ctrl Pts',(0.0130177183665245,-0.033627900751621,
0.070751738615807));
#82531=CARTESIAN_POINT('Ctrl Pts',(0.0129828004637717,-0.0335767878632059,
0.070775984980357));
#82532=CARTESIAN_POINT('Ctrl Pts',(0.012914371179375,-0.0334733198857308,
0.0708235010464587));
#82533=CARTESIAN_POINT('Ctrl Pts',(0.0128808190586996,-0.0334209645014064,
0.0708467990364622));
#82534=CARTESIAN_POINT('Ctrl Pts',(0.0128479134700578,-0.0333679869844681,
0.0708696480862338));
#82535=CARTESIAN_POINT('',(0.013019070636793,-0.0336938721132538,0.0709024371202624));
#82536=CARTESIAN_POINT('Origin',(0.00812378219310841,-0.0315241814719618,
0.07415));
#82537=CARTESIAN_POINT('',(0.0130521460713649,-0.0337108120655546,0.0707278326358923));
#82538=CARTESIAN_POINT('',(0.0130448250186083,-0.0336938721132327,0.0707173133685686));
#82539=CARTESIAN_POINT('Origin',(-0.00102429383614181,-0.0345562523061984,
0.0791416383900627));
#82540=CARTESIAN_POINT('Ctrl Pts',(0.0130448250186194,-0.0336938721132369,
0.0707173133685675));
#82541=CARTESIAN_POINT('Ctrl Pts',(0.0130460469851738,-0.0336910493032244,
0.0707190651596254));
#82542=CARTESIAN_POINT('Ctrl Pts',(0.0130472680461666,-0.0336882265893999,
0.0707208176459574));
#82543=CARTESIAN_POINT('Ctrl Pts',(0.0130497083925903,-0.0336825812712979,
0.0707243240608837));
#82544=CARTESIAN_POINT('Ctrl Pts',(0.0130509276779969,-0.0336797586670092,
0.0707260779894966));
#82545=CARTESIAN_POINT('Ctrl Pts',(0.0130521460724245,-0.033676936124375,
0.0707278326351488));
#82546=CARTESIAN_POINT('Origin',(0.000250585409215087,-0.0345562519856471,
0.0809776272350968));
#82547=CARTESIAN_POINT('Ctrl Pts',(0.0129379813152136,-0.034243627687391,
0.0710033173320588));
#82548=CARTESIAN_POINT('Ctrl Pts',(0.0128193022219425,-0.033943005420181,
0.0708217468189407));
#82549=CARTESIAN_POINT('Ctrl Pts',(0.0126872836485237,-0.0336441434784053,
0.0706496315241931));
#82550=CARTESIAN_POINT('Ctrl Pts',(0.0127966855175306,-0.034243627687391,
0.0707970759745255));
#82551=CARTESIAN_POINT('Ctrl Pts',(0.0126702279032296,-0.033943005420181,
0.0706208345202676));
#82552=CARTESIAN_POINT('Ctrl Pts',(0.0125308543132922,-0.0336441434784053,
0.0704546190551583));
#82553=CARTESIAN_POINT('',(0.0127755024240185,-0.0341934961088741,0.0707677486945316));
#82554=CARTESIAN_POINT('',(0.012632616474384,-0.0338664212865005,0.0705794904525109));
#82555=CARTESIAN_POINT('Origin',(-0.00105306743210708,-0.0345610720407014,
0.080192386592122));
#82556=CARTESIAN_POINT('Origin',(0.0212296958108869,-0.033693800507293,
0.0637714840387905));
#82557=CARTESIAN_POINT('',(0.0127091528762319,-0.0336938721132327,0.0706783288320532));
#82558=CARTESIAN_POINT('',(0.0126703521572034,-0.0336938721132427,0.0706293313402693));
#82559=CARTESIAN_POINT('',(0.0128479134700608,-0.0340203938281606,0.0708696480862382));
#82560=CARTESIAN_POINT('Origin',(-0.00125952035885906,-0.0345589643248295,
0.0797577442985207));
#82561=CARTESIAN_POINT('',(0.0128467975774529,-0.034193496108874,0.0708704229420174));
#82562=CARTESIAN_POINT('Origin',(0.0218981057441369,-0.0341934220717705,
0.0645853582045632));
#82563=CARTESIAN_POINT('',(0.0128111500007457,-0.034193496108884,0.0708190858182845));
#82564=CARTESIAN_POINT('Ctrl Pts',(0.0131824969040118,-0.0340223579322397,
0.0709236389734332));
#82565=CARTESIAN_POINT('Ctrl Pts',(0.0131379969707527,-0.0339125849573575,
0.070853866103888));
#82566=CARTESIAN_POINT('Ctrl Pts',(0.0130920841708115,-0.0338030433565231,
0.0707850633081453));
#82567=CARTESIAN_POINT('Ctrl Pts',(0.0130448250186137,-0.0336938721132327,
0.0707173133685692));
#82568=CARTESIAN_POINT('Ctrl Pts',(0.0130705710636286,-0.0340223579322397,
0.0709059249652735));
#82569=CARTESIAN_POINT('Ctrl Pts',(0.0130258268079969,-0.0339125849573575,
0.070837695844982));
#82570=CARTESIAN_POINT('Ctrl Pts',(0.012979701809388,-0.0338030433565231,
0.0707704407706237));
#82571=CARTESIAN_POINT('Ctrl Pts',(0.0129322626781393,-0.0336938721132327,
0.0707042405212325));
#82572=CARTESIAN_POINT('Ctrl Pts',(0.0129586452232454,-0.0340223579322397,
0.0708882109571139));
#82573=CARTESIAN_POINT('Ctrl Pts',(0.0129136566452411,-0.0339125849573575,
0.0708215255860761));
#82574=CARTESIAN_POINT('Ctrl Pts',(0.0128673194479645,-0.0338030433565231,
0.0707558182331021));
#82575=CARTESIAN_POINT('Ctrl Pts',(0.0128197003376649,-0.0336938721132327,
0.0706911676738957));
#82576=CARTESIAN_POINT('Ctrl Pts',(0.0128467193828622,-0.0340223579322397,
0.0708704969489542));
#82577=CARTESIAN_POINT('Ctrl Pts',(0.0128014864824853,-0.0339125849573575,
0.0708053553271701));
#82578=CARTESIAN_POINT('Ctrl Pts',(0.012754937086541,-0.0338030433565231,
0.0707411956955805));
#82579=CARTESIAN_POINT('Ctrl Pts',(0.0127071379971904,-0.0336938721132327,
0.0706780948265589));
#82580=CARTESIAN_POINT('',(0.0128769889474301,-0.0336938721132427,0.0706978211003209));
#82581=CARTESIAN_POINT('Ctrl Pts',(0.0130521460683998,-0.0337108120662685,
0.0707278326379432));
#82582=CARTESIAN_POINT('Ctrl Pts',(0.0130168267382924,-0.0337611408993663,
0.070752357746438));
#82583=CARTESIAN_POINT('Ctrl Pts',(0.0129821519075985,-0.0338121088780013,
0.0707764353261151));
#82584=CARTESIAN_POINT('Ctrl Pts',(0.012914059656656,-0.0339153382773242,
0.0708237173622393));
#82585=CARTESIAN_POINT('Ctrl Pts',(0.0128806710437265,-0.0339675558473114,
0.0708469018154012));
#82586=CARTESIAN_POINT('Ctrl Pts',(0.012847913470025,-0.0340203938281305,
0.0708696480862567));
#82587=CARTESIAN_POINT('Ctrl Pts',(0.0127751424137356,-0.0341934961088741,
0.0707697446340297));
#82588=CARTESIAN_POINT('Ctrl Pts',(0.0127285306936894,-0.0340836138575045,
0.0707056051306595));
#82589=CARTESIAN_POINT('Ctrl Pts',(0.0126806141063763,-0.0339738896631393,
0.070642460934376));
#82590=CARTESIAN_POINT('Ctrl Pts',(0.012631459396656,-0.0338644633275951,
0.0705803887508831));
#82591=CARTESIAN_POINT('Ctrl Pts',(0.0127952572963795,-0.0341934961088741,
0.0706582253506043));
#82592=CARTESIAN_POINT('Ctrl Pts',(0.0127471077914455,-0.0340836138575045,
0.0705938084749125));
#82593=CARTESIAN_POINT('Ctrl Pts',(0.0126976484174645,-0.0339738896631393,
0.0705304188606276));
#82594=CARTESIAN_POINT('Ctrl Pts',(0.0126469479149285,-0.0338644633275951,
0.0704681333951926));
#82595=CARTESIAN_POINT('Ctrl Pts',(0.0128153721790234,-0.0341934961088741,
0.070546706067179));
#82596=CARTESIAN_POINT('Ctrl Pts',(0.0127656848892016,-0.0340836138575045,
0.0704820118191656));
#82597=CARTESIAN_POINT('Ctrl Pts',(0.0127146827285526,-0.0339738896631393,
0.0704183767868792));
#82598=CARTESIAN_POINT('Ctrl Pts',(0.012662436433201,-0.0338644633275951,
0.0703558780395021));
#82599=CARTESIAN_POINT('Ctrl Pts',(0.0128354870616673,-0.0341934961088741,
0.0704351867837537));
#82600=CARTESIAN_POINT('Ctrl Pts',(0.0127842619869577,-0.0340836138575045,
0.0703702151634186));
#82601=CARTESIAN_POINT('Ctrl Pts',(0.0127317170396408,-0.0339738896631393,
0.0703063347131308));
#82602=CARTESIAN_POINT('Ctrl Pts',(0.0126779249514735,-0.0338644633275951,
0.0702436226838116));
#82603=CARTESIAN_POINT('',(0.012827541403907,-0.0341764758832422,0.0704251309734487));
#82604=CARTESIAN_POINT('',(0.0128354870616674,-0.034193496108874,0.0704351867837538));
#82605=CARTESIAN_POINT('Origin',(-0.000470986983591591,-0.0345621026585572,
0.0803029075861101));
#82606=CARTESIAN_POINT('Ctrl Pts',(0.0128275414013896,-0.0341764758830167,
0.0704251309754324));
#82607=CARTESIAN_POINT('Ctrl Pts',(0.0127938903004274,-0.0341260048543041,
0.0704517790111985));
#82608=CARTESIAN_POINT('Ctrl Pts',(0.0127608244346899,-0.0340749271282664,
0.0704779636039045));
#82609=CARTESIAN_POINT('Ctrl Pts',(0.0126958363144475,-0.033971543441391,
0.0705294271727942));
#82610=CARTESIAN_POINT('Ctrl Pts',(0.0126639394902065,-0.0339192781018031,
0.0705546860109566));
#82611=CARTESIAN_POINT('Ctrl Pts',(0.0126326164764418,-0.0338664212856164,
0.0705794904532255));
#82612=CARTESIAN_POINT('',(0.0128054947428529,-0.0341934961088841,0.0706014677391527));
#82613=CARTESIAN_POINT('Origin',(0.00812378219310841,-0.0315241814719618,
0.07415));
#82614=CARTESIAN_POINT('',(0.0128275414041477,-0.0342105180190543,0.0704251309732576));
#82615=CARTESIAN_POINT('',(0.0128195742877287,-0.0341934961088739,0.070415092155874));
#82616=CARTESIAN_POINT('Origin',(-0.000447137499422179,-0.0345621714823014,
0.0803414515509757));
#82617=CARTESIAN_POINT('Origin',(0.000164846308348061,-0.0345621031779462,
0.0811058389789641));
#82618=CARTESIAN_POINT('Origin',(0.000132796574955342,-0.0345621721125304,
0.0810737889136887));
#82619=CARTESIAN_POINT('Ctrl Pts',(0.0127100840996449,-0.0346945769586966,
0.0706795047796305));
#82620=CARTESIAN_POINT('Ctrl Pts',(0.0126373931877438,-0.0345275153362944,
0.070583442849943));
#82621=CARTESIAN_POINT('Ctrl Pts',(0.0125616624149798,-0.0343603235965186,
0.0704896421359921));
#82622=CARTESIAN_POINT('Ctrl Pts',(0.0124831198825586,-0.034193496108874,
0.0703983767297546));
#82623=CARTESIAN_POINT('Ctrl Pts',(0.0126580393994472,-0.0346945769586966,
0.070613782807614));
#82624=CARTESIAN_POINT('Ctrl Pts',(0.0125839719145285,-0.0345275153362944,
0.0705188109750097));
#82625=CARTESIAN_POINT('Ctrl Pts',(0.0125068984952447,-0.0343603235965186,
0.0704261439320513));
#82626=CARTESIAN_POINT('Ctrl Pts',(0.0124270511639208,-0.034193496108874,
0.0703360523588014));
#82627=CARTESIAN_POINT('Ctrl Pts',(0.0126059946992497,-0.0346945769586966,
0.0705480608355949));
#82628=CARTESIAN_POINT('Ctrl Pts',(0.0125305506413133,-0.0345275153362944,
0.070454179100074));
#82629=CARTESIAN_POINT('Ctrl Pts',(0.0124521345755095,-0.0343603235965186,
0.0703626457281086));
#82630=CARTESIAN_POINT('Ctrl Pts',(0.012370982445283,-0.034193496108874,
0.0702737279878472));
#82631=CARTESIAN_POINT('Ctrl Pts',(0.0125539499990518,-0.0346945769586966,
0.070482338863581));
#82632=CARTESIAN_POINT('Ctrl Pts',(0.0124771293680981,-0.0345275153362944,
0.0703895472251431));
#82633=CARTESIAN_POINT('Ctrl Pts',(0.0123973706557744,-0.0343603235965186,
0.0702991475241697));
#82634=CARTESIAN_POINT('Ctrl Pts',(0.0123149137266452,-0.034193496108874,
0.0702114036168948));
#82635=CARTESIAN_POINT('',(0.0125539500000745,-0.0346945769586966,0.0704823388648728));
#82636=CARTESIAN_POINT('',(0.0123995251710299,-0.0343667727836525,0.0703034239916618));
#82637=CARTESIAN_POINT('Origin',(-0.000279821455984584,-0.0345626474180612,
0.0813447306597584));
#82638=CARTESIAN_POINT('Origin',(0.0206160592004556,-0.0341934771024245,
0.0629115888748403));
#82639=CARTESIAN_POINT('',(0.0124821166583467,-0.034193496108874,0.0703972615746475));
#82640=CARTESIAN_POINT('',(0.0124403159257087,-0.034193496108884,0.0703507970855277));
#82641=CARTESIAN_POINT('',(0.0126326164752049,-0.0345211942962658,0.0705794904542206));
#82642=CARTESIAN_POINT('Origin',(-0.000575707125566571,-0.0345625596120814,
0.0809657317445962));
#82643=CARTESIAN_POINT('',(0.012631551438155,-0.0346945769586885,0.0705803338484653));
#82644=CARTESIAN_POINT('Origin',(0.021304944390607,-0.0346945685853822,
0.0637119446714151));
#82645=CARTESIAN_POINT('',(0.0125927507191247,-0.0346945769587026,0.0705313363566791));
#82646=CARTESIAN_POINT('Ctrl Pts',(0.0129699292337307,-0.0345231616327842,
0.0706123653579376));
#82647=CARTESIAN_POINT('Ctrl Pts',(0.012921167920781,-0.0344132092796988,
0.0705455680438119));
#82648=CARTESIAN_POINT('Ctrl Pts',(0.0128710274739373,-0.034303273855898,
0.0704797827654166));
#82649=CARTESIAN_POINT('Ctrl Pts',(0.0128195742877331,-0.0341934961088739,
0.0704150921558742));
#82650=CARTESIAN_POINT('Ctrl Pts',(0.0128571121718725,-0.0345231616327842,
0.0706017142222049));
#82651=CARTESIAN_POINT('Ctrl Pts',(0.0128082040480123,-0.0344132092796988,
0.0705364719324432));
#82652=CARTESIAN_POINT('Ctrl Pts',(0.0127579489622852,-0.034303273855898,
0.0704722446348476));
#82653=CARTESIAN_POINT('Ctrl Pts',(0.0127064134049634,-0.0341934961088739,
0.0704091129628253));
#82654=CARTESIAN_POINT('Ctrl Pts',(0.0127442951100142,-0.0345231616327842,
0.0705910630864722));
#82655=CARTESIAN_POINT('Ctrl Pts',(0.0126952401752436,-0.0344132092796988,
0.0705273758210745));
#82656=CARTESIAN_POINT('Ctrl Pts',(0.0126448704506332,-0.034303273855898,
0.0704647065042788));
#82657=CARTESIAN_POINT('Ctrl Pts',(0.0125932525221938,-0.0341934961088739,
0.0704031337697765));
#82658=CARTESIAN_POINT('Ctrl Pts',(0.012631478048156,-0.0345231616327842,
0.0705804119507396));
#82659=CARTESIAN_POINT('Ctrl Pts',(0.0125822763024749,-0.0344132092796988,
0.0705182797097059));
#82660=CARTESIAN_POINT('Ctrl Pts',(0.0125317919389812,-0.034303273855898,
0.0704571683737098));
#82661=CARTESIAN_POINT('Ctrl Pts',(0.0124800916394241,-0.0341934961088739,
0.0703971545767276));
#82662=CARTESIAN_POINT('',(0.0126508454730477,-0.0341934961088839,0.0704061768652707));
#82663=CARTESIAN_POINT('Ctrl Pts',(0.0128275414014334,-0.034210518019539,
0.070425130975398));
#82664=CARTESIAN_POINT('Ctrl Pts',(0.012793852581739,-0.0342610556240575,
0.0704518088803242));
#82665=CARTESIAN_POINT('Ctrl Pts',(0.0127607682904933,-0.0343122189868655,
0.0704780080640417));
#82666=CARTESIAN_POINT('Ctrl Pts',(0.0126957797636824,-0.0344158119695142,
0.0705294719548897));
#82667=CARTESIAN_POINT('Ctrl Pts',(0.0126639021090382,-0.0344681990450031,
0.0705547156128029));
#82668=CARTESIAN_POINT('Ctrl Pts',(0.0126326164751746,-0.0345211942962439,
0.0705794904542292));
#82669=CARTESIAN_POINT('Ctrl Pts',(0.0125537160836053,-0.0346945769586932,
0.0704843529774302));
#82670=CARTESIAN_POINT('Ctrl Pts',(0.0124779314252381,-0.0345296777079064,
0.0703927672288805));
#82671=CARTESIAN_POINT('Ctrl Pts',(0.0123984262007714,-0.0343648066255586,
0.0703043919887749));
#82672=CARTESIAN_POINT('Ctrl Pts',(0.0125539500000802,-0.0346945769586932,
0.0704823388648798));
#82673=CARTESIAN_POINT('Ctrl Pts',(0.0124781237013612,-0.0345296777079064,
0.0703907482802726));
#82674=CARTESIAN_POINT('Ctrl Pts',(0.0123985766722452,-0.0343648066255586,
0.0703023699292757));
#82675=CARTESIAN_POINT('Ctrl Pts',(0.0125929345365957,-0.0346945769586932,
0.0701466667225046));
#82676=CARTESIAN_POINT('Ctrl Pts',(0.0125101684538558,-0.0345296777079064,
0.0700542701601905));
#82677=CARTESIAN_POINT('Ctrl Pts',(0.0124236542588785,-0.0343648066255586,
0.069965373347835));
#82678=CARTESIAN_POINT('',(0.0125843731496633,-0.0346775396664998,0.0701371296667152));
#82679=CARTESIAN_POINT('',(0.0125929345365934,-0.0346945769586886,0.070146666722502));
#82680=CARTESIAN_POINT('Origin',(0.000344881563629885,-0.0345626617441152,
0.0813535348122937));
#82681=CARTESIAN_POINT('Ctrl Pts',(0.0125843731499848,-0.0346775396670096,
0.0701371296685037));
#82682=CARTESIAN_POINT('Ctrl Pts',(0.012552436677156,-0.034626974992875,
0.0701658606153561));
#82683=CARTESIAN_POINT('Ctrl Pts',(0.0125210678107356,-0.0345757902891939,
0.0701940809758775));
#82684=CARTESIAN_POINT('Ctrl Pts',(0.012459439341323,-0.0344721681090197,
0.0702495236372595));
#82685=CARTESIAN_POINT('Ctrl Pts',(0.0124292038958194,-0.0344197714292389,
0.0702767241977988));
#82686=CARTESIAN_POINT('Ctrl Pts',(0.0123995251716564,-0.0343667727834209,
0.0703034239918986));
#82687=CARTESIAN_POINT('',(0.0125734422683439,-0.0346945769587026,0.0703145027936974));
#82688=CARTESIAN_POINT('Origin',(0.00812378219310841,-0.0315241814719618,
0.07415));
#82689=CARTESIAN_POINT('',(0.0125843731482918,-0.034711613648962,0.0701371296669554));
#82690=CARTESIAN_POINT('',(0.0125757914107549,-0.0346945769586885,0.070127610918123));
#82691=CARTESIAN_POINT('Origin',(0.000376550837136767,-0.0345626695995449,
0.08138594164082));
#82692=CARTESIAN_POINT('Origin',(0.000140603155004497,-0.0345626624283481,
0.0811264668912053));
#82693=CARTESIAN_POINT('Origin',(0.00011171584856058,-0.0345626699717168,
0.0810915567704016));
#82694=CARTESIAN_POINT('Ctrl Pts',(0.012507262090966,-0.0352450361874069,
0.0704265786417996));
#82695=CARTESIAN_POINT('Ctrl Pts',(0.0123668309500735,-0.0349452760959493,
0.0702612529845839));
#82696=CARTESIAN_POINT('Ctrl Pts',(0.0122143457543109,-0.034644428984174,
0.0701069748482866));
#82697=CARTESIAN_POINT('Ctrl Pts',(0.0125055851568032,-0.0352450361874069,
0.0704246909138495));
#82698=CARTESIAN_POINT('Ctrl Pts',(0.0123650828190828,-0.0349452760959493,
0.0702594285032436));
#82699=CARTESIAN_POINT('Ctrl Pts',(0.0122125313927483,-0.034644428984174,
0.0701052187967155));
#82700=CARTESIAN_POINT('Ctrl Pts',(0.0123395520713741,-0.0352450361874069,
0.0702377871564155));
#82701=CARTESIAN_POINT('Ctrl Pts',(0.0121920005427703,-0.0349452760959493,
0.0700787867863819));
#82702=CARTESIAN_POINT('Ctrl Pts',(0.0120328916340797,-0.034644428984174,
0.0699313523045283));
#82703=CARTESIAN_POINT('Ctrl Pts',(0.0123378917405198,-0.0352450361874069,
0.0702359181188412));
#82704=CARTESIAN_POINT('Ctrl Pts',(0.0121902697200072,-0.0349452760959493,
0.0700769803692133));
#82705=CARTESIAN_POINT('Ctrl Pts',(0.012031095236493,-0.034644428984174,
0.0699296136396064));
#82706=CARTESIAN_POINT('',(0.0123149376169544,-0.0351951634053344,0.0702114255731725));
#82707=CARTESIAN_POINT('',(0.0121495594633167,-0.0348678972925434,0.0700425382082514));
#82708=CARTESIAN_POINT('Origin',(0.000726994801887408,-0.0345636767881071,
0.0822996048271035));
#82709=CARTESIAN_POINT('Origin',(0.0198841147875398,-0.0346946199340696,
0.0621510463800824));
#82710=CARTESIAN_POINT('',(0.0122378800979282,-0.0346945769330288,0.070131004674344));
#82711=CARTESIAN_POINT('',(0.012193244314101,-0.0346945769458128,0.0700872565556455));
#82712=CARTESIAN_POINT('',(0.0123995251713416,-0.0350221583435276,0.07030342399216));
#82713=CARTESIAN_POINT('Origin',(0.000355882459382666,-0.0345628458716893,
0.0819939595706483));
#82714=CARTESIAN_POINT('',(0.0123986076547722,-0.0351951360298763,0.0703042534836261));
#82715=CARTESIAN_POINT('Origin',(0.020590464340695,-0.0351951838366766,
0.0629346315196116));
#82716=CARTESIAN_POINT('',(0.0123149137278407,-0.0351951371328748,0.0702114036180501));
#82717=CARTESIAN_POINT('Ctrl Pts',(0.0127382359384145,-0.0350241211494343,
0.0703150532425499));
#82718=CARTESIAN_POINT('Ctrl Pts',(0.01268541111922,-0.0349144232818962,
0.0702514910342081));
#82719=CARTESIAN_POINT('Ctrl Pts',(0.0126312408055594,-0.0348045283579412,
0.07018898270758));
#82720=CARTESIAN_POINT('Ctrl Pts',(0.0125757914033085,-0.0346945769439157,
0.0701276109098772));
#82721=CARTESIAN_POINT('Ctrl Pts',(0.0126249726793622,-0.0350241211494343,
0.0703115069836799));
#82722=CARTESIAN_POINT('Ctrl Pts',(0.0125720990119058,-0.0349144232818962,
0.0702495049302917));
#82723=CARTESIAN_POINT('Ctrl Pts',(0.012517912070263,-0.0348045283579412,
0.0701885587021738));
#82724=CARTESIAN_POINT('Ctrl Pts',(0.0124624783560641,-0.0346945769439157,
0.0701287489464803));
#82725=CARTESIAN_POINT('Ctrl Pts',(0.0125117094203098,-0.0350241211494343,
0.0703079607248099));
#82726=CARTESIAN_POINT('Ctrl Pts',(0.0124587869045915,-0.0349144232818962,
0.0702475188263754));
#82727=CARTESIAN_POINT('Ctrl Pts',(0.0124045833349665,-0.0348045283579412,
0.0701881346967676));
#82728=CARTESIAN_POINT('Ctrl Pts',(0.0123491653088197,-0.0346945769439157,
0.0701298869830835));
#82729=CARTESIAN_POINT('Ctrl Pts',(0.0123984461612575,-0.0350241211494343,
0.0703044144659399));
#82730=CARTESIAN_POINT('Ctrl Pts',(0.0123454747972773,-0.0349144232818962,
0.0702455327224591));
#82731=CARTESIAN_POINT('Ctrl Pts',(0.0122912545996701,-0.0348045283579412,
0.0701877106913614));
#82732=CARTESIAN_POINT('Ctrl Pts',(0.0122358522615753,-0.0346945769439157,
0.0701310250196867));
#82733=CARTESIAN_POINT('',(0.0124068357546108,-0.0346945769458128,0.0701293077963898));
#82734=CARTESIAN_POINT('Ctrl Pts',(0.0125843731458412,-0.03471161364928,
0.0701371296691506));
#82735=CARTESIAN_POINT('Ctrl Pts',(0.0125524493470817,-0.0347621546531611,
0.0701658491967306));
#82736=CARTESIAN_POINT('Ctrl Pts',(0.0125210868549705,-0.0348133084095595,
0.0701940637574084));
#82737=CARTESIAN_POINT('Ctrl Pts',(0.0124594583097403,-0.0349168561544576,
0.0702495064920837));
#82738=CARTESIAN_POINT('Ctrl Pts',(0.0124292167016644,-0.0349692089015923,
0.070276712674648));
#82739=CARTESIAN_POINT('Ctrl Pts',(0.0123995251713011,-0.0350221583435,
0.0703034239921697));
#82740=CARTESIAN_POINT('Ctrl Pts',(0.0123148365325578,-0.0351951371254972,
0.0702128645974501));
#82741=CARTESIAN_POINT('Ctrl Pts',(0.0122334387283513,-0.0350307338980977,
0.0701262171785373));
#82742=CARTESIAN_POINT('Ctrl Pts',(0.0121485292467718,-0.0348659306897838,
0.0700430080584134));
#82743=CARTESIAN_POINT('Ctrl Pts',(0.0123149137277612,-0.0351951371254972,
0.0702114036181352));
#82744=CARTESIAN_POINT('Ctrl Pts',(0.012233485718724,-0.0350307338980977,
0.07012475460326));
#82745=CARTESIAN_POINT('Ctrl Pts',(0.0121485459921608,-0.0348659306897838,
0.0700415451369357));
#82746=CARTESIAN_POINT('Ctrl Pts',(0.0123278517243137,-0.0351951371254972,
0.0699665419621991));
#82747=CARTESIAN_POINT('Ctrl Pts',(0.0122413613541713,-0.0350307338980977,
0.0698796254623627));
#82748=CARTESIAN_POINT('Ctrl Pts',(0.0121513525368188,-0.0348659306897838,
0.0697963579724886));
#82749=CARTESIAN_POINT('Origin',(0.015872126049036,-0.0308609197384878,
0.0662444393516408));
#82750=CARTESIAN_POINT('',(0.0123205544025452,-0.0351951371254972,0.0701046494570405));
#82751=CARTESIAN_POINT('Origin',(0.00754815852817955,-0.0351840467441105,
0.0749395587671898));
#82752=CARTESIAN_POINT('Origin',(0.0159131566122411,-0.0352322613691046,
0.0650672331811612));
#82753=CARTESIAN_POINT('',(0.0119771554157214,-0.0351951142564674,0.0698804181246087));
#82754=CARTESIAN_POINT('',(0.0118828176741158,-0.0351951372916787,0.0697988906871318));
#82755=CARTESIAN_POINT('Origin',(0.00778760626108306,-0.03528751189993,
0.0740954534426918));
#82756=CARTESIAN_POINT('Origin',(0.0127572303630695,-0.0298325076523433,
0.0800513852894583));
#82757=CARTESIAN_POINT('Origin',(0.0155875963746084,-0.033873220915644,
0.0703365895131585));
#82758=CARTESIAN_POINT('Ctrl Pts',(0.0137509251183969,-0.0321934096636942,
0.0729611357336992));
#82759=CARTESIAN_POINT('Ctrl Pts',(0.0137296450141914,-0.0320508460845377,
0.0728604125550963));
#82760=CARTESIAN_POINT('Ctrl Pts',(0.0137056747221907,-0.0319086045665171,
0.0727603370765129));
#82761=CARTESIAN_POINT('Ctrl Pts',(0.0136790835943085,-0.0317669892871035,
0.0726611205290178));
#82762=CARTESIAN_POINT('Ctrl Pts',(0.0137318134523105,-0.0321934096636942,
0.0728794951993604));
#82763=CARTESIAN_POINT('Ctrl Pts',(0.0137090720214192,-0.0320508460845377,
0.0727791141104791));
#82764=CARTESIAN_POINT('Ctrl Pts',(0.0136836506958537,-0.0319086045665171,
0.0726794197266451));
#82765=CARTESIAN_POINT('Ctrl Pts',(0.0136556218843043,-0.0317669892871035,
0.0725806222011489));
#82766=CARTESIAN_POINT('Ctrl Pts',(0.0137127017862241,-0.0321934096636942,
0.0727978546650216));
#82767=CARTESIAN_POINT('Ctrl Pts',(0.013688499028647,-0.0320508460845377,
0.0726978156658619));
#82768=CARTESIAN_POINT('Ctrl Pts',(0.0136616266695168,-0.0319086045665171,
0.0725985023767772));
#82769=CARTESIAN_POINT('Ctrl Pts',(0.0136321601743,-0.0317669892871035,
0.0725001238732799));
#82770=CARTESIAN_POINT('Ctrl Pts',(0.0136935901201377,-0.0321934096636942,
0.0727162141306828));
#82771=CARTESIAN_POINT('Ctrl Pts',(0.0136679260358748,-0.0320508460845377,
0.0726165172212447));
#82772=CARTESIAN_POINT('Ctrl Pts',(0.0136396026431798,-0.0319086045665171,
0.0725175850269093));
#82773=CARTESIAN_POINT('Ctrl Pts',(0.0136086984642957,-0.0317669892871035,
0.0724196255454111));
#82774=CARTESIAN_POINT('',(0.0136939320316184,-0.0321934096636942,0.0727176746959757));
#82775=CARTESIAN_POINT('',(0.013630382515873,-0.0318665617511334,0.0724900367851861));
#82776=CARTESIAN_POINT('Origin',(-0.00263158734375825,-0.0326371944422963,
0.076280724228609));
#82777=CARTESIAN_POINT('Origin',(0.0241250974477546,-0.0316939261509355,
0.0693264077590119));
#82778=CARTESIAN_POINT('',(0.0137236408735195,-0.0320197221621819,0.0728388280334148));
#82779=CARTESIAN_POINT('Ctrl Pts',(0.0137236460388813,-0.0320197392094732,
0.0728386431329055));
#82780=CARTESIAN_POINT('Ctrl Pts',(0.0137169733878477,-0.0319792716576029,
0.0728101492360508));
#82781=CARTESIAN_POINT('Ctrl Pts',(0.0137100531343661,-0.0319386439829723,
0.0727815764937398));
#82782=CARTESIAN_POINT('Ctrl Pts',(0.0137028697936117,-0.0318979099381655,
0.0727528969008297));
#82783=CARTESIAN_POINT('Ctrl Pts',(0.0136956865948412,-0.0318571766984958,
0.0727242178747919));
#82784=CARTESIAN_POINT('Ctrl Pts',(0.013688278557203,-0.0318163871833608,
0.072695577335032));
#82785=CARTESIAN_POINT('Ctrl Pts',(0.0136806745702592,-0.0317755399638303,
0.0726670729114552));
#82786=CARTESIAN_POINT('',(0.0137224236774251,-0.0321934096636183,0.0728393842935138));
#82787=CARTESIAN_POINT('Origin',(0.0159646654076172,-0.0324111993426145,
0.0722928894874314));
#82788=CARTESIAN_POINT('',(0.0137081778545317,-0.0321934096636662,0.0727785294947547));
#82789=CARTESIAN_POINT('Ctrl Pts',(0.0136928625085267,-0.0321934096636618,
0.0727193980089872));
#82790=CARTESIAN_POINT('Ctrl Pts',(0.0136731333921247,-0.0320835708272592,
0.0726425960511502));
#82791=CARTESIAN_POINT('Ctrl Pts',(0.0136518263068861,-0.0319739230346489,
0.0725662469346086));
#82792=CARTESIAN_POINT('Ctrl Pts',(0.0136289760106762,-0.0318646057455573,
0.0724904462505591));
#82793=CARTESIAN_POINT('Ctrl Pts',(0.0137526178529808,-0.0321934096636618,
0.0726231147623967));
#82794=CARTESIAN_POINT('Ctrl Pts',(0.0137315609155695,-0.0320835708272592,
0.0725454887317892));
#82795=CARTESIAN_POINT('Ctrl Pts',(0.0137089097253686,-0.0319739230346489,
0.0724683434996594));
#82796=CARTESIAN_POINT('Ctrl Pts',(0.0136847008381052,-0.0318646057455573,
0.0723917755437976));
#82797=CARTESIAN_POINT('Ctrl Pts',(0.0138123731974348,-0.0321934096636618,
0.0725268315158063));
#82798=CARTESIAN_POINT('Ctrl Pts',(0.0137899884390143,-0.0320835708272592,
0.0724483814124281));
#82799=CARTESIAN_POINT('Ctrl Pts',(0.0137659931438512,-0.0319739230346489,
0.0723704400647102));
#82800=CARTESIAN_POINT('Ctrl Pts',(0.0137404256655343,-0.0318646057455573,
0.0722931048370361));
#82801=CARTESIAN_POINT('Ctrl Pts',(0.0138721285418889,-0.0321934096636618,
0.0724305482692159));
#82802=CARTESIAN_POINT('Ctrl Pts',(0.0138484159624591,-0.0320835708272592,
0.0723512740930671));
#82803=CARTESIAN_POINT('Ctrl Pts',(0.0138230765623337,-0.0319739230346489,
0.072272536629761));
#82804=CARTESIAN_POINT('Ctrl Pts',(0.0137961504929634,-0.0318646057455573,
0.0721944341302745));
#82805=CARTESIAN_POINT('',(0.0138684426467717,-0.0321763980308286,0.0724182736215178));
#82806=CARTESIAN_POINT('',(0.0138721285418775,-0.0321934096636184,0.0724305482691878));
#82807=CARTESIAN_POINT('Origin',(-0.00214121275700354,-0.0326386231564428,
0.0766036082940997));
#82808=CARTESIAN_POINT('Ctrl Pts',(0.0138684426437268,-0.0321763980306299,
0.0724182736224286));
#82809=CARTESIAN_POINT('Ctrl Pts',(0.013827350232142,-0.0321259596175181,
0.0724306609190619));
#82810=CARTESIAN_POINT('Ctrl Pts',(0.01378696979991,-0.0320749164632105,
0.0724428335897142));
#82811=CARTESIAN_POINT('Ctrl Pts',(0.0137076003971833,-0.0319716057793985,
0.0724667594752309));
#82812=CARTESIAN_POINT('Ctrl Pts',(0.0136686423517508,-0.0319193786690198,
0.0724785033677434));
#82813=CARTESIAN_POINT('Ctrl Pts',(0.0136303825140914,-0.0318665617525393,
0.0724900367857141));
#82814=CARTESIAN_POINT('',(0.0137830302867579,-0.0321934096636663,0.0725741114825918));
#82815=CARTESIAN_POINT('Origin',(0.00812378219310841,-0.0315241814719618,
0.07415));
#82816=CARTESIAN_POINT('',(0.0138684426471269,-0.032210423332377,0.0724182736214106));
#82817=CARTESIAN_POINT('',(0.0138647305447439,-0.0321934096636183,0.0724060068739045));
#82818=CARTESIAN_POINT('Origin',(-0.00213430260582455,-0.0326387241818522,
0.0766484115498298));
#82819=CARTESIAN_POINT('Origin',(-0.00178707430780203,-0.0326386237460637,
0.0777783976214467));
#82820=CARTESIAN_POINT('Origin',(-0.00180607434721047,-0.032638724687269,
0.0777372387427542));
#82821=CARTESIAN_POINT('Ctrl Pts',(0.0136747273595271,-0.0327445246967096,
0.0726449641999562));
#82822=CARTESIAN_POINT('Ctrl Pts',(0.0136179640063733,-0.0324436878339359,
0.0724356068804763));
#82823=CARTESIAN_POINT('Ctrl Pts',(0.0135455922629537,-0.0321434074405927,
0.072231119970784));
#82824=CARTESIAN_POINT('Ctrl Pts',(0.0136040777686263,-0.0327445246967096,
0.0724051546186098));
#82825=CARTESIAN_POINT('Ctrl Pts',(0.0135382698492535,-0.0324436878339359,
0.0721984618920109));
#82826=CARTESIAN_POINT('Ctrl Pts',(0.0134570799422983,-0.0321434074405927,
0.0719973132790659));
#82827=CARTESIAN_POINT('',(0.0135930041633336,-0.0326943950436612,0.0723707484606142));
#82828=CARTESIAN_POINT('',(0.0135152865462182,-0.0323666188837389,0.0721475500479665));
#82829=CARTESIAN_POINT('Origin',(-0.00236959641976738,-0.0326395579112551,
0.077643645278268));
#82830=CARTESIAN_POINT('Origin',(0.0238688493646319,-0.0321933825603049,
0.0683021490546249));
#82831=CARTESIAN_POINT('',(0.01355753425258,-0.0321934096532689,0.0722652019861543));
#82832=CARTESIAN_POINT('',(0.0135357736329072,-0.0321934096584275,0.0722066125180125));
#82833=CARTESIAN_POINT('',(0.0136303825167703,-0.0325210109756239,0.0724900367849113));
#82834=CARTESIAN_POINT('Origin',(-0.00249400463831448,-0.0326393129156579,
0.077179202574978));
#82835=CARTESIAN_POINT('',(0.0136290817962303,-0.0326943950436593,0.0724904288867702));
#82836=CARTESIAN_POINT('Origin',(0.0242207569404267,-0.0326943765538118,
0.0692975721206675));
#82837=CARTESIAN_POINT('',(0.013611042979792,-0.0326943950436702,0.0724305886737022));
#82838=CARTESIAN_POINT('Ctrl Pts',(0.0139319059659176,-0.0325229783203769,
0.0726447763489058));
#82839=CARTESIAN_POINT('Ctrl Pts',(0.0139111564908043,-0.032413025309245,
0.0725647114897128));
#82840=CARTESIAN_POINT('Ctrl Pts',(0.0138887539182925,-0.032303122220807,
0.0724850880034719));
#82841=CARTESIAN_POINT('Ctrl Pts',(0.0138647305434476,-0.0321934096576658,
0.0724060068696172));
#82842=CARTESIAN_POINT('Ctrl Pts',(0.0138309322364644,-0.0325229783203769,
0.0725933424282199));
#82843=CARTESIAN_POINT('Ctrl Pts',(0.0138094737458793,-0.032413025309245,
0.0725146694896793));
#82844=CARTESIAN_POINT('Ctrl Pts',(0.0137863910590984,-0.032303122220807,
0.0724364523798745));
#82845=CARTESIAN_POINT('Ctrl Pts',(0.0137617172787974,-0.0321934096576658,
0.0723587902460305));
#82846=CARTESIAN_POINT('Ctrl Pts',(0.0137299585070112,-0.0325229783203769,
0.072541908507534));
#82847=CARTESIAN_POINT('Ctrl Pts',(0.0137077910009542,-0.032413025309245,
0.0724646274896458));
#82848=CARTESIAN_POINT('Ctrl Pts',(0.0136840281999043,-0.032303122220807,
0.0723878167562771));
#82849=CARTESIAN_POINT('Ctrl Pts',(0.0136587040141473,-0.0321934096576658,
0.0723115736224438));
#82850=CARTESIAN_POINT('Ctrl Pts',(0.013628984777558,-0.0325229783203769,
0.0724904745868481));
#82851=CARTESIAN_POINT('Ctrl Pts',(0.0136061082560291,-0.032413025309245,
0.0724145854896122));
#82852=CARTESIAN_POINT('Ctrl Pts',(0.0135816653407102,-0.032303122220807,
0.0723391811326797));
#82853=CARTESIAN_POINT('Ctrl Pts',(0.0135556907494971,-0.0321934096576658,
0.0722643569988571));
#82854=CARTESIAN_POINT('',(0.0137111323989621,-0.0321934096584275,0.0723356044304525));
#82855=CARTESIAN_POINT('Ctrl Pts',(0.0138684426437907,-0.0322104233328904,
0.0724182736224094));
#82856=CARTESIAN_POINT('Ctrl Pts',(0.013827294551371,-0.032260942183044,
0.0724306777040157));
#82857=CARTESIAN_POINT('Ctrl Pts',(0.0137868869181465,-0.0323120888238839,
0.0724428585743929));
#82858=CARTESIAN_POINT('Ctrl Pts',(0.0137075169143957,-0.0324156524631812,
0.0724667846410882));
#82859=CARTESIAN_POINT('Ctrl Pts',(0.0136685871693151,-0.0324680267167316,
0.0724785200024743));
#82860=CARTESIAN_POINT('Ctrl Pts',(0.0136303825167275,-0.0325210109755912,
0.0724900367849197));
#82861=CARTESIAN_POINT('Origin',(0.00947084381705225,-0.0262834582511158,
0.0819016972865226));
#82862=CARTESIAN_POINT('Origin',(0.0201046183452919,-0.0342770676166929,
0.0762193053832568));
#82863=CARTESIAN_POINT('Ctrl Pts',(0.013592045191167,-0.0326943950436604,
0.0723725350952205));
#82864=CARTESIAN_POINT('Ctrl Pts',(0.0135675483934548,-0.0325844576448134,
0.0722971721824901));
#82865=CARTESIAN_POINT('Ctrl Pts',(0.0135414912334718,-0.0324744968375322,
0.0722223105701491));
#82866=CARTESIAN_POINT('Ctrl Pts',(0.0135139084201555,-0.0323646534831894,
0.0721480457147681));
#82867=CARTESIAN_POINT('Ctrl Pts',(0.0136456368694318,-0.0326943950436604,
0.0722726899170576));
#82868=CARTESIAN_POINT('Ctrl Pts',(0.0136197640180347,-0.0325844576448134,
0.0721965884105592));
#82869=CARTESIAN_POINT('Ctrl Pts',(0.0135923154316513,-0.0324744968375322,
0.072121016611225));
#82870=CARTESIAN_POINT('Ctrl Pts',(0.0135633276145464,-0.0323646534831894,
0.0720460708609689));
#82871=CARTESIAN_POINT('Ctrl Pts',(0.0136992285476966,-0.0326943950436604,
0.0721728447388946));
#82872=CARTESIAN_POINT('Ctrl Pts',(0.0136719796426146,-0.0325844576448134,
0.0720960046386282));
#82873=CARTESIAN_POINT('Ctrl Pts',(0.0136431396298308,-0.0324744968375322,
0.0720197226523008));
#82874=CARTESIAN_POINT('Ctrl Pts',(0.0136127468089373,-0.0323646534831894,
0.0719440960071696));
#82875=CARTESIAN_POINT('Ctrl Pts',(0.0137528202259614,-0.0326943950436604,
0.0720729995607317));
#82876=CARTESIAN_POINT('Ctrl Pts',(0.0137241952671946,-0.0325844576448134,
0.0719954208666973));
#82877=CARTESIAN_POINT('Ctrl Pts',(0.0136939638280103,-0.0324744968375322,
0.0719184286933768));
#82878=CARTESIAN_POINT('Ctrl Pts',(0.0136621660033283,-0.0323646534831894,
0.0718421211533704));
#82879=CARTESIAN_POINT('',(0.0137483708728123,-0.0326773559991177,0.0720609805734748));
#82880=CARTESIAN_POINT('',(0.0137528202259598,-0.0326943950436594,0.0720729995607336));
#82881=CARTESIAN_POINT('Origin',(-0.00180032032256985,-0.0326395670310402,
0.0778894890183537));
#82882=CARTESIAN_POINT('Ctrl Pts',(0.0137483708696632,-0.0326773559987436,
0.0720609805746371));
#82883=CARTESIAN_POINT('Ctrl Pts',(0.0137081049721412,-0.0326267922586234,
0.0720759356668118));
#82884=CARTESIAN_POINT('Ctrl Pts',(0.0136685527585761,-0.032575610957988,
0.0720906256907771));
#82885=CARTESIAN_POINT('Ctrl Pts',(0.0135908420383873,-0.032471998546237,
0.0721194881042563));
#82886=CARTESIAN_POINT('Ctrl Pts',(0.0135527146994713,-0.0324196091621772,
0.0721336489178222));
#82887=CARTESIAN_POINT('Ctrl Pts',(0.0135152865461725,-0.0323666188837756,
0.0721475500479834));
#82888=CARTESIAN_POINT('',(0.0136729121946567,-0.0326943950436702,0.0722218740106839));
#82889=CARTESIAN_POINT('Origin',(0.00812378219310841,-0.0315241814719618,
0.07415));
#82890=CARTESIAN_POINT('',(0.0137483708727707,-0.0327114338380042,0.0720609805734901));
#82891=CARTESIAN_POINT('',(0.0137438958601232,-0.0326943950436593,0.0720489711163711));
#82892=CARTESIAN_POINT('Origin',(-0.00178381914769819,-0.0326395676808559,
0.0779316872169131));
#82893=CARTESIAN_POINT('Origin',(-0.00183530563046278,-0.0326395675415347,
0.0777952954196774));
#82894=CARTESIAN_POINT('Origin',(-0.0018503487587794,-0.0326395682909456,
0.0777525558319516));
#82895=CARTESIAN_POINT('Ctrl Pts',(0.013569259236313,-0.0332451089994433,
0.0722993501757676));
#82896=CARTESIAN_POINT('Ctrl Pts',(0.0134994608362305,-0.0329451141710254,
0.0720939706488981));
#82897=CARTESIAN_POINT('Ctrl Pts',(0.0134143907004741,-0.0326442513127493,
0.071894432084421));
#82898=CARTESIAN_POINT('Ctrl Pts',(0.0134836896860458,-0.0332451089994433,
0.0720644505119385));
#82899=CARTESIAN_POINT('Ctrl Pts',(0.0134050319001948,-0.0329451141710254,
0.0718622982934587));
#82900=CARTESIAN_POINT('Ctrl Pts',(0.0133113706413111,-0.0326442513127493,
0.0716666451940825));
#82901=CARTESIAN_POINT('Ctrl Pts',(0.0134828339905431,-0.0332451089994433,
0.0720621015153002));
#82902=CARTESIAN_POINT('Ctrl Pts',(0.0134040876108344,-0.0329451141710254,
0.0718599815699044));
#82903=CARTESIAN_POINT('Ctrl Pts',(0.0133103404407195,-0.0326442513127493,
0.0716643673251791));
#82904=CARTESIAN_POINT('',(0.0134704917745687,-0.0331951640388616,0.0720308441181636));
#82905=CARTESIAN_POINT('',(0.0133789127710123,-0.0328677532355027,0.0718129660509484));
#82906=CARTESIAN_POINT('Origin',(-0.00181472275481337,-0.0326402808281768,
0.0789152078698814));
#82907=CARTESIAN_POINT('Origin',(0.02348081544725,-0.0326944278779034,0.0673200888768139));
#82908=CARTESIAN_POINT('',(0.0134284645353448,-0.0326943950436593,0.071927733083546));
#82909=CARTESIAN_POINT('',(0.0134030679929601,-0.0326943950436694,0.0718706255916273));
#82910=CARTESIAN_POINT('',(0.0135152865462192,-0.0330220786163545,0.0721475500479691));
#82911=CARTESIAN_POINT('Origin',(-0.00203837613684075,-0.0326396682761693,
0.0784896120410405));
#82912=CARTESIAN_POINT('',(0.013514013012634,-0.0331951640388587,0.0721480230490247));
#82913=CARTESIAN_POINT('Origin',(0.0238554318344169,-0.0331952026560145,
0.0683071343098413));
#82914=CARTESIAN_POINT('',(0.0134922523936113,-0.0331951640388701,0.0720894335836041));
#82915=CARTESIAN_POINT('Ctrl Pts',(0.0138259308863425,-0.0330240426238172,
0.072283050541571));
#82916=CARTESIAN_POINT('Ctrl Pts',(0.0138002118386719,-0.0329142774063519,
0.0722044978879874));
#82917=CARTESIAN_POINT('Ctrl Pts',(0.0137728560663424,-0.0328043479726691,
0.0721264377575992));
#82918=CARTESIAN_POINT('Ctrl Pts',(0.0137438958601305,-0.0326943950436593,
0.072048971116374));
#82919=CARTESIAN_POINT('Ctrl Pts',(0.0137219268609901,-0.0330240426238172,
0.0722380583345183));
#82920=CARTESIAN_POINT('Ctrl Pts',(0.0136955880018336,-0.0329142774063519,
0.0721609384377102));
#82921=CARTESIAN_POINT('Ctrl Pts',(0.0136676417281043,-0.0328043479726691,
0.0720843245916136));
#82922=CARTESIAN_POINT('Ctrl Pts',(0.0136381211380807,-0.0326943950436593,
0.0720083159302318));
#82923=CARTESIAN_POINT('Ctrl Pts',(0.0136179228356377,-0.0330240426238172,
0.0721930661274656));
#82924=CARTESIAN_POINT('Ctrl Pts',(0.0135909641649953,-0.0329142774063519,
0.0721173789874329));
#82925=CARTESIAN_POINT('Ctrl Pts',(0.0135624273898662,-0.0328043479726691,
0.0720422114256281));
#82926=CARTESIAN_POINT('Ctrl Pts',(0.0135323464160309,-0.0326943950436593,
0.0719676607440896));
#82927=CARTESIAN_POINT('Ctrl Pts',(0.0135139188102854,-0.0330240426238172,
0.0721480739204129));
#82928=CARTESIAN_POINT('Ctrl Pts',(0.013486340328157,-0.0329142774063519,
0.0720738195371556));
#82929=CARTESIAN_POINT('Ctrl Pts',(0.0134572130516281,-0.0328043479726691,
0.0720000982596426));
#82930=CARTESIAN_POINT('Ctrl Pts',(0.0134265716939811,-0.0326943950436593,
0.0719270055579474));
#82931=CARTESIAN_POINT('',(0.013586180197744,-0.0326943950436693,0.0719883520999685));
#82932=CARTESIAN_POINT('Ctrl Pts',(0.0137483708696573,-0.0327114338383302,
0.0720609805746394));
#82933=CARTESIAN_POINT('Ctrl Pts',(0.0137081116697189,-0.0327619876830128,
0.0720759331792754));
#82934=CARTESIAN_POINT('Ctrl Pts',(0.013668562727585,-0.0328131562602624,
0.0720906219882037));
#82935=CARTESIAN_POINT('Ctrl Pts',(0.0135908520786755,-0.0329167375858768,
0.0721194843752092));
#82936=CARTESIAN_POINT('Ctrl Pts',(0.0135527213360146,-0.032969108892062,
0.0721336464529543));
#82937=CARTESIAN_POINT('Ctrl Pts',(0.0135152865461737,-0.0330220786163187,
0.0721475500479831));
#82938=CARTESIAN_POINT('Ctrl Pts',(0.0134696467435439,-0.0331951640388604,
0.0720326877358995));
#82939=CARTESIAN_POINT('Ctrl Pts',(0.013425872669978,-0.0330306422010619,
0.0719221654137687));
#82940=CARTESIAN_POINT('Ctrl Pts',(0.0133775679972495,-0.0328657861914645,
0.0718135467606821));
#82941=CARTESIAN_POINT('Ctrl Pts',(0.0134704917745698,-0.0331951640388604,
0.0720308441181666));
#82942=CARTESIAN_POINT('Ctrl Pts',(0.0134266795853892,-0.0330306422010619,
0.0719203043255611));
#82943=CARTESIAN_POINT('Ctrl Pts',(0.0133783361075426,-0.0328657861914645,
0.0718116697922867));
#82944=CARTESIAN_POINT('Ctrl Pts',(0.0136112966685905,-0.0331951640388604,
0.071723647824121));
#82945=CARTESIAN_POINT('Ctrl Pts',(0.0135611333929865,-0.0330306422010619,
0.0716101969806073));
#82946=CARTESIAN_POINT('Ctrl Pts',(0.0135063239388799,-0.0328657861914645,
0.0714989163809781));
#82947=CARTESIAN_POINT('',(0.0136061014182251,-0.0331781648281936,0.0717119319308448));
#82948=CARTESIAN_POINT('',(0.0136112966685892,-0.0331951640388588,0.0717236478241218));
#82949=CARTESIAN_POINT('Origin',(-0.00118719467340796,-0.0326412092817283,
0.0790702521208667));
#82950=CARTESIAN_POINT('Ctrl Pts',(0.0136061014178578,-0.033178164828644,
0.0717119319326457));
#82951=CARTESIAN_POINT('Ctrl Pts',(0.0135668269985692,-0.0331276811546773,
0.0717293978583441));
#82952=CARTESIAN_POINT('Ctrl Pts',(0.0135282617674078,-0.033076566349778,
0.0717465484344126));
#82953=CARTESIAN_POINT('Ctrl Pts',(0.0134525164811448,-0.0329730614463152,
0.0717802334744865));
#82954=CARTESIAN_POINT('Ctrl Pts',(0.0134153670233181,-0.0329207133373891,
0.0717967543255685));
#82955=CARTESIAN_POINT('Ctrl Pts',(0.0133789127846533,-0.0328677532289382,
0.0718129660601775));
#82956=CARTESIAN_POINT('',(0.0135408942215889,-0.0331951640388702,0.0718772459711527));
#82957=CARTESIAN_POINT('Origin',(0.00812378219310841,-0.0315241814719618,
0.07415));
#82958=CARTESIAN_POINT('',(0.0136061014165443,-0.0332121607144411,0.0717119319308847));
#82959=CARTESIAN_POINT('',(0.0136008811544451,-0.0331951640388587,0.0717002271599729));
#82960=CARTESIAN_POINT('Origin',(-0.00116187982707517,-0.0326413661437492,
0.0791078728231921));
#82961=CARTESIAN_POINT('Origin',(-0.00176604658340047,-0.0326412096066327,
0.0777686292935566));
#82962=CARTESIAN_POINT('Origin',(-0.00177702545824643,-0.0326413667295984,
0.0777246335526917));
#82963=CARTESIAN_POINT('Ctrl Pts',(0.0134423184956348,-0.0337436976235975,
0.0719610969416829));
#82964=CARTESIAN_POINT('Ctrl Pts',(0.0134226311697909,-0.0336723290703325,
0.0719132612201318));
#82965=CARTESIAN_POINT('Ctrl Pts',(0.0134020866150368,-0.033601104548885,
0.0718657873502121));
#82966=CARTESIAN_POINT('Ctrl Pts',(0.013336491921354,-0.0333736987606857,
0.0717142126876021));
#82967=CARTESIAN_POINT('Ctrl Pts',(0.0132623070944247,-0.0331450831799192,
0.0715666520097842));
#82968=CARTESIAN_POINT('Ctrl Pts',(0.0133421691550725,-0.0337436976235975,
0.0717320333924551));
#82969=CARTESIAN_POINT('Ctrl Pts',(0.0133204215969514,-0.0336723290703325,
0.0716850984292509));
#82970=CARTESIAN_POINT('Ctrl Pts',(0.0132978333450206,-0.033601104548885,
0.0716385622290417));
#82971=CARTESIAN_POINT('Ctrl Pts',(0.0132257135310861,-0.0333736987606857,
0.0714899813600757));
#82972=CARTESIAN_POINT('Ctrl Pts',(0.0131451861379285,-0.0331450831799192,
0.0713457839913899));
#82973=CARTESIAN_POINT('Ctrl Pts',(0.0133411676616669,-0.0337436976235975,
0.0717297427569627));
#82974=CARTESIAN_POINT('Ctrl Pts',(0.013319399501223,-0.0336723290703325,
0.0716828168013421));
#82975=CARTESIAN_POINT('Ctrl Pts',(0.0132967908123204,-0.033601104548885,
0.07163628997783));
#82976=CARTESIAN_POINT('Ctrl Pts',(0.0132246057471835,-0.0333736987606857,
0.0714877390468003));
#82977=CARTESIAN_POINT('Ctrl Pts',(0.0131440149283635,-0.0331450831799192,
0.071343575311206));
#82978=CARTESIAN_POINT('',(0.0133268783657592,-0.0336938721132548,0.0716993031158164));
#82979=CARTESIAN_POINT('',(0.0132217993931271,-0.0333679869945434,0.0714876052831402));
#82980=CARTESIAN_POINT('Ctrl Pts',(0.0133268783657653,-0.0336938721132649,
0.0716993031158282));
#82981=CARTESIAN_POINT('Ctrl Pts',(0.0133173121461836,-0.0336629187933932,
0.0716789929906506));
#82982=CARTESIAN_POINT('Ctrl Pts',(0.0133076300621579,-0.033631995230104,
0.0716587453751967));
#82983=CARTESIAN_POINT('Ctrl Pts',(0.0132978333450263,-0.033601104548895,
0.0716385622290537));
#82984=CARTESIAN_POINT('Ctrl Pts',(0.013273250029495,-0.0335235892595454,
0.071587915809097));
#82985=CARTESIAN_POINT('Ctrl Pts',(0.0132479010760106,-0.0334458668660369,
0.0715375854107547));
#82986=CARTESIAN_POINT('Ctrl Pts',(0.013221799393407,-0.0333679869945385,
0.0714876052830018));
#82987=CARTESIAN_POINT('Ctrl Pts',(0.0132217794166821,-0.0333679692459108,
0.0714875655463521));
#82988=CARTESIAN_POINT('Ctrl Pts',(0.0132213804309152,-0.0333391895372506,
0.071487780600257));
#82989=CARTESIAN_POINT('Ctrl Pts',(0.0132210829123114,-0.0333104081057283,
0.0714879446520744));
#82990=CARTESIAN_POINT('Ctrl Pts',(0.0132206917694677,-0.0332532697643015,
0.071488166652919));
#82991=CARTESIAN_POINT('Ctrl Pts',(0.0132205951714736,-0.0332249168356299,
0.0714882261525571));
#82992=CARTESIAN_POINT('Ctrl Pts',(0.0132205951108887,-0.0331960985483764,
0.0714882339653226));
#82993=CARTESIAN_POINT('Ctrl Pts',(0.0132205951363545,-0.0331956312440266,
0.0714882340783684));
#82994=CARTESIAN_POINT('Ctrl Pts',(0.0132205951878506,-0.0331951640388588,
0.0714882341769745));
#82995=CARTESIAN_POINT('',(0.0132784596622649,-0.0331951640388587,0.07159903445947));
#82996=CARTESIAN_POINT('',(0.0132495274250681,-0.0331951640388688,0.0715436343182328));
#82997=CARTESIAN_POINT('',(0.013378912770842,-0.0335216366567682,0.0718129660664729));
#82998=CARTESIAN_POINT('Origin',(-0.00130623962662685,-0.0326434571526819,
0.0796689805829238));
#82999=CARTESIAN_POINT('',(0.0133776714505554,-0.0336938721132328,0.0718135180996883));
#83000=CARTESIAN_POINT('Origin',(0.0233560129331568,-0.033693886789623,
0.0673760040209701));
#83001=CARTESIAN_POINT('',(0.0133522749081673,-0.0336938721132538,0.0717564106077624));
#83002=CARTESIAN_POINT('Ctrl Pts',(0.0136974519161943,-0.0335235895815172,
0.0719286927682037));
#83003=CARTESIAN_POINT('Ctrl Pts',(0.0136668712487971,-0.0334144449262748,
0.0718519602309195));
#83004=CARTESIAN_POINT('Ctrl Pts',(0.0136346702114454,-0.0333049234473147,
0.0717757713108203));
#83005=CARTESIAN_POINT('Ctrl Pts',(0.013600881154452,-0.0331951640388587,
0.0717002271599751));
#83006=CARTESIAN_POINT('Ctrl Pts',(0.0135908278772855,-0.0335235895815172,
0.0718903197723197));
#83007=CARTESIAN_POINT('Ctrl Pts',(0.0135597189300505,-0.0334144449262748,
0.0718150551248545));
#83008=CARTESIAN_POINT('Ctrl Pts',(0.0135270193314304,-0.0333049234473147,
0.0717403466948658));
#83009=CARTESIAN_POINT('Ctrl Pts',(0.0134927622407293,-0.0331951640388587,
0.0716662937990782));
#83010=CARTESIAN_POINT('Ctrl Pts',(0.0134842038383766,-0.0335235895815172,
0.0718519467764358));
#83011=CARTESIAN_POINT('Ctrl Pts',(0.0134525666113038,-0.0334144449262748,
0.0717781500187896));
#83012=CARTESIAN_POINT('Ctrl Pts',(0.0134193684514153,-0.0333049234473147,
0.0717049220789113));
#83013=CARTESIAN_POINT('Ctrl Pts',(0.0133846433270065,-0.0331951640388587,
0.0716323604381814));
#83014=CARTESIAN_POINT('Ctrl Pts',(0.0133775797994678,-0.0335235895815172,
0.0718135737805518));
#83015=CARTESIAN_POINT('Ctrl Pts',(0.0133454142925572,-0.0334144449262748,
0.0717412449127246));
#83016=CARTESIAN_POINT('Ctrl Pts',(0.0133117175714003,-0.0333049234473147,
0.0716694974629568));
#83017=CARTESIAN_POINT('Ctrl Pts',(0.0132765244132838,-0.0331951640388587,
0.0715984270772845));
#83018=CARTESIAN_POINT('',(0.013439670408365,-0.0331951640388687,0.0716496308097315));
#83019=CARTESIAN_POINT('Ctrl Pts',(0.0136061014136768,-0.0332121607145961,
0.0717119319321526));
#83020=CARTESIAN_POINT('Ctrl Pts',(0.0135668930591495,-0.0332625444108954,
0.0717293684646345));
#83021=CARTESIAN_POINT('Ctrl Pts',(0.0135283603260961,-0.0333135300745199,
0.0717465045383006));
#83022=CARTESIAN_POINT('Ctrl Pts',(0.0134526155159261,-0.0334167203140579,
0.0717801893704949));
#83023=CARTESIAN_POINT('Ctrl Pts',(0.0134154327755747,-0.0334688847587263,
0.0717967250825318));
#83024=CARTESIAN_POINT('Ctrl Pts',(0.0133789127701246,-0.033521636656232,
0.0718129660666014));
#83025=CARTESIAN_POINT('Ctrl Pts',(0.0133265196484848,-0.0336938721132388,
0.0717002364093335));
#83026=CARTESIAN_POINT('Ctrl Pts',(0.0133121803692709,-0.0336474569764957,
0.0716697830605558));
#83027=CARTESIAN_POINT('Ctrl Pts',(0.0132974855776959,-0.033601104548885,
0.0716394996578291));
#83028=CARTESIAN_POINT('Ctrl Pts',(0.0132602817439722,-0.0334837508592656,
0.0715628290447157));
#83029=CARTESIAN_POINT('Ctrl Pts',(0.0132208223381995,-0.0333660264659097,
0.0714872945264145));
#83030=CARTESIAN_POINT('Ctrl Pts',(0.0133268783657679,-0.0336938721132388,
0.0716993031158349));
#83031=CARTESIAN_POINT('Ctrl Pts',(0.0133125336236774,-0.0336474569764957,
0.071668847667366));
#83032=CARTESIAN_POINT('Ctrl Pts',(0.0132978333450206,-0.033601104548885,
0.0716385622290417));
#83033=CARTESIAN_POINT('Ctrl Pts',(0.0132606156192675,-0.0334837508592656,
0.0715618864622633));
#83034=CARTESIAN_POINT('Ctrl Pts',(0.0132211421748518,-0.0333660264659097,
0.0714863472042099));
#83035=CARTESIAN_POINT('Ctrl Pts',(0.0134488438267941,-0.0336938721132388,
0.0713819792030978));
#83036=CARTESIAN_POINT('Ctrl Pts',(0.0134326416825432,-0.0336474569764957,
0.0713508098503131));
#83037=CARTESIAN_POINT('Ctrl Pts',(0.0134160757718449,-0.033601104548885,
0.0713198322998276));
#83038=CARTESIAN_POINT('Ctrl Pts',(0.0133741346946984,-0.0334837508592656,
0.0712414042641836));
#83039=CARTESIAN_POINT('Ctrl Pts',(0.0133298880496777,-0.0333660264659097,
0.0711642534694269));
#83040=CARTESIAN_POINT('',(0.01344219575284,-0.0336769361243754,0.0713725052281484));
#83041=CARTESIAN_POINT('',(0.0134481163985911,-0.033693872113232,0.0713838717910539));
#83042=CARTESIAN_POINT('Ctrl Pts',(0.01344219575284,-0.0336769361243754,
0.0713725052281484));
#83043=CARTESIAN_POINT('Ctrl Pts',(0.0134431846244391,-0.0336797586669775,
0.0713743987431874));
#83044=CARTESIAN_POINT('Ctrl Pts',(0.0134441724474163,-0.0336825812712343,
0.0713762927147142));
#83045=CARTESIAN_POINT('Ctrl Pts',(0.01344614599607,-0.0336882266015139,
0.0713800815695215));
#83046=CARTESIAN_POINT('Ctrl Pts',(0.0134471317217169,-0.0336910493274514,
0.0713819764527443));
#83047=CARTESIAN_POINT('Ctrl Pts',(0.0134481163985909,-0.0336938721132327,
0.0713838717910531));
#83048=CARTESIAN_POINT('Ctrl Pts',(0.01344219575284,-0.0336769361243754,
0.0713725052281485));
#83049=CARTESIAN_POINT('Ctrl Pts',(0.0134050433058289,-0.0336279007516236,
0.0713919077673034));
#83050=CARTESIAN_POINT('Ctrl Pts',(0.0133673618658974,-0.0335767878632084,
0.0714115865683656));
#83051=CARTESIAN_POINT('Ctrl Pts',(0.0132935168246351,-0.033473319885732,
0.0714501514926104));
#83052=CARTESIAN_POINT('Ctrl Pts',(0.0132573092600289,-0.0334209645014059,
0.0714690605752273));
#83053=CARTESIAN_POINT('Ctrl Pts',(0.0132217993964906,-0.0333679869844681,
0.0714876052895897));
#83054=CARTESIAN_POINT('',(0.0133874973821852,-0.0336938721132534,0.0715415874534452));
#83055=CARTESIAN_POINT('Origin',(0.00812378219310841,-0.0315241814719618,
0.07415));
#83056=CARTESIAN_POINT('',(0.0134421957516969,-0.0337108120655395,0.0713725052287529));
#83057=CARTESIAN_POINT('',(0.0134362508414152,-0.0336938721132327,0.0713611513377796));
#83058=CARTESIAN_POINT('Origin',(-0.00157777664322337,-0.0345562523507427,
0.0779557197821598));
#83059=CARTESIAN_POINT('Ctrl Pts',(0.0134362508414275,-0.0336938721132373,
0.07136115133778));
#83060=CARTESIAN_POINT('Ctrl Pts',(0.0134372436155188,-0.0336910493011037,
0.0713630424698828));
#83061=CARTESIAN_POINT('Ctrl Pts',(0.0134382354029273,-0.0336882265883395,
0.071364934176149));
#83062=CARTESIAN_POINT('Ctrl Pts',(0.0134402170357983,-0.0336825812712955,
0.0713687187977454));
#83063=CARTESIAN_POINT('Ctrl Pts',(0.0134412068812303,-0.0336797586670082,
0.0713706117130889));
#83064=CARTESIAN_POINT('Ctrl Pts',(0.01344219575284,-0.0336769361243754,
0.0713725052281484));
#83065=CARTESIAN_POINT('Origin',(-0.000543060617466345,-0.03455625200519,
0.0799370161395398));
#83066=CARTESIAN_POINT('Ctrl Pts',(0.013294403830978,-0.0342436276873909,
0.0716315090077599));
#83067=CARTESIAN_POINT('Ctrl Pts',(0.0131994173773341,-0.0339430054201809,
0.0714364957978541));
#83068=CARTESIAN_POINT('Ctrl Pts',(0.0130900115762353,-0.0336441434784052,
0.0712491913689167));
#83069=CARTESIAN_POINT('Ctrl Pts',(0.0131800710890971,-0.0342436276873909,
0.0714091848657195));
#83070=CARTESIAN_POINT('Ctrl Pts',(0.0130766995422061,-0.0339430054201809,
0.07121848378626));
#83071=CARTESIAN_POINT('Ctrl Pts',(0.0129592572763648,-0.0336441434784052,
0.0710361108370388));
#83072=CARTESIAN_POINT('Ctrl Pts',(0.0131789277616783,-0.0342436276873909,
0.071406961624299));
#83073=CARTESIAN_POINT('Ctrl Pts',(0.0130754723638549,-0.0339430054201809,
0.0712163036661441));
#83074=CARTESIAN_POINT('Ctrl Pts',(0.0129579497333661,-0.0336441434784052,
0.07103398003172));
#83075=CARTESIAN_POINT('',(0.0131627307134377,-0.0341934961088741,0.0713774338944811));
#83076=CARTESIAN_POINT('',(0.0130445664769882,-0.0338664212865394,0.0711727517674418));
#83077=CARTESIAN_POINT('Origin',(-0.00173801708148712,-0.0345610720403692,
0.0789945763319301));
#83078=CARTESIAN_POINT('Origin',(0.0224271245308364,-0.0336938005072992,
0.0654959279369191));
#83079=CARTESIAN_POINT('',(0.0131081116321623,-0.0336938721132327,0.0712804033309572));
#83080=CARTESIAN_POINT('',(0.0130757578824758,-0.0336938721132427,0.0712269291794493));
#83081=CARTESIAN_POINT('',(0.0132217993964931,-0.0340203938281605,0.0714876052895945));
#83082=CARTESIAN_POINT('Origin',(-0.00188836694114705,-0.0345589643244413,
0.078537485909832));
#83083=CARTESIAN_POINT('',(0.0132205951878513,-0.0341934961088739,0.0714882341769755));
#83084=CARTESIAN_POINT('Origin',(0.0229882585815279,-0.0341934220717601,
0.0663871587920726));
#83085=CARTESIAN_POINT('',(0.0131916629506545,-0.034193496108884,0.0714328340357383));
#83086=CARTESIAN_POINT('Ctrl Pts',(0.0135469776876582,-0.0340223579322396,
0.0715831048661921));
#83087=CARTESIAN_POINT('Ctrl Pts',(0.0135115735090194,-0.0339125849573575,
0.0715083048560346));
#83088=CARTESIAN_POINT('Ctrl Pts',(0.013474646022088,-0.0338030433565231,
0.0714342901912081));
#83089=CARTESIAN_POINT('Ctrl Pts',(0.0134362508414217,-0.0336938721132326,
0.0713611513377812));
#83090=CARTESIAN_POINT('Ctrl Pts',(0.0134381545698786,-0.0340223579322396,
0.071551502510783));
#83091=CARTESIAN_POINT('Ctrl Pts',(0.0134023145123364,-0.0339125849573575,
0.0714782034552423));
#83092=CARTESIAN_POINT('Ctrl Pts',(0.0133649825190614,-0.0338030433565231,
0.0714056977120096));
#83093=CARTESIAN_POINT('Ctrl Pts',(0.0133262145508509,-0.0336938721132326,
0.071334073771641));
#83094=CARTESIAN_POINT('Ctrl Pts',(0.0133293314520991,-0.0340223579322396,
0.0715199001553738));
#83095=CARTESIAN_POINT('Ctrl Pts',(0.0132930555156534,-0.0339125849573575,
0.0714481020544499));
#83096=CARTESIAN_POINT('Ctrl Pts',(0.0132553190160347,-0.0338030433565231,
0.071377105232811));
#83097=CARTESIAN_POINT('Ctrl Pts',(0.01321617826028,-0.0336938721132326,
0.0713069962055009));
#83098=CARTESIAN_POINT('Ctrl Pts',(0.0132205083343196,-0.0340223579322396,
0.0714882977999647));
#83099=CARTESIAN_POINT('Ctrl Pts',(0.0131837965189704,-0.0339125849573575,
0.0714180006536575));
#83100=CARTESIAN_POINT('Ctrl Pts',(0.0131456555130081,-0.0338030433565231,
0.0713485127536124));
#83101=CARTESIAN_POINT('Ctrl Pts',(0.0131061419697092,-0.0336938721132326,
0.0712799186393607));
#83102=CARTESIAN_POINT('',(0.0132721812367987,-0.0336938721132427,0.0713207773343784));
#83103=CARTESIAN_POINT('Ctrl Pts',(0.0134421957484976,-0.0337108120662676,
0.0713725052304164));
#83104=CARTESIAN_POINT('Ctrl Pts',(0.0134040811107114,-0.033761140899359,
0.071392410265253));
#83105=CARTESIAN_POINT('Ctrl Pts',(0.0133666619805022,-0.0338121088779862,
0.0714119520773659));
#83106=CARTESIAN_POINT('Ctrl Pts',(0.0132931806468089,-0.033915338277324,
0.0714503270585271));
#83107=CARTESIAN_POINT('Ctrl Pts',(0.0132571495305818,-0.0339675558473112,
0.0714691439925283));
#83108=CARTESIAN_POINT('Ctrl Pts',(0.0132217993964553,-0.0340203938281304,
0.0714876052896084));
#83109=CARTESIAN_POINT('Ctrl Pts',(0.0131621233843922,-0.0341934961088741,
0.0713793689741472));
#83110=CARTESIAN_POINT('Ctrl Pts',(0.0131048427706686,-0.0340287516182427,
0.0712752052392823));
#83111=CARTESIAN_POINT('Ctrl Pts',(0.0130433059359474,-0.0338644633275951,
0.0711734979615582));
#83112=CARTESIAN_POINT('Ctrl Pts',(0.0131627307134377,-0.0341934961088741,
0.0713774338944813));
#83113=CARTESIAN_POINT('Ctrl Pts',(0.0131054100934665,-0.0340287516182427,
0.0712732576035668));
#83114=CARTESIAN_POINT('Ctrl Pts',(0.0130438327677312,-0.0338644633275951,
0.0711715394340106));
#83115=CARTESIAN_POINT('Ctrl Pts',(0.0132639234139404,-0.0341934961088741,
0.0710550124023017));
#83116=CARTESIAN_POINT('Ctrl Pts',(0.0131999369836259,-0.0340287516182427,
0.0709487440320251));
#83117=CARTESIAN_POINT('Ctrl Pts',(0.0131316130761275,-0.0338644633275951,
0.0708452110737472));
#83118=CARTESIAN_POINT('',(0.0132573007386171,-0.0341764758832421,0.0710440400302624));
#83119=CARTESIAN_POINT('',(0.0132639234139403,-0.034193496108874,0.0710550124023019));
#83120=CARTESIAN_POINT('Origin',(-0.00117437858495977,-0.0345621027089467,
0.0791771798535414));
#83121=CARTESIAN_POINT('Ctrl Pts',(0.013257300738701,-0.0341764758837522,
0.0710440400320756));
#83122=CARTESIAN_POINT('Ctrl Pts',(0.0132205752309949,-0.0341260050040497,
0.0710662602769656));
#83123=CARTESIAN_POINT('Ctrl Pts',(0.013184488119031,-0.0340749269148259,
0.0710880943142688));
#83124=CARTESIAN_POINT('Ctrl Pts',(0.0131135626237488,-0.0339715436306283,
0.071131006738375));
#83125=CARTESIAN_POINT('Ctrl Pts',(0.01307875114497,-0.033919277823851,
0.071152068839989));
#83126=CARTESIAN_POINT('Ctrl Pts',(0.0130445664784764,-0.0338664212857068,
0.0711727517677738));
#83127=CARTESIAN_POINT('',(0.013213327063699,-0.0341934961088841,0.0712162231484015));
#83128=CARTESIAN_POINT('Origin',(0.00812378219310841,-0.0315241814719618,
0.07415));
#83129=CARTESIAN_POINT('',(0.0132573007375502,-0.0342105180190539,0.0710440400299246));
#83130=CARTESIAN_POINT('',(0.0132506546416664,-0.0341934961088739,0.0710330818271522));
#83131=CARTESIAN_POINT('Origin',(-0.00115554781581669,-0.0345621715476278,
0.0792184088855479));
#83132=CARTESIAN_POINT('Origin',(-0.000644192738700177,-0.0345621032405993,
0.0800534709426069));
#83133=CARTESIAN_POINT('Origin',(-0.000671972938710301,-0.0345621721347048,
0.0800176567189358));
#83134=CARTESIAN_POINT('Ctrl Pts',(0.0131088881272831,-0.0346945769586966,
0.0712816867190697));
#83135=CARTESIAN_POINT('Ctrl Pts',(0.013048810157204,-0.0345275153362944,
0.0711772716793509));
#83136=CARTESIAN_POINT('Ctrl Pts',(0.0129854328909929,-0.0343603235965185,
0.0710747190294156));
#83137=CARTESIAN_POINT('Ctrl Pts',(0.0129189482783755,-0.034193496108874,
0.0709743292886055));
#83138=CARTESIAN_POINT('Ctrl Pts',(0.0130654909626485,-0.0346945769586966,
0.0712099600543431));
#83139=CARTESIAN_POINT('Ctrl Pts',(0.0130039106488589,-0.0345275153362944,
0.0711064539856128));
#83140=CARTESIAN_POINT('Ctrl Pts',(0.0129390592366552,-0.0343603235965185,
0.0710048577890994));
#83141=CARTESIAN_POINT('Ctrl Pts',(0.0128711329935898,-0.034193496108874,
0.0709054690905808));
#83142=CARTESIAN_POINT('Ctrl Pts',(0.0130220937980139,-0.0346945769586966,
0.0711382333896164));
#83143=CARTESIAN_POINT('Ctrl Pts',(0.0129590111405138,-0.0345275153362944,
0.0710356362918747));
#83144=CARTESIAN_POINT('Ctrl Pts',(0.0128926855823176,-0.0343603235965185,
0.0709349965487832));
#83145=CARTESIAN_POINT('Ctrl Pts',(0.0128233177088041,-0.034193496108874,
0.0708366088925562));
#83146=CARTESIAN_POINT('Ctrl Pts',(0.0129786966333793,-0.0346945769586966,
0.0710665067248898));
#83147=CARTESIAN_POINT('Ctrl Pts',(0.0129141116321687,-0.0345275153362944,
0.0709648185981367));
#83148=CARTESIAN_POINT('Ctrl Pts',(0.0128463119279799,-0.0343603235965185,
0.0708651353084671));
#83149=CARTESIAN_POINT('Ctrl Pts',(0.0127755024240184,-0.034193496108874,
0.0707677486945316));
#83150=CARTESIAN_POINT('',(0.0129786966333732,-0.0346945769586966,0.0710665067248801));
#83151=CARTESIAN_POINT('',(0.0128479134699673,-0.0343667727831647,0.0708696480860459));
#83152=CARTESIAN_POINT('Origin',(-0.00111529414379012,-0.0345626457065037,
0.0802347492617079));
#83153=CARTESIAN_POINT('Origin',(0.021926103880993,-0.0341934771029166,
0.064565910045707));
#83154=CARTESIAN_POINT('',(0.0129180927308873,-0.034193496108874,0.0709730971895031));
#83155=CARTESIAN_POINT('',(0.0128824451541801,-0.034193496108884,0.0709217600657703));
#83156=CARTESIAN_POINT('',(0.013044566477013,-0.034521194296265,0.0711727517686283));
#83157=CARTESIAN_POINT('Origin',(-0.0013613467526906,-0.0345625596120561,
0.0798216525375073));
#83158=CARTESIAN_POINT('',(0.0130434041327692,-0.0346945769586885,0.0711734550279211));
#83159=CARTESIAN_POINT('Origin',(0.0225092423963709,-0.034694568585389,
0.065446289832958));
#83160=CARTESIAN_POINT('',(0.0130110503830812,-0.0346945769587025,0.0711199808764106));
#83161=CARTESIAN_POINT('Ctrl Pts',(0.0133750991057015,-0.0345231616327841,
0.0712476439426601));
#83162=CARTESIAN_POINT('Ctrl Pts',(0.0133350942136416,-0.0344132092796988,
0.0711752619322828));
#83163=CARTESIAN_POINT('Ctrl Pts',(0.0132935942208596,-0.0343032738558979,
0.0711037111261214));
#83164=CARTESIAN_POINT('Ctrl Pts',(0.0132506546416721,-0.0341934961088739,
0.0710330818271533));
#83165=CARTESIAN_POINT('Ctrl Pts',(0.0132645065813549,-0.0345231616327841,
0.07122293706715));
#83166=CARTESIAN_POINT('Ctrl Pts',(0.0132241611398005,-0.0344132092796988,
0.071152079419019));
#83167=CARTESIAN_POINT('Ctrl Pts',(0.0131823521453256,-0.0343032738558979,
0.0710820599404515));
#83168=CARTESIAN_POINT('Ctrl Pts',(0.0131391354578611,-0.0341934961088739,
0.0710129669624769));
#83169=CARTESIAN_POINT('Ctrl Pts',(0.0131539140570083,-0.0345231616327841,
0.0711982301916399));
#83170=CARTESIAN_POINT('Ctrl Pts',(0.0131132280659595,-0.0344132092796988,
0.0711288969057552));
#83171=CARTESIAN_POINT('Ctrl Pts',(0.0130711100697917,-0.0343032738558979,
0.0710604087547815));
#83172=CARTESIAN_POINT('Ctrl Pts',(0.0130276162740501,-0.0341934961088739,
0.0709928520978005));
#83173=CARTESIAN_POINT('Ctrl Pts',(0.0130433215326617,-0.0345231616327841,
0.0711735233161298));
#83174=CARTESIAN_POINT('Ctrl Pts',(0.0130022949921185,-0.0344132092796988,
0.0711057143924914));
#83175=CARTESIAN_POINT('Ctrl Pts',(0.0129598679942577,-0.0343032738558979,
0.0710387575691116));
#83176=CARTESIAN_POINT('Ctrl Pts',(0.012916097090239,-0.0341934961088739,
0.0709727372331242));
#83177=CARTESIAN_POINT('',(0.0130843736862868,-0.0341934961088839,0.0710030895083377));
#83178=CARTESIAN_POINT('Ctrl Pts',(0.0132573007345886,-0.0342105180195382,
0.0710440400317084));
#83179=CARTESIAN_POINT('Ctrl Pts',(0.0132205339332162,-0.034261055624049,
0.0710662852446752));
#83180=CARTESIAN_POINT('Ctrl Pts',(0.013184426893082,-0.0343122189868487,
0.0710881312787986));
#83181=CARTESIAN_POINT('Ctrl Pts',(0.0131135006843536,-0.0344158119695131,
0.0711310441392924));
#83182=CARTESIAN_POINT('Ctrl Pts',(0.0130787105252643,-0.0344681990450021,
0.0711520934138882));
#83183=CARTESIAN_POINT('Ctrl Pts',(0.0130445664769814,-0.0345211942962426,
0.0711727517686336));
#83184=CARTESIAN_POINT('Ctrl Pts',(0.0129782121260746,-0.0346945769586932,
0.0710684756384207));
#83185=CARTESIAN_POINT('Ctrl Pts',(0.0129357471627973,-0.034584662917547,
0.071001579140244));
#83186=CARTESIAN_POINT('Ctrl Pts',(0.0128918915542897,-0.0344746925049099,
0.0709355493739828));
#83187=CARTESIAN_POINT('Ctrl Pts',(0.0128467018428174,-0.034364806625142,
0.070870470712514));
#83188=CARTESIAN_POINT('Ctrl Pts',(0.0130052896307832,-0.0346945769586932,
0.0709584395974925));
#83189=CARTESIAN_POINT('Ctrl Pts',(0.0129613083152435,-0.034584662917547,
0.0708911699576144));
#83190=CARTESIAN_POINT('Ctrl Pts',(0.0129159283790597,-0.0344746925049099,
0.0708247983434604));
#83191=CARTESIAN_POINT('Ctrl Pts',(0.0128692083194506,-0.034364806625142,
0.0707594095578561));
#83192=CARTESIAN_POINT('Ctrl Pts',(0.0130323671354917,-0.0346945769586932,
0.0708484035565642));
#83193=CARTESIAN_POINT('Ctrl Pts',(0.0129868694676897,-0.034584662917547,
0.0707807607749848));
#83194=CARTESIAN_POINT('Ctrl Pts',(0.0129399652038296,-0.0344746925049099,
0.070714047312938));
#83195=CARTESIAN_POINT('Ctrl Pts',(0.0128917147960837,-0.034364806625142,
0.0706483484031981));
#83196=CARTESIAN_POINT('Ctrl Pts',(0.0130594446402003,-0.0346945769586932,
0.070738367515636));
#83197=CARTESIAN_POINT('Ctrl Pts',(0.0130124306201359,-0.034584662917547,
0.0706703515923552));
#83198=CARTESIAN_POINT('Ctrl Pts',(0.0129640020285996,-0.0344746925049099,
0.0706032962824155));
#83199=CARTESIAN_POINT('Ctrl Pts',(0.0129142212727169,-0.034364806625142,
0.0705372872485401));
#83200=CARTESIAN_POINT('',(0.0130521460711012,-0.034677539666344,0.0707278326360764));
#83201=CARTESIAN_POINT('',(0.0130594446401983,-0.0346945769586886,0.0707383675156333));
#83202=CARTESIAN_POINT('Origin',(-0.000496621982559035,-0.0345626618638833,
0.0803217779571767));
#83203=CARTESIAN_POINT('Ctrl Pts',(0.0130521460683195,-0.0346775396659408,
0.0707278326379988));
#83204=CARTESIAN_POINT('Ctrl Pts',(0.013016860365398,-0.0346269748528212,
0.0707523343963796));
#83205=CARTESIAN_POINT('Ctrl Pts',(0.0129822020560721,-0.0345757904815282,
0.0707764005039156));
#83206=CARTESIAN_POINT('Ctrl Pts',(0.0129141105025331,-0.0344721679344067,
0.0708236820557754));
#83207=CARTESIAN_POINT('Ctrl Pts',(0.0128807046965108,-0.0344197716859604,
0.0708468784475121));
#83208=CARTESIAN_POINT('Ctrl Pts',(0.0128479134701608,-0.0343667727830949,
0.0708696480861622));
#83209=CARTESIAN_POINT('',(0.0130190706367957,-0.0346945769587026,0.0709024371202667));
#83210=CARTESIAN_POINT('Origin',(0.00812378219310841,-0.0315241814719618,
0.07415));
#83211=CARTESIAN_POINT('',(0.0130521460710122,-0.0347116136489614,0.0707278326361377));
#83212=CARTESIAN_POINT('',(0.0130448250186084,-0.0346945769586885,0.0707173133685687));
#83213=CARTESIAN_POINT('Origin',(-0.00046926371922708,-0.0345626696275047,
0.0803578983563592));
#83214=CARTESIAN_POINT('Origin',(-0.000670830339955459,-0.0345626623641555,
0.0800708976830043));
#83215=CARTESIAN_POINT('Origin',(-0.000695114068535318,-0.0345626701139946,
0.0800326423598664));
#83216=CARTESIAN_POINT('Ctrl Pts',(0.012939365481435,-0.0352450361874067,
0.0710053346412036));
#83217=CARTESIAN_POINT('Ctrl Pts',(0.0128207624812432,-0.0349452760959492,
0.0708237119371942));
#83218=CARTESIAN_POINT('Ctrl Pts',(0.0126888158544847,-0.034644428984174,
0.0706515388674267));
#83219=CARTESIAN_POINT('Ctrl Pts',(0.012937938365447,-0.0352450361874067,
0.0710032516229711));
#83220=CARTESIAN_POINT('Ctrl Pts',(0.0128192568029334,-0.0349452760959492,
0.0708216827435245));
#83221=CARTESIAN_POINT('Ctrl Pts',(0.0126872358913267,-0.034644428984174,
0.0706495692630452));
#83222=CARTESIAN_POINT('Ctrl Pts',(0.0127966397527728,-0.0352450361874067,
0.0707970121940144));
#83223=CARTESIAN_POINT('Ctrl Pts',(0.0126701797425577,-0.0349452760959492,
0.0706207724791924));
#83224=CARTESIAN_POINT('Ctrl Pts',(0.0125308038954853,-0.034644428984174,
0.0704545589282497));
#83225=CARTESIAN_POINT('Ctrl Pts',(0.012795226766646,-0.0352450361874067,
0.0707949497997249));
#83226=CARTESIAN_POINT('Ctrl Pts',(0.012668688971954,-0.0349452760959492,
0.0706187633765491));
#83227=CARTESIAN_POINT('Ctrl Pts',(0.0125292395755269,-0.034644428984174,
0.0704526088249018));
#83228=CARTESIAN_POINT('',(0.0127755233731481,-0.0351951634053348,0.0707677734705648));
#83229=CARTESIAN_POINT('',(0.0126326164752035,-0.0348678972925388,0.0705794904542061));
#83230=CARTESIAN_POINT('Origin',(-0.000236095645883816,-0.0345636767883841,
0.0813082794769825));
#83231=CARTESIAN_POINT('Origin',(0.0212952490697888,-0.0346946199340833,
0.0637196226839455));
#83232=CARTESIAN_POINT('',(0.0127091528869729,-0.0346945769330288,0.0706783288465125));
#83233=CARTESIAN_POINT('',(0.0126703521628121,-0.0346945769458128,0.0706293313476771));
#83234=CARTESIAN_POINT('',(0.0128479134700692,-0.0350221583435276,0.0708696480862502));
#83235=CARTESIAN_POINT('Origin',(-0.000565974147668837,-0.0345628458717359,
0.080958531614612));
#83236=CARTESIAN_POINT('',(0.0128468992255452,-0.035195136029876,0.0708703560416109));
#83237=CARTESIAN_POINT('Origin',(0.0218978191987488,-0.0351951838366798,
0.0645855575956237));
#83238=CARTESIAN_POINT('',(0.0127755024241135,-0.0351951371328748,0.0707677486944647));
#83239=CARTESIAN_POINT('Ctrl Pts',(0.0131824958700217,-0.0350241211494342,
0.0709236373522079));
#83240=CARTESIAN_POINT('Ctrl Pts',(0.0131380540474086,-0.0349144232818962,
0.0708539556454617));
#83241=CARTESIAN_POINT('Ctrl Pts',(0.0130921452535521,-0.0348045283579412,
0.0707851508750852));
#83242=CARTESIAN_POINT('Ctrl Pts',(0.0130448250122557,-0.0346945769439158,
0.0707173133594548));
#83243=CARTESIAN_POINT('Ctrl Pts',(0.0130705701896879,-0.0350241211494342,
0.0709059234061471));
#83244=CARTESIAN_POINT('Ctrl Pts',(0.0130258843647308,-0.0349144232818962,
0.0708377834297562));
#83245=CARTESIAN_POINT('Ctrl Pts',(0.0129797632911513,-0.0348045283579412,
0.0707705263562377));
#83246=CARTESIAN_POINT('Ctrl Pts',(0.0129322628384259,-0.0346945769439158,
0.0707042405316832));
#83247=CARTESIAN_POINT('Ctrl Pts',(0.0129586445093541,-0.0350241211494342,
0.0708882094600864));
#83248=CARTESIAN_POINT('Ctrl Pts',(0.012913714682053,-0.0349144232818962,
0.0708216112140508));
#83249=CARTESIAN_POINT('Ctrl Pts',(0.0128673813287505,-0.0348045283579412,
0.0707559018373903));
#83250=CARTESIAN_POINT('Ctrl Pts',(0.0128197006645961,-0.0346945769439158,
0.0706911677039117));
#83251=CARTESIAN_POINT('Ctrl Pts',(0.0128467188290203,-0.0350241211494342,
0.0708704955140256));
#83252=CARTESIAN_POINT('Ctrl Pts',(0.0128015449993752,-0.0349144232818962,
0.0708054389983453));
#83253=CARTESIAN_POINT('Ctrl Pts',(0.0127549993663496,-0.0348045283579412,
0.0707412773185428));
#83254=CARTESIAN_POINT('Ctrl Pts',(0.0127071384907663,-0.0346945769439158,
0.0706780948761401));
#83255=CARTESIAN_POINT('',(0.0128769889530388,-0.0346945769458128,0.0706978211077288));
#83256=CARTESIAN_POINT('Ctrl Pts',(0.0130521460683053,-0.0347116136492791,
0.0707278326380088));
#83257=CARTESIAN_POINT('Ctrl Pts',(0.0130168744869824,-0.034762154653151,
0.0707523245906052));
#83258=CARTESIAN_POINT('Ctrl Pts',(0.0129822230753714,-0.0348133084095402,
0.0707763859084918));
#83259=CARTESIAN_POINT('Ctrl Pts',(0.0129141316724007,-0.0349168561544574,
0.0708236673557995));
#83260=CARTESIAN_POINT('Ctrl Pts',(0.0128807186896037,-0.034969208901592,
0.0708468687309598));
#83261=CARTESIAN_POINT('Ctrl Pts',(0.0128479134700278,-0.0350221583435,
0.0708696480862548));
#83262=CARTESIAN_POINT('Ctrl Pts',(0.0127752427282663,-0.0351951371254977,
0.0707691884784717));
#83263=CARTESIAN_POINT('Ctrl Pts',(0.0127053465712501,-0.0350307338980969,
0.0706730224503303));
#83264=CARTESIAN_POINT('Ctrl Pts',(0.0126315354943806,-0.0348659306897816,
0.0705798274790847));
#83265=CARTESIAN_POINT('Ctrl Pts',(0.0127755024240242,-0.0351951371254977,
0.0707677486945395));
#83266=CARTESIAN_POINT('Ctrl Pts',(0.0127055765003785,-0.0350307338980969,
0.0706715772973513));
#83267=CARTESIAN_POINT('Ctrl Pts',(0.0126317354604065,-0.0348659306897816,
0.0705783781919335));
#83268=CARTESIAN_POINT('Ctrl Pts',(0.012819027703724,-0.0351951371254977,
0.0705264394068399));
#83269=CARTESIAN_POINT('Ctrl Pts',(0.0127441128619576,-0.0350307338980969,
0.0704293681518025));
#83270=CARTESIAN_POINT('Ctrl Pts',(0.0126652499747703,-0.0348659306897816,
0.070335476154828));
#83271=CARTESIAN_POINT('Origin',(0.0168018575233885,-0.0308609197410378,
0.0672779020548871));
#83272=CARTESIAN_POINT('',(0.0127944784646092,-0.0351951371254977,0.0706625432859009));
#83273=CARTESIAN_POINT('Origin',(0.00745373953934053,-0.0351840467441105,
0.0748611880852274));
#83274=CARTESIAN_POINT('Origin',(0.0169900980219168,-0.0352322613677157,
0.0661151297357092));
#83275=CARTESIAN_POINT('',(0.012481890919325,-0.0351951142564676,0.0703970407790791));
#83276=CARTESIAN_POINT('',(0.0123985151563521,-0.0351951372916788,0.0703043325555947));
#83277=CARTESIAN_POINT('Origin',(0.00779709879998335,-0.0352875117969581,
0.0740537454871082));
#83278=CARTESIAN_POINT('Origin',(0.0119810545394734,-0.029832507652371,
0.0805855761454313));
#83279=CARTESIAN_POINT('Origin',(0.0160064406244031,-0.0338733155346509,
0.0713020587946091));
#83280=CARTESIAN_POINT('Ctrl Pts',(0.0138555576184494,-0.0321934096636942,
0.0736757783020904));
#83281=CARTESIAN_POINT('Ctrl Pts',(0.0138470692758913,-0.0320508460845456,
0.0735731822515703));
#83282=CARTESIAN_POINT('Ctrl Pts',(0.0138358307801348,-0.0319086045665327,
0.0734708916238262));
#83283=CARTESIAN_POINT('Ctrl Pts',(0.01382188446196,-0.0317669892871269,
0.0733691246764067));
#83284=CARTESIAN_POINT('Ctrl Pts',(0.013846828925717,-0.0321934096636942,
0.0735923862008404));
#83285=CARTESIAN_POINT('Ctrl Pts',(0.0138368479042596,-0.0320508460845456,
0.0734899463897633));
#83286=CARTESIAN_POINT('Ctrl Pts',(0.0138241220529342,-0.0319086045665327,
0.073387851988994));
#83287=CARTESIAN_POINT('Ctrl Pts',(0.0138086968702754,-0.0317669892871269,
0.0732863205699169));
#83288=CARTESIAN_POINT('Ctrl Pts',(0.0138381002329847,-0.0321934096636942,
0.0735089940995902));
#83289=CARTESIAN_POINT('Ctrl Pts',(0.013826626532628,-0.0320508460845456,
0.0734067105279564));
#83290=CARTESIAN_POINT('Ctrl Pts',(0.0138124133257338,-0.0319086045665327,
0.0733048123541618));
#83291=CARTESIAN_POINT('Ctrl Pts',(0.0137955092785906,-0.0317669892871269,
0.0732035164634271));
#83292=CARTESIAN_POINT('Ctrl Pts',(0.0138293715402524,-0.0321934096636942,
0.0734256019983401));
#83293=CARTESIAN_POINT('Ctrl Pts',(0.0138164051609964,-0.0320508460845456,
0.0733234746661493));
#83294=CARTESIAN_POINT('Ctrl Pts',(0.0138007045985332,-0.0319086045665327,
0.0732217727193296));
#83295=CARTESIAN_POINT('Ctrl Pts',(0.013782321686906,-0.0317669892871269,
0.0731207123569373));
#83296=CARTESIAN_POINT('',(0.0138295276982879,-0.0321934096636942,0.0734270938995109));
#83297=CARTESIAN_POINT('',(0.0137950098848978,-0.0318665617511339,0.0731932861153394));
#83298=CARTESIAN_POINT('Origin',(-0.00281382859954108,-0.0326371944419269,
0.0749159175898794));
#83299=CARTESIAN_POINT('Origin',(0.0246034787141099,-0.0316939261509209,
0.0713699398195629));
#83300=CARTESIAN_POINT('',(0.0138438177375588,-0.0320197221621814,0.0735510154119181));
#83301=CARTESIAN_POINT('Ctrl Pts',(0.0138438460363689,-0.0320197392094725,
0.0735508326167958));
#83302=CARTESIAN_POINT('Ctrl Pts',(0.0138407972334113,-0.0319792716576023,
0.0735217270978981));
#83303=CARTESIAN_POINT('Ctrl Pts',(0.013837512662381,-0.0319386439829719,
0.0734925123224487));
#83304=CARTESIAN_POINT('Ctrl Pts',(0.0138339804705309,-0.0318979099381651,
0.0734631585653704));
#83305=CARTESIAN_POINT('Ctrl Pts',(0.013830448348497,-0.0318571766984956,
0.07343380538849));
#83306=CARTESIAN_POINT('Ctrl Pts',(0.0138266883369074,-0.0318163871833607,
0.0734044622146292));
#83307=CARTESIAN_POINT('Ctrl Pts',(0.0138227168612495,-0.0317755399638304,
0.0733752295246743));
#83308=CARTESIAN_POINT('',(0.0138425404215422,-0.0321934096636182,0.0735514147306182));
#83309=CARTESIAN_POINT('Origin',(0.0161356974395084,-0.0324112133758613,
0.0732902449803353));
#83310=CARTESIAN_POINT('',(0.0138360340599251,-0.0321934096636661,0.0734892543150745));
#83311=CARTESIAN_POINT('Ctrl Pts',(0.0138282506203132,-0.0321934096636618,
0.0734286695768972));
#83312=CARTESIAN_POINT('Ctrl Pts',(0.0138183029116065,-0.0320835708272592,
0.0733500005114833));
#83313=CARTESIAN_POINT('Ctrl Pts',(0.0138067329207551,-0.0319739230346489,
0.0732715829446392));
#83314=CARTESIAN_POINT('Ctrl Pts',(0.0137935631507942,-0.0318646057455573,
0.0731935160701121));
#83315=CARTESIAN_POINT('Ctrl Pts',(0.0138996022666618,-0.0321934096636618,
0.0733406348830072));
#83316=CARTESIAN_POINT('Ctrl Pts',(0.0138884404909162,-0.0320835708272592,
0.073260981822782));
#83317=CARTESIAN_POINT('Ctrl Pts',(0.0138756367735125,-0.0319739230346489,
0.0731816059569377));
#83318=CARTESIAN_POINT('Ctrl Pts',(0.0138612152900516,-0.0318646057455573,
0.0731026075841559));
#83319=CARTESIAN_POINT('Ctrl Pts',(0.0139709539130104,-0.0321934096636618,
0.0732526001891172));
#83320=CARTESIAN_POINT('Ctrl Pts',(0.0139585780702258,-0.0320835708272592,
0.0731719631340806));
#83321=CARTESIAN_POINT('Ctrl Pts',(0.0139445406262699,-0.0319739230346489,
0.0730916289692363));
#83322=CARTESIAN_POINT('Ctrl Pts',(0.0139288674293091,-0.0318646057455573,
0.0730116990981997));
#83323=CARTESIAN_POINT('Ctrl Pts',(0.014042305559359,-0.0321934096636618,
0.0731645654952272));
#83324=CARTESIAN_POINT('Ctrl Pts',(0.0140287156495354,-0.0320835708272592,
0.0730829444453793));
#83325=CARTESIAN_POINT('Ctrl Pts',(0.0140134444790273,-0.0319739230346489,
0.0730016519815349));
#83326=CARTESIAN_POINT('Ctrl Pts',(0.0139965195685665,-0.0318646057455573,
0.0729207906122435));
#83327=CARTESIAN_POINT('',(0.0140401871499127,-0.0321763980308293,0.0731519256716395));
#83328=CARTESIAN_POINT('',(0.01404230555935,-0.0321934096636184,0.0731645654951994));
#83329=CARTESIAN_POINT('Origin',(-0.00236778886702764,-0.0326386231555595,
0.075297715851378));
#83330=CARTESIAN_POINT('Ctrl Pts',(0.0140401871467773,-0.0321763980306311,
0.0731519256721621));
#83331=CARTESIAN_POINT('Ctrl Pts',(0.0139978662211999,-0.0321259596175317,
0.0731590650464409));
#83332=CARTESIAN_POINT('Ctrl Pts',(0.0139562785605731,-0.0320749164632375,
0.0731660807218032));
#83333=CARTESIAN_POINT('Ctrl Pts',(0.0138745363006747,-0.031971605779399,
0.0731798703206801));
#83334=CARTESIAN_POINT('Ctrl Pts',(0.0138344135510431,-0.0319193786690198,
0.0731866388712851));
#83335=CARTESIAN_POINT('Ctrl Pts',(0.0137950098830636,-0.0318665617525401,
0.0731932861156406));
#83336=CARTESIAN_POINT('',(0.013935916628829,-0.0321934096636663,0.0732958296973652));
#83337=CARTESIAN_POINT('Origin',(0.00812378219310841,-0.0315241814719618,
0.07415));
#83338=CARTESIAN_POINT('',(0.0140401871502783,-0.0322104233323598,0.0731519256715778));
#83339=CARTESIAN_POINT('',(0.0140380417500605,-0.0321934096636183,0.0731392904012454));
#83340=CARTESIAN_POINT('Origin',(-0.00236654846093717,-0.0326387242423214,
0.0753430317953394));
#83341=CARTESIAN_POINT('Origin',(-0.00216368296648192,-0.032638623759595,
0.0765076269337747));
#83342=CARTESIAN_POINT('Origin',(-0.0021773745728056,-0.0326387247245503,
0.0764644112947523));
#83343=CARTESIAN_POINT('Ctrl Pts',(0.0138195875023524,-0.0327445246967096,
0.0733525497638174));
#83344=CARTESIAN_POINT('Ctrl Pts',(0.0137895111750135,-0.0324436878339359,
0.0731377289547349));
#83345=CARTESIAN_POINT('Ctrl Pts',(0.0137433391100204,-0.0321434074405927,
0.0729257839007813));
#83346=CARTESIAN_POINT('Ctrl Pts',(0.0137795511148478,-0.0327445246967096,
0.0731057764109699));
#83347=CARTESIAN_POINT('Ctrl Pts',(0.0137401675783539,-0.0324436878339359,
0.0728924655989273));
#83348=CARTESIAN_POINT('Ctrl Pts',(0.0136848284841527,-0.0321434074405927,
0.072682727309304));
#83349=CARTESIAN_POINT('',(0.0137728770632765,-0.0326943950436612,0.0730702536650482));
#83350=CARTESIAN_POINT('',(0.0137237464515687,-0.0323666188837389,0.0728390746382923));
#83351=CARTESIAN_POINT('Origin',(-0.00272472285463082,-0.0326395579110699,
0.0763009277693971));
#83352=CARTESIAN_POINT('Origin',(0.0244776248529026,-0.0321933825603003,
0.0703216411890648));
#83353=CARTESIAN_POINT('',(0.0137509153243003,-0.0321934096532689,0.0729610938974545));
#83354=CARTESIAN_POINT('',(0.0137366695011081,-0.0321934096584275,0.0729002390959408));
#83355=CARTESIAN_POINT('',(0.0137950098858213,-0.0325210109756239,0.07319328611518));
#83356=CARTESIAN_POINT('Origin',(-0.00278993997179763,-0.0326393129160773,
0.0758245548504547));
#83357=CARTESIAN_POINT('',(0.0137936702784574,-0.0326943950436593,0.0731935121016875));
#83358=CARTESIAN_POINT('Origin',(0.0247019979769415,-0.0326943765538214,
0.0713533209336769));
#83359=CARTESIAN_POINT('',(0.0137832736708769,-0.0326943950436702,0.0731318828833779));
#83360=CARTESIAN_POINT('Ctrl Pts',(0.0140747617225964,-0.0325229783203769,
0.0733845964203715));
#83361=CARTESIAN_POINT('Ctrl Pts',(0.0140642106509895,-0.032413025309245,
0.0733025622976969));
#83362=CARTESIAN_POINT('Ctrl Pts',(0.0140519641984515,-0.0323031222208069,
0.0732207588795742));
#83363=CARTESIAN_POINT('Ctrl Pts',(0.0140380417493126,-0.0321934096576658,
0.0731392903968298));
#83364=CARTESIAN_POINT('Ctrl Pts',(0.0139810305807535,-0.0325229783203769,
0.0733209127074952));
#83365=CARTESIAN_POINT('Ctrl Pts',(0.0139696016305573,-0.032413025309245,
0.0732401706665611));
#83366=CARTESIAN_POINT('Ctrl Pts',(0.0139565041609481,-0.0323031222208069,
0.0731596772942558));
#83367=CARTESIAN_POINT('Ctrl Pts',(0.0139417585871346,-0.0321934096576658,
0.0730795351048643));
#83368=CARTESIAN_POINT('Ctrl Pts',(0.0138872994389107,-0.0325229783203769,
0.0732572289946189));
#83369=CARTESIAN_POINT('Ctrl Pts',(0.0138749926101251,-0.032413025309245,
0.0731777790354253));
#83370=CARTESIAN_POINT('Ctrl Pts',(0.0138610441234446,-0.0323031222208069,
0.0730985957089374));
#83371=CARTESIAN_POINT('Ctrl Pts',(0.0138454754249566,-0.0321934096576658,
0.0730197798128988));
#83372=CARTESIAN_POINT('Ctrl Pts',(0.0137935682970678,-0.0325229783203769,
0.0731935452817426));
#83373=CARTESIAN_POINT('Ctrl Pts',(0.0137803835896929,-0.032413025309245,
0.0731153874042896));
#83374=CARTESIAN_POINT('Ctrl Pts',(0.0137655840859412,-0.0323031222208069,
0.073037514123619));
#83375=CARTESIAN_POINT('Ctrl Pts',(0.0137491922627787,-0.0321934096576658,
0.0729600245209332));
#83376=CARTESIAN_POINT('',(0.0138944785374258,-0.0321934096584275,0.0730501921498067));
#83377=CARTESIAN_POINT('Ctrl Pts',(0.0140401871468428,-0.0322104233328898,
0.0731519256721512));
#83378=CARTESIAN_POINT('Ctrl Pts',(0.0139978088757692,-0.0322609421830383,
0.0731590747203904));
#83379=CARTESIAN_POINT('Ctrl Pts',(0.013956193200933,-0.0323120888238738,
0.0731660951216333));
#83380=CARTESIAN_POINT('Ctrl Pts',(0.0138744503220553,-0.032415652463181,
0.0731798848249295));
#83381=CARTESIAN_POINT('Ctrl Pts',(0.0138343567188523,-0.0324680267167321,
0.0731866484586531));
#83382=CARTESIAN_POINT('Ctrl Pts',(0.0137950098857779,-0.0325210109755913,
0.0731932861151829));
#83383=CARTESIAN_POINT('Origin',(0.00848867654725678,-0.0262834582511018,
0.0820094044272593));
#83384=CARTESIAN_POINT('Origin',(0.0197508774515317,-0.0342771005519637,
0.0777046541217103));
#83385=CARTESIAN_POINT('Ctrl Pts',(0.0137717017281994,-0.0326943950436604,
0.0730719060204244));
#83386=CARTESIAN_POINT('Ctrl Pts',(0.0137568435725974,-0.0325844576448134,
0.0729940671039015));
#83387=CARTESIAN_POINT('Ctrl Pts',(0.0137403745290482,-0.0324744968375322,
0.0729165299696155));
#83388=CARTESIAN_POINT('Ctrl Pts',(0.0137223170689186,-0.0323646534831894,
0.0728393936716174));
#83389=CARTESIAN_POINT('Ctrl Pts',(0.0138373847391094,-0.0326943950436604,
0.0729795649696422));
#83390=CARTESIAN_POINT('Ctrl Pts',(0.013821253950762,-0.0325844576448134,
0.0729008208181258));
#83391=CARTESIAN_POINT('Ctrl Pts',(0.0138034934626575,-0.0324744968375322,
0.0728224047049132));
#83392=CARTESIAN_POINT('Ctrl Pts',(0.0137841274163702,-0.0323646534831894,
0.0727444167874314));
#83393=CARTESIAN_POINT('Ctrl Pts',(0.0139030677500193,-0.0326943950436604,
0.0728872239188599));
#83394=CARTESIAN_POINT('Ctrl Pts',(0.0138856643289266,-0.0325844576448134,
0.0728075745323501));
#83395=CARTESIAN_POINT('Ctrl Pts',(0.0138666123962667,-0.0324744968375322,
0.072728279440211));
#83396=CARTESIAN_POINT('Ctrl Pts',(0.0138459377638218,-0.0323646534831894,
0.0726494399032454));
#83397=CARTESIAN_POINT('Ctrl Pts',(0.0139687507609293,-0.0326943950436604,
0.0727948828680776));
#83398=CARTESIAN_POINT('Ctrl Pts',(0.0139500747070912,-0.0325844576448134,
0.0727143282465744));
#83399=CARTESIAN_POINT('Ctrl Pts',(0.0139297313298759,-0.0324744968375322,
0.0726341541755087));
#83400=CARTESIAN_POINT('Ctrl Pts',(0.0139077481112734,-0.0323646534831894,
0.0725544630190594));
#83401=CARTESIAN_POINT('',(0.013965842870796,-0.0326773559991184,0.0727824010023084));
#83402=CARTESIAN_POINT('',(0.0139687507609263,-0.0326943950436594,0.0727948828680809));
#83403=CARTESIAN_POINT('Origin',(-0.00219074803479047,-0.0326395670083038,
0.0766161821969714));
#83404=CARTESIAN_POINT('Ctrl Pts',(0.0139658428675258,-0.0326773559987448,
0.0727824010030674));
#83405=CARTESIAN_POINT('Ctrl Pts',(0.0139240201085822,-0.0326267922586369,
0.0727921915147323));
#83406=CARTESIAN_POINT('Ctrl Pts',(0.0138829386278392,-0.0325756109580141,
0.0728018084966481));
#83407=CARTESIAN_POINT('Ctrl Pts',(0.0138022232602602,-0.0324719985462373,
0.0728207035855371));
#83408=CARTESIAN_POINT('Ctrl Pts',(0.013762621746245,-0.0324196091621769,
0.0728299741141848));
#83409=CARTESIAN_POINT('Ctrl Pts',(0.0137237464515212,-0.0323666188837756,
0.0728390746383034));
#83410=CARTESIAN_POINT('',(0.0138708139121114,-0.0326943950436703,0.0729325682665746));
#83411=CARTESIAN_POINT('Origin',(0.00812378219310841,-0.0315241814719618,
0.07415));
#83412=CARTESIAN_POINT('',(0.0139658428707525,-0.0327114338379856,0.0727824010023186));
#83413=CARTESIAN_POINT('',(0.0139629083290093,-0.0326943950436593,0.0727699253755513));
#83414=CARTESIAN_POINT('Origin',(-0.00217966575170809,-0.0326395678566254,
0.076660115510202));
#83415=CARTESIAN_POINT('Origin',(-0.00221365196606142,-0.0326395673332969,
0.0765183462250016));
#83416=CARTESIAN_POINT('Origin',(-0.00222321968390699,-0.0326395683021248,
0.0764740585239133));
#83417=CARTESIAN_POINT('Ctrl Pts',(0.0137582679500085,-0.0332451089994433,
0.072996442348519));
#83418=CARTESIAN_POINT('Ctrl Pts',(0.0137147608113688,-0.0329451141710253,
0.0727839342413828));
#83419=CARTESIAN_POINT('Ctrl Pts',(0.0136553702925488,-0.0326442513127493,
0.0725753069828916));
#83420=CARTESIAN_POINT('Ctrl Pts',(0.0137028138756343,-0.0332451089994433,
0.0727526702302706));
#83421=CARTESIAN_POINT('Ctrl Pts',(0.0136501127211329,-0.0329451141710253,
0.0725422536077679));
#83422=CARTESIAN_POINT('Ctrl Pts',(0.0135817118448526,-0.0326442513127493,
0.0723364044230834));
#83423=CARTESIAN_POINT('Ctrl Pts',(0.0137022593348906,-0.0332451089994433,
0.0727502325090882));
#83424=CARTESIAN_POINT('Ctrl Pts',(0.0136494662402306,-0.0329451141710253,
0.0725398368014318));
#83425=CARTESIAN_POINT('Ctrl Pts',(0.0135809752603756,-0.0326442513127493,
0.0723340153974852));
#83426=CARTESIAN_POINT('',(0.0136939320316315,-0.0331951640388616,0.0727176746960267));
#83427=CARTESIAN_POINT('',(0.0136303825185583,-0.0328677532355029,0.072490036769806));
#83428=CARTESIAN_POINT('Origin',(-0.00233359358554788,-0.0326402808279494,
0.0776320078208817));
#83429=CARTESIAN_POINT('Origin',(0.0242157355164786,-0.0326944278779144,
0.0692986914638948));
#83430=CARTESIAN_POINT('',(0.0136651594291266,-0.0326943950436593,0.0726101093129251));
#83431=CARTESIAN_POINT('',(0.0136471206126884,-0.0326943950436693,0.0725502690998577));
#83432=CARTESIAN_POINT('',(0.0137237464515693,-0.0330220786163545,0.0728390746382951));
#83433=CARTESIAN_POINT('Origin',(-0.00250214209269808,-0.0326396682761368,
0.0771817367404983));
#83434=CARTESIAN_POINT('',(0.0137224236774251,-0.0331951640388587,0.0728393842935138));
#83435=CARTESIAN_POINT('Origin',(0.0244636883437946,-0.0331952026560045,
0.070324905639891));
#83436=CARTESIAN_POINT('',(0.0137081778545383,-0.0331951640388701,0.0727785294947803));
#83437=CARTESIAN_POINT('Ctrl Pts',(0.0140149585532739,-0.0330240426238172,
0.0730124407296694));
#83438=CARTESIAN_POINT('Ctrl Pts',(0.0139992875660548,-0.0329142774063519,
0.0729312840358132));
#83439=CARTESIAN_POINT('Ctrl Pts',(0.0139819310307149,-0.032804347972669,
0.0728504108454657));
#83440=CARTESIAN_POINT('Ctrl Pts',(0.0139629083290171,-0.0326943950436593,
0.0727699253755555));
#83441=CARTESIAN_POINT('Ctrl Pts',(0.0139174136495208,-0.0330240426238172,
0.0729547681388066));
#83442=CARTESIAN_POINT('Ctrl Pts',(0.0139009481661748,-0.0329142774063519,
0.0728749552210329));
#83443=CARTESIAN_POINT('Ctrl Pts',(0.0138828245182282,-0.032804347972669,
0.0727954429011437));
#83444=CARTESIAN_POINT('Ctrl Pts',(0.0138630631181841,-0.0326943950436593,
0.0727163336797551));
#83445=CARTESIAN_POINT('Ctrl Pts',(0.0138198687457676,-0.0330240426238172,
0.0728970955479438));
#83446=CARTESIAN_POINT('Ctrl Pts',(0.0138026087662949,-0.0329142774063519,
0.0728186264062527));
#83447=CARTESIAN_POINT('Ctrl Pts',(0.0137837180057414,-0.032804347972669,
0.0727404749568217));
#83448=CARTESIAN_POINT('Ctrl Pts',(0.0137632179073512,-0.0326943950436593,
0.0726627419839548));
#83449=CARTESIAN_POINT('Ctrl Pts',(0.0137223238420145,-0.0330240426238172,
0.072839422957081));
#83450=CARTESIAN_POINT('Ctrl Pts',(0.0137042693664149,-0.0329142774063519,
0.0727622975914724));
#83451=CARTESIAN_POINT('Ctrl Pts',(0.0136846114932546,-0.032804347972669,
0.0726855070124997));
#83452=CARTESIAN_POINT('Ctrl Pts',(0.0136633726965182,-0.0326943950436593,
0.0726091502881544));
#83453=CARTESIAN_POINT('',(0.013814033879078,-0.0326943950436693,0.0726900173442482));
#83454=CARTESIAN_POINT('Ctrl Pts',(0.0139658428675191,-0.0327114338383296,
0.0727824010030691));
#83455=CARTESIAN_POINT('Ctrl Pts',(0.0139240270651122,-0.0327619876830069,
0.0727921898862414));
#83456=CARTESIAN_POINT('Ctrl Pts',(0.0138829489822835,-0.032813156260251,
0.0728018060727214));
#83457=CARTESIAN_POINT('Ctrl Pts',(0.0138022336887511,-0.0329167375858767,
0.0728207011442764));
#83458=CARTESIAN_POINT('Ctrl Pts',(0.0137626286393872,-0.0329691088920621,
0.0728299725005327));
#83459=CARTESIAN_POINT('Ctrl Pts',(0.0137237464515224,-0.0330220786163187,
0.0728390746383033));
#83460=CARTESIAN_POINT('Ctrl Pts',(0.0136928625973565,-0.0331951640388604,
0.0727193978658153));
#83461=CARTESIAN_POINT('Ctrl Pts',(0.0136632858154489,-0.0330306422010619,
0.0726042606990196));
#83462=CARTESIAN_POINT('Ctrl Pts',(0.0136289755665096,-0.0328657861914645,
0.0724904443556262));
#83463=CARTESIAN_POINT('Ctrl Pts',(0.0136939320316322,-0.0331951640388604,
0.0727176746960298));
#83464=CARTESIAN_POINT('Ctrl Pts',(0.0136643196242942,-0.0330306422010619,
0.0726025154193661));
#83465=CARTESIAN_POINT('Ctrl Pts',(0.0136299728665419,-0.0328657861914645,
0.0724886784574339));
#83466=CARTESIAN_POINT('Ctrl Pts',(0.0138721285418799,-0.0331951640388604,
0.0724305482691856));
#83467=CARTESIAN_POINT('Ctrl Pts',(0.0138365799797552,-0.0330306422010619,
0.0723117048939216));
#83468=CARTESIAN_POINT('Ctrl Pts',(0.0137961498719495,-0.0328657861914645,
0.0721944323289454));
#83469=CARTESIAN_POINT('',(0.0138684426484039,-0.033178164828194,0.0724182736217006));
#83470=CARTESIAN_POINT('',(0.0138721285418775,-0.0331951640388588,0.0724305482691878));
#83471=CARTESIAN_POINT('Origin',(-0.00173044589592493,-0.0326412092727118,
0.0778644796218298));
#83472=CARTESIAN_POINT('Ctrl Pts',(0.0138684426478127,-0.033178164828644,
0.0724182736234421));
#83473=CARTESIAN_POINT('Ctrl Pts',(0.0138272888581054,-0.0331276811546767,
0.0724306794351338));
#83474=CARTESIAN_POINT('Ctrl Pts',(0.0137868781881544,-0.0330765663497773,
0.0724428612686628));
#83475=CARTESIAN_POINT('Ctrl Pts',(0.0137075083211081,-0.0329730614463219,
0.0724667872904782));
#83476=CARTESIAN_POINT('Ctrl Pts',(0.0136685811861452,-0.0329207133373689,
0.0724785218080462));
#83477=CARTESIAN_POINT('Ctrl Pts',(0.0136303825309352,-0.0328677532289385,
0.0724900367806722));
#83478=CARTESIAN_POINT('',(0.0137830302867645,-0.0331951640388701,0.0725741114826173));
#83479=CARTESIAN_POINT('Origin',(0.00812378219310841,-0.0315241814719618,
0.07415));
#83480=CARTESIAN_POINT('',(0.0138684426467313,-0.0332121607144407,0.0724182736215296));
#83481=CARTESIAN_POINT('',(0.0138647305447434,-0.0331951640388587,0.0724060068739042));
#83482=CARTESIAN_POINT('Origin',(-0.00171004585797308,-0.0326413662843359,
0.0779049762786882));
#83483=CARTESIAN_POINT('Origin',(-0.00214159684043429,-0.0326412095209627,
0.0765005709823073));
#83484=CARTESIAN_POINT('Origin',(-0.00214697489037763,-0.0326413667193929,
0.0764555462101574));
#83485=CARTESIAN_POINT('Ctrl Pts',(0.0136747225465772,-0.0337436976235975,
0.0726449464487163));
#83486=CARTESIAN_POINT('Ctrl Pts',(0.0136611858668398,-0.0336723290703325,
0.0725950204499091));
#83487=CARTESIAN_POINT('Ctrl Pts',(0.0136467533656632,-0.033601104548885,
0.072545346010154));
#83488=CARTESIAN_POINT('Ctrl Pts',(0.0136006732483236,-0.0333736987606857,
0.0723867453639679));
#83489=CARTESIAN_POINT('Ctrl Pts',(0.0135455676478104,-0.0331450831799191,
0.0722310504219283));
#83490=CARTESIAN_POINT('Ctrl Pts',(0.0136040721887949,-0.0337436976235975,
0.0724051370932999));
#83491=CARTESIAN_POINT('Ctrl Pts',(0.0135883786273709,-0.0336723290703325,
0.072355846534518));
#83492=CARTESIAN_POINT('Ctrl Pts',(0.0135718010230033,-0.033601104548885,
0.0723068462274921));
#83493=CARTESIAN_POINT('Ctrl Pts',(0.0135188720160962,-0.0333736987606857,
0.0721503979535722));
#83494=CARTESIAN_POINT('Ctrl Pts',(0.0134570523279748,-0.0331450831799191,
0.0719972448656332));
#83495=CARTESIAN_POINT('Ctrl Pts',(0.0136033656852171,-0.0337436976235975,
0.0724027389997458));
#83496=CARTESIAN_POINT('Ctrl Pts',(0.0135876505549762,-0.0336723290703325,
0.0723534547953641));
#83497=CARTESIAN_POINT('Ctrl Pts',(0.0135710514995767,-0.033601104548885,
0.0723044612296655));
#83498=CARTESIAN_POINT('Ctrl Pts',(0.0135180540037739,-0.0333736987606857,
0.0721480344794682));
#83499=CARTESIAN_POINT('Ctrl Pts',(0.0134561671747764,-0.0331450831799191,
0.0719949068100703));
#83500=CARTESIAN_POINT('',(0.0135930041633291,-0.0336938721132548,0.0723707484606003));
#83501=CARTESIAN_POINT('',(0.013515286543691,-0.0333679869945434,0.0721475500411451));
#83502=CARTESIAN_POINT('Ctrl Pts',(0.0135930041633334,-0.0336938721132649,
0.0723707484606119));
#83503=CARTESIAN_POINT('Ctrl Pts',(0.013586058909913,-0.0336629187933932,
0.0723493995216046));
#83504=CARTESIAN_POINT('Ctrl Pts',(0.0135789908711286,-0.033631995230104,
0.0723280980777477));
#83505=CARTESIAN_POINT('Ctrl Pts',(0.0135718010230072,-0.033601104548895,
0.072306846227504));
#83506=CARTESIAN_POINT('Ctrl Pts',(0.0135537592338432,-0.0335235892595454,
0.0722535180632687));
#83507=CARTESIAN_POINT('Ctrl Pts',(0.0135349182359992,-0.0334458668660369,
0.0722004074688427));
#83508=CARTESIAN_POINT('Ctrl Pts',(0.0135152865439844,-0.0333679869945385,
0.0721475500410432));
#83509=CARTESIAN_POINT('Ctrl Pts',(0.0135152717051053,-0.0333679692459108,
0.0721475081139829));
#83510=CARTESIAN_POINT('Ctrl Pts',(0.0135148489120665,-0.033339189537435,
0.0721476714659582));
#83511=CARTESIAN_POINT('Ctrl Pts',(0.0135145331783367,-0.0333104081060453,
0.0721477969351972));
#83512=CARTESIAN_POINT('Ctrl Pts',(0.0135141172959473,-0.0332532698004612,
0.0721479681621957));
#83513=CARTESIAN_POINT('Ctrl Pts',(0.0135140140017528,-0.0332249170152948,
0.0721480150847957));
#83514=CARTESIAN_POINT('Ctrl Pts',(0.0135140129628318,-0.0331960985410407,
0.0721480228294679));
#83515=CARTESIAN_POINT('Ctrl Pts',(0.0135140129739025,-0.0331956312514202,
0.072148022944742));
#83516=CARTESIAN_POINT('Ctrl Pts',(0.0135140130126346,-0.0331951640388587,
0.0721480230490263));
#83517=CARTESIAN_POINT('',(0.0135575342506988,-0.0331951640388587,0.072265201979884));
#83518=CARTESIAN_POINT('',(0.0135357736316764,-0.0331951640388687,0.0722066125144644));
#83519=CARTESIAN_POINT('',(0.0136303825164448,-0.0335216366567676,0.072490036785186));
#83520=CARTESIAN_POINT('Origin',(-0.00192359277031526,-0.0326434571527816,
0.0784435666451609));
#83521=CARTESIAN_POINT('',(0.0136290817962303,-0.0336938721132327,0.0724904288867702));
#83522=CARTESIAN_POINT('Origin',(0.0240849090392403,-0.0336938867896239,
0.0693385236516236));
#83523=CARTESIAN_POINT('',(0.0136110429797897,-0.0336938721132537,0.0724305886736952));
#83524=CARTESIAN_POINT('Ctrl Pts',(0.013931905483755,-0.0335235895815172,
0.072644774488413));
#83525=CARTESIAN_POINT('Ctrl Pts',(0.0139111830910717,-0.0334144449262748,
0.0725648142361747));
#83526=CARTESIAN_POINT('Ctrl Pts',(0.0138887849722353,-0.0333049234473147,
0.0724851902283316));
#83527=CARTESIAN_POINT('Ctrl Pts',(0.0138647305447509,-0.0331951640388587,
0.0724060068739076));
#83528=CARTESIAN_POINT('Ctrl Pts',(0.0138309316188954,-0.0335235895815172,
0.0725933405394907));
#83529=CARTESIAN_POINT('Ctrl Pts',(0.0138095011366411,-0.0334144449262748,
0.0725147703913015));
#83530=CARTESIAN_POINT('Ctrl Pts',(0.013786422833228,-0.0333049234473147,
0.0724365527131662));
#83531=CARTESIAN_POINT('Ctrl Pts',(0.013761717158803,-0.0331951640388587,
0.0723587901946304));
#83532=CARTESIAN_POINT('Ctrl Pts',(0.0137299577540358,-0.0335235895815172,
0.0725419065905685));
#83533=CARTESIAN_POINT('Ctrl Pts',(0.0137078191822104,-0.0334144449262748,
0.0724647265464284));
#83534=CARTESIAN_POINT('Ctrl Pts',(0.0136840606942207,-0.0333049234473147,
0.0723879151980009));
#83535=CARTESIAN_POINT('Ctrl Pts',(0.0136587037728552,-0.0331951640388587,
0.0723115735153532));
#83536=CARTESIAN_POINT('Ctrl Pts',(0.0136289838891762,-0.0335235895815172,
0.0724904726416463));
#83537=CARTESIAN_POINT('Ctrl Pts',(0.0136061372277798,-0.0334144449262748,
0.0724146827015552));
#83538=CARTESIAN_POINT('Ctrl Pts',(0.0135816985552134,-0.0333049234473147,
0.0723392776828355));
#83539=CARTESIAN_POINT('Ctrl Pts',(0.0135556903869073,-0.0331951640388587,
0.072264356836076));
#83540=CARTESIAN_POINT('',(0.0137111323977311,-0.0331951640388687,0.0723356044269041));
#83541=CARTESIAN_POINT('Ctrl Pts',(0.013868442643727,-0.0332121607145954,
0.0724182736224286));
#83542=CARTESIAN_POINT('Ctrl Pts',(0.0138273580817934,-0.0332625444108882,
0.0724306585527866));
#83543=CARTESIAN_POINT('Ctrl Pts',(0.0137869814713308,-0.033313530074506,
0.0724428300713604));
#83544=CARTESIAN_POINT('Ctrl Pts',(0.0137076121026617,-0.0334167203140572,
0.0724667559466105));
#83545=CARTESIAN_POINT('Ctrl Pts',(0.0136686500850658,-0.0334688847587245,
0.0724785010365378));
#83546=CARTESIAN_POINT('Ctrl Pts',(0.0136303825157164,-0.0335216366562309,
0.0724900367852243));
#83547=CARTESIAN_POINT('Ctrl Pts',(0.0135925313019532,-0.033693872113239,
0.0723716294356234));
#83548=CARTESIAN_POINT('Ctrl Pts',(0.013582121908914,-0.0336474569764958,
0.0723396190323659));
#83549=CARTESIAN_POINT('Ctrl Pts',(0.0135713385069467,-0.033601104548885,
0.0723077326775702));
#83550=CARTESIAN_POINT('Ctrl Pts',(0.013544037412425,-0.0334837508592656,
0.07222700375836));
#83551=CARTESIAN_POINT('Ctrl Pts',(0.0135143561412772,-0.0333660264659097,
0.0721471192773766));
#83552=CARTESIAN_POINT('Ctrl Pts',(0.0135930041633354,-0.033693872113239,
0.0723707484606199));
#83553=CARTESIAN_POINT('Ctrl Pts',(0.0135825896136571,-0.0336474569764958,
0.0723387352895478));
#83554=CARTESIAN_POINT('Ctrl Pts',(0.0135718010230033,-0.033601104548885,
0.0723068462274921));
#83555=CARTESIAN_POINT('Ctrl Pts',(0.0135444867919205,-0.0334837508592656,
0.0722261104541222));
#83556=CARTESIAN_POINT('Ctrl Pts',(0.0135147921868771,-0.0333660264659097,
0.0721462195112524));
#83557=CARTESIAN_POINT('Ctrl Pts',(0.0137537791223436,-0.033693872113239,
0.0720712130673268));
#83558=CARTESIAN_POINT('Ctrl Pts',(0.013741611292612,-0.0336474569764958,
0.0720382588270689));
#83559=CARTESIAN_POINT('Ctrl Pts',(0.0137290585256377,-0.033601104548885,
0.0720054492846667));
#83560=CARTESIAN_POINT('Ctrl Pts',(0.0136972778057211,-0.0334837508592656,
0.0719223830666911));
#83561=CARTESIAN_POINT('Ctrl Pts',(0.0136630496172911,-0.0333660264659097,
0.0718402950539));
#83562=CARTESIAN_POINT('',(0.0137483708743525,-0.0336769361243753,0.0720609805728954));
#83563=CARTESIAN_POINT('',(0.0137528202259598,-0.0336938721132327,0.0720729995607336));
#83564=CARTESIAN_POINT('Ctrl Pts',(0.0137483708743524,-0.033676936124375,
0.0720609805728951));
#83565=CARTESIAN_POINT('Ctrl Pts',(0.0137491146280473,-0.0336797586670014,
0.0720629830954948));
#83566=CARTESIAN_POINT('Ctrl Pts',(0.0137498572841759,-0.0336825812712824,
0.0720649859395555));
#83567=CARTESIAN_POINT('Ctrl Pts',(0.0137513404008548,-0.0336882265995455,
0.0720689922679143));
#83568=CARTESIAN_POINT('Ctrl Pts',(0.0137520808614061,-0.0336910493235148,
0.0720709957522001));
#83569=CARTESIAN_POINT('Ctrl Pts',(0.0137528202259612,-0.0336938721132335,
0.0720729995607319));
#83570=CARTESIAN_POINT('Ctrl Pts',(0.0137483708743525,-0.0336769361243753,
0.0720609805728955));
#83571=CARTESIAN_POINT('Ctrl Pts',(0.0137090804728812,-0.0336279018378422,
0.0720755733576525));
#83572=CARTESIAN_POINT('Ctrl Pts',(0.0136692248297723,-0.0335767825754289,
0.0720903760778966));
#83573=CARTESIAN_POINT('Ctrl Pts',(0.013591130687504,-0.0334733171799211,
0.0721193808975532));
#83574=CARTESIAN_POINT('Ctrl Pts',(0.0135528397023023,-0.0334209631321962,
0.0721336024907219));
#83575=CARTESIAN_POINT('Ctrl Pts',(0.0135152865462182,-0.0333679869844681,
0.0721475500479664));
#83576=CARTESIAN_POINT('',(0.0136729121946544,-0.0336938721132538,0.0722218740106769));
#83577=CARTESIAN_POINT('Origin',(0.00812378219310841,-0.0315241814719618,
0.07415));
#83578=CARTESIAN_POINT('',(0.0137483708731438,-0.0337108120655536,0.0720609805733511));
#83579=CARTESIAN_POINT('',(0.0137438958601233,-0.0336938721132327,0.0720489711163712));
#83580=CARTESIAN_POINT('Origin',(-0.00197825994128331,-0.0345562523539059,
0.0767097827342115));
#83581=CARTESIAN_POINT('Ctrl Pts',(0.0137438958601364,-0.0336938721132376,
0.0720489711163732));
#83582=CARTESIAN_POINT('Ctrl Pts',(0.0137446437846619,-0.0336910492993832,
0.0720509717651413));
#83583=CARTESIAN_POINT('Ctrl Pts',(0.0137453906576377,-0.0336882265874791,
0.0720529728580518));
#83584=CARTESIAN_POINT('Ctrl Pts',(0.0137468823256519,-0.0336825812712948,
0.0720569760006223));
#83585=CARTESIAN_POINT('Ctrl Pts',(0.0137476271206561,-0.0336797586670076,
0.0720589780502916));
#83586=CARTESIAN_POINT('Ctrl Pts',(0.0137483708743526,-0.033676936124375,
0.0720609805728957));
#83587=CARTESIAN_POINT('Origin',(-0.00120002537656662,-0.0345562520009487,
0.078805140333065));
#83588=CARTESIAN_POINT('Ctrl Pts',(0.0135692825547336,-0.034243627687391,
0.0722994187908822));
#83589=CARTESIAN_POINT('Ctrl Pts',(0.013499486733833,-0.033943005420181,
0.0720940383590042));
#83590=CARTESIAN_POINT('Ctrl Pts',(0.0134144190998935,-0.0336441434784053,
0.0718944986986117));
#83591=CARTESIAN_POINT('Ctrl Pts',(0.0134837159642933,-0.034243627687391,
0.0720645180488647));
#83592=CARTESIAN_POINT('Ctrl Pts',(0.013405060715858,-0.033943005420181,
0.071862364814146));
#83593=CARTESIAN_POINT('Ctrl Pts',(0.0133114019088017,-0.0336441434784053,
0.0716667105111667));
#83594=CARTESIAN_POINT('Ctrl Pts',(0.0134828602983889,-0.034243627687391,
0.0720621690414445));
#83595=CARTESIAN_POINT('Ctrl Pts',(0.0134041164556783,-0.033943005420181,
0.0718600480786975));
#83596=CARTESIAN_POINT('Ctrl Pts',(0.0133103717368908,-0.0336441434784053,
0.0716644326292922));
#83597=CARTESIAN_POINT('',(0.0134704917745694,-0.0341934961088741,0.0720308441181655));
#83598=CARTESIAN_POINT('',(0.013378912770339,-0.0338664212890971,0.071812966062671));
#83599=CARTESIAN_POINT('Origin',(-0.00226744349518236,-0.0345610818078965,
0.0777203509298478));
#83600=CARTESIAN_POINT('Origin',(0.0233989667081556,-0.0336938005044555,
0.0673568171623248));
#83601=CARTESIAN_POINT('',(0.0134284645353448,-0.0336938721132327,0.071927733083546));
#83602=CARTESIAN_POINT('',(0.0134030679929601,-0.0336938721132427,0.0718706255916271));
#83603=CARTESIAN_POINT('',(0.0135152865462201,-0.0340203938281605,0.0721475500479715));
#83604=CARTESIAN_POINT('Origin',(-0.00235931595101076,-0.0345589643245916,
0.0772480342467954));
#83605=CARTESIAN_POINT('',(0.013514013012634,-0.034193496108874,0.0721480230490246));
#83606=CARTESIAN_POINT('Origin',(0.023843989668344,-0.0341934220717674,
0.068311383821032));
#83607=CARTESIAN_POINT('',(0.0134922523936117,-0.0341934961088841,0.0720894335836051));
#83608=CARTESIAN_POINT('Ctrl Pts',(0.0138259314386953,-0.0340223579322397,
0.0722830522286004));
#83609=CARTESIAN_POINT('Ctrl Pts',(0.0138001813597235,-0.0339125849573575,
0.0722044047186742));
#83610=CARTESIAN_POINT('Ctrl Pts',(0.0137728215543302,-0.0338030433565231,
0.0721263454402424));
#83611=CARTESIAN_POINT('Ctrl Pts',(0.0137438958601307,-0.0336938721132327,
0.072048971116374));
#83612=CARTESIAN_POINT('Ctrl Pts',(0.0137219272490947,-0.0340223579322397,
0.0722380599139648));
#83613=CARTESIAN_POINT('Ctrl Pts',(0.0136955566087592,-0.0339125849573575,
0.0721608468930675));
#83614=CARTESIAN_POINT('Ctrl Pts',(0.013667606368653,-0.0338030433565231,
0.072084233939844));
#83615=CARTESIAN_POINT('Ctrl Pts',(0.0136381209574983,-0.0336938721132327,
0.0720083158608237));
#83616=CARTESIAN_POINT('Ctrl Pts',(0.0136179230594941,-0.0340223579322397,
0.0721930675993291));
#83617=CARTESIAN_POINT('Ctrl Pts',(0.0135909318577949,-0.0339125849573575,
0.0721172890674607));
#83618=CARTESIAN_POINT('Ctrl Pts',(0.0135623911829759,-0.0338030433565231,
0.0720421224394456));
#83619=CARTESIAN_POINT('Ctrl Pts',(0.0135323460548659,-0.0336938721132327,
0.0719676606052735));
#83620=CARTESIAN_POINT('Ctrl Pts',(0.0135139188698935,-0.0340223579322397,
0.0721480752846935));
#83621=CARTESIAN_POINT('Ctrl Pts',(0.0134863071068306,-0.0339125849573575,
0.072073731241854));
#83622=CARTESIAN_POINT('Ctrl Pts',(0.0134571759972988,-0.0338030433565231,
0.0720000109390472));
#83623=CARTESIAN_POINT('Ctrl Pts',(0.0134265711522335,-0.0336938721132327,
0.0719270053497232));
#83624=CARTESIAN_POINT('',(0.0135861801977441,-0.0336938721132427,0.0719883520999686));
#83625=CARTESIAN_POINT('Ctrl Pts',(0.0137483708697607,-0.033710812066267,
0.0720609805746009));
#83626=CARTESIAN_POINT('Ctrl Pts',(0.0137080620149036,-0.0337611408993504,
0.0720759516214903));
#83627=CARTESIAN_POINT('Ctrl Pts',(0.0136684887072169,-0.033812108877969,
0.0720906494799894));
#83628=CARTESIAN_POINT('Ctrl Pts',(0.013590777135298,-0.0339153382773238,
0.0721195122098083));
#83629=CARTESIAN_POINT('Ctrl Pts',(0.013552671748,-0.0339675558473113,0.0721336648703589));
#83630=CARTESIAN_POINT('Ctrl Pts',(0.0135152865461808,-0.0340203938281304,
0.0721475500479803));
#83631=CARTESIAN_POINT('Ctrl Pts',(0.0134696467056173,-0.0341934961088741,
0.0720326878186427));
#83632=CARTESIAN_POINT('Ctrl Pts',(0.0134258729446295,-0.03402875161944,
0.0719221662821851));
#83633=CARTESIAN_POINT('Ctrl Pts',(0.0133775686485661,-0.033864463329982,
0.0718135483870032));
#83634=CARTESIAN_POINT('Ctrl Pts',(0.0134704917745694,-0.0341934961088741,
0.0720308441181656));
#83635=CARTESIAN_POINT('Ctrl Pts',(0.0134266798965269,-0.03402875161944,
0.0719203051105733));
#83636=CARTESIAN_POINT('Ctrl Pts',(0.013378336793884,-0.033864463329982,
0.0718116713345922));
#83637=CARTESIAN_POINT('Ctrl Pts',(0.0136112966685901,-0.0341934961088741,
0.07172364782412));
#83638=CARTESIAN_POINT('Ctrl Pts',(0.0135611337492273,-0.03402875161944,
0.0716101977862927));
#83639=CARTESIAN_POINT('Ctrl Pts',(0.01350632471702,-0.033864463329982,
0.0714989179608504));
#83640=CARTESIAN_POINT('',(0.0136061014179077,-0.0341764758832425,0.0717119319311992));
#83641=CARTESIAN_POINT('',(0.0136112966685892,-0.0341934961088741,0.0717236478241218));
#83642=CARTESIAN_POINT('Origin',(-0.00173113244827768,-0.0345621027123507,
0.077972170446947));
#83643=CARTESIAN_POINT('Ctrl Pts',(0.0136061014177631,-0.0341764758837528,
0.0717119319330092));
#83644=CARTESIAN_POINT('Ctrl Pts',(0.0135668805667642,-0.034126005004375,
0.0717293740378841));
#83645=CARTESIAN_POINT('Ctrl Pts',(0.013528341482203,-0.0340749269154831,
0.0717465129927412));
#83646=CARTESIAN_POINT('Ctrl Pts',(0.0134525969032517,-0.0339715436319927,
0.0717801977176824));
#83647=CARTESIAN_POINT('Ctrl Pts',(0.0134154201420956,-0.0339192778252677,
0.0717967307031266));
#83648=CARTESIAN_POINT('Ctrl Pts',(0.0133789127738472,-0.0338664212873856,
0.0718129660649879));
#83649=CARTESIAN_POINT('',(0.0135408942215893,-0.0341934961088841,0.0718772459711537));
#83650=CARTESIAN_POINT('Origin',(0.00812378219310841,-0.0315241814719618,
0.07415));
#83651=CARTESIAN_POINT('',(0.0136061014168916,-0.0342105180190533,0.0717119319307304));
#83652=CARTESIAN_POINT('',(0.0136008811544452,-0.0341934961088739,0.071700227159973));
#83653=CARTESIAN_POINT('Origin',(-0.00171761757791809,-0.0345621716515909,
0.0780154343705276));
#83654=CARTESIAN_POINT('Origin',(-0.00131495569966945,-0.0345621032136264,
0.0789080016038157));
#83655=CARTESIAN_POINT('Origin',(-0.00133802805002015,-0.0345621721622157,
0.0788689880464507));
#83656=CARTESIAN_POINT('Ctrl Pts',(0.0134290740563898,-0.0346945769586965,
0.071929103672409));
#83657=CARTESIAN_POINT('Ctrl Pts',(0.01338255649361,-0.0345275153362943,
0.0718179822102097));
#83658=CARTESIAN_POINT('Ctrl Pts',(0.0133325322312999,-0.0343603235965184,
0.0717082949408414));
#83659=CARTESIAN_POINT('Ctrl Pts',(0.0132791540405434,-0.0341934961088739,
0.0716003640716408));
#83660=CARTESIAN_POINT('Ctrl Pts',(0.0133950088260619,-0.0346945769586965,
0.0718525034866133));
#83661=CARTESIAN_POINT('Ctrl Pts',(0.0133468868417216,-0.0345275153362943,
0.0717420955343021));
#83662=CARTESIAN_POINT('Ctrl Pts',(0.0132952801820946,-0.0343603235965184,
0.0716331724169535));
#83663=CARTESIAN_POINT('Ctrl Pts',(0.013240346264704,-0.0341934961088739,
0.0715260540123242));
#83664=CARTESIAN_POINT('Ctrl Pts',(0.0133609435957339,-0.0346945769586965,
0.0717759033008173));
#83665=CARTESIAN_POINT('Ctrl Pts',(0.0133112171898329,-0.0345275153362943,
0.0716662088583944));
#83666=CARTESIAN_POINT('Ctrl Pts',(0.013258028132889,-0.0343603235965184,
0.0715580498930654));
#83667=CARTESIAN_POINT('Ctrl Pts',(0.0132015384888642,-0.0341934961088739,
0.0714517439530069));
#83668=CARTESIAN_POINT('Ctrl Pts',(0.0133268783654062,-0.0346945769586965,
0.0716993031150217));
#83669=CARTESIAN_POINT('Ctrl Pts',(0.0132755475379449,-0.0345275153362943,
0.0715903221824868));
#83670=CARTESIAN_POINT('Ctrl Pts',(0.0132207760836841,-0.0343603235965184,
0.0714829273691776));
#83671=CARTESIAN_POINT('Ctrl Pts',(0.013162730713025,-0.0341934961088739,
0.071377433893691));
#83672=CARTESIAN_POINT('',(0.0133268783657636,-0.0346945769586966,0.0716993031158257));
#83673=CARTESIAN_POINT('',(0.0132217993964057,-0.0343667727832827,0.0714876052893058));
#83674=CARTESIAN_POINT('Origin',(-0.00180506282623017,-0.0345626461567213,
0.0790288053154406));
#83675=CARTESIAN_POINT('Origin',(0.0230184725557128,-0.0341934771027923,
0.0663713712913561));
#83676=CARTESIAN_POINT('',(0.0132784596622649,-0.0341934961088739,0.07159903445947));
#83677=CARTESIAN_POINT('',(0.0132495274250681,-0.0341934961088839,0.0715436343182328));
#83678=CARTESIAN_POINT('',(0.01337891277113,-0.0345211942962645,0.0718129660661669));
#83679=CARTESIAN_POINT('Origin',(-0.00199740023052754,-0.0345625596122438,
0.0785881279815846));
#83680=CARTESIAN_POINT('',(0.0133776714505554,-0.0346945769586885,0.0718135180996884));
#83681=CARTESIAN_POINT('Origin',(0.0234866728168181,-0.0346945685853836,
0.0673178972777572));
#83682=CARTESIAN_POINT('',(0.0133522749081695,-0.0346945769587025,0.0717564106077671));
#83683=CARTESIAN_POINT('Ctrl Pts',(0.0136974525729759,-0.0345231616327842,
0.0719286944161906));
#83684=CARTESIAN_POINT('Ctrl Pts',(0.0136668350028512,-0.0344132092796988,
0.0718518692171043));
#83685=CARTESIAN_POINT('Ctrl Pts',(0.0136346299438081,-0.034303273855898,
0.0717756812821324));
#83686=CARTESIAN_POINT('Ctrl Pts',(0.013600881154452,-0.0341934961088739,
0.0717002271599751));
#83687=CARTESIAN_POINT('Ctrl Pts',(0.0135908286963147,-0.0345231616327842,
0.071890321443089));
#83688=CARTESIAN_POINT('Ctrl Pts',(0.0135596822087806,-0.0344132092796988,
0.071814965904028));
#83689=CARTESIAN_POINT('Ctrl Pts',(0.0135269786583763,-0.034303273855898,
0.0717402584934932));
#83690=CARTESIAN_POINT('Ctrl Pts',(0.0134927623937467,-0.0341934961088739,
0.0716662938471031));
#83691=CARTESIAN_POINT('Ctrl Pts',(0.0134842048196535,-0.0345231616327842,
0.0718519484699873));
#83692=CARTESIAN_POINT('Ctrl Pts',(0.0134525294147101,-0.0344132092796988,
0.0717780625909517));
#83693=CARTESIAN_POINT('Ctrl Pts',(0.0134193273729444,-0.034303273855898,
0.071704835704854));
#83694=CARTESIAN_POINT('Ctrl Pts',(0.0133846436330414,-0.0341934961088739,
0.0716323605342312));
#83695=CARTESIAN_POINT('Ctrl Pts',(0.0133775809429924,-0.0345231616327842,
0.0718135754968856));
#83696=CARTESIAN_POINT('Ctrl Pts',(0.0133453766206395,-0.0344132092796988,
0.0717411592778754));
#83697=CARTESIAN_POINT('Ctrl Pts',(0.0133116760875126,-0.034303273855898,
0.0716694129162147));
#83698=CARTESIAN_POINT('Ctrl Pts',(0.0132765248723361,-0.0341934961088739,
0.0715984272213592));
#83699=CARTESIAN_POINT('',(0.0134396704083651,-0.0341934961088839,0.0716496308097315));
#83700=CARTESIAN_POINT('Ctrl Pts',(0.0136061014137292,-0.0342105180195373,
0.0717119319321293));
#83701=CARTESIAN_POINT('Ctrl Pts',(0.0135668364651007,-0.0342610556240407,
0.0717293936328412));
#83702=CARTESIAN_POINT('Ctrl Pts',(0.0135282761056708,-0.0343122189868325,
0.0717465419923636));
#83703=CARTESIAN_POINT('Ctrl Pts',(0.0134525307637046,-0.034415811969512,
0.0717802270610555));
#83704=CARTESIAN_POINT('Ctrl Pts',(0.0134153767617617,-0.034468199045001,
0.0717967499926991));
#83705=CARTESIAN_POINT('Ctrl Pts',(0.0133789127710976,-0.0345211942962416,
0.0718129660661687));
#83706=CARTESIAN_POINT('Ctrl Pts',(0.0133261509086851,-0.0346945769586932,
0.0717011957789349));
#83707=CARTESIAN_POINT('Ctrl Pts',(0.0132755236141497,-0.0345296777077528,
0.0715936404868541));
#83708=CARTESIAN_POINT('Ctrl Pts',(0.0132204942209498,-0.0343648066252516,
0.0714882695720313));
#83709=CARTESIAN_POINT('Ctrl Pts',(0.0133268783657674,-0.0346945769586932,
0.0716993031158339));
#83710=CARTESIAN_POINT('Ctrl Pts',(0.0132762119417616,-0.0345296777077528,
0.0715917327840927));
#83711=CARTESIAN_POINT('Ctrl Pts',(0.0132211428309239,-0.0343648066252516,
0.0714863484597176));
#83712=CARTESIAN_POINT('Ctrl Pts',(0.0134481163985928,-0.0346945769586932,
0.0713838717910554));
#83713=CARTESIAN_POINT('Ctrl Pts',(0.0133909286551414,-0.0345296777077528,
0.0712737949487716));
#83714=CARTESIAN_POINT('Ctrl Pts',(0.0133292402008602,-0.0343648066252516,
0.0711661757877611));
#83715=CARTESIAN_POINT('',(0.0134421957527042,-0.0346775396665007,0.0713725052290604));
#83716=CARTESIAN_POINT('',(0.0134481163985908,-0.0346945769586886,0.0713838717910534));
#83717=CARTESIAN_POINT('Origin',(-0.00120217637793559,-0.0345626618147741,
0.0791926885719967));
#83718=CARTESIAN_POINT('Ctrl Pts',(0.0134421957525685,-0.0346775396670096,
0.0713725052308742));
#83719=CARTESIAN_POINT('Ctrl Pts',(0.0134041175267979,-0.0346269749928325,
0.0713923912643912));
#83720=CARTESIAN_POINT('Ctrl Pts',(0.0133667160526948,-0.0345757902891079,
0.0714119239105586));
#83721=CARTESIAN_POINT('Ctrl Pts',(0.0132932357257123,-0.0344721681088438,
0.0714502983617085));
#83722=CARTESIAN_POINT('Ctrl Pts',(0.0132571856779471,-0.0344197714289854,
0.0714691251171155));
#83723=CARTESIAN_POINT('Ctrl Pts',(0.0132217993966978,-0.0343667727831633,
0.0714876052895225));
#83724=CARTESIAN_POINT('',(0.0133874973821872,-0.0346945769587026,0.0715415874534496));
#83725=CARTESIAN_POINT('Origin',(0.00812378219310841,-0.0315241814719618,
0.07415));
#83726=CARTESIAN_POINT('',(0.0134421957513162,-0.0347116136489609,0.0713725052289522));
#83727=CARTESIAN_POINT('',(0.0134362508414153,-0.0346945769586885,0.0713611513377796));
#83728=CARTESIAN_POINT('Origin',(-0.00117956073235415,-0.034562669603157,
0.0792319529103707));
#83729=CARTESIAN_POINT('Origin',(-0.00134356747308092,-0.0345626622155451,
0.0789219522010525));
#83730=CARTESIAN_POINT('Origin',(-0.00136286474894159,-0.0345626702618841,
0.0788809552601594));
#83731=CARTESIAN_POINT('Ctrl Pts',(0.0132955128131795,-0.0352450361874068,
0.0716336616595897));
#83732=CARTESIAN_POINT('Ctrl Pts',(0.013200607555348,-0.0349452760959492,
0.0714386066385497));
#83733=CARTESIAN_POINT('Ctrl Pts',(0.0130912795710791,-0.0346444289841739,
0.0712512544006321));
#83734=CARTESIAN_POINT('Ctrl Pts',(0.0132943694554156,-0.0352450361874068,
0.0716314384337749));
#83735=CARTESIAN_POINT('Ctrl Pts',(0.0131993803472466,-0.0349452760959492,
0.0714364265351804));
#83736=CARTESIAN_POINT('Ctrl Pts',(0.0130899719990091,-0.0346444289841739,
0.0712491236131528));
#83737=CARTESIAN_POINT('Ctrl Pts',(0.0131800336772834,-0.0352450361874068,
0.0714091158489037));
#83738=CARTESIAN_POINT('Ctrl Pts',(0.0130766595352339,-0.0349452760959492,
0.0712184161949422));
#83739=CARTESIAN_POINT('Ctrl Pts',(0.0129592147900247,-0.0346444289841739,
0.0710360448619749));
#83740=CARTESIAN_POINT('',(0.01316274824,-0.0351951633467201,0.0713774613991309));
#83741=CARTESIAN_POINT('',(0.0130445664770105,-0.0348678972925434,0.071172751768612));
#83742=CARTESIAN_POINT('Origin',(-0.00106747175712535,-0.0345631633301949,
0.080204957386172));
#83743=CARTESIAN_POINT('Origin',(0.0224986601168685,-0.0346946199341027,
0.0654526903452147));
#83744=CARTESIAN_POINT('',(0.0131081116410078,-0.0346945769330288,0.0712804033466476));
#83745=CARTESIAN_POINT('',(0.0130757578871117,-0.0346945769458128,0.0712269291875016));
#83746=CARTESIAN_POINT('',(0.0132217993964998,-0.0350221583435276,0.0714876052896075));
#83747=CARTESIAN_POINT('Origin',(-0.00135078810670648,-0.0345628458719986,
0.0798157290478429));
#83748=CARTESIAN_POINT('',(0.0132207044192628,-0.035195136029876,0.0714881805439839));
#83749=CARTESIAN_POINT('Origin',(0.0229879493288178,-0.0351951838366849,
0.0663873207389187));
#83750=CARTESIAN_POINT('',(0.0131627307160144,-0.0351951371328747,0.0713774338991642));
#83751=CARTESIAN_POINT('Ctrl Pts',(0.0135469768650149,-0.0350241211494343,
0.0715831031281574));
#83752=CARTESIAN_POINT('Ctrl Pts',(0.0135116189130739,-0.0349144232818962,
0.0715084008451483));
#83753=CARTESIAN_POINT('Ctrl Pts',(0.0134746956481253,-0.0348045283579412,
0.0714343847233541));
#83754=CARTESIAN_POINT('Ctrl Pts',(0.0134362508362562,-0.0346945769439157,
0.0713611513279417));
#83755=CARTESIAN_POINT('Ctrl Pts',(0.0134381538982397,-0.0350241211494343,
0.071551500854417));
#83756=CARTESIAN_POINT('Ctrl Pts',(0.0134023606379354,-0.0349144232818962,
0.071478297563156));
#83757=CARTESIAN_POINT('Ctrl Pts',(0.0133650327893009,-0.0348045283579412,
0.0714057903284638));
#83758=CARTESIAN_POINT('Ctrl Pts',(0.0133262147085638,-0.0346945769439157,
0.0713340738020986));
#83759=CARTESIAN_POINT('Ctrl Pts',(0.0133293309314644,-0.0350241211494343,
0.0715198985806766));
#83760=CARTESIAN_POINT('Ctrl Pts',(0.0132931023627968,-0.0349144232818962,
0.0714481942811638));
#83761=CARTESIAN_POINT('Ctrl Pts',(0.0132553699304765,-0.0348045283579412,
0.0713771959335734));
#83762=CARTESIAN_POINT('Ctrl Pts',(0.0132161785808714,-0.0346945769439157,
0.0713069962762554));
#83763=CARTESIAN_POINT('Ctrl Pts',(0.0132205079646892,-0.0350241211494343,
0.0714882963069362));
#83764=CARTESIAN_POINT('Ctrl Pts',(0.0131838440876582,-0.0349144232818962,
0.0714180909991716));
#83765=CARTESIAN_POINT('Ctrl Pts',(0.0131457070716521,-0.0348045283579412,
0.0713486015386831));
#83766=CARTESIAN_POINT('Ctrl Pts',(0.013106142453179,-0.0346945769439157,
0.0712799187504123));
#83767=CARTESIAN_POINT('',(0.0132721812414348,-0.0346945769458128,0.0713207773424309));
#83768=CARTESIAN_POINT('Ctrl Pts',(0.0134421957483956,-0.0347116136492782,
0.0713725052304696));
#83769=CARTESIAN_POINT('Ctrl Pts',(0.0134041326384174,-0.0347621546531421,
0.0713923833553611));
#83770=CARTESIAN_POINT('Ctrl Pts',(0.0133667387807672,-0.0348133084095238,
0.0714119119691021));
#83771=CARTESIAN_POINT('Ctrl Pts',(0.0132932583621568,-0.0349168561544572,
0.0714502864723691));
#83772=CARTESIAN_POINT('Ctrl Pts',(0.0132572009473367,-0.0349692089015923,
0.0714691171405796));
#83773=CARTESIAN_POINT('Ctrl Pts',(0.0132217993964582,-0.0350221583435,
0.0714876052896068));
#83774=CARTESIAN_POINT('Ctrl Pts',(0.0131622926126873,-0.0351951371254981,
0.0713788297767868));
#83775=CARTESIAN_POINT('Ctrl Pts',(0.0131241291376846,-0.0350856248736071,
0.0713094413773164));
#83776=CARTESIAN_POINT('Ctrl Pts',(0.013084500336438,-0.0349758427080755,
0.0712407847106068));
#83777=CARTESIAN_POINT('Ctrl Pts',(0.0130434517796293,-0.0348659306897848,
0.0711729506531316));
#83778=CARTESIAN_POINT('Ctrl Pts',(0.0131869140273343,-0.0351951371254981,
0.0713003807067396));
#83779=CARTESIAN_POINT('Ctrl Pts',(0.0131476701823497,-0.0350856248736071,
0.0712306532307539));
#83780=CARTESIAN_POINT('Ctrl Pts',(0.0131069531167853,-0.0349758427080755,
0.0711616795363528));
#83781=CARTESIAN_POINT('Ctrl Pts',(0.0130648097707083,-0.0348659306897848,
0.0710935509877194));
#83782=CARTESIAN_POINT('Ctrl Pts',(0.0132115354419813,-0.0351951371254981,
0.0712219316366923));
#83783=CARTESIAN_POINT('Ctrl Pts',(0.0131712112270149,-0.0350856248736071,
0.0711518650841914));
#83784=CARTESIAN_POINT('Ctrl Pts',(0.0131294058971327,-0.0349758427080755,
0.0710825743620988));
#83785=CARTESIAN_POINT('Ctrl Pts',(0.0130861677617873,-0.0348659306897848,
0.0710141513223072));
#83786=CARTESIAN_POINT('Ctrl Pts',(0.0132361568566283,-0.0351951371254981,
0.071143482566645));
#83787=CARTESIAN_POINT('Ctrl Pts',(0.01319475227168,-0.0350856248736071,
0.0710730769376289));
#83788=CARTESIAN_POINT('Ctrl Pts',(0.01315185867748,-0.0349758427080755,
0.0710034691878447));
#83789=CARTESIAN_POINT('Ctrl Pts',(0.0131075257528663,-0.0348659306897848,
0.0709347516568949));
#83790=CARTESIAN_POINT('Origin',(0.0175947305641669,-0.0308609197384946,
0.0684197418359026));
#83791=CARTESIAN_POINT('',(0.0131947428563328,-0.0351951371254981,0.0712754363904484));
#83792=CARTESIAN_POINT('Origin',(0.00736988752340133,-0.03518404674411,
0.0747716015423331));
#83793=CARTESIAN_POINT('Origin',(0.017927210120105,-0.0352322613839716,
0.0672897386084101));
#83794=CARTESIAN_POINT('',(0.0129178964449081,-0.0351951142564678,0.0709728498423726));
#83795=CARTESIAN_POINT('',(0.0128467975461564,-0.0351951372916786,0.0708704228969463));
#83796=CARTESIAN_POINT('Origin',(0.00781164895014946,-0.0352875127425782,
0.0740136130634983));
#83797=CARTESIAN_POINT('Origin',(0.0111440472267538,-0.0298325076523627,
0.081018274121231));
#83798=CARTESIAN_POINT('Origin',(0.0163016666201714,-0.0338731404305814,
0.0723126509480677));
#83799=CARTESIAN_POINT('Ctrl Pts',(0.0138697965960476,-0.0321934096636941,
0.0743978996299439));
#83800=CARTESIAN_POINT('Ctrl Pts',(0.0138742338813685,-0.0320508460845488,
0.074295048708508));
#83801=CARTESIAN_POINT('Ctrl Pts',(0.0138759044196463,-0.0319086045665392,
0.0741921561159053));
#83802=CARTESIAN_POINT('Ctrl Pts',(0.013874822852946,-0.0317669892871366,
0.0740894436941117));
#83803=CARTESIAN_POINT('Ctrl Pts',(0.013871588533368,-0.0321934096636941,
0.0743140711050352));
#83804=CARTESIAN_POINT('Ctrl Pts',(0.0138745253280139,-0.0320508460845488,
0.0742111881087748));
#83805=CARTESIAN_POINT('Ctrl Pts',(0.0138746956452045,-0.0319086045665392,
0.0741083037807555));
#83806=CARTESIAN_POINT('Ctrl Pts',(0.0138721173557796,-0.0317669892871366,
0.0740056396792251));
#83807=CARTESIAN_POINT('Ctrl Pts',(0.0138733804706884,-0.0321934096636941,
0.0742302425801266));
#83808=CARTESIAN_POINT('Ctrl Pts',(0.0138748167746594,-0.0320508460845488,
0.0741273275090414));
#83809=CARTESIAN_POINT('Ctrl Pts',(0.0138734868707628,-0.0319086045665392,
0.0740244514456057));
#83810=CARTESIAN_POINT('Ctrl Pts',(0.0138694118586132,-0.0317669892871366,
0.0739218356643386));
#83811=CARTESIAN_POINT('Ctrl Pts',(0.0138751724080088,-0.0321934096636941,
0.0741464140552179));
#83812=CARTESIAN_POINT('Ctrl Pts',(0.0138751082213048,-0.0320508460845489,
0.0740434669093081));
#83813=CARTESIAN_POINT('Ctrl Pts',(0.0138722780963211,-0.0319086045665392,
0.0739405991104559));
#83814=CARTESIAN_POINT('Ctrl Pts',(0.0138667063614468,-0.0317669892871366,
0.0738380316494521));
#83815=CARTESIAN_POINT('',(0.0138751403498937,-0.0321934096636941,0.074147913764094));
#83816=CARTESIAN_POINT('',(0.013870198605396,-0.0318665617511344,0.073911623394967));
#83817=CARTESIAN_POINT('Origin',(-0.00282357719959373,-0.0326371944423954,
0.0735390319721531));
#83818=CARTESIAN_POINT('Origin',(0.0248219653144219,-0.0316939261509308,
0.0734573150399617));
#83819=CARTESIAN_POINT('',(0.0138737862240784,-0.0320197221621802,0.0742726491351916));
#83820=CARTESIAN_POINT('Ctrl Pts',(0.0138738372100478,-0.0320197392094717,
0.0742724713282445));
#83821=CARTESIAN_POINT('Ctrl Pts',(0.0138744603366102,-0.0319792716576016,
0.0742432131987236));
#83822=CARTESIAN_POINT('Ctrl Pts',(0.0138748632476785,-0.0319386439829712,
0.0742138171245965));
#83823=CARTESIAN_POINT('Ctrl Pts',(0.0138750379095079,-0.0318979099381644,
0.0741842521296344));
#83824=CARTESIAN_POINT('Ctrl Pts',(0.013875212567885,-0.0318571766984951,
0.0741546877190454));
#83825=CARTESIAN_POINT('Ctrl Pts',(0.0138751598799729,-0.0318163871833605,
0.0741251046704643));
#83826=CARTESIAN_POINT('Ctrl Pts',(0.0138748835481446,-0.0317755399638303,
0.074095604731115));
#83827=CARTESIAN_POINT('',(0.0138724689321763,-0.0321934096636185,0.074272885214998));
#83828=CARTESIAN_POINT('Origin',(0.0161800533289082,-0.0324111828247256,
0.0743011809090815));
#83829=CARTESIAN_POINT('',(0.013873804641045,-0.0321934096636664,0.074210399489556));
#83830=CARTESIAN_POINT('Ctrl Pts',(0.0138736758573183,-0.0321934096636618,
0.0741493169564813));
#83831=CARTESIAN_POINT('Ctrl Pts',(0.0138736664376159,-0.0320835708272592,
0.0740700214416468));
#83832=CARTESIAN_POINT('Ctrl Pts',(0.0138720160068189,-0.0319739230346488,
0.0739907721163737));
#83833=CARTESIAN_POINT('Ctrl Pts',(0.0138687344582465,-0.0318646057455573,
0.0739116702126153));
#83834=CARTESIAN_POINT('Ctrl Pts',(0.0139554985474753,-0.0321934096636618,
0.0740709191750039));
#83835=CARTESIAN_POINT('Ctrl Pts',(0.0139544079612666,-0.0320835708272592,
0.0739904952615033));
#83836=CARTESIAN_POINT('Ctrl Pts',(0.0139516536389322,-0.0319739230346488,
0.0739101405667658));
#83837=CARTESIAN_POINT('Ctrl Pts',(0.0139472469946829,-0.0318646057455573,
0.0738299576285942));
#83838=CARTESIAN_POINT('Ctrl Pts',(0.0140373212376322,-0.0321934096636618,
0.0739925213935266));
#83839=CARTESIAN_POINT('Ctrl Pts',(0.0140351494849173,-0.0320835708272592,
0.0739109690813598));
#83840=CARTESIAN_POINT('Ctrl Pts',(0.0140312912710454,-0.0319739230346488,
0.073829509017158));
#83841=CARTESIAN_POINT('Ctrl Pts',(0.0140257595311193,-0.0318646057455573,
0.073748245044573));
#83842=CARTESIAN_POINT('Ctrl Pts',(0.0141191439277891,-0.0321934096636618,
0.0739141236120492));
#83843=CARTESIAN_POINT('Ctrl Pts',(0.014115891008568,-0.0320835708272592,
0.0738314429012163));
#83844=CARTESIAN_POINT('Ctrl Pts',(0.0141109289031586,-0.0319739230346488,
0.0737488774675501));
#83845=CARTESIAN_POINT('Ctrl Pts',(0.0141042720675557,-0.0318646057455573,
0.0736665324605519));
#83846=CARTESIAN_POINT('',(0.0141186264125959,-0.032176398030849,0.0739013179501406));
#83847=CARTESIAN_POINT('',(0.0141191439277825,-0.0321934096636184,0.0739141236120217));
#83848=CARTESIAN_POINT('Origin',(-0.00242890665718246,-0.0326386230140034,
0.073973723431972));
#83849=CARTESIAN_POINT('Ctrl Pts',(0.0141186264094195,-0.0321763980306323,
0.0739013179502667));
#83850=CARTESIAN_POINT('Ctrl Pts',(0.0140757443961277,-0.0321259596175455,
0.0739030968099963));
#83851=CARTESIAN_POINT('Ctrl Pts',(0.0140336053693588,-0.0320749164632659,
0.0739048448486798));
#83852=CARTESIAN_POINT('Ctrl Pts',(0.0139507793765562,-0.0319716057794,
0.0739082806906997));
#83853=CARTESIAN_POINT('Ctrl Pts',(0.0139101246824559,-0.0319193786690211,
0.0739099671553107));
#83854=CARTESIAN_POINT('Ctrl Pts',(0.013870198603538,-0.0318665617525411,
0.0739116233950369));
#83855=CARTESIAN_POINT('',(0.0139971421388481,-0.0321934096636663,0.0740310186880679));
#83856=CARTESIAN_POINT('Origin',(0.00812378219310841,-0.0315241814719618,
0.07415));
#83857=CARTESIAN_POINT('',(0.0141186264129662,-0.0322104233323764,0.0739013179501252));
#83858=CARTESIAN_POINT('',(0.0141180815491566,-0.0321934096636183,0.0738885134227272));
#83859=CARTESIAN_POINT('Origin',(-0.00243335535698296,-0.0326387242963926,
0.0740188372389752));
#83860=CARTESIAN_POINT('Origin',(-0.00237805205674754,-0.0326386237958717,
0.0751996751081487));
#83861=CARTESIAN_POINT('Origin',(-0.00238621941514002,-0.0326387247895164,
0.0751550842654159));
#83862=CARTESIAN_POINT('Ctrl Pts',(0.0138746213929418,-0.0327445246967096,
0.0740727115942768));
#83863=CARTESIAN_POINT('Ctrl Pts',(0.0138717064130665,-0.0324436878339359,
0.0738558151480787));
#83864=CARTESIAN_POINT('Ctrl Pts',(0.0138524621875469,-0.0321434074405926,
0.0736397544499746));
#83865=CARTESIAN_POINT('Ctrl Pts',(0.0138658296065809,-0.0327445246967096,
0.073822866233118));
#83866=CARTESIAN_POINT('Ctrl Pts',(0.0138534915548631,-0.0324436878339359,
0.0736063013745631));
#83867=CARTESIAN_POINT('Ctrl Pts',(0.0138248760039893,-0.0321434074405926,
0.0733912811063806));
#83868=CARTESIAN_POINT('',(0.0138636603625111,-0.0326943950436612,0.0737867871141936));
#83869=CARTESIAN_POINT('',(0.0138438915753067,-0.0323666188837389,0.0735512733046812));
#83870=CARTESIAN_POINT('Origin',(-0.00290876188441187,-0.0326395579112152,
0.0749242888442998));
#83871=CARTESIAN_POINT('Origin',(0.0248284905272715,-0.0321933825603021,
0.0724015091066871));
#83872=CARTESIAN_POINT('',(0.0138555531450554,-0.0321934096532689,0.0736757355682102));
#83873=CARTESIAN_POINT('',(0.0138490467834857,-0.0321934096584274,0.0736135751498974));
#83874=CARTESIAN_POINT('',(0.013870198606331,-0.0325210109756238,0.0739116233949256));
#83875=CARTESIAN_POINT('Origin',(-0.00291375938666434,-0.0326393129156296,
0.0744434983967485));
#83876=CARTESIAN_POINT('',(0.0138688412385515,-0.0326943950436593,0.0739116797021394));
#83877=CARTESIAN_POINT('Origin',(0.0249217906147906,-0.0326943765538174,
0.0734531747542535));
#83878=CARTESIAN_POINT('',(0.0138662508005413,-0.0326943950436702,0.0738492334081765));
#83879=CARTESIAN_POINT('Ctrl Pts',(0.0141237669771519,-0.0325229783203769,
0.0741364873635179));
#83880=CARTESIAN_POINT('Ctrl Pts',(0.0141235807057535,-0.032413025309245,
0.0740537777044809));
#83881=CARTESIAN_POINT('Ctrl Pts',(0.0141216835070616,-0.032303122220807,
0.0739710844432473));
#83882=CARTESIAN_POINT('Ctrl Pts',(0.0141180815489685,-0.0321934096576658,
0.0738885134182532));
#83883=CARTESIAN_POINT('Ctrl Pts',(0.0140387566190187,-0.0325229783203769,
0.0740615581886461));
#83884=CARTESIAN_POINT('Ctrl Pts',(0.0140375374505832,-0.032413025309245,
0.0739800203955368));
#83885=CARTESIAN_POINT('Ctrl Pts',(0.0140346317530654,-0.032303122220807,
0.0738985201892968));
#83886=CARTESIAN_POINT('Ctrl Pts',(0.0140300469322471,-0.0321934096576658,
0.0738171618345591));
#83887=CARTESIAN_POINT('Ctrl Pts',(0.0139537462608854,-0.0325229783203769,
0.0739866290137742));
#83888=CARTESIAN_POINT('Ctrl Pts',(0.0139514941954129,-0.032413025309245,
0.0739062630865928));
#83889=CARTESIAN_POINT('Ctrl Pts',(0.0139475799990693,-0.032303122220807,
0.0738259559353461));
#83890=CARTESIAN_POINT('Ctrl Pts',(0.0139420123155258,-0.0321934096576658,
0.073745810250865));
#83891=CARTESIAN_POINT('Ctrl Pts',(0.0138687359027521,-0.0325229783203769,
0.0739116998389024));
#83892=CARTESIAN_POINT('Ctrl Pts',(0.0138654509402426,-0.032413025309245,
0.0738325057776488));
#83893=CARTESIAN_POINT('Ctrl Pts',(0.0138605282450731,-0.032303122220807,
0.0737533916813956));
#83894=CARTESIAN_POINT('Ctrl Pts',(0.0138539776988044,-0.0321934096576658,
0.073674458667171));
#83895=CARTESIAN_POINT('',(0.0139868173472928,-0.0321934096584275,0.073782124495952));
#83896=CARTESIAN_POINT('Ctrl Pts',(0.0141186264094853,-0.0322104233328894,
0.073901317950264));
#83897=CARTESIAN_POINT('Ctrl Pts',(0.0140756862904063,-0.0322609421830354,
0.0739030992203759));
#83898=CARTESIAN_POINT('Ctrl Pts',(0.0140335188780103,-0.0323120888238673,
0.0739048484365637));
#83899=CARTESIAN_POINT('Ctrl Pts',(0.0139506922580386,-0.032415652463181,
0.0739082843046003));
#83900=CARTESIAN_POINT('Ctrl Pts',(0.0139100670967876,-0.0324680267167313,
0.0739099695441171));
#83901=CARTESIAN_POINT('Ctrl Pts',(0.0138701986062875,-0.0325210109755912,
0.0739116233949229));
#83902=CARTESIAN_POINT('Origin',(0.00750075467550516,-0.026283458251078,
0.0819931640652065));
#83903=CARTESIAN_POINT('Origin',(0.0192136187594495,-0.0342770745984023,
0.0791338237432995));
#83904=CARTESIAN_POINT('Ctrl Pts',(0.0138622872002598,-0.0326943950436604,
0.0737882791317084));
#83905=CARTESIAN_POINT('Ctrl Pts',(0.0138573020087576,-0.0325844576448133,
0.0737091917776052));
#83906=CARTESIAN_POINT('Ctrl Pts',(0.0138506808082973,-0.0324744968375322,
0.0736302019283006));
#83907=CARTESIAN_POINT('Ctrl Pts',(0.0138424334782875,-0.0323646534831894,
0.0735514106731837));
#83908=CARTESIAN_POINT('Ctrl Pts',(0.0139390256834958,-0.0326943950436604,
0.0737048984818396));
#83909=CARTESIAN_POINT('Ctrl Pts',(0.0139328913503664,-0.0325844576448133,
0.0736247535276142));
#83910=CARTESIAN_POINT('Ctrl Pts',(0.0139250990540479,-0.0324744968375322,
0.0735447297694723));
#83911=CARTESIAN_POINT('Ctrl Pts',(0.0139156601926969,-0.0323646534831894,
0.0734649296008111));
#83912=CARTESIAN_POINT('Ctrl Pts',(0.0140157641667319,-0.0326943950436604,
0.0736215178319709));
#83913=CARTESIAN_POINT('Ctrl Pts',(0.0140084806919753,-0.0325844576448133,
0.0735403152776232));
#83914=CARTESIAN_POINT('Ctrl Pts',(0.0139995172997985,-0.0324744968375322,
0.073459257610644));
#83915=CARTESIAN_POINT('Ctrl Pts',(0.0139888869071063,-0.0323646534831894,
0.0733784485284386));
#83916=CARTESIAN_POINT('Ctrl Pts',(0.0140925026499679,-0.0326943950436604,
0.0735381371821021));
#83917=CARTESIAN_POINT('Ctrl Pts',(0.0140840700335841,-0.0325844576448133,
0.0734558770276322));
#83918=CARTESIAN_POINT('Ctrl Pts',(0.0140739355455492,-0.0324744968375322,
0.0733737854518156));
#83919=CARTESIAN_POINT('Ctrl Pts',(0.0140621136215156,-0.0323646534831894,
0.073291967456066));
#83920=CARTESIAN_POINT('',(0.0140911820820146,-0.0326773559991189,0.0735253892843));
#83921=CARTESIAN_POINT('',(0.0140925026499634,-0.0326943950436594,0.0735381371821062));
#83922=CARTESIAN_POINT('Origin',(-0.00241850945560545,-0.0326395669502595,
0.0753039822634916));
#83923=CARTESIAN_POINT('Ctrl Pts',(0.0140911820786748,-0.032677355998746,
0.0735253892846437));
#83924=CARTESIAN_POINT('Ctrl Pts',(0.0140484620282019,-0.0326267922586494,
0.0735298608135839));
#83925=CARTESIAN_POINT('Ctrl Pts',(0.0140064991597738,-0.0325756109580394,
0.0735342530879027));
#83926=CARTESIAN_POINT('Ctrl Pts',(0.0139240520743678,-0.0324719985462376,
0.0735428828653572));
#83927=CARTESIAN_POINT('Ctrl Pts',(0.013883600924787,-0.0324196091621774,
0.073547116907312));
#83928=CARTESIAN_POINT('Ctrl Pts',(0.0138438915752582,-0.0323666188837756,
0.0735512733046863));
#83929=CARTESIAN_POINT('',(0.0139780815062472,-0.0326943950436703,0.0736624621481599));
#83930=CARTESIAN_POINT('Origin',(0.00812378219310841,-0.0315241814719618,
0.07415));
#83931=CARTESIAN_POINT('',(0.0140911820819701,-0.0327114338379853,0.0735253892843048));
#83932=CARTESIAN_POINT('',(0.0140898342906075,-0.0326943950436593,0.0735126442359757));
#83933=CARTESIAN_POINT('Origin',(-0.00241302076069148,-0.0326395678925681,
0.0753489579910992));
#83934=CARTESIAN_POINT('Origin',(-0.0024289706066625,-0.0326395674317057,
0.0752040471793359));
#83935=CARTESIAN_POINT('Origin',(-0.00243291222228821,-0.0326395682946239,
0.075158909412172));
#83936=CARTESIAN_POINT('Ctrl Pts',(0.013858417457439,-0.0332451089994433,
0.0737117268145363));
#83937=CARTESIAN_POINT('Ctrl Pts',(0.0138418877138084,-0.0329451141710254,
0.073495441506929));
#83938=CARTESIAN_POINT('Ctrl Pts',(0.0138091134358847,-0.0326442513127493,
0.0732810157309182));
#83939=CARTESIAN_POINT('Ctrl Pts',(0.0138339534028375,-0.0332451089994433,
0.073462926673796));
#83940=CARTESIAN_POINT('Ctrl Pts',(0.0138080400083743,-0.0329451141710254,
0.0732475640431037));
#83941=CARTESIAN_POINT('Ctrl Pts',(0.0137659782373769,-0.0326442513127493,
0.0730347651377216));
#83942=CARTESIAN_POINT('Ctrl Pts',(0.0138337087622915,-0.0332451089994433,
0.0734604386723885));
#83943=CARTESIAN_POINT('Ctrl Pts',(0.01380770153132,-0.0329451141710254,
0.0732450852684655));
#83944=CARTESIAN_POINT('Ctrl Pts',(0.0137655468853918,-0.0326442513127493,
0.0730323026317896));
#83945=CARTESIAN_POINT('',(0.0138295276982946,-0.0331951640388616,0.0734270938995632));
#83946=CARTESIAN_POINT('',(0.0137950098894886,-0.0328677532355034,0.0731932861004177));
#83947=CARTESIAN_POINT('Origin',(-0.00268754535352905,-0.0326402808277667,
0.0762938944285065));
#83948=CARTESIAN_POINT('Origin',(0.0246968758612786,-0.0326944278779091,
0.0713538021235014));
#83949=CARTESIAN_POINT('',(0.0138144634936381,-0.0326943950436593,0.0733167705383256));
#83950=CARTESIAN_POINT('',(0.0138040668860577,-0.0326943950436693,0.0732551413200166));
#83951=CARTESIAN_POINT('',(0.013843891575307,-0.0330220786163545,0.073551273304684));
#83952=CARTESIAN_POINT('Origin',(-0.00279833087479486,-0.032639668275823,
0.0758260491408386));
#83953=CARTESIAN_POINT('',(0.0138425404215422,-0.0331951640388587,0.0735514147306181));
#83954=CARTESIAN_POINT('Origin',(0.0248142547232573,-0.0331952026560103,
0.0724030006817456));
#83955=CARTESIAN_POINT('',(0.0138360340599284,-0.0331951640388701,0.0734892543151006));
#83956=CARTESIAN_POINT('Ctrl Pts',(0.014111078849787,-0.0330240426238172,
0.073759770907006));
#83957=CARTESIAN_POINT('Ctrl Pts',(0.0141057030638493,-0.0329142774063519,
0.0736772900624198));
#83958=CARTESIAN_POINT('Ctrl Pts',(0.0140986194884296,-0.0328043479726691,
0.0735948792306362));
#83959=CARTESIAN_POINT('Ctrl Pts',(0.0140898342906153,-0.0326943950436593,
0.0735126442359812));
#83960=CARTESIAN_POINT('Ctrl Pts',(0.0140215314090359,-0.0330240426238172,
0.0736903274635429));
#83961=CARTESIAN_POINT('Ctrl Pts',(0.014015198972009,-0.0329142774063519,
0.0736090802221948));
#83962=CARTESIAN_POINT('Ctrl Pts',(0.0140071837705996,-0.0328043479726691,
0.073527923385296));
#83963=CARTESIAN_POINT('Ctrl Pts',(0.0139974932096187,-0.0326943950436593,
0.0734469612035796));
#83964=CARTESIAN_POINT('Ctrl Pts',(0.0139319839682848,-0.0330240426238172,
0.0736208840200798));
#83965=CARTESIAN_POINT('Ctrl Pts',(0.0139246948801687,-0.0329142774063519,
0.0735408703819699));
#83966=CARTESIAN_POINT('Ctrl Pts',(0.0139157480527695,-0.0328043479726691,
0.0734609675399557));
#83967=CARTESIAN_POINT('Ctrl Pts',(0.0139051521286221,-0.0326943950436593,
0.0733812781711779));
#83968=CARTESIAN_POINT('Ctrl Pts',(0.0138424365275337,-0.0330240426238172,
0.0735514405766166));
#83969=CARTESIAN_POINT('Ctrl Pts',(0.0138341907883284,-0.0329142774063519,
0.0734726605417449));
#83970=CARTESIAN_POINT('Ctrl Pts',(0.0138243123349394,-0.0328043479726691,
0.0733940116946154));
#83971=CARTESIAN_POINT('Ctrl Pts',(0.0138128110476255,-0.0326943950436593,
0.0733155951387763));
#83972=CARTESIAN_POINT('',(0.0139521488921328,-0.0326943950436693,0.0734147073871606));
#83973=CARTESIAN_POINT('Ctrl Pts',(0.0140911820786676,-0.0327114338383291,
0.0735253892846446));
#83974=CARTESIAN_POINT('Ctrl Pts',(0.0140484691339741,-0.0327619876830032,
0.0735298600698193));
#83975=CARTESIAN_POINT('Ctrl Pts',(0.014006509736354,-0.0328131562602444,
0.0735342519808468));
#83976=CARTESIAN_POINT('Ctrl Pts',(0.0139240627265978,-0.0329167375858767,
0.073542881750383));
#83977=CARTESIAN_POINT('Ctrl Pts',(0.0138836079658183,-0.0329691088920624,
0.0735471161703238));
#83978=CARTESIAN_POINT('Ctrl Pts',(0.0138438915752594,-0.0330220786163187,
0.0735512733046862));
#83979=CARTESIAN_POINT('Ctrl Pts',(0.0138282507263866,-0.0331951640388604,
0.0734286694459876));
#83980=CARTESIAN_POINT('Ctrl Pts',(0.0138133376796565,-0.0330306422010619,
0.0733107332164269));
#83981=CARTESIAN_POINT('Ctrl Pts',(0.013793562947628,-0.0328657861914645,
0.0731935141344525));
#83982=CARTESIAN_POINT('Ctrl Pts',(0.0138295276982949,-0.0331951640388604,
0.0734270938995663));
#83983=CARTESIAN_POINT('Ctrl Pts',(0.0138145820781527,-0.0330306422010619,
0.0733091312694302));
#83984=CARTESIAN_POINT('Ctrl Pts',(0.0137947737093823,-0.0328657861914645,
0.0731918871557328));
#83985=CARTESIAN_POINT('Ctrl Pts',(0.0140423055593539,-0.0331951640388604,
0.0731645654951962));
#83986=CARTESIAN_POINT('Ctrl Pts',(0.0140219323327688,-0.0330306422010619,
0.0730422038192032));
#83987=CARTESIAN_POINT('Ctrl Pts',(0.0139965191782159,-0.0328657861914645,
0.0729207887472848));
#83988=CARTESIAN_POINT('',(0.0140401871515089,-0.0331781648281943,0.0731519256720257));
#83989=CARTESIAN_POINT('',(0.0140423055593501,-0.0331951640388588,0.0731645654951994));
#83990=CARTESIAN_POINT('Origin',(-0.00211829006564492,-0.0326412093227545,
0.0766001274957886));
#83991=CARTESIAN_POINT('Ctrl Pts',(0.0140401871507031,-0.033178164828644,
0.07315192567368));
#83992=CARTESIAN_POINT('Ctrl Pts',(0.0139978030104248,-0.033127681154676,
0.0731590757243037));
#83993=CARTESIAN_POINT('Ctrl Pts',(0.0139561842020887,-0.0330765663497757,
0.0731660967005014));
#83994=CARTESIAN_POINT('Ctrl Pts',(0.0138744414644628,-0.0329730614463108,
0.0731798863764052));
#83995=CARTESIAN_POINT('Ctrl Pts',(0.0138343505565534,-0.0329207133373549,
0.0731866495000993));
#83996=CARTESIAN_POINT('Ctrl Pts',(0.013795009900406,-0.0328677532289388,
0.0731932861127498));
#83997=CARTESIAN_POINT('',(0.0139359166288323,-0.0331951640388701,0.0732958296973913));
#83998=CARTESIAN_POINT('Origin',(0.00812378219310841,-0.0315241814719618,
0.07415));
#83999=CARTESIAN_POINT('',(0.014040187149871,-0.0332121607144211,0.0731519256716465));
#84000=CARTESIAN_POINT('',(0.01403804175006,-0.0331951640388587,0.073139290401245));
#84001=CARTESIAN_POINT('Origin',(-0.00210312635413019,-0.0326413663376525,
0.0766428616037648));
#84002=CARTESIAN_POINT('Origin',(-0.00235525584752046,-0.032641209647175,
0.0751954430371073));
#84003=CARTESIAN_POINT('Origin',(-0.00235494846232508,-0.0326413667796312,
0.0751500991739546));
#84004=CARTESIAN_POINT('Ctrl Pts',(0.0138195849521744,-0.0337436976235975,
0.0733525315493287));
#84005=CARTESIAN_POINT('Ctrl Pts',(0.0138124124000694,-0.0336723290703325,
0.0733013026360912));
#84006=CARTESIAN_POINT('Ctrl Pts',(0.0138043195616353,-0.033601104548885,
0.0732502110220896));
#84007=CARTESIAN_POINT('Ctrl Pts',(0.0137784807316163,-0.0333736987606857,
0.0730870856192612));
#84008=CARTESIAN_POINT('Ctrl Pts',(0.0137433234057579,-0.0331450831799191,
0.0729257118152436));
#84009=CARTESIAN_POINT('Ctrl Pts',(0.0137795477755188,-0.0337436976235975,
0.073105758324514));
#84010=CARTESIAN_POINT('Ctrl Pts',(0.0137701557076303,-0.0336723290703325,
0.0730548895117111));
#84011=CARTESIAN_POINT('Ctrl Pts',(0.0137598501895499,-0.033601104548885,
0.0730041978619816));
#84012=CARTESIAN_POINT('Ctrl Pts',(0.0137269467117273,-0.0333736987606857,
0.0728423494658455));
#84013=CARTESIAN_POINT('Ctrl Pts',(0.0136848096620531,-0.0331450831799191,
0.0726826559743393));
#84014=CARTESIAN_POINT('Ctrl Pts',(0.0137791474037523,-0.0337436976235975,
0.0731032905922659));
#84015=CARTESIAN_POINT('Ctrl Pts',(0.0137697331407059,-0.0336723290703325,
0.0730524253804672));
#84016=CARTESIAN_POINT('Ctrl Pts',(0.0137594054958291,-0.033601104548885,
0.0730017377303805));
#84017=CARTESIAN_POINT('Ctrl Pts',(0.0137264313715284,-0.0333736987606857,
0.0728399021043113));
#84018=CARTESIAN_POINT('Ctrl Pts',(0.0136842245246161,-0.0331450831799191,
0.0726802254159302));
#84019=CARTESIAN_POINT('',(0.0137728770632737,-0.0336938721132548,0.0730702536650338));
#84020=CARTESIAN_POINT('',(0.0137237464482251,-0.0333679870047996,0.0728390746239767));
#84021=CARTESIAN_POINT('Ctrl Pts',(0.0137728770632776,-0.0336938721132591,
0.0730702536650529));
#84022=CARTESIAN_POINT('Ctrl Pts',(0.0137686623068125,-0.0336629187933937,
0.0730482025977288));
#84023=CARTESIAN_POINT('Ctrl Pts',(0.0137643197804625,-0.0336319952301075,
0.073026183261959));
#84024=CARTESIAN_POINT('Ctrl Pts',(0.0137598501895513,-0.0336011045488985,
0.0730041978619883));
#84025=CARTESIAN_POINT('Ctrl Pts',(0.0137486344565473,-0.0335235892595488,
0.0729490289704813));
#84026=CARTESIAN_POINT('Ctrl Pts',(0.013736598548414,-0.0334458668665605,
0.0728939757672621));
#84027=CARTESIAN_POINT('Ctrl Pts',(0.0137237464511504,-0.0333679869962528,
0.072839074635416));
#84028=CARTESIAN_POINT('Ctrl Pts',(0.0137237369832191,-0.0333679692468935,
0.072839031174882));
#84029=CARTESIAN_POINT('Ctrl Pts',(0.0137232970506411,-0.0333391895415326,
0.0728391402487389));
#84030=CARTESIAN_POINT('Ctrl Pts',(0.013722968081111,-0.0333104081131989,
0.0728392251566906));
#84031=CARTESIAN_POINT('Ctrl Pts',(0.0137225340181308,-0.0332532698752625,
0.072839342909496));
#84032=CARTESIAN_POINT('Ctrl Pts',(0.0137224256564151,-0.0332249173718078,
0.0728393765136672));
#84033=CARTESIAN_POINT('Ctrl Pts',(0.0137224236555687,-0.0331960985265627,
0.0728393840696058));
#84034=CARTESIAN_POINT('Ctrl Pts',(0.0137224236520676,-0.0331956312660268,
0.0728393841851924));
#84035=CARTESIAN_POINT('Ctrl Pts',(0.0137224236774247,-0.0331951640388597,
0.0728393842935123));
#84036=CARTESIAN_POINT('',(0.0137509153232184,-0.0331951640388587,0.072961093890999));
#84037=CARTESIAN_POINT('',(0.0137366695003317,-0.0331951640388687,0.0729002390922664));
#84038=CARTESIAN_POINT('',(0.0137950098854651,-0.0335216366567671,0.0731932861154109));
#84039=CARTESIAN_POINT('Origin',(-0.00238249280895044,-0.0326434571527336,
0.0771504405968173));
#84040=CARTESIAN_POINT('',(0.0137936702784574,-0.0336938721132327,0.0731935121016875));
#84041=CARTESIAN_POINT('Origin',(0.0245620886186969,-0.0336938867896244,
0.0713769228819775));
#84042=CARTESIAN_POINT('',(0.0137832736708755,-0.0336938721132538,0.0731318828833706));
#84043=CARTESIAN_POINT('Ctrl Pts',(0.0140747614774173,-0.0335235895815172,
0.0733845945141182));
#84044=CARTESIAN_POINT('Ctrl Pts',(0.0140642241639594,-0.0334144449262748,
0.0733026675678697));
#84045=CARTESIAN_POINT('Ctrl Pts',(0.0140519821953524,-0.0333049234473147,
0.0732208641904514));
#84046=CARTESIAN_POINT('Ctrl Pts',(0.0140380417500679,-0.0331951640388587,
0.0731392904012499));
#84047=CARTESIAN_POINT('Ctrl Pts',(0.0139810302047748,-0.0335235895815172,
0.0733209107562573));
#84048=CARTESIAN_POINT('Ctrl Pts',(0.0139696161590081,-0.0334144449262748,
0.0732402742055166));
#84049=CARTESIAN_POINT('Ctrl Pts',(0.0139565231094332,-0.0333049234473147,
0.073159780818744));
#84050=CARTESIAN_POINT('Ctrl Pts',(0.0139417584745285,-0.0331951640388587,
0.0730795350388303));
#84051=CARTESIAN_POINT('Ctrl Pts',(0.0138872989321322,-0.0335235895815172,
0.0732572269983964));
#84052=CARTESIAN_POINT('Ctrl Pts',(0.0138750081540568,-0.0334144449262748,
0.0731778808431635));
#84053=CARTESIAN_POINT('Ctrl Pts',(0.013861064023514,-0.0333049234473147,
0.0730986974470365));
#84054=CARTESIAN_POINT('Ctrl Pts',(0.0138454751989892,-0.0331951640388587,
0.0730197796764107));
#84055=CARTESIAN_POINT('Ctrl Pts',(0.0137935676594896,-0.0335235895815172,
0.0731935432405355));
#84056=CARTESIAN_POINT('Ctrl Pts',(0.0137804001491055,-0.0334144449262748,
0.0731154874808105));
#84057=CARTESIAN_POINT('Ctrl Pts',(0.0137656049375948,-0.0333049234473147,
0.0730376140753291));
#84058=CARTESIAN_POINT('Ctrl Pts',(0.0137491919234499,-0.0331951640388587,
0.0729600243139911));
#84059=CARTESIAN_POINT('',(0.0138944785366492,-0.0331951640388687,0.073050192146132));
#84060=CARTESIAN_POINT('Ctrl Pts',(0.014040187146777,-0.0332121607145949,
0.0731519256721623));
#84061=CARTESIAN_POINT('Ctrl Pts',(0.0139978743055216,-0.0332625444108814,
0.0731590636826476));
#84062=CARTESIAN_POINT('Ctrl Pts',(0.0139562905809177,-0.0333135300744919,
0.0731660786940115));
#84063=CARTESIAN_POINT('Ctrl Pts',(0.0138745483561059,-0.033416720314056,
0.0731798682869693));
#84064=CARTESIAN_POINT('Ctrl Pts',(0.0138344215155566,-0.033468884758724,
0.073186637527703));
#84065=CARTESIAN_POINT('Ctrl Pts',(0.0137950098847373,-0.0335216366562299,
0.0731932861153583));
#84066=CARTESIAN_POINT('Ctrl Pts',(0.0137717018154838,-0.0336938721132589,
0.0730719058977375));
#84067=CARTESIAN_POINT('Ctrl Pts',(0.0137653913729524,-0.0336474569765057,
0.0730388467500022));
#84068=CARTESIAN_POINT('Ctrl Pts',(0.0137586943637518,-0.033601104548885,
0.0730058637391982));
#84069=CARTESIAN_POINT('Ctrl Pts',(0.0137417390761985,-0.0334837508592655,
0.0729223583391302));
#84070=CARTESIAN_POINT('Ctrl Pts',(0.0137223167960186,-0.0333660264659096,
0.0728393920288039));
#84071=CARTESIAN_POINT('Ctrl Pts',(0.0137728770632802,-0.0336938721132589,
0.0730702536650682));
#84072=CARTESIAN_POINT('Ctrl Pts',(0.0137665569496827,-0.0336474569765057,
0.0730371876382175));
#84073=CARTESIAN_POINT('Ctrl Pts',(0.0137598501895499,-0.033601104548885,
0.0730041978619816));
#84074=CARTESIAN_POINT('Ctrl Pts',(0.0137428702148784,-0.0334837508592655,
0.0729206753333953));
#84075=CARTESIAN_POINT('Ctrl Pts',(0.0137234227508674,-0.0333660264659096,
0.0728376926336029));
#84076=CARTESIAN_POINT('Ctrl Pts',(0.0139699260031527,-0.0336938721132589,
0.0727932306432676));
#84077=CARTESIAN_POINT('Ctrl Pts',(0.0139619843818822,-0.0336474569765057,
0.0727590112235839));
#84078=CARTESIAN_POINT('Ctrl Pts',(0.013953642723264,-0.033601104548885,
0.0727248871153407));
#84079=CARTESIAN_POINT('Ctrl Pts',(0.0139325235615145,-0.0334837508592655,
0.072638492718912));
#84080=CARTESIAN_POINT('Ctrl Pts',(0.0139088536286531,-0.0333660264659096,
0.0725527620650849));
#84081=CARTESIAN_POINT('',(0.0139658428723954,-0.0336769361243753,0.0727824010019275));
#84082=CARTESIAN_POINT('',(0.0139687507609263,-0.0336938721132327,0.0727948828680808));
#84083=CARTESIAN_POINT('Ctrl Pts',(0.0139658428723954,-0.0336769361243754,
0.0727824010019274));
#84084=CARTESIAN_POINT('Ctrl Pts',(0.0139663297787378,-0.0336797586670034,
0.0727844809510949));
#84085=CARTESIAN_POINT('Ctrl Pts',(0.0139668155558788,-0.0336825812712859,
0.0727865610816272));
#84086=CARTESIAN_POINT('Ctrl Pts',(0.0139677848513756,-0.0336882265979406,
0.072790721701514));
#84087=CARTESIAN_POINT('Ctrl Pts',(0.0139682683697385,-0.0336910493203049,
0.0727928021908584));
#84088=CARTESIAN_POINT('Ctrl Pts',(0.0139687507609291,-0.0336938721132341,
0.0727948828680782));
#84089=CARTESIAN_POINT('Ctrl Pts',(0.0139658428723954,-0.0336769361243753,
0.0727824010019274));
#84090=CARTESIAN_POINT('Ctrl Pts',(0.0139250333282574,-0.0336279018398638,
0.0727919543247597));
#84091=CARTESIAN_POINT('Ctrl Pts',(0.0138836366876243,-0.0335767825795099,
0.0728016450841278));
#84092=CARTESIAN_POINT('Ctrl Pts',(0.0138025230730602,-0.0334733171841404,
0.0728206334007677));
#84093=CARTESIAN_POINT('Ctrl Pts',(0.0137627515838202,-0.0334209631343284,
0.0728299437198176));
#84094=CARTESIAN_POINT('Ctrl Pts',(0.0137237464515687,-0.033367986984468,
0.0728390746382923));
#84095=CARTESIAN_POINT('',(0.01387081391211,-0.0336938721132538,0.0729325682665674));
#84096=CARTESIAN_POINT('Origin',(0.00812378219310841,-0.0315241814719618,
0.07415));
#84097=CARTESIAN_POINT('',(0.0139658428711401,-0.0337108120655386,0.0727824010022275));
#84098=CARTESIAN_POINT('',(0.0139629083290094,-0.0336938721132327,0.0727699253755514));
#84099=CARTESIAN_POINT('Origin',(-0.00221942796324656,-0.0345562523571996,
0.0754234764236254));
#84100=CARTESIAN_POINT('Ctrl Pts',(0.013962908329023,-0.0336938721132379,
0.0727699253755552));
#84101=CARTESIAN_POINT('Ctrl Pts',(0.0139633996084448,-0.0336910492977519,
0.0727720039896108));
#84102=CARTESIAN_POINT('Ctrl Pts',(0.0139638897885156,-0.0336882265866634,
0.0727740829107104));
#84103=CARTESIAN_POINT('Ctrl Pts',(0.0139648679673416,-0.0336825812712735,
0.0727782414422964));
#84104=CARTESIAN_POINT('Ctrl Pts',(0.0139653559660541,-0.0336797586669969,
0.0727803210527646));
#84105=CARTESIAN_POINT('Ctrl Pts',(0.0139658428723954,-0.0336769361243749,
0.0727824010019277));
#84106=CARTESIAN_POINT('Origin',(-0.00170994795491135,-0.0345562520832892,
0.0775998502734302));
#84107=CARTESIAN_POINT('Ctrl Pts',(0.0137582824848021,-0.0342436276873911,
0.0729965133451561));
#84108=CARTESIAN_POINT('Ctrl Pts',(0.0137147780184345,-0.033943005420181,
0.0727840046634048));
#84109=CARTESIAN_POINT('Ctrl Pts',(0.0136553901190583,-0.0336441434784052,
0.0725753766312008));
#84110=CARTESIAN_POINT('Ctrl Pts',(0.0137028314820487,-0.0342436276873911,
0.0727527405281857));
#84111=CARTESIAN_POINT('Ctrl Pts',(0.0136501329723233,-0.033943005420181,
0.07254232321548));
#84112=CARTESIAN_POINT('Ctrl Pts',(0.0135817346793883,-0.0336441434784052,
0.0723364731439784));
#84113=CARTESIAN_POINT('Ctrl Pts',(0.0137022769720212,-0.0342436276873911,
0.0727503028000161));
#84114=CARTESIAN_POINT('Ctrl Pts',(0.0136494865218622,-0.033943005420181,
0.0725399064010008));
#84115=CARTESIAN_POINT('Ctrl Pts',(0.0135809981249916,-0.0336441434784052,
0.0723340841091063));
#84116=CARTESIAN_POINT('',(0.013693932031632,-0.0341934961088741,0.0727176746960286));
#84117=CARTESIAN_POINT('',(0.013630382516674,-0.0338664212865844,0.0724900367830602));
#84118=CARTESIAN_POINT('Origin',(-0.00263298766439013,-0.0345610720407349,
0.0763898453086364));
#84119=CARTESIAN_POINT('Origin',(0.024129938861581,-0.0336938005073086,
0.0693249078803981));
#84120=CARTESIAN_POINT('',(0.0136651594291266,-0.0336938721132327,0.0726101093129251));
#84121=CARTESIAN_POINT('',(0.0136471206126884,-0.0336938721132427,0.0725502690998577));
#84122=CARTESIAN_POINT('',(0.0137237464515699,-0.0340203938281605,0.0728390746382975));
#84123=CARTESIAN_POINT('Origin',(-0.0026649402405618,-0.0345589643241833,
0.0759097247337609));
#84124=CARTESIAN_POINT('',(0.0137224236774251,-0.034193496108874,0.0728393842935138));
#84125=CARTESIAN_POINT('Origin',(0.0244518037981792,-0.0341934220717627,
0.0703276875602538));
#84126=CARTESIAN_POINT('',(0.0137081778545386,-0.0341934961088841,0.0727785294947812));
#84127=CARTESIAN_POINT('Ctrl Pts',(0.0140149588898305,-0.0340223579322397,
0.0730124424726243));
#84128=CARTESIAN_POINT('Ctrl Pts',(0.0139992690046534,-0.0339125849573575,
0.0729311877811427));
#84129=CARTESIAN_POINT('Ctrl Pts',(0.0139819083612731,-0.0338030433565231,
0.0728503149305569));
#84130=CARTESIAN_POINT('Ctrl Pts',(0.0139629083290173,-0.0336938721132327,
0.0727699253755556));
#84131=CARTESIAN_POINT('Ctrl Pts',(0.0139174138366079,-0.0340223579322397,
0.0729547697544411));
#84132=CARTESIAN_POINT('Ctrl Pts',(0.0139009284942303,-0.0339125849573575,
0.0728748604636516));
#84133=CARTESIAN_POINT('Ctrl Pts',(0.0138828007992761,-0.0338030433565231,
0.0727953485324761));
#84134=CARTESIAN_POINT('Ctrl Pts',(0.0138630629477248,-0.0336938721132327,
0.0727163335882615));
#84135=CARTESIAN_POINT('Ctrl Pts',(0.0138198687833854,-0.0340223579322397,
0.0728970970362579));
#84136=CARTESIAN_POINT('Ctrl Pts',(0.0138025879838073,-0.0339125849573575,
0.0728185331461605));
#84137=CARTESIAN_POINT('Ctrl Pts',(0.0137836932372792,-0.0338030433565231,
0.0727403821343953));
#84138=CARTESIAN_POINT('Ctrl Pts',(0.0137632175664323,-0.0336938721132327,
0.0726627418009673));
#84139=CARTESIAN_POINT('Ctrl Pts',(0.0137223237301629,-0.0340223579322397,
0.0728394243180747));
#84140=CARTESIAN_POINT('Ctrl Pts',(0.0137042474733842,-0.0339125849573575,
0.0727622058286694));
#84141=CARTESIAN_POINT('Ctrl Pts',(0.0136845856752823,-0.0338030433565231,
0.0726854157363145));
#84142=CARTESIAN_POINT('Ctrl Pts',(0.0136633721851398,-0.0336938721132327,
0.0726091500136732));
#84143=CARTESIAN_POINT('',(0.013814033879078,-0.0336938721132427,0.0726900173442483));
#84144=CARTESIAN_POINT('Ctrl Pts',(0.0139658428676264,-0.0337108120662662,
0.0727824010030439));
#84145=CARTESIAN_POINT('Ctrl Pts',(0.013923975490418,-0.0337611408993437,
0.0727922019596353));
#84146=CARTESIAN_POINT('Ctrl Pts',(0.0138828720999542,-0.033812108877957,
0.072801824070514));
#84147=CARTESIAN_POINT('Ctrl Pts',(0.0138021558477243,-0.0339153382773235,
0.0728207193664956));
#84148=CARTESIAN_POINT('Ctrl Pts',(0.0137625771340758,-0.0339675558473117,
0.0728299845576844));
#84149=CARTESIAN_POINT('Ctrl Pts',(0.0137237464515299,-0.0340203938281304,
0.0728390746383015));
#84150=CARTESIAN_POINT('Ctrl Pts',(0.0136928625482014,-0.0341934961088741,
0.0727193979450169));
#84151=CARTESIAN_POINT('Ctrl Pts',(0.0136632859777598,-0.0340287516182428,
0.0726042615960629));
#84152=CARTESIAN_POINT('Ctrl Pts',(0.0136289760072808,-0.0338644633275951,
0.0724904460510118));
#84153=CARTESIAN_POINT('Ctrl Pts',(0.0136939320316319,-0.0341934961088741,
0.0727176746960287));
#84154=CARTESIAN_POINT('Ctrl Pts',(0.0136643198343752,-0.0340287516182428,
0.0726025162363473));
#84155=CARTESIAN_POINT('Ctrl Pts',(0.0136299733536702,-0.0338644633275951,
0.0724886800719453));
#84156=CARTESIAN_POINT('Ctrl Pts',(0.0138721285418795,-0.0341934961088741,
0.0724305482691845));
#84157=CARTESIAN_POINT('Ctrl Pts',(0.0138365802319494,-0.0340287516182428,
0.072311705737039));
#84158=CARTESIAN_POINT('Ctrl Pts',(0.0137961504453558,-0.0338644633275951,
0.0721944339921828));
#84159=CARTESIAN_POINT('',(0.0138684426480446,-0.0341764758832429,0.0724182736220124));
#84160=CARTESIAN_POINT('',(0.0138721285418775,-0.034193496108874,0.0724305482691878));
#84161=CARTESIAN_POINT('Origin',(-0.00213246844137344,-0.0345621026629259,
0.0767068832286424));
#84162=CARTESIAN_POINT('Ctrl Pts',(0.0138684426476736,-0.0341764758837534,
0.0724182736237905));
#84163=CARTESIAN_POINT('Ctrl Pts',(0.0138273449891587,-0.0341260050040849,
0.0724306625164513));
#84164=CARTESIAN_POINT('Ctrl Pts',(0.0137869617159301,-0.0340749269148957,
0.0724428360975123));
#84165=CARTESIAN_POINT('Ctrl Pts',(0.0137075925896597,-0.0339715436307851,
0.0724667618954668));
#84166=CARTESIAN_POINT('Ctrl Pts',(0.0136686368456731,-0.0339192778238039,
0.0724785050297447));
#84167=CARTESIAN_POINT('Ctrl Pts',(0.0136303825183667,-0.0338664212856659,
0.0724900367844655));
#84168=CARTESIAN_POINT('',(0.0137830302867648,-0.0341934961088841,0.0725741114826183));
#84169=CARTESIAN_POINT('Origin',(0.00812378219310841,-0.0315241814719618,
0.07415));
#84170=CARTESIAN_POINT('',(0.0138684426470952,-0.0342105180190359,0.0724182736214201));
#84171=CARTESIAN_POINT('',(0.0138647305447434,-0.0341934961088739,0.0724060068739043));
#84172=CARTESIAN_POINT('Origin',(-0.00212448227071318,-0.0345621716560879,
0.076751499706941));
#84173=CARTESIAN_POINT('Origin',(-0.0018368641682059,-0.0345621029931306,
0.0776874954962821));
#84174=CARTESIAN_POINT('Origin',(-0.00185486469899319,-0.0345621722856476,
0.0776458982597908));
#84175=CARTESIAN_POINT('Ctrl Pts',(0.013665592363582,-0.0346945769586966,
0.0726115454875291));
#84176=CARTESIAN_POINT('Ctrl Pts',(0.0136333688178547,-0.0345275153362944,
0.0724954700546888));
#84177=CARTESIAN_POINT('Ctrl Pts',(0.0135974864719452,-0.0343603235965185,
0.0723803779996495));
#84178=CARTESIAN_POINT('Ctrl Pts',(0.0135580565090045,-0.034193496108874,
0.0722666081363406));
#84179=CARTESIAN_POINT('Ctrl Pts',(0.0136413962967475,-0.0346945769586966,
0.0725312798116086));
#84180=CARTESIAN_POINT('Ctrl Pts',(0.0136074915543014,-0.0345275153362944,
0.0724157111750757));
#84181=CARTESIAN_POINT('Ctrl Pts',(0.013569943515107,-0.0343603235965185,
0.0723011789195167));
#84182=CARTESIAN_POINT('Ctrl Pts',(0.0135288682640893,-0.034193496108874,
0.0721880201300037));
#84183=CARTESIAN_POINT('Ctrl Pts',(0.0136172002299135,-0.0346945769586966,
0.0724510141356857));
#84184=CARTESIAN_POINT('Ctrl Pts',(0.0135816142907487,-0.0345275153362944,
0.0723359522954619));
#84185=CARTESIAN_POINT('Ctrl Pts',(0.0135424005582692,-0.0343603235965185,
0.0722219798393845));
#84186=CARTESIAN_POINT('Ctrl Pts',(0.0134996800191743,-0.034193496108874,
0.0721094321236683));
#84187=CARTESIAN_POINT('Ctrl Pts',(0.0135930041630785,-0.0346945769586966,
0.0723707484597675));
#84188=CARTESIAN_POINT('Ctrl Pts',(0.0135557370271948,-0.0345275153362944,
0.0722561934158495));
#84189=CARTESIAN_POINT('Ctrl Pts',(0.0135148576014305,-0.0343603235965185,
0.072142780759251));
#84190=CARTESIAN_POINT('Ctrl Pts',(0.013470491774259,-0.034193496108874,
0.0720308441173299));
#84191=CARTESIAN_POINT('',(0.0135930041633322,-0.0346945769586966,0.07237074846061));
#84192=CARTESIAN_POINT('',(0.0135152865461708,-0.0343667727832834,0.0721475500476732));
#84193=CARTESIAN_POINT('Origin',(-0.00233824736348184,-0.0345626461565297,
0.0777459202266467));
#84194=CARTESIAN_POINT('Origin',(0.0238759442165926,-0.0341934771027844,
0.0682995079518087));
#84195=CARTESIAN_POINT('',(0.0135575342506988,-0.034193496108874,0.072265201979884));
#84196=CARTESIAN_POINT('',(0.0135357736316764,-0.034193496108884,0.0722066125144644));
#84197=CARTESIAN_POINT('',(0.0136303825167689,-0.0345211942962639,0.0724900367849185));
#84198=CARTESIAN_POINT('Origin',(-0.00247383661447089,-0.0345625596118539,
0.0772846114966054));
#84199=CARTESIAN_POINT('',(0.0136290817962303,-0.0346945769586886,0.0724904288867703));
#84200=CARTESIAN_POINT('Origin',(0.0242218213462858,-0.0346945685853862,
0.0692972511550581));
#84201=CARTESIAN_POINT('',(0.0136110429797913,-0.0346945769587026,0.0724305886737002));
#84202=CARTESIAN_POINT('Ctrl Pts',(0.0139319059288102,-0.0345231616327842,
0.0726447762057216));
#84203=CARTESIAN_POINT('Ctrl Pts',(0.0139111585379916,-0.0344132092796988,
0.0725647193972091));
#84204=CARTESIAN_POINT('Ctrl Pts',(0.0138887563057069,-0.0343032738558979,
0.0724850958626736));
#84205=CARTESIAN_POINT('Ctrl Pts',(0.0138647305447509,-0.0341934961088739,
0.0724060068739077));
#84206=CARTESIAN_POINT('Ctrl Pts',(0.0138309322220635,-0.0345231616327842,
0.072593342299737));
#84207=CARTESIAN_POINT('Ctrl Pts',(0.0138094758872641,-0.0344132092796988,
0.0725146772716124));
#84208=CARTESIAN_POINT('Ctrl Pts',(0.0137863935354563,-0.0343032738558979,
0.0724364601096024));
#84209=CARTESIAN_POINT('Ctrl Pts',(0.0137617173045948,-0.0341934961088739,
0.0723587902614548));
#84210=CARTESIAN_POINT('Ctrl Pts',(0.0137299585153168,-0.0345231616327842,
0.0725419083937524));
#84211=CARTESIAN_POINT('Ctrl Pts',(0.0137077932365365,-0.0344132092796988,
0.0724646351460157));
#84212=CARTESIAN_POINT('Ctrl Pts',(0.0136840307652057,-0.0343032738558979,
0.0723878243565312));
#84213=CARTESIAN_POINT('Ctrl Pts',(0.0136587040644386,-0.0341934961088739,
0.0723115736490019));
#84214=CARTESIAN_POINT('Ctrl Pts',(0.0136289848085701,-0.0345231616327842,
0.0724904744877679));
#84215=CARTESIAN_POINT('Ctrl Pts',(0.013606110585809,-0.0344132092796988,
0.072414593020419));
#84216=CARTESIAN_POINT('Ctrl Pts',(0.013581667994955,-0.0343032738558979,
0.0723391886034599));
#84217=CARTESIAN_POINT('Ctrl Pts',(0.0135556908242825,-0.0341934961088739,
0.0722643570365489));
#84218=CARTESIAN_POINT('',(0.0137111323977311,-0.0341934961088839,0.0723356044269041));
#84219=CARTESIAN_POINT('Ctrl Pts',(0.0138684426437819,-0.0342105180195366,
0.0724182736224121));
#84220=CARTESIAN_POINT('Ctrl Pts',(0.0138272987795925,-0.0342610556240338,
0.0724306764294195));
#84221=CARTESIAN_POINT('Ctrl Pts',(0.0137868932207699,-0.0343122189868186,
0.0724428566744688));
#84222=CARTESIAN_POINT('Ctrl Pts',(0.013707523294857,-0.0344158119695113,
0.0724667827176998));
#84223=CARTESIAN_POINT('Ctrl Pts',(0.0136685913908666,-0.0344681990449995,
0.0724785187298886));
#84224=CARTESIAN_POINT('Ctrl Pts',(0.013630382516736,-0.0345211942962405,
0.0724900367849169));
#84225=CARTESIAN_POINT('Ctrl Pts',(0.0135920452288826,-0.0346945769586932,
0.0723725350249574));
#84226=CARTESIAN_POINT('Ctrl Pts',(0.0135552973982297,-0.0345296777077528,
0.0722594825559492));
#84227=CARTESIAN_POINT('Ctrl Pts',(0.01351390840571,-0.0343648066252516,
0.0721480455104717));
#84228=CARTESIAN_POINT('Ctrl Pts',(0.013593004163335,-0.0346945769586932,
0.0723707484606187));
#84229=CARTESIAN_POINT('Ctrl Pts',(0.0135562193967285,-0.0345296777077528,
0.0722576761663191));
#84230=CARTESIAN_POINT('Ctrl Pts',(0.0135147926804191,-0.0343648066252516,
0.0721462208390877));
#84231=CARTESIAN_POINT('Ctrl Pts',(0.0137528202259623,-0.0346945769586932,
0.0720729995607341));
#84232=CARTESIAN_POINT('Ctrl Pts',(0.0137098797115331,-0.0345296777077528,
0.0719566231824231));
#84233=CARTESIAN_POINT('Ctrl Pts',(0.0136621659465823,-0.0343648066252516,
0.0718421210171928));
#84234=CARTESIAN_POINT('',(0.0137483708741045,-0.0346775396665011,0.0720609805737824));
#84235=CARTESIAN_POINT('',(0.0137528202259598,-0.0346945769586885,0.0720729995607336));
#84236=CARTESIAN_POINT('Origin',(-0.00176065482130531,-0.0345626617948099,
0.0779840729315746));
#84237=CARTESIAN_POINT('Ctrl Pts',(0.0137483708737416,-0.0346775396670097,
0.0720609805755654));
#84238=CARTESIAN_POINT('Ctrl Pts',(0.0137081005252722,-0.0346269749928341,
0.072075937334604));
#84239=CARTESIAN_POINT('Ctrl Pts',(0.0136685458832602,-0.0345757902891105,
0.0720906283123326));
#84240=CARTESIAN_POINT('Ctrl Pts',(0.0135908353765566,-0.034472168108849,
0.0721194906424885));
#84241=CARTESIAN_POINT('Ctrl Pts',(0.0135527099760803,-0.0344197714290295,
0.072133650674239));
#84242=CARTESIAN_POINT('Ctrl Pts',(0.013515286546433,-0.0343667727831644,
0.0721475500479254));
#84243=CARTESIAN_POINT('',(0.013672912194656,-0.0346945769587026,0.0722218740106818));
#84244=CARTESIAN_POINT('Origin',(0.00812378219310841,-0.0315241814719618,
0.07415));
#84245=CARTESIAN_POINT('',(0.0137483708727411,-0.0347116136489605,0.072060980573501));
#84246=CARTESIAN_POINT('',(0.0137438958601234,-0.0346945769586885,0.0720489711163712));
#84247=CARTESIAN_POINT('Origin',(-0.00174313866280795,-0.0345626697892552,
0.0780258618694538));
#84248=CARTESIAN_POINT('Origin',(-0.00186699873920255,-0.0345626621421502,
0.0776977502616594));
#84249=CARTESIAN_POINT('Origin',(-0.00188100566606441,-0.0345626702099699,
0.0776546580696877));
#84250=CARTESIAN_POINT('Ctrl Pts',(0.0135701215504443,-0.0352450361874068,
0.0723017169506921));
#84251=CARTESIAN_POINT('Ctrl Pts',(0.0135004124113659,-0.0349452760959492,
0.072096304891175));
#84252=CARTESIAN_POINT('Ctrl Pts',(0.0134154288318132,-0.034644428984174,
0.0718967271632779));
#84253=CARTESIAN_POINT('Ctrl Pts',(0.0135692572954986,-0.0352450361874068,
0.0722993444649938));
#84254=CARTESIAN_POINT('Ctrl Pts',(0.0134994586766537,-0.0349452760959492,
0.0720939650013869));
#84255=CARTESIAN_POINT('Ctrl Pts',(0.0134143883267945,-0.034644428984174,
0.0718944265167805));
#84256=CARTESIAN_POINT('Ctrl Pts',(0.0134836874988876,-0.0352450361874068,
0.0720644448909032));
#84257=CARTESIAN_POINT('Ctrl Pts',(0.0134050294972302,-0.0349452760959492,
0.0718622927451332));
#84258=CARTESIAN_POINT('Ctrl Pts',(0.013311368027917,-0.034644428984174,
0.0716666397348567));
#84259=CARTESIAN_POINT('Ctrl Pts',(0.0134828318009215,-0.0352450361874068,
0.0720620958951623));
#84260=CARTESIAN_POINT('Ctrl Pts',(0.013404085205436,-0.0349452760959492,
0.0718599760225706));
#84261=CARTESIAN_POINT('Ctrl Pts',(0.0133103378249283,-0.034644428984174,
0.0716643618670375));
#84262=CARTESIAN_POINT('',(0.0134705059039946,-0.0351951634053353,0.0720308733256515));
#84263=CARTESIAN_POINT('',(0.0133789127711297,-0.0348678972925388,0.0718129660661543));
#84264=CARTESIAN_POINT('Origin',(-0.00175364642638072,-0.0345636767886418,
0.0790043718872262));
#84265=CARTESIAN_POINT('Origin',(0.0234753725359348,-0.0346946199340819,
0.0673229226914049));
#84266=CARTESIAN_POINT('',(0.0134284645421554,-0.0346945769330288,0.0719277331002202));
#84267=CARTESIAN_POINT('',(0.0134030679965503,-0.0346945769458128,0.0718706256001972));
#84268=CARTESIAN_POINT('',(0.0135152865462252,-0.0350221583435276,0.0721475500479853));
#84269=CARTESIAN_POINT('Origin',(-0.00198618243163102,-0.0345628458712737,
0.0785835745506406));
#84270=CARTESIAN_POINT('',(0.0135141281047203,-0.0351951360298762,0.0721479835292734));
#84271=CARTESIAN_POINT('Origin',(0.0238436625345186,-0.0351951838366798,
0.0683115056739125));
#84272=CARTESIAN_POINT('',(0.013470491774678,-0.0351951371328748,0.0720308441181244));
#84273=CARTESIAN_POINT('Ctrl Pts',(0.0138259308403723,-0.0350241211494342,
0.072283050401166));
#84274=CARTESIAN_POINT('Ctrl Pts',(0.0138002143751275,-0.0349144232818962,
0.0722045056415219));
#84275=CARTESIAN_POINT('Ctrl Pts',(0.0137728589410318,-0.0348045283579412,
0.0721264454467658));
#84276=CARTESIAN_POINT('Ctrl Pts',(0.0137438958562392,-0.0346945769439158,
0.0720489711059647));
#84277=CARTESIAN_POINT('Ctrl Pts',(0.0137219267903495,-0.0350241211494342,
0.072238058186481));
#84278=CARTESIAN_POINT('Ctrl Pts',(0.0136955905757949,-0.0349144232818962,
0.0721609460399827));
#84279=CARTESIAN_POINT('Ctrl Pts',(0.013667644634577,-0.0348045283579412,
0.0720843321265214));
#84280=CARTESIAN_POINT('Ctrl Pts',(0.0136381211101503,-0.0346945769439158,
0.0720083159108078));
#84281=CARTESIAN_POINT('Ctrl Pts',(0.0136179227403266,-0.0350241211494342,
0.0721930659717961));
#84282=CARTESIAN_POINT('Ctrl Pts',(0.0135909667764623,-0.0349144232818962,
0.0721173864384435));
#84283=CARTESIAN_POINT('Ctrl Pts',(0.0135624303281222,-0.0348045283579412,
0.0720422188062771));
#84284=CARTESIAN_POINT('Ctrl Pts',(0.0135323463640614,-0.0346945769439158,
0.0719676607156509));
#84285=CARTESIAN_POINT('Ctrl Pts',(0.0135139186903038,-0.0350241211494342,
0.0721480737571111));
#84286=CARTESIAN_POINT('Ctrl Pts',(0.0134863429771297,-0.0349144232818962,
0.0720738268369042));
#84287=CARTESIAN_POINT('Ctrl Pts',(0.0134572160216674,-0.0348045283579412,
0.0720001054860327));
#84288=CARTESIAN_POINT('Ctrl Pts',(0.0134265716179725,-0.0346945769439158,
0.071927005520494));
#84289=CARTESIAN_POINT('',(0.0135861802013343,-0.0346945769458128,0.0719883521085386));
#84290=CARTESIAN_POINT('Ctrl Pts',(0.0137483708696529,-0.0347116136492775,
0.0720609805746409));
#84291=CARTESIAN_POINT('Ctrl Pts',(0.0137081165090017,-0.0347621546531341,
0.0720759313819251));
#84292=CARTESIAN_POINT('Ctrl Pts',(0.0136685699287866,-0.0348133084095077,
0.072090619313617));
#84293=CARTESIAN_POINT('Ctrl Pts',(0.0135908593246316,-0.0349168561544569,
0.0721194816840003));
#84294=CARTESIAN_POINT('Ctrl Pts',(0.0135527261247601,-0.0349692089015922,
0.0721336446743741));
#84295=CARTESIAN_POINT('Ctrl Pts',(0.0135152865461839,-0.0350221583435,
0.0721475500479793));
#84296=CARTESIAN_POINT('Ctrl Pts',(0.0134698821779314,-0.0351951371254984,
0.0720321740849387));
#84297=CARTESIAN_POINT('Ctrl Pts',(0.0134260974559055,-0.0350307338980976,
0.0719216468220068));
#84298=CARTESIAN_POINT('Ctrl Pts',(0.0133777819366284,-0.0348659306897824,
0.0718130236737781));
#84299=CARTESIAN_POINT('Ctrl Pts',(0.0134704917745731,-0.0351951371254984,
0.072030844118175));
#84300=CARTESIAN_POINT('Ctrl Pts',(0.0134266795563188,-0.0350307338980976,
0.071920304252215));
#84301=CARTESIAN_POINT('Ctrl Pts',(0.013378336043412,-0.0348659306897824,
0.0718116696481763));
#84302=CARTESIAN_POINT('Ctrl Pts',(0.0135726608071045,-0.0351951371254984,
0.0718079403023807));
#84303=CARTESIAN_POINT('Ctrl Pts',(0.0135242401923132,-0.0350307338980976,
0.071695288155776));
#84304=CARTESIAN_POINT('Ctrl Pts',(0.0134712049178788,-0.0348659306897824,
0.0715847335460256));
#84305=CARTESIAN_POINT('Origin',(0.0182382410915186,-0.0308609197410726,
0.069651951223391));
#84306=CARTESIAN_POINT('',(0.0135150351691523,-0.0351951371254984,0.0719336630802996));
#84307=CARTESIAN_POINT('Origin',(0.00729792487674236,-0.0351840467441107,
0.0746722119717951));
#84308=CARTESIAN_POINT('Origin',(0.0187096461764174,-0.0352322614198991,
0.0685725714915023));
#84309=CARTESIAN_POINT('',(0.0132782959248752,-0.0351951142564679,0.0715987644615895));
#84310=CARTESIAN_POINT('',(0.0132205951624505,-0.0351951372916786,0.0714882341283375));
#84311=CARTESIAN_POINT('Origin',(0.00783124796754103,-0.03528751231571,
0.0739755489261077));
#84312=CARTESIAN_POINT('Origin',(0.0102594085301971,-0.0298325076522881,
0.0813426553113457));
#84313=CARTESIAN_POINT('Origin',(0.0164673641357985,-0.0338731817900826,
0.0733520452999505));
#84314=CARTESIAN_POINT('Ctrl Pts',(0.0137934174940089,-0.0321934096636942,
0.0751161114325452));
#84315=CARTESIAN_POINT('Ctrl Pts',(0.013810710428568,-0.032050846084551,
0.075014627660664));
#84316=CARTESIAN_POINT('Ctrl Pts',(0.013825263655493,-0.0319086045665435,
0.0749127557808521));
#84317=CARTESIAN_POINT('Ctrl Pts',(0.0138370638972198,-0.031766989287143,
0.0748107177209326));
#84318=CARTESIAN_POINT('Ctrl Pts',(0.01380570180146,-0.0321934096636942,
0.0750331685098925));
#84319=CARTESIAN_POINT('Ctrl Pts',(0.0138215100972028,-0.032050846084551,
0.074931464854758));
#84320=CARTESIAN_POINT('Ctrl Pts',(0.0138345738969051,-0.0319086045665435,
0.074829413146801));
#84321=CARTESIAN_POINT('Ctrl Pts',(0.0138448831618781,-0.031766989287143,
0.0747272354370263));
#84322=CARTESIAN_POINT('Ctrl Pts',(0.0138179861089111,-0.0321934096636942,
0.0749502255872398));
#84323=CARTESIAN_POINT('Ctrl Pts',(0.0138323097658377,-0.032050846084551,
0.074848302048852));
#84324=CARTESIAN_POINT('Ctrl Pts',(0.0138438841383172,-0.0319086045665435,
0.07474607051275));
#84325=CARTESIAN_POINT('Ctrl Pts',(0.0138527024265365,-0.031766989287143,
0.07464375315312));
#84326=CARTESIAN_POINT('Ctrl Pts',(0.0138302704163622,-0.0321934096636942,
0.0748672826645872));
#84327=CARTESIAN_POINT('Ctrl Pts',(0.0138431094344726,-0.032050846084551,
0.074765139242946));
#84328=CARTESIAN_POINT('Ctrl Pts',(0.0138531943797292,-0.0319086045665435,
0.0746627278786989));
#84329=CARTESIAN_POINT('Ctrl Pts',(0.0138605216911947,-0.031766989287143,
0.0745602708692137));
#84330=CARTESIAN_POINT('',(0.0138300506476721,-0.0321934096636942,0.0748687665298636));
#84331=CARTESIAN_POINT('',(0.0138547629063297,-0.0318665617511349,0.0746337200160556));
#84332=CARTESIAN_POINT('Origin',(-0.00266067940269165,-0.0326371944422615,
0.0721717816860202));
#84333=CARTESIAN_POINT('Origin',(0.0247771115982228,-0.0316939261509145,
0.0755556143725815));
#84334=CARTESIAN_POINT('',(0.0138130737121441,-0.0320197221621798,0.074992348608336));
#84335=CARTESIAN_POINT('Ctrl Pts',(0.0138131465811933,-0.032019739209471,
0.074992178593686));
#84336=CARTESIAN_POINT('Ctrl Pts',(0.0138174318101975,-0.0319792716576008,
0.0749632292717222));
#84337=CARTESIAN_POINT('Ctrl Pts',(0.0138215158492161,-0.0319386439829705,
0.0749341154925669));
#84338=CARTESIAN_POINT('Ctrl Pts',(0.0138253946102038,-0.0318979099381637,
0.0749048055173526));
#84339=CARTESIAN_POINT('Ctrl Pts',(0.013829273294525,-0.0318571766984946,
0.074875496121471));
#84340=CARTESIAN_POINT('Ctrl Pts',(0.0138329287612101,-0.0318163871833603,
0.0748461397405178));
#84341=CARTESIAN_POINT('Ctrl Pts',(0.0138363519311294,-0.0317755399638303,
0.0748168377834398));
#84342=CARTESIAN_POINT('',(0.0138117372188363,-0.0321934096636183,0.0749924177261294));
#84343=CARTESIAN_POINT('Origin',(0.016097707842897,-0.0324112005641101,
0.0753097251637006));
#84344=CARTESIAN_POINT('',(0.0138208939332642,-0.0321934096636663,0.0749305921280065));
#84345=CARTESIAN_POINT('Ctrl Pts',(0.0138284218364189,-0.0321934096636618,
0.0748699751080699));
#84346=CARTESIAN_POINT('Ctrl Pts',(0.0138383508542749,-0.0320835708272592,
0.0747913036814525));
#84347=CARTESIAN_POINT('Ctrl Pts',(0.013846646011812,-0.0319739230346489,
0.0747124724069512));
#84348=CARTESIAN_POINT('Ctrl Pts',(0.0138533044366094,-0.0318646057455573,
0.0746335829582368));
#84349=CARTESIAN_POINT('Ctrl Pts',(0.013919425177682,-0.0321934096636618,
0.0748024506188517));
#84350=CARTESIAN_POINT('Ctrl Pts',(0.0139284229802062,-0.0320835708272592,
0.0747225241852344));
#84351=CARTESIAN_POINT('Ctrl Pts',(0.0139357614902496,-0.0319739230346489,
0.0746424579031413));
#84352=CARTESIAN_POINT('Ctrl Pts',(0.0139414391806242,-0.0318646057455573,
0.0745623549324136));
#84353=CARTESIAN_POINT('Ctrl Pts',(0.0140104285189451,-0.0321934096636618,
0.0747349261296334));
#84354=CARTESIAN_POINT('Ctrl Pts',(0.0140184951061375,-0.0320835708272592,
0.0746537446890163));
#84355=CARTESIAN_POINT('Ctrl Pts',(0.0140248769686871,-0.0319739230346489,
0.0745724433993313));
#84356=CARTESIAN_POINT('Ctrl Pts',(0.0140295739246389,-0.0318646057455573,
0.0744911269065904));
#84357=CARTESIAN_POINT('Ctrl Pts',(0.0141014318602082,-0.0321934096636618,
0.0746674016404153));
#84358=CARTESIAN_POINT('Ctrl Pts',(0.0141085672320688,-0.0320835708272592,
0.0745849651927983));
#84359=CARTESIAN_POINT('Ctrl Pts',(0.0141139924471247,-0.0319739230346489,
0.0745024288955213));
#84360=CARTESIAN_POINT('Ctrl Pts',(0.0141177086686537,-0.0318646057455573,
0.0744198988807672));
#84361=CARTESIAN_POINT('',(0.0141025234007916,-0.0321763980308495,0.0746546320931235));
#84362=CARTESIAN_POINT('',(0.0141014318602036,-0.0321934096636185,0.0746674016403882));
#84363=CARTESIAN_POINT('Origin',(-0.00232360210459169,-0.032638623159475,
0.0726525106268163));
#84364=CARTESIAN_POINT('Ctrl Pts',(0.0141025233976242,-0.0321763980306333,
0.0746546320928512));
#84365=CARTESIAN_POINT('Ctrl Pts',(0.0140597565715851,-0.0321259596175605,
0.0746510223843539));
#84366=CARTESIAN_POINT('Ctrl Pts',(0.0140177307362986,-0.032074916463295,
0.0746474752187469));
#84367=CARTESIAN_POINT('Ctrl Pts',(0.0139351272259753,-0.031971605779401,
0.0746405031186233));
#84368=CARTESIAN_POINT('Ctrl Pts',(0.0138945817362173,-0.0319193786690213,
0.0746370809006859));
#84369=CARTESIAN_POINT('Ctrl Pts',(0.0138547629044771,-0.031866561752542,
0.0746337200158928));
#84370=CARTESIAN_POINT('',(0.0139657412539479,-0.0321934096636664,0.0747680840851359));
#84371=CARTESIAN_POINT('Origin',(0.00812378219310841,-0.0315241814719618,
0.07415));
#84372=CARTESIAN_POINT('',(0.0141025234011606,-0.0322104233323761,0.0746546320931547));
#84373=CARTESIAN_POINT('',(0.0141035876665869,-0.0321934096636183,0.0746418602437372));
#84374=CARTESIAN_POINT('Origin',(-0.0023336699492245,-0.0326387244457676,
0.0726967111254948));
#84375=CARTESIAN_POINT('Origin',(-0.00242680112296162,-0.0326386236421912,
0.0738751690576688));
#84376=CARTESIAN_POINT('Origin',(-0.00242931534677929,-0.0326387248002166,
0.073829906406133));
#84377=CARTESIAN_POINT('Ctrl Pts',(0.013838961113965,-0.0327445246967099,
0.0747940923090646));
#84378=CARTESIAN_POINT('Ctrl Pts',(0.0138632534525274,-0.0324436878339361,
0.0745785408122748));
#84379=CARTESIAN_POINT('Ctrl Pts',(0.0138712405594134,-0.0321434074405928,
0.0743617718762977));
#84380=CARTESIAN_POINT('Ctrl Pts',(0.0138615525804706,-0.0327445246967099,
0.0745451151501902));
#84381=CARTESIAN_POINT('Ctrl Pts',(0.0138764545919749,-0.0324436878339361,
0.0743287116023121));
#84382=CARTESIAN_POINT('Ctrl Pts',(0.01387501386876,-0.0321434074405928,
0.0741118003536464));
#84383=CARTESIAN_POINT('',(0.0138639223541771,-0.0326943950436612,0.074509048647521));
#84384=CARTESIAN_POINT('',(0.0138738271570598,-0.0323666188837389,0.0742729142487172));
#84385=CARTESIAN_POINT('Origin',(-0.00291881110367563,-0.0326395579114917,
0.073535438921432));
#84386=CARTESIAN_POINT('Origin',(0.0249159129258074,-0.0321933825603069,
0.0745089517599611));
#84387=CARTESIAN_POINT('',(0.0138697975139044,-0.0321934096532689,0.0743978566723672));
#84388=CARTESIAN_POINT('',(0.0138711332231658,-0.0321934096584275,0.0743353709441848));
#84389=CARTESIAN_POINT('',(0.0138547629072614,-0.0325210109756238,0.0746337200161324));
#84390=CARTESIAN_POINT('Origin',(-0.00286351017779509,-0.0326393129154698,
0.0730578132976465));
#84391=CARTESIAN_POINT('',(0.0138534091855672,-0.0326943950436595,0.0746336057560539));
#84392=CARTESIAN_POINT('Origin',(0.0248766686670716,-0.0326943765538132,
0.0755640180815124));
#84393=CARTESIAN_POINT('',(0.0138586657698822,-0.0326943950436703,0.0745713272017975));
#84394=CARTESIAN_POINT('Ctrl Pts',(0.0140781488874457,-0.0325229783203769,
0.0748885914090138));
#84395=CARTESIAN_POINT('Ctrl Pts',(0.014088330353867,-0.032413025309245,
0.0748065105943457));
#84396=CARTESIAN_POINT('Ctrl Pts',(0.0140968123289778,-0.032303122220807,
0.0747242316121296));
#84397=CARTESIAN_POINT('Ctrl Pts',(0.0141035876669614,-0.0321934096576658,
0.0746418602392752));
#84398=CARTESIAN_POINT('Ctrl Pts',(0.0140031999771526,-0.0325229783203769,
0.0748035984499946));
#84399=CARTESIAN_POINT('Ctrl Pts',(0.0140122098174925,-0.032413025309245,
0.074722550804416));
#84400=CARTESIAN_POINT('Ctrl Pts',(0.0140195417166517,-0.032303122220807,
0.0746413290711794));
#84401=CARTESIAN_POINT('Ctrl Pts',(0.0140251899541918,-0.0321934096576658,
0.0745600376209509));
#84402=CARTESIAN_POINT('Ctrl Pts',(0.0139282510668594,-0.0325229783203769,
0.0747186054909755));
#84403=CARTESIAN_POINT('Ctrl Pts',(0.0139360892811179,-0.032413025309245,
0.0746385910144862));
#84404=CARTESIAN_POINT('Ctrl Pts',(0.0139422711043256,-0.032303122220807,
0.0745584265302292));
#84405=CARTESIAN_POINT('Ctrl Pts',(0.0139467922414221,-0.0321934096576658,
0.0744782150026266));
#84406=CARTESIAN_POINT('Ctrl Pts',(0.0138533021565663,-0.0325229783203769,
0.0746336125319563));
#84407=CARTESIAN_POINT('Ctrl Pts',(0.0138599687447434,-0.032413025309245,
0.0745546312245564));
#84408=CARTESIAN_POINT('Ctrl Pts',(0.0138650004919996,-0.032303122220807,
0.074475523989279));
#84409=CARTESIAN_POINT('Ctrl Pts',(0.0138683945286525,-0.0321934096576658,
0.0743963923843022));
#84410=CARTESIAN_POINT('',(0.0139866925903711,-0.0321934096584275,0.0745198584585543));
#84411=CARTESIAN_POINT('Ctrl Pts',(0.014102523397689,-0.0322104233328891,
0.0746546320928567));
#84412=CARTESIAN_POINT('Ctrl Pts',(0.0140596986219331,-0.0322609421830332,
0.0746510174931481));
#84413=CARTESIAN_POINT('Ctrl Pts',(0.0140176444772595,-0.0323120888238626,
0.0746474679380973));
#84414=CARTESIAN_POINT('Ctrl Pts',(0.0139350403414708,-0.0324156524631808,
0.0746404957851817));
#84415=CARTESIAN_POINT('Ctrl Pts',(0.0138945243052323,-0.0324680267167313,
0.0746370760532579));
#84416=CARTESIAN_POINT('Ctrl Pts',(0.0138547629072187,-0.0325210109755912,
0.0746337200161243));
#84417=CARTESIAN_POINT('Origin',(0.00652265831989126,-0.0262834582510687,
0.0818532323205447));
#84418=CARTESIAN_POINT('Origin',(0.0185015283592357,-0.0342770720633309,
0.0804844431153851));
#84419=CARTESIAN_POINT('Ctrl Pts',(0.0138623730203407,-0.0326943950436604,
0.0745103567971669));
#84420=CARTESIAN_POINT('Ctrl Pts',(0.0138673394123863,-0.0325844576448134,
0.0744312682603022));
#84421=CARTESIAN_POINT('Ctrl Pts',(0.0138706704753014,-0.0324744968375322,
0.0743520714130887));
#84422=CARTESIAN_POINT('Ctrl Pts',(0.0138723633407325,-0.0323646534831895,
0.0742728677860138));
#84423=CARTESIAN_POINT('Ctrl Pts',(0.0139489567641809,-0.0326943950436604,
0.0744372515108694));
#84424=CARTESIAN_POINT('Ctrl Pts',(0.0139529156283674,-0.0325844576448134,
0.0743569696877393));
#84425=CARTESIAN_POINT('Ctrl Pts',(0.0139552144130027,-0.0324744968375322,
0.0742766003071378));
#84426=CARTESIAN_POINT('Ctrl Pts',(0.01395585159307,-0.0323646534831895,
0.0741962463836274));
#84427=CARTESIAN_POINT('Ctrl Pts',(0.0140355405080212,-0.0326943950436604,
0.0743641462245718));
#84428=CARTESIAN_POINT('Ctrl Pts',(0.0140384918443486,-0.0325844576448134,
0.0742826711151764));
#84429=CARTESIAN_POINT('Ctrl Pts',(0.0140397583507041,-0.0324744968375322,
0.0742011292011868));
#84430=CARTESIAN_POINT('Ctrl Pts',(0.0140393398454075,-0.0323646534831895,
0.0741196249812409));
#84431=CARTESIAN_POINT('Ctrl Pts',(0.0141221242518614,-0.0326943950436604,
0.0742910409382743));
#84432=CARTESIAN_POINT('Ctrl Pts',(0.0141240680603297,-0.0325844576448134,
0.0742083725426135));
#84433=CARTESIAN_POINT('Ctrl Pts',(0.0141243022884054,-0.0324744968375322,
0.0741256580952359));
#84434=CARTESIAN_POINT('Ctrl Pts',(0.0141228280977449,-0.0323646534831895,
0.0740430035788545));
#84435=CARTESIAN_POINT('',(0.0141224118322334,-0.0326773559991375,0.0742782280504027));
#84436=CARTESIAN_POINT('',(0.0141221242518551,-0.0326943950436594,0.0742910409382789));
#84437=CARTESIAN_POINT('Origin',(-0.00248001269496984,-0.0326395671409485,
0.0739735830128659));
#84438=CARTESIAN_POINT('Ctrl Pts',(0.0141224118288766,-0.032677355998747,
0.0742782280503258));
#84439=CARTESIAN_POINT('Ctrl Pts',(0.0140794682075917,-0.0326267922586638,
0.0742773100778611));
#84440=CARTESIAN_POINT('Ctrl Pts',(0.0140372857309823,-0.0325756109580676,
0.0742764083757955));
#84441=CARTESIAN_POINT('Ctrl Pts',(0.0139544071675347,-0.0324719985462378,
0.0742746367450648));
#84442=CARTESIAN_POINT('Ctrl Pts',(0.0139137443211812,-0.0324196091621775,
0.0742737675269559));
#84443=CARTESIAN_POINT('Ctrl Pts',(0.013873827157011,-0.0323666188837757,
0.0742729142487162));
#84444=CARTESIAN_POINT('',(0.0139930233030261,-0.0326943950436702,0.07440004479291));
#84445=CARTESIAN_POINT('Origin',(0.00812378219310841,-0.0315241814719618,
0.07415));
#84446=CARTESIAN_POINT('',(0.0141224118321884,-0.0327114338380032,0.074278228050402));
#84447=CARTESIAN_POINT('',(0.0141226720466812,-0.0326943950436593,0.0742654145775365));
#84448=CARTESIAN_POINT('Origin',(-0.0024802039674448,-0.0326395680058319,
0.0740188921177947));
#84449=CARTESIAN_POINT('Origin',(-0.00247786602655803,-0.0326395674544514,
0.0738731251037909));
#84450=CARTESIAN_POINT('Origin',(-0.00247611923823949,-0.0326395684171705,
0.0738278493802772));
#84451=CARTESIAN_POINT('Ctrl Pts',(0.0138681283410459,-0.0332451089994431,
0.0744339231104998));
#84452=CARTESIAN_POINT('Ctrl Pts',(0.0138788366763559,-0.0329451141710252,
0.0742172715509252));
#84453=CARTESIAN_POINT('Ctrl Pts',(0.0138731955092698,-0.0326442513127493,
0.0740004288799743));
#84454=CARTESIAN_POINT('Ctrl Pts',(0.0138750401189723,-0.0332451089994431,
0.0741840186741128));
#84455=CARTESIAN_POINT('Ctrl Pts',(0.013876323154258,-0.0329451141710252,
0.0739671064325688));
#84456=CARTESIAN_POINT('Ctrl Pts',(0.0138612638277986,-0.0326442513127493,
0.0737507137723472));
#84457=CARTESIAN_POINT('Ctrl Pts',(0.0138751092367515,-0.0332451089994431,
0.074181519629749));
#84458=CARTESIAN_POINT('Ctrl Pts',(0.013876298019037,-0.0329451141710252,
0.0739646047813852));
#84459=CARTESIAN_POINT('Ctrl Pts',(0.0138611445109838,-0.0326442513127493,
0.0737482166212709));
#84460=CARTESIAN_POINT('',(0.0138751403498937,-0.0331951640388616,0.0741479137641467));
#84461=CARTESIAN_POINT('',(0.0138701986143845,-0.0328677532463078,0.0739116233757935));
#84462=CARTESIAN_POINT('Origin',(-0.00287100067133277,-0.0326403163408478,
0.0749219214001807));
#84463=CARTESIAN_POINT('Origin',(0.0249166461355166,-0.0326944278639039,
0.0734528619142166));
#84464=CARTESIAN_POINT('',(0.013874022114592,-0.0326943950436593,0.0740365722900837));
#84465=CARTESIAN_POINT('',(0.0138714316765818,-0.0326943950436693,0.0739741259961216));
#84466=CARTESIAN_POINT('',(0.0138738271570598,-0.0330220786163545,0.07427291424872));
#84467=CARTESIAN_POINT('Origin',(-0.00292227140940239,-0.0326396682764843,
0.0744439292436767));
#84468=CARTESIAN_POINT('',(0.0138724689321763,-0.0331951640388585,0.074272885214998));
#84469=CARTESIAN_POINT('Origin',(0.0249016024348994,-0.033195202656007,
0.0745086472152203));
#84470=CARTESIAN_POINT('',(0.013873804641045,-0.0331951640388701,0.0742103994895824));
#84471=CARTESIAN_POINT('Ctrl Pts',(0.0141127759013865,-0.0330240426238172,
0.0745132552302507));
#84472=CARTESIAN_POINT('Ctrl Pts',(0.0141177800960856,-0.0329142774063519,
0.0744307510071253));
#84473=CARTESIAN_POINT('Ctrl Pts',(0.0141210811928021,-0.0328043479726691,
0.0743481022019528));
#84474=CARTESIAN_POINT('Ctrl Pts',(0.0141226720466888,-0.0326943950436593,
0.0742654145775435));
#84475=CARTESIAN_POINT('Ctrl Pts',(0.0140326381402712,-0.0330240426238172,
0.0744331360987742));
#84476=CARTESIAN_POINT('Ctrl Pts',(0.0140365386158779,-0.0329142774063519,
0.0743517358513826));
#84477=CARTESIAN_POINT('Ctrl Pts',(0.01403875826552,-0.0328043479726691,
0.0742702143892727));
#84478=CARTESIAN_POINT('Ctrl Pts',(0.0140392913695379,-0.0326943950436593,
0.0741886760691986));
#84479=CARTESIAN_POINT('Ctrl Pts',(0.0139525003791559,-0.0330240426238172,
0.0743530169672976));
#84480=CARTESIAN_POINT('Ctrl Pts',(0.0139552971356702,-0.0329142774063519,
0.0742727206956399));
#84481=CARTESIAN_POINT('Ctrl Pts',(0.013956435338238,-0.0328043479726691,
0.0741923265765927));
#84482=CARTESIAN_POINT('Ctrl Pts',(0.013955910692387,-0.0326943950436593,
0.0741119375608538));
#84483=CARTESIAN_POINT('Ctrl Pts',(0.0138723626180405,-0.0330240426238172,
0.0742728978358211));
#84484=CARTESIAN_POINT('Ctrl Pts',(0.0138740556554625,-0.0329142774063519,
0.0741937055398971));
#84485=CARTESIAN_POINT('Ctrl Pts',(0.0138741124109559,-0.0328043479726691,
0.0741144387639126));
#84486=CARTESIAN_POINT('Ctrl Pts',(0.0138725300152361,-0.0326943950436593,
0.0740351990525089));
#84487=CARTESIAN_POINT('',(0.0139983470806466,-0.0326943950436694,0.0741509934338202));
#84488=CARTESIAN_POINT('Ctrl Pts',(0.0141224118288687,-0.0327114338383286,
0.0742782280503256));
#84489=CARTESIAN_POINT('Ctrl Pts',(0.0140794753505426,-0.032761987682999,
0.0742773102305505));
#84490=CARTESIAN_POINT('Ctrl Pts',(0.0140372963628984,-0.0328131562602354,
0.0742764086030658));
#84491=CARTESIAN_POINT('Ctrl Pts',(0.013954417875512,-0.0329167375858764,
0.074274636973961));
#84492=CARTESIAN_POINT('Ctrl Pts',(0.0139137513990614,-0.0329691088920617,
0.0742737676782542));
#84493=CARTESIAN_POINT('Ctrl Pts',(0.0138738271570123,-0.0330220786163186,
0.0742729142487162));
#84494=CARTESIAN_POINT('Ctrl Pts',(0.0138736759789704,-0.0331951640388604,
0.0741493168398912));
#84495=CARTESIAN_POINT('Ctrl Pts',(0.0138736618550735,-0.0330306422053993,
0.0740304414754913));
#84496=CARTESIAN_POINT('Ctrl Pts',(0.0138687344995519,-0.0328657862001531,
0.0739116682730077));
#84497=CARTESIAN_POINT('Ctrl Pts',(0.0138751403498937,-0.0331951640388604,
0.0741479137641499));
#84498=CARTESIAN_POINT('Ctrl Pts',(0.0138750972183061,-0.0330306422053993,
0.0740290081248209));
#84499=CARTESIAN_POINT('Ctrl Pts',(0.0138701396285862,-0.0328657862001531,
0.0739102058721961));
#84500=CARTESIAN_POINT('Ctrl Pts',(0.0141191439277879,-0.0331951640388604,
0.0739141236120178));
#84501=CARTESIAN_POINT('Ctrl Pts',(0.0141142673348248,-0.0330306422053993,
0.0737901733552893));
#84502=CARTESIAN_POINT('Ctrl Pts',(0.0141042719145513,-0.0328657862001531,
0.0736665305678915));
#84503=CARTESIAN_POINT('',(0.014118626414131,-0.0331781648281946,0.0739013179507237));
#84504=CARTESIAN_POINT('',(0.0141191439277825,-0.0331951640388588,0.0739141236120217));
#84505=CARTESIAN_POINT('Origin',(-0.00234461068657464,-0.0326412092868086,
0.0752971355224949));
#84506=CARTESIAN_POINT('Ctrl Pts',(0.0141186264131232,-0.033178164828644,
0.0739013179522645));
#84507=CARTESIAN_POINT('Ctrl Pts',(0.0140756803467012,-0.0331276811561049,
0.0739030994812001));
#84508=CARTESIAN_POINT('Ctrl Pts',(0.0140335097546218,-0.0330765663526692,
0.073904848875029));
#84509=CARTESIAN_POINT('Ctrl Pts',(0.0139506832804901,-0.0329730614522121,
0.0739082847334986));
#84510=CARTESIAN_POINT('Ctrl Pts',(0.0139100608577159,-0.0329207133440476,
0.0739099698047962));
#84511=CARTESIAN_POINT('Ctrl Pts',(0.0138701986272946,-0.0328677532371616,
0.0739116233940857));
#84512=CARTESIAN_POINT('',(0.0139971421388481,-0.0331951640388701,0.0740310186880942));
#84513=CARTESIAN_POINT('Origin',(0.00812378219310841,-0.0315241814719618,
0.07415));
#84514=CARTESIAN_POINT('',(0.0141186264125533,-0.0332121607144208,0.0739013179501391));
#84515=CARTESIAN_POINT('',(0.0141180815491561,-0.0331951640388587,0.0738885134227268));
#84516=CARTESIAN_POINT('Origin',(-0.00233492240592973,-0.0326413664721645,
0.0753414329439625));
#84517=CARTESIAN_POINT('Origin',(-0.00240365414503775,-0.0326412095253733,
0.0738738275177619));
#84518=CARTESIAN_POINT('Origin',(-0.00239766618021565,-0.032641366848677,
0.0738288799872682));
#84519=CARTESIAN_POINT('Ctrl Pts',(0.0138746211457535,-0.0337436976235975,
0.0740726932037927));
#84520=CARTESIAN_POINT('Ctrl Pts',(0.0138739258367123,-0.0336723290703325,
0.0740209692866892));
#84521=CARTESIAN_POINT('Ctrl Pts',(0.0138723002899173,-0.033601104548885,
0.0739692662437147));
#84522=CARTESIAN_POINT('Ctrl Pts',(0.0138671102410036,-0.0333736987606857,
0.073804188669293));
#84523=CARTESIAN_POINT('Ctrl Pts',(0.0138524556418306,-0.0331450831799192,
0.0736396809645867));
#84524=CARTESIAN_POINT('Ctrl Pts',(0.0138658285604175,-0.0337436976235975,
0.0738228478707503));
#84525=CARTESIAN_POINT('Ctrl Pts',(0.0138628861045857,-0.0336723290703325,
0.0737712030354918));
#84526=CARTESIAN_POINT('Ctrl Pts',(0.0138590151969688,-0.033601104548885,
0.0737196194806567));
#84527=CARTESIAN_POINT('Ctrl Pts',(0.0138466561557316,-0.0333736987606857,
0.0735549234081949));
#84528=CARTESIAN_POINT('Ctrl Pts',(0.0138248662709494,-0.0331450831799192,
0.0733912079748788));
#84529=CARTESIAN_POINT('Ctrl Pts',(0.0138657406345641,-0.0337436976235975,
0.0738203494174199));
#84530=CARTESIAN_POINT('Ctrl Pts',(0.0138627757072645,-0.0336723290703325,
0.0737687053729798));
#84531=CARTESIAN_POINT('Ctrl Pts',(0.0138588823460393,-0.033601104548885,
0.0737171230130261));
#84532=CARTESIAN_POINT('Ctrl Pts',(0.0138464516148788,-0.0333736987606857,
0.0735524307555839));
#84533=CARTESIAN_POINT('Ctrl Pts',(0.0138245903772406,-0.0331450831799192,
0.0733887232449818));
#84534=CARTESIAN_POINT('',(0.0138636603625101,-0.0336938721132548,0.0737867871141789));
#84535=CARTESIAN_POINT('',(0.0138438915742658,-0.0333679869984219,0.0735512732946507));
#84536=CARTESIAN_POINT('Ctrl Pts',(0.0138636603625113,-0.0336938721132649,
0.0737867871141894));
#84537=CARTESIAN_POINT('Ctrl Pts',(0.0138622425722313,-0.0336629187933933,
0.0737643816770694));
#84538=CARTESIAN_POINT('Ctrl Pts',(0.0138606940425518,-0.0336319952301041,
0.0737419917074741));
#84539=CARTESIAN_POINT('Ctrl Pts',(0.0138590151969695,-0.0336011045488951,
0.0737196194806673));
#84540=CARTESIAN_POINT('Ctrl Pts',(0.013854802398935,-0.0335235892595454,
0.0736634799082639));
#84541=CARTESIAN_POINT('Ctrl Pts',(0.0138497613933903,-0.0334458668673269,
0.073607352314263));
#84542=CARTESIAN_POINT('Ctrl Pts',(0.013843891574694,-0.0333679869984151,
0.0735512732946152));
#84543=CARTESIAN_POINT('Ctrl Pts',(0.0138438876290188,-0.0333679692463168,
0.0735512289972965));
#84544=CARTESIAN_POINT('Ctrl Pts',(0.0138434374948324,-0.0333391895389005,
0.0735512820729176));
#84545=CARTESIAN_POINT('Ctrl Pts',(0.0138431004775288,-0.0333104081085247,
0.0735513250805207));
#84546=CARTESIAN_POINT('Ctrl Pts',(0.0138426550780635,-0.0332532697574909,
0.0735513875024129));
#84547=CARTESIAN_POINT('Ctrl Pts',(0.0138425433603199,-0.0332249167958317,
0.0735514072639117));
#84548=CARTESIAN_POINT('Ctrl Pts',(0.0138425404278977,-0.0331960985500285,
0.0735514145054824));
#84549=CARTESIAN_POINT('Ctrl Pts',(0.0138425404099617,-0.0331956312423641,
0.0735514146199809));
#84550=CARTESIAN_POINT('Ctrl Pts',(0.0138425404215423,-0.0331951640388589,
0.0735514147306191));
#84551=CARTESIAN_POINT('',(0.0138555531447897,-0.0331951640388587,0.073675735561671));
#84552=CARTESIAN_POINT('',(0.013849046783176,-0.0331951640388687,0.0736135751461546));
#84553=CARTESIAN_POINT('',(0.0138701986059499,-0.0335216366567665,0.0739116233951092));
#84554=CARTESIAN_POINT('Origin',(-0.00267570261449968,-0.0326434571523602,
0.0758099958083109));
#84555=CARTESIAN_POINT('',(0.0138688412385516,-0.0336938721132326,0.0739116797021393));
#84556=CARTESIAN_POINT('Origin',(0.0247800263967618,-0.0336938867896239,
0.0734590558084178));
#84557=CARTESIAN_POINT('',(0.0138662508005408,-0.0336938721132537,0.0738492334081691));
#84558=CARTESIAN_POINT('Ctrl Pts',(0.0141237669728231,-0.0335235895815172,
0.074136485441567));
#84559=CARTESIAN_POINT('Ctrl Pts',(0.0141235809183186,-0.0334144449262748,
0.0740538838381913));
#84560=CARTESIAN_POINT('Ctrl Pts',(0.0141216881630988,-0.0333049234473147,
0.0739711911793267));
#84561=CARTESIAN_POINT('Ctrl Pts',(0.0141180815491639,-0.0331951640388587,
0.0738885134227331));
#84562=CARTESIAN_POINT('Ctrl Pts',(0.0140387564905596,-0.0335235895815172,
0.0740615562056717));
#84563=CARTESIAN_POINT('Ctrl Pts',(0.0140375388876008,-0.0334144449262748,
0.0739801249389546));
#84564=CARTESIAN_POINT('Ctrl Pts',(0.0140346375770773,-0.0333049234473147,
0.0738986252723384));
#84565=CARTESIAN_POINT('Ctrl Pts',(0.0140300468288053,-0.0331951640388587,
0.0738171617549326));
#84566=CARTESIAN_POINT('Ctrl Pts',(0.013953746008296,-0.0335235895815172,
0.0739866269697765));
#84567=CARTESIAN_POINT('Ctrl Pts',(0.0139514968568831,-0.0334144449262748,
0.0739063660397179));
#84568=CARTESIAN_POINT('Ctrl Pts',(0.0139475869910557,-0.0333049234473147,
0.0738260593653501));
#84569=CARTESIAN_POINT('Ctrl Pts',(0.0139420121084467,-0.0331951640388587,
0.073745810087132));
#84570=CARTESIAN_POINT('Ctrl Pts',(0.0138687355260324,-0.0335235895815172,
0.0739116977338812));
#84571=CARTESIAN_POINT('Ctrl Pts',(0.0138654548261653,-0.0334144449262748,
0.0738326071404812));
#84572=CARTESIAN_POINT('Ctrl Pts',(0.0138605364050342,-0.0333049234473147,
0.0737534934583618));
#84573=CARTESIAN_POINT('Ctrl Pts',(0.013853977388088,-0.0331951640388587,
0.0736744584193315));
#84574=CARTESIAN_POINT('',(0.0139868173469829,-0.0331951640388687,0.0737821244922089));
#84575=CARTESIAN_POINT('Ctrl Pts',(0.0141186264094187,-0.0332121607145943,
0.0739013179502668));
#84576=CARTESIAN_POINT('Ctrl Pts',(0.0140757525876135,-0.0332625444108878,
0.0739030964701918));
#84577=CARTESIAN_POINT('Ctrl Pts',(0.0140336175490379,-0.0333135300745024,
0.0739048443434276));
#84578=CARTESIAN_POINT('Ctrl Pts',(0.0139507915918182,-0.033416720314055,
0.0739082801839715));
#84579=CARTESIAN_POINT('Ctrl Pts',(0.013910132752562,-0.033468884758723,
0.0739099668205414));
#84580=CARTESIAN_POINT('Ctrl Pts',(0.0138701986052339,-0.0335216366562289,
0.0739116233949667));
#84581=CARTESIAN_POINT('Ctrl Pts',(0.0138622873042957,-0.033693872113259,
0.0737882790186871));
#84582=CARTESIAN_POINT('Ctrl Pts',(0.0138601700313599,-0.0336474569765058,
0.0737546896440262));
#84583=CARTESIAN_POINT('Ctrl Pts',(0.0138576596974606,-0.033601104548885,
0.0737211273562836));
#84584=CARTESIAN_POINT('Ctrl Pts',(0.0138513041091911,-0.0334837508592655,
0.0736361553601917));
#84585=CARTESIAN_POINT('Ctrl Pts',(0.0138424334154072,-0.0333660264659096,
0.0735514090067958));
#84586=CARTESIAN_POINT('Ctrl Pts',(0.0138636603625123,-0.033693872113259,
0.0737867871142139));
#84587=CARTESIAN_POINT('Ctrl Pts',(0.0138615343569645,-0.0336474569765058,
0.0737531897025877));
#84588=CARTESIAN_POINT('Ctrl Pts',(0.0138590151969688,-0.033601104548885,
0.0737196194806567));
#84589=CARTESIAN_POINT('Ctrl Pts',(0.0138526372630524,-0.0334837508592655,
0.0736346273970239));
#84590=CARTESIAN_POINT('Ctrl Pts',(0.0138437436381987,-0.0333660264659096,
0.0735498616270559));
#84591=CARTESIAN_POINT('Ctrl Pts',(0.0140938757037212,-0.033693872113259,
0.0735366452824997));
#84592=CARTESIAN_POINT('Ctrl Pts',(0.0140902855350262,-0.0336474569765058,
0.0735017003440875));
#84593=CARTESIAN_POINT('Ctrl Pts',(0.0140862865377063,-0.033601104548885,
0.0734667998275823));
#84594=CARTESIAN_POINT('Ctrl Pts',(0.0140761619959217,-0.0334837508592655,
0.0733784397439421));
#84595=CARTESIAN_POINT('Ctrl Pts',(0.0140634236076107,-0.0333660264659096,
0.0732904184727033));
#84596=CARTESIAN_POINT('',(0.014091182083648,-0.0336769361243753,0.0735253892841232));
#84597=CARTESIAN_POINT('',(0.0140925026499634,-0.0336938721132327,0.0735381371821062));
#84598=CARTESIAN_POINT('Ctrl Pts',(0.014091182083648,-0.033676936124375,
0.0735253892841229));
#84599=CARTESIAN_POINT('Ctrl Pts',(0.0140914044638328,-0.0336797586669926,
0.0735275138578085));
#84600=CARTESIAN_POINT('Ctrl Pts',(0.0140916257009893,-0.0336825812712647,
0.0735296384699023));
#84601=CARTESIAN_POINT('Ctrl Pts',(0.0140920658892346,-0.0336882265963423,
0.0735338877658103));
#84602=CARTESIAN_POINT('Ctrl Pts',(0.0140922848403331,-0.0336910493171086,
0.0735360124495905));
#84603=CARTESIAN_POINT('Ctrl Pts',(0.0140925026499678,-0.0336938721132347,
0.0735381371821031));
#84604=CARTESIAN_POINT('Ctrl Pts',(0.014091182083648,-0.0336769361243753,
0.0735253892841232));
#84605=CARTESIAN_POINT('Ctrl Pts',(0.014049494974309,-0.0336278994733738,
0.0735297526946009));
#84606=CARTESIAN_POINT('Ctrl Pts',(0.0140072143570136,-0.0335767852771506,
0.0735341782278523));
#84607=CARTESIAN_POINT('Ctrl Pts',(0.0139243583391074,-0.0334733172093594,
0.0735428508084751));
#84608=CARTESIAN_POINT('Ctrl Pts',(0.0138837335575755,-0.0334209631470897,
0.0735471030245721));
#84609=CARTESIAN_POINT('Ctrl Pts',(0.0138438915753067,-0.033367986984468,
0.0735512733046812));
#84610=CARTESIAN_POINT('',(0.0139780815062468,-0.0336938721132538,0.0736624621481526));
#84611=CARTESIAN_POINT('Origin',(0.00812378219310841,-0.0315241814719618,
0.07415));
#84612=CARTESIAN_POINT('',(0.014091182082366,-0.0337108120655667,0.073525389284263));
#84613=CARTESIAN_POINT('',(0.0140898342906075,-0.0336938721132327,0.0735126442359757));
#84614=CARTESIAN_POINT('Origin',(-0.00229747738884879,-0.0345562524843932,
0.0741170865180477));
#84615=CARTESIAN_POINT('Ctrl Pts',(0.0140898342906212,-0.0336938721132382,
0.0735126442359816));
#84616=CARTESIAN_POINT('Ctrl Pts',(0.0140900611768464,-0.0336910492963934,
0.0735147680342053));
#84617=CARTESIAN_POINT('Ctrl Pts',(0.0140902869337414,-0.0336882265859841,
0.073516891997733));
#84618=CARTESIAN_POINT('Ctrl Pts',(0.014090736197069,-0.0336825812712925,
0.0735211403358452));
#84619=CARTESIAN_POINT('Ctrl Pts',(0.0140909597034621,-0.0336797586670065,
0.0735232647104274));
#84620=CARTESIAN_POINT('Ctrl Pts',(0.014091182083648,-0.033676936124375,
0.0735253892841235));
#84621=CARTESIAN_POINT('Origin',(-0.00206478689373644,-0.0345562520240462,
0.0763401538921394));
#84622=CARTESIAN_POINT('Ctrl Pts',(0.0138584229793833,-0.034243627687391,
0.0737117990730362));
#84623=CARTESIAN_POINT('Ctrl Pts',(0.0138418959589715,-0.033943005420181,
0.0734955135302695));
#84624=CARTESIAN_POINT('Ctrl Pts',(0.0138091243768085,-0.0336441434784052,
0.0732810873149503));
#84625=CARTESIAN_POINT('Ctrl Pts',(0.013833962059755,-0.034243627687391,
0.0734629986240596));
#84626=CARTESIAN_POINT('Ctrl Pts',(0.0138080513757184,-0.033943005420181,
0.0732476356400853));
#84627=CARTESIAN_POINT('Ctrl Pts',(0.0137659922788434,-0.0336441434784052,
0.0730348361786582));
#84628=CARTESIAN_POINT('Ctrl Pts',(0.0138337174505587,-0.034243627687391,
0.0734605106195699));
#84629=CARTESIAN_POINT('Ctrl Pts',(0.0138077129298858,-0.033943005420181,
0.0732451568611834));
#84630=CARTESIAN_POINT('Ctrl Pts',(0.0137655609578638,-0.0336441434784052,
0.0730323736672953));
#84631=CARTESIAN_POINT('',(0.0138295276982948,-0.0341934961088741,0.0734270938995651));
#84632=CARTESIAN_POINT('',(0.0137950098862559,-0.0338664212872184,0.0731932861130012));
#84633=CARTESIAN_POINT('Origin',(-0.00282889432060436,-0.0345610751539435,
0.0750239983549795));
#84634=CARTESIAN_POINT('Origin',(0.0246084682439468,-0.0336938005063909,
0.0713690468206104));
#84635=CARTESIAN_POINT('',(0.0138144634936381,-0.0336938721132327,0.0733167705383256));
#84636=CARTESIAN_POINT('',(0.0138040668860578,-0.0336938721132427,0.0732551413200166));
#84637=CARTESIAN_POINT('',(0.0138438915753073,-0.0340203938281605,0.0735512733046865));
#84638=CARTESIAN_POINT('Origin',(-0.00280041993298706,-0.0345589643241736,
0.074543663310025));
#84639=CARTESIAN_POINT('',(0.0138425404215422,-0.034193496108874,0.0735514147306181));
#84640=CARTESIAN_POINT('Origin',(0.0248021152592256,-0.0341934220717659,
0.0724042714765647));
#84641=CARTESIAN_POINT('',(0.0138360340599285,-0.034193496108884,0.0734892543151016));
#84642=CARTESIAN_POINT('Ctrl Pts',(0.0141110789652396,-0.0340223579322397,
0.0737597726783989));
#84643=CARTESIAN_POINT('Ctrl Pts',(0.0141056967127191,-0.0339125849573575,
0.0736771922403857));
#84644=CARTESIAN_POINT('Ctrl Pts',(0.0140986090190687,-0.0338030433565231,
0.0735947812308107));
#84645=CARTESIAN_POINT('Ctrl Pts',(0.0140898342906155,-0.0336938721132327,
0.0735126442359814));
#84646=CARTESIAN_POINT('Ctrl Pts',(0.0140215313921552,-0.0340223579322397,
0.0736903290898859));
#84647=CARTESIAN_POINT('Ctrl Pts',(0.0140151913314326,-0.0339125849573575,
0.0736089837464554));
#84648=CARTESIAN_POINT('Ctrl Pts',(0.0140071720662088,-0.0338030433565231,
0.0735278267879805));
#84649=CARTESIAN_POINT('Ctrl Pts',(0.0139974930519707,-0.0336938721132327,
0.0734469610914432));
#84650=CARTESIAN_POINT('Ctrl Pts',(0.0139319838190708,-0.0340223579322397,
0.0736208855013728));
#84651=CARTESIAN_POINT('Ctrl Pts',(0.0139246859501462,-0.0339125849573575,
0.073540775252525));
#84652=CARTESIAN_POINT('Ctrl Pts',(0.0139157351133489,-0.0338030433565231,
0.0734608723451504));
#84653=CARTESIAN_POINT('Ctrl Pts',(0.013905151813326,-0.0336938721132327,
0.073381277946905));
#84654=CARTESIAN_POINT('Ctrl Pts',(0.0138424362459864,-0.0340223579322397,
0.0735514419128598));
#84655=CARTESIAN_POINT('Ctrl Pts',(0.0138341805688597,-0.0339125849573575,
0.0734725667585947));
#84656=CARTESIAN_POINT('Ctrl Pts',(0.013824298160489,-0.0338030433565231,
0.0733939179023202));
#84657=CARTESIAN_POINT('Ctrl Pts',(0.0138128105746813,-0.0336938721132327,
0.0733155948023667));
#84658=CARTESIAN_POINT('',(0.0139521488921328,-0.0336938721132427,0.0734147073871607));
#84659=CARTESIAN_POINT('Ctrl Pts',(0.0140911820787772,-0.0337108120662658,
0.0735253892846331));
#84660=CARTESIAN_POINT('Ctrl Pts',(0.0140484164527642,-0.0337611408993402,
0.0735298655839877));
#84661=CARTESIAN_POINT('Ctrl Pts',(0.0140064312045429,-0.033812108877951,
0.0735342602008106));
#84662=CARTESIAN_POINT('Ctrl Pts',(0.0139239832155212,-0.0339153382773235,
0.073542890072847));
#84663=CARTESIAN_POINT('Ctrl Pts',(0.0138835553554806,-0.0339675558473112,
0.073547121677074));
#84664=CARTESIAN_POINT('Ctrl Pts',(0.0138438915752671,-0.0340203938281304,
0.0735512733046854));
#84665=CARTESIAN_POINT('Ctrl Pts',(0.0138282506681329,-0.0341934961088741,
0.0734286695178605));
#84666=CARTESIAN_POINT('Ctrl Pts',(0.0138133377287219,-0.0340287516186244,
0.0733107341264604));
#84667=CARTESIAN_POINT('Ctrl Pts',(0.0137935631729445,-0.0338644633283559,
0.0731935158716945));
#84668=CARTESIAN_POINT('Ctrl Pts',(0.0138295276982948,-0.0341934961088741,
0.0734270938995652));
#84669=CARTESIAN_POINT('Ctrl Pts',(0.0138145821842169,-0.0340287516186244,
0.0733091321065726));
#84670=CARTESIAN_POINT('Ctrl Pts',(0.0137947739904092,-0.0338644633283559,
0.0731918888191096));
#84671=CARTESIAN_POINT('Ctrl Pts',(0.0140423055593536,-0.0341934961088741,
0.073164565495195));
#84672=CARTESIAN_POINT('Ctrl Pts',(0.014021932477351,-0.0340287516186244,
0.0730422046875642));
#84673=CARTESIAN_POINT('Ctrl Pts',(0.0139965195387595,-0.0338644633283559,
0.0729207904698361));
#84674=CARTESIAN_POINT('',(0.0140401871511133,-0.0341764758832433,0.07315192567229));
#84675=CARTESIAN_POINT('',(0.0140423055593501,-0.034193496108874,0.0731645654951994));
#84676=CARTESIAN_POINT('Origin',(-0.00237205740712093,-0.0345621027371333,
0.0754012723049952));
#84677=CARTESIAN_POINT('Ctrl Pts',(0.0140401871505218,-0.0341764758837539,
0.0731519256740081));
#84678=CARTESIAN_POINT('Ctrl Pts',(0.0139978608193925,-0.0341260050041454,
0.0731590659741078));
#84679=CARTESIAN_POINT('Ctrl Pts',(0.0139562702261054,-0.0340749269150179,
0.0731660821966222));
#84680=CARTESIAN_POINT('Ctrl Pts',(0.0138745282515552,-0.0339715436310111,
0.07317987174326));
#84681=CARTESIAN_POINT('Ctrl Pts',(0.0138344078804317,-0.0339192778242667,
0.073186639830027));
#84682=CARTESIAN_POINT('Ctrl Pts',(0.0137950098878868,-0.0338664212862372,
0.073193286114866));
#84683=CARTESIAN_POINT('',(0.0139359166288325,-0.0341934961088841,0.0732958296973923));
#84684=CARTESIAN_POINT('Origin',(0.00812378219310841,-0.0315241814719618,
0.07415));
#84685=CARTESIAN_POINT('',(0.0140401871502457,-0.0342105180190355,0.0731519256715834));
#84686=CARTESIAN_POINT('',(0.0140380417500601,-0.0341934961088739,0.0731392904012451));
#84687=CARTESIAN_POINT('Origin',(-0.00236972593437885,-0.0345621716939992,
0.0754465379162919));
#84688=CARTESIAN_POINT('Origin',(-0.00220168714295083,-0.0345621031391709,
0.0764112014501524));
#84689=CARTESIAN_POINT('Origin',(-0.00221433234995836,-0.0345621722388305,
0.0763676759181593));
#84690=CARTESIAN_POINT('Ctrl Pts',(0.0138147130138689,-0.0346945769586965,
0.0733182496493391));
#84691=CARTESIAN_POINT('Ctrl Pts',(0.0137972916697596,-0.0345275153362944,
0.0731990508247738));
#84692=CARTESIAN_POINT('Ctrl Pts',(0.0137761171262808,-0.0343603235965186,
0.0730803690545241));
#84693=CARTESIAN_POINT('Ctrl Pts',(0.0137512572252257,-0.034193496108874,
0.0729625544158142));
#84694=CARTESIAN_POINT('Ctrl Pts',(0.0138007676969557,-0.0346945769586965,
0.0732355843209515));
#84695=CARTESIAN_POINT('Ctrl Pts',(0.013781614894446,-0.0345275153362944,
0.0731166775866324));
#84696=CARTESIAN_POINT('Ctrl Pts',(0.0137587176306923,-0.0343603235965186,
0.0729983424349513));
#84697=CARTESIAN_POINT('Ctrl Pts',(0.0137321488272934,-0.034193496108874,
0.0728809278422631));
#84698=CARTESIAN_POINT('Ctrl Pts',(0.0137868223800424,-0.0346945769586965,
0.0731529189925634));
#84699=CARTESIAN_POINT('Ctrl Pts',(0.0137659381191324,-0.0345275153362944,
0.0730343043484912));
#84700=CARTESIAN_POINT('Ctrl Pts',(0.0137413181351039,-0.0343603235965186,
0.0729163158153789));
#84701=CARTESIAN_POINT('Ctrl Pts',(0.0137130404293612,-0.034193496108874,
0.0727993012687119));
#84702=CARTESIAN_POINT('Ctrl Pts',(0.0137728770631294,-0.0346945769586965,
0.0730702536641762));
#84703=CARTESIAN_POINT('Ctrl Pts',(0.0137502613438188,-0.0345275153362944,
0.0729519311103494));
#84704=CARTESIAN_POINT('Ctrl Pts',(0.0137239186395152,-0.0343603235965186,
0.0728342891958057));
#84705=CARTESIAN_POINT('Ctrl Pts',(0.0136939320314287,-0.034193496108874,
0.0727176746951608));
#84706=CARTESIAN_POINT('',(0.0137728770632756,-0.0346945769586966,0.0730702536650438));
#84707=CARTESIAN_POINT('',(0.0137237464515596,-0.034366772783284,0.0728390746379946));
#84708=CARTESIAN_POINT('Origin',(-0.0027064394453972,-0.0345626461567451,
0.0764063253273736));
#84709=CARTESIAN_POINT('Origin',(0.0244849948321285,-0.0341934771027848,
0.0703199103678021));
#84710=CARTESIAN_POINT('',(0.0137509153232184,-0.034193496108874,0.072961093890999));
#84711=CARTESIAN_POINT('',(0.0137366695003317,-0.0341934961088841,0.0729002390922665));
#84712=CARTESIAN_POINT('',(0.0137950098858203,-0.0345211942962632,0.0731932861151862));
#84713=CARTESIAN_POINT('Origin',(-0.00278314221978826,-0.0345625596120791,
0.0759316603151603));
#84714=CARTESIAN_POINT('',(0.0137936702784574,-0.0346945769586885,0.0731935121016875));
#84715=CARTESIAN_POINT('Origin',(0.0247030942457456,-0.0346945685853855,
0.0713531360797733));
#84716=CARTESIAN_POINT('',(0.0137832736708765,-0.0346945769587026,0.0731318828833757));
#84717=CARTESIAN_POINT('Ctrl Pts',(0.0140747617037272,-0.0345231616327842,
0.0733845962736656));
#84718=CARTESIAN_POINT('Ctrl Pts',(0.014064211690962,-0.0344132092796988,
0.0733025703994207));
#84719=CARTESIAN_POINT('Ctrl Pts',(0.0140519655820212,-0.034303273855898,
0.0732207669760262));
#84720=CARTESIAN_POINT('Ctrl Pts',(0.0140380417500679,-0.0341934961088739,
0.0731392904012499));
#84721=CARTESIAN_POINT('Ctrl Pts',(0.0139810305825693,-0.0345231616327842,
0.0733209125782205));
#84722=CARTESIAN_POINT('Ctrl Pts',(0.0139696027797218,-0.0344132092796988,
0.073240178655518));
#84723=CARTESIAN_POINT('Ctrl Pts',(0.0139565056489873,-0.034303273855898,
0.0731596852734025));
#84724=CARTESIAN_POINT('Ctrl Pts',(0.0139417586107953,-0.0341934961088739,
0.0730795351234002));
#84725=CARTESIAN_POINT('Ctrl Pts',(0.0138872994614113,-0.0345231616327842,
0.0732572288827755));
#84726=CARTESIAN_POINT('Ctrl Pts',(0.0138749938684816,-0.0344132092796988,
0.0731777869116153));
#84727=CARTESIAN_POINT('Ctrl Pts',(0.0138610457159534,-0.034303273855898,
0.0730986035707788));
#84728=CARTESIAN_POINT('Ctrl Pts',(0.0138454754715228,-0.0341934961088739,
0.0730197798455506));
#84729=CARTESIAN_POINT('Ctrl Pts',(0.0137935683402534,-0.0345231616327842,
0.0731935451873305));
#84730=CARTESIAN_POINT('Ctrl Pts',(0.0137803849572414,-0.0344132092796988,
0.0731153951677126));
#84731=CARTESIAN_POINT('Ctrl Pts',(0.0137655857829194,-0.034303273855898,
0.0730375218681551));
#84732=CARTESIAN_POINT('Ctrl Pts',(0.0137491923322503,-0.0341934961088739,
0.072960024567701));
#84733=CARTESIAN_POINT('',(0.0138944785366492,-0.0341934961088839,0.073050192146132));
#84734=CARTESIAN_POINT('Ctrl Pts',(0.0140401871468337,-0.034210518019536,
0.0731519256721527));
#84735=CARTESIAN_POINT('Ctrl Pts',(0.0139978132303992,-0.0342610556240281,
0.0731590739857814));
#84736=CARTESIAN_POINT('Ctrl Pts',(0.0139561996919832,-0.0343122189868071,
0.0731660940266185));
#84737=CARTESIAN_POINT('Ctrl Pts',(0.0138744568932699,-0.0344158119695103,
0.0731798837163913));
#84738=CARTESIAN_POINT('Ctrl Pts',(0.0138343610666141,-0.0344681990449984,
0.0731866477252027));
#84739=CARTESIAN_POINT('Ctrl Pts',(0.0137950098857875,-0.0345211942962394,
0.0731932861151812));
#84740=CARTESIAN_POINT('Ctrl Pts',(0.0137717017744239,-0.0346945769586932,
0.0730719059554424));
#84741=CARTESIAN_POINT('Ctrl Pts',(0.013749412942895,-0.0345296777077528,
0.0729551392144772));
#84742=CARTESIAN_POINT('Ctrl Pts',(0.0137223170801922,-0.0343648066252516,
0.0728393934671215));
#84743=CARTESIAN_POINT('Ctrl Pts',(0.0137728770632773,-0.0346945769586932,
0.0730702536650528));
#84744=CARTESIAN_POINT('Ctrl Pts',(0.0137505540718136,-0.0345296777077528,
0.0729534626258222));
#84745=CARTESIAN_POINT('Ctrl Pts',(0.0137234230740957,-0.0343648066252516,
0.0728376940128251));
#84746=CARTESIAN_POINT('Ctrl Pts',(0.0139687507609298,-0.0346945769586932,
0.0727948828680803));
#84747=CARTESIAN_POINT('Ctrl Pts',(0.0139407346730868,-0.0345296777077528,
0.0726740422787478));
#84748=CARTESIAN_POINT('Ctrl Pts',(0.0139077480720424,-0.0343648066252516,
0.0725544628768436));
#84749=CARTESIAN_POINT('',(0.0139658428720393,-0.0346775396665016,0.0727824010027757));
#84750=CARTESIAN_POINT('',(0.0139687507609263,-0.0346945769586886,0.0727948828680809));
#84751=CARTESIAN_POINT('Origin',(-0.00216324988500243,-0.0345626618546312,
0.0767149915967936));
#84752=CARTESIAN_POINT('Ctrl Pts',(0.0139658428714545,-0.0346775396670097,
0.0727824010045));
#84753=CARTESIAN_POINT('Ctrl Pts',(0.013924015487737,-0.0346269749928339,
0.0727921926120357));
#84754=CARTESIAN_POINT('Ctrl Pts',(0.0138829314781485,-0.03457579028911,
0.0728018102358312));
#84755=CARTESIAN_POINT('Ctrl Pts',(0.0138022163328588,-0.0344721681088797,
0.0728207052688002));
#84756=CARTESIAN_POINT('Ctrl Pts',(0.0137626168400041,-0.0344197714290866,
0.0728299752647442));
#84757=CARTESIAN_POINT('Ctrl Pts',(0.0137237464517877,-0.0343667727831654,
0.0728390746382783));
#84758=CARTESIAN_POINT('',(0.013870813912111,-0.0346945769587026,0.0729325682665724));
#84759=CARTESIAN_POINT('Origin',(0.00812378219310841,-0.0315241814719618,
0.07415));
#84760=CARTESIAN_POINT('',(0.0139658428707218,-0.0347116136489602,0.0727824010023258));
#84761=CARTESIAN_POINT('',(0.0139629083290095,-0.0346945769586885,0.0727699253755514));
#84762=CARTESIAN_POINT('Origin',(-0.00215110916414497,-0.034562669838981,
0.0767586463341342));
#84763=CARTESIAN_POINT('Origin',(-0.0022328693252026,-0.0345626621621979,
0.0764175983069814));
#84764=CARTESIAN_POINT('Origin',(-0.00224136492537223,-0.0345626702062483,
0.0763730903455221));
#84765=CARTESIAN_POINT('Ctrl Pts',(0.0137588268289809,-0.0352450361874068,
0.0729988985373347));
#84766=CARTESIAN_POINT('Ctrl Pts',(0.0137154123249175,-0.0349452760959493,
0.0727863693414509));
#84767=CARTESIAN_POINT('Ctrl Pts',(0.0136561125882577,-0.034644428984174,
0.072577714076724));
#84768=CARTESIAN_POINT('Ctrl Pts',(0.0137582667402476,-0.0352450361874068,
0.0729964364395278));
#84769=CARTESIAN_POINT('Ctrl Pts',(0.0137147593766418,-0.0349452760959493,
0.0727839283677371));
#84770=CARTESIAN_POINT('Ctrl Pts',(0.0136553686353968,-0.034644428984174,
0.0725753011616529));
#84771=CARTESIAN_POINT('Ctrl Pts',(0.0137028124102251,-0.0352450361874068,
0.0727526643794353));
#84772=CARTESIAN_POINT('Ctrl Pts',(0.0136501110325061,-0.0349452760959493,
0.0725422478020213));
#84773=CARTESIAN_POINT('Ctrl Pts',(0.0135817099362883,-0.034644428984174,
0.0723363986793601));
#84774=CARTESIAN_POINT('Ctrl Pts',(0.0137022578669249,-0.0352450361874068,
0.0727502266588344));
#84775=CARTESIAN_POINT('Ctrl Pts',(0.0136494645490647,-0.0349452760959493,
0.0725398309963641));
#84776=CARTESIAN_POINT('Ctrl Pts',(0.0135809733492973,-0.034644428984174,
0.0723340096545372));
#84777=CARTESIAN_POINT('',(0.0136939423889737,-0.0351951634053355,0.0727177054440917));
#84778=CARTESIAN_POINT('',(0.013630382516768,-0.0348678972925434,0.0724900367849038));
#84779=CARTESIAN_POINT('Origin',(-0.00228417407676976,-0.0345636767881962,
0.0777281236473546));
#84780=CARTESIAN_POINT('Origin',(0.0242099803342668,-0.0346946199340747,
0.0693008206829229));
#84781=CARTESIAN_POINT('',(0.013665159433795,-0.0346945769330288,0.0726101093303203));
#84782=CARTESIAN_POINT('',(0.0136471206151762,-0.0346945769458128,0.0725502691088101));
#84783=CARTESIAN_POINT('',(0.0137237464515733,-0.0350221583435275,0.0728390746383119));
#84784=CARTESIAN_POINT('Origin',(-0.00246213657583445,-0.0345628458712538,
0.0772814999335259));
#84785=CARTESIAN_POINT('',(0.0137225428151149,-0.0351951360298762,0.0728393595102533));
#84786=CARTESIAN_POINT('Origin',(0.0244514640108223,-0.0351951838366837,
0.0703277676145716));
#84787=CARTESIAN_POINT('',(0.0136939320317448,-0.0351951371328747,0.0727176746960014));
#84788=CARTESIAN_POINT('Ctrl Pts',(0.0140149585252636,-0.0350241211494342,
0.07301244058461));
#84789=CARTESIAN_POINT('Ctrl Pts',(0.0139992891107342,-0.0349144232818962,
0.0729312920461109));
#84790=CARTESIAN_POINT('Ctrl Pts',(0.0139819329190284,-0.0348045283579412,
0.0728504188342951));
#84791=CARTESIAN_POINT('Ctrl Pts',(0.0139629083264611,-0.0346945769439157,
0.0727699253647406));
#84792=CARTESIAN_POINT('Ctrl Pts',(0.0139174135979912,-0.0350241211494342,
0.072954767983083));
#84793=CARTESIAN_POINT('Ctrl Pts',(0.0139009497670223,-0.0349144232818962,
0.0728749630859621));
#84794=CARTESIAN_POINT('Ctrl Pts',(0.0138828264574081,-0.0348045283579412,
0.0727954507409142));
#84795=CARTESIAN_POINT('Ctrl Pts',(0.0138630630929085,-0.0346945769439157,
0.0727163336569837));
#84796=CARTESIAN_POINT('Ctrl Pts',(0.0138198686707187,-0.0350241211494342,
0.0728970953815561));
#84797=CARTESIAN_POINT('Ctrl Pts',(0.0138026104233105,-0.0349144232818962,
0.0728186341258134));
#84798=CARTESIAN_POINT('Ctrl Pts',(0.0137837199957878,-0.0348045283579412,
0.0727404826475332));
#84799=CARTESIAN_POINT('Ctrl Pts',(0.0137632178593558,-0.0346945769439157,
0.0726627419492268));
#84800=CARTESIAN_POINT('Ctrl Pts',(0.0137223237434462,-0.0350241211494342,
0.0728394227800291));
#84801=CARTESIAN_POINT('Ctrl Pts',(0.0137042710795987,-0.0349144232818962,
0.0727623051656646));
#84802=CARTESIAN_POINT('Ctrl Pts',(0.0136846135341675,-0.0348045283579412,
0.0726855145541522));
#84803=CARTESIAN_POINT('Ctrl Pts',(0.0136633726258032,-0.0346945769439157,
0.07260915024147));
#84804=CARTESIAN_POINT('',(0.0138140338815658,-0.0346945769458128,0.0726900173532006));
#84805=CARTESIAN_POINT('Ctrl Pts',(0.0139658428675145,-0.0347116136492769,
0.0727824010030701));
#84806=CARTESIAN_POINT('Ctrl Pts',(0.0139240320915038,-0.0347621546531278,
0.0727921887095867));
#84807=CARTESIAN_POINT('Ctrl Pts',(0.0138829564619176,-0.0348133084094943,
0.0728018043217741));
#84808=CARTESIAN_POINT('Ctrl Pts',(0.0138022412148688,-0.0349168561544567,
0.0728206993824475));
#84809=CARTESIAN_POINT('Ctrl Pts',(0.0137626336132877,-0.0349692089015918,
0.0728299713361659));
#84810=CARTESIAN_POINT('Ctrl Pts',(0.0137237464515331,-0.0350221583434999,
0.0728390746383007));
#84811=CARTESIAN_POINT('Ctrl Pts',(0.0136931605528093,-0.0351951371254986,
0.0727189177728991));
#84812=CARTESIAN_POINT('Ctrl Pts',(0.0136635738256549,-0.035030733898099,
0.0726037743696569));
#84813=CARTESIAN_POINT('Ctrl Pts',(0.0136292533790862,-0.034865930689785,
0.0724899522071348));
#84814=CARTESIAN_POINT('Ctrl Pts',(0.0136939320316345,-0.0351951371254986,
0.0727176746960388));
#84815=CARTESIAN_POINT('Ctrl Pts',(0.013664319604646,-0.035030733898099,
0.0726025153429559));
#84816=CARTESIAN_POINT('Ctrl Pts',(0.0136299728209793,-0.034865930689785,
0.0724886783064241));
#84817=CARTESIAN_POINT('Ctrl Pts',(0.0138232326868359,-0.0351951371254986,
0.0725093337186266));
#84818=CARTESIAN_POINT('Ctrl Pts',(0.0137893129408568,-0.035030733898099,
0.0723915011556234));
#84819=CARTESIAN_POINT('Ctrl Pts',(0.013750552032128,-0.034865930689785,
0.0722751712195549));
#84820=CARTESIAN_POINT('Origin',(0.0187222405616067,-0.0308609197384197,
0.0709550975151248));
#84821=CARTESIAN_POINT('',(0.0137503042019611,-0.0351951371254986,0.07262684272735));
#84822=CARTESIAN_POINT('Origin',(0.00723898649331173,-0.03518404674411,
0.0745645868065024));
#84823=CARTESIAN_POINT('Origin',(0.0193252105781808,-0.0352322614052578,
0.0699433117626999));
#84824=CARTESIAN_POINT('',(0.0135574056441349,-0.0351951142564681,0.0722649135892815));
#84825=CARTESIAN_POINT('',(0.0135140129935295,-0.0351951372916787,0.0721480229975867));
#84826=CARTESIAN_POINT('Origin',(0.00785544741042606,-0.0352875120570874,
0.0739402521274073));
#84827=CARTESIAN_POINT('Origin',(0.00934108973055431,-0.0298325076522736,
0.0815536040304091));
#84828=CARTESIAN_POINT('Origin',(0.0165013373209963,-0.0338732939252014,
0.0744038860642835));
#84829=CARTESIAN_POINT('Ctrl Pts',(0.0136276248563989,-0.0321934096636942,
0.0758190870807282));
#84830=CARTESIAN_POINT('Ctrl Pts',(0.0136575007202879,-0.0320508460845519,
0.0757205709181067));
#84831=CARTESIAN_POINT('Ctrl Pts',(0.0136847071227777,-0.0319086045665452,
0.0756213263314847));
#84832=CARTESIAN_POINT('Ctrl Pts',(0.0137092030760702,-0.0317669892871456,
0.0755215718345981));
#84833=CARTESIAN_POINT('Ctrl Pts',(0.013650207803114,-0.0321934096636942,
0.0757383378197694));
#84834=CARTESIAN_POINT('Ctrl Pts',(0.0136786382936863,-0.0320508460845519,
0.0756394174331563));
#84835=CARTESIAN_POINT('Ctrl Pts',(0.0137043895519749,-0.0319086045665452,
0.0755398077616578));
#84836=CARTESIAN_POINT('Ctrl Pts',(0.0137274237880785,-0.0317669892871456,
0.0754397278471591));
#84837=CARTESIAN_POINT('Ctrl Pts',(0.0136727907498291,-0.0321934096636942,
0.0756575885588107));
#84838=CARTESIAN_POINT('Ctrl Pts',(0.0136997758670848,-0.0320508460845519,
0.0755582639482058));
#84839=CARTESIAN_POINT('Ctrl Pts',(0.0137240719811719,-0.0319086045665452,
0.075458289191831));
#84840=CARTESIAN_POINT('Ctrl Pts',(0.0137456445000869,-0.0317669892871456,
0.07535788385972));
#84841=CARTESIAN_POINT('Ctrl Pts',(0.0136953736965441,-0.0321934096636942,
0.075576839297852));
#84842=CARTESIAN_POINT('Ctrl Pts',(0.0137209134404833,-0.0320508460845519,
0.0754771104632554));
#84843=CARTESIAN_POINT('Ctrl Pts',(0.013743754410369,-0.0319086045665452,
0.0753767706220041));
#84844=CARTESIAN_POINT('Ctrl Pts',(0.0137638652120951,-0.0317669892871456,
0.075276039872281));
#84845=CARTESIAN_POINT('',(0.0136949696831625,-0.0321934096636942,0.0755782839180869));
#84846=CARTESIAN_POINT('',(0.0137489462178941,-0.0318665617511353,0.0753481880835307));
#84847=CARTESIAN_POINT('Origin',(-0.00232770420397269,-0.032637194442055,
0.0708357290845033));
#84848=CARTESIAN_POINT('Origin',(0.0244696249328875,-0.0316939261509185,
0.0776317462801823));
#84849=CARTESIAN_POINT('',(0.0136626376743362,-0.0320197221621788,0.0756987637407324));
#84850=CARTESIAN_POINT('Ctrl Pts',(0.0136627312772773,-0.0320197392094702,
0.0756986041996119));
#84851=CARTESIAN_POINT('Ctrl Pts',(0.0136706110281021,-0.0319792716576,
0.0756704202333062));
#84852=CARTESIAN_POINT('Ctrl Pts',(0.013678311787336,-0.0319386439829698,
0.0756420478908117));
#84853=CARTESIAN_POINT('Ctrl Pts',(0.013685833477104,-0.031897909938163,
0.0756134551711632));
#84854=CARTESIAN_POINT('Ctrl Pts',(0.0136933550182004,-0.0318571766984942,
0.0755848630166707));
#84855=CARTESIAN_POINT('Ctrl Pts',(0.0137006609905895,-0.03181638718336,
0.0755561962710094));
#84856=CARTESIAN_POINT('Ctrl Pts',(0.0137077296768219,-0.0317755399638303,
0.0755275544055704));
#84857=CARTESIAN_POINT('',(0.013661303056921,-0.0321934096636183,0.0756986648064836));
#84858=CARTESIAN_POINT('Origin',(0.0158306274447591,-0.0324028746691825,
0.0762840964422932));
#84859=CARTESIAN_POINT('',(0.0136781363700518,-0.0321934096636663,0.0756384743622952));
#84860=CARTESIAN_POINT('Ctrl Pts',(0.0136932022405579,-0.0321934096636618,
0.0755792788221118));
#84861=CARTESIAN_POINT('Ctrl Pts',(0.0137129131094296,-0.0320835708272592,
0.0755024721791053));
#84862=CARTESIAN_POINT('Ctrl Pts',(0.0137310230357111,-0.0319739230346488,
0.0754253021716664));
#84863=CARTESIAN_POINT('Ctrl Pts',(0.0137475164265416,-0.0318646057455573,
0.0753478693117285));
#84864=CARTESIAN_POINT('Ctrl Pts',(0.0137919510558728,-0.0321934096636618,
0.0755236925266851));
#84865=CARTESIAN_POINT('Ctrl Pts',(0.0138108953464091,-0.0320835708272592,
0.0754455240605551));
#84866=CARTESIAN_POINT('Ctrl Pts',(0.0138282109561431,-0.0319739230346488,
0.0753670088842042));
#84867=CARTESIAN_POINT('Ctrl Pts',(0.0138438834405726,-0.0318646057455573,
0.0752882491526201));
#84868=CARTESIAN_POINT('Ctrl Pts',(0.0138906998711876,-0.0321934096636618,
0.0754681062312584));
#84869=CARTESIAN_POINT('Ctrl Pts',(0.0139088775833886,-0.0320835708272592,
0.0753885759420049));
#84870=CARTESIAN_POINT('Ctrl Pts',(0.013925398876575,-0.0319739230346488,
0.075308715596742));
#84871=CARTESIAN_POINT('Ctrl Pts',(0.0139402504546036,-0.0318646057455573,
0.0752286289935117));
#84872=CARTESIAN_POINT('Ctrl Pts',(0.0139894486865025,-0.0321934096636618,
0.0754125199358316));
#84873=CARTESIAN_POINT('Ctrl Pts',(0.0140068598203681,-0.0320835708272592,
0.0753316278234546));
#84874=CARTESIAN_POINT('Ctrl Pts',(0.014022586797007,-0.0319739230346488,
0.0752504223092798));
#84875=CARTESIAN_POINT('Ctrl Pts',(0.0140366174686345,-0.0318646057455573,
0.0751690088344033));
#84876=CARTESIAN_POINT('',(0.0139921320686152,-0.0321763980308501,0.0753999878865454));
#84877=CARTESIAN_POINT('',(0.0139894486864999,-0.0321934096636184,0.075412519935805));
#84878=CARTESIAN_POINT('Origin',(-0.00205353621687885,-0.0326386231150955,
0.0713549143724822));
#84879=CARTESIAN_POINT('Ctrl Pts',(0.0139921320655067,-0.0321763980306344,
0.075399987885879));
#84880=CARTESIAN_POINT('Ctrl Pts',(0.013950154885113,-0.0321259596175737,
0.0753910465364169));
#84881=CARTESIAN_POINT('Ctrl Pts',(0.0139089050138353,-0.0320749164633211,
0.0753822601074425));
#84882=CARTESIAN_POINT('Ctrl Pts',(0.0138278266926965,-0.0319716057794015,
0.075364990019354));
#84883=CARTESIAN_POINT('Ctrl Pts',(0.0137880298338754,-0.0319193786690214,
0.0753565130892893));
#84884=CARTESIAN_POINT('Ctrl Pts',(0.0137489462160759,-0.0318665617525426,
0.075348188083138));
#84885=CARTESIAN_POINT('',(0.0138422091848412,-0.0321934096636663,0.075495401926956));
#84886=CARTESIAN_POINT('Origin',(0.00812378219310841,-0.0315241814719618,
0.07415));
#84887=CARTESIAN_POINT('',(0.0139921320689771,-0.032210423332376,0.0753999878866226));
#84888=CARTESIAN_POINT('',(0.0139947886795379,-0.0321934096636183,0.0753874501348803));
#84889=CARTESIAN_POINT('Origin',(-0.00206906439733519,-0.0326387243756408,
0.0713975045508542));
#84890=CARTESIAN_POINT('Origin',(-0.00230916111180189,-0.0326386236553222,
0.072554997489267));
#84891=CARTESIAN_POINT('Origin',(-0.00230598258356715,-0.0326387247569551,
0.0725097765576227));
#84892=CARTESIAN_POINT('Ctrl Pts',(0.013713169049324,-0.0327445246967096,
0.0755053153033758));
#84893=CARTESIAN_POINT('Ctrl Pts',(0.0137642856016332,-0.032443687833936,
0.0752945081318633));
#84894=CARTESIAN_POINT('Ctrl Pts',(0.0137993780794782,-0.0321434074405927,
0.0750804495336249));
#84895=CARTESIAN_POINT('Ctrl Pts',(0.0137667874877737,-0.0327445246967096,
0.0752611328653132));
#84896=CARTESIAN_POINT('Ctrl Pts',(0.0138086945488767,-0.032443687833936,
0.0750483034413352));
#84897=CARTESIAN_POINT('Ctrl Pts',(0.0138344513743864,-0.0321434074405927,
0.0748329220321544));
#84898=CARTESIAN_POINT('',(0.0137736589065096,-0.0326943950436612,0.0752256477691917));
#84899=CARTESIAN_POINT('',(0.013813081094821,-0.0323666188837389,0.0749926167616255));
#84900=CARTESIAN_POINT('Origin',(-0.00275471203025378,-0.032639557911195,
0.0721562809946593));
#84901=CARTESIAN_POINT('Origin',(0.024738513391894,-0.0321933825603012,
0.0766107332495159));
#84902=CARTESIAN_POINT('',(0.0137934237886414,-0.0321934096532689,0.0751160689287386));
#84903=CARTESIAN_POINT('',(0.0138025805038011,-0.0321934096584275,0.0750542433279473));
#84904=CARTESIAN_POINT('',(0.0137489462188077,-0.0325210109756238,0.0753481880837245));
#84905=CARTESIAN_POINT('Origin',(-0.00263998480464471,-0.03263931291567,
0.0716893526347667));
#84906=CARTESIAN_POINT('',(0.0137476174921984,-0.0326943950436593,0.0753479050583036));
#84907=CARTESIAN_POINT('Origin',(0.0245673437198019,-0.0326943765538141,
0.0776525614440418));
#84908=CARTESIAN_POINT('',(0.013760638199364,-0.0326943950436702,0.0752867764137576));
#84909=CARTESIAN_POINT('Ctrl Pts',(0.0139386268780033,-0.0325229783203769,
0.0756290474267761));
#84910=CARTESIAN_POINT('Ctrl Pts',(0.0139590155144368,-0.032413025309245,
0.0755488899199571));
#84911=CARTESIAN_POINT('Ctrl Pts',(0.0139777428975359,-0.032303122220807,
0.0754683228054589));
#84912=CARTESIAN_POINT('Ctrl Pts',(0.0139947886804688,-0.0321934096576658,
0.0753874501305006));
#84913=CARTESIAN_POINT('Ctrl Pts',(0.013874921404638,-0.0325229783203769,
0.0755353310733458));
#84914=CARTESIAN_POINT('Ctrl Pts',(0.0138940181631889,-0.032413025309245,
0.075456051745084));
#84915=CARTESIAN_POINT('Ctrl Pts',(0.0139114720305956,-0.032303122220807,
0.0753763894001035));
#84916=CARTESIAN_POINT('Ctrl Pts',(0.0139272642504138,-0.0321934096576658,
0.0752964468691155));
#84917=CARTESIAN_POINT('Ctrl Pts',(0.0138112159312727,-0.0325229783203769,
0.0754416147199155));
#84918=CARTESIAN_POINT('Ctrl Pts',(0.013829020811941,-0.032413025309245,
0.0753632135702109));
#84919=CARTESIAN_POINT('Ctrl Pts',(0.0138452011636553,-0.032303122220807,
0.0752844559947481));
#84920=CARTESIAN_POINT('Ctrl Pts',(0.0138597398203589,-0.0321934096576658,
0.0752054436077304));
#84921=CARTESIAN_POINT('Ctrl Pts',(0.0137475104579075,-0.0325229783203769,
0.0753478983664852));
#84922=CARTESIAN_POINT('Ctrl Pts',(0.0137640234606932,-0.032413025309245,
0.0752703753953377));
#84923=CARTESIAN_POINT('Ctrl Pts',(0.0137789302967149,-0.032303122220807,
0.0751925225893928));
#84924=CARTESIAN_POINT('Ctrl Pts',(0.013792215390304,-0.0321934096576658,
0.0751144403463453));
#84925=CARTESIAN_POINT('',(0.0138941062341519,-0.0321934096584275,0.0752517595323228));
#84926=CARTESIAN_POINT('Ctrl Pts',(0.0139921320655695,-0.032210423332889,
0.0753999878858924));
#84927=CARTESIAN_POINT('Ctrl Pts',(0.0139500980054311,-0.0322609421830331,
0.07539103442076));
#84928=CARTESIAN_POINT('Ctrl Pts',(0.0139088203474602,-0.032312088823864,
0.0753822420730741));
#84929=CARTESIAN_POINT('Ctrl Pts',(0.0138277414124259,-0.0324156524631807,
0.0753649718542227));
#84930=CARTESIAN_POINT('Ctrl Pts',(0.0137879734632952,-0.0324680267167304,
0.0753565010820737));
#84931=CARTESIAN_POINT('Ctrl Pts',(0.0137489462187663,-0.0325210109755912,
0.0753481880837111));
#84932=CARTESIAN_POINT('Origin',(0.00556981264422981,-0.0262834582510643,
0.0815918160004898));
#84933=CARTESIAN_POINT('Origin',(0.0176257925203611,-0.0342770795666837,
0.0817351922229394));
#84934=CARTESIAN_POINT('Ctrl Pts',(0.0137719578350082,-0.0326943950436604,
0.0752267514206673));
#84935=CARTESIAN_POINT('Ctrl Pts',(0.0137867974876322,-0.0325844576448133,
0.0751489089745126));
#84936=CARTESIAN_POINT('Ctrl Pts',(0.0138000282810706,-0.0324744968375322,
0.0750707541109808));
#84937=CARTESIAN_POINT('Ctrl Pts',(0.0138116346444435,-0.0323646534831894,
0.0749923872004608));
#84938=CARTESIAN_POINT('Ctrl Pts',(0.0138670213620897,-0.0326943950436604,
0.0751650744119771));
#84939=CARTESIAN_POINT('Ctrl Pts',(0.0138810109899389,-0.0325844576448133,
0.0750859218122511));
#84940=CARTESIAN_POINT('Ctrl Pts',(0.0138933646023211,-0.0324744968375322,
0.0750064742823324));
#84941=CARTESIAN_POINT('Ctrl Pts',(0.0139040677750964,-0.0323646534831894,
0.0749268338333477));
#84942=CARTESIAN_POINT('Ctrl Pts',(0.0139620848891712,-0.0326943950436604,
0.0751033974032868));
#84943=CARTESIAN_POINT('Ctrl Pts',(0.0139752244922456,-0.0325844576448133,
0.0750229346499896));
#84944=CARTESIAN_POINT('Ctrl Pts',(0.0139867009235716,-0.0324744968375322,
0.0749421944536841));
#84945=CARTESIAN_POINT('Ctrl Pts',(0.0139965009057492,-0.0323646534831894,
0.0748612804662345));
#84946=CARTESIAN_POINT('Ctrl Pts',(0.0140571484162527,-0.0326943950436604,
0.0750417203945965));
#84947=CARTESIAN_POINT('Ctrl Pts',(0.0140694379945524,-0.0325844576448133,
0.0749599474877281));
#84948=CARTESIAN_POINT('Ctrl Pts',(0.014080037244822,-0.0324744968375322,
0.0748779146250358));
#84949=CARTESIAN_POINT('Ctrl Pts',(0.014088934036402,-0.0323646534831894,
0.0747957270991214));
#84950=CARTESIAN_POINT('',(0.0140590396096356,-0.03267735599912,0.075029044583551));
#84951=CARTESIAN_POINT('',(0.0140571484162444,-0.0326943950436586,0.0750417203946018));
#84952=CARTESIAN_POINT('Origin',(-0.00237428766991534,-0.0326395662655541,
0.0726459673924195));
#84953=CARTESIAN_POINT('Ctrl Pts',(0.0140590396063146,-0.032677355998748,
0.0750290445830547));
#84954=CARTESIAN_POINT('Ctrl Pts',(0.0140165496609305,-0.0326267922588588,
0.0750227515861847));
#84955=CARTESIAN_POINT('Ctrl Pts',(0.0139748128191324,-0.0325756109584749,
0.0750165701281463));
#84956=CARTESIAN_POINT('Ctrl Pts',(0.0138928098216551,-0.0324719985460571,
0.0750044250288342));
#84957=CARTESIAN_POINT('Ctrl Pts',(0.0138525765557734,-0.0324196091617933,
0.0749984662587221));
#84958=CARTESIAN_POINT('Ctrl Pts',(0.0138130810947728,-0.0323666188837756,
0.0749926167616184));
#84959=CARTESIAN_POINT('',(0.013915403661387,-0.0326943950436699,0.0751336840819068));
#84960=CARTESIAN_POINT('Origin',(0.00812378219310841,-0.0315241814719618,
0.07415));
#84961=CARTESIAN_POINT('',(0.0140590396095908,-0.0327114338379849,0.0750290445835446));
#84962=CARTESIAN_POINT('',(0.0140609037262011,-0.0326943950436593,0.0750163647622643));
#84963=CARTESIAN_POINT('Origin',(-0.00238015612243249,-0.0326395679685205,
0.0726908941291813));
#84964=CARTESIAN_POINT('Origin',(-0.00235956710230526,-0.0326395672643911,
0.0725465692571309));
#84965=CARTESIAN_POINT('Origin',(-0.00235215963958844,-0.0326395684013067,
0.0725018696955815));
#84966=CARTESIAN_POINT('Ctrl Pts',(0.0137872474543938,-0.0332451089994434,
0.0751516417694037));
#84967=CARTESIAN_POINT('Ctrl Pts',(0.0138250249917997,-0.0329451141710255,
0.0749380406823774));
#84968=CARTESIAN_POINT('Ctrl Pts',(0.013846605900126,-0.0326442513127494,
0.0747222008549427));
#84969=CARTESIAN_POINT('Ctrl Pts',(0.0138254260619812,-0.0332451089994434,
0.0749045741796176));
#84970=CARTESIAN_POINT('Ctrl Pts',(0.0138538852927829,-0.0329451141710255,
0.0746895331628477));
#84971=CARTESIAN_POINT('Ctrl Pts',(0.0138660659054358,-0.0326442513127494,
0.0744729593893048));
#84972=CARTESIAN_POINT('Ctrl Pts',(0.0138258078480571,-0.0332451089994434,
0.0749021035037198));
#84973=CARTESIAN_POINT('Ctrl Pts',(0.0138541738957927,-0.0329451141710255,
0.0746870480876524));
#84974=CARTESIAN_POINT('Ctrl Pts',(0.0138662605054889,-0.0326442513127494,
0.0744704669746484));
#84975=CARTESIAN_POINT('',(0.0138300506476655,-0.0331951640388616,0.0748687665299159));
#84976=CARTESIAN_POINT('',(0.0138547629144851,-0.032867753235504,0.0746337200027452));
#84977=CARTESIAN_POINT('Origin',(-0.0028810524814235,-0.0326402808280916,
0.0735378722145668));
#84978=CARTESIAN_POINT('Origin',(0.0248715877881015,-0.0326944278779112,
0.0755632105462519));
#84979=CARTESIAN_POINT('',(0.0138428960169573,-0.0326943950436593,0.0747581628645857));
#84980=CARTESIAN_POINT('',(0.0138481526012722,-0.0326943950436694,0.0746958843103298));
#84981=CARTESIAN_POINT('',(0.0138130810948206,-0.0330220786163545,0.0749926167616284));
#84982=CARTESIAN_POINT('Origin',(-0.00287200908005241,-0.0326396682761396,
0.0730571739081459));
#84983=CARTESIAN_POINT('',(0.0138117372188363,-0.0331951640388589,0.0749924177261293));
#84984=CARTESIAN_POINT('Origin',(0.0247243538844031,-0.033195202656011,
0.0766086377178643));
#84985=CARTESIAN_POINT('',(0.0138208939332609,-0.0331951640388702,0.0749305921280326));
#84986=CARTESIAN_POINT('Ctrl Pts',(0.0140200229445547,-0.0330240426238172,
0.0752610108015162));
#84987=CARTESIAN_POINT('Ctrl Pts',(0.014035328200751,-0.032914277406352,
0.075179784340736));
#84988=CARTESIAN_POINT('Ctrl Pts',(0.0140489619093364,-0.0328043479726691,
0.075098200983204));
#84989=CARTESIAN_POINT('Ctrl Pts',(0.014060903726208,-0.0326943950436594,
0.0750163647622724));
#84990=CARTESIAN_POINT('Ctrl Pts',(0.01395055868344,-0.0330240426238172,
0.0751714795085905));
#84991=CARTESIAN_POINT('Ctrl Pts',(0.0139646305588501,-0.032914277406352,
0.0750912099856829));
#84992=CARTESIAN_POINT('Ctrl Pts',(0.013977050054343,-0.0328043479726691,
0.0750106095405181));
#84993=CARTESIAN_POINT('Ctrl Pts',(0.0139877984159907,-0.0326943950436593,
0.0749297809901024));
#84994=CARTESIAN_POINT('Ctrl Pts',(0.0138810944223254,-0.0330240426238172,
0.0750819482156648));
#84995=CARTESIAN_POINT('Ctrl Pts',(0.0138939329169493,-0.032914277406352,
0.0750026356306298));
#84996=CARTESIAN_POINT('Ctrl Pts',(0.0139051381993496,-0.0328043479726691,
0.0749230180978321));
#84997=CARTESIAN_POINT('Ctrl Pts',(0.0139146931057734,-0.0326943950436593,
0.0748431972179323));
#84998=CARTESIAN_POINT('Ctrl Pts',(0.0138116301612107,-0.0330240426238172,
0.0749924169227391));
#84999=CARTESIAN_POINT('Ctrl Pts',(0.0138232352750485,-0.032914277406352,
0.0749140612755767));
#85000=CARTESIAN_POINT('Ctrl Pts',(0.0138332263443562,-0.0328043479726691,
0.0748354266551462));
#85001=CARTESIAN_POINT('Ctrl Pts',(0.0138415877955562,-0.0326943950436593,
0.0747566134457623));
#85002=CARTESIAN_POINT('',(0.0139518998715892,-0.0326943950436694,0.074887263813435));
#85003=CARTESIAN_POINT('Ctrl Pts',(0.0140590396063062,-0.0327114338383285,
0.0750290445830535));
#85004=CARTESIAN_POINT('Ctrl Pts',(0.0140165567282563,-0.0327619876829988,
0.075022752632895));
#85005=CARTESIAN_POINT('Ctrl Pts',(0.0139748233384161,-0.0328131562602352,
0.0750165716861023));
#85006=CARTESIAN_POINT('Ctrl Pts',(0.0138928204166615,-0.0329167375858765,
0.0750044265980051));
#85007=CARTESIAN_POINT('Ctrl Pts',(0.0138525835591661,-0.0329691088920618,
0.0749984672959634));
#85008=CARTESIAN_POINT('Ctrl Pts',(0.0138130810947739,-0.0330220786163186,
0.0749926167616186));
#85009=CARTESIAN_POINT('Ctrl Pts',(0.0138284219717157,-0.0331951640388604,
0.0748699750076524));
#85010=CARTESIAN_POINT('Ctrl Pts',(0.0138433069933938,-0.0330306422010619,
0.0747520352377044));
#85011=CARTESIAN_POINT('Ctrl Pts',(0.013853304721205,-0.0328657861914645,
0.0746335810328641));
#85012=CARTESIAN_POINT('Ctrl Pts',(0.013830050647665,-0.0331951640388604,
0.0748687665299189));
#85013=CARTESIAN_POINT('Ctrl Pts',(0.0138449106848409,-0.0330306422010619,
0.0747507930881399));
#85014=CARTESIAN_POINT('Ctrl Pts',(0.0138548820578066,-0.0328657861914645,
0.0746323062728766));
#85015=CARTESIAN_POINT('Ctrl Pts',(0.0141014318602109,-0.0331951640388604,
0.0746674016403838));
#85016=CARTESIAN_POINT('Ctrl Pts',(0.0141121288073988,-0.0330306422010619,
0.0745438175660289));
#85017=CARTESIAN_POINT('Ctrl Pts',(0.0141177087543631,-0.0328657861914645,
0.0744198969773231));
#85018=CARTESIAN_POINT('',(0.0141025234022412,-0.033178164828195,0.0746546320938944));
#85019=CARTESIAN_POINT('',(0.0141014318602036,-0.0331951640388588,0.0746674016403882));
#85020=CARTESIAN_POINT('Origin',(-0.00240583847027637,-0.0326412092720937,
0.0739760525074001));
#85021=CARTESIAN_POINT('Ctrl Pts',(0.0141025234010472,-0.033178164828644,
0.0746546320952973));
#85022=CARTESIAN_POINT('Ctrl Pts',(0.0140596926911923,-0.0331276811546766,
0.0746510170068694));
#85023=CARTESIAN_POINT('Ctrl Pts',(0.0140176353684742,-0.0330765663497773,
0.0746474672294402));
#85024=CARTESIAN_POINT('Ctrl Pts',(0.013935031376349,-0.0329730614463479,
0.0746404950851237));
#85025=CARTESIAN_POINT('Ctrl Pts',(0.0138945180775977,-0.0329207133374377,
0.0746370755294888));
#85026=CARTESIAN_POINT('Ctrl Pts',(0.0138547629219927,-0.0328677532289394,
0.0746337200174055));
#85027=CARTESIAN_POINT('',(0.0139657412539446,-0.0331951640388701,0.0747680840851621));
#85028=CARTESIAN_POINT('Origin',(0.00812378219310841,-0.0315241814719618,
0.07415));
#85029=CARTESIAN_POINT('',(0.0141025234007489,-0.0332121607144205,0.0746546320931199));
#85030=CARTESIAN_POINT('',(0.0141035876665865,-0.0331951640388587,0.0746418602437367));
#85031=CARTESIAN_POINT('Origin',(-0.00240177833528214,-0.0326413665497158,
0.0740212147868483));
#85032=CARTESIAN_POINT('Origin',(-0.00228602857041441,-0.0326412096280679,
0.0725565677200206));
#85033=CARTESIAN_POINT('Origin',(-0.00227445427339749,-0.0326413667757252,
0.0725127248825164));
#85034=CARTESIAN_POINT('Ctrl Pts',(0.0138389631736647,-0.0337436976235975,
0.0747940740326138));
#85035=CARTESIAN_POINT('Ctrl Pts',(0.0138447560731261,-0.0336723290703325,
0.0747426708287153));
#85036=CARTESIAN_POINT('Ctrl Pts',(0.0138496234538143,-0.033601104548885,
0.0746911717446415));
#85037=CARTESIAN_POINT('Ctrl Pts',(0.0138651640361777,-0.0333736987606856,
0.0745267453705877));
#85038=CARTESIAN_POINT('Ctrl Pts',(0.0138712432754734,-0.0331450831799191,
0.0743616981499681));
#85039=CARTESIAN_POINT('Ctrl Pts',(0.0138615538439715,-0.0337436976235975,
0.0745450968014961));
#85040=CARTESIAN_POINT('Ctrl Pts',(0.0138651074044827,-0.0336723290703325,
0.0744934904136851));
#85041=CARTESIAN_POINT('Ctrl Pts',(0.0138677321538547,-0.033601104548885,
0.0744418284572187));
#85042=CARTESIAN_POINT('Ctrl Pts',(0.0138761124586661,-0.0333736987606856,
0.0742768820638785));
#85043=CARTESIAN_POINT('Ctrl Pts',(0.0138750133782756,-0.0331450831799191,
0.0741117265789348));
#85044=CARTESIAN_POINT('Ctrl Pts',(0.0138617797506745,-0.0337436976235975,
0.0745426070291849));
#85045=CARTESIAN_POINT('Ctrl Pts',(0.0138653109177962,-0.0336723290703325,
0.0744909986095348));
#85046=CARTESIAN_POINT('Ctrl Pts',(0.0138679132408551,-0.033601104548885,
0.0744393350243445));
#85047=CARTESIAN_POINT('Ctrl Pts',(0.013876221942891,-0.0333736987606856,
0.0742743834308115));
#85048=CARTESIAN_POINT('Ctrl Pts',(0.0138750510793037,-0.0331450831799191,
0.0741092268632245));
#85049=CARTESIAN_POINT('',(0.0138639223541781,-0.0336938721132548,0.0745090486475063));
#85050=CARTESIAN_POINT('',(0.0138738271572256,-0.0333679869945434,0.0742729142414415));
#85051=CARTESIAN_POINT('Ctrl Pts',(0.0138639223541781,-0.033693872113265,
0.0745090486475155));
#85052=CARTESIAN_POINT('Ctrl Pts',(0.0138653238894816,-0.0336629187933933,
0.0744866421877192));
#85053=CARTESIAN_POINT('Ctrl Pts',(0.0138665937777099,-0.0336319952301041,
0.0744642346874896));
#85054=CARTESIAN_POINT('Ctrl Pts',(0.0138677321538542,-0.0336011045488951,
0.0744418284572279));
#85055=CARTESIAN_POINT('Ctrl Pts',(0.0138705887291307,-0.0335235892595453,
0.0743856035585208));
#85056=CARTESIAN_POINT('Ctrl Pts',(0.0138726221261806,-0.0334458668660369,
0.0743292867427685));
#85057=CARTESIAN_POINT('Ctrl Pts',(0.0138738271575316,-0.0333679869945386,
0.0742729142414548));
#85058=CARTESIAN_POINT('Ctrl Pts',(0.013873828795071,-0.0333679692459109,
0.0742728697961073));
#85059=CARTESIAN_POINT('Ctrl Pts',(0.0138733755581721,-0.033339189537426,
0.0742728660364243));
#85060=CARTESIAN_POINT('Ctrl Pts',(0.0138730358080678,-0.0333104081060745,
0.0742728664654439));
#85061=CARTESIAN_POINT('Ctrl Pts',(0.0138725860978153,-0.0332532698357313,
0.0742728725717586));
#85062=CARTESIAN_POINT('Ctrl Pts',(0.0138724727837111,-0.0332249171907008,
0.0742728781730112));
#85063=CARTESIAN_POINT('Ctrl Pts',(0.013872468966693,-0.0331960985338784,
0.0742728849926027));
#85064=CARTESIAN_POINT('Ctrl Pts',(0.0138724689345538,-0.0331956312586429,
0.0742728851037769));
#85065=CARTESIAN_POINT('Ctrl Pts',(0.0138724689321763,-0.033195164038859,
0.074272885214998));
#85066=CARTESIAN_POINT('',(0.013869797514459,-0.0331951640388587,0.0743978566658474));
#85067=CARTESIAN_POINT('',(0.0138711332233277,-0.0331951640388687,0.0743353709404327));
#85068=CARTESIAN_POINT('',(0.0138547629068615,-0.033521636656766,0.074633720016266));
#85069=CARTESIAN_POINT('Origin',(-0.00279859809327077,-0.0326434571526035,
0.0744433718934559));
#85070=CARTESIAN_POINT('',(0.0138534091855672,-0.0336938721132326,0.0746336057560541));
#85071=CARTESIAN_POINT('Origin',(0.0247352852322952,-0.0336938867896224,
0.0755520847427957));
#85072=CARTESIAN_POINT('',(0.0138586657698826,-0.0336938721132536,0.0745713272017903));
#85073=CARTESIAN_POINT('Ctrl Pts',(0.0140781491240354,-0.0335235895815172,
0.0748885895016754));
#85074=CARTESIAN_POINT('Ctrl Pts',(0.0140883172626749,-0.0334144449262748,
0.0748066159178015));
#85075=CARTESIAN_POINT('Ctrl Pts',(0.0140968035707229,-0.0333049234473147,
0.0747243380901192));
#85076=CARTESIAN_POINT('Ctrl Pts',(0.0141035876665938,-0.0331951640388587,
0.0746418602437443));
#85077=CARTESIAN_POINT('Ctrl Pts',(0.014003200098239,-0.0335235895815172,
0.0748035964665564));
#85078=CARTESIAN_POINT('Ctrl Pts',(0.0140121981404142,-0.0334144449262748,
0.0747226547035836));
#85079=CARTESIAN_POINT('Ctrl Pts',(0.0140195343243421,-0.0333049234473147,
0.074641434055552));
#85080=CARTESIAN_POINT('Ctrl Pts',(0.0140251898615454,-0.0331951640388587,
0.0745600375289875));
#85081=CARTESIAN_POINT('Ctrl Pts',(0.0139282510724427,-0.0335235895815172,
0.0747186034314374));
#85082=CARTESIAN_POINT('Ctrl Pts',(0.0139360790181536,-0.0334144449262748,
0.0746386934893658));
#85083=CARTESIAN_POINT('Ctrl Pts',(0.0139422650779614,-0.0333049234473147,
0.0745585300209849));
#85084=CARTESIAN_POINT('Ctrl Pts',(0.0139467920564971,-0.0331951640388587,
0.0744782148142308));
#85085=CARTESIAN_POINT('Ctrl Pts',(0.0138533020466464,-0.0335235895815172,
0.0746336103963184));
#85086=CARTESIAN_POINT('Ctrl Pts',(0.0138599598958929,-0.0334144449262748,
0.0745547322751479));
#85087=CARTESIAN_POINT('Ctrl Pts',(0.0138649958315807,-0.0333049234473147,
0.0744756259864177));
#85088=CARTESIAN_POINT('Ctrl Pts',(0.0138683942514488,-0.0331951640388587,
0.074396392099474));
#85089=CARTESIAN_POINT('',(0.0139866925905328,-0.0331951640388687,0.074519858454802));
#85090=CARTESIAN_POINT('Ctrl Pts',(0.0141025233976227,-0.0332121607145939,
0.0746546320928511));
#85091=CARTESIAN_POINT('Ctrl Pts',(0.0140597647410649,-0.0332625444108758,
0.074651023073894));
#85092=CARTESIAN_POINT('Ctrl Pts',(0.0140177428832558,-0.0333135300744814,
0.0746474762439968));
#85093=CARTESIAN_POINT('Ctrl Pts',(0.0139351394084258,-0.0334167203140546,
0.074640504146869));
#85094=CARTESIAN_POINT('Ctrl Pts',(0.013894589784646,-0.0334688847587227,
0.0746370815800088));
#85095=CARTESIAN_POINT('Ctrl Pts',(0.0138547629061685,-0.0335216366562281,
0.0746337200160356));
#85096=CARTESIAN_POINT('Ctrl Pts',(0.0138631583902534,-0.033693872113239,
0.0745096936854851));
#85097=CARTESIAN_POINT('Ctrl Pts',(0.0138652637967536,-0.0336474569764958,
0.0744760992120762));
#85098=CARTESIAN_POINT('Ctrl Pts',(0.0138669757932624,-0.033601104548885,
0.0744424823941408));
#85099=CARTESIAN_POINT('Ctrl Pts',(0.0138713101748101,-0.0334837508592656,
0.0743573723401193));
#85100=CARTESIAN_POINT('Ctrl Pts',(0.013873120665654,-0.0333660264659097,
0.0742721712234493));
#85101=CARTESIAN_POINT('Ctrl Pts',(0.0138639223541767,-0.033693872113239,
0.0745090486475269));
#85102=CARTESIAN_POINT('Ctrl Pts',(0.0138660239850557,-0.0336474569764958,
0.0744754497023837));
#85103=CARTESIAN_POINT('Ctrl Pts',(0.0138677321538547,-0.033601104548885,
0.0744418284572187));
#85104=CARTESIAN_POINT('Ctrl Pts',(0.0138720568445213,-0.0334837508592656,
0.07435670719447));
#85105=CARTESIAN_POINT('Ctrl Pts',(0.0138738573166017,-0.0333660264659097,
0.0742714951611556));
#85106=CARTESIAN_POINT('Ctrl Pts',(0.0141236734632555,-0.033693872113239,
0.074289732892016));
#85107=CARTESIAN_POINT('Ctrl Pts',(0.0141244913662408,-0.0336474569764958,
0.0742546135374367));
#85108=CARTESIAN_POINT('Ctrl Pts',(0.0141248980967959,-0.033601104548885,
0.0742194870146711));
#85109=CARTESIAN_POINT('Ctrl Pts',(0.0141259278450482,-0.0334837508592656,
0.0741305547351223));
#85110=CARTESIAN_POINT('Ctrl Pts',(0.0141243218932809,-0.0333660264659097,
0.0740416309945008));
#85111=CARTESIAN_POINT('',(0.0141224118338749,-0.0336769361243753,0.0742782280504327));
#85112=CARTESIAN_POINT('',(0.0141221242518552,-0.0336938721132327,0.0742910409382789));
#85113=CARTESIAN_POINT('Ctrl Pts',(0.0141224118338749,-0.033676936124375,
0.0742782280504324));
#85114=CARTESIAN_POINT('Ctrl Pts',(0.0141223661808355,-0.0336797586669966,
0.0742803637428505));
#85115=CARTESIAN_POINT('Ctrl Pts',(0.0141223193889672,-0.0336825812712728,
0.0742824993301146));
#85116=CARTESIAN_POINT('Ctrl Pts',(0.0141222235282267,-0.0336882265947832,
0.0742867702880857));
#85117=CARTESIAN_POINT('Ctrl Pts',(0.0141221744593723,-0.0336910493139906,
0.0742889056587687));
#85118=CARTESIAN_POINT('Ctrl Pts',(0.0141221242518612,-0.0336938721132353,
0.0742910409382756));
#85119=CARTESIAN_POINT('Ctrl Pts',(0.0141224118338748,-0.0336769361243754,
0.0742782280504327));
#85120=CARTESIAN_POINT('Ctrl Pts',(0.014080508590939,-0.0336279018505204,
0.0742773323173286));
#85121=CARTESIAN_POINT('Ctrl Pts',(0.0140380025168502,-0.0335767826010746,
0.0742764236979712));
#85122=CARTESIAN_POINT('Ctrl Pts',(0.0139547150328192,-0.0334733172064637,
0.0742746433260626));
#85123=CARTESIAN_POINT('Ctrl Pts',(0.0139138776469841,-0.0334209631456282,
0.0742737703769581));
#85124=CARTESIAN_POINT('Ctrl Pts',(0.0138738271570598,-0.0333679869844681,
0.0742729142487173));
#85125=CARTESIAN_POINT('',(0.0139930233030266,-0.0336938721132538,0.0744000447929027));
#85126=CARTESIAN_POINT('Origin',(0.00812378219310841,-0.0315241814719618,
0.07415));
#85127=CARTESIAN_POINT('',(0.0141224118325865,-0.0337108120655527,0.0742782280504102));
#85128=CARTESIAN_POINT('',(0.0141226720466813,-0.0336938721132327,0.0742654145775366));
#85129=CARTESIAN_POINT('Origin',(-0.00221117739885073,-0.0345562524779775,
0.0728112158998784));
#85130=CARTESIAN_POINT('Ctrl Pts',(0.0141226720466944,-0.0336938721132384,
0.0742654145775444));
#85131=CARTESIAN_POINT('Ctrl Pts',(0.0141226309613475,-0.0336910492958727,
0.0742675500657631));
#85132=CARTESIAN_POINT('Ctrl Pts',(0.0141225887348685,-0.0336882265857238,
0.0742696855758484));
#85133=CARTESIAN_POINT('Ctrl Pts',(0.0141225019976713,-0.0336825812712687,
0.0742739567219923));
#85134=CARTESIAN_POINT('Ctrl Pts',(0.0141224574869142,-0.0336797586669946,
0.0742760923580164));
#85135=CARTESIAN_POINT('Ctrl Pts',(0.0141224118338749,-0.033676936124375,
0.074278228050433));
#85136=CARTESIAN_POINT('Origin',(-0.00225894604208123,-0.0345562520800193,
0.0750459176398226));
#85137=CARTESIAN_POINT('Ctrl Pts',(0.0138681247630567,-0.034243627687391,
0.0744339954913032));
#85138=CARTESIAN_POINT('Ctrl Pts',(0.0138788358295853,-0.0339430054201809,
0.0742173440397331));
#85139=CARTESIAN_POINT('Ctrl Pts',(0.0138731973920629,-0.0336441434784052,
0.0740005012708061));
#85140=CARTESIAN_POINT('Ctrl Pts',(0.0138750396898682,-0.034243627687391,
0.0741840911420269));
#85141=CARTESIAN_POINT('Ctrl Pts',(0.0138763254584859,-0.0339430054201809,
0.0739671788896928));
#85142=CARTESIAN_POINT('Ctrl Pts',(0.0138612688547536,-0.0336441434784052,
0.073750786012967));
#85143=CARTESIAN_POINT('Ctrl Pts',(0.0138751088391363,-0.034243627687391,
0.0741815920985342));
#85144=CARTESIAN_POINT('Ctrl Pts',(0.0138763003547749,-0.0339430054201809,
0.0739646772381924));
#85145=CARTESIAN_POINT('Ctrl Pts',(0.0138611495693806,-0.0336441434784052,
0.0737482888603886));
#85146=CARTESIAN_POINT('',(0.0138751403498937,-0.034193496108874,0.0741479137641487));
#85147=CARTESIAN_POINT('',(0.0138701986066189,-0.033866421286332,0.0739116233931666));
#85148=CARTESIAN_POINT('Origin',(-0.00285207083601065,-0.0345610720404536,
0.0736443765677451));
#85149=CARTESIAN_POINT('Origin',(0.0248270276664345,-0.033693800507288,
0.0734570671026286));
#85150=CARTESIAN_POINT('',(0.013874022114592,-0.0336938721132327,0.0740365722900837));
#85151=CARTESIAN_POINT('',(0.0138714316765818,-0.0336938721132426,0.0739741259961215));
#85152=CARTESIAN_POINT('',(0.0138738271570597,-0.0340203938281605,0.0742729142487225));
#85153=CARTESIAN_POINT('Origin',(-0.0027636184318799,-0.0345589643244419,
0.0731713935802988));
#85154=CARTESIAN_POINT('',(0.0138724689321763,-0.0341934961088739,0.074272885214998));
#85155=CARTESIAN_POINT('Origin',(0.0248893994280871,-0.0341934220717642,
0.0745083861920761));
#85156=CARTESIAN_POINT('',(0.013873804641045,-0.034193496108884,0.0742103994895834));
#85157=CARTESIAN_POINT('Ctrl Pts',(0.0141127757939143,-0.0340223579322396,
0.0745132570021457));
#85158=CARTESIAN_POINT('Ctrl Pts',(0.0141177860553879,-0.0339125849573574,
0.0744306531604395));
#85159=CARTESIAN_POINT('Ctrl Pts',(0.0141210830886303,-0.0338030433565231,
0.0743480036627263));
#85160=CARTESIAN_POINT('Ctrl Pts',(0.014122672046689,-0.0336938721132327,
0.0742654145775436));
#85161=CARTESIAN_POINT('Ctrl Pts',(0.0140326379196887,-0.0340223579322396,
0.0744331377101772));
#85162=CARTESIAN_POINT('Ctrl Pts',(0.0140365431271662,-0.0339125849573574,
0.074351639178765));
#85163=CARTESIAN_POINT('Ctrl Pts',(0.0140387587602758,-0.0338030433565231,
0.0742701170867068));
#85164=CARTESIAN_POINT('Ctrl Pts',(0.0140392912271874,-0.0336938721132327,
0.0741886759381879));
#85165=CARTESIAN_POINT('Ctrl Pts',(0.0139525000454631,-0.0340223579322396,
0.0743530184182088));
#85166=CARTESIAN_POINT('Ctrl Pts',(0.0139553001989445,-0.0339125849573574,
0.0742726251970905));
#85167=CARTESIAN_POINT('Ctrl Pts',(0.0139564344319213,-0.0338030433565231,
0.0741922305106874));
#85168=CARTESIAN_POINT('Ctrl Pts',(0.0139559104076859,-0.0336938721132327,
0.0741119372988321));
#85169=CARTESIAN_POINT('Ctrl Pts',(0.0138723621712376,-0.0340223579322396,
0.0742728991262404));
#85170=CARTESIAN_POINT('Ctrl Pts',(0.0138740572707228,-0.0339125849573574,
0.0741936112154159));
#85171=CARTESIAN_POINT('Ctrl Pts',(0.0138741101035668,-0.0338030433565231,
0.074114343934668));
#85172=CARTESIAN_POINT('Ctrl Pts',(0.0138725295881843,-0.0336938721132327,
0.0740351986594764));
#85173=CARTESIAN_POINT('',(0.0139983470806467,-0.0336938721132427,0.0741509934338202));
#85174=CARTESIAN_POINT('Ctrl Pts',(0.014122411828979,-0.0337108120662654,
0.0742782280503281));
#85175=CARTESIAN_POINT('Ctrl Pts',(0.0140794223936299,-0.0337611408993377,
0.0742773090985317));
#85176=CARTESIAN_POINT('Ctrl Pts',(0.0140372174200965,-0.0338121088779457,
0.0742764069155668));
#85177=CARTESIAN_POINT('Ctrl Pts',(0.0139543379483227,-0.0339153382773231,
0.0742746352654196));
#85178=CARTESIAN_POINT('Ctrl Pts',(0.0139136985133928,-0.0339675558473107,
0.0742737665477584));
#85179=CARTESIAN_POINT('Ctrl Pts',(0.0138738271570199,-0.0340203938281304,
0.0742729142487164));
#85180=CARTESIAN_POINT('Ctrl Pts',(0.0138736759116553,-0.0341934961088741,
0.0741493169043875));
#85181=CARTESIAN_POINT('Ctrl Pts',(0.0138736617891916,-0.0340287516182428,
0.074030442381591));
#85182=CARTESIAN_POINT('Ctrl Pts',(0.0138687345045831,-0.0338644633275951,
0.0739116700184927));
#85183=CARTESIAN_POINT('Ctrl Pts',(0.0138751403498937,-0.0341934961088741,
0.0741479137641487));
#85184=CARTESIAN_POINT('Ctrl Pts',(0.013875097218611,-0.0340287516182428,
0.0740290089652454));
#85185=CARTESIAN_POINT('Ctrl Pts',(0.0138701396986365,-0.0338644633275951,
0.0739102075508671));
#85186=CARTESIAN_POINT('Ctrl Pts',(0.0141191439277879,-0.034193496108874,
0.0739141236120166));
#85187=CARTESIAN_POINT('Ctrl Pts',(0.0141142673692925,-0.0340287516182428,
0.0737901742313691));
#85188=CARTESIAN_POINT('Ctrl Pts',(0.0141042720557859,-0.0338644633275951,
0.073666532314959));
#85189=CARTESIAN_POINT('',(0.0141186264137054,-0.0341764758832436,0.0739013179509364));
#85190=CARTESIAN_POINT('',(0.0141191439277825,-0.034193496108874,0.0739141236120217));
#85191=CARTESIAN_POINT('Origin',(-0.00244612043510156,-0.0345621026295853,
0.0740759282701026));
#85192=CARTESIAN_POINT('Ctrl Pts',(0.0141186264129026,-0.0341764758837543,
0.0739013179525675));
#85193=CARTESIAN_POINT('Ctrl Pts',(0.0140757389205321,-0.0341260050040233,
0.0739030970533271));
#85194=CARTESIAN_POINT('Ctrl Pts',(0.0140335969155405,-0.0340749269147708,
0.0739048452672929));
#85195=CARTESIAN_POINT('Ctrl Pts',(0.013950771212202,-0.0339715436304957,
0.0739082810932569));
#85196=CARTESIAN_POINT('Ctrl Pts',(0.0139101189358853,-0.033919277823606,
0.0739099673957978));
#85197=CARTESIAN_POINT('Ctrl Pts',(0.0138701986078372,-0.033866421285466,
0.0739116233948971));
#85198=CARTESIAN_POINT('',(0.0139971421388481,-0.0341934961088841,0.0740310186880953));
#85199=CARTESIAN_POINT('Origin',(0.00812378219310841,-0.0315241814719618,
0.07415));
#85200=CARTESIAN_POINT('',(0.0141186264129331,-0.0342105180190352,0.0739013179501266));
#85201=CARTESIAN_POINT('',(0.0141180815491561,-0.0341934961088739,0.0738885134227268));
#85202=CARTESIAN_POINT('Origin',(-0.00244948063736381,-0.0345621718631018,
0.0741211287917469));
#85203=CARTESIAN_POINT('Origin',(-0.00240367129296537,-0.0345621029826751,
0.0750992465279169));
#85204=CARTESIAN_POINT('Origin',(-0.00241076155520861,-0.0345621722654536,
0.0750544795851669));
#85205=CARTESIAN_POINT('Ctrl Pts',(0.0138740842855151,-0.0346945769586965,
0.0740380710110408));
#85206=CARTESIAN_POINT('Ctrl Pts',(0.0138717398880274,-0.0345275153362944,
0.07391762863142));
#85207=CARTESIAN_POINT('Ctrl Pts',(0.0138656070821789,-0.0343603235965185,
0.0737972288283738));
#85208=CARTESIAN_POINT('Ctrl Pts',(0.0138557092984996,-0.034193496108874,
0.0736772274214943));
#85209=CARTESIAN_POINT('Ctrl Pts',(0.0138706096445053,-0.0346945769586965,
0.0739543097118885));
#85210=CARTESIAN_POINT('Ctrl Pts',(0.0138665108330707,-0.0345275153362944,
0.0738339401100148));
#85211=CARTESIAN_POINT('Ctrl Pts',(0.0138586254482872,-0.0343603235965185,
0.0737136682782436));
#85212=CARTESIAN_POINT('Ctrl Pts',(0.0138469820984099,-0.034193496108874,
0.0735938495806466));
#85213=CARTESIAN_POINT('Ctrl Pts',(0.0138671350034952,-0.0346945769586965,
0.0738705484127371));
#85214=CARTESIAN_POINT('Ctrl Pts',(0.0138612817781137,-0.0345275153362944,
0.07375025158861));
#85215=CARTESIAN_POINT('Ctrl Pts',(0.0138516438143953,-0.0343603235965185,
0.0736301077281143));
#85216=CARTESIAN_POINT('Ctrl Pts',(0.0138382548983204,-0.034193496108874,
0.0735104717398013));
#85217=CARTESIAN_POINT('Ctrl Pts',(0.0138636603624858,-0.0346945769586965,
0.0737867871135838));
#85218=CARTESIAN_POINT('Ctrl Pts',(0.0138560527231573,-0.0345275153362944,
0.0736665630672044));
#85219=CARTESIAN_POINT('Ctrl Pts',(0.0138446621805036,-0.0343603235965185,
0.0735465471779831));
#85220=CARTESIAN_POINT('Ctrl Pts',(0.0138295276982305,-0.034193496108874,
0.0734270938989512));
#85221=CARTESIAN_POINT('',(0.0138636603625108,-0.0346945769586966,0.0737867871141892));
#85222=CARTESIAN_POINT('',(0.013843891575329,-0.034366772783152,0.0735512733044807));
#85223=CARTESIAN_POINT('Origin',(-0.00290383243116199,-0.0345626457065536,
0.075031147453749));
#85224=CARTESIAN_POINT('Origin',(0.0248360194119435,-0.0341934771029141,
0.0724007168948601));
#85225=CARTESIAN_POINT('',(0.0138555531447897,-0.034193496108874,0.073675735561671));
#85226=CARTESIAN_POINT('',(0.0138490467831759,-0.034193496108884,0.0736135751461545));
#85227=CARTESIAN_POINT('',(0.0138701986063303,-0.0345211942962626,0.0739116233949307));
#85228=CARTESIAN_POINT('Origin',(-0.00292043911146928,-0.0345625596119892,
0.0745506112866318));
#85229=CARTESIAN_POINT('',(0.0138688412385515,-0.0346945769586885,0.0739116797021393));
#85230=CARTESIAN_POINT('Origin',(0.024922901402722,-0.0346945685853913,
0.0734531286106225));
#85231=CARTESIAN_POINT('',(0.0138662508005412,-0.0346945769587026,0.0738492334081743));
#85232=CARTESIAN_POINT('Ctrl Pts',(0.0141237669768187,-0.0345231616327841,
0.0741364872156039));
#85233=CARTESIAN_POINT('Ctrl Pts',(0.0141235807221103,-0.0344132092796987,
0.0740537858726633));
#85234=CARTESIAN_POINT('Ctrl Pts',(0.0141216838649669,-0.0343032738558979,
0.0739710926492636));
#85235=CARTESIAN_POINT('Ctrl Pts',(0.0141180815491638,-0.0341934961088739,
0.073888513422733));
#85236=CARTESIAN_POINT('Ctrl Pts',(0.0140387566370225,-0.0345231616327841,
0.0740615580606184));
#85237=CARTESIAN_POINT('Ctrl Pts',(0.0140375375894044,-0.0344132092796987,
0.0739800284655269));
#85238=CARTESIAN_POINT('Ctrl Pts',(0.0140346322293188,-0.0343032738558979,
0.0738985282920262));
#85239=CARTESIAN_POINT('Ctrl Pts',(0.0140300469533981,-0.0341934961088739,
0.0738171618559144));
#85240=CARTESIAN_POINT('Ctrl Pts',(0.0139537462972263,-0.0345231616327841,
0.0739866289056329));
#85241=CARTESIAN_POINT('Ctrl Pts',(0.0139514944566985,-0.0344132092796987,
0.0739062710583905));
#85242=CARTESIAN_POINT('Ctrl Pts',(0.0139475805936706,-0.0343032738558979,
0.0738259639347888));
#85243=CARTESIAN_POINT('Ctrl Pts',(0.0139420123576324,-0.0341934961088739,
0.0737458102890957));
#85244=CARTESIAN_POINT('Ctrl Pts',(0.0138687359574301,-0.0345231616327841,
0.0739116997506474));
#85245=CARTESIAN_POINT('Ctrl Pts',(0.0138654513239927,-0.0344132092796987,
0.0738325136512541));
#85246=CARTESIAN_POINT('Ctrl Pts',(0.0138605289580224,-0.0343032738558979,
0.0737533995775514));
#85247=CARTESIAN_POINT('Ctrl Pts',(0.0138539777618667,-0.0341934961088739,
0.0736744587222771));
#85248=CARTESIAN_POINT('',(0.0139868173469829,-0.0341934961088839,0.0737821244922089));
#85249=CARTESIAN_POINT('Ctrl Pts',(0.014118626409476,-0.0342105180195356,
0.0739013179502644));
#85250=CARTESIAN_POINT('Ctrl Pts',(0.0140756907027709,-0.0342610556240236,
0.0739030990373393));
#85251=CARTESIAN_POINT('Ctrl Pts',(0.0140335254551187,-0.0343122189867999,
0.0739048481637278));
#85252=CARTESIAN_POINT('Ctrl Pts',(0.0139506989163743,-0.0344158119695098,
0.0739082840283949));
#85253=CARTESIAN_POINT('Ctrl Pts',(0.0139100715021913,-0.0344681990449982,
0.0739099693613693));
#85254=CARTESIAN_POINT('Ctrl Pts',(0.0138701986062979,-0.0345211942962385,
0.0739116233949225));
#85255=CARTESIAN_POINT('Ctrl Pts',(0.0138622872541964,-0.0346945769586932,
0.073788279073106));
#85256=CARTESIAN_POINT('Ctrl Pts',(0.0138548089299784,-0.034529677707698,
0.0736696395414039));
#85257=CARTESIAN_POINT('Ctrl Pts',(0.0138424335150294,-0.034364806625142,
0.0735514104717111));
#85258=CARTESIAN_POINT('Ctrl Pts',(0.0138636603625113,-0.0346945769586932,
0.0737867871141982));
#85259=CARTESIAN_POINT('Ctrl Pts',(0.0138561511930985,-0.034529677707698,
0.0736681191944533));
#85260=CARTESIAN_POINT('Ctrl Pts',(0.0138437437860077,-0.034364806625142,
0.0735498630358351));
#85261=CARTESIAN_POINT('Ctrl Pts',(0.0140925026499682,-0.0346945769586932,
0.0735381371821048));
#85262=CARTESIAN_POINT('Ctrl Pts',(0.0140798528191484,-0.034529677707698,
0.0734147381099904));
#85263=CARTESIAN_POINT('Ctrl Pts',(0.0140621136004066,-0.034364806625142,
0.073291967309973));
#85264=CARTESIAN_POINT('',(0.0140911820831894,-0.0346775396665019,0.0735253892849195));
#85265=CARTESIAN_POINT('',(0.0140925026499634,-0.0346945769586886,0.0735381371821062));
#85266=CARTESIAN_POINT('Origin',(-0.00240361219251233,-0.0345626617870493,
0.0754054589616631));
#85267=CARTESIAN_POINT('Ctrl Pts',(0.0140911820823922,-0.0346775396670096,
0.0735253892865576));
#85268=CARTESIAN_POINT('Ctrl Pts',(0.0140484573062415,-0.0346269749928188,
0.0735298613230917));
#85269=CARTESIAN_POINT('Ctrl Pts',(0.0140064918484378,-0.0345757902890792,
0.0735342539172826));
#85270=CARTESIAN_POINT('Ctrl Pts',(0.0139240449905657,-0.0344721681088079,
0.0735428836671196));
#85271=CARTESIAN_POINT('Ctrl Pts',(0.013883595912953,-0.0344197714289862,
0.0735471174338918));
#85272=CARTESIAN_POINT('Ctrl Pts',(0.013843891575457,-0.0343667727830735,
0.0735512733047019));
#85273=CARTESIAN_POINT('',(0.0139780815062471,-0.0346945769587026,0.0736624621481577));
#85274=CARTESIAN_POINT('Origin',(0.00812378219310841,-0.0315241814719618,
0.07415));
#85275=CARTESIAN_POINT('',(0.0140911820819387,-0.0347116136489598,0.073525389284308));
#85276=CARTESIAN_POINT('',(0.0140898342906076,-0.0346945769586885,0.0735126442359758));
#85277=CARTESIAN_POINT('Origin',(-0.00239703850763679,-0.0345626698387949,
0.0754502910047274));
#85278=CARTESIAN_POINT('Origin',(-0.00243540937305093,-0.0345626621451001,
0.075101684961038));
#85279=CARTESIAN_POINT('Origin',(-0.00243825970237095,-0.0345626702598509,
0.0750564632766638));
#85280=CARTESIAN_POINT('Ctrl Pts',(0.0138586640873972,-0.0352450361874068,
0.0737142336816784));
#85281=CARTESIAN_POINT('Ctrl Pts',(0.0138422288910126,-0.0349452760959493,
0.0734979390618055));
#85282=CARTESIAN_POINT('Ctrl Pts',(0.0138095481895168,-0.034644428984174,
0.0732834968784183));
#85283=CARTESIAN_POINT('Ctrl Pts',(0.0138584169978104,-0.0352450361874068,
0.073711720800516));
#85284=CARTESIAN_POINT('Ctrl Pts',(0.0138418870265576,-0.0349452760959493,
0.0734954354997799));
#85285=CARTESIAN_POINT('Ctrl Pts',(0.0138091125213945,-0.034644428984174,
0.0732810097478855));
#85286=CARTESIAN_POINT('Ctrl Pts',(0.0138339526822875,-0.0352450361874068,
0.0734629206854316));
#85287=CARTESIAN_POINT('Ctrl Pts',(0.0138080390607158,-0.0349452760959493,
0.073247558071496));
#85288=CARTESIAN_POINT('Ctrl Pts',(0.0137659770637416,-0.034644428984174,
0.0730347592000829));
#85289=CARTESIAN_POINT('Ctrl Pts',(0.0138337080391323,-0.0352450361874068,
0.0734604326842808));
#85290=CARTESIAN_POINT('Ctrl Pts',(0.0138077005810574,-0.0349452760959493,
0.0732450792972131));
#85291=CARTESIAN_POINT('Ctrl Pts',(0.0137655457091651,-0.034644428984174,
0.0730322966946049));
#85292=CARTESIAN_POINT('',(0.0138295341202117,-0.0351951634053356,0.0734271257032898));
#85293=CARTESIAN_POINT('',(0.0137950098858205,-0.0348678972925388,0.0731932861151756));
#85294=CARTESIAN_POINT('Origin',(-0.00265056203983165,-0.0345636767886071,
0.0763954462590038));
#85295=CARTESIAN_POINT('Origin',(0.0246908991536606,-0.0346946199340847,
0.0713551929864585));
#85296=CARTESIAN_POINT('',(0.0138144634960909,-0.0346945769330288,0.0733167705561675));
#85297=CARTESIAN_POINT('',(0.0138040668874039,-0.0346945769458128,0.0732551413292101));
#85298=CARTESIAN_POINT('',(0.0138438915753088,-0.0350221583435275,0.0735512733047011));
#85299=CARTESIAN_POINT('Origin',(-0.00277114445682109,-0.0345628458713436,
0.0759300396914979));
#85300=CARTESIAN_POINT('',(0.0138426617259621,-0.0351951360298763,0.073551405074696));
#85301=CARTESIAN_POINT('Origin',(0.0248017680866508,-0.0351951838366776,
0.0724043080274679));
#85302=CARTESIAN_POINT('',(0.0138295276984102,-0.0351951371328747,0.0734270938995524));
#85303=CARTESIAN_POINT('Ctrl Pts',(0.0141110788401785,-0.0350241211494342,
0.0737597707595798));
#85304=CARTESIAN_POINT('Ctrl Pts',(0.0141057035923919,-0.0349144232818961,
0.0736772982031536));
#85305=CARTESIAN_POINT('Ctrl Pts',(0.0140986203605874,-0.0348045283579412,
0.0735948873931399));
#85306=CARTESIAN_POINT('Ctrl Pts',(0.0140898342894349,-0.0346945769439158,
0.0735126442249313));
#85307=CARTESIAN_POINT('Ctrl Pts',(0.01402153137743,-0.0350241211494342,
0.0736903273025889));
#85308=CARTESIAN_POINT('Ctrl Pts',(0.0140151995744963,-0.0349144232818961,
0.0736090882257461));
#85309=CARTESIAN_POINT('Ctrl Pts',(0.0140071847119047,-0.0348045283579412,
0.0735279314062912));
#85310=CARTESIAN_POINT('Ctrl Pts',(0.0139974931873964,-0.0346945769439158,
0.0734469611778199));
#85311=CARTESIAN_POINT('Ctrl Pts',(0.0139319839146816,-0.0350241211494342,
0.0736208838455979));
#85312=CARTESIAN_POINT('Ctrl Pts',(0.0139246955566008,-0.0349144232818961,
0.0735408782483386));
#85313=CARTESIAN_POINT('Ctrl Pts',(0.013915749063222,-0.0348045283579412,
0.0734609754194426));
#85314=CARTESIAN_POINT('Ctrl Pts',(0.0139051520853578,-0.0346945769439158,
0.0733812781307084));
#85315=CARTESIAN_POINT('Ctrl Pts',(0.0138424364519331,-0.0350241211494342,
0.0735514403886069));
#85316=CARTESIAN_POINT('Ctrl Pts',(0.0138341915387052,-0.0349144232818961,
0.0734726682709311));
#85317=CARTESIAN_POINT('Ctrl Pts',(0.0138243134145394,-0.0348045283579412,
0.0733940194325939));
#85318=CARTESIAN_POINT('Ctrl Pts',(0.0138128109833192,-0.0346945769439158,
0.073315595083597));
#85319=CARTESIAN_POINT('',(0.013952148893479,-0.0346945769458128,0.0734147073963542));
#85320=CARTESIAN_POINT('Ctrl Pts',(0.0140911820786628,-0.0347116136492764,
0.073525389284645));
#85321=CARTESIAN_POINT('Ctrl Pts',(0.0140484742682065,-0.0347621546531224,
0.0735298595324166));
#85322=CARTESIAN_POINT('Ctrl Pts',(0.0140065173764627,-0.0348133084094853,
0.0735342511811529));
#85323=CARTESIAN_POINT('Ctrl Pts',(0.0139240704141856,-0.0349168561544567,
0.0735428809457194));
#85324=CARTESIAN_POINT('Ctrl Pts',(0.0138836130464321,-0.034969208901592,
0.0735471156385334));
#85325=CARTESIAN_POINT('Ctrl Pts',(0.0138438915752704,-0.0350221583434999,
0.073551273304685));
#85326=CARTESIAN_POINT('Ctrl Pts',(0.0138286065039693,-0.0351951371254987,
0.0734282304824678));
#85327=CARTESIAN_POINT('Ctrl Pts',(0.0138136843720475,-0.0350307338980978,
0.073310286819166));
#85328=CARTESIAN_POINT('Ctrl Pts',(0.013793900252131,-0.0348659306897824,
0.0731930606858455));
#85329=CARTESIAN_POINT('Ctrl Pts',(0.0138295276982961,-0.0351951371254987,
0.0734270938995756));
#85330=CARTESIAN_POINT('Ctrl Pts',(0.0138145820682361,-0.0350307338980978,
0.0733091311911591));
#85331=CARTESIAN_POINT('Ctrl Pts',(0.0137947736831052,-0.0348659306897824,
0.0731918870002012));
#85332=CARTESIAN_POINT('Ctrl Pts',(0.0139839208275945,-0.0351951371254987,
0.0732366014222163));
#85333=CARTESIAN_POINT('Ctrl Pts',(0.0139650368850841,-0.0350307338980978,
0.0731154467327211));
#85334=CARTESIAN_POINT('Ctrl Pts',(0.0139411616247454,-0.0348659306897824,
0.0729951760629167));
#85335=CARTESIAN_POINT('Origin',(0.0190390960087422,-0.0308609197410804,
0.0723086293392043));
#85336=CARTESIAN_POINT('',(0.0138968396215688,-0.0351951371254987,0.0733440434744802));
#85337=CARTESIAN_POINT('Origin',(0.00719400186664153,-0.0351840467441097,
0.0744504233596003));
#85338=CARTESIAN_POINT('Origin',(0.0197640715593353,-0.0352322614264454,
0.0713804061305721));
#85339=CARTESIAN_POINT('',(0.0137508238756827,-0.0351951142564683,0.0729607916557664));
#85340=CARTESIAN_POINT('',(0.0137224236649182,-0.0351951372916787,0.0728393842400868));
#85341=CARTESIAN_POINT('Origin',(0.0078838425506991,-0.0352875121025588,
0.0739082761889738));
#85342=CARTESIAN_POINT('Origin',(0.00840357326387426,-0.0298325076522763,
0.0816477934911835));
#85343=CARTESIAN_POINT('Origin',(0.0164034792812193,-0.0338732827791975,
0.0754518908483954));
#85344=CARTESIAN_POINT('Ctrl Pts',(0.0133750333321527,-0.0321934096636942,
0.0764957402285839));
#85345=CARTESIAN_POINT('Ctrl Pts',(0.0134170209651515,-0.0320508460845506,
0.0764017453339559));
#85346=CARTESIAN_POINT('Ctrl Pts',(0.013456451481987,-0.0319086045665427,
0.0763066931869392));
#85347=CARTESIAN_POINT('Ctrl Pts',(0.0134932568310288,-0.0317669892871418,
0.0762107954410903));
#85348=CARTESIAN_POINT('Ctrl Pts',(0.0134075587715715,-0.0321934096636942,
0.0764184580934016));
#85349=CARTESIAN_POINT('Ctrl Pts',(0.0134481630911541,-0.0320508460845506,
0.0763238810088974));
#85350=CARTESIAN_POINT('Ctrl Pts',(0.0134861956953029,-0.0319086045665427,
0.0762282842778795));
#85351=CARTESIAN_POINT('Ctrl Pts',(0.0135215916388741,-0.0317669892871418,
0.0761318804786917));
#85352=CARTESIAN_POINT('Ctrl Pts',(0.0134400842109905,-0.0321934096636942,
0.0763411759582195));
#85353=CARTESIAN_POINT('Ctrl Pts',(0.0134793052171566,-0.0320508460845506,
0.0762460166838389));
#85354=CARTESIAN_POINT('Ctrl Pts',(0.0135159399086188,-0.0319086045665427,
0.0761498753688198));
#85355=CARTESIAN_POINT('Ctrl Pts',(0.0135499264467195,-0.0317669892871418,
0.076052965516293));
#85356=CARTESIAN_POINT('Ctrl Pts',(0.0134726096504094,-0.0321934096636942,
0.0762638938230372));
#85357=CARTESIAN_POINT('Ctrl Pts',(0.0135104473431592,-0.0320508460845506,
0.0761681523587804));
#85358=CARTESIAN_POINT('Ctrl Pts',(0.0135456841219348,-0.0319086045665427,
0.0760714664597601));
#85359=CARTESIAN_POINT('Ctrl Pts',(0.0135782612545649,-0.0317669892871418,
0.0759740505538944));
#85360=CARTESIAN_POINT('',(0.0134720277638687,-0.0321934096636942,0.0762652764157065));
#85361=CARTESIAN_POINT('',(0.0135544173324776,-0.0318665617511356,0.0760437600091658));
#85362=CARTESIAN_POINT('Origin',(-0.0018299028211601,-0.032637194442213,
0.0695519445147125));
#85363=CARTESIAN_POINT('Origin',(0.0239043545394918,-0.0316939261509371,
0.0796529690538259));
#85364=CARTESIAN_POINT('',(0.0134248505768375,-0.0320197221621774,0.0763807539437511));
#85365=CARTESIAN_POINT('Ctrl Pts',(0.0134249634374963,-0.0320197392094696,
0.0763806073922188));
#85366=CARTESIAN_POINT('Ctrl Pts',(0.0134363134417641,-0.0319792716575994,
0.0763536332595562));
#85367=CARTESIAN_POINT('Ctrl Pts',(0.0134475094756399,-0.0319386439829692,
0.0763264498025123));
#85368=CARTESIAN_POINT('Ctrl Pts',(0.0134585554726475,-0.0318979099381624,
0.0762990252626989));
#85369=CARTESIAN_POINT('Ctrl Pts',(0.0134696012513228,-0.0318571766984938,
0.0762716012649517));
#85370=CARTESIAN_POINT('Ctrl Pts',(0.0134804425098669,-0.0318163871833599,
0.0762440762462864));
#85371=CARTESIAN_POINT('Ctrl Pts',(0.0134910452350077,-0.0317755399638304,
0.076216546171814));
#85372=CARTESIAN_POINT('',(0.0134235388830286,-0.0321934096636185,0.0763804885177123));
#85373=CARTESIAN_POINT('Origin',(0.015559901238655,-0.0324113659936054,
0.0772567846722962));
#85374=CARTESIAN_POINT('',(0.0134477833234587,-0.0321934096636663,0.0763228824667194));
#85375=CARTESIAN_POINT('Ctrl Pts',(0.0134701495635384,-0.0321934096636618,
0.0762660419553193));
#85376=CARTESIAN_POINT('Ctrl Pts',(0.0134993314312489,-0.0320835708272592,
0.076192311382566));
#85377=CARTESIAN_POINT('Ctrl Pts',(0.013526970521919,-0.0319739230346488,
0.0761180196593057));
#85378=CARTESIAN_POINT('Ctrl Pts',(0.0135530387681566,-0.0318646057455573,
0.0760432645506017));
#85379=CARTESIAN_POINT('Ctrl Pts',(0.0135750865250978,-0.0321934096636618,
0.0762232704827687));
#85380=CARTESIAN_POINT('Ctrl Pts',(0.0136036785408677,-0.0320835708272592,
0.0761480927475324));
#85381=CARTESIAN_POINT('Ctrl Pts',(0.0136306981727829,-0.0319739230346488,
0.0760723669081574));
#85382=CARTESIAN_POINT('Ctrl Pts',(0.0136561182868257,-0.0318646057455573,
0.0759961925037328));
#85383=CARTESIAN_POINT('Ctrl Pts',(0.0136800234866572,-0.0321934096636618,
0.0761804990102181));
#85384=CARTESIAN_POINT('Ctrl Pts',(0.0137080256504864,-0.0320835708272592,
0.0761038741124988));
#85385=CARTESIAN_POINT('Ctrl Pts',(0.0137344258236468,-0.0319739230346488,
0.0760267141570091));
#85386=CARTESIAN_POINT('Ctrl Pts',(0.0137591978054947,-0.0318646057455573,
0.0759491204568639));
#85387=CARTESIAN_POINT('Ctrl Pts',(0.0137849604482166,-0.0321934096636618,
0.0761377275376675));
#85388=CARTESIAN_POINT('Ctrl Pts',(0.0138123727601052,-0.0320835708272592,
0.0760596554774652));
#85389=CARTESIAN_POINT('Ctrl Pts',(0.0138381534745107,-0.0319739230346488,
0.0759810614058609));
#85390=CARTESIAN_POINT('Ctrl Pts',(0.0138622773241637,-0.0318646057455573,
0.075902048409995));
#85391=CARTESIAN_POINT('',(0.0137891933533198,-0.0321763980308505,0.0761256306242902));
#85392=CARTESIAN_POINT('',(0.0137849604482159,-0.0321934096636184,0.0761377275376413));
#85393=CARTESIAN_POINT('Origin',(-0.00162296792311563,-0.0326386230949013,
0.0701013982530169));
#85394=CARTESIAN_POINT('Ctrl Pts',(0.013789193350319,-0.0321763980306353,
0.0761256306232402));
#85395=CARTESIAN_POINT('Ctrl Pts',(0.0137486678207805,-0.0321259596175861,
0.0761114986432377));
#85396=CARTESIAN_POINT('Ctrl Pts',(0.0137088444486216,-0.032074916463345,
0.0760976115181317));
#85397=CARTESIAN_POINT('Ctrl Pts',(0.0136305699702279,-0.0319716057794018,
0.0760703158016795));
#85398=CARTESIAN_POINT('Ctrl Pts',(0.0135921493625819,-0.0319193786690228,
0.0760569178457389));
#85399=CARTESIAN_POINT('Ctrl Pts',(0.0135544173307223,-0.0318665617525432,
0.0760437600085492));
#85400=CARTESIAN_POINT('',(0.0136284941060523,-0.0321934096636664,0.0762015019766839));
#85401=CARTESIAN_POINT('Origin',(0.00812378219310841,-0.0315241814719618,
0.07415));
#85402=CARTESIAN_POINT('',(0.013789193353669,-0.032210423332359,0.076125630624412));
#85403=CARTESIAN_POINT('',(0.0137934004130286,-0.0321934096636183,0.0761135246981795));
#85404=CARTESIAN_POINT('Origin',(-0.00164371153138138,-0.0326387243762393,
0.0701417064010209));
#85405=CARTESIAN_POINT('Origin',(-0.00202698748102215,-0.0326386237268996,
0.0712599801182748));
#85406=CARTESIAN_POINT('Origin',(-0.00201816615670545,-0.0326387247445193,
0.0712155140851446));
#85407=CARTESIAN_POINT('Ctrl Pts',(0.0134992290150224,-0.0327445246967099,
0.0761951641657272));
#85408=CARTESIAN_POINT('Ctrl Pts',(0.0135763636425132,-0.032443687833936,
0.0759924258745165));
#85409=CARTESIAN_POINT('Ctrl Pts',(0.0136380080619782,-0.0321434074405927,
0.0757844534459835));
#85410=CARTESIAN_POINT('Ctrl Pts',(0.013583028830612,-0.0327445246967099,
0.075959627351392));
#85411=CARTESIAN_POINT('Ctrl Pts',(0.0136512800419259,-0.032443687833936,
0.0757537284984683));
#85412=CARTESIAN_POINT('Ctrl Pts',(0.0137038282156356,-0.0321434074405927,
0.0755432736222576));
#85413=CARTESIAN_POINT('',(0.0135942935279991,-0.0326943950436612,0.0759252832829815));
#85414=CARTESIAN_POINT('',(0.0136626113902798,-0.0323666188837389,0.0756990307048482));
#85415=CARTESIAN_POINT('Origin',(-0.00241905260426027,-0.0326395579112032,
0.0708085652071837));
#85416=CARTESIAN_POINT('Origin',(0.0242990896511115,-0.03219338256031,0.0786737074993454));
#85417=CARTESIAN_POINT('',(0.0136276364285373,-0.0321934096532689,0.0758190457010026));
#85418=CARTESIAN_POINT('',(0.0136444697427272,-0.0321934096584275,0.0757588552542595));
#85419=CARTESIAN_POINT('',(0.0135544173333586,-0.0325210109756238,0.0760437600094734));
#85420=CARTESIAN_POINT('Origin',(-0.00224670839597938,-0.0326393129158107,
0.0703596978508215));
#85421=CARTESIAN_POINT('',(0.0135531345566467,-0.0326943950436595,0.0760433126821901));
#85422=CARTESIAN_POINT('Origin',(0.0239986938429456,-0.0326943765538175,
0.0796858678152558));
#85423=CARTESIAN_POINT('',(0.0135737140423329,-0.0326943950436703,0.0759842979825958));
#85424=CARTESIAN_POINT('Ctrl Pts',(0.0137074012942602,-0.0325229783203769,
0.076346177983078));
#85425=CARTESIAN_POINT('Ctrl Pts',(0.0137376755597297,-0.032413025309245,
0.0762692079158743));
#85426=CARTESIAN_POINT('Ctrl Pts',(0.0137663530087985,-0.032303122220807,
0.0761916232606182));
#85427=CARTESIAN_POINT('Ctrl Pts',(0.0137934004145011,-0.0321934096576658,
0.0761135246939511));
#85428=CARTESIAN_POINT('Ctrl Pts',(0.0136559439311935,-0.0325229783203769,
0.0762452161981136));
#85429=CARTESIAN_POINT('Ctrl Pts',(0.0136848264406652,-0.032413025309245,
0.0761689554695345));
#85430=CARTESIAN_POINT('Ctrl Pts',(0.0137121270184039,-0.032303122220807,
0.0760921088355785));
#85431=CARTESIAN_POINT('Ctrl Pts',(0.01373781416776,-0.0321934096576658,
0.0760147759653));
#85432=CARTESIAN_POINT('Ctrl Pts',(0.0136044865681269,-0.0325229783203769,
0.0761442544131492));
#85433=CARTESIAN_POINT('Ctrl Pts',(0.0136319773216007,-0.032413025309245,
0.0760687030231947));
#85434=CARTESIAN_POINT('Ctrl Pts',(0.0136579010280093,-0.032303122220807,
0.0759925944105388));
#85435=CARTESIAN_POINT('Ctrl Pts',(0.0136822279210189,-0.0321934096576658,
0.0759160272366489));
#85436=CARTESIAN_POINT('Ctrl Pts',(0.0135530292050603,-0.0325229783203769,
0.0760432926281848));
#85437=CARTESIAN_POINT('Ctrl Pts',(0.0135791282025363,-0.032413025309245,
0.0759684505768548));
#85438=CARTESIAN_POINT('Ctrl Pts',(0.0136036750376147,-0.032303122220807,
0.0758930799854991));
#85439=CARTESIAN_POINT('Ctrl Pts',(0.0136266416742778,-0.0321934096576658,
0.0758172785079978));
#85440=CARTESIAN_POINT('',(0.013710518420781,-0.0321934096584275,0.0759662852001075));
#85441=CARTESIAN_POINT('Ctrl Pts',(0.013789193350379,-0.0322104233328888,
0.0761256306232612));
#85442=CARTESIAN_POINT('Ctrl Pts',(0.0137486129080943,-0.0322609421830356,
0.0761114794941978));
#85443=CARTESIAN_POINT('Ctrl Pts',(0.0137087627101504,-0.0323120888238684,
0.0760975830144516));
#85444=CARTESIAN_POINT('Ctrl Pts',(0.0136304876391121,-0.0324156524631808,
0.0760702870913336));
#85445=CARTESIAN_POINT('Ctrl Pts',(0.0135920949414026,-0.0324680267167306,
0.0760568988680963));
#85446=CARTESIAN_POINT('Ctrl Pts',(0.0135544173333192,-0.0325210109755912,
0.0760437600094549));
#85447=CARTESIAN_POINT('Origin',(0.00465724459401615,-0.0262834582510581,
0.081213037796583));
#85448=CARTESIAN_POINT('Origin',(0.0166002198596635,-0.0342771039346039,
0.0828663732632542));
#85449=CARTESIAN_POINT('Ctrl Pts',(0.0135924675457463,-0.0326943950436604,
0.0759261650310439));
#85450=CARTESIAN_POINT('Ctrl Pts',(0.0136169464287621,-0.0325844576448134,
0.0758507962974757));
#85451=CARTESIAN_POINT('Ctrl Pts',(0.0136398682952076,-0.0324744968375322,
0.0757749159665108));
#85452=CARTESIAN_POINT('Ctrl Pts',(0.0136612051172386,-0.0323646534831894,
0.0756986216655388));
#85453=CARTESIAN_POINT('Ctrl Pts',(0.0136945116474589,-0.0326943950436604,
0.075876888983232));
#85454=CARTESIAN_POINT('Ctrl Pts',(0.0137183114141827,-0.0325844576448134,
0.0758001138906913));
#85455=CARTESIAN_POINT('Ctrl Pts',(0.0137405250304648,-0.0324744968375322,
0.0757228411464619));
#85456=CARTESIAN_POINT('Ctrl Pts',(0.0137611254005196,-0.0323646534831894,
0.0756451701494581));
#85457=CARTESIAN_POINT('Ctrl Pts',(0.0137965557491715,-0.0326943950436604,
0.0758276129354202));
#85458=CARTESIAN_POINT('Ctrl Pts',(0.0138196763996034,-0.0325844576448134,
0.0757494314839068));
#85459=CARTESIAN_POINT('Ctrl Pts',(0.013841181765722,-0.0324744968375322,
0.0756707663264129));
#85460=CARTESIAN_POINT('Ctrl Pts',(0.0138610456838007,-0.0323646534831894,
0.0755917186333774));
#85461=CARTESIAN_POINT('Ctrl Pts',(0.0138985998508842,-0.0326943950436604,
0.0757783368876083));
#85462=CARTESIAN_POINT('Ctrl Pts',(0.013921041385024,-0.0325844576448134,
0.0756987490771223));
#85463=CARTESIAN_POINT('Ctrl Pts',(0.0139418385009792,-0.0324744968375322,
0.075618691506364));
#85464=CARTESIAN_POINT('Ctrl Pts',(0.0139609659670817,-0.0323646534831894,
0.0755382671172967));
#85465=CARTESIAN_POINT('',(0.0139020648320283,-0.0326773559991386,0.0757659980585012));
#85466=CARTESIAN_POINT('',(0.0138985998508739,-0.0326943950436594,0.0757783368876127));
#85467=CARTESIAN_POINT('Origin',(-0.00210300197949981,-0.0326395669973887,
0.07134206908712));
#85468=CARTESIAN_POINT('Ctrl Pts',(0.0139020648287955,-0.0326773559987492,
0.0757659980575934));
#85469=CARTESIAN_POINT('Ctrl Pts',(0.0138606986508299,-0.0326267922586907,
0.0757544292805956));
#85470=CARTESIAN_POINT('Ctrl Pts',(0.0138200656584954,-0.0325756109581209,
0.0757430655518155));
#85471=CARTESIAN_POINT('Ctrl Pts',(0.0137402314641275,-0.0324719985462385,
0.0757207385195185));
#85472=CARTESIAN_POINT('Ctrl Pts',(0.0137010622816187,-0.0324196091621774,
0.0757097841708231));
#85473=CARTESIAN_POINT('Ctrl Pts',(0.0136626113902329,-0.0323666188837756,
0.0756990307048351));
#85474=CARTESIAN_POINT('',(0.0137464466894465,-0.0326943950436703,0.0758518100853071));
#85475=CARTESIAN_POINT('Origin',(0.00812378219310841,-0.0315241814719618,
0.07415));
#85476=CARTESIAN_POINT('',(0.0139020648319844,-0.0327114338380031,0.0757659980584892));
#85477=CARTESIAN_POINT('',(0.0139055034524797,-0.0326943950436593,0.07575365185715));
#85478=CARTESIAN_POINT('Origin',(-0.00211445486482875,-0.0326395680973115,
0.0713859069133253));
#85479=CARTESIAN_POINT('Origin',(-0.00207593974010854,-0.0326395673974004,
0.0712453008667923));
#85480=CARTESIAN_POINT('Origin',(-0.00206298814364472,-0.0326395684136933,
0.0712018820662543));
#85481=CARTESIAN_POINT('Ctrl Pts',(0.013617050337381,-0.0332451089994434,
0.075853563939252));
#85482=CARTESIAN_POINT('Ctrl Pts',(0.0136813013025508,-0.0329451141710254,
0.0756463819415156));
#85483=CARTESIAN_POINT('Ctrl Pts',(0.0137297639424734,-0.0326442513127493,
0.0754349488806122));
#85484=CARTESIAN_POINT('Ctrl Pts',(0.0136858936751811,-0.0332451089994434,
0.0756132295995488));
#85485=CARTESIAN_POINT('Ctrl Pts',(0.0137410802824282,-0.0329451141710254,
0.0754034511328469));
#85486=CARTESIAN_POINT('Ctrl Pts',(0.0137803087386556,-0.0326442513127493,
0.0751901117437663));
#85487=CARTESIAN_POINT('Ctrl Pts',(0.013686582108559,-0.0332451089994434,
0.0756108262561518));
#85488=CARTESIAN_POINT('Ctrl Pts',(0.013741678072227,-0.0329451141710254,
0.0754010218247602));
#85489=CARTESIAN_POINT('Ctrl Pts',(0.0137808141866174,-0.0326442513127493,
0.0751876633723979));
#85490=CARTESIAN_POINT('',(0.0136949696831494,-0.0331951640388616,0.0755782839181379));
#85491=CARTESIAN_POINT('',(0.0137489462276525,-0.0328677532355042,0.0753481880713479));
#85492=CARTESIAN_POINT('Origin',(-0.00271755611842626,-0.0326402808279871,
0.0721634275105179));
#85493=CARTESIAN_POINT('Origin',(0.0245624040873967,-0.0326944278779078,
0.0776511236085911));
#85494=CARTESIAN_POINT('',(0.0137215760778875,-0.0326943950436593,0.0754701623474143));
#85495=CARTESIAN_POINT('',(0.013734596785053,-0.0326943950436693,0.0754090337028689));
#85496=CARTESIAN_POINT('',(0.0136626113902791,-0.0330220786163545,0.0756990307048509));
#85497=CARTESIAN_POINT('Origin',(-0.00264833655376976,-0.0326396682764074,
0.0716876530920411));
#85498=CARTESIAN_POINT('',(0.013661303056921,-0.0331951640388588,0.0756986648064837));
#85499=CARTESIAN_POINT('Origin',(0.0242853043275887,-0.0331952026560181,
0.078669854226103));
#85500=CARTESIAN_POINT('',(0.0136781363700452,-0.0331951640388702,0.0756384743623208));
#85501=CARTESIAN_POINT('Ctrl Pts',(0.013834282748829,-0.0330240426238172,
0.0759912450687558));
#85502=CARTESIAN_POINT('Ctrl Pts',(0.0138596476934892,-0.0329142774063519,
0.0759125773601296));
#85503=CARTESIAN_POINT('Ctrl Pts',(0.0138833990022148,-0.0328043479726691,
0.075833346068522));
#85504=CARTESIAN_POINT('Ctrl Pts',(0.0139055034524855,-0.0326943950436593,
0.0757536518571589));
#85505=CARTESIAN_POINT('Ctrl Pts',(0.0137765874806087,-0.0330240426238172,
0.0758937135763538));
#85506=CARTESIAN_POINT('Ctrl Pts',(0.0138006088339408,-0.0329142774063519,
0.0758158406762571));
#85507=CARTESIAN_POINT('Ctrl Pts',(0.0138230323124214,-0.0328043479726691,
0.075737432365206));
#85508=CARTESIAN_POINT('Ctrl Pts',(0.0138438264236151,-0.0326943950436593,
0.0756585882989735));
#85509=CARTESIAN_POINT('Ctrl Pts',(0.0137188922123885,-0.0330240426238172,
0.0757961820839519));
#85510=CARTESIAN_POINT('Ctrl Pts',(0.0137415699743924,-0.0329142774063519,
0.0757191039923847));
#85511=CARTESIAN_POINT('Ctrl Pts',(0.013762665622628,-0.0328043479726691,
0.07564151866189));
#85512=CARTESIAN_POINT('Ctrl Pts',(0.0137821493947446,-0.0326943950436593,
0.0755635247407881));
#85513=CARTESIAN_POINT('Ctrl Pts',(0.0136611969441682,-0.0330240426238172,
0.0756986505915499));
#85514=CARTESIAN_POINT('Ctrl Pts',(0.013682531114844,-0.0329142774063519,
0.0756223673085122));
#85515=CARTESIAN_POINT('Ctrl Pts',(0.0137022989328347,-0.0328043479726691,
0.075545604958574));
#85516=CARTESIAN_POINT('Ctrl Pts',(0.0137204723658742,-0.0326943950436593,
0.0754684611826027));
#85517=CARTESIAN_POINT('',(0.0138135397651936,-0.0326943950436694,0.0756119071022922));
#85518=CARTESIAN_POINT('Ctrl Pts',(0.0139020648287864,-0.0327114338383284,
0.0757659980575908));
#85519=CARTESIAN_POINT('Ctrl Pts',(0.0138607055313769,-0.032761987683,0.0757544312048612));
#85520=CARTESIAN_POINT('Ctrl Pts',(0.0138200758998282,-0.0328131562602372,
0.0757430684159838));
#85521=CARTESIAN_POINT('Ctrl Pts',(0.0137402417787694,-0.0329167375858765,
0.075720741404189));
#85522=CARTESIAN_POINT('Ctrl Pts',(0.0137010690995078,-0.0329691088920621,
0.0757097860775654));
#85523=CARTESIAN_POINT('Ctrl Pts',(0.0136626113902341,-0.0330220786163187,
0.0756990307048355));
#85524=CARTESIAN_POINT('Ctrl Pts',(0.0136932023873735,-0.0331951640388604,
0.0755792787394434));
#85525=CARTESIAN_POINT('Ctrl Pts',(0.0137227518089432,-0.0330306422010619,
0.0754641345477069));
#85526=CARTESIAN_POINT('Ctrl Pts',(0.0137475169502063,-0.0328657861914645,
0.0753478674372073));
#85527=CARTESIAN_POINT('Ctrl Pts',(0.0136949696831486,-0.0331951640388604,
0.075578283918141));
#85528=CARTESIAN_POINT('Ctrl Pts',(0.0137244985374257,-0.0330306422010619,
0.0754631031886974));
#85529=CARTESIAN_POINT('Ctrl Pts',(0.0137492416188289,-0.0328657861914645,
0.0753468004217798));
#85530=CARTESIAN_POINT('Ctrl Pts',(0.0139894486865091,-0.0331951640388604,
0.0754125199358008));
#85531=CARTESIAN_POINT('Ctrl Pts',(0.0140155504767293,-0.0330306422010619,
0.0752912510417652));
#85532=CARTESIAN_POINT('Ctrl Pts',(0.0140366177922328,-0.0328657861914645,
0.0751690069567108));
#85533=CARTESIAN_POINT('',(0.0139921320699566,-0.0331781648281952,0.075399987887492));
#85534=CARTESIAN_POINT('',(0.0139894486864998,-0.0331951640388588,0.075412519935805));
#85535=CARTESIAN_POINT('Origin',(-0.00230100785000773,-0.0326412091906117,
0.0726577128430273));
#85536=CARTESIAN_POINT('Ctrl Pts',(0.0139921320685952,-0.033178164828644,
0.0753999878887349));
#85537=CARTESIAN_POINT('Ctrl Pts',(0.0139500921824034,-0.0331276811546773,
0.0753910331949971));
#85538=CARTESIAN_POINT('Ctrl Pts',(0.0139088113993209,-0.0330765663497786,
0.0753822402283719));
#85539=CARTESIAN_POINT('Ctrl Pts',(0.0138277326057297,-0.0329730614463383,
0.0753649700360556));
#85540=CARTESIAN_POINT('Ctrl Pts',(0.0137879673504078,-0.0329207133374314,
0.075356499781904));
#85541=CARTESIAN_POINT('Ctrl Pts',(0.0137489462332635,-0.0328677532289396,
0.075348188086834));
#85542=CARTESIAN_POINT('',(0.0138422091848346,-0.0331951640388702,0.0754954019269815));
#85543=CARTESIAN_POINT('Origin',(0.00812378219310841,-0.0315241814719618,
0.07415));
#85544=CARTESIAN_POINT('',(0.0139921320685731,-0.0332121607144397,0.0753999878865365));
#85545=CARTESIAN_POINT('',(0.0139947886795375,-0.0331951640388587,0.0753874501348798));
#85546=CARTESIAN_POINT('Origin',(-0.00230263995881673,-0.032641366587239,
0.0727030277353702));
#85547=CARTESIAN_POINT('Origin',(-0.00200423392533245,-0.0326412095231821,
0.0712644370570124));
#85548=CARTESIAN_POINT('Origin',(-0.00198725603646544,-0.0326413668431202,
0.0712223907886903));
#85549=CARTESIAN_POINT('Ctrl Pts',(0.0137131733834289,-0.0337436976235975,
0.0755052974291894));
#85550=CARTESIAN_POINT('Ctrl Pts',(0.013725363133908,-0.0336723290703325,
0.0754550255977284));
#85551=CARTESIAN_POINT('Ctrl Pts',(0.0137366466805782,-0.033601104548885,
0.0754045426438751));
#85552=CARTESIAN_POINT('Ctrl Pts',(0.0137726728099513,-0.0333736987606857,
0.0752433605723316));
#85553=CARTESIAN_POINT('Ctrl Pts',(0.0137993900144804,-0.0331450831799193,
0.0750803767290625));
#85554=CARTESIAN_POINT('Ctrl Pts',(0.0137667910410127,-0.0337436976235975,
0.0752611148196628));
#85555=CARTESIAN_POINT('Ctrl Pts',(0.0137767845760948,-0.0336723290703325,
0.0752103607428634));
#85556=CARTESIAN_POINT('Ctrl Pts',(0.0137858635885902,-0.033601104548885,
0.0751594351246805));
#85557=CARTESIAN_POINT('Ctrl Pts',(0.0138148510770372,-0.0333736987606857,
0.0749968397136192));
#85558=CARTESIAN_POINT('Ctrl Pts',(0.0138344601341928,-0.0331450831799193,
0.0748328487777047));
#85559=CARTESIAN_POINT('Ctrl Pts',(0.0137673272175885,-0.0337436976235975,
0.0752586729935675));
#85560=CARTESIAN_POINT('Ctrl Pts',(0.0137772987905167,-0.0336723290703325,
0.0752079140943148));
#85561=CARTESIAN_POINT('Ctrl Pts',(0.0137863557576704,-0.033601104548885,
0.0751569840494886));
#85562=CARTESIAN_POINT('Ctrl Pts',(0.013815272859708,-0.0333736987606857,
0.0749943745050321));
#85563=CARTESIAN_POINT('Ctrl Pts',(0.0138348108353899,-0.0331450831799193,
0.0748303734981911));
#85564=CARTESIAN_POINT('',(0.0137736589065124,-0.0336938721132548,0.0752256477691773));
#85565=CARTESIAN_POINT('',(0.0138130810958987,-0.0333679869945434,0.0749926167544268));
#85566=CARTESIAN_POINT('Ctrl Pts',(0.0137736589065116,-0.033693872113265,
0.075225647769185));
#85567=CARTESIAN_POINT('Ctrl Pts',(0.0137778576643496,-0.0336629187933933,
0.0752035936499681));
#85568=CARTESIAN_POINT('Ctrl Pts',(0.0137819259435898,-0.0336319952301041,
0.0751815219987686));
#85569=CARTESIAN_POINT('Ctrl Pts',(0.0137858635885888,-0.0336011045488951,
0.0751594351246881));
#85570=CARTESIAN_POINT('Ctrl Pts',(0.0137957444872779,-0.0335235892595455,
0.0751040115999173));
#85571=CARTESIAN_POINT('Ctrl Pts',(0.0138048202190069,-0.033445866866037,
0.0750483937113056));
#85572=CARTESIAN_POINT('Ctrl Pts',(0.0138130810961996,-0.0333679869945386,
0.0749926167544781));
#85573=CARTESIAN_POINT('Ctrl Pts',(0.0138130882913061,-0.0333679692459662,
0.0749925728648361));
#85574=CARTESIAN_POINT('Ctrl Pts',(0.0138126390995285,-0.0333391895375448,
0.0749925123291621));
#85575=CARTESIAN_POINT('Ctrl Pts',(0.0138123019746852,-0.0333104081062116,
0.0749924701728113));
#85576=CARTESIAN_POINT('Ctrl Pts',(0.0138118550452382,-0.0332532698397309,
0.0749924198673398));
#85577=CARTESIAN_POINT('Ctrl Pts',(0.0138117419226178,-0.0332249172105485,
0.0749924112222633));
#85578=CARTESIAN_POINT('Ctrl Pts',(0.0138117372809526,-0.0331960985330548,
0.0749924175098249));
#85579=CARTESIAN_POINT('Ctrl Pts',(0.0138117372351345,-0.0331956312594731,
0.074992417616085));
#85580=CARTESIAN_POINT('Ctrl Pts',(0.013811737218836,-0.0331951640388587,
0.0749924177261313));
#85581=CARTESIAN_POINT('',(0.0137934237900075,-0.0331951640388587,0.0751160689223408));
#85582=CARTESIAN_POINT('',(0.0138025805044319,-0.0331951640388689,0.0750542433242451));
#85583=CARTESIAN_POINT('',(0.0137489462183953,-0.0335216366567655,0.0753481880838062));
#85584=CARTESIAN_POINT('Origin',(-0.00274924111042168,-0.032643457152848,
0.0730721213285905));
#85585=CARTESIAN_POINT('',(0.0137476174921985,-0.0336938721132328,0.0753479050583037));
#85586=CARTESIAN_POINT('Origin',(0.0244285706859872,-0.0336938867896299,
0.0776230026007841));
#85587=CARTESIAN_POINT('',(0.0137606381993654,-0.0336938721132539,0.0752867764137505));
#85588=CARTESIAN_POINT('Ctrl Pts',(0.0139386273517803,-0.0335235895815171,
0.0756290455641303));
#85589=CARTESIAN_POINT('Ctrl Pts',(0.0139589893259433,-0.0334144449262748,
0.0755489927721446));
#85590=CARTESIAN_POINT('Ctrl Pts',(0.0139777208631117,-0.0333049234473147,
0.0754684273461374));
#85591=CARTESIAN_POINT('Ctrl Pts',(0.0139947886795439,-0.0331951640388587,
0.0753874501348884));
#85592=CARTESIAN_POINT('Ctrl Pts',(0.0138749217733604,-0.0335235895815171,
0.0755353291207238));
#85593=CARTESIAN_POINT('Ctrl Pts',(0.0138939935561692,-0.0334144449262748,
0.0754561533614498));
#85594=CARTESIAN_POINT('Ctrl Pts',(0.0139114515385457,-0.0333049234473147,
0.075376492630141));
#85595=CARTESIAN_POINT('Ctrl Pts',(0.0139272641700241,-0.0331951640388587,
0.0752964467662657));
#85596=CARTESIAN_POINT('Ctrl Pts',(0.0138112161949406,-0.0335235895815171,
0.0754416126773173));
#85597=CARTESIAN_POINT('Ctrl Pts',(0.0138289977863952,-0.0334144449262748,
0.075363313950755));
#85598=CARTESIAN_POINT('Ctrl Pts',(0.0138451822139797,-0.0333049234473147,
0.0752845579141447));
#85599=CARTESIAN_POINT('Ctrl Pts',(0.0138597396605043,-0.0331951640388587,
0.0752054433976429));
#85600=CARTESIAN_POINT('Ctrl Pts',(0.0137475106165207,-0.0335235895815171,
0.0753478962339108));
#85601=CARTESIAN_POINT('Ctrl Pts',(0.0137640020166211,-0.0334144449262748,
0.0752704745400602));
#85602=CARTESIAN_POINT('Ctrl Pts',(0.0137789128894136,-0.0333049234473147,
0.0751926231981483));
#85603=CARTESIAN_POINT('Ctrl Pts',(0.0137922151509845,-0.0331951640388587,
0.0751144400290202));
#85604=CARTESIAN_POINT('',(0.0138941062347825,-0.0331951640388687,0.0752517595286203));
#85605=CARTESIAN_POINT('Ctrl Pts',(0.0139921320655044,-0.0332121607145939,
0.0753999878858787));
#85606=CARTESIAN_POINT('Ctrl Pts',(0.0139501629037396,-0.0332625444108773,
0.0753910482444246));
#85607=CARTESIAN_POINT('Ctrl Pts',(0.013908916936489,-0.0333135300744848,
0.0753822626470206));
#85608=CARTESIAN_POINT('Ctrl Pts',(0.0138278386502114,-0.0334167203140541,
0.0753649925663576));
#85609=CARTESIAN_POINT('Ctrl Pts',(0.0137880377336986,-0.0334688847587219,
0.0753565147719912));
#85610=CARTESIAN_POINT('Ctrl Pts',(0.013748946217736,-0.0335216366562274,
0.0753481880834917));
#85611=CARTESIAN_POINT('Ctrl Pts',(0.0137728201219758,-0.0336938721132391,
0.0752261919707698));
#85612=CARTESIAN_POINT('Ctrl Pts',(0.0137791194306991,-0.0336474569764958,
0.0751931262772226));
#85613=CARTESIAN_POINT('Ctrl Pts',(0.0137850312320981,-0.033601104548885,
0.0751599891079957));
#85614=CARTESIAN_POINT('Ctrl Pts',(0.0137999985540321,-0.0334837508592656,
0.0750760934142263));
#85615=CARTESIAN_POINT('Ctrl Pts',(0.0138124733000704,-0.0333660264659097,
0.0749917910484813));
#85616=CARTESIAN_POINT('Ctrl Pts',(0.0137736589065085,-0.0336938721132391,
0.0752256477691974));
#85617=CARTESIAN_POINT('Ctrl Pts',(0.0137799550298394,-0.0336474569764958,
0.075192577165966));
#85618=CARTESIAN_POINT('Ctrl Pts',(0.0137858635885902,-0.033601104548885,
0.0751594351246804));
#85619=CARTESIAN_POINT('Ctrl Pts',(0.0138008227008845,-0.0334837508592656,
0.0750755270959784));
#85620=CARTESIAN_POINT('Ctrl Pts',(0.0138132888753787,-0.0333660264659097,
0.074991212643986));
#85621=CARTESIAN_POINT('Ctrl Pts',(0.0140588493533195,-0.0336938721132391,
0.0750406168303471));
#85622=CARTESIAN_POINT('Ctrl Pts',(0.0140640624291655,-0.0336474569764958,
0.0750058769127942));
#85623=CARTESIAN_POINT('Ctrl Pts',(0.0140688684732108,-0.033601104548885,
0.074971078350008));
#85624=CARTESIAN_POINT('Ctrl Pts',(0.0140810362717547,-0.0334837508592656,
0.0748829763897245));
#85625=CARTESIAN_POINT('Ctrl Pts',(0.0140905880833494,-0.0333660264659097,
0.07479455256023));
#85626=CARTESIAN_POINT('',(0.0140590396112592,-0.0336769361243754,0.0750290445837871));
#85627=CARTESIAN_POINT('',(0.0140571484162445,-0.0336938721132327,0.0750417203946012));
#85628=CARTESIAN_POINT('Ctrl Pts',(0.0140590396112593,-0.0336769361243751,
0.0750290445837868));
#85629=CARTESIAN_POINT('Ctrl Pts',(0.0140587266449707,-0.0336797586670006,
0.0750311577137922));
#85630=CARTESIAN_POINT('Ctrl Pts',(0.0140584125620124,-0.0336825812712807,
0.0750332705967396));
#85631=CARTESIAN_POINT('Ctrl Pts',(0.0140577821643453,-0.0336882265933959,
0.0750374958613505));
#85632=CARTESIAN_POINT('Ctrl Pts',(0.0140574658496594,-0.0336910493112157,
0.0750396082430009));
#85633=CARTESIAN_POINT('Ctrl Pts',(0.0140571484162523,-0.0336938721132359,
0.0750417203945982));
#85634=CARTESIAN_POINT('Ctrl Pts',(0.0140590396112592,-0.0336769361243754,
0.075029044583787));
#85635=CARTESIAN_POINT('Ctrl Pts',(0.0140175781345869,-0.0336279007642955,
0.0750229039088446));
#85636=CARTESIAN_POINT('Ctrl Pts',(0.0139755263106284,-0.0335767878888528,
0.0750166758001912));
#85637=CARTESIAN_POINT('Ctrl Pts',(0.0138931165229763,-0.0334733199122762,
0.0750044704529951));
#85638=CARTESIAN_POINT('Ctrl Pts',(0.0138527094975521,-0.0334209645148418,
0.0749984859481377));
#85639=CARTESIAN_POINT('Ctrl Pts',(0.0138130810948211,-0.0333679869844681,
0.0749926167616255));
#85640=CARTESIAN_POINT('',(0.0139154036613885,-0.0336938721132538,0.0751336840818993));
#85641=CARTESIAN_POINT('Origin',(0.00812378219310841,-0.0315241814719618,
0.07415));
#85642=CARTESIAN_POINT('',(0.0140590396099847,-0.0337108120655525,0.0750290445836027));
#85643=CARTESIAN_POINT('',(0.0140609037262012,-0.0336938721132327,0.0750163647622644));
#85644=CARTESIAN_POINT('Origin',(-0.00196188876620853,-0.034556252508419,
0.0715264587038875));
#85645=CARTESIAN_POINT('Ctrl Pts',(0.0140609037262135,-0.0336938721132384,
0.0750163647622739));
#85646=CARTESIAN_POINT('Ctrl Pts',(0.0140605953171296,-0.0336910492952914,
0.0750184782626061));
#85647=CARTESIAN_POINT('Ctrl Pts',(0.014060285773266,-0.0336882265854332,
0.0750205916409574));
#85648=CARTESIAN_POINT('Ctrl Pts',(0.0140596644034946,-0.0336825812712899,
0.0750248182365514));
#85649=CARTESIAN_POINT('Ctrl Pts',(0.0140593525775484,-0.0336797586670054,
0.0750269314537783));
#85650=CARTESIAN_POINT('Ctrl Pts',(0.0140590396112593,-0.0336769361243754,
0.0750290445837871));
#85651=CARTESIAN_POINT('Origin',(-0.00228936319632219,-0.0345562520762143,
0.0737375521816172));
#85652=CARTESIAN_POINT('Ctrl Pts',(0.0137872348328979,-0.034243627687391,
0.0751517131310215));
#85653=CARTESIAN_POINT('Ctrl Pts',(0.0138250150664495,-0.0339430054201809,
0.0749381124934607));
#85654=CARTESIAN_POINT('Ctrl Pts',(0.0138465986950957,-0.0336441434784052,
0.0747222729109276));
#85655=CARTESIAN_POINT('Ctrl Pts',(0.0138254165536227,-0.034243627687391,
0.0749046460223194));
#85656=CARTESIAN_POINT('Ctrl Pts',(0.0138538784975556,-0.0339430054201809,
0.0746896053374219));
#85657=CARTESIAN_POINT('Ctrl Pts',(0.0138660618386013,-0.0336441434784052,
0.0744730316903302));
#85658=CARTESIAN_POINT('Ctrl Pts',(0.01382579837083,-0.034243627687391,
0.0749021753512324));
#85659=CARTESIAN_POINT('Ctrl Pts',(0.0138541671318667,-0.0339430054201809,
0.0746871202658616));
#85660=CARTESIAN_POINT('Ctrl Pts',(0.0138662564700364,-0.0336441434784052,
0.0744705392781243));
#85661=CARTESIAN_POINT('',(0.0138300506476653,-0.0341934961088741,0.0748687665299178));
#85662=CARTESIAN_POINT('',(0.0138547629078723,-0.0338664212862961,0.0746337200149233));
#85663=CARTESIAN_POINT('Origin',(-0.00270215153662594,-0.0345610720404767,
0.0722727244082535));
#85664=CARTESIAN_POINT('Origin',(0.0247821651368593,-0.0336938005073037,
0.0755560024812745));
#85665=CARTESIAN_POINT('',(0.0138428960169573,-0.0336938721132327,0.0747581628645857));
#85666=CARTESIAN_POINT('',(0.0138481526012722,-0.0336938721132427,0.07469588431033));
#85667=CARTESIAN_POINT('',(0.0138130810948203,-0.0340203938281605,0.0749926167616308));
#85668=CARTESIAN_POINT('Origin',(-0.00255511611877068,-0.0345589643245864,
0.0718145570586121));
#85669=CARTESIAN_POINT('',(0.0138117372188363,-0.0341934961088739,0.0749924177261294));
#85670=CARTESIAN_POINT('Origin',(0.0247122797882539,-0.0341934220717659,
0.0766068495011657));
#85671=CARTESIAN_POINT('',(0.0138208939332608,-0.034193496108884,0.0749305921280336));
#85672=CARTESIAN_POINT('Ctrl Pts',(0.0140200226158527,-0.0340223579322396,
0.0752610125459693));
#85673=CARTESIAN_POINT('Ctrl Pts',(0.0140353463765039,-0.0339125849573575,
0.0751796880124991));
#85674=CARTESIAN_POINT('Ctrl Pts',(0.0140489761404553,-0.0338030433565231,
0.0750981034585989));
#85675=CARTESIAN_POINT('Ctrl Pts',(0.0140609037262082,-0.0336938721132327,
0.0750163647622726));
#85676=CARTESIAN_POINT('Ctrl Pts',(0.0139505582626346,-0.0340223579322396,
0.0751714810796408));
#85677=CARTESIAN_POINT('Ctrl Pts',(0.0139646471508573,-0.0339125849573575,
0.075091114640772));
#85678=CARTESIAN_POINT('Ctrl Pts',(0.0139770627404427,-0.0338030433565231,
0.0750105130672212));
#85679=CARTESIAN_POINT('Ctrl Pts',(0.0139877982911827,-0.0336938721132327,
0.0749297808422835));
#85680=CARTESIAN_POINT('Ctrl Pts',(0.0138810939094166,-0.0340223579322396,
0.0750819496133122));
#85681=CARTESIAN_POINT('Ctrl Pts',(0.0138939479252108,-0.0339125849573575,
0.0750025412690449));
#85682=CARTESIAN_POINT('Ctrl Pts',(0.0139051493404301,-0.0338030433565231,
0.0749229226758435));
#85683=CARTESIAN_POINT('Ctrl Pts',(0.0139146928561573,-0.0336938721132327,
0.0748431969222943));
#85684=CARTESIAN_POINT('Ctrl Pts',(0.0138116295561985,-0.0340223579322396,
0.0749924181469836));
#85685=CARTESIAN_POINT('Ctrl Pts',(0.0138232486995642,-0.0339125849573575,
0.0749139678973179));
#85686=CARTESIAN_POINT('Ctrl Pts',(0.0138332359404174,-0.0338030433565231,
0.0748353322844658));
#85687=CARTESIAN_POINT('Ctrl Pts',(0.0138415874211319,-0.0336938721132327,
0.0747566130023051));
#85688=CARTESIAN_POINT('',(0.0139518998715892,-0.0336938721132427,0.0748872638134351));
#85689=CARTESIAN_POINT('Ctrl Pts',(0.0140590396064153,-0.0337108120662652,
0.0750290445830697));
#85690=CARTESIAN_POINT('Ctrl Pts',(0.0140165043308049,-0.0337611408993368,
0.0750227448725414));
#85691=CARTESIAN_POINT('Ctrl Pts',(0.013974745229603,-0.0338121088779436,
0.0750165601177533));
#85692=CARTESIAN_POINT('Ctrl Pts',(0.0138927413338591,-0.0339153382773232,
0.0750044148854029));
#85693=CARTESIAN_POINT('Ctrl Pts',(0.0138525312322051,-0.0339675558473114,
0.0749984595460499));
#85694=CARTESIAN_POINT('Ctrl Pts',(0.0138130810947816,-0.0340203938281304,
0.0749926167616198));
#85695=CARTESIAN_POINT('Ctrl Pts',(0.0138284218968565,-0.0341934961088741,
0.074869975063197));
#85696=CARTESIAN_POINT('Ctrl Pts',(0.0138433068140832,-0.0340287516182428,
0.0747520361315048));
#85697=CARTESIAN_POINT('Ctrl Pts',(0.0138533045069107,-0.0338644633275951,
0.0746335827714525));
#85698=CARTESIAN_POINT('Ctrl Pts',(0.0138300506476652,-0.0341934961088741,
0.0748687665299179));
#85699=CARTESIAN_POINT('Ctrl Pts',(0.0138449105794185,-0.0340287516182428,
0.0747507939250858));
#85700=CARTESIAN_POINT('Ctrl Pts',(0.0138548819163858,-0.0338644633275951,
0.0746323079533354));
#85701=CARTESIAN_POINT('Ctrl Pts',(0.014101431860211,-0.0341934961088741,
0.0746674016403827));
#85702=CARTESIAN_POINT('Ctrl Pts',(0.0141121287315108,-0.0340287516182428,
0.0745438184427786));
#85703=CARTESIAN_POINT('Ctrl Pts',(0.0141177086752243,-0.0338644633275951,
0.0744198987348472));
#85704=CARTESIAN_POINT('',(0.0141025234017923,-0.0341764758832439,0.074654632094052));
#85705=CARTESIAN_POINT('',(0.0141014318602036,-0.034193496108874,0.0746674016403882));
#85706=CARTESIAN_POINT('Origin',(-0.00235348998283771,-0.0345621027072709,
0.0727517521663097));
#85707=CARTESIAN_POINT('Ctrl Pts',(0.0141025234007908,-0.0341764758837548,
0.0746546320955703));
#85708=CARTESIAN_POINT('Ctrl Pts',(0.0140597511086489,-0.0341260050040147,
0.0746510219394901));
#85709=CARTESIAN_POINT('Ctrl Pts',(0.0140177222966369,-0.0340749269147527,
0.0746474745745116));
#85710=CARTESIAN_POINT('Ctrl Pts',(0.0139351190755364,-0.0339715436304845,
0.0746405024947405));
#85711=CARTESIAN_POINT('Ctrl Pts',(0.0138945760049236,-0.0339192778237439,
0.0746370804190492));
#85712=CARTESIAN_POINT('Ctrl Pts',(0.0138547629087952,-0.0338664212855138,
0.074633720016296));
#85713=CARTESIAN_POINT('',(0.0139657412539445,-0.0341934961088841,0.0747680840851631));
#85714=CARTESIAN_POINT('Origin',(0.00812378219310841,-0.0315241814719618,
0.07415));
#85715=CARTESIAN_POINT('',(0.0141025234011276,-0.0342105180190351,0.074654632093152));
#85716=CARTESIAN_POINT('',(0.0141035876665865,-0.0341934961088739,0.0746418602437368));
#85717=CARTESIAN_POINT('Origin',(-0.00236248866054473,-0.0345621718794165,
0.0727961752181882));
#85718=CARTESIAN_POINT('Origin',(-0.00243963130953617,-0.0345621030710607,
0.0737723217671398));
#85719=CARTESIAN_POINT('Origin',(-0.00244105481376565,-0.0345621723112166,
0.0737270191282932));
#85720=CARTESIAN_POINT('Ctrl Pts',(0.0138427698581003,-0.0346945769586966,
0.0747596575597633));
#85721=CARTESIAN_POINT('Ctrl Pts',(0.0138555393797831,-0.0345275153362944,
0.0746398710733623));
#85722=CARTESIAN_POINT('Ctrl Pts',(0.0138645450295769,-0.0343603235965185,
0.0745196520143369));
#85723=CARTESIAN_POINT('Ctrl Pts',(0.0138697654572347,-0.034193496108874,
0.0743993563331597));
#85724=CARTESIAN_POINT('Ctrl Pts',(0.0138498206901431,-0.0346945769586966,
0.0746761212554798));
#85725=CARTESIAN_POINT('Ctrl Pts',(0.0138608405104866,-0.0345275153362944,
0.0745561870865787));
#85726=CARTESIAN_POINT('Ctrl Pts',(0.0138680913618999,-0.0343603235965185,
0.0744358753333516));
#85727=CARTESIAN_POINT('Ctrl Pts',(0.0138715570881254,-0.034193496108874,
0.0743155421432836));
#85728=CARTESIAN_POINT('Ctrl Pts',(0.0138568715221862,-0.0346945769586966,
0.074592584951197));
#85729=CARTESIAN_POINT('Ctrl Pts',(0.0138661416411903,-0.0345275153362944,
0.0744725030997953));
#85730=CARTESIAN_POINT('Ctrl Pts',(0.0138716376942231,-0.0343603235965185,
0.0743520986523658));
#85731=CARTESIAN_POINT('Ctrl Pts',(0.0138733487190162,-0.034193496108874,
0.0742317279534062));
#85732=CARTESIAN_POINT('Ctrl Pts',(0.0138639223542286,-0.0346945769586966,
0.0745090486469129));
#85733=CARTESIAN_POINT('Ctrl Pts',(0.0138714427718934,-0.0345275153362944,
0.0743888191130115));
#85734=CARTESIAN_POINT('Ctrl Pts',(0.0138751840265459,-0.0343603235965185,
0.0742683219713809));
#85735=CARTESIAN_POINT('Ctrl Pts',(0.0138751403499068,-0.034193496108874,
0.0741479137635315));
#85736=CARTESIAN_POINT('',(0.0138639223541774,-0.0346945769586966,0.0745090486475165));
#85737=CARTESIAN_POINT('',(0.0138738271571082,-0.0343667727831525,0.0742729142485203));
#85738=CARTESIAN_POINT('Origin',(-0.00292731345553948,-0.0345626457063063,
0.0736420727438767));
#85739=CARTESIAN_POINT('Origin',(0.0249234817099851,-0.0341934771028971,
0.0745091106384679));
#85740=CARTESIAN_POINT('',(0.013869797514459,-0.034193496108874,0.0743978566658474));
#85741=CARTESIAN_POINT('',(0.0138711332233277,-0.0341934961088839,0.0743353709404327));
#85742=CARTESIAN_POINT('',(0.0138547629072613,-0.034521194296262,0.0746337200161366));
#85743=CARTESIAN_POINT('Origin',(-0.00288356203575707,-0.0345625596117302,
0.0731632443790331));
#85744=CARTESIAN_POINT('',(0.0138534091855672,-0.0346945769586885,0.0746336057560541));
#85745=CARTESIAN_POINT('Origin',(0.0248777764432598,-0.0346945685853899,
0.0755641119509239));
#85746=CARTESIAN_POINT('',(0.0138586657698823,-0.0346945769587026,0.0745713272017954));
#85747=CARTESIAN_POINT('Ctrl Pts',(0.0140781489056537,-0.0345231616327841,
0.0748885912622242));
#85748=CARTESIAN_POINT('Ctrl Pts',(0.0140883293463501,-0.0344132092796988,
0.0748065187001696));
#85749=CARTESIAN_POINT('Ctrl Pts',(0.0140968116555745,-0.0343032738558979,
0.0747242397982963));
#85750=CARTESIAN_POINT('Ctrl Pts',(0.0141035876665937,-0.0341934961088739,
0.0746418602437442));
#85751=CARTESIAN_POINT('Ctrl Pts',(0.0140032000110606,-0.0345231616327841,
0.0748035983252329));
#85752=CARTESIAN_POINT('Ctrl Pts',(0.0140122089437811,-0.0344132092796988,
0.0747225588281706));
#85753=CARTESIAN_POINT('Ctrl Pts',(0.0140195411736084,-0.0343032738558979,
0.0746413371697067));
#85754=CARTESIAN_POINT('Ctrl Pts',(0.0140251899724995,-0.0341934961088739,
0.0745600376447887));
#85755=CARTESIAN_POINT('Ctrl Pts',(0.0139282511164675,-0.0345231616327841,
0.0747186053882416));
#85756=CARTESIAN_POINT('Ctrl Pts',(0.0139360885412121,-0.0344132092796988,
0.0746385989561717));
#85757=CARTESIAN_POINT('Ctrl Pts',(0.0139422706916424,-0.0343032738558979,
0.0745584345411171));
#85758=CARTESIAN_POINT('Ctrl Pts',(0.0139467922784052,-0.0341934961088739,
0.0744782150458331));
#85759=CARTESIAN_POINT('Ctrl Pts',(0.0138533022218744,-0.0345231616327841,
0.0746336124512502));
#85760=CARTESIAN_POINT('Ctrl Pts',(0.013859968138643,-0.0344132092796988,
0.0745546390841727));
#85761=CARTESIAN_POINT('Ctrl Pts',(0.0138650002096763,-0.034303273855898,
0.0744755319125275));
#85762=CARTESIAN_POINT('Ctrl Pts',(0.0138683945843109,-0.0341934961088739,
0.0743963924468776));
#85763=CARTESIAN_POINT('',(0.0139866925905328,-0.0341934961088839,0.074519858454802));
#85764=CARTESIAN_POINT('Ctrl Pts',(0.0141025233976798,-0.0342105180195353,
0.074654632092856));
#85765=CARTESIAN_POINT('Ctrl Pts',(0.0140597030224438,-0.0342610556240235,
0.0746510178645706));
#85766=CARTESIAN_POINT('Ctrl Pts',(0.014017651036698,-0.0343122189867991,
0.0746474684917428));
#85767=CARTESIAN_POINT('Ctrl Pts',(0.0139350469819218,-0.0344158119695089,
0.074640496345665));
#85768=CARTESIAN_POINT('Ctrl Pts',(0.0138945286988031,-0.0344681990449974,
0.0746370764240947));
#85769=CARTESIAN_POINT('Ctrl Pts',(0.0138547629072297,-0.0345211942962376,
0.0746337200161253));
#85770=CARTESIAN_POINT('Ctrl Pts',(0.0138623730811969,-0.0346945769586931,
0.0745103567457866));
#85771=CARTESIAN_POINT('Ctrl Pts',(0.0138698232019357,-0.034529677707698,
0.0743917154396721));
#85772=CARTESIAN_POINT('Ctrl Pts',(0.0138723634024359,-0.034364806625142,
0.0742728675907348));
#85773=CARTESIAN_POINT('Ctrl Pts',(0.0138639223541768,-0.0346945769586931,
0.0745090486475256));
#85774=CARTESIAN_POINT('Ctrl Pts',(0.0138713454309097,-0.034529677707698,
0.0743903753112884));
#85775=CARTESIAN_POINT('Ctrl Pts',(0.0138738572866782,-0.034364806625142,
0.0742714965773515));
#85776=CARTESIAN_POINT('Ctrl Pts',(0.0141221242518614,-0.0346945769586931,
0.0742910409382769));
#85777=CARTESIAN_POINT('Ctrl Pts',(0.0141250401734628,-0.034529677707698,
0.074167029460503));
#85778=CARTESIAN_POINT('Ctrl Pts',(0.0141228280951127,-0.034364806625142,
0.0740430034312678));
#85779=CARTESIAN_POINT('',(0.0141224118333211,-0.0346775396665023,0.0742782280511647));
#85780=CARTESIAN_POINT('',(0.0141221242518551,-0.0346945769586886,0.0742910409382789));
#85781=CARTESIAN_POINT('Origin',(-0.00247795130349033,-0.0345626617742155,
0.074076126929863));
#85782=CARTESIAN_POINT('Ctrl Pts',(0.0141224118323239,-0.0346775396670097,
0.0742782280526905));
#85783=CARTESIAN_POINT('Ctrl Pts',(0.0140794634589947,-0.0346269749928184,
0.0742773099915325));
#85784=CARTESIAN_POINT('Ctrl Pts',(0.0140372783733264,-0.0345757902890787,
0.0742764082822817));
#85785=CARTESIAN_POINT('Ctrl Pts',(0.0139544000390993,-0.0344721681088035,
0.0742746366526692));
#85786=CARTESIAN_POINT('Ctrl Pts',(0.0139137392828609,-0.0344197714289755,
0.0742737674212339));
#85787=CARTESIAN_POINT('Ctrl Pts',(0.0138738271572069,-0.0343667727830744,
0.0742729142487566));
#85788=CARTESIAN_POINT('',(0.0139930233030263,-0.0346945769587026,0.0744000447929077));
#85789=CARTESIAN_POINT('Origin',(0.00812378219310841,-0.0315241814719618,
0.07415));
#85790=CARTESIAN_POINT('',(0.0141224118321568,-0.034711613648978,0.0742782280504013));
#85791=CARTESIAN_POINT('',(0.0141226720466814,-0.0346945769586885,0.0742654145775367));
#85792=CARTESIAN_POINT('Origin',(-0.00247704821473885,-0.034562669910531,
0.0741214292513686));
#85793=CARTESIAN_POINT('Origin',(-0.00247142466767664,-0.0345626621993952,
0.0737707630919827));
#85794=CARTESIAN_POINT('Origin',(-0.00246858475451511,-0.0345626701270886,
0.0737255405042681));
#85795=CARTESIAN_POINT('Ctrl Pts',(0.0138680588324882,-0.0352450361874068,
0.0744364411211761));
#85796=CARTESIAN_POINT('Ctrl Pts',(0.0138788621366473,-0.0349452760959493,
0.0742197921726778));
#85797=CARTESIAN_POINT('Ctrl Pts',(0.0138733158645005,-0.034644428984174,
0.0740029449519637));
#85798=CARTESIAN_POINT('Ctrl Pts',(0.0138681286387982,-0.0352450361874068,
0.0744339170862953));
#85799=CARTESIAN_POINT('Ctrl Pts',(0.0138788367474198,-0.0349452760959493,
0.0742172655050089));
#85800=CARTESIAN_POINT('Ctrl Pts',(0.0138731953518635,-0.034644428984174,
0.0740004228295035));
#85801=CARTESIAN_POINT('Ctrl Pts',(0.0138750401546451,-0.0352450361874068,
0.0741840126426598));
#85802=CARTESIAN_POINT('Ctrl Pts',(0.0138763229625129,-0.0349452760959493,
0.0739671003892759));
#85803=CARTESIAN_POINT('Ctrl Pts',(0.0138612634076013,-0.034644428984174,
0.0737507077344328));
#85804=CARTESIAN_POINT('Ctrl Pts',(0.0138751092698036,-0.0352450361874068,
0.0741815135982235));
#85805=CARTESIAN_POINT('Ctrl Pts',(0.0138762978246639,-0.0349452760959493,
0.0739645987381186));
#85806=CARTESIAN_POINT('Ctrl Pts',(0.0138611440881586,-0.034644428984174,
0.0737482105834822));
#85807=CARTESIAN_POINT('',(0.0138751427351082,-0.0351951634053356,0.0741479461219711));
#85808=CARTESIAN_POINT('',(0.0138701986062541,-0.0348678972934091,0.0739116233943468));
#85809=CARTESIAN_POINT('Origin',(-0.00284703215792656,-0.0345636767885614,
0.0750273568423855));
#85810=CARTESIAN_POINT('Origin',(0.0249105444510711,-0.0346946199326491,
0.0734536263611325));
#85811=CARTESIAN_POINT('',(0.0138740221147906,-0.0346945769330288,0.0740365723080913));
#85812=CARTESIAN_POINT('',(0.013871431676765,-0.0346945769458128,0.0739741260054113));
#85813=CARTESIAN_POINT('',(0.0138738271570594,-0.0350221583435276,0.0742729142487372));
#85814=CARTESIAN_POINT('Origin',(-0.00290833283662269,-0.0345628458712561,
0.0745505071604989));
#85815=CARTESIAN_POINT('',(0.0138725904902828,-0.0351951360298763,0.0742728908386952));
#85816=CARTESIAN_POINT('Origin',(0.0248890503995137,-0.0351951838366758,
0.0745083795262769));
#85817=CARTESIAN_POINT('',(0.0138751403500098,-0.0351951371328746,0.0741479137641504));
#85818=CARTESIAN_POINT('Ctrl Pts',(0.014112775910331,-0.0350241211494342,
0.0745132550827827));
#85819=CARTESIAN_POINT('Ctrl Pts',(0.014117779600156,-0.0349144232818961,
0.074430759149911));
#85820=CARTESIAN_POINT('Ctrl Pts',(0.0141210810350496,-0.0348045283579412,
0.0743481104094029));
#85821=CARTESIAN_POINT('Ctrl Pts',(0.0141226720469026,-0.0346945769439157,
0.0742654145664327));
#85822=CARTESIAN_POINT('Ctrl Pts',(0.0140326381290873,-0.0350241211494342,
0.074433135935128));
#85823=CARTESIAN_POINT('Ctrl Pts',(0.0140365382105035,-0.0349144232818961,
0.0743517438673352));
#85824=CARTESIAN_POINT('Ctrl Pts',(0.0140387581941054,-0.0348045283579412,
0.0742702224649968));
#85825=CARTESIAN_POINT('Ctrl Pts',(0.0140392913507192,-0.0346945769439157,
0.0741886760408568));
#85826=CARTESIAN_POINT('Ctrl Pts',(0.0139525003478436,-0.0350241211494342,
0.0743530167874733));
#85827=CARTESIAN_POINT('Ctrl Pts',(0.013955296820851,-0.0349144232818961,
0.0742727285847594));
#85828=CARTESIAN_POINT('Ctrl Pts',(0.0139564353531612,-0.0348045283579412,
0.0741923345205907));
#85829=CARTESIAN_POINT('Ctrl Pts',(0.0139559106545359,-0.0346945769439157,
0.0741119375152809));
#85830=CARTESIAN_POINT('Ctrl Pts',(0.0138723625665999,-0.0350241211494342,
0.0742728976398186));
#85831=CARTESIAN_POINT('Ctrl Pts',(0.0138740554311984,-0.0349144232818961,
0.0741937133021835));
#85832=CARTESIAN_POINT('Ctrl Pts',(0.013874112512217,-0.0348045283579412,
0.0741144465761847));
#85833=CARTESIAN_POINT('Ctrl Pts',(0.0138725299583526,-0.0346945769439157,
0.0740351989897051));
#85834=CARTESIAN_POINT('',(0.0139983470808299,-0.0346945769458128,0.07415099344311));
#85835=CARTESIAN_POINT('Ctrl Pts',(0.0141224118288639,-0.034711613649276,
0.0742782280503256));
#85836=CARTESIAN_POINT('Ctrl Pts',(0.0140794805116427,-0.0347621546531202,
0.0742773103408754));
#85837=CARTESIAN_POINT('Ctrl Pts',(0.0140373040429872,-0.0348133084094808,
0.0742764087672371));
#85838=CARTESIAN_POINT('Ctrl Pts',(0.0139544256033316,-0.0349168561544568,
0.0742746371391526));
#85839=CARTESIAN_POINT('Ctrl Pts',(0.0139137565062636,-0.0349692089015918,
0.074273767787427));
#85840=CARTESIAN_POINT('Ctrl Pts',(0.0138738271570232,-0.0350221583435,
0.0742729142487165));
#85841=CARTESIAN_POINT('Ctrl Pts',(0.013874083967851,-0.0351951371254987,
0.0741489259284914));
#85842=CARTESIAN_POINT('Ctrl Pts',(0.0138740617620965,-0.035030733898539,
0.0740300420474763));
#85843=CARTESIAN_POINT('Ctrl Pts',(0.0138691259762484,-0.0348659306906667,
0.0739112606698267));
#85844=CARTESIAN_POINT('Ctrl Pts',(0.0138751403498936,-0.0351951371254987,
0.0741479137641592));
#85845=CARTESIAN_POINT('Ctrl Pts',(0.0138750972182767,-0.035030733898539,
0.0740290080431083));
#85846=CARTESIAN_POINT('Ctrl Pts',(0.0138701396217749,-0.0348659306906667,
0.0739102057089735));
#85847=CARTESIAN_POINT('Ctrl Pts',(0.0140521910814103,-0.0351951371254987,
0.0739782739670158));
#85848=CARTESIAN_POINT('Ctrl Pts',(0.0140486407534324,-0.035030733898539,
0.073855707833186));
#85849=CARTESIAN_POINT('Ctrl Pts',(0.0140400276686389,-0.0348659306906667,
0.0737333931702829));
#85850=CARTESIAN_POINT('Origin',(0.0191838114618603,-0.0308609188508581,
0.0736911989231954));
#85851=CARTESIAN_POINT('',(0.0139523304768724,-0.0351951371254987,0.0740739546374729));
#85852=CARTESIAN_POINT('Origin',(0.00716368043114226,-0.0351840467441104,
0.0743315220568552));
#85853=CARTESIAN_POINT('Origin',(0.0200194708629429,-0.0352322613860026,
0.0728611531253263));
#85854=CARTESIAN_POINT('',(0.0138555002984642,-0.0351951142564684,0.0736754242482386));
#85855=CARTESIAN_POINT('',(0.01384254041583,-0.0351951372916788,0.0735514146760448));
#85856=CARTESIAN_POINT('Origin',(0.00791606459898444,-0.0352875118039944,
0.0738801088396702));
#85857=CARTESIAN_POINT('Origin',(0.00746164432488242,-0.0298325076522886,
0.0816237382696252));
#85858=CARTESIAN_POINT('Origin',(0.016174955010655,-0.0338733209737903,
0.0764792659156153));
#85859=CARTESIAN_POINT('Ctrl Pts',(0.0130396264404983,-0.0321934096636942,
0.0771353996517576));
#85860=CARTESIAN_POINT('Ctrl Pts',(0.0130930636725526,-0.0320508460845492,
0.0770474083807612));
#85861=CARTESIAN_POINT('Ctrl Pts',(0.0131440964609289,-0.0319086045665399,
0.0769580477024896));
#85862=CARTESIAN_POINT('Ctrl Pts',(0.0131926307633795,-0.0317669892871375,
0.076867519072417));
#85863=CARTESIAN_POINT('Ctrl Pts',(0.0130815814270117,-0.0321934096636942,
0.0770628034277897));
#85864=CARTESIAN_POINT('Ctrl Pts',(0.0131337192212289,-0.0320508460845492,
0.0769740611825147));
#85865=CARTESIAN_POINT('Ctrl Pts',(0.0131834333743513,-0.0319086045665399,
0.0768839850095321));
#85866=CARTESIAN_POINT('Ctrl Pts',(0.0132306328102157,-0.0317669892871375,
0.0767927776711573));
#85867=CARTESIAN_POINT('Ctrl Pts',(0.0131235364135251,-0.0321934096636942,
0.0769902072038219));
#85868=CARTESIAN_POINT('Ctrl Pts',(0.0131743747699051,-0.0320508460845492,
0.0769007139842681));
#85869=CARTESIAN_POINT('Ctrl Pts',(0.0132227702877738,-0.0319086045665399,
0.0768099223165747));
#85870=CARTESIAN_POINT('Ctrl Pts',(0.013268634857052,-0.0317669892871375,
0.0767180362698976));
#85871=CARTESIAN_POINT('Ctrl Pts',(0.0131654914000384,-0.0321934096636942,
0.0769176109798541));
#85872=CARTESIAN_POINT('Ctrl Pts',(0.0132150303185813,-0.0320508460845492,
0.0768273667860216));
#85873=CARTESIAN_POINT('Ctrl Pts',(0.0132621072011962,-0.0319086045665399,
0.0767358596236172));
#85874=CARTESIAN_POINT('Ctrl Pts',(0.0133066369038883,-0.0317669892871375,
0.0766432948686379));
#85875=CARTESIAN_POINT('',(0.0131647408170369,-0.0321934096636942,0.0769189097406456));
#85876=CARTESIAN_POINT('',(0.013274244086809,-0.0318665617511358,0.0767094662081792));
#85877=CARTESIAN_POINT('Origin',(-0.00117512587987898,-0.0326371944420287,
0.0683406740270635));
#85878=CARTESIAN_POINT('Origin',(0.0230902151182577,-0.0316939261509049,
0.0815874066423466));
#85879=CARTESIAN_POINT('',(0.0131034624642231,-0.0320197221621771,0.0770275638244887));
#85880=CARTESIAN_POINT('Ctrl Pts',(0.0131035928027192,-0.0320197392094689,
0.0770274325737502));
#85881=CARTESIAN_POINT('Ctrl Pts',(0.0131182340640825,-0.0319792716575987,
0.0770020936729162));
#85882=CARTESIAN_POINT('Ctrl Pts',(0.013132748804458,-0.0319386439829682,
0.076976527800679));
#85883=CARTESIAN_POINT('Ctrl Pts',(0.0131471449067337,-0.0318979099381615,
0.0769507039420763));
#85884=CARTESIAN_POINT('Ctrl Pts',(0.0131615407244598,-0.0318571766984932,
0.0769248805939013));
#85885=CARTESIAN_POINT('Ctrl Pts',(0.0131757462960352,-0.0318163871833596,
0.076898931388219));
#85886=CARTESIAN_POINT('Ctrl Pts',(0.0131897158487752,-0.0317755399638304,
0.0768729472704333));
#85887=CARTESIAN_POINT('',(0.0131021943802151,-0.0321934096636182,0.0770271360925871));
#85888=CARTESIAN_POINT('Origin',(0.0151107385009172,-0.0324111866099997,
0.0781636326709294));
#85889=CARTESIAN_POINT('',(0.013133467598636,-0.0321934096636662,0.0769730229166264));
#85890=CARTESIAN_POINT('Ctrl Pts',(0.0131627814793221,-0.0321934096636618,
0.0769194338428291));
#85891=CARTESIAN_POINT('Ctrl Pts',(0.0132009741303853,-0.0320835708272592,
0.0768499421155059));
#85892=CARTESIAN_POINT('Ctrl Pts',(0.0132377065004733,-0.0319739230346489,
0.0767797003012799));
#85893=CARTESIAN_POINT('Ctrl Pts',(0.0132729384903025,-0.0318646057455573,
0.0767088018765306));
#85894=CARTESIAN_POINT('Ctrl Pts',(0.013272251668556,-0.0321934096636618,
0.0768901517248274));
#85895=CARTESIAN_POINT('Ctrl Pts',(0.0133100404963907,-0.0320835708272592,
0.0768191503182785));
#85896=CARTESIAN_POINT('Ctrl Pts',(0.0133463380347512,-0.0319739230346489,
0.0767474080576029));
#85897=CARTESIAN_POINT('Ctrl Pts',(0.0133811048880234,-0.0318646057455573,
0.0766750202961999));
#85898=CARTESIAN_POINT('Ctrl Pts',(0.0133817218577899,-0.0321934096636618,
0.0768608696068256));
#85899=CARTESIAN_POINT('Ctrl Pts',(0.0134191068623962,-0.0320835708272592,
0.0767883585210511));
#85900=CARTESIAN_POINT('Ctrl Pts',(0.0134549695690291,-0.0319739230346489,
0.0767151158139259));
#85901=CARTESIAN_POINT('Ctrl Pts',(0.0134892712857444,-0.0318646057455573,
0.0766412387158692));
#85902=CARTESIAN_POINT('Ctrl Pts',(0.0134911920470238,-0.0321934096636618,
0.0768315874888238));
#85903=CARTESIAN_POINT('Ctrl Pts',(0.0135281732284017,-0.0320835708272592,
0.0767575667238238));
#85904=CARTESIAN_POINT('Ctrl Pts',(0.0135636011033069,-0.0319739230346489,
0.0766828235702489));
#85905=CARTESIAN_POINT('Ctrl Pts',(0.0135974376834654,-0.0318646057455573,
0.0766074571355385));
#85906=CARTESIAN_POINT('',(0.0134969077196753,-0.032176398030832,0.0768201164869055));
#85907=CARTESIAN_POINT('',(0.013491192047025,-0.0321934096636185,0.0768315874887981));
#85908=CARTESIAN_POINT('Origin',(-0.00103868750143187,-0.0326386231233297,
0.0689117309547281));
#85909=CARTESIAN_POINT('Ctrl Pts',(0.0134969077168294,-0.0321763980306362,
0.0768201164854885));
#85910=CARTESIAN_POINT('Ctrl Pts',(0.0134584729499547,-0.0321259596175984,
0.0768010167447148));
#85911=CARTESIAN_POINT('Ctrl Pts',(0.0134207041152833,-0.0320749164633703,
0.0767822479317384));
#85912=CARTESIAN_POINT('Ctrl Pts',(0.013346467914919,-0.0319716057794025,
0.0767453570566718));
#85913=CARTESIAN_POINT('Ctrl Pts',(0.0133100294743802,-0.0319193786690223,
0.0767272493686233));
#85914=CARTESIAN_POINT('Ctrl Pts',(0.0132742440851441,-0.0318665617525436,
0.0767094662073484));
#85915=CARTESIAN_POINT('',(0.0133279664320409,-0.0321934096636663,0.0768752486147319));
#85916=CARTESIAN_POINT('Origin',(0.00812378219310841,-0.0315241814719618,
0.07415));
#85917=CARTESIAN_POINT('',(0.0134969077200062,-0.0322104233323591,0.07682011648707));
#85918=CARTESIAN_POINT('',(0.0135025988803254,-0.0321934096636183,0.0768086333040356));
#85919=CARTESIAN_POINT('Origin',(-0.00106431922441187,-0.0326387244918799,
0.0689491214002542));
#85920=CARTESIAN_POINT('Origin',(-0.00158472984669416,-0.0326386235719424,
0.0700105398946128));
#85921=CARTESIAN_POINT('Origin',(-0.00157040526565379,-0.0326387248819868,
0.0699675304009003));
#85922=CARTESIAN_POINT('Ctrl Pts',(0.0132005149732031,-0.0327445246967096,
0.0768527595674627));
#85923=CARTESIAN_POINT('Ctrl Pts',(0.0133024512167218,-0.032443687833936,
0.0766612874605166));
#85924=CARTESIAN_POINT('Ctrl Pts',(0.0133896754084872,-0.0321434074405928,
0.0764626810511237));
#85925=CARTESIAN_POINT('Ctrl Pts',(0.013313174592781,-0.0327445246967096,
0.07662958293312));
#85926=CARTESIAN_POINT('Ctrl Pts',(0.0134066935919321,-0.032443687833936,
0.0764338617991594));
#85927=CARTESIAN_POINT('Ctrl Pts',(0.0134852043977516,-0.0321434074405928,
0.0762316524550363));
#85928=CARTESIAN_POINT('',(0.0133286549178122,-0.0326943950436612,0.0765969215188958));
#85929=CARTESIAN_POINT('',(0.013424791040563,-0.0323666188837389,0.0763810155085093));
#85930=CARTESIAN_POINT('Origin',(-0.00191712637556098,-0.0326395579112203,
0.0695135458424481));
#85931=CARTESIAN_POINT('Origin',(0.0236045717473434,-0.0321933825603084,
0.080665340028318));
#85932=CARTESIAN_POINT('',(0.0133750499992974,-0.0321934096532689,0.0764957006255223));
#85933=CARTESIAN_POINT('',(0.013399294441097,-0.0321934096584275,0.0764380945721288));
#85934=CARTESIAN_POINT('',(0.0132742440876436,-0.0325210109756239,0.0767094662085955));
#85935=CARTESIAN_POINT('Origin',(-0.00168988315583584,-0.0326393129156433,
0.0690898183963548));
#85936=CARTESIAN_POINT('',(0.0132730274909841,-0.0326943950436593,0.0767088616340681));
#85937=CARTESIAN_POINT('Origin',(0.0231796872344863,-0.0326943765538153,
0.0816318698022489));
#85938=CARTESIAN_POINT('',(0.0133008412044081,-0.0326943950436702,0.076652891576492));
#85939=CARTESIAN_POINT('Ctrl Pts',(0.0133881187017994,-0.0325229783203769,
0.0770286735006535));
#85940=CARTESIAN_POINT('Ctrl Pts',(0.0134278011530535,-0.032413025309245,
0.0769561047370046));
#85941=CARTESIAN_POINT('Ctrl Pts',(0.0134659764075891,-0.0323031222208069,
0.0768827260973508));
#85942=CARTESIAN_POINT('Ctrl Pts',(0.0135025988823162,-0.0321934096576658,
0.0768086333000249));
#85943=CARTESIAN_POINT('Ctrl Pts',(0.0133497209623862,-0.0325229783203769,
0.0769220585118155));
#85944=CARTESIAN_POINT('Ctrl Pts',(0.0133879337283506,-0.032413025309245,
0.0768500190601648));
#85945=CARTESIAN_POINT('Ctrl Pts',(0.0134246504700018,-0.0323031222208069,
0.0767772000545567));
#85946=CARTESIAN_POINT('Ctrl Pts',(0.0134598274472057,-0.0321934096576658,
0.0767036964305483));
#85947=CARTESIAN_POINT('Ctrl Pts',(0.0133113232229729,-0.0325229783203769,
0.0768154435229776));
#85948=CARTESIAN_POINT('Ctrl Pts',(0.0133480663036478,-0.032413025309245,
0.076743933383325));
#85949=CARTESIAN_POINT('Ctrl Pts',(0.0133833245324145,-0.0323031222208069,
0.0766716740117626));
#85950=CARTESIAN_POINT('Ctrl Pts',(0.0134170560120952,-0.0321934096576658,
0.0765987595610717));
#85951=CARTESIAN_POINT('Ctrl Pts',(0.0132729254835597,-0.0325229783203769,
0.0767088285341397));
#85952=CARTESIAN_POINT('Ctrl Pts',(0.0133081988789449,-0.032413025309245,
0.0766378477064852));
#85953=CARTESIAN_POINT('Ctrl Pts',(0.0133419985948273,-0.0323031222208069,
0.0765661479689685));
#85954=CARTESIAN_POINT('Ctrl Pts',(0.0133742845769847,-0.0321934096576658,
0.0764938226915951));
#85955=CARTESIAN_POINT('',(0.0134388244397454,-0.0321934096584275,0.0766521669652904));
#85956=CARTESIAN_POINT('Ctrl Pts',(0.0134969077168855,-0.032210423332889,
0.0768201164855165));
#85957=CARTESIAN_POINT('Ctrl Pts',(0.0134584208702708,-0.0322609421830388,
0.0768009908642805));
#85958=CARTESIAN_POINT('Ctrl Pts',(0.0134206265937799,-0.0323120888238748,
0.0767822094082601));
#85959=CARTESIAN_POINT('Ctrl Pts',(0.0133463898313685,-0.0324156524631808,
0.0767453182538903));
#85960=CARTESIAN_POINT('Ctrl Pts',(0.0133099778608568,-0.032468026716732,
0.0767272237198424));
#85961=CARTESIAN_POINT('Ctrl Pts',(0.0132742440876067,-0.0325210109755912,
0.0767094662085722));
#85962=CARTESIAN_POINT('Origin',(0.00379934591254904,-0.0262834582510528,
0.080722871267367));
#85963=CARTESIAN_POINT('Origin',(0.015440934589309,-0.0342771100866737,
0.083860041158149));
#85964=CARTESIAN_POINT('Ctrl Pts',(0.013326732821639,-0.0326943950436603,
0.0765975674578511));
#85965=CARTESIAN_POINT('Ctrl Pts',(0.0133604648884385,-0.0325844576448133,
0.0765258610468212));
#85966=CARTESIAN_POINT('Ctrl Pts',(0.0133927163363644,-0.0324744968375322,
0.0764534519265712));
#85967=CARTESIAN_POINT('Ctrl Pts',(0.0134234471226241,-0.0323646534831894,
0.0763804334418495));
#85968=CARTESIAN_POINT('Ctrl Pts',(0.0134341482015404,-0.0326943950436603,
0.076561469483628));
#85969=CARTESIAN_POINT('Ctrl Pts',(0.0134673827706003,-0.0325844576448133,
0.0764882826873452));
#85970=CARTESIAN_POINT('Ctrl Pts',(0.0134991060687837,-0.0324744968375322,
0.0764144033661421));
#85971=CARTESIAN_POINT('Ctrl Pts',(0.0135292787559763,-0.0323646534831894,
0.0763399267391404));
#85972=CARTESIAN_POINT('Ctrl Pts',(0.0135415635814418,-0.0326943950436603,
0.0765253715094049));
#85973=CARTESIAN_POINT('Ctrl Pts',(0.013574300652762,-0.0325844576448133,
0.0764507043278692));
#85974=CARTESIAN_POINT('Ctrl Pts',(0.013605495801203,-0.0324744968375322,
0.0763753548057129));
#85975=CARTESIAN_POINT('Ctrl Pts',(0.0136351103893286,-0.0323646534831894,
0.0762994200364314));
#85976=CARTESIAN_POINT('Ctrl Pts',(0.0136489789613431,-0.0326943950436603,
0.0764892735351818));
#85977=CARTESIAN_POINT('Ctrl Pts',(0.0136812185349238,-0.0325844576448133,
0.0764131259683932));
#85978=CARTESIAN_POINT('Ctrl Pts',(0.0137118855336223,-0.0324744968375322,
0.0763363062452838));
#85979=CARTESIAN_POINT('Ctrl Pts',(0.0137409420226808,-0.0323646534831894,
0.0762589133337223));
#85980=CARTESIAN_POINT('',(0.0136539630854264,-0.0326773559991209,0.0764774662787185));
#85981=CARTESIAN_POINT('',(0.0136489789613314,-0.0326943950436594,0.0764892735351852));
#85982=CARTESIAN_POINT('Origin',(-0.00167043362836957,-0.0326395670146922,
0.0700824545246432));
#85983=CARTESIAN_POINT('Ctrl Pts',(0.0136539630823324,-0.0326773559987497,
0.0764774662774134));
#85984=CARTESIAN_POINT('Ctrl Pts',(0.0136143730414135,-0.0326267922588807,
0.0764608041668955));
#85985=CARTESIAN_POINT('Ctrl Pts',(0.013575484705366,-0.0325756109585183,
0.0764444373802571));
#85986=CARTESIAN_POINT('Ctrl Pts',(0.0134990783461931,-0.0324719985460573,
0.0764122805253699));
#85987=CARTESIAN_POINT('Ctrl Pts',(0.0134615909682089,-0.0324196091617922,
0.0763965033546255));
#85988=CARTESIAN_POINT('Ctrl Pts',(0.0134247910405181,-0.0323666188837756,
0.0763810155084904));
#85989=CARTESIAN_POINT('',(0.0134888169395818,-0.0326943950436703,0.0765430975270505));
#85990=CARTESIAN_POINT('Origin',(0.00812378219310841,-0.0315241814719618,
0.07415));
#85991=CARTESIAN_POINT('',(0.0136539630853841,-0.0327114338379849,0.076477466278701));
#85992=CARTESIAN_POINT('',(0.0136589219806651,-0.0326943950436593,0.0764656484042732));
#85993=CARTESIAN_POINT('Origin',(-0.00168729056429505,-0.0326395680341498,
0.0701245113554134));
#85994=CARTESIAN_POINT('Origin',(-0.00163145640073906,-0.0326395673206855,
0.0699898411083458));
#85995=CARTESIAN_POINT('Origin',(-0.00161316525169613,-0.0326395684286114,
0.0699483880173138));
#85996=CARTESIAN_POINT('Ctrl Pts',(0.0133602211002138,-0.0332451089994433,
0.0765286198881184));
#85997=CARTESIAN_POINT('Ctrl Pts',(0.0134499322170449,-0.0329451141710254,
0.076331124363541));
#85998=CARTESIAN_POINT('Ctrl Pts',(0.0135245123037821,-0.0326442513127494,
0.0761274324948434));
#85999=CARTESIAN_POINT('Ctrl Pts',(0.0134586434676643,-0.0332451089994433,
0.0762988090146041));
#86000=CARTESIAN_POINT('Ctrl Pts',(0.0135396871255938,-0.0329451141710254,
0.0760976014297058));
#86001=CARTESIAN_POINT('Ctrl Pts',(0.0136053447692069,-0.0326442513127494,
0.0758908609146963));
#86002=CARTESIAN_POINT('Ctrl Pts',(0.0134596276913388,-0.0332451089994433,
0.076296510905869));
#86003=CARTESIAN_POINT('Ctrl Pts',(0.0135405846746793,-0.0329451141710254,
0.0760952662003675));
#86004=CARTESIAN_POINT('Ctrl Pts',(0.0136061530938611,-0.0326442513127494,
0.0758884951988948));
#86005=CARTESIAN_POINT('',(0.0134720277638493,-0.0331951640388616,0.0762652764157555));
#86006=CARTESIAN_POINT('',(0.013554417343685,-0.0328677532355043,0.0760437599983026));
#86007=CARTESIAN_POINT('Origin',(-0.00238308537357132,-0.0326402808283806,
0.0708203122407319));
#86008=CARTESIAN_POINT('Origin',(0.0239939736023976,-0.0326944278779173,
0.0796838215450741));
#86009=CARTESIAN_POINT('',(0.0135119755852948,-0.0326943950436593,0.0761613420813975));
#86010=CARTESIAN_POINT('',(0.0135325550709807,-0.0326943950436694,0.0761023273818038));
#86011=CARTESIAN_POINT('',(0.0134247910405619,-0.0330220786163545,0.0763810155085119));
#86012=CARTESIAN_POINT('Origin',(-0.00225478128003319,-0.0326396682762709,
0.0703569649581177));
#86013=CARTESIAN_POINT('',(0.0134235388830287,-0.0331951640388587,0.0763804885177121));
#86014=CARTESIAN_POINT('Origin',(0.023591378025755,-0.0331952026560144,
0.080659789479558));
#86015=CARTESIAN_POINT('',(0.013447783323449,-0.0331951640388701,0.0763228824667439));
#86016=CARTESIAN_POINT('Ctrl Pts',(0.0135584845480517,-0.0330240426238172,
0.0766924418013544));
#86017=CARTESIAN_POINT('Ctrl Pts',(0.0135935091608463,-0.032914277406352,
0.0766175734816411));
#86018=CARTESIAN_POINT('Ctrl Pts',(0.013627003497385,-0.0328043479726691,
0.0765419437807571));
#86019=CARTESIAN_POINT('Ctrl Pts',(0.0136589219806696,-0.0326943950436593,
0.0764656484042827));
#86020=CARTESIAN_POINT('Ctrl Pts',(0.0135134681615712,-0.0330240426238172,
0.0765884482393739));
#86021=CARTESIAN_POINT('Ctrl Pts',(0.0135470601617336,-0.032914277406352,
0.0765142000642417));
#86022=CARTESIAN_POINT('Ctrl Pts',(0.0135791339915511,-0.0328043479726691,
0.0764392204332085));
#86023=CARTESIAN_POINT('Ctrl Pts',(0.0136096459167354,-0.0326943950436593,
0.0763636042691828));
#86024=CARTESIAN_POINT('Ctrl Pts',(0.0134684517750907,-0.0330240426238172,
0.0764844546773935));
#86025=CARTESIAN_POINT('Ctrl Pts',(0.0135006111626208,-0.032914277406352,
0.0764108266468424));
#86026=CARTESIAN_POINT('Ctrl Pts',(0.0135312644857172,-0.0328043479726691,
0.0763364970856598));
#86027=CARTESIAN_POINT('Ctrl Pts',(0.0135603698528012,-0.0326943950436593,
0.0762615601340828));
#86028=CARTESIAN_POINT('Ctrl Pts',(0.0134234353886103,-0.0330240426238172,
0.076380461115413));
#86029=CARTESIAN_POINT('Ctrl Pts',(0.0134541621635081,-0.032914277406352,
0.0763074532294431));
#86030=CARTESIAN_POINT('Ctrl Pts',(0.0134833949798833,-0.0328043479726691,
0.0762337737381112));
#86031=CARTESIAN_POINT('Ctrl Pts',(0.013511093788867,-0.0326943950436593,
0.0761595159989829));
#86032=CARTESIAN_POINT('',(0.0135854487829899,-0.0326943950436693,0.0763134952428454));
#86033=CARTESIAN_POINT('Ctrl Pts',(0.0136539630823231,-0.0327114338383285,
0.0764774662774096));
#86034=CARTESIAN_POINT('Ctrl Pts',(0.0136143796263787,-0.0327619876830041,
0.0764608069382849));
#86035=CARTESIAN_POINT('Ctrl Pts',(0.0135754945066797,-0.0328131562602455,
0.07644444150529));
#86036=CARTESIAN_POINT('Ctrl Pts',(0.0134990882181012,-0.0329167375858761,
0.0764122846801135));
#86037=CARTESIAN_POINT('Ctrl Pts',(0.0134615974936266,-0.0329691088920614,
0.0763965061009534));
#86038=CARTESIAN_POINT('Ctrl Pts',(0.0134247910405192,-0.0330220786163187,
0.0763810155084909));
#86039=CARTESIAN_POINT('Ctrl Pts',(0.0134701497195573,-0.0331951640388604,
0.0762660418917036));
#86040=CARTESIAN_POINT('Ctrl Pts',(0.0135138975289884,-0.0330306422010619,
0.0761555091708662));
#86041=CARTESIAN_POINT('Ctrl Pts',(0.0135530395226318,-0.0328657861914645,
0.0760432627564943));
#86042=CARTESIAN_POINT('Ctrl Pts',(0.0134720277638481,-0.0331951640388604,
0.0762652764157584));
#86043=CARTESIAN_POINT('Ctrl Pts',(0.0135157597475548,-0.0330306422010619,
0.0761547048675594));
#86044=CARTESIAN_POINT('Ctrl Pts',(0.013554884324221,-0.0328657861914645,
0.0760424203130974));
#86045=CARTESIAN_POINT('Ctrl Pts',(0.0137849604482271,-0.0331951640388604,
0.0761377275376377));
#86046=CARTESIAN_POINT('Ctrl Pts',(0.0138260554406554,-0.0330306422010619,
0.0760206863068229));
#86047=CARTESIAN_POINT('Ctrl Pts',(0.0138622778805476,-0.0328657861914645,
0.0759020465876663));
#86048=CARTESIAN_POINT('',(0.0137891933545318,-0.0331781648281955,0.0761256306253974));
#86049=CARTESIAN_POINT('',(0.0137849604482159,-0.0331951640388588,0.0761377275376413));
#86050=CARTESIAN_POINT('Origin',(-0.00203177214281177,-0.0326412091605797,
0.0713629073520702));
#86051=CARTESIAN_POINT('Ctrl Pts',(0.0137891933530245,-0.033178164828644,
0.0761256306264603));
#86052=CARTESIAN_POINT('Ctrl Pts',(0.0137486072846126,-0.0331276811546759,
0.0761114775482818));
#86053=CARTESIAN_POINT('Ctrl Pts',(0.0137087540637734,-0.0330765663497757,
0.0760975800627967));
#86054=CARTESIAN_POINT('Ctrl Pts',(0.0136304791297395,-0.0329730614463427,
0.0760702841837328));
#86055=CARTESIAN_POINT('Ctrl Pts',(0.0135920890396722,-0.0329207133374321,
0.0760568968120312));
#86056=CARTESIAN_POINT('Ctrl Pts',(0.0135544173473107,-0.0328677532289397,
0.0760437600143701));
#86057=CARTESIAN_POINT('',(0.0136284941060426,-0.0331951640388701,0.0762015019767084));
#86058=CARTESIAN_POINT('Origin',(0.00812378219310841,-0.0315241814719618,
0.07415));
#86059=CARTESIAN_POINT('',(0.0137891933532789,-0.0332121607144397,0.0761256306242759));
#86060=CARTESIAN_POINT('',(0.0137934004130283,-0.0331951640388587,0.0761135246981789));
#86061=CARTESIAN_POINT('Origin',(-0.00203907066499096,-0.0326413666255414,
0.0714076603317704));
#86062=CARTESIAN_POINT('Origin',(-0.00156271436733097,-0.0326412093978695,
0.0700178134636139));
#86063=CARTESIAN_POINT('Origin',(-0.00154060066727734,-0.0326413667802714,
0.0699782266867448));
#86064=CARTESIAN_POINT('Ctrl Pts',(0.0134992355551813,-0.0337436976235975,
0.0761951469756912));
#86065=CARTESIAN_POINT('Ctrl Pts',(0.0135176299170312,-0.0336723290703325,
0.0761467993334805));
#86066=CARTESIAN_POINT('Ctrl Pts',(0.0135351516814119,-0.033601104548885,
0.0760981286561872));
#86067=CARTESIAN_POINT('Ctrl Pts',(0.0135910952042136,-0.0333736987606857,
0.0759427328247077));
#86068=CARTESIAN_POINT('Ctrl Pts',(0.0136380290277007,-0.0331450831799192,
0.075784382711359));
#86069=CARTESIAN_POINT('Ctrl Pts',(0.0135830346175524,-0.0337436976235975,
0.0759596098933756));
#86070=CARTESIAN_POINT('Ctrl Pts',(0.0135993105231873,-0.0336723290703325,
0.0759105085496979));
#86071=CARTESIAN_POINT('Ctrl Pts',(0.0136147006173555,-0.033601104548885,
0.0758611223972187));
#86072=CARTESIAN_POINT('Ctrl Pts',(0.013663838139429,-0.0333736987606857,
0.0757034421951985));
#86073=CARTESIAN_POINT('Ctrl Pts',(0.0137038460875853,-0.0331450831799192,
0.0755432020433358));
#86074=CARTESIAN_POINT('Ctrl Pts',(0.0135838726081761,-0.0337436976235975,
0.0759572545225524));
#86075=CARTESIAN_POINT('Ctrl Pts',(0.0136001273292488,-0.0336723290703325,
0.0759081456418601));
#86076=CARTESIAN_POINT('Ctrl Pts',(0.013615496106715,-0.033601104548885,
0.075858752334629));
#86077=CARTESIAN_POINT('Ctrl Pts',(0.0136645655687811,-0.0333736987606857,
0.0757010492889033));
#86078=CARTESIAN_POINT('Ctrl Pts',(0.0137045042581842,-0.0331450831799192,
0.0755407902366555));
#86079=CARTESIAN_POINT('',(0.0135942935280036,-0.0336938721132548,0.0759252832829675));
#86080=CARTESIAN_POINT('',(0.0136626113922525,-0.0333679869945434,0.07569903069784));
#86081=CARTESIAN_POINT('Ctrl Pts',(0.0135942935280024,-0.033693872113265,
0.0759252832829736));
#86082=CARTESIAN_POINT('Ctrl Pts',(0.0136012232914556,-0.0336629187933933,
0.0759039293109708));
#86083=CARTESIAN_POINT('Ctrl Pts',(0.0136080258025137,-0.0336319952301041,
0.0758825415919257));
#86084=CARTESIAN_POINT('Ctrl Pts',(0.0136147006173536,-0.0336011045488951,
0.0758611223972248));
#86085=CARTESIAN_POINT('Ctrl Pts',(0.0136314500117803,-0.0335235892595455,
0.0758073743084842));
#86086=CARTESIAN_POINT('Ctrl Pts',(0.0136474249484776,-0.033445866866037,
0.0757533324743409));
#86087=CARTESIAN_POINT('Ctrl Pts',(0.0136626113925438,-0.0333679869945386,
0.0756990306979284));
#86088=CARTESIAN_POINT('Ctrl Pts',(0.0136626240317451,-0.0333679692459663,
0.0756989880561563));
#86089=CARTESIAN_POINT('Ctrl Pts',(0.013662185969107,-0.0333391895373257,
0.0756988716991663));
#86090=CARTESIAN_POINT('Ctrl Pts',(0.0136618567861838,-0.0333104081057764,
0.0756987876222839));
#86091=CARTESIAN_POINT('Ctrl Pts',(0.0136614196850596,-0.0332532697346145,
0.0756986816981781));
#86092=CARTESIAN_POINT('Ctrl Pts',(0.0136613085378268,-0.0332249166877988,
0.0756986589465388));
#86093=CARTESIAN_POINT('Ctrl Pts',(0.01366130314572,-0.0331960985544231,
0.075698664599457));
#86094=CARTESIAN_POINT('Ctrl Pts',(0.0136613030868818,-0.033195631237939,
0.0756986646993534));
#86095=CARTESIAN_POINT('Ctrl Pts',(0.0136613030569208,-0.0331951640388594,
0.0756986648064842));
#86096=CARTESIAN_POINT('',(0.0136276364306931,-0.0331951640388587,0.0758190456948274));
#86097=CARTESIAN_POINT('',(0.013644469743817,-0.0331951640388688,0.0757588552506657));
#86098=CARTESIAN_POINT('',(0.0135544173329402,-0.0335216366567652,0.0760437600095019));
#86099=CARTESIAN_POINT('Origin',(-0.00252841005498943,-0.0326434571526939,
0.0717178695547645));
#86100=CARTESIAN_POINT('',(0.0135531345566467,-0.0336938721132327,0.0760433126821901));
#86101=CARTESIAN_POINT('Origin',(0.0238647199702471,-0.0336938867896168,
0.0796391486340378));
#86102=CARTESIAN_POINT('',(0.0135737140423351,-0.0336938721132538,0.0759842979825888));
#86103=CARTESIAN_POINT('Ctrl Pts',(0.0137074019977526,-0.0335235895815172,
0.0763461761944996));
#86104=CARTESIAN_POINT('Ctrl Pts',(0.0137376366869429,-0.0334144449262749,
0.0762693066747529));
#86105=CARTESIAN_POINT('Ctrl Pts',(0.0137663180457009,-0.0333049234473147,
0.0761917242153164));
#86106=CARTESIAN_POINT('Ctrl Pts',(0.0137934004130336,-0.0331951640388587,
0.0761135246981882));
#86107=CARTESIAN_POINT('Ctrl Pts',(0.0136559445417368,-0.0335235895815172,
0.0762452143071017));
#86108=CARTESIAN_POINT('Ctrl Pts',(0.0136847892917715,-0.0334144449262749,
0.0761690532005474));
#86109=CARTESIAN_POINT('Ctrl Pts',(0.0137120937497854,-0.0333049234473147,
0.0760922086832813));
#86110=CARTESIAN_POINT('Ctrl Pts',(0.0137378141008947,-0.0331951640388587,
0.0760147758531855));
#86111=CARTESIAN_POINT('Ctrl Pts',(0.013604487085721,-0.0335235895815172,
0.0761442524197038));
#86112=CARTESIAN_POINT('Ctrl Pts',(0.0136319418966,-0.0334144449262749,
0.076068799726342));
#86113=CARTESIAN_POINT('Ctrl Pts',(0.01365786945387,-0.0333049234473147,
0.0759926931512462));
#86114=CARTESIAN_POINT('Ctrl Pts',(0.0136822277887558,-0.0331951640388587,
0.0759160270081828));
#86115=CARTESIAN_POINT('Ctrl Pts',(0.0135530296297052,-0.0335235895815172,
0.0760432905323059));
#86116=CARTESIAN_POINT('Ctrl Pts',(0.0135790945014285,-0.0334144449262749,
0.0759685462521365));
#86117=CARTESIAN_POINT('Ctrl Pts',(0.0136036451579545,-0.0333049234473147,
0.075893177619211));
#86118=CARTESIAN_POINT('Ctrl Pts',(0.0136266414766169,-0.0331951640388587,
0.0758172781631801));
#86119=CARTESIAN_POINT('',(0.0137105184218707,-0.0331951640388687,0.0759662851965132));
#86120=CARTESIAN_POINT('Ctrl Pts',(0.013789193350316,-0.0332121607145939,
0.0761256306232392));
#86121=CARTESIAN_POINT('Ctrl Pts',(0.0137486755620964,-0.033262544410879,
0.0761115013427737));
#86122=CARTESIAN_POINT('Ctrl Pts',(0.0137088559589482,-0.033313530074487,
0.0760976155319822));
#86123=CARTESIAN_POINT('Ctrl Pts',(0.0136305815142302,-0.0334167203140537,
0.0760703198272733));
#86124=CARTESIAN_POINT('Ctrl Pts',(0.0135921569892141,-0.0334688847587207,
0.0760569205052826));
#86125=CARTESIAN_POINT('Ctrl Pts',(0.013554417332325,-0.0335216366562267,
0.0760437600091083));
#86126=CARTESIAN_POINT('Ctrl Pts',(0.0135933931509884,-0.0336938721132389,
0.0759257180657895));
#86127=CARTESIAN_POINT('Ctrl Pts',(0.0136037870180731,-0.0336474569764957,
0.0758937026178437));
#86128=CARTESIAN_POINT('Ctrl Pts',(0.0136138053917227,-0.033601104548885,
0.0758615676902795));
#86129=CARTESIAN_POINT('Ctrl Pts',(0.0136391696104349,-0.0334837508592656,
0.0757802094419696));
#86130=CARTESIAN_POINT('Ctrl Pts',(0.0136621118774707,-0.0333660264659097,
0.0756981353258173));
#86131=CARTESIAN_POINT('Ctrl Pts',(0.0135942935279973,-0.0336938721132389,
0.0759252832829869));
#86132=CARTESIAN_POINT('Ctrl Pts',(0.013604684850154,-0.0336474569764957,
0.0758932625648357));
#86133=CARTESIAN_POINT('Ctrl Pts',(0.0136147006173555,-0.033601104548885,
0.0758611223972187));
#86134=CARTESIAN_POINT('Ctrl Pts',(0.0136400582371406,-0.0334837508592656,
0.0757797508823002));
#86135=CARTESIAN_POINT('Ctrl Pts',(0.0136629935150297,-0.0333660264659097,
0.0756976637009048));
#86136=CARTESIAN_POINT('Ctrl Pts',(0.0139004256888299,-0.0336938721132389,
0.0757774552092352));
#86137=CARTESIAN_POINT('Ctrl Pts',(0.0139099517242165,-0.0336474569764957,
0.0757436425979612));
#86138=CARTESIAN_POINT('Ctrl Pts',(0.0139190812875663,-0.033601104548885,
0.0757097207892773));
#86139=CARTESIAN_POINT('Ctrl Pts',(0.01394219524295,-0.0334837508592656,
0.0756238385688022));
#86140=CARTESIAN_POINT('Ctrl Pts',(0.013962754180132,-0.0333660264659097,
0.0755373091470478));
#86141=CARTESIAN_POINT('',(0.0139020648336084,-0.0336769361243753,0.0757659980589394));
#86142=CARTESIAN_POINT('',(0.0138985998508737,-0.033693872113232,0.0757783368876132));
#86143=CARTESIAN_POINT('Ctrl Pts',(0.0139020648336085,-0.0336769361243753,
0.0757659980589393));
#86144=CARTESIAN_POINT('Ctrl Pts',(0.0139014894897374,-0.0336797586669941,
0.0757680553012016));
#86145=CARTESIAN_POINT('Ctrl Pts',(0.0139009130689664,-0.0336825812712675,
0.0757701121583982));
#86146=CARTESIAN_POINT('Ctrl Pts',(0.0138997580762776,-0.0336882265924994,
0.0757742250951142));
#86147=CARTESIAN_POINT('Ctrl Pts',(0.0138991795043904,-0.033691049309423,
0.0757762811746089));
#86148=CARTESIAN_POINT('Ctrl Pts',(0.0138985998508829,-0.033693872113236,
0.0757783368876103));
#86149=CARTESIAN_POINT('Ctrl Pts',(0.0139020648336084,-0.0336769361243753,
0.0757659980589394));
#86150=CARTESIAN_POINT('Ctrl Pts',(0.0138616988599108,-0.0336278994719898,
0.0757547090066031));
#86151=CARTESIAN_POINT('Ctrl Pts',(0.0138207581875897,-0.0335767852743495,
0.0757432592297203));
#86152=CARTESIAN_POINT('Ctrl Pts',(0.0137405280206276,-0.0334733172064609,
0.0757208214567442));
#86153=CARTESIAN_POINT('Ctrl Pts',(0.0137011907099758,-0.0334209631456226,
0.075709820088065));
#86154=CARTESIAN_POINT('Ctrl Pts',(0.0136626113902799,-0.0333679869844681,
0.0756990307048481));
#86155=CARTESIAN_POINT('',(0.0137464466894487,-0.0336938721132534,0.0758518100853004));
#86156=CARTESIAN_POINT('Origin',(0.00812378219310841,-0.0315241814719618,
0.07415));
#86157=CARTESIAN_POINT('',(0.0139020648323678,-0.0337108120655378,0.0757659980585962));
#86158=CARTESIAN_POINT('',(0.0139055034524797,-0.0336938721132327,0.07575365185715));
#86159=CARTESIAN_POINT('Origin',(-0.00155354328806278,-0.0345562524833384,
0.0702830764010626));
#86160=CARTESIAN_POINT('Ctrl Pts',(0.0139055034524908,-0.0336938721132385,
0.0757536518571611));
#86161=CARTESIAN_POINT('Ctrl Pts',(0.013904932583456,-0.0336910492952032,
0.0757557100380685));
#86162=CARTESIAN_POINT('Ctrl Pts',(0.0139043606039045,-0.033688226585389,
0.0757577679556348));
#86163=CARTESIAN_POINT('Ctrl Pts',(0.0139032144009328,-0.0336825812712763,
0.0757618833449552));
#86164=CARTESIAN_POINT('Ctrl Pts',(0.0139026401774804,-0.0336797586669984,
0.075763940816674));
#86165=CARTESIAN_POINT('Ctrl Pts',(0.0139020648336084,-0.033676936124375,
0.0757659980589397));
#86166=CARTESIAN_POINT('Origin',(-0.00215555888469551,-0.0345562520271967,
0.0724356912422816));
#86167=CARTESIAN_POINT('Ctrl Pts',(0.0136170288714271,-0.0342436276873911,
0.0758536331562695));
#86168=CARTESIAN_POINT('Ctrl Pts',(0.0136812824551496,-0.0339430054201811,
0.0756464519423711));
#86169=CARTESIAN_POINT('Ctrl Pts',(0.0137297477632473,-0.0336441434784052,
0.0754350194653847));
#86170=CARTESIAN_POINT('Ctrl Pts',(0.0136858752375207,-0.0342436276873911,
0.0756132996840362));
#86171=CARTESIAN_POINT('Ctrl Pts',(0.0137410644949106,-0.0339430054201811,
0.0754035218866354));
#86172=CARTESIAN_POINT('Ctrl Pts',(0.013780295642168,-0.0336441434784052,
0.0751901829649674));
#86173=CARTESIAN_POINT('Ctrl Pts',(0.0136865637011816,-0.0342436276873911,
0.0756108963493139));
#86174=CARTESIAN_POINT('Ctrl Pts',(0.0137416623153082,-0.0339430054201811,
0.075401092586078));
#86175=CARTESIAN_POINT('Ctrl Pts',(0.0137808011209572,-0.0336441434784052,
0.0751877345999632));
#86176=CARTESIAN_POINT('',(0.0136949696831489,-0.0341934961088741,0.0755782839181398));
#86177=CARTESIAN_POINT('',(0.0137489462195366,-0.0338664212863854,0.0753481880820869));
#86178=CARTESIAN_POINT('Origin',(-0.00238150079543393,-0.034561072040523,
0.0709306780062336));
#86179=CARTESIAN_POINT('Origin',(0.024474590049207,-0.0336938005073029,
0.0776327643813499));
#86180=CARTESIAN_POINT('',(0.0137215760778875,-0.0336938721132327,0.0754701623474144));
#86181=CARTESIAN_POINT('',(0.013734596785053,-0.0336938721132427,0.075409033702869));
#86182=CARTESIAN_POINT('',(0.0136626113902784,-0.0340203938281605,0.0756990307048533));
#86183=CARTESIAN_POINT('Origin',(-0.00217820120041667,-0.0345589643244919,
0.0704945518675342));
#86184=CARTESIAN_POINT('',(0.013661303056921,-0.0341934961088741,0.0756986648064836));
#86185=CARTESIAN_POINT('Origin',(0.0242735496589752,-0.0341934220717668,
0.0786665664771319));
#86186=CARTESIAN_POINT('',(0.013678136370045,-0.0341934961088841,0.0756384743623218));
#86187=CARTESIAN_POINT('Ctrl Pts',(0.0138342822040808,-0.0340223579322396,
0.0759912467582561));
#86188=CARTESIAN_POINT('Ctrl Pts',(0.0138596777990503,-0.0339125849573575,
0.0759124840694955));
#86189=CARTESIAN_POINT('Ctrl Pts',(0.0138834253441911,-0.0338030433565231,
0.0758332510965597));
#86190=CARTESIAN_POINT('Ctrl Pts',(0.0139055034524856,-0.0336938721132327,
0.0757536518571592));
#86191=CARTESIAN_POINT('Ctrl Pts',(0.0137765868662166,-0.0340223579322396,
0.075893715082275));
#86192=CARTESIAN_POINT('Ctrl Pts',(0.013800637245001,-0.0339125849573575,
0.0758157481626994));
#86193=CARTESIAN_POINT('Ctrl Pts',(0.0138230569897976,-0.0338030433565231,
0.0757373382426199));
#86194=CARTESIAN_POINT('Ctrl Pts',(0.0138438263183178,-0.0336938721132327,
0.0756585881366776));
#86195=CARTESIAN_POINT('Ctrl Pts',(0.0137188915283524,-0.0340223579322396,
0.075796183406294));
#86196=CARTESIAN_POINT('Ctrl Pts',(0.0137415966909517,-0.0339125849573575,
0.0757190122559032));
#86197=CARTESIAN_POINT('Ctrl Pts',(0.0137626886354041,-0.0338030433565231,
0.07564142538868));
#86198=CARTESIAN_POINT('Ctrl Pts',(0.01378214918415,-0.0336938721132327,
0.0755635244161961));
#86199=CARTESIAN_POINT('Ctrl Pts',(0.0136611961904882,-0.0340223579322396,
0.0756986517303129));
#86200=CARTESIAN_POINT('Ctrl Pts',(0.0136825561369025,-0.0339125849573575,
0.0756222763491071));
#86201=CARTESIAN_POINT('Ctrl Pts',(0.0137023202810106,-0.0338030433565231,
0.0755455125347402));
#86202=CARTESIAN_POINT('Ctrl Pts',(0.0137204720499822,-0.0336938721132327,
0.0754684606957146));
#86203=CARTESIAN_POINT('',(0.0138135397651936,-0.0336938721132427,0.0756119071022923));
#86204=CARTESIAN_POINT('Ctrl Pts',(0.0139020648288926,-0.0337108120662651,
0.0757659980576206));
#86205=CARTESIAN_POINT('Ctrl Pts',(0.0138606545197245,-0.0337611408993388,
0.0757544169385582));
#86206=CARTESIAN_POINT('Ctrl Pts',(0.0138199998568237,-0.0338121088779471,
0.0757430471492243));
#86207=CARTESIAN_POINT('Ctrl Pts',(0.0137401647875367,-0.0339153382773231,
0.0757207198722408));
#86208=CARTESIAN_POINT('Ctrl Pts',(0.0137010181564829,-0.0339675558473108,
0.0757097718304552));
#86209=CARTESIAN_POINT('Ctrl Pts',(0.0136626113902414,-0.0340203938281304,
0.0756990307048375));
#86210=CARTESIAN_POINT('Ctrl Pts',(0.0136932023061429,-0.0341934961088741,
0.0755792787851676));
#86211=CARTESIAN_POINT('Ctrl Pts',(0.0137227515190235,-0.0340287516182428,
0.0754641354119857));
#86212=CARTESIAN_POINT('Ctrl Pts',(0.0137475165196988,-0.0338644633275951,
0.075347869135228));
#86213=CARTESIAN_POINT('Ctrl Pts',(0.0136949696831488,-0.0341934961088741,
0.0755782839181399));
#86214=CARTESIAN_POINT('Ctrl Pts',(0.0137244983279374,-0.0340287516182428,
0.0754631040058308));
#86215=CARTESIAN_POINT('Ctrl Pts',(0.0137492412679059,-0.0338644633275951,
0.0753468020712627));
#86216=CARTESIAN_POINT('Ctrl Pts',(0.0139894486865093,-0.0341934961088741,
0.0754125199357997));
#86217=CARTESIAN_POINT('Ctrl Pts',(0.0140155502915538,-0.0340287516182428,
0.0752912519020902));
#86218=CARTESIAN_POINT('Ctrl Pts',(0.0140366174934418,-0.0338644633275951,
0.0751690086904575));
#86219=CARTESIAN_POINT('',(0.0139921320694915,-0.0341764758832442,0.0753999878875921));
#86220=CARTESIAN_POINT('',(0.0139894486864998,-0.034193496108874,0.075412519935805));
#86221=CARTESIAN_POINT('Origin',(-0.00209562656239066,-0.0345621027449978,
0.0714496273328017));
#86222=CARTESIAN_POINT('Ctrl Pts',(0.0139921320683069,-0.0341764758837551,
0.0753999878889735));
#86223=CARTESIAN_POINT('Ctrl Pts',(0.0139501495210267,-0.0341260050040482,
0.0753910454103771));
#86224=CARTESIAN_POINT('Ctrl Pts',(0.0139088967215007,-0.0340749269148198,
0.0753822584105242));
#86225=CARTESIAN_POINT('Ctrl Pts',(0.0138278186848013,-0.0339715436305913,
0.0753649883788871));
#86226=CARTESIAN_POINT('Ctrl Pts',(0.0137880242080292,-0.0339192778235948,
0.0753565118931052));
#86227=CARTESIAN_POINT('Ctrl Pts',(0.0137489462203027,-0.0338664212855055,
0.0753481880840776));
#86228=CARTESIAN_POINT('',(0.0138422091848344,-0.0341934961088841,0.0754954019269825));
#86229=CARTESIAN_POINT('Origin',(0.00812378219310841,-0.0315241814719618,
0.07415));
#86230=CARTESIAN_POINT('',(0.0139921320689447,-0.0342105180190349,0.0753999878866158));
#86231=CARTESIAN_POINT('',(0.0139947886795375,-0.0341934961088739,0.0753874501348798));
#86232=CARTESIAN_POINT('Origin',(-0.00211012187497052,-0.0345621719126634,
0.0714925722877832));
#86233=CARTESIAN_POINT('Origin',(-0.0023089998855343,-0.0345621029764121,
0.0724513529978932));
#86234=CARTESIAN_POINT('Origin',(-0.00230473429099848,-0.0345621723551039,
0.0724062293487591));
#86235=CARTESIAN_POINT('Ctrl Pts',(0.013721263578851,-0.0346945769586966,
0.0754716294445764));
#86236=CARTESIAN_POINT('Ctrl Pts',(0.0137489456367192,-0.0345275153362944,
0.0753543879558428));
#86237=CARTESIAN_POINT('Ctrl Pts',(0.0137729477176782,-0.0343603235965185,
0.0752362455672146));
#86238=CARTESIAN_POINT('Ctrl Pts',(0.0137932040274104,-0.0341934961088739,
0.0751175527464929));
#86239=CARTESIAN_POINT('Ctrl Pts',(0.0137387286881129,-0.0346945769586966,
0.0753896355525826));
#86240=CARTESIAN_POINT('Ctrl Pts',(0.0137646933510848,-0.0345275153362944,
0.0752720282501428));
#86241=CARTESIAN_POINT('Ctrl Pts',(0.0137869660884367,-0.0343603235965185,
0.075153573963679));
#86242=CARTESIAN_POINT('Ctrl Pts',(0.0138054862341921,-0.0341934961088739,
0.075034624007431));
#86243=CARTESIAN_POINT('Ctrl Pts',(0.0137561937973755,-0.0346945769586966,
0.0753076416605875));
#86244=CARTESIAN_POINT('Ctrl Pts',(0.0137804410654508,-0.0345275153362944,
0.0751896685444432));
#86245=CARTESIAN_POINT('Ctrl Pts',(0.0138009844591957,-0.0343603235965185,
0.0750709023601439));
#86246=CARTESIAN_POINT('Ctrl Pts',(0.0138177684409741,-0.0341934961088739,
0.0749516952683679));
#86247=CARTESIAN_POINT('Ctrl Pts',(0.0137736589066369,-0.0346945769586966,
0.0752256477685948));
#86248=CARTESIAN_POINT('Ctrl Pts',(0.013796188779816,-0.0345275153362944,
0.0751073088387428));
#86249=CARTESIAN_POINT('Ctrl Pts',(0.0138150028299539,-0.0343603235965185,
0.0749882307566079));
#86250=CARTESIAN_POINT('Ctrl Pts',(0.0138300506477557,-0.0341934961088739,
0.0748687665293071));
#86251=CARTESIAN_POINT('',(0.0137736589065105,-0.0346945769586966,0.0752256477691874));
#86252=CARTESIAN_POINT('',(0.0138130810948949,-0.0343667727831529,0.0749926167614355));
#86253=CARTESIAN_POINT('Origin',(-0.00277651210024045,-0.0345626457061547,
0.0722610083501191));
#86254=CARTESIAN_POINT('Origin',(0.0247460026132076,-0.0341934771028947,
0.0766118392771571));
#86255=CARTESIAN_POINT('',(0.0137934237900075,-0.034193496108874,0.0751160689223408));
#86256=CARTESIAN_POINT('',(0.0138025805044319,-0.0341934961088839,0.0750542433242452));
#86257=CARTESIAN_POINT('',(0.0137489462188082,-0.0345211942962618,0.0753481880837279));
#86258=CARTESIAN_POINT('Origin',(-0.00267309256536622,-0.0345625596124823,
0.0717914391957437));
#86259=CARTESIAN_POINT('',(0.0137476174921984,-0.0346945769586885,0.0753479050583037));
#86260=CARTESIAN_POINT('Origin',(0.0245684310177836,-0.0346945685853916,
0.0776527933114799));
#86261=CARTESIAN_POINT('',(0.0137606381993645,-0.0346945769587026,0.0752867764137555));
#86262=CARTESIAN_POINT('Ctrl Pts',(0.0139386269144654,-0.0345231616327842,
0.0756290472834263));
#86263=CARTESIAN_POINT('Ctrl Pts',(0.0139590134989354,-0.0344132092796988,
0.0755488978355889));
#86264=CARTESIAN_POINT('Ctrl Pts',(0.0139777412034438,-0.034303273855898,
0.0754683308426755));
#86265=CARTESIAN_POINT('Ctrl Pts',(0.0139947886795439,-0.034193496108874,
0.0753874501348884));
#86266=CARTESIAN_POINT('Ctrl Pts',(0.0138749214539155,-0.0345231616327842,
0.0755353309538178));
#86267=CARTESIAN_POINT('Ctrl Pts',(0.0138940162907239,-0.0344132092796988,
0.075456059596064));
#86268=CARTESIAN_POINT('Ctrl Pts',(0.0139114704768197,-0.034303273855898,
0.0753763973667102));
#86269=CARTESIAN_POINT('Ctrl Pts',(0.0139272642655895,-0.034193496108874,
0.0752964468950599));
#86270=CARTESIAN_POINT('Ctrl Pts',(0.0138112159933657,-0.0345231616327842,
0.0754416146242093));
#86271=CARTESIAN_POINT('Ctrl Pts',(0.0138290190825124,-0.0344132092796988,
0.075363221356539));
#86272=CARTESIAN_POINT('Ctrl Pts',(0.0138451997501957,-0.034303273855898,
0.0752844638907449));
#86273=CARTESIAN_POINT('Ctrl Pts',(0.0138597398516351,-0.034193496108874,
0.0752054436552315));
#86274=CARTESIAN_POINT('Ctrl Pts',(0.0137475105328158,-0.0345231616327842,
0.0753478982946008));
#86275=CARTESIAN_POINT('Ctrl Pts',(0.013764021874301,-0.0344132092796988,
0.0752703831170141));
#86276=CARTESIAN_POINT('Ctrl Pts',(0.0137789290235716,-0.034303273855898,
0.0751925304147796));
#86277=CARTESIAN_POINT('Ctrl Pts',(0.0137922154376807,-0.034193496108874,
0.0751144404154031));
#86278=CARTESIAN_POINT('',(0.0138941062347825,-0.0341934961088839,0.0752517595286203));
#86279=CARTESIAN_POINT('Ctrl Pts',(0.0139921320655605,-0.0342105180195352,
0.0753999878858906));
#86280=CARTESIAN_POINT('Ctrl Pts',(0.0139501023246918,-0.0342610556240224,
0.0753910353407842));
#86281=CARTESIAN_POINT('Ctrl Pts',(0.0139088267857885,-0.0343122189867966,
0.0753822434444702));
#86282=CARTESIAN_POINT('Ctrl Pts',(0.0138277479302679,-0.0344158119695087,
0.0753649732425556));
#86283=CARTESIAN_POINT('Ctrl Pts',(0.0137879777757433,-0.0344681990449964,
0.0753565020006467));
#86284=CARTESIAN_POINT('Ctrl Pts',(0.0137489462187776,-0.034521194296237,
0.0753481880837135));
#86285=CARTESIAN_POINT('Ctrl Pts',(0.0137719579018241,-0.0346945769586932,
0.0752267513773195));
#86286=CARTESIAN_POINT('Ctrl Pts',(0.0137942189746654,-0.034529677707698,
0.0751099793410628));
#86287=CARTESIAN_POINT('Ctrl Pts',(0.0138116347301353,-0.034364806625142,
0.0749923870144551));
#86288=CARTESIAN_POINT('Ctrl Pts',(0.0137736589065087,-0.0346945769586932,
0.0752256477691962));
#86289=CARTESIAN_POINT('Ctrl Pts',(0.0137958971630329,-0.034529677707698,
0.0751088405658712));
#86290=CARTESIAN_POINT('Ctrl Pts',(0.0138132886681948,-0.034364806625142,
0.0749912140452645));
#86291=CARTESIAN_POINT('Ctrl Pts',(0.0140571484162524,-0.0346945769586932,
0.0750417203945992));
#86292=CARTESIAN_POINT('Ctrl Pts',(0.0140755841044496,-0.034529677707698,
0.0749190522462509));
#86293=CARTESIAN_POINT('Ctrl Pts',(0.0140889340522881,-0.034364806625142,
0.0747957269523684));
#86294=CARTESIAN_POINT('',(0.014059039610619,-0.0346775396665025,0.0750290445844434));
#86295=CARTESIAN_POINT('',(0.0140571484162445,-0.0346945769586886,0.0750417203946012));
#86296=CARTESIAN_POINT('Origin',(-0.00238509473027414,-0.0345626617186812,
0.0727479599732545));
#86297=CARTESIAN_POINT('Ctrl Pts',(0.0140590396094374,-0.0346775396670096,
0.0750290445858327));
#86298=CARTESIAN_POINT('Ctrl Pts',(0.0140165449604337,-0.0346269749928185,
0.0750227509053555));
#86299=CARTESIAN_POINT('Ctrl Pts',(0.0139748055309025,-0.0345757902890792,
0.0750165691131565));
#86300=CARTESIAN_POINT('Ctrl Pts',(0.0138928027611549,-0.0344721681087934,
0.0750044240437503));
#86301=CARTESIAN_POINT('Ctrl Pts',(0.0138525715707228,-0.0344197714289811,
0.0749984655224078));
#86302=CARTESIAN_POINT('Ctrl Pts',(0.0138130810949626,-0.0343667727830751,
0.0749926167616832));
#86303=CARTESIAN_POINT('',(0.0139154036613875,-0.0346945769587026,0.0751336840819043));
#86304=CARTESIAN_POINT('Origin',(0.00812378219310841,-0.0315241814719618,
0.07415));
#86305=CARTESIAN_POINT('',(0.0140590396095596,-0.0347116136489778,0.0750290445835401));
#86306=CARTESIAN_POINT('',(0.0140609037262012,-0.0346945769586885,0.0750163647622645));
#86307=CARTESIAN_POINT('Origin',(-0.00238987658608596,-0.0345626699728473,
0.0727930181104228));
#86308=CARTESIAN_POINT('Origin',(-0.00234034722035878,-0.0345626621420261,
0.0724458218881048));
#86309=CARTESIAN_POINT('Origin',(-0.00233186185881384,-0.0345626703330979,
0.0724013121759761));
#86310=CARTESIAN_POINT('Ctrl Pts',(0.0137868629035117,-0.0352450361874067,
0.075154131213081));
#86311=CARTESIAN_POINT('Ctrl Pts',(0.0138247343336543,-0.0349452760959492,
0.0749405446192951));
#86312=CARTESIAN_POINT('Ctrl Pts',(0.0138464099588815,-0.034644428984174,
0.0747247121714631));
#86313=CARTESIAN_POINT('Ctrl Pts',(0.0137872485048313,-0.0352450361874067,
0.0751516358300198));
#86314=CARTESIAN_POINT('Ctrl Pts',(0.0138250258200575,-0.0349452760959492,
0.0749380346930414));
#86315=CARTESIAN_POINT('Ctrl Pts',(0.013846606502286,-0.034644428984174,
0.0747221948324533));
#86316=CARTESIAN_POINT('Ctrl Pts',(0.0138254268533143,-0.0352450361874067,
0.0749045682001953));
#86317=CARTESIAN_POINT('Ctrl Pts',(0.0138538858599753,-0.0349452760959492,
0.0746895271431759));
#86318=CARTESIAN_POINT('Ctrl Pts',(0.0138660662453032,-0.034644428984174,
0.0744729533463366));
#86319=CARTESIAN_POINT('Ctrl Pts',(0.0138258086367991,-0.0352450361874067,
0.074902097523897));
#86320=CARTESIAN_POINT('Ctrl Pts',(0.0138541744603744,-0.0349452760959492,
0.0746870420676772));
#86321=CARTESIAN_POINT('Ctrl Pts',(0.0138662608427333,-0.034644428984174,
0.0744704609314754));
#86322=CARTESIAN_POINT('',(0.0138300489585611,-0.0351951634053356,0.0748687989315356));
#86323=CARTESIAN_POINT('',(0.0138547629072621,-0.0348678972925434,0.0746337200161246));
#86324=CARTESIAN_POINT('Origin',(-0.00287048597998444,-0.0345636767886427,
0.0736454309840678));
#86325=CARTESIAN_POINT('Origin',(0.0248654530858629,-0.0346946199341076,
0.0755630697984134));
#86326=CARTESIAN_POINT('',(0.0138428960148987,-0.0346945769330288,0.0747581628824752));
#86327=CARTESIAN_POINT('',(0.0138481526002897,-0.0346945769458128,0.0746958843195694));
#86328=CARTESIAN_POINT('',(0.0138130810948181,-0.0350221583435276,0.0749926167616453));
#86329=CARTESIAN_POINT('Origin',(-0.0028715381721229,-0.0345628458715597,
0.0731646583917354));
#86330=CARTESIAN_POINT('',(0.0138118571135841,-0.0351951360298762,0.0749924385407569));
#86331=CARTESIAN_POINT('Origin',(0.0247119344431038,-0.035195183836679,
0.0766067984976786));
#86332=CARTESIAN_POINT('',(0.0138300506477803,-0.0351951371328746,0.0748687665299341));
#86333=CARTESIAN_POINT('Ctrl Pts',(0.0140200229719114,-0.0350241211494343,
0.0752610106563321));
#86334=CARTESIAN_POINT('Ctrl Pts',(0.0140353266881703,-0.0349144232818962,
0.0751797923571569));
#86335=CARTESIAN_POINT('Ctrl Pts',(0.0140489607241615,-0.0348045283579412,
0.0750982091061643));
#86336=CARTESIAN_POINT('Ctrl Pts',(0.0140609037278127,-0.0346945769439157,
0.0750163647512761));
#86337=CARTESIAN_POINT('Ctrl Pts',(0.0139505586928547,-0.0350241211494343,
0.0751714793448331));
#86338=CARTESIAN_POINT('Ctrl Pts',(0.0139646291520069,-0.0349144232818962,
0.0750912178876204));
#86339=CARTESIAN_POINT('Ctrl Pts',(0.0139770489713349,-0.0348045283579412,
0.075010617543612));
#86340=CARTESIAN_POINT('Ctrl Pts',(0.0139877984008727,-0.0346945769439157,
0.0749297809596255));
#86341=CARTESIAN_POINT('Ctrl Pts',(0.013881094413798,-0.0350241211494343,
0.075081948033334));
#86342=CARTESIAN_POINT('Ctrl Pts',(0.0138939316158436,-0.0349144232818962,
0.0750026434180839));
#86343=CARTESIAN_POINT('Ctrl Pts',(0.0139051372185082,-0.0348045283579412,
0.0749230259810597));
#86344=CARTESIAN_POINT('Ctrl Pts',(0.0139146930739326,-0.0346945769439157,
0.0748431971679748));
#86345=CARTESIAN_POINT('Ctrl Pts',(0.0138116301347413,-0.0350241211494343,
0.074992416721835));
#86346=CARTESIAN_POINT('Ctrl Pts',(0.0138232340796803,-0.0349144232818962,
0.0749140689485474));
#86347=CARTESIAN_POINT('Ctrl Pts',(0.0138332254656815,-0.0348045283579412,
0.0748354344185074));
#86348=CARTESIAN_POINT('Ctrl Pts',(0.0138415877469926,-0.0346945769439157,
0.0747566133763242));
#86349=CARTESIAN_POINT('',(0.0139518998706068,-0.0346945769458128,0.0748872638226747));
#86350=CARTESIAN_POINT('Ctrl Pts',(0.0140590396063014,-0.0347116136492757,
0.0750290445830529));
#86351=CARTESIAN_POINT('Ctrl Pts',(0.0140165618348323,-0.03476215465312,
0.0750227533892073));
#86352=CARTESIAN_POINT('Ctrl Pts',(0.0139748309373691,-0.0348133084094805,
0.0750165728115495));
#86353=CARTESIAN_POINT('Ctrl Pts',(0.0138928280628412,-0.0349168561544566,
0.0750044277304468));
#86354=CARTESIAN_POINT('Ctrl Pts',(0.013852588612414,-0.0349692089015913,
0.0749984680443775));
#86355=CARTESIAN_POINT('Ctrl Pts',(0.0138130810947848,-0.0350221583435,
0.0749926167616203));
#86356=CARTESIAN_POINT('Ctrl Pts',(0.0138288757376796,-0.0351951371254987,
0.0748696383132657));
#86357=CARTESIAN_POINT('Ctrl Pts',(0.0138437538082903,-0.035030733898099,
0.0747516890837268));
#86358=CARTESIAN_POINT('Ctrl Pts',(0.0138537441967495,-0.034865930689785,
0.0746332257143997));
#86359=CARTESIAN_POINT('Ctrl Pts',(0.0138300506476639,-0.0351951371254987,
0.0748687665299282));
#86360=CARTESIAN_POINT('Ctrl Pts',(0.013844910694701,-0.035030733898099,
0.0747507930098626));
#86361=CARTESIAN_POINT('Ctrl Pts',(0.0138548820710341,-0.034865930689785,
0.0746323061156986));
#86362=CARTESIAN_POINT('Ctrl Pts',(0.0140269667855979,-0.0351951371254987,
0.0747226547339397));
#86363=CARTESIAN_POINT('Ctrl Pts',(0.0140388060629266,-0.035030733898099,
0.0746006100962716));
#86364=CARTESIAN_POINT('Ctrl Pts',(0.0140455909870978,-0.034865930689785,
0.0744781804149227));
#86365=CARTESIAN_POINT('Origin',(0.0191541016189813,-0.0308609197383775,
0.0750810075408726));
#86366=CARTESIAN_POINT('',(0.013915901643935,-0.0351951371254987,0.0748050650812598));
#86367=CARTESIAN_POINT('Origin',(0.00714850037396323,-0.0351840467441105,
0.0742097580428411));
#86368=CARTESIAN_POINT('Origin',(0.020087224815563,-0.0352322614134536,
0.0743622414773902));
#86369=CARTESIAN_POINT('',(0.0138697841027619,-0.0351951142564685,0.0743975411838139));
#86370=CARTESIAN_POINT('',(0.0138724689333491,-0.0351951372916788,0.0742728851601393));
#86371=CARTESIAN_POINT('Origin',(0.00795151354200019,-0.0352875119606938,
0.0738562016325136));
#86372=CARTESIAN_POINT('Origin',(0.00653015769557002,-0.0298325076522644,
0.0814818177310111));
#86373=CARTESIAN_POINT('Origin',(0.015819487519279,-0.0338733536828882,
0.0774699035959178));
#86374=CARTESIAN_POINT('Ctrl Pts',(0.0126266937484795,-0.0321934096636942,
0.0777279775390318));
#86375=CARTESIAN_POINT('Ctrl Pts',(0.0126907378425213,-0.0320508460845409,
0.0776473775665703));
#86376=CARTESIAN_POINT('Ctrl Pts',(0.0127525680848831,-0.0319086045665233,
0.0775651176283178));
#86377=CARTESIAN_POINT('Ctrl Pts',(0.0128120659258028,-0.0317669892871128,
0.0774813858045927));
#86378=CARTESIAN_POINT('Ctrl Pts',(0.0126774166268874,-0.0321934096636942,
0.0776612121120972));
#86379=CARTESIAN_POINT('Ctrl Pts',(0.012740265651582,-0.0320508460845409,
0.0775797042242675));
#86380=CARTESIAN_POINT('Ctrl Pts',(0.0128008773317886,-0.0319086045665233,
0.0774965691643733));
#86381=CARTESIAN_POINT('Ctrl Pts',(0.0128591358966499,-0.0317669892871128,
0.077411996681018));
#86382=CARTESIAN_POINT('Ctrl Pts',(0.0127281395052951,-0.0321934096636942,
0.0775944466851627));
#86383=CARTESIAN_POINT('Ctrl Pts',(0.0127897934606427,-0.0320508460845409,
0.0775120308819648));
#86384=CARTESIAN_POINT('Ctrl Pts',(0.0128491865786941,-0.0319086045665233,
0.0774280207004287));
#86385=CARTESIAN_POINT('Ctrl Pts',(0.0129062058674971,-0.0317669892871128,
0.0773426075574432));
#86386=CARTESIAN_POINT('Ctrl Pts',(0.012778862383703,-0.0321934096636942,
0.0775276812582281));
#86387=CARTESIAN_POINT('Ctrl Pts',(0.0128393212697036,-0.0320508460845409,
0.0774443575396621));
#86388=CARTESIAN_POINT('Ctrl Pts',(0.0128974958255996,-0.0319086045665233,
0.0773594722364842));
#86389=CARTESIAN_POINT('Ctrl Pts',(0.0129532758383442,-0.0317669892871128,
0.0772732184338684));
#86390=CARTESIAN_POINT('',(0.0127779549413831,-0.0321934096636942,0.0775288757049082));
#86391=CARTESIAN_POINT('',(0.0129128449803401,-0.031866561751136,0.0773348080961386));
#86392=CARTESIAN_POINT('Origin',(-0.000373699603126572,-0.0326371944422049,
0.0672210200799123));
#86393=CARTESIAN_POINT('Origin',(0.0220400460991528,-0.0316939261509554,
0.083404551897409));
#86394=CARTESIAN_POINT('',(0.0127035418190161,-0.0320197221621763,0.077628992804741));
#86395=CARTESIAN_POINT('Ctrl Pts',(0.0127036875798339,-0.0320197392094682,
0.0776288789246988));
#86396=CARTESIAN_POINT('Ctrl Pts',(0.0127213891968547,-0.031979271657598,
0.0776055748652964));
#86397=CARTESIAN_POINT('Ctrl Pts',(0.0127389937376033,-0.0319386439829675,
0.0775820297669435));
#86398=CARTESIAN_POINT('Ctrl Pts',(0.0127565129100146,-0.0318979099381607,
0.0775582138472279));
#86399=CARTESIAN_POINT('Ctrl Pts',(0.0127740317361464,-0.0318571766984925,
0.0775343983982515));
#86400=CARTESIAN_POINT('Ctrl Pts',(0.0127913775904035,-0.0318163871833591,
0.0775104342400269));
#86401=CARTESIAN_POINT('Ctrl Pts',(0.0128084936625507,-0.0317755399638303,
0.0774864058639879));
#86402=CARTESIAN_POINT('',(0.0127023373432517,-0.0321934096636184,0.0776284095125642));
#86403=CARTESIAN_POINT('Origin',(0.0145533252831688,-0.0324113096967968,
0.0790082204358468));
#86404=CARTESIAN_POINT('',(0.0127401461423274,-0.0321934096636663,0.0775786426087462));
#86405=CARTESIAN_POINT('Ctrl Pts',(0.01277594536621,-0.0321934096636618,
0.077529150104258));
#86406=CARTESIAN_POINT('Ctrl Pts',(0.0128225464797032,-0.0320835708272592,
0.077464993148417));
#86407=CARTESIAN_POINT('Ctrl Pts',(0.0128677928377901,-0.0319739230346489,
0.077399908998596));
#86408=CARTESIAN_POINT('Ctrl Pts',(0.0129116329416846,-0.0318646057455573,
0.0773339853683124));
#86409=CARTESIAN_POINT('Ctrl Pts',(0.0128882223728398,-0.0321934096636618,
0.0775138191372984));
#86410=CARTESIAN_POINT('Ctrl Pts',(0.0129346120603504,-0.0320835708272592,
0.0774481137940323));
#86411=CARTESIAN_POINT('Ctrl Pts',(0.0129796150712931,-0.0319739230346489,
0.0773814865303636));
#86412=CARTESIAN_POINT('Ctrl Pts',(0.01302318036975,-0.0318646057455573,
0.077314027010222));
#86413=CARTESIAN_POINT('Ctrl Pts',(0.0130004993794696,-0.0321934096636618,
0.0774984881703387));
#86414=CARTESIAN_POINT('Ctrl Pts',(0.0130466776409976,-0.0320835708272592,
0.0774312344396476));
#86415=CARTESIAN_POINT('Ctrl Pts',(0.013091437304796,-0.0319739230346489,
0.0773630640621313));
#86416=CARTESIAN_POINT('Ctrl Pts',(0.0131347277978154,-0.0318646057455573,
0.0772940686521315));
#86417=CARTESIAN_POINT('Ctrl Pts',(0.0131127763860994,-0.0321934096636618,
0.077483157203379));
#86418=CARTESIAN_POINT('Ctrl Pts',(0.0131587432216448,-0.0320835708272592,
0.0774143550852629));
#86419=CARTESIAN_POINT('Ctrl Pts',(0.0132032595382989,-0.0319739230346489,
0.077344641593899));
#86420=CARTESIAN_POINT('Ctrl Pts',(0.0132462752258808,-0.0318646057455573,
0.0772741102940411));
#86421=CARTESIAN_POINT('',(0.0131198846867272,-0.0321763980308324,0.0774724930174722));
#86422=CARTESIAN_POINT('',(0.0131127763861026,-0.0321934096636184,0.0774831572033539));
#86423=CARTESIAN_POINT('Origin',(-0.000309909663595976,-0.0326386230113314,
0.0678046743817851));
#86424=CARTESIAN_POINT('Ctrl Pts',(0.013119884684081,-0.032176398030637,
0.0774724930157105));
#86425=CARTESIAN_POINT('Ctrl Pts',(0.0130841468191009,-0.0321259596176084,
0.0774487267284882));
#86426=CARTESIAN_POINT('Ctrl Pts',(0.0130490281589977,-0.0320749164633889,
0.0774253722230343));
#86427=CARTESIAN_POINT('Ctrl Pts',(0.0129800009858953,-0.0319716057794026,
0.077379467980489));
#86428=CARTESIAN_POINT('Ctrl Pts',(0.0129461193684401,-0.0319193786690236,
0.0773569361293911));
#86429=CARTESIAN_POINT('Ctrl Pts',(0.0129128449787917,-0.0318665617525439,
0.0773348080951066));
#86430=CARTESIAN_POINT('',(0.0129453656637528,-0.0321934096636663,0.077506016454141));
#86431=CARTESIAN_POINT('Origin',(0.00812378219310841,-0.0315241814719618,
0.07415));
#86432=CARTESIAN_POINT('',(0.0131198846870346,-0.0322104233323591,0.0774724930176767));
#86433=CARTESIAN_POINT('',(0.0131269701953155,-0.0321934096636183,0.0774618136744965));
#86434=CARTESIAN_POINT('Origin',(-0.000340025323281201,-0.0326387245328339,
0.0678385573848768));
#86435=CARTESIAN_POINT('Origin',(-0.000989363387862653,-0.0326386236000299,
0.068826381625835));
#86436=CARTESIAN_POINT('Origin',(-0.000969761349190316,-0.0326387248904986,
0.0687855065180588));
#86437=CARTESIAN_POINT('Ctrl Pts',(0.0128217378227486,-0.0327445246967096,
0.0774677308362694));
#86438=CARTESIAN_POINT('Ctrl Pts',(0.0129468680868411,-0.0324436878339359,
0.0772905445430941));
#86439=CARTESIAN_POINT('Ctrl Pts',(0.0130582964732978,-0.0321434074405926,
0.077104436294559));
#86440=CARTESIAN_POINT('Ctrl Pts',(0.0129614805368145,-0.0327445246967096,
0.0772604340107619));
#86441=CARTESIAN_POINT('Ctrl Pts',(0.0130787924733207,-0.0324436878339359,
0.0770779772349648));
#86442=CARTESIAN_POINT('Ctrl Pts',(0.0131820277489421,-0.0321434074405926,
0.0768872023850803));
#86443=CARTESIAN_POINT('',(0.0129809323555165,-0.0326943950436612,0.0772299703407371));
#86444=CARTESIAN_POINT('',(0.0131033706146527,-0.0323666188837389,0.0770278158648571));
#86445=CARTESIAN_POINT('Origin',(-0.00125684902059955,-0.0326395579112007,
0.068291646129512));
#86446=CARTESIAN_POINT('Origin',(0.0226659123405023,-0.0321933825603058,
0.0825542222542162));
#86447=CARTESIAN_POINT('',(0.0130396479397987,-0.032193409653269,0.077135362449924));
#86448=CARTESIAN_POINT('',(0.013070921159878,-0.0321934096584274,0.077081249271754));
#86449=CARTESIAN_POINT('',(0.0129128449811149,-0.0325210109756239,0.077334808096657));
#86450=CARTESIAN_POINT('Origin',(-0.000978290550343325,-0.0326393129159159,
0.0678997410280831));
#86451=CARTESIAN_POINT('',(0.0129117137509639,-0.0326943950436593,0.0773340558093872));
#86452=CARTESIAN_POINT('Origin',(0.0221232398451764,-0.0326943765538176,
0.0834598785069575));
#86453=CARTESIAN_POINT('',(0.0129463230532502,-0.0326943950436702,0.0772820130750721));
#86454=CARTESIAN_POINT('Ctrl Pts',(0.0129858143778344,-0.0325229783203769,
0.0776657706174871));
#86455=CARTESIAN_POINT('Ctrl Pts',(0.0130342791989117,-0.032413025309245,
0.0775987476101464));
#86456=CARTESIAN_POINT('Ctrl Pts',(0.0130813502123452,-0.032303122220807,
0.0775307322110764));
#86457=CARTESIAN_POINT('Ctrl Pts',(0.0131269701977931,-0.0321934096576658,
0.0774618136707666));
#86458=CARTESIAN_POINT('Ctrl Pts',(0.0129610818173628,-0.0325229783203769,
0.0775551838068385));
#86459=CARTESIAN_POINT('Ctrl Pts',(0.0130080222016736,-0.032413025309245,
0.077488501737303));
#86460=CARTESIAN_POINT('Ctrl Pts',(0.0130535760622879,-0.032303122220807,
0.0774208587592611));
#86461=CARTESIAN_POINT('Ctrl Pts',(0.0130976881053954,-0.0321934096576658,
0.0773523435775825));
#86462=CARTESIAN_POINT('Ctrl Pts',(0.0129363492568912,-0.0325229783203769,
0.0774445969961899));
#86463=CARTESIAN_POINT('Ctrl Pts',(0.0129817652044356,-0.032413025309245,
0.0773782558644595));
#86464=CARTESIAN_POINT('Ctrl Pts',(0.0130258019122307,-0.032303122220807,
0.0773109853074458));
#86465=CARTESIAN_POINT('Ctrl Pts',(0.0130684060129976,-0.0321934096576658,
0.0772428734843984));
#86466=CARTESIAN_POINT('Ctrl Pts',(0.0129116166964196,-0.0325229783203769,
0.0773340101855413));
#86467=CARTESIAN_POINT('Ctrl Pts',(0.0129555082071976,-0.032413025309245,
0.0772680099916161));
#86468=CARTESIAN_POINT('Ctrl Pts',(0.0129980277621734,-0.032303122220807,
0.0772011118556305));
#86469=CARTESIAN_POINT('Ctrl Pts',(0.0130391239205998,-0.0321934096576658,
0.0771334033912143));
#86470=CARTESIAN_POINT('',(0.0130833090674282,-0.0321934096584275,0.0772985880627087));
#86471=CARTESIAN_POINT('Ctrl Pts',(0.0131198846841324,-0.0322104233328892,
0.0774724930157448));
#86472=CARTESIAN_POINT('Ctrl Pts',(0.013084098393749,-0.0322609421830435,
0.0774486945248067));
#86473=CARTESIAN_POINT('Ctrl Pts',(0.0130489560770285,-0.0323120888238835,
0.0774253242872924));
#86474=CARTESIAN_POINT('Ctrl Pts',(0.0129799283813352,-0.0324156524631806,
0.0773794196972153));
#86475=CARTESIAN_POINT('Ctrl Pts',(0.01294607137655,-0.0324680267167298,
0.0773569042139691));
#86476=CARTESIAN_POINT('Ctrl Pts',(0.0129128449810812,-0.0325210109755912,
0.0773348080966293));
#86477=CARTESIAN_POINT('Origin',(0.00300964617453292,-0.0262834582510559,
0.0801290466318158));
#86478=CARTESIAN_POINT('Origin',(0.0141662311167886,-0.0342770764397661,
0.0847004464407597));
#86479=CARTESIAN_POINT('Ctrl Pts',(0.0129789444580278,-0.0326943950436604,
0.0772303702837421));
#86480=CARTESIAN_POINT('Ctrl Pts',(0.013021397733767,-0.0325844576448134,
0.0771634570481876));
#86481=CARTESIAN_POINT('Ctrl Pts',(0.0130624701385734,-0.0324744968375322,
0.0770956610737341));
#86482=CARTESIAN_POINT('Ctrl Pts',(0.0131021102462047,-0.0323646534831894,
0.0770270699503859));
#86483=CARTESIAN_POINT('Ctrl Pts',(0.0130900371114099,-0.0326943950436604,
0.0772080196697253));
#86484=CARTESIAN_POINT('Ctrl Pts',(0.0131321823537985,-0.0325844576448134,
0.0771395753691973));
#86485=CARTESIAN_POINT('Ctrl Pts',(0.0131729150385204,-0.0324744968375322,
0.0770702545920493));
#86486=CARTESIAN_POINT('Ctrl Pts',(0.0132121842015494,-0.0323646534831894,
0.0770001468759478));
#86487=CARTESIAN_POINT('Ctrl Pts',(0.0132011297647921,-0.0326943950436604,
0.0771856690557084));
#86488=CARTESIAN_POINT('Ctrl Pts',(0.0132429669738299,-0.0325844576448133,
0.0771156936902071));
#86489=CARTESIAN_POINT('Ctrl Pts',(0.0132833599384673,-0.0324744968375322,
0.0770448481103644));
#86490=CARTESIAN_POINT('Ctrl Pts',(0.013322258156894,-0.0323646534831894,
0.0769732238015097));
#86491=CARTESIAN_POINT('Ctrl Pts',(0.0133122224181742,-0.0326943950436604,
0.0771633184416916));
#86492=CARTESIAN_POINT('Ctrl Pts',(0.0133537515938614,-0.0325844576448133,
0.0770918120112168));
#86493=CARTESIAN_POINT('Ctrl Pts',(0.0133938048384143,-0.0324744968375322,
0.0770194416286796));
#86494=CARTESIAN_POINT('Ctrl Pts',(0.0134323321122387,-0.0323646534831894,
0.0769463007270716));
#86495=CARTESIAN_POINT('',(0.0133186470825827,-0.032677355999139,0.0771522289653595));
#86496=CARTESIAN_POINT('',(0.0133122224181615,-0.0326943950436595,0.0771633184416936));
#86497=CARTESIAN_POINT('Origin',(-0.00108340451308647,-0.032639567087523,
0.0688869875836626));
#86498=CARTESIAN_POINT('Ctrl Pts',(0.0133186470796761,-0.03267735599875,
0.0771522289636776));
#86499=CARTESIAN_POINT('Ctrl Pts',(0.0132814575341154,-0.0326267922587063,
0.0771307362909582));
#86500=CARTESIAN_POINT('Ctrl Pts',(0.0132449271463918,-0.0325756109581517,
0.077109624560341));
#86501=CARTESIAN_POINT('Ctrl Pts',(0.0131731535971661,-0.0324719985462385,
0.0770681450160186));
#86502=CARTESIAN_POINT('Ctrl Pts',(0.0131379392222946,-0.0324196091621783,
0.0770477938387531));
#86503=CARTESIAN_POINT('Ctrl Pts',(0.0131033706146104,-0.0323666188837757,
0.0770278158648328));
#86504=CARTESIAN_POINT('',(0.013146577386849,-0.0326943950436703,0.0771966443912254));
#86505=CARTESIAN_POINT('Origin',(0.00812378219310841,-0.0315241814719618,
0.07415));
#86506=CARTESIAN_POINT('',(0.0133186470825428,-0.032711433838003,0.0771522289653367));
#86507=CARTESIAN_POINT('',(0.0133250480478684,-0.0326943950436593,0.0771411257927597));
#86508=CARTESIAN_POINT('Origin',(-0.001105399748007,-0.0326395680729595,
0.0689266000423664));
#86509=CARTESIAN_POINT('Origin',(-0.00103312703808973,-0.0326395672038611,
0.0687999895580363));
#86510=CARTESIAN_POINT('Origin',(-0.00100978475184705,-0.0326395683429341,
0.0687611558268961));
#86511=CARTESIAN_POINT('Ctrl Pts',(0.0130208100933845,-0.0332451089994434,
0.0771661635804309));
#86512=CARTESIAN_POINT('Ctrl Pts',(0.0131345665639738,-0.0329451141710254,
0.0769814691514128));
#86513=CARTESIAN_POINT('Ctrl Pts',(0.0132340879250057,-0.0326442513127493,
0.0767887308173699));
#86514=CARTESIAN_POINT('Ctrl Pts',(0.0131472593109561,-0.0332451089994434,
0.076950500427863));
#86515=CARTESIAN_POINT('Ctrl Pts',(0.0132528819126693,-0.0329451141710254,
0.0767610368885774));
#86516=CARTESIAN_POINT('Ctrl Pts',(0.0133439332834064,-0.0326442513127493,
0.0765641556690614));
#86517=CARTESIAN_POINT('Ctrl Pts',(0.0131485238031318,-0.0332451089994434,
0.0769483437963373));
#86518=CARTESIAN_POINT('Ctrl Pts',(0.0132540650661562,-0.0329451141710254,
0.0767588325659491));
#86519=CARTESIAN_POINT('Ctrl Pts',(0.0133450317369904,-0.0326442513127493,
0.0765619099175782));
#86520=CARTESIAN_POINT('',(0.0131647408170115,-0.0331951640388616,0.0769189097406918));
#86521=CARTESIAN_POINT('',(0.0132742440992889,-0.0328677532355045,0.0767094661988068));
#86522=CARTESIAN_POINT('Origin',(-0.00188291505151877,-0.032640280827965,
0.0695297081368198));
#86523=CARTESIAN_POINT('Origin',(0.0231752604518522,-0.0326944278779147,
0.0816292485253018));
#86524=CARTESIAN_POINT('',(0.0132174000641565,-0.0326943950436593,0.0768208017492394));
#86525=CARTESIAN_POINT('',(0.0132452137775803,-0.0326943950436693,0.0767648316916638));
#86526=CARTESIAN_POINT('',(0.0131033706146512,-0.0330220786163545,0.0770278158648596));
#86527=CARTESIAN_POINT('Origin',(-0.00169754986071946,-0.0326396682761177,
0.0690860952525217));
#86528=CARTESIAN_POINT('',(0.0131021943802152,-0.0331951640388588,0.0770271360925872));
#86529=CARTESIAN_POINT('Origin',(0.0226535182158981,-0.0331952026560063,
0.0825470620455517));
#86530=CARTESIAN_POINT('',(0.0131334675986233,-0.0331951640388701,0.0769730229166495));
#86531=CARTESIAN_POINT('Ctrl Pts',(0.0131969778446032,-0.0330240426238171,
0.0773535427079646));
#86532=CARTESIAN_POINT('Ctrl Pts',(0.0132411097664658,-0.0329142774063519,
0.0772836544952902));
#86533=CARTESIAN_POINT('Ctrl Pts',(0.0132838189051219,-0.032804347972669,
0.0772128191106915));
#86534=CARTESIAN_POINT('Ctrl Pts',(0.0133250480478717,-0.0326943950436593,
0.0771411257927695));
#86535=CARTESIAN_POINT('Ctrl Pts',(0.0131653502751687,-0.0330240426238171,
0.0772447271170008));
#86536=CARTESIAN_POINT('Ctrl Pts',(0.013207983156252,-0.0329142774063519,
0.0771752746049086));
#86537=CARTESIAN_POINT('Ctrl Pts',(0.0132492015139503,-0.032804347972669,
0.077104906127465));
#86538=CARTESIAN_POINT('Ctrl Pts',(0.013288950061838,-0.0326943950436593,
0.0770337103777238));
#86539=CARTESIAN_POINT('Ctrl Pts',(0.0131337227057343,-0.0330240426238171,
0.077135911526037));
#86540=CARTESIAN_POINT('Ctrl Pts',(0.0131748565460381,-0.0329142774063519,
0.077066894714527));
#86541=CARTESIAN_POINT('Ctrl Pts',(0.0132145841227786,-0.032804347972669,
0.0769969931442386));
#86542=CARTESIAN_POINT('Ctrl Pts',(0.0132528520758044,-0.0326943950436593,
0.0769262949626781));
#86543=CARTESIAN_POINT('Ctrl Pts',(0.0131020951362999,-0.0330240426238171,
0.0770270959350732));
#86544=CARTESIAN_POINT('Ctrl Pts',(0.0131417299358243,-0.0329142774063519,
0.0769585148241454));
#86545=CARTESIAN_POINT('Ctrl Pts',(0.0131799667316069,-0.032804347972669,
0.0768890801610122));
#86546=CARTESIAN_POINT('Ctrl Pts',(0.0132167540897707,-0.0326943950436593,
0.0768188795476324));
#86547=CARTESIAN_POINT('',(0.0132712240560225,-0.0326943950436693,0.0769809637710096));
#86548=CARTESIAN_POINT('Ctrl Pts',(0.013318647079667,-0.0327114338383286,
0.0771522289636724));
#86549=CARTESIAN_POINT('Ctrl Pts',(0.0132814637199353,-0.0327619876830068,
0.0771307398658825));
#86550=CARTESIAN_POINT('Ctrl Pts',(0.0132449363536533,-0.0328131562602515,
0.0771096298814241));
#86551=CARTESIAN_POINT('Ctrl Pts',(0.013173162870366,-0.0329167375858766,
0.077068150375209));
#86552=CARTESIAN_POINT('Ctrl Pts',(0.0131379453517996,-0.0329691088920611,
0.0770477973811317));
#86553=CARTESIAN_POINT('Ctrl Pts',(0.0131033706146114,-0.0330220786163186,
0.0770278158648334));
#86554=CARTESIAN_POINT('Ctrl Pts',(0.0131627816420839,-0.0331951640388604,
0.0769194337992695));
#86555=CARTESIAN_POINT('Ctrl Pts',(0.013220037910288,-0.0330306422010619,
0.0768152557163678));
#86556=CARTESIAN_POINT('Ctrl Pts',(0.0132729394636896,-0.0328657861914645,
0.0767088001911311));
#86557=CARTESIAN_POINT('Ctrl Pts',(0.0131647408170099,-0.0331951640388604,
0.0769189097406946));
#86558=CARTESIAN_POINT('Ctrl Pts',(0.013221986250639,-0.0330306422010619,
0.0768146911531074));
#86559=CARTESIAN_POINT('Ctrl Pts',(0.0132748753046224,-0.0328657861914645,
0.0767081956056004));
#86560=CARTESIAN_POINT('Ctrl Pts',(0.0134911920470379,-0.0331951640388604,
0.0768315874887956));
#86561=CARTESIAN_POINT('Ctrl Pts',(0.0135466321490948,-0.0330306422010619,
0.0767206197313287));
#86562=CARTESIAN_POINT('Ctrl Pts',(0.0135974384638604,-0.0328657861914645,
0.0766074553973127));
#86563=CARTESIAN_POINT('',(0.0134969077207388,-0.0331781648281956,0.0768201164881559));
#86564=CARTESIAN_POINT('',(0.013491192047025,-0.0331951640388588,0.0768315874887981));
#86565=CARTESIAN_POINT('Origin',(-0.00160237718115885,-0.0326412092602053,
0.0701120558230257));
#86566=CARTESIAN_POINT('Ctrl Pts',(0.0134969077191093,-0.033178164828644,
0.076820116489022));
#86567=CARTESIAN_POINT('Ctrl Pts',(0.0134584155350228,-0.0331276811546765,
0.0768009882289008));
#86568=CARTESIAN_POINT('Ctrl Pts',(0.0134206183855283,-0.0330765663497771,
0.0767822053962043));
#86569=CARTESIAN_POINT('Ctrl Pts',(0.0133463817535232,-0.0329730614463557,
0.0767453143027143));
#86570=CARTESIAN_POINT('Ctrl Pts',(0.013309972263362,-0.0329207133374385,
0.0767272209403097));
#86571=CARTESIAN_POINT('Ctrl Pts',(0.0132742441008721,-0.0328677532289399,
0.0767094662152024));
#86572=CARTESIAN_POINT('',(0.0133279664320283,-0.0331951640388702,0.0768752486147549));
#86573=CARTESIAN_POINT('Origin',(0.00812378219310841,-0.0315241814719618,
0.07415));
#86574=CARTESIAN_POINT('',(0.0134969077196362,-0.0332121607144205,0.0768201164868861));
#86575=CARTESIAN_POINT('',(0.0135025988803252,-0.0331951640388587,0.076808633304035));
#86576=CARTESIAN_POINT('Origin',(-0.0016152271314213,-0.0326413666921275,
0.0701555412417527));
#86577=CARTESIAN_POINT('Origin',(-0.000968433154056809,-0.032641209404409,
0.06883635705972));
#86578=CARTESIAN_POINT('Origin',(-0.000941532136059744,-0.0326413667252248,
0.0687998540025973));
#86579=CARTESIAN_POINT('Ctrl Pts',(0.0132005236162736,-0.0337436976235975,
0.0768527433326748));
#86580=CARTESIAN_POINT('Ctrl Pts',(0.0132248324994197,-0.0336723290703325,
0.0768070823509136));
#86581=CARTESIAN_POINT('Ctrl Pts',(0.0132483161528197,-0.033601104548885,
0.0767609915158356));
#86582=CARTESIAN_POINT('Ctrl Pts',(0.0133232948062763,-0.0333736987606857,
0.0766138326095115));
#86583=CARTESIAN_POINT('Ctrl Pts',(0.013389705074288,-0.0331450831799191,
0.0764626135019646));
#86584=CARTESIAN_POINT('Ctrl Pts',(0.0133131825221592,-0.0337436976235975,
0.0766295663380615));
#86585=CARTESIAN_POINT('Ctrl Pts',(0.0133354841175923,-0.0336723290703325,
0.0765828920850269));
#86586=CARTESIAN_POINT('Ctrl Pts',(0.0133569425824548,-0.033601104548885,
0.0765358242473779));
#86587=CARTESIAN_POINT('Ctrl Pts',(0.0134254552100782,-0.0333736987606857,
0.0763855459653781));
#86588=CARTESIAN_POINT('Ctrl Pts',(0.0134852310999934,-0.0331450831799191,
0.076231583680485));
#86589=CARTESIAN_POINT('Ctrl Pts',(0.0133143091112181,-0.0337436976235975,
0.0766273345681153));
#86590=CARTESIAN_POINT('Ctrl Pts',(0.013336590633774,-0.0336723290703325,
0.0765806501823679));
#86591=CARTESIAN_POINT('Ctrl Pts',(0.0133580288467511,-0.033601104548885,
0.0765335725746933));
#86592=CARTESIAN_POINT('Ctrl Pts',(0.0134264768141163,-0.0333736987606857,
0.0763832630989368));
#86593=CARTESIAN_POINT('Ctrl Pts',(0.0134861863602505,-0.0331450831799191,
0.0762292733822702));
#86594=CARTESIAN_POINT('',(0.0133286549178185,-0.0336938721132548,0.0765969215188825));
#86595=CARTESIAN_POINT('',(0.0134247910462803,-0.0333679870047996,0.0763810154949585));
#86596=CARTESIAN_POINT('Ctrl Pts',(0.0133286549178133,-0.0336938721132587,
0.0765969215188945));
#86597=CARTESIAN_POINT('Ctrl Pts',(0.0133382064003763,-0.0336629187933933,
0.0765766044589929));
#86598=CARTESIAN_POINT('Ctrl Pts',(0.0133476358635913,-0.0336319952301071,
0.0765562379692043));
#86599=CARTESIAN_POINT('Ctrl Pts',(0.0133569425824547,-0.0336011045488981,
0.0765358242473785));
#86600=CARTESIAN_POINT('Ctrl Pts',(0.0133802963246631,-0.0335235892595485,
0.0764845992341352));
#86601=CARTESIAN_POINT('Ctrl Pts',(0.0134029185313843,-0.0334458668665602,
0.0764329857278372));
#86602=CARTESIAN_POINT('Ctrl Pts',(0.0134247910419178,-0.0333679869962525,
0.0763810155059306));
#86603=CARTESIAN_POINT('Ctrl Pts',(0.013424808927659,-0.0333679692468938,
0.0763809747805152));
#86604=CARTESIAN_POINT('Ctrl Pts',(0.0134243889027203,-0.0333391895412975,
0.0763808044372332));
#86605=CARTESIAN_POINT('Ctrl Pts',(0.0134240728531347,-0.0333104081127487,
0.0763806797657752));
#86606=CARTESIAN_POINT('Ctrl Pts',(0.0134236524748471,-0.0332532697931203,
0.0763805198937491));
#86607=CARTESIAN_POINT('Ctrl Pts',(0.0134235450558214,-0.0332249169638106,
0.0763804833894381));
#86608=CARTESIAN_POINT('Ctrl Pts',(0.0134235389970316,-0.0331960985432299,
0.0763804883235465));
#86609=CARTESIAN_POINT('Ctrl Pts',(0.013423538926182,-0.0331956312492137,
0.0763804884151774));
#86610=CARTESIAN_POINT('Ctrl Pts',(0.0134235388830291,-0.0331951640388587,
0.0763804885177109));
#86611=CARTESIAN_POINT('',(0.0133750500022088,-0.0331951640388587,0.076495700619667));
#86612=CARTESIAN_POINT('',(0.0133992944426288,-0.0331951640388687,0.0764380945686996));
#86613=CARTESIAN_POINT('',(0.013274244087226,-0.0335216366567648,0.0767094662085707));
#86614=CARTESIAN_POINT('Origin',(-0.00213958756456626,-0.0326434571524483,
0.0704019739310167));
#86615=CARTESIAN_POINT('',(0.0132730274909841,-0.0336938721132327,0.0767088616340682));
#86616=CARTESIAN_POINT('Origin',(0.0230526250392022,-0.0336938867896158,
0.0815687280640452));
#86617=CARTESIAN_POINT('',(0.0133008412044113,-0.0336938721132538,0.0766528915764853));
#86618=CARTESIAN_POINT('Ctrl Pts',(0.0133881196239129,-0.0335235895815172,
0.0770286718143495));
#86619=CARTESIAN_POINT('Ctrl Pts',(0.0134277502090207,-0.0334144449262749,
0.0769561978450879));
#86620=CARTESIAN_POINT('Ctrl Pts',(0.0134659290672072,-0.0333049234473147,
0.0768828218739531));
#86621=CARTESIAN_POINT('Ctrl Pts',(0.0135025988803291,-0.0331951640388587,
0.0768086333040447));
#86622=CARTESIAN_POINT('Ctrl Pts',(0.0133497218051218,-0.0335235895815172,
0.0769220567122362));
#86623=CARTESIAN_POINT('Ctrl Pts',(0.0133878846234432,-0.0334144449262749,
0.0768501113645486));
#86624=CARTESIAN_POINT('Ctrl Pts',(0.0134246049494809,-0.0333049234473147,
0.0767772949452671));
#86625=CARTESIAN_POINT('Ctrl Pts',(0.0134598273949193,-0.0331951640388587,
0.0767036963109375));
#86626=CARTESIAN_POINT('Ctrl Pts',(0.0133113239863307,-0.0335235895815172,
0.0768154416101229));
#86627=CARTESIAN_POINT('Ctrl Pts',(0.0133480190378656,-0.0334144449262749,
0.0767440248840093));
#86628=CARTESIAN_POINT('Ctrl Pts',(0.0133832808317546,-0.0333049234473147,
0.0766717680165811));
#86629=CARTESIAN_POINT('Ctrl Pts',(0.0134170559095094,-0.0331951640388587,
0.0765987593178303));
#86630=CARTESIAN_POINT('Ctrl Pts',(0.0132729261675395,-0.0335235895815172,
0.0767088265080096));
#86631=CARTESIAN_POINT('Ctrl Pts',(0.0133081534522881,-0.0334144449262749,
0.07663793840347));
#86632=CARTESIAN_POINT('Ctrl Pts',(0.0133419567140284,-0.0333049234473147,
0.0765662410878951));
#86633=CARTESIAN_POINT('Ctrl Pts',(0.0133742844240995,-0.0331951640388587,
0.0764938223247231));
#86634=CARTESIAN_POINT('',(0.013438824441277,-0.0331951640388687,0.076652166961861));
#86635=CARTESIAN_POINT('Ctrl Pts',(0.0134969077168258,-0.033212160714594,
0.0768201164854868));
#86636=CARTESIAN_POINT('Ctrl Pts',(0.0134584802918743,-0.0332625444108826,
0.0768010203932022));
#86637=CARTESIAN_POINT('Ctrl Pts',(0.0134207150317549,-0.0333135300744947,
0.0767822533565532));
#86638=CARTESIAN_POINT('Ctrl Pts',(0.013346478863352,-0.0334167203140538,
0.0767453624973694));
#86639=CARTESIAN_POINT('Ctrl Pts',(0.0133100367075453,-0.0334688847587207,
0.0767272529630664));
#86640=CARTESIAN_POINT('Ctrl Pts',(0.0132742440866642,-0.0335216366562262,
0.0767094662081039));
#86641=CARTESIAN_POINT('Ctrl Pts',(0.0133267329643754,-0.0336938721132584,
0.0765975674098968));
#86642=CARTESIAN_POINT('Ctrl Pts',(0.0133410593886174,-0.0336474569765055,
0.076567112812504));
#86643=CARTESIAN_POINT('Ctrl Pts',(0.0133550283216894,-0.033601104548885,
0.0765364925929956));
#86644=CARTESIAN_POINT('Ctrl Pts',(0.0133903944485611,-0.0334837508592655,
0.0764589692372461));
#86645=CARTESIAN_POINT('Ctrl Pts',(0.0134234478674729,-0.0333660264659096,
0.0763804319523758));
#86646=CARTESIAN_POINT('Ctrl Pts',(0.0133286549178037,-0.0336938721132584,
0.0765969215189137));
#86647=CARTESIAN_POINT('Ctrl Pts',(0.0133429775614315,-0.0336474569765055,
0.0765664556716898));
#86648=CARTESIAN_POINT('Ctrl Pts',(0.0133569425824548,-0.033601104548885,
0.0765358242473779));
#86649=CARTESIAN_POINT('Ctrl Pts',(0.0133922988049186,-0.0334837508592655,
0.0764582725236422));
#86650=CARTESIAN_POINT('Ctrl Pts',(0.0134253414831697,-0.0333660264659096,
0.0763797071767308));
#86651=CARTESIAN_POINT('Ctrl Pts',(0.0136509009056519,-0.0336938721132584,
0.0764886276472783));
#86652=CARTESIAN_POINT('Ctrl Pts',(0.0136645896693132,-0.0336474569765055,
0.0764562755873546));
#86653=CARTESIAN_POINT('Ctrl Pts',(0.0136778987733026,-0.033601104548885,
0.0764237654999526));
#86654=CARTESIAN_POINT('Ctrl Pts',(0.0137115943646418,-0.0334837508592655,
0.0763414574332058));
#86655=CARTESIAN_POINT('Ctrl Pts',(0.0137428362006902,-0.0333660264659096,
0.0762581870398619));
#86656=CARTESIAN_POINT('',(0.0136539630869382,-0.0336769361243754,0.0764774662793518));
#86657=CARTESIAN_POINT('',(0.0136489789613314,-0.0336938721132327,0.0764892735351852));
#86658=CARTESIAN_POINT('Ctrl Pts',(0.0136539630869382,-0.0336769361243754,
0.0764774662793518));
#86659=CARTESIAN_POINT('Ctrl Pts',(0.0136531344389964,-0.0336797586670078,
0.0764794351899461));
#86660=CARTESIAN_POINT('Ctrl Pts',(0.013652304770908,-0.0336825812712947,
0.0764814035835397));
#86661=CARTESIAN_POINT('Ctrl Pts',(0.013650643398562,-0.0336882265906967,
0.076485339328277));
#86662=CARTESIAN_POINT('Ctrl Pts',(0.0136498116943304,-0.0336910493058177,
0.0764873066794294));
#86663=CARTESIAN_POINT('Ctrl Pts',(0.0136489789613424,-0.0336938721132368,
0.0764892735351839));
#86664=CARTESIAN_POINT('Ctrl Pts',(0.0136539630869382,-0.0336769361243754,
0.0764774662793518));
#86665=CARTESIAN_POINT('Ctrl Pts',(0.0136153321799088,-0.0336279018525342,
0.0764612078358799));
#86666=CARTESIAN_POINT('Ctrl Pts',(0.0135761455183466,-0.0335767826051548,
0.076444715494104));
#86667=CARTESIAN_POINT('Ctrl Pts',(0.0134993621726489,-0.0334733172106852,
0.0764123999783265));
#86668=CARTESIAN_POINT('Ctrl Pts',(0.0134617138840055,-0.0334209631477636,
0.0763965550857312));
#86669=CARTESIAN_POINT('Ctrl Pts',(0.013424791040563,-0.0333679869844681,
0.0763810155085093));
#86670=CARTESIAN_POINT('',(0.013488816939585,-0.0336938721132538,0.0765430975270439));
#86671=CARTESIAN_POINT('Origin',(0.00812378219310841,-0.0315241814719618,
0.07415));
#86672=CARTESIAN_POINT('',(0.0136539630857512,-0.0337108120655378,0.0764774662788552));
#86673=CARTESIAN_POINT('',(0.0136589219806651,-0.0336938721132327,0.0764656484042733));
#86674=CARTESIAN_POINT('Origin',(-0.000992580517952669,-0.0345562525600667,
0.0691006776982423));
#86675=CARTESIAN_POINT('Ctrl Pts',(0.0136589219806746,-0.0336938721132384,
0.0764656484042855));
#86676=CARTESIAN_POINT('Ctrl Pts',(0.0136580976547706,-0.0336910492956357,
0.0764676188066577));
#86677=CARTESIAN_POINT('Ctrl Pts',(0.0136572722599229,-0.0336882265856054,
0.0764695888090337));
#86678=CARTESIAN_POINT('Ctrl Pts',(0.0136556192999888,-0.0336825812712732,
0.0764735280901084));
#86679=CARTESIAN_POINT('Ctrl Pts',(0.0136547917348769,-0.033679758666997,
0.0764754973687649));
#86680=CARTESIAN_POINT('Ctrl Pts',(0.0136539630869382,-0.0336769361243754,
0.0764774662793518));
#86681=CARTESIAN_POINT('Origin',(-0.00185964346467866,-0.0345562522792228,
0.0711608663359108));
#86682=CARTESIAN_POINT('Ctrl Pts',(0.0133601911283327,-0.034243627687391,
0.0765286858689418));
#86683=CARTESIAN_POINT('Ctrl Pts',(0.0134499047448276,-0.033943005420181,
0.0763311914502129));
#86684=CARTESIAN_POINT('Ctrl Pts',(0.0135244874055163,-0.0336441434784052,
0.076127500495239));
#86685=CARTESIAN_POINT('Ctrl Pts',(0.013458616391475,-0.034243627687391,
0.0762988762356028));
#86686=CARTESIAN_POINT('Ctrl Pts',(0.0135396625947644,-0.033943005420181,
0.0760976696468787));
#86687=CARTESIAN_POINT('Ctrl Pts',(0.0136053228496057,-0.0336441434784052,
0.0758909299328715));
#86688=CARTESIAN_POINT('Ctrl Pts',(0.0134596006441064,-0.034243627687391,
0.0762965781392694));
#86689=CARTESIAN_POINT('Ctrl Pts',(0.0135405601732637,-0.033943005420181,
0.0760953344288453));
#86690=CARTESIAN_POINT('Ctrl Pts',(0.0136061312040465,-0.0336441434784052,
0.0758885642272479));
#86691=CARTESIAN_POINT('',(0.0134720277638486,-0.0341934961088741,0.0762652764157573));
#86692=CARTESIAN_POINT('',(0.0135544173338659,-0.033866421286606,0.0760437600087977));
#86693=CARTESIAN_POINT('Origin',(-0.00189517546600665,-0.0345610720406586,
0.0696394022350303));
#86694=CARTESIAN_POINT('Origin',(0.0239091527297719,-0.033693800507295,
0.0796546019243239));
#86695=CARTESIAN_POINT('',(0.0135119755852947,-0.0336938721132327,0.0761613420813975));
#86696=CARTESIAN_POINT('',(0.0135325550709807,-0.0336938721132427,0.0761023273818038));
#86697=CARTESIAN_POINT('',(0.013424791040561,-0.0340203938281605,0.0763810155085142));
#86698=CARTESIAN_POINT('Origin',(-0.00163881785010329,-0.0345589643243111,
0.0692321952771803));
#86699=CARTESIAN_POINT('',(0.0134235388830286,-0.034193496108874,0.0763804885177123));
#86700=CARTESIAN_POINT('Origin',(0.0235801278517751,-0.0341934220717693,
0.0806550550213423));
#86701=CARTESIAN_POINT('',(0.0134477833234486,-0.0341934961088841,0.0763228824667448));
#86702=CARTESIAN_POINT('Ctrl Pts',(0.0135584837958485,-0.0340223579322396,
0.0766924434092575));
#86703=CARTESIAN_POINT('Ctrl Pts',(0.013593550721433,-0.0339125849573575,
0.0766174846998589));
#86704=CARTESIAN_POINT('Ctrl Pts',(0.0136270415347902,-0.0338030433565231,
0.0765418528592022));
#86705=CARTESIAN_POINT('Ctrl Pts',(0.0136589219806698,-0.0336938721132327,
0.076465648404283));
#86706=CARTESIAN_POINT('Ctrl Pts',(0.0135134673632818,-0.0340223579322396,
0.0765884496564168));
#86707=CARTESIAN_POINT('Ctrl Pts',(0.0135470999437875,-0.0339125849573575,
0.0765141118410311));
#86708=CARTESIAN_POINT('Ctrl Pts',(0.013579170271027,-0.0338030433565231,
0.0764391301457024));
#86709=CARTESIAN_POINT('Ctrl Pts',(0.0136096458326096,-0.0336938721132327,
0.0763636040949694));
#86710=CARTESIAN_POINT('Ctrl Pts',(0.0134684509307151,-0.0340223579322396,
0.0764844559035761));
#86711=CARTESIAN_POINT('Ctrl Pts',(0.013500649166142,-0.0339125849573575,
0.0764107389822032));
#86712=CARTESIAN_POINT('Ctrl Pts',(0.0135312990072637,-0.0338030433565231,
0.0763364074322026));
#86713=CARTESIAN_POINT('Ctrl Pts',(0.0135603696845494,-0.0336938721132327,
0.0762615597856559));
#86714=CARTESIAN_POINT('Ctrl Pts',(0.0134234344981484,-0.0340223579322396,
0.0763804621507353));
#86715=CARTESIAN_POINT('Ctrl Pts',(0.0134541983884965,-0.0339125849573575,
0.0763073661233754));
#86716=CARTESIAN_POINT('Ctrl Pts',(0.0134834277435004,-0.0338030433565231,
0.0762336847187027));
#86717=CARTESIAN_POINT('Ctrl Pts',(0.0135110935364892,-0.0336938721132327,
0.0761595154763423));
#86718=CARTESIAN_POINT('',(0.0135854487829899,-0.0336938721132427,0.0763134952428453));
#86719=CARTESIAN_POINT('Ctrl Pts',(0.0136539630824248,-0.0337108120662652,
0.0764774662774524));
#86720=CARTESIAN_POINT('Ctrl Pts',(0.0136143308050121,-0.0337611408993406,
0.0764607863910214));
#86721=CARTESIAN_POINT('Ctrl Pts',(0.0135754217287318,-0.0338121088779513,
0.0764444108755108));
#86722=CARTESIAN_POINT('Ctrl Pts',(0.0134990145326359,-0.0339153382773231,
0.0764122536683909));
#86723=CARTESIAN_POINT('Ctrl Pts',(0.0134615487379387,-0.0339675558473106,
0.0763964855813318));
#86724=CARTESIAN_POINT('Ctrl Pts',(0.0134247910405263,-0.0340203938281304,
0.076381015508494));
#86725=CARTESIAN_POINT('Ctrl Pts',(0.0134701496332366,-0.0341934961088741,
0.0762660419268864));
#86726=CARTESIAN_POINT('Ctrl Pts',(0.0135138971330321,-0.0340287516182428,
0.0761555099919934));
#86727=CARTESIAN_POINT('Ctrl Pts',(0.0135530388827007,-0.0338644633275951,
0.0760432643871688));
#86728=CARTESIAN_POINT('Ctrl Pts',(0.0134720277638485,-0.0341934961088741,
0.0762652764157574));
#86729=CARTESIAN_POINT('Ctrl Pts',(0.0135157594373044,-0.0340287516182428,
0.0761547056519936));
#86730=CARTESIAN_POINT('Ctrl Pts',(0.0135548837693301,-0.0338644633275951,
0.0760424219055914));
#86731=CARTESIAN_POINT('Ctrl Pts',(0.0137849604482274,-0.0341934961088741,
0.0761377275376366));
#86732=CARTESIAN_POINT('Ctrl Pts',(0.0138260551491127,-0.0340287516182428,
0.0760206871371553));
#86733=CARTESIAN_POINT('Ctrl Pts',(0.0138622773668167,-0.0338644633275951,
0.0759020482702934));
#86734=CARTESIAN_POINT('',(0.0137891933540578,-0.0341764758832445,0.0761256306254384));
#86735=CARTESIAN_POINT('',(0.0137849604482159,-0.0341934961088741,0.0761377275376413));
#86736=CARTESIAN_POINT('Origin',(-0.00167659701415602,-0.0345621027032399,
0.0701900890989704));
#86737=CARTESIAN_POINT('Ctrl Pts',(0.0137891933527088,-0.0341764758837555,
0.076125630626661));
#86738=CARTESIAN_POINT('Ctrl Pts',(0.013748662640142,-0.0341260050040858,
0.0761114968537859));
#86739=CARTESIAN_POINT('Ctrl Pts',(0.0137088364343957,-0.0340749269148957,
0.0760976087953033));
#86740=CARTESIAN_POINT('Ctrl Pts',(0.0136305622312432,-0.0339715436308062,
0.0760703131705489));
#86741=CARTESIAN_POINT('Ctrl Pts',(0.0135921439311717,-0.0339192778238088,
0.076056915953935));
#86742=CARTESIAN_POINT('Ctrl Pts',(0.0135544173348583,-0.0338664212855904,
0.0760437600100322));
#86743=CARTESIAN_POINT('',(0.0136284941060423,-0.0341934961088841,0.0762015019767093));
#86744=CARTESIAN_POINT('Origin',(0.00812378219310841,-0.0315241814719618,
0.07415));
#86745=CARTESIAN_POINT('',(0.0137891933536377,-0.0342105180190519,0.0761256306244011));
#86746=CARTESIAN_POINT('',(0.0137934004130283,-0.0341934961088739,0.076113524698179));
#86747=CARTESIAN_POINT('Origin',(-0.00169636026059117,-0.0345621720468637,
0.0702308784965533));
#86748=CARTESIAN_POINT('Origin',(-0.0020138373063663,-0.0345621029228079,
0.0711571729676889));
#86749=CARTESIAN_POINT('Origin',(-0.00200394991402754,-0.0345621724125657,
0.0711129398881292));
#86750=CARTESIAN_POINT('Ctrl Pts',(0.0135114816743752,-0.0346945769586965,
0.0761627584435455));
#86751=CARTESIAN_POINT('Ctrl Pts',(0.0135536397058397,-0.0345275153362944,
0.0760499109207932));
#86752=CARTESIAN_POINT('Ctrl Pts',(0.0135922596908091,-0.0343603235965185,
0.0759357083786057));
#86753=CARTESIAN_POINT('Ctrl Pts',(0.0136272324285107,-0.034193496108874,
0.0758204902750261));
#86754=CARTESIAN_POINT('Ctrl Pts',(0.0135390856256502,-0.0346945769586965,
0.0760836000564988));
#86755=CARTESIAN_POINT('Ctrl Pts',(0.0135795856530047,-0.0345275153362944,
0.075970174357935));
#86756=CARTESIAN_POINT('Ctrl Pts',(0.0136165290219222,-0.0343603235965185,
0.0758554456330932));
#86757=CARTESIAN_POINT('Ctrl Pts',(0.0136498115134455,-0.034193496108874,
0.0757397548225325));
#86758=CARTESIAN_POINT('Ctrl Pts',(0.0135666895769253,-0.0346945769586965,
0.0760044416694547));
#86759=CARTESIAN_POINT('Ctrl Pts',(0.0136055316001701,-0.0345275153362944,
0.0758904377950791));
#86760=CARTESIAN_POINT('Ctrl Pts',(0.0136407983530358,-0.0343603235965185,
0.075775182887582));
#86761=CARTESIAN_POINT('Ctrl Pts',(0.0136723905983807,-0.034193496108874,
0.0756590193700381));
#86762=CARTESIAN_POINT('Ctrl Pts',(0.0135942935282001,-0.0346945769586965,
0.0759252832824053));
#86763=CARTESIAN_POINT('Ctrl Pts',(0.0136314775473348,-0.0345275153362944,
0.0758107012322185));
#86764=CARTESIAN_POINT('Ctrl Pts',(0.0136650676841485,-0.0343603235965185,
0.0756949201420684));
#86765=CARTESIAN_POINT('Ctrl Pts',(0.0136949696833151,-0.034193496108874,
0.0755782839175453));
#86766=CARTESIAN_POINT('',(0.0135942935280005,-0.0346945769586966,0.0759252832829772));
#86767=CARTESIAN_POINT('',(0.013662611390378,-0.0343667727831535,0.0756990307046681));
#86768=CARTESIAN_POINT('Origin',(-0.00245380659277795,-0.0345626457059982,
0.0709097344829956));
#86769=CARTESIAN_POINT('Origin',(0.0243063813591365,-0.0341934771029176,
0.0786757428621937));
#86770=CARTESIAN_POINT('',(0.0136276364306931,-0.034193496108874,0.0758190456948274));
#86771=CARTESIAN_POINT('',(0.013644469743817,-0.034193496108884,0.0757588552506655));
#86772=CARTESIAN_POINT('',(0.0135544173333597,-0.0345211942962613,0.076043760009476));
#86773=CARTESIAN_POINT('Origin',(-0.00229234993127616,-0.0345625596119914,
0.0704568299268693));
#86774=CARTESIAN_POINT('',(0.0135531345566467,-0.0346945769586887,0.07604331268219));
#86775=CARTESIAN_POINT('Origin',(0.0239997435906502,-0.0346945685853902,
0.0796862338863267));
#86776=CARTESIAN_POINT('',(0.0135737140423336,-0.0346945769587026,0.0759842979825937));
#86777=CARTESIAN_POINT('Ctrl Pts',(0.0137074013484012,-0.0345231616327841,
0.0763461778454283));
#86778=CARTESIAN_POINT('Ctrl Pts',(0.0137376725680293,-0.0344132092796987,
0.0762692155164796));
#86779=CARTESIAN_POINT('Ctrl Pts',(0.0137663503207344,-0.0343032738558979,
0.0761916310221329));
#86780=CARTESIAN_POINT('Ctrl Pts',(0.0137934004130336,-0.034193496108874,
0.0761135246981883));
#86781=CARTESIAN_POINT('Ctrl Pts',(0.0136559439950633,-0.0345231616327841,
0.0762452160857041));
#86782=CARTESIAN_POINT('Ctrl Pts',(0.0136848235989764,-0.0344132092796987,
0.076168963023925));
#86783=CARTESIAN_POINT('Ctrl Pts',(0.0137121244783994,-0.0343032738558979,
0.0760921165446263));
#86784=CARTESIAN_POINT('Ctrl Pts',(0.0137378141795643,-0.034193496108874,
0.0760147759929418));
#86785=CARTESIAN_POINT('Ctrl Pts',(0.0136044866417254,-0.0345231616327841,
0.0761442543259799));
#86786=CARTESIAN_POINT('Ctrl Pts',(0.0136319746299235,-0.0344132092796987,
0.0760687105313704));
#86787=CARTESIAN_POINT('Ctrl Pts',(0.0136578986360644,-0.0343032738558979,
0.0759926020671198));
#86788=CARTESIAN_POINT('Ctrl Pts',(0.013682227946095,-0.034193496108874,
0.0759160272876954));
#86789=CARTESIAN_POINT('Ctrl Pts',(0.0135530292883875,-0.0345231616327841,
0.0760432925662557));
#86790=CARTESIAN_POINT('Ctrl Pts',(0.0135791256608706,-0.0344132092796987,
0.0759684580388158));
#86791=CARTESIAN_POINT('Ctrl Pts',(0.0136036727937294,-0.0343032738558979,
0.0758930875896132));
#86792=CARTESIAN_POINT('Ctrl Pts',(0.0136266417126257,-0.034193496108874,
0.0758172785824489));
#86793=CARTESIAN_POINT('',(0.0137105184218707,-0.0341934961088839,0.0759662851965132));
#86794=CARTESIAN_POINT('Ctrl Pts',(0.0137891933503703,-0.0342105180195351,
0.0761256306232581));
#86795=CARTESIAN_POINT('Ctrl Pts',(0.0137486170779876,-0.0342610556240237,
0.0761114809483146));
#86796=CARTESIAN_POINT('Ctrl Pts',(0.0137087689258297,-0.0343122189868,
0.0760975851819707));
#86797=CARTESIAN_POINT('Ctrl Pts',(0.0136304939315549,-0.0344158119695084,
0.0760702892856214));
#86798=CARTESIAN_POINT('Ctrl Pts',(0.0135920991047184,-0.0344681990449961,
0.0760569003199194));
#86799=CARTESIAN_POINT('Ctrl Pts',(0.0135544173333305,-0.0345211942962363,
0.0760437600094589));
#86800=CARTESIAN_POINT('Ctrl Pts',(0.0135924676174683,-0.0346945769586932,
0.075926164996412));
#86801=CARTESIAN_POINT('Ctrl Pts',(0.0136291885719951,-0.034529677707698,
0.075813103794781));
#86802=CARTESIAN_POINT('Ctrl Pts',(0.0136612052255674,-0.034364806625142,
0.0756986214917398));
#86803=CARTESIAN_POINT('Ctrl Pts',(0.0135942935279976,-0.0346945769586932,
0.0759252832829858));
#86804=CARTESIAN_POINT('Ctrl Pts',(0.0136309962537231,-0.034529677707698,
0.0758121843319466));
#86805=CARTESIAN_POINT('Ctrl Pts',(0.0136629931338528,-0.034364806625142,
0.0756976650651667));
#86806=CARTESIAN_POINT('Ctrl Pts',(0.0138985998508835,-0.0346945769586932,
0.075778336887611));
#86807=CARTESIAN_POINT('Ctrl Pts',(0.0139322645638606,-0.034529677707698,
0.0756589466186663));
#86808=CARTESIAN_POINT('Ctrl Pts',(0.0139609660012355,-0.034364806625142,
0.0755382669736921));
#86809=CARTESIAN_POINT('',(0.013902064832892,-0.0346775396665028,0.0757659980595097));
#86810=CARTESIAN_POINT('',(0.0138985998508739,-0.0346945769586886,0.0757783368876127));
#86811=CARTESIAN_POINT('Origin',(-0.00212650686149166,-0.0345626617939533,
0.0714419038548436));
#86812=CARTESIAN_POINT('Ctrl Pts',(0.0139020648315447,-0.0346775396670096,
0.0757659980607406));
#86813=CARTESIAN_POINT('Ctrl Pts',(0.0138606940728663,-0.0346269749928189,
0.0757544280160451));
#86814=CARTESIAN_POINT('Ctrl Pts',(0.0138200585552095,-0.0345757902890797,
0.0757430636314537));
#86815=CARTESIAN_POINT('Ctrl Pts',(0.0137402245826297,-0.034472168108813,
0.0757207366572577));
#86816=CARTESIAN_POINT('Ctrl Pts',(0.0137010574279038,-0.0344197714290103,
0.0757097828154504));
#86817=CARTESIAN_POINT('Ctrl Pts',(0.0136626113904136,-0.0343667727830759,
0.0756990307049232));
#86818=CARTESIAN_POINT('',(0.0137464466894472,-0.0346945769587026,0.075851810085305));
#86819=CARTESIAN_POINT('Origin',(0.00812378219310841,-0.0315241814719618,
0.07415));
#86820=CARTESIAN_POINT('',(0.0139020648319539,-0.0347116136489593,0.0757659980584807));
#86821=CARTESIAN_POINT('',(0.0139055034524797,-0.0346945769586885,0.0757536518571501));
#86822=CARTESIAN_POINT('Origin',(-0.00213689806546748,-0.0345626700684398,
0.0714860074050638));
#86823=CARTESIAN_POINT('Origin',(-0.0020442441421476,-0.0345626620276843,
0.0711477565467771));
#86824=CARTESIAN_POINT('Origin',(-0.00203024708750737,-0.0345626702762116,
0.0711046614002162));
#86825=CARTESIAN_POINT('Ctrl Pts',(0.0136163568087717,-0.0352450361874067,
0.0758559855559169));
#86826=CARTESIAN_POINT('Ctrl Pts',(0.0136806991098211,-0.0349452760959492,
0.0756488297050176));
#86827=CARTESIAN_POINT('Ctrl Pts',(0.0137292547948641,-0.034644428984174,
0.0754374158367021));
#86828=CARTESIAN_POINT('Ctrl Pts',(0.0136170521239378,-0.0352450361874067,
0.0758535581783566));
#86829=CARTESIAN_POINT('Ctrl Pts',(0.0136813028749403,-0.0349452760959492,
0.0756463761032156));
#86830=CARTESIAN_POINT('Ctrl Pts',(0.0137297652947032,-0.034644428984174,
0.0754349429810827));
#86831=CARTESIAN_POINT('Ctrl Pts',(0.0136858952096946,-0.0352450361874067,
0.0756132237664564));
#86832=CARTESIAN_POINT('Ctrl Pts',(0.0137410815996131,-0.0349452760959492,
0.0754034452317301));
#86833=CARTESIAN_POINT('Ctrl Pts',(0.0137803098332277,-0.034644428984174,
0.0751901057910455));
#86834=CARTESIAN_POINT('Ctrl Pts',(0.0136865836405522,-0.0352450361874067,
0.0756108204223374));
#86835=CARTESIAN_POINT('Ctrl Pts',(0.0137416793868598,-0.0349452760959492,
0.0754010159230152));
#86836=CARTESIAN_POINT('Ctrl Pts',(0.013780815278613,-0.034644428984174,
0.0751876574191451));
#86837=CARTESIAN_POINT('',(0.0136949639463645,-0.0351951634053355,0.0755783158525603));
#86838=CARTESIAN_POINT('',(0.0137489462188087,-0.0348678972925388,0.07534818808372));
#86839=CARTESIAN_POINT('Origin',(-0.00272055362522045,-0.0345636767885179,
0.072271462480856));
#86840=CARTESIAN_POINT('Origin',(0.0245563350308239,-0.0346946199340772,
0.0776502168342705));
#86841=CARTESIAN_POINT('',(0.0137215760736043,-0.0346945769330289,0.0754701623649035));
#86842=CARTESIAN_POINT('',(0.0137345967829202,-0.0346945769458128,0.0754090337119125));
#86843=CARTESIAN_POINT('',(0.0136626113902745,-0.0350221583435276,0.0756990307048674));
#86844=CARTESIAN_POINT('Origin',(-0.00266134073650105,-0.0345628458720691,
0.0717943490485694));
#86845=CARTESIAN_POINT('',(0.0136614193974968,-0.0351951360298762,0.0756987004837829));
#86846=CARTESIAN_POINT('Origin',(0.0242732133076599,-0.0351951838366722,
0.0786664730246426));
#86847=CARTESIAN_POINT('',(0.013694969683261,-0.0351951371328746,0.0755782839181704));
#86848=CARTESIAN_POINT('Ctrl Pts',(0.0138342827941664,-0.0350241211494343,
0.0759912449281452));
#86849=CARTESIAN_POINT('Ctrl Pts',(0.0138596451881117,-0.0349144232818962,
0.075912585123762));
#86850=CARTESIAN_POINT('Ctrl Pts',(0.0138833968083085,-0.0348045283579412,
0.0758333539788886));
#86851=CARTESIAN_POINT('Ctrl Pts',(0.0139055034554557,-0.0346945769439158,
0.0757536518464505));
#86852=CARTESIAN_POINT('Ctrl Pts',(0.0137765875104734,-0.0350241211494343,
0.0758937134150676));
#86853=CARTESIAN_POINT('Ctrl Pts',(0.0138006064478156,-0.0349144232818962,
0.0758158483395613));
#86854=CARTESIAN_POINT('Ctrl Pts',(0.0138230302348995,-0.0348045283579412,
0.0757374401694563));
#86855=CARTESIAN_POINT('Ctrl Pts',(0.013843826412436,-0.0346945769439158,
0.0756585882668422));
#86856=CARTESIAN_POINT('Ctrl Pts',(0.0137188922267805,-0.0350241211494342,
0.0757961819019901));
#86857=CARTESIAN_POINT('Ctrl Pts',(0.0137415677075195,-0.0349144232818962,
0.0757191115553607));
#86858=CARTESIAN_POINT('Ctrl Pts',(0.0137626636614904,-0.0348045283579412,
0.075641526360024));
#86859=CARTESIAN_POINT('Ctrl Pts',(0.0137821493694162,-0.0346945769439158,
0.0755635246872338));
#86860=CARTESIAN_POINT('Ctrl Pts',(0.0136611969430875,-0.0350241211494342,
0.0756986503889125));
#86861=CARTESIAN_POINT('Ctrl Pts',(0.0136825289672234,-0.0349144232818962,
0.07562237477116));
#86862=CARTESIAN_POINT('Ctrl Pts',(0.0137022970880814,-0.0348045283579412,
0.0755456125505917));
#86863=CARTESIAN_POINT('Ctrl Pts',(0.0137204723263965,-0.0346945769439158,
0.0754684611076255));
#86864=CARTESIAN_POINT('',(0.0138135397630608,-0.0346945769458128,0.0756119071113357));
#86865=CARTESIAN_POINT('Ctrl Pts',(0.0139020648287818,-0.0347116136492756,
0.0757659980575896));
#86866=CARTESIAN_POINT('Ctrl Pts',(0.0138607105028954,-0.0347621546531205,
0.0757544325952337));
#86867=CARTESIAN_POINT('Ctrl Pts',(0.0138200832978061,-0.0348133084094813,
0.0757430704849581));
#86868=CARTESIAN_POINT('Ctrl Pts',(0.0137402492227238,-0.0349168561544569,
0.0757207434860214));
#86869=CARTESIAN_POINT('Ctrl Pts',(0.013701074019108,-0.0349692089015919,
0.0757097874534179));
#86870=CARTESIAN_POINT('Ctrl Pts',(0.0136626113902445,-0.0350221583434999,
0.0756990307048384));
#86871=CARTESIAN_POINT('Ctrl Pts',(0.0136936947742535,-0.0351951371254986,
0.0755790015719479));
#86872=CARTESIAN_POINT('Ctrl Pts',(0.0137232384851682,-0.0350307338980977,
0.0754638471240117));
#86873=CARTESIAN_POINT('Ctrl Pts',(0.0137479974935673,-0.0348659306897824,
0.0753475700014242));
#86874=CARTESIAN_POINT('Ctrl Pts',(0.0136949696831463,-0.0351951371254986,
0.0755782839181499));
#86875=CARTESIAN_POINT('Ctrl Pts',(0.013724498557019,-0.0350307338980977,
0.0754631031122722));
#86876=CARTESIAN_POINT('Ctrl Pts',(0.0137492416516522,-0.0348659306897824,
0.075346800267497));
#86877=CARTESIAN_POINT('Ctrl Pts',(0.0139086457423704,-0.0351951371254986,
0.0754580043936221));
#86878=CARTESIAN_POINT('Ctrl Pts',(0.0139356879125394,-0.0350307338980977,
0.0753384059692847));
#86879=CARTESIAN_POINT('Ctrl Pts',(0.0139577638434049,-0.0348659306897824,
0.0752177920590261));
#86880=CARTESIAN_POINT('Origin',(0.0189504380659447,-0.0308609197410153,
0.076456131873351));
#86881=CARTESIAN_POINT('',(0.0137881276272136,-0.0351951371254986,0.0755258447573984));
#86882=CARTESIAN_POINT('Origin',(0.0071487010936216,-0.0351840467441095,
0.0740870516087876));
#86883=CARTESIAN_POINT('Origin',(0.0199662307642446,-0.0352322614040111,
0.0758599766870974));
#86884=CARTESIAN_POINT('',(0.0137934500244489,-0.0351951142564686,0.0751157542470464));
#86885=CARTESIAN_POINT('',(0.0138117372268754,-0.0351951372916787,0.0749924176718502));
#86886=CARTESIAN_POINT('Origin',(0.00798966007799802,-0.0352875122926663,
0.073836919555656));
#86887=CARTESIAN_POINT('Origin',(0.00562380347660242,-0.0298325076522691,
0.0812242700469244));
#86888=CARTESIAN_POINT('Origin',(0.0153427804016229,-0.0338732925202731,
0.0784084029538063));
#86889=CARTESIAN_POINT('Ctrl Pts',(0.0121427474513236,-0.0321934096636942,
0.0782641285831352));
#86890=CARTESIAN_POINT('Ctrl Pts',(0.0122163883937301,-0.0320508460845378,
0.078192191018926));
#86891=CARTESIAN_POINT('Ctrl Pts',(0.0122880409902187,-0.0319086045665173,
0.0781183291090622));
#86892=CARTESIAN_POINT('Ctrl Pts',(0.0123575640531126,-0.0317669892871038,
0.0780427145925674));
#86893=CARTESIAN_POINT('Ctrl Pts',(0.0122014382915331,-0.0321934096636942,
0.0782042468839004));
#86894=CARTESIAN_POINT('Ctrl Pts',(0.0122740073800401,-0.0320508460845378,
0.0781312587816013));
#86895=CARTESIAN_POINT('Ctrl Pts',(0.012344560704925,-0.0319086045665173,
0.0780563759243559));
#86896=CARTESIAN_POINT('Ctrl Pts',(0.0124129596264122,-0.0317669892871038,
0.0779797720546076));
#86897=CARTESIAN_POINT('Ctrl Pts',(0.0122601291317424,-0.0321934096636942,
0.0781443651846656));
#86898=CARTESIAN_POINT('Ctrl Pts',(0.0123316263663501,-0.0320508460845379,
0.0780703265442765));
#86899=CARTESIAN_POINT('Ctrl Pts',(0.0124010804196314,-0.0319086045665173,
0.0779944227396497));
#86900=CARTESIAN_POINT('Ctrl Pts',(0.0124683551997119,-0.0317669892871038,
0.0779168295166477));
#86901=CARTESIAN_POINT('Ctrl Pts',(0.0123188199719519,-0.0321934096636942,
0.0780844834854308));
#86902=CARTESIAN_POINT('Ctrl Pts',(0.0123892453526602,-0.0320508460845379,
0.0780093943069517));
#86903=CARTESIAN_POINT('Ctrl Pts',(0.0124576001343378,-0.0319086045665173,
0.0779324695549435));
#86904=CARTESIAN_POINT('Ctrl Pts',(0.0125237507730115,-0.0317669892871038,
0.0778538869786879));
#86905=CARTESIAN_POINT('',(0.0123177699812209,-0.0321934096636942,0.0780855547808618));
#86906=CARTESIAN_POINT('',(0.0124759194928693,-0.0318665617511361,0.0779099236579099));
#86907=CARTESIAN_POINT('Origin',(0.000561737037247611,-0.0326371944419988,
0.0662106402855537));
#86908=CARTESIAN_POINT('Origin',(0.0207704093038825,-0.0316939261509443,
0.0850757473283274));
#86909=CARTESIAN_POINT('',(0.0122313956286931,-0.0320197221621762,0.0781755559902131));
#86910=CARTESIAN_POINT('Ctrl Pts',(0.0122315545130972,-0.0320197392094677,
0.0781754612768234));
#86911=CARTESIAN_POINT('Ctrl Pts',(0.0122520373207006,-0.0319792716575975,
0.0781545595777905));
#86912=CARTESIAN_POINT('Ctrl Pts',(0.0122724540276985,-0.0319386439829667,
0.078133406573588));
#86913=CARTESIAN_POINT('Ctrl Pts',(0.0122928199824309,-0.03189790993816,
0.0781119741840404));
#86914=CARTESIAN_POINT('Ctrl Pts',(0.012313185534615,-0.031857176698492,
0.07809054221812));
#86915=CARTESIAN_POINT('Ctrl Pts',(0.0123333981170701,-0.0318163871833588,
0.0780689410364438));
#86916=CARTESIAN_POINT('Ctrl Pts',(0.0123533907779421,-0.0317755399638303,
0.0780472473439951));
#86917=CARTESIAN_POINT('',(0.0122302737564742,-0.0321934096636183,0.078174826336627));
#86918=CARTESIAN_POINT('Origin',(0.0138933921029899,-0.032411245654862,
0.0797754222134512));
#86919=CARTESIAN_POINT('',(0.0122740218688575,-0.0321934096636663,0.0781301905587545));
#86920=CARTESIAN_POINT('Ctrl Pts',(0.0123157418607905,-0.0321934096636618,
0.0780855751499363));
#86921=CARTESIAN_POINT('Ctrl Pts',(0.012370016509316,-0.0320835708272592,
0.0780277647590967));
#86922=CARTESIAN_POINT('Ctrl Pts',(0.0124230632933058,-0.0319739230346488,
0.0779688646896027));
#86923=CARTESIAN_POINT('Ctrl Pts',(0.0124748201266384,-0.0318646057455573,
0.0779089555088152));
#86924=CARTESIAN_POINT('Ctrl Pts',(0.0124290550093506,-0.0321934096636618,
0.0780844371125261));
#86925=CARTESIAN_POINT('Ctrl Pts',(0.0124833139634533,-0.0320835708272592,
0.0780250640450567));
#86926=CARTESIAN_POINT('Ctrl Pts',(0.012536312722612,-0.0319739230346488,
0.0779646025301442));
#86927=CARTESIAN_POINT('Ctrl Pts',(0.0125879894154724,-0.0318646057455573,
0.0779031351281948));
#86928=CARTESIAN_POINT('Ctrl Pts',(0.0125423681579107,-0.0321934096636618,
0.0780832990751159));
#86929=CARTESIAN_POINT('Ctrl Pts',(0.0125966114175906,-0.0320835708272592,
0.0780223633310167));
#86930=CARTESIAN_POINT('Ctrl Pts',(0.0126495621519182,-0.0319739230346488,
0.0779603403706857));
#86931=CARTESIAN_POINT('Ctrl Pts',(0.0127011587043063,-0.0318646057455573,
0.0778973147475744));
#86932=CARTESIAN_POINT('Ctrl Pts',(0.0126556813064708,-0.0321934096636618,
0.0780821610377056));
#86933=CARTESIAN_POINT('Ctrl Pts',(0.0127099088717279,-0.0320835708272592,
0.0780196626169768));
#86934=CARTESIAN_POINT('Ctrl Pts',(0.0127628115812245,-0.0319739230346488,
0.0779560782112272));
#86935=CARTESIAN_POINT('Ctrl Pts',(0.0128143279931403,-0.0318646057455573,
0.077891494366954));
#86936=CARTESIAN_POINT('',(0.0126640701329279,-0.0321763980308326,0.0780724718483922));
#86937=CARTESIAN_POINT('',(0.0126556813064761,-0.0321934096636185,0.0780821610376811));
#86938=CARTESIAN_POINT('Origin',(0.000551872876335866,-0.0326386231316345,
0.0667976872454305));
#86939=CARTESIAN_POINT('Ctrl Pts',(0.0126640701305228,-0.0321763980306375,
0.0780724718463136));
#86940=CARTESIAN_POINT('Ctrl Pts',(0.0126315927749162,-0.0321259596176189,
0.0780444138211916));
#86941=CARTESIAN_POINT('Ctrl Pts',(0.0125996781316311,-0.0320749164634115,
0.0780168419377658));
#86942=CARTESIAN_POINT('Ctrl Pts',(0.0125369485855449,-0.0319716057794027,
0.0779626482650633));
#86943=CARTESIAN_POINT('Ctrl Pts',(0.0125061581245192,-0.031919378669023,
0.0779360475916668));
#86944=CARTESIAN_POINT('Ctrl Pts',(0.0124759194914615,-0.0318665617525441,
0.0779099236566928));
#86945=CARTESIAN_POINT('',(0.0124867256438585,-0.0321934096636663,0.0780838579092815));
#86946=CARTESIAN_POINT('Origin',(0.00812378219310841,-0.0315241814719618,
0.07415));
#86947=CARTESIAN_POINT('',(0.0126640701332069,-0.0322104233323761,0.0780724718486335));
#86948=CARTESIAN_POINT('',(0.0126724382467512,-0.0321934096636183,0.078062764764929));
#86949=CARTESIAN_POINT('Origin',(0.000517747781834131,-0.0326387244823149,
0.0668275286705876));
#86950=CARTESIAN_POINT('Origin',(-0.000250277107460089,-0.0326386235201794,
0.0677261798898456));
#86951=CARTESIAN_POINT('Origin',(-0.00022570672338414,-0.0326387249176944,
0.0676880839863557));
#86952=CARTESIAN_POINT('Ctrl Pts',(0.0123688711055919,-0.0327445246967096,
0.0780303795078716));
#86953=CARTESIAN_POINT('Ctrl Pts',(0.0125152220112444,-0.032443687833936,
0.0778702733621565));
#86954=CARTESIAN_POINT('Ctrl Pts',(0.0126490973001736,-0.0321434074405927,
0.0776995983127345));
#86955=CARTESIAN_POINT('Ctrl Pts',(0.0125334930880667,-0.0327445246967096,
0.0778422316859708));
#86956=CARTESIAN_POINT('Ctrl Pts',(0.0126727478826105,-0.032443687833936,
0.0776759167206861));
#86957=CARTESIAN_POINT('Ctrl Pts',(0.0127990795460675,-0.0321434074405927,
0.0774995849983862));
#86958=CARTESIAN_POINT('',(0.0125566096336387,-0.0326943950436612,0.0778144461904198));
#86959=CARTESIAN_POINT('',(0.0127034191046726,-0.0323666188837389,0.0776292313458923));
#86960=CARTESIAN_POINT('Origin',(-0.000448633507967139,-0.0326395579110996,
0.0671621361566276));
#86961=CARTESIAN_POINT('Origin',(0.0214979151808044,-0.0321933825603007,
0.0843105643423937));
#86962=CARTESIAN_POINT('',(0.012626719740879,-0.0321934096532689,0.0777279433251215));
#86963=CARTESIAN_POINT('',(0.0126645285418757,-0.0321934096584275,0.0776781764193205));
#86964=CARTESIAN_POINT('',(0.012475919493572,-0.0325210109756239,0.0779099236585222));
#86965=CARTESIAN_POINT('Origin',(-0.000123152820681168,-0.0326393129157583,
0.0668082339780196));
#86966=CARTESIAN_POINT('',(0.0124748914701047,-0.0326943950436593,0.0779090355225293));
#86967=CARTESIAN_POINT('Origin',(0.0208460127915698,-0.032694376553814,
0.085141064595157));
#86968=CARTESIAN_POINT('',(0.0125157505518817,-0.0326943950436702,0.0778617408564845));
#86969=CARTESIAN_POINT('Ctrl Pts',(0.0125068329018791,-0.0325229783203769,
0.0782474219314632));
#86970=CARTESIAN_POINT('Ctrl Pts',(0.0125633157735996,-0.032413025309245,
0.0781870016732939));
#86971=CARTESIAN_POINT('Ctrl Pts',(0.0126185402079304,-0.0323031222208069,
0.0781254221582815));
#86972=CARTESIAN_POINT('Ctrl Pts',(0.0126724382496766,-0.0321934096576658,
0.0780627647615384));
#86973=CARTESIAN_POINT('Ctrl Pts',(0.0124961555676023,-0.0325229783203769,
0.0781346073190692));
#86974=CARTESIAN_POINT('Ctrl Pts',(0.012551083292358,-0.032413025309245,
0.0780743342477194));
#86975=CARTESIAN_POINT('Ctrl Pts',(0.012604755860341,-0.0323031222208069,
0.0780129340674154));
#86976=CARTESIAN_POINT('Ctrl Pts',(0.0126571072960809,-0.0321934096576658,
0.0779504878534107));
#86977=CARTESIAN_POINT('Ctrl Pts',(0.0124854782333254,-0.0325229783203769,
0.0780217927066752));
#86978=CARTESIAN_POINT('Ctrl Pts',(0.0125388508111164,-0.032413025309245,
0.0779616668221448));
#86979=CARTESIAN_POINT('Ctrl Pts',(0.0125909715127516,-0.0323031222208069,
0.0779004459765494));
#86980=CARTESIAN_POINT('Ctrl Pts',(0.0126417763424852,-0.0321934096576658,
0.077838210945283));
#86981=CARTESIAN_POINT('Ctrl Pts',(0.0124748008990486,-0.0325229783203769,
0.0779089780942812));
#86982=CARTESIAN_POINT('Ctrl Pts',(0.0125266183298748,-0.032413025309245,
0.0778489993965703));
#86983=CARTESIAN_POINT('Ctrl Pts',(0.0125771871651622,-0.0323031222208069,
0.0777879578856833));
#86984=CARTESIAN_POINT('Ctrl Pts',(0.0126264453888895,-0.0321934096576658,
0.0777259340371553));
#86985=CARTESIAN_POINT('',(0.0126495789936254,-0.0321934096584274,0.077895354045503));
#86986=CARTESIAN_POINT('Ctrl Pts',(0.0126640701305689,-0.0322104233328896,
0.0780724718463536));
#86987=CARTESIAN_POINT('Ctrl Pts',(0.0126315487675926,-0.032260942183051,
0.0780443758021299));
#86988=CARTESIAN_POINT('Ctrl Pts',(0.0125996126259685,-0.0323120888238984,
0.0780167853457256));
#86989=CARTESIAN_POINT('Ctrl Pts',(0.0125368826049921,-0.0324156524631807,
0.0779625912627532));
#86990=CARTESIAN_POINT('Ctrl Pts',(0.0125061145111221,-0.0324680267167311,
0.0779360099129284));
#86991=CARTESIAN_POINT('Ctrl Pts',(0.0124759194935421,-0.0325210109755912,
0.0779099236584905));
#86992=CARTESIAN_POINT('Origin',(0.00230059941656284,-0.0262834582510572,
0.079440928859173));
#86993=CARTESIAN_POINT('Origin',(0.0127962631772917,-0.0342770831689207,
0.0853745949748125));
#86994=CARTESIAN_POINT('Ctrl Pts',(0.0125545872851655,-0.0326943950436604,
0.0778145938301346));
#86995=CARTESIAN_POINT('Ctrl Pts',(0.0126050922563256,-0.0325844576448134,
0.0777535290317522));
#86996=CARTESIAN_POINT('Ctrl Pts',(0.0126543378816533,-0.0324744968375323,
0.0776914153861116));
#86997=CARTESIAN_POINT('Ctrl Pts',(0.012702262162479,-0.0323646534831895,
0.0776283333471264));
#86998=CARTESIAN_POINT('Ctrl Pts',(0.012667605214521,-0.0326943950436604,
0.0778063430588587));
#86999=CARTESIAN_POINT('Ctrl Pts',(0.0127179964745893,-0.0325844576448134,
0.0777437206615916));
#87000=CARTESIAN_POINT('Ctrl Pts',(0.0127670961670791,-0.0324744968375323,
0.0776800516585644));
#87001=CARTESIAN_POINT('Ctrl Pts',(0.0128148425077852,-0.0323646534831895,
0.0776154184939263));
#87002=CARTESIAN_POINT('Ctrl Pts',(0.0127806231438765,-0.0326943950436604,
0.0777980922875828));
#87003=CARTESIAN_POINT('Ctrl Pts',(0.012830900692853,-0.0325844576448134,
0.077733912291431));
#87004=CARTESIAN_POINT('Ctrl Pts',(0.0128798544525049,-0.0324744968375323,
0.0776686879310172));
#87005=CARTESIAN_POINT('Ctrl Pts',(0.0129274228530915,-0.0323646534831895,
0.0776025036407263));
#87006=CARTESIAN_POINT('Ctrl Pts',(0.012893641073232,-0.0326943950436604,
0.0777898415163069));
#87007=CARTESIAN_POINT('Ctrl Pts',(0.0129438049111168,-0.0325844576448134,
0.0777241039212704));
#87008=CARTESIAN_POINT('Ctrl Pts',(0.0129926127379307,-0.0324744968375323,
0.07765732420347));
#87009=CARTESIAN_POINT('Ctrl Pts',(0.0130400031983977,-0.0323646534831895,
0.0775895887875262));
#87010=CARTESIAN_POINT('',(0.0129014049571702,-0.0326773559991391,0.0777796447077724));
#87011=CARTESIAN_POINT('',(0.0128936410732186,-0.0326943950436595,0.0777898415163072));
#87012=CARTESIAN_POINT('Origin',(-0.000351172866345553,-0.0326395670215677,
0.0677745215341868));
#87013=CARTESIAN_POINT('Ctrl Pts',(0.0129014049544966,-0.0326773559987503,
0.07777964470574));
#87014=CARTESIAN_POINT('Ctrl Pts',(0.0128672024057852,-0.0326267922587135,
0.0777536604231683));
#87015=CARTESIAN_POINT('Ctrl Pts',(0.0128336060725491,-0.0325756109581668,
0.0777281366932396));
#87016=CARTESIAN_POINT('Ctrl Pts',(0.0127675972446041,-0.0324719985462389,
0.0776779886164975));
#87017=CARTESIAN_POINT('Ctrl Pts',(0.0127352112244493,-0.0324196091621776,
0.0776533843828722));
#87018=CARTESIAN_POINT('Ctrl Pts',(0.0127034191046338,-0.0323666188837756,
0.0776292313458628));
#87019=CARTESIAN_POINT('',(0.0127251253534387,-0.0326943950436703,0.0778021438533735));
#87020=CARTESIAN_POINT('Origin',(0.00812378219310841,-0.0315241814719618,
0.07415));
#87021=CARTESIAN_POINT('',(0.0129014049571333,-0.0327114338380031,0.0777796447077446));
#87022=CARTESIAN_POINT('',(0.0129091470454567,-0.0326943950436593,0.0777694313406825));
#87023=CARTESIAN_POINT('Origin',(-0.00037795912897998,-0.0326395681488619,
0.0678110648869237));
#87024=CARTESIAN_POINT('Origin',(-0.000290388076978256,-0.0326395672708735,
0.0676945109721873));
#87025=CARTESIAN_POINT('Origin',(-0.000262362806127849,-0.0326395685118704,
0.0676589091060391));
#87026=CARTESIAN_POINT('Ctrl Pts',(0.0126041700312253,-0.0332451089994432,
0.0777561405713108));
#87027=CARTESIAN_POINT('Ctrl Pts',(0.0127401778480767,-0.0329451141710253,
0.077587159979329));
#87028=CARTESIAN_POINT('Ctrl Pts',(0.0128630709720886,-0.0326442513127493,
0.0774084147786052));
#87029=CARTESIAN_POINT('Ctrl Pts',(0.0127566519192198,-0.0332451089994432,
0.0775580262764363));
#87030=CARTESIAN_POINT('Ctrl Pts',(0.0128851877331916,-0.0329451141710253,
0.0773832947359585));
#87031=CARTESIAN_POINT('Ctrl Pts',(0.0130001968965448,-0.0326442513127493,
0.0771993777463787));
#87032=CARTESIAN_POINT('Ctrl Pts',(0.0127581767380997,-0.0332451089994432,
0.0775560451334876));
#87033=CARTESIAN_POINT('Ctrl Pts',(0.0128866378320428,-0.0329451141710253,
0.0773812560835247));
#87034=CARTESIAN_POINT('Ctrl Pts',(0.0130015681557894,-0.0326442513127493,
0.0771972873760565));
#87035=CARTESIAN_POINT('',(0.0127779549413521,-0.0331951640388616,0.0775288757049508));
#87036=CARTESIAN_POINT('',(0.0129128449938955,-0.0328677532355046,0.0773348080884048));
#87037=CARTESIAN_POINT('Origin',(-0.0012249331354173,-0.0326402808281172,
0.0683119687951164));
#87038=CARTESIAN_POINT('Origin',(0.0221191769029498,-0.0326944278779093,
0.0834567224738829));
#87039=CARTESIAN_POINT('',(0.012842495146412,-0.0326943950436593,0.0774381412780363));
#87040=CARTESIAN_POINT('',(0.0128771044486979,-0.0326943950436693,0.0773860985437217));
#87041=CARTESIAN_POINT('',(0.0127034191046709,-0.0330220786163545,0.0776292313458946));
#87042=CARTESIAN_POINT('Origin',(-0.000985430167367684,-0.0326396682762316,
0.067895086349666));
#87043=CARTESIAN_POINT('',(0.0127023373432517,-0.0331951640388587,0.0776284095125642));
#87044=CARTESIAN_POINT('Origin',(0.0214865161934399,-0.0331952026560077,
0.0843019072061792));
#87045=CARTESIAN_POINT('',(0.0127401461423119,-0.0331951640388701,0.0775786426087675));
#87046=CARTESIAN_POINT('Ctrl Pts',(0.0127554638151504,-0.0330240426238172,
0.0779641218323661));
#87047=CARTESIAN_POINT('Ctrl Pts',(0.0128080070593101,-0.0329142774063519,
0.0779003159055937));
#87048=CARTESIAN_POINT('Ctrl Pts',(0.0128592574514538,-0.0328043479726691,
0.0778353919536107));
#87049=CARTESIAN_POINT('Ctrl Pts',(0.0129091470454586,-0.0326943950436593,
0.0777694313406921));
#87050=CARTESIAN_POINT('Ctrl Pts',(0.0127377238484254,-0.0330240426238172,
0.0778522002992919));
#87051=CARTESIAN_POINT('Ctrl Pts',(0.0127887252644271,-0.0329142774063519,
0.0777886387578444));
#87052=CARTESIAN_POINT('Ctrl Pts',(0.0128384381118826,-0.0328043479726691,
0.0777239911869161));
#87053=CARTESIAN_POINT('Ctrl Pts',(0.0128867964241291,-0.0326943950436593,
0.0776583386509629));
#87054=CARTESIAN_POINT('Ctrl Pts',(0.0127199838817004,-0.0330240426238172,
0.0777402787662177));
#87055=CARTESIAN_POINT('Ctrl Pts',(0.0127694434695442,-0.032914277406352,
0.077676961610095));
#87056=CARTESIAN_POINT('Ctrl Pts',(0.0128176187723115,-0.0328043479726691,
0.0776125904202215));
#87057=CARTESIAN_POINT('Ctrl Pts',(0.0128644458027996,-0.0326943950436593,
0.0775472459612337));
#87058=CARTESIAN_POINT('Ctrl Pts',(0.0127022439149754,-0.0330240426238172,
0.0776283572331435));
#87059=CARTESIAN_POINT('Ctrl Pts',(0.0127501616746612,-0.032914277406352,
0.0775652844623457));
#87060=CARTESIAN_POINT('Ctrl Pts',(0.0127967994327403,-0.0328043479726691,
0.0775011896535269));
#87061=CARTESIAN_POINT('Ctrl Pts',(0.0128420951814701,-0.0326943950436593,
0.0774361532715045));
#87062=CARTESIAN_POINT('',(0.0128758210959444,-0.0326943950436693,0.0776037863093694));
#87063=CARTESIAN_POINT('Ctrl Pts',(0.0129014049544878,-0.0327114338383289,
0.0777796447057335));
#87064=CARTESIAN_POINT('Ctrl Pts',(0.0128672080947621,-0.0327619876830131,
0.077753664745185));
#87065=CARTESIAN_POINT('Ctrl Pts',(0.0128336145402828,-0.0328131562602634,
0.077728143126327));
#87066=CARTESIAN_POINT('Ctrl Pts',(0.0127676057729972,-0.0329167375858765,
0.0776779950956691));
#87067=CARTESIAN_POINT('Ctrl Pts',(0.012735216861643,-0.0329691088920629,
0.0776533886655483));
#87068=CARTESIAN_POINT('Ctrl Pts',(0.0127034191046347,-0.0330220786163187,
0.0776292313458637));
#87069=CARTESIAN_POINT('Ctrl Pts',(0.0127759455331478,-0.0331951640388604,
0.0775291500814413));
#87070=CARTESIAN_POINT('Ctrl Pts',(0.0128458072945721,-0.0330306422010619,
0.0774329695870756));
#87071=CARTESIAN_POINT('Ctrl Pts',(0.0129116341186329,-0.0328657861914645,
0.0773339838182005));
#87072=CARTESIAN_POINT('Ctrl Pts',(0.0127779549413502,-0.0331951640388604,
0.0775288757049533));
#87073=CARTESIAN_POINT('Ctrl Pts',(0.0128478110302165,-0.0330306422010619,
0.0774326536673613));
#87074=CARTESIAN_POINT('Ctrl Pts',(0.0129136304695413,-0.0328657861914645,
0.0773336266252111));
#87075=CARTESIAN_POINT('Ctrl Pts',(0.013112776386117,-0.0331951640388604,
0.0774831572033527));
#87076=CARTESIAN_POINT('Ctrl Pts',(0.0131816872742748,-0.0330306422010619,
0.0773800129470578));
#87077=CARTESIAN_POINT('Ctrl Pts',(0.0132462762179797,-0.0328657861914645,
0.0772741086673313));
#87078=CARTESIAN_POINT('',(0.0131198846876255,-0.0331781648281957,0.0774724930188458));
#87079=CARTESIAN_POINT('',(0.0131127763861026,-0.0331951640388588,0.0774831572033539));
#87080=CARTESIAN_POINT('Origin',(-0.0010195947541991,-0.0326412093102044,
0.0689248852377839));
#87081=CARTESIAN_POINT('Ctrl Pts',(0.0131198846858996,-0.033178164828644,
0.0774724930195014));
#87082=CARTESIAN_POINT('Ctrl Pts',(0.0130840934308751,-0.0331276811546766,
0.0774486912415261));
#87083=CARTESIAN_POINT('Ctrl Pts',(0.0130489484363515,-0.0330765663497776,
0.0774253192781101));
#87084=CARTESIAN_POINT('Ctrl Pts',(0.0129799208623961,-0.0329730614463504,
0.0773794147647705));
#87085=CARTESIAN_POINT('Ctrl Pts',(0.0129460661715751,-0.0329207133374634,
0.0773569007548111));
#87086=CARTESIAN_POINT('Ctrl Pts',(0.0129128449934111,-0.0328677532289399,
0.0773348081048698));
#87087=CARTESIAN_POINT('',(0.0129453656637373,-0.0331951640388702,0.0775060164541623));
#87088=CARTESIAN_POINT('Origin',(0.00812378219310841,-0.0315241814719618,
0.07415));
#87089=CARTESIAN_POINT('',(0.0131198846866907,-0.0332121607144205,0.0774724930174478));
#87090=CARTESIAN_POINT('',(0.0131269701953153,-0.0331951640388587,0.0774618136744959));
#87091=CARTESIAN_POINT('Origin',(-0.00103779367125268,-0.0326413666455162,
0.0689664173061276));
#87092=CARTESIAN_POINT('Origin',(-0.000230762201290447,-0.0326412093881342,
0.0677386999905375));
#87093=CARTESIAN_POINT('Origin',(-0.000199498376431669,-0.0326413668167375,
0.0677058564566509));
#87094=CARTESIAN_POINT('Ctrl Pts',(0.0128217484324243,-0.0337436976235975,
0.0774677158127615));
#87095=CARTESIAN_POINT('Ctrl Pts',(0.0128515884712579,-0.0336723290703325,
0.0774254615924088));
#87096=CARTESIAN_POINT('Ctrl Pts',(0.0128806636624346,-0.033601104548885,
0.0773826774795486));
#87097=CARTESIAN_POINT('Ctrl Pts',(0.0129734949883911,-0.0333736987606857,
0.0772460762822411));
#87098=CARTESIAN_POINT('Ctrl Pts',(0.0130583343713293,-0.0331450831799192,
0.077104372996156));
#87099=CARTESIAN_POINT('Ctrl Pts',(0.0129614904835795,-0.0337436976235975,
0.0772604185403749));
#87100=CARTESIAN_POINT('Ctrl Pts',(0.0129894660593284,-0.0336723290703325,
0.0772169074588357));
#87101=CARTESIAN_POINT('Ctrl Pts',(0.0130166544820755,-0.033601104548885,
0.0771729002239336));
#87102=CARTESIAN_POINT('Ctrl Pts',(0.013103461730184,-0.0333736987606857,
0.0770323938402334));
#87103=CARTESIAN_POINT('Ctrl Pts',(0.0131820628603656,-0.0331450831799192,
0.0768871374995152));
#87104=CARTESIAN_POINT('Ctrl Pts',(0.012962887904091,-0.0337436976235975,
0.077258345567651));
#87105=CARTESIAN_POINT('Ctrl Pts',(0.0129908448352091,-0.0336723290703325,
0.0772148219174999));
#87106=CARTESIAN_POINT('Ctrl Pts',(0.0130180143902719,-0.033601104548885,
0.0771708024513775));
#87107=CARTESIAN_POINT('Ctrl Pts',(0.0131047613976019,-0.0333736987606857,
0.0770302570158134));
#87108=CARTESIAN_POINT('Ctrl Pts',(0.0131833001452559,-0.0331450831799192,
0.0768849651445488));
#87109=CARTESIAN_POINT('',(0.0129809323555244,-0.0336938721132548,0.0772299703407246));
#87110=CARTESIAN_POINT('',(0.0131033706183091,-0.0333679869945434,0.0770278158585576));
#87111=CARTESIAN_POINT('Ctrl Pts',(0.0129809323555235,-0.033693872113265,
0.0772299703407274));
#87112=CARTESIAN_POINT('Ctrl Pts',(0.0129929549246028,-0.0336629187933933,
0.0772110106051136));
#87113=CARTESIAN_POINT('Ctrl Pts',(0.0130048626317031,-0.0336319952301041,
0.077191986536299));
#87114=CARTESIAN_POINT('Ctrl Pts',(0.013016654482074,-0.0336011045488951,
0.0771729002239361));
#87115=CARTESIAN_POINT('Ctrl Pts',(0.0130462442695989,-0.0335235892595455,
0.0771250061352493));
#87116=CARTESIAN_POINT('Ctrl Pts',(0.0130751569819193,-0.033445866866037,
0.0770766349299063));
#87117=CARTESIAN_POINT('Ctrl Pts',(0.0131033706185681,-0.0333679869945386,
0.0770278158587149));
#87118=CARTESIAN_POINT('Ctrl Pts',(0.0131033934652619,-0.0333679692459665,
0.0770277776998562));
#87119=CARTESIAN_POINT('Ctrl Pts',(0.0131029981019756,-0.0333391895373163,
0.0770275560566834));
#87120=CARTESIAN_POINT('Ctrl Pts',(0.0131027001700079,-0.0333104081057696,
0.0770273927567706));
#87121=CARTESIAN_POINT('Ctrl Pts',(0.0131023031435285,-0.0332532697426299,
0.0770271814578659));
#87122=CARTESIAN_POINT('Ctrl Pts',(0.013102201146355,-0.0332249167276877,
0.0770271317795956));
#87123=CARTESIAN_POINT('Ctrl Pts',(0.0131021945177025,-0.0331960985527834,
0.0770271359141604));
#87124=CARTESIAN_POINT('Ctrl Pts',(0.0131021944358776,-0.0331956312395902,
0.0770271359962724));
#87125=CARTESIAN_POINT('Ctrl Pts',(0.0131021943802153,-0.0331951640388594,
0.0770271360925869));
#87126=CARTESIAN_POINT('',(0.0130396479434198,-0.0331951640388587,0.0771353624444808));
#87127=CARTESIAN_POINT('',(0.0130709211618275,-0.0331951640388687,0.077081249268544));
#87128=CARTESIAN_POINT('',(0.0129128449807048,-0.0335216366567648,0.0773348080965793));
#87129=CARTESIAN_POINT('Origin',(-0.00158890560126417,-0.0326434571530048,
0.0691451869164799));
#87130=CARTESIAN_POINT('',(0.0129117137509639,-0.0336938721132327,0.0773340558093871));
#87131=CARTESIAN_POINT('Origin',(0.0220050936674813,-0.0336938867896241,
0.0833813090403592));
#87132=CARTESIAN_POINT('',(0.0129463230532542,-0.0336938721132538,0.0772820130750659));
#87133=CARTESIAN_POINT('Ctrl Pts',(0.0129858155040267,-0.0335235895815172,
0.0776657690600517));
#87134=CARTESIAN_POINT('Ctrl Pts',(0.0130342169870506,-0.0334144449262748,
0.0775988335990642));
#87135=CARTESIAN_POINT('Ctrl Pts',(0.0130812912412651,-0.0333049234473147,
0.0775308212991283));
#87136=CARTESIAN_POINT('Ctrl Pts',(0.013126970195318,-0.0331951640388587,
0.0774618136745056));
#87137=CARTESIAN_POINT('Ctrl Pts',(0.0129610828790003,-0.0335235895815172,
0.0775551821270721));
#87138=CARTESIAN_POINT('Ctrl Pts',(0.0130079619151661,-0.0334144449262748,
0.0774885871593622));
#87139=CARTESIAN_POINT('Ctrl Pts',(0.0130535190077504,-0.0333049234473147,
0.0774209471964957));
#87140=CARTESIAN_POINT('Ctrl Pts',(0.0130976880685124,-0.0331951640388587,
0.0773523434523616));
#87141=CARTESIAN_POINT('Ctrl Pts',(0.0129363502539739,-0.0335235895815172,
0.0774445951940926));
#87142=CARTESIAN_POINT('Ctrl Pts',(0.0129817068432816,-0.0334144449262748,
0.0773783407196602));
#87143=CARTESIAN_POINT('Ctrl Pts',(0.0130257467742356,-0.0333049234473147,
0.0773110730938632));
#87144=CARTESIAN_POINT('Ctrl Pts',(0.0130684059417069,-0.0331951640388587,
0.0772428732302176));
#87145=CARTESIAN_POINT('Ctrl Pts',(0.0129116176289475,-0.0335235895815172,
0.0773340082611131));
#87146=CARTESIAN_POINT('Ctrl Pts',(0.0129554517713971,-0.0334144449262748,
0.0772680942799582));
#87147=CARTESIAN_POINT('Ctrl Pts',(0.0129979745407209,-0.0333049234473147,
0.0772011989912306));
#87148=CARTESIAN_POINT('Ctrl Pts',(0.0130391238149014,-0.0331951640388587,
0.0771334030080735));
#87149=CARTESIAN_POINT('',(0.0130833090693776,-0.0331951640388687,0.0772985880594984));
#87150=CARTESIAN_POINT('Ctrl Pts',(0.013119884684077,-0.0332121607145942,
0.0774724930157079));
#87151=CARTESIAN_POINT('Ctrl Pts',(0.01308415364584,-0.0332625444108875,
0.0774487312683857));
#87152=CARTESIAN_POINT('Ctrl Pts',(0.0130490383094607,-0.0333135300745053,
0.0774253789732565));
#87153=CARTESIAN_POINT('Ctrl Pts',(0.0129800111660968,-0.0334167203140531,
0.0773794747504879));
#87154=CARTESIAN_POINT('Ctrl Pts',(0.012946126094066,-0.0334688847587198,
0.0773569406020467));
#87155=CARTESIAN_POINT('Ctrl Pts',(0.0129128449802051,-0.033521636656226,
0.0773348080960466));
#87156=CARTESIAN_POINT('Ctrl Pts',(0.0129799521394177,-0.033693872113239,
0.0772301675493867));
#87157=CARTESIAN_POINT('Ctrl Pts',(0.0129979813821922,-0.0336474569764958,
0.0772017427752429));
#87158=CARTESIAN_POINT('Ctrl Pts',(0.0130156766417212,-0.033601104548885,
0.0771731088937324));
#87159=CARTESIAN_POINT('Ctrl Pts',(0.0130604769704531,-0.0334837508592656,
0.0771006144890902));
#87160=CARTESIAN_POINT('Ctrl Pts',(0.0131031094666671,-0.0333660264659097,
0.0770268243920209));
#87161=CARTESIAN_POINT('Ctrl Pts',(0.0129809323555133,-0.033693872113239,
0.077229970340742));
#87162=CARTESIAN_POINT('Ctrl Pts',(0.0129989604439602,-0.0336474569764958,
0.0772015398290681));
#87163=CARTESIAN_POINT('Ctrl Pts',(0.0130166544820755,-0.033601104548885,
0.0771729002239336));
#87164=CARTESIAN_POINT('Ctrl Pts',(0.0130614517184691,-0.0334837508592656,
0.0771003913283911));
#87165=CARTESIAN_POINT('Ctrl Pts',(0.0131040806943073,-0.0333660264659097,
0.0770265868384173));
#87166=CARTESIAN_POINT('Ctrl Pts',(0.0133142101585596,-0.033693872113239,
0.0771629185302985));
#87167=CARTESIAN_POINT('Ctrl Pts',(0.0133318457705099,-0.0336474569764958,
0.07713253723305));
#87168=CARTESIAN_POINT('Ctrl Pts',(0.0133491245226131,-0.033601104548885,
0.0771019515704431));
#87169=CARTESIAN_POINT('Ctrl Pts',(0.0133928703503042,-0.0334837508592656,
0.0770245157048068));
#87170=CARTESIAN_POINT('Ctrl Pts',(0.0134343023828019,-0.0333660264659097,
0.0769458175637212));
#87171=CARTESIAN_POINT('',(0.0133186470840024,-0.0336769361243753,0.0771522289661778));
#87172=CARTESIAN_POINT('',(0.0133122224181615,-0.0336938721132327,0.0771633184416936));
#87173=CARTESIAN_POINT('Ctrl Pts',(0.0133186470840025,-0.0336769361243749,
0.0771522289661776));
#87174=CARTESIAN_POINT('Ctrl Pts',(0.0133175782002636,-0.0336797586670132,
0.0771540784942017));
#87175=CARTESIAN_POINT('Ctrl Pts',(0.0133165083692196,-0.0336825812713061,
0.0771559273814434));
#87176=CARTESIAN_POINT('Ctrl Pts',(0.0133143668181204,-0.0336882265895377,
0.0771596238657232));
#87177=CARTESIAN_POINT('Ctrl Pts',(0.0133132950980859,-0.0336910493035001,
0.0771614714627857));
#87178=CARTESIAN_POINT('Ctrl Pts',(0.0133122224181737,-0.0336938721132372,
0.0771633184416937));
#87179=CARTESIAN_POINT('Ctrl Pts',(0.0133186470840023,-0.0336769361243753,
0.0771522289661778));
#87180=CARTESIAN_POINT('Ctrl Pts',(0.013282359462025,-0.0336279031301491,
0.0771312575353318));
#87181=CARTESIAN_POINT('Ctrl Pts',(0.0132455497517024,-0.033576785189935,
0.0771099843779186));
#87182=CARTESIAN_POINT('Ctrl Pts',(0.013173422021026,-0.033473319885733,
0.0770683001441899));
#87183=CARTESIAN_POINT('Ctrl Pts',(0.0131380555712316,-0.0334209645014095,
0.077047861079414));
#87184=CARTESIAN_POINT('Ctrl Pts',(0.0131033706146526,-0.0333679869844681,
0.0770278158648571));
#87185=CARTESIAN_POINT('',(0.013146577386853,-0.0336938721132538,0.0771966443912191));
#87186=CARTESIAN_POINT('Origin',(0.00812378219310841,-0.0315241814719618,
0.07415));
#87187=CARTESIAN_POINT('',(0.0133186470828877,-0.0337108120655662,0.0771522289655357));
#87188=CARTESIAN_POINT('',(0.0133250480478685,-0.0336938721132327,0.0771411257927597));
#87189=CARTESIAN_POINT('Origin',(-0.000287847130412359,-0.0345562526275983,
0.0679979099388204));
#87190=CARTESIAN_POINT('Ctrl Pts',(0.0133250480478763,-0.0336938721132384,
0.0771411257927729));
#87191=CARTESIAN_POINT('Ctrl Pts',(0.0133239832652973,-0.0336910492960854,
0.0771429773422077));
#87192=CARTESIAN_POINT('Ctrl Pts',(0.0133229174720819,-0.0336882265858302,
0.0771448283612693));
#87193=CARTESIAN_POINT('Ctrl Pts',(0.0133207838233142,-0.0336825812712828,
0.0771485294092638));
#87194=CARTESIAN_POINT('Ctrl Pts',(0.0133197159677367,-0.0336797586670016,
0.0771503794381617));
#87195=CARTESIAN_POINT('Ctrl Pts',(0.0133186470840022,-0.033676936124375,
0.0771522289661781));
#87196=CARTESIAN_POINT('Origin',(-0.00140628322933532,-0.0345562521941869,
0.069933181487582));
#87197=CARTESIAN_POINT('Ctrl Pts',(0.0130207720882508,-0.0342436276873909,
0.0771662252845027));
#87198=CARTESIAN_POINT('Ctrl Pts',(0.0131345309001936,-0.0339430054201809,
0.0769815322659044));
#87199=CARTESIAN_POINT('Ctrl Pts',(0.0132340547003607,-0.0336441434784052,
0.0767887951609819));
#87200=CARTESIAN_POINT('Ctrl Pts',(0.0131472240232456,-0.0342436276873909,
0.0769505637252575));
#87201=CARTESIAN_POINT('Ctrl Pts',(0.0132528490253939,-0.0339430054201809,
0.0767611014933095));
#87202=CARTESIAN_POINT('Ctrl Pts',(0.0133439028863766,-0.0336441434784052,
0.0765642213957533));
#87203=CARTESIAN_POINT('Ctrl Pts',(0.0131484885425955,-0.0342436276873909,
0.0769484071096651));
#87204=CARTESIAN_POINT('Ctrl Pts',(0.0132540322066459,-0.0339430054201809,
0.0767588971855835));
#87205=CARTESIAN_POINT('Ctrl Pts',(0.0133450013682368,-0.0336441434784052,
0.0765619756581011));
#87206=CARTESIAN_POINT('',(0.0131647408170106,-0.0341934961088741,0.0769189097406935));
#87207=CARTESIAN_POINT('',(0.0132742440887522,-0.0338664212863332,0.0767094662071803));
#87208=CARTESIAN_POINT('Origin',(-0.00125084518927599,-0.0345610720405465,
0.0684192612854017));
#87209=CARTESIAN_POINT('Origin',(0.0230947708325115,-0.0336938005072996,
0.0815896279783451));
#87210=CARTESIAN_POINT('',(0.0132174000641565,-0.0336938721132327,0.0768208017492394));
#87211=CARTESIAN_POINT('',(0.0132452137775803,-0.0336938721132427,0.0767648316916638));
#87212=CARTESIAN_POINT('',(0.01310337061465,-0.0340203938281605,0.0770278158648617));
#87213=CARTESIAN_POINT('Origin',(-0.000945472464625923,-0.0345589643243393,
0.0680473954049685));
#87214=CARTESIAN_POINT('',(0.0131021943802151,-0.0341934961088739,0.0770271360925872));
#87215=CARTESIAN_POINT('Origin',(0.0226429506561994,-0.0341934220717619,
0.0825409540025416));
#87216=CARTESIAN_POINT('',(0.0131334675986228,-0.034193496108884,0.0769730229166503));
#87217=CARTESIAN_POINT('Ctrl Pts',(0.0131969768968076,-0.0340223579322396,
0.0773535442089127));
#87218=CARTESIAN_POINT('Ctrl Pts',(0.0132411621266426,-0.0339125849573575,
0.0772835716225015));
#87219=CARTESIAN_POINT('Ctrl Pts',(0.0132838680380833,-0.0338030433565231,
0.0772127336734312));
#87220=CARTESIAN_POINT('Ctrl Pts',(0.0133250480478718,-0.0336938721132327,
0.0771411257927697));
#87221=CARTESIAN_POINT('Ctrl Pts',(0.0131653493055715,-0.0340223579322396,
0.0772447284228175));
#87222=CARTESIAN_POINT('Ctrl Pts',(0.0132080336819127,-0.0339125849573575,
0.0771751920633777));
#87223=CARTESIAN_POINT('Ctrl Pts',(0.0132492488233767,-0.0338030433565231,
0.077104821098927));
#87224=CARTESIAN_POINT('Ctrl Pts',(0.0132889500002103,-0.0336938721132327,
0.0770337101943404));
#87225=CARTESIAN_POINT('Ctrl Pts',(0.0131337217143354,-0.0340223579322396,
0.0771359126367224));
#87226=CARTESIAN_POINT('Ctrl Pts',(0.0131749052371829,-0.0339125849573575,
0.0770668125042538));
#87227=CARTESIAN_POINT('Ctrl Pts',(0.0132146296086701,-0.0338030433565231,
0.0769969085244227));
#87228=CARTESIAN_POINT('Ctrl Pts',(0.0132528519525488,-0.0336938721132327,
0.076926294595911));
#87229=CARTESIAN_POINT('Ctrl Pts',(0.0131020941230993,-0.0340223579322396,
0.0770270968506272));
#87230=CARTESIAN_POINT('Ctrl Pts',(0.013141776792453,-0.0339125849573575,
0.07695843294513));
#87231=CARTESIAN_POINT('Ctrl Pts',(0.0131800103939636,-0.0338030433565231,
0.0768889959499185));
#87232=CARTESIAN_POINT('Ctrl Pts',(0.0132167539048873,-0.0336938721132327,
0.0768188789974817));
#87233=CARTESIAN_POINT('',(0.0132712240560225,-0.0336938721132427,0.0769809637710096));
#87234=CARTESIAN_POINT('Ctrl Pts',(0.0133186470797625,-0.0337108120662653,
0.0771522289637276));
#87235=CARTESIAN_POINT('Ctrl Pts',(0.0132814178587936,-0.033761140899345,
0.0771307133616997));
#87236=CARTESIAN_POINT('Ctrl Pts',(0.0132448679885092,-0.0338121088779593,
0.0771095903716735));
#87237=CARTESIAN_POINT('Ctrl Pts',(0.0131730936527325,-0.033915338277323,
0.0770681103727856));
#87238=CARTESIAN_POINT('Ctrl Pts',(0.0131378995523547,-0.0339675558473115,
0.0770477709126048));
#87239=CARTESIAN_POINT('Ctrl Pts',(0.0131033706146181,-0.0340203938281304,
0.0770278158648373));
#87240=CARTESIAN_POINT('Ctrl Pts',(0.0131627815520343,-0.0341934961088741,
0.076919433823356));
#87241=CARTESIAN_POINT('Ctrl Pts',(0.0132200374145394,-0.0340287516182427,
0.0768152564813936));
#87242=CARTESIAN_POINT('Ctrl Pts',(0.0132729386244269,-0.033864463327595,
0.0767088017287426));
#87243=CARTESIAN_POINT('Ctrl Pts',(0.0131647408170105,-0.0341934961088741,
0.0769189097406936));
#87244=CARTESIAN_POINT('Ctrl Pts',(0.0132219858445194,-0.0340287516182427,
0.0768146918924713));
#87245=CARTESIAN_POINT('Ctrl Pts',(0.0132748745545145,-0.033864463327595,
0.0767081971159909));
#87246=CARTESIAN_POINT('Ctrl Pts',(0.0134911920470384,-0.0341934961088741,
0.0768315874887945));
#87247=CARTESIAN_POINT('Ctrl Pts',(0.0135466317557828,-0.0340287516182427,
0.0767206205185736));
#87248=CARTESIAN_POINT('Ctrl Pts',(0.0135974377432913,-0.033864463327595,
0.0766074570022843));
#87249=CARTESIAN_POINT('',(0.0134969077202634,-0.0341764758832445,0.0768201164881371));
#87250=CARTESIAN_POINT('',(0.013491192047025,-0.034193496108874,0.0768315874887981));
#87251=CARTESIAN_POINT('Origin',(-0.00110300971133633,-0.0345621026930054,
0.0689930009521826));
#87252=CARTESIAN_POINT('Ctrl Pts',(0.0134969077187711,-0.0341764758837556,
0.0768201164891816));
#87253=CARTESIAN_POINT('Ctrl Pts',(0.0134584680344027,-0.0341260050040425,
0.0768010143200461));
#87254=CARTESIAN_POINT('Ctrl Pts',(0.0134206965054292,-0.0340749269148072,
0.0767822442258898));
#87255=CARTESIAN_POINT('Ctrl Pts',(0.0133464605665924,-0.0339715436306174,
0.0767453534762698));
#87256=CARTESIAN_POINT('Ctrl Pts',(0.0133100243228328,-0.033919277823705,
0.0767272468109652));
#87257=CARTESIAN_POINT('Ctrl Pts',(0.0132742440889785,-0.033866421285468,
0.0767094662092968));
#87258=CARTESIAN_POINT('',(0.0133279664320278,-0.0341934961088841,0.0768752486147559));
#87259=CARTESIAN_POINT('Origin',(0.00812378219310841,-0.0315241814719618,
0.07415));
#87260=CARTESIAN_POINT('',(0.0134969077199765,-0.034210518019052,0.0768201164870552));
#87261=CARTESIAN_POINT('',(0.0135025988803252,-0.0341934961088739,0.076808633304035));
#87262=CARTESIAN_POINT('Origin',(-0.00112772924295306,-0.0345621720562641,
0.0690309917632668));
#87263=CARTESIAN_POINT('Origin',(-0.00155879843018354,-0.0345621029387208,
0.0699101917082476));
#87264=CARTESIAN_POINT('Origin',(-0.00154344515286301,-0.0345621724837831,
0.0698675467084598));
#87265=CARTESIAN_POINT('Ctrl Pts',(0.0132167325306213,-0.0346945769586966,
0.0768221450395019));
#87266=CARTESIAN_POINT('Ctrl Pts',(0.0132727016783422,-0.0345275153362944,
0.0767154711555767));
#87267=CARTESIAN_POINT('Ctrl Pts',(0.0133253305070886,-0.0343603235965186,
0.0766070095021413));
#87268=CARTESIAN_POINT('Ctrl Pts',(0.0133744681317945,-0.034193496108874,
0.0764970831740252));
#87269=CARTESIAN_POINT('Ctrl Pts',(0.0132540399932634,-0.0346945769586966,
0.0767470705321401));
#87270=CARTESIAN_POINT('Ctrl Pts',(0.0133084366753693,-0.0345275153362944,
0.0766396152284727));
#87271=CARTESIAN_POINT('Ctrl Pts',(0.013359468056849,-0.0343603235965186,
0.0765304214057763));
#87272=CARTESIAN_POINT('Ctrl Pts',(0.0134069880093603,-0.034193496108874,
0.0764198142540929));
#87273=CARTESIAN_POINT('Ctrl Pts',(0.0132913474559052,-0.0346945769586966,
0.07667199602478));
#87274=CARTESIAN_POINT('Ctrl Pts',(0.0133441716723965,-0.0345275153362944,
0.0765637593013699));
#87275=CARTESIAN_POINT('Ctrl Pts',(0.0133936056066094,-0.0343603235965186,
0.0764538333094117));
#87276=CARTESIAN_POINT('Ctrl Pts',(0.0134395078869257,-0.034193496108874,
0.0763425453341601));
#87277=CARTESIAN_POINT('Ctrl Pts',(0.0133286549185474,-0.0346945769586966,
0.0765969215174165));
#87278=CARTESIAN_POINT('Ctrl Pts',(0.0133799066694237,-0.0345275153362944,
0.0764879033742648));
#87279=CARTESIAN_POINT('Ctrl Pts',(0.01342774315637,-0.0343603235965186,
0.0763772452130463));
#87280=CARTESIAN_POINT('Ctrl Pts',(0.013472027764492,-0.034193496108874,
0.0762652764142282));
#87281=CARTESIAN_POINT('',(0.0133286549178141,-0.0346945769586966,0.0765969215188918));
#87282=CARTESIAN_POINT('',(0.0134247910408858,-0.0343667727836576,0.0763810155080322));
#87283=CARTESIAN_POINT('Origin',(-0.00196428515163209,-0.0345626474178896,
0.0696095594035448));
#87284=CARTESIAN_POINT('Origin',(0.0236115535692648,-0.0341934771024212,
0.0806682671964958));
#87285=CARTESIAN_POINT('',(0.0133750500022089,-0.034193496108874,0.076495700619667));
#87286=CARTESIAN_POINT('',(0.0133992944426288,-0.034193496108884,0.0764380945686997));
#87287=CARTESIAN_POINT('',(0.0132742440876453,-0.0345211942962611,0.0767094662085974));
#87288=CARTESIAN_POINT('Origin',(-0.00174733867117582,-0.034562559612015,
0.0691804641554648));
#87289=CARTESIAN_POINT('',(0.0132730274909841,-0.0346945769586885,0.0767088616340682));
#87290=CARTESIAN_POINT('Origin',(0.0231806829138335,-0.0346945685853897,
0.0816323643750059));
#87291=CARTESIAN_POINT('',(0.0133008412044091,-0.0346945769587026,0.07665289157649));
#87292=CARTESIAN_POINT('Ctrl Pts',(0.0133881187727655,-0.0345231616327842,
0.0770286733708747));
#87293=CARTESIAN_POINT('Ctrl Pts',(0.0134277972323351,-0.0344132092796988,
0.0769561119027172));
#87294=CARTESIAN_POINT('Ctrl Pts',(0.0134659727679454,-0.0343032738558979,
0.0768827334607597));
#87295=CARTESIAN_POINT('Ctrl Pts',(0.0135025988803292,-0.0341934961088739,
0.0768086333040446));
#87296=CARTESIAN_POINT('Ctrl Pts',(0.0133497210398409,-0.0345231616327842,
0.0769220584082974));
#87297=CARTESIAN_POINT('Ctrl Pts',(0.0133879299622532,-0.0344132092796988,
0.0768500261988285));
#87298=CARTESIAN_POINT('Ctrl Pts',(0.0134246469838261,-0.0343032738558979,
0.0767772073844693));
#87299=CARTESIAN_POINT('Ctrl Pts',(0.0134598274554525,-0.0341934961088739,
0.0767036964594516));
#87300=CARTESIAN_POINT('Ctrl Pts',(0.0133113233069162,-0.0345231616327842,
0.07681544344572));
#87301=CARTESIAN_POINT('Ctrl Pts',(0.0133480626921713,-0.0344132092796988,
0.0767439404949398));
#87302=CARTESIAN_POINT('Ctrl Pts',(0.0133833211997068,-0.0343032738558979,
0.0766716813081789));
#87303=CARTESIAN_POINT('Ctrl Pts',(0.0134170560305758,-0.0341934961088739,
0.0765987596148585));
#87304=CARTESIAN_POINT('Ctrl Pts',(0.0132729255739916,-0.0345231616327842,
0.0767088284831427));
#87305=CARTESIAN_POINT('Ctrl Pts',(0.0133081954220894,-0.0344132092796988,
0.0766378547910511));
#87306=CARTESIAN_POINT('Ctrl Pts',(0.0133419954155875,-0.0343032738558979,
0.0765661552318885));
#87307=CARTESIAN_POINT('Ctrl Pts',(0.013374284605699,-0.0341934961088739,
0.0764938227702655));
#87308=CARTESIAN_POINT('',(0.013438824441277,-0.0341934961088839,0.076652166961861));
#87309=CARTESIAN_POINT('Ctrl Pts',(0.0134969077168772,-0.0342105180195352,
0.0768201164855123));
#87310=CARTESIAN_POINT('Ctrl Pts',(0.0134584248250332,-0.0342610556240281,
0.0768009928295567));
#87311=CARTESIAN_POINT('Ctrl Pts',(0.013420632488783,-0.0343122189868086,
0.076782212337718));
#87312=CARTESIAN_POINT('Ctrl Pts',(0.0133463957991769,-0.0344158119695077,
0.0767453212195279));
#87313=CARTESIAN_POINT('Ctrl Pts',(0.0133099818093831,-0.0344681990449958,
0.0767272256820197));
#87314=CARTESIAN_POINT('Ctrl Pts',(0.0132742440876178,-0.0345211942962359,
0.0767094662085777));
#87315=CARTESIAN_POINT('Ctrl Pts',(0.0133267328974969,-0.0346945769586932,
0.0765975674323603));
#87316=CARTESIAN_POINT('Ctrl Pts',(0.0133773346222538,-0.0345296777079064,
0.0764900001081728));
#87317=CARTESIAN_POINT('Ctrl Pts',(0.0134234472521205,-0.0343648066255586,
0.076380433283139));
#87318=CARTESIAN_POINT('Ctrl Pts',(0.0133286549178102,-0.0346945769586932,
0.0765969215189));
#87319=CARTESIAN_POINT('Ctrl Pts',(0.0133792432887634,-0.0345296777079064,
0.0764893144583026));
#87320=CARTESIAN_POINT('Ctrl Pts',(0.0134253409338946,-0.0343648066255586,
0.076379708482738));
#87321=CARTESIAN_POINT('Ctrl Pts',(0.0136489789613425,-0.0346945769586932,
0.0764892735351842));
#87322=CARTESIAN_POINT('Ctrl Pts',(0.0136973417864045,-0.0345296777079064,
0.0763750440016491));
#87323=CARTESIAN_POINT('Ctrl Pts',(0.0137409420744539,-0.0343648066255586,
0.0762589131958239));
#87324=CARTESIAN_POINT('',(0.0136539630861568,-0.0346775396665029,0.0764774662798272));
#87325=CARTESIAN_POINT('',(0.0136489789613314,-0.0346945769586886,0.0764892735351852));
#87326=CARTESIAN_POINT('Origin',(-0.0017062658188191,-0.0345626617714647,
0.0701785561643568));
#87327=CARTESIAN_POINT('Ctrl Pts',(0.013653963084665,-0.0346775396670096,
0.0764774662808801));
#87328=CARTESIAN_POINT('Ctrl Pts',(0.0136143686579338,-0.034626974992875,
0.0764608023385011));
#87329=CARTESIAN_POINT('Ctrl Pts',(0.0135754778985822,-0.034575790289194,
0.0764444345846692));
#87330=CARTESIAN_POINT('Ctrl Pts',(0.0134990717526567,-0.0344721681090205,
0.0764122778154287));
#87331=CARTESIAN_POINT('Ctrl Pts',(0.0134615863230428,-0.0344197714291976,
0.0763965014017779));
#87332=CARTESIAN_POINT('Ctrl Pts',(0.0134247910409318,-0.0343667727834294,
0.0763810155087038));
#87333=CARTESIAN_POINT('',(0.0134888169395828,-0.0346945769587026,0.0765430975270484));
#87334=CARTESIAN_POINT('Origin',(0.00812378219310841,-0.0315241814719618,
0.07415));
#87335=CARTESIAN_POINT('',(0.013653963085355,-0.0347116136489593,0.0764774662786887));
#87336=CARTESIAN_POINT('',(0.0136589219806651,-0.0346945769586885,0.0764656484042733));
#87337=CARTESIAN_POINT('Origin',(-0.00172210266274787,-0.0345626700989541,
0.070221009531519));
#87338=CARTESIAN_POINT('Origin',(-0.00158778538746057,-0.0345626621003631,
0.0698970385973882));
#87339=CARTESIAN_POINT('Origin',(-0.00156849731980765,-0.0345626702685647,
0.0698560375039974));
#87340=CARTESIAN_POINT('Ctrl Pts',(0.0133592295312375,-0.0352450361874068,
0.0765309354874297));
#87341=CARTESIAN_POINT('Ctrl Pts',(0.0134490279866701,-0.0349452760959493,
0.0763334773509347));
#87342=CARTESIAN_POINT('Ctrl Pts',(0.01352369797937,-0.034644428984174,
0.0761298161851315));
#87343=CARTESIAN_POINT('Ctrl Pts',(0.0133602235947146,-0.0352450361874068,
0.0765286143965647));
#87344=CARTESIAN_POINT('Ctrl Pts',(0.0134499345087687,-0.0349452760959493,
0.0763311187683505));
#87345=CARTESIAN_POINT('Ctrl Pts',(0.0135245143847563,-0.034644428984174,
0.0761274268113129));
#87346=CARTESIAN_POINT('Ctrl Pts',(0.013458645721158,-0.0352450361874068,
0.0762988034198331));
#87347=CARTESIAN_POINT('Ctrl Pts',(0.0135396891719982,-0.0349452760959493,
0.076097595740208));
#87348=CARTESIAN_POINT('Ctrl Pts',(0.0136053466012218,-0.034644428984174,
0.0758908551461006));
#87349=CARTESIAN_POINT('Ctrl Pts',(0.0134596299424225,-0.0352450361874068,
0.0762965053100657));
#87350=CARTESIAN_POINT('Ctrl Pts',(0.0135405867186305,-0.0349452760959493,
0.0760952605099267));
#87351=CARTESIAN_POINT('Ctrl Pts',(0.0136061549233864,-0.034644428984174,
0.0758884894294485));
#87352=CARTESIAN_POINT('',(0.0134720180698563,-0.0351951634053353,0.0762653073793554));
#87353=CARTESIAN_POINT('',(0.0135544173333601,-0.0348678972925388,0.0760437600094691));
#87354=CARTESIAN_POINT('Origin',(-0.00239959961656829,-0.0345636767894925,
0.070927119634889));
#87355=CARTESIAN_POINT('Origin',(0.0239880660027397,-0.0346946199340779,
0.0796821614080363));
#87356=CARTESIAN_POINT('',(0.0135119755788547,-0.0346945769330288,0.0761613420982109));
#87357=CARTESIAN_POINT('',(0.0135325550677313,-0.0346945769458128,0.0761023273905086));
#87358=CARTESIAN_POINT('',(0.0134247910405553,-0.0350221583435276,0.0763810155085277));
#87359=CARTESIAN_POINT('Origin',(-0.00228105547016616,-0.0345628458718364,
0.0704611897290196));
#87360=CARTESIAN_POINT('',(0.0134236498346712,-0.0351951360298762,0.0763805384950308));
#87361=CARTESIAN_POINT('Origin',(0.0235798061659101,-0.0351951838366828,
0.080654919438589));
#87362=CARTESIAN_POINT('',(0.0134720277639559,-0.0351951371328746,0.0762652764158017));
#87363=CARTESIAN_POINT('Ctrl Pts',(0.0135584846106547,-0.0350241211494343,
0.0766924416675349));
#87364=CARTESIAN_POINT('Ctrl Pts',(0.0135935057021833,-0.0349144232818962,
0.076617580870048));
#87365=CARTESIAN_POINT('Ctrl Pts',(0.0136270003293466,-0.0348045283579412,
0.0765419513537787));
#87366=CARTESIAN_POINT('Ctrl Pts',(0.0136589219849586,-0.0346945769439157,
0.076465648394031));
#87367=CARTESIAN_POINT('Ctrl Pts',(0.0135134682114149,-0.0350241211494343,
0.0765884480831026));
#87368=CARTESIAN_POINT('Ctrl Pts',(0.013547056833957,-0.0349144232818962,
0.0765142073680578));
#87369=CARTESIAN_POINT('Ctrl Pts',(0.0135791309522792,-0.0348045283579412,
0.0764392279155374));
#87370=CARTESIAN_POINT('Ctrl Pts',(0.0136096459096716,-0.0346945769439157,
0.0763636042359037));
#87371=CARTESIAN_POINT('Ctrl Pts',(0.0134684518121751,-0.0350241211494343,
0.0764844544986704));
#87372=CARTESIAN_POINT('Ctrl Pts',(0.0135006079657307,-0.0349144232818962,
0.0764108338660676));
#87373=CARTESIAN_POINT('Ctrl Pts',(0.0135312615752117,-0.0348045283579412,
0.076336504477296));
#87374=CARTESIAN_POINT('Ctrl Pts',(0.0135603698343847,-0.0346945769439157,
0.0762615600777764));
#87375=CARTESIAN_POINT('Ctrl Pts',(0.0134234354129353,-0.0350241211494343,
0.0763804609142381));
#87376=CARTESIAN_POINT('Ctrl Pts',(0.0134541590975043,-0.0349144232818962,
0.0763074603640774));
#87377=CARTESIAN_POINT('Ctrl Pts',(0.0134833921981443,-0.0348045283579412,
0.0762337810390547));
#87378=CARTESIAN_POINT('Ctrl Pts',(0.0135110937590977,-0.0346945769439157,
0.0761595159196492));
#87379=CARTESIAN_POINT('',(0.0135854487797405,-0.0346945769458128,0.0763134952515503));
#87380=CARTESIAN_POINT('Ctrl Pts',(0.0136539630823187,-0.0347116136492757,
0.0764774662774077));
#87381=CARTESIAN_POINT('Ctrl Pts',(0.0136143843844361,-0.0347621546531239,
0.0764608089407906));
#87382=CARTESIAN_POINT('Ctrl Pts',(0.0135755015870122,-0.0348133084094881,
0.0764444444851627));
#87383=CARTESIAN_POINT('Ctrl Pts',(0.0134990953424351,-0.0349168561544565,
0.076412287678505));
#87384=CARTESIAN_POINT('Ctrl Pts',(0.0134616022019935,-0.0349692089015922,
0.076396508082546));
#87385=CARTESIAN_POINT('Ctrl Pts',(0.0134247910405293,-0.0350221583435,
0.0763810155084952));
#87386=CARTESIAN_POINT('Ctrl Pts',(0.0134706729621182,-0.0351951371254983,
0.0762658286221963));
#87387=CARTESIAN_POINT('Ctrl Pts',(0.0135144163913672,-0.0350307338980975,
0.0761552850102975));
#87388=CARTESIAN_POINT('Ctrl Pts',(0.0135535535553534,-0.0348659306897824,
0.0760430278941345));
#87389=CARTESIAN_POINT('Ctrl Pts',(0.0134720277638447,-0.0351951371254983,
0.0762652764157668));
#87390=CARTESIAN_POINT('Ctrl Pts',(0.0135157597765723,-0.0350307338980975,
0.0761547047941924));
#87391=CARTESIAN_POINT('Ctrl Pts',(0.0135548843761222,-0.0348659306897824,
0.076042420164145));
#87392=CARTESIAN_POINT('Ctrl Pts',(0.0136990939452612,-0.0351951371254983,
0.0761727260426533));
#87393=CARTESIAN_POINT('Ctrl Pts',(0.0137409125370927,-0.0350307338980975,
0.0760574599702441));
#87394=CARTESIAN_POINT('Ctrl Pts',(0.013777931324035,-0.0348659306897824,
0.0759405639844929));
#87395=CARTESIAN_POINT('Origin',(0.0185760316857582,-0.0308609197410827,
0.0777948871241319));
#87396=CARTESIAN_POINT('',(0.0135710234992805,-0.0351951371254983,0.0762249265398228));
#87397=CARTESIAN_POINT('Origin',(0.00716427942480549,-0.0351840467441103,
0.0739653379084833));
#87398=CARTESIAN_POINT('Origin',(0.0196585700113253,-0.0352322614166343,
0.0773307555606667));
#87399=CARTESIAN_POINT('',(0.0136277018975404,-0.0351951142564687,0.0758187367888895));
#87400=CARTESIAN_POINT('',(0.0136613030716997,-0.0351951372916787,0.0756986647536401));
#87401=CARTESIAN_POINT('Origin',(0.00802995437358576,-0.0352875123094998,
0.0738225773521353));
#87402=CARTESIAN_POINT('Origin',(0.00475687541542284,-0.0298325076522812,
0.0808551568982295));
#87403=CARTESIAN_POINT('Origin',(0.0147521803846405,-0.033873240455648,
0.0792797391933933));
#87404=CARTESIAN_POINT('Ctrl Pts',(0.0115954196712322,-0.0321934096636941,
0.0787353973618213));
#87405=CARTESIAN_POINT('Ctrl Pts',(0.0116774961003548,-0.0320508460845284,
0.0786732567042231));
#87406=CARTESIAN_POINT('Ctrl Pts',(0.0117578410467241,-0.0319086045664984,
0.0786089576691867));
#87407=CARTESIAN_POINT('Ctrl Pts',(0.0118362929113632,-0.0317669892870756,
0.0785426529460147));
#87408=CARTESIAN_POINT('Ctrl Pts',(0.0116611528836329,-0.0321934096636941,
0.0786833437604548));
#87409=CARTESIAN_POINT('Ctrl Pts',(0.0117422975780799,-0.0320508460845284,
0.078620026509658));
#87410=CARTESIAN_POINT('Ctrl Pts',(0.0118216798795671,-0.0319086045664984,
0.0785545768024505));
#87411=CARTESIAN_POINT('Ctrl Pts',(0.0118991404658326,-0.0317669892870756,
0.0784871496350933));
#87412=CARTESIAN_POINT('Ctrl Pts',(0.0117268860960335,-0.0321934096636941,
0.0786312901590883));
#87413=CARTESIAN_POINT('Ctrl Pts',(0.0118070990558051,-0.0320508460845284,
0.0785667963150929));
#87414=CARTESIAN_POINT('Ctrl Pts',(0.0118855187124101,-0.0319086045664984,
0.0785001959357143));
#87415=CARTESIAN_POINT('Ctrl Pts',(0.011961988020302,-0.0317669892870756,
0.0784316463241718));
#87416=CARTESIAN_POINT('Ctrl Pts',(0.0117926193084342,-0.0321934096636941,
0.0785792365577218));
#87417=CARTESIAN_POINT('Ctrl Pts',(0.0118719005335303,-0.0320508460845284,
0.0785135661205279));
#87418=CARTESIAN_POINT('Ctrl Pts',(0.0119493575452532,-0.0319086045664984,
0.0784458150689781));
#87419=CARTESIAN_POINT('Ctrl Pts',(0.0120248355747714,-0.0317669892870756,
0.0783761430132503));
#87420=CARTESIAN_POINT('',(0.0117914433282733,-0.0321934096636941,0.0785801678069348));
#87421=CARTESIAN_POINT('',(0.0119703582003404,-0.0318665617511361,0.0784257429775266));
#87422=CARTESIAN_POINT('Origin',(0.00161643164797298,-0.0326371944421894,
0.0653254689367773));
#87423=CARTESIAN_POINT('Origin',(0.0193013276456433,-0.031693926150848,
0.0865746372135666));
#87424=CARTESIAN_POINT('',(0.0116944699207213,-0.0320197221621754,0.0786586337529689));
#87425=CARTESIAN_POINT('Ctrl Pts',(0.01169463942301,-0.0320197392094672,
0.0786585596999187));
#87426=CARTESIAN_POINT('Ctrl Pts',(0.0117175803950843,-0.031979271657597,
0.0786403899935351));
#87427=CARTESIAN_POINT('Ctrl Pts',(0.0117404872846657,-0.0319386439829661,
0.0786219626789956));
#87428=CARTESIAN_POINT('Ctrl Pts',(0.0117633788384472,-0.0318979099381593,
0.0786032518212021));
#87429=CARTESIAN_POINT('Ctrl Pts',(0.01178626993976,-0.0318571766984914,
0.0785845413332429));
#87430=CARTESIAN_POINT('Ctrl Pts',(0.0118090304859134,-0.0318163871833585,
0.078565643791654));
#87431=CARTESIAN_POINT('Ctrl Pts',(0.011831584439305,-0.0317755399638303,
0.078546626905285));
#87432=CARTESIAN_POINT('',(0.0116934483446432,-0.0321934096636182,0.0786577692450465));
#87433=CARTESIAN_POINT('Origin',(0.0131427450436533,-0.0324112239851953,
0.0804540644982482));
#87434=CARTESIAN_POINT('',(0.0117424458364682,-0.0321934096636662,0.0786189685260008));
#87435=CARTESIAN_POINT('Ctrl Pts',(0.0117894286472563,-0.0321934096636617,
0.0785799338245015));
#87436=CARTESIAN_POINT('Ctrl Pts',(0.0118505208871847,-0.0320835708272591,
0.078529381703061));
#87437=CARTESIAN_POINT('Ctrl Pts',(0.0119105315176052,-0.0319739230346488,
0.0784775946031752));
#87438=CARTESIAN_POINT('Ctrl Pts',(0.0119693888441963,-0.0318646057455572,
0.0784246446754529));
#87439=CARTESIAN_POINT('Ctrl Pts',(0.0119019909217039,-0.0321934096636617,
0.0785930066641706));
#87440=CARTESIAN_POINT('Ctrl Pts',(0.0119632634462797,-0.0320835708272591,
0.0785409022212396));
#87441=CARTESIAN_POINT('Ctrl Pts',(0.0120234221315626,-0.0319739230346488,
0.0784875599692914));
#87442=CARTESIAN_POINT('Ctrl Pts',(0.0120823952465098,-0.0318646057455572,
0.0784330540631819));
#87443=CARTESIAN_POINT('Ctrl Pts',(0.0120145531961515,-0.0321934096636617,
0.0786060795038397));
#87444=CARTESIAN_POINT('Ctrl Pts',(0.0120760060053747,-0.0320835708272591,
0.0785524227394181));
#87445=CARTESIAN_POINT('Ctrl Pts',(0.0121363127455201,-0.0319739230346488,
0.0784975253354075));
#87446=CARTESIAN_POINT('Ctrl Pts',(0.0121954016488234,-0.0318646057455572,
0.0784414634509109));
#87447=CARTESIAN_POINT('Ctrl Pts',(0.0121271154705991,-0.0321934096636617,
0.0786191523435088));
#87448=CARTESIAN_POINT('Ctrl Pts',(0.0121887485644697,-0.0320835708272591,
0.0785639432575967));
#87449=CARTESIAN_POINT('Ctrl Pts',(0.0122492033594775,-0.0319739230346488,
0.0785074907015237));
#87450=CARTESIAN_POINT('Ctrl Pts',(0.0123084080511369,-0.0318646057455572,
0.0784498728386399));
#87451=CARTESIAN_POINT('',(0.012136652526081,-0.0321763980308519,0.0786105909550923));
#87452=CARTESIAN_POINT('',(0.0121271154706063,-0.0321934096636184,0.078619152343485));
#87453=CARTESIAN_POINT('Origin',(0.00153306867489026,-0.0326386230729961,
0.0659066505538681));
#87454=CARTESIAN_POINT('Ctrl Pts',(0.0121366525239549,-0.0321763980306382,
0.0786105909527295));
#87455=CARTESIAN_POINT('Ctrl Pts',(0.0121079478650179,-0.0321259596176269,
0.0785786836815249));
#87456=CARTESIAN_POINT('Ctrl Pts',(0.0120797405515362,-0.0320749164634262,
0.078547329245198));
#87457=CARTESIAN_POINT('Ctrl Pts',(0.0120242979148881,-0.0319716057794031,
0.0784857008089321));
#87458=CARTESIAN_POINT('Ctrl Pts',(0.0119970841942555,-0.0319193786690225,
0.0784554508217467));
#87459=CARTESIAN_POINT('Ctrl Pts',(0.0119703581990953,-0.0318665617525441,
0.0784257429761435));
#87460=CARTESIAN_POINT('',(0.0119592793994498,-0.0321934096636663,0.07859966007522));
#87461=CARTESIAN_POINT('Origin',(0.00812378219310841,-0.0315241814719618,
0.07415));
#87462=CARTESIAN_POINT('',(0.0121366525263274,-0.0322104233323596,0.0786105909553662));
#87463=CARTESIAN_POINT('',(0.0121461712749854,-0.0321934096636183,0.0786020092176462));
#87464=CARTESIAN_POINT('Origin',(0.00149547255801582,-0.0326387244654018,
0.0659319795943699));
#87465=CARTESIAN_POINT('Origin',(0.000620872838852224,-0.0326386236434395,
0.0667272857683929));
#87466=CARTESIAN_POINT('Origin',(0.000650024392563257,-0.0326387248628074,
0.0666925696519535));
#87467=CARTESIAN_POINT('Ctrl Pts',(0.0118490568003921,-0.0327445246967096,
0.0785318322766084));
#87468=CARTESIAN_POINT('Ctrl Pts',(0.0120143203063967,-0.0324436878339359,
0.078391331247914));
#87469=CARTESIAN_POINT('Ctrl Pts',(0.0121685312045189,-0.0321434074405927,
0.0782387810450908));
#87470=CARTESIAN_POINT('Ctrl Pts',(0.0120359618642719,-0.0327445246967096,
0.0783658006618596));
#87471=CARTESIAN_POINT('Ctrl Pts',(0.0121949633855566,-0.0324436878339359,
0.0782182503934416));
#87472=CARTESIAN_POINT('Ctrl Pts',(0.0123423991110496,-0.0321434074405927,
0.0780591426553223));
#87473=CARTESIAN_POINT('',(0.0120623785749811,-0.0326943950436612,0.0783411315346456));
#87474=CARTESIAN_POINT('',(0.0122312439848547,-0.0323666188837389,0.0781757772702107));
#87475=CARTESIAN_POINT('Origin',(0.000494774121628024,-0.0326395579112568,
0.0661428289707638));
#87476=CARTESIAN_POINT('Origin',(0.0201189997075469,-0.0321933825603027,
0.0859066686481697));
#87477=CARTESIAN_POINT('',(0.0121427775269064,-0.0321934096532689,0.0782640978967223));
#87478=CARTESIAN_POINT('',(0.012186525641443,-0.0321934096584274,0.0782194621171241));
#87479=CARTESIAN_POINT('',(0.0119703582009599,-0.0325210109756239,0.0784257429782228));
#87480=CARTESIAN_POINT('Origin',(0.000862044000621341,-0.0326393129157105,
0.0658325109636758));
#87481=CARTESIAN_POINT('',(0.0119694495967206,-0.0326943950436593,0.0784247329999422));
#87482=CARTESIAN_POINT('Origin',(0.0193681487055648,-0.0326943765538236,
0.0866489149168529));
#87483=CARTESIAN_POINT('',(0.0120159140858608,-0.0326943950436702,0.078382932267304));
#87484=CARTESIAN_POINT('Ctrl Pts',(0.0119587280979391,-0.0325229783203769,
0.0787644544538986));
#87485=CARTESIAN_POINT('Ctrl Pts',(0.0120223382516747,-0.032413025309245,
0.0787115898084653));
#87486=CARTESIAN_POINT('Ctrl Pts',(0.0120848451845838,-0.0323031222208069,
0.0786574173232481));
#87487=CARTESIAN_POINT('Ctrl Pts',(0.0121461712783128,-0.0321934096576658,
0.078602009214648));
#87488=CARTESIAN_POINT('Ctrl Pts',(0.0119622743777968,-0.0325229783203769,
0.078651191193589));
#87489=CARTESIAN_POINT('Ctrl Pts',(0.0120243231999659,-0.032413025309245,
0.0785982776627653));
#87490=CARTESIAN_POINT('Ctrl Pts',(0.012085268026858,-0.0323031222208069,
0.0785440885977215));
#87491=CARTESIAN_POINT('Ctrl Pts',(0.0121450332418156,-0.0321934096576658,
0.078488696165489));
#87492=CARTESIAN_POINT('Ctrl Pts',(0.0119658206576546,-0.0325229783203769,
0.0785379279332794));
#87493=CARTESIAN_POINT('Ctrl Pts',(0.0120263081482572,-0.032413025309245,
0.0784849655170654));
#87494=CARTESIAN_POINT('Ctrl Pts',(0.0120856908691323,-0.0323031222208069,
0.0784307598721948));
#87495=CARTESIAN_POINT('Ctrl Pts',(0.0121438952053184,-0.0321934096576658,
0.0783753831163299));
#87496=CARTESIAN_POINT('Ctrl Pts',(0.0119693669375123,-0.0325229783203769,
0.0784246646729697));
#87497=CARTESIAN_POINT('Ctrl Pts',(0.0120282930965484,-0.032413025309245,
0.0783716533713655));
#87498=CARTESIAN_POINT('Ctrl Pts',(0.0120861137114065,-0.0323031222208069,
0.0783174311466682));
#87499=CARTESIAN_POINT('Ctrl Pts',(0.0121427571688211,-0.0321934096576658,
0.0782620700671708));
#87500=CARTESIAN_POINT('',(0.0121444744006986,-0.0321934096584275,0.0784330535576338));
#87501=CARTESIAN_POINT('Ctrl Pts',(0.0121366525239949,-0.0322104233328902,
0.078610590952774));
#87502=CARTESIAN_POINT('Ctrl Pts',(0.0121079089697485,-0.0322609421830583,
0.078578640446665));
#87503=CARTESIAN_POINT('Ctrl Pts',(0.0120796826552531,-0.0323120888239129,
0.0785472648893489));
#87504=CARTESIAN_POINT('Ctrl Pts',(0.0120242395988951,-0.0324156524631811,
0.0784856359865455));
#87505=CARTESIAN_POINT('Ctrl Pts',(0.0119970456471616,-0.032468026716731,
0.0784554079739085));
#87506=CARTESIAN_POINT('Ctrl Pts',(0.0119703582009342,-0.0325210109755912,
0.0784257429781876));
#87507=CARTESIAN_POINT('Origin',(0.00168338772958699,-0.0262834582510625,
0.0786693699777735));
#87508=CARTESIAN_POINT('Origin',(0.0113525993087552,-0.0342770963326899,
0.0858717464226988));
#87509=CARTESIAN_POINT('Ctrl Pts',(0.0120603536691667,-0.0326943950436604,
0.0783410245427036));
#87510=CARTESIAN_POINT('Ctrl Pts',(0.0121181138421823,-0.0325844576448134,
0.0782867712098422));
#87511=CARTESIAN_POINT('Ctrl Pts',(0.0121747560551019,-0.0324744968375322,
0.0782313194623111));
#87512=CARTESIAN_POINT('Ctrl Pts',(0.0122302087145849,-0.0323646534831895,
0.0781747413491271));
#87513=CARTESIAN_POINT('Ctrl Pts',(0.012173514514236,-0.0326943950436604,
0.0783470037337604));
#87514=CARTESIAN_POINT('Ctrl Pts',(0.0122313570917106,-0.0325844576448134,
0.0782911908323679));
#87515=CARTESIAN_POINT('Ctrl Pts',(0.0122880494604869,-0.0324744968375322,
0.0782341777016734));
#87516=CARTESIAN_POINT('Ctrl Pts',(0.012343519990555,-0.0323646534831895,
0.0781760383921151));
#87517=CARTESIAN_POINT('Ctrl Pts',(0.0122866753593053,-0.0326943950436604,
0.0783529829248173));
#87518=CARTESIAN_POINT('Ctrl Pts',(0.0123446003412388,-0.0325844576448134,
0.0782956104548937));
#87519=CARTESIAN_POINT('Ctrl Pts',(0.0124013428658719,-0.0324744968375322,
0.0782370359410357));
#87520=CARTESIAN_POINT('Ctrl Pts',(0.0124568312665252,-0.0323646534831895,
0.078177335435103));
#87521=CARTESIAN_POINT('Ctrl Pts',(0.0123998362043746,-0.0326943950436604,
0.0783589621158741));
#87522=CARTESIAN_POINT('Ctrl Pts',(0.0124578435907671,-0.0325844576448134,
0.0783000300774195));
#87523=CARTESIAN_POINT('Ctrl Pts',(0.0125146362712568,-0.0324744968375322,
0.078239894180398));
#87524=CARTESIAN_POINT('Ctrl Pts',(0.0125701425424953,-0.0323646534831895,
0.078178632478091));
#87525=CARTESIAN_POINT('',(0.0124088168667548,-0.0326773559991213,0.078349818784899));
#87526=CARTESIAN_POINT('',(0.0123998362043608,-0.0326943950436594,0.0783589621158728));
#87527=CARTESIAN_POINT('Origin',(0.000514714023868693,-0.0326395669367224,
0.066762600728777));
#87528=CARTESIAN_POINT('Ctrl Pts',(0.0124088168643565,-0.0326773559987506,
0.0783498187825483));
#87529=CARTESIAN_POINT('Ctrl Pts',(0.0123781407071167,-0.0326267922587182,
0.0783197526777822));
#87530=CARTESIAN_POINT('Ctrl Pts',(0.0123480082626104,-0.0325756109581767,
0.07829021947301));
#87531=CARTESIAN_POINT('Ctrl Pts',(0.0122888051545989,-0.0324719985462387,
0.0782321937289757));
#87532=CARTESIAN_POINT('Ctrl Pts',(0.0122597582360467,-0.0324196091621789,
0.078203724462454));
#87533=CARTESIAN_POINT('Ctrl Pts',(0.0122312439848199,-0.0323666188837756,
0.0781757772701765));
#87534=CARTESIAN_POINT('',(0.0122311073896809,-0.0326943950436703,0.0783500468252692));
#87535=CARTESIAN_POINT('Origin',(0.00812378219310841,-0.0315241814719618,
0.07415));
#87536=CARTESIAN_POINT('',(0.0124088168667217,-0.0327114338379851,0.0783498187848666));
#87537=CARTESIAN_POINT('',(0.012417777980685,-0.0326943950436593,0.0783406562942192));
#87538=CARTESIAN_POINT('Origin',(0.000483558929968489,-0.032639568145509,
0.0667954986120342));
#87539=CARTESIAN_POINT('Origin',(0.000585047604623338,-0.032639567204889,
0.0666908392600542));
#87540=CARTESIAN_POINT('Origin',(0.000617313923548154,-0.0326395685020944,
0.066659030667844));
#87541=CARTESIAN_POINT('Ctrl Pts',(0.0121168715764049,-0.0332451089994433,
0.0782892465711775));
#87542=CARTESIAN_POINT('Ctrl Pts',(0.0122729858149996,-0.0329451141710253,
0.0781386447411115));
#87543=CARTESIAN_POINT('Ctrl Pts',(0.0124173126040131,-0.0326442513127493,
0.0779767115922992));
#87544=CARTESIAN_POINT('Ctrl Pts',(0.0122929814043604,-0.0332451089994433,
0.0781118055147743));
#87545=CARTESIAN_POINT('Ctrl Pts',(0.0124424033440211,-0.0329451141710253,
0.0779545615938766));
#87546=CARTESIAN_POINT('Ctrl Pts',(0.012579556536781,-0.0326442513127493,
0.0777865093150257));
#87547=CARTESIAN_POINT('Ctrl Pts',(0.0122947425026399,-0.0332451089994433,
0.0781100311042103));
#87548=CARTESIAN_POINT('Ctrl Pts',(0.0124440975193113,-0.0329451141710253,
0.0779527207624043));
#87549=CARTESIAN_POINT('Ctrl Pts',(0.0125811789761087,-0.0326442513127493,
0.077784607292253));
#87550=CARTESIAN_POINT('',(0.0123177699811848,-0.0331951640388616,0.0780855547809003));
#87551=CARTESIAN_POINT('',(0.0124759195072863,-0.0328677532355047,0.0779099236519366));
#87552=CARTESIAN_POINT('Origin',(-0.000419516393849347,-0.0326402808282463,
0.0671862986931509));
#87553=CARTESIAN_POINT('Origin',(0.0208423773160607,-0.0326944278779179,
0.0851374243729753));
#87554=CARTESIAN_POINT('',(0.0123931733065714,-0.0326943950436593,0.0780036248546381));
#87555=CARTESIAN_POINT('',(0.0124340323883481,-0.0326943950436694,0.0779563301885937));
#87556=CARTESIAN_POINT('',(0.0122312439848527,-0.0330220786163545,0.0781757772702127));
#87557=CARTESIAN_POINT('Origin',(-0.000129652753292978,-0.0326396682763325,
0.0668027211718298));
#87558=CARTESIAN_POINT('',(0.0122302737564742,-0.0331951640388587,0.078174826336627));
#87559=CARTESIAN_POINT('Origin',(0.0201087757104031,-0.0331952026560029,
0.0858966510234808));
#87560=CARTESIAN_POINT('',(0.0122740218688395,-0.0331951640388701,0.0781301905587737));
#87561=CARTESIAN_POINT('Ctrl Pts',(0.0122409053996857,-0.0330240426238172,
0.0785145499770249));
#87562=CARTESIAN_POINT('Ctrl Pts',(0.0123010313277942,-0.0329142774063519,
0.0784578325937355));
#87563=CARTESIAN_POINT('Ctrl Pts',(0.0123600147241259,-0.0328043479726691,
0.0783998439638745));
#87564=CARTESIAN_POINT('Ctrl Pts',(0.0124177779806857,-0.0326943950436593,
0.0783406562942282));
#87565=CARTESIAN_POINT('Ctrl Pts',(0.0122373328055426,-0.0330240426238172,
0.0784012875712757));
#87566=CARTESIAN_POINT('Ctrl Pts',(0.0122958984336657,-0.0329142774063519,
0.0783446194039512));
#87567=CARTESIAN_POINT('Ctrl Pts',(0.0123533217695771,-0.0328043479726691,
0.0782867122703503));
#87568=CARTESIAN_POINT('Ctrl Pts',(0.0124095272067103,-0.0326943950436593,
0.0782276383278962));
#87569=CARTESIAN_POINT('Ctrl Pts',(0.0122337602113996,-0.0330240426238172,
0.0782880251655264));
#87570=CARTESIAN_POINT('Ctrl Pts',(0.0122907655395373,-0.0329142774063519,
0.0782314062141669));
#87571=CARTESIAN_POINT('Ctrl Pts',(0.0123466288150282,-0.032804347972669,
0.078173580576826));
#87572=CARTESIAN_POINT('Ctrl Pts',(0.0124012764327349,-0.0326943950436593,
0.0781146203615641));
#87573=CARTESIAN_POINT('Ctrl Pts',(0.0122301876172566,-0.0330240426238172,
0.0781747627597772));
#87574=CARTESIAN_POINT('Ctrl Pts',(0.0122856326454088,-0.0329142774063519,
0.0781181930243826));
#87575=CARTESIAN_POINT('Ctrl Pts',(0.0123399358604794,-0.032804347972669,
0.0780604488833018));
#87576=CARTESIAN_POINT('Ctrl Pts',(0.0123930256587595,-0.0326943950436593,
0.0780016023952321));
#87577=CARTESIAN_POINT('',(0.0124054756436382,-0.0326943950436693,0.0781721405744387));
#87578=CARTESIAN_POINT('Ctrl Pts',(0.0124088168643483,-0.0327114338383293,
0.0783498187825402));
#87579=CARTESIAN_POINT('Ctrl Pts',(0.0123781458095351,-0.03276198768302,
0.0783197576787295));
#87580=CARTESIAN_POINT('Ctrl Pts',(0.0123480158572798,-0.032813156260278,
0.0782902269166453));
#87581=CARTESIAN_POINT('Ctrl Pts',(0.0122888128036875,-0.0329167375858768,
0.0782322012259481));
#87582=CARTESIAN_POINT('Ctrl Pts',(0.0122597632920272,-0.0329691088920627,
0.078203729417887));
#87583=CARTESIAN_POINT('Ctrl Pts',(0.0122312439848207,-0.0330220786163187,
0.0781757772701774));
#87584=CARTESIAN_POINT('Ctrl Pts',(0.0123157420292715,-0.0331951640388604,
0.0780855751482224));
#87585=CARTESIAN_POINT('Ctrl Pts',(0.012397107522205,-0.0330306422010619,
0.0779989090662443));
#87586=CARTESIAN_POINT('Ctrl Pts',(0.0124748214885866,-0.0328657861914645,
0.0779089541184372));
#87587=CARTESIAN_POINT('Ctrl Pts',(0.0123177699811826,-0.0331951640388604,
0.0780855547809025));
#87588=CARTESIAN_POINT('Ctrl Pts',(0.0123991350530348,-0.0330306422010619,
0.0779988467723189));
#87589=CARTESIAN_POINT('Ctrl Pts',(0.0124768468658241,-0.0328657861914645,
0.0779088499511359));
#87590=CARTESIAN_POINT('Ctrl Pts',(0.0126556813064915,-0.0331951640388604,
0.0780821610376819));
#87591=CARTESIAN_POINT('Ctrl Pts',(0.0127369762148785,-0.0330306422010619,
0.077988466929096));
#87592=CARTESIAN_POINT('Ctrl Pts',(0.012814329181297,-0.0328657861914645,
0.0778914928774142));
#87593=CARTESIAN_POINT('',(0.0126640701336466,-0.0331781648281957,0.0780724718498676));
#87594=CARTESIAN_POINT('',(0.0126556813064761,-0.0331951640388588,0.0780821610376811));
#87595=CARTESIAN_POINT('Origin',(-0.000292616017096561,-0.0326412092982242,
0.0678201178075067));
#87596=CARTESIAN_POINT('Ctrl Pts',(0.0126640701318514,-0.033178164828644,
0.0780724718503024));
#87597=CARTESIAN_POINT('Ctrl Pts',(0.0126315442553613,-0.0331276811546764,
0.0780443719227299));
#87598=CARTESIAN_POINT('Ctrl Pts',(0.0125996056733662,-0.033076566349777,
0.0780167794184189));
#87599=CARTESIAN_POINT('Ctrl Pts',(0.0125368757635288,-0.0329730614463296,
0.0779625854268184));
#87600=CARTESIAN_POINT('Ctrl Pts',(0.0125061097806984,-0.0329207133373935,
0.0779360058286567));
#87601=CARTESIAN_POINT('Ctrl Pts',(0.0124759195047419,-0.03286775322894,
0.0779099236682114));
#87602=CARTESIAN_POINT('',(0.0124867256438404,-0.0331951640388701,0.0780838579093006));
#87603=CARTESIAN_POINT('Origin',(0.00812378219310841,-0.0315241814719618,
0.07415));
#87604=CARTESIAN_POINT('',(0.0126640701328944,-0.0332121607144207,0.0780724718483633));
#87605=CARTESIAN_POINT('',(0.0126724382467511,-0.0331951640388587,0.0780627647649284));
#87606=CARTESIAN_POINT('Origin',(-0.000315876451106127,-0.0326413667720304,
0.0678590414940439));
#87607=CARTESIAN_POINT('Origin',(0.000638664815378747,-0.0326412093957853,
0.0667421529359667));
#87608=CARTESIAN_POINT('Origin',(0.000673798557899307,-0.0326413668042006,
0.0667134867922949));
#87609=CARTESIAN_POINT('Ctrl Pts',(0.012368883514552,-0.0337436976235975,
0.0780303659325736));
#87610=CARTESIAN_POINT('Ctrl Pts',(0.0124037841138351,-0.0336723290703325,
0.0779921848479258));
#87611=CARTESIAN_POINT('Ctrl Pts',(0.012437992309655,-0.033601104548885,
0.0779533821883012));
#87612=CARTESIAN_POINT('Ctrl Pts',(0.0125472123026462,-0.0333736987606857,
0.0778294929824934));
#87613=CARTESIAN_POINT('Ctrl Pts',(0.0126491428327614,-0.0331450831799191,
0.077699540263341));
#87614=CARTESIAN_POINT('Ctrl Pts',(0.0125335048953521,-0.0337436976235975,
0.0778422175842325));
#87615=CARTESIAN_POINT('Ctrl Pts',(0.0125667132598756,-0.0336723290703325,
0.0778025558699368));
#87616=CARTESIAN_POINT('Ctrl Pts',(0.0125992028628391,-0.033601104548885,
0.0777623032581647));
#87617=CARTESIAN_POINT('Ctrl Pts',(0.0127029357292737,-0.0333736987606857,
0.0776337846423694));
#87618=CARTESIAN_POINT('Ctrl Pts',(0.0127991225129448,-0.0331450831799191,
0.0774995250250913));
#87619=CARTESIAN_POINT('Ctrl Pts',(0.0125351511091601,-0.0337436976235975,
0.0778403361007492));
#87620=CARTESIAN_POINT('Ctrl Pts',(0.012568342551336,-0.0336723290703325,
0.0778006595801569));
#87621=CARTESIAN_POINT('Ctrl Pts',(0.0126008149683709,-0.033601104548885,
0.0777603924688633));
#87622=CARTESIAN_POINT('Ctrl Pts',(0.01270449296354,-0.0333736987606857,
0.0776318275589682));
#87623=CARTESIAN_POINT('Ctrl Pts',(0.0128006223097466,-0.0331450831799191,
0.0774975248727087));
#87624=CARTESIAN_POINT('',(0.0125566096336481,-0.0336938721132548,0.0778144461904084));
#87625=CARTESIAN_POINT('',(0.012703419113583,-0.0333679870047996,0.0776292313341869));
#87626=CARTESIAN_POINT('Ctrl Pts',(0.0125566096336415,-0.033693872113258,
0.077814446190417));
#87627=CARTESIAN_POINT('Ctrl Pts',(0.0125709136861504,-0.0336629187933925,
0.0777971427854336));
#87628=CARTESIAN_POINT('Ctrl Pts',(0.0125851118454865,-0.0336319952301064,
0.0777797611585158));
#87629=CARTESIAN_POINT('Ctrl Pts',(0.0125992028628405,-0.0336011045488974,
0.0777623032581634));
#87630=CARTESIAN_POINT('Ctrl Pts',(0.0126345620470564,-0.0335235892595478,
0.0777184954124219));
#87631=CARTESIAN_POINT('Ctrl Pts',(0.0126693092926114,-0.0334458668665594,
0.0776741293533719));
#87632=CARTESIAN_POINT('Ctrl Pts',(0.0127034191066276,-0.0333679869962518,
0.0776292313437298));
#87633=CARTESIAN_POINT('Ctrl Pts',(0.0127034465584522,-0.0333679692468939,
0.0776291963457838));
#87634=CARTESIAN_POINT('Ctrl Pts',(0.0127030820920156,-0.0333391895414168,
0.0776289268982052));
#87635=CARTESIAN_POINT('Ctrl Pts',(0.0127028069762463,-0.033310408112934,
0.0776287275451851));
#87636=CARTESIAN_POINT('Ctrl Pts',(0.0127024395635659,-0.0332532698080884,
0.0776284681520712));
#87637=CARTESIAN_POINT('Ctrl Pts',(0.0127023445977535,-0.0332249170382467,
0.0776284060801511));
#87638=CARTESIAN_POINT('Ctrl Pts',(0.0127023375019387,-0.0331960985401869,
0.0776284093528773));
#87639=CARTESIAN_POINT('Ctrl Pts',(0.0127023374105474,-0.0331956312522822,
0.0776284094239842));
#87640=CARTESIAN_POINT('Ctrl Pts',(0.0127023373432507,-0.0331951640388592,
0.0776284095125653));
#87641=CARTESIAN_POINT('',(0.0126267197451524,-0.0331951640388587,0.0777279433201761));
#87642=CARTESIAN_POINT('',(0.012664528544212,-0.0331951640388687,0.0776781764163801));
#87643=CARTESIAN_POINT('',(0.0124759194931757,-0.0335216366567645,0.0779099236583928));
#87644=CARTESIAN_POINT('Origin',(-0.000885048750426973,-0.032643457152579,
0.0679673287949028));
#87645=CARTESIAN_POINT('',(0.0124748914701048,-0.0336938721132327,0.0779090355225293));
#87646=CARTESIAN_POINT('Origin',(0.0207386455233593,-0.0336938867896231,
0.0850483071168731));
#87647=CARTESIAN_POINT('',(0.0125157505518864,-0.0336938721132537,0.0778617408564788));
#87648=CARTESIAN_POINT('Ctrl Pts',(0.0125068342143895,-0.0335235895815172,
0.0782474205274581));
#87649=CARTESIAN_POINT('Ctrl Pts',(0.0125632432750286,-0.0334144449262749,
0.0781870791869498));
#87650=CARTESIAN_POINT('Ctrl Pts',(0.0126184705361613,-0.0333049234473147,
0.0781255031528116));
#87651=CARTESIAN_POINT('Ctrl Pts',(0.0126724382467524,-0.0331951640388587,
0.0780627647649378));
#87652=CARTESIAN_POINT('Ctrl Pts',(0.012496156831399,-0.0335235895815172,
0.0781346057856069));
#87653=CARTESIAN_POINT('Ctrl Pts',(0.0125510127750048,-0.0334144449262749,
0.0780744114402973));
#87654=CARTESIAN_POINT('Ctrl Pts',(0.0126046881715709,-0.0333049234473147,
0.0780130146564665));
#87655=CARTESIAN_POINT('Ctrl Pts',(0.0126571072751832,-0.0331951640388587,
0.0779504877245545));
#87656=CARTESIAN_POINT('Ctrl Pts',(0.0124854794484085,-0.0335235895815172,
0.0780217910437557));
#87657=CARTESIAN_POINT('Ctrl Pts',(0.0125387822749809,-0.0334144449262749,
0.0779617436936448));
#87658=CARTESIAN_POINT('Ctrl Pts',(0.0125909058069806,-0.0333049234473147,
0.0779005261601214));
#87659=CARTESIAN_POINT('Ctrl Pts',(0.012641776303614,-0.0331951640388587,
0.0778382106841713));
#87660=CARTESIAN_POINT('Ctrl Pts',(0.012474802065418,-0.0335235895815172,
0.0779089763019045));
#87661=CARTESIAN_POINT('Ctrl Pts',(0.012526551774957,-0.0334144449262749,
0.0778490759469923));
#87662=CARTESIAN_POINT('Ctrl Pts',(0.0125771234423902,-0.0333049234473147,
0.0777880376637764));
#87663=CARTESIAN_POINT('Ctrl Pts',(0.0126264453320448,-0.0331951640388587,
0.077725933643788));
#87664=CARTESIAN_POINT('',(0.0126495789959617,-0.0331951640388687,0.0778953540425622));
#87665=CARTESIAN_POINT('Ctrl Pts',(0.0126640701305185,-0.0332121607145946,
0.0780724718463101));
#87666=CARTESIAN_POINT('Ctrl Pts',(0.0126315989788135,-0.033262544410894,
0.0780444191808985));
#87667=CARTESIAN_POINT('Ctrl Pts',(0.0125996873560065,-0.0333135300745174,
0.0780168499069326));
#87668=CARTESIAN_POINT('Ctrl Pts',(0.0125369578369668,-0.033416720314053,
0.0779626562575963));
#87669=CARTESIAN_POINT('Ctrl Pts',(0.0125061642365394,-0.0334688847587201,
0.0779360528719987));
#87670=CARTESIAN_POINT('Ctrl Pts',(0.0124759194927459,-0.0335216366562258,
0.0779099236578027));
#87671=CARTESIAN_POINT('Ctrl Pts',(0.0125545874353461,-0.0336938721132576,
0.0778145938191832));
#87672=CARTESIAN_POINT('Ctrl Pts',(0.0125760375190152,-0.0336474569765051,
0.0777886588457981));
#87673=CARTESIAN_POINT('Ctrl Pts',(0.012597182531302,-0.033601104548885,
0.0777624745491818));
#87674=CARTESIAN_POINT('Ctrl Pts',(0.0126507168408582,-0.0334837508592655,
0.0776961819303098));
#87675=CARTESIAN_POINT('Ctrl Pts',(0.0127022632543466,-0.0333660264659096,
0.0776283320896833));
#87676=CARTESIAN_POINT('Ctrl Pts',(0.0125566096336264,-0.0336938721132576,
0.0778144461904346));
#87677=CARTESIAN_POINT('Ctrl Pts',(0.0125780588531755,-0.0336474569765051,
0.0777884993804519));
#87678=CARTESIAN_POINT('Ctrl Pts',(0.0125992028628391,-0.033601104548885,
0.0777623032581647));
#87679=CARTESIAN_POINT('Ctrl Pts',(0.012652734633984,-0.0334837508592655,
0.0776959806994129));
#87680=CARTESIAN_POINT('Ctrl Pts',(0.012704277622995,-0.0333660264659096,
0.0776281010072723));
#87681=CARTESIAN_POINT('Ctrl Pts',(0.0128956632619176,-0.0336938721132576,
0.0777896938882721));
#87682=CARTESIAN_POINT('Ctrl Pts',(0.0129169675980284,-0.0336474569765051,
0.0777617624848927));
#87683=CARTESIAN_POINT('Ctrl Pts',(0.0129379435020098,-0.033601104548885,
0.077733583601238));
#87684=CARTESIAN_POINT('Ctrl Pts',(0.0129910496682173,-0.0334837508592655,
0.07766224114657));
#87685=CARTESIAN_POINT('Ctrl Pts',(0.0130420184892613,-0.0333660264659096,
0.0775893563744383));
#87686=CARTESIAN_POINT('',(0.0129014049584752,-0.0336769361243754,0.0777796447087626));
#87687=CARTESIAN_POINT('',(0.0128936410732186,-0.0336938721132327,0.0777898415163072));
#87688=CARTESIAN_POINT('Ctrl Pts',(0.0129014049584754,-0.0336769361243751,
0.0777796447087624));
#87689=CARTESIAN_POINT('Ctrl Pts',(0.0129001126958818,-0.0336797586670012,
0.0777813456860429));
#87690=CARTESIAN_POINT('Ctrl Pts',(0.0128988195737642,-0.0336825812712819,
0.0777830459088651));
#87691=CARTESIAN_POINT('Ctrl Pts',(0.012896231617541,-0.0336882265885678,
0.0777864448371688));
#87692=CARTESIAN_POINT('Ctrl Pts',(0.0128949367834719,-0.0336910493015603,
0.0777881435426561));
#87693=CARTESIAN_POINT('Ctrl Pts',(0.0128936410732317,-0.0336938721132376,
0.077789841516309));
#87694=CARTESIAN_POINT('Ctrl Pts',(0.0129014049584752,-0.0336769361243754,
0.0777796447087626));
#87695=CARTESIAN_POINT('Ctrl Pts',(0.0128680310229009,-0.0336279018525357,
0.07775428993828));
#87696=CARTESIAN_POINT('Ctrl Pts',(0.0128341769609851,-0.0335767826051547,
0.0777285704073053));
#87697=CARTESIAN_POINT('Ctrl Pts',(0.012767842447259,-0.0334733172106842,
0.0776781749013019));
#87698=CARTESIAN_POINT('Ctrl Pts',(0.0127353174133851,-0.0334209631477619,
0.0776534650564892));
#87699=CARTESIAN_POINT('Ctrl Pts',(0.0127034191046726,-0.033367986984468,
0.0776292313458923));
#87700=CARTESIAN_POINT('',(0.0127251253534434,-0.0336938721132538,0.0778021438533678));
#87701=CARTESIAN_POINT('Origin',(0.00812378219310841,-0.0315241814719618,
0.07415));
#87702=CARTESIAN_POINT('',(0.0129014049574505,-0.0337108120655664,0.0777796447079852));
#87703=CARTESIAN_POINT('',(0.0129091470454567,-0.0336938721132327,0.0777694313406826));
#87704=CARTESIAN_POINT('Origin',(0.000549542511272994,-0.034556252669366,
0.066992164303698));
#87705=CARTESIAN_POINT('Ctrl Pts',(0.0129091470454626,-0.0336938721132382,
0.0777694313406962));
#87706=CARTESIAN_POINT('Ctrl Pts',(0.0129078585987974,-0.0336910492970996,
0.077771134836855));
#87707=CARTESIAN_POINT('Ctrl Pts',(0.0129065692152446,-0.0336882265863373,
0.0777728376810751));
#87708=CARTESIAN_POINT('Ctrl Pts',(0.0129039885263747,-0.0336825812712489,
0.0777762421284276));
#87709=CARTESIAN_POINT('Ctrl Pts',(0.0129026972210611,-0.0336797586669847,
0.0777779437314923));
#87710=CARTESIAN_POINT('Ctrl Pts',(0.0129014049584751,-0.0336769361243751,
0.0777796447087628));
#87711=CARTESIAN_POINT('Origin',(-0.000802628279970289,-0.0345562522332008,
0.0687719985390831));
#87712=CARTESIAN_POINT('Ctrl Pts',(0.0126041245922024,-0.034243627687391,
0.0777561970255215));
#87713=CARTESIAN_POINT('Ctrl Pts',(0.0127401345551726,-0.0339430054201809,
0.0775872181262872));
#87714=CARTESIAN_POINT('Ctrl Pts',(0.0128630299450369,-0.0336441434784052,
0.0774084744506964));
#87715=CARTESIAN_POINT('Ctrl Pts',(0.0127566089764962,-0.034243627687391,
0.0775580846519893));
#87716=CARTESIAN_POINT('Ctrl Pts',(0.0128851470081222,-0.0339430054201809,
0.0773833547093942));
#87717=CARTESIAN_POINT('Ctrl Pts',(0.0130001585014659,-0.0336441434784052,
0.077199439145038));
#87718=CARTESIAN_POINT('Ctrl Pts',(0.0127581338203391,-0.034243627687391,
0.077556103528254));
#87719=CARTESIAN_POINT('Ctrl Pts',(0.0128865971326517,-0.0339430054201809,
0.0773813160752254));
#87720=CARTESIAN_POINT('Ctrl Pts',(0.0130015297870302,-0.0336441434784052,
0.0771973487919815));
#87721=CARTESIAN_POINT('',(0.0127779549413509,-0.0341934961088741,0.0775288757049524));
#87722=CARTESIAN_POINT('',(0.0129128449824874,-0.0338664212865843,0.0773348080954013));
#87723=CARTESIAN_POINT('Origin',(-0.000458671437912886,-0.0345610720407566,
0.0672894975086063));
#87724=CARTESIAN_POINT('Origin',(0.022044287513203,-0.0336938005072887,
0.0834073266643943));
#87725=CARTESIAN_POINT('',(0.012842495146412,-0.0336938721132327,0.0774381412780363));
#87726=CARTESIAN_POINT('',(0.012877104448698,-0.0336938721132427,0.0773860985437216));
#87727=CARTESIAN_POINT('',(0.0127034191046694,-0.0340203938281605,0.0776292313458965));
#87728=CARTESIAN_POINT('Origin',(-0.000109099515416648,-0.0345589643244507,
0.0669588372527201));
#87729=CARTESIAN_POINT('',(0.0127023373432517,-0.0341934961088739,0.0776284095125642));
#87730=CARTESIAN_POINT('Origin',(0.0214767972526703,-0.0341934220717625,
0.084294523189698));
#87731=CARTESIAN_POINT('',(0.0127401461423113,-0.0341934961088841,0.0775786426087683));
#87732=CARTESIAN_POINT('Ctrl Pts',(0.0127554626867099,-0.0340223579322396,
0.0779641232026885));
#87733=CARTESIAN_POINT('Ctrl Pts',(0.0128080693933258,-0.0339125849573574,
0.0779002402487519));
#87734=CARTESIAN_POINT('Ctrl Pts',(0.0128593169051152,-0.0338030433565231,
0.0778353133480415));
#87735=CARTESIAN_POINT('Ctrl Pts',(0.0129091470454587,-0.0336938721132327,
0.0777694313406923));
#87736=CARTESIAN_POINT('Ctrl Pts',(0.0127377227228115,-0.0340223579322396,
0.0778522014732892));
#87737=CARTESIAN_POINT('Ctrl Pts',(0.012788785736875,-0.0339125849573574,
0.0777885631997224));
#87738=CARTESIAN_POINT('Ctrl Pts',(0.0128384957051617,-0.0338030433565231,
0.0777239127582967));
#87739=CARTESIAN_POINT('Ctrl Pts',(0.0128867963859714,-0.0336938721132327,
0.0776583384613015));
#87740=CARTESIAN_POINT('Ctrl Pts',(0.0127199827589131,-0.0340223579322396,
0.0777402797438898));
#87741=CARTESIAN_POINT('Ctrl Pts',(0.0127695020804241,-0.0339125849573574,
0.077676886150693));
#87742=CARTESIAN_POINT('Ctrl Pts',(0.0128176745052083,-0.0338030433565231,
0.0776125121685519));
#87743=CARTESIAN_POINT('Ctrl Pts',(0.012864445726484,-0.0336938721132327,
0.0775472455819107));
#87744=CARTESIAN_POINT('Ctrl Pts',(0.0127022427950148,-0.0340223579322396,
0.0776283580144904));
#87745=CARTESIAN_POINT('Ctrl Pts',(0.0127502184239732,-0.0339125849573574,
0.0775652091016636));
#87746=CARTESIAN_POINT('Ctrl Pts',(0.0127968533052548,-0.0338030433565231,
0.0775011115788072));
#87747=CARTESIAN_POINT('Ctrl Pts',(0.0128420950669967,-0.0336938721132327,
0.0774361527025199));
#87748=CARTESIAN_POINT('',(0.0128758210959443,-0.0336938721132427,0.0776037863093694));
#87749=CARTESIAN_POINT('Ctrl Pts',(0.0129014049545757,-0.0337108120662656,
0.0777796447058001));
#87750=CARTESIAN_POINT('Ctrl Pts',(0.0128671659171043,-0.0337611408993509,
0.0777536327020706));
#87751=CARTESIAN_POINT('Ctrl Pts',(0.0128335516661034,-0.0338121088779705,
0.0777280953596984));
#87752=CARTESIAN_POINT('Ctrl Pts',(0.0127675421147982,-0.0339153382773232,
0.0776779467334068));
#87753=CARTESIAN_POINT('Ctrl Pts',(0.0127351747407274,-0.0339675558473114,
0.0776533566655421));
#87754=CARTESIAN_POINT('Ctrl Pts',(0.0127034191046408,-0.0340203938281304,
0.0776292313458683));
#87755=CARTESIAN_POINT('Ctrl Pts',(0.0127759454407895,-0.0341934961088741,
0.0775291500940517));
#87756=CARTESIAN_POINT('Ctrl Pts',(0.0128458067068495,-0.0340287516182428,
0.0774329702839352));
#87757=CARTESIAN_POINT('Ctrl Pts',(0.0129116330932742,-0.0338644633275951,
0.0773339852385));
#87758=CARTESIAN_POINT('Ctrl Pts',(0.0127779549413508,-0.0341934961088741,
0.0775288757049524));
#87759=CARTESIAN_POINT('Ctrl Pts',(0.0128478105346324,-0.0340287516182428,
0.077432654349995));
#87760=CARTESIAN_POINT('Ctrl Pts',(0.0129136295360461,-0.0338644633275951,
0.0773336280296782));
#87761=CARTESIAN_POINT('Ctrl Pts',(0.0131127763861176,-0.0341934961088741,
0.0774831572033518));
#87762=CARTESIAN_POINT('Ctrl Pts',(0.0131816867853961,-0.0340287516182428,
0.0773800136788001));
#87763=CARTESIAN_POINT('Ctrl Pts',(0.0132462753019362,-0.0338644633275951,
0.0772741101693359));
#87764=CARTESIAN_POINT('',(0.0131198846871562,-0.0341764758832447,0.0774724930187678));
#87765=CARTESIAN_POINT('',(0.0131127763861026,-0.034193496108874,0.0774831572033539));
#87766=CARTESIAN_POINT('Origin',(-0.000383910481475924,-0.0345621026348341,
0.0678772417603383));
#87767=CARTESIAN_POINT('Ctrl Pts',(0.013119884685544,-0.0341764758837558,
0.0774724930196175));
#87768=CARTESIAN_POINT('Ctrl Pts',(0.0130841422462247,-0.034126005004086,
0.0774487237068725));
#87769=CARTESIAN_POINT('Ctrl Pts',(0.013049021073664,-0.0340749269148957,
0.0774253675926721));
#87770=CARTESIAN_POINT('Ctrl Pts',(0.01297999414439,-0.0339715436308211,
0.0773794635074193));
#87771=CARTESIAN_POINT('Ctrl Pts',(0.0129461145781926,-0.0339192778238913,
0.0773569329463197));
#87772=CARTESIAN_POINT('Ctrl Pts',(0.0129128449824776,-0.0338664212856685,
0.077334808097604));
#87773=CARTESIAN_POINT('',(0.0129453656637368,-0.0341934961088841,0.0775060164541632));
#87774=CARTESIAN_POINT('Origin',(0.00812378219310841,-0.0315241814719618,
0.07415));
#87775=CARTESIAN_POINT('',(0.013119884687007,-0.034210518019052,0.0774724930176583));
#87776=CARTESIAN_POINT('',(0.0131269701953153,-0.0341934961088739,0.0774618136744959));
#87777=CARTESIAN_POINT('Origin',(-0.00041319630938822,-0.0345621720619559,
0.0679118349174756));
#87778=CARTESIAN_POINT('Origin',(-0.000951059373476715,-0.0345621029033183,
0.0687300747565296));
#87779=CARTESIAN_POINT('Origin',(-0.000930482404601438,-0.0345621725052226,
0.0686896903395078));
#87780=CARTESIAN_POINT('Ctrl Pts',(0.0128416645176694,-0.0346945769586965,
0.077439390311912));
#87781=CARTESIAN_POINT('Ctrl Pts',(0.0129105621147524,-0.0345275153362943,
0.0773405723776871));
#87782=CARTESIAN_POINT('Ctrl Pts',(0.0129763697992073,-0.0343603235965185,
0.0772395621180704));
#87783=CARTESIAN_POINT('Ctrl Pts',(0.0130388973812223,-0.0341934961088739,
0.0771366611692789));
#87784=CARTESIAN_POINT('Ctrl Pts',(0.0128880871303978,-0.0346945769586965,
0.0773695836546843));
#87785=CARTESIAN_POINT('Ctrl Pts',(0.0129555225990961,-0.0345275153362943,
0.0772697933802492));
#87786=CARTESIAN_POINT('Ctrl Pts',(0.0130198371977804,-0.0343603235965185,
0.0771678565115172));
#87787=CARTESIAN_POINT('Ctrl Pts',(0.0130808451932546,-0.0341934961088739,
0.0770640773595722));
#87788=CARTESIAN_POINT('Ctrl Pts',(0.0129345097431261,-0.0346945769586965,
0.0772997769974551));
#87789=CARTESIAN_POINT('Ctrl Pts',(0.0130004830834395,-0.0345275153362943,
0.0771990143828112));
#87790=CARTESIAN_POINT('Ctrl Pts',(0.0130633045963531,-0.0343603235965185,
0.0770961509049639));
#87791=CARTESIAN_POINT('Ctrl Pts',(0.0131227930052867,-0.0341934961088739,
0.0769914935498638));
#87792=CARTESIAN_POINT('Ctrl Pts',(0.0129809323558545,-0.0346945769586965,
0.0772299703402289));
#87793=CARTESIAN_POINT('Ctrl Pts',(0.0130454435677835,-0.0345275153362943,
0.0771282353853734));
#87794=CARTESIAN_POINT('Ctrl Pts',(0.0131067719949265,-0.0343603235965185,
0.0770244452984109));
#87795=CARTESIAN_POINT('Ctrl Pts',(0.0131647408173194,-0.0341934961088739,
0.0769189097401589));
#87796=CARTESIAN_POINT('',(0.0129809323555189,-0.0346945769586966,0.0772299703407333));
#87797=CARTESIAN_POINT('',(0.0131033706147947,-0.034366772783154,0.0770278158647057));
#87798=CARTESIAN_POINT('Origin',(-0.00131567092393877,-0.0345626457064043,
0.0683809940206447));
#87799=CARTESIAN_POINT('Origin',(0.0226724682876334,-0.0341934771029036,
0.0825580079216642));
#87800=CARTESIAN_POINT('',(0.0130396479434198,-0.034193496108874,0.0771353624444808));
#87801=CARTESIAN_POINT('',(0.0130709211618275,-0.0341934961088839,0.077081249268544));
#87802=CARTESIAN_POINT('',(0.0129128449811174,-0.0345211942962608,0.0773348080966584));
#87803=CARTESIAN_POINT('Origin',(-0.00104665393795225,-0.0345625596120493,
0.0679824709331373));
#87804=CARTESIAN_POINT('',(0.0129117137509639,-0.0346945769586885,0.0773340558093871));
#87805=CARTESIAN_POINT('Origin',(0.0221241656625528,-0.034694568585385,
0.0834604940055356));
#87806=CARTESIAN_POINT('',(0.0129463230532514,-0.0346945769587025,0.0772820130750702));
#87807=CARTESIAN_POINT('Ctrl Pts',(0.0129858144645065,-0.0345231616327842,
0.0776657704976263));
#87808=CARTESIAN_POINT('Ctrl Pts',(0.0130342744110074,-0.0344132092796988,
0.0775987542279589));
#87809=CARTESIAN_POINT('Ctrl Pts',(0.0130813456785214,-0.0343032738558979,
0.0775307390602543));
#87810=CARTESIAN_POINT('Ctrl Pts',(0.013126970195318,-0.0341934961088739,
0.0774618136745056));
#87811=CARTESIAN_POINT('Ctrl Pts',(0.012961081907181,-0.0345231616327842,
0.0775551837138443));
#87812=CARTESIAN_POINT('Ctrl Pts',(0.0130080175705612,-0.0344132092796988,
0.077488508347659));
#87813=CARTESIAN_POINT('Ctrl Pts',(0.0130535716849201,-0.0343032738558979,
0.0774208655944415));
#87814=CARTESIAN_POINT('Ctrl Pts',(0.0130976881099546,-0.0341934961088739,
0.0773523436072915));
#87815=CARTESIAN_POINT('Ctrl Pts',(0.0129363493498555,-0.0345231616327842,
0.0774445969300623));
#87816=CARTESIAN_POINT('Ctrl Pts',(0.012981760730115,-0.0344132092796988,
0.0773782624673591));
#87817=CARTESIAN_POINT('Ctrl Pts',(0.0130257976913189,-0.0343032738558979,
0.0773109921286286));
#87818=CARTESIAN_POINT('Ctrl Pts',(0.0130684060245911,-0.0341934961088739,
0.0772428735400773));
#87819=CARTESIAN_POINT('Ctrl Pts',(0.01291161679253,-0.0345231616327842,
0.0773340101462804));
#87820=CARTESIAN_POINT('Ctrl Pts',(0.0129555038896688,-0.0344132092796988,
0.0772680165870592));
#87821=CARTESIAN_POINT('Ctrl Pts',(0.0129980236977176,-0.0343032738558979,
0.0772011186628158));
#87822=CARTESIAN_POINT('Ctrl Pts',(0.0130391239392277,-0.0341934961088739,
0.0771334034728632));
#87823=CARTESIAN_POINT('',(0.0130833090693775,-0.0341934961088839,0.0772985880594983));
#87824=CARTESIAN_POINT('Ctrl Pts',(0.0131198846841247,-0.0342105180195354,
0.0774724930157396));
#87825=CARTESIAN_POINT('Ctrl Pts',(0.013084102071013,-0.0342610556240321,
0.0774486969702496));
#87826=CARTESIAN_POINT('Ctrl Pts',(0.0130489615583901,-0.034312218986816,
0.077425327932491));
#87827=CARTESIAN_POINT('Ctrl Pts',(0.0129799339303926,-0.0344158119695075,
0.0773794233874327));
#87828=CARTESIAN_POINT('Ctrl Pts',(0.012946075048014,-0.034468199044995,
0.0773569066555551));
#87829=CARTESIAN_POINT('Ctrl Pts',(0.0129128449810918,-0.0345211942962356,
0.0773348080966363));
#87830=CARTESIAN_POINT('Ctrl Pts',(0.0129789445361091,-0.0346945769586932,
0.077230370268035));
#87831=CARTESIAN_POINT('Ctrl Pts',(0.0130426290118006,-0.034529677707698,
0.077129993221996));
#87832=CARTESIAN_POINT('Ctrl Pts',(0.0131021103943521,-0.0343648066251421,
0.0770270698089874));
#87833=CARTESIAN_POINT('Ctrl Pts',(0.012980932355514,-0.0346945769586932,
0.0772299703407409));
#87834=CARTESIAN_POINT('Ctrl Pts',(0.0130446085629917,-0.034529677707698,
0.0771295521979423));
#87835=CARTESIAN_POINT('Ctrl Pts',(0.0131040799858276,-0.0343648066251421,
0.0770265880650236));
#87836=CARTESIAN_POINT('Ctrl Pts',(0.0133122224181741,-0.0346945769586932,
0.0771633184416937));
#87837=CARTESIAN_POINT('Ctrl Pts',(0.0133745206448003,-0.034529677707698,
0.0770560511112629));
#87838=CARTESIAN_POINT('Ctrl Pts',(0.0134323321810336,-0.0343648066251421,
0.0769463005964721));
#87839=CARTESIAN_POINT('',(0.0133186470831683,-0.0346775396665031,0.0771522289665511));
#87840=CARTESIAN_POINT('',(0.0133122224181615,-0.0346945769586886,0.0771633184416935));
#87841=CARTESIAN_POINT('Origin',(-0.00113099879810727,-0.0345626618834468,
0.0689778404592653));
#87842=CARTESIAN_POINT('Ctrl Pts',(0.0133186470815555,-0.0346775396670097,
0.0771522289674092));
#87843=CARTESIAN_POINT('Ctrl Pts',(0.0132814534144467,-0.0346269749928195,
0.0771307339276362));
#87844=CARTESIAN_POINT('Ctrl Pts',(0.0132449207438227,-0.0345757902890808,
0.0771096209337837));
#87845=CARTESIAN_POINT('Ctrl Pts',(0.0131731473949716,-0.0344721681087884,
0.0770681415008954));
#87846=CARTESIAN_POINT('Ctrl Pts',(0.0131379348580869,-0.0344197714289365,
0.0770477913188639));
#87847=CARTESIAN_POINT('Ctrl Pts',(0.0131033706147641,-0.0343667727830768,
0.0770278158649634));
#87848=CARTESIAN_POINT('',(0.0131465773868502,-0.0346945769587026,0.0771966443912234));
#87849=CARTESIAN_POINT('Origin',(0.00812378219310841,-0.0315241814719618,
0.07415));
#87850=CARTESIAN_POINT('',(0.0133186470825154,-0.0347116136489778,0.0771522289653209));
#87851=CARTESIAN_POINT('',(0.0133250480478685,-0.0346945769586885,0.0771411257927598));
#87852=CARTESIAN_POINT('Origin',(-0.00115203163608611,-0.0345626701708096,
0.0690179742157668));
#87853=CARTESIAN_POINT('Origin',(-0.000978169355718683,-0.0345626620963308,
0.0687133923034704));
#87854=CARTESIAN_POINT('Origin',(-0.000953894743002916,-0.0345626704262437,
0.0686751321063215));
#87855=CARTESIAN_POINT('Ctrl Pts',(0.0130195361216765,-0.0352450361874067,
0.0771683366440036));
#87856=CARTESIAN_POINT('Ctrl Pts',(0.013133374556207,-0.0349452760959492,
0.0769836902546812));
#87857=CARTESIAN_POINT('Ctrl Pts',(0.0132329812661732,-0.034644428984174,
0.0767909936496363));
#87858=CARTESIAN_POINT('Ctrl Pts',(0.0130208132564897,-0.0352450361874067,
0.0771661584448234));
#87859=CARTESIAN_POINT('Ctrl Pts',(0.01313456953889,-0.0349452760959492,
0.076981463887571));
#87860=CARTESIAN_POINT('Ctrl Pts',(0.013234090701906,-0.034644428984174,
0.0767887254394709));
#87861=CARTESIAN_POINT('Ctrl Pts',(0.0131472622478912,-0.0352450361874067,
0.0769504951596458));
#87862=CARTESIAN_POINT('Ctrl Pts',(0.0132528846560204,-0.0349452760959492,
0.0767610315004255));
#87863=CARTESIAN_POINT('Ctrl Pts',(0.0133439358239721,-0.034644428984174,
0.0765641501755652));
#87864=CARTESIAN_POINT('Ctrl Pts',(0.0131485267378052,-0.0352450361874067,
0.076948338526794));
#87865=CARTESIAN_POINT('Ctrl Pts',(0.0132540678071917,-0.0349452760959492,
0.0767588271765541));
#87866=CARTESIAN_POINT('Ctrl Pts',(0.0133450342751927,-0.034644428984174,
0.0765619044229261));
#87867=CARTESIAN_POINT('',(0.0131647273186907,-0.0351951634053349,0.0769189392451548));
#87868=CARTESIAN_POINT('',(0.0132742440876456,-0.0348678972925388,0.0767094662085914));
#87869=CARTESIAN_POINT('Origin',(-0.00191268559069225,-0.0345636767881609,
0.0696336035408099));
#87870=CARTESIAN_POINT('Origin',(0.0231696076725555,-0.0346946199340784,
0.0816268607243761));
#87871=CARTESIAN_POINT('',(0.0132174000556613,-0.0346945769330289,0.076820801765112));
#87872=CARTESIAN_POINT('',(0.0132452137732655,-0.0346945769458128,0.0767648316998928));
#87873=CARTESIAN_POINT('',(0.0131033706146427,-0.0350221583435276,0.0770278158648744));
#87874=CARTESIAN_POINT('Origin',(-0.00173667969852291,-0.0345628458715479,
0.0691862051510017));
#87875=CARTESIAN_POINT('',(0.0131022981931494,-0.0351951360298762,0.0770271995817522));
#87876=CARTESIAN_POINT('Origin',(0.0226426482481184,-0.0351951838366873,
0.0825407796087665));
#87877=CARTESIAN_POINT('',(0.0131647408171114,-0.0351951371328746,0.076918909740751));
#87878=CARTESIAN_POINT('Ctrl Pts',(0.0131969779234846,-0.0350241211494343,
0.0773535425830464));
#87879=CARTESIAN_POINT('Ctrl Pts',(0.0132411054090624,-0.0349144232818962,
0.0772836613919517));
#87880=CARTESIAN_POINT('Ctrl Pts',(0.0132838148129131,-0.0348045283579412,
0.0772128262269371));
#87881=CARTESIAN_POINT('Ctrl Pts',(0.0133250480534117,-0.0346945769439158,
0.0771411257831361));
#87882=CARTESIAN_POINT('Ctrl Pts',(0.0131653503442054,-0.0350241211494343,
0.0772447269682087));
#87883=CARTESIAN_POINT('Ctrl Pts',(0.013207978939305,-0.0349144232818962,
0.0771752814340508));
#87884=CARTESIAN_POINT('Ctrl Pts',(0.0132491975608594,-0.0348045283579412,
0.0771049131698718));
#87885=CARTESIAN_POINT('Ctrl Pts',(0.0132889500590009,-0.0346945769439158,
0.0770337103438218));
#87886=CARTESIAN_POINT('Ctrl Pts',(0.0131337227649262,-0.0350241211494343,
0.077135911353371));
#87887=CARTESIAN_POINT('Ctrl Pts',(0.0131748524695475,-0.0349144232818962,
0.0770669014761498));
#87888=CARTESIAN_POINT('Ctrl Pts',(0.0132145803088056,-0.0348045283579412,
0.0769970001128065));
#87889=CARTESIAN_POINT('Ctrl Pts',(0.0132528520645901,-0.0346945769439158,
0.0769262949045074));
#87890=CARTESIAN_POINT('Ctrl Pts',(0.013102095185647,-0.0350241211494343,
0.0770270957385332));
#87891=CARTESIAN_POINT('Ctrl Pts',(0.0131417259997901,-0.0349144232818962,
0.0769585215182488));
#87892=CARTESIAN_POINT('Ctrl Pts',(0.0131799630567519,-0.0348045283579412,
0.0768890870557412));
#87893=CARTESIAN_POINT('Ctrl Pts',(0.0132167540701793,-0.0346945769439158,
0.0768188794651931));
#87894=CARTESIAN_POINT('',(0.0132712240517077,-0.0346945769458128,0.0769809637792386));
#87895=CARTESIAN_POINT('Ctrl Pts',(0.0133186470796628,-0.034711613649276,
0.07715222896367));
#87896=CARTESIAN_POINT('Ctrl Pts',(0.0132814681894934,-0.0347621546531267,
0.0771307424489404));
#87897=CARTESIAN_POINT('Ctrl Pts',(0.0132449430046785,-0.0348133084094936,
0.0771096337252008));
#87898=CARTESIAN_POINT('Ctrl Pts',(0.0131731695627246,-0.0349168561544566,
0.0770681542428732));
#87899=CARTESIAN_POINT('Ctrl Pts',(0.0131379497746807,-0.0349692089015913,
0.0770477999372138));
#87900=CARTESIAN_POINT('Ctrl Pts',(0.013103370614621,-0.0350221583435,0.0770278158648389));
#87901=CARTESIAN_POINT('Ctrl Pts',(0.0131633274884781,-0.0351951371254979,
0.0769192877911379));
#87902=CARTESIAN_POINT('Ctrl Pts',(0.013220580776051,-0.0350307338980974,
0.0768150983540717));
#87903=CARTESIAN_POINT('Ctrl Pts',(0.0132734788791687,-0.0348659306897824,
0.0767086316061143));
#87904=CARTESIAN_POINT('Ctrl Pts',(0.0131647408170057,-0.0351951371254979,
0.0769189097407023));
#87905=CARTESIAN_POINT('Ctrl Pts',(0.0132219862886231,-0.0350307338980974,
0.0768146910839556));
#87906=CARTESIAN_POINT('Ctrl Pts',(0.013274875374783,-0.0348659306897824,
0.0767081954643276));
#87907=CARTESIAN_POINT('Ctrl Pts',(0.0134016161512906,-0.0351951371254979,
0.0768555480936741));
#87908=CARTESIAN_POINT('Ctrl Pts',(0.0134575516606101,-0.0350307338980974,
0.0767464321880115));
#87909=CARTESIAN_POINT('Ctrl Pts',(0.0135089294952453,-0.0348659306897824,
0.0766350976462934));
#87910=CARTESIAN_POINT('Origin',(0.0180367870874105,-0.0308609197410571,
0.0790761603273267));
#87911=CARTESIAN_POINT('',(0.0132680131219248,-0.0351951371254979,0.0768912854912133));
#87912=CARTESIAN_POINT('Origin',(0.00719498968780964,-0.0351840467441105,
0.0738465364396827));
#87913=CARTESIAN_POINT('Origin',(0.0191690556789188,-0.0352322613362849,
0.0787514059328649));
#87914=CARTESIAN_POINT('',(0.0133751536690105,-0.0351951142564687,0.0764954023547165));
#87915=CARTESIAN_POINT('',(0.0134235389043139,-0.0351951372916787,0.0763804884671374));
#87916=CARTESIAN_POINT('Origin',(0.00807170863840627,-0.0352875125435763,
0.07381338790932));
#87917=CARTESIAN_POINT('Origin',(0.00394304548537184,-0.0298325076522644,
0.0803802994198087));
#87918=CARTESIAN_POINT('Origin',(0.0140569765020341,-0.0338732607737469,
0.0800699940465063));
#87919=CARTESIAN_POINT('Origin',(0.00812378219310841,-0.0315241814719618,
0.07415));
#87920=CARTESIAN_POINT('',(0.0115459495571206,-0.0322104233323599,0.0790783638781051));
#87921=CARTESIAN_POINT('',(0.0115564688245398,-0.0321934096636183,0.0790710428254998));
#87922=CARTESIAN_POINT('Origin',(0.00257773023980595,-0.0326387245949053,
0.0651660339478818));
#87923=CARTESIAN_POINT('',(0.0115459495569106,-0.032176398030852,0.0790783638778025));
#87924=CARTESIAN_POINT('Origin',(0.00161034854614262,-0.032638623529467,
0.0658454522903156));
#87925=CARTESIAN_POINT('',(0.0115354146774751,-0.0321934096636184,0.0790856624470899));
#87926=CARTESIAN_POINT('Origin',(0.00261820415429388,-0.0326386230888073,
0.0651456164874627));
#87927=CARTESIAN_POINT('Origin',(0.00164362107438124,-0.032638724894122,
0.0658146635723998));
#87928=CARTESIAN_POINT('Ctrl Pts',(0.0109933420942546,-0.0321934096636941,
0.079134351684928));
#87929=CARTESIAN_POINT('Ctrl Pts',(0.011082559615781,-0.0320508460845128,
0.0790829879292312));
#87930=CARTESIAN_POINT('Ctrl Pts',(0.011170329824236,-0.0319086045664672,
0.0790292658032143));
#87931=CARTESIAN_POINT('Ctrl Pts',(0.0112564732578548,-0.031766989287029,
0.0789733165384563));
#87932=CARTESIAN_POINT('Ctrl Pts',(0.0110650810268201,-0.0321934096636941,
0.0790909470978186));
#87933=CARTESIAN_POINT('Ctrl Pts',(0.0111535216269072,-0.0320508460845128,
0.0790382992493922));
#87934=CARTESIAN_POINT('Ctrl Pts',(0.0112404809986863,-0.0319086045664672,
0.0789833148732019));
#87935=CARTESIAN_POINT('Ctrl Pts',(0.0113257816500166,-0.031766989287029,
0.0789261277749424));
#87936=CARTESIAN_POINT('Ctrl Pts',(0.0111368199593854,-0.0321934096636941,
0.0790475425107093));
#87937=CARTESIAN_POINT('Ctrl Pts',(0.0112244836380333,-0.0320508460845128,
0.0789936105695533));
#87938=CARTESIAN_POINT('Ctrl Pts',(0.0113106321731366,-0.0319086045664672,
0.0789373639431895));
#87939=CARTESIAN_POINT('Ctrl Pts',(0.0113950900421785,-0.031766989287029,
0.0788789390114283));
#87940=CARTESIAN_POINT('Ctrl Pts',(0.0112085588919508,-0.0321934096636941,
0.0790041379235999));
#87941=CARTESIAN_POINT('Ctrl Pts',(0.0112954456491594,-0.0320508460845128,
0.0789489218897142));
#87942=CARTESIAN_POINT('Ctrl Pts',(0.0113807833475869,-0.0319086045664672,
0.0788914130131771));
#87943=CARTESIAN_POINT('Ctrl Pts',(0.0114643984343405,-0.031766989287029,
0.0788317502479143));
#87944=CARTESIAN_POINT('',(0.0112072754682696,-0.0321934096636941,0.0790049144402385));
#87945=CARTESIAN_POINT('',(0.0114041341063444,-0.031866561751136,0.0788741312761827));
#87946=CARTESIAN_POINT('Origin',(0.0027737510633533,-0.032637194442029,
0.0645794657143673));
#87947=CARTESIAN_POINT('Origin',(0.0176559693908919,-0.0316939261509218,
0.0878775831536998));
#87948=CARTESIAN_POINT('',(0.0111012323342595,-0.0320197221621754,0.0790706076681135));
#87949=CARTESIAN_POINT('Ctrl Pts',(0.0111014097812802,-0.0320197392094669,
0.0790705554432635));
#87950=CARTESIAN_POINT('Ctrl Pts',(0.0111264471249915,-0.0319792716575967,
0.0790554042766529));
#87951=CARTESIAN_POINT('Ctrl Pts',(0.0111514829418241,-0.0319386439829653,
0.0790399932615345));
#87952=CARTESIAN_POINT('Ctrl Pts',(0.011176539081177,-0.0318979099381586,
0.0790242990169));
#87953=CARTESIAN_POINT('Ctrl Pts',(0.0112015947252764,-0.0318571766984909,
0.0790086050824741));
#87954=CARTESIAN_POINT('Ctrl Pts',(0.0112265442877187,-0.0318163871833581,
0.0789927092064922));
#87955=CARTESIAN_POINT('Ctrl Pts',(0.0112513038443118,-0.0317755399638303,
0.0789766690338607));
#87956=CARTESIAN_POINT('',(0.0111003271651873,-0.0321934096636183,0.0790696219396608));
#87957=CARTESIAN_POINT('Origin',(0.0123129570727762,-0.0324111971803128,
0.0810332308586919));
#87958=CARTESIAN_POINT('',(0.0111538013167385,-0.0321934096636663,0.0790372681899597));
#87959=CARTESIAN_POINT('Ctrl Pts',(0.0112053059993892,-0.0321934096636617,
0.0790044297963401));
#87960=CARTESIAN_POINT('Ctrl Pts',(0.011272252369602,-0.0320835708272591,
0.0789619331814523));
#87961=CARTESIAN_POINT('Ctrl Pts',(0.011338280442963,-0.0319739230346488,
0.078918075764676));
#87962=CARTESIAN_POINT('Ctrl Pts',(0.0114033100476125,-0.0318646057455572,
0.0788729201420098));
#87963=CARTESIAN_POINT('Ctrl Pts',(0.0113153422254146,-0.0321934096636617,
0.0790315073465977));
#87964=CARTESIAN_POINT('Ctrl Pts',(0.0113826620161486,-0.0320835708272591,
0.0789874932463957));
#87965=CARTESIAN_POINT('Ctrl Pts',(0.0114490318891518,-0.0319739230346488,
0.0789421114965902));
#87966=CARTESIAN_POINT('Ctrl Pts',(0.0115143713849343,-0.0318646057455572,
0.0788954266770202));
#87967=CARTESIAN_POINT('Ctrl Pts',(0.0114253784514401,-0.0321934096636617,
0.0790585848968552));
#87968=CARTESIAN_POINT('Ctrl Pts',(0.0114930716626951,-0.0320835708272591,
0.0790130533113391));
#87969=CARTESIAN_POINT('Ctrl Pts',(0.0115597833353406,-0.0319739230346488,
0.0789661472285044));
#87970=CARTESIAN_POINT('Ctrl Pts',(0.0116254327222561,-0.0318646057455572,
0.0789179332120306));
#87971=CARTESIAN_POINT('Ctrl Pts',(0.0115354146774656,-0.0321934096636617,
0.0790856624471127));
#87972=CARTESIAN_POINT('Ctrl Pts',(0.0116034813092416,-0.0320835708272591,
0.0790386133762826));
#87973=CARTESIAN_POINT('Ctrl Pts',(0.0116705347815294,-0.0319739230346488,
0.0789901829604186));
#87974=CARTESIAN_POINT('Ctrl Pts',(0.0117364940595778,-0.0318646057455572,
0.0789404397470411));
#87975=CARTESIAN_POINT('Ctrl Pts',(0.0115459495550968,-0.0321763980306386,
0.0790783638751927));
#87976=CARTESIAN_POINT('Ctrl Pts',(0.0115214702824469,-0.0321259596176341,
0.0790431105546337));
#87977=CARTESIAN_POINT('Ctrl Pts',(0.0114974151449519,-0.0320749164634415,
0.0790084680435985));
#87978=CARTESIAN_POINT('Ctrl Pts',(0.0114501337812436,-0.0319716057794034,
0.0789403767610218));
#87979=CARTESIAN_POINT('Ctrl Pts',(0.0114269259776363,-0.0319193786690241,
0.0789069545204173));
#87980=CARTESIAN_POINT('Ctrl Pts',(0.0114041341052815,-0.0318665617525439,
0.0788741312746552));
#87981=CARTESIAN_POINT('',(0.0113713450728824,-0.0321934096636663,0.0790452884436742));
#87982=CARTESIAN_POINT('Ctrl Pts',(0.0112704926892643,-0.0327445246967096,
0.0789641809327634));
#87983=CARTESIAN_POINT('Ctrl Pts',(0.0114520624914076,-0.032443687833936,
0.0788455008062437));
#87984=CARTESIAN_POINT('Ctrl Pts',(0.0116241770007383,-0.0321434074405927,
0.0787134812578467));
#87985=CARTESIAN_POINT('Ctrl Pts',(0.0114767332300399,-0.0327445246967096,
0.0788228839429136));
#87986=CARTESIAN_POINT('Ctrl Pts',(0.011652973929092,-0.032443687833936,
0.0786964253272376));
#87987=CARTESIAN_POINT('Ctrl Pts',(0.0118191885671562,-0.0321434074405927,
0.0785570507973754));
#87988=CARTESIAN_POINT('',(0.0115060334985778,-0.0326943950436612,0.0788017202309093));
#87989=CARTESIAN_POINT('',(0.0116942917389023,-0.0323666188837389,0.0786588342820951));
#87990=CARTESIAN_POINT('Origin',(0.0015584957656978,-0.0326395579111893,
0.0652497996555712));
#87991=CARTESIAN_POINT('Origin',(0.0185509122750033,-0.0321933825603024,
0.0873173634101982));
#87992=CARTESIAN_POINT('',(0.0115954533556887,-0.032193409653269,0.0787353706868489));
#87993=CARTESIAN_POINT('',(0.011644450849865,-0.0321934096584275,0.078696569966362));
#87994=CARTESIAN_POINT('',(0.0114041341068709,-0.0325210109756239,0.078874131276952));
#87995=CARTESIAN_POINT('Origin',(0.00196176277145783,-0.0326393129156889,
0.0649879597203443));
#87996=CARTESIAN_POINT('',(0.0114033592510911,-0.0326943950436593,0.0788730153843445));
#87997=CARTESIAN_POINT('Origin',(0.0177129541740383,-0.0326943765538247,
0.0879596499987013));
#87998=CARTESIAN_POINT('',(0.0114546963748445,-0.0326943950436702,0.0788373678076369));
#87999=CARTESIAN_POINT('Ctrl Pts',(0.0113501439061946,-0.0325229783203769,
0.0792087142730545));
#88000=CARTESIAN_POINT('Ctrl Pts',(0.0114198781718219,-0.032413025309245,
0.0791642389473955));
#88001=CARTESIAN_POINT('Ctrl Pts',(0.0114886818316376,-0.032303122220807,
0.0791183278244265));
#88002=CARTESIAN_POINT('Ctrl Pts',(0.0115564688282168,-0.0321934096576658,
0.0790710428229413));
#88003=CARTESIAN_POINT('Ctrl Pts',(0.011367857873235,-0.0325229783203769,
0.0790967885941045));
#88004=CARTESIAN_POINT('Ctrl Pts',(0.0114360492458256,-0.032413025309245,
0.0790520690817973));
#88005=CARTESIAN_POINT('Ctrl Pts',(0.0115033051953001,-0.032303122220807,
0.0790059457259401));
#88006=CARTESIAN_POINT('Ctrl Pts',(0.0115695416563333,-0.0321934096576658,
0.078958480647226));
#88007=CARTESIAN_POINT('Ctrl Pts',(0.0113855718402754,-0.0325229783203769,
0.0789848629151546));
#88008=CARTESIAN_POINT('Ctrl Pts',(0.0114522203198293,-0.032413025309245,
0.078939899216199));
#88009=CARTESIAN_POINT('Ctrl Pts',(0.0115179285589626,-0.032303122220807,
0.0788935636274538));
#88010=CARTESIAN_POINT('Ctrl Pts',(0.0115826144844499,-0.0321934096576658,
0.0788459184715107));
#88011=CARTESIAN_POINT('Ctrl Pts',(0.0114032858073158,-0.0325229783203769,
0.0788729372362046));
#88012=CARTESIAN_POINT('Ctrl Pts',(0.0114683913938331,-0.032413025309245,
0.0788277293506008));
#88013=CARTESIAN_POINT('Ctrl Pts',(0.0115325519226251,-0.032303122220807,
0.0787811815289674));
#88014=CARTESIAN_POINT('Ctrl Pts',(0.0115956873125665,-0.0321934096576658,
0.0787333562957954));
#88015=CARTESIAN_POINT('',(0.0115759610898133,-0.0321934096584275,0.0789032067565886));
#88016=CARTESIAN_POINT('Ctrl Pts',(0.0115459495551305,-0.0322104233328908,
0.0790783638752414));
#88017=CARTESIAN_POINT('Ctrl Pts',(0.0115214371126354,-0.0322609421830669,
0.0790430627858127));
#88018=CARTESIAN_POINT('Ctrl Pts',(0.0114973657711097,-0.0323120888239312,
0.0790083969388642));
#88019=CARTESIAN_POINT('Ctrl Pts',(0.0114500840494887,-0.0324156524631813,
0.078940305140847));
#88020=CARTESIAN_POINT('Ctrl Pts',(0.0114268931047555,-0.0324680267167303,
0.0789069071792147));
#88021=CARTESIAN_POINT('Ctrl Pts',(0.0114041341068498,-0.0325210109755912,
0.0788741312769138));
#88022=CARTESIAN_POINT('Origin',(0.00116774491061051,-0.0262834582510706,
0.0778265379320862));
#88023=CARTESIAN_POINT('Origin',(0.00985802840244437,-0.034277079370463,
0.0861839400837242));
#88024=CARTESIAN_POINT('Ctrl Pts',(0.0115040379693967,-0.0326943950436604,
0.0788013602946374));
#88025=CARTESIAN_POINT('Ctrl Pts',(0.011568142431835,-0.0325844576448134,
0.0787547740347656));
#88026=CARTESIAN_POINT('Ctrl Pts',(0.0116312879508125,-0.0324744968375323,
0.0787068586925279));
#88027=CARTESIAN_POINT('Ctrl Pts',(0.0116933944673868,-0.0323646534831895,
0.0786576767757881));
#88028=CARTESIAN_POINT('Ctrl Pts',(0.011615557116054,-0.0326943950436604,
0.0788214751526123));
#88029=CARTESIAN_POINT('Ctrl Pts',(0.0116799387989345,-0.0325844576448134,
0.0787733519498904));
#88030=CARTESIAN_POINT('Ctrl Pts',(0.0117433297714754,-0.0324744968375323,
0.0787238938226575));
#88031=CARTESIAN_POINT('Ctrl Pts',(0.0118056496875099,-0.0323646534831895,
0.0786731652598213));
#88032=CARTESIAN_POINT('Ctrl Pts',(0.0117270762627113,-0.0326943950436604,
0.0788415900105872));
#88033=CARTESIAN_POINT('Ctrl Pts',(0.011791735166034,-0.0325844576448134,
0.0787919298650152));
#88034=CARTESIAN_POINT('Ctrl Pts',(0.0118553715921384,-0.0324744968375323,
0.0787409289527872));
#88035=CARTESIAN_POINT('Ctrl Pts',(0.011917904907633,-0.0323646534831895,
0.0786886537438546));
#88036=CARTESIAN_POINT('Ctrl Pts',(0.0118385954093686,-0.0326943950436604,
0.0788617048685621));
#88037=CARTESIAN_POINT('Ctrl Pts',(0.0119035315331335,-0.0325844576448134,
0.07881050778014));
#88038=CARTESIAN_POINT('Ctrl Pts',(0.0119674134128014,-0.0324744968375323,
0.0787579640829168));
#88039=CARTESIAN_POINT('Ctrl Pts',(0.0120301601277561,-0.0323646534831895,
0.0787041422278879));
#88040=CARTESIAN_POINT('',(0.0118486512197805,-0.0326773559991214,0.0788537592109377));
#88041=CARTESIAN_POINT('',(0.0118385954093546,-0.0326943950436594,0.078861704868559));
#88042=CARTESIAN_POINT('Origin',(0.00150060062565762,-0.0326395670099125,
0.0658671835419942));
#88043=CARTESIAN_POINT('Ctrl Pts',(0.0118486512176951,-0.0326773559987507,
0.0788537592083056));
#88044=CARTESIAN_POINT('Ctrl Pts',(0.0118219852332526,-0.0326267922587257,
0.0788200854417806));
#88045=CARTESIAN_POINT('Ctrl Pts',(0.0117957918841262,-0.0325756109581914,
0.0787870085184482));
#88046=CARTESIAN_POINT('Ctrl Pts',(0.0117443281644271,-0.0324719985462387,
0.0787220202077638));
#88047=CARTESIAN_POINT('Ctrl Pts',(0.0117190784347338,-0.0324196091621786,
0.0786901348856845));
#88048=CARTESIAN_POINT('Ctrl Pts',(0.011694291738872,-0.0323666188837757,
0.0786588342820569));
#88049=CARTESIAN_POINT('',(0.0116723144539762,-0.0326943950436703,0.0788317125497442));
#88050=CARTESIAN_POINT('Origin',(0.00812378219310841,-0.0315241814719618,
0.07415));
#88051=CARTESIAN_POINT('',(0.0118486512197516,-0.0327114338379854,0.0788537592109012));
#88052=CARTESIAN_POINT('',(0.0118586900372345,-0.0326943950436593,0.0788457920946194));
#88053=CARTESIAN_POINT('Origin',(0.00146556789155393,-0.0326395682109143,
0.0658959171250404));
#88054=CARTESIAN_POINT('Origin',(0.00157937342544954,-0.0326395672564601,
0.0658048029865228));
#88055=CARTESIAN_POINT('Origin',(0.00161537198770351,-0.0326395685302088,
0.0657772892051259));
#88056=CARTESIAN_POINT('Ctrl Pts',(0.0115665997166451,-0.0332451089994585,
0.0787570741799572));
#88057=CARTESIAN_POINT('Ctrl Pts',(0.0117403583622355,-0.0329451141709491,
0.0786272261925931));
#88058=CARTESIAN_POINT('Ctrl Pts',(0.0119038426966181,-0.0326442513125814,
0.0784846588781363));
#88059=CARTESIAN_POINT('Ctrl Pts',(0.0117635601273721,-0.0332451089994585,
0.0786031047134833));
#88060=CARTESIAN_POINT('Ctrl Pts',(0.0119315117195243,-0.0329451141709491,
0.07846582824269));
#88061=CARTESIAN_POINT('Ctrl Pts',(0.0120886459539547,-0.0326442513125814,
0.078316290959346));
#88062=CARTESIAN_POINT('Ctrl Pts',(0.0117655297314794,-0.0332451089994585,
0.0786015650188185));
#88063=CARTESIAN_POINT('Ctrl Pts',(0.0119334232530972,-0.0329451141709491,
0.0784642142631909));
#88064=CARTESIAN_POINT('Ctrl Pts',(0.012090493986528,-0.0326442513125814,
0.0783146072801581));
#88065=CARTESIAN_POINT('',(0.0117914433282327,-0.0331951640388616,0.0785801678069685));
#88066=CARTESIAN_POINT('',(0.0119703582153917,-0.0328677532355047,0.0784257429734079));
#88067=CARTESIAN_POINT('Origin',(0.00052063326854975,-0.0326402808277589,
0.0661704503204892));
#88068=CARTESIAN_POINT('Origin',(0.0193649979077478,-0.0326944278779025,
0.0866448479610499));
#88069=CARTESIAN_POINT('',(0.011876520618294,-0.032694395043354,0.0785083344653819));
#88070=CARTESIAN_POINT('',(0.0119229851075173,-0.0326943950435166,0.0784665337326721));
#88071=CARTESIAN_POINT('',(0.0116942917389,-0.0330220786163545,0.0786588342820969));
#88072=CARTESIAN_POINT('Origin',(0.000856285506988594,-0.0326396675542845,
0.0658262276307959));
#88073=CARTESIAN_POINT('',(0.0116934483446432,-0.0331951640388587,0.0786577692450465));
#88074=CARTESIAN_POINT('Origin',(0.0185420247646317,-0.0331952026560106,
0.0873061431128978));
#88075=CARTESIAN_POINT('',(0.0117424458364479,-0.0331951640388701,0.0786189685260174));
#88076=CARTESIAN_POINT('Ctrl Pts',(0.0116614174918026,-0.0330240426238182,
0.0789961465612907));
#88077=CARTESIAN_POINT('Ctrl Pts',(0.0117281778820919,-0.0329142774062944,
0.0789474121884741));
#88078=CARTESIAN_POINT('Ctrl Pts',(0.011793964079251,-0.0328043479725528,
0.0788972733960413));
#88079=CARTESIAN_POINT('Ctrl Pts',(0.0118586900373371,-0.0326943950434843,
0.0788457920945455));
#88080=CARTESIAN_POINT('Ctrl Pts',(0.0116720686121853,-0.0330240426238182,
0.0788833294986647));
#88081=CARTESIAN_POINT('Ctrl Pts',(0.0117372748375237,-0.0329142774062944,
0.0788344483962879));
#88082=CARTESIAN_POINT('Ctrl Pts',(0.0118015030616142,-0.0328043479725528,
0.0787841949300757));
#88083=CARTESIAN_POINT('Ctrl Pts',(0.0118646692303477,-0.0326943950434843,
0.0787326312124532));
#88084=CARTESIAN_POINT('Ctrl Pts',(0.011682719732568,-0.0330240426238182,
0.0787705124360388));
#88085=CARTESIAN_POINT('Ctrl Pts',(0.0117463717929555,-0.0329142774062944,
0.0787214846041017));
#88086=CARTESIAN_POINT('Ctrl Pts',(0.0118090420439774,-0.0328043479725527,
0.0786711164641102));
#88087=CARTESIAN_POINT('Ctrl Pts',(0.0118706484233582,-0.0326943950434843,
0.078619470330361));
#88088=CARTESIAN_POINT('Ctrl Pts',(0.0116933708529506,-0.0330240426238182,
0.0786576953734128));
#88089=CARTESIAN_POINT('Ctrl Pts',(0.0117554687483874,-0.0329142774062944,
0.0786085208119155));
#88090=CARTESIAN_POINT('Ctrl Pts',(0.0118165810263407,-0.0328043479725527,
0.0785580379981446));
#88091=CARTESIAN_POINT('Ctrl Pts',(0.0118766276163688,-0.0326943950434843,
0.0785063094482687));
#88092=CARTESIAN_POINT('',(0.0118676053277743,-0.0326943950435166,0.0786770632800107));
#88093=CARTESIAN_POINT('Ctrl Pts',(0.0118486512176875,-0.03271143383833,
0.0788537592082961));
#88094=CARTESIAN_POINT('Ctrl Pts',(0.0118219896686433,-0.0327619876830289,
0.0788200910427856));
#88095=CARTESIAN_POINT('Ctrl Pts',(0.0117957984859586,-0.0328131562602952,
0.0787870168552327));
#88096=CARTESIAN_POINT('Ctrl Pts',(0.0117443348135807,-0.0329167375858764,
0.0787220286043055));
#88097=CARTESIAN_POINT('Ctrl Pts',(0.0117190828297671,-0.0329691088920605,
0.0786901404357263));
#88098=CARTESIAN_POINT('Ctrl Pts',(0.0116942917388726,-0.0330220786163186,
0.0786588342820579));
#88099=CARTESIAN_POINT('Ctrl Pts',(0.0117894288146236,-0.0331951640388604,
0.0785799338439174));
#88100=CARTESIAN_POINT('Ctrl Pts',(0.0118810148566372,-0.0330306422010619,
0.0785041489502114));
#88101=CARTESIAN_POINT('Ctrl Pts',(0.0119693903696656,-0.0328657861914644,
0.0784246434667358));
#88102=CARTESIAN_POINT('Ctrl Pts',(0.0117914433282302,-0.0331951640388604,
0.0785801678069704));
#88103=CARTESIAN_POINT('Ctrl Pts',(0.01188303420728,-0.0330306422010619,
0.0785043412644872));
#88104=CARTESIAN_POINT('Ctrl Pts',(0.0119714128318235,-0.0328657861914644,
0.0784247939679032));
#88105=CARTESIAN_POINT('Ctrl Pts',(0.0121271154706225,-0.0331951640388604,
0.0786191523434878));
#88106=CARTESIAN_POINT('Ctrl Pts',(0.0122195123299703,-0.0330306422010619,
0.0785363859946736));
#88107=CARTESIAN_POINT('Ctrl Pts',(0.0123084094166135,-0.0328657861914644,
0.0784498715097611));
#88108=CARTESIAN_POINT('',(0.012136652526609,-0.0331781648281957,0.078610590956646));
#88109=CARTESIAN_POINT('',(0.0121271154706064,-0.0331951640388588,0.078619152343485));
#88110=CARTESIAN_POINT('Origin',(0.000567094400286078,-0.0326412092823903,
0.0668151764484132));
#88111=CARTESIAN_POINT('Ctrl Pts',(0.0121366525247728,-0.033178164828644,
0.0786105909568528));
#88112=CARTESIAN_POINT('Ctrl Pts',(0.012107904979319,-0.0331276811546757,
0.0785786360323269));
#88113=CARTESIAN_POINT('Ctrl Pts',(0.0120796765003694,-0.0330765663497754,
0.0785472581373964));
#88114=CARTESIAN_POINT('Ctrl Pts',(0.0120242335428182,-0.0329730614463344,
0.0784856293391694));
#88115=CARTESIAN_POINT('Ctrl Pts',(0.0119970414659523,-0.0329207133374308,
0.0784554033289843));
#88116=CARTESIAN_POINT('Ctrl Pts',(0.0119703582108274,-0.03286775322894,
0.0784257429892357));
#88117=CARTESIAN_POINT('',(0.0119592793994295,-0.0331951640388701,0.0785996600752367));
#88118=CARTESIAN_POINT('Origin',(0.00812378219310841,-0.0315241814719618,
0.07415));
#88119=CARTESIAN_POINT('',(0.0121366525260512,-0.0332121607144401,0.078610590955059));
#88120=CARTESIAN_POINT('',(0.0121461712749854,-0.0331951640388587,0.0786020092176456));
#88121=CARTESIAN_POINT('Origin',(0.000539138682391462,-0.0326413666972893,
0.0668508777240834));
#88122=CARTESIAN_POINT('Origin',(0.00162613652128707,-0.0326412094582721,
0.0658624320638465));
#88123=CARTESIAN_POINT('Origin',(0.00166458628039381,-0.0326413667783289,
0.0658383954743563));
#88124=CARTESIAN_POINT('Ctrl Pts',(0.0118490708129398,-0.0337436976235975,
0.0785318203636108));
#88125=CARTESIAN_POINT('Ctrl Pts',(0.0118884815693732,-0.0336723290703325,
0.0784983145531811));
#88126=CARTESIAN_POINT('Ctrl Pts',(0.0119272832861533,-0.033601104548885,
0.0784641052879139));
#88127=CARTESIAN_POINT('Ctrl Pts',(0.0120511694816449,-0.0333736987606857,
0.0783548818803893));
#88128=CARTESIAN_POINT('Ctrl Pts',(0.0121685836535868,-0.0331450831799191,
0.0782387291601807));
#88129=CARTESIAN_POINT('Ctrl Pts',(0.0120359753458697,-0.0337436976235975,
0.0783657881511631));
#88130=CARTESIAN_POINT('Ctrl Pts',(0.0120738927834215,-0.0336723290703325,
0.0783306012930381));
#88131=CARTESIAN_POINT('Ctrl Pts',(0.0121111711861542,-0.033601104548885,
0.0782947381121293));
#88132=CARTESIAN_POINT('Ctrl Pts',(0.0122301937416443,-0.0333736987606857,
0.0781802340795834));
#88133=CARTESIAN_POINT('Ctrl Pts',(0.0123424492557671,-0.0331450831799191,
0.0780590885401124));
#88134=CARTESIAN_POINT('Ctrl Pts',(0.012037844391199,-0.0337436976235975,
0.0783641278290386));
#88135=CARTESIAN_POINT('Ctrl Pts',(0.012075746895562,-0.0336723290703325,
0.0783289241604367));
#88136=CARTESIAN_POINT('Ctrl Pts',(0.0121130100651542,-0.033601104548885,
0.0782930444403715));
#88137=CARTESIAN_POINT('Ctrl Pts',(0.0122319839842443,-0.0333736987606857,
0.0781784876015754));
#88138=CARTESIAN_POINT('Ctrl Pts',(0.0123441879117889,-0.0331450831799191,
0.0780572921339118));
#88139=CARTESIAN_POINT('',(0.0120623785749918,-0.0336938721132548,0.0783411315346355));
#88140=CARTESIAN_POINT('',(0.0122312439899657,-0.0333679869945434,0.0781757772650163));
#88141=CARTESIAN_POINT('Ctrl Pts',(0.0120623785749929,-0.033693872113265,
0.0783411315346356));
#88142=CARTESIAN_POINT('Ctrl Pts',(0.012078738527467,-0.0336629187933934,
0.0783257573453283));
#88143=CARTESIAN_POINT('Ctrl Pts',(0.0120950032255789,-0.0336319952301041,
0.0783102922789536));
#88144=CARTESIAN_POINT('Ctrl Pts',(0.0121111711861547,-0.0336011045488951,
0.078294738112129));
#88145=CARTESIAN_POINT('Ctrl Pts',(0.0121517421316042,-0.0335235892595455,
0.0782557073852299));
#88146=CARTESIAN_POINT('Ctrl Pts',(0.0121917759274989,-0.0334458668660371,
0.0782160461494159));
#88147=CARTESIAN_POINT('Ctrl Pts',(0.0122312439901772,-0.0333679869945386,
0.0781757772652327));
#88148=CARTESIAN_POINT('Ctrl Pts',(0.0122312756088197,-0.0333679692459666,
0.0781757459869489));
#88149=CARTESIAN_POINT('Ctrl Pts',(0.0122309477870204,-0.03333918953733,
0.0781754329842461));
#88150=CARTESIAN_POINT('Ctrl Pts',(0.0122306998261648,-0.0333104081058397,
0.0781752007220402));
#88151=CARTESIAN_POINT('Ctrl Pts',(0.0122303678211688,-0.0332532697887149,
0.0781748973252528));
#88152=CARTESIAN_POINT('Ctrl Pts',(0.0122302813836111,-0.0332249169570396,
0.0781748238408584));
#88153=CARTESIAN_POINT('Ctrl Pts',(0.0122302739339486,-0.0331960985434463,
0.0781748261980636));
#88154=CARTESIAN_POINT('Ctrl Pts',(0.0122302738343412,-0.033195631249,0.0781748262571799));
#88155=CARTESIAN_POINT('Ctrl Pts',(0.0122302737564736,-0.0331951640388607,
0.0781748263366275));
#88156=CARTESIAN_POINT('',(0.0121427775317648,-0.0331951640388587,0.0782640978923525));
#88157=CARTESIAN_POINT('',(0.0121865256441295,-0.0331951640388687,0.0782194621144997));
#88158=CARTESIAN_POINT('',(0.011970358200584,-0.0335216366567644,0.0784257429780441));
#88159=CARTESIAN_POINT('Origin',(-3.91172530374529E-5,-0.0326434571528741,
0.0668869750910637));
#88160=CARTESIAN_POINT('',(0.0119694495967205,-0.0336938721132327,0.0784247329999423));
#88161=CARTESIAN_POINT('Origin',(0.0192732533708569,-0.0336938867896295,
0.0865434324267544));
#88162=CARTESIAN_POINT('',(0.0120159140858662,-0.0336938721132537,0.0783829322672988));
#88163=CARTESIAN_POINT('Ctrl Pts',(0.0119587295760685,-0.0335235895815172,
0.0787644532254655));
#88164=CARTESIAN_POINT('Ctrl Pts',(0.0120222566097394,-0.0334144449262748,
0.0787116576244225));
#88165=CARTESIAN_POINT('Ctrl Pts',(0.012084765910891,-0.0333049234473147,
0.078657488946924));
#88166=CARTESIAN_POINT('Ctrl Pts',(0.0121461712749855,-0.0331951640388587,
0.0786020092176541));
#88167=CARTESIAN_POINT('Ctrl Pts',(0.0119622758238219,-0.0335235895815172,
0.0786511898306141));
#88168=CARTESIAN_POINT('Ctrl Pts',(0.0120242435638676,-0.0334144449262748,
0.0785983454084889));
#88169=CARTESIAN_POINT('Ctrl Pts',(0.0120851907713478,-0.0333049234473147,
0.0785441600676514));
#88170=CARTESIAN_POINT('Ctrl Pts',(0.0121450332372326,-0.0331951640388587,
0.0784886960350297));
#88171=CARTESIAN_POINT('Ctrl Pts',(0.0119658220715754,-0.0335235895815172,
0.0785379264357627));
#88172=CARTESIAN_POINT('Ctrl Pts',(0.0120262305179959,-0.0334144449262748,
0.0784850331925552));
#88173=CARTESIAN_POINT('Ctrl Pts',(0.0120856156318045,-0.0333049234473147,
0.0784308311883788));
#88174=CARTESIAN_POINT('Ctrl Pts',(0.0121438951994796,-0.0331951640388587,
0.0783753828524054));
#88175=CARTESIAN_POINT('Ctrl Pts',(0.0119693683193289,-0.0335235895815172,
0.0784246630409113));
#88176=CARTESIAN_POINT('Ctrl Pts',(0.0120282174721241,-0.0334144449262748,
0.0783717209766216));
#88177=CARTESIAN_POINT('Ctrl Pts',(0.0120860404922612,-0.0333049234473147,
0.0783175023091062));
#88178=CARTESIAN_POINT('Ctrl Pts',(0.0121427571617266,-0.0331951640388587,
0.078262069669781));
#88179=CARTESIAN_POINT('',(0.0121444744033851,-0.0331951640388687,0.078433053555009));
#88180=CARTESIAN_POINT('Ctrl Pts',(0.0121366525239504,-0.0332121607145951,
0.0786105909527245));
#88181=CARTESIAN_POINT('Ctrl Pts',(0.0121079533482372,-0.033262544410902,
0.0785786897765133));
#88182=CARTESIAN_POINT('Ctrl Pts',(0.0120797487043566,-0.0333135300745334,
0.0785473383076279));
#88183=CARTESIAN_POINT('Ctrl Pts',(0.0120243060916295,-0.0334167203140529,
0.078485709897952));
#88184=CARTESIAN_POINT('Ctrl Pts',(0.0119970895962799,-0.03346888475872,
0.0784554568264812));
#88185=CARTESIAN_POINT('Ctrl Pts',(0.0119703582002306,-0.0335216366562256,
0.0784257429774055));
#88186=CARTESIAN_POINT('Ctrl Pts',(0.0120613801103767,-0.0336938721132391,
0.0783410787777918));
#88187=CARTESIAN_POINT('Ctrl Pts',(0.0120859118852105,-0.0336474569764958,
0.0783180307105484));
#88188=CARTESIAN_POINT('Ctrl Pts',(0.012110172172384,-0.033601104548885,
0.0782946970471753));
#88189=CARTESIAN_POINT('Ctrl Pts',(0.0121715936417173,-0.0334837508592656,
0.0782356215762601));
#88190=CARTESIAN_POINT('Ctrl Pts',(0.0122312376105811,-0.0333660264659097,
0.0781747520014537));
#88191=CARTESIAN_POINT('Ctrl Pts',(0.0120623785749768,-0.0336938721132391,
0.0783411315346495));
#88192=CARTESIAN_POINT('Ctrl Pts',(0.012086910658614,-0.0336474569764958,
0.0783180776230615));
#88193=CARTESIAN_POINT('Ctrl Pts',(0.0121111711861542,-0.033601104548885,
0.0782947381121293));
#88194=CARTESIAN_POINT('Ctrl Pts',(0.0121725932640411,-0.0334837508592656,
0.0782356478365389));
#88195=CARTESIAN_POINT('Ctrl Pts',(0.0122322374024979,-0.0333660264659097,
0.0781747634455257));
#88196=CARTESIAN_POINT('Ctrl Pts',(0.012401860950161,-0.0336938721132391,
0.078359069099365));
#88197=CARTESIAN_POINT('Ctrl Pts',(0.0124264980283168,-0.0336474569764958,
0.0783340280847828));
#88198=CARTESIAN_POINT('Ctrl Pts',(0.0124508402816319,-0.033601104548885,
0.0783087003779206));
#88199=CARTESIAN_POINT('Ctrl Pts',(0.0125124692703907,-0.0334837508592656,
0.0782445764473504));
#88200=CARTESIAN_POINT('Ctrl Pts',(0.012572171071226,-0.0333660264659097,
0.0781786544805695));
#88201=CARTESIAN_POINT('',(0.0124088168679248,-0.0336769361243753,0.0783498187860456));
#88202=CARTESIAN_POINT('',(0.0123998362043608,-0.0336938721132327,0.0783589621158728));
#88203=CARTESIAN_POINT('Ctrl Pts',(0.0124088168679248,-0.0336769361243754,
0.0783498187860455));
#88204=CARTESIAN_POINT('Ctrl Pts',(0.0124073216062175,-0.0336797586670156,
0.0783513443871703));
#88205=CARTESIAN_POINT('Ctrl Pts',(0.0124058255863224,-0.0336825812713104,
0.0783528691320589));
#88206=CARTESIAN_POINT('Ctrl Pts',(0.0124028320387384,-0.0336882265876415,
0.0783559169013605));
#88207=CARTESIAN_POINT('Ctrl Pts',(0.0124013345110642,-0.0336910492997076,
0.078357439925808));
#88208=CARTESIAN_POINT('Ctrl Pts',(0.0123998362043744,-0.0336938721132379,
0.0783589621158764));
#88209=CARTESIAN_POINT('Ctrl Pts',(0.0124088168679248,-0.0336769361243754,
0.0783498187860455));
#88210=CARTESIAN_POINT('Ctrl Pts',(0.0123788824302282,-0.0336278994593125,
0.0783204796503493));
#88211=CARTESIAN_POINT('Ctrl Pts',(0.0123485218101857,-0.0335767852487005,
0.0782907228077369));
#88212=CARTESIAN_POINT('Ctrl Pts',(0.0122890250589367,-0.033473317179916,
0.0782324092601074));
#88213=CARTESIAN_POINT('Ctrl Pts',(0.0122598534681551,-0.033420963132189,
0.0782038178006946));
#88214=CARTESIAN_POINT('Ctrl Pts',(0.0122312439848548,-0.0333679869844682,
0.0781757772702107));
#88215=CARTESIAN_POINT('',(0.0122311073896863,-0.0336938721132538,0.0783500468252642));
#88216=CARTESIAN_POINT('Origin',(0.00812378219310841,-0.0315241814719618,
0.07415));
#88217=CARTESIAN_POINT('',(0.0124088168670061,-0.0337108120655666,0.078349818785145));
#88218=CARTESIAN_POINT('',(0.012417777980685,-0.0336938721132327,0.0783406562942192));
#88219=CARTESIAN_POINT('Origin',(0.00150638244369434,-0.0345562526942704,
0.0660993020739212));
#88220=CARTESIAN_POINT('Ctrl Pts',(0.012417777980689,-0.033693872113238,
0.0783406562942328));
#88221=CARTESIAN_POINT('Ctrl Pts',(0.0124162861899165,-0.0336910492985901,
0.0783421848718215));
#88222=CARTESIAN_POINT('Ctrl Pts',(0.0124147935501724,-0.0336882265870826,
0.0783437126864011));
#88223=CARTESIAN_POINT('Ctrl Pts',(0.0124118065200469,-0.0336825812713082,
0.0783467668429596));
#88224=CARTESIAN_POINT('Ctrl Pts',(0.0124103121296314,-0.0336797586670143,
0.0783482931849215));
#88225=CARTESIAN_POINT('Ctrl Pts',(0.0124088168679246,-0.033676936124375,
0.0783498187860458));
#88226=CARTESIAN_POINT('Origin',(-5.81985527356521E-5,-0.034556252294033,
0.0676956299121895));
#88227=CARTESIAN_POINT('Ctrl Pts',(0.0121168194200936,-0.034243627687391,
0.0782892968852102));
#88228=CARTESIAN_POINT('Ctrl Pts',(0.0122729355757268,-0.0339430054201809,
0.0781386970035239));
#88229=CARTESIAN_POINT('Ctrl Pts',(0.0124172644215758,-0.0336441434784052,
0.077976765651805));
#88230=CARTESIAN_POINT('Ctrl Pts',(0.0122929314838561,-0.034243627687391,
0.0781118580478681));
#88231=CARTESIAN_POINT('Ctrl Pts',(0.0124423554234164,-0.0339430054201809,
0.0779546159901993));
#88232=CARTESIAN_POINT('Ctrl Pts',(0.0125795107491663,-0.0336441434784052,
0.0777865654173588));
#88233=CARTESIAN_POINT('Ctrl Pts',(0.0122946926044938,-0.034243627687391,
0.0781100836594947));
#88234=CARTESIAN_POINT('Ctrl Pts',(0.0124440496218933,-0.0339430054201809,
0.0779527751800661));
#88235=CARTESIAN_POINT('Ctrl Pts',(0.0125811332124422,-0.0336441434784052,
0.0777846634150143));
#88236=CARTESIAN_POINT('',(0.0123177699811834,-0.0341934961088741,0.0780855547809017));
#88237=CARTESIAN_POINT('',(0.0124759194944158,-0.0338664212864897,0.077909923657779));
#88238=CARTESIAN_POINT('Origin',(0.00046885273275643,-0.0345610720403415,
0.0662679279544497));
#88239=CARTESIAN_POINT('Origin',(0.0207742693606469,-0.0336938005072936,
0.0850790319675171));
#88240=CARTESIAN_POINT('',(0.0123931733065714,-0.0336938721132327,0.078003624854638));
#88241=CARTESIAN_POINT('',(0.0124340323883481,-0.0336938721132427,0.0779563301885937));
#88242=CARTESIAN_POINT('',(0.012231243984851,-0.0340203938281605,0.0781757772702145));
#88243=CARTESIAN_POINT('Origin',(0.000857110895691337,-0.0345589643242984,
0.0659836880327022));
#88244=CARTESIAN_POINT('',(0.0122302737564741,-0.034193496108874,0.078174826336627));
#88245=CARTESIAN_POINT('Origin',(0.0201000588175834,-0.0341934220717647,
0.0858881071786148));
#88246=CARTESIAN_POINT('',(0.0122740218688388,-0.0341934961088841,0.0781301905587744));
#88247=CARTESIAN_POINT('Ctrl Pts',(0.0122409041083963,-0.0340223579322396,
0.0785145511951107));
#88248=CARTESIAN_POINT('Ctrl Pts',(0.0123011026526042,-0.0339125849573575,
0.0784577653459942));
#88249=CARTESIAN_POINT('Ctrl Pts',(0.0123600835608676,-0.0338030433565231,
0.0783997734296534));
#88250=CARTESIAN_POINT('Ctrl Pts',(0.0124177779806857,-0.0336938721132327,
0.0783406562942283));
#88251=CARTESIAN_POINT('Ctrl Pts',(0.0122373315416637,-0.0340223579322396,
0.0784012885949387));
#88252=CARTESIAN_POINT('Ctrl Pts',(0.012295967899214,-0.0339125849573575,
0.078344552020835));
#88253=CARTESIAN_POINT('Ctrl Pts',(0.0123533887384284,-0.0338030433565231,
0.0782866416785159));
#88254=CARTESIAN_POINT('Ctrl Pts',(0.0124095271926243,-0.0336938721132327,
0.0782276381349478));
#88255=CARTESIAN_POINT('Ctrl Pts',(0.0122337589749311,-0.0340223579322396,
0.0782880259947666));
#88256=CARTESIAN_POINT('Ctrl Pts',(0.0122908331458238,-0.0339125849573575,
0.0782313386956758));
#88257=CARTESIAN_POINT('Ctrl Pts',(0.0123466939159893,-0.0338030433565231,
0.0781735099273784));
#88258=CARTESIAN_POINT('Ctrl Pts',(0.0124012764045629,-0.0336938721132327,
0.0781146199756672));
#88259=CARTESIAN_POINT('Ctrl Pts',(0.0122301864081985,-0.0340223579322396,
0.0781747633945945));
#88260=CARTESIAN_POINT('Ctrl Pts',(0.0122856983924335,-0.0339125849573575,
0.0781181253705167));
#88261=CARTESIAN_POINT('Ctrl Pts',(0.0123399990935502,-0.0338030433565231,
0.0780603781762409));
#88262=CARTESIAN_POINT('Ctrl Pts',(0.0123930256165015,-0.0336938721132327,
0.0780016018163867));
#88263=CARTESIAN_POINT('',(0.0124054756436382,-0.0336938721132427,0.0781721405744386));
#88264=CARTESIAN_POINT('Ctrl Pts',(0.012408816864427,-0.0337108120662662,
0.0783498187826173));
#88265=CARTESIAN_POINT('Ctrl Pts',(0.0123781079805278,-0.0337611408993578,
0.0783197206020225));
#88266=CARTESIAN_POINT('Ctrl Pts',(0.0123479594656285,-0.0338121088779845,
0.078290171646447));
#88267=CARTESIAN_POINT('Ctrl Pts',(0.0122887557088512,-0.0339153382773235,
0.0782321452665488));
#88268=CARTESIAN_POINT('Ctrl Pts',(0.0122597255139114,-0.0339675558473122,
0.0782036923910593));
#88269=CARTESIAN_POINT('Ctrl Pts',(0.0122312439848262,-0.0340203938281304,
0.0781757772701829));
#88270=CARTESIAN_POINT('Ctrl Pts',(0.0123157419360611,-0.0341934961088741,
0.0780855751491577));
#88271=CARTESIAN_POINT('Ctrl Pts',(0.0123971068517772,-0.0340287516182428,
0.0779989096839477));
#88272=CARTESIAN_POINT('Ctrl Pts',(0.0124748202933024,-0.0338644633275951,
0.0779089553990256));
#88273=CARTESIAN_POINT('Ctrl Pts',(0.0123177699811834,-0.0341934961088741,
0.0780855547809017));
#88274=CARTESIAN_POINT('Ctrl Pts',(0.0123991344758018,-0.0340287516182428,
0.0779988473874565));
#88275=CARTESIAN_POINT('Ctrl Pts',(0.0124768457636635,-0.0338644633275951,
0.0779088512275303));
#88276=CARTESIAN_POINT('Ctrl Pts',(0.0126556813064923,-0.0341934961088741,
0.078082161037681));
#88277=CARTESIAN_POINT('Ctrl Pts',(0.0127369756381432,-0.0340287516182428,
0.0779884675937955));
#88278=CARTESIAN_POINT('Ctrl Pts',(0.0128143280842256,-0.0338644633275951,
0.0778914942527643));
#88279=CARTESIAN_POINT('',(0.0126640701331909,-0.0341764758832446,0.0780724718497314));
#88280=CARTESIAN_POINT('',(0.0126556813064761,-0.034193496108874,0.0780821610376811));
#88281=CARTESIAN_POINT('Origin',(0.000469360212365722,-0.0345621026190861,
0.0668604076600941));
#88282=CARTESIAN_POINT('Ctrl Pts',(0.0126640701314842,-0.0341764758837558,
0.078072471850373));
#88283=CARTESIAN_POINT('Ctrl Pts',(0.0126315886167829,-0.0341260050040584,
0.0780444102502477));
#88284=CARTESIAN_POINT('Ctrl Pts',(0.012599671682457,-0.0340749269148397,
0.0780168364558454));
#88285=CARTESIAN_POINT('Ctrl Pts',(0.0125369423585455,-0.0339715436307112,
0.0779626429697402));
#88286=CARTESIAN_POINT('Ctrl Pts',(0.0125061537708994,-0.0339192778237382,
0.0779360438332403));
#88287=CARTESIAN_POINT('Ctrl Pts',(0.0124759194946897,-0.0338664212854664,
0.0779099236595325));
#88288=CARTESIAN_POINT('',(0.0124867256438398,-0.0341934961088841,0.0780838579093015));
#88289=CARTESIAN_POINT('Origin',(0.00812378219310841,-0.0315241814719618,
0.07415));
#88290=CARTESIAN_POINT('',(0.0126640701331818,-0.0342105180190352,0.0780724718486117));
#88291=CARTESIAN_POINT('',(0.012672438246751,-0.0341934961088739,0.0780627647649283));
#88292=CARTESIAN_POINT('Origin',(0.000435969997987811,-0.0345621721966557,
0.0668910575975215));
#88293=CARTESIAN_POINT('Origin',(-0.000200204842937758,-0.0345621029191649,
0.0676354332226913));
#88294=CARTESIAN_POINT('Origin',(-0.000174728215152024,-0.034562172372312,
0.0675979463160218));
#88295=CARTESIAN_POINT('Ctrl Pts',(0.0123921926821259,-0.0346945769586966,
0.0780047599341273));
#88296=CARTESIAN_POINT('Ctrl Pts',(0.0124729321723079,-0.0345275153362944,
0.0779153563674564));
#88297=CARTESIAN_POINT('Ctrl Pts',(0.0125508808859761,-0.0343603235965185,
0.0778233904937933));
#88298=CARTESIAN_POINT('Ctrl Pts',(0.0126258123279797,-0.034193496108874,
0.0777291377337591));
#88299=CARTESIAN_POINT('Ctrl Pts',(0.0124469983329902,-0.0346945769586966,
0.0779413220191414));
#88300=CARTESIAN_POINT('Ctrl Pts',(0.0125264090906437,-0.0345275153362944,
0.0778507705261702));
#88301=CARTESIAN_POINT('Ctrl Pts',(0.0126029926268795,-0.0343603235965185,
0.0777576982167093));
#88302=CARTESIAN_POINT('Ctrl Pts',(0.0126765265327713,-0.034193496108874,
0.0776623837237165));
#88303=CARTESIAN_POINT('Ctrl Pts',(0.0125018039838545,-0.0346945769586966,
0.0778778841041562));
#88304=CARTESIAN_POINT('Ctrl Pts',(0.0125798860089796,-0.0345275153362944,
0.0777861846848856));
#88305=CARTESIAN_POINT('Ctrl Pts',(0.012655104367783,-0.0343603235965185,
0.0776920059396272));
#88306=CARTESIAN_POINT('Ctrl Pts',(0.0127272407375627,-0.034193496108874,
0.0775956297136759));
#88307=CARTESIAN_POINT('Ctrl Pts',(0.0125566096347188,-0.0346945769586966,
0.0778144461891698));
#88308=CARTESIAN_POINT('Ctrl Pts',(0.0126333629273152,-0.0345275153362944,
0.077721598843598));
#88309=CARTESIAN_POINT('Ctrl Pts',(0.0127072161086863,-0.0343603235965185,
0.0776263136625413));
#88310=CARTESIAN_POINT('Ctrl Pts',(0.0127779549423545,-0.034193496108874,
0.0775288757036314));
#88311=CARTESIAN_POINT('',(0.0125566096336416,-0.0346945769586966,0.0778144461904163));
#88312=CARTESIAN_POINT('',(0.0127034191051059,-0.0343667727836579,0.0776292313455091));
#88313=CARTESIAN_POINT('Origin',(-0.000518188304912433,-0.0345626474181758,
0.067243405364632));
#88314=CARTESIAN_POINT('Origin',(0.0215039495486088,-0.034193477102429,
0.0843151360524152));
#88315=CARTESIAN_POINT('',(0.0126267197451524,-0.0341934961088739,0.0777279433201761));
#88316=CARTESIAN_POINT('',(0.0126645285442121,-0.034193496108884,0.0776781764163802));
#88317=CARTESIAN_POINT('',(0.0124759194935752,-0.0345211942962607,0.0779099236585232));
#88318=CARTESIAN_POINT('Origin',(-0.000201345948739516,-0.0345625596121062,
0.0668817433285368));
#88319=CARTESIAN_POINT('',(0.0124748914701046,-0.0346945769586886,0.0779090355225294));
#88320=CARTESIAN_POINT('Origin',(0.0208468542829956,-0.0346945685853896,
0.085141791143449));
#88321=CARTESIAN_POINT('',(0.0125157505518831,-0.0346945769587026,0.0778617408564829));
#88322=CARTESIAN_POINT('Ctrl Pts',(0.0125068330028904,-0.0345231616327841,
0.0782474218234103));
#88323=CARTESIAN_POINT('Ctrl Pts',(0.0125633101940176,-0.0344132092796987,
0.0781870076388393));
#88324=CARTESIAN_POINT('Ctrl Pts',(0.0126185348514276,-0.0343032738558979,
0.0781254283852128));
#88325=CARTESIAN_POINT('Ctrl Pts',(0.0126724382467524,-0.0341934961088739,
0.0780627647649376));
#88326=CARTESIAN_POINT('Ctrl Pts',(0.0124961556683675,-0.0345231616327841,
0.0781346072380655));
#88327=CARTESIAN_POINT('Ctrl Pts',(0.012551077869266,-0.0344132092796987,
0.0780743402255184));
#88328=CARTESIAN_POINT('Ctrl Pts',(0.0126047506608148,-0.0343032738558979,
0.0780129403000687));
#88329=CARTESIAN_POINT('Ctrl Pts',(0.0126571072968806,-0.0341934961088739,
0.0779504878834568));
#88330=CARTESIAN_POINT('Ctrl Pts',(0.0124854783338447,-0.0345231616327841,
0.0780217926527206));
#88331=CARTESIAN_POINT('Ctrl Pts',(0.0125388455445144,-0.0344132092796988,
0.0779616728121975));
#88332=CARTESIAN_POINT('Ctrl Pts',(0.012590966470202,-0.0343032738558979,
0.0779004522149246));
#88333=CARTESIAN_POINT('Ctrl Pts',(0.0126417763470089,-0.0341934961088739,
0.0778382110019759));
#88334=CARTESIAN_POINT('Ctrl Pts',(0.0124748009993219,-0.0345231616327841,
0.0779089780673758));
#88335=CARTESIAN_POINT('Ctrl Pts',(0.0125266132197628,-0.0344132092796988,
0.0778490053988766));
#88336=CARTESIAN_POINT('Ctrl Pts',(0.0125771822795893,-0.0343032738558979,
0.0777879641297806));
#88337=CARTESIAN_POINT('Ctrl Pts',(0.0126264453971372,-0.0341934961088739,
0.0777259341204951));
#88338=CARTESIAN_POINT('',(0.0126495789959617,-0.0341934961088839,0.0778953540425622));
#88339=CARTESIAN_POINT('Ctrl Pts',(0.0126640701305619,-0.0342105180195359,
0.0780724718463475));
#88340=CARTESIAN_POINT('Ctrl Pts',(0.0126315521093654,-0.034261055624039,
0.0780443786891735));
#88341=CARTESIAN_POINT('Ctrl Pts',(0.0125996176072439,-0.0343122189868302,
0.0780167896491778));
#88342=CARTESIAN_POINT('Ctrl Pts',(0.0125368876477865,-0.0344158119695079,
0.0779625956193533));
#88343=CARTESIAN_POINT('Ctrl Pts',(0.0125061178476239,-0.0344681990449959,
0.0779360127954183));
#88344=CARTESIAN_POINT('Ctrl Pts',(0.0124759194935518,-0.0345211942962354,
0.0779099236584989));
#88345=CARTESIAN_POINT('Ctrl Pts',(0.0125545873649794,-0.0346945769586931,
0.0778145938243097));
#88346=CARTESIAN_POINT('Ctrl Pts',(0.0126303502492178,-0.0345296777079064,
0.0777229900626341));
#88347=CARTESIAN_POINT('Ctrl Pts',(0.0127022623273767,-0.0343648066255586,
0.0776283332256064));
#88348=CARTESIAN_POINT('Ctrl Pts',(0.0125566096336358,-0.0346945769586931,
0.0778144461904233));
#88349=CARTESIAN_POINT('Ctrl Pts',(0.0126323694656481,-0.0345296777079064,
0.0777228006197742));
#88350=CARTESIAN_POINT('Ctrl Pts',(0.0127042767661856,-0.0343648066255586,
0.0776281021356496));
#88351=CARTESIAN_POINT('Ctrl Pts',(0.0128936410732322,-0.0346945769586931,
0.0777898415163088));
#88352=CARTESIAN_POINT('Ctrl Pts',(0.0129688922210175,-0.0345296777079064,
0.0776912280591307));
#88353=CARTESIAN_POINT('Ctrl Pts',(0.0130400032828396,-0.0343648066255586,
0.0775895886668355));
#88354=CARTESIAN_POINT('',(0.0129014049576017,-0.0346775396665031,0.0777796447090279));
#88355=CARTESIAN_POINT('',(0.0128936410732186,-0.0346945769586886,0.0777898415163072));
#88356=CARTESIAN_POINT('Origin',(-0.000409778919642414,-0.0345626618041964,
0.0678586927481973));
#88357=CARTESIAN_POINT('Ctrl Pts',(0.0129014049558933,-0.0346775396670096,
0.0777796447096775));
#88358=CARTESIAN_POINT('Ctrl Pts',(0.0128671986149924,-0.034626974993105,
0.0777536575622933));
#88359=CARTESIAN_POINT('Ctrl Pts',(0.0128336001753502,-0.0345757902896753,
0.0777281322931075));
#88360=CARTESIAN_POINT('Ctrl Pts',(0.0127675915318585,-0.0344721681087866,
0.0776779843517497));
#88361=CARTESIAN_POINT('Ctrl Pts',(0.0127352072103651,-0.0344197714287363,
0.0776533813357851));
#88362=CARTESIAN_POINT('Ctrl Pts',(0.0127034191049817,-0.03436677278343,
0.0776292313461726));
#88363=CARTESIAN_POINT('',(0.0127251253534401,-0.0346945769587026,0.0778021438533718));
#88364=CARTESIAN_POINT('Origin',(0.00812378219310841,-0.0315241814719618,
0.07415));
#88365=CARTESIAN_POINT('',(0.0129014049571081,-0.0347116136489595,0.0777796447077254));
#88366=CARTESIAN_POINT('',(0.0129091470454567,-0.0346945769586885,0.0777694313406826));
#88367=CARTESIAN_POINT('Origin',(-0.000435675480596656,-0.0345626702815683,
0.0678958740026416));
#88368=CARTESIAN_POINT('Origin',(-0.000225010134284166,-0.0345626620959895,
0.0676154845536354));
#88369=CARTESIAN_POINT('Origin',(-0.000196131731250116,-0.0345626704986924,
0.0675805685326128));
#88370=CARTESIAN_POINT('Ctrl Pts',(0.0126026337480803,-0.0352450361874068,
0.0777581368286348));
#88371=CARTESIAN_POINT('Ctrl Pts',(0.0127387168615924,-0.0349452760959492,
0.077589214170347));
#88372=CARTESIAN_POINT('Ctrl Pts',(0.0128616894315066,-0.0346444289841739,
0.0774105210666332));
#88373=CARTESIAN_POINT('Ctrl Pts',(0.0126041738130506,-0.0352450361874068,
0.0777561358726414));
#88374=CARTESIAN_POINT('Ctrl Pts',(0.012740181459269,-0.0349452760959492,
0.0775871551298502));
#88375=CARTESIAN_POINT('Ctrl Pts',(0.0128630744011217,-0.0346444289841739,
0.0774084097911503));
#88376=CARTESIAN_POINT('Ctrl Pts',(0.0127566554932788,-0.0352450361874068,
0.0775580214178564));
#88377=CARTESIAN_POINT('Ctrl Pts',(0.0128851911302251,-0.0349452760959492,
0.0773832897341268));
#88378=CARTESIAN_POINT('Ctrl Pts',(0.013000200105595,-0.0346444289841739,
0.0771993726146177));
#88379=CARTESIAN_POINT('Ctrl Pts',(0.0127581803100811,-0.0352450361874068,
0.0775560402733086));
#88380=CARTESIAN_POINT('Ctrl Pts',(0.0128866412269346,-0.0349452760959492,
0.0773812510801696));
#88381=CARTESIAN_POINT('Ctrl Pts',(0.0130015713626397,-0.0346444289841739,
0.0771972822428523));
#88382=CARTESIAN_POINT('',(0.0127779378515802,-0.0351951634053346,0.0775289032849739));
#88383=CARTESIAN_POINT('',(0.0129128449811174,-0.0348678972925388,0.0773348080966532));
#88384=CARTESIAN_POINT('Origin',(-0.00126749047167203,-0.0345636767889031,
0.0684113137140681));
#88385=CARTESIAN_POINT('Origin',(0.022113868460618,-0.0346946199341121,
0.083453644271531));
#88386=CARTESIAN_POINT('',(0.0128424951359957,-0.0346945769330289,0.0774381412927178));
#88387=CARTESIAN_POINT('',(0.0128771044433858,-0.0346945769458128,0.077386098551345));
#88388=CARTESIAN_POINT('',(0.0127034191046605,-0.0350221583435276,0.0776292313459082));
#88389=CARTESIAN_POINT('Origin',(-0.00103679855261937,-0.0345628458713947,
0.0679895025826022));
#88390=CARTESIAN_POINT('',(0.0127024323802842,-0.0351951360298763,0.0776284855123135));
#88391=CARTESIAN_POINT('Origin',(0.0214765190564826,-0.0351951838366868,
0.0842943123085817));
#88392=CARTESIAN_POINT('',(0.0127779549414438,-0.0351951371328746,0.0775288757050221));
#88393=CARTESIAN_POINT('Ctrl Pts',(0.0127554639090662,-0.0350241211494343,
0.0779641217183193));
#88394=CARTESIAN_POINT('Ctrl Pts',(0.0128080018718853,-0.0349144232818962,
0.0779003222017455));
#88395=CARTESIAN_POINT('Ctrl Pts',(0.0128592524996112,-0.0348045283579412,
0.0778353985008526));
#88396=CARTESIAN_POINT('Ctrl Pts',(0.0129091470521623,-0.0346945769439157,
0.0777694313318289));
#88397=CARTESIAN_POINT('Ctrl Pts',(0.0127377239355663,-0.0350241211494343,
0.0778522001603256));
#88398=CARTESIAN_POINT('Ctrl Pts',(0.0127887202248136,-0.0349144232818962,
0.077788645004613));
#88399=CARTESIAN_POINT('Ctrl Pts',(0.0128384333073155,-0.0348045283579412,
0.0777239976783375));
#88400=CARTESIAN_POINT('Ctrl Pts',(0.0128867964255634,-0.0346945769439157,
0.0776583386169725));
#88401=CARTESIAN_POINT('Ctrl Pts',(0.0127199839620663,-0.0350241211494343,
0.0777402786023319));
#88402=CARTESIAN_POINT('Ctrl Pts',(0.0127694385777419,-0.0349144232818962,
0.0776769678074806));
#88403=CARTESIAN_POINT('Ctrl Pts',(0.0128176141150197,-0.0348045283579412,
0.0776125968558225));
#88404=CARTESIAN_POINT('Ctrl Pts',(0.0128644457989645,-0.0346945769439157,
0.0775472459021162));
#88405=CARTESIAN_POINT('Ctrl Pts',(0.0127022439885664,-0.0350241211494343,
0.0776283570443381));
#88406=CARTESIAN_POINT('Ctrl Pts',(0.0127501569306702,-0.0349144232818962,
0.0775652906103481));
#88407=CARTESIAN_POINT('Ctrl Pts',(0.012796794922724,-0.0348045283579412,
0.0775011960333074));
#88408=CARTESIAN_POINT('Ctrl Pts',(0.0128420951723656,-0.0346945769439157,
0.0774361531872598));
#88409=CARTESIAN_POINT('',(0.0128758210906322,-0.0346945769458128,0.0776037863169928));
#88410=CARTESIAN_POINT('Ctrl Pts',(0.012901404954484,-0.0347116136492762,
0.0777796447057305));
#88411=CARTESIAN_POINT('Ctrl Pts',(0.0128672122053332,-0.0347621546531334,
0.0777536678680586));
#88412=CARTESIAN_POINT('Ctrl Pts',(0.012833620657109,-0.0348133084095068,
0.0777281477733883));
#88413=CARTESIAN_POINT('Ctrl Pts',(0.0127676119278375,-0.0349168561544567,
0.0776779997716103));
#88414=CARTESIAN_POINT('Ctrl Pts',(0.0127352209292868,-0.034969208901592,
0.0776533917558094));
#88415=CARTESIAN_POINT('Ctrl Pts',(0.0127034191046435,-0.0350221583435,
0.0776292313458702));
#88416=CARTESIAN_POINT('Ctrl Pts',(0.0127765053750515,-0.0351951371254975,
0.0775290736373207));
#88417=CARTESIAN_POINT('Ctrl Pts',(0.0128463656024019,-0.0350307338980971,
0.0774328815047496));
#88418=CARTESIAN_POINT('Ctrl Pts',(0.0129121904099651,-0.0348659306897824,
0.0773338841692132));
#88419=CARTESIAN_POINT('Ctrl Pts',(0.0127779549413452,-0.0351951371254975,
0.0775288757049602));
#88420=CARTESIAN_POINT('Ctrl Pts',(0.0128478110765682,-0.0350307338980971,
0.0774326536035154));
#88421=CARTESIAN_POINT('Ctrl Pts',(0.0129136305568548,-0.0348659306897824,
0.0773336264938456));
#88422=CARTESIAN_POINT('Ctrl Pts',(0.0130209037629744,-0.0351951371254975,
0.0774957020350415));
#88423=CARTESIAN_POINT('Ctrl Pts',(0.0130900740533857,-0.0350307338980971,
0.0773944571191407));
#88424=CARTESIAN_POINT('Ctrl Pts',(0.0131550006765698,-0.0348659306897824,
0.0772904398336865));
#88425=CARTESIAN_POINT('Origin',(0.0173412084800945,-0.0308609197410323,
0.0802797450395314));
#88426=CARTESIAN_POINT('',(0.0128838751498071,-0.0351951371254975,0.0775144127328426));
#88427=CARTESIAN_POINT('Origin',(0.00724034756344459,-0.0351840467441114,
0.0737325207725142));
#88428=CARTESIAN_POINT('Origin',(0.0185052740279725,-0.0352322612843293,
0.0800994752299718));
#88429=CARTESIAN_POINT('',(0.0130397881752884,-0.0351951142564687,0.0771350795243343));
#88430=CARTESIAN_POINT('',(0.0131021944076713,-0.0351951372916787,0.0770271360450789));
#88431=CARTESIAN_POINT('Origin',(0.00811441848004271,-0.0352875113587952,
0.0738095910710146));
#88432=CARTESIAN_POINT('Origin',(0.00319514827069109,-0.0298325076522705,
0.0798071863977184));
#88433=CARTESIAN_POINT('Origin',(0.0132682144054627,-0.0338732916933875,
0.0807668555657059));
#88434=CARTESIAN_POINT('Origin',(0.00812378219310841,-0.0315241814719618,
0.07415));
#88435=CARTESIAN_POINT('',(0.0112297421631025,-0.032711433838004,0.0792835185442903));
#88436=CARTESIAN_POINT('',(0.0112407003659563,-0.0326943950436593,0.0792768724485572));
#88437=CARTESIAN_POINT('Origin',(0.00255258075290883,-0.032639568195616,
0.065126507472656));
#88438=CARTESIAN_POINT('',(0.0112297421631267,-0.0326773559991214,0.0792835185443304));
#88439=CARTESIAN_POINT('Origin',(0.00267690876419085,-0.0326395671481778,
0.0650503754881189));
#88440=CARTESIAN_POINT('',(0.0112187697908064,-0.0326943950436594,0.0792901412208319));
#88441=CARTESIAN_POINT('Origin',(0.0025909384096225,-0.032639567029855,
0.0651023909603269));
#88442=CARTESIAN_POINT('Origin',(0.00271607179587666,-0.0326395685042469,
0.0650275905864274));
#88443=CARTESIAN_POINT('Origin',(0.00812378219310841,-0.0315241814719618,
0.07415));
#88444=CARTESIAN_POINT('',(0.0109012769642797,-0.0322104233323771,0.0794684135584242));
#88445=CARTESIAN_POINT('',(0.0109126308553288,-0.0321934096636183,0.0794624686483067));
#88446=CARTESIAN_POINT('Origin',(0.00374745183614647,-0.0326387245399829,
0.0645417703628711));
#88447=CARTESIAN_POINT('',(0.0109012769641094,-0.032176398030833,0.079468413558098));
#88448=CARTESIAN_POINT('Origin',(0.00270254459298124,-0.0326386235886941,
0.0650945863296164));
#88449=CARTESIAN_POINT('',(0.010889910402055,-0.0321934096636184,0.0794743342054824));
#88450=CARTESIAN_POINT('Origin',(0.0037901657731102,-0.0326386231182652,
0.0645265867379557));
#88451=CARTESIAN_POINT('Origin',(0.00273941365981018,-0.0326387249493187,
0.0650682106328434));
#88452=CARTESIAN_POINT('Ctrl Pts',(0.0103460098434445,-0.0321934096636941,
0.0794546998044557));
#88453=CARTESIAN_POINT('Ctrl Pts',(0.0104409614437598,-0.0320508460845056,
0.0794149229877757));
#88454=CARTESIAN_POINT('Ctrl Pts',(0.0105347727256777,-0.0319086045664529,
0.0793726250008024));
#88455=CARTESIAN_POINT('Ctrl Pts',(0.0106272491948647,-0.0317669892870077,
0.0793279135477917));
#88456=CARTESIAN_POINT('Ctrl Pts',(0.0104226231303532,-0.0321934096636941,
0.0794206287478709));
#88457=CARTESIAN_POINT('Ctrl Pts',(0.0105169648749808,-0.0320508460845056,
0.0793794805898398));
#88458=CARTESIAN_POINT('Ctrl Pts',(0.010610129915808,-0.0319086045664529,
0.0793358286811301));
#88459=CARTESIAN_POINT('Ctrl Pts',(0.0107019253899721,-0.0317669892870077,
0.0792897835266752));
#88460=CARTESIAN_POINT('Ctrl Pts',(0.0104992364172618,-0.0321934096636941,
0.0793865576912862));
#88461=CARTESIAN_POINT('Ctrl Pts',(0.0105929683062018,-0.0320508460845056,
0.0793440381919037));
#88462=CARTESIAN_POINT('Ctrl Pts',(0.0106854871059383,-0.0319086045664529,
0.0792990323614578));
#88463=CARTESIAN_POINT('Ctrl Pts',(0.0107766015850794,-0.0317669892870077,
0.0792516535055587));
#88464=CARTESIAN_POINT('Ctrl Pts',(0.0105758497041705,-0.0321934096636941,
0.0793524866347013));
#88465=CARTESIAN_POINT('Ctrl Pts',(0.0106689717374229,-0.0320508460845056,
0.0793085957939678));
#88466=CARTESIAN_POINT('Ctrl Pts',(0.0107608442960687,-0.0319086045664529,
0.0792622360417856));
#88467=CARTESIAN_POINT('Ctrl Pts',(0.0108512777801867,-0.0317669892870077,
0.0792135234844422));
#88468=CARTESIAN_POINT('',(0.010574479077327,-0.0321934096636941,0.0793530961726343));
#88469=CARTESIAN_POINT('',(0.0107861769030896,-0.0318665617511359,0.0792480172025542));
#88470=CARTESIAN_POINT('Origin',(0.0040154436663245,-0.0326371944423981,
0.0639843955346272));
#88471=CARTESIAN_POINT('Origin',(0.0158602828240402,-0.0316939261509356,
0.0889640369233801));
#88472=CARTESIAN_POINT('',(0.010461038580429,-0.0320197221621739,0.0794049806609027));
#88473=CARTESIAN_POINT('Ctrl Pts',(0.0104612211737369,-0.0320197392094664,
0.0794049510878703));
#88474=CARTESIAN_POINT('Ctrl Pts',(0.0104879600352183,-0.0319792716575962,
0.0793930574039811));
#88475=CARTESIAN_POINT('Ctrl Pts',(0.0105147299495146,-0.0319386439829649,
0.0793809057291985));
#88476=CARTESIAN_POINT('Ctrl Pts',(0.0105415555241534,-0.0318979099381581,
0.0793684756053362));
#88477=CARTESIAN_POINT('Ctrl Pts',(0.0105683805685643,-0.0318571766984905,
0.0793560457271647));
#88478=CARTESIAN_POINT('Ctrl Pts',(0.0105951256777918,-0.0318163871833577,
0.0793434022042498));
#88479=CARTESIAN_POINT('Ctrl Pts',(0.0106217003645882,-0.0317755399638303,
0.0793305917084602));
#88480=CARTESIAN_POINT('',(0.01046026409342,-0.0321934096636183,0.079403889257447));
#88481=CARTESIAN_POINT('Origin',(0.0114171723695981,-0.0324111793032775,
0.0815038783672763));
#88482=CARTESIAN_POINT('',(0.0105173715853835,-0.0321934096636663,0.0793784927150506));
#88483=CARTESIAN_POINT('Ctrl Pts',(0.0105725858802839,-0.0321934096636618,
0.0793523685103946));
#88484=CARTESIAN_POINT('Ctrl Pts',(0.0106443305965311,-0.0320835708272592,
0.0793185975990625));
#88485=CARTESIAN_POINT('Ctrl Pts',(0.0107153348106724,-0.0319739230346488,
0.0792833615230574));
#88486=CARTESIAN_POINT('Ctrl Pts',(0.0107855111376682,-0.0318646057455573,
0.0792467123365913));
#88487=CARTESIAN_POINT('Ctrl Pts',(0.0106783607208703,-0.0321934096636618,
0.0793930237420977));
#88488=CARTESIAN_POINT('Ctrl Pts',(0.0107506661044475,-0.0320835708272592,
0.0793577941132779));
#88489=CARTESIAN_POINT('Ctrl Pts',(0.0108222004726264,-0.0319739230346488,
0.0793210885629191));
#88490=CARTESIAN_POINT('Ctrl Pts',(0.0108928759063637,-0.0318646057455573,
0.0792829610773814));
#88491=CARTESIAN_POINT('Ctrl Pts',(0.0107841355614567,-0.0321934096636618,
0.0794336789738009));
#88492=CARTESIAN_POINT('Ctrl Pts',(0.0108570016123639,-0.0320835708272592,
0.0793969906274932));
#88493=CARTESIAN_POINT('Ctrl Pts',(0.0109290661345804,-0.0319739230346488,
0.0793588156027809));
#88494=CARTESIAN_POINT('Ctrl Pts',(0.0110002406750592,-0.0318646057455573,
0.0793192098181715));
#88495=CARTESIAN_POINT('Ctrl Pts',(0.0108899104020431,-0.0321934096636618,
0.079474334205504));
#88496=CARTESIAN_POINT('Ctrl Pts',(0.0109633371202803,-0.0320835708272592,
0.0794361871417086));
#88497=CARTESIAN_POINT('Ctrl Pts',(0.0110359317965343,-0.0319739230346488,
0.0793965426426427));
#88498=CARTESIAN_POINT('Ctrl Pts',(0.0111076054437547,-0.0318646057455573,
0.0793554585589616));
#88499=CARTESIAN_POINT('Ctrl Pts',(0.0109012769626364,-0.0321763980306388,
0.0794684135552823));
#88500=CARTESIAN_POINT('Ctrl Pts',(0.0108814091290246,-0.0321259596176398,
0.0794303701512932));
#88501=CARTESIAN_POINT('Ctrl Pts',(0.0108618855314024,-0.0320749164634525,
0.0793929858986422));
#88502=CARTESIAN_POINT('Ctrl Pts',(0.0108235110959878,-0.0319716057794028,
0.0793195056099573));
#88503=CARTESIAN_POINT('Ctrl Pts',(0.0108046752103315,-0.0319193786690229,
0.0792834382046323));
#88504=CARTESIAN_POINT('Ctrl Pts',(0.0107861769022256,-0.0318665617525437,
0.0792480172009062));
#88505=CARTESIAN_POINT('',(0.010732194739701,-0.0321934096636663,0.0794137151890684));
#88506=CARTESIAN_POINT('Ctrl Pts',(0.010640079839047,-0.0327445246967097,
0.0793217504200265));
#88507=CARTESIAN_POINT('Ctrl Pts',(0.0108351355948679,-0.032443687833936,
0.0792268467028444));
#88508=CARTESIAN_POINT('Ctrl Pts',(0.0110224886820328,-0.0321434074405927,
0.0791175202003684));
#88509=CARTESIAN_POINT('Ctrl Pts',(0.0106423030738584,-0.0327445246967097,
0.0793206070797563));
#88510=CARTESIAN_POINT('Ctrl Pts',(0.010837315707896,-0.032443687833936,
0.0792256195119026));
#88511=CARTESIAN_POINT('Ctrl Pts',(0.0110246194798068,-0.0321434074405927,
0.0791162126450747));
#88512=CARTESIAN_POINT('Ctrl Pts',(0.0108646265549997,-0.0327445246967097,
0.0792062730527424));
#88513=CARTESIAN_POINT('Ctrl Pts',(0.0110553270107139,-0.032443687833936,
0.0791029004177201));
#88514=CARTESIAN_POINT('Ctrl Pts',(0.0112376992572152,-0.0321434074405927,
0.0789854571157094));
#88515=CARTESIAN_POINT('',(0.0108963482986283,-0.0326943950436612,0.0791889485203287));
#88516=CARTESIAN_POINT('',(0.0111010304244936,-0.0323666188837389,0.0790707842839038));
#88517=CARTESIAN_POINT('Origin',(0.00272575589853286,-0.0326395579110424,
0.064497131816589));
#88518=CARTESIAN_POINT('Origin',(0.0168183829353055,-0.032193382560293,
0.0885204007911214));
#88519=CARTESIAN_POINT('',(0.0109933788563795,-0.0321934096536377,0.0791343294423074));
#88520=CARTESIAN_POINT('',(0.0110468530104245,-0.0321934096584275,0.0791019756912412));
#88521=CARTESIAN_POINT('',(0.0107861769035146,-0.0325210109756239,0.0792480172033843));
#88522=CARTESIAN_POINT('Origin',(0.00315866026972931,-0.0326393129159093,
0.0642878993250712));
#88523=CARTESIAN_POINT('',(0.0107855480161328,-0.0326943950436593,0.0792468129947429));
#88524=CARTESIAN_POINT('Origin',(0.0159065328648442,-0.0326943765538137,
0.089052598576396));
#88525=CARTESIAN_POINT('',(0.0108409481573906,-0.0326943950436702,0.0792178807575459));
#88526=CARTESIAN_POINT('Ctrl Pts',(0.0106906780628999,-0.0325229783203769,
0.0795731951461946));
#88527=CARTESIAN_POINT('Ctrl Pts',(0.0107654366893927,-0.032413025309245,
0.0795378105427639));
#88528=CARTESIAN_POINT('Ctrl Pts',(0.0108394520012984,-0.032303122220807,
0.0795008848278783));
#88529=CARTESIAN_POINT('Ctrl Pts',(0.0109126308592978,-0.0321934096576658,
0.079462468646228));
#88530=CARTESIAN_POINT('Ctrl Pts',(0.0107222803572808,-0.0325229783203769,
0.0794643721834226));
#88531=CARTESIAN_POINT('Ctrl Pts',(0.0107955388616117,-0.032413025309245,
0.079428551943055));
#88532=CARTESIAN_POINT('Ctrl Pts',(0.0108680452671686,-0.032303122220807,
0.0793912216892592));
#88533=CARTESIAN_POINT('Ctrl Pts',(0.0109397083857194,-0.0321934096576658,
0.079352432516709));
#88534=CARTESIAN_POINT('Ctrl Pts',(0.0107538826516618,-0.0325229783203769,
0.0793555492206506));
#88535=CARTESIAN_POINT('Ctrl Pts',(0.0108256410338306,-0.032413025309245,
0.079319293343346));
#88536=CARTESIAN_POINT('Ctrl Pts',(0.0108966385330388,-0.032303122220807,
0.0792815585506402));
#88537=CARTESIAN_POINT('Ctrl Pts',(0.0109667859121409,-0.0321934096576658,
0.0792423963871901));
#88538=CARTESIAN_POINT('Ctrl Pts',(0.0107854849460427,-0.0325229783203769,
0.0792467262578786));
#88539=CARTESIAN_POINT('Ctrl Pts',(0.0108557432060496,-0.032413025309245,
0.079210034743637));
#88540=CARTESIAN_POINT('Ctrl Pts',(0.010925231798909,-0.032303122220807,
0.0791718954120211));
#88541=CARTESIAN_POINT('Ctrl Pts',(0.0109938634385624,-0.0321934096576658,
0.0791323602576712));
#88542=CARTESIAN_POINT('',(0.0109530048554953,-0.0321934096584275,0.0792983990455642));
#88543=CARTESIAN_POINT('Ctrl Pts',(0.0109012769626633,-0.0322104233328916,
0.079468413555334));
#88544=CARTESIAN_POINT('Ctrl Pts',(0.0108813822077813,-0.0322609421830778,
0.0794303186018514));
#88545=CARTESIAN_POINT('Ctrl Pts',(0.0108618454586623,-0.0323120888239514,
0.0793929091663844));
#88546=CARTESIAN_POINT('Ctrl Pts',(0.0108234707327709,-0.0324156524631813,
0.0793194283214878));
#88547=CARTESIAN_POINT('Ctrl Pts',(0.0108046485300895,-0.0324680267167303,
0.0792833871166656));
#88548=CARTESIAN_POINT('Ctrl Pts',(0.0107861769034984,-0.0325210109755912,
0.0792480172033438));
#88549=CARTESIAN_POINT('Origin',(0.000761802954915682,-0.0262834582510798,
0.0769257246869562));
#88550=CARTESIAN_POINT('Origin',(0.00833608579388862,-0.0342770918174247,
0.0863064460005147));
#88551=CARTESIAN_POINT('Ctrl Pts',(0.0108944136167676,-0.0326943950436604,
0.0791883413161367));
#88552=CARTESIAN_POINT('Ctrl Pts',(0.010963851402962,-0.0325844576448134,
0.079150156822402));
#88553=CARTESIAN_POINT('Ctrl Pts',(0.0110325043854416,-0.0324744968375322,
0.079110533539028));
#88554=CARTESIAN_POINT('Ctrl Pts',(0.0111002853022404,-0.0323646534831894,
0.0790695234469394));
#88555=CARTESIAN_POINT('Ctrl Pts',(0.0110025323414518,-0.0326943950436604,
0.0792222746177034));
#88556=CARTESIAN_POINT('Ctrl Pts',(0.0110724377921395,-0.0325844576448134,
0.0791826000453065));
#88557=CARTESIAN_POINT('Ctrl Pts',(0.0111415276549402,-0.0324744968375322,
0.0791414769057466));
#88558=CARTESIAN_POINT('Ctrl Pts',(0.011209714134637,-0.0323646534831894,
0.0790989591093723));
#88559=CARTESIAN_POINT('Ctrl Pts',(0.011110651066136,-0.0326943950436604,
0.0792562079192702));
#88560=CARTESIAN_POINT('Ctrl Pts',(0.0111810241813171,-0.0325844576448134,
0.0792150432682109));
#88561=CARTESIAN_POINT('Ctrl Pts',(0.0112505509244387,-0.0324744968375322,
0.0791724202724651));
#88562=CARTESIAN_POINT('Ctrl Pts',(0.0113191429670336,-0.0323646534831894,
0.0791283947718053));
#88563=CARTESIAN_POINT('Ctrl Pts',(0.0112187697908201,-0.0326943950436604,
0.0792901412208369));
#88564=CARTESIAN_POINT('Ctrl Pts',(0.0112896105704947,-0.0325844576448134,
0.0792474864911154));
#88565=CARTESIAN_POINT('Ctrl Pts',(0.0113595741939372,-0.0324744968375322,
0.0792033636391837));
#88566=CARTESIAN_POINT('Ctrl Pts',(0.0114285717994302,-0.0323646534831894,
0.0791578304342382));
#88567=CARTESIAN_POINT('Ctrl Pts',(0.011229742161387,-0.0326773559987508,
0.0792835185414584));
#88568=CARTESIAN_POINT('Ctrl Pts',(0.0112075068882425,-0.0326267922587282,
0.0792467681685858));
#88569=CARTESIAN_POINT('Ctrl Pts',(0.0111856657192562,-0.0325756109581965,
0.0792106691695312));
#88570=CARTESIAN_POINT('Ctrl Pts',(0.0111427530014782,-0.0324719985462387,
0.0791397431966829));
#88571=CARTESIAN_POINT('Ctrl Pts',(0.0111216986639644,-0.0324196091621777,
0.0791049446696223));
#88572=CARTESIAN_POINT('Ctrl Pts',(0.0111010304244683,-0.0323666188837756,
0.0790707842838621));
#88573=CARTESIAN_POINT('',(0.0110575590447274,-0.0326943950436702,0.0792395448705903));
#88574=CARTESIAN_POINT('Ctrl Pts',(0.0109620325679172,-0.0332451089994433,
0.0791522454767732));
#88575=CARTESIAN_POINT('Ctrl Pts',(0.0111506953427584,-0.0329451141710254,
0.0790451991125171));
#88576=CARTESIAN_POINT('Ctrl Pts',(0.0113307589768031,-0.0326442513127493,
0.0789242460042235));
#88577=CARTESIAN_POINT('Ctrl Pts',(0.0111767373780794,-0.0332451089994433,
0.0790241757906911));
#88578=CARTESIAN_POINT('Ctrl Pts',(0.0113605699256834,-0.0329451141710254,
0.0789090317020339));
#88579=CARTESIAN_POINT('Ctrl Pts',(0.011535207100951,-0.0326442513127493,
0.0787803677065814));
#88580=CARTESIAN_POINT('',(0.0112072754682251,-0.0331951640388616,0.0790049144402668));
#88581=CARTESIAN_POINT('',(0.0114041341068746,-0.0328677532092642,0.0788741312769494));
#88582=CARTESIAN_POINT('Origin',(0.00158059036077552,-0.0326401908899661,
0.0652805208277939));
#88583=CARTESIAN_POINT('Origin',(0.0177100237123225,-0.0326944279134184,
0.0879554269733298));
#88584=CARTESIAN_POINT('',(0.0113006850036053,-0.0326943950436593,0.0789443105377789));
#88585=CARTESIAN_POINT('',(0.0113520221273582,-0.0326943950436693,0.0789086629610717));
#88586=CARTESIAN_POINT('',(0.0111010304244912,-0.0330220786163546,0.0790707842839053));
#88587=CARTESIAN_POINT('Origin',(0.00195683802494221,-0.0326396682762585,
0.0649810036409999));
#88588=CARTESIAN_POINT('',(0.0111003271651873,-0.0331951640388587,0.0790696219396608));
#88589=CARTESIAN_POINT('Origin',(0.016810972093738,-0.0331952026560192,
0.0885081548797547));
#88590=CARTESIAN_POINT('',(0.0111538013167162,-0.0331951640388701,0.0790372681899738));
#88591=CARTESIAN_POINT('Ctrl Pts',(0.0110261389619798,-0.0330240426238172,
0.0794013165193361));
#88592=CARTESIAN_POINT('Ctrl Pts',(0.0110984809631435,-0.032914277406352,
0.0793613337272157));
#88593=CARTESIAN_POINT('Ctrl Pts',(0.0111700324734335,-0.0328043479726691,
0.0793198354909738));
#88594=CARTESIAN_POINT('Ctrl Pts',(0.0112407003659551,-0.0326943950436593,
0.0792768724485639));
#88595=CARTESIAN_POINT('Ctrl Pts',(0.011050845822357,-0.0330240426238172,
0.0792907239923048));
#88596=CARTESIAN_POINT('Ctrl Pts',(0.0111216643037157,-0.032914277406352,
0.079250400839112));
#88597=CARTESIAN_POINT('Ctrl Pts',(0.0111916844984564,-0.0328043479726691,
0.0792085935675254));
#88598=CARTESIAN_POINT('Ctrl Pts',(0.0112608152305108,-0.0326943950436593,
0.0791653532654215));
#88599=CARTESIAN_POINT('Ctrl Pts',(0.0110755526827341,-0.0330240426238172,
0.0791801314652736));
#88600=CARTESIAN_POINT('Ctrl Pts',(0.0111448476442879,-0.032914277406352,
0.0791394679510084));
#88601=CARTESIAN_POINT('Ctrl Pts',(0.0112133365234794,-0.0328043479726691,
0.079097351644077));
#88602=CARTESIAN_POINT('Ctrl Pts',(0.0112809300950666,-0.0326943950436593,
0.079053834082279));
#88603=CARTESIAN_POINT('Ctrl Pts',(0.0111002595431113,-0.0330240426238172,
0.0790695389382423));
#88604=CARTESIAN_POINT('Ctrl Pts',(0.0111680309848601,-0.032914277406352,
0.0790285350629047));
#88605=CARTESIAN_POINT('Ctrl Pts',(0.0112349885485024,-0.0328043479726691,
0.0789861097206286));
#88606=CARTESIAN_POINT('Ctrl Pts',(0.0113010449596223,-0.0326943950436593,
0.0789423148991366));
#88607=CARTESIAN_POINT('',(0.0112706926847908,-0.0326943950436693,0.079110591493178));
#88608=CARTESIAN_POINT('Ctrl Pts',(0.0112297421613803,-0.0327114338383308,
0.0792835185414474));
#88609=CARTESIAN_POINT('Ctrl Pts',(0.0112075105866604,-0.0327619876830409,
0.0792467742813165));
#88610=CARTESIAN_POINT('Ctrl Pts',(0.0111856712241432,-0.0328131562603187,
0.0792106782679871));
#88611=CARTESIAN_POINT('Ctrl Pts',(0.0111427585458354,-0.0329167375858767,
0.0791397523603752));
#88612=CARTESIAN_POINT('Ctrl Pts',(0.0111217023287364,-0.0329691088920623,
0.0791049507267435));
#88613=CARTESIAN_POINT('Ctrl Pts',(0.0111010304244689,-0.0330220786163187,
0.0790707842838632));
#88614=CARTESIAN_POINT('Ctrl Pts',(0.0112053061629769,-0.0331951640388604,
0.0790044298365731));
#88615=CARTESIAN_POINT('Ctrl Pts',(0.0112721661213289,-0.0330855618127442,
0.0789619880728187));
#88616=CARTESIAN_POINT('Ctrl Pts',(0.0113381970792849,-0.032975722417194,
0.0789181338321737));
#88617=CARTESIAN_POINT('Ctrl Pts',(0.0114033117255521,-0.0328657861694598,
0.0788729191249603));
#88618=CARTESIAN_POINT('Ctrl Pts',(0.0113153423344818,-0.0331951640388604,
0.0790315073734137));
#88619=CARTESIAN_POINT('Ctrl Pts',(0.0113825752311698,-0.0330855618127442,
0.0789875500838217));
#88620=CARTESIAN_POINT('Ctrl Pts',(0.0114489480729757,-0.032975722417194,
0.0789421715168187));
#88621=CARTESIAN_POINT('Ctrl Pts',(0.0115143730150545,-0.0328657861694598,
0.0788954256132438));
#88622=CARTESIAN_POINT('Ctrl Pts',(0.0114253785059866,-0.0331951640388604,
0.0790585849102543));
#88623=CARTESIAN_POINT('Ctrl Pts',(0.0114929843410107,-0.0330855618127442,
0.0790131120948247));
#88624=CARTESIAN_POINT('Ctrl Pts',(0.0115596990666664,-0.032975722417194,
0.0789662092014639));
#88625=CARTESIAN_POINT('Ctrl Pts',(0.0116254343045569,-0.0328657861694598,
0.0789179321015274));
#88626=CARTESIAN_POINT('Ctrl Pts',(0.0115354146774915,-0.0331951640388604,
0.0790856624470949));
#88627=CARTESIAN_POINT('Ctrl Pts',(0.0116033934508515,-0.0330855618127442,
0.0790386741058277));
#88628=CARTESIAN_POINT('Ctrl Pts',(0.0116704500603572,-0.032975722417194,
0.078990246886109));
#88629=CARTESIAN_POINT('Ctrl Pts',(0.0117364955940593,-0.0328657861694598,
0.0789404385898109));
#88630=CARTESIAN_POINT('',(0.0115459495571488,-0.0331781648279232,0.0790783638781455));
#88631=CARTESIAN_POINT('',(0.0115354146774751,-0.0331951640388588,0.0790856624470899));
#88632=CARTESIAN_POINT('Origin',(0.00154597830059997,-0.0326412092733268,
0.065925909637409));
#88633=CARTESIAN_POINT('Ctrl Pts',(0.0115459495551421,-0.0331781648273463,
0.079078363875258));
#88634=CARTESIAN_POINT('Ctrl Pts',(0.0115214336445196,-0.0331276810208762,
0.079043057791277));
#88635=CARTESIAN_POINT('Ctrl Pts',(0.011497360599278,-0.0330765665171629,
0.0790083894907572));
#88636=CARTESIAN_POINT('Ctrl Pts',(0.0114500788061185,-0.032973061271521,
0.0789402975897152));
#88637=CARTESIAN_POINT('Ctrl Pts',(0.0114268896345128,-0.0329207135598926,
0.0789069021816162));
#88638=CARTESIAN_POINT('Ctrl Pts',(0.0114041341068486,-0.0328677532092985,
0.0788741312769121));
#88639=CARTESIAN_POINT('',(0.0113713450728601,-0.0331951640388701,0.0790452884436883));
#88640=CARTESIAN_POINT('Origin',(0.00812378219310841,-0.0315241814719618,
0.07415));
#88641=CARTESIAN_POINT('',(0.011545949556885,-0.0332121607144212,0.0790783638777656));
#88642=CARTESIAN_POINT('',(0.0115564688245398,-0.0331951640388587,0.0790710428254991));
#88643=CARTESIAN_POINT('Origin',(0.00151376860635569,-0.0326413667272291,
0.0659578257290841));
#88644=CARTESIAN_POINT('Origin',(0.00271608011466119,-0.0326412094323411,
0.0651134110508832));
#88645=CARTESIAN_POINT('Origin',(0.0027572391845267,-0.0326413668283485,
0.0650943830840143));
#88646=CARTESIAN_POINT('Ctrl Pts',(0.0112705080844135,-0.0337436976235975,
0.0789641708699412));
#88647=CARTESIAN_POINT('Ctrl Pts',(0.0113138074668253,-0.0336723290703325,
0.0789358687403755));
#88648=CARTESIAN_POINT('Ctrl Pts',(0.0113565907783128,-0.033601104548885,
0.0789067923700146));
#88649=CARTESIAN_POINT('Ctrl Pts',(0.011493189416996,-0.0333736987606857,
0.0788139572791567));
#88650=CARTESIAN_POINT('Ctrl Pts',(0.0116242355391332,-0.0331450831799191,
0.0787134363556759));
#88651=CARTESIAN_POINT('Ctrl Pts',(0.0114767481733374,-0.0337436976235975,
0.0788228732205599));
#88652=CARTESIAN_POINT('Ctrl Pts',(0.0115187767032764,-0.0336723290703325,
0.0787927161363779));
#88653=CARTESIAN_POINT('Ctrl Pts',(0.0115602560030983,-0.033601104548885,
0.078761807970119));
#88654=CARTESIAN_POINT('Ctrl Pts',(0.0116926911908432,-0.0333736987606857,
0.078663124317817));
#88655=CARTESIAN_POINT('Ctrl Pts',(0.0118192450989018,-0.0331450831799191,
0.0785570033936798));
#88656=CARTESIAN_POINT('Ctrl Pts',(0.0114788105742266,-0.0337436976235975,
0.0788214602440662));
#88657=CARTESIAN_POINT('Ctrl Pts',(0.0115208263956409,-0.0336723290703325,
0.0787912846103379));
#88658=CARTESIAN_POINT('Ctrl Pts',(0.0115622926553462,-0.033601104548885,
0.07876035812612));
#88659=CARTESIAN_POINT('Ctrl Pts',(0.0116946862085817,-0.0333736987606857,
0.0786616159882036));
#88660=CARTESIAN_POINT('Ctrl Pts',(0.0118211951944995,-0.0331450831799191,
0.0785554390640598));
#88661=CARTESIAN_POINT('',(0.0115060334985897,-0.0336938721132548,0.0788017202309007));
#88662=CARTESIAN_POINT('',(0.0116942917446253,-0.0333679869945434,0.078658834277581));
#88663=CARTESIAN_POINT('Ctrl Pts',(0.0115060334985922,-0.033693872113265,
0.0788017202308998));
#88664=CARTESIAN_POINT('Ctrl Pts',(0.011524191344814,-0.0336629187933934,
0.0787885177174118));
#88665=CARTESIAN_POINT('Ctrl Pts',(0.0115422660776993,-0.0336319952301041,
0.078775213104912));
#88666=CARTESIAN_POINT('Ctrl Pts',(0.0115602560031003,-0.0336011045488951,
0.0787618079701178));
#88667=CARTESIAN_POINT('Ctrl Pts',(0.0116053988817375,-0.0335235892595455,
0.0787281698999402));
#88668=CARTESIAN_POINT('Ctrl Pts',(0.0116500878701258,-0.033445866866037,
0.078693838969908));
#88669=CARTESIAN_POINT('Ctrl Pts',(0.011694291744808,-0.0333679869945386,
0.0786588342778223));
#88670=CARTESIAN_POINT('Ctrl Pts',(0.0116943270343373,-0.0333679692459667,
0.0786588072090433));
#88671=CARTESIAN_POINT('Ctrl Pts',(0.0116940410271472,-0.0333391895375561,
0.0786584555875025));
#88672=CARTESIAN_POINT('Ctrl Pts',(0.011693824131719,-0.0333104081062525,
0.0786581940790117));
#88673=CARTESIAN_POINT('Ctrl Pts',(0.0116935327705736,-0.033253269827004,
0.0786578514635641));
#88674=CARTESIAN_POINT('Ctrl Pts',(0.0116934562254131,-0.0332249171466895,
0.0786577677241525));
#88675=CARTESIAN_POINT('Ctrl Pts',(0.0116934485380219,-0.0331960985356852,
0.0786577691298677));
#88676=CARTESIAN_POINT('Ctrl Pts',(0.011693448431858,-0.0331956312568221,
0.0786577691759818));
#88677=CARTESIAN_POINT('Ctrl Pts',(0.0116934483446455,-0.0331951640388597,
0.0786577692450447));
#88678=CARTESIAN_POINT('',(0.0115954533610552,-0.0331951640388587,0.0787353706831235));
#88679=CARTESIAN_POINT('',(0.0116444508528592,-0.0331951640388687,0.078696569964095));
#88680=CARTESIAN_POINT('',(0.0114041341065212,-0.0335216366567644,0.0788741312767267));
#88681=CARTESIAN_POINT('Origin',(0.000935548044213429,-0.0326434571526759,
0.0659211636290065));
#88682=CARTESIAN_POINT('',(0.0114033592510911,-0.0336938721132327,0.0788730153843445));
#88683=CARTESIAN_POINT('Origin',(0.0176320276870547,-0.0336938867896355,
0.0878431056559906));
#88684=CARTESIAN_POINT('',(0.0114546963748504,-0.0336938721132538,0.0788373678076325));
#88685=CARTESIAN_POINT('Ctrl Pts',(0.0113501455266319,-0.0335235895815172,
0.0792087132395667));
#88686=CARTESIAN_POINT('Ctrl Pts',(0.0114197886740644,-0.0334144449262748,
0.0791642959961559));
#88687=CARTESIAN_POINT('Ctrl Pts',(0.0114885942062146,-0.0333049234473147,
0.0791183889477));
#88688=CARTESIAN_POINT('Ctrl Pts',(0.011556468824539,-0.0331951640388587,
0.0790710428255066));
#88689=CARTESIAN_POINT('Ctrl Pts',(0.0113678594786838,-0.0335235895815172,
0.0790967874231122));
#88690=CARTESIAN_POINT('Ctrl Pts',(0.0114359617468911,-0.0334144449262748,
0.0790521263122758));
#88691=CARTESIAN_POINT('Ctrl Pts',(0.0115032195914152,-0.0333049234473147,
0.0790060069496254));
#88692=CARTESIAN_POINT('Ctrl Pts',(0.0115695416681373,-0.0331951640388587,
0.0789584805172211));
#88693=CARTESIAN_POINT('Ctrl Pts',(0.0113855734307357,-0.0335235895815172,
0.0789848616066576));
#88694=CARTESIAN_POINT('Ctrl Pts',(0.0114521348197178,-0.0334144449262748,
0.0789399566283957));
#88695=CARTESIAN_POINT('Ctrl Pts',(0.0115178449766157,-0.0333049234473147,
0.0788936249515508));
#88696=CARTESIAN_POINT('Ctrl Pts',(0.0115826145117357,-0.0331951640388587,
0.0788459182089356));
#88697=CARTESIAN_POINT('Ctrl Pts',(0.0114032873827875,-0.0335235895815172,
0.078872935790203));
#88698=CARTESIAN_POINT('Ctrl Pts',(0.0114683078925445,-0.0334144449262748,
0.0788277869445156));
#88699=CARTESIAN_POINT('Ctrl Pts',(0.0115324703618162,-0.0333049234473147,
0.0787812429534761));
#88700=CARTESIAN_POINT('Ctrl Pts',(0.0115956873553341,-0.0331951640388587,
0.07873335590065));
#88701=CARTESIAN_POINT('',(0.0115759610928075,-0.0331951640388687,0.0789032067543213));
#88702=CARTESIAN_POINT('Ctrl Pts',(0.0115459495550925,-0.0332121607145958,
0.0790783638751866));
#88703=CARTESIAN_POINT('Ctrl Pts',(0.011521474958517,-0.0332625444109105,
0.0790431172887799));
#88704=CARTESIAN_POINT('Ctrl Pts',(0.0114974220976462,-0.0333135300745512,
0.0790084780563661));
#88705=CARTESIAN_POINT('Ctrl Pts',(0.0114501407543524,-0.0334167203140533,
0.0789403868031891));
#88706=CARTESIAN_POINT('Ctrl Pts',(0.0114269305844705,-0.0334688847587202,
0.0789069611548547));
#88707=CARTESIAN_POINT('Ctrl Pts',(0.0114041341062497,-0.0335216366562257,
0.0788741312760496));
#88708=CARTESIAN_POINT('Ctrl Pts',(0.0115050495193523,-0.0336938721132389,
0.0788015427492615));
#88709=CARTESIAN_POINT('Ctrl Pts',(0.0115322765426092,-0.0336474569764957,
0.0787817510695775));
#88710=CARTESIAN_POINT('Ctrl Pts',(0.0115592700136535,-0.033601104548885,
0.0787616420193482));
#88711=CARTESIAN_POINT('Ctrl Pts',(0.0116276112761496,-0.0334837508592655,
0.0787107305275279));
#88712=CARTESIAN_POINT('Ctrl Pts',(0.0116944139151403,-0.0333660264659097,
0.0786578162989802));
#88713=CARTESIAN_POINT('Ctrl Pts',(0.0115060334985732,-0.0336938721132389,
0.0788017202309126));
#88714=CARTESIAN_POINT('Ctrl Pts',(0.0115332615606891,-0.0336474569764957,
0.0787819227916717));
#88715=CARTESIAN_POINT('Ctrl Pts',(0.0115602560030983,-0.033601104548885,
0.078761807970119));
#88716=CARTESIAN_POINT('Ctrl Pts',(0.0116285997248671,-0.0334837508592655,
0.0787108818666348));
#88717=CARTESIAN_POINT('Ctrl Pts',(0.0116954043890766,-0.0333660264659097,
0.078657952959966));
#88718=CARTESIAN_POINT('Ctrl Pts',(0.0118405907808433,-0.0336938721132389,
0.0788620647763927));
#88719=CARTESIAN_POINT('Ctrl Pts',(0.0118681720596084,-0.0336474569764957,
0.0788403090623608));
#88720=CARTESIAN_POINT('Ctrl Pts',(0.0118954967703852,-0.033601104548885,
0.0788182319653524));
#88721=CARTESIAN_POINT('Ctrl Pts',(0.0119646766557272,-0.0334837508592655,
0.07876233783157));
#88722=CARTESIAN_POINT('Ctrl Pts',(0.0120321699032904,-0.0333660264659097,
0.0787044182989356));
#88723=CARTESIAN_POINT('',(0.0118486512207968,-0.0336769361243753,0.0788537592122224));
#88724=CARTESIAN_POINT('',(0.0118385954093542,-0.033693872113232,0.0788617048685593));
#88725=CARTESIAN_POINT('Ctrl Pts',(0.0118486512207971,-0.033676936124375,
0.0788537592122222));
#88726=CARTESIAN_POINT('Ctrl Pts',(0.0118469765411615,-0.0336797586670006,
0.0788550853775348));
#88727=CARTESIAN_POINT('Ctrl Pts',(0.0118453012166317,-0.0336825812712807,
0.0788564105983367));
#88728=CARTESIAN_POINT('Ctrl Pts',(0.0118419492873817,-0.0336882265874452,
0.0788590591439903));
#88729=CARTESIAN_POINT('Ctrl Pts',(0.0118402726826985,-0.0336910492993153,
0.0788603824688577));
#88730=CARTESIAN_POINT('Ctrl Pts',(0.011838595409368,-0.0336938721132378,
0.0788617048685643));
#88731=CARTESIAN_POINT('Ctrl Pts',(0.0118486512207968,-0.0336769361243753,
0.0788537592122224));
#88732=CARTESIAN_POINT('Ctrl Pts',(0.0118226306795899,-0.0336279007516194,
0.0788209005104803));
#88733=CARTESIAN_POINT('Ctrl Pts',(0.0117962396464481,-0.0335767878632062,
0.0787875739520604));
#88734=CARTESIAN_POINT('Ctrl Pts',(0.0117445206321308,-0.0334733198857316,
0.0787222632557021));
#88735=CARTESIAN_POINT('Ctrl Pts',(0.0117191618603002,-0.0334209645014074,
0.0786902402353689));
#88736=CARTESIAN_POINT('Ctrl Pts',(0.0116942917389024,-0.0333679869844683,
0.0786588342820951));
#88737=CARTESIAN_POINT('',(0.011672314453982,-0.0336938721132534,0.07883171254974));
#88738=CARTESIAN_POINT('Origin',(0.00812378219310841,-0.0315241814719618,
0.07415));
#88739=CARTESIAN_POINT('',(0.0118486512199988,-0.0337108120655385,0.0788537592112131));
#88740=CARTESIAN_POINT('',(0.0118586900372345,-0.0336938721132327,0.0788457920946194));
#88741=CARTESIAN_POINT('Origin',(0.00256758261447966,-0.0345562526817935,
0.0653334041418887));
#88742=CARTESIAN_POINT('Ctrl Pts',(0.0118586900372366,-0.0336938721132377,
0.0788457920946326));
#88743=CARTESIAN_POINT('Ctrl Pts',(0.011857018429022,-0.0336910493001332,
0.0788471216472421));
#88744=CARTESIAN_POINT('Ctrl Pts',(0.0118553460727901,-0.0336882265878542,
0.0788484503375465));
#88745=CARTESIAN_POINT('Ctrl Pts',(0.0118519998085138,-0.0336825812713067,
0.0788511060373876));
#88746=CARTESIAN_POINT('Ctrl Pts',(0.0118503259004399,-0.0336797586670136,
0.078852433046904));
#88747=CARTESIAN_POINT('Ctrl Pts',(0.0118486512207966,-0.033676936124375,
0.0788537592122226));
#88748=CARTESIAN_POINT('Origin',(0.000815265691572346,-0.0345562523865742,
0.0667210503996088));
#88749=CARTESIAN_POINT('Ctrl Pts',(0.0115665416655903,-0.0342436276873911,
0.0787571175603229));
#88750=CARTESIAN_POINT('Ctrl Pts',(0.0117403019688528,-0.033943005420181,
0.0786272717462829));
#88751=CARTESIAN_POINT('Ctrl Pts',(0.0119037881185698,-0.0336441434784052,
0.0784847064725858));
#88752=CARTESIAN_POINT('Ctrl Pts',(0.0117635040163719,-0.0342436276873911,
0.0786031505756328));
#88753=CARTESIAN_POINT('Ctrl Pts',(0.0119314573590779,-0.033943005420181,
0.0784658762040717));
#88754=CARTESIAN_POINT('Ctrl Pts',(0.0120885934958144,-0.0336441434784052,
0.0783163408806692));
#88755=CARTESIAN_POINT('Ctrl Pts',(0.0117654736398797,-0.0342436276873911,
0.0786016109057859));
#88756=CARTESIAN_POINT('Ctrl Pts',(0.0119333689129802,-0.033943005420181,
0.0784642622486496));
#88757=CARTESIAN_POINT('Ctrl Pts',(0.0120904415495869,-0.0336441434784052,
0.07831465722475));
#88758=CARTESIAN_POINT('',(0.0117914433282312,-0.0341934961088741,0.0785801678069697));
#88759=CARTESIAN_POINT('',(0.0119703582026119,-0.0338664212864873,0.0784257429773084));
#88760=CARTESIAN_POINT('Origin',(0.00151709971471466,-0.0345610720404953,
0.0653706633845988));
#88761=CARTESIAN_POINT('Origin',(0.0193047456575757,-0.0336938005072917,
0.0865783796737805));
#88762=CARTESIAN_POINT('',(0.0118765206184609,-0.0336938721132327,0.0785083344652383));
#88763=CARTESIAN_POINT('',(0.0119229851076007,-0.0336938721132427,0.0784665337326003));
#88764=CARTESIAN_POINT('',(0.0116942917388981,-0.0340203938281605,0.0786588342820984));
#88765=CARTESIAN_POINT('Origin',(0.00193792105499299,-0.0345589643245715,
0.0651373264308059));
#88766=CARTESIAN_POINT('',(0.0116934483446432,-0.034193496108874,0.0786577692450465));
#88767=CARTESIAN_POINT('Origin',(0.0185344473858077,-0.0341934220717648,
0.0872965741613755));
#88768=CARTESIAN_POINT('',(0.0117424458364472,-0.0341934961088841,0.0786189685260182));
#88769=CARTESIAN_POINT('Ctrl Pts',(0.0116614160580294,-0.0340223579322396,
0.0789961476079296));
#88770=CARTESIAN_POINT('Ctrl Pts',(0.0117282570728263,-0.0339125849573574,
0.0789473544103959));
#88771=CARTESIAN_POINT('Ctrl Pts',(0.0117940412134068,-0.0338030433565231,
0.0788972120455879));
#88772=CARTESIAN_POINT('Ctrl Pts',(0.011858690037234,-0.0336938721132326,
0.0788457920946276));
#88773=CARTESIAN_POINT('Ctrl Pts',(0.011672067229974,-0.0340223579322396,
0.0788833303558494));
#88774=CARTESIAN_POINT('Ctrl Pts',(0.011737352200625,-0.0339125849573574,
0.0788343902508751));
#88775=CARTESIAN_POINT('Ctrl Pts',(0.0118015783498311,-0.0338030433565231,
0.0787841332883549));
#88776=CARTESIAN_POINT('Ctrl Pts',(0.011864669240455,-0.0336938721132326,
0.078732631019343));
#88777=CARTESIAN_POINT('Ctrl Pts',(0.0116827184019186,-0.0340223579322396,
0.0787705131037693));
#88778=CARTESIAN_POINT('Ctrl Pts',(0.0117464473284237,-0.0339125849573574,
0.0787214260913545));
#88779=CARTESIAN_POINT('Ctrl Pts',(0.0118091154862554,-0.0338030433565231,
0.0786710545311219));
#88780=CARTESIAN_POINT('Ctrl Pts',(0.0118706484436759,-0.0336938721132326,
0.0786194699440584));
#88781=CARTESIAN_POINT('Ctrl Pts',(0.0116933695738632,-0.0340223579322396,
0.0786576958516891));
#88782=CARTESIAN_POINT('Ctrl Pts',(0.0117555424562223,-0.0339125849573574,
0.0786084619318338));
#88783=CARTESIAN_POINT('Ctrl Pts',(0.0118166526226797,-0.0338030433565231,
0.0785579757738889));
#88784=CARTESIAN_POINT('Ctrl Pts',(0.0118766276468969,-0.0336938721132326,
0.0785063088687738));
#88785=CARTESIAN_POINT('',(0.0118676053278577,-0.0336938721132427,0.0786770632799389));
#88786=CARTESIAN_POINT('Ctrl Pts',(0.0118486512177558,-0.0337108120662667,
0.0788537592083825));
#88787=CARTESIAN_POINT('Ctrl Pts',(0.011821956784873,-0.0337611408993659,
0.0788200495172082));
#88788=CARTESIAN_POINT('Ctrl Pts',(0.0117957494661654,-0.0338121088780008,
0.0787869549531089));
#88789=CARTESIAN_POINT('Ctrl Pts',(0.0117442851825266,-0.0339153382773234,
0.0787219659302822));
#88790=CARTESIAN_POINT('Ctrl Pts',(0.0117190462010022,-0.0339675637691194,
0.0786900941809752));
#88791=CARTESIAN_POINT('Ctrl Pts',(0.0116942879989058,-0.0340204018098272,
0.0786588295592332));
#88792=CARTESIAN_POINT('Ctrl Pts',(0.011789428722031,-0.0341934961088741,
0.0785799338331629));
#88793=CARTESIAN_POINT('Ctrl Pts',(0.0118810141140772,-0.0340287516182428,
0.0785041494790173));
#88794=CARTESIAN_POINT('Ctrl Pts',(0.0119693890233064,-0.0338644633275951,
0.0784246445874175));
#88795=CARTESIAN_POINT('Ctrl Pts',(0.0117914433282311,-0.0341934961088741,
0.0785801678069697));
#88796=CARTESIAN_POINT('Ctrl Pts',(0.0118830335575015,-0.0340287516182428,
0.0785043418024279));
#88797=CARTESIAN_POINT('Ctrl Pts',(0.011971411578379,-0.0338644633275951,
0.0784247950960955));
#88798=CARTESIAN_POINT('Ctrl Pts',(0.0121271154706234,-0.0341934961088741,
0.078619152343487));
#88799=CARTESIAN_POINT('Ctrl Pts',(0.0122195116744737,-0.0340287516182428,
0.0785363865818478));
#88800=CARTESIAN_POINT('Ctrl Pts',(0.0123084081558157,-0.0338644633275951,
0.0784498727367667));
#88801=CARTESIAN_POINT('',(0.0121366525261739,-0.0341764758832446,0.0786105909564536));
#88802=CARTESIAN_POINT('',(0.0121271154706064,-0.034193496108874,0.078619152343485));
#88803=CARTESIAN_POINT('Origin',(0.00144334588065161,-0.0345621026416435,
0.0659585348654658));
#88804=CARTESIAN_POINT('Ctrl Pts',(0.0121366525243996,-0.0341764758837558,
0.0786105909568769));
#88805=CARTESIAN_POINT('Ctrl Pts',(0.012107944187226,-0.0341260050040581,
0.0785786796175815));
#88806=CARTESIAN_POINT('Ctrl Pts',(0.0120797348402744,-0.0340749269148394,
0.0785473229981994));
#88807=CARTESIAN_POINT('Ctrl Pts',(0.0120242924006475,-0.0339715436306688,
0.0784856947748888));
#88808=CARTESIAN_POINT('Ctrl Pts',(0.0119970803460565,-0.0339192778238052,
0.0784554465473427));
#88809=CARTESIAN_POINT('Ctrl Pts',(0.0119703582020076,-0.0338664212855959,
0.0784257429794382));
#88810=CARTESIAN_POINT('',(0.0119592793994288,-0.0341934961088841,0.0785996600752375));
#88811=CARTESIAN_POINT('Origin',(0.00812378219310841,-0.0315241814719618,
0.07415));
#88812=CARTESIAN_POINT('',(0.0121366525263052,-0.0342105180190354,0.0786105909553415));
#88813=CARTESIAN_POINT('',(0.0121461712749854,-0.0341934961088739,0.0786020092176454));
#88814=CARTESIAN_POINT('Origin',(0.00140637764150144,-0.0345621722724057,
0.0659847582638457));
#88815=CARTESIAN_POINT('Origin',(0.000681924122869572,-0.0345621028456128,
0.0666435303060728));
#88816=CARTESIAN_POINT('Origin',(0.000711897734075975,-0.0345621725703317,
0.0666095320673899));
#88817=CARTESIAN_POINT('Ctrl Pts',(0.011875405463354,-0.0346945769586966,
0.0785093376894498));
#88818=CARTESIAN_POINT('Ctrl Pts',(0.0119667135366431,-0.0345275153362944,
0.0784307584379865));
#88819=CARTESIAN_POINT('Ctrl Pts',(0.0120555739817455,-0.0343603235965185,
0.0783492873070423));
#88820=CARTESIAN_POINT('Ctrl Pts',(0.0121417275701354,-0.034193496108874,
0.0782651691580946));
#88821=CARTESIAN_POINT('Ctrl Pts',(0.0119377298340476,-0.0346945769586966,
0.0784532689710457));
#88822=CARTESIAN_POINT('Ctrl Pts',(0.0120278635255811,-0.0345275153362944,
0.0783733843106849));
#88823=CARTESIAN_POINT('Ctrl Pts',(0.0121155082312643,-0.0343603235965185,
0.0782906443664228));
#88824=CARTESIAN_POINT('Ctrl Pts',(0.0122004083739621,-0.034193496108874,
0.0782052976988833));
#88825=CARTESIAN_POINT('Ctrl Pts',(0.0120000542047416,-0.0346945769586966,
0.0783972002526438));
#88826=CARTESIAN_POINT('Ctrl Pts',(0.0120890135145195,-0.0345275153362944,
0.0783160101833845));
#88827=CARTESIAN_POINT('Ctrl Pts',(0.0121754424807835,-0.0343603235965185,
0.078232001425804));
#88828=CARTESIAN_POINT('Ctrl Pts',(0.0122590891777892,-0.034193496108874,
0.0781454262396725));
#88829=CARTESIAN_POINT('Ctrl Pts',(0.0120623785754349,-0.0346945769586966,
0.0783411315342375));
#88830=CARTESIAN_POINT('Ctrl Pts',(0.012150163503457,-0.0345275153362944,
0.0782586360560816));
#88831=CARTESIAN_POINT('Ctrl Pts',(0.0122353767303018,-0.0343603235965185,
0.0781733584851839));
#88832=CARTESIAN_POINT('Ctrl Pts',(0.0123177699816155,-0.034193496108874,
0.0780855547804608));
#88833=CARTESIAN_POINT('',(0.0120623785749843,-0.0346945769586966,0.0783411315346425));
#88834=CARTESIAN_POINT('',(0.012231243985032,-0.0343667727831542,0.078175777270098));
#88835=CARTESIAN_POINT('Origin',(0.000415580299837392,-0.0345626457064528,
0.0662147414213684));
#88836=CARTESIAN_POINT('Origin',(0.0201244088264278,-0.0341934771029137,
0.0859119651688161));
#88837=CARTESIAN_POINT('',(0.0121427775317648,-0.034193496108874,0.0782640978923525));
#88838=CARTESIAN_POINT('',(0.0121865256441295,-0.034193496108884,0.0782194621144998));
#88839=CARTESIAN_POINT('',(0.011970358200964,-0.0345211942962608,0.0784257429782233));
#88840=CARTESIAN_POINT('Origin',(0.000775254284101102,-0.0345625596120131,
0.0658956404734609));
#88841=CARTESIAN_POINT('',(0.0119694495967205,-0.0346945769586885,0.0784247329999423));
#88842=CARTESIAN_POINT('Origin',(0.0193688924135947,-0.0346945685853941,
0.0866497412808417));
#88843=CARTESIAN_POINT('',(0.0120159140858624,-0.0346945769587026,0.0783829322673024));
#88844=CARTESIAN_POINT('Ctrl Pts',(0.0119587282116965,-0.0345231616327842,
0.0787644543593578));
#88845=CARTESIAN_POINT('Ctrl Pts',(0.0120223319684082,-0.0344132092796988,
0.0787115950276637));
#88846=CARTESIAN_POINT('Ctrl Pts',(0.0120848390898771,-0.0343032738558979,
0.0786574228297305));
#88847=CARTESIAN_POINT('Ctrl Pts',(0.0121461712749856,-0.0341934961088739,
0.0786020092176541));
#88848=CARTESIAN_POINT('Ctrl Pts',(0.01196227448792,-0.0345231616327842,
0.0786511911258532));
#88849=CARTESIAN_POINT('Ctrl Pts',(0.0120243170704197,-0.0344132092796988,
0.0785982829137341));
#88850=CARTESIAN_POINT('Ctrl Pts',(0.0120852620871731,-0.0343032738558979,
0.0785440941295551));
#88851=CARTESIAN_POINT('Ctrl Pts',(0.0121450332388432,-0.0341934961088739,
0.0784886961953984));
#88852=CARTESIAN_POINT('Ctrl Pts',(0.0119658207641435,-0.0345231616327842,
0.0785379278923486));
#88853=CARTESIAN_POINT('Ctrl Pts',(0.0120263021724312,-0.0344132092796988,
0.0784849707998045));
#88854=CARTESIAN_POINT('Ctrl Pts',(0.012085685084469,-0.0343032738558979,
0.0784307654293796));
#88855=CARTESIAN_POINT('Ctrl Pts',(0.0121438952027009,-0.0341934961088739,
0.0783753831731428));
#88856=CARTESIAN_POINT('Ctrl Pts',(0.0119693670403671,-0.0345231616327842,
0.0784246646588441));
#88857=CARTESIAN_POINT('Ctrl Pts',(0.0120282872744428,-0.0344132092796988,
0.078371658685875));
#88858=CARTESIAN_POINT('Ctrl Pts',(0.0120861080817649,-0.0343032738558979,
0.0783174367292042));
#88859=CARTESIAN_POINT('Ctrl Pts',(0.0121427571665586,-0.0341934961088739,
0.0782620701508871));
#88860=CARTESIAN_POINT('',(0.0121444744033851,-0.0341934961088839,0.078433053555009));
#88861=CARTESIAN_POINT('Ctrl Pts',(0.0121366525239888,-0.0342105180195365,
0.0786105909527672));
#88862=CARTESIAN_POINT('Ctrl Pts',(0.0121079119233284,-0.0342610556240453,
0.0785786437297793));
#88863=CARTESIAN_POINT('Ctrl Pts',(0.0120796870578849,-0.0343122189868431,
0.0785472697831875));
#88864=CARTESIAN_POINT('Ctrl Pts',(0.0120242440558992,-0.0344158119695077,
0.0784856409408228));
#88865=CARTESIAN_POINT('Ctrl Pts',(0.0119970485960829,-0.0344681990449947,
0.0784554112518445));
#88866=CARTESIAN_POINT('Ctrl Pts',(0.0119703582009428,-0.0345211942962355,
0.0784257429781971));
#88867=CARTESIAN_POINT('Ctrl Pts',(0.0120603537487011,-0.0346945769586932,
0.0783410245469078));
#88868=CARTESIAN_POINT('Ctrl Pts',(0.0121470002157346,-0.034529677707698,
0.0782596387154246));
#88869=CARTESIAN_POINT('Ctrl Pts',(0.0122302088932423,-0.0343648066251421,
0.0781747412490137));
#88870=CARTESIAN_POINT('Ctrl Pts',(0.0120623785749777,-0.0346945769586932,
0.0783411315346486));
#88871=CARTESIAN_POINT('Ctrl Pts',(0.012149027253907,-0.034529677707698,
0.0782597038413149));
#88872=CARTESIAN_POINT('Ctrl Pts',(0.0122322364112318,-0.0343648066251421,
0.0781747644574042));
#88873=CARTESIAN_POINT('Ctrl Pts',(0.012399836204375,-0.0346945769586932,
0.0783589621158761));
#88874=CARTESIAN_POINT('Ctrl Pts',(0.0124868535179547,-0.034529677707698,
0.0782705577248319));
#88875=CARTESIAN_POINT('Ctrl Pts',(0.0125701426416088,-0.0343648066251421,
0.0781786323687029));
#88876=CARTESIAN_POINT('',(0.0124088168670256,-0.034677539666503,0.0783498187861985));
#88877=CARTESIAN_POINT('',(0.0123998362043608,-0.0346945769586887,0.0783589621158728));
#88878=CARTESIAN_POINT('Origin',(0.000446020694324284,-0.0345626618039033,
0.066838762831078));
#88879=CARTESIAN_POINT('Ctrl Pts',(0.0124088168652486,-0.0346775396670096,
0.0783498187866297));
#88880=CARTESIAN_POINT('Ctrl Pts',(0.0123781373046023,-0.0346269749928197,
0.0783197493641814));
#88881=CARTESIAN_POINT('Ctrl Pts',(0.012348002963064,-0.0345757902890816,
0.0782902143681198));
#88882=CARTESIAN_POINT('Ctrl Pts',(0.0122888000214345,-0.0344721681087906,
0.0782321887818647));
#88883=CARTESIAN_POINT('Ctrl Pts',(0.0122597546356236,-0.0344197714289445,
0.0782037209364014));
#88884=CARTESIAN_POINT('Ctrl Pts',(0.0122312439849364,-0.0343667727830771,
0.0781757772703416));
#88885=CARTESIAN_POINT('',(0.0122311073896826,-0.0346945769587026,0.0783500468252676));
#88886=CARTESIAN_POINT('Origin',(0.00812378219310841,-0.0315241814719618,
0.07415));
#88887=CARTESIAN_POINT('',(0.012408816866699,-0.0347116136489781,0.0783498187848444));
#88888=CARTESIAN_POINT('',(0.012417777980685,-0.0346945769586885,0.0783406562942192));
#88889=CARTESIAN_POINT('Origin',(0.000415668195806348,-0.0345626702675865,
0.0668724051349416));
#88890=CARTESIAN_POINT('Origin',(0.000659814792040836,-0.0345626619863005,
0.0666206300659209));
#88891=CARTESIAN_POINT('Origin',(0.000692841233989324,-0.0345626706114569,
0.0665896088296775));
#88892=CARTESIAN_POINT('Ctrl Pts',(0.012115097209926,-0.0352450361874068,
0.0782910345400819));
#88893=CARTESIAN_POINT('Ctrl Pts',(0.0122712788904274,-0.0349452760959493,
0.0781404996240595));
#88894=CARTESIAN_POINT('Ctrl Pts',(0.0124156779694018,-0.034644428984174,
0.0779786281186687));
#88895=CARTESIAN_POINT('Ctrl Pts',(0.0121168759173089,-0.0352450361874068,
0.0782892423835469));
#88896=CARTESIAN_POINT('Ctrl Pts',(0.0122729900055175,-0.0349452760959493,
0.0781386403824747));
#88897=CARTESIAN_POINT('Ctrl Pts',(0.0124173166311011,-0.034644428984174,
0.0779767070739437));
#88898=CARTESIAN_POINT('Ctrl Pts',(0.0122929855591785,-0.0352450361874068,
0.078111801142454));
#88899=CARTESIAN_POINT('Ctrl Pts',(0.0124424073411636,-0.0349452760959493,
0.0779545570572472));
#88900=CARTESIAN_POINT('Ctrl Pts',(0.0125795603637071,-0.034644428984174,
0.0777865046259309));
#88901=CARTESIAN_POINT('Ctrl Pts',(0.0122947466555972,-0.0352450361874068,
0.0781100267300432));
#88902=CARTESIAN_POINT('Ctrl Pts',(0.01244410151452,-0.0349452760959493,
0.0779527162239949));
#88903=CARTESIAN_POINT('Ctrl Pts',(0.0125811828010331,-0.034644428984174,
0.0777846026014507));
#88904=CARTESIAN_POINT('',(0.0123177495694777,-0.0351951634053343,0.0780855800015301));
#88905=CARTESIAN_POINT('',(0.012475919493575,-0.0348678972925388,0.0779099236585187));
#88906=CARTESIAN_POINT('Origin',(-0.000474189373535641,-0.0345636767883037,
0.0672795263998118));
#88907=CARTESIAN_POINT('Origin',(0.0208374958163375,-0.0346946199340759,
0.0851337059576703));
#88908=CARTESIAN_POINT('',(0.0123931732943985,-0.0346945769330289,0.0780036248678973));
#88909=CARTESIAN_POINT('',(0.0124340323821223,-0.0346945769458128,0.0779563301954911));
#88910=CARTESIAN_POINT('',(0.0122312439848407,-0.0350221583435276,0.0781757772702249));
#88911=CARTESIAN_POINT('Origin',(-0.000192449574958003,-0.0345628458716686,
0.0668899547387003));
#88912=CARTESIAN_POINT('',(0.0122303585188129,-0.0351951360298763,0.0781749136483986));
#88913=CARTESIAN_POINT('Origin',(0.0200998093611332,-0.0351951838366795,
0.0858878629742999));
#88914=CARTESIAN_POINT('',(0.0123177699812669,-0.0351951371328746,0.0780855547809824));
#88915=CARTESIAN_POINT('Ctrl Pts',(0.0122409055071548,-0.0350241211494343,
0.0785145498756483));
#88916=CARTESIAN_POINT('Ctrl Pts',(0.0123010253921567,-0.0349144232818962,
0.0784578381900836));
#88917=CARTESIAN_POINT('Ctrl Pts',(0.0123600089907431,-0.0348045283579412,
0.0783998498388591));
#88918=CARTESIAN_POINT('Ctrl Pts',(0.0124177779884474,-0.0346945769439157,
0.0783406562862751));
#88919=CARTESIAN_POINT('Ctrl Pts',(0.0122373329094135,-0.0350241211494343,
0.0784012874443269));
#88920=CARTESIAN_POINT('Ctrl Pts',(0.0122958926508634,-0.0349144232818962,
0.0783446249698312));
#88921=CARTESIAN_POINT('Ctrl Pts',(0.0123533161893045,-0.0348045283579412,
0.0782867181084131));
#88922=CARTESIAN_POINT('Ctrl Pts',(0.0124095272123934,-0.0346945769439157,
0.0782276382943536));
#88923=CARTESIAN_POINT('Ctrl Pts',(0.0122337603116722,-0.0350241211494343,
0.0782880250130055));
#88924=CARTESIAN_POINT('Ctrl Pts',(0.01229075990957,-0.0349144232818962,
0.0782314117495789));
#88925=CARTESIAN_POINT('Ctrl Pts',(0.0123466233878659,-0.0348045283579412,
0.078173586377967));
#88926=CARTESIAN_POINT('Ctrl Pts',(0.0124012764363395,-0.0346945769439157,
0.0781146203024321));
#88927=CARTESIAN_POINT('Ctrl Pts',(0.0122301877139309,-0.0350241211494343,
0.078174762581684));
#88928=CARTESIAN_POINT('Ctrl Pts',(0.0122856271682766,-0.0349144232818962,
0.0781181985293265));
#88929=CARTESIAN_POINT('Ctrl Pts',(0.0123399305864274,-0.0348045283579412,
0.0780604546475209));
#88930=CARTESIAN_POINT('Ctrl Pts',(0.0123930256602855,-0.0346945769439157,
0.0780016023105106));
#88931=CARTESIAN_POINT('',(0.0124054756374125,-0.0346945769458128,0.0781721405813361));
#88932=CARTESIAN_POINT('Ctrl Pts',(0.0124088168643448,-0.0347116136492768,
0.0783498187825369));
#88933=CARTESIAN_POINT('Ctrl Pts',(0.0123781494962928,-0.034762154653141,
0.0783197612921692));
#88934=CARTESIAN_POINT('Ctrl Pts',(0.0123480213434412,-0.0348133084095223,
0.0782902322937043));
#88935=CARTESIAN_POINT('Ctrl Pts',(0.0122888183239445,-0.0349168561544567,
0.0782322066364244));
#88936=CARTESIAN_POINT('Ctrl Pts',(0.0122597669402842,-0.0349692089015915,
0.0782037329935917));
#88937=CARTESIAN_POINT('Ctrl Pts',(0.0122312439848286,-0.0350221583435001,
0.0781757772701851));
#88938=CARTESIAN_POINT('Ctrl Pts',(0.0123163070376437,-0.0351951371254971,
0.0780855694736824));
#88939=CARTESIAN_POINT('Ctrl Pts',(0.0123976724672537,-0.0350307338980969,
0.0779988916529992));
#88940=CARTESIAN_POINT('Ctrl Pts',(0.0124753858827252,-0.0348659306897824,
0.0779089249770034));
#88941=CARTESIAN_POINT('Ctrl Pts',(0.012317769981177,-0.0351951371254971,
0.0780855547809085));
#88942=CARTESIAN_POINT('Ctrl Pts',(0.0123991351070231,-0.0350307338980969,
0.0779988467147856));
#88943=CARTESIAN_POINT('Ctrl Pts',(0.0124768469689137,-0.0348659306897824,
0.0779088498317496));
#88944=CARTESIAN_POINT('Ctrl Pts',(0.0125629608421027,-0.0351951371254971,
0.078083092256691));
#88945=CARTESIAN_POINT('Ctrl Pts',(0.0126442750568056,-0.0350307338980969,
0.0779913150233564));
#88946=CARTESIAN_POINT('Ctrl Pts',(0.0127217265369057,-0.0348659306897824,
0.0778962554088947));
#88947=CARTESIAN_POINT('Origin',(0.0165002655538542,-0.0308609197411036,
0.0813866600107244));
#88948=CARTESIAN_POINT('',(0.0124246676682205,-0.0351951371254971,0.0780844811758722));
#88949=CARTESIAN_POINT('Origin',(0.00729963773095405,-0.0351840467441134,
0.0736250890021826));
#88950=CARTESIAN_POINT('Origin',(0.0176776632668949,-0.0352322613094349,
0.081353645914016));
#88951=CARTESIAN_POINT('',(0.0126268943305477,-0.0351951142564687,0.077727680206653));
#88952=CARTESIAN_POINT('',(0.0127023373764456,-0.0351951372916788,0.0776284094688718));
#88953=CARTESIAN_POINT('Origin',(0.00815708642437748,-0.0352875121843913,
0.0738110393723901));
#88954=CARTESIAN_POINT('Origin',(0.00252497855717473,-0.0298325076522683,
0.0791448561667019));
#88955=CARTESIAN_POINT('Origin',(0.0123983407151583,-0.0338733119721242,
0.0813593929882444));
#88956=CARTESIAN_POINT('Origin',(0.00812378219310841,-0.0315241814719618,
0.07415));
#88957=CARTESIAN_POINT('',(0.0102128016197025,-0.032210423332361,0.0797745886798604));
#88958=CARTESIAN_POINT('',(0.0102248110767376,-0.0321934096636183,0.0797701136670138));
#88959=CARTESIAN_POINT('Origin',(0.00498619218089495,-0.0326387250794343,
0.0640690356156492));
#88960=CARTESIAN_POINT('',(0.0102128016195757,-0.032176398030855,0.0797745886795186));
#88961=CARTESIAN_POINT('Origin',(0.00388023441440586,-0.0326386249069991,
0.0644865279611796));
#88962=CARTESIAN_POINT('',(0.0102007826323785,-0.0321934096636185,0.0797790380328533));
#88963=CARTESIAN_POINT('Origin',(0.00503047312598455,-0.0326386266482349,
0.0640593159491066));
#88964=CARTESIAN_POINT('Origin',(0.00392012137274927,-0.0326387236954171,
0.0644649790481927));
#88965=CARTESIAN_POINT('Origin',(0.00812378219310841,-0.0315241814719618,
0.07415));
#88966=CARTESIAN_POINT('',(0.0109012769640885,-0.0332121607144216,0.079468413558058));
#88967=CARTESIAN_POINT('',(0.010912630855329,-0.0331951640388587,0.079462468648306));
#88968=CARTESIAN_POINT('Origin',(0.00259264235951201,-0.0326413667686659,
0.0651939692242149));
#88969=CARTESIAN_POINT('',(0.0109012769642343,-0.0331781648281954,0.0794684135597341));
#88970=CARTESIAN_POINT('Origin',(0.00389130651643295,-0.032641209385684,
0.0645069026047347));
#88971=CARTESIAN_POINT('',(0.010889910402055,-0.0331951640388588,0.0794743342054824));
#88972=CARTESIAN_POINT('Origin',(0.00262859804245172,-0.0326412092525031,
0.0651663415884814));
#88973=CARTESIAN_POINT('Origin',(0.00393452553582239,-0.0326413669275042,
0.0644931830535462));
#88974=CARTESIAN_POINT('Origin',(0.00812378219310841,-0.0315241814719618,
0.07415));
#88975=CARTESIAN_POINT('',(0.0105618502623162,-0.0327114338380043,0.0796323192236207));
#88976=CARTESIAN_POINT('',(0.0105735550331357,-0.0326943950436593,0.0796270989613361));
#88977=CARTESIAN_POINT('Origin',(0.00372745508006589,-0.0326395683095568,
0.0644994038884998));
#88978=CARTESIAN_POINT('',(0.0105618502623353,-0.0326773559991214,0.0796323192236637));
#88979=CARTESIAN_POINT('Origin',(0.0038603443629257,-0.0326395671738251,
0.0644394545930779));
#88980=CARTESIAN_POINT('',(0.0105501343689866,-0.0326943950436594,0.0796375144754808));
#88981=CARTESIAN_POINT('Origin',(0.00376853268769228,-0.0326395670095084,
0.0644802850492608));
#88982=CARTESIAN_POINT('Origin',(0.00390205414765034,-0.0326395685694152,
0.0644217576004931));
#88983=CARTESIAN_POINT('Ctrl Pts',(0.00997439487967158,-0.0327445246967097,
0.0795954896643306));
#88984=CARTESIAN_POINT('Ctrl Pts',(0.0101797748798699,-0.032443687833936,
0.0795256926658306));
#88985=CARTESIAN_POINT('Ctrl Pts',(0.0103793140219879,-0.0321434074405927,
0.0794406238922183));
#88986=CARTESIAN_POINT('Ctrl Pts',(0.0102092951270713,-0.0327445246967097,
0.0795099217160583));
#88987=CARTESIAN_POINT('Ctrl Pts',(0.0104114478793422,-0.032443687833936,
0.0794312653098958));
#88988=CARTESIAN_POINT('Ctrl Pts',(0.0106071016150094,-0.0321434074405927,
0.0793376053867665));
#88989=CARTESIAN_POINT('',(0.0102429380749441,-0.0326943950436612,0.0794967095814606));
#88990=CARTESIAN_POINT('',(0.0104608161269541,-0.0323666188837389,0.0794051305780213));
#88991=CARTESIAN_POINT('Origin',(0.00397814613099812,-0.0326395579111258,
0.0638966954752427));
#88992=CARTESIAN_POINT('Origin',(0.0149487344831154,-0.0321933825602998,
0.0894968083710972));
#88993=CARTESIAN_POINT('',(0.0103460491034406,-0.032193409653269,0.0794546823445082));
#88994=CARTESIAN_POINT('',(0.0104031565980373,-0.0321934096584275,0.0794292858013028));
#88995=CARTESIAN_POINT('',(0.0101262321451377,-0.0325210109756239,0.0795415043531114));
#88996=CARTESIAN_POINT('Origin',(0.00443386070631231,-0.0326393129158185,
0.0637433701488976));
#88997=CARTESIAN_POINT('',(0.0101257591440836,-0.0326943950436593,0.0795402308195257));
#88998=CARTESIAN_POINT('Origin',(0.0139773724095966,-0.0326943765538131,
0.0899105245446342));
#88999=CARTESIAN_POINT('',(0.0101843486095239,-0.0326943950436702,0.0795184702005032));
#89000=CARTESIAN_POINT('Ctrl Pts',(0.00999073073834982,-0.0325229783203769,
0.0798521489922192));
#89001=CARTESIAN_POINT('Ctrl Pts',(0.0100693347375098,-0.032413025309245,
0.0798264131473505));
#89002=CARTESIAN_POINT('Ctrl Pts',(0.0101473944358221,-0.032303122220807,
0.0797990551811304));
#89003=CARTESIAN_POINT('Ctrl Pts',(0.0102248110809361,-0.0321934096576658,
0.0797701136654483));
#89004=CARTESIAN_POINT('Ctrl Pts',(0.0100357229730105,-0.0325229783203769,
0.0797481449487558));
#89005=CARTESIAN_POINT('Ctrl Pts',(0.0101128932787057,-0.032413025309245,
0.0797217888869163));
#89006=CARTESIAN_POINT('Ctrl Pts',(0.0101895066710162,-0.032303122220807,
0.0796938404555844));
#89007=CARTESIAN_POINT('Ctrl Pts',(0.0102654662768954,-0.0321934096576658,
0.0796643389176207));
#89008=CARTESIAN_POINT('Ctrl Pts',(0.0100807152076711,-0.0325229783203769,
0.0796441409052925));
#89009=CARTESIAN_POINT('Ctrl Pts',(0.0101564518199016,-0.032413025309245,
0.0796171646264821));
#89010=CARTESIAN_POINT('Ctrl Pts',(0.0102316189062103,-0.032303122220807,
0.0795886257300383));
#89011=CARTESIAN_POINT('Ctrl Pts',(0.0103061214728548,-0.0321934096576658,
0.0795585641697932));
#89012=CARTESIAN_POINT('Ctrl Pts',(0.0101257074423317,-0.0325229783203769,
0.0795401368618291));
#89013=CARTESIAN_POINT('Ctrl Pts',(0.0102000103610976,-0.032413025309245,
0.0795125403660479));
#89014=CARTESIAN_POINT('Ctrl Pts',(0.0102737311414044,-0.032303122220807,
0.0794834110044923));
#89015=CARTESIAN_POINT('Ctrl Pts',(0.0103467766688141,-0.0321934096576658,
0.0794527894219656));
#89016=CARTESIAN_POINT('',(0.0102854300896961,-0.0321934096584275,0.0796123980060863));
#89017=CARTESIAN_POINT('Ctrl Pts',(0.0102128016184853,-0.0322104233328928,
0.0797745886765923));
#89018=CARTESIAN_POINT('Ctrl Pts',(0.0101978383033872,-0.0322609421830893,
0.0797343006392277));
#89019=CARTESIAN_POINT('Ctrl Pts',(0.0101831442528801,-0.032312088823975,
0.0796947375843842));
#89020=CARTESIAN_POINT('Ctrl Pts',(0.0101542817150667,-0.0324156524631818,
0.0796170265294315));
#89021=CARTESIAN_POINT('Ctrl Pts',(0.0101401250918172,-0.032468026716731,
0.0795789104727493));
#89022=CARTESIAN_POINT('Ctrl Pts',(0.0101262321451267,-0.0325210109755912,
0.0795415043530692));
#89023=CARTESIAN_POINT('Origin',(0.00047196380965428,-0.0262834582510976,
0.0759811366053846));
#89024=CARTESIAN_POINT('Origin',(0.00681081577538088,-0.0342770849357031,
0.0862371777635268));
#89025=CARTESIAN_POINT('Ctrl Pts',(0.0102410947514925,-0.0326943950436604,
0.0794958646853215));
#89026=CARTESIAN_POINT('Ctrl Pts',(0.0103147707860745,-0.0325844576448134,
0.0794666841500003));
#89027=CARTESIAN_POINT('Ctrl Pts',(0.0103878485335113,-0.0324744968375322,
0.0794359778083386));
#89028=CARTESIAN_POINT('Ctrl Pts',(0.0104602349049862,-0.0323646534831894,
0.0794037862945516));
#89029=CARTESIAN_POINT('Ctrl Pts',(0.0103441079573282,-0.0326943950436604,
0.0795430812820435));
#89030=CARTESIAN_POINT('Ctrl Pts',(0.0104184347251064,-0.0325844576448134,
0.0795124810316786));
#89031=CARTESIAN_POINT('Ctrl Pts',(0.010492133889758,-0.0324744968375322,
0.0794803414162683));
#89032=CARTESIAN_POINT('Ctrl Pts',(0.0105651115915997,-0.0323646534831894,
0.0794467049174037));
#89033=CARTESIAN_POINT('Ctrl Pts',(0.010447121163164,-0.0326943950436604,
0.0795902978787655));
#89034=CARTESIAN_POINT('Ctrl Pts',(0.0105220986641383,-0.0325844576448134,
0.0795582779133568));
#89035=CARTESIAN_POINT('Ctrl Pts',(0.0105964192460048,-0.0324744968375322,
0.079524705024198));
#89036=CARTESIAN_POINT('Ctrl Pts',(0.0106699882782133,-0.0323646534831894,
0.0794896235402558));
#89037=CARTESIAN_POINT('Ctrl Pts',(0.0105501343689998,-0.0326943950436604,
0.0796375144754875));
#89038=CARTESIAN_POINT('Ctrl Pts',(0.0106257626031702,-0.0325844576448134,
0.079604074795035));
#89039=CARTESIAN_POINT('Ctrl Pts',(0.0107007046022515,-0.0324744968375322,
0.0795690686321276));
#89040=CARTESIAN_POINT('Ctrl Pts',(0.0107748649648269,-0.0323646534831894,
0.079532542163108));
#89041=CARTESIAN_POINT('Ctrl Pts',(0.0105618502609686,-0.0326773559987509,
0.079632319220597));
#89042=CARTESIAN_POINT('Ctrl Pts',(0.0105443963626624,-0.0326267922587325,
0.0795930718167121));
#89043=CARTESIAN_POINT('Ctrl Pts',(0.0105272518220983,-0.0325756109582045,
0.079554520044716));
#89044=CARTESIAN_POINT('Ctrl Pts',(0.0104935668654355,-0.0324719985462386,
0.0794787749546622));
#89045=CARTESIAN_POINT('Ctrl Pts',(0.0104770399595816,-0.0324196091621784,
0.0794416120161806));
#89046=CARTESIAN_POINT('Ctrl Pts',(0.0104608161269342,-0.0323666188837756,
0.0794051305779768));
#89047=CARTESIAN_POINT('',(0.0103965362219753,-0.0326943950436703,0.0795671120284807));
#89048=CARTESIAN_POINT('Ctrl Pts',(0.0103104138834163,-0.0332451089994434,
0.0794695298759328));
#89049=CARTESIAN_POINT('Ctrl Pts',(0.0105110432351552,-0.0329451141710254,
0.0793870597124503));
#89050=CARTESIAN_POINT('Ctrl Pts',(0.0107048906302263,-0.0326442513127493,
0.0792897116150461));
#89051=CARTESIAN_POINT('Ctrl Pts',(0.0103127045152811,-0.0332451089994434,
0.0794685283742304));
#89052=CARTESIAN_POINT('Ctrl Pts',(0.0105132960947654,-0.0329451141710254,
0.0793859718181537));
#89053=CARTESIAN_POINT('Ctrl Pts',(0.0107070993174453,-0.0326442513127493,
0.0792885404187481));
#89054=CARTESIAN_POINT('Ctrl Pts',(0.0105417677017643,-0.0332451089994434,
0.0793683782039951));
#89055=CARTESIAN_POINT('Ctrl Pts',(0.0107385820557795,-0.0329451141710254,
0.0792771823884944));
#89056=CARTESIAN_POINT('Ctrl Pts',(0.0109279680393519,-0.0326442513127493,
0.0791714207889529));
#89057=CARTESIAN_POINT('Ctrl Pts',(0.0105440812399477,-0.0332451089994434,
0.0793673666872757));
#89058=CARTESIAN_POINT('Ctrl Pts',(0.0107408574439857,-0.0329451141710254,
0.0792760836152549));
#89059=CARTESIAN_POINT('Ctrl Pts',(0.0109301988134431,-0.0326442513127493,
0.079170237880692));
#89060=CARTESIAN_POINT('',(0.0105744790772793,-0.0331951640388616,0.0793530961726568));
#89061=CARTESIAN_POINT('',(0.010786176918691,-0.0328677532355045,0.0792480172023093));
#89062=CARTESIAN_POINT('Origin',(0.00274393348338891,-0.0326402808279978,
0.0645303162996148));
#89063=CARTESIAN_POINT('Origin',(0.0159044919433389,-0.0326944278779235,
0.08904787609129));
#89064=CARTESIAN_POINT('',(0.0106747477336384,-0.0326943950436593,0.0793046774691565));
#89065=CARTESIAN_POINT('',(0.0107301478748956,-0.0326943950436694,0.0792757452319597));
#89066=CARTESIAN_POINT('',(0.0104608161269515,-0.0330220786163546,0.0794051305780225));
#89067=CARTESIAN_POINT('Origin',(0.0031546461841902,-0.0326396682763683,
0.0642803808623885));
#89068=CARTESIAN_POINT('',(0.0104602640934199,-0.0331951640388588,0.079403889257447));
#89069=CARTESIAN_POINT('Origin',(0.0149429170789886,-0.0331952026560129,
0.0894837301171005));
#89070=CARTESIAN_POINT('',(0.0105173715853596,-0.0331951640388701,0.0793784927150619));
#89071=CARTESIAN_POINT('Ctrl Pts',(0.0103450885321277,-0.0330240426238172,
0.0797236700788876));
#89072=CARTESIAN_POINT('Ctrl Pts',(0.010421871267628,-0.032914277406352,
0.0796930694199537));
#89073=CARTESIAN_POINT('Ctrl Pts',(0.0104980596810234,-0.0328043479726691,
0.0796608661918505));
#89074=CARTESIAN_POINT('Ctrl Pts',(0.010573555033134,-0.0326943950436593,
0.0796270989613414));
#89075=CARTESIAN_POINT('Ctrl Pts',(0.0103834614905519,-0.0330240426238172,
0.0796170461976671));
#89076=CARTESIAN_POINT('Ctrl Pts',(0.0104587753782098,-0.032914277406352,
0.0795859169138459));
#89077=CARTESIAN_POINT('Ctrl Pts',(0.0105334832833355,-0.0328043479726691,
0.0795532151625046));
#89078=CARTESIAN_POINT('Ctrl Pts',(0.0106074883458023,-0.0326943950436593,
0.0795189802012852));
#89079=CARTESIAN_POINT('Ctrl Pts',(0.0104218344489761,-0.0330240426238172,
0.0795104223164465));
#89080=CARTESIAN_POINT('Ctrl Pts',(0.0104956794887916,-0.032914277406352,
0.0794787644077381));
#89081=CARTESIAN_POINT('Ctrl Pts',(0.0105689068856476,-0.0328043479726691,
0.0794455641331588));
#89082=CARTESIAN_POINT('Ctrl Pts',(0.0106414216584705,-0.0326943950436593,
0.0794108614412289));
#89083=CARTESIAN_POINT('Ctrl Pts',(0.0104602074074004,-0.0330240426238172,
0.079403798435226));
#89084=CARTESIAN_POINT('Ctrl Pts',(0.0105325835993734,-0.032914277406352,
0.0793716119016304));
#89085=CARTESIAN_POINT('Ctrl Pts',(0.0106043304879597,-0.0328043479726691,
0.0793379131038129));
#89086=CARTESIAN_POINT('Ctrl Pts',(0.0106753549711388,-0.0326943950436593,
0.0793027426811726));
#89087=CARTESIAN_POINT('',(0.010624151383397,-0.0326943950436693,0.0794658882152563));
#89088=CARTESIAN_POINT('Ctrl Pts',(0.010561850260963,-0.0327114338383315,
0.0796323192205846));
#89089=CARTESIAN_POINT('Ctrl Pts',(0.010544399265784,-0.0327619876830508,
0.0795930783447659));
#89090=CARTESIAN_POINT('Ctrl Pts',(0.0105272561432298,-0.0328131562603382,
0.079554529761353));
#89091=CARTESIAN_POINT('Ctrl Pts',(0.0104935712175586,-0.0329167375858771,
0.0794787847409879));
#89092=CARTESIAN_POINT('Ctrl Pts',(0.0104770428362969,-0.0329691088920626,
0.0794416184848567));
#89093=CARTESIAN_POINT('Ctrl Pts',(0.0104608161269346,-0.0330220786163188,
0.079405130577978));
#89094=CARTESIAN_POINT('Ctrl Pts',(0.0105725860375645,-0.0331951640388604,
0.079352368570823));
#89095=CARTESIAN_POINT('Ctrl Pts',(0.0106801416723178,-0.0330306422010619,
0.0793017411213658));
#89096=CARTESIAN_POINT('Ctrl Pts',(0.0107855129158078,-0.0328657861914644,
0.079246711545217));
#89097=CARTESIAN_POINT('Ctrl Pts',(0.0105744790772765,-0.0331951640388604,
0.0793530961726581));
#89098=CARTESIAN_POINT('Ctrl Pts',(0.0106820497547313,-0.0330306422010619,
0.0793024295858185));
#89099=CARTESIAN_POINT('Ctrl Pts',(0.0107874344104796,-0.0328657861914644,
0.0792473602839994));
#89100=CARTESIAN_POINT('Ctrl Pts',(0.0108899104020711,-0.0331951640388604,
0.0794743342054896));
#89101=CARTESIAN_POINT('Ctrl Pts',(0.0109999875981241,-0.0330306422010619,
0.0794171462782456));
#89102=CARTESIAN_POINT('Ctrl Pts',(0.0111076070968112,-0.0328657861914644,
0.0793554576114121));
#89103=CARTESIAN_POINT('Ctrl Pts',(0.0109012769624029,-0.033178164828644,
0.0794684135594792));
#89104=CARTESIAN_POINT('Ctrl Pts',(0.0108813794405278,-0.0331276811546772,
0.0794303133338342));
#89105=CARTESIAN_POINT('Ctrl Pts',(0.0108618411763031,-0.0330765663497778,
0.0793929010959286));
#89106=CARTESIAN_POINT('Ctrl Pts',(0.0108234665200749,-0.0329730614462884,
0.0793194203768333));
#89107=CARTESIAN_POINT('Ctrl Pts',(0.0108046456353499,-0.0329207133373271,
0.0792833815777759));
#89108=CARTESIAN_POINT('Ctrl Pts',(0.0107861769103332,-0.0328677532289398,
0.079248017216505));
#89109=CARTESIAN_POINT('',(0.0107321947396771,-0.0331951640388701,0.0794137151890796));
#89110=CARTESIAN_POINT('Ctrl Pts',(0.0106734180977772,-0.033693872113265,
0.0793053718598066));
#89111=CARTESIAN_POINT('Ctrl Pts',(0.0107813411936073,-0.0335278710435226,
0.0792519975140652));
#89112=CARTESIAN_POINT('Ctrl Pts',(0.0108875525167375,-0.0333620469224385,
0.0791952575050686));
#89113=CARTESIAN_POINT('Ctrl Pts',(0.0109920954511926,-0.0331951640388587,
0.0791351059479975));
#89114=CARTESIAN_POINT('Ctrl Pts',(0.0107477281647204,-0.033693872113265,
0.0792665640799846));
#89115=CARTESIAN_POINT('Ctrl Pts',(0.0108548388544128,-0.0335278710435226,
0.0792116341194991));
#89116=CARTESIAN_POINT('Ctrl Pts',(0.0109601892735341,-0.0333620469224385,
0.0791533645198656));
#89117=CARTESIAN_POINT('Ctrl Pts',(0.0110638221235362,-0.0331951640388587,
0.0790917087787543));
#89118=CARTESIAN_POINT('Ctrl Pts',(0.0108220382316635,-0.033693872113265,
0.0792277563001626));
#89119=CARTESIAN_POINT('Ctrl Pts',(0.0109283365152184,-0.0335278710435226,
0.0791712707249331));
#89120=CARTESIAN_POINT('Ctrl Pts',(0.0110328260303307,-0.0333620469224385,
0.0791114715346625));
#89121=CARTESIAN_POINT('Ctrl Pts',(0.0111355487958798,-0.0331951640388587,
0.079048311609511));
#89122=CARTESIAN_POINT('Ctrl Pts',(0.0108963482986067,-0.033693872113265,
0.0791889485203406));
#89123=CARTESIAN_POINT('Ctrl Pts',(0.0110018341760239,-0.0335278710435226,
0.0791309073303671));
#89124=CARTESIAN_POINT('Ctrl Pts',(0.0111054627871273,-0.0333620469224385,
0.0790695785494594));
#89125=CARTESIAN_POINT('Ctrl Pts',(0.0112072754682234,-0.0331951640388587,
0.0790049144402678));
#89126=CARTESIAN_POINT('',(0.0108963482986413,-0.0336938721132548,0.0791889485203216));
#89127=CARTESIAN_POINT('',(0.0111010304411501,-0.033367984620877,0.0790707843089641));
#89128=CARTESIAN_POINT('Ctrl Pts',(0.010896348298657,-0.0336938721132388,
0.079188948520342));
#89129=CARTESIAN_POINT('Ctrl Pts',(0.0109160176785375,-0.0336629187933905,
0.0791781258941925));
#89130=CARTESIAN_POINT('Ctrl Pts',(0.0109356173968631,-0.0336319952301045,
0.0791671915572488));
#89131=CARTESIAN_POINT('Ctrl Pts',(0.0110041484568814,-0.033523589259546,
0.0791284319404732));
#89132=CARTESIAN_POINT('Ctrl Pts',(0.0110527878648309,-0.0334458668645768,
0.0790999727380171));
#89133=CARTESIAN_POINT('Ctrl Pts',(0.0111010304285895,-0.0333679869902211,
0.0790707842881225));
#89134=CARTESIAN_POINT('Ctrl Pts',(0.0111010308214529,-0.0333679128829521,
0.0790707849399957));
#89135=CARTESIAN_POINT('Ctrl Pts',(0.0111007961598316,-0.0333391359256885,
0.0790703970921813));
#89136=CARTESIAN_POINT('Ctrl Pts',(0.0111006202934607,-0.033310357818173,
0.0790701064209276));
#89137=CARTESIAN_POINT('Ctrl Pts',(0.0111005030686477,-0.0332815781851602,
0.0790699126722103));
#89138=CARTESIAN_POINT('Ctrl Pts',(0.0111003857431915,-0.0332527738434303,
0.0790697187571504));
#89139=CARTESIAN_POINT('Ctrl Pts',(0.0111003271651869,-0.0332239691038149,
0.079069621939661));
#89140=CARTESIAN_POINT('Ctrl Pts',(0.0111003271651869,-0.0331951640388587,
0.079069621939661));
#89141=CARTESIAN_POINT('',(0.0109933788621512,-0.0331951640388587,0.079134329439054));
#89142=CARTESIAN_POINT('',(0.0110468530136792,-0.0331951640388687,0.0791019756893674));
#89143=CARTESIAN_POINT('',(0.0107861769034134,-0.0335216366558398,0.0792480172031858));
#89144=CARTESIAN_POINT('Origin',(0.00202357608885349,-0.0326434571527828,
0.0650851258327308));
#89145=CARTESIAN_POINT('',(0.0107855480161328,-0.0336938721132327,0.0792468129947429));
#89146=CARTESIAN_POINT('Origin',(0.0158408513303333,-0.0336938867896141,
0.0889268304697));
#89147=CARTESIAN_POINT('',(0.010840948157397,-0.0336938721132538,0.0792178807575423));
#89148=CARTESIAN_POINT('Ctrl Pts',(0.01069067980009,-0.0335235895815172,
0.0795731943239509));
#89149=CARTESIAN_POINT('Ctrl Pts',(0.0107653407472462,-0.0334144449262748,
0.0795378559246344));
#89150=CARTESIAN_POINT('Ctrl Pts',(0.0108393574060506,-0.0333049234473147,
0.079500934486799));
#89151=CARTESIAN_POINT('Ctrl Pts',(0.0109126308553275,-0.0331951640388587,
0.0794624686483122));
#89152=CARTESIAN_POINT('Ctrl Pts',(0.0107222820968345,-0.0335235895815172,
0.07946437122288));
#89153=CARTESIAN_POINT('Ctrl Pts',(0.0107954448797515,-0.0334144449262748,
0.0794285977557297));
#89154=CARTESIAN_POINT('Ctrl Pts',(0.0108679526649334,-0.0333049234473147,
0.0793912717011658));
#89155=CARTESIAN_POINT('Ctrl Pts',(0.0109397084137242,-0.0331951640388587,
0.0793524323892087));
#89156=CARTESIAN_POINT('Ctrl Pts',(0.0107538843935789,-0.0335235895815172,
0.0793555481218091));
#89157=CARTESIAN_POINT('Ctrl Pts',(0.0108255490122568,-0.0334144449262748,
0.0793193395868249));
#89158=CARTESIAN_POINT('Ctrl Pts',(0.0108965479238162,-0.0333049234473147,
0.0792816089155325));
#89159=CARTESIAN_POINT('Ctrl Pts',(0.0109667859721209,-0.0331951640388587,
0.0792423961301052));
#89160=CARTESIAN_POINT('Ctrl Pts',(0.0107854866903234,-0.0335235895815172,
0.0792467250207382));
#89161=CARTESIAN_POINT('Ctrl Pts',(0.010855653144762,-0.0334144449262748,
0.0792100814179201));
#89162=CARTESIAN_POINT('Ctrl Pts',(0.0109251431826991,-0.0333049234473147,
0.0791719461298993));
#89163=CARTESIAN_POINT('Ctrl Pts',(0.0109938635305176,-0.0331951640388587,
0.0791323598710018));
#89164=CARTESIAN_POINT('',(0.0109530048587501,-0.0331951640388687,0.07929839904369));
#89165=CARTESIAN_POINT('Ctrl Pts',(0.0109012769626324,-0.0332121607145966,
0.079468413555275));
#89166=CARTESIAN_POINT('Ctrl Pts',(0.010881412924295,-0.0332625444106898,
0.079430377418568));
#89167=CARTESIAN_POINT('Ctrl Pts',(0.0108618911745105,-0.0333135300740933,
0.0793929967041725));
#89168=CARTESIAN_POINT('Ctrl Pts',(0.0108235167555749,-0.0334167203138383,
0.079319516447042));
#89169=CARTESIAN_POINT('Ctrl Pts',(0.0108046789494215,-0.0334688847584559,
0.0792834453643316));
#89170=CARTESIAN_POINT('Ctrl Pts',(0.0107861769032448,-0.0335216366555605,
0.079248017202858));
#89171=CARTESIAN_POINT('Ctrl Pts',(0.0108963482986233,-0.0336938721132388,
0.0791889485203314));
#89172=CARTESIAN_POINT('Ctrl Pts',(0.0109258429364132,-0.0336474569764957,
0.0791727197708809));
#89173=CARTESIAN_POINT('Ctrl Pts',(0.0109551455752089,-0.033601104548885,
0.0791561468614595));
#89174=CARTESIAN_POINT('Ctrl Pts',(0.0110293331195408,-0.0334837508592656,
0.0791141880651553));
#89175=CARTESIAN_POINT('Ctrl Pts',(0.0111022447600412,-0.0333660264659097,
0.0790700493633073));
#89176=CARTESIAN_POINT('Ctrl Pts',(0.011220704319783,-0.0336938721132388,
0.0792907483770459));
#89177=CARTESIAN_POINT('Ctrl Pts',(0.0112507948259149,-0.0336474569764957,
0.0792726210641708));
#89178=CARTESIAN_POINT('Ctrl Pts',(0.0112806710671415,-0.033601104548885,
0.0792541427460243));
#89179=CARTESIAN_POINT('Ctrl Pts',(0.0113563108409488,-0.0334837508592656,
0.0792073598929091));
#89180=CARTESIAN_POINT('Ctrl Pts',(0.0114305311264073,-0.0333660264659097,
0.0791583562200499));
#89181=CARTESIAN_POINT('',(0.0112297421639733,-0.0336769361243754,0.079283518545733));
#89182=CARTESIAN_POINT('',(0.011218769790806,-0.033693872113232,0.0792901412208322));
#89183=CARTESIAN_POINT('Ctrl Pts',(0.0112297421639733,-0.0336769361243754,
0.079283518545733));
#89184=CARTESIAN_POINT('Ctrl Pts',(0.011227914477107,-0.0336797586669902,
0.0792846243608178));
#89185=CARTESIAN_POINT('Ctrl Pts',(0.0112260862688101,-0.0336825812712596,
0.0792857291580131));
#89186=CARTESIAN_POINT('Ctrl Pts',(0.011222428820045,-0.0336882265869416,
0.0792879367107729));
#89187=CARTESIAN_POINT('Ctrl Pts',(0.0112205995796331,-0.0336910492983079,
0.0792890394663461));
#89188=CARTESIAN_POINT('Ctrl Pts',(0.0112187697908194,-0.033693872113238,
0.0792901412208391));
#89189=CARTESIAN_POINT('Ctrl Pts',(0.0112297421639733,-0.0336769361243754,
0.079283518545733));
#89190=CARTESIAN_POINT('Ctrl Pts',(0.0112080455760862,-0.0336279018505222,
0.0792476585097562));
#89191=CARTESIAN_POINT('Ctrl Pts',(0.0111860368553374,-0.0335767826010775,
0.0792112825818021));
#89192=CARTESIAN_POINT('Ctrl Pts',(0.0111429124074254,-0.0334733172064619,
0.079140006662213));
#89193=CARTESIAN_POINT('Ctrl Pts',(0.0111217676971637,-0.0334209631456238,
0.0791050587674256));
#89194=CARTESIAN_POINT('Ctrl Pts',(0.0111010304244935,-0.033367986984468,
0.0790707842839039));
#89195=CARTESIAN_POINT('',(0.0110575590447336,-0.0336938721132534,0.0792395448705869));
#89196=CARTESIAN_POINT('Ctrl Pts',(0.0096636317672152,-0.0321934096636942,
0.0796913896295103));
#89197=CARTESIAN_POINT('Ctrl Pts',(0.00981230007270001,-0.0319797282160735,
0.0796500774601468));
#89198=CARTESIAN_POINT('Ctrl Pts',(0.00995853940576728,-0.0317669959606461,
0.0796008533008619));
#89199=CARTESIAN_POINT('Ctrl Pts',(0.00990303373244094,-0.0321934096636942,
0.0796192219702425));
#89200=CARTESIAN_POINT('Ctrl Pts',(0.0100497658731131,-0.0319797282160735,
0.0795714869562714));
#89201=CARTESIAN_POINT('Ctrl Pts',(0.010193727441266,-0.0317669959606461,
0.0795159530066551));
#89202=CARTESIAN_POINT('Ctrl Pts',(0.00990446994694649,-0.0321934096636942,
0.0796187890237586));
#89203=CARTESIAN_POINT('Ctrl Pts',(0.0100511904722253,-0.0319797282160735,
0.0795710154780128));
#89204=CARTESIAN_POINT('Ctrl Pts',(0.0101951383756658,-0.0317669959606461,
0.0795154436748543));
#89205=CARTESIAN_POINT('',(0.00990303373254501,-0.0321934096636942,0.0796192219702087));
#89206=CARTESIAN_POINT('',(0.010126232145142,-0.0318665617561286,0.0795415043531098));
#89207=CARTESIAN_POINT('Origin',(0.00532192722094431,-0.0326371944421877,
0.0635496430093242));
#89208=CARTESIAN_POINT('Origin',(0.0139425870835524,-0.0316939261509089,
0.0898168644506043));
#89209=CARTESIAN_POINT('',(0.00978398701925707,-0.0320197259213214,0.0796564807125462));
#89210=CARTESIAN_POINT('Ctrl Pts',(0.00978416991441515,-0.0320197391311199,
0.0796564733134607));
#89211=CARTESIAN_POINT('Ctrl Pts',(0.00981218862409361,-0.0319792715672864,
0.0796480247259767));
#89212=CARTESIAN_POINT('Ctrl Pts',(0.00984027045301016,-0.0319386438886474,
0.0796393239931166));
#89213=CARTESIAN_POINT('Ctrl Pts',(0.00986844231933618,-0.0318979098685815,
0.079630353953209));
#89214=CARTESIAN_POINT('Ctrl Pts',(0.00989661362870992,-0.0318571766538192,
0.0796213840906373));
#89215=CARTESIAN_POINT('Ctrl Pts',(0.00992473250423351,-0.0318163871807252,
0.079612192158285));
#89216=CARTESIAN_POINT('Ctrl Pts',(0.00995270322272097,-0.0317755399642118,
0.0796028133577372));
#89217=CARTESIAN_POINT('',(0.00978335330633817,-0.0321934096636185,0.0796552996031219));
#89218=CARTESIAN_POINT('Origin',(0.0103384426816057,-0.0323427921796758,
0.0814966990457025));
#89219=CARTESIAN_POINT('',(0.0098431935194516,-0.0321934096636664,0.0796372607866753));
#89220=CARTESIAN_POINT('Ctrl Pts',(0.00990124666418742,-0.0321934096636618,
0.0796182627652958));
#89221=CARTESIAN_POINT('Ctrl Pts',(0.00997665826943559,-0.0320835708272593,
0.0795937501449649));
#89222=CARTESIAN_POINT('Ctrl Pts',(0.0100515188454842,-0.0319739230346489,
0.0795676911036986));
#89223=CARTESIAN_POINT('Ctrl Pts',(0.0101257351722283,-0.0318646057455573,
0.0795401263329965));
#89224=CARTESIAN_POINT('Ctrl Pts',(0.0100010919869124,-0.0321934096636618,
0.0796718545211547));
#89225=CARTESIAN_POINT('Ctrl Pts',(0.0100772426642408,-0.0320835708272593,
0.0796459649560085));
#89226=CARTESIAN_POINT('Ctrl Pts',(0.0101528133878765,-0.0319739230346489,
0.0796185144735526));
#89227=CARTESIAN_POINT('Ctrl Pts',(0.0102277101657592,-0.0318646057455573,
0.0795895456152703));
#89228=CARTESIAN_POINT('Ctrl Pts',(0.0101009373096374,-0.0321934096636618,
0.0797254462770135));
#89229=CARTESIAN_POINT('Ctrl Pts',(0.0101778270590461,-0.0320835708272593,
0.0796981797670521));
#89230=CARTESIAN_POINT('Ctrl Pts',(0.0102541079302688,-0.0319739230346489,
0.0796693378434066));
#89231=CARTESIAN_POINT('Ctrl Pts',(0.0103296851592901,-0.0318646057455573,
0.0796389648975441));
#89232=CARTESIAN_POINT('Ctrl Pts',(0.0102007826323624,-0.0321934096636618,
0.0797790380328724));
#89233=CARTESIAN_POINT('Ctrl Pts',(0.0102784114538514,-0.0320835708272593,
0.0797503945780957));
#89234=CARTESIAN_POINT('Ctrl Pts',(0.0103554024726611,-0.0319739230346489,
0.0797201612132606));
#89235=CARTESIAN_POINT('Ctrl Pts',(0.0104316601528211,-0.0318646057455573,
0.0796883841798179));
#89236=CARTESIAN_POINT('Ctrl Pts',(0.0102128016184661,-0.0321763980306411,
0.0797745886765405));
#89237=CARTESIAN_POINT('Ctrl Pts',(0.010197858551582,-0.0321259596179381,
0.0797343551565603));
#89238=CARTESIAN_POINT('Ctrl Pts',(0.0101831743927205,-0.0320749164640418,
0.0796948187345174));
#89239=CARTESIAN_POINT('Ctrl Pts',(0.0101543120737603,-0.0319716057814256,
0.0796171082688167));
#89240=CARTESIAN_POINT('Ctrl Pts',(0.0101401451595835,-0.0319193786724667,
0.0795789645042865));
#89241=CARTESIAN_POINT('Ctrl Pts',(0.010126232145124,-0.0318665617561676,
0.0795415043530615));
#89242=CARTESIAN_POINT('',(0.0100519081824717,-0.0321934096636664,0.079699130001541));
#89243=CARTESIAN_POINT('Origin',(0.00812378219310841,-0.0315241814719618,
0.07415));
#89244=CARTESIAN_POINT('',(0.0112297421633088,-0.0337108120655389,0.0792835185446306));
#89245=CARTESIAN_POINT('',(0.0112407003659563,-0.0336938721132327,0.0792768724485572));
#89246=CARTESIAN_POINT('Origin',(0.0037164075845662,-0.0345562527130611,
0.0647065494387839));
#89247=CARTESIAN_POINT('Ctrl Pts',(0.0112407003659567,-0.0336938721132373,
0.0792768724485696));
#89248=CARTESIAN_POINT('Ctrl Pts',(0.011238875303069,-0.0336910493021816,
0.0792779820083915));
#89249=CARTESIAN_POINT('Ctrl Pts',(0.0112370496041514,-0.0336882265888785,
0.0792790906201662));
#89250=CARTESIAN_POINT('Ctrl Pts',(0.0112333968780567,-0.0336825812713059,
0.079281305981301));
#89251=CARTESIAN_POINT('Ctrl Pts',(0.0112315698508547,-0.0336797586670134,
0.0792824127306391));
#89252=CARTESIAN_POINT('Ctrl Pts',(0.0112297421639734,-0.0336769361243754,
0.079283518545733));
#89253=CARTESIAN_POINT('Origin',(0.00180399000269284,-0.0345562523252851,
0.0658636300553531));
#89254=CARTESIAN_POINT('Ctrl Pts',(0.0109619695376012,-0.0342436276873911,
0.0791522812393508));
#89255=CARTESIAN_POINT('Ctrl Pts',(0.0111506336847112,-0.033943005420181,
0.0790452372390105));
#89256=CARTESIAN_POINT('Ctrl Pts',(0.0113306988640532,-0.0336441434784052,
0.0789242863828657));
#89257=CARTESIAN_POINT('Ctrl Pts',(0.0111766759614705,-0.0342436276873911,
0.0790242142586365));
#89258=CARTESIAN_POINT('Ctrl Pts',(0.0113605099827772,-0.033943005420181,
0.0789090724720263));
#89259=CARTESIAN_POINT('Ctrl Pts',(0.0115351487997555,-0.0336441434784052,
0.0787804106594397));
#89260=CARTESIAN_POINT('Ctrl Pts',(0.0111788230257092,-0.0342436276873911,
0.0790229335888294));
#89261=CARTESIAN_POINT('Ctrl Pts',(0.0113626087457579,-0.033943005420181,
0.0789077108243564));
#89262=CARTESIAN_POINT('Ctrl Pts',(0.0115371932991125,-0.0336441434784052,
0.0787789719022055));
#89263=CARTESIAN_POINT('',(0.0112072754682234,-0.0341934961088741,0.0790049144402678));
#89264=CARTESIAN_POINT('',(0.0114041341081436,-0.0338664212862963,0.078874131276693));
#89265=CARTESIAN_POINT('Origin',(0.00266953802630421,-0.0345610720406482,
0.0646118541980884));
#89266=CARTESIAN_POINT('Origin',(0.0176588912847395,-0.0336938005072858,
0.0878817245803645));
#89267=CARTESIAN_POINT('',(0.0113006850036053,-0.0336938721132327,0.0789443105377789));
#89268=CARTESIAN_POINT('',(0.0113520221273582,-0.0336938721132427,0.0789086629610717));
#89269=CARTESIAN_POINT('',(0.011101030424489,-0.0340203938281605,0.0790707842839066));
#89270=CARTESIAN_POINT('Origin',(0.00311628593912468,-0.0345589643245431,
0.0644331000750157));
#89271=CARTESIAN_POINT('',(0.0111003271651873,-0.034193496108874,0.0790696219396609));
#89272=CARTESIAN_POINT('Origin',(0.0168046534788821,-0.0341934220717595,
0.0884977118607877));
#89273=CARTESIAN_POINT('',(0.0111538013167154,-0.0341934961088841,0.0790372681899744));
#89274=CARTESIAN_POINT('Ctrl Pts',(0.011026137408333,-0.0340223579322397,
0.0794013173780229));
#89275=CARTESIAN_POINT('Ctrl Pts',(0.0110985667709867,-0.0339125849573575,
0.0793612863299448));
#89276=CARTESIAN_POINT('Ctrl Pts',(0.0111701166886898,-0.0338030433565231,
0.0793197842917163));
#89277=CARTESIAN_POINT('Ctrl Pts',(0.0112407003659551,-0.0336938721132327,
0.0792768724485641));
#89278=CARTESIAN_POINT('Ctrl Pts',(0.0110508443436105,-0.0340223579322397,
0.0792907246694937));
#89279=CARTESIAN_POINT('Ctrl Pts',(0.0111217483443756,-0.0339125849573575,
0.0792503528483397));
#89280=CARTESIAN_POINT('Ctrl Pts',(0.0111917669188336,-0.0338030433565231,
0.0792085418479394));
#89281=CARTESIAN_POINT('Ctrl Pts',(0.0112608152648517,-0.0336938721132327,
0.0791653530750319));
#89282=CARTESIAN_POINT('Ctrl Pts',(0.0110755512788879,-0.0340223579322397,
0.0791801319609645));
#89283=CARTESIAN_POINT('Ctrl Pts',(0.0111449299177645,-0.0339125849573575,
0.0791394193667346));
#89284=CARTESIAN_POINT('Ctrl Pts',(0.0112134171489773,-0.0338030433565231,
0.0790972994041623));
#89285=CARTESIAN_POINT('Ctrl Pts',(0.0112809301637483,-0.0336938721132327,
0.0790538337014997));
#89286=CARTESIAN_POINT('Ctrl Pts',(0.0111002582141653,-0.0340223579322397,
0.0790695392524353));
#89287=CARTESIAN_POINT('Ctrl Pts',(0.0111681114911534,-0.0339125849573575,
0.0790284858851296));
#89288=CARTESIAN_POINT('Ctrl Pts',(0.011235067379121,-0.0338030433565231,
0.0789860569603853));
#89289=CARTESIAN_POINT('Ctrl Pts',(0.0113010450626449,-0.0336938721132327,
0.0789423143279675));
#89290=CARTESIAN_POINT('',(0.0112706926847908,-0.0336938721132427,0.0791105914931781));
#89291=CARTESIAN_POINT('Ctrl Pts',(0.0112297421614374,-0.0337108120662675,
0.0792835185415416));
#89292=CARTESIAN_POINT('Ctrl Pts',(0.0112074831667248,-0.0337611408993745,
0.0792467289617537));
#89293=CARTESIAN_POINT('Ctrl Pts',(0.0111856303492812,-0.0338121088780191,
0.0792106107101743));
#89294=CARTESIAN_POINT('Ctrl Pts',(0.011142717161275,-0.0339153382773236,
0.0791396839601347));
#89295=CARTESIAN_POINT('Ctrl Pts',(0.0111216749456874,-0.0339675558473115,
0.0791049054681465));
#89296=CARTESIAN_POINT('Ctrl Pts',(0.0111010304244729,-0.0340203938281304,
0.0790707842838698));
#89297=CARTESIAN_POINT('Ctrl Pts',(0.0112053060724886,-0.0341934961088741,
0.079004429814305));
#89298=CARTESIAN_POINT('Ctrl Pts',(0.011305667584522,-0.0340287516182428,
0.0789407217357598));
#89299=CARTESIAN_POINT('Ctrl Pts',(0.011403310236344,-0.0338644633275951,
0.078872920077117));
#89300=CARTESIAN_POINT('Ctrl Pts',(0.0112072754682234,-0.0341934961088741,
0.0790049144402679));
#89301=CARTESIAN_POINT('Ctrl Pts',(0.0113076469995168,-0.0340287516182428,
0.0789411656460174));
#89302=CARTESIAN_POINT('Ctrl Pts',(0.0114052979792265,-0.0338644633275951,
0.0788733228923564));
#89303=CARTESIAN_POINT('Ctrl Pts',(0.0115354146774924,-0.0341934961088741,
0.0790856624470942));
#89304=CARTESIAN_POINT('Ctrl Pts',(0.0116374556102127,-0.0340287516182428,
0.079015129633204));
#89305=CARTESIAN_POINT('Ctrl Pts',(0.0117364941761993,-0.0338644633275951,
0.0789404396590909));
#89306=CARTESIAN_POINT('',(0.011545949556832,-0.0341764758832445,0.0790783638791647));
#89307=CARTESIAN_POINT('',(0.0115354146774751,-0.034193496108874,0.0790856624470899));
#89308=CARTESIAN_POINT('Origin',(0.00252268601302544,-0.0345621026753412,
0.0651858463722302));
#89309=CARTESIAN_POINT('Ctrl Pts',(0.011545949555018,-0.0341764758837557,
0.0790783638793629));
#89310=CARTESIAN_POINT('Ctrl Pts',(0.0115214671429795,-0.0341260050040178,
0.0790431060617529));
#89311=CARTESIAN_POINT('Ctrl Pts',(0.0114974102616361,-0.0340749269147575,
0.0790084611299829));
#89312=CARTESIAN_POINT('Ctrl Pts',(0.011450129066672,-0.0339715436304948,
0.078940370083328));
#89313=CARTESIAN_POINT('Ctrl Pts',(0.0114269226954664,-0.0339192778237157,
0.0789069497973535));
#89314=CARTESIAN_POINT('Ctrl Pts',(0.0114041341077238,-0.0338664212855168,
0.0788741312782399));
#89315=CARTESIAN_POINT('',(0.0113713450728593,-0.0341934961088841,0.0790452884436889));
#89316=CARTESIAN_POINT('Origin',(0.00812378219310841,-0.0315241814719618,
0.07415));
#89317=CARTESIAN_POINT('',(0.0115459495571016,-0.0342105180190358,0.0790783638780777));
#89318=CARTESIAN_POINT('',(0.0115564688245398,-0.0341934961088739,0.079071042825499));
#89319=CARTESIAN_POINT('Origin',(0.00248272241089273,-0.0345621722253858,
0.0652072295348258));
#89320=CARTESIAN_POINT('Origin',(0.00168141573312356,-0.0345621027514389,
0.0657700090192215));
#89321=CARTESIAN_POINT('Origin',(0.00171541396284715,-0.0345621725656518,
0.0657400355638129));
#89322=CARTESIAN_POINT('Ctrl Pts',(0.0112994529044899,-0.0346945769586965,
0.078945166085276));
#89323=CARTESIAN_POINT('Ctrl Pts',(0.0113998895780257,-0.0345275153362944,
0.0788786503907569));
#89324=CARTESIAN_POINT('Ctrl Pts',(0.0114982603722607,-0.0343603235965185,
0.0788089588509352));
#89325=CARTESIAN_POINT('Ctrl Pts',(0.0115942774134824,-0.0341934961088739,
0.078736301906533));
#89326=CARTESIAN_POINT('Ctrl Pts',(0.0113683131029715,-0.0346945769586965,
0.0788973508001731));
#89327=CARTESIAN_POINT('Ctrl Pts',(0.0114677482662167,-0.0345275153362944,
0.0788293928012267));
#89328=CARTESIAN_POINT('Ctrl Pts',(0.0115650719319724,-0.0343603235965185,
0.0787582900805006));
#89329=CARTESIAN_POINT('Ctrl Pts',(0.0116599993854989,-0.0341934961088739,
0.0786842572063352));
#89330=CARTESIAN_POINT('Ctrl Pts',(0.0114371733014532,-0.0346945769586965,
0.0788495355150717));
#89331=CARTESIAN_POINT('Ctrl Pts',(0.0115356069544074,-0.0345275153362944,
0.078780135211697));
#89332=CARTESIAN_POINT('Ctrl Pts',(0.0116318834916838,-0.0343603235965185,
0.0787076213100663));
#89333=CARTESIAN_POINT('Ctrl Pts',(0.0117257213575149,-0.0341934961088739,
0.078632212506138));
#89334=CARTESIAN_POINT('Ctrl Pts',(0.0115060334999348,-0.0346945769586965,
0.0788017202299672));
#89335=CARTESIAN_POINT('Ctrl Pts',(0.0116034656425987,-0.0345275153362944,
0.0787308776221661));
#89336=CARTESIAN_POINT('Ctrl Pts',(0.0116986950513959,-0.0343603235965185,
0.0786569525396315));
#89337=CARTESIAN_POINT('Ctrl Pts',(0.0117914433295318,-0.0341934961088739,
0.0785801678059397));
#89338=CARTESIAN_POINT('',(0.0115060334985815,-0.0346945769586966,0.0788017202309067));
#89339=CARTESIAN_POINT('',(0.0116942917394192,-0.0343667727836579,0.07865883428183));
#89340=CARTESIAN_POINT('Origin',(0.00147091532982184,-0.0345626474181511,
0.0653112180668012));
#89341=CARTESIAN_POINT('Origin',(0.0185556194816323,-0.0341934771024039,
0.0873232926903192));
#89342=CARTESIAN_POINT('',(0.0115954533610552,-0.0341934961088739,0.0787353706831235));
#89343=CARTESIAN_POINT('',(0.0116444508528592,-0.0341934961088841,0.0786965699640951));
#89344=CARTESIAN_POINT('',(0.0114041341068758,-0.0345211942962608,0.0788741312769521));
#89345=CARTESIAN_POINT('Origin',(0.00186774519205461,-0.0345625596119161,
0.0650397137992776));
#89346=CARTESIAN_POINT('',(0.0114033592510911,-0.0346945769586886,0.0788730153843444));
#89347=CARTESIAN_POINT('Origin',(0.0177135881722783,-0.0346945685853921,
0.0879605632483003));
#89348=CARTESIAN_POINT('',(0.0114546963748463,-0.0346945769587026,0.0788373678076356));
#89349=CARTESIAN_POINT('Ctrl Pts',(0.011350144030904,-0.0345231616327842,
0.0792087141935167));
#89350=CARTESIAN_POINT('Ctrl Pts',(0.0114198712839617,-0.0344132092796988,
0.0791642433379369));
#89351=CARTESIAN_POINT('Ctrl Pts',(0.0114886750948442,-0.0343032738558979,
0.0791183325236193));
#89352=CARTESIAN_POINT('Ctrl Pts',(0.011556468824539,-0.0341934961088739,
0.0790710428255065));
#89353=CARTESIAN_POINT('Ctrl Pts',(0.0113678579909793,-0.0345231616327842,
0.079096788540705));
#89354=CARTESIAN_POINT('Ctrl Pts',(0.0114360425064917,-0.0344132092796988,
0.0790520735231247));
#89355=CARTESIAN_POINT('Ctrl Pts',(0.0115032986091287,-0.0343032738558979,
0.0790059504697136));
#89356=CARTESIAN_POINT('Ctrl Pts',(0.0115695416496358,-0.0341934961088739,
0.078958480676527));
#89357=CARTESIAN_POINT('Ctrl Pts',(0.0113855719510546,-0.0345231616327842,
0.0789848628878932));
#89358=CARTESIAN_POINT('Ctrl Pts',(0.0114522137290217,-0.0344132092796988,
0.0789399037083125));
#89359=CARTESIAN_POINT('Ctrl Pts',(0.0115179221234131,-0.0343032738558979,
0.078893568415808));
#89360=CARTESIAN_POINT('Ctrl Pts',(0.0115826144747325,-0.0341934961088739,
0.0788459185275475));
#89361=CARTESIAN_POINT('Ctrl Pts',(0.0114032859111299,-0.0345231616327842,
0.0788729372350814));
#89362=CARTESIAN_POINT('Ctrl Pts',(0.0114683849515517,-0.0344132092796988,
0.0788277338935004));
#89363=CARTESIAN_POINT('Ctrl Pts',(0.0115325456376976,-0.0343032738558979,
0.0787811863619023));
#89364=CARTESIAN_POINT('Ctrl Pts',(0.0115956872998293,-0.0341934961088739,
0.0787333563785681));
#89365=CARTESIAN_POINT('',(0.0115759610928075,-0.0341934961088839,0.0789032067543212));
#89366=CARTESIAN_POINT('Ctrl Pts',(0.0115459495551251,-0.0342105180195371,
0.0790783638752337));
#89367=CARTESIAN_POINT('Ctrl Pts',(0.0115214396314411,-0.0342610556240559,
0.079043066413219));
#89368=CARTESIAN_POINT('Ctrl Pts',(0.0114973695256638,-0.0343122189868635,
0.0790084023459081));
#89369=CARTESIAN_POINT('Ctrl Pts',(0.0114500878504123,-0.0344158119695081,
0.0789403106146687));
#89370=CARTESIAN_POINT('Ctrl Pts',(0.0114268956195889,-0.0344681990449949,
0.0789069108009003));
#89371=CARTESIAN_POINT('Ctrl Pts',(0.0114041341068571,-0.0345211942962355,
0.0788741312769241));
#89372=CARTESIAN_POINT('Ctrl Pts',(0.0115040380481517,-0.0346945769586932,
0.0788013603088443));
#89373=CARTESIAN_POINT('Ctrl Pts',(0.0116002016312185,-0.0345296777079064,
0.0787314759109219));
#89374=CARTESIAN_POINT('Ctrl Pts',(0.0116933946573247,-0.0343648066255587,
0.0786576766990943));
#89375=CARTESIAN_POINT('Ctrl Pts',(0.0115060334985741,-0.0346945769586932,
0.0788017202309119));
#89376=CARTESIAN_POINT('Ctrl Pts',(0.011602204522775,-0.0345296777079064,
0.078731794578464));
#89377=CARTESIAN_POINT('Ctrl Pts',(0.0116954032785695,-0.0343648066255587,
0.0786579538398135));
#89378=CARTESIAN_POINT('Ctrl Pts',(0.0118385954093691,-0.0346945769586932,
0.0788617048685642));
#89379=CARTESIAN_POINT('Ctrl Pts',(0.0119360065735081,-0.0345296777079064,
0.0787849037339326));
#89380=CARTESIAN_POINT('Ctrl Pts',(0.0120301602395604,-0.0343648066255587,
0.0787041421319887));
#89381=CARTESIAN_POINT('',(0.0118486512198862,-0.034677539666503,0.0788537592122609));
#89382=CARTESIAN_POINT('',(0.0118385954093546,-0.0346945769586886,0.078861704868559));
#89383=CARTESIAN_POINT('Origin',(0.00142290311163744,-0.0345626617986891,
0.065934135429138));
#89384=CARTESIAN_POINT('Ctrl Pts',(0.0118486512180685,-0.0346775396670096,
0.0788537592124665));
#89385=CARTESIAN_POINT('Ctrl Pts',(0.0118219822728979,-0.0346269749928757,
0.0788200817278928));
#89386=CARTESIAN_POINT('Ctrl Pts',(0.0117957872662314,-0.0345757902891947,
0.0787870027896662));
#89387=CARTESIAN_POINT('Ctrl Pts',(0.0117443236918964,-0.0344721681090353,
0.0787220146564573));
#89388=CARTESIAN_POINT('Ctrl Pts',(0.0117190753047894,-0.0344197714292724,
0.0786901309363811));
#89389=CARTESIAN_POINT('Ctrl Pts',(0.0116942917391319,-0.03436677278343,
0.0786588342824434));
#89390=CARTESIAN_POINT('',(0.011672314453978,-0.0346945769587026,0.0788317125497428));
#89391=CARTESIAN_POINT('Origin',(0.00812378219310841,-0.0315241814719618,
0.07415));
#89392=CARTESIAN_POINT('',(0.0118486512197319,-0.0347116136489784,0.0788537592108763));
#89393=CARTESIAN_POINT('',(0.0118586900372345,-0.0346945769586885,0.0788457920946193));
#89394=CARTESIAN_POINT('Origin',(0.00138857391637728,-0.0345626704533082,
0.0659637084523159));
#89395=CARTESIAN_POINT('Origin',(0.00166235086465093,-0.0345626619289644,
0.0657445183313168));
#89396=CARTESIAN_POINT('Origin',(0.00169900477058736,-0.0345626705785499,
0.0657178809380879));
#89397=CARTESIAN_POINT('Ctrl Pts',(0.0115646152496605,-0.0352450361874068,
0.0787586256630979));
#89398=CARTESIAN_POINT('Ctrl Pts',(0.0117384324187514,-0.0349452760959493,
0.0786288525148916));
#89399=CARTESIAN_POINT('Ctrl Pts',(0.0119019807470506,-0.034644428984174,
0.078486355418161));
#89400=CARTESIAN_POINT('Ctrl Pts',(0.011566604548178,-0.0352450361874068,
0.0787570705694002));
#89401=CARTESIAN_POINT('Ctrl Pts',(0.0117403630659476,-0.0349452760959493,
0.0786272223935692));
#89402=CARTESIAN_POINT('Ctrl Pts',(0.0119038472581602,-0.034644428984174,
0.078484654900217));
#89403=CARTESIAN_POINT('Ctrl Pts',(0.0117635647974338,-0.0352450361874068,
0.0786031008963699));
#89404=CARTESIAN_POINT('Ctrl Pts',(0.0119315162536957,-0.0349452760959493,
0.0784658242428426));
#89405=CARTESIAN_POINT('Ctrl Pts',(0.012088650338316,-0.034644428984174,
0.0783162867869505));
#89406=CARTESIAN_POINT('Ctrl Pts',(0.0117655343999264,-0.0352450361874068,
0.0786015611996396));
#89407=CARTESIAN_POINT('Ctrl Pts',(0.0119334277855732,-0.0349452760959493,
0.0784642102613353));
#89408=CARTESIAN_POINT('Ctrl Pts',(0.0120904983691176,-0.034644428984174,
0.0783146031058178));
#89409=CARTESIAN_POINT('',(0.0117914199164955,-0.0351951634053338,0.0785801902704607));
#89410=CARTESIAN_POINT('',(0.0119703582009633,-0.0348678972925388,0.0784257429782198));
#89411=CARTESIAN_POINT('Origin',(0.000454706872257089,-0.0345636767878005,
0.066256090558175));
#89412=CARTESIAN_POINT('Origin',(0.0193606208052998,-0.0346946199340733,
0.0866405471726442));
#89413=CARTESIAN_POINT('',(0.0118765206047234,-0.0346945769330289,0.0785083344768662));
#89414=CARTESIAN_POINT('',(0.0119229851005596,-0.0346945769458128,0.0784665337386631));
#89415=CARTESIAN_POINT('',(0.0116942917388866,-0.0350221583435276,0.0786588342821075));
#89416=CARTESIAN_POINT('Origin',(0.000783051344888556,-0.0345628458717962,
0.0659049021452045));
#89417=CARTESIAN_POINT('',(0.0116935214955351,-0.0351951360298762,0.0786578664918798));
#89418=CARTESIAN_POINT('Origin',(0.0185342304354016,-0.0351951838366766,
0.0872963006705578));
#89419=CARTESIAN_POINT('',(0.0117914433283039,-0.0351951371328746,0.0785801678070603));
#89420=CARTESIAN_POINT('Ctrl Pts',(0.0116614176111308,-0.0350241211494343,
0.0789961464741824));
#89421=CARTESIAN_POINT('Ctrl Pts',(0.0117281712918152,-0.0349144232818962,
0.0789474169967862));
#89422=CARTESIAN_POINT('Ctrl Pts',(0.0117939576546772,-0.0348045283579413,
0.0788972785061695));
#89423=CARTESIAN_POINT('Ctrl Pts',(0.0118586900459313,-0.0346945769439158,
0.0788457920877099));
#89424=CARTESIAN_POINT('Ctrl Pts',(0.0116720687311486,-0.0350241211494343,
0.078883329385735));
#89425=CARTESIAN_POINT('Ctrl Pts',(0.0117372684026965,-0.0349144232818962,
0.0788344531935276));
#89426=CARTESIAN_POINT('Ctrl Pts',(0.0118014967935725,-0.0348045283579413,
0.0787842000227632));
#89427=CARTESIAN_POINT('Ctrl Pts',(0.0118646692400894,-0.0346945769439158,
0.0787326311799696));
#89428=CARTESIAN_POINT('Ctrl Pts',(0.0116827198511664,-0.0350241211494343,
0.0787705122972876));
#89429=CARTESIAN_POINT('Ctrl Pts',(0.0117463655135778,-0.0349144232818962,
0.0787214893902691));
#89430=CARTESIAN_POINT('Ctrl Pts',(0.0118090359324679,-0.0348045283579413,
0.078671121539357));
#89431=CARTESIAN_POINT('Ctrl Pts',(0.0118706484342475,-0.0346945769439158,
0.0786194702722293));
#89432=CARTESIAN_POINT('Ctrl Pts',(0.0116933709711842,-0.0350241211494343,
0.0786576952088402));
#89433=CARTESIAN_POINT('Ctrl Pts',(0.011755462624459,-0.0349144232818962,
0.0786085255870105));
#89434=CARTESIAN_POINT('Ctrl Pts',(0.0118165750713632,-0.0348045283579413,
0.0785580430559507));
#89435=CARTESIAN_POINT('Ctrl Pts',(0.0118766276284056,-0.0346945769439158,
0.078506309364489));
#89436=CARTESIAN_POINT('',(0.0118676053208166,-0.0346945769458128,0.0786770632860016));
#89437=CARTESIAN_POINT('Ctrl Pts',(0.0118486512176845,-0.0347116136492773,
0.0788537592082923));
#89438=CARTESIAN_POINT('Ctrl Pts',(0.0118219928734454,-0.0347621546531506,
0.0788200950898051));
#89439=CARTESIAN_POINT('Ctrl Pts',(0.0117958032549355,-0.0348133084095404,
0.0787870228774897));
#89440=CARTESIAN_POINT('Ctrl Pts',(0.011744339612196,-0.0349168561544569,
0.0787220346639899));
#89441=CARTESIAN_POINT('Ctrl Pts',(0.0117190860011002,-0.0349692089015928,
0.0786901444404812));
#89442=CARTESIAN_POINT('Ctrl Pts',(0.0116942917388795,-0.0350221583435,
0.0786588342820665));
#89443=CARTESIAN_POINT('Ctrl Pts',(0.0117899900789448,-0.0351951371254965,
0.0785799990284488));
#89444=CARTESIAN_POINT('Ctrl Pts',(0.0118815775293839,-0.0350307338980967,
0.0785042024806646));
#89445=CARTESIAN_POINT('Ctrl Pts',(0.0119699539657781,-0.0348659306897824,
0.0784246852924333));
#89446=CARTESIAN_POINT('Ctrl Pts',(0.0117914433282243,-0.0351951371254965,
0.0785801678069754));
#89447=CARTESIAN_POINT('Ctrl Pts',(0.0118830342680536,-0.0350307338980967,
0.0785043412141741));
#89448=CARTESIAN_POINT('Ctrl Pts',(0.0119714129490632,-0.0348659306897824,
0.0784247938623788));
#89449=CARTESIAN_POINT('Ctrl Pts',(0.0120350094220996,-0.0351951371254965,
0.0786084552639372));
#89450=CARTESIAN_POINT('Ctrl Pts',(0.0121271851873534,-0.0350307338980967,
0.0785275930949634));
#89451=CARTESIAN_POINT('Ctrl Pts',(0.012215940068261,-0.0348659306897824,
0.0784429902984002));
#89452=CARTESIAN_POINT('Origin',(0.0155272204812442,-0.030860919741085,
0.0823794485306077));
#89453=CARTESIAN_POINT('',(0.0118976326534671,-0.0351951371254965,0.0785925005004132));
#89454=CARTESIAN_POINT('Origin',(0.00737192514890434,-0.0351840467441131,
0.0735259353918352));
#89455=CARTESIAN_POINT('Origin',(0.0166993788085855,-0.0352322614023337,
0.0824941719226236));
#89456=CARTESIAN_POINT('',(0.0121429837173709,-0.0351951142564686,0.0782638587349102));
#89457=CARTESIAN_POINT('',(0.0122302737948824,-0.0351951372916788,0.0781748262974395));
#89458=CARTESIAN_POINT('Origin',(0.00819929833909993,-0.0352875122865233,
0.0738178766097156));
#89459=CARTESIAN_POINT('Origin',(0.00194310532157468,-0.0298325076522745,
0.0784037540701524));
#89460=CARTESIAN_POINT('Origin',(0.0114610257463966,-0.0338732494652423,
0.0818384554366706));
#89461=CARTESIAN_POINT('Origin',(0.00812378219310841,-0.0315241814719618,
0.07415));
#89462=CARTESIAN_POINT('',(0.00949138119084906,-0.0322104233323586,0.0799920606778519));
#89463=CARTESIAN_POINT('',(0.00950385681755529,-0.0321934096636184,0.0799891261359044));
#89464=CARTESIAN_POINT('Origin',(0.00627440703209637,-0.0326387220729212,
0.0637552752997748));
#89465=CARTESIAN_POINT('',(0.00949138119076482,-0.0321763980308521,0.0799920606774919));
#89466=CARTESIAN_POINT('Origin',(0.00512484983222103,-0.0326386251608966,
0.0640308694007681));
#89467=CARTESIAN_POINT('',(0.00947889932502759,-0.0321934096636185,0.0799949685678179));
#89468=CARTESIAN_POINT('Origin',(0.00631955989060436,-0.0326386231321022,
0.0637511974334642));
#89469=CARTESIAN_POINT('Origin',(0.00516712361018345,-0.0326387236420496,
0.0640144901082834));
#89470=CARTESIAN_POINT('Origin',(0.00812378219310841,-0.0315241814719618,
0.07415));
#89471=CARTESIAN_POINT('',(0.00985550857164737,-0.0327114338380051,0.0798946604538155));
#89472=CARTESIAN_POINT('',(0.0098677753192046,-0.0326943950436593,0.079890948351634));
#89473=CARTESIAN_POINT('Origin',(0.00497166242930612,-0.032639568603193,
0.0640244963981889));
#89474=CARTESIAN_POINT('',(0.00985550857166181,-0.0326773559991423,0.0798946604538637));
#89475=CARTESIAN_POINT('Origin',(0.00511101403725754,-0.0326395686209864,
0.0639816718949373));
#89476=CARTESIAN_POINT('',(0.00984323392392406,-0.0326943950436595,0.0798983463487712));
#89477=CARTESIAN_POINT('Origin',(0.00501481363260089,-0.0326395701950183,
0.0640106676017419));
#89478=CARTESIAN_POINT('Origin',(0.00515461686738233,-0.0326395670478704,
0.0639693413694236));
#89479=CARTESIAN_POINT('Origin',(0.00812378219310841,-0.0315241814719618,
0.07415));
#89480=CARTESIAN_POINT('',(0.0105618502624782,-0.0337108120655393,0.0796323192239842));
#89481=CARTESIAN_POINT('',(0.0105735550331356,-0.0336938721132327,0.0796270989613361));
#89482=CARTESIAN_POINT('Origin',(0.00493473930959288,-0.0345562527080821,
0.0642286235176398));
#89483=CARTESIAN_POINT('',(0.0105618502629987,-0.0336769361243754,0.079632319225162));
#89484=CARTESIAN_POINT('Ctrl Pts',(0.0105735550331346,-0.0336938721132368,
0.0796270989613472));
#89485=CARTESIAN_POINT('Ctrl Pts',(0.0105716052984816,-0.0336910493047713,
0.0796279710301252));
#89486=CARTESIAN_POINT('Ctrl Pts',(0.0105696550489526,-0.0336882265901734,
0.0796288420798184));
#89487=CARTESIAN_POINT('Ctrl Pts',(0.0105657534663952,-0.0336825812712632,
0.0796305821646085));
#89488=CARTESIAN_POINT('Ctrl Pts',(0.0105638021333898,-0.033679758666992,
0.0796314511996638));
#89489=CARTESIAN_POINT('Ctrl Pts',(0.0105618502629988,-0.0336769361243754,
0.079632319225162));
#89490=CARTESIAN_POINT('',(0.0105501343689866,-0.0336938721132327,0.0796375144754808));
#89491=CARTESIAN_POINT('Ctrl Pts',(0.0105618502629987,-0.0336769361243754,
0.079632319225162));
#89492=CARTESIAN_POINT('Ctrl Pts',(0.0105598983926042,-0.0336797586669971,
0.0796331872506618));
#89493=CARTESIAN_POINT('Ctrl Pts',(0.0105579461324662,-0.0336825812712733,
0.0796340542009459));
#89494=CARTESIAN_POINT('Ctrl Pts',(0.0105540408446128,-0.0336882265861437,
0.0796357859463635));
#89495=CARTESIAN_POINT('Ctrl Pts',(0.0105520878169393,-0.0336910492967122,
0.0796366507415207));
#89496=CARTESIAN_POINT('Ctrl Pts',(0.0105501343689991,-0.0336938721132385,
0.0796375144754901));
#89497=CARTESIAN_POINT('Origin',(0.0028923809378903,-0.0345562523741628,
0.0651368906056583));
#89498=CARTESIAN_POINT('Origin',(0.00812378219310841,-0.0315241814719618,
0.07415));
#89499=CARTESIAN_POINT('',(0.0102128016195588,-0.0332121607144412,0.0797745886794734));
#89500=CARTESIAN_POINT('',(0.0102248110767375,-0.0331951640388587,0.0797701136670142));
#89501=CARTESIAN_POINT('Origin',(0.00375874516735174,-0.0326413667221338,
0.0645713542574781));
#89502=CARTESIAN_POINT('',(0.01021280161972,-0.0331781648279234,0.0797745886799076));
#89503=CARTESIAN_POINT('Origin',(0.0051332813547961,-0.0326412094385113,
0.064052471445194));
#89504=CARTESIAN_POINT('',(0.0102007826323748,-0.0331951640388588,0.0797790380328514));
#89505=CARTESIAN_POINT('Origin',(0.00379788014756742,-0.032641209245444,
0.0645484511901365));
#89506=CARTESIAN_POINT('Origin',(0.00517787917726456,-0.0326413669324096,
0.0640442768962168));
#89507=CARTESIAN_POINT('Ctrl Pts',(0.00962885585002558,-0.0332451089994433,
0.0797009349020912));
#89508=CARTESIAN_POINT('Ctrl Pts',(0.00983821278511685,-0.0329451141710254,
0.0796441701204001));
#89509=CARTESIAN_POINT('Ctrl Pts',(0.0100426992038379,-0.0326442513127493,
0.0795717969812538));
#89510=CARTESIAN_POINT('Ctrl Pts',(0.00986866494954309,-0.0332451089994433,
0.079630283675714));
#89511=CARTESIAN_POINT('Ctrl Pts',(0.0100753572300355,-0.0329451141710254,
0.079564474345858));
#89512=CARTESIAN_POINT('Ctrl Pts',(0.010276505291818,-0.0326442513127493,
0.0794832830658313));
#89513=CARTESIAN_POINT('',(0.00990303373249483,-0.0331951640388616,0.079619221970225));
#89514=CARTESIAN_POINT('',(0.0101262321451419,-0.0328677532092642,0.0795415043531098));
#89515=CARTESIAN_POINT('Origin',(0.00399190653859828,-0.0326401908899454,
0.0639319461867883));
#89516=CARTESIAN_POINT('Origin',(0.0139755840460193,-0.0326944279134342,
0.0899057054876056));
#89517=CARTESIAN_POINT('',(0.0100085802132244,-0.0326943950436593,0.0795837520575904));
#89518=CARTESIAN_POINT('',(0.010067169678664,-0.0326943950436694,0.079561991438568));
#89519=CARTESIAN_POINT('',(0.00978374540819871,-0.0330220786163545,0.0796566003236614));
#89520=CARTESIAN_POINT('Origin',(0.00443082058661673,-0.0326396682764334,
0.0637354078735713));
#89521=CARTESIAN_POINT('',(0.00978335330633811,-0.0331951640388587,0.0796552996031219));
#89522=CARTESIAN_POINT('Origin',(0.0129673198884641,-0.0331952026560064,
0.090217483389793));
#89523=CARTESIAN_POINT('',(0.00984319351942647,-0.0331951640388701,0.0796372607866835));
#89524=CARTESIAN_POINT('Ctrl Pts',(0.00962900677436569,-0.0330240426238172,
0.0799581235317457));
#89525=CARTESIAN_POINT('Ctrl Pts',(0.00970901933459606,-0.032914277406352,
0.0799373875966696));
#89526=CARTESIAN_POINT('Ctrl Pts',(0.0097886431143048,-0.0328043479726691,
0.0799149872408496));
#89527=CARTESIAN_POINT('Ctrl Pts',(0.00986777531920278,-0.0326943950436593,
0.079890948351638));
#89528=CARTESIAN_POINT('Ctrl Pts',(0.00968044066635957,-0.0330240426238172,
0.0798571498186368));
#89529=CARTESIAN_POINT('Ctrl Pts',(0.00975906221531795,-0.032914277406352,
0.079835705331589));
#89530=CARTESIAN_POINT('Ctrl Pts',(0.00983727964253634,-0.0328043479726691,
0.0798126248266467));
#89531=CARTESIAN_POINT('Ctrl Pts',(0.00991499193137186,-0.0326943950436593,
0.079787935112101));
#89532=CARTESIAN_POINT('Ctrl Pts',(0.00973187455835346,-0.0330240426238172,
0.079756176105528));
#89533=CARTESIAN_POINT('Ctrl Pts',(0.00980910509603984,-0.032914277406352,
0.0797340230665083));
#89534=CARTESIAN_POINT('Ctrl Pts',(0.00988591617076787,-0.0328043479726691,
0.0797102624124438));
#89535=CARTESIAN_POINT('Ctrl Pts',(0.00996220854354094,-0.0326943950436593,
0.079684921872564));
#89536=CARTESIAN_POINT('Ctrl Pts',(0.00978330845034735,-0.0330240426238172,
0.0796552023924192));
#89537=CARTESIAN_POINT('Ctrl Pts',(0.00985914797676173,-0.032914277406352,
0.0796323408014276));
#89538=CARTESIAN_POINT('Ctrl Pts',(0.00993455269899941,-0.0328043479726691,
0.0796078999982409));
#89539=CARTESIAN_POINT('Ctrl Pts',(0.01000942515571,-0.0326943950436593,
0.0795819086330271));
#89540=CARTESIAN_POINT('',(0.00993817776622448,-0.0326943950436694,0.0797373502046222));
#89541=CARTESIAN_POINT('Ctrl Pts',(0.00985550857068446,-0.0327114338383326,
0.0798946604506341));
#89542=CARTESIAN_POINT('Ctrl Pts',(0.00984311336766662,-0.0327619876830619,
0.0798535418111791));
#89543=CARTESIAN_POINT('Ctrl Pts',(0.00983093684236038,-0.0328131562603596,
0.0798131485918699));
#89544=CARTESIAN_POINT('Ctrl Pts',(0.00980701090072301,-0.0329167375858771,
0.0797337790029739));
#89545=CARTESIAN_POINT('Ctrl Pts',(0.00979527101774495,-0.0329691088920623,
0.0796948342584043));
#89546=CARTESIAN_POINT('Ctrl Pts',(0.00978374540818771,-0.0330220786163186,
0.0796566003236151));
#89547=CARTESIAN_POINT('Ctrl Pts',(0.00990124681263013,-0.0331951640388604,
0.0796182628449475));
#89548=CARTESIAN_POINT('Ctrl Pts',(0.00997656107988286,-0.0330855618127442,
0.0795937818627447));
#89549=CARTESIAN_POINT('Ctrl Pts',(0.0100514236600299,-0.032975722417194,
0.0795677266151953));
#89550=CARTESIAN_POINT('Ctrl Pts',(0.0101257370503822,-0.0328657861694598,
0.079540125765186));
#89551=CARTESIAN_POINT('Ctrl Pts',(0.0100010920858834,-0.0331951640388604,
0.0796718545742519));
#89552=CARTESIAN_POINT('Ctrl Pts',(0.0100771444708781,-0.0330855618127442,
0.0796459984252353));
#89553=CARTESIAN_POINT('Ctrl Pts',(0.0101527172785152,-0.032975722417194,
0.0796185517638996));
#89554=CARTESIAN_POINT('Ctrl Pts',(0.010227712009216,-0.0328657861694598,
0.0795895449903085));
#89555=CARTESIAN_POINT('Ctrl Pts',(0.0101009373591368,-0.0331951640388604,
0.0797254463035562));
#89556=CARTESIAN_POINT('Ctrl Pts',(0.0101777278618733,-0.0330855618127442,
0.0796982149877258));
#89557=CARTESIAN_POINT('Ctrl Pts',(0.0102540108970005,-0.032975722417194,
0.0796693769126038));
#89558=CARTESIAN_POINT('Ctrl Pts',(0.0103296869680498,-0.0328657861694598,
0.079638964215431));
#89559=CARTESIAN_POINT('Ctrl Pts',(0.0102007826323901,-0.0331951640388604,
0.0797790380328606));
#89560=CARTESIAN_POINT('Ctrl Pts',(0.0102783112528686,-0.0330855618127442,
0.0797504315502163));
#89561=CARTESIAN_POINT('Ctrl Pts',(0.0103553045154857,-0.032975722417194,
0.0797202020613081));
#89562=CARTESIAN_POINT('Ctrl Pts',(0.0104316619268837,-0.0328657861694598,
0.0796883834405535));
#89563=CARTESIAN_POINT('Ctrl Pts',(0.010212801618493,-0.0331781648273467,
0.0797745886766133));
#89564=CARTESIAN_POINT('Ctrl Pts',(0.0101978361863283,-0.0331276810208849,
0.079734294939144));
#89565=CARTESIAN_POINT('Ctrl Pts',(0.0101831410958168,-0.0330765665171798,
0.0796947290841366));
#89566=CARTESIAN_POINT('Ctrl Pts',(0.0101542785143168,-0.032973061271521,
0.0796170179115595));
#89567=CARTESIAN_POINT('Ctrl Pts',(0.0101401229734508,-0.0329207135598918,
0.0795789047691451));
#89568=CARTESIAN_POINT('Ctrl Pts',(0.010126232145126,-0.0328677532092985,
0.0795415043530671));
#89569=CARTESIAN_POINT('',(0.0100519081824448,-0.0331951640388701,0.0796991300015482));
#89570=CARTESIAN_POINT('Ctrl Pts',(0.00997206329393836,-0.0337436976235975,
0.0795963394332629));
#89571=CARTESIAN_POINT('Ctrl Pts',(0.0100210484962165,-0.0336723290703325,
0.0795797157129274));
#89572=CARTESIAN_POINT('Ctrl Pts',(0.010069726765511,-0.033601104548885,
0.0795622135925272));
#89573=CARTESIAN_POINT('Ctrl Pts',(0.0102251468367468,-0.0333736987606857,
0.0795063327890642));
#89574=CARTESIAN_POINT('Ctrl Pts',(0.0103771040252922,-0.0331450831799192,
0.0794416251729128));
#89575=CARTESIAN_POINT('Ctrl Pts',(0.00997441229367598,-0.0337436976235975,
0.0795954837462684));
#89576=CARTESIAN_POINT('Ctrl Pts',(0.0100233897997755,-0.0336723290703325,
0.0795788388986732));
#89577=CARTESIAN_POINT('Ctrl Pts',(0.0100720599941239,-0.033601104548885,
0.0795613157928613));
#89578=CARTESIAN_POINT('Ctrl Pts',(0.0102274542836558,-0.0333736987606857,
0.0795053679871355));
#89579=CARTESIAN_POINT('Ctrl Pts',(0.0103793818880073,-0.0331450831799192,
0.0794405949586385));
#89580=CARTESIAN_POINT('Ctrl Pts',(0.0102093122674387,-0.0337436976235975,
0.0795099150468142));
#89581=CARTESIAN_POINT('Ctrl Pts',(0.0102575201556871,-0.0336723290703325,
0.0794911574732549));
#89582=CARTESIAN_POINT('Ctrl Pts',(0.0103053828554093,-0.033601104548885,
0.0794715358262675));
#89583=CARTESIAN_POINT('Ctrl Pts',(0.0104581989745559,-0.0333736987606857,
0.0794088877942661));
#89584=CARTESIAN_POINT('Ctrl Pts',(0.010607168159526,-0.0331450831799192,
0.0793375735312187));
#89585=CARTESIAN_POINT('Ctrl Pts',(0.0102116847571737,-0.0337436976235975,
0.0795090508029497));
#89586=CARTESIAN_POINT('Ctrl Pts',(0.0102598848722818,-0.0336723290703325,
0.0794902718908582));
#89587=CARTESIAN_POINT('Ctrl Pts',(0.0103077394163083,-0.033601104548885,
0.0794706290486049));
#89588=CARTESIAN_POINT('Ctrl Pts',(0.010460529495934,-0.0333736987606857,
0.0794079133443181));
#89589=CARTESIAN_POINT('Ctrl Pts',(0.0106094688008683,-0.0331450831799192,
0.0793365330148017));
#89590=CARTESIAN_POINT('',(0.0102429380749578,-0.0336938721132548,0.0794967095814551));
#89591=CARTESIAN_POINT('',(0.0104608161336227,-0.0333679869945434,0.0794051305750701));
#89592=CARTESIAN_POINT('Ctrl Pts',(0.0102429380749636,-0.033693872113265,
0.0794967095814539));
#89593=CARTESIAN_POINT('Ctrl Pts',(0.0102638087906459,-0.0336629187933933,
0.0794884375219329));
#89594=CARTESIAN_POINT('Ctrl Pts',(0.0102846243951419,-0.0336319952301041,
0.0794800459015819));
#89595=CARTESIAN_POINT('Ctrl Pts',(0.0103053828554147,-0.0336011045488951,
0.0794715358262656));
#89596=CARTESIAN_POINT('Ctrl Pts',(0.0103574729353847,-0.0335235892595454,
0.0794501811353131));
#89597=CARTESIAN_POINT('Ctrl Pts',(0.0104092956921413,-0.033445866866037,
0.079428042474058));
#89598=CARTESIAN_POINT('Ctrl Pts',(0.0104608161337401,-0.0333679869945386,
0.0794051305753502));
#89599=CARTESIAN_POINT('Ctrl Pts',(0.0104608570463099,-0.0333679692459114,
0.0794051131331372));
#89600=CARTESIAN_POINT('Ctrl Pts',(0.0104606674692765,-0.0333391895373239,
0.0794047014313379));
#89601=CARTESIAN_POINT('Ctrl Pts',(0.0104605224225366,-0.0333104081058199,
0.0794043941989144));
#89602=CARTESIAN_POINT('Ctrl Pts',(0.0104603254318856,-0.0332532732632664,
0.0794039899131119));
#89603=CARTESIAN_POINT('Ctrl Pts',(0.0104602721166528,-0.0332249238958137,
0.0794038897693094));
#89604=CARTESIAN_POINT('Ctrl Pts',(0.0104602643111526,-0.0331961055014437,
0.0794038891936719));
#89605=CARTESIAN_POINT('Ctrl Pts',(0.0104602641958236,-0.0331956347265782,
0.0794038892119066));
#89606=CARTESIAN_POINT('Ctrl Pts',(0.0104602640934209,-0.0331951640388588,
0.0794038892574465));
#89607=CARTESIAN_POINT('',(0.0103460491095624,-0.0331951640388587,0.0794546823422364));
#89608=CARTESIAN_POINT('',(0.0104031566015012,-0.0331951640388687,0.0794292857998518));
#89609=CARTESIAN_POINT('',(0.0101262321448569,-0.0335216366567647,0.0795415043528045));
#89610=CARTESIAN_POINT('Origin',(0.00320780802711184,-0.0326434571527953,
0.0643920465162114));
#89611=CARTESIAN_POINT('',(0.0101257591440837,-0.0336938721132327,0.0795402308195257));
#89612=CARTESIAN_POINT('Origin',(0.0139279719481104,-0.0336938867896106,
0.0897775159923261));
#89613=CARTESIAN_POINT('',(0.0101843486095307,-0.0336938721132538,0.0795184702005004));
#89614=CARTESIAN_POINT('Ctrl Pts',(0.00999073256489598,-0.0335235895815172,
0.0798521483941871));
#89615=CARTESIAN_POINT('Ctrl Pts',(0.0100692338640391,-0.0334144449262749,
0.0798264461466324));
#89616=CARTESIAN_POINT('Ctrl Pts',(0.0101472943625728,-0.0333049234473147,
0.0797990925925477));
#89617=CARTESIAN_POINT('Ctrl Pts',(0.0102248110767357,-0.0331951640388587,
0.0797701136670188));
#89618=CARTESIAN_POINT('Ctrl Pts',(0.010035724819235,-0.0335235895815172,
0.0797481442138115));
#89619=CARTESIAN_POINT('Ctrl Pts',(0.0101127942960698,-0.0334144449262749,
0.0797218225592942));
#89620=CARTESIAN_POINT('Ctrl Pts',(0.0101894085308233,-0.0333049234473147,
0.0796938784669947));
#89621=CARTESIAN_POINT('Ctrl Pts',(0.0102654663206594,-0.0331951640388587,
0.0796643387946359));
#89622=CARTESIAN_POINT('Ctrl Pts',(0.010080717073574,-0.0335235895815172,
0.0796441400334359));
#89623=CARTESIAN_POINT('Ctrl Pts',(0.0101563547281006,-0.0334144449262749,
0.079617198971956));
#89624=CARTESIAN_POINT('Ctrl Pts',(0.0102315226990737,-0.0333049234473147,
0.0795886643414417));
#89625=CARTESIAN_POINT('Ctrl Pts',(0.0103061215645831,-0.0331951640388587,
0.0795585639222531));
#89626=CARTESIAN_POINT('Ctrl Pts',(0.0101257093279131,-0.0335235895815172,
0.0795401358530602));
#89627=CARTESIAN_POINT('Ctrl Pts',(0.0101999151601314,-0.0334144449262749,
0.0795125753846178));
#89628=CARTESIAN_POINT('Ctrl Pts',(0.0102736368673242,-0.0333049234473147,
0.0794834502158887));
#89629=CARTESIAN_POINT('Ctrl Pts',(0.0103467768085067,-0.0331951640388587,
0.0794527890498702));
#89630=CARTESIAN_POINT('',(0.0102854300931599,-0.0331951640388687,0.0796123980046354));
#89631=CARTESIAN_POINT('Ctrl Pts',(0.0102128016184622,-0.0332121607145974,
0.0797745886765301));
#89632=CARTESIAN_POINT('Ctrl Pts',(0.0101978614059338,-0.0332625444109337,
0.0797343628417714));
#89633=CARTESIAN_POINT('Ctrl Pts',(0.0101831786367119,-0.033313530074597,
0.079694830161269));
#89634=CARTESIAN_POINT('Ctrl Pts',(0.0101543163298441,-0.0334167203140542,
0.0796171197281268));
#89635=CARTESIAN_POINT('Ctrl Pts',(0.0101401479708421,-0.0334688847587215,
0.079578972073471));
#89636=CARTESIAN_POINT('Ctrl Pts',(0.0101262321447603,-0.0335216366562264,
0.0795415043520825));
#89637=CARTESIAN_POINT('Ctrl Pts',(0.0102420291471262,-0.033693872113239,
0.0794962929700426));
#89638=CARTESIAN_POINT('Ctrl Pts',(0.010273322773968,-0.0336474569764958,
0.0794838941677118));
#89639=CARTESIAN_POINT('Ctrl Pts',(0.0103044691129145,-0.033601104548885,
0.0794711298835416));
#89640=CARTESIAN_POINT('Ctrl Pts',(0.0103833244821347,-0.0334837508592656,
0.0794388136507153));
#89641=CARTESIAN_POINT('Ctrl Pts',(0.010461187626907,-0.0333660264659097,
0.0794041749607128));
#89642=CARTESIAN_POINT('Ctrl Pts',(0.0102429380749387,-0.033693872113239,
0.0794967095814627));
#89643=CARTESIAN_POINT('Ctrl Pts',(0.0102742341403453,-0.0336474569764958,
0.0794843054588758));
#89644=CARTESIAN_POINT('Ctrl Pts',(0.0103053828554093,-0.033601104548885,
0.0794715358262675));
#89645=CARTESIAN_POINT('Ctrl Pts',(0.0103842442404127,-0.0334837508592656,
0.0794392060524259));
#89646=CARTESIAN_POINT('Ctrl Pts',(0.010462112997078,-0.0333660264659097,
0.079404553649094));
#89647=CARTESIAN_POINT('Ctrl Pts',(0.0105519775467729,-0.033693872113239,
0.0796383593048589));
#89648=CARTESIAN_POINT('Ctrl Pts',(0.010584102735015,-0.0336474569764958,
0.0796241462716933));
#89649=CARTESIAN_POINT('Ctrl Pts',(0.0106160593405201,-0.033601104548885,
0.0796095581465242));
#89650=CARTESIAN_POINT('Ctrl Pts',(0.0106969661183747,-0.0334837508592656,
0.0795726243676165));
#89651=CARTESIAN_POINT('Ctrl Pts',(0.0107767429434898,-0.0333660264659097,
0.0795333093717271));
#89652=CARTESIAN_POINT('Ctrl Pts',(0.0105618502629987,-0.0336769361243754,
0.079632319225162));
#89653=CARTESIAN_POINT('Ctrl Pts',(0.0105448196623067,-0.0336279031428237,
0.0795940236620713));
#89654=CARTESIAN_POINT('Ctrl Pts',(0.0105275440335534,-0.0335767852155838,
0.079555177120907));
#89655=CARTESIAN_POINT('Ctrl Pts',(0.0104936928512639,-0.0334733199122769,
0.079479058250498));
#89656=CARTESIAN_POINT('Ctrl Pts',(0.0104770945689073,-0.0334209645148416,
0.079441734812488));
#89657=CARTESIAN_POINT('Ctrl Pts',(0.0104608161269541,-0.0333679869844681,
0.0794051305780214));
#89658=CARTESIAN_POINT('',(0.0103965362219822,-0.0336938721132538,0.079567112028478));
#89659=CARTESIAN_POINT('Ctrl Pts',(0.0103126374997385,-0.034243627687391,
0.0794685559550161));
#89660=CARTESIAN_POINT('Ctrl Pts',(0.0105132301443936,-0.033943005420181,
0.079386001916206));
#89661=CARTESIAN_POINT('Ctrl Pts',(0.0107070346179166,-0.0336441434784052,
0.0792885729448674));
#89662=CARTESIAN_POINT('Ctrl Pts',(0.0105417019481317,-0.034243627687391,
0.0793684086710672));
#89663=CARTESIAN_POINT('Ctrl Pts',(0.0107385174757061,-0.033943005420181,
0.079277215324165));
#89664=CARTESIAN_POINT('Ctrl Pts',(0.010927904814458,-0.0336441434784052,
0.0791714560960379));
#89665=CARTESIAN_POINT('',(0.0105744790772775,-0.0341934961088741,0.0793530961726576));
#89666=CARTESIAN_POINT('',(0.0107861769053515,-0.0338664212865018,0.0792480172028979));
#89667=CARTESIAN_POINT('Origin',(0.00390799302620703,-0.034561072040514,
0.0640034672689447));
#89668=CARTESIAN_POINT('Origin',(0.0158626625724525,-0.033693800507292,
0.0889685119293432));
#89669=CARTESIAN_POINT('',(0.0106747477336384,-0.0336938721132327,0.0793046774691565));
#89670=CARTESIAN_POINT('',(0.0107301478748956,-0.0336938721132427,0.0792757452319597));
#89671=CARTESIAN_POINT('',(0.0104608161269492,-0.0340203938281606,0.0794051305780235));
#89672=CARTESIAN_POINT('Origin',(0.00437362203041919,-0.0345589643244381,
0.0638821150356397));
#89673=CARTESIAN_POINT('',(0.01046026409342,-0.034193496108874,0.079403889257447));
#89674=CARTESIAN_POINT('Origin',(0.0149379570872416,-0.0341934220717664,
0.0894725775394897));
#89675=CARTESIAN_POINT('',(0.0105173715853588,-0.0341934961088841,0.0793784927150624));
#89676=CARTESIAN_POINT('Ctrl Pts',(0.0103450868831099,-0.0340223579322397,
0.0797236707360799));
#89677=CARTESIAN_POINT('Ctrl Pts',(0.0104219623393039,-0.0339125849573575,
0.0796930331509989));
#89678=CARTESIAN_POINT('Ctrl Pts',(0.0104981496491858,-0.0338030433565231,
0.079660825951285));
#89679=CARTESIAN_POINT('Ctrl Pts',(0.0105735550331339,-0.0336938721132327,
0.0796270989613416));
#89680=CARTESIAN_POINT('Ctrl Pts',(0.0103834599385915,-0.0340223579322397,
0.0796170466841801));
#89681=CARTESIAN_POINT('Ctrl Pts',(0.0104588647710227,-0.0339125849573575,
0.0795858798345829));
#89682=CARTESIAN_POINT('Ctrl Pts',(0.0105335715359862,-0.0338030433565231,
0.0795531741807553));
#89683=CARTESIAN_POINT('Ctrl Pts',(0.0106074884037344,-0.0336938721132327,
0.0795189800167009));
#89684=CARTESIAN_POINT('Ctrl Pts',(0.0104218329940731,-0.0340223579322397,
0.0795104226322802));
#89685=CARTESIAN_POINT('Ctrl Pts',(0.0104957672027414,-0.0339125849573575,
0.0794787265181668));
#89686=CARTESIAN_POINT('Ctrl Pts',(0.0105689934227867,-0.0338030433565231,
0.0794455224102258));
#89687=CARTESIAN_POINT('Ctrl Pts',(0.010641421774335,-0.0336938721132327,
0.0794108610720602));
#89688=CARTESIAN_POINT('Ctrl Pts',(0.0104602060495547,-0.0340223579322397,
0.0794037985803804));
#89689=CARTESIAN_POINT('Ctrl Pts',(0.0105326696344601,-0.0339125849573575,
0.0793715732017507));
#89690=CARTESIAN_POINT('Ctrl Pts',(0.0106044153095872,-0.0338030433565231,
0.0793378706396961));
#89691=CARTESIAN_POINT('Ctrl Pts',(0.0106753551449355,-0.0336938721132327,
0.0793027421274195));
#89692=CARTESIAN_POINT('',(0.010624151383397,-0.0336938721132427,0.0794658882152563));
#89693=CARTESIAN_POINT('Ctrl Pts',(0.0105618502610078,-0.0337108120662682,
0.0796323192206852));
#89694=CARTESIAN_POINT('Ctrl Pts',(0.0105443777421099,-0.0337611408993851,
0.0795930299459316));
#89695=CARTESIAN_POINT('Ctrl Pts',(0.0105272240579175,-0.0338121088780384,
0.0795544576132753));
#89696=CARTESIAN_POINT('Ctrl Pts',(0.0104935387321512,-0.0339153382773238,
0.0794787116932433));
#89697=CARTESIAN_POINT('Ctrl Pts',(0.0104770213415777,-0.0339675558473118,
0.0794415701511311));
#89698=CARTESIAN_POINT('Ctrl Pts',(0.0104608161269378,-0.0340203938281305,
0.0794051305779849));
#89699=CARTESIAN_POINT('Ctrl Pts',(0.0105725859505553,-0.0341934961088741,
0.0793523685373797));
#89700=CARTESIAN_POINT('Ctrl Pts',(0.0106443235323612,-0.0340836138575045,
0.0793186009835022));
#89701=CARTESIAN_POINT('Ctrl Pts',(0.0107153279444492,-0.0339738896631393,
0.0792833651731941));
#89702=CARTESIAN_POINT('Ctrl Pts',(0.0107855113330447,-0.0338644633275951,
0.0792467122958646));
#89703=CARTESIAN_POINT('Ctrl Pts',(0.0106783607677275,-0.0341934961088741,
0.0793930237600828));
#89704=CARTESIAN_POINT('Ctrl Pts',(0.0107506589609826,-0.0340836138575045,
0.0793577976341058));
#89705=CARTESIAN_POINT('Ctrl Pts',(0.0108221935334385,-0.0339738896631393,
0.0793210923508709));
#89706=CARTESIAN_POINT('Ctrl Pts',(0.0108928760788564,-0.0338644633275951,
0.0792829610260169));
#89707=CARTESIAN_POINT('Ctrl Pts',(0.0107841355848998,-0.0341934961088741,
0.0794336789827859));
#89708=CARTESIAN_POINT('Ctrl Pts',(0.0108569943896039,-0.0340836138575045,
0.0793969942847094));
#89709=CARTESIAN_POINT('Ctrl Pts',(0.0109290591224277,-0.0339738896631393,
0.0793588195285476));
#89710=CARTESIAN_POINT('Ctrl Pts',(0.011000240824668,-0.0338644633275951,
0.0793192097561692));
#89711=CARTESIAN_POINT('Ctrl Pts',(0.010889910402072,-0.0341934961088741,
0.079474334205489));
#89712=CARTESIAN_POINT('Ctrl Pts',(0.0109633298182253,-0.0340836138575045,
0.079436190935313));
#89713=CARTESIAN_POINT('Ctrl Pts',(0.011035924711417,-0.0339738896631393,
0.0793965467062244));
#89714=CARTESIAN_POINT('Ctrl Pts',(0.0111076055704797,-0.0338644633275951,
0.0793554584863215));
#89715=CARTESIAN_POINT('',(0.0109012769641236,-0.0341764758832481,0.0794684135581252));
#89716=CARTESIAN_POINT('',(0.010889910402055,-0.034193496108874,0.0794743342054824));
#89717=CARTESIAN_POINT('Origin',(0.00369035864568257,-0.0345621026671577,
0.0645545278443666));
#89718=CARTESIAN_POINT('Ctrl Pts',(0.0109012769626372,-0.0341764758830279,
0.079468413555284));
#89719=CARTESIAN_POINT('Ctrl Pts',(0.010881406524438,-0.0341260048544556,
0.0794303651639684));
#89720=CARTESIAN_POINT('Ctrl Pts',(0.010861881658299,-0.0340749271285665,
0.0793929784823163));
#89721=CARTESIAN_POINT('Ctrl Pts',(0.0108235072099956,-0.0339715434413963,
0.0793194981689518));
#89722=CARTESIAN_POINT('Ctrl Pts',(0.0108046726441579,-0.0339192781018088,
0.0792834332908616));
#89723=CARTESIAN_POINT('Ctrl Pts',(0.0107861769042516,-0.0338664212856217,
0.0792480172047858));
#89724=CARTESIAN_POINT('',(0.0107321947396763,-0.0341934961088841,0.0794137151890801));
#89725=CARTESIAN_POINT('Ctrl Pts',(0.00895696931268619,-0.0321934096636942,
0.0798406884434743));
#89726=CARTESIAN_POINT('Ctrl Pts',(0.00910964311196116,-0.0319797282160566,
0.0798183351123587));
#89727=CARTESIAN_POINT('Ctrl Pts',(0.00926089872727212,-0.0317669959606124,
0.079787827748757));
#89728=CARTESIAN_POINT('Ctrl Pts',(0.00920352852800519,-0.0321934096636942,
0.0797990948701785));
#89729=CARTESIAN_POINT('Ctrl Pts',(0.00935508642558856,-0.0319797282160566,
0.0797701266747063));
#89730=CARTESIAN_POINT('Ctrl Pts',(0.00950487306326706,-0.0317669959606124,
0.0797330737957119));
#89731=CARTESIAN_POINT('Ctrl Pts',(0.00920500768011314,-0.0321934096636942,
0.0797988453430151));
#89732=CARTESIAN_POINT('Ctrl Pts',(0.00935655888320595,-0.0319797282160566,
0.0797698374638079));
#89733=CARTESIAN_POINT('Ctrl Pts',(0.00950633670822921,-0.0317669959606124,
0.0797327453171151));
#89734=CARTESIAN_POINT('',(0.00920352852811267,-0.0321934096636942,0.079799094870158));
#89735=CARTESIAN_POINT('',(0.00943470755481606,-0.0318665617561286,0.0797499642584603));
#89736=CARTESIAN_POINT('Origin',(0.00667259770270094,-0.0326371944420838,
0.0632820644467268));
#89737=CARTESIAN_POINT('Origin',(0.0119331252814131,-0.0316939261508561,
0.0904226161825828));
#89738=CARTESIAN_POINT('',(0.00908075077506004,-0.0320197259213198,0.0798211393066617));
#89739=CARTESIAN_POINT('Ctrl Pts',(0.00908093315538712,-0.0320197391311199,
0.0798211548887622));
#89740=CARTESIAN_POINT('Ctrl Pts',(0.00910978981795955,-0.0319792715672862,
0.0798162845963983));
#89741=CARTESIAN_POINT('Ctrl Pts',(0.0091387407042514,-0.0319386438886469,
0.079811172057838));
#89742=CARTESIAN_POINT('Ctrl Pts',(0.00916781467110402,-0.0318979098685809,
0.0798058036204764));
#89743=CARTESIAN_POINT('Ctrl Pts',(0.00919688806317048,-0.031857176653818,
0.0798004352892477));
#89744=CARTESIAN_POINT('Ctrl Pts',(0.00922593726756676,-0.0318163871807232,
0.079794840067621));
#89745=CARTESIAN_POINT('Ctrl Pts',(0.00925486290398387,-0.0317755399642096,
0.0797890408823101));
#89746=CARTESIAN_POINT('',(0.0090802700914209,-0.0321934096636184,0.079819888085349));
#89747=CARTESIAN_POINT('Origin',(0.00940054856919069,-0.032343065755914,
0.0817184413106508));
#89748=CARTESIAN_POINT('',(0.00914189930977679,-0.0321934096636664,0.0798094914777636));
#89749=CARTESIAN_POINT('Ctrl Pts',(0.00920187577157625,-0.0321934096636618,
0.0797979192498066));
#89750=CARTESIAN_POINT('Ctrl Pts',(0.00927976497976191,-0.0320835708272592,
0.0797830514991425));
#89751=CARTESIAN_POINT('Ctrl Pts',(0.00935730132171413,-0.0319739230346489,
0.0797665804592627));
#89752=CARTESIAN_POINT('Ctrl Pts',(0.00943438721239903,-0.0318646057455573,
0.0797485348172249));
#89753=CARTESIAN_POINT('Ctrl Pts',(0.00929421695605448,-0.0321934096636618,
0.0798636023558164));
#89754=CARTESIAN_POINT('Ctrl Pts',(0.00937301198546243,-0.0320835708272592,
0.0798474611482519));
#89755=CARTESIAN_POINT('Ctrl Pts',(0.00945142726909945,-0.0319739230346489,
0.0798296986442053));
#89756=CARTESIAN_POINT('Ctrl Pts',(0.00952936422419915,-0.0318646057455573,
0.0798103452693787));
#89757=CARTESIAN_POINT('Ctrl Pts',(0.00938655814053272,-0.0321934096636618,
0.0799292854618262));
#89758=CARTESIAN_POINT('Ctrl Pts',(0.00946625899116296,-0.0320835708272592,
0.0799118707973613));
#89759=CARTESIAN_POINT('Ctrl Pts',(0.00954555321648478,-0.0319739230346489,
0.0798928168291479));
#89760=CARTESIAN_POINT('Ctrl Pts',(0.00962434123599927,-0.0318646057455573,
0.0798721557215325));
#89761=CARTESIAN_POINT('Ctrl Pts',(0.00947889932501095,-0.0321934096636618,
0.0799949685678361));
#89762=CARTESIAN_POINT('Ctrl Pts',(0.00955950599686348,-0.0320835708272592,
0.0799762804464707));
#89763=CARTESIAN_POINT('Ctrl Pts',(0.0096396791638701,-0.0319739230346489,
0.0799559350140904));
#89764=CARTESIAN_POINT('Ctrl Pts',(0.00971931824779939,-0.0318646057455573,
0.0799339661736864));
#89765=CARTESIAN_POINT('Ctrl Pts',(0.00949138119003686,-0.032176398030639,
0.0799920606743997));
#89766=CARTESIAN_POINT('Ctrl Pts',(0.00948159855085754,-0.0321259596179479,
0.0799502715448598));
#89767=CARTESIAN_POINT('Ctrl Pts',(0.00947198540859514,-0.032074916464065,
0.0799092064662113));
#89768=CARTESIAN_POINT('Ctrl Pts',(0.00945309038158429,-0.0319716057814246,
0.0798284913629612));
#89769=CARTESIAN_POINT('Ctrl Pts',(0.00944381585910628,-0.0319193786724659,
0.0797888727882441));
#89770=CARTESIAN_POINT('Ctrl Pts',(0.0094347075548043,-0.0318665617561676,
0.0797499642584101));
#89771=CARTESIAN_POINT('',(0.00934121392658013,-0.0321934096636664,0.079897031718998));
#89772=CARTESIAN_POINT('Ctrl Pts',(0.00927486369295094,-0.0327445246967098,
0.0797850481480393));
#89773=CARTESIAN_POINT('Ctrl Pts',(0.00948739300823782,-0.0324436878339361,
0.079741634399554));
#89774=CARTESIAN_POINT('Ctrl Pts',(0.00969604844921609,-0.0321434074405928,
0.0796823354082979));
#89775=CARTESIAN_POINT('Ctrl Pts',(0.00927730141791528,-0.0327445246967098,
0.0797844936239206));
#89776=CARTESIAN_POINT('Ctrl Pts',(0.00948980981898312,-0.0324436878339361,
0.0797409879351353));
#89777=CARTESIAN_POINT('Ctrl Pts',(0.00969843747983829,-0.0321434074405928,
0.0796815988401161));
#89778=CARTESIAN_POINT('Ctrl Pts',(0.0095210739143494,-0.0327445246967098,
0.07972904121205));
#89779=CARTESIAN_POINT('Ctrl Pts',(0.00973149089351344,-0.0324436878339361,
0.0796763414932596));
#89780=CARTESIAN_POINT('Ctrl Pts',(0.00993734054205709,-0.0321434074405928,
0.0796079420219492));
#89781=CARTESIAN_POINT('Ctrl Pts',(0.00952353601656339,-0.0327445246967098,
0.0797284811426901));
#89782=CARTESIAN_POINT('Ctrl Pts',(0.00973393187236619,-0.0324436878339361,
0.0796756885641967));
#89783=CARTESIAN_POINT('Ctrl Pts',(0.0099397534629855,-0.0321434074405928,
0.0796071980880857));
#89784=CARTESIAN_POINT('',(0.00955610749708096,-0.0326943950436612,0.0797201498385232));
#89785=CARTESIAN_POINT('',(0.00978374540820148,-0.0323666188837389,0.0796566003236606));
#89786=CARTESIAN_POINT('Origin',(0.0052959155205112,-0.0326395579111105,
0.0634579598715753));
#89787=CARTESIAN_POINT('Origin',(0.0129714528185447,-0.0321933825603156,
0.0902311874680557));
#89788=CARTESIAN_POINT('',(0.0096636728737861,-0.0321934096536378,0.0796913772377324));
#89789=CARTESIAN_POINT('',(0.00972351308965225,-0.0321934096584275,0.0796733384205856));
#89790=CARTESIAN_POINT('',(0.0094347075548117,-0.032521010975624,0.0797499642584613));
#89791=CARTESIAN_POINT('Origin',(0.00576725340923381,-0.0326393129159137,
0.0633629597420143));
#89792=CARTESIAN_POINT('',(0.00943439789959461,-0.0326943950436595,0.0797486414843167));
#89793=CARTESIAN_POINT('Origin',(0.0119558975382756,-0.0326943765538136,
0.090519897504833));
#89794=CARTESIAN_POINT('',(0.00949525269834778,-0.0326943950436704,0.07973439566143));
#89795=CARTESIAN_POINT('Ctrl Pts',(0.00926134051997949,-0.032522978320377,
0.0800411765423401));
#89796=CARTESIAN_POINT('Ctrl Pts',(0.00934255025978414,-0.0324130253092451,
0.0800254953256809));
#89797=CARTESIAN_POINT('Ctrl Pts',(0.00942342329643002,-0.0323031222208071,
0.0800081365595964));
#89798=CARTESIAN_POINT('Ctrl Pts',(0.0095038568219188,-0.0321934096576659,
0.0799891261348738));
#89799=CARTESIAN_POINT('Ctrl Pts',(0.00931901314050244,-0.032522978320377,
0.0799436316240791));
#89800=CARTESIAN_POINT('Ctrl Pts',(0.00939887822574202,-0.0324130253092451,
0.0799271553916072));
#89801=CARTESIAN_POINT('Ctrl Pts',(0.0094783903658427,-0.0323031222208071,
0.0799090295461967));
#89802=CARTESIAN_POINT('Ctrl Pts',(0.00955744853068966,-0.0321934096576659,
0.0798892808996967));
#89803=CARTESIAN_POINT('Ctrl Pts',(0.00937668576102538,-0.032522978320377,
0.079846086705818));
#89804=CARTESIAN_POINT('Ctrl Pts',(0.0094552061916999,-0.0324130253092451,
0.0798288154575335));
#89805=CARTESIAN_POINT('Ctrl Pts',(0.00953335743525537,-0.0323031222208071,
0.079809922532797));
#89806=CARTESIAN_POINT('Ctrl Pts',(0.00961104023946051,-0.0321934096576659,
0.0797894356645198));
#89807=CARTESIAN_POINT('Ctrl Pts',(0.00943435838154833,-0.032522978320377,
0.079748541787557));
#89808=CARTESIAN_POINT('Ctrl Pts',(0.00951153415765779,-0.0324130253092451,
0.0797304755234598));
#89809=CARTESIAN_POINT('Ctrl Pts',(0.00958832450466805,-0.0323031222208071,
0.0797108155193974));
#89810=CARTESIAN_POINT('Ctrl Pts',(0.00966463194823136,-0.0321934096576659,
0.0796895904293427));
#89811=CARTESIAN_POINT('',(0.00958376484526082,-0.0321934096584275,0.0798402516869768));
#89812=CARTESIAN_POINT('Ctrl Pts',(0.00949138119005014,-0.0322104233328915,
0.0799920606744565));
#89813=CARTESIAN_POINT('Ctrl Pts',(0.00948158529515375,-0.0322609421831088,
0.0799502149196166));
#89814=CARTESIAN_POINT('Ctrl Pts',(0.00947196567721331,-0.0323120888240161,
0.0799091221783973));
#89815=CARTESIAN_POINT('Ctrl Pts',(0.00945307050693992,-0.0324156524631812,
0.0798284064631636));
#89816=CARTESIAN_POINT('Ctrl Pts',(0.00944380272152753,-0.032468026716732,
0.0797888166676036));
#89817=CARTESIAN_POINT('Ctrl Pts',(0.00943470755480609,-0.0325210109755913,
0.0797499642584181));
#89818=CARTESIAN_POINT('Origin',(0.000302798411271529,-0.0262834582511148,
0.0750076704056847));
#89819=CARTESIAN_POINT('Origin',(0.00530621998124759,-0.0342770973722091,
0.0859773416106945));
#89820=CARTESIAN_POINT('Ctrl Pts',(0.0095543846023505,-0.0326943950436604,
0.0797190805749539));
#89821=CARTESIAN_POINT('Ctrl Pts',(0.00963113697024279,-0.0325844576448134,
0.0796993641925199));
#89822=CARTESIAN_POINT('Ctrl Pts',(0.00970748700290522,-0.0324744968375323,
0.0796780590499216));
#89823=CARTESIAN_POINT('Ctrl Pts',(0.00978333725273647,-0.0323646534831895,
0.0796551937938388));
#89824=CARTESIAN_POINT('Ctrl Pts',(0.00965066770954531,-0.0326943950436604,
0.0797788358328955));
#89825=CARTESIAN_POINT('Ctrl Pts',(0.00972824361688532,-0.0325844576448134,
0.0797577924887905));
#89826=CARTESIAN_POINT('Ctrl Pts',(0.0098053898035357,-0.0324744968375323,
0.0797351432584642));
#89827=CARTESIAN_POINT('Ctrl Pts',(0.00988200782556948,-0.0323646534831895,
0.0797109185247898));
#89828=CARTESIAN_POINT('Ctrl Pts',(0.00974695081674012,-0.0326943950436604,
0.0798385910908371));
#89829=CARTESIAN_POINT('Ctrl Pts',(0.00982535026352786,-0.0325844576448134,
0.0798162207850612));
#89830=CARTESIAN_POINT('Ctrl Pts',(0.00990329260416619,-0.0324744968375323,
0.0797922274670068));
#89831=CARTESIAN_POINT('Ctrl Pts',(0.00998067839840248,-0.0323646534831895,
0.0797666432557407));
#89832=CARTESIAN_POINT('Ctrl Pts',(0.00984323392393492,-0.0326943950436604,
0.0798983463487787));
#89833=CARTESIAN_POINT('Ctrl Pts',(0.00992245691017039,-0.0325844576448134,
0.0798746490813319));
#89834=CARTESIAN_POINT('Ctrl Pts',(0.0100011954047967,-0.0324744968375323,
0.0798493116755494));
#89835=CARTESIAN_POINT('Ctrl Pts',(0.0100793489712355,-0.0323646534831895,
0.0798223679866917));
#89836=CARTESIAN_POINT('Ctrl Pts',(0.00985550857068935,-0.0326773559987533,
0.07989466045065));
#89837=CARTESIAN_POINT('Ctrl Pts',(0.00984311130562075,-0.032626792258728,
0.0798535349707487));
#89838=CARTESIAN_POINT('Ctrl Pts',(0.00983093377312217,-0.0325756109581931,
0.0798131384102777));
#89839=CARTESIAN_POINT('Ctrl Pts',(0.00980700780946977,-0.0324719985462395,
0.0797337687483512));
#89840=CARTESIAN_POINT('Ctrl Pts',(0.00979526897445343,-0.0324196091621788,
0.0796948274801878));
#89841=CARTESIAN_POINT('Ctrl Pts',(0.00978374540818738,-0.0323666188837757,
0.0796566003236139));
#89842=CARTESIAN_POINT('',(0.00969967071051251,-0.0326943950436704,0.0798092480936573));
#89843=CARTESIAN_POINT('Origin',(0.00812378219310841,-0.0315241814719618,
0.07415));
#89844=CARTESIAN_POINT('',(0.0109012769642642,-0.0342105180190362,0.0794684135583947));
#89845=CARTESIAN_POINT('',(0.010912630855329,-0.0341934961088739,0.0794624686483059));
#89846=CARTESIAN_POINT('Origin',(0.00364803044415716,-0.0345621723243437,
0.0645707338869119));
#89847=CARTESIAN_POINT('Origin',(0.00278250704172717,-0.0345621027604414,
0.0650286450762808));
#89848=CARTESIAN_POINT('Origin',(0.00281999399346116,-0.0345621725530212,
0.0650031692818173));
#89849=CARTESIAN_POINT('Ctrl Pts',(0.0106734181214623,-0.0346945769586966,
0.0793053718474377));
#89850=CARTESIAN_POINT('Ctrl Pts',(0.0107813994489052,-0.0345275153362944,
0.0792519687020998));
#89851=CARTESIAN_POINT('Ctrl Pts',(0.0108877292260835,-0.0343603235965186,
0.0791951558306151));
#89852=CARTESIAN_POINT('Ctrl Pts',(0.010992095474039,-0.034193496108874,
0.0791351059341747));
#89853=CARTESIAN_POINT('Ctrl Pts',(0.0107477281807789,-0.0346945769586966,
0.0792665640715983));
#89854=CARTESIAN_POINT('Ctrl Pts',(0.010854896663819,-0.0345275153362944,
0.0792116044723159));
#89855=CARTESIAN_POINT('Ctrl Pts',(0.0109603644373075,-0.0343603235965186,
0.0791532603075162));
#89856=CARTESIAN_POINT('Ctrl Pts',(0.0110638221390214,-0.034193496108874,
0.0790917087693853));
#89857=CARTESIAN_POINT('Ctrl Pts',(0.0108220382400957,-0.0346945769586966,
0.0792277562957589));
#89858=CARTESIAN_POINT('Ctrl Pts',(0.0109283938787331,-0.0345275153362944,
0.0791712402425335));
#89859=CARTESIAN_POINT('Ctrl Pts',(0.0110329996485315,-0.0343603235965186,
0.0791113647844187));
#89860=CARTESIAN_POINT('Ctrl Pts',(0.0111355488040033,-0.034193496108874,
0.0790483116045955));
#89861=CARTESIAN_POINT('Ctrl Pts',(0.0108963482994122,-0.0346945769586966,
0.0791889485199195));
#89862=CARTESIAN_POINT('Ctrl Pts',(0.0110018910936468,-0.0345275153362944,
0.0791308760127481));
#89863=CARTESIAN_POINT('Ctrl Pts',(0.0111056348597555,-0.0343603235965186,
0.0790694692613185));
#89864=CARTESIAN_POINT('Ctrl Pts',(0.011207275468986,-0.034193496108874,
0.0790049144398064));
#89865=CARTESIAN_POINT('',(0.0108963482986323,-0.0346945769586966,0.0791889485203265));
#89866=CARTESIAN_POINT('',(0.011101030424786,-0.0343667727832864,0.0790707842838023));
#89867=CARTESIAN_POINT('Origin',(0.00263116674820189,-0.0345626461566267,
0.0645470900085804));
#89868=CARTESIAN_POINT('Origin',(0.0168223057555468,-0.0341934771027721,
0.0885268756521276));
#89869=CARTESIAN_POINT('',(0.0109933788621512,-0.034193496108874,0.0791343294390539));
#89870=CARTESIAN_POINT('',(0.0110468530136792,-0.034193496108884,0.0791019756893674));
#89871=CARTESIAN_POINT('',(0.0107861769035202,-0.0345211942962611,0.0792480172033841));
#89872=CARTESIAN_POINT('Origin',(0.00305889754078945,-0.0345625596120682,
0.0643274617802946));
#89873=CARTESIAN_POINT('',(0.0107855480161328,-0.0346945769586886,0.0792468129947429));
#89874=CARTESIAN_POINT('Origin',(0.0159070470656408,-0.0346945685853798,
0.089053584261013));
#89875=CARTESIAN_POINT('',(0.0108409481573925,-0.0346945769587026,0.0792178807575448));
#89876=CARTESIAN_POINT('Ctrl Pts',(0.0106906781965947,-0.0345231616327842,
0.0795731950829144));
#89877=CARTESIAN_POINT('Ctrl Pts',(0.0107654293055647,-0.0344132092796988,
0.0795378140354068));
#89878=CARTESIAN_POINT('Ctrl Pts',(0.0108394447286616,-0.0343032738558979,
0.0795008886456725));
#89879=CARTESIAN_POINT('Ctrl Pts',(0.0109126308553275,-0.0341934961088739,
0.0794624686483121));
#89880=CARTESIAN_POINT('Ctrl Pts',(0.0107222804807894,-0.0345231616327842,
0.0794643721452014));
#89881=CARTESIAN_POINT('Ctrl Pts',(0.0107955316187736,-0.0344132092796988,
0.0794285555046987));
#89882=CARTESIAN_POINT('Ctrl Pts',(0.0108680381383786,-0.0343032738558979,
0.0793912255701605));
#89883=CARTESIAN_POINT('Ctrl Pts',(0.0109397083754022,-0.0341934961088739,
0.0793524325449396));
#89884=CARTESIAN_POINT('Ctrl Pts',(0.0107538827649842,-0.0345231616327842,
0.0793555492074885));
#89885=CARTESIAN_POINT('Ctrl Pts',(0.0108256339319824,-0.0344132092796988,
0.0793192969739906));
#89886=CARTESIAN_POINT('Ctrl Pts',(0.0108966315480957,-0.0343032738558979,
0.0792815624946485));
#89887=CARTESIAN_POINT('Ctrl Pts',(0.0109667858954769,-0.0341934961088739,
0.0792423964415671));
#89888=CARTESIAN_POINT('Ctrl Pts',(0.010785485049179,-0.0345231616327842,
0.0792467262697756));
#89889=CARTESIAN_POINT('Ctrl Pts',(0.0108557362451913,-0.0344132092796988,
0.0792100384432825));
#89890=CARTESIAN_POINT('Ctrl Pts',(0.0109252249578127,-0.0343032738558979,
0.0791718994191365));
#89891=CARTESIAN_POINT('Ctrl Pts',(0.0109938634155516,-0.0341934961088739,
0.0791323603381946));
#89892=CARTESIAN_POINT('',(0.0109530048587501,-0.0341934961088839,0.0792983990436899));
#89893=CARTESIAN_POINT('Ctrl Pts',(0.0109012769626589,-0.0342105180195379,
0.0794684135553258));
#89894=CARTESIAN_POINT('Ctrl Pts',(0.0108813842520914,-0.0342610556240654,
0.0794303225163456));
#89895=CARTESIAN_POINT('Ctrl Pts',(0.0108618485059288,-0.0343122189868824,
0.0793929150013635));
#89896=CARTESIAN_POINT('Ctrl Pts',(0.010823473817671,-0.0344158119695087,
0.0793194342285284));
#89897=CARTESIAN_POINT('Ctrl Pts',(0.0108046505711748,-0.034468199044996,
0.0792833910249845));
#89898=CARTESIAN_POINT('Ctrl Pts',(0.0107861769035042,-0.0345211942962359,
0.0792480172033548));
#89899=CARTESIAN_POINT('Ctrl Pts',(0.0108944136928532,-0.0346945769586932,
0.0791883413400184));
#89900=CARTESIAN_POINT('Ctrl Pts',(0.0109985778350075,-0.0345296777077528,
0.0791310604942161));
#89901=CARTESIAN_POINT('Ctrl Pts',(0.0111002855002113,-0.0343648066252516,
0.0790695233944684));
#89902=CARTESIAN_POINT('Ctrl Pts',(0.0108963482986243,-0.0346945769586932,
0.0791889485203309));
#89903=CARTESIAN_POINT('Ctrl Pts',(0.0110005249938019,-0.0345296777077528,
0.0791316276779232));
#89904=CARTESIAN_POINT('Ctrl Pts',(0.0111022435482061,-0.0343648066252516,
0.0790700500969187));
#89905=CARTESIAN_POINT('Ctrl Pts',(0.0112187697908207,-0.0346945769586932,
0.079290141220839));
#89906=CARTESIAN_POINT('Ctrl Pts',(0.011325038573479,-0.0345296777077528,
0.0792261545422206));
#89907=CARTESIAN_POINT('Ctrl Pts',(0.0114285719225654,-0.0343648066252516,
0.079157830352981));
#89908=CARTESIAN_POINT('',(0.0112297421630657,-0.0346775396665029,0.0792835185456563));
#89909=CARTESIAN_POINT('',(0.0112187697908064,-0.0346945769586885,0.0792901412208319));
#89910=CARTESIAN_POINT('Origin',(0.00250546247597207,-0.0345626617644253,
0.0651590773166458));
#89911=CARTESIAN_POINT('Ctrl Pts',(0.0112297421612359,-0.0346775396670097,
0.0792835185456332));
#89912=CARTESIAN_POINT('Ctrl Pts',(0.0112075044166854,-0.0346269749928345,
0.0792467641129203));
#89913=CARTESIAN_POINT('Ctrl Pts',(0.011185661855744,-0.0345757902891116,
0.0792106629070845));
#89914=CARTESIAN_POINT('Ctrl Pts',(0.0111427492599009,-0.0344721681088468,
0.0791397371284662));
#89915=CARTESIAN_POINT('Ctrl Pts',(0.0111216960535753,-0.0344197714290097,
0.0791049403590022));
#89916=CARTESIAN_POINT('Ctrl Pts',(0.0111010304245763,-0.0343667727831696,
0.0790707842841105));
#89917=CARTESIAN_POINT('',(0.0110575590447293,-0.0346945769587026,0.0792395448705892));
#89918=CARTESIAN_POINT('Origin',(0.00812378219310841,-0.0315241814719618,
0.07415));
#89919=CARTESIAN_POINT('',(0.0112297421630861,-0.0347116136489789,0.0792835185442631));
#89920=CARTESIAN_POINT('',(0.0112407003659563,-0.0346945769586885,0.0792768724485571));
#89921=CARTESIAN_POINT('Origin',(0.00246769736427044,-0.03456267041358,
0.0651841143581137));
#89922=CARTESIAN_POINT('Origin',(0.00276678724085952,-0.0345626619669717,
0.0650009658547634));
#89923=CARTESIAN_POINT('Origin',(0.0028064909336834,-0.0345626705879003,
0.0649791328195147));
#89924=CARTESIAN_POINT('Ctrl Pts',(0.010959869296639,-0.0352450361874068,
0.0791535360063471));
#89925=CARTESIAN_POINT('Ctrl Pts',(0.0111485807537295,-0.0349452760959493,
0.0790465712260271));
#89926=CARTESIAN_POINT('Ctrl Pts',(0.0113286990765173,-0.034644428984174,
0.0789256958022957));
#89927=CARTESIAN_POINT('Ctrl Pts',(0.0109620378138651,-0.0352450361874068,
0.0791522425002436));
#89928=CARTESIAN_POINT('Ctrl Pts',(0.0111507004855723,-0.0349452760959493,
0.0790451959329542));
#89929=CARTESIAN_POINT('Ctrl Pts',(0.011330764001042,-0.034644428984174,
0.0789242426293166));
#89930=CARTESIAN_POINT('Ctrl Pts',(0.0111767424897182,-0.0352450361874068,
0.0790241725889964));
#89931=CARTESIAN_POINT('Ctrl Pts',(0.0113605749254622,-0.0349452760959493,
0.0789090283019799));
#89932=CARTESIAN_POINT('Ctrl Pts',(0.0115352119737776,-0.034644428984174,
0.0787803641165208));
#89933=CARTESIAN_POINT('Ctrl Pts',(0.0111788895364767,-0.0352450361874068,
0.079022891889884));
#89934=CARTESIAN_POINT('Ctrl Pts',(0.0113626736698611,-0.0349452760959493,
0.0789076666256701));
#89935=CARTESIAN_POINT('Ctrl Pts',(0.0115372564535049,-0.034644428984174,
0.0787789253313928));
#89936=CARTESIAN_POINT('',(0.0112072494256749,-0.0351951634053333,0.0790049337923587));
#89937=CARTESIAN_POINT('',(0.0114041341068746,-0.0348678972925388,0.0788741312769493));
#89938=CARTESIAN_POINT('Origin',(0.00150454901844235,-0.0345636767886206,
0.0653571463827068));
#89939=CARTESIAN_POINT('Origin',(0.0177065356927869,-0.034694619934102,
0.0879504038316923));
#89940=CARTESIAN_POINT('',(0.01130068498852,-0.0346945769330288,0.0789443105475923));
#89941=CARTESIAN_POINT('',(0.0113520221196127,-0.0346945769458128,0.0789086629662042));
#89942=CARTESIAN_POINT('',(0.0111010304244765,-0.0350221583435276,0.0790707842839142));
#89943=CARTESIAN_POINT('Origin',(0.00187431997553251,-0.0345628458717802,
0.0650498796708099));
#89944=CARTESIAN_POINT('',(0.0111003875509974,-0.0351951360298762,0.0790697275879148));
#89945=CARTESIAN_POINT('Origin',(0.0168044724593228,-0.0351951838366688,
0.088497413369347));
#89946=CARTESIAN_POINT('',(0.0112072754682841,-0.0351951371328746,0.0790049144403668));
#89947=CARTESIAN_POINT('Ctrl Pts',(0.0110261390912839,-0.0350241211494343,
0.0794013164478708));
#89948=CARTESIAN_POINT('Ctrl Pts',(0.0110984738222298,-0.0349144232818962,
0.079361337671611));
#89949=CARTESIAN_POINT('Ctrl Pts',(0.0111700254591262,-0.0348045283579412,
0.0793198397555504));
#89950=CARTESIAN_POINT('Ctrl Pts',(0.0112407003754508,-0.0346945769439157,
0.0792768724427908));
#89951=CARTESIAN_POINT('Ctrl Pts',(0.0110508459545354,-0.0350241211494343,
0.079290723895176));
#89952=CARTESIAN_POINT('Ctrl Pts',(0.0111216573184126,-0.0349144232818962,
0.0792504047920051));
#89953=CARTESIAN_POINT('Ctrl Pts',(0.0111916776416313,-0.0348045283579412,
0.0792085978344172));
#89954=CARTESIAN_POINT('Ctrl Pts',(0.0112608152443571,-0.0346945769439157,
0.079165353234346));
#89955=CARTESIAN_POINT('Ctrl Pts',(0.0110755528177869,-0.0350241211494343,
0.0791801313424811));
#89956=CARTESIAN_POINT('Ctrl Pts',(0.0111448408145954,-0.0349144232818962,
0.0791394719123993));
#89957=CARTESIAN_POINT('Ctrl Pts',(0.0112133298241363,-0.0348045283579412,
0.0790973559132841));
#89958=CARTESIAN_POINT('Ctrl Pts',(0.0112809301132634,-0.0346945769439157,
0.0790538340259012));
#89959=CARTESIAN_POINT('Ctrl Pts',(0.0111002596810383,-0.0350241211494343,
0.0790695387897863));
#89960=CARTESIAN_POINT('Ctrl Pts',(0.0111680243107782,-0.0349144232818962,
0.0790285390327934));
#89961=CARTESIAN_POINT('Ctrl Pts',(0.0112349820066414,-0.0348045283579412,
0.0789861139921509));
#89962=CARTESIAN_POINT('Ctrl Pts',(0.0113010449821697,-0.0346945769439157,
0.0789423148174564));
#89963=CARTESIAN_POINT('',(0.0112706926770453,-0.0346945769458128,0.0791105914983105));
#89964=CARTESIAN_POINT('Ctrl Pts',(0.0112297421613777,-0.0347116136492782,
0.0792835185414432));
#89965=CARTESIAN_POINT('Ctrl Pts',(0.0112075132589665,-0.0347621546531604,
0.0792467786980937));
#89966=CARTESIAN_POINT('Ctrl Pts',(0.0111856752007276,-0.0348133084095606,
0.0792106848404703));
#89967=CARTESIAN_POINT('Ctrl Pts',(0.0111427625471322,-0.0349168561544574,
0.0791397589737028));
#89968=CARTESIAN_POINT('Ctrl Pts',(0.0111217049731347,-0.0349692089015925,
0.0791049550973945));
#89969=CARTESIAN_POINT('Ctrl Pts',(0.0111010304244746,-0.0350221583435,
0.0790707842838725));
#89970=CARTESIAN_POINT('Ctrl Pts',(0.0112058548317998,-0.0351951371254959,
0.0790045648521835));
#89971=CARTESIAN_POINT('Ctrl Pts',(0.011306219914263,-0.0350307338980963,
0.0789408449341354));
#89972=CARTESIAN_POINT('Ctrl Pts',(0.0114038656223842,-0.0348659306897824,
0.0788730312672282));
#89973=CARTESIAN_POINT('Ctrl Pts',(0.0112072754682162,-0.0351951371254959,
0.0790049144402723));
#89974=CARTESIAN_POINT('Ctrl Pts',(0.0113076477781938,-0.0350307338980963,
0.0789411651514578));
#89975=CARTESIAN_POINT('Ctrl Pts',(0.0114052994937281,-0.0348659306897824,
0.0788733218401601));
#89976=CARTESIAN_POINT('Ctrl Pts',(0.0114453756122413,-0.0351951371254959,
0.0790635057683189));
#89977=CARTESIAN_POINT('Ctrl Pts',(0.0115469592611649,-0.0350307338980963,
0.0789948339084156));
#89978=CARTESIAN_POINT('Ctrl Pts',(0.0116456178253884,-0.0348659306897824,
0.0789220221663916));
#89979=CARTESIAN_POINT('Origin',(0.0144374187644613,-0.0308609197409942,
0.0832424537310675));
#89980=CARTESIAN_POINT('',(0.011311081762565,-0.0351951371254959,0.0790304589382414));
#89981=CARTESIAN_POINT('Origin',(0.00745606980158198,-0.0351840467441142,
0.0734366236531671));
#89982=CARTESIAN_POINT('Origin',(0.0155860364218439,-0.0352322614707685,
0.0835032834717993));
#89983=CARTESIAN_POINT('',(0.0115956878952019,-0.0351951142564685,0.0787351592534177));
#89984=CARTESIAN_POINT('',(0.0116934483876602,-0.0351951372916787,0.0786577692109817));
#89985=CARTESIAN_POINT('Origin',(0.00824036220661084,-0.0352875117674211,
0.073830009294775));
#89986=CARTESIAN_POINT('Origin',(0.00145870505261403,-0.0298325076523997,
0.0775955677308751));
#89987=CARTESIAN_POINT('Origin',(0.0104711808944681,-0.0338733549886737,
0.0821958249366702));
#89988=CARTESIAN_POINT('Origin',(0.00812378219310841,-0.0315241814719618,
0.07415));
#89989=CARTESIAN_POINT('',(0.00912185652150633,-0.0327114338380027,0.0800664049569627));
#89990=CARTESIAN_POINT('',(0.00913449179186172,-0.0326943950436593,0.0800642595569543));
#89991=CARTESIAN_POINT('Origin',(0.00626557442642693,-0.0326395653589518,
0.0637092669314688));
#89992=CARTESIAN_POINT('',(0.00912185652151372,-0.0326773559991391,0.0800664049570073));
#89993=CARTESIAN_POINT('Origin',(0.0064092000078735,-0.0326395686496682,
0.0636842521244812));
#89994=CARTESIAN_POINT('',(0.009109216697909,-0.0326943950436595,0.0800685233662416));
#89995=CARTESIAN_POINT('Origin',(0.00631012128950666,-0.0326395670829588,
0.0637009704823884));
#89996=CARTESIAN_POINT('Origin',(0.00645400448005014,-0.0326395670474682,
0.0636774837085538));
#89997=CARTESIAN_POINT('Origin',(0.00812378219310841,-0.0315241814719618,
0.07415));
#89998=CARTESIAN_POINT('',(0.00949138119075433,-0.033212160714423,0.0799920606774468));
#89999=CARTESIAN_POINT('',(0.00950385681755752,-0.0331951640388587,0.0799891261359001));
#90000=CARTESIAN_POINT('Origin',(0.00499368834011878,-0.032641367224474,
0.0640998014851968));
#90001=CARTESIAN_POINT('',(0.00949138119047968,-0.0331781648281979,0.0799920606791099));
#90002=CARTESIAN_POINT('Origin',(0.0064224159774812,-0.0326412105969763,
0.063757281394915));
#90003=CARTESIAN_POINT('',(0.0094788993250309,-0.0331951640388588,0.0799949685678203));
#90004=CARTESIAN_POINT('Origin',(0.00503538584783144,-0.0326412118339323,
0.0640819743322511));
#90005=CARTESIAN_POINT('Origin',(0.00646769267691926,-0.0326413655043729,
0.0637547409009615));
#90006=CARTESIAN_POINT('Origin',(0.00812378219310841,-0.0315241814719618,
0.07415));
#90007=CARTESIAN_POINT('',(0.00874839290883649,-0.0322104233323589,0.0801173998890733));
#90008=CARTESIAN_POINT('',(0.00876113795713054,-0.0321934096636184,0.0801160520975022));
#90009=CARTESIAN_POINT('Origin',(0.00759179442432658,-0.0326387220923027,
0.0636054529442552));
#90010=CARTESIAN_POINT('',(0.00874839290805402,-0.0321763980308051,0.0801173998898277));
#90011=CARTESIAN_POINT('Origin',(0.0064167606925355,-0.0326386251392104,
0.0637347958322026));
#90012=CARTESIAN_POINT('',(0.00873564501100219,-0.0321934096636185,0.080118720456855));
#90013=CARTESIAN_POINT('Origin',(0.00763710227032919,-0.0326386231416166,
0.0636070659319768));
#90014=CARTESIAN_POINT('Origin',(0.00646075389492646,-0.0326387237046156,
0.0637238440867132));
#90015=CARTESIAN_POINT('Origin',(0.00812378219310841,-0.0315241814719618,
0.07415));
#90016=CARTESIAN_POINT('',(0.010212801619691,-0.0342105180190367,0.0797745886798295));
#90017=CARTESIAN_POINT('',(0.0102248110767376,-0.0341934961088739,0.079770113667014));
#90018=CARTESIAN_POINT('Origin',(0.00488392365083045,-0.0345621723898461,
0.0640853090295975));
#90019=CARTESIAN_POINT('',(0.0102128016191596,-0.0341764758832441,0.0797745886808157));
#90020=CARTESIAN_POINT('Origin',(0.00396783352876945,-0.0345621027326488,
0.064431130373545));
#90021=CARTESIAN_POINT('',(0.0102007826323748,-0.034193496108874,0.0797790380328514));
#90022=CARTESIAN_POINT('Origin',(0.00492794907776644,-0.0345621026475164,
0.0640745358026033));
#90023=CARTESIAN_POINT('Origin',(0.0040082180216118,-0.0345621724697839,
0.0644105540793245));
#90024=CARTESIAN_POINT('Origin',(0.00812378219310841,-0.0315241814719618,
0.07415));
#90025=CARTESIAN_POINT('',(0.00985550857176248,-0.0337108120655544,0.0798946604541967));
#90026=CARTESIAN_POINT('',(0.00986777531920442,-0.0336938721132327,0.0798909483516344));
#90027=CARTESIAN_POINT('Origin',(0.0062033642301923,-0.0345562527952255,
0.0639071636382977));
#90028=CARTESIAN_POINT('',(0.00985550857213072,-0.0336769361243754,0.0798946604554315));
#90029=CARTESIAN_POINT('Ctrl Pts',(0.00986777531920224,-0.0336938721132364,
0.0798909483516442));
#90030=CARTESIAN_POINT('Ctrl Pts',(0.00986573166119598,-0.0336910493069898,
0.0798915691768627));
#90031=CARTESIAN_POINT('Ctrl Pts',(0.00986368761768907,-0.0336882265912827,
0.0798921889272351));
#90032=CARTESIAN_POINT('Ctrl Pts',(0.00985959870904877,-0.0336825812713049,
0.079893426293213));
#90033=CARTESIAN_POINT('Ctrl Pts',(0.00985755384389822,-0.0336797586670127,
0.0798940439087966));
#90034=CARTESIAN_POINT('Ctrl Pts',(0.00985550857213048,-0.033676936124375,
0.0798946604554315));
#90035=CARTESIAN_POINT('',(0.00984323392392004,-0.033693872113232,0.0798983463487693));
#90036=CARTESIAN_POINT('Ctrl Pts',(0.0098555085721307,-0.0336769361243754,
0.0798946604554314));
#90037=CARTESIAN_POINT('Ctrl Pts',(0.00985346330039176,-0.0336797586669733,
0.0798952770020577));
#90038=CARTESIAN_POINT('Ctrl Pts',(0.00985141777674278,-0.0336825812712258,
0.0798958924330988));
#90039=CARTESIAN_POINT('Ctrl Pts',(0.00984732623777634,-0.0336882265864016,
0.0798971210608983));
#90040=CARTESIAN_POINT('Ctrl Pts',(0.00984528022254873,-0.0336910492972279,
0.0798977342576694));
#90041=CARTESIAN_POINT('Ctrl Pts',(0.00984323392393173,-0.0336938721132382,
0.0798983463487797));
#90042=CARTESIAN_POINT('Origin',(0.00406327432682986,-0.0345562523471192,
0.0645522933807731));
#90043=CARTESIAN_POINT('Ctrl Pts',(0.00931122775127138,-0.033693872113265,
0.0797774750382086));
#90044=CARTESIAN_POINT('Ctrl Pts',(0.00942903390460924,-0.0335278710435226,
0.0797526169282116));
#90045=CARTESIAN_POINT('Ctrl Pts',(0.0095460190701494,-0.0333620469224385,
0.0797240731929003));
#90046=CARTESIAN_POINT('Ctrl Pts',(0.0096622366800184,-0.0331951640388587,
0.079691810178179));
#90047=CARTESIAN_POINT('Ctrl Pts',(0.00939285433319994,-0.033693872113265,
0.0797583666383155));
#90048=CARTESIAN_POINT('Ctrl Pts',(0.00951026046928805,-0.0335278710435226,
0.0797317997488816));
#90049=CARTESIAN_POINT('Ctrl Pts',(0.00962679217142473,-0.0333620469224385,
0.0797015603797149));
#90050=CARTESIAN_POINT('Ctrl Pts',(0.00974250236417658,-0.0331951640388587,
0.0796676141088612));
#90051=CARTESIAN_POINT('Ctrl Pts',(0.00947448091512851,-0.033693872113265,
0.0797392582384225));
#90052=CARTESIAN_POINT('Ctrl Pts',(0.00959148703396686,-0.0335278710435226,
0.0797109825695516));
#90053=CARTESIAN_POINT('Ctrl Pts',(0.00970756527270005,-0.0333620469224385,
0.0796790475665296));
#90054=CARTESIAN_POINT('Ctrl Pts',(0.00982276804833477,-0.0331951640388587,
0.0796434180395434));
#90055=CARTESIAN_POINT('Ctrl Pts',(0.00955610749705708,-0.033693872113265,
0.0797201498385294));
#90056=CARTESIAN_POINT('Ctrl Pts',(0.00967271359864567,-0.0335278710435226,
0.0796901653902217));
#90057=CARTESIAN_POINT('Ctrl Pts',(0.00978833837397538,-0.0333620469224385,
0.0796565347533442));
#90058=CARTESIAN_POINT('Ctrl Pts',(0.00990303373249296,-0.0331951640388587,
0.0796192219702256));
#90059=CARTESIAN_POINT('',(0.00955610749709523,-0.0336938721132548,0.0797201498385196));
#90060=CARTESIAN_POINT('',(0.00978374541810405,-0.0333679846208752,0.0796566003520759));
#90061=CARTESIAN_POINT('Ctrl Pts',(0.00955610749710581,-0.0336938721132388,
0.0797201498385436));
#90062=CARTESIAN_POINT('Ctrl Pts',(0.00957785040492485,-0.0336629187933892,
0.0797145588009588));
#90063=CARTESIAN_POINT('Ctrl Pts',(0.00959955362107873,-0.0336319952301031,
0.0797088422380559));
#90064=CARTESIAN_POINT('Ctrl Pts',(0.0096755707765491,-0.0335235892595445,
0.0796883433074983));
#90065=CARTESIAN_POINT('Ctrl Pts',(0.00972975960390407,-0.0334458668645755,
0.079672874332095));
#90066=CARTESIAN_POINT('Ctrl Pts',(0.00978374541112119,-0.0333679869902197,
0.0796566003287654));
#90067=CARTESIAN_POINT('Ctrl Pts',(0.00978374562952784,-0.0333679128829496,
0.0796566010578595));
#90068=CARTESIAN_POINT('Ctrl Pts',(0.00978361479406216,-0.0333391359256877,
0.0796561670370252));
#90069=CARTESIAN_POINT('Ctrl Pts',(0.00978351673985758,-0.033310357818174,
0.0796558417615556));
#90070=CARTESIAN_POINT('Ctrl Pts',(0.00978345138122428,-0.0332815781851602,
0.0796556249471851));
#90071=CARTESIAN_POINT('Ctrl Pts',(0.00978338596645222,-0.033252773832338,
0.0796554079465853));
#90072=CARTESIAN_POINT('Ctrl Pts',(0.00978335330633778,-0.0332239690390847,
0.079655299603122));
#90073=CARTESIAN_POINT('Ctrl Pts',(0.00978335330633771,-0.0331951640388587,
0.079655299603122));
#90074=CARTESIAN_POINT('',(0.00966367288018325,-0.0331951640388587,0.0796913772360182));
#90075=CARTESIAN_POINT('',(0.00972351309327069,-0.0331951640388687,0.0796733384195801));
#90076=CARTESIAN_POINT('',(0.00943470755476085,-0.0335216366559682,0.0797499642582251));
#90077=CARTESIAN_POINT('Origin',(0.00446956781469179,-0.0326434571526632,
0.0638528559558026));
#90078=CARTESIAN_POINT('',(0.0094343978995946,-0.0336938721132327,0.0797486414843167));
#90079=CARTESIAN_POINT('Origin',(0.0119235566863759,-0.0336938867896348,
0.0903817463226168));
#90080=CARTESIAN_POINT('',(0.00949525269835491,-0.0336938721132538,0.0797343956614282));
#90081=CARTESIAN_POINT('Ctrl Pts',(0.00926134240707744,-0.0335235895815171,
0.0800411761779483));
#90082=CARTESIAN_POINT('Ctrl Pts',(0.00934244604582544,-0.0334144449262748,
0.0800255154219531));
#90083=CARTESIAN_POINT('Ctrl Pts',(0.00942331932339555,-0.0333049234473147,
0.0800081611335073));
#90084=CARTESIAN_POINT('Ctrl Pts',(0.0095038568175559,-0.0331951640388587,
0.0799891261359032));
#90085=CARTESIAN_POINT('Ctrl Pts',(0.00931901506428282,-0.0335235895815171,
0.0799436311263217));
#90086=CARTESIAN_POINT('Ctrl Pts',(0.00939877580334664,-0.0334144449262748,
0.0799271763926531));
#90087=CARTESIAN_POINT('Ctrl Pts',(0.00947828823542234,-0.0333049234473147,
0.0799090549576465));
#90088=CARTESIAN_POINT('Ctrl Pts',(0.00955744858952339,-0.0331951640388587,
0.0798892807831653));
#90089=CARTESIAN_POINT('Ctrl Pts',(0.0093766877214882,-0.0335235895815171,
0.0798460860746951));
#90090=CARTESIAN_POINT('Ctrl Pts',(0.00945510556086785,-0.0334144449262748,
0.079828837363353));
#90091=CARTESIAN_POINT('Ctrl Pts',(0.00953325714744913,-0.0333049234473147,
0.0798099487817857));
#90092=CARTESIAN_POINT('Ctrl Pts',(0.00961104036149088,-0.0331951640388587,
0.0797894354304274));
#90093=CARTESIAN_POINT('Ctrl Pts',(0.00943436037869357,-0.0335235895815171,
0.0797485410230685));
#90094=CARTESIAN_POINT('Ctrl Pts',(0.00951143531838905,-0.0334144449262748,
0.079730498334053));
#90095=CARTESIAN_POINT('Ctrl Pts',(0.00958822605947593,-0.0333049234473147,
0.0797108426059249));
#90096=CARTESIAN_POINT('Ctrl Pts',(0.00966463213345837,-0.0331951640388587,
0.0796895900776896));
#90097=CARTESIAN_POINT('',(0.00958376484888039,-0.0331951640388687,0.0798402516859692));
#90098=CARTESIAN_POINT('Ctrl Pts',(0.00949138119003446,-0.0332121607145987,
0.0799920606743897));
#90099=CARTESIAN_POINT('Ctrl Pts',(0.00948160041949585,-0.0332625444108916,
0.0799502795272426));
#90100=CARTESIAN_POINT('Ctrl Pts',(0.00947198818698186,-0.0333135300745102,
0.079909218334825));
#90101=CARTESIAN_POINT('Ctrl Pts',(0.00945309364375762,-0.0334167177151439,
0.0798285052981974));
#90102=CARTESIAN_POINT('Ctrl Pts',(0.00944381724049779,-0.0334688874167211,
0.0797888786892237));
#90103=CARTESIAN_POINT('Ctrl Pts',(0.00943470755466547,-0.0335216366556511,
0.0797499642578176));
#90104=CARTESIAN_POINT('Ctrl Pts',(0.00955610749707543,-0.0336938721132388,
0.0797201498385247));
#90105=CARTESIAN_POINT('Ctrl Pts',(0.00958871143245195,-0.0336474569764957,
0.0797117659632246));
#90106=CARTESIAN_POINT('Ctrl Pts',(0.00962121498994013,-0.033601104548885,
0.0797030009921639));
#90107=CARTESIAN_POINT('Ctrl Pts',(0.00970350652446392,-0.0334837508592656,
0.0796808101006312));
#90108=CARTESIAN_POINT('Ctrl Pts',(0.00978510436048511,-0.0333660264659097,
0.0796561904849163));
#90109=CARTESIAN_POINT('Ctrl Pts',(0.00984495668250204,-0.0336938721132388,
0.0798994155278473));
#90110=CARTESIAN_POINT('Ctrl Pts',(0.00987860991944483,-0.0336474569764957,
0.0798893409224146));
#90111=CARTESIAN_POINT('Ctrl Pts',(0.00991214291446956,-0.033601104548885,
0.0798788730536715));
#90112=CARTESIAN_POINT('Ctrl Pts',(0.00999704074815335,-0.0334837508592656,
0.0798523708167278));
#90113=CARTESIAN_POINT('Ctrl Pts',(0.0100811159847366,-0.0333660264659097,
0.0798233645187791));
#90114=CARTESIAN_POINT('Ctrl Pts',(0.00985550857213072,-0.0336769361243754,
0.0798946604554315));
#90115=CARTESIAN_POINT('Ctrl Pts',(0.00984341164762209,-0.033627901837843,
0.0798545312960567));
#90116=CARTESIAN_POINT('Ctrl Pts',(0.00983114069370158,-0.0335767825754286,
0.0798138248284599));
#90117=CARTESIAN_POINT('Ctrl Pts',(0.00980709668019615,-0.0334733171799197,
0.0797340635594466));
#90118=CARTESIAN_POINT('Ctrl Pts',(0.00979530746094694,-0.0334209631321944,
0.0796949551515336));
#90119=CARTESIAN_POINT('Ctrl Pts',(0.00978374540820146,-0.0333679869844681,
0.0796566003236606));
#90120=CARTESIAN_POINT('',(0.00969967071051763,-0.0336938721132534,0.0798092480936544));
#90121=CARTESIAN_POINT('Ctrl Pts',(0.00962638780623428,-0.034243627687391,
0.0797016603481663));
#90122=CARTESIAN_POINT('Ctrl Pts',(0.00983577212800967,-0.033943005420181,
0.0796449886432224));
#90123=CARTESIAN_POINT('Ctrl Pts',(0.0100402928658562,-0.0336441434784052,
0.0795727062516094));
#90124=CARTESIAN_POINT('Ctrl Pts',(0.00962878590613157,-0.034243627687391,
0.0797009538661194));
#90125=CARTESIAN_POINT('Ctrl Pts',(0.0098381435824973,-0.033943005420181,
0.0796441917153468));
#90126=CARTESIAN_POINT('Ctrl Pts',(0.0100426309378806,-0.0336441434784052,
0.0795718211418938));
#90127=CARTESIAN_POINT('Ctrl Pts',(0.00986859589586089,-0.034243627687391,
0.0796303056614287));
#90128=CARTESIAN_POINT('Ctrl Pts',(0.0100752890312612,-0.033943005420181,
0.0795644989277917));
#90129=CARTESIAN_POINT('Ctrl Pts',(0.0102764381403202,-0.0336441434784052,
0.079483310170329));
#90130=CARTESIAN_POINT('Ctrl Pts',(0.00987101797675716,-0.034243627687391,
0.0796295921145613));
#90131=CARTESIAN_POINT('Ctrl Pts',(0.0100776842002937,-0.033943005420181,
0.0795636940306374));
#90132=CARTESIAN_POINT('Ctrl Pts',(0.0102787995930649,-0.0336441434784052,
0.0794824162095161));
#90133=CARTESIAN_POINT('',(0.00990303373249299,-0.0341934961088741,0.0796192219702256));
#90134=CARTESIAN_POINT('',(0.0101262321469139,-0.0338664212863443,0.0795415043528434));
#90135=CARTESIAN_POINT('Origin',(0.00521293353933639,-0.0345610720404037,
0.0635550972214448));
#90136=CARTESIAN_POINT('Origin',(0.0139443877772785,-0.0336938005072992,
0.0898216022135932));
#90137=CARTESIAN_POINT('',(0.0100085802132244,-0.0336938721132327,0.0795837520575904));
#90138=CARTESIAN_POINT('',(0.010067169678664,-0.0336938721132427,0.079561991438568));
#90139=CARTESIAN_POINT('',(0.00978374540819636,-0.0340203938281605,0.0796566003236621));
#90140=CARTESIAN_POINT('Origin',(0.00569010038791695,-0.0345589643244747,
0.0634930606758832));
#90141=CARTESIAN_POINT('',(0.00978335330633812,-0.0341934961088739,0.0796552996031219));
#90142=CARTESIAN_POINT('Origin',(0.0129637971165719,-0.0341934220717703,
0.0902057970063492));
#90143=CARTESIAN_POINT('',(0.00984319351942556,-0.0341934961088841,0.0796372607866838));
#90144=CARTESIAN_POINT('Ctrl Pts',(0.00962900505598272,-0.0340223579322396,
0.0799581239770792));
#90145=CARTESIAN_POINT('Ctrl Pts',(0.00970911423384991,-0.0339125849573575,
0.0799373630280142));
#90146=CARTESIAN_POINT('Ctrl Pts',(0.00978873741652145,-0.0338030433565231,
0.0799149585935938));
#90147=CARTESIAN_POINT('Ctrl Pts',(0.00986777531920265,-0.0336938721132327,
0.0798909483516383));
#90148=CARTESIAN_POINT('Ctrl Pts',(0.00968043906566049,-0.0340223579322396,
0.0798571501068014));
#90149=CARTESIAN_POINT('Ctrl Pts',(0.00975915555050563,-0.0339125849573575,
0.0798356797485974));
#90150=CARTESIAN_POINT('Ctrl Pts',(0.00983737233566366,-0.0338030433565231,
0.079812595229041));
#90151=CARTESIAN_POINT('Ctrl Pts',(0.00991499201198173,-0.0336938721132327,
0.0797879349362332));
#90152=CARTESIAN_POINT('Ctrl Pts',(0.00973187307533826,-0.0340223579322396,
0.0797561762365236));
#90153=CARTESIAN_POINT('Ctrl Pts',(0.00980919686716136,-0.0339125849573575,
0.0797339964691805));
#90154=CARTESIAN_POINT('Ctrl Pts',(0.00988600725480587,-0.0338030433565231,
0.0797102318644881));
#90155=CARTESIAN_POINT('Ctrl Pts',(0.00996220870476081,-0.0336938721132327,
0.0796849215208281));
#90156=CARTESIAN_POINT('Ctrl Pts',(0.00978330708501602,-0.0340223579322396,
0.0796552023662457));
#90157=CARTESIAN_POINT('Ctrl Pts',(0.00985923818381708,-0.0339125849573575,
0.0796323131897637));
#90158=CARTESIAN_POINT('Ctrl Pts',(0.00993464217394808,-0.0338030433565231,
0.0796078684999353));
#90159=CARTESIAN_POINT('Ctrl Pts',(0.0100094253975399,-0.0336938721132327,
0.079581908105423));
#90160=CARTESIAN_POINT('',(0.0099381777662244,-0.0336938721132427,0.0797373502046224));
#90161=CARTESIAN_POINT('Ctrl Pts',(0.00985550857071632,-0.0337108120662692,
0.0798946604507397));
#90162=CARTESIAN_POINT('Ctrl Pts',(0.00984309807969535,-0.0337611408993968,
0.0798534910963519));
#90163=CARTESIAN_POINT('Ctrl Pts',(0.00983091405260156,-0.0338121088780625,
0.0798130729913432));
#90164=CARTESIAN_POINT('Ctrl Pts',(0.00980698782678264,-0.0339153382773241,
0.0797337024597311));
#90165=CARTESIAN_POINT('Ctrl Pts',(0.00979525575034011,-0.0339675558473111,
0.0796947836118023));
#90166=CARTESIAN_POINT('Ctrl Pts',(0.00978374540818986,-0.0340203938281304,
0.0796566003236224));
#90167=CARTESIAN_POINT('Ctrl Pts',(0.00990124673052261,-0.0341934961088741,
0.0796182628008755));
#90168=CARTESIAN_POINT('Ctrl Pts',(0.0100142987559685,-0.0340287516182428,
0.0795815151218721));
#90169=CARTESIAN_POINT('Ctrl Pts',(0.0101257353711686,-0.0338644633275951,
0.0795401263170781));
#90170=CARTESIAN_POINT('Ctrl Pts',(0.00990303373249295,-0.0341934961088741,
0.0796192219702256));
#90171=CARTESIAN_POINT('Ctrl Pts',(0.0100161055880095,-0.0340287516182428,
0.0795824373463643));
#90172=CARTESIAN_POINT('Ctrl Pts',(0.0101275604893769,-0.0338644633275951,
0.0795410108086892));
#90173=CARTESIAN_POINT('Ctrl Pts',(0.0102007826323912,-0.0341934961088741,
0.0797790380328602));
#90174=CARTESIAN_POINT('Ctrl Pts',(0.0103171585590977,-0.0340287516182428,
0.0797360976850636));
#90175=CARTESIAN_POINT('Ctrl Pts',(0.0104316602876492,-0.0338644633275951,
0.0796883841236326));
#90176=CARTESIAN_POINT('Ctrl Pts',(0.0102128016173517,-0.0341764758837552,
0.0797745886805576));
#90177=CARTESIAN_POINT('Ctrl Pts',(0.0101978566280018,-0.0341260050040553,
0.0797343500238654));
#90178=CARTESIAN_POINT('Ctrl Pts',(0.0101831713820069,-0.0340749269148336,
0.0796948108232568));
#90179=CARTESIAN_POINT('Ctrl Pts',(0.010154309167467,-0.0339715436306863,
0.0796171006270857));
#90180=CARTESIAN_POINT('Ctrl Pts',(0.0101401431541839,-0.0339192778237251,
0.079578959110878));
#90181=CARTESIAN_POINT('Ctrl Pts',(0.0101262321456331,-0.0338664212854771,
0.0795415043545428));
#90182=CARTESIAN_POINT('',(0.0100519081824439,-0.0341934961088841,0.0796991300015486));
#90183=CARTESIAN_POINT('Ctrl Pts',(0.0100071740567672,-0.0346945769586966,
0.0795842743158962));
#90184=CARTESIAN_POINT('Ctrl Pts',(0.0101209971080783,-0.0345275153362944,
0.0795448259192429));
#90185=CARTESIAN_POINT('Ctrl Pts',(0.0102336089840957,-0.0343603235965185,
0.0795017876890168));
#90186=CARTESIAN_POINT('Ctrl Pts',(0.0103446785207095,-0.034193496108874,
0.079455291863277));
#90187=CARTESIAN_POINT('Ctrl Pts',(0.010085762062824,-0.0346945769586966,
0.0795550860710852));
#90188=CARTESIAN_POINT('Ctrl Pts',(0.0101989737546612,-0.0345275153362944,
0.0795139916171801));
#90189=CARTESIAN_POINT('Ctrl Pts',(0.0103109223460903,-0.0343603235965185,
0.0794693261306403));
#90190=CARTESIAN_POINT('Ctrl Pts',(0.0104212787062321,-0.034193496108874,
0.0794212266330705));
#90191=CARTESIAN_POINT('Ctrl Pts',(0.0101643500688808,-0.0346945769586966,
0.0795258978262741));
#90192=CARTESIAN_POINT('Ctrl Pts',(0.0102769504012441,-0.0345275153362944,
0.0794831573151173));
#90193=CARTESIAN_POINT('Ctrl Pts',(0.010388235708085,-0.0343603235965185,
0.0794368645722637));
#90194=CARTESIAN_POINT('Ctrl Pts',(0.0104978788917548,-0.034193496108874,
0.079387161402864));
#90195=CARTESIAN_POINT('Ctrl Pts',(0.0102429380749375,-0.0346945769586966,
0.0794967095814631));
#90196=CARTESIAN_POINT('Ctrl Pts',(0.010354927047827,-0.0345275153362944,
0.0794523230130545));
#90197=CARTESIAN_POINT('Ctrl Pts',(0.0104655490700796,-0.0343603235965185,
0.0794044030138871));
#90198=CARTESIAN_POINT('Ctrl Pts',(0.0105744790772775,-0.034193496108874,
0.0793530961726575));
#90199=CARTESIAN_POINT('',(0.0102429380749483,-0.0346945769586966,0.0794967095814589));
#90200=CARTESIAN_POINT('',(0.010460816127266,-0.0343667727833015,0.0794051305779478));
#90201=CARTESIAN_POINT('Origin',(0.00387804142253948,-0.0345626461565472,
0.0639344045683027));
#90202=CARTESIAN_POINT('Origin',(0.0149518158849197,-0.0341934771027857,
0.0895037233757803));
#90203=CARTESIAN_POINT('',(0.0103460491095624,-0.034193496108874,0.0794546823422364));
#90204=CARTESIAN_POINT('',(0.0104031566015012,-0.034193496108884,0.0794292857998518));
#90205=CARTESIAN_POINT('',(0.0101262321451442,-0.0345211942962613,0.0795415043531111));
#90206=CARTESIAN_POINT('Origin',(0.00432992614611196,-0.0345625596120916,
0.0637701170572003));
#90207=CARTESIAN_POINT('',(0.0101257591440837,-0.0346945769586885,0.0795402308195257));
#90208=CARTESIAN_POINT('Origin',(0.0139777595158368,-0.034694568585392,
0.0899115667198707));
#90209=CARTESIAN_POINT('',(0.010184348609526,-0.0346945769587026,0.0795184702005023));
#90210=CARTESIAN_POINT('Ctrl Pts',(0.00999073087892141,-0.0345231616327842,
0.0798521489461946));
#90211=CARTESIAN_POINT('Ctrl Pts',(0.0100693269741611,-0.0344132092796988,
0.0798264156870141));
#90212=CARTESIAN_POINT('Ctrl Pts',(0.0101473867420356,-0.0343032738558979,
0.0797990580573173));
#90213=CARTESIAN_POINT('Ctrl Pts',(0.0102248110767358,-0.0341934961088739,
0.0797701136670187));
#90214=CARTESIAN_POINT('Ctrl Pts',(0.0100357231003355,-0.0345231616327842,
0.079748144926316));
#90215=CARTESIAN_POINT('Ctrl Pts',(0.0101128856465871,-0.0344132092796988,
0.0797217915127073));
#90216=CARTESIAN_POINT('Ctrl Pts',(0.0101894991120329,-0.0343032738558979,
0.0796938434124094));
#90217=CARTESIAN_POINT('Ctrl Pts',(0.0102654662631213,-0.0341934961088739,
0.0796643389443358));
#90218=CARTESIAN_POINT('Ctrl Pts',(0.0100807153217496,-0.0345231616327842,
0.0796441409064373));
#90219=CARTESIAN_POINT('Ctrl Pts',(0.0101564443190132,-0.0344132092796988,
0.0796171673384005));
#90220=CARTESIAN_POINT('Ctrl Pts',(0.0102316114820302,-0.0343032738558979,
0.0795886287675016));
#90221=CARTESIAN_POINT('Ctrl Pts',(0.0103061214495069,-0.0341934961088739,
0.0795585642216529));
#90222=CARTESIAN_POINT('Ctrl Pts',(0.0101257075431637,-0.0345231616327842,
0.0795401368865587));
#90223=CARTESIAN_POINT('Ctrl Pts',(0.0102000029914392,-0.0344132092796988,
0.0795125431640937));
#90224=CARTESIAN_POINT('Ctrl Pts',(0.0102737238520275,-0.0343032738558979,
0.0794834141225937));
#90225=CARTESIAN_POINT('Ctrl Pts',(0.0103467766358924,-0.0341934961088739,
0.0794527894989701));
#90226=CARTESIAN_POINT('',(0.01028543009316,-0.0341934961088839,0.0796123980046352));
#90227=CARTESIAN_POINT('Ctrl Pts',(0.010212801618482,-0.0342105180195389,
0.0797745886765839));
#90228=CARTESIAN_POINT('Ctrl Pts',(0.0101978398409612,-0.0342610556240768,
0.0797343047790751));
#90229=CARTESIAN_POINT('Ctrl Pts',(0.0101831465448014,-0.0343122189869054,
0.0796947437552769));
#90230=CARTESIAN_POINT('Ctrl Pts',(0.010154284035293,-0.0344158119695089,
0.079617032776534));
#90231=CARTESIAN_POINT('Ctrl Pts',(0.0101401266269656,-0.0344681990449969,
0.0795789146060657));
#90232=CARTESIAN_POINT('Ctrl Pts',(0.010126232145131,-0.0345211942962363,
0.0795415043530806));
#90233=CARTESIAN_POINT('Ctrl Pts',(0.0102410948239851,-0.0346945769586932,
0.0794958647185508));
#90234=CARTESIAN_POINT('Ctrl Pts',(0.0103147635418812,-0.0345846629175835,
0.0794666870802989));
#90235=CARTESIAN_POINT('Ctrl Pts',(0.0103878414609988,-0.034474692504983,
0.0794359810196021));
#90236=CARTESIAN_POINT('Ctrl Pts',(0.0104602351079724,-0.0343648066252516,
0.0794037862673067));
#90237=CARTESIAN_POINT('Ctrl Pts',(0.0103441080056568,-0.0346945769586932,
0.0795430813041972));
#90238=CARTESIAN_POINT('Ctrl Pts',(0.0104184273919688,-0.0345846629175835,
0.0795124840922336));
#90239=CARTESIAN_POINT('Ctrl Pts',(0.0104921267344367,-0.034474692504983,
0.079480344759803));
#90240=CARTESIAN_POINT('Ctrl Pts',(0.0105651117710401,-0.0343648066252516,
0.0794467048775126));
#90241=CARTESIAN_POINT('Ctrl Pts',(0.0104471211873285,-0.0346945769586932,
0.0795902978898435));
#90242=CARTESIAN_POINT('Ctrl Pts',(0.0105220912420564,-0.0345846629175835,
0.0795582811041683));
#90243=CARTESIAN_POINT('Ctrl Pts',(0.0105964120078746,-0.034474692504983,
0.0795247085000038));
#90244=CARTESIAN_POINT('Ctrl Pts',(0.0106699884341078,-0.0343648066252516,
0.0794896234877185));
#90245=CARTESIAN_POINT('Ctrl Pts',(0.0105501343690003,-0.0346945769586932,
0.0796375144754899));
#90246=CARTESIAN_POINT('Ctrl Pts',(0.010625755092144,-0.0345846629175835,
0.0796040781161031));
#90247=CARTESIAN_POINT('Ctrl Pts',(0.0107006972813125,-0.034474692504983,
0.0795690722402047));
#90248=CARTESIAN_POINT('Ctrl Pts',(0.0107748650971756,-0.0343648066252516,
0.0795325420979245));
#90249=CARTESIAN_POINT('',(0.0105618502623488,-0.0346775396663675,0.0796323192236938));
#90250=CARTESIAN_POINT('',(0.0105501343689865,-0.0346945769586885,0.0796375144754808));
#90251=CARTESIAN_POINT('Origin',(0.00367662592449391,-0.0345626617272025,
0.0645258111618288));
#90252=CARTESIAN_POINT('Ctrl Pts',(0.010561850260972,-0.0346775396659522,
0.0796323192206047));
#90253=CARTESIAN_POINT('Ctrl Pts',(0.0105443943775465,-0.034626974852986,
0.0795930673529158));
#90254=CARTESIAN_POINT('Ctrl Pts',(0.0105272488665522,-0.0345757904818561,
0.0795545133987788));
#90255=CARTESIAN_POINT('Ctrl Pts',(0.0104935638856951,-0.0344721679344753,
0.0794787682543209));
#90256=CARTESIAN_POINT('Ctrl Pts',(0.0104770379896808,-0.0344197716860446,
0.0794416075865975));
#90257=CARTESIAN_POINT('Ctrl Pts',(0.0104608161270357,-0.034366772783195,
0.0794051305782049));
#90258=CARTESIAN_POINT('',(0.0103965362219774,-0.0346945769587026,0.0795671120284798));
#90259=CARTESIAN_POINT('Ctrl Pts',(0.00823716696603865,-0.0321934096636942,
0.0799002417026225));
#90260=CARTESIAN_POINT('Ctrl Pts',(0.00834009355419282,-0.0320508460844559,
0.079898212169182));
#90261=CARTESIAN_POINT('Ctrl Pts',(0.00844288800580094,-0.0319086045663539,
0.079893418731684));
#90262=CARTESIAN_POINT('Ctrl Pts',(0.00854532983602395,-0.0317669892868596,
0.0798858899328736));
#90263=CARTESIAN_POINT('Ctrl Pts',(0.00832094259117809,-0.0321934096636942,
0.0798967664673334));
#90264=CARTESIAN_POINT('Ctrl Pts',(0.00842380697427553,-0.0320508460844559,
0.0798932373900978));
#90265=CARTESIAN_POINT('Ctrl Pts',(0.00852649897794681,-0.0319086045663539,
0.0798869472107927));
#90266=CARTESIAN_POINT('Ctrl Pts',(0.00862879860325792,-0.0317669892868596,
0.0798779276767516));
#90267=CARTESIAN_POINT('Ctrl Pts',(0.00840471821631753,-0.0321934096636942,
0.0798932912320445));
#90268=CARTESIAN_POINT('Ctrl Pts',(0.00850752039435823,-0.0320508460844559,
0.0798882626110136));
#90269=CARTESIAN_POINT('Ctrl Pts',(0.00861010995009268,-0.0319086045663539,
0.0798804756899015));
#90270=CARTESIAN_POINT('Ctrl Pts',(0.0087122673704919,-0.0317669892868596,
0.0798699654206294));
#90271=CARTESIAN_POINT('Ctrl Pts',(0.00848849384145697,-0.0321934096636942,
0.0798898159967555));
#90272=CARTESIAN_POINT('Ctrl Pts',(0.00859123381444095,-0.0320508460844559,
0.0798832878319295));
#90273=CARTESIAN_POINT('Ctrl Pts',(0.00869372092223854,-0.0319086045663539,
0.0798740041690102));
#90274=CARTESIAN_POINT('Ctrl Pts',(0.00879573613772587,-0.0317669892868596,
0.0798620031645074));
#90275=CARTESIAN_POINT('',(0.00848699507896817,-0.0321934096636943,0.0798898781693993));
#90276=CARTESIAN_POINT('',(0.00872250888832501,-0.0318665617511176,0.0798701093812739));
#90277=CARTESIAN_POINT('Origin',(0.00804615423106609,-0.0326371944421524,
0.0631858797206531));
#90278=CARTESIAN_POINT('Origin',(0.00986358784496523,-0.0316939261509064,
0.09077173903016));
#90279=CARTESIAN_POINT('',(0.00836242081836886,-0.0320197221621732,0.0798963589143967));
#90280=CARTESIAN_POINT('Ctrl Pts',(0.0083626014758925,-0.032019739209466,
0.0798963986351664));
#90281=CARTESIAN_POINT('Ctrl Pts',(0.00839184099761886,-0.0319792716575958,
0.0798951833989777));
#90282=CARTESIAN_POINT('Ctrl Pts',(0.00842120436430534,-0.0319386439829634,
0.0798937397202264));
#90283=CARTESIAN_POINT('Ctrl Pts',(0.00845072198661272,-0.0318979099381565,
0.0798920576360069));
#90284=CARTESIAN_POINT('Ctrl Pts',(0.00848023902548181,-0.0318571766984891,
0.079890375585035));
#90285=CARTESIAN_POINT('Ctrl Pts',(0.00850976039037138,-0.0318163871833566,
0.0798884654661008));
#90286=CARTESIAN_POINT('Ctrl Pts',(0.00853918476730417,-0.0317755399638303,
0.0798863373630329));
#90287=CARTESIAN_POINT('',(0.00836210249096908,-0.0321934096636184,0.0798950590454431));
#90288=CARTESIAN_POINT('Origin',(0.00847876190393271,-0.0324111959063637,
0.0821999623964788));
#90289=CARTESIAN_POINT('',(0.00842454878497862,-0.0321934096636663,0.0798924686074312));
#90290=CARTESIAN_POINT('Ctrl Pts',(0.00848550269921074,-0.0321934096636619,
0.0798885046738444));
#90291=CARTESIAN_POINT('Ctrl Pts',(0.00860414169261537,-0.0320287467381911,
0.0798810263917523));
#90292=CARTESIAN_POINT('Ctrl Pts',(0.00872237022849805,-0.0318646057455573,
0.079868651062983));
#90293=CARTESIAN_POINT('Ctrl Pts',(0.00848699507888224,-0.0321934096636619,
0.0798898781694046));
#90294=CARTESIAN_POINT('Ctrl Pts',(0.0086056624682088,-0.0320287467381911,
0.0798823690335567));
#90295=CARTESIAN_POINT('Ctrl Pts',(0.00872391810054128,-0.0318646057455573,
0.0798699617037712));
#90296=CARTESIAN_POINT('Ctrl Pts',(0.00873564501098324,-0.0321934096636619,
0.0801187204568708));
#90297=CARTESIAN_POINT('Ctrl Pts',(0.00885904353153239,-0.0320287467381911,
0.0801060706825933));
#90298=CARTESIAN_POINT('Ctrl Pts',(0.00898181378606981,-0.0318646057455573,
0.0800883315658226));
#90299=CARTESIAN_POINT('Ctrl Pts',(0.00874839290636016,-0.0321763980313108,
0.0801173998891418));
#90300=CARTESIAN_POINT('Ctrl Pts',(0.00874392497408026,-0.0321259597686371,
0.0800747143334848));
#90301=CARTESIAN_POINT('Ctrl Pts',(0.00873953437589611,-0.0320749162466965,
0.0800327679795527));
#90302=CARTESIAN_POINT('Ctrl Pts',(0.00873090466420057,-0.0319716059708271,
0.0799503214831995));
#90303=CARTESIAN_POINT('Ctrl Pts',(0.00872666881486074,-0.0319193783877868,
0.0799098524679891));
#90304=CARTESIAN_POINT('Ctrl Pts',(0.00872250888809975,-0.0318665617525138,
0.079870109379442));
#90305=CARTESIAN_POINT('',(0.00861132004499518,-0.0321934096636664,0.0800042993131371));
#90306=CARTESIAN_POINT('Ctrl Pts',(0.00855950338579825,-0.0327445246967097,
0.0798848853229917));
#90307=CARTESIAN_POINT('Ctrl Pts',(0.00877579812169474,-0.0324436878339361,
0.0798684518295582));
#90308=CARTESIAN_POINT('Ctrl Pts',(0.0089902405492005,-0.0321434074405928,
0.0798357728184288));
#90309=CARTESIAN_POINT('Ctrl Pts',(0.00856201626890479,-0.0327445246967097,
0.0798846382531779));
#90310=CARTESIAN_POINT('Ctrl Pts',(0.00877830168641091,-0.0324436878339361,
0.0798681099848087));
#90311=CARTESIAN_POINT('Ctrl Pts',(0.00899272768316337,-0.0321434074405928,
0.0798353371698884));
#90312=CARTESIAN_POINT('Ctrl Pts',(0.00881081657648191,-0.0327445246967097,
0.0798601758953698));
#90313=CARTESIAN_POINT('Ctrl Pts',(0.00902617938108062,-0.0324436878339361,
0.0798342639699983));
#90314=CARTESIAN_POINT('Ctrl Pts',(0.0092389785705746,-0.0321434074405928,
0.0797922036510292));
#90315=CARTESIAN_POINT('Ctrl Pts',(0.00881330457955768,-0.0327445246967097,
0.0798599312717918));
#90316=CARTESIAN_POINT('Ctrl Pts',(0.00902865815802732,-0.0324436878339361,
0.0798339255098502));
#90317=CARTESIAN_POINT('Ctrl Pts',(0.00924144107944872,-0.0321434074405928,
0.0797917723158406));
#90318=CARTESIAN_POINT('',(0.00884668829354451,-0.0326943950436612,0.0798557455051863));
#90319=CARTESIAN_POINT('',(0.00908049607793287,-0.0323666188837389,0.0798212276927121));
#90320=CARTESIAN_POINT('Origin',(0.00665828205650578,-0.0326395579111469,
0.0631878441266393));
#90321=CARTESIAN_POINT('Origin',(0.0109177201753066,-0.0321933825603152,
0.0907119567516225));
#90322=CARTESIAN_POINT('',(0.00895701164822238,-0.0321934096536378,0.0798406813014275));
#90323=CARTESIAN_POINT('',(0.00901864086939592,-0.0321934096584275,0.0798302846934935));
#90324=CARTESIAN_POINT('',(0.00872250888842273,-0.0325210109756239,0.0798701093821988));
#90325=CARTESIAN_POINT('Origin',(0.0071378099786331,-0.0326393129158301,
0.0631526674044951));
#90326=CARTESIAN_POINT('',(0.00872236746249035,-0.0326943950436594,0.0798687582284338));
#90327=CARTESIAN_POINT('Origin',(0.00987398789441971,-0.0326943765538268,
0.0908711073916663));
#90328=CARTESIAN_POINT('',(0.00878452787802743,-0.0326943950436703,0.07986225186682));
#90329=CARTESIAN_POINT('Ctrl Pts',(0.00851401032725098,-0.0325229783203769,
0.0801372967191685));
#90330=CARTESIAN_POINT('Ctrl Pts',(0.00859654508159117,-0.0324130253092451,
0.0801319174328731));
#90331=CARTESIAN_POINT('Ctrl Pts',(0.00867895604047152,-0.0323031222208071,
0.0801248316250349));
#90332=CARTESIAN_POINT('Ctrl Pts',(0.00876113796158937,-0.0321934096576659,
0.0801160520970259));
#90333=CARTESIAN_POINT('Ctrl Pts',(0.00858345380195833,-0.0325229783203769,
0.0800477492677418));
#90334=CARTESIAN_POINT('Ctrl Pts',(0.00866475414663888,-0.0324130253092451,
0.0800414127046661));
#90335=CARTESIAN_POINT('Ctrl Pts',(0.00874591108058209,-0.0323031222208071,
0.080033395300587));
#90336=CARTESIAN_POINT('Ctrl Pts',(0.00882682100991003,-0.0321934096576659,
0.0800237109935033));
#90337=CARTESIAN_POINT('Ctrl Pts',(0.00865289727666568,-0.0325229783203769,
0.079958201816315));
#90338=CARTESIAN_POINT('Ctrl Pts',(0.00873296321168659,-0.0324130253092451,
0.0799509079764592));
#90339=CARTESIAN_POINT('Ctrl Pts',(0.00881286612069266,-0.032303122220807,
0.0799419589761392));
#90340=CARTESIAN_POINT('Ctrl Pts',(0.00889250405823068,-0.0321934096576659,
0.0799313698899808));
#90341=CARTESIAN_POINT('Ctrl Pts',(0.00872234075137304,-0.0325229783203769,
0.0798686543648883));
#90342=CARTESIAN_POINT('Ctrl Pts',(0.0088011722767343,-0.0324130253092451,
0.0798604032482522));
#90343=CARTESIAN_POINT('Ctrl Pts',(0.00887982116080323,-0.032303122220807,
0.0798505226516913));
#90344=CARTESIAN_POINT('Ctrl Pts',(0.00895818710655133,-0.0321934096576659,
0.0798390287864582));
#90345=CARTESIAN_POINT('',(0.00885907480225073,-0.0321934096584275,0.0799783666995701));
#90346=CARTESIAN_POINT('Ctrl Pts',(0.00874839290846872,-0.0322104233328921,
0.0801173998856049));
#90347=CARTESIAN_POINT('Ctrl Pts',(0.00874391892089375,-0.0322609421831179,
0.0800746563458506));
#90348=CARTESIAN_POINT('Ctrl Pts',(0.0087395254426463,-0.0323120888240345,
0.0800326819753405));
#90349=CARTESIAN_POINT('Ctrl Pts',(0.0087308956280255,-0.0324156524631809,
0.0799502345348557));
#90350=CARTESIAN_POINT('Ctrl Pts',(0.00872666283896298,-0.0324680267167311,
0.0799097953551453));
#90351=CARTESIAN_POINT('Ctrl Pts',(0.00872250888842266,-0.0325210109755913,
0.0798701093821553));
#90352=CARTESIAN_POINT('Origin',(0.000256974599154325,-0.0262834582511321,
0.0740206782313454));
#90353=CARTESIAN_POINT('Origin',(0.00384607110080342,-0.0342771004391969,
0.0855309532453021));
#90354=CARTESIAN_POINT('Ctrl Pts',(0.0088451129986142,-0.0326943950436605,
0.0798544687371118));
#90355=CARTESIAN_POINT('Ctrl Pts',(0.0089237312691255,-0.0325844576448134,
0.0798445274466939));
#90356=CARTESIAN_POINT('Ctrl Pts',(0.00900214950138914,-0.0324744968375323,
0.0798329594979849));
#90357=CARTESIAN_POINT('Ctrl Pts',(0.00908026742582625,-0.0323646534831894,
0.0798197810983539));
#90358=CARTESIAN_POINT('Ctrl Pts',(0.00893314756504952,-0.0326943950436605,
0.0799258202801583));
#90359=CARTESIAN_POINT('Ctrl Pts',(0.00901274919355104,-0.0325844576448134,
0.0799146657084206));
#90360=CARTESIAN_POINT('Ctrl Pts',(0.00909212576075179,-0.0324744968375323,
0.0799018640550705));
#90361=CARTESIAN_POINT('Ctrl Pts',(0.00917117579100079,-0.0323646534831894,
0.0798874331251075));
#90362=CARTESIAN_POINT('Ctrl Pts',(0.00902118213148483,-0.0326943950436605,
0.0799971718232049));
#90363=CARTESIAN_POINT('Ctrl Pts',(0.00910176711797658,-0.0325844576448134,
0.0799848039701473));
#90364=CARTESIAN_POINT('Ctrl Pts',(0.00918210202011443,-0.0324744968375323,
0.0799707686121561));
#90365=CARTESIAN_POINT('Ctrl Pts',(0.00926208415617532,-0.0323646534831894,
0.0799550851518611));
#90366=CARTESIAN_POINT('Ctrl Pts',(0.00910921669792015,-0.0326943950436605,
0.0800685233662514));
#90367=CARTESIAN_POINT('Ctrl Pts',(0.00919078504240212,-0.0325844576448134,
0.080054942231874));
#90368=CARTESIAN_POINT('Ctrl Pts',(0.00927207827947707,-0.0324744968375323,
0.0800396731692416));
#90369=CARTESIAN_POINT('Ctrl Pts',(0.00935299252134986,-0.0323646534831894,
0.0800227371786146));
#90370=CARTESIAN_POINT('Ctrl Pts',(0.00912185652095127,-0.0326773559987509,
0.0800664049536984));
#90371=CARTESIAN_POINT('Ctrl Pts',(0.0091147114014,-0.032626792258736,0.0800240499711801));
#90372=CARTESIAN_POINT('Ctrl Pts',(0.00910769292393254,-0.0325756109582124,
0.0799824457001378));
#90373=CARTESIAN_POINT('Ctrl Pts',(0.00909390328002329,-0.0324719985462383,
0.0799007031732955));
#90374=CARTESIAN_POINT('Ctrl Pts',(0.00908713764428535,-0.032419609162178,
0.0798605977025121));
#90375=CARTESIAN_POINT('Ctrl Pts',(0.00908049607792469,-0.0323666188837756,
0.079821227692664));
#90376=CARTESIAN_POINT('',(0.00897795249573675,-0.0326943950436703,0.0799621344357239));
#90377=CARTESIAN_POINT('Ctrl Pts',(0.00891880354331507,-0.0332451089994434,
0.0798462002512828));
#90378=CARTESIAN_POINT('Ctrl Pts',(0.00913363925068852,-0.0329451141710254,
0.0798162155304841));
#90379=CARTESIAN_POINT('Ctrl Pts',(0.0093456060607421,-0.0326442513127494,
0.079770133689378));
#90380=CARTESIAN_POINT('Ctrl Pts',(0.00892127127411304,-0.0332451089994434,
0.0798457998705782));
#90381=CARTESIAN_POINT('Ctrl Pts',(0.00913609188088116,-0.0329451141710254,
0.0798157220777897));
#90382=CARTESIAN_POINT('Ctrl Pts',(0.00934803662266587,-0.0326442513127494,
0.0797695485665407));
#90383=CARTESIAN_POINT('Ctrl Pts',(0.00916804435391047,-0.0332451089994434,
0.0798057618001041));
#90384=CARTESIAN_POINT('Ctrl Pts',(0.00938135490014477,-0.0329451141710254,
0.0797663768083373));
#90385=CARTESIAN_POINT('Ctrl Pts',(0.0095910928150431,-0.0326442513127494,
0.0797110362828126));
#90386=CARTESIAN_POINT('Ctrl Pts',(0.00917053676201642,-0.0332451089994434,
0.0798053574155923));
#90387=CARTESIAN_POINT('Ctrl Pts',(0.00938383205663933,-0.0329451141710254,
0.0797658784211159));
#90388=CARTESIAN_POINT('Ctrl Pts',(0.00959354768258612,-0.0326442513127494,
0.079710445308747));
#90389=CARTESIAN_POINT('',(0.00920352852806092,-0.0331951640388616,0.0797990948701679));
#90390=CARTESIAN_POINT('',(0.00943470756977919,-0.0328677532355042,0.079749964261194));
#90391=CARTESIAN_POINT('Origin',(0.00530526937757678,-0.0326402808281488,
0.0634946223833793));
#90392=CARTESIAN_POINT('Origin',(0.0119550957035538,-0.0326944278779005,
0.0905148157064891));
#90393=CARTESIAN_POINT('',(0.00931268830210941,-0.0326943950436593,0.0797771331301099));
#90394=CARTESIAN_POINT('',(0.00937354310086201,-0.0326943950436694,0.0797628873072233));
#90395=CARTESIAN_POINT('',(0.00908049607793007,-0.0330220786163546,0.0798212276927126));
#90396=CARTESIAN_POINT('Origin',(0.00576523519911172,-0.0326396682762719,
0.0633546792233742));
#90397=CARTESIAN_POINT('',(0.00908027009142097,-0.0331951640388588,0.079819888085349));
#90398=CARTESIAN_POINT('Origin',(0.0109153372257397,-0.0331952026560021,
0.0906978427710935));
#90399=CARTESIAN_POINT('',(0.00914189930975095,-0.0331951640388702,0.0798094914777685));
#90400=CARTESIAN_POINT('Ctrl Pts',(0.0088891867257789,-0.0330240426238172,
0.0801009794069052));
#90401=CARTESIAN_POINT('Ctrl Pts',(0.00897116726486732,-0.032914277406352,
0.0800904352137702));
#90402=CARTESIAN_POINT('Ctrl Pts',(0.00905297069631849,-0.0328043479726691,
0.080078190997226));
#90403=CARTESIAN_POINT('Ctrl Pts',(0.0091344917918614,-0.0326943950436593,
0.0800642595569548));
#90404=CARTESIAN_POINT('Ctrl Pts',(0.00895287040814085,-0.0330240426238172,
0.0800072482776819));
#90405=CARTESIAN_POINT('Ctrl Pts',(0.0090335597096064,-0.032914277406352,
0.0799958267797783));
#90406=CARTESIAN_POINT('Ctrl Pts',(0.00911405312336546,-0.0328043479726691,
0.0799827315145858));
#90407=CARTESIAN_POINT('Ctrl Pts',(0.00919424706935178,-0.0326943950436593,
0.0799679764182612));
#90408=CARTESIAN_POINT('Ctrl Pts',(0.0090165540905028,-0.0330240426238172,
0.0799135171484586));
#90409=CARTESIAN_POINT('Ctrl Pts',(0.00909595215434549,-0.032914277406352,
0.0799012183457865));
#90410=CARTESIAN_POINT('Ctrl Pts',(0.00917513555041244,-0.0328043479726691,
0.0798872720319455));
#90411=CARTESIAN_POINT('Ctrl Pts',(0.00925400234684215,-0.0326943950436593,
0.0798716932795675));
#90412=CARTESIAN_POINT('Ctrl Pts',(0.00908023777286475,-0.0330240426238172,
0.0798197860192353));
#90413=CARTESIAN_POINT('Ctrl Pts',(0.00915834459908457,-0.032914277406352,
0.0798066099117946));
#90414=CARTESIAN_POINT('Ctrl Pts',(0.00923621797745941,-0.0328043479726691,
0.0797918125493052));
#90415=CARTESIAN_POINT('Ctrl Pts',(0.00931375762433253,-0.0326943950436593,
0.0797754101408738));
#90416=CARTESIAN_POINT('',(0.00922359004699556,-0.0326943950436694,0.0799206963435421));
#90417=CARTESIAN_POINT('Ctrl Pts',(0.00912185652094892,-0.0327114338383315,
0.080066404953685));
#90418=CARTESIAN_POINT('Ctrl Pts',(0.00911471258984867,-0.032761987683083,
0.0800240570160902));
#90419=CARTESIAN_POINT('Ctrl Pts',(0.00910769469286847,-0.0328131562604049,
0.0799824561860719));
#90420=CARTESIAN_POINT('Ctrl Pts',(0.00909390506165631,-0.0329167375858767,
0.0799007137344954));
#90421=CARTESIAN_POINT('Ctrl Pts',(0.00908713882192933,-0.0329691088920617,
0.0798606046833739));
#90422=CARTESIAN_POINT('Ctrl Pts',(0.00908049607792491,-0.0330220786163187,
0.0798212276926652));
#90423=CARTESIAN_POINT('Ctrl Pts',(0.00920187590888759,-0.0331951640388604,
0.0797979193474506));
#90424=CARTESIAN_POINT('Ctrl Pts',(0.00931864302028713,-0.033030642201062,
0.0797756304510862));
#90425=CARTESIAN_POINT('Ctrl Pts',(0.00943438913148185,-0.0328657861914645,
0.0797485344929184));
#90426=CARTESIAN_POINT('Ctrl Pts',(0.00920352852805782,-0.0331951640388604,
0.0797990948701685));
#90427=CARTESIAN_POINT('Ctrl Pts',(0.00932031994263588,-0.033030642201062,
0.0797767718069623));
#90428=CARTESIAN_POINT('Ctrl Pts',(0.00943608892409072,-0.0328657861914645,
0.0797496407066721));
#90429=CARTESIAN_POINT('Ctrl Pts',(0.00947889932504337,-0.0331951640388604,
0.0799949685678302));
#90430=CARTESIAN_POINT('Ctrl Pts',(0.00959974030273804,-0.033030642201062,
0.0799669523899477));
#90431=CARTESIAN_POINT('Ctrl Pts',(0.0097193200845696,-0.0328657861914645,
0.0799339656670055));
#90432=CARTESIAN_POINT('Ctrl Pts',(0.00949138118876774,-0.0331781648286476,
0.0799920606784095));
#90433=CARTESIAN_POINT('Ctrl Pts',(0.00948158392494805,-0.0331276811546812,
0.0799502091289448));
#90434=CARTESIAN_POINT('Ctrl Pts',(0.0094719635364457,-0.0330765663497823,
0.0799091132965642));
#90435=CARTESIAN_POINT('Ctrl Pts',(0.00945306840235603,-0.0329730614463283,
0.0798283977204811));
#90436=CARTESIAN_POINT('Ctrl Pts',(0.00944380129521076,-0.0329207133374032,
0.0797888105828929));
#90437=CARTESIAN_POINT('Ctrl Pts',(0.00943470755815306,-0.0328677532289396,
0.0797499642728653));
#90438=CARTESIAN_POINT('',(0.00934121392655591,-0.0331951640388702,0.0798970317190041));
#90439=CARTESIAN_POINT('Origin',(0.00812378219310841,-0.0315241814719618,
0.07415));
#90440=CARTESIAN_POINT('',(0.0105618502623033,-0.0347116136489609,0.0796323192235916));
#90441=CARTESIAN_POINT('',(0.0105735550331357,-0.0346945769586885,0.0796270989613359));
#90442=CARTESIAN_POINT('Origin',(0.00363602083277754,-0.0345626704646042,
0.0645459177258107));
#90443=CARTESIAN_POINT('Origin',(0.00395570707162937,-0.034562661854009,
0.0644016995088073));
#90444=CARTESIAN_POINT('Origin',(0.00399783382564541,-0.0345626705763338,
0.0643850145551682));
#90445=CARTESIAN_POINT('Ctrl Pts',(0.0103103965557986,-0.0352450361874068,
0.0794695375978088));
#90446=CARTESIAN_POINT('Ctrl Pts',(0.0105110262084795,-0.0349452760959493,
0.0793870680838582));
#90447=CARTESIAN_POINT('Ctrl Pts',(0.0107048739522082,-0.034644428984174,
0.079289720610766));
#90448=CARTESIAN_POINT('Ctrl Pts',(0.0103127100929213,-0.0352450361874068,
0.0794685260786632));
#90449=CARTESIAN_POINT('Ctrl Pts',(0.0105133015955316,-0.0349452760959493,
0.0793859693082281));
#90450=CARTESIAN_POINT('Ctrl Pts',(0.0107071047250546,-0.034644428984174,
0.0792885377001574));
#90451=CARTESIAN_POINT('Ctrl Pts',(0.0105417731743749,-0.0352450361874068,
0.079368375668205));
#90452=CARTESIAN_POINT('Ctrl Pts',(0.0107385874422733,-0.0349452760959493,
0.0792771796418894));
#90453=CARTESIAN_POINT('Ctrl Pts',(0.0109279733237086,-0.034644428984174,
0.0791714178379282));
#90454=CARTESIAN_POINT('Ctrl Pts',(0.0105440638051894,-0.0352450361874068,
0.0793673741641004));
#90455=CARTESIAN_POINT('Ctrl Pts',(0.0107408403007407,-0.0349452760959493,
0.079276091745226));
#90456=CARTESIAN_POINT('Ctrl Pts',(0.0109301820096952,-0.034644428984174,
0.0791702466393059));
#90457=CARTESIAN_POINT('',(0.0105744508146227,-0.0351951634053328,0.0793531121081548));
#90458=CARTESIAN_POINT('',(0.0107861769035186,-0.0348678972925388,0.0792480172033822));
#90459=CARTESIAN_POINT('Origin',(0.00265878042524815,-0.0345636767885836,
0.0645968707624761));
#90460=CARTESIAN_POINT('Origin',(0.0159013235930254,-0.0346946199341236,
0.0890426209992575));
#90461=CARTESIAN_POINT('',(0.0106747477174434,-0.0346945769330289,0.0793046774770006));
#90462=CARTESIAN_POINT('',(0.0107301478665679,-0.0346945769458128,0.0792757452360809));
#90463=CARTESIAN_POINT('',(0.0104608161269358,-0.0350221583435276,0.0794051305780295));
#90464=CARTESIAN_POINT('Origin',(0.00306414635805795,-0.0345628458716434,
0.0643383715295872));
#90465=CARTESIAN_POINT('',(0.0104603107618279,-0.0351951360298763,0.079404001640984));
#90466=CARTESIAN_POINT('Origin',(0.0149378146759128,-0.0351951838366768,
0.089472258816035));
#90467=CARTESIAN_POINT('',(0.0105744790773254,-0.0351951371328746,0.0793530961727634));
#90468=CARTESIAN_POINT('Ctrl Pts',(0.0103450886693692,-0.0350241211494342,
0.0797236700241919));
#90469=CARTESIAN_POINT('Ctrl Pts',(0.0104218636886588,-0.0349144232818962,
0.0796930724382525));
#90470=CARTESIAN_POINT('Ctrl Pts',(0.0104980521875328,-0.0348045283579412,
0.0796608695436739));
#90471=CARTESIAN_POINT('Ctrl Pts',(0.0105735550432784,-0.0346945769439157,
0.079627098956804));
#90472=CARTESIAN_POINT('Ctrl Pts',(0.0103834616338616,-0.0350241211494342,
0.0796170461178704));
#90473=CARTESIAN_POINT('Ctrl Pts',(0.0104587679525591,-0.0349144232818962,
0.0795859199600787));
#90474=CARTESIAN_POINT('Ctrl Pts',(0.0105334759457951,-0.0348045283579412,
0.0795532185363627));
#90475=CARTESIAN_POINT('Ctrl Pts',(0.0106074883634341,-0.0346945769439157,
0.0795189801721901));
#90476=CARTESIAN_POINT('Ctrl Pts',(0.010421834598354,-0.0350241211494342,
0.0795104222115489));
#90477=CARTESIAN_POINT('Ctrl Pts',(0.0104956722164594,-0.0349144232818962,
0.0794787674819048));
#90478=CARTESIAN_POINT('Ctrl Pts',(0.0105688997040573,-0.0348045283579412,
0.0794455675290515));
#90479=CARTESIAN_POINT('Ctrl Pts',(0.0106414216835899,-0.0346945769439157,
0.0794108613875762));
#90480=CARTESIAN_POINT('Ctrl Pts',(0.0104602075628463,-0.0350241211494342,
0.0794037983052275));
#90481=CARTESIAN_POINT('Ctrl Pts',(0.0105325764803597,-0.0349144232818962,
0.079371615003731));
#90482=CARTESIAN_POINT('Ctrl Pts',(0.0106043234623195,-0.0348045283579412,
0.0793379165217403));
#90483=CARTESIAN_POINT('Ctrl Pts',(0.0106753550037457,-0.0346945769439157,
0.0793027426029622));
#90484=CARTESIAN_POINT('',(0.0106241513750694,-0.0346945769458128,0.0794658882193774));
#90485=CARTESIAN_POINT('Ctrl Pts',(0.010561850260961,-0.034711613649279,
0.0796323192205801));
#90486=CARTESIAN_POINT('Ctrl Pts',(0.0105444013634492,-0.0347621546531703,
0.0795930830616442));
#90487=CARTESIAN_POINT('Ctrl Pts',(0.010527259264707,-0.0348133084095802,
0.0795545367804084));
#90488=CARTESIAN_POINT('Ctrl Pts',(0.0104935743584344,-0.0349168561544574,
0.0794787918036634));
#90489=CARTESIAN_POINT('Ctrl Pts',(0.0104770449120557,-0.0349692089015921,
0.0794416231524752));
#90490=CARTESIAN_POINT('Ctrl Pts',(0.0104608161269391,-0.0350221583435,
0.0794051305779879));
#90491=CARTESIAN_POINT('Ctrl Pts',(0.0105731134580019,-0.0351951371254953,
0.079352571288223));
#90492=CARTESIAN_POINT('Ctrl Pts',(0.0106806733551835,-0.035030733898096,
0.0793019329010831));
#90493=CARTESIAN_POINT('Ctrl Pts',(0.0107860484038839,-0.0348659306897825,
0.0792468922175369));
#90494=CARTESIAN_POINT('Ctrl Pts',(0.0105744790772703,-0.0351951371254953,
0.0793530961726611));
#90495=CARTESIAN_POINT('Ctrl Pts',(0.0106820498261083,-0.035030733898096,
0.0793024295521997));
#90496=CARTESIAN_POINT('Ctrl Pts',(0.0107874345502788,-0.0348659306897825,
0.0792473602109466));
#90497=CARTESIAN_POINT('Ctrl Pts',(0.0108033582899396,-0.0351951371254953,
0.0794410673515482));
#90498=CARTESIAN_POINT('Ctrl Pts',(0.0109127477877062,-0.035030733898096,
0.0793856687969685));
#90499=CARTESIAN_POINT('Ctrl Pts',(0.0110197541307519,-0.0348659306897825,
0.0793257963941513));
#90500=CARTESIAN_POINT('Origin',(0.0132480472269558,-0.0308609197411241,
0.0839620655045698));
#90501=CARTESIAN_POINT('',(0.0106742652534521,-0.0351951371254953,0.0793914496231688));
#90502=CARTESIAN_POINT('Origin',(0.00755074467756133,-0.035184046744115,
0.0733585622856818));
#90503=CARTESIAN_POINT('Origin',(0.0143548902956506,-0.0352322613037122,
0.0843647549503665));
#90504=CARTESIAN_POINT('',(0.0109936380460948,-0.0351951142564684,0.0791341490714577));
#90505=CARTESIAN_POINT('',(0.0111003272121345,-0.0351951372916787,0.0790696219112562));
#90506=CARTESIAN_POINT('Origin',(0.00827955227021354,-0.0352875117694839,
0.0738471516112963));
#90507=CARTESIAN_POINT('Origin',(0.00107941703142758,-0.0298325076523859,
0.0767330427301951));
#90508=CARTESIAN_POINT('Origin',(0.0094440988976966,-0.0338732150591158,
0.082426931938526));
#90509=CARTESIAN_POINT('Origin',(0.00812378219310841,-0.0315241814719618,
0.07415));
#90510=CARTESIAN_POINT('',(0.00874839290879345,-0.0332121607144206,0.0801173998886622));
#90511=CARTESIAN_POINT('',(0.00876113795713088,-0.0331951640388587,0.0801160520975017));
#90512=CARTESIAN_POINT('Origin',(0.00627798841830207,-0.0326413635833112,
0.0637867391944952));
#90513=CARTESIAN_POINT('',(0.00874839290831179,-0.0331781648281947,0.0801173998902725));
#90514=CARTESIAN_POINT('Origin',(0.00773838482252226,-0.0326412105611727,
0.0636259931678058));
#90515=CARTESIAN_POINT('',(0.00873564501100219,-0.0331951640388588,0.080118720456855));
#90516=CARTESIAN_POINT('Origin',(0.00632159444987085,-0.0326412092830655,
0.0637742933550843));
#90517=CARTESIAN_POINT('Origin',(0.0077836230719809,-0.0326413653378089,
0.0636291472617185));
#90518=CARTESIAN_POINT('Origin',(0.00812378219310841,-0.0315241814719618,
0.07415));
#90519=CARTESIAN_POINT('',(0.00912185652157204,-0.0337108120655696,0.0800664049573521));
#90520=CARTESIAN_POINT('',(0.00913449179186386,-0.0336938721132327,0.0800642595569508));
#90521=CARTESIAN_POINT('Origin',(0.00750227557297375,-0.0345562530068284,
0.0637472403724542));
#90522=CARTESIAN_POINT('',(0.00912185652178286,-0.033676936124379,0.080066404958628));
#90523=CARTESIAN_POINT('Ctrl Pts',(0.00913449179186099,-0.0336938721132359,
0.0800642595569588));
#90524=CARTESIAN_POINT('Ctrl Pts',(0.0091323864415022,-0.0336910493107781,
0.080064619348036));
#90525=CARTESIAN_POINT('Ctrl Pts',(0.0091302808391578,-0.0336882265931775,
0.0800649780251539));
#90526=CARTESIAN_POINT('Ctrl Pts',(0.00912606908823685,-0.0336825812712327,
0.080065693158239));
#90527=CARTESIAN_POINT('Ctrl Pts',(0.00912396293972832,-0.0336797586669777,
0.080066049614173));
#90528=CARTESIAN_POINT('Ctrl Pts',(0.00912185652178378,-0.0336769361243774,
0.0800664049586247));
#90529=CARTESIAN_POINT('',(0.009109216697909,-0.0336938721132328,0.0800685233662416));
#90530=CARTESIAN_POINT('Ctrl Pts',(0.00912185652178066,-0.0336769361243777,
0.0800664049586253));
#90531=CARTESIAN_POINT('Ctrl Pts',(0.00911975010381738,-0.0336797586670032,
0.0800667603030801));
#90532=CARTESIAN_POINT('Ctrl Pts',(0.00911764357575037,-0.0336825812712832,
0.0800671145091738));
#90533=CARTESIAN_POINT('Ctrl Pts',(0.00911343031216495,-0.0336882265860984,
0.0800678206430221));
#90534=CARTESIAN_POINT('Ctrl Pts',(0.00911132357667191,-0.0336910492966202,
0.0800681725708117));
#90535=CARTESIAN_POINT('Ctrl Pts',(0.00910921669791881,-0.0336938721132386,
0.0800685233662538));
#90536=CARTESIAN_POINT('Origin',(0.00529820345362548,-0.0345562530596106,
0.0641190585384484));
#90537=CARTESIAN_POINT('Origin',(0.00812378219310841,-0.0315241814719618,
0.07415));
#90538=CARTESIAN_POINT('',(0.00837246424298519,-0.0327114338379848,0.0801448442196473));
#90539=CARTESIAN_POINT('',(0.00838526877037963,-0.0326943950436593,0.0801442993560501));
#90540=CARTESIAN_POINT('Origin',(0.00758879780582063,-0.0326395653650527,
0.0635587003231629));
#90541=CARTESIAN_POINT('',(0.008372464242277,-0.0326773559992502,0.0801448442207892));
#90542=CARTESIAN_POINT('Origin',(0.00773442609091764,-0.0326395686091014,
0.063551883863096));
#90543=CARTESIAN_POINT('',(0.00835965858108669,-0.0326943950436595,0.0801453617346741));
#90544=CARTESIAN_POINT('Origin',(0.00763403304173427,-0.0326395669694838,
0.0635560519265562));
#90545=CARTESIAN_POINT('Origin',(0.00777972546240625,-0.0326395670659013,
0.063550783508722));
#90546=CARTESIAN_POINT('Origin',(0.00812378219310841,-0.0315241814719618,
0.07415));
#90547=CARTESIAN_POINT('',(0.00799555414271255,-0.032210423332359,0.0801486296392922));
#90548=CARTESIAN_POINT('',(0.00800836761556929,-0.0321934096636183,0.0801488898535757));
#90549=CARTESIAN_POINT('Origin',(0.00891757153313832,-0.0326387221312259,
0.0636219243157334));
#90550=CARTESIAN_POINT('',(0.00799555414184183,-0.0321763980308046,0.0801486296399426));
#90551=CARTESIAN_POINT('Origin',(0.00773559231001018,-0.0326386251174431,
0.0636029764171086));
#90552=CARTESIAN_POINT('',(0.0079827412548295,-0.0321934096636185,0.0801483420587467));
#90553=CARTESIAN_POINT('Origin',(0.00896231991809475,-0.0326386231523553,
0.0636292029887929));
#90554=CARTESIAN_POINT('Origin',(0.00778061111138152,-0.0326387237755826,
0.0635976246480955));
#90555=CARTESIAN_POINT('Origin',(0.00812378219310841,-0.0315241814719618,
0.07415));
#90556=CARTESIAN_POINT('',(0.0098555085716382,-0.0347116136489614,0.0798946604537853));
#90557=CARTESIAN_POINT('',(0.00986777531920451,-0.0346945769586885,0.0798909483516342));
#90558=CARTESIAN_POINT('Origin',(0.00487511900430214,-0.0345626705531907,
0.0640591832160391));
#90559=CARTESIAN_POINT('',(0.00985550857127204,-0.0346775396665025,0.0798946604551301));
#90560=CARTESIAN_POINT('Origin',(0.00521035946764333,-0.0345626618993397,
0.063956169170596));
#90561=CARTESIAN_POINT('',(0.00984323392392057,-0.0346945769586886,0.0798983463487691));
#90562=CARTESIAN_POINT('Origin',(0.00491792381413625,-0.0345626617996805,
0.0640443240441348));
#90563=CARTESIAN_POINT('Origin',(0.00525424527900612,-0.0345626706176323,
0.0639448958454014));
#90564=CARTESIAN_POINT('Origin',(0.00812378219310841,-0.0315241814719618,
0.07415));
#90565=CARTESIAN_POINT('',(0.00949138119084094,-0.0342105180190372,0.0799920606778171));
#90566=CARTESIAN_POINT('',(0.00950385681755749,-0.0341934961088739,0.0799891261359002));
#90567=CARTESIAN_POINT('Origin',(0.00617091115087495,-0.0345621724038967,
0.0637586100252421));
#90568=CARTESIAN_POINT('',(0.00949138119077186,-0.0341764758832668,0.0799920606775218));
#90569=CARTESIAN_POINT('Origin',(0.00521870190545053,-0.0345621027020113,
0.0639868884251929));
#90570=CARTESIAN_POINT('',(0.00947889932502756,-0.034193496108874,0.0799949685678179));
#90571=CARTESIAN_POINT('Origin',(0.00621593979425685,-0.0345621027111292,
0.0637534398504798));
#90572=CARTESIAN_POINT('Origin',(0.00526134665942937,-0.0345621724286372,
0.0639715350338382));
#90573=CARTESIAN_POINT('Ctrl Pts',(0.00892119950492447,-0.034243627687391,
0.079845809918775));
#90574=CARTESIAN_POINT('Ctrl Pts',(0.0091360205173804,-0.0339430054201809,
0.0798157348290657));
#90575=CARTESIAN_POINT('Ctrl Pts',(0.00934796586687492,-0.0336441434784052,
0.0797695639806734));
#90576=CARTESIAN_POINT('Ctrl Pts',(0.00916797308919641,-0.034243627687391,
0.0798057749577337));
#90577=CARTESIAN_POINT('Ctrl Pts',(0.00938128415820492,-0.0339430054201809,
0.0797663926488621));
#90578=CARTESIAN_POINT('Ctrl Pts',(0.00959102279596063,-0.0336441434784052,
0.0797110547572688));
#90579=CARTESIAN_POINT('',(0.00920352852805892,-0.0341934961088741,0.0797990948701683));
#90580=CARTESIAN_POINT('',(0.00943470755858997,-0.0338664212895226,0.0797499642584328));
#90581=CARTESIAN_POINT('Origin',(0.00656379352345093,-0.0345610818076477,
0.0632738144364997));
#90582=CARTESIAN_POINT('Origin',(0.0119343541146342,-0.0336938005044268,
0.090427534726314));
#90583=CARTESIAN_POINT('',(0.00931268830210938,-0.0336938721132327,0.07977713313011));
#90584=CARTESIAN_POINT('',(0.00937354310086199,-0.0336938721132427,0.0797628873072233));
#90585=CARTESIAN_POINT('',(0.00908049607792758,-0.0340203938281605,0.079821227692713));
#90586=CARTESIAN_POINT('Origin',(0.00704495936124007,-0.0345589643245042,
0.0632720726151595));
#90587=CARTESIAN_POINT('Origin',(0.01091330714871,-0.0341934220717635,0.0906858069796352));
#90588=CARTESIAN_POINT('',(0.0091418993097499,-0.0341934961088841,0.0798094914777686));
#90589=CARTESIAN_POINT('Ctrl Pts',(0.00888918496513205,-0.0340223579322396,
0.0801009796333548));
#90590=CARTESIAN_POINT('Ctrl Pts',(0.00897126449508248,-0.0339125849573575,
0.0800904227328744));
#90591=CARTESIAN_POINT('Ctrl Pts',(0.00905306784538844,-0.0338030433565231,
0.0800781743950622));
#90592=CARTESIAN_POINT('Ctrl Pts',(0.00913449179186244,-0.0336938721132327,
0.0800642595569531));
#90593=CARTESIAN_POINT('Ctrl Pts',(0.00895286878394797,-0.0340223579322396,
0.0800072483629521));
#90594=CARTESIAN_POINT('Ctrl Pts',(0.00903365551521813,-0.0339125849573575,
0.0799958130965159));
#90595=CARTESIAN_POINT('Ctrl Pts',(0.00911414879514424,-0.0338030433565231,
0.0799827137678941));
#90596=CARTESIAN_POINT('Ctrl Pts',(0.0091942471713689,-0.0336938721132327,
0.0799679762538819));
#90597=CARTESIAN_POINT('Ctrl Pts',(0.00901655260276389,-0.0340223579322396,
0.0799135170925495));
#90598=CARTESIAN_POINT('Ctrl Pts',(0.00909604653535378,-0.0339125849573575,
0.0799012034601574));
#90599=CARTESIAN_POINT('Ctrl Pts',(0.00917522974490004,-0.0338030433565231,
0.079887253140726));
#90600=CARTESIAN_POINT('Ctrl Pts',(0.00925400255087535,-0.0336938721132326,
0.0798716929508106));
#90601=CARTESIAN_POINT('Ctrl Pts',(0.00908023642157981,-0.0340223579322396,
0.0798197858221469));
#90602=CARTESIAN_POINT('Ctrl Pts',(0.00915843755548943,-0.0339125849573575,
0.0798065938237989));
#90603=CARTESIAN_POINT('Ctrl Pts',(0.00923631069465584,-0.0338030433565231,
0.0797917925135579));
#90604=CARTESIAN_POINT('Ctrl Pts',(0.00931375793038181,-0.0336938721132326,
0.0797754096477394));
#90605=CARTESIAN_POINT('',(0.00922359004699662,-0.0336938721132427,0.0799206963435404));
#90606=CARTESIAN_POINT('Ctrl Pts',(0.00912185652096689,-0.0337108120662708,
0.0800664049537917));
#90607=CARTESIAN_POINT('Ctrl Pts',(0.00911470377868284,-0.0337611408994039,
0.0800240047850855));
#90608=CARTESIAN_POINT('Ctrl Pts',(0.00910768155807646,-0.033812108878075,
0.0799823783253896));
#90609=CARTESIAN_POINT('Ctrl Pts',(0.00909389176307279,-0.0339153382773247,
0.0799006349028868));
#90610=CARTESIAN_POINT('Ctrl Pts',(0.00908713002261463,-0.0339675558473124,
0.0798605525226209));
#90611=CARTESIAN_POINT('Ctrl Pts',(0.00908049607792608,-0.0340203938281304,
0.0798212276926728));
#90612=CARTESIAN_POINT('Ctrl Pts',(0.0092018758347171,-0.0341934961088741,
0.0797979192946915));
#90613=CARTESIAN_POINT('Ctrl Pts',(0.00927975729708932,-0.0340836138583034,
0.0797830530218215));
#90614=CARTESIAN_POINT('Ctrl Pts',(0.00935729376414901,-0.0339738896647348,
0.0797665822886252));
#90615=CARTESIAN_POINT('Ctrl Pts',(0.00943438741192324,-0.0338644633299819,
0.0797485348279564));
#90616=CARTESIAN_POINT('Ctrl Pts',(0.00929421699815897,-0.0341934961088741,
0.0798636023857373));
#90617=CARTESIAN_POINT('Ctrl Pts',(0.00937300419145915,-0.0340836138583034,
0.0798474627829079));
#90618=CARTESIAN_POINT('Ctrl Pts',(0.00945141960596841,-0.0339738896647348,
0.0798297005885188));
#90619=CARTESIAN_POINT('Ctrl Pts',(0.00952936440357235,-0.0338644633299819,
0.0798103452637452));
#90620=CARTESIAN_POINT('Ctrl Pts',(0.00938655816160085,-0.0341934961088741,
0.079929285476783));
#90621=CARTESIAN_POINT('Ctrl Pts',(0.00946625108582898,-0.0340836138583034,
0.0799118725439943));
#90622=CARTESIAN_POINT('Ctrl Pts',(0.00954554544778781,-0.0339738896647348,
0.0798928188884124));
#90623=CARTESIAN_POINT('Ctrl Pts',(0.00962434139522147,-0.0338644633299819,
0.0798721556995341));
#90624=CARTESIAN_POINT('Ctrl Pts',(0.00947889932504273,-0.0341934961088741,
0.0799949685678288));
#90625=CARTESIAN_POINT('Ctrl Pts',(0.00955949798019881,-0.0340836138583034,
0.0799762823050806));
#90626=CARTESIAN_POINT('Ctrl Pts',(0.00963967128960721,-0.0339738896647348,
0.079955937188306));
#90627=CARTESIAN_POINT('Ctrl Pts',(0.00971931838687058,-0.0338644633299819,
0.0799339661353229));
#90628=CARTESIAN_POINT('Ctrl Pts',(0.00949138119003726,-0.0341764758830281,
0.0799920606744016));
#90629=CARTESIAN_POINT('Ctrl Pts',(0.00948159726840954,-0.0341260048548333,
0.0799502660665442));
#90630=CARTESIAN_POINT('Ctrl Pts',(0.00947198350155604,-0.0340749271293304,
0.0799091983197897));
#90631=CARTESIAN_POINT('Ctrl Pts',(0.009453088468083,-0.033971543442926,
0.0798284831889346));
#90632=CARTESIAN_POINT('Ctrl Pts',(0.00944381459525593,-0.0339192781035265,
0.0797888673893735));
#90633=CARTESIAN_POINT('Ctrl Pts',(0.0094347075555425,-0.0338664212877434,
0.0797499642615637));
#90634=CARTESIAN_POINT('',(0.00934121392655325,-0.0341934961088841,0.0798970317190032));
#90635=CARTESIAN_POINT('Ctrl Pts',(0.00931122777606145,-0.0346945769586966,
0.0797774750324058));
#90636=CARTESIAN_POINT('Ctrl Pts',(0.00948807830358499,-0.0344439193968194,
0.0797401580516033));
#90637=CARTESIAN_POINT('Ctrl Pts',(0.00966223670437822,-0.0341934961088739,
0.0796918101708358));
#90638=CARTESIAN_POINT('Ctrl Pts',(0.00931268830210382,-0.0346945769586966,
0.0797771331301111));
#90639=CARTESIAN_POINT('Ctrl Pts',(0.00948952808491488,-0.0344439193968194,
0.0797397702504286));
#90640=CARTESIAN_POINT('Ctrl Pts',(0.00966367288018335,-0.0341934961088739,
0.0796913772360181));
#90641=CARTESIAN_POINT('Ctrl Pts',(0.00955610749707416,-0.0346945769586966,
0.079720149838525));
#90642=CARTESIAN_POINT('Ctrl Pts',(0.00973115650780379,-0.0344439193968194,
0.0796751372024612));
#90643=CARTESIAN_POINT('Ctrl Pts',(0.009903033732493,-0.0341934961088739,
0.0796192219702256));
#90644=CARTESIAN_POINT('Ctrl Pts',(0.00955708048208011,-0.0346945769586966,
0.0797199220672997));
#90645=CARTESIAN_POINT('Ctrl Pts',(0.00973212233481061,-0.0344439193968194,
0.0796748788539503));
#90646=CARTESIAN_POINT('Ctrl Pts',(0.00990399049566172,-0.0341934961088739,
0.0796189335542208));
#90647=CARTESIAN_POINT('',(0.00955610749708528,-0.0346945769586966,0.0797201498385222));
#90648=CARTESIAN_POINT('',(0.00978374540824895,-0.0343667727783613,0.0796566003227611));
#90649=CARTESIAN_POINT('Origin',(0.00519187396474237,-0.0345626461564454,
0.0634828251698361));
#90650=CARTESIAN_POINT('Origin',(0.0129736430949094,-0.0341934771027892,
0.0902384341944277));
#90651=CARTESIAN_POINT('',(0.00966367288018327,-0.034193496108874,0.0796913772360182));
#90652=CARTESIAN_POINT('',(0.0097235130932707,-0.034193496108884,0.0796733384195801));
#90653=CARTESIAN_POINT('',(0.00943470755461163,-0.0345211943011844,0.0797499642575745));
#90654=CARTESIAN_POINT('Origin',(0.00566078612732884,-0.0345625596119786,
0.0633764692885998));
#90655=CARTESIAN_POINT('Origin',(0.0119561510488986,-0.0346945685853894,
0.0905209799622138));
#90656=CARTESIAN_POINT('',(0.0094952526983499,-0.0346945769587026,0.0797343956614295));
#90657=CARTESIAN_POINT('Ctrl Pts',(0.00926134066521218,-0.0345231616327842,
0.0800411765142948));
#90658=CARTESIAN_POINT('Ctrl Pts',(0.00934254223934864,-0.0344132092796988,
0.080025496872311));
#90659=CARTESIAN_POINT('Ctrl Pts',(0.00942341530283064,-0.034303273855898,
0.0800081384488146));
#90660=CARTESIAN_POINT('Ctrl Pts',(0.00950385681755585,-0.034193496108874,
0.0799891261359033));
#90661=CARTESIAN_POINT('Ctrl Pts',(0.00931901326963669,-0.0345231616327842,
0.0799436316177729));
#90662=CARTESIAN_POINT('Ctrl Pts',(0.00939887032470682,-0.0344132092796988,
0.0799271570401337));
#90663=CARTESIAN_POINT('Ctrl Pts',(0.0094783824958765,-0.034303273855898,
0.0799090315323132));
#90664=CARTESIAN_POINT('Ctrl Pts',(0.00955744851367657,-0.034193496108874,
0.0798892809244735));
#90665=CARTESIAN_POINT('Ctrl Pts',(0.0093766858740612,-0.0345231616327842,
0.0798460867212511));
#90666=CARTESIAN_POINT('Ctrl Pts',(0.00945519841006501,-0.0344132092796988,
0.0798288172079564));
#90667=CARTESIAN_POINT('Ctrl Pts',(0.00953334968892237,-0.034303273855898,
0.0798099246158118));
#90668=CARTESIAN_POINT('Ctrl Pts',(0.00961104020979729,-0.034193496108874,
0.0797894357130436));
#90669=CARTESIAN_POINT('Ctrl Pts',(0.00943435847848571,-0.0345231616327842,
0.0797485418247292));
#90670=CARTESIAN_POINT('Ctrl Pts',(0.00951152649542319,-0.0344132092796988,
0.0797304773757791));
#90671=CARTESIAN_POINT('Ctrl Pts',(0.00958831688196824,-0.034303273855898,
0.0797108176993104));
#90672=CARTESIAN_POINT('Ctrl Pts',(0.00966463190591801,-0.034193496108874,
0.0796895905016138));
#90673=CARTESIAN_POINT('',(0.00958376484888037,-0.0341934961088839,0.0798402516859692));
#90674=CARTESIAN_POINT('Ctrl Pts',(0.00949138119004756,-0.0342105180195399,
0.0799920606744457));
#90675=CARTESIAN_POINT('Ctrl Pts',(0.00948158630167239,-0.034261055624461,
0.0799502192192273));
#90676=CARTESIAN_POINT('Ctrl Pts',(0.00947196717751276,-0.0343122189876677,
0.0799091285872833));
#90677=CARTESIAN_POINT('Ctrl Pts',(0.00945307250016098,-0.0344158093694418,
0.0798284149776943));
#90678=CARTESIAN_POINT('Ctrl Pts',(0.00944380326859656,-0.0344682017128875,
0.0797888190045534));
#90679=CARTESIAN_POINT('Ctrl Pts',(0.00943470755419452,-0.0345211942998157,
0.0797499642558054));
#90680=CARTESIAN_POINT('Ctrl Pts',(0.00955438467010664,-0.0346945769586932,
0.079719080617007));
#90681=CARTESIAN_POINT('Ctrl Pts',(0.00966952147126994,-0.0345296777077528,
0.0796895039230667));
#90682=CARTESIAN_POINT('Ctrl Pts',(0.00978333745753671,-0.0343648066252515,
0.0796551937922497));
#90683=CARTESIAN_POINT('Ctrl Pts',(0.00955610749707654,-0.0346945769586932,
0.0797201498385244));
#90684=CARTESIAN_POINT('Ctrl Pts',(0.00967126640363815,-0.0345296777077528,
0.0796905375263556));
#90685=CARTESIAN_POINT('Ctrl Pts',(0.00978510300428032,-0.0343648066252515,
0.0796561908941089));
#90686=CARTESIAN_POINT('Ctrl Pts',(0.00984323392393309,-0.0346945769586932,
0.0798983463487799));
#90687=CARTESIAN_POINT('Ctrl Pts',(0.00996207691725521,-0.0345296777077528,
0.0798627979009019));
#90688=CARTESIAN_POINT('Ctrl Pts',(0.0100793491107082,-0.0343648066252515,
0.0798223679386087));
#90689=CARTESIAN_POINT('Ctrl Pts',(0.00985550856950412,-0.0346775396670096,
0.079894660454654));
#90690=CARTESIAN_POINT('Ctrl Pts',(0.00984310992023194,-0.0346269749924949,
0.0798535304275722));
#90691=CARTESIAN_POINT('Ctrl Pts',(0.00983093158822074,-0.0345757902884401,
0.0798131313832144));
#90692=CARTESIAN_POINT('Ctrl Pts',(0.0098070062949466,-0.0344721707091871,
0.0797337639320363));
#90693=CARTESIAN_POINT('Ctrl Pts',(0.00979526693812728,-0.034419768761444,
0.07969482073193));
#90694=CARTESIAN_POINT('Ctrl Pts',(0.00978374540745166,-0.0343667727795891,
0.0796566003212991));
#90695=CARTESIAN_POINT('',(0.00969967071051292,-0.0346945769587026,0.0798092480936557));
#90696=CARTESIAN_POINT('Ctrl Pts',(0.00962646358114103,-0.0352450361874068,
0.0797016398384676));
#90697=CARTESIAN_POINT('Ctrl Pts',(0.0098358471134729,-0.0349452760959493,
0.0796449652799317));
#90698=CARTESIAN_POINT('Ctrl Pts',(0.0100403668495881,-0.034644428984174,
0.079572680103468));
#90699=CARTESIAN_POINT('Ctrl Pts',(0.00962886167139528,-0.0352450361874068,
0.079700933323689));
#90700=CARTESIAN_POINT('Ctrl Pts',(0.00983821855708501,-0.0349452760959493,
0.0796441683196949));
#90701=CARTESIAN_POINT('Ctrl Pts',(0.0100427049095364,-0.034644428984174,
0.0795717949618532));
#90702=CARTESIAN_POINT('Ctrl Pts',(0.00986867070047367,-0.0352450361874068,
0.0796302818447427));
#90703=CARTESIAN_POINT('Ctrl Pts',(0.0100753629219099,-0.0349452760959493,
0.079564472294803));
#90704=CARTESIAN_POINT('Ctrl Pts',(0.0102765109079304,-0.034644428984174,
0.079483280799033));
#90705=CARTESIAN_POINT('',(0.00990300343087755,-0.0351951633467188,0.079619234032487));
#90706=CARTESIAN_POINT('',(0.0101262321451419,-0.0348678972925388,0.0795415043531098));
#90707=CARTESIAN_POINT('Origin',(0.00389834399728346,-0.034563163330209,
0.0639869625528435));
#90708=CARTESIAN_POINT('Origin',(0.0139734550134733,-0.034694619934117,
0.0898999726470576));
#90709=CARTESIAN_POINT('',(0.0100085801961753,-0.0346945769330289,0.0795837520633418));
#90710=CARTESIAN_POINT('',(0.0100671696698855,-0.0346945769458128,0.079561991441613));
#90711=CARTESIAN_POINT('',(0.00978374540818223,-0.0350221583435275,0.0796566003236664));
#90712=CARTESIAN_POINT('Origin',(0.004333766220623,-0.0345628458714157,
0.0637815986319168));
#90713=CARTESIAN_POINT('',(0.00978338552135528,-0.0351951360298762,0.079655416949585));
#90714=CARTESIAN_POINT('Origin',(0.0129636962171911,-0.0351951838366802,
0.0902054628140545));
#90715=CARTESIAN_POINT('',(0.00990303372741004,-0.0351951371328746,0.0796192219718791));
#90716=CARTESIAN_POINT('Ctrl Pts',(0.0096290069173802,-0.0350241211494342,
0.0799581234946824));
#90717=CARTESIAN_POINT('Ctrl Pts',(0.00970901143709608,-0.0349144232818961,
0.0799373896412717));
#90718=CARTESIAN_POINT('Ctrl Pts',(0.00978863525980772,-0.0348045283579412,
0.0799149896270596));
#90719=CARTESIAN_POINT('Ctrl Pts',(0.00986777532983583,-0.0346945769439157,
0.0798909483484079));
#90720=CARTESIAN_POINT('Ctrl Pts',(0.00968044081854037,-0.0350241211494342,
0.079857149757431));
#90721=CARTESIAN_POINT('Ctrl Pts',(0.00975905446642646,-0.0349144232818961,
0.0798357074231205));
#90722=CARTESIAN_POINT('Ctrl Pts',(0.00983727193999802,-0.0348045283579412,
0.0798126272542633));
#90723=CARTESIAN_POINT('Ctrl Pts',(0.00991499195251126,-0.0346945769439157,
0.0797879350854453));
#90724=CARTESIAN_POINT('Ctrl Pts',(0.00973187471970054,-0.0350241211494342,
0.0797561760201796));
#90725=CARTESIAN_POINT('Ctrl Pts',(0.00980909749575684,-0.0349144232818961,
0.0797340252049694));
#90726=CARTESIAN_POINT('Ctrl Pts',(0.00988590862018833,-0.0348045283579412,
0.0797102648814671));
#90727=CARTESIAN_POINT('Ctrl Pts',(0.00996220857518668,-0.0346945769439157,
0.0796849218224828));
#90728=CARTESIAN_POINT('Ctrl Pts',(0.0097833086208607,-0.0350241211494342,
0.0796552022829283));
#90729=CARTESIAN_POINT('Ctrl Pts',(0.00985914052508721,-0.0349144232818961,
0.0796323429868183));
#90730=CARTESIAN_POINT('Ctrl Pts',(0.00993454530037863,-0.0348045283579412,
0.0796079025086708));
#90731=CARTESIAN_POINT('Ctrl Pts',(0.0100094251978621,-0.0346945769439157,
0.0795819085595203));
#90732=CARTESIAN_POINT('',(0.00993817775744595,-0.0346945769458128,0.0797373502076673));
#90733=CARTESIAN_POINT('Ctrl Pts',(0.00985550857068307,-0.0347116136492799,
0.0798946604506295));
#90734=CARTESIAN_POINT('Ctrl Pts',(0.00984311485760916,-0.0347621546531828,
0.0798535467537695));
#90735=CARTESIAN_POINT('Ctrl Pts',(0.00983093905950229,-0.0348133084096042,
0.0798131559468007));
#90736=CARTESIAN_POINT('Ctrl Pts',(0.00980701313164405,-0.0349168561544573,
0.0797337864036143));
#90737=CARTESIAN_POINT('Ctrl Pts',(0.00979527249212791,-0.0349692089015919,
0.0796948391493789));
#90738=CARTESIAN_POINT('Ctrl Pts',(0.00978374540819085,-0.0350221583435,
0.0796566003236256));
#90739=CARTESIAN_POINT('Ctrl Pts',(0.00990174466699582,-0.0351951371254965,
0.0796185300671819));
#90740=CARTESIAN_POINT('Ctrl Pts',(0.0099770551292594,-0.0350856248736052,
0.079594044661753));
#90741=CARTESIAN_POINT('Ctrl Pts',(0.0100519213945189,-0.0349758427080733,
0.0795679827719899));
#90742=CARTESIAN_POINT('Ctrl Pts',(0.0101262456568789,-0.0348659306897824,
0.0795403721328392));
#90743=CARTESIAN_POINT('Ctrl Pts',(0.00997419059529331,-0.0351951371254965,
0.0796574152587592));
#90744=CARTESIAN_POINT('Ctrl Pts',(0.0100500365692423,-0.0350856248736052,
0.0796319321562741));
#90745=CARTESIAN_POINT('Ctrl Pts',(0.0101254181671598,-0.0349758427080733,
0.0796048606834117));
#90746=CARTESIAN_POINT('Ctrl Pts',(0.0102002368474823,-0.0348659306897824,
0.0795762298288608));
#90747=CARTESIAN_POINT('Ctrl Pts',(0.0100466365235908,-0.0351951371254965,
0.0796963004503364));
#90748=CARTESIAN_POINT('Ctrl Pts',(0.0101230180092252,-0.0350856248736052,
0.0796698196507952));
#90749=CARTESIAN_POINT('Ctrl Pts',(0.0101989149398007,-0.0349758427080734,
0.0796417385948336));
#90750=CARTESIAN_POINT('Ctrl Pts',(0.0102742280380856,-0.0348659306897824,
0.0796120875248825));
#90751=CARTESIAN_POINT('Ctrl Pts',(0.0101190824518883,-0.0351951371254965,
0.0797351856419137));
#90752=CARTESIAN_POINT('Ctrl Pts',(0.0101959994492081,-0.0350856248736052,
0.0797077071453163));
#90753=CARTESIAN_POINT('Ctrl Pts',(0.0102724117124416,-0.0349758427080734,
0.0796786165062554));
#90754=CARTESIAN_POINT('Ctrl Pts',(0.010348219228689,-0.0348659306897824,
0.0796479452209042));
#90755=CARTESIAN_POINT('Origin',(0.0119778629691043,-0.0308609197410555,
0.0845269351437275));
#90756=CARTESIAN_POINT('',(0.00999722610289499,-0.0351951371254965,0.0796697795164507));
#90757=CARTESIAN_POINT('Ctrl Pts',(0.00751557654030228,-0.0321934096636942,
0.0798691102123334));
#90758=CARTESIAN_POINT('Ctrl Pts',(0.00766901285885221,-0.0319797282160096,
0.079885427582138));
#90759=CARTESIAN_POINT('Ctrl Pts',(0.00782310337371433,-0.0317669959605189,
0.0798934944053677));
#90760=CARTESIAN_POINT('Ctrl Pts',(0.00776473354553151,-0.0321934096636942,
0.0798901401610652));
#90761=CARTESIAN_POINT('Ctrl Pts',(0.00791873407036402,-0.0319797282160096,
0.0798997729711736));
#90762=CARTESIAN_POINT('Ctrl Pts',(0.00807302956171172,-0.0317669959605189,
0.0799011345985298));
#90763=CARTESIAN_POINT('Ctrl Pts',(0.00776622828223816,-0.0321934096636942,
0.0798902663234273));
#90764=CARTESIAN_POINT('Ctrl Pts',(0.00792023219184342,-0.0319797282160096,
0.0798998590316861));
#90765=CARTESIAN_POINT('Ctrl Pts',(0.0080745289128811,-0.0317669959605189,
0.0799011804333927));
#90766=CARTESIAN_POINT('',(0.00776473354564076,-0.0321934096636943,0.0798901401610721));
#90767=CARTESIAN_POINT('',(0.00800086794439121,-0.0318665617561286,0.0799000449639514));
#90768=CARTESIAN_POINT('Origin',(0.00942093499841772,-0.032637194442062,
0.0632626057202205));
#90769=CARTESIAN_POINT('Origin',(0.00776661269360889,-0.0316939261509253,
0.0908587271204895));
#90770=CARTESIAN_POINT('',(0.00764033085304629,-0.0320197259213214,0.0798809584455136));
#90771=CARTESIAN_POINT('Ctrl Pts',(0.00764050362844855,-0.0320197391311198,
0.0798810188942161));
#90772=CARTESIAN_POINT('Ctrl Pts',(0.00766966489836095,-0.0319792715672862,
0.0798834779712017));
#90773=CARTESIAN_POINT('Ctrl Pts',(0.00769897767596132,-0.031938643888646,
0.0798857258450869));
#90774=CARTESIAN_POINT('Ctrl Pts',(0.00772847330676439,-0.0318979098685801,
0.0798877564685929));
#90775=CARTESIAN_POINT('Ctrl Pts',(0.0077579683544451,-0.0318571766538172,
0.079889787051954));
#90776=CARTESIAN_POINT('Ctrl Pts',(0.00778749639970253,-0.0318163871807225,
0.0798915918578671));
#90777=CARTESIAN_POINT('Ctrl Pts',(0.00781695548280018,-0.0317755399642095,
0.0798931683778834));
#90778=CARTESIAN_POINT('Origin',(0.0074784479685726,-0.0323427512858111,
0.0817957411220363));
#90779=CARTESIAN_POINT('',(0.00770245499135762,-0.0321934096636663,0.0798848835767754));
#90780=CARTESIAN_POINT('Ctrl Pts',(0.0077634250783826,-0.0321934096636618,
0.0798885904511592));
#90781=CARTESIAN_POINT('Ctrl Pts',(0.00788206584516462,-0.032028746738191,
0.0798960405462253));
#90782=CARTESIAN_POINT('Ctrl Pts',(0.00800091315369981,-0.0318646057455573,
0.0798985807653214));
#90783=CARTESIAN_POINT('Ctrl Pts',(0.00776473354555483,-0.0321934096636618,
0.0798901401610666));
#90784=CARTESIAN_POINT('Ctrl Pts',(0.00788340635134942,-0.032028746738191,
0.0798975632046207));
#90785=CARTESIAN_POINT('Ctrl Pts',(0.00800228455346166,-0.0318646057455573,
0.0799000750711239));
#90786=CARTESIAN_POINT('Ctrl Pts',(0.00798274125480844,-0.0321934096636618,
0.0801483420587596));
#90787=CARTESIAN_POINT('Ctrl Pts',(0.00810675217827977,-0.032028746738191,
0.0801512579673282));
#90788=CARTESIAN_POINT('Ctrl Pts',(0.00823077765355593,-0.0318646057455573,
0.0801490459217784));
#90789=CARTESIAN_POINT('Ctrl Pts',(0.00799555414024659,-0.0321763980313103,
0.0801486296390504));
#90790=CARTESIAN_POINT('Ctrl Pts',(0.00799647135765932,-0.0321259597689058,
0.0801057206915783));
#90791=CARTESIAN_POINT('Ctrl Pts',(0.0079973726528313,-0.0320749162472279,
0.080063554809537));
#90792=CARTESIAN_POINT('Ctrl Pts',(0.00799914427494874,-0.0319716059728889,
0.0799806768399453));
#90793=CARTESIAN_POINT('Ctrl Pts',(0.00800001393905037,-0.0319193783913111,
0.0799399960433909));
#90794=CARTESIAN_POINT('Ctrl Pts',(0.00800086794435303,-0.031866561756148,
0.0799000449639248));
#90795=CARTESIAN_POINT('',(0.00787373740024513,-0.0321934096636664,0.0800192411099193));
#90796=CARTESIAN_POINT('Ctrl Pts',(0.00783732086283825,-0.0327445246967097,
0.0798942750766532));
#90797=CARTESIAN_POINT('Ctrl Pts',(0.00805396973908347,-0.032443687833936,
0.0799050791423469));
#90798=CARTESIAN_POINT('Ctrl Pts',(0.00827081694513738,-0.0321434074405928,
0.0798995336360174));
#90799=CARTESIAN_POINT('Ctrl Pts',(0.00783981990673068,-0.0327445246967097,
0.0798943442114757));
#90800=CARTESIAN_POINT('Ctrl Pts',(0.00805647139043836,-0.032443687833936,
0.0799050540241882));
#90801=CARTESIAN_POINT('Ctrl Pts',(0.00827331409702744,-0.0321434074405928,
0.0798994143362355));
#90802=CARTESIAN_POINT('Ctrl Pts',(0.0080897242959742,-0.0327445246967097,
0.079901257693726));
#90803=CARTESIAN_POINT('Ctrl Pts',(0.00830663652592757,-0.032443687833936,
0.0799025422083154));
#90804=CARTESIAN_POINT('Ctrl Pts',(0.0085230292860335,-0.0321434074405928,
0.0798874843580433));
#90805=CARTESIAN_POINT('',(0.00812586842896101,-0.0326943950436612,0.0799013581567853));
#90806=CARTESIAN_POINT('',(0.00836215879818742,-0.0323666188837389,0.0798964164132224));
#90807=CARTESIAN_POINT('Origin',(0.00804376040539544,-0.0326395579112528,
0.0630906081289521));
#90808=CARTESIAN_POINT('Origin',(0.00881992596082919,-0.0321933825603174,
0.0909315340399853));
#90809=CARTESIAN_POINT('',(0.00823720989640445,-0.0321934096536378,0.0799002399215511));
#90810=CARTESIAN_POINT('',(0.00829965619325201,-0.0321934096584275,0.0798976494835474));
#90811=CARTESIAN_POINT('',(0.00800086794438665,-0.0325210109756239,0.0799000449639513));
#90812=CARTESIAN_POINT('Origin',(0.00852391591854703,-0.0326393129156286,
0.0631158095705174));
#90813=CARTESIAN_POINT('Origin',(0.00776447660749309,-0.0326943765538264,
0.0909586154069157));
#90814=CARTESIAN_POINT('',(0.00806338270354571,-0.0326943950436703,0.0799000224479366));
#90815=CARTESIAN_POINT('Ctrl Pts',(0.00776052600373539,-0.032522978320377,
0.0801389936500988));
#90816=CARTESIAN_POINT('Ctrl Pts',(0.00784308415023136,-0.0324130253092451,
0.0801440011287255));
#90817=CARTESIAN_POINT('Ctrl Pts',(0.00792573336129477,-0.032303122220807,
0.0801473000265561));
#90818=CARTESIAN_POINT('Ctrl Pts',(0.00800836762005261,-0.0321934096576659,
0.0801488898536619));
#90819=CARTESIAN_POINT('Ctrl Pts',(0.00784064516754767,-0.032522978320377,
0.0800588558823081));
#90820=CARTESIAN_POINT('Ctrl Pts',(0.00792209861666714,-0.0324130253092451,
0.0800627589200137));
#90821=CARTESIAN_POINT('Ctrl Pts',(0.00800362045112385,-0.032303122220807,
0.0800649763965177));
#90822=CARTESIAN_POINT('Ctrl Pts',(0.00808510614701406,-0.0321934096576659,
0.080065509156158));
#90823=CARTESIAN_POINT('Ctrl Pts',(0.00792076433135995,-0.032522978320377,
0.0799787181145175));
#90824=CARTESIAN_POINT('Ctrl Pts',(0.00800111308310293,-0.0324130253092451,
0.079981516711302));
#90825=CARTESIAN_POINT('Ctrl Pts',(0.00808150754095293,-0.032303122220807,
0.0799826527664793));
#90826=CARTESIAN_POINT('Ctrl Pts',(0.0081618446739755,-0.0321934096576659,
0.0799821284586541));
#90827=CARTESIAN_POINT('Ctrl Pts',(0.00800088349517223,-0.032522978320377,
0.0798985803467268));
#90828=CARTESIAN_POINT('Ctrl Pts',(0.00808012754953871,-0.0324130253092451,
0.0799002745025902));
#90829=CARTESIAN_POINT('Ctrl Pts',(0.00815939463078201,-0.032303122220807,
0.0799003291364409));
#90830=CARTESIAN_POINT('Ctrl Pts',(0.00823858320093694,-0.0321934096576659,
0.0798987477611502));
#90831=CARTESIAN_POINT('',(0.00812278875555212,-0.0321934096584275,0.0800245648876137));
#90832=CARTESIAN_POINT('Ctrl Pts',(0.00799555414278173,-0.032210423332892,
0.080148629635806));
#90833=CARTESIAN_POINT('Ctrl Pts',(0.0079964726199866,-0.0322609421831223,
0.080105662402296));
#90834=CARTESIAN_POINT('Ctrl Pts',(0.00799737456921036,-0.0323120888240433,
0.0800634683633959));
#90835=CARTESIAN_POINT('Ctrl Pts',(0.00799914620757039,-0.0324156524631811,
0.0799805894430405));
#90836=CARTESIAN_POINT('Ctrl Pts',(0.00800001516846968,-0.0324680267167311,
0.0799399386292009));
#90837=CARTESIAN_POINT('Ctrl Pts',(0.00800086794439211,-0.0325210109755913,
0.0799000449639081));
#90838=CARTESIAN_POINT('Origin',(0.000335215042199046,-0.0262834582511539,
0.0730357255385635));
#90839=CARTESIAN_POINT('Origin',(0.00245340408136264,-0.0342770951788246,
0.0849050601642025));
#90840=CARTESIAN_POINT('Ctrl Pts',(0.00812446557717303,-0.0326943950436605,
0.0798998940196011));
#90841=CARTESIAN_POINT('Ctrl Pts',(0.00824334049677372,-0.0325294772287039,
0.0798998798911275));
#90842=CARTESIAN_POINT('Ctrl Pts',(0.00836211325541952,-0.0323646534831895,
0.0798949525679849));
#90843=CARTESIAN_POINT('Ctrl Pts',(0.00812586842895898,-0.0326943950436605,
0.0799013581567853));
#90844=CARTESIAN_POINT('Ctrl Pts',(0.00824477361854195,-0.0325294772287039,
0.0799013150253609));
#90845=CARTESIAN_POINT('Ctrl Pts',(0.00836357542258684,-0.0323646534831895,
0.0798963574729647));
#90846=CARTESIAN_POINT('Ctrl Pts',(0.00835965858109641,-0.0326943950436605,
0.0801453617346851));
#90847=CARTESIAN_POINT('Ctrl Pts',(0.00848360836899827,-0.0325294772287039,
0.0801404851601669));
#90848=CARTESIAN_POINT('Ctrl Pts',(0.00860725069029517,-0.0323646534831895,
0.0801304897970287));
#90849=CARTESIAN_POINT('Ctrl Pts',(0.00837246424067422,-0.0326773559997669,
0.0801448442199106));
#90850=CARTESIAN_POINT('Ctrl Pts',(0.00837068394198459,-0.0326267924002051,
0.0801019278325357));
#90851=CARTESIAN_POINT('Ctrl Pts',(0.00836893514681326,-0.0325756107621945,
0.0800597717534306));
#90852=CARTESIAN_POINT('Ctrl Pts',(0.00836549930955373,-0.0324719987229852,
0.079976945783095));
#90853=CARTESIAN_POINT('Ctrl Pts',(0.00836381361313338,-0.0324196089018781,
0.0799363081939324));
#90854=CARTESIAN_POINT('Ctrl Pts',(0.00836215879814982,-0.0323666188837573,
0.0798964164131996));
#90855=CARTESIAN_POINT('',(0.00824276350503385,-0.0326943950436704,0.0800233599457397));
#90856=CARTESIAN_POINT('Ctrl Pts',(0.00819858638145413,-0.0332451089994434,
0.0799009274868521));
#90857=CARTESIAN_POINT('Ctrl Pts',(0.00841548616028705,-0.0329451141710254,
0.0798981062007301));
#90858=CARTESIAN_POINT('Ctrl Pts',(0.00863155723893576,-0.0326442513127494,
0.079878955151549));
#90859=CARTESIAN_POINT('Ctrl Pts',(0.00820110981899618,-0.0332451089994434,
0.0799008386726003));
#90860=CARTESIAN_POINT('Ctrl Pts',(0.00841800624814479,-0.0329451141710254,
0.0798979222134742));
#90861=CARTESIAN_POINT('Ctrl Pts',(0.00863406681780555,-0.0326442513127494,
0.0798786765139776));
#90862=CARTESIAN_POINT('Ctrl Pts',(0.00845095512019007,-0.0332451089994434,
0.0798920451823184));
#90863=CARTESIAN_POINT('Ctrl Pts',(0.00866751989742658,-0.0329451141710254,
0.0798797056534881));
#90864=CARTESIAN_POINT('Ctrl Pts',(0.00888253997323141,-0.0326442513127494,
0.0798510886356119));
#90865=CARTESIAN_POINT('Ctrl Pts',(0.00845345357320201,-0.0332451089994434,
0.0798919572474155));
#90866=CARTESIAN_POINT('Ctrl Pts',(0.00867001503391939,-0.0329451141710254,
0.0798795234878883));
#90867=CARTESIAN_POINT('Ctrl Pts',(0.00888502470478567,-0.0326442513127494,
0.0798508127568282));
#90868=CARTESIAN_POINT('',(0.00848699507891553,-0.0331951640388616,0.0798898781694026));
#90869=CARTESIAN_POINT('',(0.00872250890292996,-0.032867753235504,0.0798701093867858));
#90870=CARTESIAN_POINT('Origin',(0.00666296712443024,-0.0326402808280718,
0.0632253898936535));
#90871=CARTESIAN_POINT('Origin',(0.0098738294798772,-0.0326944278779006,
0.0908659651477627));
#90872=CARTESIAN_POINT('',(0.00859804663143739,-0.0326943950436593,0.0798817709516813));
#90873=CARTESIAN_POINT('',(0.00866020704697387,-0.0326943950436694,0.0798752645900675));
#90874=CARTESIAN_POINT('',(0.00836215879818454,-0.0330220786163546,0.0798964164132225));
#90875=CARTESIAN_POINT('Origin',(0.0071368455069605,-0.0326396682763202,
0.0631441992304724));
#90876=CARTESIAN_POINT('Origin',(0.00881933068583198,-0.0331952026560064,
0.0909172326935325));
#90877=CARTESIAN_POINT('',(0.00842454878495234,-0.0331951640388702,0.0798924686074329));
#90878=CARTESIAN_POINT('Ctrl Pts',(0.00813729579048197,-0.0330240426238173,
0.0801499847818743));
#90879=CARTESIAN_POINT('Ctrl Pts',(0.00821995142635422,-0.032914277406352,
0.0801497986189048));
#90880=CARTESIAN_POINT('Ctrl Pts',(0.00830264442056684,-0.0328043479726691,
0.0801479036402456));
#90881=CARTESIAN_POINT('Ctrl Pts',(0.00838526877037963,-0.0326943950436594,
0.0801442993560502));
#90882=CARTESIAN_POINT('Ctrl Pts',(0.00821222493349814,-0.0330240426238173,
0.0800649744324369));
#90883=CARTESIAN_POINT('Ctrl Pts',(0.00829370946898532,-0.032914277406352,
0.0800637560475224));
#90884=CARTESIAN_POINT('Ctrl Pts',(0.00837520944006565,-0.0328043479726691,
0.0800608525422343));
#90885=CARTESIAN_POINT('Ctrl Pts',(0.00845662033676901,-0.0326943950436594,
0.0800562647608141));
#90886=CARTESIAN_POINT('Ctrl Pts',(0.00828715407651431,-0.0330240426238173,
0.0799799640829995));
#90887=CARTESIAN_POINT('Ctrl Pts',(0.00836746751161642,-0.032914277406352,
0.07997771347614));
#90888=CARTESIAN_POINT('Ctrl Pts',(0.00844777445956445,-0.0328043479726691,
0.0799738014442229));
#90889=CARTESIAN_POINT('Ctrl Pts',(0.00852797190315839,-0.0326943950436594,
0.079968230165578));
#90890=CARTESIAN_POINT('Ctrl Pts',(0.00836208321953047,-0.0330240426238173,
0.0798949537335621));
#90891=CARTESIAN_POINT('Ctrl Pts',(0.00844122555424752,-0.032914277406352,
0.0798916709047577));
#90892=CARTESIAN_POINT('Ctrl Pts',(0.00852033947906325,-0.0328043479726691,
0.0798867503462116));
#90893=CARTESIAN_POINT('Ctrl Pts',(0.00859932346954776,-0.0326943950436594,
0.0798801955703419));
#90894=CARTESIAN_POINT('',(0.00849165770091852,-0.0326943950436694,0.0800130351538757));
#90895=CARTESIAN_POINT('Ctrl Pts',(0.00837246424284239,-0.0327114338383319,
0.0801448442163262));
#90896=CARTESIAN_POINT('Ctrl Pts',(0.00837068424772592,-0.0327619876830903,
0.0801019348328769));
#90897=CARTESIAN_POINT('Ctrl Pts',(0.00836893565550443,-0.0328131562604201,
0.0800597824621015));
#90898=CARTESIAN_POINT('Ctrl Pts',(0.00836549980542918,-0.0329167375858768,
0.0799769562751137));
#90899=CARTESIAN_POINT('Ctrl Pts',(0.00836381391659571,-0.0329691088920615,
0.0799363154611364));
#90900=CARTESIAN_POINT('Ctrl Pts',(0.00836215879818539,-0.0330220786163187,
0.0798964164131748));
#90901=CARTESIAN_POINT('Ctrl Pts',(0.0084855028232013,-0.0331951640388604,
0.0798885047879282));
#90902=CARTESIAN_POINT('Ctrl Pts',(0.00860414273050473,-0.033030642201062,
0.0798810264458146));
#90903=CARTESIAN_POINT('Ctrl Pts',(0.0087223721730947,-0.0328657861914645,
0.0798686509817587));
#90904=CARTESIAN_POINT('Ctrl Pts',(0.0084869950789124,-0.0331951640388604,
0.0798898781694028));
#90905=CARTESIAN_POINT('Ctrl Pts',(0.00860566337999729,-0.033030642201062,
0.0798823689758592));
#90906=CARTESIAN_POINT('Ctrl Pts',(0.00872391991698437,-0.0328657861914645,
0.0798699615131906));
#90907=CARTESIAN_POINT('Ctrl Pts',(0.00873564501101464,-0.0331951640388604,
0.0801187204568676));
#90908=CARTESIAN_POINT('Ctrl Pts',(0.00885904447967284,-0.033030642201062,
0.0801060705853973));
#90909=CARTESIAN_POINT('Ctrl Pts',(0.00898181567185892,-0.0328657861914645,
0.0800883312933441));
#90910=CARTESIAN_POINT('Ctrl Pts',(0.0087483929067007,-0.033178164828644,
0.0801173998893635));
#90911=CARTESIAN_POINT('Ctrl Pts',(0.00874391828725666,-0.033127681154678,
0.0800746504291126));
#90912=CARTESIAN_POINT('Ctrl Pts',(0.00873952443194941,-0.0330765663497795,
0.0800326728952462));
#90913=CARTESIAN_POINT('Ctrl Pts',(0.00873089463578463,-0.0329730614463183,
0.0799502255973295));
#90914=CARTESIAN_POINT('Ctrl Pts',(0.00872666218650641,-0.0329207133373643,
0.0799097891396196));
#90915=CARTESIAN_POINT('Ctrl Pts',(0.00872250888993246,-0.0328677532289395,
0.0798701093969079));
#90916=CARTESIAN_POINT('',(0.00861132004496886,-0.0331951640388702,0.0800042993131388));
#90917=CARTESIAN_POINT('Ctrl Pts',(0.00855954660528496,-0.0337436976235976,
0.0798848814832637));
#90918=CARTESIAN_POINT('Ctrl Pts',(0.00861112699849052,-0.0336723290703325,
0.0798809621520986));
#90919=CARTESIAN_POINT('Ctrl Pts',(0.00866262855078964,-0.033601104548885,
0.0798761156862932));
#90920=CARTESIAN_POINT('Ctrl Pts',(0.00882706280539791,-0.0333736987606857,
0.0798606418810075));
#90921=CARTESIAN_POINT('Ctrl Pts',(0.00899033810919476,-0.0331450831799192,
0.0798357573896796));
#90922=CARTESIAN_POINT('Ctrl Pts',(0.00856203460757845,-0.0337436976235976,
0.0798846368517293));
#90923=CARTESIAN_POINT('Ctrl Pts',(0.0086136128005309,-0.0336723290703325,
0.0798806951430946));
#90924=CARTESIAN_POINT('Ctrl Pts',(0.00866511175043273,-0.033601104548885,
0.0798758263430152));
#90925=CARTESIAN_POINT('Ctrl Pts',(0.00882953769610195,-0.0333736987606857,
0.0798602812288169));
#90926=CARTESIAN_POINT('Ctrl Pts',(0.00899280061253565,-0.0331450831799192,
0.0798353260229029));
#90927=CARTESIAN_POINT('Ctrl Pts',(0.00881083483692663,-0.0337436976235976,
0.0798601736982883));
#90928=CARTESIAN_POINT('Ctrl Pts',(0.00886219300456955,-0.0336723290703325,
0.079853994242684));
#90929=CARTESIAN_POINT('Ctrl Pts',(0.00891343171474199,-0.033601104548885,
0.0798468920152118));
#90930=CARTESIAN_POINT('Ctrl Pts',(0.00907702676650588,-0.0333736987606857,
0.079824216009765));
#90931=CARTESIAN_POINT('Ctrl Pts',(0.00923905094662548,-0.0331450831799192,
0.0797921893452301));
#90932=CARTESIAN_POINT('Ctrl Pts',(0.00881334771924304,-0.0337436976235976,
0.0798599266204385));
#90933=CARTESIAN_POINT('Ctrl Pts',(0.00886470366463034,-0.0336723290703325,
0.0798537245635899));
#90934=CARTESIAN_POINT('Ctrl Pts',(0.00891593974638151,-0.033601104548885,
0.079846599778501));
#90935=CARTESIAN_POINT('Ctrl Pts',(0.00907952640611696,-0.0333736987606857,
0.0798238517510526));
#90936=CARTESIAN_POINT('Ctrl Pts',(0.0092415380749998,-0.0331450831799192,
0.0797917536647857));
#90937=CARTESIAN_POINT('',(0.00884668829355914,-0.0336938721132548,0.0798557455051844));
#90938=CARTESIAN_POINT('',(0.00908049609245075,-0.0333679870047996,0.0798212276902747));
#90939=CARTESIAN_POINT('Ctrl Pts',(0.00884668829355328,-0.0336938721132542,
0.0798557455051857));
#90940=CARTESIAN_POINT('Ctrl Pts',(0.00886896049488146,-0.0336629187933887,
0.0798529236635531));
#90941=CARTESIAN_POINT('Ctrl Pts',(0.00889120905000746,-0.0336319952301025,
0.0798499723117194));
#90942=CARTESIAN_POINT('Ctrl Pts',(0.00891343171474876,-0.0336011045488936,
0.0798468920152112));
#90943=CARTESIAN_POINT('Ctrl Pts',(0.00896919598475278,-0.0335235892595438,
0.0798391624972537));
#90944=CARTESIAN_POINT('Ctrl Pts',(0.00902489629397583,-0.0334458668665558,
0.0798306071584675));
#90945=CARTESIAN_POINT('Ctrl Pts',(0.00908049608084341,-0.0333679869962482,
0.0798212276924733));
#90946=CARTESIAN_POINT('Ctrl Pts',(0.00908054005010003,-0.0333679692468943,
0.0798212209721364));
#90947=CARTESIAN_POINT('Ctrl Pts',(0.00908045881507262,-0.0333391895412312,
0.0798207750588555));
#90948=CARTESIAN_POINT('Ctrl Pts',(0.00908039473082887,-0.0333104081126143,
0.0798204414070563));
#90949=CARTESIAN_POINT('Ctrl Pts',(0.00908030447069118,-0.0332532732084331,
0.0798200008325513));
#90950=CARTESIAN_POINT('Ctrl Pts',(0.00908027773360654,-0.0332249236067027,
0.079819890576674));
#90951=CARTESIAN_POINT('Ctrl Pts',(0.0090802703182882,-0.0331961055133883,
0.0798198880777076));
#90952=CARTESIAN_POINT('Ctrl Pts',(0.00908027020192905,-0.0331956347145507,
0.0798198880667067));
#90953=CARTESIAN_POINT('Ctrl Pts',(0.0090802700914211,-0.0331951640388597,
0.0798198880853489));
#90954=CARTESIAN_POINT('',(0.00895701165478286,-0.0331951640388587,0.0798406813005297));
#90955=CARTESIAN_POINT('',(0.00901864087311192,-0.0331951640388688,0.0798302846929493));
#90956=CARTESIAN_POINT('',(0.00872250888822892,-0.0335216366567653,0.07987010938183));
#90957=CARTESIAN_POINT('Origin',(0.00578895674576758,-0.0326434571525012,
0.0634760575075271));
#90958=CARTESIAN_POINT('Origin',(0.00985921721683401,-0.0336938867896249,
0.0907299921631417));
#90959=CARTESIAN_POINT('',(0.00878452787803477,-0.0336938721132539,0.0798622518668191));
#90960=CARTESIAN_POINT('Ctrl Pts',(0.00851401224513785,-0.0335235895815172,
0.0801372965941676));
#90961=CARTESIAN_POINT('Ctrl Pts',(0.00859643917065879,-0.0334144449262749,
0.0801319243092091));
#90962=CARTESIAN_POINT('Ctrl Pts',(0.00867884980736672,-0.0333049234473147,
0.080124842973898));
#90963=CARTESIAN_POINT('Ctrl Pts',(0.00876113795713087,-0.0331951640388588,
0.0801160520975017));
#90964=CARTESIAN_POINT('Ctrl Pts',(0.0085834557729539,-0.0335235895815172,
0.0800477490150239));
#90965=CARTESIAN_POINT('Ctrl Pts',(0.00866464989974497,-0.0334144449262749,
0.0800414207031833));
#90966=CARTESIAN_POINT('Ctrl Pts',(0.00874580657059074,-0.0333049234473147,
0.0800334077113251));
#90967=CARTESIAN_POINT('Ctrl Pts',(0.00882682108288447,-0.0331951640388588,
0.0800237108852655));
#90968=CARTESIAN_POINT('Ctrl Pts',(0.00865289930076994,-0.0335235895815172,
0.0799582014358803));
#90969=CARTESIAN_POINT('Ctrl Pts',(0.00873286062883114,-0.0334144449262749,
0.0799509170971576));
#90970=CARTESIAN_POINT('Ctrl Pts',(0.00881276333381477,-0.0333049234473147,
0.0799419724487521));
#90971=CARTESIAN_POINT('Ctrl Pts',(0.00889250420863806,-0.0331951640388588,
0.0799313696730293));
#90972=CARTESIAN_POINT('Ctrl Pts',(0.00872234282858598,-0.0335235895815172,
0.0798686538567367));
#90973=CARTESIAN_POINT('Ctrl Pts',(0.00880107135791731,-0.0334144449262749,
0.0798604134911319));
#90974=CARTESIAN_POINT('Ctrl Pts',(0.0088797200970388,-0.0333049234473147,
0.0798505371861792));
#90975=CARTESIAN_POINT('Ctrl Pts',(0.00895818733439166,-0.0331951640388588,
0.079839028460793));
#90976=CARTESIAN_POINT('',(0.00885907480596688,-0.0331951640388687,0.0799783666990257));
#90977=CARTESIAN_POINT('Ctrl Pts',(0.00874839290846162,-0.0332121607145976,
0.0801173998855383));
#90978=CARTESIAN_POINT('Ctrl Pts',(0.00874392582848732,-0.0332625444109666,
0.080074722339553));
#90979=CARTESIAN_POINT('Ctrl Pts',(0.00873953572331102,-0.0333135300746638,
0.0800327801946574));
#90980=CARTESIAN_POINT('Ctrl Pts',(0.00873090597774284,-0.0334167203140545,
0.0799503334138866));
#90981=CARTESIAN_POINT('Ctrl Pts',(0.00872666967972461,-0.0334688847587225,
0.0799098607103485));
#90982=CARTESIAN_POINT('Ctrl Pts',(0.00872250888831297,-0.0335216366562276,
0.0798701093811075));
#90983=CARTESIAN_POINT('Ctrl Pts',(0.00884511311559296,-0.0336938721132538,
0.0798544688319359));
#90984=CARTESIAN_POINT('Ctrl Pts',(0.00887850326461507,-0.0336474569765032,
0.079850246642683));
#90985=CARTESIAN_POINT('Ctrl Pts',(0.00891184169966668,-0.033601104548885,
0.0798456338688845));
#90986=CARTESIAN_POINT('Ctrl Pts',(0.0089962469522171,-0.0334837508592655,
0.0798339553861718));
#90987=CARTESIAN_POINT('Ctrl Pts',(0.00908026908254489,-0.0333660264659097,
0.079819780929154));
#90988=CARTESIAN_POINT('Ctrl Pts',(0.00884668829352812,-0.0336938721132538,
0.0798557455051882));
#90989=CARTESIAN_POINT('Ctrl Pts',(0.00888008591534243,-0.0336474569765032,
0.0798515140958961));
#90990=CARTESIAN_POINT('Ctrl Pts',(0.00891343171474199,-0.033601104548885,
0.0798468920152118));
#90991=CARTESIAN_POINT('Ctrl Pts',(0.00899785561212824,-0.0334837508592655,
0.0798351899696039));
#90992=CARTESIAN_POINT('Ctrl Pts',(0.009081895680887,-0.0333660264659097,
0.0798209914075528));
#90993=CARTESIAN_POINT('Ctrl Pts',(0.00911079186838175,-0.0336938721132538,
0.080069800033461));
#90994=CARTESIAN_POINT('Ctrl Pts',(0.00914544242238106,-0.0336474569765032,
0.0800640227383062));
#90995=CARTESIAN_POINT('Ctrl Pts',(0.00918002297156805,-0.033601104548885,
0.080057840210531));
#90996=CARTESIAN_POINT('Ctrl Pts',(0.00926757297152882,-0.0334837508592655,
0.080042187471659));
#90997=CARTESIAN_POINT('Ctrl Pts',(0.00935462070287566,-0.0333660264659097,
0.0800239473182964));
#90998=CARTESIAN_POINT('Ctrl Pts',(0.00912185652178284,-0.033676936124379,
0.080066404958628));
#90999=CARTESIAN_POINT('Ctrl Pts',(0.00911488450272859,-0.0336279018398637,
0.0800250760846962));
#91000=CARTESIAN_POINT('Ctrl Pts',(0.00910781218243291,-0.0335767825795119,
0.0799831526430637));
#91001=CARTESIAN_POINT('Ctrl Pts',(0.00909395450089789,-0.0334733171841433,
0.0799010068014231));
#91002=CARTESIAN_POINT('Ctrl Pts',(0.00908715982610767,-0.0334209631343313,
0.079860729192362));
#91003=CARTESIAN_POINT('Ctrl Pts',(0.00908049607793282,-0.033367986984468,
0.0798212276927121));
#91004=CARTESIAN_POINT('',(0.00897795249574407,-0.0336938721132539,0.079962134435723));
#91005=CARTESIAN_POINT('Origin',(0.00765445669747421,-0.035184046744118,
0.0732929823637694));
#91006=CARTESIAN_POINT('Origin',(0.013025539739254,-0.0352322612269297,
0.0850652437968551));
#91007=CARTESIAN_POINT('',(0.0103463288558176,-0.0351951142564682,0.0794545358812543));
#91008=CARTESIAN_POINT('',(0.010460264143557,-0.0351951372916788,0.0794038892351504));
#91009=CARTESIAN_POINT('Origin',(0.00831624652060065,-0.0352875124757075,
0.0738689662138883));
#91010=CARTESIAN_POINT('Origin',(0.000811222856913943,-0.0298325076523561,
0.0758297816026072));
#91011=CARTESIAN_POINT('Origin',(0.00839652175620651,-0.0338733578222048,
0.0825268187365329));
#91012=CARTESIAN_POINT('Origin',(0.00776557026075048,-0.0351840467441154,
0.0732409181218339));
#91013=CARTESIAN_POINT('Origin',(0.0116188984722422,-0.0352322613082597,
0.085593699579905));
#91014=CARTESIAN_POINT('',(0.00966396877698428,-0.0351951142564682,0.0796912669914274));
#91015=CARTESIAN_POINT('',(0.00978335335887432,-0.0351951372916787,0.0796552995872849));
#91016=CARTESIAN_POINT('Origin',(0.0083499774120584,-0.0352875115206849,
0.0738954205468797));
#91017=CARTESIAN_POINT('Origin',(0.00065835211145613,-0.0298325076523315,
0.074900029315683));
#91018=CARTESIAN_POINT('Origin',(0.00734423629191548,-0.0338732189113031,
0.0824952379909252));
#91019=CARTESIAN_POINT('Origin',(0.000536285841831988,-0.0262834582511432,
0.0720683456196365));
#91020=CARTESIAN_POINT('Origin',(0.00115017850853305,-0.0342770850471981,
0.0841095482703805));
#91021=CARTESIAN_POINT('Origin',(0.00812378219310841,-0.0201741814719619,
0.07415));
#91022=CARTESIAN_POINT('Origin',(0.00812378219310841,-0.0315241814719618,
0.07415));
#91023=CARTESIAN_POINT('Origin',(0.00812378219310841,-0.0355241814719619,
0.07415));
#91024=CARTESIAN_POINT('Ctrl Pts',(0.00876113795712712,-0.034193496108874,
0.0801160520975069));
#91025=CARTESIAN_POINT('Ctrl Pts',(0.00867886963199231,-0.0340836138585569,
0.08012484085603));
#91026=CARTESIAN_POINT('Ctrl Pts',(0.00859645891583077,-0.033973889665241,
0.0801319230271821));
#91027=CARTESIAN_POINT('Ctrl Pts',(0.00851401189180612,-0.0338644633307392,
0.0801372966172012));
#91028=CARTESIAN_POINT('Ctrl Pts',(0.00882682104902294,-0.034193496108874,
0.0800237109328699));
#91029=CARTESIAN_POINT('Ctrl Pts',(0.00874582605386104,-0.0340836138585569,
0.0800334054223306));
#91030=CARTESIAN_POINT('Ctrl Pts',(0.00866466931450355,-0.033973889665241,
0.0800414192387254));
#91031=CARTESIAN_POINT('Ctrl Pts',(0.00858345538911046,-0.0338644633307392,
0.0800477490883149));
#91032=CARTESIAN_POINT('Ctrl Pts',(0.00889250414091876,-0.034193496108874,
0.079931369768233));
#91033=CARTESIAN_POINT('Ctrl Pts',(0.00881278247572977,-0.0340836138585569,
0.0799419699886312));
#91034=CARTESIAN_POINT('Ctrl Pts',(0.00873287971317634,-0.033973889665241,
0.0799509154502688));
#91035=CARTESIAN_POINT('Ctrl Pts',(0.00865289888641481,-0.0338644633307392,
0.0799582015594285));
#91036=CARTESIAN_POINT('Ctrl Pts',(0.00895818723281458,-0.034193496108874,
0.079839028603596));
#91037=CARTESIAN_POINT('Ctrl Pts',(0.0088797388975985,-0.0340836138585569,
0.0798505345549318));
#91038=CARTESIAN_POINT('Ctrl Pts',(0.00880109011184912,-0.033973889665241,
0.0798604116618121));
#91039=CARTESIAN_POINT('Ctrl Pts',(0.00872234238371916,-0.0338644633307393,
0.0798686540305422));
#91040=CARTESIAN_POINT('Origin',(0.00602946434434258,-0.0345610621862962,
0.0633639504231319));
#91041=CARTESIAN_POINT('Ctrl Pts',(0.00908026834983082,-0.0340223579322365,
0.0798197804359761));
#91042=CARTESIAN_POINT('Ctrl Pts',(0.00900206729021133,-0.0339125849573555,
0.0798329728746978));
#91043=CARTESIAN_POINT('Ctrl Pts',(0.00892364812874447,-0.0338030433565222,
0.0798445374630256));
#91044=CARTESIAN_POINT('Ctrl Pts',(0.00884511246131604,-0.0336938721132328,
0.0798544683016339));
#91045=CARTESIAN_POINT('Ctrl Pts',(0.00917117691759601,-0.0340223579322365,
0.0798874325766501));
#91046=CARTESIAN_POINT('Ctrl Pts',(0.00909204275851244,-0.0339125849573555,
0.0799018788816208));
#91047=CARTESIAN_POINT('Ctrl Pts',(0.00901266520114192,-0.0338030433565222,
0.0799146771421296));
#91048=CARTESIAN_POINT('Ctrl Pts',(0.00893314720684988,-0.0336938721132328,
0.0799258199898388));
#91049=CARTESIAN_POINT('Ctrl Pts',(0.00926208548536119,-0.0340223579322365,
0.0799550847173242));
#91050=CARTESIAN_POINT('Ctrl Pts',(0.00918201822681355,-0.0339125849573555,
0.0799707848885438));
#91051=CARTESIAN_POINT('Ctrl Pts',(0.00910168227353937,-0.0338030433565222,
0.0799848168212336));
#91052=CARTESIAN_POINT('Ctrl Pts',(0.00902118195238373,-0.0336938721132328,
0.0799971716780437));
#91053=CARTESIAN_POINT('Ctrl Pts',(0.00935299405312637,-0.0340223579322365,
0.0800227368579982));
#91054=CARTESIAN_POINT('Ctrl Pts',(0.00927199369511466,-0.0339125849573555,
0.0800396908954668));
#91055=CARTESIAN_POINT('Ctrl Pts',(0.00919069934593683,-0.0338030433565222,
0.0800549565003376));
#91056=CARTESIAN_POINT('Ctrl Pts',(0.00910921669791757,-0.0336938721132328,
0.0800685233662486));
#91057=CARTESIAN_POINT('Origin',(0.00557432929956971,-0.0345589643415202,
0.0635201621466345));
#91058=CARTESIAN_POINT('Ctrl Pts',(0.0089927908359826,-0.03424362768739,
0.0798353275172685));
#91059=CARTESIAN_POINT('Ctrl Pts',(0.0087783651738213,-0.0339430054201861,
0.0798681027185399));
#91060=CARTESIAN_POINT('Ctrl Pts',(0.00856207991003499,-0.0336441434784164,
0.079884633389445));
#91061=CARTESIAN_POINT('Ctrl Pts',(0.0092390412442504,-0.03424362768739,
0.0797921912630507));
#91062=CARTESIAN_POINT('Ctrl Pts',(0.00902624249273686,-0.0339430054201861,
0.079834253951576));
#91063=CARTESIAN_POINT('Ctrl Pts',(0.00881087994612146,-0.0336441434784164,
0.0798601682705334));
#91064=CARTESIAN_POINT('Ctrl Pts',(0.00872236994997309,-0.0335235895815127,
0.0798686510179241));
#91065=CARTESIAN_POINT('Ctrl Pts',(0.00864364145972468,-0.0334144449262719,
0.079876891756908));
#91066=CARTESIAN_POINT('Ctrl Pts',(0.00856465227251364,-0.0333049234473133,
0.079883515492144));
#91067=CARTESIAN_POINT('Ctrl Pts',(0.00848550262403521,-0.0331951640388589,
0.0798885046046268));
#91068=CARTESIAN_POINT('Ctrl Pts',(0.00880885115926208,-0.0335235895815127,
0.079941877877251));
#91069=CARTESIAN_POINT('Ctrl Pts',(0.00872911455712463,-0.0334144449262719,
0.0799513092003467));
#91070=CARTESIAN_POINT('Ctrl Pts',(0.0086490915032544,-0.0333049234473133,
0.0799591040606983));
#91071=CARTESIAN_POINT('Ctrl Pts',(0.00856888341969378,-0.0331951640388589,
0.0799652432220389));
#91072=CARTESIAN_POINT('Ctrl Pts',(0.00889533236855107,-0.0335235895815127,
0.080015104736578));
#91073=CARTESIAN_POINT('Ctrl Pts',(0.00881458765452459,-0.0334144449262719,
0.0800257266437853));
#91074=CARTESIAN_POINT('Ctrl Pts',(0.00873353073399516,-0.0333049234473133,
0.0800346926292525));
#91075=CARTESIAN_POINT('Ctrl Pts',(0.00865226421535234,-0.0331951640388589,
0.080041981839451));
#91076=CARTESIAN_POINT('Ctrl Pts',(0.00898181357784006,-0.0335235895815127,
0.0800883315959049));
#91077=CARTESIAN_POINT('Ctrl Pts',(0.00890006075192454,-0.0334144449262719,
0.0801001440872239));
#91078=CARTESIAN_POINT('Ctrl Pts',(0.00881796996473591,-0.0333049234473133,
0.0801102811978068));
#91079=CARTESIAN_POINT('Ctrl Pts',(0.0087356450110109,-0.0331951640388589,
0.0801187204568631));
#91080=CARTESIAN_POINT('Origin',(0.00819772362135878,-0.0326434571771167,
0.0632239306732631));
#91081=CARTESIAN_POINT('Ctrl Pts',(0.00838399210321821,-0.0336938721132464,
0.0801458745264825));
#91082=CARTESIAN_POINT('Ctrl Pts',(0.00834889625996981,-0.0336474569764995,
0.0801473976214333));
#91083=CARTESIAN_POINT('Ctrl Pts',(0.00831378499176157,-0.033601104548885,
0.0801485097708635));
#91084=CARTESIAN_POINT('Ctrl Pts',(0.00822489133855471,-0.0334837508662659,
0.0801513254773534));
#91085=CARTESIAN_POINT('Ctrl Pts',(0.00813595328566807,-0.0333660264799515,
0.0801515058442983));
#91086=CARTESIAN_POINT('Ctrl Pts',(0.00859804663144723,-0.0336938721132464,
0.0798817709516805));
#91087=CARTESIAN_POINT('Ctrl Pts',(0.00856449667406112,-0.0336474569764995,
0.0798845469788159));
#91088=CARTESIAN_POINT('Ctrl Pts',(0.00853091651863692,-0.033601104548885,
0.0798869300711249));
#91089=CARTESIAN_POINT('Ctrl Pts',(0.0084458992907428,-0.0334837508662659,
0.0798929635125836));
#91090=CARTESIAN_POINT('Ctrl Pts',(0.0083607406127759,-0.0333660264799515,
0.0798964750680177));
#91091=CARTESIAN_POINT('Ctrl Pts',(0.00859804663144739,-0.0336938721132427,
0.0798817709516913));
#91092=CARTESIAN_POINT('Ctrl Pts',(0.0085644966740662,-0.0336474569765027,
0.0798845469788263));
#91093=CARTESIAN_POINT('Ctrl Pts',(0.00853091651864692,-0.0336011045488949,
0.0798869300711349));
#91094=CARTESIAN_POINT('Ctrl Pts',(0.00844660736846413,-0.0334847282626114,
0.0798929132622442));
#91095=CARTESIAN_POINT('Ctrl Pts',(0.00836215880828412,-0.0333679869984219,
0.079896416412814));
#91096=CARTESIAN_POINT('Ctrl Pts',(0.0085980466314447,-0.0336938721132429,
0.0798817709516807));
#91097=CARTESIAN_POINT('Ctrl Pts',(0.0084780571365088,-0.0335278710435085,
0.0798916992532303));
#91098=CARTESIAN_POINT('Ctrl Pts',(0.00835779850464323,-0.0333620469224321,
0.0798978612226623));
#91099=CARTESIAN_POINT('Ctrl Pts',(0.00823720990302569,-0.0331951640388602,
0.0799002399214836));
#91100=CARTESIAN_POINT('Ctrl Pts',(0.00868142448093768,-0.0336938721132429,
0.0798730437506859));
#91101=CARTESIAN_POINT('Ctrl Pts',(0.00856161768214375,-0.0335278710435085,
0.0798847174928915));
#91102=CARTESIAN_POINT('Ctrl Pts',(0.00844148694558292,-0.0333620469224321,
0.0798926300182409));
#91103=CARTESIAN_POINT('Ctrl Pts',(0.00832097121086305,-0.0331951640388602,
0.0798967652801135));
#91104=CARTESIAN_POINT('Ctrl Pts',(0.00876480233043065,-0.0336938721132429,
0.0798643165496912));
#91105=CARTESIAN_POINT('Ctrl Pts',(0.0086451782277787,-0.0335278710435085,
0.0798777357325528));
#91106=CARTESIAN_POINT('Ctrl Pts',(0.00852517538652261,-0.0333620469224321,
0.0798873988138196));
#91107=CARTESIAN_POINT('Ctrl Pts',(0.00840473251870041,-0.0331951640388602,
0.0798932906387434));
#91108=CARTESIAN_POINT('Ctrl Pts',(0.00884818017992363,-0.0336938721132429,
0.0798555893486965));
#91109=CARTESIAN_POINT('Ctrl Pts',(0.00872873877341365,-0.0335278710435085,
0.079870753972214));
#91110=CARTESIAN_POINT('Ctrl Pts',(0.00860886382746229,-0.0333620469224321,
0.0798821676093983));
#91111=CARTESIAN_POINT('Ctrl Pts',(0.00848849382653776,-0.0331951640388602,
0.0798898159973733));
#91112=CARTESIAN_POINT('Ctrl Pts',(0.00836211297397097,-0.0330240426238156,
0.0798949524992678));
#91113=CARTESIAN_POINT('Ctrl Pts',(0.00828297065625796,-0.0329142774063509,
0.0798982357379686));
#91114=CARTESIAN_POINT('Ctrl Pts',(0.00820372100949799,-0.0328043479726687,
0.0798998845207034));
#91115=CARTESIAN_POINT('Ctrl Pts',(0.00812446550022084,-0.0326943950436595,
0.0798998939392863));
#91116=CARTESIAN_POINT('Ctrl Pts',(0.00844382547624734,-0.0330240426238156,
0.0799734649374992));
#91117=CARTESIAN_POINT('Ctrl Pts',(0.00836360157320673,-0.0329142774063509,
0.0799778738455274));
#91118=CARTESIAN_POINT('Ctrl Pts',(0.00828324653118004,-0.0328043479726687,
0.0799806264993869));
#91119=CARTESIAN_POINT('Ctrl Pts',(0.0082028631938455,-0.0326943950436595,
0.0799817165377517));
#91120=CARTESIAN_POINT('Ctrl Pts',(0.0085255379785237,-0.0330240426238156,
0.0800519773757305));
#91121=CARTESIAN_POINT('Ctrl Pts',(0.0084442324901555,-0.0329142774063509,
0.0800575119530863));
#91122=CARTESIAN_POINT('Ctrl Pts',(0.00836277205286208,-0.0328043479726687,
0.0800613684780704));
#91123=CARTESIAN_POINT('Ctrl Pts',(0.00828126088747015,-0.0326943950436595,
0.0800635391362171));
#91124=CARTESIAN_POINT('Ctrl Pts',(0.00860725048080007,-0.0330240426238156,
0.0801304898139618));
#91125=CARTESIAN_POINT('Ctrl Pts',(0.00852486340710428,-0.0329142774063509,
0.0801371500606451));
#91126=CARTESIAN_POINT('Ctrl Pts',(0.00844229757454413,-0.0328043479726687,
0.0801421104567539));
#91127=CARTESIAN_POINT('Ctrl Pts',(0.00835965858109481,-0.0326943950436595,
0.0801453617346825));
#91128=CARTESIAN_POINT('Origin',(0.00819579695600056,-0.03263966828562,
0.0631002711133243));
#91129=CARTESIAN_POINT('Ctrl Pts',(0.00800836761556648,-0.0331951640388588,
0.0801488898535787));
#91130=CARTESIAN_POINT('Ctrl Pts',(0.00792574503386902,-0.0330855618127431,
0.0801473002510698));
#91131=CARTESIAN_POINT('Ctrl Pts',(0.007843095745071,-0.0329757224171935,
0.080144001834907));
#91132=CARTESIAN_POINT('Ctrl Pts',(0.00776052579376048,-0.0328657861694599,
0.0801389936373661));
#91133=CARTESIAN_POINT('Ctrl Pts',(0.00808510617188339,-0.0331951640388588,
0.0800655091243034));
#91134=CARTESIAN_POINT('Ctrl Pts',(0.00800363199118756,-0.0330855618127431,
0.08006497644029));
#91135=CARTESIAN_POINT('Ctrl Pts',(0.0079221100865563,-0.0329757224171935,
0.080062759440029));
#91136=CARTESIAN_POINT('Ctrl Pts',(0.007840644990966,-0.0328657861694599,
0.0800588558417936));
#91137=CARTESIAN_POINT('Ctrl Pts',(0.0081618447282003,-0.0331951640388588,
0.0799821283950282));
#91138=CARTESIAN_POINT('Ctrl Pts',(0.0080815189485061,-0.0330855618127431,
0.0799826526295103));
#91139=CARTESIAN_POINT('Ctrl Pts',(0.0080011244280416,-0.0329757224171935,
0.0799815170451511));
#91140=CARTESIAN_POINT('Ctrl Pts',(0.00792076418817151,-0.0328657861694599,
0.0799787180462211));
#91141=CARTESIAN_POINT('Ctrl Pts',(0.00823858328451721,-0.0331951640388588,
0.079898747665753));
#91142=CARTESIAN_POINT('Ctrl Pts',(0.00815940590582465,-0.0330855618127431,
0.0799003288187305));
#91143=CARTESIAN_POINT('Ctrl Pts',(0.0080801387695269,-0.0329757224171935,
0.0799002746502731));
#91144=CARTESIAN_POINT('Ctrl Pts',(0.00800088338537702,-0.0328657861694599,
0.0798985802506486));
#91145=CARTESIAN_POINT('Origin',(0.00867489634889909,-0.0326401908832791,
0.0631419441633169));
#91146=CARTESIAN_POINT('Ctrl Pts',(0.00827330551698484,-0.0332451089994433,
0.0798994145593807));
#91147=CARTESIAN_POINT('Ctrl Pts',(0.00805646279914546,-0.0329451141710259,
0.0799050539238054));
#91148=CARTESIAN_POINT('Ctrl Pts',(0.00783981132859943,-0.0326442513127504,
0.0798943437874235));
#91149=CARTESIAN_POINT('Ctrl Pts',(0.00852302072379411,-0.0332451089994433,
0.0798874849538466));
#91150=CARTESIAN_POINT('Ctrl Pts',(0.00830662793838874,-0.0329451141710259,
0.0799025424813854));
#91151=CARTESIAN_POINT('Ctrl Pts',(0.00808971570751864,-0.0326442513127504,
0.0799012576428604));
#91152=CARTESIAN_POINT('Ctrl Pts',(0.00800091499146258,-0.0325229783203385,
0.0798985810160486));
#91153=CARTESIAN_POINT('Ctrl Pts',(0.00792167092931193,-0.032413025311208,
0.0798968872943917));
#91154=CARTESIAN_POINT('Ctrl Pts',(0.00784247392288333,-0.0323031222247695,
0.0798935545644289));
#91155=CARTESIAN_POINT('Ctrl Pts',(0.00776342526726939,-0.0321934096636185,
0.0798885906748361));
#91156=CARTESIAN_POINT('Ctrl Pts',(0.00807753644924918,-0.0325229783203385,
0.0799820693077831));
#91157=CARTESIAN_POINT('Ctrl Pts',(0.00799714150284369,-0.032413025311208,
0.0799814318112269));
#91158=CARTESIAN_POINT('Ctrl Pts',(0.00791677193734176,-0.0323031222247695,
0.0799791313386489));
#91159=CARTESIAN_POINT('Ctrl Pts',(0.00783653059645855,-0.0321934096636185,
0.0799751744694758));
#91160=CARTESIAN_POINT('Ctrl Pts',(0.00815415790703578,-0.0325229783203385,
0.0800655575995175));
#91161=CARTESIAN_POINT('Ctrl Pts',(0.00807261207637545,-0.032413025311208,
0.0800659763280621));
#91162=CARTESIAN_POINT('Ctrl Pts',(0.0079910699518002,-0.0323031222247695,
0.0800647081128688));
#91163=CARTESIAN_POINT('Ctrl Pts',(0.00790963592564772,-0.0321934096636185,
0.0800617582641156));
#91164=CARTESIAN_POINT('Ctrl Pts',(0.00823077936482238,-0.0325229783203385,
0.080149045891252));
#91165=CARTESIAN_POINT('Ctrl Pts',(0.00814808264990721,-0.032413025311208,
0.0801505208448973));
#91166=CARTESIAN_POINT('Ctrl Pts',(0.00806536796625863,-0.0323031222247695,
0.0801502848870888));
#91167=CARTESIAN_POINT('Ctrl Pts',(0.00798274125483688,-0.0321934096636185,
0.0801483420587554));
#91168=CARTESIAN_POINT('Origin',(0.00819550299769431,-0.0326393375178307,
0.063108791946804));
#91169=CARTESIAN_POINT('Ctrl Pts',(0.00763192194936668,-0.0326943950436594,
0.080129805473483));
#91170=CARTESIAN_POINT('Ctrl Pts',(0.00754950902259242,-0.0325844576448127,
0.0801230267174799));
#91171=CARTESIAN_POINT('Ctrl Pts',(0.00746723045911536,-0.0324744968375319,
0.0801145430472902));
#91172=CARTESIAN_POINT('Ctrl Pts',(0.00738519152910246,-0.0323646534831895,
0.0801043667867468));
#91173=CARTESIAN_POINT('Ctrl Pts',(0.00771374452105953,-0.0326943950436594,
0.0800514078055102));
#91174=CARTESIAN_POINT('Ctrl Pts',(0.00763241206108282,-0.0325844576448127,
0.0800457567178969));
#91175=CARTESIAN_POINT('Ctrl Pts',(0.00755119071883849,-0.0324744968375319,
0.0800384231417286));
#91176=CARTESIAN_POINT('Ctrl Pts',(0.00747018443024492,-0.0323646534831895,
0.0800294179085872));
#91177=CARTESIAN_POINT('Ctrl Pts',(0.00779556709275238,-0.0326943950436594,
0.0799730101375374));
#91178=CARTESIAN_POINT('Ctrl Pts',(0.00771531509957322,-0.0325844576448127,
0.0799684867183139));
#91179=CARTESIAN_POINT('Ctrl Pts',(0.00763515097856162,-0.0324744968375319,
0.079962303236167));
#91180=CARTESIAN_POINT('Ctrl Pts',(0.00755517733138738,-0.0323646534831895,
0.0799544690304276));
#91181=CARTESIAN_POINT('Ctrl Pts',(0.00787738966444523,-0.0326943950436594,
0.0798946124695647));
#91182=CARTESIAN_POINT('Ctrl Pts',(0.00779821813806362,-0.0325844576448127,
0.0798912167187309));
#91183=CARTESIAN_POINT('Ctrl Pts',(0.00771911123828475,-0.0324744968375319,
0.0798861833306055));
#91184=CARTESIAN_POINT('Ctrl Pts',(0.00764017023252984,-0.0323646534831895,
0.0798795201522679));
#91185=CARTESIAN_POINT('Origin',(0.00867633101255401,-0.0326395579067508,
0.063104130100388));
#91186=CARTESIAN_POINT('Ctrl Pts',(0.00791204093642377,-0.0327445246961877,
0.0798974594944391));
#91187=CARTESIAN_POINT('Ctrl Pts',(0.00769527196015635,-0.0324436878365475,
0.0798894735424739));
#91188=CARTESIAN_POINT('Ctrl Pts',(0.00747972033617851,-0.0321434074463188,
0.0798651823526856));
#91189=CARTESIAN_POINT('Ctrl Pts',(0.00816201247917376,-0.0327445246961877,
0.0799012314720613));
#91190=CARTESIAN_POINT('Ctrl Pts',(0.00794510124044614,-0.0324436878365475,
0.0799026733508568));
#91191=CARTESIAN_POINT('Ctrl Pts',(0.00772869761542315,-0.0321434074463188,
0.0798877724925685));
#91192=CARTESIAN_POINT('Ctrl Pts',(0.00725741743083938,-0.0321934096636185,
0.0800871215330967));
#91193=CARTESIAN_POINT('Ctrl Pts',(0.00717553989778692,-0.0320835708272305,
0.0800751736878214));
#91194=CARTESIAN_POINT('Ctrl Pts',(0.00709395711706809,-0.0319739230346347,
0.080061538321491));
#91195=CARTESIAN_POINT('Ctrl Pts',(0.00701277212929694,-0.0318646057455576,
0.0800462408904464));
#91196=CARTESIAN_POINT('Ctrl Pts',(0.00734400130003629,-0.0321934096636185,
0.0800140161409567));
#91197=CARTESIAN_POINT('Ctrl Pts',(0.00726313194731632,-0.0320835708272305,
0.080003262354717));
#91198=CARTESIAN_POINT('Ctrl Pts',(0.00718253205115473,-0.0319739230346347,
0.079990841219059));
#91199=CARTESIAN_POINT('Ctrl Pts',(0.0071023035138616,-0.0318646057455576,
0.0799767765402876));
#91200=CARTESIAN_POINT('Ctrl Pts',(0.00743058516923321,-0.0321934096636185,
0.0799409107488167));
#91201=CARTESIAN_POINT('Ctrl Pts',(0.00735072399684572,-0.0320835708272305,
0.0799313510216126));
#91202=CARTESIAN_POINT('Ctrl Pts',(0.00727110698524138,-0.0319739230346347,
0.0799201441166271));
#91203=CARTESIAN_POINT('Ctrl Pts',(0.00719183489842626,-0.0318646057455576,
0.0799073121901288));
#91204=CARTESIAN_POINT('Ctrl Pts',(0.00751716903843012,-0.0321934096636185,
0.0798678053566767));
#91205=CARTESIAN_POINT('Ctrl Pts',(0.00743831604637512,-0.0320835708272305,
0.0798594396885082));
#91206=CARTESIAN_POINT('Ctrl Pts',(0.00735968191932802,-0.0319739230346347,
0.0798494470141951));
#91207=CARTESIAN_POINT('Ctrl Pts',(0.00728136628299092,-0.0318646057455576,
0.07983784783997));
#91208=CARTESIAN_POINT('Origin',(0.0086698683816937,-0.0326371942644933,
0.0631992123700286));
#91209=CARTESIAN_POINT('Ctrl Pts',(0.00764056873150404,-0.0320218834582349,
0.0798803841538758));
#91210=CARTESIAN_POINT('Ctrl Pts',(0.00758092928557567,-0.0319391099350626,
0.0798753550699015));
#91211=CARTESIAN_POINT('Ctrl Pts',(0.00752140450352376,-0.0318564869454889,
0.0798693977546107));
#91212=CARTESIAN_POINT('Ctrl Pts',(0.00746203733617003,-0.0317740741446463,
0.0798625205946922));
#91213=CARTESIAN_POINT('Ctrl Pts',(0.0076717219673248,-0.0320218834582349,
0.0799189367665705));
#91214=CARTESIAN_POINT('Ctrl Pts',(0.00761168128189862,-0.0319391099350626,
0.0799142319124686));
#91215=CARTESIAN_POINT('Ctrl Pts',(0.00755175044055479,-0.0318564869454889,
0.0799085923651966));
#91216=CARTESIAN_POINT('Ctrl Pts',(0.007491972711483,-0.0317740741446463,
0.0799020263076026));
#91217=CARTESIAN_POINT('Ctrl Pts',(0.00770287520314557,-0.0320218834582349,
0.0799574893792652));
#91218=CARTESIAN_POINT('Ctrl Pts',(0.00764243327822157,-0.0319391099350626,
0.0799531087550357));
#91219=CARTESIAN_POINT('Ctrl Pts',(0.00758209637758582,-0.0318564869454889,
0.0799477869757825));
#91220=CARTESIAN_POINT('Ctrl Pts',(0.00752190808679598,-0.0317740741446463,
0.0799415320205131));
#91221=CARTESIAN_POINT('Ctrl Pts',(0.00773402843896634,-0.0320218834582349,
0.0799960419919599));
#91222=CARTESIAN_POINT('Ctrl Pts',(0.00767318527454453,-0.0319391099350626,
0.0799919855976028));
#91223=CARTESIAN_POINT('Ctrl Pts',(0.00761244231461685,-0.0318564869454889,
0.0799869815863684));
#91224=CARTESIAN_POINT('Ctrl Pts',(0.00755184346210895,-0.0317740741446463,
0.0799810377334236));
#91225=CARTESIAN_POINT('Origin',(0.00819179220557225,-0.0326352985526525,
0.0632314705245195));
#91226=CARTESIAN_POINT('Ctrl Pts',(0.00754600788596507,-0.0322357242816073,
0.0798722636997962));
#91227=CARTESIAN_POINT('Ctrl Pts',(0.00736376120863064,-0.0319819883628706,
0.0798538623374596));
#91228=CARTESIAN_POINT('Ctrl Pts',(0.0071830548081292,-0.0317295851069886,
0.0798239013903267));
#91229=CARTESIAN_POINT('Ctrl Pts',(0.00779523028038902,-0.0322357242816073,
0.0798919664437063));
#91230=CARTESIAN_POINT('Ctrl Pts',(0.00761235609621458,-0.0319819883628706,
0.0798815024914024));
#91231=CARTESIAN_POINT('Ctrl Pts',(0.00743051838048631,-0.0317295851069886,
0.0798594229381006));
#91232=CARTESIAN_POINT('Origin',(0.00653733631511826,-0.0391228853390952,
0.0861234626489958));
#91233=CARTESIAN_POINT('Ctrl Pts',(0.00995668358200857,-0.0352722978779648,
0.0796020305429413));
#91234=CARTESIAN_POINT('Ctrl Pts',(0.00993866330670262,-0.0352466642097253,
0.0796077193350789));
#91235=CARTESIAN_POINT('Ctrl Pts',(0.00992068268751648,-0.0352210183808319,
0.0796134778231547));
#91236=CARTESIAN_POINT('Ctrl Pts',(0.00990274125235295,-0.0351953608940152,
0.0796193067175269));
#91237=CARTESIAN_POINT('Origin',(0.0112580326694923,-0.0352456003065096,
0.0843260366550522));
#91238=CARTESIAN_POINT('Ctrl Pts',(0.00978333676035485,-0.0350241211493338,
0.0796551938002844));
#91239=CARTESIAN_POINT('Ctrl Pts',(0.00970750497639259,-0.0349144232867421,
0.0796780534829736));
#91240=CARTESIAN_POINT('Ctrl Pts',(0.00963115527749999,-0.0348045283677512,
0.0796993593511939));
#91241=CARTESIAN_POINT('Ctrl Pts',(0.00955438444240266,-0.0346945769586886,
0.0797190804756865));
#91242=CARTESIAN_POINT('Ctrl Pts',(0.00988200738449934,-0.0350241211493338,
0.0797109185679786));
#91243=CARTESIAN_POINT('Ctrl Pts',(0.00980540801474475,-0.0349144232867421,
0.0797351373979976));
#91244=CARTESIAN_POINT('Ctrl Pts',(0.0097282621760775,-0.0348045283677512,
0.0797577873605168));
#91245=CARTESIAN_POINT('Ctrl Pts',(0.00965066760291177,-0.0346945769586886,
0.079778835766716));
#91246=CARTESIAN_POINT('Ctrl Pts',(0.00998067800864383,-0.0350241211493338,
0.0797666433356729));
#91247=CARTESIAN_POINT('Ctrl Pts',(0.00990331105309691,-0.0349144232867421,
0.0797922213130217));
#91248=CARTESIAN_POINT('Ctrl Pts',(0.00982536907465503,-0.0348045283677512,
0.0798162153698396));
#91249=CARTESIAN_POINT('Ctrl Pts',(0.00974695076342089,-0.0346945769586886,
0.0798385910577455));
#91250=CARTESIAN_POINT('Ctrl Pts',(0.0100793486327883,-0.0350241211493338,
0.0798223681033672));
#91251=CARTESIAN_POINT('Ctrl Pts',(0.0100012140914491,-0.0349144232867421,
0.0798493052280457));
#91252=CARTESIAN_POINT('Ctrl Pts',(0.00992247597323254,-0.0348045283677512,
0.0798746433791625));
#91253=CARTESIAN_POINT('Ctrl Pts',(0.00984323392393,-0.0346945769586886,
0.079898346348775));
#91254=CARTESIAN_POINT('Origin',(0.00555190943416128,-0.0345629067942252,
0.0634143835178251));
#91255=CARTESIAN_POINT('Ctrl Pts',(0.00954912843121769,-0.0351970973651596,
0.0799070747675207));
#91256=CARTESIAN_POINT('Ctrl Pts',(0.00946937196253186,-0.0350869349321763,
0.0799268210079634));
#91257=CARTESIAN_POINT('Ctrl Pts',(0.00938913891111949,-0.0349764985129723,
0.0799449255131765));
#91258=CARTESIAN_POINT('Ctrl Pts',(0.00930853184056139,-0.0348659306849652,
0.0799613587094737));
#91259=CARTESIAN_POINT('Ctrl Pts',(0.00958799576292898,-0.0351970973651596,
0.0798346192558197));
#91260=CARTESIAN_POINT('Ctrl Pts',(0.00950924306716316,-0.0350869349321763,
0.0798549039504687));
#91261=CARTESIAN_POINT('Ctrl Pts',(0.00943000342602006,-0.0349764985129723,
0.0798735682238201));
#91262=CARTESIAN_POINT('Ctrl Pts',(0.009350378073399,-0.0348659306849652,
0.0798905818527512));
#91263=CARTESIAN_POINT('Ctrl Pts',(0.00962686309464028,-0.0351970973651596,
0.0797621637441187));
#91264=CARTESIAN_POINT('Ctrl Pts',(0.00954911417179447,-0.0350869349321763,
0.079782986892974));
#91265=CARTESIAN_POINT('Ctrl Pts',(0.00947086794092062,-0.0349764985129723,
0.0798022109344636));
#91266=CARTESIAN_POINT('Ctrl Pts',(0.00939222430623661,-0.0348659306849652,
0.0798198049960288));
#91267=CARTESIAN_POINT('Ctrl Pts',(0.00966573042635158,-0.0351970973651596,
0.0796897082324177));
#91268=CARTESIAN_POINT('Ctrl Pts',(0.00958898527642577,-0.0350869349321763,
0.0797110698354793));
#91269=CARTESIAN_POINT('Ctrl Pts',(0.00951173245582118,-0.0349764985129723,
0.0797308536451072));
#91270=CARTESIAN_POINT('Ctrl Pts',(0.00943407053907422,-0.0348659306849652,
0.0797490281393064));
#91271=CARTESIAN_POINT('Origin',(0.00602813602901201,-0.0345637187965951,
0.0633470516033824));
#91272=CARTESIAN_POINT('Ctrl Pts',(0.00969842342285979,-0.0352450361861252,
0.0796816028416335));
#91273=CARTESIAN_POINT('Ctrl Pts',(0.00948979560363212,-0.0349452761023764,
0.0797409914086066));
#91274=CARTESIAN_POINT('Ctrl Pts',(0.00927728708429922,-0.0346444289983475,
0.0797844965583448));
#91275=CARTESIAN_POINT('Ctrl Pts',(0.00993732667225551,-0.0352450361861252,
0.0796079466305705));
#91276=CARTESIAN_POINT('Ctrl Pts',(0.00973147684254131,-0.0349452761023764,
0.0796763455812163));
#91277=CARTESIAN_POINT('Ctrl Pts',(0.00952105972179818,-0.0346444289983475,
0.0797290447666083));
#91278=CARTESIAN_POINT('Ctrl Pts',(0.00931268830210933,-0.0346945769586885,
0.07977713313011));
#91279=CARTESIAN_POINT('Ctrl Pts',(0.00919482574571989,-0.034527515336289,
0.0798020352445747));
#91280=CARTESIAN_POINT('Ctrl Pts',(0.00907614955545729,-0.0343603235965158,
0.0798232371310882));
#91281=CARTESIAN_POINT('Ctrl Pts',(0.00895701165478281,-0.034193496108874,
0.0798406813005298));
#91282=CARTESIAN_POINT('Ctrl Pts',(0.00939431487537028,-0.0346945769586885,
0.0797580247322456));
#91283=CARTESIAN_POINT('Ctrl Pts',(0.00927685255202469,-0.034527515336289,
0.0797846365479687));
#91284=CARTESIAN_POINT('Ctrl Pts',(0.0091585229297958,-0.0343603235965158,
0.0798075611649178));
#91285=CARTESIAN_POINT('Ctrl Pts',(0.00903967698287652,-0.034193496108874,
0.0798267359836661));
#91286=CARTESIAN_POINT('Ctrl Pts',(0.00947594144863123,-0.0346945769586885,
0.0797389163343812));
#91287=CARTESIAN_POINT('Ctrl Pts',(0.00935887935832949,-0.034527515336289,
0.0797672378513627));
#91288=CARTESIAN_POINT('Ctrl Pts',(0.00924089630413431,-0.0343603235965158,
0.0797918851987474));
#91289=CARTESIAN_POINT('Ctrl Pts',(0.00912234231097024,-0.034193496108874,
0.0798127906668024));
#91290=CARTESIAN_POINT('Ctrl Pts',(0.00955756802189218,-0.0346945769586885,
0.0797198079365168));
#91291=CARTESIAN_POINT('Ctrl Pts',(0.00944090616463429,-0.034527515336289,
0.0797498391547567));
#91292=CARTESIAN_POINT('Ctrl Pts',(0.00932326967847282,-0.0343603235965158,
0.079776209232577));
#91293=CARTESIAN_POINT('Ctrl Pts',(0.00920500763906395,-0.034193496108874,
0.0797988453499388));
#91294=CARTESIAN_POINT('Origin',(0.00601624531389674,-0.0345626446731352,
0.0632898437234962));
#91295=CARTESIAN_POINT('Origin',(0.00554884660254213,-0.0345625596230794,
0.0634026738054348));
#91296=CARTESIAN_POINT('Ctrl Pts',(0.00913449179185841,-0.0346945769586886,
0.0800642595569595));
#91297=CARTESIAN_POINT('Ctrl Pts',(0.00905299030585987,-0.034584662917669,
0.0800781876460834));
#91298=CARTESIAN_POINT('Ctrl Pts',(0.0089711868720442,-0.0344746925051587,
0.0800904326969005));
#91299=CARTESIAN_POINT('Ctrl Pts',(0.0088891863711939,-0.0343648066255171,
0.0801009794525156));
#91300=CARTESIAN_POINT('Ctrl Pts',(0.00919424703583845,-0.0346945769586886,
0.0799679764722608));
#91301=CARTESIAN_POINT('Ctrl Pts',(0.00911407237941238,-0.034584662917669,
0.0799827280188495));
#91302=CARTESIAN_POINT('Ctrl Pts',(0.00903357897303276,-0.0344746925051587,
0.0799958241060704));
#91303=CARTESIAN_POINT('Ctrl Pts',(0.00895287002342734,-0.0343648066255171,
0.0800072483796505));
#91304=CARTESIAN_POINT('Ctrl Pts',(0.00925400227981849,-0.0346945769586886,
0.0798716933875621));
#91305=CARTESIAN_POINT('Ctrl Pts',(0.0091751544529649,-0.034584662917669,
0.0798872683916155));
#91306=CARTESIAN_POINT('Ctrl Pts',(0.00909597107402132,-0.0344746925051587,
0.0799012155152404));
#91307=CARTESIAN_POINT('Ctrl Pts',(0.00901655367566078,-0.0343648066255171,
0.0799135173067855));
#91308=CARTESIAN_POINT('Ctrl Pts',(0.00931375752379853,-0.0346945769586886,
0.0797754103028634));
#91309=CARTESIAN_POINT('Ctrl Pts',(0.00923623652651741,-0.034584662917669,
0.0797918087643815));
#91310=CARTESIAN_POINT('Ctrl Pts',(0.00915836317500988,-0.0344746925051587,
0.0798066069244103));
#91311=CARTESIAN_POINT('Ctrl Pts',(0.00908023732789422,-0.0343648066255171,
0.0798197862339205));
#91312=CARTESIAN_POINT('Ctrl Pts',(0.0094343889890219,-0.0345231616327822,
0.0797485346823557));
#91313=CARTESIAN_POINT('Ctrl Pts',(0.00935722107053248,-0.0344132092796975,
0.0797665995518505));
#91314=CARTESIAN_POINT('Ctrl Pts',(0.00927968347597679,-0.0343032738558974,
0.0797830673317564));
#91315=CARTESIAN_POINT('Ctrl Pts',(0.00920187608038533,-0.0341934961088741,
0.0797979194694375));
#91316=CARTESIAN_POINT('Ctrl Pts',(0.00952936591106417,-0.0345231616327822,
0.0798103450408606));
#91317=CARTESIAN_POINT('Ctrl Pts',(0.00945134602380479,-0.0344132092796975,
0.079829719033509));
#91318=CARTESIAN_POINT('Ctrl Pts',(0.009372929426257,-0.0343032738558974,
0.0798474782467216));
#91319=CARTESIAN_POINT('Ctrl Pts',(0.00929421716193573,-0.0341934961088741,
0.0798636025022331));
#91320=CARTESIAN_POINT('Ctrl Pts',(0.00962434283310644,-0.0345231616327822,
0.0798721553993656));
#91321=CARTESIAN_POINT('Ctrl Pts',(0.0095454709770771,-0.0344132092796975,
0.0798928385151674));
#91322=CARTESIAN_POINT('Ctrl Pts',(0.00946617537653722,-0.0343032738558974,
0.0799118891616869));
#91323=CARTESIAN_POINT('Ctrl Pts',(0.00938655824348613,-0.0341934961088741,
0.0799292855350287));
#91324=CARTESIAN_POINT('Ctrl Pts',(0.00971931975514871,-0.0345231616327822,
0.0799339657578705));
#91325=CARTESIAN_POINT('Ctrl Pts',(0.00963959593034941,-0.0344132092796975,
0.0799559579968259));
#91326=CARTESIAN_POINT('Ctrl Pts',(0.00955942132681743,-0.0343032738558974,
0.0799763000766521));
#91327=CARTESIAN_POINT('Ctrl Pts',(0.00947889932503654,-0.0341934961088741,
0.0799949685678243));
#91328=CARTESIAN_POINT('Origin',(0.00805051870546373,-0.0391228853391069,
0.0862278827114944));
#91329=CARTESIAN_POINT('Ctrl Pts',(0.0106255512245337,-0.0352722978779642,
0.0793293161957926));
#91330=CARTESIAN_POINT('Ctrl Pts',(0.0106083860391948,-0.0352466642097249,
0.0793372186694786));
#91331=CARTESIAN_POINT('Ctrl Pts',(0.0105912689324926,-0.0352210183808317,
0.0793451853193));
#91332=CARTESIAN_POINT('Ctrl Pts',(0.0105741995250841,-0.0351953608940152,
0.0793532169091828));
#91333=CARTESIAN_POINT('Origin',(0.0125087137471874,-0.0352456003065102,
0.0838529698196086));
#91334=CARTESIAN_POINT('Ctrl Pts',(0.010460234417295,-0.0350241211493339,
0.079403786362658));
#91335=CARTESIAN_POINT('Ctrl Pts',(0.0103878656675488,-0.0349144232867421,
0.0794359700326123));
#91336=CARTESIAN_POINT('Ctrl Pts',(0.0103147883421944,-0.0348045283677512,
0.0794666770523418));
#91337=CARTESIAN_POINT('Ctrl Pts',(0.0102410945803643,-0.0346945769586886,
0.0794958646068836));
#91338=CARTESIAN_POINT('Ctrl Pts',(0.0105651111594214,-0.0350241211493339,
0.079446705015533));
#91339=CARTESIAN_POINT('Ctrl Pts',(0.0104921512228558,-0.0349144232867421,
0.0794803333195438));
#91340=CARTESIAN_POINT('Ctrl Pts',(0.0104184524952114,-0.0348045283677512,
0.0795124736177594));
#91341=CARTESIAN_POINT('Ctrl Pts',(0.0103441078432417,-0.0346945769586886,
0.0795430812297508));
#91342=CARTESIAN_POINT('Ctrl Pts',(0.0106699879015477,-0.0350241211493339,
0.079489623668408));
#91343=CARTESIAN_POINT('Ctrl Pts',(0.0105964367781628,-0.0349144232867421,
0.0795246966064752));
#91344=CARTESIAN_POINT('Ctrl Pts',(0.0105221166482283,-0.0348045283677512,
0.079558270183177));
#91345=CARTESIAN_POINT('Ctrl Pts',(0.0104471211061191,-0.0346945769586886,
0.0795902978526181));
#91346=CARTESIAN_POINT('Ctrl Pts',(0.0107748646436741,-0.0350241211493339,
0.079532542321283));
#91347=CARTESIAN_POINT('Ctrl Pts',(0.0107007223334698,-0.0349144232867421,
0.0795690598934067));
#91348=CARTESIAN_POINT('Ctrl Pts',(0.0106257808012453,-0.0348045283677512,
0.0796040667485947));
#91349=CARTESIAN_POINT('Ctrl Pts',(0.0105501343689965,-0.0346945769586886,
0.0796375144754854));
#91350=CARTESIAN_POINT('Origin',(0.00422665989078905,-0.0345629067942693,
0.0638213781891361));
#91351=CARTESIAN_POINT('Ctrl Pts',(0.0102594419468846,-0.0351970973651597,
0.0796830352604534));
#91352=CARTESIAN_POINT('Ctrl Pts',(0.0101827892419419,-0.0350869349321763,
0.0797126219320104));
#91353=CARTESIAN_POINT('Ctrl Pts',(0.0101054579482848,-0.0349764985129723,
0.0797406395455647));
#91354=CARTESIAN_POINT('Ctrl Pts',(0.0100275461141839,-0.0348659306849652,
0.0797670459060018));
#91355=CARTESIAN_POINT('Ctrl Pts',(0.0102889217145051,-0.0351970973651597,
0.0796062797137405));
#91356=CARTESIAN_POINT('Ctrl Pts',(0.0102133323536399,-0.0350869349321763,
0.0796362747875257));
#91357=CARTESIAN_POINT('Ctrl Pts',(0.0101370567944662,-0.0349764985129723,
0.079664723247958));
#91358=CARTESIAN_POINT('Ctrl Pts',(0.010060191684662,-0.0348659306849652,
0.0796915824222609));
#91359=CARTESIAN_POINT('Ctrl Pts',(0.0103184014821256,-0.0351970973651597,
0.0795295241670276));
#91360=CARTESIAN_POINT('Ctrl Pts',(0.0102438754653379,-0.0350869349321763,
0.079559927643041));
#91361=CARTESIAN_POINT('Ctrl Pts',(0.0101686556406475,-0.0349764985129723,
0.0795888069503512));
#91362=CARTESIAN_POINT('Ctrl Pts',(0.0100928372551402,-0.0348659306849652,
0.07961611893852));
#91363=CARTESIAN_POINT('Ctrl Pts',(0.0103478812497461,-0.0351970973651597,
0.0794527686203147));
#91364=CARTESIAN_POINT('Ctrl Pts',(0.0102744185770359,-0.0350869349321763,
0.0794835804985563));
#91365=CARTESIAN_POINT('Ctrl Pts',(0.0102002544868289,-0.0349764985129723,
0.0795128906527445));
#91366=CARTESIAN_POINT('Ctrl Pts',(0.0101254828256183,-0.0348659306849652,
0.0795406554547791));
#91367=CARTESIAN_POINT('Origin',(0.00469069237055749,-0.0345637187965033,
0.0636948901884269));
#91368=CARTESIAN_POINT('Ctrl Pts',(0.0103793005773761,-0.0352450361861253,
0.0794406296239892));
#91369=CARTESIAN_POINT('Ctrl Pts',(0.0101797612119527,-0.0349452761023765,
0.0795256978935684));
#91370=CARTESIAN_POINT('Ctrl Pts',(0.0099743810268613,-0.0346444289983475,
0.0795954943720945));
#91371=CARTESIAN_POINT('Ctrl Pts',(0.0106070884321888,-0.0352450361861253,
0.0793376116973946));
#91372=CARTESIAN_POINT('Ctrl Pts',(0.0104114344515231,-0.0349452761023765,
0.0794312711266716));
#91373=CARTESIAN_POINT('Ctrl Pts',(0.010209281491937,-0.0346444289983475,
0.0795099270213863));
#91374=CARTESIAN_POINT('Ctrl Pts',(0.009133422612805,-0.0336938721132462,
0.0800659823155221));
#91375=CARTESIAN_POINT('Ctrl Pts',(0.0090987944051785,-0.0336474569764994,
0.0800718920759333));
#91376=CARTESIAN_POINT('Ctrl Pts',(0.00906409938909167,-0.033601104548885,
0.0800773960645121));
#91377=CARTESIAN_POINT('Ctrl Pts',(0.00897625959288491,-0.0334837508694645,
0.0800913308969353));
#91378=CARTESIAN_POINT('Ctrl Pts',(0.00888804545149575,-0.0333660264863675,
0.0801026567351507));
#91379=CARTESIAN_POINT('Ctrl Pts',(0.00931268830211894,-0.0336938721132462,
0.0797771331301079));
#91380=CARTESIAN_POINT('Ctrl Pts',(0.00927975082462513,-0.0336474569764994,
0.0797840921920854));
#91381=CARTESIAN_POINT('Ctrl Pts',(0.00924673413942139,-0.033601104548885,
0.0797906652024626));
#91382=CARTESIAN_POINT('Ctrl Pts',(0.00916314349076854,-0.0334837508694645,
0.0798073065520604));
#91383=CARTESIAN_POINT('Ctrl Pts',(0.00907909643131272,-0.0333660264863675,
0.0798214636299887));
#91384=CARTESIAN_POINT('Ctrl Pts',(0.00931268830211937,-0.0336938721132426,
0.07977713313012));
#91385=CARTESIAN_POINT('Ctrl Pts',(0.00927975082463032,-0.0336474569765026,
0.0797840921920964));
#91386=CARTESIAN_POINT('Ctrl Pts',(0.00924673413943139,-0.0336011045488949,
0.0797906652024726));
#91387=CARTESIAN_POINT('Ctrl Pts',(0.00916383968703325,-0.033484728265791,
0.0798071679522935));
#91388=CARTESIAN_POINT('Ctrl Pts',(0.00908049609245075,-0.0333679870047996,
0.0798212276902747));
#91389=CARTESIAN_POINT('Ctrl Pts',(0.00943438693042286,-0.0335235895815127,
0.0797485348074296));
#91390=CARTESIAN_POINT('Ctrl Pts',(0.00935731207629897,-0.0334144449262719,
0.0797665778619818));
#91391=CARTESIAN_POINT('Ctrl Pts',(0.00927977591657743,-0.0333049234473133,
0.0797830493373368));
#91392=CARTESIAN_POINT('Ctrl Pts',(0.00920187568831821,-0.0331951640388588,
0.0797979191905567));
#91393=CARTESIAN_POINT('Ctrl Pts',(0.0095293639686092,-0.0335235895815127,
0.0798103452814962));
#91394=CARTESIAN_POINT('Ctrl Pts',(0.00945143817161617,-0.0334144449262719,
0.0798296958819716));
#91395=CARTESIAN_POINT('Ctrl Pts',(0.00937302307848049,-0.0333049234473133,
0.0798474588256224));
#91396=CARTESIAN_POINT('Ctrl Pts',(0.00929421690055794,-0.0331951640388588,
0.0798636023163128));
#91397=CARTESIAN_POINT('Ctrl Pts',(0.00962434100679553,-0.0335235895815127,
0.0798721557555629));
#91398=CARTESIAN_POINT('Ctrl Pts',(0.00954556426693336,-0.0334144449262719,
0.0798928139019615));
#91399=CARTESIAN_POINT('Ctrl Pts',(0.00946627024038355,-0.0333049234473133,
0.079911868313908));
#91400=CARTESIAN_POINT('Ctrl Pts',(0.00938655811279768,-0.0331951640388588,
0.0799292854420688));
#91401=CARTESIAN_POINT('Ctrl Pts',(0.00971931804498187,-0.0335235895815127,
0.0799339662296295));
#91402=CARTESIAN_POINT('Ctrl Pts',(0.00963969036225056,-0.0334144449262719,
0.0799559319219513));
#91403=CARTESIAN_POINT('Ctrl Pts',(0.00955951740228661,-0.0333049234473133,
0.0799762778021936));
#91404=CARTESIAN_POINT('Ctrl Pts',(0.00947889932503741,-0.0331951640388588,
0.0799949685678249));
#91405=CARTESIAN_POINT('Origin',(0.00682774097248567,-0.0326434571769517,
0.0633008186751137));
#91406=CARTESIAN_POINT('Ctrl Pts',(0.00931268830211658,-0.0336938721132428,
0.0797771331301084));
#91407=CARTESIAN_POINT('Ctrl Pts',(0.00919488930632441,-0.0335278710435084,
0.079802021815429));
#91408=CARTESIAN_POINT('Ctrl Pts',(0.00907635124924464,-0.0333620469224321,
0.0798232075990872));
#91409=CARTESIAN_POINT('Ctrl Pts',(0.00895701165478389,-0.0331951640388602,
0.0798406813005296));
#91410=CARTESIAN_POINT('Ctrl Pts',(0.00939431488404191,-0.0336938721132428,
0.0797580247302156));
#91411=CARTESIAN_POINT('Ctrl Pts',(0.00927691590549946,-0.0335278710435084,
0.079784622194973));
#91412=CARTESIAN_POINT('Ctrl Pts',(0.00915872413806543,-0.0333620469224321,
0.0798075287013603));
#91413=CARTESIAN_POINT('Ctrl Pts',(0.00903967699165226,-0.0331951640388602,
0.0798267359821857));
#91414=CARTESIAN_POINT('Ctrl Pts',(0.00947594146596724,-0.0336938721132428,
0.0797389163303228));
#91415=CARTESIAN_POINT('Ctrl Pts',(0.00935894250467452,-0.0335278710435084,
0.079767222574517));
#91416=CARTESIAN_POINT('Ctrl Pts',(0.00924109702688621,-0.0333620469224321,
0.0797918498036334));
#91417=CARTESIAN_POINT('Ctrl Pts',(0.00912234232852063,-0.0331951640388602,
0.0798127906638418));
#91418=CARTESIAN_POINT('Ctrl Pts',(0.00955756804789257,-0.0336938721132428,
0.0797198079304301));
#91419=CARTESIAN_POINT('Ctrl Pts',(0.00944096910384957,-0.0335278710435084,
0.079749822954061));
#91420=CARTESIAN_POINT('Ctrl Pts',(0.009323469915707,-0.0333620469224321,
0.0797761709059064));
#91421=CARTESIAN_POINT('Ctrl Pts',(0.00920500766538901,-0.0331951640388602,
0.0797988453454978));
#91422=CARTESIAN_POINT('Ctrl Pts',(0.00908026713798448,-0.0330240426238156,
0.0798197810654535));
#91423=CARTESIAN_POINT('Ctrl Pts',(0.00900216038000823,-0.0329142774063509,
0.0798329575774273));
#91424=CARTESIAN_POINT('Ctrl Pts',(0.00892374228765528,-0.0328043479726686,
0.079844525973505));
#91425=CARTESIAN_POINT('Ctrl Pts',(0.00884511291220273,-0.0326943950436595,
0.0798544686670751));
#91426=CARTESIAN_POINT('Ctrl Pts',(0.00917117553053269,-0.0330240426238156,
0.079887433117526));
#91427=CARTESIAN_POINT('Ctrl Pts',(0.00909213679962896,-0.0329142774063509,
0.0799018619811748));
#91428=CARTESIAN_POINT('Ctrl Pts',(0.00901276038011862,-0.0328043479726686,
0.0799146640867869));
#91429=CARTESIAN_POINT('Ctrl Pts',(0.00893314750744128,-0.0326943950436595,
0.0799258202334665));
#91430=CARTESIAN_POINT('Ctrl Pts',(0.00926208392308091,-0.0330240426238156,
0.0799550851695986));
#91431=CARTESIAN_POINT('Ctrl Pts',(0.00918211321924968,-0.0329142774063509,
0.0799707663849225));
#91432=CARTESIAN_POINT('Ctrl Pts',(0.00910177847258196,-0.0328043479726686,
0.0799848022000688));
#91433=CARTESIAN_POINT('Ctrl Pts',(0.00902118210267983,-0.0326943950436595,
0.0799971717998579));
#91434=CARTESIAN_POINT('Ctrl Pts',(0.00935299231562913,-0.0330240426238156,
0.080022737221671));
#91435=CARTESIAN_POINT('Ctrl Pts',(0.0092720896388704,-0.0329142774063509,
0.0800396707886701));
#91436=CARTESIAN_POINT('Ctrl Pts',(0.00919079656504529,-0.0328043479726686,
0.0800549403133507));
#91437=CARTESIAN_POINT('Ctrl Pts',(0.00910921669791839,-0.0326943950436595,
0.0800685233662492));
#91438=CARTESIAN_POINT('Origin',(0.00681033084667279,-0.032639668285655,
0.0631783756830151));
#91439=CARTESIAN_POINT('Ctrl Pts',(0.00876113795712716,-0.0331951640388588,
0.0801160520975069));
#91440=CARTESIAN_POINT('Ctrl Pts',(0.00867896765870916,-0.0330855618255042,
0.0801248303837961));
#91441=CARTESIAN_POINT('Ctrl Pts',(0.00859655669269932,-0.0329757224427709,
0.0801319166786189));
#91442=CARTESIAN_POINT('Ctrl Pts',(0.00851401014616768,-0.0328657862078597,
0.0801372967309752));
#91443=CARTESIAN_POINT('Ctrl Pts',(0.00882682103059012,-0.0331951640388588,
0.080023710958784));
#91444=CARTESIAN_POINT('Ctrl Pts',(0.00874592254455342,-0.0330855618255042,
0.0800333938965343));
#91445=CARTESIAN_POINT('Ctrl Pts',(0.00866476561015732,-0.0329757224427709,
0.0800414117811568));
#91446=CARTESIAN_POINT('Ctrl Pts',(0.00858345365009207,-0.0328657862078597,
0.0800477492474656));
#91447=CARTESIAN_POINT('Ctrl Pts',(0.00889250410405308,-0.0331951640388588,
0.079931369820061));
#91448=CARTESIAN_POINT('Ctrl Pts',(0.00881287743039768,-0.0330855618255042,
0.0799419574092724));
#91449=CARTESIAN_POINT('Ctrl Pts',(0.00873297452761533,-0.0329757224427709,
0.0799509068836947));
#91450=CARTESIAN_POINT('Ctrl Pts',(0.00865289715401646,-0.0328657862078597,
0.0799582017639559));
#91451=CARTESIAN_POINT('Ctrl Pts',(0.00895818717751604,-0.0331951640388588,
0.079839028681338));
#91452=CARTESIAN_POINT('Ctrl Pts',(0.00887983231624194,-0.0330855618255042,
0.0798505209220106));
#91453=CARTESIAN_POINT('Ctrl Pts',(0.00880118344507333,-0.0329757224427709,
0.0798604019862326));
#91454=CARTESIAN_POINT('Ctrl Pts',(0.00872234065794085,-0.0328657862078597,
0.0798686542804464));
#91455=CARTESIAN_POINT('Origin',(0.00729087541601512,-0.032640190883449,
0.0631596730550064));
#91456=CARTESIAN_POINT('Ctrl Pts',(0.00899271919874454,-0.0332451089994434,
0.0798353384666383));
#91457=CARTESIAN_POINT('Ctrl Pts',(0.00877829315028171,-0.0329451141710259,
0.079868110961992));
#91458=CARTESIAN_POINT('Ctrl Pts',(0.00856200770526691,-0.0326442513127504,
0.0798846389075943));
#91459=CARTESIAN_POINT('Ctrl Pts',(0.00923897015052509,-0.0332451089994434,
0.0797922053152676));
#91460=CARTESIAN_POINT('Ctrl Pts',(0.00902617089548194,-0.0329451141710259,
0.0798342653172192));
#91461=CARTESIAN_POINT('Ctrl Pts',(0.00881080804937383,-0.0326442513127504,
0.0798601769213243));
#91462=CARTESIAN_POINT('Ctrl Pts',(0.00872237208319403,-0.0325229783203385,
0.0798686510814005));
#91463=CARTESIAN_POINT('Ctrl Pts',(0.00864354060453047,-0.032413025311208,
0.0798769026297948));
#91464=CARTESIAN_POINT('Ctrl Pts',(0.00856455038832971,-0.0323031222247695,
0.0798835221963075));
#91465=CARTESIAN_POINT('Ctrl Pts',(0.00848550291464223,-0.0321934096636185,
0.0798885048720837));
#91466=CARTESIAN_POINT('Ctrl Pts',(0.00880885321546822,-0.0325229783203385,
0.0799418778279532));
#91467=CARTESIAN_POINT('Ctrl Pts',(0.00872901230772316,-0.032413025311208,
0.079951321516843));
#91468=CARTESIAN_POINT('Ctrl Pts',(0.0086489881545835,-0.0323031222247695,
0.0799591121617028));
#91469=CARTESIAN_POINT('Ctrl Pts',(0.00856888361343182,-0.0321934096636185,
0.0799652434003435));
#91470=CARTESIAN_POINT('Ctrl Pts',(0.00889533434774241,-0.0325229783203385,
0.0800151045745059));
#91471=CARTESIAN_POINT('Ctrl Pts',(0.00881448401091586,-0.032413025311208,
0.0800257404038912));
#91472=CARTESIAN_POINT('Ctrl Pts',(0.00873342592083729,-0.0323031222247695,
0.0800347021270982));
#91473=CARTESIAN_POINT('Ctrl Pts',(0.0086522643122214,-0.0321934096636185,
0.0800419819286032));
#91474=CARTESIAN_POINT('Ctrl Pts',(0.00898181548001659,-0.0325229783203385,
0.0800883313210586));
#91475=CARTESIAN_POINT('Ctrl Pts',(0.00889995571410855,-0.032413025311208,
0.0801001592909393));
#91476=CARTESIAN_POINT('Ctrl Pts',(0.00881786368709107,-0.0323031222247695,
0.0801102920924935));
#91477=CARTESIAN_POINT('Ctrl Pts',(0.00873564501101099,-0.0321934096636185,
0.080118720456863));
#91478=CARTESIAN_POINT('Origin',(0.00681110715004839,-0.032639337517817,
0.0631868661705152));
#91479=CARTESIAN_POINT('Ctrl Pts',(0.00838526877037612,-0.0326943950436593,
0.0801442993560545));
#91480=CARTESIAN_POINT('Ctrl Pts',(0.00830265609073561,-0.0325844576448127,
0.0801479031311673));
#91481=CARTESIAN_POINT('Ctrl Pts',(0.0082199630324896,-0.0324744968375319,
0.0801497985956645));
#91482=CARTESIAN_POINT('Ctrl Pts',(0.00813729558030421,-0.0323646534831895,
0.0801499847823517));
#91483=CARTESIAN_POINT('Ctrl Pts',(0.0084566203134214,-0.0326943950436593,
0.0800562647896207));
#91484=CARTESIAN_POINT('Ctrl Pts',(0.0083752209151007,-0.0325844576448127,
0.0800608519227237));
#91485=CARTESIAN_POINT('Ctrl Pts',(0.00829372088658485,-0.0324744968375319,
0.0800637559074518));
#91486=CARTESIAN_POINT('Ctrl Pts',(0.00821222470178364,-0.0323646534831895,
0.0800649744633519));
#91487=CARTESIAN_POINT('Ctrl Pts',(0.00852797185646668,-0.0326943950436593,
0.0799682302231869));
#91488=CARTESIAN_POINT('Ctrl Pts',(0.00844778573946581,-0.0325844576448127,
0.07997380071428));
#91489=CARTESIAN_POINT('Ctrl Pts',(0.0083674787406801,-0.0324744968375319,
0.0799777132192391));
#91490=CARTESIAN_POINT('Ctrl Pts',(0.00828715382326307,-0.0323646534831895,
0.0799799641443521));
#91491=CARTESIAN_POINT('Ctrl Pts',(0.00859932339951197,-0.0326943950436593,
0.0798801956567531));
#91492=CARTESIAN_POINT('Ctrl Pts',(0.00852035056383091,-0.0325844576448127,
0.0798867495058364));
#91493=CARTESIAN_POINT('Ctrl Pts',(0.00844123659477534,-0.0324744968375319,
0.0798916705310263));
#91494=CARTESIAN_POINT('Ctrl Pts',(0.0083620829447425,-0.0323646534831895,
0.0798949538253523));
#91495=CARTESIAN_POINT('Origin',(0.00728755940808319,-0.0326395579067199,
0.0631219773537602));
#91496=CARTESIAN_POINT('Ctrl Pts',(0.00863405826269475,-0.0327445246961877,
0.0798786772760218));
#91497=CARTESIAN_POINT('Ctrl Pts',(0.00841799766936803,-0.0324436878365475,
0.0798979226524051));
#91498=CARTESIAN_POINT('Ctrl Pts',(0.00820110124096409,-0.0321434074463187,
0.079900838787937));
#91499=CARTESIAN_POINT('Ctrl Pts',(0.00888253145931961,-0.0327445246961877,
0.0798510897687218));
#91500=CARTESIAN_POINT('Ctrl Pts',(0.00866751134582941,-0.0324436878365475,
0.0798797064648185));
#91501=CARTESIAN_POINT('Ctrl Pts',(0.00845094655527419,-0.0321434074463187,
0.0798920456703277));
#91502=CARTESIAN_POINT('Ctrl Pts',(0.00800836761556641,-0.0321934096636184,
0.0801488898535788));
#91503=CARTESIAN_POINT('Ctrl Pts',(0.00792563824923524,-0.0320835708272304,
0.0801472981966059));
#91504=CARTESIAN_POINT('Ctrl Pts',(0.00784298980855697,-0.0319739230346347,
0.0801439953829223));
#91505=CARTESIAN_POINT('Ctrl Pts',(0.00776052771216514,-0.0318646057455575,
0.0801389937537248));
#91506=CARTESIAN_POINT('Ctrl Pts',(0.00808510620990588,-0.0321934096636184,
0.08006550908299));
#91507=CARTESIAN_POINT('Ctrl Pts',(0.00800352672938415,-0.0320835708272304,
0.0800649757110394));
#91508=CARTESIAN_POINT('Ctrl Pts',(0.00792200560638128,-0.0319739230346347,
0.0800627543653569));
#91509=CARTESIAN_POINT('Ctrl Pts',(0.00784064692339837,-0.0318646057455575,
0.0800588558927816));
#91510=CARTESIAN_POINT('Ctrl Pts',(0.00816184480424535,-0.0321934096636184,
0.0799821283124011));
#91511=CARTESIAN_POINT('Ctrl Pts',(0.00808141520953306,-0.0320835708272304,
0.0799826532254729));
#91512=CARTESIAN_POINT('Ctrl Pts',(0.0080010214042056,-0.0319739230346346,
0.0799815133477915));
#91513=CARTESIAN_POINT('Ctrl Pts',(0.00792076613463159,-0.0318646057455575,
0.0799787180318383));
#91514=CARTESIAN_POINT('Ctrl Pts',(0.00823858339858482,-0.0321934096636184,
0.0798987475418123));
#91515=CARTESIAN_POINT('Ctrl Pts',(0.00815930368968197,-0.0320835708272304,
0.0799003307399064));
#91516=CARTESIAN_POINT('Ctrl Pts',(0.00808003720202992,-0.0319739230346346,
0.0799002723302261));
#91517=CARTESIAN_POINT('Ctrl Pts',(0.00800088534586482,-0.0318646057455575,
0.0798985801708951));
#91518=CARTESIAN_POINT('Origin',(0.00729306470512945,-0.0326371942645793,
0.0632171198538876));
#91519=CARTESIAN_POINT('Ctrl Pts',(0.00836258658954841,-0.0320218834582342,
0.0798957610688848));
#91520=CARTESIAN_POINT('Ctrl Pts',(0.0083027871071084,-0.0319391099350621,
0.0798982464453459));
#91521=CARTESIAN_POINT('Ctrl Pts',(0.00824298504615354,-0.0318564869454885,
0.0798997965386773));
#91522=CARTESIAN_POINT('Ctrl Pts',(0.00818322406995633,-0.0317740741446461,
0.0799004142862709));
#91523=CARTESIAN_POINT('Ctrl Pts',(0.00839832609641107,-0.0320218834582342,
0.0799301051469319));
#91524=CARTESIAN_POINT('Ctrl Pts',(0.00833816917514486,-0.0319391099350621,
0.0799329624852597));
#91525=CARTESIAN_POINT('Ctrl Pts',(0.0082780040836902,-0.0318564869454885,
0.0799348787336382));
#91526=CARTESIAN_POINT('Ctrl Pts',(0.00821787477463702,-0.0317740741446461,
0.0799358565874493));
#91527=CARTESIAN_POINT('Ctrl Pts',(0.00843406560327374,-0.0320218834582342,
0.0799644492249789));
#91528=CARTESIAN_POINT('Ctrl Pts',(0.00837355124318133,-0.0319391099350621,
0.0799676785251735));
#91529=CARTESIAN_POINT('Ctrl Pts',(0.00831302312122687,-0.0318564869454885,
0.0799699609285991));
#91530=CARTESIAN_POINT('Ctrl Pts',(0.00825252547931771,-0.0317740741446461,
0.0799712988886277));
#91531=CARTESIAN_POINT('Ctrl Pts',(0.00846980511013641,-0.0320218834582342,
0.079998793303026));
#91532=CARTESIAN_POINT('Ctrl Pts',(0.00840893331121779,-0.0319391099350621,
0.0800023945650873));
#91533=CARTESIAN_POINT('Ctrl Pts',(0.00834804215876353,-0.0318564869454885,
0.08000504312356));
#91534=CARTESIAN_POINT('Ctrl Pts',(0.00828717618399839,-0.0317740741446461,
0.0800067411898061));
#91535=CARTESIAN_POINT('Origin',(0.00682280132131256,-0.0326352985526838,
0.0633090424749645));
#91536=CARTESIAN_POINT('Ctrl Pts',(0.008267748577978,-0.0322357172926636,
0.0798995563898468));
#91537=CARTESIAN_POINT('Ctrl Pts',(0.00808466288433491,-0.0319820232604284,
0.07990414077578));
#91538=CARTESIAN_POINT('Ctrl Pts',(0.00790165644468594,-0.0317296613809579,
0.0798970675263033));
#91539=CARTESIAN_POINT('Ctrl Pts',(0.00851747519824071,-0.0322357172926636,
0.079887868142238));
#91540=CARTESIAN_POINT('Ctrl Pts',(0.00833476169868981,-0.0319820232604284,
0.079900404684545));
#91541=CARTESIAN_POINT('Ctrl Pts',(0.0081516207639664,-0.0317296613809579,
0.0799012911605981));
#91542=CARTESIAN_POINT('Ctrl Pts',(0.0101257369179384,-0.0345231616327822,
0.079540125976521));
#91543=CARTESIAN_POINT('Ctrl Pts',(0.0100514416200429,-0.0344132092796975,
0.0795677201038758));
#91544=CARTESIAN_POINT('Ctrl Pts',(0.00997657939268488,-0.0343032738558974,
0.0795937760678668));
#91545=CARTESIAN_POINT('Ctrl Pts',(0.00990124699808852,-0.034193496108874,
0.0796182629444909));
#91546=CARTESIAN_POINT('Ctrl Pts',(0.0102277118106814,-0.0345231616327822,
0.0795895451771336));
#91547=CARTESIAN_POINT('Ctrl Pts',(0.0101527353386821,-0.0344132092796975,
0.0796185448848157));
#91548=CARTESIAN_POINT('Ctrl Pts',(0.0100771628990454,-0.0343032738558974,
0.0796459922670635));
#91549=CARTESIAN_POINT('Ctrl Pts',(0.0100010922095206,-0.034193496108874,
0.0796718546406128));
#91550=CARTESIAN_POINT('Ctrl Pts',(0.0103296867034243,-0.0345231616327822,
0.0796389643777463));
#91551=CARTESIAN_POINT('Ctrl Pts',(0.0102540290573213,-0.0344132092796975,
0.0796693696657557));
#91552=CARTESIAN_POINT('Ctrl Pts',(0.0101777464054059,-0.0343032738558974,
0.0796982084662603));
#91553=CARTESIAN_POINT('Ctrl Pts',(0.0101009374209526,-0.034193496108874,
0.0797254463367347));
#91554=CARTESIAN_POINT('Ctrl Pts',(0.0104316615961673,-0.0345231616327822,
0.079688383578359));
#91555=CARTESIAN_POINT('Ctrl Pts',(0.0103553227759604,-0.0344132092796975,
0.0797201944466957));
#91556=CARTESIAN_POINT('Ctrl Pts',(0.0102783299117663,-0.0343032738558974,
0.079750424665457));
#91557=CARTESIAN_POINT('Ctrl Pts',(0.0102007826323846,-0.034193496108874,
0.0797790380328567));
#91558=CARTESIAN_POINT('Origin',(0.00422215359472562,-0.0345625596230656,
0.0638101446865464));
#91559=CARTESIAN_POINT('Ctrl Pts',(0.00986777531919962,-0.0346945769586886,
0.0798909483516449));
#91560=CARTESIAN_POINT('Ctrl Pts',(0.00978866214920874,-0.034584662917669,
0.0799149814584064));
#91561=CARTESIAN_POINT('Ctrl Pts',(0.00970903847171624,-0.0344746925051586,
0.0799373826422171));
#91562=CARTESIAN_POINT('Ctrl Pts',(0.00962900642829233,-0.0343648066255171,
0.0799581236214394));
#91563=CARTESIAN_POINT('Ctrl Pts',(0.00991499190489023,-0.0346945769586886,
0.0797879351698764));
#91564=CARTESIAN_POINT('Ctrl Pts',(0.00983729830861111,-0.034584662917669,
0.0798126189450539));
#91565=CARTESIAN_POINT('Ctrl Pts',(0.00975908099174143,-0.0344746925051586,
0.0798357002646177));
#91566=CARTESIAN_POINT('Ctrl Pts',(0.00968044029745914,-0.0343648066255171,
0.0798571499680199));
#91567=CARTESIAN_POINT('Ctrl Pts',(0.00996220849058084,-0.0346945769586886,
0.0796849219881079));
#91568=CARTESIAN_POINT('Ctrl Pts',(0.00988593446801348,-0.034584662917669,
0.0797102564317014));
#91569=CARTESIAN_POINT('Ctrl Pts',(0.00980912351176662,-0.0344746925051586,
0.0797340178870183));
#91570=CARTESIAN_POINT('Ctrl Pts',(0.00973187416662595,-0.0343648066255171,
0.0797561763146005));
#91571=CARTESIAN_POINT('Ctrl Pts',(0.0100094250762715,-0.0346945769586886,
0.0795819088063395));
#91572=CARTESIAN_POINT('Ctrl Pts',(0.00993457062741585,-0.034584662917669,
0.0796078939183489));
#91573=CARTESIAN_POINT('Ctrl Pts',(0.00985916603179181,-0.0344746925051586,
0.0796323355094189));
#91574=CARTESIAN_POINT('Ctrl Pts',(0.00978330803579277,-0.0343648066255171,
0.079655202661181));
#91575=CARTESIAN_POINT('Origin',(0.00467172536872588,-0.034562644672989,
0.0636396237114132));
#91576=CARTESIAN_POINT('Ctrl Pts',(0.0100085802132244,-0.0346945769586885,
0.0795837520575904));
#91577=CARTESIAN_POINT('Ctrl Pts',(0.00989476810082433,-0.0345275153362891,
0.079623229906753));
#91578=CARTESIAN_POINT('Ctrl Pts',(0.00977968500876321,-0.0343603235965159,
0.0796591386807315));
#91579=CARTESIAN_POINT('Ctrl Pts',(0.00966367288018324,-0.0341934961088739,
0.0796913772360182));
#91580=CARTESIAN_POINT('Ctrl Pts',(0.0100871682192819,-0.0346945769586885,
0.079554563812779));
#91581=CARTESIAN_POINT('Ctrl Pts',(0.00997396746635576,-0.0345275153362891,
0.0795956877191934));
#91582=CARTESIAN_POINT('Ctrl Pts',(0.00985944412491194,-0.0343603235965159,
0.0796332622028711));
#91583=CARTESIAN_POINT('Ctrl Pts',(0.0097439385558184,-0.0341934961088739,
0.0796671811692697));
#91584=CARTESIAN_POINT('Ctrl Pts',(0.0101657562253394,-0.0346945769586885,
0.0795253755679676));
#91585=CARTESIAN_POINT('Ctrl Pts',(0.0100531668318872,-0.0345275153362891,
0.0795681455316338));
#91586=CARTESIAN_POINT('Ctrl Pts',(0.00993920324106068,-0.0343603235965159,
0.0796073857250107));
#91587=CARTESIAN_POINT('Ctrl Pts',(0.00982420423145356,-0.0341934961088739,
0.0796429851025211));
#91588=CARTESIAN_POINT('Ctrl Pts',(0.010244344231397,-0.0346945769586885,
0.0794961873231562));
#91589=CARTESIAN_POINT('Ctrl Pts',(0.0101323661974186,-0.0345275153362891,
0.0795406033440742));
#91590=CARTESIAN_POINT('Ctrl Pts',(0.0100189623572094,-0.0343603235965159,
0.0795815092471503));
#91591=CARTESIAN_POINT('Ctrl Pts',(0.00990446990708872,-0.0341934961088739,
0.0796187890357726));
#91592=CARTESIAN_POINT('Ctrl Pts',(0.0096984989248846,-0.03424362768739,
0.0796815813484631));
#91593=CARTESIAN_POINT('Ctrl Pts',(0.0094898718950713,-0.033943005420186,
0.0797409727690808));
#91594=CARTESIAN_POINT('Ctrl Pts',(0.00927736394762871,-0.0336441434784162,
0.0797844808221911));
#91595=CARTESIAN_POINT('Ctrl Pts',(0.00993740116890683,-0.03424362768739,
0.0796079218765593));
#91596=CARTESIAN_POINT('Ctrl Pts',(0.00973155225187409,-0.033943005420186,
0.0796763236438477));
#91597=CARTESIAN_POINT('Ctrl Pts',(0.00952113582865493,-0.0336441434784162,
0.0797290257050157));
#91598=CARTESIAN_POINT('Origin',(0.0046941281949332,-0.0345610621863657,
0.0637114892728983));
#91599=CARTESIAN_POINT('Origin',(0.00426216054678368,-0.0345589643415055,
0.0639235127682916));
#91600=CARTESIAN_POINT('Ctrl Pts',(0.00950385681755227,-0.034193496108874,
0.0799891261359099));
#91601=CARTESIAN_POINT('Ctrl Pts',(0.00942333872695702,-0.0340836138595105,
0.0800081565474908));
#91602=CARTESIAN_POINT('Ctrl Pts',(0.00934246547602342,-0.0339738896671456,
0.0800255116750088));
#91603=CARTESIAN_POINT('Ctrl Pts',(0.00926134206153027,-0.0338644633335883,
0.0800411762446778));
#91604=CARTESIAN_POINT('Ctrl Pts',(0.00955744856189494,-0.034193496108874,
0.0798892808346391));
#91605=CARTESIAN_POINT('Ctrl Pts',(0.00947830727886063,-0.0340836138595105,
0.0799090502446293));
#91606=CARTESIAN_POINT('Ctrl Pts',(0.00939879488284858,-0.0339738896671456,
0.0799271725061145));
#91607=CARTESIAN_POINT('Ctrl Pts',(0.0093190146947287,-0.0338644633335883,
0.0799436312467152));
#91608=CARTESIAN_POINT('Ctrl Pts',(0.00961104030623761,-0.034193496108874,
0.0797894355333683));
#91609=CARTESIAN_POINT('Ctrl Pts',(0.00953327583076425,-0.0340836138595105,
0.0798099439417678));
#91610=CARTESIAN_POINT('Ctrl Pts',(0.00945512428967374,-0.0339738896671456,
0.0798288333372201));
#91611=CARTESIAN_POINT('Ctrl Pts',(0.00937668732792713,-0.0338644633335883,
0.0798460862487527));
#91612=CARTESIAN_POINT('Ctrl Pts',(0.00966463205058028,-0.034193496108874,
0.0796895902320975));
#91613=CARTESIAN_POINT('Ctrl Pts',(0.00958824438266786,-0.0340836138595105,
0.0797108376389063));
#91614=CARTESIAN_POINT('Ctrl Pts',(0.0095114536964989,-0.0339738896671456,
0.0797304941683257));
#91615=CARTESIAN_POINT('Ctrl Pts',(0.00943435996112556,-0.0338644633335883,
0.0797485412507902));
#91616=CARTESIAN_POINT('Ctrl Pts',(0.00978333808643704,-0.0340223579322365,
0.0796551930208755));
#91617=CARTESIAN_POINT('Ctrl Pts',(0.00970740711653357,-0.0339125849573551,
0.0796780826249479));
#91618=CARTESIAN_POINT('Ctrl Pts',(0.00963105574082732,-0.0338030433565216,
0.0796993845501226));
#91619=CARTESIAN_POINT('Ctrl Pts',(0.00955438401470863,-0.033693872113232,
0.0797190802102514));
#91620=CARTESIAN_POINT('Ctrl Pts',(0.00988200887454069,-0.0340223579322365,
0.079710917839457));
#91621=CARTESIAN_POINT('Ctrl Pts',(0.00980530931405256,-0.0339125849573551,
0.0797351683710415));
#91622=CARTESIAN_POINT('Ctrl Pts',(0.00972816171980421,-0.0338030433565216,
0.0797578143593813));
#91623=CARTESIAN_POINT('Ctrl Pts',(0.00965066731778236,-0.033693872113232,
0.0797788355897594));
#91624=CARTESIAN_POINT('Ctrl Pts',(0.00998067966264434,-0.0340223579322365,
0.0797666426580385));
#91625=CARTESIAN_POINT('Ctrl Pts',(0.00990321151157155,-0.0339125849573551,
0.0797922541171351));
#91626=CARTESIAN_POINT('Ctrl Pts',(0.0098252676987811,-0.0338030433565216,
0.0798162441686399));
#91627=CARTESIAN_POINT('Ctrl Pts',(0.00974695062085609,-0.033693872113232,
0.0798385909692674));
#91628=CARTESIAN_POINT('Ctrl Pts',(0.010079350450748,-0.0340223579322365,
0.07982236747662));
#91629=CARTESIAN_POINT('Ctrl Pts',(0.0100011137090905,-0.0339125849573551,
0.0798493398632287));
#91630=CARTESIAN_POINT('Ctrl Pts',(0.00992237367775799,-0.0338030433565216,
0.0798746739778985));
#91631=CARTESIAN_POINT('Ctrl Pts',(0.00984323392392981,-0.033693872113232,
0.0798983463487754));
#91632=CARTESIAN_POINT('Origin',(0.00956485650479092,-0.0391228853390991,
0.0861418273486221));
#91633=CARTESIAN_POINT('Ctrl Pts',(0.011254964474949,-0.0352722978779635,
0.0789749209382626));
#91634=CARTESIAN_POINT('Ctrl Pts',(0.0112389250848038,-0.0352466642097244,
0.0789849124667666));
#91635=CARTESIAN_POINT('Ctrl Pts',(0.0112229414375835,-0.0352210183808315,
0.0789949616395067));
#91636=CARTESIAN_POINT('Ctrl Pts',(0.0112070132526816,-0.0351953608940152,
0.0790050692619298));
#91637=CARTESIAN_POINT('Origin',(0.0136902418348352,-0.0352456003065078,
0.0832268813538167));
#91638=CARTESIAN_POINT('Ctrl Pts',(0.0111002848269308,-0.035024121149334,
0.0790695235756326));
#91639=CARTESIAN_POINT('Ctrl Pts',(0.0110325204098152,-0.0349144232867421,
0.0791105236771512));
#91640=CARTESIAN_POINT('Ctrl Pts',(0.0109638679310742,-0.0348045283677512,
0.0791501475803453));
#91641=CARTESIAN_POINT('Ctrl Pts',(0.0108944134371579,-0.0346945769586886,
0.0791883412597654));
#91642=CARTESIAN_POINT('Ctrl Pts',(0.0112097137181652,-0.035024121149334,
0.0790989592608941));
#91643=CARTESIAN_POINT('Ctrl Pts',(0.0111415438365725,-0.0349144232867421,
0.0791414667004539));
#91644=CARTESIAN_POINT('Ctrl Pts',(0.0110724544929114,-0.0348045283677512,
0.0791825904626635));
#91645=CARTESIAN_POINT('Ctrl Pts',(0.0110025322217108,-0.0346945769586886,
0.079222274580122));
#91646=CARTESIAN_POINT('Ctrl Pts',(0.0113191426093997,-0.035024121149334,
0.0791283949461555));
#91647=CARTESIAN_POINT('Ctrl Pts',(0.0112505672633299,-0.0349144232867421,
0.0791724097237565));
#91648=CARTESIAN_POINT('Ctrl Pts',(0.0111810410547486,-0.0348045283677512,
0.0792150333449817));
#91649=CARTESIAN_POINT('Ctrl Pts',(0.0111106510062636,-0.0346945769586886,
0.0792562079004785));
#91650=CARTESIAN_POINT('Ctrl Pts',(0.0114285715006341,-0.035024121149334,
0.079157830631417));
#91651=CARTESIAN_POINT('Ctrl Pts',(0.0113595906900872,-0.0349144232867421,
0.0792033527470592));
#91652=CARTESIAN_POINT('Ctrl Pts',(0.0112896276165859,-0.0348045283677512,
0.0792474762272999));
#91653=CARTESIAN_POINT('Ctrl Pts',(0.0112187697908165,-0.0346945769586886,
0.0792901412208351));
#91654=CARTESIAN_POINT('Origin',(0.00296287029434561,-0.0345629067943208,
0.0643912613970295));
#91655=CARTESIAN_POINT('Ctrl Pts',(0.0109360748324534,-0.0351970973651599,
0.0793717364820537));
#91656=CARTESIAN_POINT('Ctrl Pts',(0.0108637347502008,-0.0350869349321765,
0.0794106969852403));
#91657=CARTESIAN_POINT('Ctrl Pts',(0.0107905247749954,-0.0349764985129724,
0.079448185852633));
#91658=CARTESIAN_POINT('Ctrl Pts',(0.0107165368935177,-0.0348659306849652,
0.0794841489331317));
#91659=CARTESIAN_POINT('Ctrl Pts',(0.0109557021224374,-0.0351970973651599,
0.0792918913811521));
#91660=CARTESIAN_POINT('Ctrl Pts',(0.0108844681858485,-0.0350869349321765,
0.0793311237938417));
#91661=CARTESIAN_POINT('Ctrl Pts',(0.0108123596197771,-0.0349764985129724,
0.0793689077921395));
#91662=CARTESIAN_POINT('Ctrl Pts',(0.0107394669614885,-0.0348659306849652,
0.0794051889265907));
#91663=CARTESIAN_POINT('Ctrl Pts',(0.0109753294124215,-0.03519709736516,
0.0792120462802505));
#91664=CARTESIAN_POINT('Ctrl Pts',(0.0109052016214963,-0.0350869349321765,
0.0792515506024431));
#91665=CARTESIAN_POINT('Ctrl Pts',(0.0108341944645589,-0.0349764985129724,
0.0792896297316459));
#91666=CARTESIAN_POINT('Ctrl Pts',(0.0107623970294593,-0.0348659306849652,
0.0793262289200496));
#91667=CARTESIAN_POINT('Ctrl Pts',(0.0109949567024055,-0.03519709736516,
0.0791322011793488));
#91668=CARTESIAN_POINT('Ctrl Pts',(0.010925935057144,-0.0350869349321765,
0.0791719774110446));
#91669=CARTESIAN_POINT('Ctrl Pts',(0.0108560293093406,-0.0349764985129724,
0.0792103516711524));
#91670=CARTESIAN_POINT('Ctrl Pts',(0.0107853270974301,-0.0348659306849652,
0.0792472689135086));
#91671=CARTESIAN_POINT('Origin',(0.0034073905888549,-0.0345637187967157,
0.0642076121005219));
#91672=CARTESIAN_POINT('Ctrl Pts',(0.0110246068595911,-0.0352450361861253,
0.0791162200167056));
#91673=CARTESIAN_POINT('Ctrl Pts',(0.0108373028029637,-0.0349452761023765,
0.0792256264114625));
#91674=CARTESIAN_POINT('Ctrl Pts',(0.0106422899203209,-0.0346444289983475,
0.0793206134866157));
#91675=CARTESIAN_POINT('Ctrl Pts',(0.0112376869692765,-0.0352450361861253,
0.0789854650288218));
#91676=CARTESIAN_POINT('Ctrl Pts',(0.0110553144178124,-0.0349452761023765,
0.0791029078715807));
#91677=CARTESIAN_POINT('Ctrl Pts',(0.0108646136923163,-0.0346444289983475,
0.0792062800251718));
#91678=CARTESIAN_POINT('Ctrl Pts',(0.0107855128249345,-0.0345231616327822,
0.0792467117641312));
#91679=CARTESIAN_POINT('Ctrl Pts',(0.0107152618288626,-0.0344132092796975,
0.0792833999734737));
#91680=CARTESIAN_POINT('Ctrl Pts',(0.0106442555907482,-0.0343032738558974,
0.0793186332034327));
#91681=CARTESIAN_POINT('Ctrl Pts',(0.0105725862340111,-0.0341934961088741,
0.0793523686463277));
#91682=CARTESIAN_POINT('Ctrl Pts',(0.0108928774834027,-0.0345231616327822,
0.0792829604365364));
#91683=CARTESIAN_POINT('Ctrl Pts',(0.0108221268504157,-0.0344132092796975,
0.0793211285165385));
#91684=CARTESIAN_POINT('Ctrl Pts',(0.0107505903912079,-0.0343032738558974,
0.0793578312062072));
#91685=CARTESIAN_POINT('Ctrl Pts',(0.0106783609566958,-0.0341934961088741,
0.0793930238327139));
#91686=CARTESIAN_POINT('Ctrl Pts',(0.0110002421418708,-0.0345231616327822,
0.0793192091089416));
#91687=CARTESIAN_POINT('Ctrl Pts',(0.0109289918719688,-0.0344132092796975,
0.0793588570596033));
#91688=CARTESIAN_POINT('Ctrl Pts',(0.0108569251916676,-0.0343032738558974,
0.0793970292089817));
#91689=CARTESIAN_POINT('Ctrl Pts',(0.0107841356793805,-0.0341934961088741,
0.0794336790191002));
#91690=CARTESIAN_POINT('Ctrl Pts',(0.011107606800339,-0.0345231616327822,
0.0793554577813468));
#91691=CARTESIAN_POINT('Ctrl Pts',(0.0110358568935219,-0.0344132092796975,
0.0793965856026682));
#91692=CARTESIAN_POINT('Ctrl Pts',(0.0109632599921274,-0.0343032738558974,
0.0794362272117561));
#91693=CARTESIAN_POINT('Ctrl Pts',(0.0108899104020652,-0.0341934961088741,
0.0794743342054864));
#91694=CARTESIAN_POINT('Origin',(0.00295699160068082,-0.0345625596230115,
0.0643806812625355));
#91695=CARTESIAN_POINT('Ctrl Pts',(0.0105735550331317,-0.0346945769586885,
0.0796270989613485));
#91696=CARTESIAN_POINT('Ctrl Pts',(0.0104980778410992,-0.034584662917669,
0.0796608580692974));
#91697=CARTESIAN_POINT('Ctrl Pts',(0.0104218896328888,-0.0344746925051586,
0.0796930621060512));
#91698=CARTESIAN_POINT('Ctrl Pts',(0.0103450882000249,-0.0343648066255171,
0.0797236702112484));
#91699=CARTESIAN_POINT('Ctrl Pts',(0.0106074883267706,-0.0346945769586885,
0.0795189802619239));
#91700=CARTESIAN_POINT('Ctrl Pts',(0.0105335010650637,-0.034584662917669,
0.0795532069878103));
#91701=CARTESIAN_POINT('Ctrl Pts',(0.0104587933715158,-0.0344746925051586,
0.0795859095335193));
#91702=CARTESIAN_POINT('Ctrl Pts',(0.0103834611432831,-0.0343648066255171,
0.0796170463921076));
#91703=CARTESIAN_POINT('Ctrl Pts',(0.0106414216204095,-0.0346945769586886,
0.0794108615624993));
#91704=CARTESIAN_POINT('Ctrl Pts',(0.0105689242890282,-0.034584662917669,
0.0794455559063233));
#91705=CARTESIAN_POINT('Ctrl Pts',(0.0104956971101427,-0.0344746925051586,
0.0794787569609873));
#91706=CARTESIAN_POINT('Ctrl Pts',(0.0104218340865413,-0.0343648066255171,
0.0795104225729668));
#91707=CARTESIAN_POINT('Ctrl Pts',(0.0106753549140484,-0.0346945769586886,
0.0793027428630747));
#91708=CARTESIAN_POINT('Ctrl Pts',(0.0106043475129927,-0.034584662917669,
0.0793379048248363));
#91709=CARTESIAN_POINT('Ctrl Pts',(0.0105326008487697,-0.0344746925051586,
0.0793716043884554));
#91710=CARTESIAN_POINT('Ctrl Pts',(0.0104602070297995,-0.0343648066255171,
0.0794037987538261));
#91711=CARTESIAN_POINT('Origin',(0.00338164642133868,-0.0345626446732309,
0.0641551586121303));
#91712=CARTESIAN_POINT('Ctrl Pts',(0.0106747477336384,-0.0346945769586886,
0.0793046774691565));
#91713=CARTESIAN_POINT('Ctrl Pts',(0.0105667809502284,-0.0345275153362891,
0.0793581084637529));
#91714=CARTESIAN_POINT('Ctrl Pts',(0.0104571058854778,-0.0343603235965159,
0.0794081578223798));
#91715=CARTESIAN_POINT('Ctrl Pts',(0.0103460491095624,-0.034193496108874,
0.0794546823422365));
#91716=CARTESIAN_POINT('Ctrl Pts',(0.0107490577926908,-0.0346945769586886,
0.0792658696934549));
#91717=CARTESIAN_POINT('Ctrl Pts',(0.0106419038536806,-0.0345275153362891,
0.0793208571419903));
#91718=CARTESIAN_POINT('Ctrl Pts',(0.0105329928945294,-0.0343603235965159,
0.079372488920343));
#91719=CARTESIAN_POINT('Ctrl Pts',(0.0104226492950858,-0.034193496108874,
0.0794206171120296));
#91720=CARTESIAN_POINT('Ctrl Pts',(0.0108233678517432,-0.0346945769586886,
0.0792270619177534));
#91721=CARTESIAN_POINT('Ctrl Pts',(0.0107170267571329,-0.0345275153362891,
0.0792836058202278));
#91722=CARTESIAN_POINT('Ctrl Pts',(0.0106088799035809,-0.0343603235965159,
0.0793368200183063));
#91723=CARTESIAN_POINT('Ctrl Pts',(0.0104992494806093,-0.034193496108874,
0.0793865518818228));
#91724=CARTESIAN_POINT('Ctrl Pts',(0.0108976779107956,-0.0346945769586886,
0.0791882541420519));
#91725=CARTESIAN_POINT('Ctrl Pts',(0.0107921496605851,-0.0345275153362891,
0.0792463544984652));
#91726=CARTESIAN_POINT('Ctrl Pts',(0.0106847669126324,-0.0343603235965159,
0.0793011511162696));
#91727=CARTESIAN_POINT('Ctrl Pts',(0.0105758496661327,-0.034193496108874,
0.0793524866516159));
#91728=CARTESIAN_POINT('Ctrl Pts',(0.00950385681755174,-0.0331951640388587,
0.0799891261359108));
#91729=CARTESIAN_POINT('Ctrl Pts',(0.00942343466748559,-0.0330855618255041,
0.0800081338719943));
#91730=CARTESIAN_POINT('Ctrl Pts',(0.00934256168480182,-0.0329757224427708,
0.080025493122117));
#91731=CARTESIAN_POINT('Ctrl Pts',(0.00926134034180358,-0.0328657862078597,
0.0800411765767499));
#91732=CARTESIAN_POINT('Ctrl Pts',(0.00955744854685499,-0.0331951640388587,
0.0798892808626596));
#91733=CARTESIAN_POINT('Ctrl Pts',(0.00947840156344252,-0.0330855618255041,
0.079909026716399));
#91734=CARTESIAN_POINT('Ctrl Pts',(0.00939888948312063,-0.0329757224427708,
0.0799271530386205));
#91735=CARTESIAN_POINT('Ctrl Pts',(0.00931901298729227,-0.0328657862078597,
0.0799436316229969));
#91736=CARTESIAN_POINT('Ctrl Pts',(0.00961104027615824,-0.0331951640388587,
0.0797894355894083));
#91737=CARTESIAN_POINT('Ctrl Pts',(0.00953336845939947,-0.0330855618255041,
0.0798099195608037));
#91738=CARTESIAN_POINT('Ctrl Pts',(0.00945521728143943,-0.0329757224427708,
0.079828812955124));
#91739=CARTESIAN_POINT('Ctrl Pts',(0.00937668563278096,-0.0328657862078597,
0.079846086669244));
#91740=CARTESIAN_POINT('Ctrl Pts',(0.00966463200546148,-0.0331951640388587,
0.0796895903161571));
#91741=CARTESIAN_POINT('Ctrl Pts',(0.00958833535535641,-0.0330855618255041,
0.0797108124052084));
#91742=CARTESIAN_POINT('Ctrl Pts',(0.00951154507975823,-0.0329757224427708,
0.0797304728716274));
#91743=CARTESIAN_POINT('Ctrl Pts',(0.00943435827826964,-0.0328657862078597,
0.079748541715491));
#91744=CARTESIAN_POINT('Origin',(0.00591998992064455,-0.0326401908834881,
0.0633507259648979));
#91745=CARTESIAN_POINT('Ctrl Pts',(0.00978333696304077,-0.0330240426238155,
0.079655193797274));
#91746=CARTESIAN_POINT('Ctrl Pts',(0.00970749755503332,-0.0329142774063509,
0.0796780557810556));
#91747=CARTESIAN_POINT('Ctrl Pts',(0.00963114771724851,-0.0328043479726687,
0.0796993613499594));
#91748=CARTESIAN_POINT('Ctrl Pts',(0.00955438450784236,-0.0326943950436595,
0.0797190805162996));
#91749=CARTESIAN_POINT('Ctrl Pts',(0.00988200756620427,-0.0330240426238155,
0.079710918549913));
#91750=CARTESIAN_POINT('Ctrl Pts',(0.00980540049543922,-0.0329142774063509,
0.0797351398173833));
#91751=CARTESIAN_POINT('Ctrl Pts',(0.00972825451199812,-0.0328043479726687,
0.0797577894778947));
#91752=CARTESIAN_POINT('Ctrl Pts',(0.00965066764653855,-0.0326943950436595,
0.0797788357937915));
#91753=CARTESIAN_POINT('Ctrl Pts',(0.00998067816936777,-0.0330240426238155,
0.0797666433025521));
#91754=CARTESIAN_POINT('Ctrl Pts',(0.00990330343584513,-0.0329142774063509,
0.079792223853711));
#91755=CARTESIAN_POINT('Ctrl Pts',(0.00982536130674774,-0.0328043479726687,
0.07981621760583));
#91756=CARTESIAN_POINT('Ctrl Pts',(0.00974695078523475,-0.0326943950436595,
0.0798385910712835));
#91757=CARTESIAN_POINT('Ctrl Pts',(0.0100793487725313,-0.0330240426238155,
0.0798223680551911));
#91758=CARTESIAN_POINT('Ctrl Pts',(0.010001206376251,-0.0329142774063509,
0.0798493078900387));
#91759=CARTESIAN_POINT('Ctrl Pts',(0.00992246810149735,-0.0328043479726687,
0.0798746457337654));
#91760=CARTESIAN_POINT('Ctrl Pts',(0.00984323392393094,-0.0326943950436595,
0.0798983463487755));
#91761=CARTESIAN_POINT('Origin',(0.00544557864969214,-0.0326396682856814,
0.0634295093221238));
#91762=CARTESIAN_POINT('Ctrl Pts',(0.00969842922484738,-0.0332451089994432,
0.0796816011900205));
#91763=CARTESIAN_POINT('Ctrl Pts',(0.00948980147263735,-0.0329451141710259,
0.0797409899744738));
#91764=CARTESIAN_POINT('Ctrl Pts',(0.0092772930038244,-0.0326442513127504,
0.0797844953464851));
#91765=CARTESIAN_POINT('Ctrl Pts',(0.00993733239698644,-0.0332451089994432,
0.0796079447283767));
#91766=CARTESIAN_POINT('Ctrl Pts',(0.00973148264367773,-0.0329451141710259,
0.0796763438933848));
#91767=CARTESIAN_POINT('Ctrl Pts',(0.00952106558306633,-0.0326442513127504,
0.0797290432986444));
#91768=CARTESIAN_POINT('Ctrl Pts',(0.00943438905477848,-0.0325229783203386,
0.079748534603042));
#91769=CARTESIAN_POINT('Ctrl Pts',(0.00935721337911216,-0.0324130253112081,
0.0797666012896402));
#91770=CARTESIAN_POINT('Ctrl Pts',(0.00927967567603521,-0.0323031222247696,
0.0797830687581102));
#91771=CARTESIAN_POINT('Ctrl Pts',(0.0092018760101549,-0.0321934096636185,
0.0797979194194819));
#91772=CARTESIAN_POINT('Ctrl Pts',(0.00952936600242293,-0.0325229783203386,
0.0798103449748761));
#91773=CARTESIAN_POINT('Ctrl Pts',(0.00945133827214809,-0.0324130253112081,
0.0798297209165968));
#91774=CARTESIAN_POINT('Ctrl Pts',(0.00937292156006982,-0.0323031222247696,
0.0798474798157712));
#91775=CARTESIAN_POINT('Ctrl Pts',(0.00929421711511575,-0.0321934096636185,
0.0798636024689296));
#91776=CARTESIAN_POINT('Ctrl Pts',(0.00962434295006738,-0.0325229783203386,
0.0798721553467102));
#91777=CARTESIAN_POINT('Ctrl Pts',(0.00954546316518402,-0.0324130253112081,
0.0798928405435533));
#91778=CARTESIAN_POINT('Ctrl Pts',(0.00946616744410443,-0.0323031222247696,
0.0799118908734322));
#91779=CARTESIAN_POINT('Ctrl Pts',(0.0093865582200766,-0.0321934096636185,
0.0799292855183772));
#91780=CARTESIAN_POINT('Ctrl Pts',(0.00971931989771183,-0.0325229783203386,
0.0799339657185444));
#91781=CARTESIAN_POINT('Ctrl Pts',(0.00963958805821995,-0.0324130253112081,
0.0799559601705099));
#91782=CARTESIAN_POINT('Ctrl Pts',(0.00955941332813904,-0.0323031222247696,
0.0799763019310933));
#91783=CARTESIAN_POINT('Ctrl Pts',(0.00947889932503745,-0.0321934096636185,
0.0799949685678249));
#91784=CARTESIAN_POINT('Origin',(0.00544741297196231,-0.0326393375178632,
0.0634378355632368));
#91785=CARTESIAN_POINT('Ctrl Pts',(0.00913449179185795,-0.0326943950436594,
0.0800642595569604));
#91786=CARTESIAN_POINT('Ctrl Pts',(0.00905298221065953,-0.0325844576448127,
0.0800781890295027));
#91787=CARTESIAN_POINT('Ctrl Pts',(0.00897117877657155,-0.0324744968375319,
0.0800904337360795));
#91788=CARTESIAN_POINT('Ctrl Pts',(0.00888918651731774,-0.0323646534831895,
0.080100979433722));
#91789=CARTESIAN_POINT('Ctrl Pts',(0.00919424704979836,-0.0326943950436594,
0.0799679764497674));
#91790=CARTESIAN_POINT('Ctrl Pts',(0.00911406443027083,-0.0325844576448127,
0.0799827294617575));
#91791=CARTESIAN_POINT('Ctrl Pts',(0.00903357101961889,-0.0324744968375319,
0.0799958252098081));
#91792=CARTESIAN_POINT('Ctrl Pts',(0.00895287018212779,-0.0323646534831895,
0.0800072483373953));
#91793=CARTESIAN_POINT('Ctrl Pts',(0.00925400230773878,-0.0326943950436594,
0.0798716933425744));
#91794=CARTESIAN_POINT('Ctrl Pts',(0.00917514664988214,-0.0325844576448127,
0.0798872698940122));
#91795=CARTESIAN_POINT('Ctrl Pts',(0.00909596326266623,-0.0324744968375319,
0.0799012166835366));
#91796=CARTESIAN_POINT('Ctrl Pts',(0.00901655384693785,-0.0323646534831895,
0.0799135172410685));
#91797=CARTESIAN_POINT('Ctrl Pts',(0.00931375756567919,-0.0326943950436594,
0.0797754102353815));
#91798=CARTESIAN_POINT('Ctrl Pts',(0.00923622886949344,-0.0325844576448127,
0.0797918103262669));
#91799=CARTESIAN_POINT('Ctrl Pts',(0.00915835550571357,-0.0324744968375319,
0.0798066081572652));
#91800=CARTESIAN_POINT('Ctrl Pts',(0.0090802375117479,-0.0323646534831895,
0.0798197861447417));
#91801=CARTESIAN_POINT('Origin',(0.00591197553634447,-0.0326395579067306,
0.0633137431114539));
#91802=CARTESIAN_POINT('Ctrl Pts',(0.00934802823052416,-0.0327445246961878,
0.0797695503948157));
#91803=CARTESIAN_POINT('Ctrl Pts',(0.00913608342476325,-0.0324436878365476,
0.0798157235884653));
#91804=CARTESIAN_POINT('Ctrl Pts',(0.00892126277817681,-0.0321434074463187,
0.0798458010601179));
#91805=CARTESIAN_POINT('Ctrl Pts',(0.00959108451028239,-0.0327445246961878,
0.0797110384740637));
#91806=CARTESIAN_POINT('Ctrl Pts',(0.00938134651766616,-0.0324436878365476,
0.0797663786850693));
#91807=CARTESIAN_POINT('Ctrl Pts',(0.00916803591769531,-0.0321434074463187,
0.0798057633577341));
#91808=CARTESIAN_POINT('Ctrl Pts',(0.00876113795712711,-0.0321934096636184,
0.080116052097507));
#91809=CARTESIAN_POINT('Ctrl Pts',(0.00867886144904434,-0.0320835708272304,
0.0801248417302177));
#91810=CARTESIAN_POINT('Ctrl Pts',(0.00859645076368787,-0.0319739230346347,
0.0801319235565257));
#91811=CARTESIAN_POINT('Ctrl Pts',(0.00851401203519589,-0.0318646057455576,
0.0801372966078556));
#91812=CARTESIAN_POINT('Ctrl Pts',(0.00882682106313487,-0.0321934096636184,
0.0800237109130306));
#91813=CARTESIAN_POINT('Ctrl Pts',(0.00874581801195238,-0.0320835708272304,
0.0800334063669634));
#91814=CARTESIAN_POINT('Ctrl Pts',(0.0086646612989163,-0.0319739230346347,
0.0800414198432049));
#91815=CARTESIAN_POINT('Ctrl Pts',(0.00858345554527552,-0.0318646057455576,
0.080047749058067));
#91816=CARTESIAN_POINT('Ctrl Pts',(0.00889250416914263,-0.0321934096636184,
0.0799313697285542));
#91817=CARTESIAN_POINT('Ctrl Pts',(0.00881277457486041,-0.0320835708272304,
0.0799419710037092));
#91818=CARTESIAN_POINT('Ctrl Pts',(0.00873287183414474,-0.0319739230346347,
0.0799509161298841));
#91819=CARTESIAN_POINT('Ctrl Pts',(0.00865289905535515,-0.0318646057455576,
0.0799582015082784));
#91820=CARTESIAN_POINT('Ctrl Pts',(0.00895818727515039,-0.0321934096636184,
0.0798390285440778));
#91821=CARTESIAN_POINT('Ctrl Pts',(0.00887973113776844,-0.0320835708272304,
0.079850535640455));
#91822=CARTESIAN_POINT('Ctrl Pts',(0.00880108236937318,-0.0319739230346347,
0.0798604124165632));
#91823=CARTESIAN_POINT('Ctrl Pts',(0.00872234256543479,-0.0318646057455576,
0.0798686539584898));
#91824=CARTESIAN_POINT('Origin',(0.00592936193985411,-0.032637194264516,
0.0634074453883521));
#91825=CARTESIAN_POINT('Ctrl Pts',(0.00908083835960602,-0.0320218834582334,
0.0798205238994861));
#91826=CARTESIAN_POINT('Ctrl Pts',(0.00902182191421492,-0.0319391099350615,
0.079830484540511));
#91827=CARTESIAN_POINT('Ctrl Pts',(0.0089626856885824,-0.0318564869454882,
0.0798395175965668));
#91828=CARTESIAN_POINT('Ctrl Pts',(0.00890347336983581,-0.031774074144646,
0.0798476205094238));
#91829=CARTESIAN_POINT('Ctrl Pts',(0.0091206005041376,-0.0320218834582334,
0.0798501178162585));
#91830=CARTESIAN_POINT('Ctrl Pts',(0.00906127605761572,-0.0319391099350615,
0.0798604922850837));
#91831=CARTESIAN_POINT('Ctrl Pts',(0.00900182555548336,-0.0318564869454882,
0.0798699341087311));
#91832=CARTESIAN_POINT('Ctrl Pts',(0.00894229294157205,-0.031774074144646,
0.0798784404526084));
#91833=CARTESIAN_POINT('Ctrl Pts',(0.00916036264866917,-0.0320218834582334,
0.079879711733031));
#91834=CARTESIAN_POINT('Ctrl Pts',(0.00910073020101652,-0.0319391099350615,
0.0798905000296564));
#91835=CARTESIAN_POINT('Ctrl Pts',(0.00904096542238433,-0.0318564869454882,
0.0799003506208954));
#91836=CARTESIAN_POINT('Ctrl Pts',(0.0089811125133083,-0.031774074144646,
0.079909260395793));
#91837=CARTESIAN_POINT('Ctrl Pts',(0.00920012479320074,-0.0320218834582334,
0.0799093056498034));
#91838=CARTESIAN_POINT('Ctrl Pts',(0.00914018434441733,-0.0319391099350615,
0.0799205077742291));
#91839=CARTESIAN_POINT('Ctrl Pts',(0.0090801052892853,-0.0318564869454882,
0.0799307671330597));
#91840=CARTESIAN_POINT('Ctrl Pts',(0.00901993208504454,-0.031774074144646,
0.0799400803389776));
#91841=CARTESIAN_POINT('Origin',(0.00547432768211527,-0.0326352985528673,
0.0635575828015964));
#91842=CARTESIAN_POINT('Ctrl Pts',(0.00898722884210647,-0.0322357242816073,
0.0798361748904105));
#91843=CARTESIAN_POINT('Ctrl Pts',(0.00880613154654552,-0.0319819883628705,
0.0798636745463319));
#91844=CARTESIAN_POINT('Ctrl Pts',(0.00862365138534982,-0.0317295851069886,
0.0798795947317981));
#91845=CARTESIAN_POINT('Ctrl Pts',(0.0092335213298815,-0.0322357242816073,
0.0797932795472415));
#91846=CARTESIAN_POINT('Ctrl Pts',(0.00905379019536725,-0.0319819883628705,
0.0798286232994688));
#91847=CARTESIAN_POINT('Ctrl Pts',(0.00887217428423548,-0.0317295851069886,
0.0798524586169422));
#91848=CARTESIAN_POINT('Ctrl Pts',(0.0104602356352348,-0.0340223579322365,
0.0794037854231929));
#91849=CARTESIAN_POINT('Ctrl Pts',(0.010387772231802,-0.0339125849573554,
0.0794360112098859));
#91850=CARTESIAN_POINT('Ctrl Pts',(0.0103146927486617,-0.0338030433565221,
0.0794667145278224));
#91851=CARTESIAN_POINT('Ctrl Pts',(0.0102410941227755,-0.0336938721132327,
0.0794958643971455));
#91852=CARTESIAN_POINT('Ctrl Pts',(0.0105651125464053,-0.0340223579322365,
0.0794467041060043));
#91853=CARTESIAN_POINT('Ctrl Pts',(0.0104920571823999,-0.0339125849573554,
0.0794803764188328));
#91854=CARTESIAN_POINT('Ctrl Pts',(0.0104183562149211,-0.0338030433565221,
0.0795125129942392));
#91855=CARTESIAN_POINT('Ctrl Pts',(0.0103441075381826,-0.0336938721132327,
0.0795430810899255));
#91856=CARTESIAN_POINT('Ctrl Pts',(0.0106699894575757,-0.0340223579322365,
0.0794896227888156));
#91857=CARTESIAN_POINT('Ctrl Pts',(0.0105963421329978,-0.0339125849573554,
0.0795247416277796));
#91858=CARTESIAN_POINT('Ctrl Pts',(0.0105220196811805,-0.0338030433565221,
0.0795583114606561));
#91859=CARTESIAN_POINT('Ctrl Pts',(0.0104471209535897,-0.0336938721132327,
0.0795902977827055));
#91860=CARTESIAN_POINT('Ctrl Pts',(0.0107748663687462,-0.0340223579322365,
0.079532541471627));
#91861=CARTESIAN_POINT('Ctrl Pts',(0.0107006270835957,-0.0339125849573554,
0.0795691068367265));
#91862=CARTESIAN_POINT('Ctrl Pts',(0.0106256831474399,-0.0338030433565221,
0.079604109927073));
#91863=CARTESIAN_POINT('Ctrl Pts',(0.0105501343689969,-0.0336938721132327,
0.0796375144754855));
#91864=CARTESIAN_POINT('Origin',(0.00301089187414373,-0.0345589643415107,
0.0644881412024376));
#91865=CARTESIAN_POINT('Ctrl Pts',(0.0102248110767331,-0.034193496108874,
0.0797701136670256));
#91866=CARTESIAN_POINT('Ctrl Pts',(0.0101473130373639,-0.0340836138581107,
0.079799085611151));
#91867=CARTESIAN_POINT('Ctrl Pts',(0.0100692526694187,-0.0339738896643499,
0.0798264399946811));
#91868=CARTESIAN_POINT('Ctrl Pts',(0.00999073222743623,-0.0338644633294062,
0.0798521485046812));
#91869=CARTESIAN_POINT('Ctrl Pts',(0.0102654662997002,-0.034193496108874,
0.0796643388491664));
#91870=CARTESIAN_POINT('Ctrl Pts',(0.010189426832432,-0.0340836138581107,
0.0796938714047413));
#91871=CARTESIAN_POINT('Ctrl Pts',(0.0101128127360598,-0.0339738896643499,
0.0797218163128183));
#91872=CARTESIAN_POINT('Ctrl Pts',(0.0100357244647382,-0.0338644633294062,
0.0797481443805791));
#91873=CARTESIAN_POINT('Ctrl Pts',(0.0103061215226674,-0.034193496108874,
0.0795585640313071));
#91874=CARTESIAN_POINT('Ctrl Pts',(0.0102315406275001,-0.0340836138581107,
0.0795886571983317));
#91875=CARTESIAN_POINT('Ctrl Pts',(0.0101563728027009,-0.0339738896643499,
0.0796171926309556));
#91876=CARTESIAN_POINT('Ctrl Pts',(0.0100807167020402,-0.0338644633294062,
0.0796441402564771));
#91877=CARTESIAN_POINT('Ctrl Pts',(0.0103467767456346,-0.034193496108874,
0.0794527892134478));
#91878=CARTESIAN_POINT('Ctrl Pts',(0.0102736544225682,-0.0340836138581107,
0.0794834429919221));
#91879=CARTESIAN_POINT('Ctrl Pts',(0.010199932869342,-0.0339738896643499,
0.0795125689490928));
#91880=CARTESIAN_POINT('Ctrl Pts',(0.0101257089393421,-0.0338644633294062,
0.079540136132375));
#91881=CARTESIAN_POINT('Origin',(0.00341287973882487,-0.0345610621861447,
0.0642236496744578));
#91882=CARTESIAN_POINT('Ctrl Pts',(0.0103793727902364,-0.03424362768739,
0.0794405988373859));
#91883=CARTESIAN_POINT('Ctrl Pts',(0.010179834565659,-0.033943005420186,
0.0795256698391681));
#91884=CARTESIAN_POINT('Ctrl Pts',(0.00997445531183739,-0.0336441434784162,
0.0795954691264955));
#91885=CARTESIAN_POINT('Ctrl Pts',(0.0106071592389115,-0.03424362768739,
0.0793375778016699));
#91886=CARTESIAN_POINT('Ctrl Pts',(0.0104115065167494,-0.033943005420186,
0.07943123991099));
#91887=CARTESIAN_POINT('Ctrl Pts',(0.0102093546096173,-0.0336441434784162,
0.0795098985713815));
#91888=CARTESIAN_POINT('Ctrl Pts',(0.0100085802132314,-0.0336938721132429,
0.079583752057588));
#91889=CARTESIAN_POINT('Ctrl Pts',(0.00989482947711622,-0.0335278710435085,
0.0796232086172443));
#91890=CARTESIAN_POINT('Ctrl Pts',(0.00977988141079358,-0.0333620469224321,
0.0796590841026647));
#91891=CARTESIAN_POINT('Ctrl Pts',(0.00966367288018423,-0.0331951640388602,
0.079691377236018));
#91892=CARTESIAN_POINT('Ctrl Pts',(0.0100871682276307,-0.0336938721132429,
0.0795545638096783));
#91893=CARTESIAN_POINT('Ctrl Pts',(0.00997402852136208,-0.0335278710435085,
0.0795956655390796));
#91894=CARTESIAN_POINT('Ctrl Pts',(0.00985963967783158,-0.0333620469224321,
0.0796332047772154));
#91895=CARTESIAN_POINT('Ctrl Pts',(0.00974393856433933,-0.0331951640388602,
0.0796671811667011));
#91896=CARTESIAN_POINT('Ctrl Pts',(0.0101657562420301,-0.0336938721132429,
0.0795253755617685));
#91897=CARTESIAN_POINT('Ctrl Pts',(0.0100532275656079,-0.0335278710435085,
0.079568122460915));
#91898=CARTESIAN_POINT('Ctrl Pts',(0.00993939794486958,-0.0333620469224321,
0.0796073254517662));
#91899=CARTESIAN_POINT('Ctrl Pts',(0.00982420424849443,-0.0331951640388602,
0.0796429850973842));
#91900=CARTESIAN_POINT('Ctrl Pts',(0.0102443442564294,-0.0336938721132429,
0.0794961873138587));
#91901=CARTESIAN_POINT('Ctrl Pts',(0.0101324266098538,-0.0335278710435085,
0.0795405793827504));
#91902=CARTESIAN_POINT('Ctrl Pts',(0.0100191562119076,-0.0333620469224321,
0.0795814461263169));
#91903=CARTESIAN_POINT('Ctrl Pts',(0.00990446993264953,-0.0331951640388602,
0.0796187890280672));
#91904=CARTESIAN_POINT('Ctrl Pts',(0.0100085802132344,-0.0336938721132427,
0.0795837520576004));
#91905=CARTESIAN_POINT('Ctrl Pts',(0.00997677465933334,-0.0336474569765026,
0.0795947844058536));
#91906=CARTESIAN_POINT('Ctrl Pts',(0.0099448421372035,-0.0336011045488949,
0.0796054436739975));
#91907=CARTESIAN_POINT('Ctrl Pts',(0.00986466967179713,-0.0334847282606778,
0.0796322057256462));
#91908=CARTESIAN_POINT('Ctrl Pts',(0.00978374541518868,-0.0333679869945434,
0.0796566003215673));
#91909=CARTESIAN_POINT('Origin',(0.00547819766777445,-0.0326434571768956,
0.0635488047474904));
#91910=CARTESIAN_POINT('Ctrl Pts',(0.00986693048984509,-0.033693872113246,
0.0798927915294063));
#91911=CARTESIAN_POINT('Ctrl Pts',(0.00983331602536066,-0.0336474569764993,
0.0799029947548258));
#91912=CARTESIAN_POINT('Ctrl Pts',(0.00979958442252474,-0.033601104548885,
0.0799128037813654));
#91913=CARTESIAN_POINT('Ctrl Pts',(0.00971418376321095,-0.0334837508643205,
0.0799376379802556));
#91914=CARTESIAN_POINT('Ctrl Pts',(0.00962808471679835,-0.0333660264760493,
0.0799599306753055));
#91915=CARTESIAN_POINT('Ctrl Pts',(0.0100085802132335,-0.033693872113246,
0.0795837520575873));
#91916=CARTESIAN_POINT('Ctrl Pts',(0.00997677465932791,-0.0336474569764993,
0.0795947844058422));
#91917=CARTESIAN_POINT('Ctrl Pts',(0.0099448421371935,-0.033601104548885,
0.0796054436739875));
#91918=CARTESIAN_POINT('Ctrl Pts',(0.00986399633638482,-0.0334837508643205,
0.0796324304890475));
#91919=CARTESIAN_POINT('Ctrl Pts',(0.00978238636184186,-0.0333660264760493,
0.0796570098248924));
#91920=CARTESIAN_POINT('Ctrl Pts',(0.0101257348912479,-0.0335235895815128,
0.0795401263586193));
#91921=CARTESIAN_POINT('Ctrl Pts',(0.0100515291897403,-0.0334144449262719,
0.079567687178991));
#91922=CARTESIAN_POINT('Ctrl Pts',(0.00997666884906489,-0.0333049234473133,
0.0795937466294591));
#91923=CARTESIAN_POINT('Ctrl Pts',(0.00990124657415982,-0.0331951640388588,
0.0796182627169481));
#91924=CARTESIAN_POINT('Ctrl Pts',(0.0102277099137026,-0.0335235895815128,
0.0795895456593257));
#91925=CARTESIAN_POINT('Ctrl Pts',(0.0101528238582231,-0.0334144449262719,
0.0796185103666518));
#91926=CARTESIAN_POINT('Ctrl Pts',(0.0100772533786836,-0.0333049234473133,
0.0796459612613693));
#91927=CARTESIAN_POINT('Ctrl Pts',(0.0100010919269015,-0.0331951640388588,
0.0796718544889176));
#91928=CARTESIAN_POINT('Ctrl Pts',(0.0103296849361572,-0.0335235895815128,
0.0796389649600321));
#91929=CARTESIAN_POINT('Ctrl Pts',(0.0102541185267059,-0.0334144449262719,
0.0796693335543126));
#91930=CARTESIAN_POINT('Ctrl Pts',(0.0101778379083023,-0.0333049234473133,
0.0796981758932794));
#91931=CARTESIAN_POINT('Ctrl Pts',(0.0101009372796431,-0.0331951640388588,
0.0797254462608871));
#91932=CARTESIAN_POINT('Ctrl Pts',(0.0104316599586119,-0.0335235895815128,
0.0796883842607385));
#91933=CARTESIAN_POINT('Ctrl Pts',(0.0103554131951887,-0.0334144449262719,
0.0797201567419734));
#91934=CARTESIAN_POINT('Ctrl Pts',(0.010278422437921,-0.0333049234473132,
0.0797503905251896));
#91935=CARTESIAN_POINT('Ctrl Pts',(0.0102007826323847,-0.0331951640388588,
0.0797790380328566));
#91936=CARTESIAN_POINT('Origin',(0.0110564677013646,-0.0391228853390852,
0.0858666537048777));
#91937=CARTESIAN_POINT('Ctrl Pts',(0.0118349971103021,-0.0352722978779628,
0.0785444337952683));
#91938=CARTESIAN_POINT('Ctrl Pts',(0.0118203364661147,-0.0352466642097239,
0.0785563568062168));
#91939=CARTESIAN_POINT('Ctrl Pts',(0.0118057383500412,-0.0352210183808312,
0.0785683300204186));
#91940=CARTESIAN_POINT('Ctrl Pts',(0.0117912025846368,-0.0351953608940152,
0.0785803542721384));
#91941=CARTESIAN_POINT('Origin',(0.0147839835286742,-0.0352456003065068,
0.0824576450467876));
#91942=CARTESIAN_POINT('Ctrl Pts',(0.0116933940119547,-0.035024121149334,
0.0786576769630387));
#91943=CARTESIAN_POINT('Ctrl Pts',(0.0116313026128081,-0.0349144232867422,
0.0787068469000283));
#91944=CARTESIAN_POINT('Ctrl Pts',(0.0115681576712812,-0.0348045283677512,
0.0787547627940635));
#91945=CARTESIAN_POINT('Ctrl Pts',(0.011504037784138,-0.0346945769586886,
0.0788013602612215));
#91946=CARTESIAN_POINT('Ctrl Pts',(0.0118056492933128,-0.035024121149334,
0.078673165462346));
#91947=CARTESIAN_POINT('Ctrl Pts',(0.0117433445464483,-0.0349144232867422,
0.0787238816697402));
#91948=CARTESIAN_POINT('Ctrl Pts',(0.0116799541669921,-0.0348045283677512,
0.0787733403496477));
#91949=CARTESIAN_POINT('Ctrl Pts',(0.0116155569925468,-0.0346945769586886,
0.0788214751303346));
#91950=CARTESIAN_POINT('Ctrl Pts',(0.0119179045746708,-0.035024121149334,
0.0786886539616534));
#91951=CARTESIAN_POINT('Ctrl Pts',(0.0118553864800886,-0.0349144232867422,
0.0787409164394521));
#91952=CARTESIAN_POINT('Ctrl Pts',(0.0117917506627029,-0.0348045283677512,
0.0787919179052318));
#91953=CARTESIAN_POINT('Ctrl Pts',(0.0117270762009556,-0.0346945769586886,
0.0788415899994477));
#91954=CARTESIAN_POINT('Ctrl Pts',(0.0120301598560289,-0.035024121149334,
0.0787041424609608));
#91955=CARTESIAN_POINT('Ctrl Pts',(0.0119674284137288,-0.0349144232867422,
0.0787579512091641));
#91956=CARTESIAN_POINT('Ctrl Pts',(0.0119035471584137,-0.0348045283677512,
0.078810495460816));
#91957=CARTESIAN_POINT('Ctrl Pts',(0.0118385954093645,-0.0346945769586886,
0.0788617048685608));
#91958=CARTESIAN_POINT('Origin',(0.00178047136194146,-0.034562906794219,
0.065115045742413));
#91959=CARTESIAN_POINT('Ctrl Pts',(0.0115683561831177,-0.0351970973651602,
0.0789780878000176));
#91960=CARTESIAN_POINT('Ctrl Pts',(0.0115014695698662,-0.0350869349321767,
0.0790258077044247));
#91961=CARTESIAN_POINT('Ctrl Pts',(0.0114335354781549,-0.0349764985129725,
0.0790721766038223));
#91962=CARTESIAN_POINT('Ctrl Pts',(0.0113646383823896,-0.0348659306849652,
0.0791171292451199));
#91963=CARTESIAN_POINT('Ctrl Pts',(0.0115778214613775,-0.0351970973651602,
0.0788964123498657));
#91964=CARTESIAN_POINT('Ctrl Pts',(0.011512066350798,-0.0350869349321767,
0.0789442633828754));
#91965=CARTESIAN_POINT('Ctrl Pts',(0.0114452619729914,-0.0349764985129725,
0.0789907870428144));
#91966=CARTESIAN_POINT('Ctrl Pts',(0.0113774913269834,-0.0348659306849652,
0.0790359179622504));
#91967=CARTESIAN_POINT('Ctrl Pts',(0.0115872867396373,-0.0351970973651602,
0.0788147368997138));
#91968=CARTESIAN_POINT('Ctrl Pts',(0.0115226631317298,-0.0350869349321767,
0.078862719061326));
#91969=CARTESIAN_POINT('Ctrl Pts',(0.0114569884678279,-0.0349764985129725,
0.0789093974818066));
#91970=CARTESIAN_POINT('Ctrl Pts',(0.0113903442715773,-0.0348659306849652,
0.0789547066793808));
#91971=CARTESIAN_POINT('Ctrl Pts',(0.0115967520178971,-0.0351970973651602,
0.0787330614495619));
#91972=CARTESIAN_POINT('Ctrl Pts',(0.0115332599126616,-0.0350869349321767,
0.0787811747397767));
#91973=CARTESIAN_POINT('Ctrl Pts',(0.0114687149626644,-0.0349764985129725,
0.0788280079207987));
#91974=CARTESIAN_POINT('Ctrl Pts',(0.0114031972161712,-0.0348659306849652,
0.0788734953965113));
#91975=CARTESIAN_POINT('Origin',(0.00219846912065955,-0.0345637187966843,
0.064877131409313));
#91976=CARTESIAN_POINT('Ctrl Pts',(0.011624165403947,-0.0352450361861252,
0.0787134901530824));
#91977=CARTESIAN_POINT('Ctrl Pts',(0.0114520505529786,-0.0349452761023765,
0.0788455092688154));
#91978=CARTESIAN_POINT('Ctrl Pts',(0.0112704804424388,-0.0346444289983475,
0.0789641889376781));
#91979=CARTESIAN_POINT('Ctrl Pts',(0.0118191773678874,-0.0352450361861252,
0.0785570601881776));
#91980=CARTESIAN_POINT('Ctrl Pts',(0.0116529623697057,-0.0349452761023765,
0.0786964343006313));
#91981=CARTESIAN_POINT('Ctrl Pts',(0.0114767213426597,-0.0346444289983475,
0.078822892472485));
#91982=CARTESIAN_POINT('Ctrl Pts',(0.011403311649826,-0.0345231616327822,
0.078872919362593));
#91983=CARTESIAN_POINT('Ctrl Pts',(0.0113382128557516,-0.0344132092796975,
0.0789181230589455));
#91984=CARTESIAN_POINT('Ctrl Pts',(0.011272182417673,-0.0343032738558974,
0.0789619779057887));
#91985=CARTESIAN_POINT('Ctrl Pts',(0.0112053063673641,-0.0341934961088741,
0.0790044298868675));
#91986=CARTESIAN_POINT('Ctrl Pts',(0.0115143728692186,-0.0345231616327822,
0.078895425843573));
#91987=CARTESIAN_POINT('Ctrl Pts',(0.0114489638549906,-0.0344132092796975,
0.078942160362473));
#91988=CARTESIAN_POINT('Ctrl Pts',(0.0113825915489072,-0.0343032738558974,
0.0789875395362214));
#91989=CARTESIAN_POINT('Ctrl Pts',(0.0113153424707378,-0.0341934961088741,
0.0790315074069425));
#91990=CARTESIAN_POINT('Ctrl Pts',(0.0116254340886112,-0.0345231616327822,
0.078917932324553));
#91991=CARTESIAN_POINT('Ctrl Pts',(0.0115597148542295,-0.0344132092796975,
0.0789661976660006));
#91992=CARTESIAN_POINT('Ctrl Pts',(0.0114930006801414,-0.0343032738558974,
0.079013101166654));
#91993=CARTESIAN_POINT('Ctrl Pts',(0.0114253785741115,-0.0341934961088741,
0.0790585849270175));
#91994=CARTESIAN_POINT('Ctrl Pts',(0.0117364953080039,-0.0345231616327822,
0.0789404388055329));
#91995=CARTESIAN_POINT('Ctrl Pts',(0.0116704658534684,-0.0344132092796975,
0.0789902349695282));
#91996=CARTESIAN_POINT('Ctrl Pts',(0.0116034098113757,-0.0343032738558974,
0.0790386627970866));
#91997=CARTESIAN_POINT('Ctrl Pts',(0.0115354146774852,-0.0341934961088741,
0.0790856624470924));
#91998=CARTESIAN_POINT('Origin',(0.00177331298048502,-0.0345625596230865,
0.0651052858307627));
#91999=CARTESIAN_POINT('Ctrl Pts',(0.0112407003659537,-0.0346945769586886,
0.0792768724485713));
#92000=CARTESIAN_POINT('Ctrl Pts',(0.0111700494722858,-0.034584662917669,
0.0793198251564084));
#92001=CARTESIAN_POINT('Ctrl Pts',(0.0110984982669136,-0.0344746925051586,
0.079361324169208));
#92002=CARTESIAN_POINT('Ctrl Pts',(0.0110261386490849,-0.0343648066255171,
0.0794013166922767));
#92003=CARTESIAN_POINT('Ctrl Pts',(0.0112608152192293,-0.0346945769586886,
0.0791653533279674));
#92004=CARTESIAN_POINT('Ctrl Pts',(0.0111917011154095,-0.034584662917669,
0.0792085832286495));
#92005=CARTESIAN_POINT('Ctrl Pts',(0.0111216812301388,-0.0344746925051586,
0.0792503912618223));
#92006=CARTESIAN_POINT('Ctrl Pts',(0.0110508455021963,-0.0343648066255171,
0.0792907242287365));
#92007=CARTESIAN_POINT('Ctrl Pts',(0.0112809300725049,-0.0346945769586886,
0.0790538342073635));
#92008=CARTESIAN_POINT('Ctrl Pts',(0.0112133527585333,-0.034584662917669,
0.0790973413008906));
#92009=CARTESIAN_POINT('Ctrl Pts',(0.011144864193364,-0.0344746925051586,
0.0791394583544365));
#92010=CARTESIAN_POINT('Ctrl Pts',(0.0110755523553077,-0.0343648066255171,
0.0791801317651963));
#92011=CARTESIAN_POINT('Ctrl Pts',(0.0113010449257805,-0.0346945769586886,
0.0789423150867597));
#92012=CARTESIAN_POINT('Ctrl Pts',(0.011235004401657,-0.034584662917669,
0.0789860993731318));
#92013=CARTESIAN_POINT('Ctrl Pts',(0.0111680471565892,-0.0344746925051586,
0.0790285254470508));
#92014=CARTESIAN_POINT('Ctrl Pts',(0.0111002592084191,-0.0343648066255171,
0.0790695393016561));
#92015=CARTESIAN_POINT('Origin',(0.00216635378845963,-0.0345626446731195,
0.0648283181321802));
#92016=CARTESIAN_POINT('Ctrl Pts',(0.0113006850036053,-0.0346945769586886,
0.0789443105377789));
#92017=CARTESIAN_POINT('Ctrl Pts',(0.0112002662498559,-0.0345275153362891,
0.0790108520391062));
#92018=CARTESIAN_POINT('Ctrl Pts',(0.0110977288537038,-0.0343603235965159,
0.0790742526740977));
#92019=CARTESIAN_POINT('Ctrl Pts',(0.0109933788621512,-0.034193496108874,
0.0791343294390539));
#92020=CARTESIAN_POINT('Ctrl Pts',(0.0113695452016306,-0.0346945769586886,
0.0788964952529927));
#92021=CARTESIAN_POINT('Ctrl Pts',(0.0112701279581652,-0.0345275153362891,
0.0789644790587378));
#92022=CARTESIAN_POINT('Ctrl Pts',(0.0111685469721926,-0.0343603235965159,
0.0790293538677774));
#92023=CARTESIAN_POINT('Ctrl Pts',(0.0110651055268785,-0.034193496108874,
0.0790909322744188));
#92024=CARTESIAN_POINT('Ctrl Pts',(0.0114384053996559,-0.0346945769586886,
0.0788486799682066));
#92025=CARTESIAN_POINT('Ctrl Pts',(0.0113399896664746,-0.0345275153362891,
0.0789181060783693));
#92026=CARTESIAN_POINT('Ctrl Pts',(0.0112393650906815,-0.0343603235965159,
0.0789844550614572));
#92027=CARTESIAN_POINT('Ctrl Pts',(0.0111368321916058,-0.034193496108874,
0.0790475351097837));
#92028=CARTESIAN_POINT('Ctrl Pts',(0.0115072655976812,-0.0346945769586886,
0.0788008646834204));
#92029=CARTESIAN_POINT('Ctrl Pts',(0.0114098513747839,-0.0345275153362891,
0.0788717330980009));
#92030=CARTESIAN_POINT('Ctrl Pts',(0.0113101832091703,-0.0343603235965159,
0.0789395562551369));
#92031=CARTESIAN_POINT('Ctrl Pts',(0.011208558856333,-0.034193496108874,
0.0790041379451486));
#92032=CARTESIAN_POINT('Ctrl Pts',(0.0111002859175206,-0.0340223579322365,
0.0790695224909273));
#92033=CARTESIAN_POINT('Ctrl Pts',(0.0110324328717179,-0.0339125849573551,
0.0791105762403342));
#92034=CARTESIAN_POINT('Ctrl Pts',(0.0109637777882479,-0.0338030433565216,
0.0791501967413674));
#92035=CARTESIAN_POINT('Ctrl Pts',(0.0108944129568897,-0.033693872113232,
0.0791883411090325));
#92036=CARTESIAN_POINT('Ctrl Pts',(0.0112097149802182,-0.0340223579322365,
0.0790989581847022));
#92037=CARTESIAN_POINT('Ctrl Pts',(0.0111414559394269,-0.0339125849573551,
0.0791415212462867));
#92038=CARTESIAN_POINT('Ctrl Pts',(0.0110723639070013,-0.0338030433565216,
0.0791826415957684));
#92039=CARTESIAN_POINT('Ctrl Pts',(0.011002531901532,-0.033693872113232,
0.0792222744796335));
#92040=CARTESIAN_POINT('Ctrl Pts',(0.0113191440429158,-0.0340223579322365,
0.0791283938784772));
#92041=CARTESIAN_POINT('Ctrl Pts',(0.0112504790071358,-0.0339125849573551,
0.0791724662522392));
#92042=CARTESIAN_POINT('Ctrl Pts',(0.0111809500257546,-0.0338030433565216,
0.0792150864501694));
#92043=CARTESIAN_POINT('Ctrl Pts',(0.0111106508461742,-0.033693872113232,
0.0792562078502345));
#92044=CARTESIAN_POINT('Ctrl Pts',(0.0114285731056134,-0.0340223579322365,
0.0791578295722521));
#92045=CARTESIAN_POINT('Ctrl Pts',(0.0113595020748448,-0.0339125849573551,
0.0792034112581918));
#92046=CARTESIAN_POINT('Ctrl Pts',(0.011289536144508,-0.0338030433565216,
0.0792475313045704));
#92047=CARTESIAN_POINT('Ctrl Pts',(0.0112187697908164,-0.033693872113232,
0.0792901412208355));
#92048=CARTESIAN_POINT('Origin',(0.00184025653614732,-0.0345589643414859,
0.0652051429214359));
#92049=CARTESIAN_POINT('Ctrl Pts',(0.0109126308553257,-0.034193496108874,
0.0794624686483194));
#92050=CARTESIAN_POINT('Ctrl Pts',(0.0108393750585844,-0.0340836138581107,
0.0795009252198808));
#92051=CARTESIAN_POINT('Ctrl Pts',(0.0107653586332959,-0.03397388966435,
0.0795378474642542));
#92052=CARTESIAN_POINT('Ctrl Pts',(0.0106906794791397,-0.0338644633294062,
0.0795731944758687));
#92053=CARTESIAN_POINT('Ctrl Pts',(0.0109397083997648,-0.034193496108874,
0.0793524324459361));
#92054=CARTESIAN_POINT('Ctrl Pts',(0.0108679699370935,-0.0340836138581107,
0.0793912624008006));
#92055=CARTESIAN_POINT('Ctrl Pts',(0.0107954623914456,-0.03397388966435,
0.0794285892473656));
#92056=CARTESIAN_POINT('Ctrl Pts',(0.0107222817660344,-0.0338644633294062,
0.0794643714327629));
#92057=CARTESIAN_POINT('Ctrl Pts',(0.0109667859442039,-0.034193496108874,
0.0792423962435528));
#92058=CARTESIAN_POINT('Ctrl Pts',(0.0108965648156026,-0.0340836138581107,
0.0792815995817204));
#92059=CARTESIAN_POINT('Ctrl Pts',(0.0108255661495953,-0.03397388966435,
0.0793193310304769));
#92060=CARTESIAN_POINT('Ctrl Pts',(0.0107538840529292,-0.0338644633294062,
0.0793555483896571));
#92061=CARTESIAN_POINT('Ctrl Pts',(0.010993863488643,-0.034193496108874,
0.0791323600411695));
#92062=CARTESIAN_POINT('Ctrl Pts',(0.0109251596941117,-0.0340836138581107,
0.0791719367626402));
#92063=CARTESIAN_POINT('Ctrl Pts',(0.010855669907745,-0.03397388966435,
0.0792100728135884));
#92064=CARTESIAN_POINT('Ctrl Pts',(0.0107854863398239,-0.0338644633294062,
0.0792467253465512));
#92065=CARTESIAN_POINT('Origin',(0.00220592502735406,-0.0345610621863664,
0.0648923545487759));
#92066=CARTESIAN_POINT('Ctrl Pts',(0.0110246746444469,-0.0342436276873901,
0.0791161804221925));
#92067=CARTESIAN_POINT('Ctrl Pts',(0.0108373720621055,-0.0339430054201861,
0.0792255893846222));
#92068=CARTESIAN_POINT('Ctrl Pts',(0.0106423604554252,-0.0336441434784163,
0.0793205791297093));
#92069=CARTESIAN_POINT('Ctrl Pts',(0.0112377529694063,-0.0342436276873901,
0.0789854225259395));
#92070=CARTESIAN_POINT('Ctrl Pts',(0.0110553820024206,-0.0339430054201861,
0.0791028678698763));
#92071=CARTESIAN_POINT('Ctrl Pts',(0.0108646826677109,-0.0336441434784163,
0.0792062426354285));
#92072=CARTESIAN_POINT('Ctrl Pts',(0.00986777531919926,-0.0326943950436593,
0.0798909483516457));
#92073=CARTESIAN_POINT('Ctrl Pts',(0.00978865429122989,-0.0325844576448127,
0.0799149838455146));
#92074=CARTESIAN_POINT('Ctrl Pts',(0.0097090305703225,-0.0324744968375319,
0.0799373846878336));
#92075=CARTESIAN_POINT('Ctrl Pts',(0.00962900657090852,-0.0323646534831895,
0.0799581235844798));
#92076=CARTESIAN_POINT('Ctrl Pts',(0.00991499191592088,-0.0326943950436593,
0.0797879351458107));
#92077=CARTESIAN_POINT('Ctrl Pts',(0.00983729060299523,-0.0325844576448127,
0.0798126213728758));
#92078=CARTESIAN_POINT('Ctrl Pts',(0.00975907323937763,-0.0324744968375319,
0.0798357023564791));
#92079=CARTESIAN_POINT('Ctrl Pts',(0.00968044044961222,-0.0323646534831895,
0.0798571499062074));
#92080=CARTESIAN_POINT('Ctrl Pts',(0.0099622085126425,-0.0326943950436593,
0.0796849219399757));
#92081=CARTESIAN_POINT('Ctrl Pts',(0.00988592691476058,-0.0325844576448127,
0.0797102589002369));
#92082=CARTESIAN_POINT('Ctrl Pts',(0.00980911590843275,-0.0324744968375319,
0.0797340200251246));
#92083=CARTESIAN_POINT('Ctrl Pts',(0.00973187432831593,-0.0323646534831895,
0.079756176227935));
#92084=CARTESIAN_POINT('Ctrl Pts',(0.0100094251093641,-0.0326943950436593,
0.0795819087341407));
#92085=CARTESIAN_POINT('Ctrl Pts',(0.00993456322652593,-0.0325844576448127,
0.0796078964275981));
#92086=CARTESIAN_POINT('Ctrl Pts',(0.00985915857748787,-0.0324744968375319,
0.0796323376937701));
#92087=CARTESIAN_POINT('Ctrl Pts',(0.00978330820701964,-0.0323646534831895,
0.0796552025496625));
#92088=CARTESIAN_POINT('Origin',(0.00457127317689149,-0.0326395579068152,
0.0636764031143487));
#92089=CARTESIAN_POINT('Ctrl Pts',(0.0101257369732358,-0.0325229783203385,
0.0795401258895911));
#92090=CARTESIAN_POINT('Ctrl Pts',(0.0100514342070745,-0.032413025311208,
0.079567722791953));
#92091=CARTESIAN_POINT('Ctrl Pts',(0.00997657183301764,-0.0323031222247695,
0.0795937784605653));
#92092=CARTESIAN_POINT('Ctrl Pts',(0.00990124692215074,-0.0321934096636184,
0.0796182629037315));
#92093=CARTESIAN_POINT('Ctrl Pts',(0.0102277118930496,-0.0325229783203385,
0.0795895451002191));
#92094=CARTESIAN_POINT('Ctrl Pts',(0.0101527278841629,-0.032413025311208,
0.079618547724595));
#92095=CARTESIAN_POINT('Ctrl Pts',(0.0100771552915394,-0.0323031222247695,
0.0796459948096354));
#92096=CARTESIAN_POINT('Ctrl Pts',(0.0100010921588956,-0.0321934096636184,
0.07967185461344));
#92097=CARTESIAN_POINT('Ctrl Pts',(0.0103296868128634,-0.0325229783203385,
0.0796389643108472));
#92098=CARTESIAN_POINT('Ctrl Pts',(0.0102540215612513,-0.032413025311208,
0.0796693726572371));
#92099=CARTESIAN_POINT('Ctrl Pts',(0.0101777387500611,-0.0323031222247695,
0.0796982111587055));
#92100=CARTESIAN_POINT('Ctrl Pts',(0.0101009373956406,-0.0321934096636184,
0.0797254463231485));
#92101=CARTESIAN_POINT('Ctrl Pts',(0.0104316617326772,-0.0325229783203385,
0.0796883835214752));
#92102=CARTESIAN_POINT('Ctrl Pts',(0.0103553152383397,-0.032413025311208,
0.0797201975898791));
#92103=CARTESIAN_POINT('Ctrl Pts',(0.0102783222085829,-0.0323031222247695,
0.0797504275077756));
#92104=CARTESIAN_POINT('Ctrl Pts',(0.0102007826323855,-0.0321934096636184,
0.079779038032857));
#92105=CARTESIAN_POINT('Origin',(0.0041259267352345,-0.0326393375178154,
0.0638577421876095));
#92106=CARTESIAN_POINT('Ctrl Pts',(0.0100426911070143,-0.0327445246961877,
0.0795717998469266));
#92107=CARTESIAN_POINT('Ctrl Pts',(0.00983820458501583,-0.0324436878365475,
0.0796441726789962));
#92108=CARTESIAN_POINT('Ctrl Pts',(0.00962884757017125,-0.0321434074463188,
0.0797009371470741));
#92109=CARTESIAN_POINT('Ctrl Pts',(0.0102764973271794,-0.0327445246961877,
0.0794832862806662));
#92110=CARTESIAN_POINT('Ctrl Pts',(0.0100753491488722,-0.0324436878365475,
0.0795644772583946));
#92111=CARTESIAN_POINT('Ctrl Pts',(0.00986865677507285,-0.0321434074463188,
0.0796302862783996));
#92112=CARTESIAN_POINT('Ctrl Pts',(0.00950385681755172,-0.0321934096636184,
0.079989126135911));
#92113=CARTESIAN_POINT('Ctrl Pts',(0.00942333071739944,-0.0320835708272304,
0.0800081584405468));
#92114=CARTESIAN_POINT('Ctrl Pts',(0.00934245745310258,-0.0319739230346347,
0.0800255132222151));
#92115=CARTESIAN_POINT('Ctrl Pts',(0.00926134220050527,-0.0318646057455576,
0.0800411762178432));
#92116=CARTESIAN_POINT('Ctrl Pts',(0.00955744857340869,-0.0321934096636184,
0.0798892808131882));
#92117=CARTESIAN_POINT('Ctrl Pts',(0.00947829941807147,-0.0320835708272304,
0.0799090521899041));
#92118=CARTESIAN_POINT('Ctrl Pts',(0.00939878700484743,-0.0319739230346347,
0.0799271741107622));
#92119=CARTESIAN_POINT('Ctrl Pts',(0.00931901484379366,-0.0318646057455576,
0.0799436311975624));
#92120=CARTESIAN_POINT('Ctrl Pts',(0.00961104032926566,-0.0321934096636184,
0.0797894354904654));
#92121=CARTESIAN_POINT('Ctrl Pts',(0.0095332681187435,-0.0320835708272304,
0.0798099459392615));
#92122=CARTESIAN_POINT('Ctrl Pts',(0.00945511655659229,-0.0319739230346347,
0.0798288349993092));
#92123=CARTESIAN_POINT('Ctrl Pts',(0.00937668748708205,-0.0318646057455576,
0.0798460861772817));
#92124=CARTESIAN_POINT('Ctrl Pts',(0.00966463208512263,-0.0321934096636184,
0.0796895901677426));
#92125=CARTESIAN_POINT('Ctrl Pts',(0.00958823681941552,-0.0320835708272304,
0.0797108396886189));
#92126=CARTESIAN_POINT('Ctrl Pts',(0.00951144610833714,-0.0319739230346347,
0.0797304958878563));
#92127=CARTESIAN_POINT('Ctrl Pts',(0.00943436013037044,-0.0318646057455576,
0.0797485411570009));
#92128=CARTESIAN_POINT('Origin',(0.00460026649247057,-0.0326371942646895,
0.0637671874260098));
#92129=CARTESIAN_POINT('Ctrl Pts',(0.00978399678220021,-0.0320218834582328,
0.0796558591807856));
#92130=CARTESIAN_POINT('Ctrl Pts',(0.00972669409845655,-0.0319391099350611,
0.0796731380011153));
#92131=CARTESIAN_POINT('Ctrl Pts',(0.00966915632175085,-0.0318564869454879,
0.0796895115632053));
#92132=CARTESIAN_POINT('Ctrl Pts',(0.00961142647409324,-0.0317740741446459,
0.0797049718535495));
#92133=CARTESIAN_POINT('Ctrl Pts',(0.0098271544916287,-0.0320218834582328,
0.0796802362225375));
#92134=CARTESIAN_POINT('Ctrl Pts',(0.00976959810181152,-0.0319391099350611,
0.0796979642102892));
#92135=CARTESIAN_POINT('Ctrl Pts',(0.00971179975893409,-0.0318564869454879,
0.0797147827060062));
#92136=CARTESIAN_POINT('Ctrl Pts',(0.00965380270504909,-0.0317740741446459,
0.0797306833898253));
#92137=CARTESIAN_POINT('Ctrl Pts',(0.00987031220105719,-0.0320218834582328,
0.0797046132642893));
#92138=CARTESIAN_POINT('Ctrl Pts',(0.00981250210516649,-0.0319391099350611,
0.0797227904194631));
#92139=CARTESIAN_POINT('Ctrl Pts',(0.00975444319611733,-0.0318564869454879,
0.0797400538488072));
#92140=CARTESIAN_POINT('Ctrl Pts',(0.00969617893600494,-0.0317740741446459,
0.0797563949261011));
#92141=CARTESIAN_POINT('Ctrl Pts',(0.00991346991048568,-0.0320218834582328,
0.0797289903060412));
#92142=CARTESIAN_POINT('Ctrl Pts',(0.00985540610852146,-0.0319391099350611,
0.079747616628637));
#92143=CARTESIAN_POINT('Ctrl Pts',(0.00979708663330056,-0.0318564869454879,
0.0797653249916081));
#92144=CARTESIAN_POINT('Ctrl Pts',(0.00973855516696078,-0.0317740741446459,
0.0797821064623769));
#92145=CARTESIAN_POINT('Origin',(0.00416763752318638,-0.0326352985531528,
0.0639731718762183));
#92146=CARTESIAN_POINT('Ctrl Pts',(0.00969308699300744,-0.0322357242816073,
0.0796831191424922));
#92147=CARTESIAN_POINT('Ctrl Pts',(0.00951686432451163,-0.0319819883628706,
0.0797330994650554));
#92148=CARTESIAN_POINT('Ctrl Pts',(0.00933781840221456,-0.0317295851069886,
0.0797717649437681));
#92149=CARTESIAN_POINT('Ctrl Pts',(0.00993206117888817,-0.0322357242816073,
0.079609693408021));
#92150=CARTESIAN_POINT('Ctrl Pts',(0.00975817702480558,-0.0319819883628706,
0.0796672847484662));
#92151=CARTESIAN_POINT('Ctrl Pts',(0.00958098056679106,-0.0317295851069886,
0.079713694626751));
#92152=CARTESIAN_POINT('Ctrl Pts',(0.0107855108621147,-0.0335235895815127,
0.0792467123972283));
#92153=CARTESIAN_POINT('Ctrl Pts',(0.0107153445814646,-0.0334144449262719,
0.0792833563328182));
#92154=CARTESIAN_POINT('Ctrl Pts',(0.0106443406521271,-0.0333049234473133,
0.0793185927852983));
#92155=CARTESIAN_POINT('Ctrl Pts',(0.0105725857849066,-0.0331951640388588,
0.0793523684737116));
#92156=CARTESIAN_POINT('Ctrl Pts',(0.0108928756618168,-0.0335235895815127,
0.0792829611526807));
#92157=CARTESIAN_POINT('Ctrl Pts',(0.0108222103456806,-0.0334144449262719,
0.0793210831761204));
#92158=CARTESIAN_POINT('Ctrl Pts',(0.0107506762713432,-0.0333049234473133,
0.0793577891048965));
#92159=CARTESIAN_POINT('Ctrl Pts',(0.0106783606572928,-0.0331951640388588,
0.0793930237176365));
#92160=CARTESIAN_POINT('Ctrl Pts',(0.0110002404615188,-0.0335235895815127,
0.0793192099081332));
#92161=CARTESIAN_POINT('Ctrl Pts',(0.0109290761098966,-0.0334144449262719,
0.0793588100194225));
#92162=CARTESIAN_POINT('Ctrl Pts',(0.0108570118905593,-0.0333049234473133,
0.0793969854244946));
#92163=CARTESIAN_POINT('Ctrl Pts',(0.010784135529679,-0.0331951640388588,
0.0794336789615614));
#92164=CARTESIAN_POINT('Ctrl Pts',(0.0111076052612209,-0.0335235895815127,
0.0793554586635856));
#92165=CARTESIAN_POINT('Ctrl Pts',(0.0110359418741126,-0.0334144449262719,
0.0793965368627246));
#92166=CARTESIAN_POINT('Ctrl Pts',(0.0109633475097754,-0.0333049234473133,
0.0794361817440927));
#92167=CARTESIAN_POINT('Ctrl Pts',(0.0108899104020652,-0.0331951640388588,
0.0794743342054864));
#92168=CARTESIAN_POINT('Origin',(0.00417037681106416,-0.0326434571770334,
0.0639639780016505));
#92169=CARTESIAN_POINT('Ctrl Pts',(0.0105729478769377,-0.0336938721132457,
0.0796290334902976));
#92170=CARTESIAN_POINT('Ctrl Pts',(0.0105408772757806,-0.0336474569764991,
0.0796433692697655));
#92171=CARTESIAN_POINT('Ctrl Pts',(0.0105086410537226,-0.033601104548885,
0.0796573286400577));
#92172=CARTESIAN_POINT('Ctrl Pts',(0.0104270263545652,-0.0334837508643204,
0.0796926705546524));
#92173=CARTESIAN_POINT('Ctrl Pts',(0.0103444002404054,-0.033366026476049,
0.0797255785370371));
#92174=CARTESIAN_POINT('Ctrl Pts',(0.0106747477336468,-0.0336938721132457,
0.0793046774691523));
#92175=CARTESIAN_POINT('Ctrl Pts',(0.0106445756959143,-0.0336474569764991,
0.0793196091169623));
#92176=CARTESIAN_POINT('Ctrl Pts',(0.0106142309317989,-0.033601104548885,
0.0793341865398494));
#92177=CARTESIAN_POINT('Ctrl Pts',(0.0105374049690721,-0.0334837508643204,
0.0793710932214476));
#92178=CARTESIAN_POINT('Ctrl Pts',(0.0104595191211943,-0.033366026476049,
0.0794057071838885));
#92179=CARTESIAN_POINT('Ctrl Pts',(0.0106747477336484,-0.0336938721132426,
0.0793046774691665));
#92180=CARTESIAN_POINT('Ctrl Pts',(0.0106445756959201,-0.0336474569765026,
0.0793196091169743));
#92181=CARTESIAN_POINT('Ctrl Pts',(0.0106142309318089,-0.0336011045488949,
0.0793341865398594));
#92182=CARTESIAN_POINT('Ctrl Pts',(0.0105380448247086,-0.0334847282606778,
0.0793707858390697));
#92183=CARTESIAN_POINT('Ctrl Pts',(0.0104608161336227,-0.0333679869945434,
0.0794051305750701));
#92184=CARTESIAN_POINT('Ctrl Pts',(0.010674747733645,-0.0336938721132429,
0.0793046774691532));
#92185=CARTESIAN_POINT('Ctrl Pts',(0.0105668391742669,-0.0335278710435085,
0.0793580796496291));
#92186=CARTESIAN_POINT('Ctrl Pts',(0.0104572938983739,-0.0333620469224321,
0.0794080790589757));
#92187=CARTESIAN_POINT('Ctrl Pts',(0.0103460491095634,-0.0331951640388602,
0.0794546823422361));
#92188=CARTESIAN_POINT('Ctrl Pts',(0.0107490578005851,-0.0336938721132429,
0.0792658696893323));
#92189=CARTESIAN_POINT('Ctrl Pts',(0.0106419616473445,-0.0335278710435085,
0.079320827484552));
#92190=CARTESIAN_POINT('Ctrl Pts',(0.0105331797081127,-0.0333620469224321,
0.079372407438226));
#92191=CARTESIAN_POINT('Ctrl Pts',(0.0104226493032177,-0.0331951640388602,
0.0794206171084133));
#92192=CARTESIAN_POINT('Ctrl Pts',(0.0108233678675252,-0.0336938721132429,
0.0792270619095114));
#92193=CARTESIAN_POINT('Ctrl Pts',(0.0107170841204222,-0.0335278710435085,
0.0792835753194749));
#92194=CARTESIAN_POINT('Ctrl Pts',(0.0106090655178514,-0.0333620469224321,
0.0793367358174764));
#92195=CARTESIAN_POINT('Ctrl Pts',(0.010499249496872,-0.0331951640388602,
0.0793865518745905));
#92196=CARTESIAN_POINT('Ctrl Pts',(0.0108976779344653,-0.0336938721132429,
0.0791882541296904));
#92197=CARTESIAN_POINT('Ctrl Pts',(0.0107922065934999,-0.0335278710435085,
0.0792463231543978));
#92198=CARTESIAN_POINT('Ctrl Pts',(0.0106849513275902,-0.0333620469224321,
0.0793010641967267));
#92199=CARTESIAN_POINT('Ctrl Pts',(0.0105758496905263,-0.0331951640388602,
0.0793524866407678));
#92200=CARTESIAN_POINT('Ctrl Pts',(0.0103793061266113,-0.0332451089994433,
0.0794406272582177));
#92201=CARTESIAN_POINT('Ctrl Pts',(0.0101797668549345,-0.0329451141710259,
0.0795256957351628));
#92202=CARTESIAN_POINT('Ctrl Pts',(0.00997438674782287,-0.0326442513127503,
0.0795954924278775));
#92203=CARTESIAN_POINT('Ctrl Pts',(0.0106070938733704,-0.0332451089994433,
0.0793376090927011));
#92204=CARTESIAN_POINT('Ctrl Pts',(0.0104114399953744,-0.0329451141710259,
0.0794312687250738));
#92205=CARTESIAN_POINT('Ctrl Pts',(0.0102092871230025,-0.0326442513127503,
0.079509924830386));
#92206=CARTESIAN_POINT('Origin',(0.00458385954554729,-0.0326401908831853,
0.0637120898756703));
#92207=CARTESIAN_POINT('Origin',(0.00412306332237759,-0.0326396682857103,
0.0638497115031866));
#92208=CARTESIAN_POINT('Ctrl Pts',(0.010224811076733,-0.0331951640388588,
0.0797701136670258));
#92209=CARTESIAN_POINT('Ctrl Pts',(0.0101474053713548,-0.0330855618127431,
0.0797990510929201));
#92210=CARTESIAN_POINT('Ctrl Pts',(0.0100693457780804,-0.0329757224171935,
0.0798264095355998));
#92211=CARTESIAN_POINT('Ctrl Pts',(0.00999073053843142,-0.0328657861694599,
0.0798521490576809));
#92212=CARTESIAN_POINT('Ctrl Pts',(0.010265466288291,-0.0331951640388588,
0.0796643388788503));
#92213=CARTESIAN_POINT('Ctrl Pts',(0.0101895174168088,-0.0330855618127431,
0.0796938362481042));
#92214=CARTESIAN_POINT('Ctrl Pts',(0.0101129041345685,-0.0329757224171935,
0.0797217851480688));
#92215=CARTESIAN_POINT('Ctrl Pts',(0.0100357227939136,-0.0328657861694599,
0.0797481449760927));
#92216=CARTESIAN_POINT('Ctrl Pts',(0.010306121499849,-0.0331951640388588,
0.0795585640906749));
#92217=CARTESIAN_POINT('Ctrl Pts',(0.0102316294622629,-0.0330855618127431,
0.0795886214032884));
#92218=CARTESIAN_POINT('Ctrl Pts',(0.0101564624910565,-0.0329757224171935,
0.0796171607605378));
#92219=CARTESIAN_POINT('Ctrl Pts',(0.0100807150493959,-0.0328657861694599,
0.0796441408945044));
#92220=CARTESIAN_POINT('Ctrl Pts',(0.0103467767114071,-0.0331951640388588,
0.0794527893024995));
#92221=CARTESIAN_POINT('Ctrl Pts',(0.010273741507717,-0.0330855618127431,
0.0794834065584725));
#92222=CARTESIAN_POINT('Ctrl Pts',(0.0102000208475445,-0.0329757224171935,
0.0795125363730068));
#92223=CARTESIAN_POINT('Ctrl Pts',(0.0101257073048781,-0.0328657861694599,
0.0795401368129162));
#92224=CARTESIAN_POINT('Ctrl Pts',(0.0104602346180054,-0.0330240426238156,
0.0794037863342683));
#92225=CARTESIAN_POINT('Ctrl Pts',(0.0103878585927352,-0.0329142774063509,
0.0794359732427163));
#92226=CARTESIAN_POINT('Ctrl Pts',(0.0103147810920695,-0.0328043479726686,
0.0794666799828973));
#92227=CARTESIAN_POINT('Ctrl Pts',(0.0102410946503782,-0.0326943950436594,
0.0794958646389747));
#92228=CARTESIAN_POINT('Ctrl Pts',(0.010565111337429,-0.0330240426238156,
0.0794467049748362));
#92229=CARTESIAN_POINT('Ctrl Pts',(0.0104921440660714,-0.0329142774063509,
0.0794803366622707));
#92230=CARTESIAN_POINT('Ctrl Pts',(0.0104184451569431,-0.0328043479726686,
0.079512476679005));
#92231=CARTESIAN_POINT('Ctrl Pts',(0.0103441078899177,-0.0326943950436594,
0.0795430812511449));
#92232=CARTESIAN_POINT('Ctrl Pts',(0.0106699880568526,-0.0330240426238156,
0.0794896236154041));
#92233=CARTESIAN_POINT('Ctrl Pts',(0.0105964295394076,-0.0329142774063509,
0.0795247000818251));
#92234=CARTESIAN_POINT('Ctrl Pts',(0.0105221092218167,-0.0328043479726686,
0.0795582733751128));
#92235=CARTESIAN_POINT('Ctrl Pts',(0.0104471211294572,-0.0326943950436594,
0.0795902978633152));
#92236=CARTESIAN_POINT('Ctrl Pts',(0.0107748647762762,-0.0330240426238156,
0.079532542255972));
#92237=CARTESIAN_POINT('Ctrl Pts',(0.0107007150127437,-0.0329142774063509,
0.0795690635013796));
#92238=CARTESIAN_POINT('Ctrl Pts',(0.0106257732866902,-0.0328043479726686,
0.0796040700712205));
#92239=CARTESIAN_POINT('Ctrl Pts',(0.0105501343689966,-0.0326943950436594,
0.0796375144754854));
#92240=CARTESIAN_POINT('Origin',(0.0125018286955665,-0.0391228853390791,
0.0854067014330336));
#92241=CARTESIAN_POINT('Ctrl Pts',(0.0123565016694387,-0.0352722978779621,
0.0780446438062154));
#92242=CARTESIAN_POINT('Ctrl Pts',(0.0123434509783258,-0.0352466642097234,
0.0780583102666033));
#92243=CARTESIAN_POINT('Ctrl Pts',(0.0123304686144099,-0.0352210183808309,
0.0780720186975263));
#92244=CARTESIAN_POINT('Ctrl Pts',(0.0123175545062067,-0.0351953608940152,
0.0780857699489101));
#92245=CARTESIAN_POINT('Origin',(0.0157726898688784,-0.0352456003065063,
0.0815573922146694));
#92246=CARTESIAN_POINT('Ctrl Pts',(0.0122302082862127,-0.035024121149334,
0.0781747415919819));
#92247=CARTESIAN_POINT('Ctrl Pts',(0.0121747691234912,-0.0349144232867422,
0.0782313059251637));
#92248=CARTESIAN_POINT('Ctrl Pts',(0.0121181275526273,-0.0348045283677513,
0.0782867581477673));
#92249=CARTESIAN_POINT('Ctrl Pts',(0.0120603534811807,-0.0346945769586887,
0.0783410245327702));
#92250=CARTESIAN_POINT('Ctrl Pts',(0.0123435196248492,-0.035024121149334,
0.0781760386424488));
#92251=CARTESIAN_POINT('Ctrl Pts',(0.0122880625957901,-0.0349144232867422,
0.0782341637927904));
#92252=CARTESIAN_POINT('Ctrl Pts',(0.0122313708846903,-0.0348045283677513,
0.0782911773974682));
#92253=CARTESIAN_POINT('Ctrl Pts',(0.0121735143889105,-0.0346945769586887,
0.0783470037271379));
#92254=CARTESIAN_POINT('Ctrl Pts',(0.0124568309634857,-0.035024121149334,
0.0781773356929156));
#92255=CARTESIAN_POINT('Ctrl Pts',(0.0124013560680891,-0.0349144232867422,
0.0782370216604171));
#92256=CARTESIAN_POINT('Ctrl Pts',(0.0123446142167533,-0.0348045283677513,
0.0782955966471692));
#92257=CARTESIAN_POINT('Ctrl Pts',(0.0122866752966402,-0.0346945769586887,
0.0783529829215056));
#92258=CARTESIAN_POINT('Ctrl Pts',(0.0125701423021222,-0.035024121149334,
0.0781786327433825));
#92259=CARTESIAN_POINT('Ctrl Pts',(0.012514649540388,-0.0349144232867422,
0.0782398795280439));
#92260=CARTESIAN_POINT('Ctrl Pts',(0.0124578575488162,-0.0348045283677513,
0.0783000158968701));
#92261=CARTESIAN_POINT('Ctrl Pts',(0.01239983620437,-0.0346945769586887,
0.0783589621158733));
#92262=CARTESIAN_POINT('Origin',(0.000698110229997924,-0.0345629067942725,
0.0659813167131262));
#92263=CARTESIAN_POINT('Ctrl Pts',(0.0121463145442708,-0.0351970973651605,
0.0785082972892153));
#92264=CARTESIAN_POINT('Ctrl Pts',(0.0120859362418675,-0.0350869349321769,
0.0785640240234439));
#92265=CARTESIAN_POINT('Ctrl Pts',(0.0120243493948586,-0.0349764985129726,
0.0786185416896035));
#92266=CARTESIAN_POINT('Ctrl Pts',(0.011961629633163,-0.0348659306849652,
0.0786717749616932));
#92267=CARTESIAN_POINT('Ctrl Pts',(0.012145468537714,-0.0351970973651605,
0.0784260795604525));
#92268=CARTESIAN_POINT('Ctrl Pts',(0.012086229250518,-0.0350869349321769,
0.0784817945744068));
#92269=CARTESIAN_POINT('Ctrl Pts',(0.0120257826059213,-0.0349764985129726,
0.0785363241900781));
#92270=CARTESIAN_POINT('Ctrl Pts',(0.0119642027557658,-0.0348659306849652,
0.0785895931529392));
#92271=CARTESIAN_POINT('Ctrl Pts',(0.0121446225311572,-0.0351970973651605,
0.0783438618316897));
#92272=CARTESIAN_POINT('Ctrl Pts',(0.0120865222591685,-0.0350869349321769,
0.0783995651253697));
#92273=CARTESIAN_POINT('Ctrl Pts',(0.0120272158169839,-0.0349764985129726,
0.0784541066905527));
#92274=CARTESIAN_POINT('Ctrl Pts',(0.0119667758783686,-0.0348659306849652,
0.0785074113441852));
#92275=CARTESIAN_POINT('Ctrl Pts',(0.0121437765246004,-0.0351970973651605,
0.0782616441029269));
#92276=CARTESIAN_POINT('Ctrl Pts',(0.0120868152678189,-0.0350869349321769,
0.0783173356763326));
#92277=CARTESIAN_POINT('Ctrl Pts',(0.0120286490280466,-0.0349764985129726,
0.0783718891910273));
#92278=CARTESIAN_POINT('Ctrl Pts',(0.0119693490009714,-0.0348659306849652,
0.0784252295354313));
#92279=CARTESIAN_POINT('Origin',(0.00108299337951375,-0.0345637187966319,
0.0656928893953538));
#92280=CARTESIAN_POINT('Ctrl Pts',(0.0121685208140405,-0.0352450361861253,
0.0782387913236483));
#92281=CARTESIAN_POINT('Ctrl Pts',(0.0120143095227472,-0.0349452761023765,
0.0783913411400379));
#92282=CARTESIAN_POINT('Ctrl Pts',(0.0118490456534183,-0.0346444289983475,
0.0785318417533363));
#92283=CARTESIAN_POINT('Ctrl Pts',(0.0123423891770701,-0.0352450361861253,
0.0780591533757158));
#92284=CARTESIAN_POINT('Ctrl Pts',(0.012194953041984,-0.0349452761023765,
0.0782182607448527));
#92285=CARTESIAN_POINT('Ctrl Pts',(0.0120359511396659,-0.0346444289983475,
0.0783658106140565));
#92286=CARTESIAN_POINT('Ctrl Pts',(0.0119693903360891,-0.0345231616327822,
0.0784246437013716));
#92287=CARTESIAN_POINT('Ctrl Pts',(0.011910470390883,-0.0344132092796975,
0.0784776499954391));
#92288=CARTESIAN_POINT('Ctrl Pts',(0.0118504570922933,-0.0343032738558974,
0.0785294348420343));
#92289=CARTESIAN_POINT('Ctrl Pts',(0.0117894290236758,-0.0341934961088741,
0.0785799338681956));
#92290=CARTESIAN_POINT('Ctrl Pts',(0.0120823966146316,-0.0345231616327822,
0.0784330530502766));
#92291=CARTESIAN_POINT('Ctrl Pts',(0.0120233607583902,-0.0344132092796975,
0.0784876169767936));
#92292=CARTESIAN_POINT('Ctrl Pts',(0.0119631993363471,-0.0343032738558974,
0.0785409569779434));
#92293=CARTESIAN_POINT('Ctrl Pts',(0.0119019911726559,-0.0341934961088741,
0.0785930066932924));
#92294=CARTESIAN_POINT('Ctrl Pts',(0.012195402893174,-0.0345231616327822,
0.0784414623991816));
#92295=CARTESIAN_POINT('Ctrl Pts',(0.0121362511258975,-0.0344132092796975,
0.0784975839581482));
#92296=CARTESIAN_POINT('Ctrl Pts',(0.012075941580401,-0.0343032738558974,
0.0785524791138525));
#92297=CARTESIAN_POINT('Ctrl Pts',(0.0120145533216359,-0.0341934961088741,
0.0786060795183893));
#92298=CARTESIAN_POINT('Ctrl Pts',(0.0123084091717165,-0.0345231616327822,
0.0784498717480865));
#92299=CARTESIAN_POINT('Ctrl Pts',(0.0122491414934047,-0.0344132092796975,
0.0785075509395027));
#92300=CARTESIAN_POINT('Ctrl Pts',(0.0121886838244549,-0.0343032738558974,
0.0785640012497616));
#92301=CARTESIAN_POINT('Ctrl Pts',(0.012127115470616,-0.0341934961088741,
0.0786191523434861));
#92302=CARTESIAN_POINT('Origin',(0.000689785054019144,-0.0345625596229105,
0.0659725309447745));
#92303=CARTESIAN_POINT('Ctrl Pts',(0.0118586900372337,-0.0346945769586886,
0.0788457920946348));
#92304=CARTESIAN_POINT('Ctrl Pts',(0.0117939796488334,-0.0345846629178476,
0.0788972610124152));
#92305=CARTESIAN_POINT('Ctrl Pts',(0.0117281938516594,-0.0344746925055161,
0.0789474005369592));
#92306=CARTESIAN_POINT('Ctrl Pts',(0.0116614172033764,-0.0343648066260528,
0.0789961467718455));
#92307=CARTESIAN_POINT('Ctrl Pts',(0.0118646692268936,-0.0346945769586886,
0.078732631276002));
#92308=CARTESIAN_POINT('Ctrl Pts',(0.0118015182517676,-0.0345846629178476,
0.0787841825900379));
#92309=CARTESIAN_POINT('Ctrl Pts',(0.0117372904302988,-0.0344746925055161,
0.0788344367729368));
#92310=CARTESIAN_POINT('Ctrl Pts',(0.0116720683245006,-0.0343648066260528,
0.07888332977312));
#92311=CARTESIAN_POINT('Ctrl Pts',(0.0118706484165536,-0.0346945769586886,
0.0786194704573692));
#92312=CARTESIAN_POINT('Ctrl Pts',(0.0118090568547018,-0.0345846629178476,
0.0786711041676606));
#92313=CARTESIAN_POINT('Ctrl Pts',(0.0117463870089381,-0.0344746925055161,
0.0787214730089145));
#92314=CARTESIAN_POINT('Ctrl Pts',(0.0116827194456247,-0.0343648066260528,
0.0787705127743945));
#92315=CARTESIAN_POINT('Ctrl Pts',(0.0118766276062136,-0.0346945769586886,
0.0785063096387363));
#92316=CARTESIAN_POINT('Ctrl Pts',(0.011816595457636,-0.0345846629178476,
0.0785580257452832));
#92317=CARTESIAN_POINT('Ctrl Pts',(0.0117554835875775,-0.034474692505516,
0.0786085092448922));
#92318=CARTESIAN_POINT('Ctrl Pts',(0.0116933705667488,-0.0343648066260528,
0.0786576957756689));
#92319=CARTESIAN_POINT('Origin',(0.00104501336031176,-0.0345626446730462,
0.0656484861437726));
#92320=CARTESIAN_POINT('Ctrl Pts',(0.0118765206184609,-0.0346945769586885,
0.0785083344652383));
#92321=CARTESIAN_POINT('Ctrl Pts',(0.011785233558106,-0.0345275153362891,
0.0785869370740706));
#92322=CARTESIAN_POINT('Ctrl Pts',(0.0116914509065426,-0.0343603235965159,
0.0786626891195394));
#92323=CARTESIAN_POINT('Ctrl Pts',(0.0115954533610552,-0.034193496108874,
0.0787353706831235));
#92324=CARTESIAN_POINT('Ctrl Pts',(0.0119388449890012,-0.0346945769586885,
0.078452265746972));
#92325=CARTESIAN_POINT('Ctrl Pts',(0.0118487323103991,-0.0345275153362891,
0.0785321737646985));
#92326=CARTESIAN_POINT('Ctrl Pts',(0.0117560832904355,-0.0343603235965159,
0.0786092684899324));
#92327=CARTESIAN_POINT('Ctrl Pts',(0.0116611753326362,-0.034193496108874,
0.0786833259832705));
#92328=CARTESIAN_POINT('Ctrl Pts',(0.0120011693595415,-0.0346945769586885,
0.0783961970287057));
#92329=CARTESIAN_POINT('Ctrl Pts',(0.0119122310626921,-0.0345275153362891,
0.0784774104553265));
#92330=CARTESIAN_POINT('Ctrl Pts',(0.0118207156743284,-0.0343603235965159,
0.0785558478603254));
#92331=CARTESIAN_POINT('Ctrl Pts',(0.0117268973042172,-0.034193496108874,
0.0786312812834176));
#92332=CARTESIAN_POINT('Ctrl Pts',(0.0120634937300818,-0.0346945769586885,
0.0783401283104393));
#92333=CARTESIAN_POINT('Ctrl Pts',(0.0119757298149852,-0.0345275153362891,
0.0784226471459544));
#92334=CARTESIAN_POINT('Ctrl Pts',(0.0118853480582213,-0.0343603235965159,
0.0785024272307183));
#92335=CARTESIAN_POINT('Ctrl Pts',(0.0117926192757981,-0.034193496108874,
0.0785792365835646));
#92336=CARTESIAN_POINT('Ctrl Pts',(0.0116933949579953,-0.0340223579322365,
0.0786576757501994));
#92337=CARTESIAN_POINT('Ctrl Pts',(0.0116312223528886,-0.0339125849573552,
0.0787069100201677));
#92338=CARTESIAN_POINT('Ctrl Pts',(0.011568074400768,-0.0338030433565217,
0.0787548228653281));
#92339=CARTESIAN_POINT('Ctrl Pts',(0.0115040372887651,-0.033693872113232,
0.0788013601718708));
#92340=CARTESIAN_POINT('Ctrl Pts',(0.0118056504105315,-0.0340223579322365,
0.0786731642364631));
#92341=CARTESIAN_POINT('Ctrl Pts',(0.0117432641788035,-0.0339125849573552,
0.0787239468018964));
#92342=CARTESIAN_POINT('Ctrl Pts',(0.0116798707040562,-0.0338030433565217,
0.0787734024329777));
#92343=CARTESIAN_POINT('Ctrl Pts',(0.0116155566622982,-0.033693872113232,
0.0788214750707676));
#92344=CARTESIAN_POINT('Ctrl Pts',(0.0119179058630677,-0.0340223579322365,
0.0786886527227268));
#92345=CARTESIAN_POINT('Ctrl Pts',(0.0118553060047185,-0.0339125849573552,
0.078740983583625));
#92346=CARTESIAN_POINT('Ctrl Pts',(0.0117916670073445,-0.0338030433565217,
0.0787919820006274));
#92347=CARTESIAN_POINT('Ctrl Pts',(0.0117270760358313,-0.033693872113232,
0.0788415899696644));
#92348=CARTESIAN_POINT('Ctrl Pts',(0.0120301613156039,-0.0340223579322365,
0.0787041412089905));
#92349=CARTESIAN_POINT('Ctrl Pts',(0.0119673478306335,-0.0339125849573552,
0.0787580203653537));
#92350=CARTESIAN_POINT('Ctrl Pts',(0.0119034633106328,-0.0338030433565217,
0.0788105615682771));
#92351=CARTESIAN_POINT('Ctrl Pts',(0.0118385954093644,-0.033693872113232,
0.0788617048685612));
#92352=CARTESIAN_POINT('Origin',(0.000768716151143632,-0.0345589643415323,
0.0660632103798417));
#92353=CARTESIAN_POINT('Ctrl Pts',(0.0115564688245381,-0.034193496108874,
0.079071042825514));
#92354=CARTESIAN_POINT('Ctrl Pts',(0.0114886105581001,-0.0340836138581107,
0.079118377541405));
#92355=CARTESIAN_POINT('Ctrl Pts',(0.0114198053587104,-0.03397388966435,
0.0791642853607716));
#92356=CARTESIAN_POINT('Ctrl Pts',(0.0113501452272528,-0.0338644633294063,
0.0792087134305122));
#92357=CARTESIAN_POINT('Ctrl Pts',(0.0115695416613978,-0.034193496108874,
0.0789584805752507));
#92358=CARTESIAN_POINT('Ctrl Pts',(0.0115032355617342,-0.0340836138581107,
0.0790059955578207));
#92359=CARTESIAN_POINT('Ctrl Pts',(0.0114359780541195,-0.03397388966435,
0.0790521156762053));
#92360=CARTESIAN_POINT('Ctrl Pts',(0.0113678591767975,-0.0338644633294063,
0.0790967876728002));
#92361=CARTESIAN_POINT('Ctrl Pts',(0.0115826144982575,-0.034193496108874,
0.0788459183249875));
#92362=CARTESIAN_POINT('Ctrl Pts',(0.0115178605653684,-0.0340836138581107,
0.0788936135742363));
#92363=CARTESIAN_POINT('Ctrl Pts',(0.0114521507495286,-0.03397388966435,
0.078939945991639));
#92364=CARTESIAN_POINT('Ctrl Pts',(0.0113855731263423,-0.0338644633294063,
0.0789848619150882));
#92365=CARTESIAN_POINT('Ctrl Pts',(0.0115956873351173,-0.034193496108874,
0.0787333560747242));
#92366=CARTESIAN_POINT('Ctrl Pts',(0.0115324855690025,-0.0340836138581107,
0.078781231590652));
#92367=CARTESIAN_POINT('Ctrl Pts',(0.0114683234449377,-0.03397388966435,
0.0788277763070727));
#92368=CARTESIAN_POINT('Ctrl Pts',(0.011403287075887,-0.0338644633294063,
0.0788729361573761));
#92369=CARTESIAN_POINT('Origin',(0.00109229845921002,-0.0345610621864549,
0.0657070580230232));
#92370=CARTESIAN_POINT('Ctrl Pts',(0.0116242276917907,-0.0342436276873901,
0.0787134423750888));
#92371=CARTESIAN_POINT('Ctrl Pts',(0.0114521146252978,-0.0339430054201861,
0.0788454638534707));
#92372=CARTESIAN_POINT('Ctrl Pts',(0.0112705461152906,-0.0336441434784162,
0.0789641460112935));
#92373=CARTESIAN_POINT('Ctrl Pts',(0.0118192375205629,-0.0342436276873901,
0.0785570097484337));
#92374=CARTESIAN_POINT('Ctrl Pts',(0.0116530244078461,-0.0339430054201861,
0.0786963861437548));
#92375=CARTESIAN_POINT('Ctrl Pts',(0.0114767850879853,-0.0336441434784162,
0.0788228467326618));
#92376=CARTESIAN_POINT('Ctrl Pts',(0.0114033097818316,-0.0335235895815127,
0.0788729202367046));
#92377=CARTESIAN_POINT('Ctrl Pts',(0.0113382894862,-0.0334144449262718,
0.0789180693907584));
#92378=CARTESIAN_POINT('Ctrl Pts',(0.011272261742582,-0.0333049234473132,
0.0789619271453457));
#92379=CARTESIAN_POINT('Ctrl Pts',(0.0112053059001663,-0.0331951640388588,
0.0790044297719002));
#92380=CARTESIAN_POINT('Ctrl Pts',(0.0115143711517532,-0.0335235895815127,
0.0788954267823756));
#92381=CARTESIAN_POINT('Ctrl Pts',(0.0114490410092091,-0.0334144449262718,
0.0789421049148461));
#92382=CARTESIAN_POINT('Ctrl Pts',(0.0113826714751586,-0.0333049234473132,
0.078987487003257));
#92383=CARTESIAN_POINT('Ctrl Pts',(0.0113153421592727,-0.0331951640388588,
0.0790315073302976));
#92384=CARTESIAN_POINT('Ctrl Pts',(0.0116254325216747,-0.0335235895815127,
0.0789179333280467));
#92385=CARTESIAN_POINT('Ctrl Pts',(0.0115597925322182,-0.0334144449262718,
0.0789661404389338));
#92386=CARTESIAN_POINT('Ctrl Pts',(0.0114930812077352,-0.0333049234473132,
0.0790130468611683));
#92387=CARTESIAN_POINT('Ctrl Pts',(0.011425378418379,-0.0331951640388588,
0.079058584888695));
#92388=CARTESIAN_POINT('Ctrl Pts',(0.0117364938915962,-0.0335235895815127,
0.0789404398737177));
#92389=CARTESIAN_POINT('Ctrl Pts',(0.0116705440552272,-0.0334144449262718,
0.0789901759630215));
#92390=CARTESIAN_POINT('Ctrl Pts',(0.0116034909403119,-0.0333049234473132,
0.0790386067190796));
#92391=CARTESIAN_POINT('Ctrl Pts',(0.0115354146774854,-0.0331951640388588,
0.0790856624470924));
#92392=CARTESIAN_POINT('Origin',(0.00292490351896382,-0.032643457177084,
0.0645397909075513));
#92393=CARTESIAN_POINT('Ctrl Pts',(0.011240340458136,-0.0336938721132453,
0.0792788678200312));
#92394=CARTESIAN_POINT('Ctrl Pts',(0.0112103194928445,-0.0336474569764989,
0.0792971100697413));
#92395=CARTESIAN_POINT('Ctrl Pts',(0.0111800870360433,-0.033601104548885,
0.0793149996361777));
#92396=CARTESIAN_POINT('Ctrl Pts',(0.0111035454096023,-0.0334837508643202,
0.0793602919033715));
#92397=CARTESIAN_POINT('Ctrl Pts',(0.0110256952908741,-0.0333660264760487,
0.0794032961945505));
#92398=CARTESIAN_POINT('Ctrl Pts',(0.0113006850036129,-0.0336938721132453,
0.0789443105377739));
#92399=CARTESIAN_POINT('Ctrl Pts',(0.0112726223131125,-0.0336474569764989,
0.0789629060041331));
#92400=CARTESIAN_POINT('Ctrl Pts',(0.0112443438620732,-0.033601104548885,
0.078981171687095));
#92401=CARTESIAN_POINT('Ctrl Pts',(0.011172749328754,-0.0334837508643202,
0.0790274161948155));
#92402=CARTESIAN_POINT('Ctrl Pts',(0.0110998159138892,-0.0333660264760487,
0.0790715189009874));
#92403=CARTESIAN_POINT('Ctrl Pts',(0.0113006850036153,-0.0336938721132426,
0.0789443105377889));
#92404=CARTESIAN_POINT('Ctrl Pts',(0.0112726223131186,-0.0336474569765026,
0.0789629060041457));
#92405=CARTESIAN_POINT('Ctrl Pts',(0.0112443438620832,-0.0336011045488949,
0.078981171687105));
#92406=CARTESIAN_POINT('Ctrl Pts',(0.0111733456137093,-0.0334847282606778,
0.0790270310410649));
#92407=CARTESIAN_POINT('Ctrl Pts',(0.0111010304307386,-0.0333679869945434,
0.0790707842801414));
#92408=CARTESIAN_POINT('Ctrl Pts',(0.0113006850036114,-0.0336938721132429,
0.0789443105377748));
#92409=CARTESIAN_POINT('Ctrl Pts',(0.0112003204034131,-0.0335278710435085,
0.0790108161547833));
#92410=CARTESIAN_POINT('Ctrl Pts',(0.0110979055123899,-0.0333620469224321,
0.0790741509675024));
#92411=CARTESIAN_POINT('Ctrl Pts',(0.0109933788621521,-0.0331951640388602,
0.0791343294390534));
#92412=CARTESIAN_POINT('Ctrl Pts',(0.011369545208946,-0.0336938721132429,
0.0788964952479131));
#92413=CARTESIAN_POINT('Ctrl Pts',(0.0112701815790462,-0.0335278710435085,
0.0789644423916903));
#92414=CARTESIAN_POINT('Ctrl Pts',(0.0111687221002778,-0.0333620469224321,
0.0790292496142208));
#92415=CARTESIAN_POINT('Ctrl Pts',(0.0110651055344929,-0.0331951640388602,
0.0790909322698118));
#92416=CARTESIAN_POINT('Ctrl Pts',(0.0114384054142805,-0.0336938721132429,
0.0788486799580514));
#92417=CARTESIAN_POINT('Ctrl Pts',(0.0113400427546793,-0.0335278710435085,
0.0789180686285973));
#92418=CARTESIAN_POINT('Ctrl Pts',(0.0112395386881658,-0.0333620469224321,
0.0789843482609392));
#92419=CARTESIAN_POINT('Ctrl Pts',(0.0111368322068337,-0.0331951640388602,
0.0790475351005702));
#92420=CARTESIAN_POINT('Ctrl Pts',(0.011507265619615,-0.0336938721132429,
0.0788008646681897));
#92421=CARTESIAN_POINT('Ctrl Pts',(0.0114099039303124,-0.0335278710435085,
0.0788716948655044));
#92422=CARTESIAN_POINT('Ctrl Pts',(0.0113103552760537,-0.0333620469224321,
0.0789394469076575));
#92423=CARTESIAN_POINT('Ctrl Pts',(0.0112085588791746,-0.0331951640388602,
0.0790041379313286));
#92424=CARTESIAN_POINT('Ctrl Pts',(0.0102248110767327,-0.0321934096636183,
0.0797701136670266));
#92425=CARTESIAN_POINT('Ctrl Pts',(0.0101473053292143,-0.0320835708272304,
0.0797990884927741));
#92426=CARTESIAN_POINT('Ctrl Pts',(0.0100692449056664,-0.0319739230346346,
0.0798264425345285));
#92427=CARTESIAN_POINT('Ctrl Pts',(0.00999073236495321,-0.0318646057455576,
0.0798521484596572));
#92428=CARTESIAN_POINT('Ctrl Pts',(0.0102654663084347,-0.0321934096636183,
0.0796643388264415));
#92429=CARTESIAN_POINT('Ctrl Pts',(0.0101894192784039,-0.0320835708272304,
0.0796938743195189));
#92430=CARTESIAN_POINT('Ctrl Pts',(0.0101128051232469,-0.0319739230346346,
0.079721818891476));
#92431=CARTESIAN_POINT('Ctrl Pts',(0.0100357246094136,-0.0318646057455576,
0.0797481443121247));
#92432=CARTESIAN_POINT('Ctrl Pts',(0.0103061215401367,-0.0321934096636183,
0.0795585639858563));
#92433=CARTESIAN_POINT('Ctrl Pts',(0.0102315332275934,-0.0320835708272304,
0.0795886601462637));
#92434=CARTESIAN_POINT('Ctrl Pts',(0.0101563653408273,-0.0319739230346346,
0.0796171952484235));
#92435=CARTESIAN_POINT('Ctrl Pts',(0.0100807168538739,-0.0318646057455576,
0.0796441401645921));
#92436=CARTESIAN_POINT('Ctrl Pts',(0.0103467767718387,-0.0321934096636183,
0.0794527891452712));
#92437=CARTESIAN_POINT('Ctrl Pts',(0.010273647176783,-0.0320835708272304,
0.0794834459730085));
#92438=CARTESIAN_POINT('Ctrl Pts',(0.0101999255584078,-0.0319739230346346,
0.079512571605371));
#92439=CARTESIAN_POINT('Ctrl Pts',(0.0101257090983343,-0.0318646057455576,
0.0795401360170596));
#92440=CARTESIAN_POINT('Origin',(0.00332673899329973,-0.0326371942644191,
0.0642906726208783));
#92441=CARTESIAN_POINT('Ctrl Pts',(0.0103741962697567,-0.0322357242816073,
0.0794428028003719));
#92442=CARTESIAN_POINT('Ctrl Pts',(0.0102056273650785,-0.0319819883628705,
0.079514475570033));
#92443=CARTESIAN_POINT('Ctrl Pts',(0.0100328393428316,-0.0317295851069886,
0.0795752765642952));
#92444=CARTESIAN_POINT('Ctrl Pts',(0.0106020833880755,-0.0322357242816073,
0.0793400046422932));
#92445=CARTESIAN_POINT('Ctrl Pts',(0.0104367884714078,-0.0319819883628705,
0.0794189353211141));
#92446=CARTESIAN_POINT('Ctrl Pts',(0.0102668059605056,-0.0317295851069886,
0.0794871878487057));
#92447=CARTESIAN_POINT('Origin',(0.00292333812954877,-0.0326352985530547,
0.0645492556096483));
#92448=CARTESIAN_POINT('Ctrl Pts',(0.01046097262896,-0.032021883458232,
0.0794043637737633));
#92449=CARTESIAN_POINT('Ctrl Pts',(0.0104062874044174,-0.0319391099350606,
0.0794286882760792));
#92450=CARTESIAN_POINT('Ctrl Pts',(0.0103512554817486,-0.0318564869454878,
0.0794521441233481));
#92451=CARTESIAN_POINT('Ctrl Pts',(0.0102959185393638,-0.0317740741446461,
0.0794747179731653));
#92452=CARTESIAN_POINT('Ctrl Pts',(0.0105068452804265,-0.032021883458232,
0.079423139499984));
#92453=CARTESIAN_POINT('Ctrl Pts',(0.010451964645964,-0.0319391099350606,
0.0794479414257052));
#92454=CARTESIAN_POINT('Ctrl Pts',(0.0103967299767358,-0.0318564869454878,
0.0794718713557675));
#92455=CARTESIAN_POINT('Ctrl Pts',(0.0103411831310627,-0.0317740741446461,
0.0794949156162459));
#92456=CARTESIAN_POINT('Ctrl Pts',(0.0105527179318931,-0.032021883458232,
0.0794419152262047));
#92457=CARTESIAN_POINT('Ctrl Pts',(0.0104976418875106,-0.0319391099350606,
0.0794671945753313));
#92458=CARTESIAN_POINT('Ctrl Pts',(0.010442204471723,-0.0318564869454878,
0.0794915985881868));
#92459=CARTESIAN_POINT('Ctrl Pts',(0.0103864477227617,-0.0317740741446461,
0.0795151132593266));
#92460=CARTESIAN_POINT('Ctrl Pts',(0.0105985905833596,-0.032021883458232,
0.0794606909524254));
#92461=CARTESIAN_POINT('Ctrl Pts',(0.0105433191290573,-0.0319391099350606,
0.0794864477249573));
#92462=CARTESIAN_POINT('Ctrl Pts',(0.0104876789667102,-0.0318564869454878,
0.0795113258206062));
#92463=CARTESIAN_POINT('Ctrl Pts',(0.0104317123144606,-0.0317740741446461,
0.0795353109024072));
#92464=CARTESIAN_POINT('Ctrl Pts',(0.0111002850225003,-0.0330240426238156,
0.0790695235223111));
#92465=CARTESIAN_POINT('Ctrl Pts',(0.0110325137931213,-0.0329142774063509,
0.0791105277486519));
#92466=CARTESIAN_POINT('Ctrl Pts',(0.0109638611054147,-0.0328043479726686,
0.0791501513964742));
#92467=CARTESIAN_POINT('Ctrl Pts',(0.0108944135106418,-0.0326943950436594,
0.0791883412828284));
#92468=CARTESIAN_POINT('Ctrl Pts',(0.0112097138896685,-0.0330240426238156,
0.079098959198208));
#92469=CARTESIAN_POINT('Ctrl Pts',(0.0111415371551763,-0.0329142774063509,
0.0791414709138054));
#92470=CARTESIAN_POINT('Ctrl Pts',(0.0110724475961834,-0.0328043479726686,
0.0791825944194992));
#92471=CARTESIAN_POINT('Ctrl Pts',(0.0110025322707001,-0.0326943950436594,
0.0792222745954973));
#92472=CARTESIAN_POINT('Ctrl Pts',(0.0113191427568367,-0.0330240426238156,
0.0791283948741049));
#92473=CARTESIAN_POINT('Ctrl Pts',(0.0112505605172312,-0.0329142774063509,
0.0791724140789589));
#92474=CARTESIAN_POINT('Ctrl Pts',(0.0111810340869521,-0.0328043479726686,
0.0792150374425243));
#92475=CARTESIAN_POINT('Ctrl Pts',(0.0111106510307583,-0.0326943950436594,
0.0792562079081662));
#92476=CARTESIAN_POINT('Ctrl Pts',(0.0114285716240049,-0.0330240426238156,
0.0791578305500018));
#92477=CARTESIAN_POINT('Ctrl Pts',(0.0113595838792861,-0.0329142774063509,
0.0792033572441124));
#92478=CARTESIAN_POINT('Ctrl Pts',(0.0112896205777207,-0.0328043479726686,
0.0792474804655494));
#92479=CARTESIAN_POINT('Ctrl Pts',(0.0112187697908166,-0.0326943950436594,
0.0792901412208352));
#92480=CARTESIAN_POINT('Origin',(0.00286364172159143,-0.032639668285722,
0.0644323553870705));
#92481=CARTESIAN_POINT('Ctrl Pts',(0.0109126308553257,-0.0331951640388587,
0.0794624686483194));
#92482=CARTESIAN_POINT('Ctrl Pts',(0.0108394623467316,-0.0330855618255041,
0.0795008793968466));
#92483=CARTESIAN_POINT('Ctrl Pts',(0.0107654472074681,-0.0329757224427708,
0.0795378055671436));
#92484=CARTESIAN_POINT('Ctrl Pts',(0.0106906778988787,-0.0328657862078596,
0.0795731952238349));
#92485=CARTESIAN_POINT('Ctrl Pts',(0.0109397083921659,-0.0331951640388587,
0.079352432476816));
#92486=CARTESIAN_POINT('Ctrl Pts',(0.010868055409233,-0.0330855618255041,
0.0793912161636357));
#92487=CARTESIAN_POINT('Ctrl Pts',(0.0107955491801548,-0.0329757224427708,
0.0794285468643961));
#92488=CARTESIAN_POINT('Ctrl Pts',(0.0107222802086147,-0.0328657862078596,
0.079464372220477));
#92489=CARTESIAN_POINT('Ctrl Pts',(0.0109667859290061,-0.0331951640388587,
0.0792423963053125));
#92490=CARTESIAN_POINT('Ctrl Pts',(0.0108966484717343,-0.0330855618255041,
0.0792815529304248));
#92491=CARTESIAN_POINT('Ctrl Pts',(0.0108256511528415,-0.0329757224427708,
0.0793192881616486));
#92492=CARTESIAN_POINT('Ctrl Pts',(0.0107538825183506,-0.0328657862078596,
0.0793555492171192));
#92493=CARTESIAN_POINT('Ctrl Pts',(0.0109938634658464,-0.0331951640388587,
0.079132360133809));
#92494=CARTESIAN_POINT('Ctrl Pts',(0.0109252415342356,-0.0330855618255041,
0.0791718896972139));
#92495=CARTESIAN_POINT('Ctrl Pts',(0.0108557531255281,-0.0329757224427708,
0.0792100294589011));
#92496=CARTESIAN_POINT('Ctrl Pts',(0.0107854848280865,-0.0328657862078596,
0.0792467262137613));
#92497=CARTESIAN_POINT('Origin',(0.00330355586658263,-0.0326401908834077,
0.0642380658693673));
#92498=CARTESIAN_POINT('Ctrl Pts',(0.0110246120685592,-0.0332451089994432,
0.0791162169740853));
#92499=CARTESIAN_POINT('Ctrl Pts',(0.0108373081309289,-0.0329451141710258,
0.0792256235628233));
#92500=CARTESIAN_POINT('Ctrl Pts',(0.010642295352496,-0.0326442513127503,
0.0793206108407027));
#92501=CARTESIAN_POINT('Ctrl Pts',(0.0112376920410981,-0.0332451089994432,
0.0789854617627062));
#92502=CARTESIAN_POINT('Ctrl Pts',(0.0110553196169488,-0.0329451141710258,
0.0791029047940915));
#92503=CARTESIAN_POINT('Ctrl Pts',(0.0108646190043741,-0.0326442513127503,
0.0792062771456886));
#92504=CARTESIAN_POINT('Ctrl Pts',(0.0107070916436316,-0.0327445246961877,
0.0792885442766252));
#92505=CARTESIAN_POINT('Ctrl Pts',(0.0105132882800017,-0.0324436878365475,
0.0793859753843197));
#92506=CARTESIAN_POINT('Ctrl Pts',(0.0103126965820868,-0.0321434074463187,
0.079468531639252));
#92507=CARTESIAN_POINT('Ctrl Pts',(0.0109279605404424,-0.0327445246961877,
0.0791714249766719));
#92508=CARTESIAN_POINT('Ctrl Pts',(0.0107385744033761,-0.0324436878365475,
0.0792771862909031));
#92509=CARTESIAN_POINT('Ctrl Pts',(0.0105417599179551,-0.0321434074463187,
0.0793683818106906));
#92510=CARTESIAN_POINT('Origin',(0.00328659600653958,-0.0326395579069779,
0.0642042379962714));
#92511=CARTESIAN_POINT('Origin',(0.00286748906709375,-0.0326393375179411,
0.0644399638664167));
#92512=CARTESIAN_POINT('Ctrl Pts',(0.010573555033132,-0.0326943950436593,
0.0796270989613478));
#92513=CARTESIAN_POINT('Ctrl Pts',(0.0104980703442673,-0.0325844576448127,
0.0796608614224468));
#92514=CARTESIAN_POINT('Ctrl Pts',(0.0104218820501841,-0.0324744968375319,
0.0796930651258431));
#92515=CARTESIAN_POINT('Ctrl Pts',(0.0103450883368848,-0.0323646534831894,
0.0797236701567042));
#92516=CARTESIAN_POINT('Ctrl Pts',(0.0106074883346984,-0.0326943950436593,
0.0795189802366644));
#92517=CARTESIAN_POINT('Ctrl Pts',(0.010533493724496,-0.0325844576448127,
0.0795532103622568));
#92518=CARTESIAN_POINT('Ctrl Pts',(0.0104587859424617,-0.0324744968375319,
0.0795859125805135));
#92519=CARTESIAN_POINT('Ctrl Pts',(0.0103834612864896,-0.0323646534831894,
0.0796170463117117));
#92520=CARTESIAN_POINT('Ctrl Pts',(0.0106414216362648,-0.0326943950436593,
0.0794108615119809));
#92521=CARTESIAN_POINT('Ctrl Pts',(0.0105689171047246,-0.0325844576448127,
0.0794455593020667));
#92522=CARTESIAN_POINT('Ctrl Pts',(0.0104956898347393,-0.0324744968375319,
0.0794787600351839));
#92523=CARTESIAN_POINT('Ctrl Pts',(0.0104218342360944,-0.0323646534831894,
0.0795104224667191));
#92524=CARTESIAN_POINT('Ctrl Pts',(0.0106753549378313,-0.0326943950436593,
0.0793027427872974));
#92525=CARTESIAN_POINT('Ctrl Pts',(0.0106043404849533,-0.0325844576448127,
0.0793379082418766));
#92526=CARTESIAN_POINT('Ctrl Pts',(0.0105325937270169,-0.0324744968375319,
0.0793716074898543));
#92527=CARTESIAN_POINT('Ctrl Pts',(0.0104602071856992,-0.0323646534831894,
0.0794037986217265));
#92528=CARTESIAN_POINT('Ctrl Pts',(0.0107855128689007,-0.0325229783203385,
0.0792467116709563));
#92529=CARTESIAN_POINT('Ctrl Pts',(0.0107152548112531,-0.032413025311208,
0.079283403569446));
#92530=CARTESIAN_POINT('Ctrl Pts',(0.0106442483905759,-0.0323031222247695,
0.0793186365247416));
#92531=CARTESIAN_POINT('Ctrl Pts',(0.0105725861535637,-0.0321934096636184,
0.0793523686154071));
#92532=CARTESIAN_POINT('Ctrl Pts',(0.0108928775554811,-0.0325229783203385,
0.0792829603499048));
#92533=CARTESIAN_POINT('Ctrl Pts',(0.0108221198105961,-0.032413025311208,
0.0793211322682242));
#92534=CARTESIAN_POINT('Ctrl Pts',(0.0107505831623579,-0.0323031222247695,
0.0793578346822033));
#92535=CARTESIAN_POINT('Ctrl Pts',(0.0106783609030641,-0.0321934096636184,
0.0793930238121002));
#92536=CARTESIAN_POINT('Ctrl Pts',(0.0110002422420616,-0.0325229783203385,
0.0793192090288534));
#92537=CARTESIAN_POINT('Ctrl Pts',(0.010928984809939,-0.032413025311208,
0.0793588609670024));
#92538=CARTESIAN_POINT('Ctrl Pts',(0.0108569179341398,-0.0323031222247695,
0.079397032839665));
#92539=CARTESIAN_POINT('Ctrl Pts',(0.0107841356525646,-0.0321934096636184,
0.0794336790087933));
#92540=CARTESIAN_POINT('Ctrl Pts',(0.0111076069286421,-0.0325229783203385,
0.079355457707802));
#92541=CARTESIAN_POINT('Ctrl Pts',(0.011035849809282,-0.032413025311208,
0.0793965896657807));
#92542=CARTESIAN_POINT('Ctrl Pts',(0.0109632527059218,-0.0323031222247695,
0.0794362309971267));
#92543=CARTESIAN_POINT('Ctrl Pts',(0.0108899104020651,-0.0321934096636184,
0.0794743342054863));
#92544=CARTESIAN_POINT('Origin',(0.0138781452811081,-0.0391228853390915,
0.0847692242551965));
#92545=CARTESIAN_POINT('Ctrl Pts',(0.0128112537139296,-0.0352722978779613,
0.077483432957791));
#92546=CARTESIAN_POINT('Ctrl Pts',(0.0128000187930861,-0.0352466642097229,
0.0774986273393741));
#92547=CARTESIAN_POINT('Ctrl Pts',(0.0127888569209621,-0.0352210183808307,
0.0775138547968734));
#92548=CARTESIAN_POINT('Ctrl Pts',(0.012777768133161,-0.0351953608940152,
0.0775291161824723));
#92549=CARTESIAN_POINT('Origin',(0.0166407683657512,-0.0352456003065054,
0.0805403203823156));
#92550=CARTESIAN_POINT('Ctrl Pts',(0.0127022617679223,-0.035024121149334,
0.0776283336417555));
#92551=CARTESIAN_POINT('Ctrl Pts',(0.0126543491503399,-0.0349144232867421,
0.0776914003178052));
#92552=CARTESIAN_POINT('Ctrl Pts',(0.0126051042215475,-0.0348045283677512,
0.0777535143543013));
#92553=CARTESIAN_POINT('Ctrl Pts',(0.0125545870974168,-0.0346945769586886,
0.0778145938438405));
#92554=CARTESIAN_POINT('Ctrl Pts',(0.012814842176338,-0.035024121149334,
0.0776154187881212));
#92555=CARTESIAN_POINT('Ctrl Pts',(0.0127671074555611,-0.0349144232867421,
0.0776800362130671));
#92556=CARTESIAN_POINT('Ctrl Pts',(0.0127180084749677,-0.0348045283677512,
0.0777437056039114));
#92557=CARTESIAN_POINT('Ctrl Pts',(0.0126676050893535,-0.0346945769586886,
0.0778063430679958));
#92558=CARTESIAN_POINT('Ctrl Pts',(0.0129274225847537,-0.035024121149334,
0.0776025039344869));
#92559=CARTESIAN_POINT('Ctrl Pts',(0.0128798657607823,-0.0349144232867421,
0.077668672108329));
#92560=CARTESIAN_POINT('Ctrl Pts',(0.0128309127283878,-0.0348045283677512,
0.0777338968535214));
#92561=CARTESIAN_POINT('Ctrl Pts',(0.0127806230812902,-0.0346945769586886,
0.0777980922921512));
#92562=CARTESIAN_POINT('Ctrl Pts',(0.0130400029931695,-0.035024121149334,
0.0775895890808527));
#92563=CARTESIAN_POINT('Ctrl Pts',(0.0129926240660035,-0.0349144232867421,
0.077657308003591));
#92564=CARTESIAN_POINT('Ctrl Pts',(0.012943816981808,-0.0348045283677512,
0.0777240881031315));
#92565=CARTESIAN_POINT('Ctrl Pts',(0.0128936410732269,-0.0346945769586886,
0.0777898415163066));
#92566=CARTESIAN_POINT('Origin',(-0.000267143618523518,-0.0345629067940785,
0.0669764126992258));
#92567=CARTESIAN_POINT('Ctrl Pts',(0.0126608351673018,-0.0351970973651608,
0.0779697738266411));
#92568=CARTESIAN_POINT('Ctrl Pts',(0.0126079173776439,-0.0350869349321771,
0.078032628546803));
#92569=CARTESIAN_POINT('Ctrl Pts',(0.0125536490367048,-0.0349764985129727,
0.078094435203562));
#92570=CARTESIAN_POINT('Ctrl Pts',(0.0124980957371878,-0.0348659306849652,
0.078155109585943));
#92571=CARTESIAN_POINT('Ctrl Pts',(0.0126496912179573,-0.0351970973651608,
0.0778883104419646));
#92572=CARTESIAN_POINT('Ctrl Pts',(0.0125979019930916,-0.0350869349321771,
0.077951010777811));
#92573=CARTESIAN_POINT('Ctrl Pts',(0.0125447663613991,-0.0349764985129727,
0.0780126863846009));
#92574=CARTESIAN_POINT('Ctrl Pts',(0.0124903484581191,-0.0348659306849652,
0.0780732533075217));
#92575=CARTESIAN_POINT('Ctrl Pts',(0.0126385472686127,-0.0351970973651608,
0.077806847057288));
#92576=CARTESIAN_POINT('Ctrl Pts',(0.0125878866085394,-0.0350869349321771,
0.0778693930088189));
#92577=CARTESIAN_POINT('Ctrl Pts',(0.0125358836860934,-0.0349764985129727,
0.0779309375656399));
#92578=CARTESIAN_POINT('Ctrl Pts',(0.0124826011790504,-0.0348659306849652,
0.0779913970291004));
#92579=CARTESIAN_POINT('Ctrl Pts',(0.0126274033192682,-0.0351970973651608,
0.0777253836726114));
#92580=CARTESIAN_POINT('Ctrl Pts',(0.0125778712239871,-0.0350869349321771,
0.0777877752398269));
#92581=CARTESIAN_POINT('Ctrl Pts',(0.0125270010107877,-0.0349764985129727,
0.0778491887466789));
#92582=CARTESIAN_POINT('Ctrl Pts',(0.0124748538999816,-0.0348659306849652,
0.0779095407506791));
#92583=CARTESIAN_POINT('Origin',(7.85550839694687E-5,-0.0345637187964175,
0.0666420210672609));
#92584=CARTESIAN_POINT('Ctrl Pts',(0.0126490882798721,-0.0352450361861253,
0.0776996098125146));
#92585=CARTESIAN_POINT('Ctrl Pts',(0.0125152125524391,-0.0349452761023765,
0.0778702845278275));
#92586=CARTESIAN_POINT('Ctrl Pts',(0.0123688612342642,-0.0346444289983475,
0.0780303903069589));
#92587=CARTESIAN_POINT('Ctrl Pts',(0.0127990710340421,-0.0352450361861253,
0.0774995968793039));
#92588=CARTESIAN_POINT('Ctrl Pts',(0.0126727389179759,-0.0349452761023765,
0.0776759282868667));
#92589=CARTESIAN_POINT('Ctrl Pts',(0.0125334836953686,-0.0346444289983475,
0.0778422429038412));
#92590=CARTESIAN_POINT('Ctrl Pts',(0.0124748214846824,-0.0345231616327822,
0.0779089543554312));
#92591=CARTESIAN_POINT('Ctrl Pts',(0.0124230095910775,-0.0344132092796975,
0.0779689273062918));
#92592=CARTESIAN_POINT('Ctrl Pts',(0.0123699598775457,-0.0343032738558974,
0.0780278254746732));
#92593=CARTESIAN_POINT('Ctrl Pts',(0.0123157422397181,-0.0341934961088741,
0.078085575146108));
#92594=CARTESIAN_POINT('Ctrl Pts',(0.0125879906458554,-0.0345231616327822,
0.0779031339518055));
#92595=CARTESIAN_POINT('Ctrl Pts',(0.01253625897832,-0.0344132092796975,
0.0779646667802234));
#92596=CARTESIAN_POINT('Ctrl Pts',(0.0124832572218815,-0.0343032738558974,
0.0780251264050927));
#92597=CARTESIAN_POINT('Ctrl Pts',(0.0124290552619737,-0.0341934961088741,
0.0780844371099657));
#92598=CARTESIAN_POINT('Ctrl Pts',(0.0127011598070283,-0.0345231616327822,
0.0778973135481798));
#92599=CARTESIAN_POINT('Ctrl Pts',(0.0126495083655625,-0.0344132092796975,
0.077960406254155));
#92600=CARTESIAN_POINT('Ctrl Pts',(0.0125965545662173,-0.0343032738558974,
0.0780224273355121));
#92601=CARTESIAN_POINT('Ctrl Pts',(0.0125423682842293,-0.0341934961088741,
0.0780832990738234));
#92602=CARTESIAN_POINT('Ctrl Pts',(0.0128143289682013,-0.0345231616327822,
0.0778914931445541));
#92603=CARTESIAN_POINT('Ctrl Pts',(0.012762757752805,-0.0344132092796975,
0.0779561457280867));
#92604=CARTESIAN_POINT('Ctrl Pts',(0.0127098519105532,-0.0343032738558974,
0.0780197282659315));
#92605=CARTESIAN_POINT('Ctrl Pts',(0.0126556813064849,-0.0341934961088741,
0.078082161037681));
#92606=CARTESIAN_POINT('Origin',(-0.000276504297481307,-0.0345625596229775,
0.0669687396303667));
#92607=CARTESIAN_POINT('Ctrl Pts',(0.0124177779806862,-0.0346945769586885,
0.0783406562942356));
#92608=CARTESIAN_POINT('Ctrl Pts',(0.0123600286187926,-0.0345846629176052,
0.0783998297265801));
#92609=CARTESIAN_POINT('Ctrl Pts',(0.0123010457108863,-0.0344746925050311,
0.0784578190328047));
#92610=CARTESIAN_POINT('Ctrl Pts',(0.012240905139525,-0.034364806625326,
0.0785145502224446));
#92611=CARTESIAN_POINT('Ctrl Pts',(0.0124095272113377,-0.0346945769586885,
0.0782276383912827));
#92612=CARTESIAN_POINT('Ctrl Pts',(0.0123533352932715,-0.0345846629176052,
0.0782866981238552));
#92613=CARTESIAN_POINT('Ctrl Pts',(0.0122959124464725,-0.0344746925050311,
0.0783446059181864));
#92614=CARTESIAN_POINT('Ctrl Pts',(0.0122373325541367,-0.034364806625326,
0.0784012878799986));
#92615=CARTESIAN_POINT('Ctrl Pts',(0.0124012764419893,-0.0346945769586885,
0.0781146204883298));
#92616=CARTESIAN_POINT('Ctrl Pts',(0.0123466419677505,-0.0345846629176052,
0.0781735665211304));
#92617=CARTESIAN_POINT('Ctrl Pts',(0.0122907791820586,-0.0344746925050311,
0.0782313928035682));
#92618=CARTESIAN_POINT('Ctrl Pts',(0.0122337599687485,-0.034364806625326,
0.0782880255375526));
#92619=CARTESIAN_POINT('Ctrl Pts',(0.0123930256726408,-0.0346945769586885,
0.0780016025853769));
#92620=CARTESIAN_POINT('Ctrl Pts',(0.0123399486422294,-0.0345846629176052,
0.0780604349184056));
#92621=CARTESIAN_POINT('Ctrl Pts',(0.0122856459176447,-0.0344746925050311,
0.0781181796889499));
#92622=CARTESIAN_POINT('Ctrl Pts',(0.0122301873833602,-0.034364806625326,
0.0781747631951066));
#92623=CARTESIAN_POINT('Origin',(3.5309344467477E-5,-0.0345626446732227,
0.0666027281070317));
#92624=CARTESIAN_POINT('Ctrl Pts',(0.0123931733065714,-0.0346945769586886,
0.078003624854638));
#92625=CARTESIAN_POINT('Ctrl Pts',(0.0123124575910851,-0.0345275153362891,
0.078093048960879));
#92626=CARTESIAN_POINT('Ctrl Pts',(0.0122289086925484,-0.0343603235965159,
0.0781799577618159));
#92627=CARTESIAN_POINT('Ctrl Pts',(0.0121427775317648,-0.034193496108874,
0.0782640978923524));
#92628=CARTESIAN_POINT('Ctrl Pts',(0.0124479789570725,-0.0346945769586886,
0.0779401869400725));
#92629=CARTESIAN_POINT('Ctrl Pts',(0.0123685919741059,-0.0345275153362891,
0.0780307589726062));
#92630=CARTESIAN_POINT('Ctrl Pts',(0.0122863360505419,-0.0343603235965159,
0.0781188577841631));
#92631=CARTESIAN_POINT('Ctrl Pts',(0.0122014583354472,-0.034193496108874,
0.0782042264332884));
#92632=CARTESIAN_POINT('Ctrl Pts',(0.0125027846075736,-0.0346945769586886,
0.0778767490255069));
#92633=CARTESIAN_POINT('Ctrl Pts',(0.0124247263571267,-0.0345275153362891,
0.0779684689843333));
#92634=CARTESIAN_POINT('Ctrl Pts',(0.0123437634085354,-0.0343603235965159,
0.0780577578065103));
#92635=CARTESIAN_POINT('Ctrl Pts',(0.0122601391391296,-0.034193496108874,
0.0781443549742244));
#92636=CARTESIAN_POINT('Ctrl Pts',(0.0125575902580747,-0.0346945769586886,
0.0778133111109414));
#92637=CARTESIAN_POINT('Ctrl Pts',(0.0124808607401475,-0.0345275153362891,
0.0779061789960605));
#92638=CARTESIAN_POINT('Ctrl Pts',(0.0124011907665289,-0.0343603235965159,
0.0779966578288574));
#92639=CARTESIAN_POINT('Ctrl Pts',(0.012318819942812,-0.034193496108874,
0.0780844835151603));
#92640=CARTESIAN_POINT('Ctrl Pts',(0.0122302090727844,-0.0340223579322365,
0.0781747402701359));
#92641=CARTESIAN_POINT('Ctrl Pts',(0.0121746974074964,-0.0339125849573554,
0.078231378606817));
#92642=CARTESIAN_POINT('Ctrl Pts',(0.012118052467653,-0.0338030433565221,
0.0782868281819145));
#92643=CARTESIAN_POINT('Ctrl Pts',(0.0120603529785157,-0.0336938721132328,
0.0783410245062105));
#92644=CARTESIAN_POINT('Ctrl Pts',(0.0123435205796144,-0.0340223579322365,
0.0781760372862076));
#92645=CARTESIAN_POINT('Ctrl Pts',(0.0122879910250921,-0.0339125849573554,
0.0782342384840967));
#92646=CARTESIAN_POINT('Ctrl Pts',(0.0122312958609895,-0.0338030433565221,
0.0782912494519321));
#92647=CARTESIAN_POINT('Ctrl Pts',(0.0121735140538006,-0.0336938721132328,
0.0783470037094314));
#92648=CARTESIAN_POINT('Ctrl Pts',(0.0124568320864445,-0.0340223579322365,
0.0781773343022793));
#92649=CARTESIAN_POINT('Ctrl Pts',(0.0124012846426878,-0.0339125849573554,
0.0782370983613764));
#92650=CARTESIAN_POINT('Ctrl Pts',(0.0123445392543259,-0.0338030433565221,
0.0782956707219498));
#92651=CARTESIAN_POINT('Ctrl Pts',(0.0122866751290855,-0.0336938721132328,
0.0783529829126524));
#92652=CARTESIAN_POINT('Ctrl Pts',(0.0125701435932746,-0.0340223579322365,
0.0781786313183511));
#92653=CARTESIAN_POINT('Ctrl Pts',(0.0125145782602835,-0.0339125849573554,
0.0782399582386561));
#92654=CARTESIAN_POINT('Ctrl Pts',(0.0124577826476623,-0.0338030433565221,
0.0783000919919674));
#92655=CARTESIAN_POINT('Ctrl Pts',(0.0123998362043704,-0.0336938721132328,
0.0783589621158733));
#92656=CARTESIAN_POINT('Origin',(-0.00018683044819935,-0.0345589643413972,
0.0670488113415833));
#92657=CARTESIAN_POINT('Ctrl Pts',(0.0121461712749856,-0.034193496108874,
0.0786020092176615));
#92658=CARTESIAN_POINT('Ctrl Pts',(0.0120847807042492,-0.0340836138581107,
0.0786574755811364));
#92659=CARTESIAN_POINT('Ctrl Pts',(0.0120222718298549,-0.0339738896643499,
0.0787116449817608));
#92660=CARTESIAN_POINT('Ctrl Pts',(0.0119587293029819,-0.0338644633294062,
0.0787644534524276));
#92661=CARTESIAN_POINT('Ctrl Pts',(0.0121450332378193,-0.034193496108874,
0.0784886960934465));
#92662=CARTESIAN_POINT('Ctrl Pts',(0.0120852051879644,-0.0340836138581107,
0.0785441467640628));
#92663=CARTESIAN_POINT('Ctrl Pts',(0.0120242584094556,-0.0339738896643499,
0.0785983328124494));
#92664=CARTESIAN_POINT('Ctrl Pts',(0.0119622755556104,-0.0338644633294062,
0.0786511901161698));
#92665=CARTESIAN_POINT('Ctrl Pts',(0.0121438952006529,-0.034193496108874,
0.0783753829692315));
#92666=CARTESIAN_POINT('Ctrl Pts',(0.0120856296716796,-0.0340836138581107,
0.0784308179469892));
#92667=CARTESIAN_POINT('Ctrl Pts',(0.0120262449890562,-0.0339738896643499,
0.0784850206431379));
#92668=CARTESIAN_POINT('Ctrl Pts',(0.0119658218082389,-0.0338644633294062,
0.0785379267799119));
#92669=CARTESIAN_POINT('Ctrl Pts',(0.0121427571634866,-0.034193496108874,
0.0782620698450165));
#92670=CARTESIAN_POINT('Ctrl Pts',(0.0120860541553949,-0.0340836138581107,
0.0783174891299155));
#92671=CARTESIAN_POINT('Ctrl Pts',(0.0120282315686569,-0.0339738896643499,
0.0783717084738264));
#92672=CARTESIAN_POINT('Ctrl Pts',(0.0119693680608674,-0.0338644633294062,
0.0784246634436541));
#92673=CARTESIAN_POINT('Origin',(8.95625897499976E-5,-0.0345610621864118,
0.0666549117351775));
#92674=CARTESIAN_POINT('Ctrl Pts',(0.0121685766225554,-0.03424362768739,
0.0782387361156615));
#92675=CARTESIAN_POINT('Ctrl Pts',(0.012014367397785,-0.033943005420186,
0.0783912880524157));
#92676=CARTESIAN_POINT('Ctrl Pts',(0.0118491054283175,-0.0336441434784162,
0.0785317909344483));
#92677=CARTESIAN_POINT('Ctrl Pts',(0.0123424425336475,-0.03424362768739,
0.078059095794575));
#92678=CARTESIAN_POINT('Ctrl Pts',(0.0121950085552781,-0.033943005420186,
0.0782182051922669));
#92679=CARTESIAN_POINT('Ctrl Pts',(0.0120360086496206,-0.0336441434784162,
0.0783657572454977));
#92680=CARTESIAN_POINT('Ctrl Pts',(0.0119693885923796,-0.0335235895815127,
0.0784246448027122));
#92681=CARTESIAN_POINT('Ctrl Pts',(0.01191053969067,-0.0334144449262719,
0.0784775871460997));
#92682=CARTESIAN_POINT('Ctrl Pts',(0.0118505294297312,-0.0333049234473133,
0.078529374539805));
#92683=CARTESIAN_POINT('Ctrl Pts',(0.0117894285457527,-0.0331951640388588,
0.0785799338126902));
#92684=CARTESIAN_POINT('Ctrl Pts',(0.012082395028372,-0.0335235895815127,
0.0784330541969319));
#92685=CARTESIAN_POINT('Ctrl Pts',(0.0120234303547943,-0.0334144449262719,
0.0784875522964));
#92686=CARTESIAN_POINT('Ctrl Pts',(0.0119632720482299,-0.0333049234473133,
0.0785408948418015));
#92687=CARTESIAN_POINT('Ctrl Pts',(0.0119019908540405,-0.0331951640388588,
0.0785930066562889));
#92688=CARTESIAN_POINT('Ctrl Pts',(0.0121954014643643,-0.0335235895815127,
0.0784414635911516));
#92689=CARTESIAN_POINT('Ctrl Pts',(0.0121363210189186,-0.0334144449262719,
0.0784975174467003));
#92690=CARTESIAN_POINT('Ctrl Pts',(0.0120760146667286,-0.0333049234473133,
0.078552415143798));
#92691=CARTESIAN_POINT('Ctrl Pts',(0.0120145531623283,-0.0331951640388588,
0.0786060794998875));
#92692=CARTESIAN_POINT('Ctrl Pts',(0.0123084079003567,-0.0335235895815127,
0.0784498729853713));
#92693=CARTESIAN_POINT('Ctrl Pts',(0.012249211683043,-0.0334144449262719,
0.0785074825970005));
#92694=CARTESIAN_POINT('Ctrl Pts',(0.0121887572852272,-0.0333049234473133,
0.0785639354457945));
#92695=CARTESIAN_POINT('Ctrl Pts',(0.0121271154706161,-0.0331951640388588,
0.0786191523434861));
#92696=CARTESIAN_POINT('Origin',(0.0017614196500452,-0.0326434571768189,
0.065267162552053));
#92697=CARTESIAN_POINT('Ctrl Pts',(0.0118585830537535,-0.0336938721132448,
0.0788478168404056));
#92698=CARTESIAN_POINT('Ctrl Pts',(0.0118310851728839,-0.0336474569764987,
0.0788696778691827));
#92699=CARTESIAN_POINT('Ctrl Pts',(0.0118033332652433,-0.033601104548885,
0.0788912155026138));
#92700=CARTESIAN_POINT('Ctrl Pts',(0.0117330718186913,-0.03348375086432,
0.0789457438362969));
#92701=CARTESIAN_POINT('Ctrl Pts',(0.0116612254382725,-0.0333660264760483,
0.0789981662329088));
#92702=CARTESIAN_POINT('Ctrl Pts',(0.0118765206184675,-0.0336938721132448,
0.0785083344652326));
#92703=CARTESIAN_POINT('Ctrl Pts',(0.0118510098405922,-0.0336474569764987,
0.0785303004885282));
#92704=CARTESIAN_POINT('Ctrl Pts',(0.0118252436706948,-0.033601104548885,
0.0785519663708331));
#92705=CARTESIAN_POINT('Ctrl Pts',(0.0117600096553422,-0.03348375086432,
0.0786068194011643));
#92706=CARTESIAN_POINT('Ctrl Pts',(0.0116931788770111,-0.0333660264760483,
0.0786597153250451));
#92707=CARTESIAN_POINT('Ctrl Pts',(0.0118765206184709,-0.0336938721132426,
0.0785083344652483));
#92708=CARTESIAN_POINT('Ctrl Pts',(0.0118510098405988,-0.0336474569765026,
0.0785303004885411));
#92709=CARTESIAN_POINT('Ctrl Pts',(0.0118252436707048,-0.0336011045488949,
0.0785519663708431));
#92710=CARTESIAN_POINT('Ctrl Pts',(0.0117605529658464,-0.0334847282606778,
0.0786063625501455));
#92711=CARTESIAN_POINT('Ctrl Pts',(0.0116942917446253,-0.0333679869945434,
0.078658834277581));
#92712=CARTESIAN_POINT('Ctrl Pts',(0.0118765206184665,-0.0336938721132429,
0.0785083344652336));
#92713=CARTESIAN_POINT('Ctrl Pts',(0.0117852827871481,-0.0335278710435085,
0.0785868946854659));
#92714=CARTESIAN_POINT('Ctrl Pts',(0.0116916134250057,-0.0333620469224321,
0.0786625660737266));
#92715=CARTESIAN_POINT('Ctrl Pts',(0.011595453361056,-0.0331951640388601,
0.0787353706831229));
#92716=CARTESIAN_POINT('Ctrl Pts',(0.0119388449956222,-0.0336938721132429,
0.0784522657410156));
#92717=CARTESIAN_POINT('Ctrl Pts',(0.0118487809128638,-0.0335278710435085,
0.0785321306663034));
#92718=CARTESIAN_POINT('Ctrl Pts',(0.011756243971148,-0.0333620469224321,
0.078609143109077));
#92719=CARTESIAN_POINT('Ctrl Pts',(0.0116611753396131,-0.0331951640388601,
0.0786833259777455));
#92720=CARTESIAN_POINT('Ctrl Pts',(0.012001169372778,-0.0336938721132429,
0.0783961970167977));
#92721=CARTESIAN_POINT('Ctrl Pts',(0.0119122790385795,-0.0335278710435085,
0.0784773666471409));
#92722=CARTESIAN_POINT('Ctrl Pts',(0.0118208745172904,-0.0333620469224321,
0.0785557201444273));
#92723=CARTESIAN_POINT('Ctrl Pts',(0.0117268973181703,-0.0331951640388601,
0.0786312812723682));
#92724=CARTESIAN_POINT('Ctrl Pts',(0.0120634937499337,-0.0336938721132429,
0.0783401282925797));
#92725=CARTESIAN_POINT('Ctrl Pts',(0.0119757771642952,-0.0335278710435085,
0.0784226026279784));
#92726=CARTESIAN_POINT('Ctrl Pts',(0.0118855050634327,-0.0333620469224321,
0.0785022971797777));
#92727=CARTESIAN_POINT('Ctrl Pts',(0.0117926192967274,-0.0331951640388601,
0.0785792365669909));
#92728=CARTESIAN_POINT('Ctrl Pts',(0.0116933941992991,-0.0330240426238155,
0.0786576768856262));
#92729=CARTESIAN_POINT('Ctrl Pts',(0.0116312965585832,-0.0329142774063508,
0.0787068517687157));
#92730=CARTESIAN_POINT('Ctrl Pts',(0.0115681513777318,-0.0328043479726686,
0.078754767435583));
#92731=CARTESIAN_POINT('Ctrl Pts',(0.0115040378599329,-0.0326943950436594,
0.0788013602748927));
#92732=CARTESIAN_POINT('Ctrl Pts',(0.011805649455607,-0.0330240426238155,
0.0786731653786591));
#92733=CARTESIAN_POINT('Ctrl Pts',(0.0117433384458098,-0.0329142774063508,
0.0787238866872692));
#92734=CARTESIAN_POINT('Ctrl Pts',(0.0116799478205698,-0.0328043479726686,
0.0787733451396718));
#92735=CARTESIAN_POINT('Ctrl Pts',(0.0116155570430768,-0.0326943950436594,
0.0788214751394487));
#92736=CARTESIAN_POINT('Ctrl Pts',(0.0119179047119149,-0.0330240426238155,
0.078688653871692));
#92737=CARTESIAN_POINT('Ctrl Pts',(0.0118553803330365,-0.0329142774063509,
0.0787409216058228));
#92738=CARTESIAN_POINT('Ctrl Pts',(0.0117917442634077,-0.0328043479726686,
0.0787919228437605));
#92739=CARTESIAN_POINT('Ctrl Pts',(0.0117270762262207,-0.0326943950436594,
0.0788415900040047));
#92740=CARTESIAN_POINT('Ctrl Pts',(0.0120301599682228,-0.0330240426238155,
0.078704142364725));
#92741=CARTESIAN_POINT('Ctrl Pts',(0.0119674222202632,-0.0329142774063509,
0.0787579565243764));
#92742=CARTESIAN_POINT('Ctrl Pts',(0.0119035407062456,-0.0328043479726686,
0.0788105005478493));
#92743=CARTESIAN_POINT('Ctrl Pts',(0.0118385954093646,-0.0326943950436594,
0.0788617048685608));
#92744=CARTESIAN_POINT('Origin',(0.00168717567872209,-0.0326396682856143,
0.0651682523318792));
#92745=CARTESIAN_POINT('Ctrl Pts',(0.0115564688245381,-0.0331951640388587,
0.0790710428255139));
#92746=CARTESIAN_POINT('Ctrl Pts',(0.0114886914069139,-0.0330855618127431,
0.079118321145098));
#92747=CARTESIAN_POINT('Ctrl Pts',(0.0114198879673268,-0.0329757224171935,
0.0791642327034358));
#92748=CARTESIAN_POINT('Ctrl Pts',(0.0113501437288367,-0.0328657861694599,
0.0792087143861768));
#92749=CARTESIAN_POINT('Ctrl Pts',(0.0115695416577292,-0.0331951640388587,
0.0789584806068394));
#92750=CARTESIAN_POINT('Ctrl Pts',(0.0115033145571362,-0.0330855618127431,
0.0790059389782755));
#92751=CARTESIAN_POINT('Ctrl Pts',(0.0114360588308179,-0.0329757224171935,
0.0790520627606689));
#92752=CARTESIAN_POINT('Ctrl Pts',(0.0113678577065632,-0.0328657861694599,
0.0790967886651217));
#92753=CARTESIAN_POINT('Ctrl Pts',(0.0115826144909202,-0.0331951640388587,
0.0788459183881649));
#92754=CARTESIAN_POINT('Ctrl Pts',(0.0115179377073585,-0.0330855618127431,
0.078893556811453));
#92755=CARTESIAN_POINT('Ctrl Pts',(0.011452229694309,-0.0329757224171935,
0.078939892817902));
#92756=CARTESIAN_POINT('Ctrl Pts',(0.0113855716842898,-0.0328657861694599,
0.0789848629440667));
#92757=CARTESIAN_POINT('Ctrl Pts',(0.0115956873241113,-0.0331951640388587,
0.0787333561694903));
#92758=CARTESIAN_POINT('Ctrl Pts',(0.0115325608575808,-0.0330855618127431,
0.0787811746446305));
#92759=CARTESIAN_POINT('Ctrl Pts',(0.0114684005578001,-0.0329757224171935,
0.0788277228751352));
#92760=CARTESIAN_POINT('Ctrl Pts',(0.0114032856620164,-0.0328657861694599,
0.0788729372230117));
#92761=CARTESIAN_POINT('Origin',(0.00209927003337273,-0.0326401908833287,
0.0649203589795844));
#92762=CARTESIAN_POINT('Ctrl Pts',(0.0116241701904994,-0.0332451089994432,
0.0787134864815975));
#92763=CARTESIAN_POINT('Ctrl Pts',(0.0114520554819021,-0.0329451141710258,
0.0788455057748676));
#92764=CARTESIAN_POINT('Ctrl Pts',(0.0112704855001587,-0.0326442513127503,
0.0789641856317969));
#92765=CARTESIAN_POINT('Ctrl Pts',(0.0118191819903634,-0.0332451089994432,
0.0785570563121486));
#92766=CARTESIAN_POINT('Ctrl Pts',(0.0116529671421337,-0.0329451141710258,
0.0786964305957846));
#92767=CARTESIAN_POINT('Ctrl Pts',(0.0114767262519354,-0.0326442513127503,
0.07882288894993));
#92768=CARTESIAN_POINT('Ctrl Pts',(0.0114033116817675,-0.0325229783203385,
0.0788729192646424));
#92769=CARTESIAN_POINT('Ctrl Pts',(0.0113382063441729,-0.0324130253112079,
0.0789181275061021));
#92770=CARTESIAN_POINT('Ctrl Pts',(0.0112721756905466,-0.0323031222247695,
0.078961982103329));
#92771=CARTESIAN_POINT('Ctrl Pts',(0.0112053062836757,-0.0321934096636184,
0.0790044298662736));
#92772=CARTESIAN_POINT('Ctrl Pts',(0.0115143729298709,-0.0325229783203385,
0.0788954257485908));
#92773=CARTESIAN_POINT('Ctrl Pts',(0.0114489573408929,-0.0324130253112079,
0.0789421649668989));
#92774=CARTESIAN_POINT('Ctrl Pts',(0.0113825848127166,-0.0323031222247695,
0.0789875438908234));
#92775=CARTESIAN_POINT('Ctrl Pts',(0.0113153424149455,-0.0321934096636184,
0.0790315073932132));
#92776=CARTESIAN_POINT('Ctrl Pts',(0.0116254341779743,-0.0325229783203385,
0.0789179322325391));
#92777=CARTESIAN_POINT('Ctrl Pts',(0.0115597083376129,-0.0324130253112079,
0.0789662024276958));
#92778=CARTESIAN_POINT('Ctrl Pts',(0.0114929939348867,-0.0323031222247695,
0.0790131056783178));
#92779=CARTESIAN_POINT('Ctrl Pts',(0.0114253785462154,-0.0321934096636184,
0.0790585849201528));
#92780=CARTESIAN_POINT('Ctrl Pts',(0.0117364954260777,-0.0325229783203385,
0.0789404387164875));
#92781=CARTESIAN_POINT('Ctrl Pts',(0.0116704593343329,-0.0324130253112079,
0.0789902398884926));
#92782=CARTESIAN_POINT('Ctrl Pts',(0.0116034030570568,-0.0323031222247695,
0.0790386674658122));
#92783=CARTESIAN_POINT('Ctrl Pts',(0.0115354146774852,-0.0321934096636184,
0.0790856624470925));
#92784=CARTESIAN_POINT('Origin',(0.00169194628218417,-0.0326393375177923,
0.0651753186159354));
#92785=CARTESIAN_POINT('Ctrl Pts',(0.011240700365954,-0.0326943950436593,
0.0792768724485699));
#92786=CARTESIAN_POINT('Ctrl Pts',(0.0111700424548299,-0.0325844576448126,
0.0793198294227188));
#92787=CARTESIAN_POINT('Ctrl Pts',(0.0110984911224813,-0.0324744968375318,
0.0793613281155522));
#92788=CARTESIAN_POINT('Ctrl Pts',(0.0110261387780296,-0.0323646534831894,
0.0794013166210089));
#92789=CARTESIAN_POINT('Ctrl Pts',(0.0112608152239288,-0.0326943950436593,
0.0791653533019131));
#92790=CARTESIAN_POINT('Ctrl Pts',(0.0111916942556548,-0.0325844576448126,
0.0792085874965041));
#92791=CARTESIAN_POINT('Ctrl Pts',(0.0111216742415548,-0.0324744968375318,
0.079250395215897));
#92792=CARTESIAN_POINT('Ctrl Pts',(0.0110508456341974,-0.0323646534831894,
0.0792907241310255));
#92793=CARTESIAN_POINT('Ctrl Pts',(0.0112809300819036,-0.0326943950436593,
0.0790538341552562));
#92794=CARTESIAN_POINT('Ctrl Pts',(0.0112133460564797,-0.0325844576448126,
0.0790973455702894));
#92795=CARTESIAN_POINT('Ctrl Pts',(0.0111448573606284,-0.0324744968375318,
0.0791394623162418));
#92796=CARTESIAN_POINT('Ctrl Pts',(0.0110755524903652,-0.0323646534831894,
0.0791801316410422));
#92797=CARTESIAN_POINT('Ctrl Pts',(0.0113010449398784,-0.0326943950436593,
0.0789423150085994));
#92798=CARTESIAN_POINT('Ctrl Pts',(0.0112349978573045,-0.0325844576448126,
0.0789861036440747));
#92799=CARTESIAN_POINT('Ctrl Pts',(0.0111680404797019,-0.0324744968375318,
0.0790285294165866));
#92800=CARTESIAN_POINT('Ctrl Pts',(0.011100259346533,-0.0323646534831894,
0.0790695391510588));
#92801=CARTESIAN_POINT('Origin',(0.00207820415296465,-0.032639557906635,
0.0648889234867131));
#92802=CARTESIAN_POINT('Ctrl Pts',(0.0113307518470199,-0.0327445246961876,
0.078924250793464));
#92803=CARTESIAN_POINT('Ctrl Pts',(0.0111506880365756,-0.0324436878365475,
0.0790452036300124));
#92804=CARTESIAN_POINT('Ctrl Pts',(0.0109620251064942,-0.0321434074463187,
0.079152249710342));
#92805=CARTESIAN_POINT('Ctrl Pts',(0.0115352001860331,-0.0327445246961876,
0.0787803728011415));
#92806=CARTESIAN_POINT('Ctrl Pts',(0.011360562822723,-0.0324436878365475,
0.0789090365327715));
#92807=CARTESIAN_POINT('Ctrl Pts',(0.0111767301076868,-0.0321434074463187,
0.0790241803445167));
#92808=CARTESIAN_POINT('Ctrl Pts',(0.011019815172185,-0.0322357242816073,
0.0791190157963224));
#92809=CARTESIAN_POINT('Ctrl Pts',(0.0108615584636495,-0.0319819883628705,
0.0792112506906888));
#92810=CARTESIAN_POINT('Ctrl Pts',(0.0106977533117821,-0.0317295851069886,
0.0792932283325005));
#92811=CARTESIAN_POINT('Ctrl Pts',(0.0112330213069529,-0.0322357242816073,
0.078988466402998));
#92812=CARTESIAN_POINT('Ctrl Pts',(0.0110789224272784,-0.0319819883628705,
0.0790874916362385));
#92813=CARTESIAN_POINT('Ctrl Pts',(0.0109188345892279,-0.0317295851069886,
0.0791765104300049));
#92814=CARTESIAN_POINT('Origin',(0.00212886373024658,-0.032637194264519,
0.0649696452976313));
#92815=CARTESIAN_POINT('Origin',(0.00176105284582072,-0.0326352985527993,
0.065276748817572));
#92816=CARTESIAN_POINT('Ctrl Pts',(0.0109126308553257,-0.0321934096636183,
0.0794624686483194));
#92817=CARTESIAN_POINT('Ctrl Pts',(0.0108393677723792,-0.0320835708272304,
0.0795009290448678));
#92818=CARTESIAN_POINT('Ctrl Pts',(0.0107653512490906,-0.0319739230346346,
0.0795378509571295));
#92819=CARTESIAN_POINT('Ctrl Pts',(0.0106906796099296,-0.0318646057455575,
0.0795731944139634));
#92820=CARTESIAN_POINT('Ctrl Pts',(0.0109397084055824,-0.0321934096636183,
0.079352432422295));
#92821=CARTESIAN_POINT('Ctrl Pts',(0.0108679628079498,-0.0320835708272304,
0.0793912662393644));
#92822=CARTESIAN_POINT('Ctrl Pts',(0.0107954551618537,-0.0319739230346346,
0.0794285927598277));
#92823=CARTESIAN_POINT('Ctrl Pts',(0.0107222819009896,-0.0318646057455575,
0.079464371346715));
#92824=CARTESIAN_POINT('Ctrl Pts',(0.010966785955839,-0.0321934096636183,
0.0792423961962706));
#92825=CARTESIAN_POINT('Ctrl Pts',(0.0108965578435203,-0.0320835708272304,
0.079281603433861));
#92826=CARTESIAN_POINT('Ctrl Pts',(0.0108255590746167,-0.0319739230346346,
0.0793193345625259));
#92827=CARTESIAN_POINT('Ctrl Pts',(0.0107538841920495,-0.0318646057455575,
0.0793555482794666));
#92828=CARTESIAN_POINT('Ctrl Pts',(0.0109938635060957,-0.0321934096636183,
0.0791323599702462));
#92829=CARTESIAN_POINT('Ctrl Pts',(0.0109251528790909,-0.0320835708272304,
0.0791719406283576));
#92830=CARTESIAN_POINT('Ctrl Pts',(0.0108556629873797,-0.0319739230346346,
0.0792100763652241));
#92831=CARTESIAN_POINT('Ctrl Pts',(0.0107854864831095,-0.0318646057455575,
0.0792467252122182));
#92832=CARTESIAN_POINT('Ctrl Pts',(0.0111010895863765,-0.0320218834582313,
0.0790700039112242));
#92833=CARTESIAN_POINT('Ctrl Pts',(0.0110498842396934,-0.0319391099350602,
0.0791009904835938));
#92834=CARTESIAN_POINT('Ctrl Pts',(0.0109982260573564,-0.0318564869454876,
0.0791311587033183));
#92835=CARTESIAN_POINT('Ctrl Pts',(0.0109461547168824,-0.0317740741446462,
0.0791604901095118));
#92836=CARTESIAN_POINT('Ctrl Pts',(0.0111489537407645,-0.0320218834582313,
0.0790828822174951));
#92837=CARTESIAN_POINT('Ctrl Pts',(0.0110976143620462,-0.0319391099350602,
0.0791143669400011));
#92838=CARTESIAN_POINT('Ctrl Pts',(0.0110458144501965,-0.0318564869454876,
0.0791450309151164));
#92839=CARTESIAN_POINT('Ctrl Pts',(0.0109935938196735,-0.0317740741446462,
0.0791748553305004));
#92840=CARTESIAN_POINT('Ctrl Pts',(0.0111968178951524,-0.0320218834582313,
0.079095760523766));
#92841=CARTESIAN_POINT('Ctrl Pts',(0.011145344484399,-0.0319391099350602,
0.0791277433964083));
#92842=CARTESIAN_POINT('Ctrl Pts',(0.0110934028430365,-0.0318564869454876,
0.0791589031269145));
#92843=CARTESIAN_POINT('Ctrl Pts',(0.0110410329224647,-0.0317740741446462,
0.079189220551489));
#92844=CARTESIAN_POINT('Ctrl Pts',(0.0112446820495404,-0.0320218834582313,
0.0791086388300369));
#92845=CARTESIAN_POINT('Ctrl Pts',(0.0111930746067518,-0.0319391099350602,
0.0791411198528156));
#92846=CARTESIAN_POINT('Ctrl Pts',(0.0111409912358765,-0.0318564869454876,
0.0791727753387125));
#92847=CARTESIAN_POINT('Ctrl Pts',(0.0110884720252559,-0.0317740741446462,
0.0792035857724777));
#92848=CARTESIAN_POINT('Origin',(0.0151637121232632,-0.0391228853390932,
0.0839642755672192));
#92849=CARTESIAN_POINT('Ctrl Pts',(0.0131920815323775,-0.0352722978779604,
0.076869651880326));
#92850=CARTESIAN_POINT('Ctrl Pts',(0.0131828395632165,-0.0352466642097223,
0.07688613455863));
#92851=CARTESIAN_POINT('Ctrl Pts',(0.0131736742122756,-0.0352210183808304,
0.0769026408966044));
#92852=CARTESIAN_POINT('Ctrl Pts',(0.0131645856216842,-0.0351953608940152,
0.0769191717352508));
#92853=CARTESIAN_POINT('Origin',(0.0173745289028921,-0.0352456003065049,
0.0794224693801586));
#92854=CARTESIAN_POINT('Ctrl Pts',(0.0131021098916861,-0.035024121149334,
0.0770270702921428));
#92855=CARTESIAN_POINT('Ctrl Pts',(0.0130624794298435,-0.0349144232867422,
0.0770956447119049));
#92856=CARTESIAN_POINT('Ctrl Pts',(0.0130214077650672,-0.0348045283677513,
0.0771634409868329));
#92857=CARTESIAN_POINT('Ctrl Pts',(0.0129789442734774,-0.0346945769586886,
0.0772303703208712));
#92858=CARTESIAN_POINT('Ctrl Pts',(0.0132121839095879,-0.035024121149334,
0.0770001472093643));
#92859=CARTESIAN_POINT('Ctrl Pts',(0.013172924302155,-0.0349144232867422,
0.0770702378535225));
#92860=CARTESIAN_POINT('Ctrl Pts',(0.0131321923723223,-0.0348045283677513,
0.0771395589262053));
#92861=CARTESIAN_POINT('Ctrl Pts',(0.0130900369883744,-0.0346945769586886,
0.0772080196944782));
#92862=CARTESIAN_POINT('Ctrl Pts',(0.0133222579274898,-0.035024121149334,
0.0769732241265858));
#92863=CARTESIAN_POINT('Ctrl Pts',(0.0132833691744665,-0.0349144232867422,
0.0770448309951401));
#92864=CARTESIAN_POINT('Ctrl Pts',(0.0132429769795774,-0.0348045283677513,
0.0771156768655777));
#92865=CARTESIAN_POINT('Ctrl Pts',(0.0132011297032715,-0.0346945769586886,
0.0771856690680852));
#92866=CARTESIAN_POINT('Ctrl Pts',(0.0134323319453916,-0.035024121149334,
0.0769463010438072));
#92867=CARTESIAN_POINT('Ctrl Pts',(0.013393814046778,-0.0349144232867422,
0.0770194241367577));
#92868=CARTESIAN_POINT('Ctrl Pts',(0.0133537615868325,-0.0348045283677513,
0.0770917948049501));
#92869=CARTESIAN_POINT('Ctrl Pts',(0.0133122224181685,-0.0346945769586886,
0.0771633184416922));
#92870=CARTESIAN_POINT('Origin',(-0.00110006755546588,-0.0345629067944436,
0.0680846404425669));
#92871=CARTESIAN_POINT('Ctrl Pts',(0.0131038037546256,-0.0351970973651611,
0.0773710102489984));
#92872=CARTESIAN_POINT('Ctrl Pts',(0.0130591810228675,-0.0350869349321773,
0.077440001698609));
#92873=CARTESIAN_POINT('Ctrl Pts',(0.0130130870321533,-0.0349764985129728,
0.0775081226180688));
#92874=CARTESIAN_POINT('Ctrl Pts',(0.0129655763035342,-0.0348659306849652,
0.077575281239486));
#92875=CARTESIAN_POINT('Ctrl Pts',(0.0130825376092316,-0.0351970973651611,
0.0772915859346482));
#92876=CARTESIAN_POINT('Ctrl Pts',(0.0130390151937099,-0.0350869349321773,
0.0773602827706351));
#92877=CARTESIAN_POINT('Ctrl Pts',(0.0129940285555751,-0.0349764985129728,
0.0774281317073815));
#92878=CARTESIAN_POINT('Ctrl Pts',(0.0129476308020129,-0.0348659306849652,
0.0774950414138066));
#92879=CARTESIAN_POINT('Ctrl Pts',(0.0130612714638377,-0.0351970973651611,
0.077212161620298));
#92880=CARTESIAN_POINT('Ctrl Pts',(0.0130188493645523,-0.0350869349321773,
0.0772805638426612));
#92881=CARTESIAN_POINT('Ctrl Pts',(0.012974970078997,-0.0349764985129728,
0.0773481407966943));
#92882=CARTESIAN_POINT('Ctrl Pts',(0.0129296853004916,-0.0348659306849652,
0.0774148015881272));
#92883=CARTESIAN_POINT('Ctrl Pts',(0.0130400053184437,-0.0351970973651611,
0.0771327373059478));
#92884=CARTESIAN_POINT('Ctrl Pts',(0.0129986835353946,-0.0350869349321773,
0.0772008449146873));
#92885=CARTESIAN_POINT('Ctrl Pts',(0.0129559116024188,-0.0349764985129728,
0.077268149886007));
#92886=CARTESIAN_POINT('Ctrl Pts',(0.0129117397989703,-0.0348659306849652,
0.0773345617624478));
#92887=CARTESIAN_POINT('Origin',(-0.000799005175002816,-0.0345637187966945,
0.0677095580521295));
#92888=CARTESIAN_POINT('Ctrl Pts',(0.0130582889654286,-0.0352450361861252,
0.0771044488342036));
#92889=CARTESIAN_POINT('Ctrl Pts',(0.012946860102051,-0.0349452761023764,
0.0772905568062231));
#92890=CARTESIAN_POINT('Ctrl Pts',(0.0128217293827438,-0.0346444289983474,
0.077467742787408));
#92891=CARTESIAN_POINT('Ctrl Pts',(0.0131820207931102,-0.0352450361861252,
0.0768872152391532));
#92892=CARTESIAN_POINT('Ctrl Pts',(0.0130787850290016,-0.0349452761023764,
0.0770779898335093));
#92893=CARTESIAN_POINT('Ctrl Pts',(0.0129614726241525,-0.0346444289983474,
0.0772604463173933));
#92894=CARTESIAN_POINT('Ctrl Pts',(0.0129116341444627,-0.0345231616327822,
0.077333984053815));
#92895=CARTESIAN_POINT('Ctrl Pts',(0.0128677474069721,-0.0344132092796975,
0.0773999778522077));
#92896=CARTESIAN_POINT('Ctrl Pts',(0.0128224979041709,-0.0343032738558973,
0.0774650604830761));
#92897=CARTESIAN_POINT('Ctrl Pts',(0.0127759457416698,-0.034193496108874,
0.0775291500529677));
#92898=CARTESIAN_POINT('Ctrl Pts',(0.0130231814429904,-0.0345231616327822,
0.0773140256889009));
#92899=CARTESIAN_POINT('Ctrl Pts',(0.0129795698034611,-0.0344132092796975,
0.0773815570097577));
#92900=CARTESIAN_POINT('Ctrl Pts',(0.0129345635819879,-0.0343032738558973,
0.0774481827739455));
#92901=CARTESIAN_POINT('Ctrl Pts',(0.01288822262315,-0.034193496108874,
0.077513819103096));
#92902=CARTESIAN_POINT('Ctrl Pts',(0.0131347287415182,-0.0345231616327822,
0.0772940673239867));
#92903=CARTESIAN_POINT('Ctrl Pts',(0.01309139219995,-0.0344132092796975,
0.0773631361673077));
#92904=CARTESIAN_POINT('Ctrl Pts',(0.0130466292598048,-0.0343032738558973,
0.0774313050648149));
#92905=CARTESIAN_POINT('Ctrl Pts',(0.0130004995046302,-0.034193496108874,
0.0774984881532244));
#92906=CARTESIAN_POINT('Ctrl Pts',(0.0132462760400459,-0.0345231616327822,
0.0772741089590726));
#92907=CARTESIAN_POINT('Ctrl Pts',(0.0132032145964389,-0.0344132092796975,
0.0773447153248577));
#92908=CARTESIAN_POINT('Ctrl Pts',(0.0131586949376218,-0.0343032738558973,
0.0774144273556843));
#92909=CARTESIAN_POINT('Ctrl Pts',(0.0131127763861103,-0.034193496108874,
0.0774831572033528));
#92910=CARTESIAN_POINT('Origin',(-0.00111031611238196,-0.0345625596228078,
0.068078201081954));
#92911=CARTESIAN_POINT('Ctrl Pts',(0.0129091470454601,-0.0346945769586886,
0.0777694313406994));
#92912=CARTESIAN_POINT('Ctrl Pts',(0.0128592694522607,-0.0345846629178476,
0.0778353760869727));
#92913=CARTESIAN_POINT('Ctrl Pts',(0.0128080196295779,-0.034474692505516,
0.0779003006486292));
#92914=CARTESIAN_POINT('Ctrl Pts',(0.012755463588148,-0.0343648066260528,
0.0779641221080353));
#92915=CARTESIAN_POINT('Ctrl Pts',(0.0128867964366645,-0.0346945769586886,
0.0776583387132696));
#92916=CARTESIAN_POINT('Ctrl Pts',(0.0128384497560193,-0.0345846629178476,
0.0777239754568573));
#92917=CARTESIAN_POINT('Ctrl Pts',(0.0127887374767434,-0.034474692505516,
0.0777886236218635));
#92918=CARTESIAN_POINT('Ctrl Pts',(0.0127377236380325,-0.0343648066260528,
0.0778522006366695));
#92919=CARTESIAN_POINT('Ctrl Pts',(0.012864445827869,-0.0346945769586886,
0.0775472460858398));
#92920=CARTESIAN_POINT('Ctrl Pts',(0.012817630059778,-0.0345846629178476,
0.0776125748267419));
#92921=CARTESIAN_POINT('Ctrl Pts',(0.0127694553239088,-0.034474692505516,
0.0776769465950977));
#92922=CARTESIAN_POINT('Ctrl Pts',(0.0127199836879171,-0.0343648066260528,
0.0777402791653037));
#92923=CARTESIAN_POINT('Ctrl Pts',(0.0128420952190734,-0.0346945769586886,
0.07743615345841));
#92924=CARTESIAN_POINT('Ctrl Pts',(0.0127968103635366,-0.0345846629178476,
0.0775011741966266));
#92925=CARTESIAN_POINT('Ctrl Pts',(0.0127501731710742,-0.034474692505516,
0.0775652695683319));
#92926=CARTESIAN_POINT('Ctrl Pts',(0.0127022437378016,-0.0343648066260528,
0.0776283576939379));
#92927=CARTESIAN_POINT('Origin',(-0.000846834622031316,-0.0345626446732096,
0.0676759950569512));
#92928=CARTESIAN_POINT('Ctrl Pts',(0.012842495146412,-0.0346945769586885,
0.0774381412780363));
#92929=CARTESIAN_POINT('Ctrl Pts',(0.0127736237108447,-0.034527515336289,
0.0775369766101112));
#92930=CARTESIAN_POINT('Ctrl Pts',(0.0127016261813744,-0.0343603235965158,
0.0776336715628087));
#92931=CARTESIAN_POINT('Ctrl Pts',(0.0126267197451524,-0.0341934961088739,
0.0777279433201761));
#92932=CARTESIAN_POINT('Ctrl Pts',(0.0128889177590261,-0.0346945769586885,
0.0773683346209802));
#92933=CARTESIAN_POINT('Ctrl Pts',(0.0128215084518399,-0.034527515336289,
0.0774681422932629));
#92934=CARTESIAN_POINT('Ctrl Pts',(0.0127509428497275,-0.0343603235965158,
0.0775658558202569));
#92935=CARTESIAN_POINT('Ctrl Pts',(0.0126774339496079,-0.0341934961088739,
0.0776611893105759));
#92936=CARTESIAN_POINT('Ctrl Pts',(0.0129353403716402,-0.0346945769586885,
0.0772985279639242));
#92937=CARTESIAN_POINT('Ctrl Pts',(0.0128693931928351,-0.034527515336289,
0.0773993079764147));
#92938=CARTESIAN_POINT('Ctrl Pts',(0.0128002595180805,-0.0343603235965158,
0.0774980400777052));
#92939=CARTESIAN_POINT('Ctrl Pts',(0.0127281481540635,-0.0341934961088739,
0.0775944353009757));
#92940=CARTESIAN_POINT('Ctrl Pts',(0.0129817629842544,-0.0346945769586885,
0.0772287213068681));
#92941=CARTESIAN_POINT('Ctrl Pts',(0.0129172779338303,-0.034527515336289,
0.0773304736595664));
#92942=CARTESIAN_POINT('Ctrl Pts',(0.0128495761864335,-0.0343603235965158,
0.0774302243351535));
#92943=CARTESIAN_POINT('Ctrl Pts',(0.012778862358519,-0.0341934961088739,
0.0775276812913754));
#92944=CARTESIAN_POINT('Ctrl Pts',(0.0127022623826205,-0.0340223579322366,
0.0776283322317491));
#92945=CARTESIAN_POINT('Ctrl Pts',(0.0126542871092738,-0.0339125849573554,
0.0776914814147395));
#92946=CARTESIAN_POINT('Ctrl Pts',(0.0126050385062468,-0.0338030433565221,
0.077753593246851));
#92947=CARTESIAN_POINT('Ctrl Pts',(0.0125545865953867,-0.0336938721132328,
0.0778145938804907));
#92948=CARTESIAN_POINT('Ctrl Pts',(0.0128148429535926,-0.0340223579322366,
0.0776154173229107));
#92949=CARTESIAN_POINT('Ctrl Pts',(0.0127670458105223,-0.0339125849573554,
0.0776801192855972));
#92950=CARTESIAN_POINT('Ctrl Pts',(0.0127179430736701,-0.0338030433565221,
0.0777437864931673));
#92951=CARTESIAN_POINT('Ctrl Pts',(0.0126676047546669,-0.0336938721132328,
0.0778063430924294));
#92952=CARTESIAN_POINT('Ctrl Pts',(0.0129274235245647,-0.0340223579322366,
0.0776025024140722));
#92953=CARTESIAN_POINT('Ctrl Pts',(0.0128798045117708,-0.0339125849573554,
0.0776687571564549));
#92954=CARTESIAN_POINT('Ctrl Pts',(0.0128308476410933,-0.0338030433565221,
0.0777339797394836));
#92955=CARTESIAN_POINT('Ctrl Pts',(0.012780622913947,-0.0336938721132328,
0.077798092304368));
#92956=CARTESIAN_POINT('Ctrl Pts',(0.0130400040955369,-0.0340223579322366,
0.0775895875052338));
#92957=CARTESIAN_POINT('Ctrl Pts',(0.0129925632130193,-0.0339125849573554,
0.0776573950273126));
#92958=CARTESIAN_POINT('Ctrl Pts',(0.0129437522085166,-0.0338030433565221,
0.0777241729858));
#92959=CARTESIAN_POINT('Ctrl Pts',(0.0128936410732272,-0.0336938721132328,
0.0777898415163066));
#92960=CARTESIAN_POINT('Origin',(-0.00101131372167616,-0.0345589643412299,
0.0681464022903583));
#92961=CARTESIAN_POINT('Ctrl Pts',(0.0126724382467533,-0.0341934961088739,
0.0780627647649451));
#92962=CARTESIAN_POINT('Ctrl Pts',(0.012618483537692,-0.0340836138581106,
0.0781254880383177));
#92963=CARTESIAN_POINT('Ctrl Pts',(0.0125632567905833,-0.0339738896643499,
0.0781870647363929));
#92964=CARTESIAN_POINT('Ctrl Pts',(0.0125068339719022,-0.0338644633294062,
0.0782474207868571));
#92965=CARTESIAN_POINT('Ctrl Pts',(0.0126571072830868,-0.0341934961088739,
0.0779504877824372));
#92966=CARTESIAN_POINT('Ctrl Pts',(0.0126047008071265,-0.0340836138581106,
0.0780129996508995));
#92967=CARTESIAN_POINT('Ctrl Pts',(0.0125510259248284,-0.0339738896643499,
0.0780743970829358));
#92968=CARTESIAN_POINT('Ctrl Pts',(0.012496156601092,-0.0338644633294062,
0.0781346061025266));
#92969=CARTESIAN_POINT('Ctrl Pts',(0.0126417763194202,-0.0341934961088739,
0.0778382107999292));
#92970=CARTESIAN_POINT('Ctrl Pts',(0.0125909180765609,-0.0340836138581106,
0.0779005112634812));
#92971=CARTESIAN_POINT('Ctrl Pts',(0.0125387950590736,-0.0339738896643499,
0.0779617294294786));
#92972=CARTESIAN_POINT('Ctrl Pts',(0.0124854792302818,-0.0338644633294062,
0.078021791418196));
#92973=CARTESIAN_POINT('Ctrl Pts',(0.0126264453557537,-0.0341934961088739,
0.0777259338174213));
#92974=CARTESIAN_POINT('Ctrl Pts',(0.0125771353459954,-0.0340836138581106,
0.0777880228760629));
#92975=CARTESIAN_POINT('Ctrl Pts',(0.0125265641933187,-0.0339738896643499,
0.0778490617760215));
#92976=CARTESIAN_POINT('Ctrl Pts',(0.0124748018594716,-0.0338644633294062,
0.0779089767338654));
#92977=CARTESIAN_POINT('Origin',(-0.000786468836533358,-0.0345610621861424,
0.0677209674668325));
#92978=CARTESIAN_POINT('Ctrl Pts',(0.0126491367289247,-0.03424362768739,
0.0776995480451978));
#92979=CARTESIAN_POINT('Ctrl Pts',(0.0125152633174715,-0.033943005420186,
0.0778702246051515));
#92980=CARTESIAN_POINT('Ctrl Pts',(0.0123689141685249,-0.0336441434784162,
0.0780303323970116));
#92981=CARTESIAN_POINT('Ctrl Pts',(0.0127991167530562,-0.03424362768739,
0.0774995330648552));
#92982=CARTESIAN_POINT('Ctrl Pts',(0.0126727870309459,-0.033943005420186,
0.0776758662146689));
#92983=CARTESIAN_POINT('Ctrl Pts',(0.012533534062986,-0.0336441434784162,
0.0778421827482009));
#92984=CARTESIAN_POINT('Ctrl Pts',(0.0124748198927572,-0.0335235895815128,
0.0779089556666321));
#92985=CARTESIAN_POINT('Ctrl Pts',(0.012423070467304,-0.0334144449262719,
0.0779688562669718));
#92986=CARTESIAN_POINT('Ctrl Pts',(0.0123700240867079,-0.0333049234473133,
0.0780277565816601));
#92987=CARTESIAN_POINT('Ctrl Pts',(0.0123157417586069,-0.0331951640388588,
0.0780855751509399));
#92988=CARTESIAN_POINT('Ctrl Pts',(0.0125879892158179,-0.0335235895815128,
0.0779031352882301));
#92989=CARTESIAN_POINT('Ctrl Pts',(0.0125363199193327,-0.0334144449262719,
0.0779645938871116));
#92990=CARTESIAN_POINT('Ctrl Pts',(0.0124833215726857,-0.0333049234473133,
0.0780250556456975));
#92991=CARTESIAN_POINT('Ctrl Pts',(0.0124290549412329,-0.0331951640388588,
0.078084437113187));
#92992=CARTESIAN_POINT('Ctrl Pts',(0.0127011585388787,-0.0335235895815128,
0.0778973149098281));
#92993=CARTESIAN_POINT('Ctrl Pts',(0.0126495693713615,-0.0334144449262719,
0.0779603315072514));
#92994=CARTESIAN_POINT('Ctrl Pts',(0.0125966190586635,-0.0333049234473133,
0.0780223547097348));
#92995=CARTESIAN_POINT('Ctrl Pts',(0.0125423681238589,-0.0331951640388588,
0.078083299075434));
#92996=CARTESIAN_POINT('Ctrl Pts',(0.0128143278619394,-0.0335235895815128,
0.0778914945314261));
#92997=CARTESIAN_POINT('Ctrl Pts',(0.0127628188233902,-0.0334144449262719,
0.0779560691273912));
#92998=CARTESIAN_POINT('Ctrl Pts',(0.0127099165446413,-0.0333049234473133,
0.0780196537737722));
#92999=CARTESIAN_POINT('Ctrl Pts',(0.012655681306485,-0.0331951640388588,
0.0780821610376811));
#93000=CARTESIAN_POINT('Origin',(0.000698274037872084,-0.0326434571769895,
0.0661346218489206));
#93001=CARTESIAN_POINT('Ctrl Pts',(0.012417925608737,-0.0336938721132443,
0.0783426784828669));
#93002=CARTESIAN_POINT('Ctrl Pts',(0.0123933844702971,-0.0336474569764985,
0.0783678135292279));
#93003=CARTESIAN_POINT('Ctrl Pts',(0.0123685507759787,-0.033601104548885,
0.0783926595683084));
#93004=CARTESIAN_POINT('Ctrl Pts',(0.0123056775743001,-0.0334837508643197,
0.078455564024085));
#93005=CARTESIAN_POINT('Ctrl Pts',(0.0122409679925288,-0.0333660264760478,
0.0785165777936198));
#93006=CARTESIAN_POINT('Ctrl Pts',(0.0123931733065771,-0.0336938721132443,
0.0780036248546317));
#93007=CARTESIAN_POINT('Ctrl Pts',(0.0123706167615333,-0.0336474569764985,
0.0780286150175544));
#93008=CARTESIAN_POINT('Ctrl Pts',(0.0123477692206689,-0.033601104548885,
0.0780533394152957));
#93009=CARTESIAN_POINT('Ctrl Pts',(0.0122899245026739,-0.0334837508643197,
0.0781159359031816));
#93010=CARTESIAN_POINT('Ctrl Pts',(0.0122302503221735,-0.0333660264760478,
0.0781767908444534));
#93011=CARTESIAN_POINT('Ctrl Pts',(0.0123931733065814,-0.0336938721132426,
0.0780036248546481));
#93012=CARTESIAN_POINT('Ctrl Pts',(0.0123706167615404,-0.0336474569765026,
0.0780286150175676));
#93013=CARTESIAN_POINT('Ctrl Pts',(0.0123477692206789,-0.0336011045488949,
0.0780533394153058));
#93014=CARTESIAN_POINT('Ctrl Pts',(0.012290406270396,-0.0334847282606778,
0.0781154145597085));
#93015=CARTESIAN_POINT('Ctrl Pts',(0.0122312439899657,-0.0333679869945434,
0.0781757772650163));
#93016=CARTESIAN_POINT('Ctrl Pts',(0.0123931733065764,-0.0336938721132429,
0.0780036248546325));
#93017=CARTESIAN_POINT('Ctrl Pts',(0.0123125011192406,-0.0335278710435084,
0.0780930007364861));
#93018=CARTESIAN_POINT('Ctrl Pts',(0.0122290545077754,-0.0333620469224321,
0.0781798153172916));
#93019=CARTESIAN_POINT('Ctrl Pts',(0.0121427775317655,-0.0331951640388601,
0.0782640978923517));
#93020=CARTESIAN_POINT('Ctrl Pts',(0.0124479789628948,-0.0336938721132429,
0.0779401869333332));
#93021=CARTESIAN_POINT('Ctrl Pts',(0.0123686347916644,-0.0335278710435084,
0.0780307101225508));
#93022=CARTESIAN_POINT('Ctrl Pts',(0.012286479749851,-0.0333620469224321,
0.0781187132533399));
#93023=CARTESIAN_POINT('Ctrl Pts',(0.0122014583416767,-0.0331951640388601,
0.0782042264269325));
#93024=CARTESIAN_POINT('Ctrl Pts',(0.0125027846192132,-0.0336938721132429,
0.0778767490120339));
#93025=CARTESIAN_POINT('Ctrl Pts',(0.0124247684640883,-0.0335278710435084,
0.0779684195086153));
#93026=CARTESIAN_POINT('Ctrl Pts',(0.0123439049919267,-0.0333620469224321,
0.0780576111893881));
#93027=CARTESIAN_POINT('Ctrl Pts',(0.0122601391515879,-0.0331951640388601,
0.0781443549615133));
#93028=CARTESIAN_POINT('Ctrl Pts',(0.0125575902755317,-0.0336938721132429,
0.0778133110907345));
#93029=CARTESIAN_POINT('Ctrl Pts',(0.0124809021365122,-0.0335278710435084,
0.0779061288946799));
#93030=CARTESIAN_POINT('Ctrl Pts',(0.0124013302340024,-0.0333620469224321,
0.0779965091254364));
#93031=CARTESIAN_POINT('Ctrl Pts',(0.012318819961499,-0.0331951640388601,
0.0780844834960941));
#93032=CARTESIAN_POINT('Ctrl Pts',(0.0122302084623775,-0.0330240426238155,
0.0781747414916993));
#93033=CARTESIAN_POINT('Ctrl Pts',(0.0121747637272139,-0.0329142774063509,
0.0782313115142555));
#93034=CARTESIAN_POINT('Ctrl Pts',(0.0121181218904411,-0.0328043479726686,
0.0782867635414779));
#93035=CARTESIAN_POINT('Ctrl Pts',(0.0120603535580914,-0.0326943950436594,
0.078341024536834));
#93036=CARTESIAN_POINT('Ctrl Pts',(0.012343519775375,-0.0330240426238155,
0.0781760385390808));
#93037=CARTESIAN_POINT('Ctrl Pts',(0.0122880571721201,-0.0329142774063509,
0.0782341695353674));
#93038=CARTESIAN_POINT('Ctrl Pts',(0.0122313651886606,-0.0328043479726686,
0.0782911829451392));
#93039=CARTESIAN_POINT('Ctrl Pts',(0.0121735144401843,-0.0326943950436594,
0.0783470037298471));
#93040=CARTESIAN_POINT('Ctrl Pts',(0.0124568310883725,-0.0330240426238155,
0.0781773355864623));
#93041=CARTESIAN_POINT('Ctrl Pts',(0.0124013506170263,-0.0329142774063509,
0.0782370275564793));
#93042=CARTESIAN_POINT('Ctrl Pts',(0.0123446084868802,-0.0328043479726686,
0.0782956023488005));
#93043=CARTESIAN_POINT('Ctrl Pts',(0.0122866753222772,-0.0326943950436594,
0.0783529829228602));
#93044=CARTESIAN_POINT('Ctrl Pts',(0.01257014240137,-0.0330240426238155,
0.0781786326338438));
#93045=CARTESIAN_POINT('Ctrl Pts',(0.0125146440619325,-0.0329142774063509,
0.0782398855775912));
#93046=CARTESIAN_POINT('Ctrl Pts',(0.0124578517850998,-0.0328043479726686,
0.0783000217524617));
#93047=CARTESIAN_POINT('Ctrl Pts',(0.0123998362043701,-0.0326943950436594,
0.0783589621158732));
#93048=CARTESIAN_POINT('Origin',(0.000612218764699066,-0.0326396682859389,
0.0660457968026155));
#93049=CARTESIAN_POINT('Ctrl Pts',(0.0121461712749856,-0.0331951640388587,
0.0786020092176616));
#93050=CARTESIAN_POINT('Ctrl Pts',(0.0120848538543536,-0.0330855618255041,
0.0786574094900376));
#93051=CARTESIAN_POINT('Ctrl Pts',(0.0120223472019189,-0.0329757224427707,
0.0787115823734241));
#93052=CARTESIAN_POINT('Ctrl Pts',(0.0119587279583793,-0.0328657862078596,
0.07876445456989));
#93053=CARTESIAN_POINT('Ctrl Pts',(0.0121450332381386,-0.0331951640388587,
0.078488696125246));
#93054=CARTESIAN_POINT('Ctrl Pts',(0.0120852764761241,-0.0330855618255041,
0.0785440807234667));
#93055=CARTESIAN_POINT('Ctrl Pts',(0.012024331931322,-0.0329757224427708,
0.0785982701775445));
#93056=CARTESIAN_POINT('Ctrl Pts',(0.0119622742430163,-0.0328657862078596,
0.078651191266451));
#93057=CARTESIAN_POINT('Ctrl Pts',(0.0121438952012916,-0.0331951640388587,
0.0783753830328304));
#93058=CARTESIAN_POINT('Ctrl Pts',(0.0120856990978947,-0.0330855618255041,
0.0784307519568958));
#93059=CARTESIAN_POINT('Ctrl Pts',(0.012026316660725,-0.0329757224427708,
0.0784849579816649));
#93060=CARTESIAN_POINT('Ctrl Pts',(0.0119658205276534,-0.0328657862078596,
0.078537927963012));
#93061=CARTESIAN_POINT('Ctrl Pts',(0.0121427571644447,-0.0331951640388587,
0.0782620699404148));
#93062=CARTESIAN_POINT('Ctrl Pts',(0.0120861217196652,-0.0330855618255041,
0.0783174231903249));
#93063=CARTESIAN_POINT('Ctrl Pts',(0.012028301390128,-0.0329757224427708,
0.0783716457857853));
#93064=CARTESIAN_POINT('Ctrl Pts',(0.0119693668122904,-0.0328657862078596,
0.078424664659573));
#93065=CARTESIAN_POINT('Origin',(0.000989994360189074,-0.0326401908831897,
0.06574820904801));
#93066=CARTESIAN_POINT('Ctrl Pts',(0.0121685251026903,-0.0332451089994432,
0.0782387870811999));
#93067=CARTESIAN_POINT('Ctrl Pts',(0.0120143139748969,-0.0329451141710257,
0.0783913370558828));
#93068=CARTESIAN_POINT('Ctrl Pts',(0.0118490502569198,-0.0326442513127503,
0.0785318378396225));
#93069=CARTESIAN_POINT('Ctrl Pts',(0.0123423932773012,-0.0332451089994432,
0.0780591489509005));
#93070=CARTESIAN_POINT('Ctrl Pts',(0.0121949573124395,-0.0329451141710257,
0.0782182564710759));
#93071=CARTESIAN_POINT('Ctrl Pts',(0.0120359555687373,-0.0326442513127503,
0.0783658065039826));
#93072=CARTESIAN_POINT('Ctrl Pts',(0.0119693903555023,-0.0325229783203385,
0.0784246436001899));
#93073=CARTESIAN_POINT('Ctrl Pts',(0.0119104644880265,-0.0324130253112079,
0.0784776552236457));
#93074=CARTESIAN_POINT('Ctrl Pts',(0.0118504509443035,-0.0323031222247695,
0.0785294398496081));
#93075=CARTESIAN_POINT('Ctrl Pts',(0.0117894289380661,-0.0321934096636184,
0.078579933858253));
#93076=CARTESIAN_POINT('Ctrl Pts',(0.0120823966629012,-0.0325229783203385,
0.0784330529484414));
#93077=CARTESIAN_POINT('Ctrl Pts',(0.0120233548727458,-0.0324130253112079,
0.078487622361345));
#93078=CARTESIAN_POINT('Ctrl Pts',(0.0119631931990498,-0.0323031222247695,
0.0785409621424765));
#93079=CARTESIAN_POINT('Ctrl Pts',(0.0119019911155827,-0.0321934096636184,
0.078593006686664));
#93080=CARTESIAN_POINT('Ctrl Pts',(0.0121954029703001,-0.0325229783203385,
0.0784414622966929));
#93081=CARTESIAN_POINT('Ctrl Pts',(0.012136245257465,-0.0324130253112079,
0.0784975894990444));
#93082=CARTESIAN_POINT('Ctrl Pts',(0.0120759354537961,-0.0323031222247695,
0.078552484435345));
#93083=CARTESIAN_POINT('Ctrl Pts',(0.0120145532930994,-0.0321934096636184,
0.0786060795150751));
#93084=CARTESIAN_POINT('Ctrl Pts',(0.012308409277699,-0.0325229783203385,
0.0784498716449445));
#93085=CARTESIAN_POINT('Ctrl Pts',(0.0122491356421843,-0.0324130253112079,
0.0785075566367438));
#93086=CARTESIAN_POINT('Ctrl Pts',(0.0121886777085424,-0.0323031222247695,
0.0785640067282135));
#93087=CARTESIAN_POINT('Ctrl Pts',(0.012127115470616,-0.0321934096636184,
0.0786191523434861));
#93088=CARTESIAN_POINT('Origin',(0.000617837391061115,-0.0326393375179294,
0.0660522094516855));
#93089=CARTESIAN_POINT('Ctrl Pts',(0.0118586900372337,-0.0326943950436593,
0.0788457920946329));
#93090=CARTESIAN_POINT('Ctrl Pts',(0.0117939732213176,-0.0325844576448127,
0.0788972661246881));
#93091=CARTESIAN_POINT('Ctrl Pts',(0.0117281872579574,-0.0324744968375319,
0.0789474053477826));
#93092=CARTESIAN_POINT('Ctrl Pts',(0.0116614173220466,-0.0323646534831895,
0.0789961466852158));
#93093=CARTESIAN_POINT('Ctrl Pts',(0.0118646692282906,-0.0326943950436593,
0.0787326312495637));
#93094=CARTESIAN_POINT('Ctrl Pts',(0.0118015119809055,-0.0325844576448127,
0.0787841876840779));
#93095=CARTESIAN_POINT('Ctrl Pts',(0.0117372839921901,-0.0324744968375319,
0.0788344415718974));
#93096=CARTESIAN_POINT('Ctrl Pts',(0.0116720684428964,-0.0323646534831895,
0.0788833296598734));
#93097=CARTESIAN_POINT('Ctrl Pts',(0.0118706484193474,-0.0326943950436593,
0.0786194704044945));
#93098=CARTESIAN_POINT('Ctrl Pts',(0.0118090507404934,-0.0325844576448127,
0.0786711092434677));
#93099=CARTESIAN_POINT('Ctrl Pts',(0.0117463807264229,-0.0324744968375319,
0.0787214777960122));
#93100=CARTESIAN_POINT('Ctrl Pts',(0.0116827195637462,-0.0323646534831895,
0.078770512634531));
#93101=CARTESIAN_POINT('Ctrl Pts',(0.0118766276104042,-0.0326943950436593,
0.0785063095594253));
#93102=CARTESIAN_POINT('Ctrl Pts',(0.0118165895000813,-0.0325844576448127,
0.0785580308028574));
#93103=CARTESIAN_POINT('Ctrl Pts',(0.0117554774606557,-0.0324744968375319,
0.078608514020127));
#93104=CARTESIAN_POINT('Ctrl Pts',(0.011693370684596,-0.0323646534831895,
0.0786576956091886));
#93105=CARTESIAN_POINT('Origin',(0.000965154675876512,-0.0326395579066209,
0.0657196616857234));
#93106=CARTESIAN_POINT('Ctrl Pts',(0.0119038362232152,-0.0327445246961876,
0.0784846645232906));
#93107=CARTESIAN_POINT('Ctrl Pts',(0.011740351679812,-0.0324436878365474,
0.0786272315902069));
#93108=CARTESIAN_POINT('Ctrl Pts',(0.0115665928446733,-0.0321434074463186,
0.0787570793153007));
#93109=CARTESIAN_POINT('Ctrl Pts',(0.0120886397319929,-0.0327445246961876,
0.0783162968804865));
#93110=CARTESIAN_POINT('Ctrl Pts',(0.0119315052779819,-0.0324436878365474,
0.0784658339256074));
#93111=CARTESIAN_POINT('Ctrl Pts',(0.0117635534850628,-0.0321434074463186,
0.0786031101426155));
#93112=CARTESIAN_POINT('Ctrl Pts',(0.011619761904527,-0.0322357242816072,
0.0787168644448188));
#93113=CARTESIAN_POINT('Ctrl Pts',(0.0114743131949657,-0.0319819883628704,
0.0788282068645079));
#93114=CARTESIAN_POINT('Ctrl Pts',(0.0113220742185753,-0.0317295851069886,
0.0789300683174863));
#93115=CARTESIAN_POINT('Ctrl Pts',(0.0118149246676354,-0.0322357242816072,
0.0785606226581679));
#93116=CARTESIAN_POINT('Ctrl Pts',(0.0116744520563408,-0.0319819883628704,
0.0786781807587451));
#93117=CARTESIAN_POINT('Ctrl Pts',(0.01152678357198,-0.0317295851069886,
0.0787865619391311));
#93118=CARTESIAN_POINT('Origin',(0.00102553191220463,-0.0326371942646883,
0.0657933976519712));
#93119=CARTESIAN_POINT('Origin',(0.000699111604263792,-0.0326352985529171,
0.0661441784971164));
#93120=CARTESIAN_POINT('Ctrl Pts',(0.0115564688245381,-0.0321934096636184,
0.0790710428255141));
#93121=CARTESIAN_POINT('Ctrl Pts',(0.0114886038087468,-0.0320835708272304,
0.0791183822494348));
#93122=CARTESIAN_POINT('Ctrl Pts',(0.0114197984705051,-0.0319739230346346,
0.0791642897515911));
#93123=CARTESIAN_POINT('Ctrl Pts',(0.0113501453492525,-0.0318646057455575,
0.079208713352703));
#93124=CARTESIAN_POINT('Ctrl Pts',(0.0115695416642065,-0.0321934096636184,
0.0789584805510671));
#93125=CARTESIAN_POINT('Ctrl Pts',(0.0115032289699055,-0.0320835708272304,
0.079006000259635));
#93126=CARTESIAN_POINT('Ctrl Pts',(0.0114359713217632,-0.0319739230346346,
0.079052120067079));
#93127=CARTESIAN_POINT('Ctrl Pts',(0.0113678592999038,-0.0318646057455575,
0.0790967875705166));
#93128=CARTESIAN_POINT('Ctrl Pts',(0.0115826145038749,-0.0321934096636184,
0.0788459182766199));
#93129=CARTESIAN_POINT('Ctrl Pts',(0.0115178541310643,-0.0320835708272304,
0.0788936182698353));
#93130=CARTESIAN_POINT('Ctrl Pts',(0.0114521441730213,-0.0319739230346346,
0.0789399503825667));
#93131=CARTESIAN_POINT('Ctrl Pts',(0.011385573250555,-0.0318646057455575,
0.0789848617883303));
#93132=CARTESIAN_POINT('Ctrl Pts',(0.0115956873435434,-0.0321934096636184,
0.0787333560021728));
#93133=CARTESIAN_POINT('Ctrl Pts',(0.011532479292223,-0.0320835708272304,
0.0787812362800356));
#93134=CARTESIAN_POINT('Ctrl Pts',(0.0114683170242795,-0.0319739230346346,
0.0788277806980545));
#93135=CARTESIAN_POINT('Ctrl Pts',(0.0114032872012063,-0.0318646057455575,
0.078872936006144));
#93136=CARTESIAN_POINT('Ctrl Pts',(0.0116942526276437,-0.0320218834582307,
0.0786580526479372));
#93137=CARTESIAN_POINT('Ctrl Pts',(0.0116473346977258,-0.0319391099350599,
0.078695212613604));
#93138=CARTESIAN_POINT('Ctrl Pts',(0.0115998649361153,-0.0318564869454876,
0.0787316174349374));
#93139=CARTESIAN_POINT('Ctrl Pts',(0.0115518803936972,-0.0317740741446464,
0.0787672438237096));
#93140=CARTESIAN_POINT('Ctrl Pts',(0.0117433534386458,-0.0320218834582307,
0.0786648304356753));
#93141=CARTESIAN_POINT('Ctrl Pts',(0.0116963649683427,-0.0319391099350599,
0.0787025014220842));
#93142=CARTESIAN_POINT('Ctrl Pts',(0.0116488167294251,-0.0318564869454876,
0.0787394158530472));
#93143=CARTESIAN_POINT('Ctrl Pts',(0.0116007458645908,-0.0317740741446464,
0.0787755500744898));
#93144=CARTESIAN_POINT('Ctrl Pts',(0.0117924542496478,-0.0320218834582307,
0.0786716082234135));
#93145=CARTESIAN_POINT('Ctrl Pts',(0.0117453952389596,-0.0319391099350599,
0.0787097902305645));
#93146=CARTESIAN_POINT('Ctrl Pts',(0.0116977685227349,-0.0318564869454876,
0.078747214271157));
#93147=CARTESIAN_POINT('Ctrl Pts',(0.0116496113354845,-0.0317740741446464,
0.07878385632527));
#93148=CARTESIAN_POINT('Ctrl Pts',(0.0118415550606499,-0.0320218834582307,
0.0786783860111516));
#93149=CARTESIAN_POINT('Ctrl Pts',(0.0117944255095765,-0.0319391099350599,
0.0787170790390447));
#93150=CARTESIAN_POINT('Ctrl Pts',(0.0117467203160448,-0.0318564869454876,
0.0787550126892669));
#93151=CARTESIAN_POINT('Ctrl Pts',(0.0116984768063782,-0.0317740741446464,
0.0787921625760503));
#93152=CARTESIAN_POINT('Origin',(0.0163382550649517,-0.0391228853390709,
0.0830045498907383));
#93153=CARTESIAN_POINT('Ctrl Pts',(0.0134929792425902,-0.0352722978779597,
0.0762129802680671));
#93154=CARTESIAN_POINT('Ctrl Pts',(0.0134858759764861,-0.0352466642097219,
0.0762304913014088));
#93155=CARTESIAN_POINT('Ctrl Pts',(0.0134788516897875,-0.0352210183808301,
0.0762480162050482));
#93156=CARTESIAN_POINT('Ctrl Pts',(0.0134719066289087,-0.0351953608940152,
0.0762655557955414));
#93157=CARTESIAN_POINT('Origin',(0.0179623996382882,-0.0352456003065037,
0.0782214683862578));
#93158=CARTESIAN_POINT('Ctrl Pts',(0.0134234468137344,-0.035024121149334,
0.0763804338253446));
#93159=CARTESIAN_POINT('Ctrl Pts',(0.0133927235036891,-0.0349144232867422,
0.076453434529255));
#93160=CARTESIAN_POINT('Ctrl Pts',(0.0133604728276174,-0.0348045283677513,
0.0765258438548597));
#93161=CARTESIAN_POINT('Ctrl Pts',(0.0133267326431973,-0.0346945769586886,
0.0765975675178176));
#93162=CARTESIAN_POINT('Ctrl Pts',(0.013529278508105,-0.035024121149334,
0.0763399271065204));
#93163=CARTESIAN_POINT('Ctrl Pts',(0.0134991131614779,-0.0349144232867422,
0.0764143855985624));
#93164=CARTESIAN_POINT('Ctrl Pts',(0.0134673906492715,-0.0348045283677513,
0.0764882651183571));
#93165=CARTESIAN_POINT('Ctrl Pts',(0.0134341480825772,-0.0346945769586886,
0.0765614695236062));
#93166=CARTESIAN_POINT('Ctrl Pts',(0.0136351102024756,-0.035024121149334,
0.0762994203876963));
#93167=CARTESIAN_POINT('Ctrl Pts',(0.0136055028192668,-0.0349144232867422,
0.0763753366678697));
#93168=CARTESIAN_POINT('Ctrl Pts',(0.0135743084709256,-0.0348045283677513,
0.0764506863818545));
#93169=CARTESIAN_POINT('Ctrl Pts',(0.013541563521957,-0.0346945769586886,
0.0765253715293948));
#93170=CARTESIAN_POINT('Ctrl Pts',(0.0137409418968463,-0.035024121149334,
0.0762589136688721));
#93171=CARTESIAN_POINT('Ctrl Pts',(0.0137118924770557,-0.0349144232867422,
0.0763362877371771));
#93172=CARTESIAN_POINT('Ctrl Pts',(0.0136812262925797,-0.0348045283677513,
0.0764131076453519));
#93173=CARTESIAN_POINT('Ctrl Pts',(0.0136489789613369,-0.0346945769586886,
0.0764892735351834));
#93174=CARTESIAN_POINT('Origin',(-0.001787525871552,-0.0345629067946148,
0.0692885225293325));
#93175=CARTESIAN_POINT('Ctrl Pts',(0.0134682344270035,-0.0351970973651615,
0.0767214494155905));
#93176=CARTESIAN_POINT('Ctrl Pts',(0.0134326104802814,-0.0350869349321775,
0.076795489558276));
#93177=CARTESIAN_POINT('Ctrl Pts',(0.0133954177695608,-0.0349764985129729,
0.0768688504328433));
#93178=CARTESIAN_POINT('Ctrl Pts',(0.0133566988844116,-0.0348659306849652,
0.0769414341617182));
#93179=CARTESIAN_POINT('Ctrl Pts',(0.0134371814653768,-0.0351970973651615,
0.0766453167404497));
#93180=CARTESIAN_POINT('Ctrl Pts',(0.0134026122336908,-0.0350869349321775,
0.0767189266864361));
#93181=CARTESIAN_POINT('Ctrl Pts',(0.0133664840552708,-0.0349764985129729,
0.0767918789348754));
#93182=CARTESIAN_POINT('Ctrl Pts',(0.0133288381717169,-0.0348659306849652,
0.0768640762187645));
#93183=CARTESIAN_POINT('Ctrl Pts',(0.0134061285037501,-0.0351970973651615,
0.076569184065309));
#93184=CARTESIAN_POINT('Ctrl Pts',(0.0133726139871001,-0.0350869349321775,
0.0766423638145962));
#93185=CARTESIAN_POINT('Ctrl Pts',(0.0133375503409809,-0.0349764985129729,
0.0767149074369076));
#93186=CARTESIAN_POINT('Ctrl Pts',(0.0133009774590221,-0.0348659306849652,
0.0767867182758109));
#93187=CARTESIAN_POINT('Ctrl Pts',(0.0133750755421234,-0.0351970973651615,
0.0764930513901682));
#93188=CARTESIAN_POINT('Ctrl Pts',(0.0133426157405095,-0.0350869349321775,
0.0765658009427563));
#93189=CARTESIAN_POINT('Ctrl Pts',(0.0133086166266909,-0.0349764985129729,
0.0766379359389398));
#93190=CARTESIAN_POINT('Ctrl Pts',(0.0132731167463274,-0.0348659306849652,
0.0767093603328572));
#93191=CARTESIAN_POINT('Origin',(-0.00153584774646322,-0.0345637187967202,
0.0688786646538233));
#93192=CARTESIAN_POINT('Ctrl Pts',(0.0133896695314542,-0.0352450361861253,
0.076462694432875));
#93193=CARTESIAN_POINT('Ctrl Pts',(0.0133024448318717,-0.0349452761023765,
0.0766613006277069));
#93194=CARTESIAN_POINT('Ctrl Pts',(0.0132005080976252,-0.0346444289983475,
0.0768527724821762));
#93195=CARTESIAN_POINT('Ctrl Pts',(0.0134851991078111,-0.0352450361861253,
0.0762316660795478));
#93196=CARTESIAN_POINT('Ctrl Pts',(0.0134066877853302,-0.0349452761023765,
0.076433875231381));
#93197=CARTESIAN_POINT('Ctrl Pts',(0.0133131682849427,-0.0346444289983475,
0.0766295961344295));
#93198=CARTESIAN_POINT('Ctrl Pts',(0.0132729395188461,-0.0345231616327823,
0.0767088004216502));
#93199=CARTESIAN_POINT('Ctrl Pts',(0.0132376700575367,-0.0344132092796975,
0.0767797743059514));
#93200=CARTESIAN_POINT('Ctrl Pts',(0.013200934377156,-0.0343032738558974,
0.0768500150073395));
#93201=CARTESIAN_POINT('Ctrl Pts',(0.013162781845393,-0.034193496108874,
0.0769194337448856));
#93202=CARTESIAN_POINT('Ctrl Pts',(0.0133811057871956,-0.0345231616327823,
0.076675018850785));
#93203=CARTESIAN_POINT('Ctrl Pts',(0.0133463019572799,-0.0344132092796975,
0.0767474836548095));
#93204=CARTESIAN_POINT('Ctrl Pts',(0.0133100010457701,-0.0343032738558974,
0.0768192248302143));
#93205=CARTESIAN_POINT('Ctrl Pts',(0.0132722519126058,-0.034193496108874,
0.0768901516595225));
#93206=CARTESIAN_POINT('Ctrl Pts',(0.0134892720555451,-0.0345231616327823,
0.0766412372799198));
#93207=CARTESIAN_POINT('Ctrl Pts',(0.0134549338570232,-0.0344132092796976,
0.0767151930036676));
#93208=CARTESIAN_POINT('Ctrl Pts',(0.0134190677143842,-0.0343032738558974,
0.0767884346530891));
#93209=CARTESIAN_POINT('Ctrl Pts',(0.0133817219798186,-0.034193496108874,
0.0768608695741595));
#93210=CARTESIAN_POINT('Ctrl Pts',(0.0135974383238946,-0.0345231616327823,
0.0766074557090546));
#93211=CARTESIAN_POINT('Ctrl Pts',(0.0135635657567664,-0.0344132092796976,
0.0766829023525256));
#93212=CARTESIAN_POINT('Ctrl Pts',(0.0135281343829983,-0.0343032738558974,
0.0767576444759639));
#93213=CARTESIAN_POINT('Ctrl Pts',(0.0134911920470314,-0.034193496108874,
0.0768315874887964));
#93214=CARTESIAN_POINT('Origin',(-0.00179850068158374,-0.0345625596231899,
0.0692834184300123));
#93215=CARTESIAN_POINT('Ctrl Pts',(0.0133250480478741,-0.0346945769586886,
0.0771411257927765));
#93216=CARTESIAN_POINT('Ctrl Pts',(0.0132838288225909,-0.0345846629176053,
0.0772128018652248));
#93217=CARTESIAN_POINT('Ctrl Pts',(0.0132411203252203,-0.0344746925050311,
0.0772836377834714));
#93218=CARTESIAN_POINT('Ctrl Pts',(0.0131969776536493,-0.0343648066253259,
0.0773535430103733));
#93219=CARTESIAN_POINT('Ctrl Pts',(0.0132889500820837,-0.0346945769586886,
0.0770337104379681));
#93220=CARTESIAN_POINT('Ctrl Pts',(0.0132492110946827,-0.0345846629176053,
0.0771048890622021));
#93221=CARTESIAN_POINT('Ctrl Pts',(0.0132079933750472,-0.0344746925050311,
0.0771752580579806));
#93222=CARTESIAN_POINT('Ctrl Pts',(0.0131653501084374,-0.0343648066253259,
0.0772447274785468));
#93223=CARTESIAN_POINT('Ctrl Pts',(0.0132528521162933,-0.0346945769586886,
0.0769262950831597));
#93224=CARTESIAN_POINT('Ctrl Pts',(0.0132145933667745,-0.0345846629176053,
0.0769969762591795));
#93225=CARTESIAN_POINT('Ctrl Pts',(0.0131748664248742,-0.0344746925050311,
0.0770668783324899));
#93226=CARTESIAN_POINT('Ctrl Pts',(0.0131337225632256,-0.0343648066253259,
0.0771359119467202));
#93227=CARTESIAN_POINT('Ctrl Pts',(0.013216754150503,-0.0346945769586886,
0.0768188797283513));
#93228=CARTESIAN_POINT('Ctrl Pts',(0.0131799756388663,-0.0345846629176053,
0.0768890634561569));
#93229=CARTESIAN_POINT('Ctrl Pts',(0.0131417394747012,-0.0344746925050311,
0.0769584986069991));
#93230=CARTESIAN_POINT('Ctrl Pts',(0.0131020950180138,-0.0343648066253259,
0.0770270964148937));
#93231=CARTESIAN_POINT('Origin',(-0.00158750660273259,-0.0345626446733096,
0.0688513609322516));
#93232=CARTESIAN_POINT('Ctrl Pts',(0.0132174000641565,-0.0346945769586885,
0.0768208017492395));
#93233=CARTESIAN_POINT('Ctrl Pts',(0.0131614590521889,-0.034527515336289,
0.0769274896149203));
#93234=CARTESIAN_POINT('Ctrl Pts',(0.013102148335834,-0.0343603235965158,
0.0770324457822115));
#93235=CARTESIAN_POINT('Ctrl Pts',(0.0130396479434197,-0.0341934961088739,
0.077135362444481));
#93236=CARTESIAN_POINT('Ctrl Pts',(0.0132547075265512,-0.0346945769586885,
0.0767457272423751));
#93237=CARTESIAN_POINT('Ctrl Pts',(0.0132003389801881,-0.034527515336289,
0.0768531965277928));
#93238=CARTESIAN_POINT('Ctrl Pts',(0.0131425765612264,-0.0343603235965158,
0.076958983769532));
#93239=CARTESIAN_POINT('Ctrl Pts',(0.013081595755349,-0.0341934961088739,
0.0770627786349528));
#93240=CARTESIAN_POINT('Ctrl Pts',(0.013292014988946,-0.0346945769586885,
0.0766706527355107));
#93241=CARTESIAN_POINT('Ctrl Pts',(0.0132392189081873,-0.034527515336289,
0.0767789034406653));
#93242=CARTESIAN_POINT('Ctrl Pts',(0.0131830047866187,-0.0343603235965158,
0.0768855217568525));
#93243=CARTESIAN_POINT('Ctrl Pts',(0.0131235435672782,-0.0341934961088739,
0.0769901948254245));
#93244=CARTESIAN_POINT('Ctrl Pts',(0.0133293224513408,-0.0346945769586885,
0.0765955782286463));
#93245=CARTESIAN_POINT('Ctrl Pts',(0.0132780988361865,-0.034527515336289,
0.0767046103535378));
#93246=CARTESIAN_POINT('Ctrl Pts',(0.013223433012011,-0.0343603235965158,
0.076812059744173));
#93247=CARTESIAN_POINT('Ctrl Pts',(0.0131654913792074,-0.0341934961088739,
0.0769176110158964));
#93248=CARTESIAN_POINT('Ctrl Pts',(0.0131021103248165,-0.0340223579322365,
0.0770270688162126));
#93249=CARTESIAN_POINT('Ctrl Pts',(0.0130624280421308,-0.0339125849573554,
0.077095732945173));
#93250=CARTESIAN_POINT('Ctrl Pts',(0.0130213524558096,-0.0338030433565221,
0.0771635274936023));
#93251=CARTESIAN_POINT('Ctrl Pts',(0.0129789437799994,-0.0336938721132327,
0.0772303704201534));
#93252=CARTESIAN_POINT('Ctrl Pts',(0.013212184497074,-0.0340223579322365,
0.0770001456582915));
#93253=CARTESIAN_POINT('Ctrl Pts',(0.0131728735549546,-0.0339125849573554,
0.0770703279971728));
#93254=CARTESIAN_POINT('Ctrl Pts',(0.0131321376248455,-0.0338030433565221,
0.0771396473745813));
#93255=CARTESIAN_POINT('Ctrl Pts',(0.0130900366593892,-0.0336938721132327,
0.0772080197606663));
#93256=CARTESIAN_POINT('Ctrl Pts',(0.0133222586693315,-0.0340223579322365,
0.0769732225003704));
#93257=CARTESIAN_POINT('Ctrl Pts',(0.0132833190677784,-0.0339125849573554,
0.0770449230491726));
#93258=CARTESIAN_POINT('Ctrl Pts',(0.0132429227938813,-0.0338030433565221,
0.0771157672555604));
#93259=CARTESIAN_POINT('Ctrl Pts',(0.013201129538779,-0.0336938721132327,
0.0771856691011792));
#93260=CARTESIAN_POINT('Ctrl Pts',(0.0134323328415891,-0.0340223579322365,
0.0769462993424493));
#93261=CARTESIAN_POINT('Ctrl Pts',(0.0133937645806022,-0.0339125849573554,
0.0770195181011725));
#93262=CARTESIAN_POINT('Ctrl Pts',(0.0133537079629172,-0.0338030433565221,
0.0770918871365395));
#93263=CARTESIAN_POINT('Ctrl Pts',(0.0133122224181688,-0.0336938721132327,
0.0771633184416921));
#93264=CARTESIAN_POINT('Origin',(-0.00169173107631589,-0.0345589643414446,
0.0693386735614597));
#93265=CARTESIAN_POINT('Ctrl Pts',(0.0131269701953199,-0.034193496108874,
0.0774618136745128));
#93266=CARTESIAN_POINT('Ctrl Pts',(0.0130813022459265,-0.0340836138581107,
0.077530804674293));
#93267=CARTESIAN_POINT('Ctrl Pts',(0.0130342285848961,-0.03397388966435,
0.0775988175685062));
#93268=CARTESIAN_POINT('Ctrl Pts',(0.0129858152959628,-0.0338644633294062,
0.0776657693477972));
#93269=CARTESIAN_POINT('Ctrl Pts',(0.0130976880836083,-0.034193496108874,
0.0773523435087971));
#93270=CARTESIAN_POINT('Ctrl Pts',(0.0130535296629745,-0.0340836138581107,
0.0774209307255971));
#93271=CARTESIAN_POINT('Ctrl Pts',(0.013007973161845,-0.03397388966435,
0.0774885712671029));
#93272=CARTESIAN_POINT('Ctrl Pts',(0.0129610826902299,-0.0338644633294062,
0.077555182470358));
#93273=CARTESIAN_POINT('Ctrl Pts',(0.0130684059718968,-0.034193496108874,
0.0772428733430816));
#93274=CARTESIAN_POINT('Ctrl Pts',(0.0130257570800226,-0.0340836138581107,
0.0773110567769012));
#93275=CARTESIAN_POINT('Ctrl Pts',(0.0129817177387938,-0.03397388966435,
0.0773783249656995));
#93276=CARTESIAN_POINT('Ctrl Pts',(0.0129363500844969,-0.0338644633294062,
0.0774445955929188));
#93277=CARTESIAN_POINT('Ctrl Pts',(0.0130391238601852,-0.034193496108874,
0.077133403177366));
#93278=CARTESIAN_POINT('Ctrl Pts',(0.0129979844970706,-0.0340836138581107,
0.0772011828282052));
#93279=CARTESIAN_POINT('Ctrl Pts',(0.0129554623157426,-0.03397388966435,
0.0772680786642962));
#93280=CARTESIAN_POINT('Ctrl Pts',(0.012911617478764,-0.0338644633294062,
0.0773340087154796));
#93281=CARTESIAN_POINT('Origin',(-0.00152198028231409,-0.0345610621864561,
0.0688884128822638));
#93282=CARTESIAN_POINT('Ctrl Pts',(0.0130583292909483,-0.0342436276873899,
0.0771043814816642));
#93283=CARTESIAN_POINT('Ctrl Pts',(0.0129469029564832,-0.033943005420186,
0.0772904909935097));
#93284=CARTESIAN_POINT('Ctrl Pts',(0.012821774641561,-0.0336441434784162,
0.0774676786996759));
#93285=CARTESIAN_POINT('Ctrl Pts',(0.0131820581535451,-0.0342436276873899,
0.0768871461977886));
#93286=CARTESIAN_POINT('Ctrl Pts',(0.0130788249828772,-0.033943005420186,
0.0770779222206153));
#93287=CARTESIAN_POINT('Ctrl Pts',(0.0129615150551054,-0.0336441434784162,
0.0772603803233617));
#93288=CARTESIAN_POINT('Ctrl Pts',(0.0129116327294273,-0.0335235895815128,
0.0773339855541979));
#93289=CARTESIAN_POINT('Ctrl Pts',(0.0128677988995837,-0.0334144449262719,
0.0773998997432397));
#93290=CARTESIAN_POINT('Ctrl Pts',(0.0128225529724405,-0.0333049234473133,
0.077464984085763));
#93291=CARTESIAN_POINT('Ctrl Pts',(0.0127759452649579,-0.0331951640388588,
0.0775291501180608));
#93292=CARTESIAN_POINT('Ctrl Pts',(0.0130231801917276,-0.0335235895815128,
0.0773140271940187));
#93293=CARTESIAN_POINT('Ctrl Pts',(0.0129796211280063,-0.0334144449262719,
0.0773814770534957));
#93294=CARTESIAN_POINT('Ctrl Pts',(0.0129346185568629,-0.0333049234473133,
0.0774481045072149));
#93295=CARTESIAN_POINT('Ctrl Pts',(0.012888222305342,-0.0331951640388588,
0.0775138191464914));
#93296=CARTESIAN_POINT('Ctrl Pts',(0.013134727654028,-0.0335235895815128,
0.0772940688338394));
#93297=CARTESIAN_POINT('Ctrl Pts',(0.0130914433564288,-0.0334144449262719,
0.0773630543637517));
#93298=CARTESIAN_POINT('Ctrl Pts',(0.0130466841412852,-0.0333049234473133,
0.0774312249286668));
#93299=CARTESIAN_POINT('Ctrl Pts',(0.0130004993457262,-0.0331951640388588,
0.0774984881749221));
#93300=CARTESIAN_POINT('Ctrl Pts',(0.0132462751163283,-0.0335235895815128,
0.0772741104736601));
#93301=CARTESIAN_POINT('Ctrl Pts',(0.0132032655848514,-0.0334144449262719,
0.0773446316740077));
#93302=CARTESIAN_POINT('Ctrl Pts',(0.0131587497257076,-0.0333049234473133,
0.0774143453501187));
#93303=CARTESIAN_POINT('Ctrl Pts',(0.0131127763861104,-0.0331951640388588,
0.0774831572033528));
#93304=CARTESIAN_POINT('Origin',(-0.000247766874356772,-0.0326434571769543,
0.0671284884476075));
#93305=CARTESIAN_POINT('Ctrl Pts',(0.0129095469568594,-0.0336938721132437,
0.0777714190810689));
#93306=CARTESIAN_POINT('Ctrl Pts',(0.0128883495892626,-0.0336474569764982,
0.0777994317503177));
#93307=CARTESIAN_POINT('Ctrl Pts',(0.0128668257504606,-0.033601104548885,
0.0778271943581689));
#93308=CARTESIAN_POINT('Ctrl Pts',(0.0128123323439931,-0.0334837508694633,
0.0778974828921133));
#93309=CARTESIAN_POINT('Ctrl Pts',(0.0127557800721974,-0.0333660264863652,
0.0779661258080421));
#93310=CARTESIAN_POINT('Ctrl Pts',(0.0128424951464166,-0.0336938721132437,
0.0774381412780297));
#93311=CARTESIAN_POINT('Ctrl Pts',(0.0128232485643943,-0.0336474569764982,
0.0774657614707818));
#93312=CARTESIAN_POINT('Ctrl Pts',(0.0128036799719308,-0.033601104548885,
0.0774931544654374));
#93313=CARTESIAN_POINT('Ctrl Pts',(0.0127541367992225,-0.0334837508694633,
0.0775625072238309));
#93314=CARTESIAN_POINT('Ctrl Pts',(0.0127025603163759,-0.0333660264863652,
0.0776303614608095));
#93315=CARTESIAN_POINT('Ctrl Pts',(0.012842495146422,-0.0336938721132426,
0.0774381412780463));
#93316=CARTESIAN_POINT('Ctrl Pts',(0.012823248564402,-0.0336474569765026,
0.0774657614707951));
#93317=CARTESIAN_POINT('Ctrl Pts',(0.0128036799719408,-0.0336011045488949,
0.0774931544654473));
#93318=CARTESIAN_POINT('Ctrl Pts',(0.012754549426385,-0.033484728265791,
0.0775619296098196));
#93319=CARTESIAN_POINT('Ctrl Pts',(0.012703419113583,-0.0333679870047996,
0.0776292313341869));
#93320=CARTESIAN_POINT('Ctrl Pts',(0.0128424951464162,-0.0336938721132429,
0.0774381412780302));
#93321=CARTESIAN_POINT('Ctrl Pts',(0.0127736608516485,-0.0335278710435084,
0.0775369233104576));
#93322=CARTESIAN_POINT('Ctrl Pts',(0.0127017529937719,-0.033362046922432,
0.0776335119660081));
#93323=CARTESIAN_POINT('Ctrl Pts',(0.012626719745153,-0.0331951640388601,
0.0777279433201753));
#93324=CARTESIAN_POINT('Ctrl Pts',(0.0128889177639579,-0.0336938721132429,
0.0773683346135643));
#93325=CARTESIAN_POINT('Ctrl Pts',(0.0128215448092338,-0.0335278710435084,
0.0774680884619416));
#93326=CARTESIAN_POINT('Ctrl Pts',(0.0127510673014092,-0.033362046922432,
0.0775656944188034));
#93327=CARTESIAN_POINT('Ctrl Pts',(0.0126774339549917,-0.0331951640388601,
0.0776611893034893));
#93328=CARTESIAN_POINT('Ctrl Pts',(0.0129353403814995,-0.0336938721132429,
0.0772985279490984));
#93329=CARTESIAN_POINT('Ctrl Pts',(0.012869428766819,-0.0335278710435084,
0.0773992536134257));
#93330=CARTESIAN_POINT('Ctrl Pts',(0.0128003816090465,-0.033362046922432,
0.0774978768715986));
#93331=CARTESIAN_POINT('Ctrl Pts',(0.0127281481648304,-0.0331951640388601,
0.0775944352868034));
#93332=CARTESIAN_POINT('Ctrl Pts',(0.0129817629990412,-0.0336938721132429,
0.0772287212846325));
#93333=CARTESIAN_POINT('Ctrl Pts',(0.0129173127244043,-0.0335278710435084,
0.0773304187649098));
#93334=CARTESIAN_POINT('Ctrl Pts',(0.0128496959166838,-0.033362046922432,
0.0774300593243939));
#93335=CARTESIAN_POINT('Ctrl Pts',(0.0127788623746691,-0.0331951640388601,
0.0775276812701174));
#93336=CARTESIAN_POINT('Ctrl Pts',(0.0127022619301293,-0.0330240426238156,
0.0776283335201845));
#93337=CARTESIAN_POINT('Ctrl Pts',(0.0126543444971128,-0.0329142774063509,
0.0776914065391582));
#93338=CARTESIAN_POINT('Ctrl Pts',(0.0126050992800205,-0.0328043479726686,
0.0777535204151411));
#93339=CARTESIAN_POINT('Ctrl Pts',(0.0125545871742304,-0.0326943950436595,
0.0778145938382327));
#93340=CARTESIAN_POINT('Ctrl Pts',(0.0128148423127214,-0.0330240426238156,
0.0776154186667026));
#93341=CARTESIAN_POINT('Ctrl Pts',(0.012767102794394,-0.0329142774063509,
0.0776800425901283));
#93342=CARTESIAN_POINT('Ctrl Pts',(0.0127180035191604,-0.0328043479726686,
0.0777437118217391));
#93343=CARTESIAN_POINT('Ctrl Pts',(0.0126676051405626,-0.0326943950436595,
0.0778063430642574));
#93344=CARTESIAN_POINT('Ctrl Pts',(0.0129274226953136,-0.0330240426238156,
0.0776025038132207));
#93345=CARTESIAN_POINT('Ctrl Pts',(0.0128798610916752,-0.0329142774063509,
0.0776686786410984));
#93346=CARTESIAN_POINT('Ctrl Pts',(0.0128309077583004,-0.0328043479726686,
0.0777339032283372));
#93347=CARTESIAN_POINT('Ctrl Pts',(0.0127806231068947,-0.0326943950436595,
0.077798092290282));
#93348=CARTESIAN_POINT('Ctrl Pts',(0.0130400030779058,-0.0330240426238156,
0.0775895889597388));
#93349=CARTESIAN_POINT('Ctrl Pts',(0.0129926193889564,-0.0329142774063509,
0.0776573146920685));
#93350=CARTESIAN_POINT('Ctrl Pts',(0.0129438119974403,-0.0328043479726686,
0.0777240946349353));
#93351=CARTESIAN_POINT('Ctrl Pts',(0.0128936410732269,-0.0326943950436595,
0.0777898415163066));
#93352=CARTESIAN_POINT('Origin',(-0.000344276306308796,-0.0326396682859005,
0.0670511493989361));
#93353=CARTESIAN_POINT('Ctrl Pts',(0.0126724382467533,-0.0331951640388588,
0.0780627647649451));
#93354=CARTESIAN_POINT('Ctrl Pts',(0.0126185478275749,-0.0330855618255041,
0.0781254133002278));
#93355=CARTESIAN_POINT('Ctrl Pts',(0.0125633237214108,-0.0329757224427708,
0.078186993175117));
#93356=CARTESIAN_POINT('Ctrl Pts',(0.0125068327779574,-0.0328657862078596,
0.0782474220640313));
#93357=CARTESIAN_POINT('Ctrl Pts',(0.0126571072873892,-0.0331951640388588,
0.0779504878139458));
#93358=CARTESIAN_POINT('Ctrl Pts',(0.0126047632560763,-0.0330855618255041,
0.0780129251962775));
#93359=CARTESIAN_POINT('Ctrl Pts',(0.0125510910167178,-0.0329757224427708,
0.0780743257271925));
#93360=CARTESIAN_POINT('Ctrl Pts',(0.0124961554430166,-0.0328657862078596,
0.078134607408249));
#93361=CARTESIAN_POINT('Ctrl Pts',(0.012641776328025,-0.0331951640388588,
0.0778382108629465));
#93362=CARTESIAN_POINT('Ctrl Pts',(0.0125909786845777,-0.0330855618255041,
0.0779004370923273));
#93363=CARTESIAN_POINT('Ctrl Pts',(0.0125388583120248,-0.0329757224427708,
0.077961658279268));
#93364=CARTESIAN_POINT('Ctrl Pts',(0.0124854781080758,-0.0328657862078596,
0.0780217927524668));
#93365=CARTESIAN_POINT('Ctrl Pts',(0.0126264453686608,-0.0331951640388588,
0.0777259339119473));
#93366=CARTESIAN_POINT('Ctrl Pts',(0.0125771941130792,-0.0330855618255041,
0.0777879489883771));
#93367=CARTESIAN_POINT('Ctrl Pts',(0.0125266256073318,-0.0329757224427708,
0.0778489908313435));
#93368=CARTESIAN_POINT('Ctrl Pts',(0.012474800773135,-0.0328657862078596,
0.0779089780966845));
#93369=CARTESIAN_POINT('Origin',(-6.77721975676001E-6,-0.0326401908831744,
0.0667085603757756));
#93370=CARTESIAN_POINT('Ctrl Pts',(0.0126490920029848,-0.0332451089994431,
0.0776996050660091));
#93371=CARTESIAN_POINT('Ctrl Pts',(0.0125152164576019,-0.0329451141710257,
0.077870279917875));
#93372=CARTESIAN_POINT('Ctrl Pts',(0.0123688653109474,-0.0326442513127503,
0.0780303858471343));
#93373=CARTESIAN_POINT('Ctrl Pts',(0.0127990745473651,-0.0332451089994431,
0.0774995919754844));
#93374=CARTESIAN_POINT('Ctrl Pts',(0.0126727426191114,-0.0329451141710257,
0.0776759235115599));
#93375=CARTESIAN_POINT('Ctrl Pts',(0.0125334875743865,-0.0326442513127503,
0.0778422382710665));
#93376=CARTESIAN_POINT('Ctrl Pts',(0.012474821491261,-0.0325229783203385,
0.0779089542526142));
#93377=CARTESIAN_POINT('Ctrl Pts',(0.0124230043900348,-0.0324130253112079,
0.0779689332330966));
#93378=CARTESIAN_POINT('Ctrl Pts',(0.01236995440565,-0.0323031222247695,
0.0780278312133084));
#93379=CARTESIAN_POINT('Ctrl Pts',(0.0123157421535373,-0.0321934096636185,
0.0780855751469736));
#93380=CARTESIAN_POINT('Ctrl Pts',(0.012587990680981,-0.0325229783203385,
0.0779031338447236));
#93381=CARTESIAN_POINT('Ctrl Pts',(0.0125362538139488,-0.0324130253112079,
0.077964672859983));
#93382=CARTESIAN_POINT('Ctrl Pts',(0.0124832517802662,-0.0323031222247695,
0.0780251322981094));
#93383=CARTESIAN_POINT('Ctrl Pts',(0.0124290552045198,-0.0321934096636185,
0.0780844371105427));
#93384=CARTESIAN_POINT('Ctrl Pts',(0.0127011598707009,-0.0325229783203385,
0.077897313436833));
#93385=CARTESIAN_POINT('Ctrl Pts',(0.0126495032378628,-0.0324130253112079,
0.0779604124868694));
#93386=CARTESIAN_POINT('Ctrl Pts',(0.0125965491548823,-0.0323031222247695,
0.0780224333829103));
#93387=CARTESIAN_POINT('Ctrl Pts',(0.0125423682555023,-0.0321934096636185,
0.0780832990741119));
#93388=CARTESIAN_POINT('Ctrl Pts',(0.0128143290604209,-0.0325229783203385,
0.0778914930289423));
#93389=CARTESIAN_POINT('Ctrl Pts',(0.0127627526617768,-0.0324130253112079,
0.0779561521137558));
#93390=CARTESIAN_POINT('Ctrl Pts',(0.0127098465294984,-0.0323031222247695,
0.0780197344677113));
#93391=CARTESIAN_POINT('Ctrl Pts',(0.0126556813064848,-0.0321934096636185,
0.078082161037681));
#93392=CARTESIAN_POINT('Origin',(-0.000337898267003137,-0.0326393375182276,
0.0670568072818518));
#93393=CARTESIAN_POINT('Ctrl Pts',(0.012417777980686,-0.0326943950436593,
0.0783406562942332));
#93394=CARTESIAN_POINT('Ctrl Pts',(0.0123600228828247,-0.0325844576448127,
0.0783998356039916));
#93395=CARTESIAN_POINT('Ctrl Pts',(0.0123010397723938,-0.0324744968375319,
0.0784578246318473));
#93396=CARTESIAN_POINT('Ctrl Pts',(0.0122409052467996,-0.0323646534831895,
0.0785145501212491));
#93397=CARTESIAN_POINT('Ctrl Pts',(0.0124095272094101,-0.0326943950436593,
0.0782276383648774));
#93398=CARTESIAN_POINT('Ctrl Pts',(0.0123533297104334,-0.0325844576448127,
0.0782867039635441));
#93399=CARTESIAN_POINT('Ctrl Pts',(0.0122959066608527,-0.0324744968375319,
0.0783446114859591));
#93400=CARTESIAN_POINT('Ctrl Pts',(0.0122373326577929,-0.0323646534831895,
0.0784012877524309));
#93401=CARTESIAN_POINT('Ctrl Pts',(0.0124012764381341,-0.0326943950436593,
0.0781146204355217));
#93402=CARTESIAN_POINT('Ctrl Pts',(0.0123466365380422,-0.0325844576448127,
0.0781735723230966));
#93403=CARTESIAN_POINT('Ctrl Pts',(0.0122907735493116,-0.0324744968375319,
0.0782313983400709));
#93404=CARTESIAN_POINT('Ctrl Pts',(0.0122337600687862,-0.0323646534831895,
0.0782880253836128));
#93405=CARTESIAN_POINT('Ctrl Pts',(0.0123930256668581,-0.0326943950436593,
0.078001602506166));
#93406=CARTESIAN_POINT('Ctrl Pts',(0.0123399433656509,-0.0325844576448127,
0.0780604406826491));
#93407=CARTESIAN_POINT('Ctrl Pts',(0.0122856404377706,-0.0324744968375319,
0.0781181851941828));
#93408=CARTESIAN_POINT('Ctrl Pts',(0.0122301874797795,-0.0323646534831895,
0.0781747630147946));
#93409=CARTESIAN_POINT('Origin',(-3.49989696872885E-5,-0.032639557906955,
0.0666833513559041));
#93410=CARTESIAN_POINT('Ctrl Pts',(0.0124173068892609,-0.0327445246961876,
0.0779767180041819));
#93411=CARTESIAN_POINT('Ctrl Pts',(0.0122729798618093,-0.0324436878365475,
0.0781386509336553));
#93412=CARTESIAN_POINT('Ctrl Pts',(0.0121168654022419,-0.0321434074463187,
0.0782892525273214));
#93413=CARTESIAN_POINT('Ctrl Pts',(0.0125795511060735,-0.0327445246961876,
0.0777865159692011));
#93414=CARTESIAN_POINT('Ctrl Pts',(0.0124423976655688,-0.0324436878365475,
0.0779545680392822));
#93415=CARTESIAN_POINT('Ctrl Pts',(0.0122929754948708,-0.0321434074463187,
0.0781118117336063));
#93416=CARTESIAN_POINT('Ctrl Pts',(0.012164574948423,-0.0322357242816073,
0.0782426909129078));
#93417=CARTESIAN_POINT('Ctrl Pts',(0.0120342280508725,-0.0319819883628705,
0.0783713849214484));
#93418=CARTESIAN_POINT('Ctrl Pts',(0.0118959561495598,-0.0317295851069886,
0.078491523769631));
#93419=CARTESIAN_POINT('Ctrl Pts',(0.0123386165065131,-0.0322357242816073,
0.07806322075924));
#93420=CARTESIAN_POINT('Ctrl Pts',(0.0122139855005927,-0.0319819883628705,
0.0781974577656821));
#93421=CARTESIAN_POINT('Ctrl Pts',(0.0120810651901328,-0.0317295851069886,
0.0783234920967294));
#93422=CARTESIAN_POINT('Origin',(3.41437415837766E-5,-0.0326371942648999,
0.0667489386179022));
#93423=CARTESIAN_POINT('Origin',(-0.000245738147881846,-0.0326352985532511,
0.0671378647634999));
#93424=CARTESIAN_POINT('Ctrl Pts',(0.0121461712749856,-0.0321934096636183,
0.0786020092176618));
#93425=CARTESIAN_POINT('Ctrl Pts',(0.0120847745981891,-0.0320835708272304,
0.0786574810979602));
#93426=CARTESIAN_POINT('Ctrl Pts',(0.0120222655462808,-0.0319739230346346,
0.0787116502012785));
#93427=CARTESIAN_POINT('Ctrl Pts',(0.0119587294142675,-0.0318646057455575,
0.0787644533599413));
#93428=CARTESIAN_POINT('Ctrl Pts',(0.0121450332375747,-0.0321934096636183,
0.0784886960691015));
#93429=CARTESIAN_POINT('Ctrl Pts',(0.0120851992374078,-0.0320835708272304,
0.0785441522549771));
#93430=CARTESIAN_POINT('Ctrl Pts',(0.0120242522805083,-0.0319739230346346,
0.0785983380124876));
#93431=CARTESIAN_POINT('Ctrl Pts',(0.0119622756649264,-0.0318646057455575,
0.0786511899992634));
#93432=CARTESIAN_POINT('Ctrl Pts',(0.0121438952001639,-0.0321934096636183,
0.0783753829205412));
#93433=CARTESIAN_POINT('Ctrl Pts',(0.0120856238766265,-0.0320835708272304,
0.078430823411994));
#93434=CARTESIAN_POINT('Ctrl Pts',(0.0120262390147359,-0.0319739230346346,
0.0784850258236967));
#93435=CARTESIAN_POINT('Ctrl Pts',(0.0119658219155852,-0.0318646057455575,
0.0785379266385855));
#93436=CARTESIAN_POINT('Ctrl Pts',(0.012142757162753,-0.0321934096636183,
0.078262069771981));
#93437=CARTESIAN_POINT('Ctrl Pts',(0.0120860485158452,-0.0320835708272304,
0.0783174945690109));
#93438=CARTESIAN_POINT('Ctrl Pts',(0.0120282257489634,-0.0319739230346346,
0.0783717136349058));
#93439=CARTESIAN_POINT('Ctrl Pts',(0.0119693681662441,-0.0318646057455575,
0.0784246632779076));
#93440=CARTESIAN_POINT('Ctrl Pts',(0.0122311072172625,-0.0320218834582301,
0.0781750067014124));
#93441=CARTESIAN_POINT('Ctrl Pts',(0.012189216627892,-0.0319391099350596,
0.0782177540255193));
#93442=CARTESIAN_POINT('Ctrl Pts',(0.0121466839135055,-0.0318564869454876,
0.0782598213226819));
#93443=CARTESIAN_POINT('Ctrl Pts',(0.0121035429140419,-0.0317740741446466,
0.0783011808445998));
#93444=CARTESIAN_POINT('Ctrl Pts',(0.0122806703357578,-0.0320218834582301,
0.0781755770808563));
#93445=CARTESIAN_POINT('Ctrl Pts',(0.0122387738101161,-0.0319391099350596,
0.0782188402372087));
#93446=CARTESIAN_POINT('Ctrl Pts',(0.0121962271082623,-0.0318564869454876,
0.0782614229613914));
#93447=CARTESIAN_POINT('Ctrl Pts',(0.0121530641153712,-0.0317740741446466,
0.0783032971306349));
#93448=CARTESIAN_POINT('Ctrl Pts',(0.012330233454253,-0.0320218834582301,
0.0781761474603001));
#93449=CARTESIAN_POINT('Ctrl Pts',(0.0122883309923403,-0.0319391099350596,
0.078219926448898));
#93450=CARTESIAN_POINT('Ctrl Pts',(0.0122457703030191,-0.0318564869454876,
0.0782630246001008));
#93451=CARTESIAN_POINT('Ctrl Pts',(0.0122025853167005,-0.0317740741446466,
0.07830541341667));
#93452=CARTESIAN_POINT('Ctrl Pts',(0.0123797965727482,-0.0320218834582301,
0.078176717839744));
#93453=CARTESIAN_POINT('Ctrl Pts',(0.0123378881745644,-0.0319391099350596,
0.0782210126605874));
#93454=CARTESIAN_POINT('Ctrl Pts',(0.0122953134977759,-0.0318564869454876,
0.0782646262388103));
#93455=CARTESIAN_POINT('Ctrl Pts',(0.0122521065180299,-0.0317740741446466,
0.0783075297027051));
#93456=CARTESIAN_POINT('Origin',(0.0173832508623868,-0.0391228853390823,
0.0819051826730895));
#93457=CARTESIAN_POINT('Ctrl Pts',(0.0137092015079296,-0.035272297877959,
0.0755237742246161));
#93458=CARTESIAN_POINT('Ctrl Pts',(0.0137043489676322,-0.0352466642097214,
0.0755420374535391));
#93459=CARTESIAN_POINT('Ctrl Pts',(0.0136995765223734,-0.0352210183808299,
0.075560304544644));
#93460=CARTESIAN_POINT('Ctrl Pts',(0.013694884518966,-0.0351953608940152,
0.0755785762771645));
#93461=CARTESIAN_POINT('Origin',(0.0183951094992704,-0.0352456003065037,
0.0769562579037339));
#93462=CARTESIAN_POINT('Ctrl Pts',(0.0136612048588493,-0.035024121149334,
0.075698622084724));
#93463=CARTESIAN_POINT('Ctrl Pts',(0.0136398732255539,-0.0349144232867422,
0.0757748978080736));
#93464=CARTESIAN_POINT('Ctrl Pts',(0.0136169521506141,-0.0348045283677513,
0.0758507782460351));
#93465=CARTESIAN_POINT('Ctrl Pts',(0.0135924673762274,-0.0346945769586886,
0.0759261651129022));
#93466=CARTESIAN_POINT('Ctrl Pts',(0.0137611252006477,-0.035024121149334,
0.0756451705450078));
#93467=CARTESIAN_POINT('Ctrl Pts',(0.0137405298403627,-0.0349144232867422,
0.0757228226300346));
#93468=CARTESIAN_POINT('Ctrl Pts',(0.01371831702875,-0.0348045283677513,
0.0758000954727807));
#93469=CARTESIAN_POINT('Ctrl Pts',(0.0136945115344442,-0.0346945769586886,
0.0758768890378051));
#93470=CARTESIAN_POINT('Ctrl Pts',(0.013861045542446,-0.035024121149334,
0.0755917190052915));
#93471=CARTESIAN_POINT('Ctrl Pts',(0.0138411864551714,-0.0349144232867422,
0.0756707474519956));
#93472=CARTESIAN_POINT('Ctrl Pts',(0.013819681906886,-0.0348045283677513,
0.0757494126995263));
#93473=CARTESIAN_POINT('Ctrl Pts',(0.013796555692661,-0.0346945769586886,
0.075827612962708));
#93474=CARTESIAN_POINT('Ctrl Pts',(0.0139609658842444,-0.035024121149334,
0.0755382674655752));
#93475=CARTESIAN_POINT('Ctrl Pts',(0.0139418430699802,-0.0349144232867422,
0.0756186722739566));
#93476=CARTESIAN_POINT('Ctrl Pts',(0.013921046785022,-0.0348045283677513,
0.0756987299262718));
#93477=CARTESIAN_POINT('Ctrl Pts',(0.0138985998508777,-0.0346945769586886,
0.0757783368876108));
#93478=CARTESIAN_POINT('Origin',(-0.00231867693836035,-0.0345629067947109,
0.0705690730199885));
#93479=CARTESIAN_POINT('Ctrl Pts',(0.0137483798950316,-0.0351970973651619,
0.0760313352887893));
#93480=CARTESIAN_POINT('Ctrl Pts',(0.0137223165442662,-0.0350869349321778,
0.0761092564672701));
#93481=CARTESIAN_POINT('Ctrl Pts',(0.0136946116648051,-0.034976498512973,
0.0761867003521294));
#93482=CARTESIAN_POINT('Ctrl Pts',(0.0136652952430741,-0.0348659306849652,
0.0762635644996982));
#93483=CARTESIAN_POINT('Ctrl Pts',(0.0137080298409273,-0.0351970973651619,
0.0759596949106244));
#93484=CARTESIAN_POINT('Ctrl Pts',(0.0136829589705114,-0.0350869349321778,
0.0760370570937895));
#93485=CARTESIAN_POINT('Ctrl Pts',(0.0136562590147619,-0.034976498512973,
0.0761139621533845));
#93486=CARTESIAN_POINT('Ctrl Pts',(0.0136279586992884,-0.0348659306849652,
0.076190308420442));
#93487=CARTESIAN_POINT('Ctrl Pts',(0.0136676797868229,-0.0351970973651619,
0.0758880545324594));
#93488=CARTESIAN_POINT('Ctrl Pts',(0.0136436013967566,-0.0350869349321778,
0.0759648577203089));
#93489=CARTESIAN_POINT('Ctrl Pts',(0.0136179063647187,-0.034976498512973,
0.0760412239546396));
#93490=CARTESIAN_POINT('Ctrl Pts',(0.0135906221555027,-0.0348659306849652,
0.0761170523411859));
#93491=CARTESIAN_POINT('Ctrl Pts',(0.0136273297327185,-0.0351970973651619,
0.0758164141542945));
#93492=CARTESIAN_POINT('Ctrl Pts',(0.0136042438230018,-0.0350869349321778,
0.0758926583468284));
#93493=CARTESIAN_POINT('Ctrl Pts',(0.0135795537146755,-0.034976498512973,
0.0759684857558946));
#93494=CARTESIAN_POINT('Ctrl Pts',(0.013553285611717,-0.0348659306849652,
0.0760437962619298));
#93495=CARTESIAN_POINT('Origin',(-0.00212035218267538,-0.0345637187963098,
0.0701309033624755));
#93496=CARTESIAN_POINT('Ctrl Pts',(0.0136380039084654,-0.0352450361861252,
0.0757844674588033));
#93497=CARTESIAN_POINT('Ctrl Pts',(0.0135763589582961,-0.0349452761023765,
0.0759924397381133));
#93498=CARTESIAN_POINT('Ctrl Pts',(0.0134992238123034,-0.0346444289983475,
0.0761951778403425));
#93499=CARTESIAN_POINT('Ctrl Pts',(0.013703824675012,-0.0352450361861252,
0.0755432878023411));
#93500=CARTESIAN_POINT('Ctrl Pts',(0.0136512759646145,-0.0349452761023765,
0.075753742552533));
#93501=CARTESIAN_POINT('Ctrl Pts',(0.0135830242270757,-0.0346444289983475,
0.0759596412391868));
#93502=CARTESIAN_POINT('Ctrl Pts',(0.013553039606245,-0.0345231616327822,
0.0760432629782829));
#93503=CARTESIAN_POINT('Ctrl Pts',(0.0135269436415907,-0.0344132092796975,
0.0761180976479395));
#93504=CARTESIAN_POINT('Ctrl Pts',(0.013499301127255,-0.0343032738558974,
0.0761923886820265));
#93505=CARTESIAN_POINT('Ctrl Pts',(0.0134701499144472,-0.0341934961088741,
0.0762660418122672));
#93506=CARTESIAN_POINT('Ctrl Pts',(0.0136561189977491,-0.0345231616327822,
0.0759961909570195));
#93507=CARTESIAN_POINT('Ctrl Pts',(0.0136306718546357,-0.0344132092796975,
0.0760724464309637));
#93508=CARTESIAN_POINT('Ctrl Pts',(0.0136036487401489,-0.0343032738558974,
0.0761481716163932));
#93509=CARTESIAN_POINT('Ctrl Pts',(0.0135750867590384,-0.0341934961088741,
0.0762232703873912));
#93510=CARTESIAN_POINT('Ctrl Pts',(0.0137591983892531,-0.0345231616327822,
0.0759491189357559));
#93511=CARTESIAN_POINT('Ctrl Pts',(0.0137344000676807,-0.0344132092796975,
0.0760267952139879));
#93512=CARTESIAN_POINT('Ctrl Pts',(0.0137079963530427,-0.0343032738558974,
0.0761039545507599));
#93513=CARTESIAN_POINT('Ctrl Pts',(0.0136800236036295,-0.0341934961088741,
0.0761804989625153));
#93514=CARTESIAN_POINT('Ctrl Pts',(0.0138622777807571,-0.0345231616327822,
0.0759020469144925));
#93515=CARTESIAN_POINT('Ctrl Pts',(0.0138381282807258,-0.0344132092796975,
0.0759811439970121));
#93516=CARTESIAN_POINT('Ctrl Pts',(0.0138123439659366,-0.0343032738558974,
0.0760597374851266));
#93517=CARTESIAN_POINT('Ctrl Pts',(0.0137849604482207,-0.0341934961088741,
0.0761377275376394));
#93518=CARTESIAN_POINT('Origin',(-0.00233020492228257,-0.0345625596232513,
0.0705653846762973));
#93519=CARTESIAN_POINT('Ctrl Pts',(0.0136589219806728,-0.0346945769586885,
0.0764656484042893));
#93520=CARTESIAN_POINT('Ctrl Pts',(0.0136270111752922,-0.0345846629178476,
0.0765419254281193));
#93521=CARTESIAN_POINT('Ctrl Pts',(0.0135935175419434,-0.034474692505516,
0.0766175555779037));
#93522=CARTESIAN_POINT('Ctrl Pts',(0.0135584843967371,-0.0343648066260528,
0.0766924421248161));
#93523=CARTESIAN_POINT('Ctrl Pts',(0.013609645944372,-0.0346945769586885,
0.0763636043264145));
#93524=CARTESIAN_POINT('Ctrl Pts',(0.0135791413579593,-0.0345846629178476,
0.0764392023015593));
#93525=CARTESIAN_POINT('Ctrl Pts',(0.0135470682262121,-0.034474692505516,
0.076514182366706));
#93526=CARTESIAN_POINT('Ctrl Pts',(0.0135134680416907,-0.0343648066260528,
0.0765884486184748));
#93527=CARTESIAN_POINT('Ctrl Pts',(0.0135603699080712,-0.0346945769586885,
0.0762615602485397));
#93528=CARTESIAN_POINT('Ctrl Pts',(0.0135312715406265,-0.0345846629178476,
0.0763364791749993));
#93529=CARTESIAN_POINT('Ctrl Pts',(0.0135006189104809,-0.034474692505516,
0.0764108091555083));
#93530=CARTESIAN_POINT('Ctrl Pts',(0.0134684516866442,-0.0343648066260528,
0.0764844551121334));
#93531=CARTESIAN_POINT('Ctrl Pts',(0.0135110938717704,-0.0346945769586885,
0.0761595161706649));
#93532=CARTESIAN_POINT('Ctrl Pts',(0.0134834017232937,-0.0345846629178476,
0.0762337560484393));
#93533=CARTESIAN_POINT('Ctrl Pts',(0.0134541695947496,-0.034474692505516,
0.0763074359443106));
#93534=CARTESIAN_POINT('Ctrl Pts',(0.0134234353315977,-0.0343648066260528,
0.0763804616057921));
#93535=CARTESIAN_POINT('Origin',(-0.00217502575729261,-0.0345626446729475,
0.070110289510456));
#93536=CARTESIAN_POINT('Ctrl Pts',(0.0135119755852948,-0.0346945769586886,
0.0761613420813974));
#93537=CARTESIAN_POINT('Ctrl Pts',(0.0134698472201032,-0.0345275153362891,
0.0762741999493099));
#93538=CARTESIAN_POINT('Ctrl Pts',(0.0134241586822912,-0.0343603235965159,
0.0763857621097389));
#93539=CARTESIAN_POINT('Ctrl Pts',(0.0133750500022089,-0.034193496108874,
0.076495700619667));
#93540=CARTESIAN_POINT('Ctrl Pts',(0.0135395795365018,-0.0346945769586886,
0.0760821836945452));
#93541=CARTESIAN_POINT('Ctrl Pts',(0.0134991091754161,-0.0345275153362891,
0.0761956197382678));
#93542=CARTESIAN_POINT('Ctrl Pts',(0.0134550608874577,-0.0343603235965159,
0.0763078123667558));
#93543=CARTESIAN_POINT('Ctrl Pts',(0.0134075698795593,-0.034193496108874,
0.0764184317002467));
#93544=CARTESIAN_POINT('Ctrl Pts',(0.0135671834877089,-0.0346945769586886,
0.0760030253076931));
#93545=CARTESIAN_POINT('Ctrl Pts',(0.013528371130729,-0.0345275153362891,
0.0761170395272257));
#93546=CARTESIAN_POINT('Ctrl Pts',(0.0134859630926242,-0.0343603235965159,
0.0762298626237727));
#93547=CARTESIAN_POINT('Ctrl Pts',(0.0134400897569097,-0.034193496108874,
0.0763411627808263));
#93548=CARTESIAN_POINT('Ctrl Pts',(0.0135947874389159,-0.0346945769586886,
0.0759238669208409));
#93549=CARTESIAN_POINT('Ctrl Pts',(0.0135576330860419,-0.0345275153362891,
0.0760384593161836));
#93550=CARTESIAN_POINT('Ctrl Pts',(0.0135168652977908,-0.0343603235965159,
0.0761519128807895));
#93551=CARTESIAN_POINT('Ctrl Pts',(0.0134726096342601,-0.034193496108874,
0.076263893861406));
#93552=CARTESIAN_POINT('Ctrl Pts',(0.0134234470584664,-0.0340223579322365,
0.0763804323067669));
#93553=CARTESIAN_POINT('Ctrl Pts',(0.0133926835797447,-0.0339125849573554,
0.0764535285073657));
#93554=CARTESIAN_POINT('Ctrl Pts',(0.0133604287966631,-0.0338030433565221,
0.0765259366115855));
#93555=CARTESIAN_POINT('Ctrl Pts',(0.013326732166054,-0.0336938721132328,
0.0765975676781663));
#93556=CARTESIAN_POINT('Ctrl Pts',(0.0135292788965577,-0.0340223579322365,
0.0763399254940468));
#93557=CARTESIAN_POINT('Ctrl Pts',(0.0134990741124296,-0.0339125849573554,
0.0764144813917138));
#93558=CARTESIAN_POINT('Ctrl Pts',(0.0134673474190159,-0.0338030433565221,
0.0764883597309696));
#93559=CARTESIAN_POINT('Ctrl Pts',(0.0134341477644818,-0.0336938721132328,
0.0765614696305053));
#93560=CARTESIAN_POINT('Ctrl Pts',(0.013635110734649,-0.0340223579322365,
0.0762994186813266));
#93561=CARTESIAN_POINT('Ctrl Pts',(0.0136054646451145,-0.0339125849573554,
0.076375434276062));
#93562=CARTESIAN_POINT('Ctrl Pts',(0.0135742660413688,-0.0338030433565221,
0.0764507828503537));
#93563=CARTESIAN_POINT('Ctrl Pts',(0.0135415633629095,-0.0336938721132328,
0.0765253715828443));
#93564=CARTESIAN_POINT('Ctrl Pts',(0.0137409425727403,-0.0340223579322365,
0.0762589118686065));
#93565=CARTESIAN_POINT('Ctrl Pts',(0.0137118551777994,-0.0339125849573554,
0.0763363871604101));
#93566=CARTESIAN_POINT('Ctrl Pts',(0.0136811846637216,-0.0338030433565221,
0.0764132059697378));
#93567=CARTESIAN_POINT('Ctrl Pts',(0.0136489789613373,-0.0336938721132328,
0.0764892735351833));
#93568=CARTESIAN_POINT('Origin',(-0.00221735192247542,-0.0345589643412543,
0.0706068223244746));
#93569=CARTESIAN_POINT('Ctrl Pts',(0.013502598880332,-0.034193496108874,
0.0768086333040515));
#93570=CARTESIAN_POINT('Ctrl Pts',(0.0134659379014492,-0.0340836138581107,
0.0768828040009596));
#93571=CARTESIAN_POINT('Ctrl Pts',(0.0134277597062521,-0.0339738896643499,
0.0769561804873401));
#93572=CARTESIAN_POINT('Ctrl Pts',(0.0133881194535538,-0.0338644633294062,
0.0770286721259033));
#93573=CARTESIAN_POINT('Ctrl Pts',(0.0134598274169694,-0.034193496108874,
0.076703696365036));
#93574=CARTESIAN_POINT('Ctrl Pts',(0.0134246134563345,-0.0340836138581107,
0.0767772772687925));
#93575=CARTESIAN_POINT('Ctrl Pts',(0.0133878937896103,-0.0339738896643499,
0.0768500941880218));
#93576=CARTESIAN_POINT('Ctrl Pts',(0.013349721660865,-0.0338644633294062,
0.0769220570764743));
#93577=CARTESIAN_POINT('Ctrl Pts',(0.0134170559536069,-0.034193496108874,
0.0765987594260205));
#93578=CARTESIAN_POINT('Ctrl Pts',(0.0133832890112198,-0.0340836138581107,
0.0766717505366255));
#93579=CARTESIAN_POINT('Ctrl Pts',(0.0133480278729686,-0.0339738896643499,
0.0767440078887034));
#93580=CARTESIAN_POINT('Ctrl Pts',(0.0133113238681763,-0.0338644633294062,
0.0768154420270453));
#93581=CARTESIAN_POINT('Ctrl Pts',(0.0133742844902443,-0.034193496108874,
0.076493822487005));
#93582=CARTESIAN_POINT('Ctrl Pts',(0.0133419645661051,-0.0340836138581107,
0.0765662238044585));
#93583=CARTESIAN_POINT('Ctrl Pts',(0.0133081619563269,-0.0339738896643499,
0.0766379215893851));
#93584=CARTESIAN_POINT('Ctrl Pts',(0.0132729260754875,-0.0338644633294062,
0.0767088269776163));
#93585=CARTESIAN_POINT('Origin',(-0.0021053722911509,-0.0345610621863108,
0.0701388366693302));
#93586=CARTESIAN_POINT('Ctrl Pts',(0.0133897010974836,-0.03424362768739,
0.0764626225573025));
#93587=CARTESIAN_POINT('Ctrl Pts',(0.0133024790998638,-0.033943005420186,
0.0766612299628616));
#93588=CARTESIAN_POINT('Ctrl Pts',(0.0132005449672405,-0.0336441434784163,
0.076852703227361));
#93589=CARTESIAN_POINT('Ctrl Pts',(0.0134852275204704,-0.03424362768739,
0.0762315929000909));
#93590=CARTESIAN_POINT('Ctrl Pts',(0.0134067189500149,-0.033943005420186,
0.0764338031440864));
#93591=CARTESIAN_POINT('Ctrl Pts',(0.0133132021100695,-0.0336441434784163,
0.0766295253427721));
#93592=CARTESIAN_POINT('Ctrl Pts',(0.0132729383030164,-0.0335235895815127,
0.0767088020875533));
#93593=CARTESIAN_POINT('Ctrl Pts',(0.013237711354464,-0.0334144449262719,
0.0767796903591607));
#93594=CARTESIAN_POINT('Ctrl Pts',(0.0132009794360736,-0.0333049234473133,
0.0768499323105579));
#93595=CARTESIAN_POINT('Ctrl Pts',(0.0131627813805983,-0.0331951640388588,
0.0769194338692133));
#93596=CARTESIAN_POINT('Ctrl Pts',(0.0133811047344406,-0.0335235895815127,
0.0766750205008595));
#93597=CARTESIAN_POINT('Ctrl Pts',(0.0133463428559389,-0.0334144449262719,
0.0767473978963555));
#93598=CARTESIAN_POINT('Ctrl Pts',(0.0133100457777294,-0.0333049234473133,
0.0768191402904615));
#93599=CARTESIAN_POINT('Ctrl Pts',(0.0132722516027427,-0.0331951640388588,
0.0768901517424077));
#93600=CARTESIAN_POINT('Ctrl Pts',(0.0134892711658648,-0.0335235895815127,
0.0766412389141656));
#93601=CARTESIAN_POINT('Ctrl Pts',(0.0134549743574137,-0.0334144449262719,
0.0767151054335503));
#93602=CARTESIAN_POINT('Ctrl Pts',(0.0134191121193851,-0.0333049234473133,
0.0767883482703651));
#93603=CARTESIAN_POINT('Ctrl Pts',(0.013381721824887,-0.0331951640388588,
0.0768608696156021));
#93604=CARTESIAN_POINT('Ctrl Pts',(0.0135974375972889,-0.0335235895815127,
0.0766074573274718));
#93605=CARTESIAN_POINT('Ctrl Pts',(0.0135636058588885,-0.0334144449262719,
0.0766828129707451));
#93606=CARTESIAN_POINT('Ctrl Pts',(0.0135281784610409,-0.0333049234473133,
0.0767575562502687));
#93607=CARTESIAN_POINT('Ctrl Pts',(0.0134911920470314,-0.0331951640388588,
0.0768315874887965));
#93608=CARTESIAN_POINT('Origin',(-0.00106178345708809,-0.0326434571771455,
0.0682330884781778));
#93609=CARTESIAN_POINT('Ctrl Pts',(0.0133256939357804,-0.0336938721132431,
0.077143047737031));
#93610=CARTESIAN_POINT('Ctrl Pts',(0.0133081746341762,-0.0336474569764979,
0.0771734962526395));
#93611=CARTESIAN_POINT('Ctrl Pts',(0.0132903000946864,-0.033601104548885,
0.0772037375963512));
#93612=CARTESIAN_POINT('Ctrl Pts',(0.0132450458722633,-0.0334837508643191,
0.0772803017224079));
#93613=CARTESIAN_POINT('Ctrl Pts',(0.0131975427684567,-0.0333660264760466,
0.0773554912507659));
#93614=CARTESIAN_POINT('Ctrl Pts',(0.01321740006416,-0.0336938721132431,
0.0768208017492327));
#93615=CARTESIAN_POINT('Ctrl Pts',(0.0132017669752551,-0.0336474569764979,
0.0768506163848749));
#93616=CARTESIAN_POINT('Ctrl Pts',(0.0131857859395853,-0.033601104548885,
0.0768802459725553));
#93617=CARTESIAN_POINT('Ctrl Pts',(0.0131453256332841,-0.0334837508643191,
0.076955261273059));
#93618=CARTESIAN_POINT('Ctrl Pts',(0.0131026602353754,-0.0333660264760466,
0.0770290447096619));
#93619=CARTESIAN_POINT('Ctrl Pts',(0.0132174000641665,-0.0336938721132426,
0.0768208017492494));
#93620=CARTESIAN_POINT('Ctrl Pts',(0.0132017669752633,-0.0336474569765026,
0.0768506163848883));
#93621=CARTESIAN_POINT('Ctrl Pts',(0.0131857859395953,-0.0336011045488949,
0.0768802459725653));
#93622=CARTESIAN_POINT('Ctrl Pts',(0.0131456626125359,-0.0334847282606778,
0.0769546364977918));
#93623=CARTESIAN_POINT('Ctrl Pts',(0.0131033706183091,-0.0333679869945434,
0.0770278158585576));
#93624=CARTESIAN_POINT('Ctrl Pts',(0.0132174000641599,-0.0336938721132429,
0.0768208017492329));
#93625=CARTESIAN_POINT('Ctrl Pts',(0.0131614892199085,-0.0335278710435085,
0.0769274320805731));
#93626=CARTESIAN_POINT('Ctrl Pts',(0.0131022541454949,-0.0333620469224321,
0.0770322715500714));
#93627=CARTESIAN_POINT('Ctrl Pts',(0.0130396479434203,-0.0331951640388602,
0.07713536244448));
#93628=CARTESIAN_POINT('Ctrl Pts',(0.0132547075305147,-0.0336938721132429,
0.0767457272343995));
#93629=CARTESIAN_POINT('Ctrl Pts',(0.0132003683040395,-0.0335278710435085,
0.0768531385641577));
#93630=CARTESIAN_POINT('Ctrl Pts',(0.0131426798026034,-0.0333620469224321,
0.0769588080428453));
#93631=CARTESIAN_POINT('Ctrl Pts',(0.0130815957598022,-0.0331951640388602,
0.0770627786272473));
#93632=CARTESIAN_POINT('Ctrl Pts',(0.0132920149968694,-0.0336938721132429,
0.0766706527195662));
#93633=CARTESIAN_POINT('Ctrl Pts',(0.0132392473881706,-0.0335278710435085,
0.0767788450477423));
#93634=CARTESIAN_POINT('Ctrl Pts',(0.013183105459712,-0.0333620469224321,
0.0768853445356193));
#93635=CARTESIAN_POINT('Ctrl Pts',(0.013123543576184,-0.0331951640388602,
0.0769901948100146));
#93636=CARTESIAN_POINT('Ctrl Pts',(0.0133293224632242,-0.0336938721132429,
0.0765955782047328));
#93637=CARTESIAN_POINT('Ctrl Pts',(0.0132781264723017,-0.0335278710435085,
0.0767045515313269));
#93638=CARTESIAN_POINT('Ctrl Pts',(0.0132235311168205,-0.0333620469224321,
0.0768118810283932));
#93639=CARTESIAN_POINT('Ctrl Pts',(0.0131654913925659,-0.0331951640388602,
0.0769176109927819));
#93640=CARTESIAN_POINT('Ctrl Pts',(0.013102110037377,-0.0330240426238155,
0.0770270701512004));
#93641=CARTESIAN_POINT('Ctrl Pts',(0.0130624755930508,-0.0329142774063509,
0.0770956514674047));
#93642=CARTESIAN_POINT('Ctrl Pts',(0.0130214036221302,-0.0328043479726686,
0.0771634476192186));
#93643=CARTESIAN_POINT('Ctrl Pts',(0.0129789443489825,-0.0326943950436594,
0.0772303703056803));
#93644=CARTESIAN_POINT('Ctrl Pts',(0.0132121840296781,-0.0330240426238155,
0.0770001470718097));
#93645=CARTESIAN_POINT('Ctrl Pts',(0.0131729204770003,-0.0329142774063509,
0.0770702447644978));
#93646=CARTESIAN_POINT('Ctrl Pts',(0.0131321882348935,-0.0328043479726686,
0.0771395657161309));
#93647=CARTESIAN_POINT('Ctrl Pts',(0.0130900370387112,-0.0326943950436594,
0.0772080196843509));
#93648=CARTESIAN_POINT('Ctrl Pts',(0.0133222580219791,-0.0330240426238155,
0.0769732239924189));
#93649=CARTESIAN_POINT('Ctrl Pts',(0.0132833653609499,-0.0329142774063509,
0.0770448380615909));
#93650=CARTESIAN_POINT('Ctrl Pts',(0.0132429728476568,-0.0328043479726686,
0.0771156838130433));
#93651=CARTESIAN_POINT('Ctrl Pts',(0.0132011297284398,-0.0326943950436594,
0.0771856690630216));
#93652=CARTESIAN_POINT('Ctrl Pts',(0.0134323320142801,-0.0330240426238155,
0.0769463009130282));
#93653=CARTESIAN_POINT('Ctrl Pts',(0.0133938102448994,-0.0329142774063509,
0.0770194313586839));
#93654=CARTESIAN_POINT('Ctrl Pts',(0.0133537574604201,-0.0328043479726686,
0.0770918019099556));
#93655=CARTESIAN_POINT('Ctrl Pts',(0.0133122224181685,-0.0326943950436594,
0.0771633184416921));
#93656=CARTESIAN_POINT('Origin',(-0.00116722503613692,-0.0326396682859212,
0.0681684551100529));
#93657=CARTESIAN_POINT('Ctrl Pts',(0.0131269701953199,-0.0331951640388587,
0.0774618136745128));
#93658=CARTESIAN_POINT('Ctrl Pts',(0.013081356661698,-0.0330855618255041,
0.0775307224678763));
#93659=CARTESIAN_POINT('Ctrl Pts',(0.013034286018948,-0.0329757224427708,
0.0775987381828553));
#93660=CARTESIAN_POINT('Ctrl Pts',(0.0129858142715051,-0.0328657862078596,
0.0776657707645413));
#93661=CARTESIAN_POINT('Ctrl Pts',(0.0130976880918259,-0.0331951640388587,
0.0773523435395182));
#93662=CARTESIAN_POINT('Ctrl Pts',(0.0130535822878572,-0.0330855618255041,
0.0774208490311433));
#93663=CARTESIAN_POINT('Ctrl Pts',(0.0130080287972194,-0.0329757224427708,
0.077488492315844));
#93664=CARTESIAN_POINT('Ctrl Pts',(0.0129610817049368,-0.0328657862078596,
0.0775551839109298));
#93665=CARTESIAN_POINT('Ctrl Pts',(0.0130684059883319,-0.0331951640388587,
0.0772428734045236));
#93666=CARTESIAN_POINT('Ctrl Pts',(0.0130258079140165,-0.0330855618255041,
0.0773109755944103));
#93667=CARTESIAN_POINT('Ctrl Pts',(0.0129817715754907,-0.0329757224427708,
0.0773782464488327));
#93668=CARTESIAN_POINT('Ctrl Pts',(0.0129363491383684,-0.0328657862078596,
0.0774445970573182));
#93669=CARTESIAN_POINT('Ctrl Pts',(0.0130391238848379,-0.0331951640388587,
0.077133403269529));
#93670=CARTESIAN_POINT('Ctrl Pts',(0.0129980335401758,-0.0330855618255041,
0.0772011021576773));
#93671=CARTESIAN_POINT('Ctrl Pts',(0.012955514353762,-0.0329757224427708,
0.0772680005818214));
#93672=CARTESIAN_POINT('Ctrl Pts',(0.0129116165718001,-0.0328657862078596,
0.0773340102037066));
#93673=CARTESIAN_POINT('Origin',(-0.000875325020341547,-0.0326401908829857,
0.0677862676517416));
#93674=CARTESIAN_POINT('Ctrl Pts',(0.0130582920642887,-0.0332451089994433,
0.0771044436584957));
#93675=CARTESIAN_POINT('Ctrl Pts',(0.0129468633986402,-0.0329451141710258,
0.0772905517431748));
#93676=CARTESIAN_POINT('Ctrl Pts',(0.0128217328683168,-0.0326442513127503,
0.0774677378518065));
#93677=CARTESIAN_POINT('Ctrl Pts',(0.0131820236641183,-0.0332451089994433,
0.0768872099336655));
#93678=CARTESIAN_POINT('Ctrl Pts',(0.013078788102448,-0.0329451141710258,
0.0770779846319819));
#93679=CARTESIAN_POINT('Ctrl Pts',(0.0129614758919426,-0.0326442513127503,
0.0772604412349795));
#93680=CARTESIAN_POINT('Ctrl Pts',(0.0129116341381032,-0.0325229783203385,
0.0773339839509843));
#93681=CARTESIAN_POINT('Ctrl Pts',(0.0128677429897669,-0.032413025311208,
0.0773999843841413));
#93682=CARTESIAN_POINT('Ctrl Pts',(0.0128224931946646,-0.0323031222247695,
0.0774650668622706));
#93683=CARTESIAN_POINT('Ctrl Pts',(0.0127759456562771,-0.0321934096636184,
0.0775291500646277));
#93684=CARTESIAN_POINT('Ctrl Pts',(0.0130231814644182,-0.0325229783203385,
0.077314025578261));
#93685=CARTESIAN_POINT('Ctrl Pts',(0.0129795654418084,-0.032413025311208,
0.0773815636888438));
#93686=CARTESIAN_POINT('Ctrl Pts',(0.0129345589218722,-0.0323031222247695,
0.0774481893025091));
#93687=CARTESIAN_POINT('Ctrl Pts',(0.0128882225662215,-0.0321934096636184,
0.0775138191108694));
#93688=CARTESIAN_POINT('Ctrl Pts',(0.0131347287907332,-0.0325229783203385,
0.0772940672055376));
#93689=CARTESIAN_POINT('Ctrl Pts',(0.01309138789385,-0.032413025311208,
0.0773631429935464));
#93690=CARTESIAN_POINT('Ctrl Pts',(0.0130466246490798,-0.0323031222247695,
0.0774313117427476));
#93691=CARTESIAN_POINT('Ctrl Pts',(0.0130004994761659,-0.0321934096636184,
0.0774984881571111));
#93692=CARTESIAN_POINT('Ctrl Pts',(0.0132462761170482,-0.0325229783203385,
0.0772741088328143));
#93693=CARTESIAN_POINT('Ctrl Pts',(0.0132032103458915,-0.032413025311208,
0.0773447222982489));
#93694=CARTESIAN_POINT('Ctrl Pts',(0.0131586903762874,-0.0323031222247695,
0.0774144341829861));
#93695=CARTESIAN_POINT('Ctrl Pts',(0.0131127763861102,-0.0321934096636184,
0.0774831572033528));
#93696=CARTESIAN_POINT('Origin',(-0.00116018816837294,-0.0326393375179027,
0.0681732689983203));
#93697=CARTESIAN_POINT('Ctrl Pts',(0.0129091470454595,-0.0326943950436593,
0.0777694313406965));
#93698=CARTESIAN_POINT('Ctrl Pts',(0.0128592644980476,-0.0325844576448127,
0.0778353826370912));
#93699=CARTESIAN_POINT('Ctrl Pts',(0.0128080144394322,-0.0324744968375319,
0.0779003069480977));
#93700=CARTESIAN_POINT('Ctrl Pts',(0.0127554636815458,-0.0323646534831895,
0.0779641219946141));
#93701=CARTESIAN_POINT('Ctrl Pts',(0.0128867964314425,-0.0326943950436593,
0.0776583386873139));
#93702=CARTESIAN_POINT('Ctrl Pts',(0.012838444949004,-0.0325844576448127,
0.077723981950358));
#93703=CARTESIAN_POINT('Ctrl Pts',(0.0127887324343526,-0.0324744968375319,
0.0777886298711476));
#93704=CARTESIAN_POINT('Ctrl Pts',(0.0127377237245454,-0.0323646534831895,
0.0778522004975362));
#93705=CARTESIAN_POINT('Ctrl Pts',(0.0128644458174256,-0.0326943950436593,
0.0775472460339312));
#93706=CARTESIAN_POINT('Ctrl Pts',(0.0128176253999605,-0.0325844576448127,
0.0776125812636247));
#93707=CARTESIAN_POINT('Ctrl Pts',(0.0127694504292731,-0.0324744968375319,
0.0776769527941975));
#93708=CARTESIAN_POINT('Ctrl Pts',(0.0127199837675449,-0.0323646534831895,
0.0777402790004584));
#93709=CARTESIAN_POINT('Ctrl Pts',(0.0128420952034086,-0.0326943950436593,
0.0774361533805486));
#93710=CARTESIAN_POINT('Ctrl Pts',(0.012796805850917,-0.0325844576448127,
0.0775011805768914));
#93711=CARTESIAN_POINT('Ctrl Pts',(0.0127501684241935,-0.0324744968375319,
0.0775652757172474));
#93712=CARTESIAN_POINT('Ctrl Pts',(0.0127022438105445,-0.0323646534831895,
0.0776283575033805));
#93713=CARTESIAN_POINT('Origin',(-0.000906483761463371,-0.0326395579068527,
0.0677647945357601));
#93714=CARTESIAN_POINT('Ctrl Pts',(0.0128630661060209,-0.0327445246961876,
0.0774084218561767));
#93715=CARTESIAN_POINT('Ctrl Pts',(0.0127401727179607,-0.0324436878365475,
0.0775871668691753));
#93716=CARTESIAN_POINT('Ctrl Pts',(0.0126041646522502,-0.0321434074463188,
0.0777561472543167));
#93717=CARTESIAN_POINT('Ctrl Pts',(0.0130001923426494,-0.0327445246961876,
0.077199385028732));
#93718=CARTESIAN_POINT('Ctrl Pts',(0.0128851829073392,-0.0324436878365475,
0.0773833018422387));
#93719=CARTESIAN_POINT('Ctrl Pts',(0.0127566468357546,-0.0321434074463188,
0.0775580331868864));
#93720=CARTESIAN_POINT('Ctrl Pts',(0.0126456622767151,-0.0322357242816073,
0.0777039732004452));
#93721=CARTESIAN_POINT('Ctrl Pts',(0.0125324728396152,-0.0319819883628706,
0.0778479892164446));
#93722=CARTESIAN_POINT('Ctrl Pts',(0.0124103486438636,-0.0317295851069886,
0.0779845107984281));
#93723=CARTESIAN_POINT('Ctrl Pts',(0.0127958378904485,-0.0322357242816073,
0.0775041050312941));
#93724=CARTESIAN_POINT('Ctrl Pts',(0.0126890139953167,-0.0319819883628706,
0.0776529039458202));
#93725=CARTESIAN_POINT('Ctrl Pts',(0.0125729380914563,-0.0317295851069886,
0.0777946037908388));
#93726=CARTESIAN_POINT('Origin',(-0.000829665997267067,-0.0326371942646419,
0.0678211987429648));
#93727=CARTESIAN_POINT('Origin',(-0.00105859556252852,-0.0326352985529724,
0.0682421365922654));
#93728=CARTESIAN_POINT('Ctrl Pts',(0.0126724382467534,-0.0321934096636183,
0.0780627647649452));
#93729=CARTESIAN_POINT('Ctrl Pts',(0.0126184781712214,-0.0320835708272304,
0.0781254942769318));
#93730=CARTESIAN_POINT('Ctrl Pts',(0.0125632512107361,-0.0319739230346346,
0.0781870707022936));
#93731=CARTESIAN_POINT('Ctrl Pts',(0.0125068340707187,-0.0318646057455575,
0.0782474206811522));
#93732=CARTESIAN_POINT('Ctrl Pts',(0.012657107279793,-0.0321934096636183,
0.0779504877583147));
#93733=CARTESIAN_POINT('Ctrl Pts',(0.0126046955916858,-0.0320835708272304,
0.0780130058443187));
#93734=CARTESIAN_POINT('Ctrl Pts',(0.0125510204959474,-0.0319739230346346,
0.0780744030101308));
#93735=CARTESIAN_POINT('Ctrl Pts',(0.0124961566948937,-0.0318646057455575,
0.078134605972841));
#93736=CARTESIAN_POINT('Ctrl Pts',(0.0126417763128326,-0.0321934096636183,
0.0778382107516842));
#93737=CARTESIAN_POINT('Ctrl Pts',(0.0125909130121503,-0.0320835708272303,
0.0779005174117056));
#93738=CARTESIAN_POINT('Ctrl Pts',(0.0125387897811587,-0.0319739230346346,
0.077961735317968));
#93739=CARTESIAN_POINT('Ctrl Pts',(0.0124854793190688,-0.0318646057455575,
0.0780217912645298));
#93740=CARTESIAN_POINT('Ctrl Pts',(0.0126264453458722,-0.0321934096636183,
0.0777259337450536));
#93741=CARTESIAN_POINT('Ctrl Pts',(0.0125771304326147,-0.0320835708272303,
0.0777880289790925));
#93742=CARTESIAN_POINT('Ctrl Pts',(0.01252655906637,-0.0319739230346346,
0.0778490676258052));
#93743=CARTESIAN_POINT('Ctrl Pts',(0.0124748019432438,-0.0318646057455575,
0.0779089765562186));
#93744=CARTESIAN_POINT('Ctrl Pts',(0.0127031868376533,-0.0320218834582296,
0.077628483994784));
#93745=CARTESIAN_POINT('Ctrl Pts',(0.0126669842284488,-0.0319391099350593,
0.077676144526494));
#93746=CARTESIAN_POINT('Ctrl Pts',(0.0126300593276,-0.0318564869454876,
0.0777232108730797));
#93747=CARTESIAN_POINT('Ctrl Pts',(0.0125924422304235,-0.031774074144647,
0.0777696512637756));
#93748=CARTESIAN_POINT('Ctrl Pts',(0.0127524306236555,-0.0320218834582296,
0.0776228379707091));
#93749=CARTESIAN_POINT('Ctrl Pts',(0.0127162867759124,-0.0319391099350593,
0.0776710110111852));
#93750=CARTESIAN_POINT('Ctrl Pts',(0.0126794125980267,-0.0318564869454876,
0.0777185904735896));
#93751=CARTESIAN_POINT('Ctrl Pts',(0.012641838183261,-0.031774074144647,
0.0777655442099706));
#93752=CARTESIAN_POINT('Ctrl Pts',(0.0128016744096576,-0.0320218834582296,
0.0776171919466342));
#93753=CARTESIAN_POINT('Ctrl Pts',(0.012765589323376,-0.0319391099350593,
0.0776658774958765));
#93754=CARTESIAN_POINT('Ctrl Pts',(0.0127287658684534,-0.0318564869454876,
0.0777139700740995));
#93755=CARTESIAN_POINT('Ctrl Pts',(0.0126912341360985,-0.031774074144647,
0.0777614371561656));
#93756=CARTESIAN_POINT('Ctrl Pts',(0.0128509181956598,-0.0320218834582296,
0.0776115459225593));
#93757=CARTESIAN_POINT('Ctrl Pts',(0.0128148918708396,-0.0319391099350593,
0.0776607439805678));
#93758=CARTESIAN_POINT('Ctrl Pts',(0.0127781191388802,-0.0318564869454876,
0.0777093496746093));
#93759=CARTESIAN_POINT('Ctrl Pts',(0.012740630088936,-0.031774074144647,
0.0777573301023607));
#93760=CARTESIAN_POINT('Origin',(0.0182822193075388,-0.0391228853390615,
0.0806835115919135));
#93761=CARTESIAN_POINT('Ctrl Pts',(0.0138373383741067,-0.0352722978779582,
0.0748129029409901));
#93762=CARTESIAN_POINT('Ctrl Pts',(0.0138348130870752,-0.0352466642097209,
0.0748316303434644));
#93763=CARTESIAN_POINT('Ctrl Pts',(0.0138323677475688,-0.0352210183808297,
0.0748503515390959));
#93764=CARTESIAN_POINT('Ctrl Pts',(0.0138300027973293,-0.0351953608940152,
0.0748690672575067));
#93765=CARTESIAN_POINT('Origin',(0.0186658343928198,-0.0352456003065022,
0.0756467910576931));
#93766=CARTESIAN_POINT('Ctrl Pts',(0.0138116344406295,-0.035024121149334,
0.0749923876487254));
#93767=CARTESIAN_POINT('Ctrl Pts',(0.0138000308966839,-0.0349144232867422,
0.0750707354777921));
#93768=CARTESIAN_POINT('Ctrl Pts',(0.0137868009019202,-0.0348045283677513,
0.0751488903482748));
#93769=CARTESIAN_POINT('Ctrl Pts',(0.0137719576770855,-0.0346945769586886,
0.0752267515231267));
#93770=CARTESIAN_POINT('Ctrl Pts',(0.013904067626376,-0.035024121149334,
0.0749268342508288));
#93771=CARTESIAN_POINT('Ctrl Pts',(0.0138933670535677,-0.0349144232867422,
0.0750064553090727));
#93772=CARTESIAN_POINT('Ctrl Pts',(0.0138810142518574,-0.0348045283677513,
0.0750859028358794));
#93773=CARTESIAN_POINT('Ctrl Pts',(0.0138670212568059,-0.0346945769586886,
0.0751650744802844));
#93774=CARTESIAN_POINT('Ctrl Pts',(0.0139965008121224,-0.035024121149334,
0.0748612808529322));
#93775=CARTESIAN_POINT('Ctrl Pts',(0.0139867032104516,-0.0349144232867422,
0.0749421751403532));
#93776=CARTESIAN_POINT('Ctrl Pts',(0.0139752276017946,-0.0348045283677513,
0.0750229153234839));
#93777=CARTESIAN_POINT('Ctrl Pts',(0.0139620848365264,-0.0346945769586886,
0.0751033974374421));
#93778=CARTESIAN_POINT('Ctrl Pts',(0.0140889339978689,-0.035024121149334,
0.0747957274550357));
#93779=CARTESIAN_POINT('Ctrl Pts',(0.0140800393673354,-0.0349144232867422,
0.0748778949716338));
#93780=CARTESIAN_POINT('Ctrl Pts',(0.0140694409517319,-0.0348045283677513,
0.0749599278110884));
#93781=CARTESIAN_POINT('Ctrl Pts',(0.0140571484162468,-0.0346945769586886,
0.0750417203945998));
#93782=CARTESIAN_POINT('Origin',(-0.00268514418653433,-0.0345629067947195,
0.0719060968681436));
#93783=CARTESIAN_POINT('Ctrl Pts',(0.0139398220973284,-0.0351970973651623,
0.0753115513806286));
#93784=CARTESIAN_POINT('Ctrl Pts',(0.0139237303771306,-0.0350869349321781,
0.0753921247313721));
#93785=CARTESIAN_POINT('Ctrl Pts',(0.0139059502514284,-0.0349764985129732,
0.0754724302901964));
#93786=CARTESIAN_POINT('Ctrl Pts',(0.013886498630599,-0.0348659306849652,
0.0755523626629356));
#93787=CARTESIAN_POINT('Ctrl Pts',(0.0138908112952035,-0.0351970973651623,
0.0752455331109989));
#93788=CARTESIAN_POINT('Ctrl Pts',(0.0138756341686609,-0.0350869349321781,
0.0753254274835004));
#93789=CARTESIAN_POINT('Ctrl Pts',(0.0138587835098339,-0.0349764985129732,
0.0754050725155202));
#93790=CARTESIAN_POINT('Ctrl Pts',(0.0138402750753216,-0.0348659306849652,
0.0754843637395078));
#93791=CARTESIAN_POINT('Ctrl Pts',(0.0138418004930787,-0.0351970973651623,
0.0751795148413693));
#93792=CARTESIAN_POINT('Ctrl Pts',(0.0138275379601911,-0.0350869349321781,
0.0752587302356287));
#93793=CARTESIAN_POINT('Ctrl Pts',(0.0138116167682393,-0.0349764985129732,
0.075337714740844));
#93794=CARTESIAN_POINT('Ctrl Pts',(0.0137940515200442,-0.0348659306849652,
0.07541636481608));
#93795=CARTESIAN_POINT('Ctrl Pts',(0.0137927896909538,-0.0351970973651623,
0.0751134965717397));
#93796=CARTESIAN_POINT('Ctrl Pts',(0.0137794417517213,-0.0350869349321781,
0.075192032987757));
#93797=CARTESIAN_POINT('Ctrl Pts',(0.0137644500266448,-0.0349764985129732,
0.0752703569661678));
#93798=CARTESIAN_POINT('Ctrl Pts',(0.0137478279647668,-0.0348659306849652,
0.0753483658926522));
#93799=CARTESIAN_POINT('Origin',(-0.00254330050109684,-0.0345637187962885,
0.0714465256262351));
#93800=CARTESIAN_POINT('Ctrl Pts',(0.013799375714989,-0.0352450361861252,
0.0750804639565227));
#93801=CARTESIAN_POINT('Ctrl Pts',(0.013764282691922,-0.0349452761023764,
0.0752945224732297));
#93802=CARTESIAN_POINT('Ctrl Pts',(0.0137131656015136,-0.0346444289983475,
0.0755053295222366));
#93803=CARTESIAN_POINT('Ctrl Pts',(0.0138344496389174,-0.0352450361861252,
0.0748329365441815));
#93804=CARTESIAN_POINT('Ctrl Pts',(0.0138086922651574,-0.0349452761023764,
0.0750483178956022));
#93805=CARTESIAN_POINT('Ctrl Pts',(0.0137667846611399,-0.0346444289983475,
0.075261147220575));
#93806=CARTESIAN_POINT('Ctrl Pts',(0.0137475170609577,-0.0345231616327823,
0.0753478676467675));
#93807=CARTESIAN_POINT('Ctrl Pts',(0.0137310061419098,-0.0344132092796976,
0.0754253829143349));
#93808=CARTESIAN_POINT('Ctrl Pts',(0.0137128927325831,-0.0343032738558974,
0.075502552667134));
#93809=CARTESIAN_POINT('Ctrl Pts',(0.0136932025707705,-0.0341934961088741,
0.0755792786362073));
#93810=CARTESIAN_POINT('Ctrl Pts',(0.0138438839520356,-0.0345231616327823,
0.0752882475290006));
#93811=CARTESIAN_POINT('Ctrl Pts',(0.0138281948123727,-0.0344132092796976,
0.0753670910784878));
#93812=CARTESIAN_POINT('Ctrl Pts',(0.0138108756655672,-0.0343032738558974,
0.0754456060425318));
#93813=CARTESIAN_POINT('Ctrl Pts',(0.0137919512760146,-0.0341934961088741,
0.0755236924027393));
#93814=CARTESIAN_POINT('Ctrl Pts',(0.0139402508431135,-0.0345231616327823,
0.0752286274112337));
#93815=CARTESIAN_POINT('Ctrl Pts',(0.0139253834828356,-0.0344132092796976,
0.0753087992426407));
#93816=CARTESIAN_POINT('Ctrl Pts',(0.0139088585985512,-0.0343032738558974,
0.0753886594179296));
#93817=CARTESIAN_POINT('Ctrl Pts',(0.0138906999812588,-0.0341934961088741,
0.0754681061692713));
#93818=CARTESIAN_POINT('Ctrl Pts',(0.0140366177341914,-0.0345231616327823,
0.0751690072934668));
#93819=CARTESIAN_POINT('Ctrl Pts',(0.0140225721532985,-0.0344132092796976,
0.0752505074067936));
#93820=CARTESIAN_POINT('Ctrl Pts',(0.0140068415315353,-0.0343032738558974,
0.0753317127933274));
#93821=CARTESIAN_POINT('Ctrl Pts',(0.013989448686503,-0.0341934961088741,
0.0754125199358033));
#93822=CARTESIAN_POINT('Origin',(-0.0026970435407176,-0.0345625596231899,
0.0719038824475933));
#93823=CARTESIAN_POINT('Ctrl Pts',(0.0139055034524896,-0.0346945769586885,
0.0757536518571653));
#93824=CARTESIAN_POINT('Ctrl Pts',(0.0138834043193351,-0.0345846629176052,
0.0758333268984792));
#93825=CARTESIAN_POINT('Ctrl Pts',(0.0138596537644608,-0.0344746925050311,
0.075912558547488));
#93826=CARTESIAN_POINT('Ctrl Pts',(0.0138342826390803,-0.0343648066253259,
0.0759912454091523));
#93827=CARTESIAN_POINT('Ctrl Pts',(0.0138438264582068,-0.0346945769586885,
0.0756585883522903));
#93828=CARTESIAN_POINT('Ctrl Pts',(0.0138230373481992,-0.0345846629176052,
0.0757374134534485));
#93829=CARTESIAN_POINT('Ctrl Pts',(0.0138006146166402,-0.0344746925050311,
0.0758158221078704));
#93830=CARTESIAN_POINT('Ctrl Pts',(0.0137765874090285,-0.0343648066253259,
0.0758937139680057));
#93831=CARTESIAN_POINT('Ctrl Pts',(0.0137821494639241,-0.0346945769586885,
0.0755635248474153));
#93832=CARTESIAN_POINT('Ctrl Pts',(0.0137626703770633,-0.0345846629176052,
0.0756415000084178));
#93833=CARTESIAN_POINT('Ctrl Pts',(0.0137415754688197,-0.0344746925050311,
0.0757190856682528));
#93834=CARTESIAN_POINT('Ctrl Pts',(0.0137188921789766,-0.0343648066253259,
0.0757961825268591));
#93835=CARTESIAN_POINT('Ctrl Pts',(0.0137204724696414,-0.0346945769586885,
0.0754684613425404));
#93836=CARTESIAN_POINT('Ctrl Pts',(0.0137023034059274,-0.0345846629176052,
0.0755455865633871));
#93837=CARTESIAN_POINT('Ctrl Pts',(0.0136825363209992,-0.0344746925050311,
0.0756223492286352));
#93838=CARTESIAN_POINT('Ctrl Pts',(0.0136611969489248,-0.0343648066253259,
0.0756986510857125));
#93839=CARTESIAN_POINT('Origin',(-0.00260012655906958,-0.0345626446730747,
0.0714329267366677));
#93840=CARTESIAN_POINT('Ctrl Pts',(0.0137215760778875,-0.0346945769586885,
0.0754701623474144));
#93841=CARTESIAN_POINT('Ctrl Pts',(0.0136939247489572,-0.0345275153362891,
0.0755874103815636));
#93842=CARTESIAN_POINT('Ctrl Pts',(0.0136625789252224,-0.0343603235965159,
0.0757038191332164));
#93843=CARTESIAN_POINT('Ctrl Pts',(0.0136276364306931,-0.0341934961088741,
0.0758190456948274));
#93844=CARTESIAN_POINT('Ctrl Pts',(0.0137390411871065,-0.0346945769586885,
0.0753881684556221));
#93845=CARTESIAN_POINT('Ctrl Pts',(0.0137131072530683,-0.0345275153362891,
0.0755057823034765));
#93846=CARTESIAN_POINT('Ctrl Pts',(0.0136834677639275,-0.0343603235965159,
0.0756226109739413));
#93847=CARTESIAN_POINT('Ctrl Pts',(0.0136502155155724,-0.0341934961088741,
0.0757383102425323));
#93848=CARTESIAN_POINT('Ctrl Pts',(0.0137565062963254,-0.0346945769586885,
0.0753061745638298));
#93849=CARTESIAN_POINT('Ctrl Pts',(0.0137322897571793,-0.0345275153362891,
0.0754241542253895));
#93850=CARTESIAN_POINT('Ctrl Pts',(0.0137043566026327,-0.0343603235965159,
0.0755414028146662));
#93851=CARTESIAN_POINT('Ctrl Pts',(0.0136727946004517,-0.0341934961088741,
0.0756575747902372));
#93852=CARTESIAN_POINT('Ctrl Pts',(0.0137739714055443,-0.0346945769586885,
0.0752241806720375));
#93853=CARTESIAN_POINT('Ctrl Pts',(0.0137514722612904,-0.0345275153362891,
0.0753425261473024));
#93854=CARTESIAN_POINT('Ctrl Pts',(0.0137252454413379,-0.0343603235965159,
0.0754601946553911));
#93855=CARTESIAN_POINT('Ctrl Pts',(0.013695373685331,-0.0341934961088741,
0.0755768393379421));
#93856=CARTESIAN_POINT('Ctrl Pts',(0.0136612049113232,-0.0340223579322365,
0.0756986205474476));
#93857=CARTESIAN_POINT('Ctrl Pts',(0.0136398453950021,-0.0339125849573552,
0.075774996048936));
#93858=CARTESIAN_POINT('Ctrl Pts',(0.0136169200923572,-0.0338030433565217,
0.0758508757898885));
#93859=CARTESIAN_POINT('Ctrl Pts',(0.0135924669229434,-0.0336938721132321,
0.0759261653317888));
#93860=CARTESIAN_POINT('Ctrl Pts',(0.0137611253839407,-0.0340223579322365,
0.0756451688965628));
#93861=CARTESIAN_POINT('Ctrl Pts',(0.0137405031052931,-0.0339125849573552,
0.0757229225619721));
#93862=CARTESIAN_POINT('Ctrl Pts',(0.0137182859974825,-0.0338030433565217,
0.0758001947575325));
#93863=CARTESIAN_POINT('Ctrl Pts',(0.0136945112322549,-0.0336938721132321,
0.0758768891837296));
#93864=CARTESIAN_POINT('Ctrl Pts',(0.0138610458565582,-0.0340223579322365,
0.075591717245678));
#93865=CARTESIAN_POINT('Ctrl Pts',(0.013841160815584,-0.0339125849573552,
0.0756708490750082));
#93866=CARTESIAN_POINT('Ctrl Pts',(0.0138196519026078,-0.0338030433565217,
0.0757495137251764));
#93867=CARTESIAN_POINT('Ctrl Pts',(0.0137965555415665,-0.0336938721132321,
0.0758276130356704));
#93868=CARTESIAN_POINT('Ctrl Pts',(0.0139609663291757,-0.0340223579322365,
0.0755382655947932));
#93869=CARTESIAN_POINT('Ctrl Pts',(0.013941818525875,-0.0339125849573552,
0.0756187755880443));
#93870=CARTESIAN_POINT('Ctrl Pts',(0.0139210178077331,-0.0338030433565217,
0.0756988326928203));
#93871=CARTESIAN_POINT('Ctrl Pts',(0.013898599850878,-0.0336938721132321,
0.0757783368876112));
#93872=CARTESIAN_POINT('Origin',(-0.00257988690662493,-0.034558964341444,
0.0719308491163725));
#93873=CARTESIAN_POINT('Ctrl Pts',(0.0137934004130372,-0.034193496108874,
0.0761135246981947));
#93874=CARTESIAN_POINT('Ctrl Pts',(0.0137663245702022,-0.0340836138581107,
0.076191705376033));
#93875=CARTESIAN_POINT('Ctrl Pts',(0.0137376439337832,-0.03397388966435,
0.0762692882635576));
#93876=CARTESIAN_POINT('Ctrl Pts',(0.0137074018677849,-0.0338644633294062,
0.0763461765249485));
#93877=CARTESIAN_POINT('Ctrl Pts',(0.0137378141295513,-0.034193496108874,
0.0760147759040939));
#93878=CARTESIAN_POINT('Ctrl Pts',(0.0137120999741102,-0.0340836138581107,
0.0760921900799998));
#93879=CARTESIAN_POINT('Ctrl Pts',(0.0136847962328711,-0.03397388966435,
0.0761690350106375));
#93880=CARTESIAN_POINT('Ctrl Pts',(0.0136559444442687,-0.0338644633294062,
0.0762452146865479));
#93881=CARTESIAN_POINT('Ctrl Pts',(0.0136822278460653,-0.034193496108874,
0.0759160271099931));
#93882=CARTESIAN_POINT('Ctrl Pts',(0.0136578753780183,-0.0340836138581107,
0.0759926747839666));
#93883=CARTESIAN_POINT('Ctrl Pts',(0.0136319485319589,-0.03397388966435,
0.0760687817577173));
#93884=CARTESIAN_POINT('Ctrl Pts',(0.0136044870207526,-0.0338644633294062,
0.0761442528481473));
#93885=CARTESIAN_POINT('Ctrl Pts',(0.0136266415625794,-0.034193496108874,
0.0758172783158922));
#93886=CARTESIAN_POINT('Ctrl Pts',(0.0136036507819263,-0.0340836138581107,
0.0758931594879334));
#93887=CARTESIAN_POINT('Ctrl Pts',(0.0135791008310468,-0.03397388966435,
0.0759685285047972));
#93888=CARTESIAN_POINT('Ctrl Pts',(0.0135530295972365,-0.0338644633294062,
0.0760432910097467));
#93889=CARTESIAN_POINT('Origin',(-0.00252744442335263,-0.0345610621864089,
0.0714525188985465));
#93890=CARTESIAN_POINT('Ctrl Pts',(0.0136380262171894,-0.0342436276873901,
0.0757843921937186));
#93891=CARTESIAN_POINT('Ctrl Pts',(0.0135763840994213,-0.0339430054201861,
0.0759923653355634));
#93892=CARTESIAN_POINT('Ctrl Pts',(0.0134992517112607,-0.0336441434784162,
0.0761951045106342));
#93893=CARTESIAN_POINT('Ctrl Pts',(0.013703843691811,-0.0342436276873901,
0.0755432116388755));
#93894=CARTESIAN_POINT('Ctrl Pts',(0.0136512978486226,-0.0339430054201861,
0.0757536671276976));
#93895=CARTESIAN_POINT('Ctrl Pts',(0.0135830489129339,-0.0336441434784162,
0.0759595667663303));
#93896=CARTESIAN_POINT('Ctrl Pts',(0.0135530386087955,-0.0335235895815128,
0.0760432647834336));
#93897=CARTESIAN_POINT('Ctrl Pts',(0.0135269740915566,-0.0334144449262719,
0.0761180091872167));
#93898=CARTESIAN_POINT('Ctrl Pts',(0.0134993354662144,-0.0333049234473133,
0.0761923009899538));
#93899=CARTESIAN_POINT('Ctrl Pts',(0.0134701494688998,-0.0331951640388588,
0.0762660419938688));
#93900=CARTESIAN_POINT('Ctrl Pts',(0.0136561181601045,-0.0335235895815128,
0.0759961927260275));
#93901=CARTESIAN_POINT('Ctrl Pts',(0.0136307016824121,-0.0334144449262719,
0.0760723562227794));
#93902=CARTESIAN_POINT('Ctrl Pts',(0.0136036825237426,-0.0333049234473133,
0.0761480821368605));
#93903=CARTESIAN_POINT('Ctrl Pts',(0.0135750864620068,-0.0331951640388588,
0.076223270508459));
#93904=CARTESIAN_POINT('Ctrl Pts',(0.0137591977114134,-0.0335235895815128,
0.0759491206686215));
#93905=CARTESIAN_POINT('Ctrl Pts',(0.0137344292732676,-0.0334144449262719,
0.0760267032583421));
#93906=CARTESIAN_POINT('Ctrl Pts',(0.0137080295812708,-0.0333049234473133,
0.0761038632837671));
#93907=CARTESIAN_POINT('Ctrl Pts',(0.0136800234551138,-0.0331951640388588,
0.0761804990230492));
#93908=CARTESIAN_POINT('Ctrl Pts',(0.0138622772627224,-0.0335235895815128,
0.0759020486112155));
#93909=CARTESIAN_POINT('Ctrl Pts',(0.013838156864123,-0.0334144449262719,
0.0759810502939047));
#93910=CARTESIAN_POINT('Ctrl Pts',(0.013812376638799,-0.0333049234473133,
0.0760596444306737));
#93911=CARTESIAN_POINT('Ctrl Pts',(0.0137849604482207,-0.0331951640388588,
0.0761377275376394));
#93912=CARTESIAN_POINT('Origin',(-0.00173093818158889,-0.0326434571768067,
0.0694310017375691));
#93913=CARTESIAN_POINT('Ctrl Pts',(0.0136598036590481,-0.0336938721132425,
0.0764674742422201));
#93914=CARTESIAN_POINT('Ctrl Pts',(0.0136462387132884,-0.0336474569764975,
0.0764998784129082));
#93915=CARTESIAN_POINT('Ctrl Pts',(0.0136322953652761,-0.033601104548885,
0.0765321215684246));
#93916=CARTESIAN_POINT('Ctrl Pts',(0.0135969940169545,-0.0334837508694627,
0.0766137538179296));
#93917=CARTESIAN_POINT('Ctrl Pts',(0.0135592892377864,-0.0333660264863639,
0.0766943041685213));
#93918=CARTESIAN_POINT('Ctrl Pts',(0.0135119755852972,-0.0336938721132425,
0.0761613420813908));
#93919=CARTESIAN_POINT('Ctrl Pts',(0.0135002025326603,-0.0336474569764975,
0.0761928809653086));
#93920=CARTESIAN_POINT('Ctrl Pts',(0.0134880610842634,-0.033601104548885,
0.0762242798697162));
#93921=CARTESIAN_POINT('Ctrl Pts',(0.0134573217310885,-0.0334837508694627,
0.076303774669705));
#93922=CARTESIAN_POINT('Ctrl Pts',(0.0134242402808307,-0.0333660264863639,
0.0763823236907537));
#93923=CARTESIAN_POINT('Ctrl Pts',(0.0135119755853047,-0.0336938721132427,
0.0761613420814074));
#93924=CARTESIAN_POINT('Ctrl Pts',(0.0135002025326691,-0.0336474569765026,
0.076192880965322));
#93925=CARTESIAN_POINT('Ctrl Pts',(0.0134880610842734,-0.0336011045488949,
0.0762242798697262));
#93926=CARTESIAN_POINT('Ctrl Pts',(0.0134575777480446,-0.033484728265791,
0.0763031125863));
#93927=CARTESIAN_POINT('Ctrl Pts',(0.0134247910462803,-0.0333679870047996,
0.0763810154949585));
#93928=CARTESIAN_POINT('Ctrl Pts',(0.0135119755852973,-0.0336938721132429,
0.0761613420813906));
#93929=CARTESIAN_POINT('Ctrl Pts',(0.0134698699389755,-0.0335278710435085,
0.0762741390876206));
#93930=CARTESIAN_POINT('Ctrl Pts',(0.0134242418205336,-0.0333620469224321,
0.0763855759900045));
#93931=CARTESIAN_POINT('Ctrl Pts',(0.0133750500022093,-0.0331951640388601,
0.0764957006196661));
#93932=CARTESIAN_POINT('Ctrl Pts',(0.0135395795394343,-0.0336938721132429,
0.076082183686136));
#93933=CARTESIAN_POINT('Ctrl Pts',(0.0134991310032703,-0.0335278710435085,
0.0761955585564404));
#93934=CARTESIAN_POINT('Ctrl Pts',(0.0134551412903517,-0.0333620469224321,
0.076307625086151));
#93935=CARTESIAN_POINT('Ctrl Pts',(0.0134075698830115,-0.0331951640388601,
0.0764184316920439));
#93936=CARTESIAN_POINT('Ctrl Pts',(0.0135671834935713,-0.0336938721132429,
0.0760030252908814));
#93937=CARTESIAN_POINT('Ctrl Pts',(0.0135283920675652,-0.0335278710435085,
0.0761169780252601));
#93938=CARTESIAN_POINT('Ctrl Pts',(0.0134860407601697,-0.0333620469224321,
0.0762296741822976));
#93939=CARTESIAN_POINT('Ctrl Pts',(0.0134400897638137,-0.0331951640388601,
0.0763411627644218));
#93940=CARTESIAN_POINT('Ctrl Pts',(0.0135947874477083,-0.0336938721132429,
0.0759238668956268));
#93941=CARTESIAN_POINT('Ctrl Pts',(0.01355765313186,-0.0335278710435085,
0.0760383974940798));
#93942=CARTESIAN_POINT('Ctrl Pts',(0.0135169402299878,-0.0333620469224321,
0.0761517232784441));
#93943=CARTESIAN_POINT('Ctrl Pts',(0.013472609644616,-0.0331951640388601,
0.0762638938367996));
#93944=CARTESIAN_POINT('Ctrl Pts',(0.0134234469406118,-0.0330240426238156,
0.0763804336672536));
#93945=CARTESIAN_POINT('Ctrl Pts',(0.0133927205438393,-0.0329142774063509,
0.0764534417123633));
#93946=CARTESIAN_POINT('Ctrl Pts',(0.0133604695486071,-0.0328043479726686,
0.0765258509541948));
#93947=CARTESIAN_POINT('Ctrl Pts',(0.0133267327162031,-0.0326943950436594,
0.0765975674932834));
#93948=CARTESIAN_POINT('Ctrl Pts',(0.013529278610008,-0.0330240426238156,
0.0763399269549991));
#93949=CARTESIAN_POINT('Ctrl Pts',(0.0134991102326606,-0.0329142774063509,
0.0764143929344615));
#93950=CARTESIAN_POINT('Ctrl Pts',(0.0134673873954709,-0.0328043479726686,
0.0764882723732995));
#93951=CARTESIAN_POINT('Ctrl Pts',(0.0134341481312477,-0.0326943950436594,
0.07656146950725));
#93952=CARTESIAN_POINT('Ctrl Pts',(0.0136351102794043,-0.0330240426238156,
0.0762994202427447));
#93953=CARTESIAN_POINT('Ctrl Pts',(0.013605499921482,-0.0329142774063509,
0.0763753441565598));
#93954=CARTESIAN_POINT('Ctrl Pts',(0.0135743052423347,-0.0328043479726686,
0.0764506937924042));
#93955=CARTESIAN_POINT('Ctrl Pts',(0.0135415635462923,-0.0326943950436594,
0.0765253715212167));
#93956=CARTESIAN_POINT('Ctrl Pts',(0.0137409419488005,-0.0330240426238156,
0.0762589135304902));
#93957=CARTESIAN_POINT('Ctrl Pts',(0.0137118896103033,-0.0329142774063509,
0.076336295378658));
#93958=CARTESIAN_POINT('Ctrl Pts',(0.0136812230891986,-0.0328043479726686,
0.0764131152115089));
#93959=CARTESIAN_POINT('Ctrl Pts',(0.0136489789613369,-0.0326943950436594,
0.0764892735351834));
#93960=CARTESIAN_POINT('Origin',(-0.00184364903173004,-0.0326396682859487,
0.0693800933573045));
#93961=CARTESIAN_POINT('Ctrl Pts',(0.0135025988803319,-0.0331951640388588,
0.0768086333040516));
#93962=CARTESIAN_POINT('Ctrl Pts',(0.01346598158494,-0.0330855618255041,
0.0768827156226605));
#93963=CARTESIAN_POINT('Ctrl Pts',(0.013427806737759,-0.0329757224427708,
0.0769560945292735));
#93964=CARTESIAN_POINT('Ctrl Pts',(0.0133881186147393,-0.0328657862078596,
0.0770286736598748));
#93965=CARTESIAN_POINT('Ctrl Pts',(0.0134598274289725,-0.0331951640388588,
0.0767036963944849));
#93966=CARTESIAN_POINT('Ctrl Pts',(0.0134246554272242,-0.0330855618255041,
0.0767771896228773));
#93967=CARTESIAN_POINT('Ctrl Pts',(0.0133879390910666,-0.0329757224427708,
0.0768500088863559));
#93968=CARTESIAN_POINT('Ctrl Pts',(0.0133497208638927,-0.0328657862078596,
0.0769220586291769));
#93969=CARTESIAN_POINT('Ctrl Pts',(0.013417055977613,-0.0331951640388587,
0.0765987594849182));
#93970=CARTESIAN_POINT('Ctrl Pts',(0.0133833292695084,-0.0330855618255041,
0.0766716636230941));
#93971=CARTESIAN_POINT('Ctrl Pts',(0.0133480714443742,-0.0329757224427708,
0.0767439232434383));
#93972=CARTESIAN_POINT('Ctrl Pts',(0.0133113231130462,-0.0328657862078596,
0.0768154435984789));
#93973=CARTESIAN_POINT('Ctrl Pts',(0.0133742845262536,-0.0331951640388587,
0.0764938225753515));
#93974=CARTESIAN_POINT('Ctrl Pts',(0.0133420031117926,-0.0330855618255041,
0.0765661376233108));
#93975=CARTESIAN_POINT('Ctrl Pts',(0.0133082037976819,-0.0329757224427708,
0.0766378376005208));
#93976=CARTESIAN_POINT('Ctrl Pts',(0.0132729253621996,-0.0328657862078596,
0.0767088285677809));
#93977=CARTESIAN_POINT('Origin',(-0.00160195152521618,-0.032640190883275,
0.0689643347885643));
#93978=CARTESIAN_POINT('Ctrl Pts',(0.0133896719571905,-0.0332451089994432,
0.076462688909589));
#93979=CARTESIAN_POINT('Ctrl Pts',(0.0133024474678981,-0.0329451141710257,
0.07666129519141));
#93980=CARTESIAN_POINT('Ctrl Pts',(0.0132005109371185,-0.0326442513127503,
0.0768527671486353));
#93981=CARTESIAN_POINT('Ctrl Pts',(0.0134852012912264,-0.0332451089994432,
0.0762316604560629));
#93982=CARTESIAN_POINT('Ctrl Pts',(0.0134066901826171,-0.0329451141710257,
0.0764338696856644));
#93983=CARTESIAN_POINT('Ctrl Pts',(0.0133131708899699,-0.0326442513127503,
0.0766295906825294));
#93984=CARTESIAN_POINT('Ctrl Pts',(0.0132729394996485,-0.0325229783203385,
0.0767088003204275));
#93985=CARTESIAN_POINT('Ctrl Pts',(0.0132376664938307,-0.032413025311208,
0.0767797813400015));
#93986=CARTESIAN_POINT('Ctrl Pts',(0.0132009305043106,-0.0323031222247695,
0.0768500219264899));
#93987=CARTESIAN_POINT('Ctrl Pts',(0.013162781762135,-0.0321934096636185,
0.0769194337671563));
#93988=CARTESIAN_POINT('Ctrl Pts',(0.0133811057945875,-0.0325229783203385,
0.076675018738332));
#93989=CARTESIAN_POINT('Ctrl Pts',(0.0133462984671316,-0.032413025311208,
0.0767474908278892));
#93990=CARTESIAN_POINT('Ctrl Pts',(0.0133099972406468,-0.0323031222247695,
0.0768192318913657));
#93991=CARTESIAN_POINT('Ctrl Pts',(0.0132722518571004,-0.0321934096636185,
0.0768901516743697));
#93992=CARTESIAN_POINT('Ctrl Pts',(0.0134892720895264,-0.0325229783203385,
0.0766412371562365));
#93993=CARTESIAN_POINT('Ctrl Pts',(0.0134549304404326,-0.032413025311208,
0.0767152003157768));
#93994=CARTESIAN_POINT('Ctrl Pts',(0.0134190639769829,-0.0323031222247695,
0.0767884418562415));
#93995=CARTESIAN_POINT('Ctrl Pts',(0.0133817219520658,-0.0321934096636185,
0.0768608695815831));
#93996=CARTESIAN_POINT('Ctrl Pts',(0.0135974383844654,-0.0325229783203385,
0.076607455574141));
#93997=CARTESIAN_POINT('Ctrl Pts',(0.0135635624137335,-0.032413025311208,
0.0766829098036644));
#93998=CARTESIAN_POINT('Ctrl Pts',(0.0135281307133191,-0.0323031222247695,
0.0767576518211172));
#93999=CARTESIAN_POINT('Ctrl Pts',(0.0134911920470313,-0.0321934096636185,
0.0768315874887965));
#94000=CARTESIAN_POINT('Origin',(-0.00183606431180876,-0.0326393375181179,
0.0693839873334145));
#94001=CARTESIAN_POINT('Ctrl Pts',(0.0133250480478731,-0.0326943950436593,
0.0771411257927735));
#94002=CARTESIAN_POINT('Ctrl Pts',(0.0132838247284816,-0.0325844576448127,
0.0772128089844631));
#94003=CARTESIAN_POINT('Ctrl Pts',(0.0132411159657214,-0.0324744968375319,
0.077283644683452));
#94004=CARTESIAN_POINT('Ctrl Pts',(0.0131969777323871,-0.0323646534831895,
0.0773535428856782));
#94005=CARTESIAN_POINT('Ctrl Pts',(0.0132889500736497,-0.0326943950436593,
0.0770337104128714));
#94006=CARTESIAN_POINT('Ctrl Pts',(0.0132492071395111,-0.0325844576448127,
0.0771048961068213));
#94007=CARTESIAN_POINT('Ctrl Pts',(0.013207989155842,-0.0324744968375319,
0.0771752648896561));
#94008=CARTESIAN_POINT('Ctrl Pts',(0.0131653501771121,-0.0323646534831895,
0.0772447273292081));
#94009=CARTESIAN_POINT('Ctrl Pts',(0.0132528520994263,-0.0326943950436593,
0.0769262950329692));
#94010=CARTESIAN_POINT('Ctrl Pts',(0.0132145895505407,-0.0325844576448127,
0.0769969832291796));
#94011=CARTESIAN_POINT('Ctrl Pts',(0.0131748623459625,-0.0324744968375319,
0.0770668850958601));
#94012=CARTESIAN_POINT('Ctrl Pts',(0.0131337226218371,-0.0323646534831895,
0.077135911772738));
#94013=CARTESIAN_POINT('Ctrl Pts',(0.013216754125203,-0.0326943950436593,
0.076818879653067));
#94014=CARTESIAN_POINT('Ctrl Pts',(0.0131799719615702,-0.0325844576448127,
0.0768890703515378));
#94015=CARTESIAN_POINT('Ctrl Pts',(0.0131417355360831,-0.0324744968375319,
0.0769585053020642));
#94016=CARTESIAN_POINT('Ctrl Pts',(0.0131020950665621,-0.0323646534831895,
0.077027096216268));
#94017=CARTESIAN_POINT('Origin',(-0.00163555586517919,-0.0326395579070148,
0.0689469362202125));
#94018=CARTESIAN_POINT('Ctrl Pts',(0.0132340839843633,-0.0327445246961876,
0.0767887384490127));
#94019=CARTESIAN_POINT('Ctrl Pts',(0.013134562337837,-0.0324436878365474,
0.0769814766299047));
#94020=CARTESIAN_POINT('Ctrl Pts',(0.013020805594427,-0.0321434074463185,
0.0771661708849035));
#94021=CARTESIAN_POINT('Ctrl Pts',(0.0133439296781406,-0.0327445246961876,
0.0765641634647457));
#94022=CARTESIAN_POINT('Ctrl Pts',(0.0132528780155232,-0.0324436878365474,
0.0767610445436624));
#94023=CARTESIAN_POINT('Ctrl Pts',(0.0131472551336846,-0.0321434074463185,
0.0769505079209493));
#94024=CARTESIAN_POINT('Ctrl Pts',(0.0130554368548483,-0.0322357242816071,
0.077109207207571));
#94025=CARTESIAN_POINT('Ctrl Pts',(0.0129611899432383,-0.0319819883628704,
0.0772662740124256));
#94026=CARTESIAN_POINT('Ctrl Pts',(0.0128571394245683,-0.0317295851069886,
0.0774170253013081));
#94027=CARTESIAN_POINT('Ctrl Pts',(0.0131793781650859,-0.0322357242816071,
0.0768920930633598));
#94028=CARTESIAN_POINT('Ctrl Pts',(0.0130920460573823,-0.0319819883628704,
0.0770531072381995));
#94029=CARTESIAN_POINT('Ctrl Pts',(0.0129946451464659,-0.0317295851069886,
0.0772082379059861));
#94030=CARTESIAN_POINT('Origin',(-0.00155227451048989,-0.0326371942648798,
0.0689932678446254));
#94031=CARTESIAN_POINT('Origin',(-0.00172664139655714,-0.0326352985534453,
0.0694395789559609));
#94032=CARTESIAN_POINT('Ctrl Pts',(0.0131269701953199,-0.0321934096636184,
0.0774618136745129));
#94033=CARTESIAN_POINT('Ctrl Pts',(0.0130812977036778,-0.0320835708272304,
0.0775308115363109));
#94034=CARTESIAN_POINT('Ctrl Pts',(0.0130342237967733,-0.0319739230346346,
0.0775988241867043));
#94035=CARTESIAN_POINT('Ctrl Pts',(0.0129858153807518,-0.0318646057455575,
0.0776657692305408));
#94036=CARTESIAN_POINT('Ctrl Pts',(0.0130976880773171,-0.0321934096636184,
0.0773523434852778));
#94037=CARTESIAN_POINT('Ctrl Pts',(0.0130535252649005,-0.0320835708272304,
0.0774209375238474));
#94038=CARTESIAN_POINT('Ctrl Pts',(0.0130079685186468,-0.0319739230346346,
0.0774885778279795));
#94039=CARTESIAN_POINT('Ctrl Pts',(0.0129610827670381,-0.0318646057455575,
0.0775551823299387));
#94040=CARTESIAN_POINT('Ctrl Pts',(0.0130684059593144,-0.0321934096636184,
0.0772428732960427));
#94041=CARTESIAN_POINT('Ctrl Pts',(0.0130257528261232,-0.0320835708272304,
0.0773110635113839));
#94042=CARTESIAN_POINT('Ctrl Pts',(0.0129817132405203,-0.0319739230346346,
0.0773783314692546));
#94043=CARTESIAN_POINT('Ctrl Pts',(0.0129363501533244,-0.0318646057455575,
0.0774445954293365));
#94044=CARTESIAN_POINT('Ctrl Pts',(0.0130391238413116,-0.0321934096636184,
0.0771334031068076));
#94045=CARTESIAN_POINT('Ctrl Pts',(0.0129979803873458,-0.0320835708272304,
0.0772011894989205));
#94046=CARTESIAN_POINT('Ctrl Pts',(0.0129554579623938,-0.0319739230346346,
0.0772680851105298));
#94047=CARTESIAN_POINT('Ctrl Pts',(0.0129116175396107,-0.0318646057455575,
0.0773340085287344));
#94048=CARTESIAN_POINT('Ctrl Pts',(0.0131030465111959,-0.0320218834582293,
0.0770271035176127));
#94049=CARTESIAN_POINT('Ctrl Pts',(0.0130731028189308,-0.0319391099350593,
0.0770789256218695));
#94050=CARTESIAN_POINT('Ctrl Pts',(0.0130423680593638,-0.0318564869454878,
0.0771302487534767));
#94051=CARTESIAN_POINT('Ctrl Pts',(0.0130108681085682,-0.0317740741446474,
0.0771810376202471));
#94052=CARTESIAN_POINT('Ctrl Pts',(0.0131511943607829,-0.0320218834582293,
0.0770153301311914));
#94053=CARTESIAN_POINT('Ctrl Pts',(0.0131213732010085,-0.0319391099350593,
0.0770676533381657));
#94054=CARTESIAN_POINT('Ctrl Pts',(0.0130907530749037,-0.0318564869454878,
0.077119479182247));
#94055=CARTESIAN_POINT('Ctrl Pts',(0.0130593598092299,-0.0317740741446474,
0.077170771997294));
#94056=CARTESIAN_POINT('Ctrl Pts',(0.01319934221037,-0.0320218834582293,
0.0770035567447701));
#94057=CARTESIAN_POINT('Ctrl Pts',(0.0131696435830863,-0.0319391099350593,
0.0770563810544619));
#94058=CARTESIAN_POINT('Ctrl Pts',(0.0131391380904436,-0.0318564869454878,
0.0771087096110174));
#94059=CARTESIAN_POINT('Ctrl Pts',(0.0131078515098917,-0.0317740741446474,
0.0771605063743409));
#94060=CARTESIAN_POINT('Ctrl Pts',(0.013247490059957,-0.0320218834582293,
0.0769917833583488));
#94061=CARTESIAN_POINT('Ctrl Pts',(0.013217913965164,-0.0319391099350593,
0.0770451087707582));
#94062=CARTESIAN_POINT('Ctrl Pts',(0.0131875231059834,-0.0318564869454878,
0.0770979400397877));
#94063=CARTESIAN_POINT('Ctrl Pts',(0.0131563432105534,-0.0317740741446474,
0.0771502407513878));
#94064=CARTESIAN_POINT('Origin',(0.0190209831310754,-0.0391228853390752,
0.0793588031300553));
#94065=CARTESIAN_POINT('Ctrl Pts',(0.0138753690461966,-0.0352722978779574,
0.0740915772819855));
#94066=CARTESIAN_POINT('Ctrl Pts',(0.013875210837716,-0.0352466642097203,
0.0741104735156868));
#94067=CARTESIAN_POINT('Ctrl Pts',(0.0138751311684267,-0.0352210183808294,
0.0741293535714064));
#94068=CARTESIAN_POINT('Ctrl Pts',(0.0138751305680331,-0.0351953608940152,
0.074148218117648));
#94069=CARTESIAN_POINT('Origin',(0.0187703048256994,-0.0352456003065023,
0.0743137189225401));
#94070=CARTESIAN_POINT('Ctrl Pts',(0.013872363194708,-0.0350241211493339,
0.0742728682562885));
#94071=CARTESIAN_POINT('Ctrl Pts',(0.0138706707349319,-0.0349144232867421,
0.0743520525990051));
#94072=CARTESIAN_POINT('Ctrl Pts',(0.0138673404652649,-0.0348045283677512,
0.0744312493530141));
#94073=CARTESIAN_POINT('Ctrl Pts',(0.0138623728765049,-0.0346945769586886,
0.0745103569186112));
#94074=CARTESIAN_POINT('Ctrl Pts',(0.0139558514978465,-0.0350241211493339,
0.0741962468164563));
#94075=CARTESIAN_POINT('Ctrl Pts',(0.0139552144669405,-0.0349144232867421,
0.0742765811762652));
#94076=CARTESIAN_POINT('Ctrl Pts',(0.0139529164861946,-0.0348045283677512,
0.0743569504521751));
#94077=CARTESIAN_POINT('Ctrl Pts',(0.0139489566682885,-0.0346945769586886,
0.0744372515918336));
#94078=CARTESIAN_POINT('Ctrl Pts',(0.014039339800985,-0.0350241211493339,
0.0741196253766241));
#94079=CARTESIAN_POINT('Ctrl Pts',(0.0140397581989491,-0.0349144232867421,
0.0742011097535254));
#94080=CARTESIAN_POINT('Ctrl Pts',(0.0140384925071243,-0.0348045283677512,
0.0742826515513361));
#94081=CARTESIAN_POINT('Ctrl Pts',(0.0140355404600722,-0.0346945769586886,
0.0743641462650559));
#94082=CARTESIAN_POINT('Ctrl Pts',(0.0141228281041235,-0.0350241211493339,
0.0740430039367919));
#94083=CARTESIAN_POINT('Ctrl Pts',(0.0141243019309577,-0.0349144232867421,
0.0741256383307855));
#94084=CARTESIAN_POINT('Ctrl Pts',(0.014124068528054,-0.0348045283677512,
0.0742083526504972));
#94085=CARTESIAN_POINT('Ctrl Pts',(0.0141221242518559,-0.0346945769586886,
0.0742910409382783));
#94086=CARTESIAN_POINT('Origin',(-0.00288114820865989,-0.03456290679414,
0.073278508408283));
#94087=CARTESIAN_POINT('Ctrl Pts',(0.0140395418760017,-0.0351970973651627,
0.074573449113318));
#94088=CARTESIAN_POINT('Ctrl Pts',(0.0140336755624119,-0.0350869349321799,
0.0746554039464499));
#94089=CARTESIAN_POINT('Ctrl Pts',(0.0140261005936722,-0.0349764985129763,
0.0747373047126031));
#94090=CARTESIAN_POINT('Ctrl Pts',(0.014016820537425,-0.0348659306849698,
0.0748190447292442));
#94091=CARTESIAN_POINT('Ctrl Pts',(0.0139826432554834,-0.0351970973651627,
0.0745140940997731));
#94092=CARTESIAN_POINT('Ctrl Pts',(0.013977599225166,-0.0350869349321799,
0.074595260679629));
#94093=CARTESIAN_POINT('Ctrl Pts',(0.0139708636082174,-0.0349764985129763,
0.0746763896343399));
#94094=CARTESIAN_POINT('Ctrl Pts',(0.0139624389437352,-0.0348659306849698,
0.0747573753452878));
#94095=CARTESIAN_POINT('Ctrl Pts',(0.0139257446349652,-0.0351970973651627,
0.0744547390862282));
#94096=CARTESIAN_POINT('Ctrl Pts',(0.0139215228879201,-0.0350869349321799,
0.074535117412808));
#94097=CARTESIAN_POINT('Ctrl Pts',(0.0139156266227625,-0.0349764985129763,
0.0746154745560767));
#94098=CARTESIAN_POINT('Ctrl Pts',(0.0139080573500455,-0.0348659306849698,
0.0746957059613315));
#94099=CARTESIAN_POINT('Ctrl Pts',(0.0138688460144469,-0.0351970973651627,
0.0743953840726833));
#94100=CARTESIAN_POINT('Ctrl Pts',(0.0138654465506742,-0.0350869349321799,
0.0744749741459871));
#94101=CARTESIAN_POINT('Ctrl Pts',(0.0138603896373077,-0.0349764985129763,
0.0745545594778135));
#94102=CARTESIAN_POINT('Ctrl Pts',(0.0138536757563557,-0.0348659306849698,
0.0746340365773751));
#94103=CARTESIAN_POINT('Origin',(-0.00279802255310622,-0.034563718796424,
0.0728047832961103));
#94104=CARTESIAN_POINT('Ctrl Pts',(0.0138712400212374,-0.0352450361861253,
0.0743617864818154));
#94105=CARTESIAN_POINT('Ctrl Pts',(0.0138632523632099,-0.0349452761023764,
0.0745785554052386));
#94106=CARTESIAN_POINT('Ctrl Pts',(0.0138389594754375,-0.0346444289983475,
0.0747941068479304));
#94107=CARTESIAN_POINT('Ctrl Pts',(0.013875013965815,-0.0352450361861253,
0.0741118149687537));
#94108=CARTESIAN_POINT('Ctrl Pts',(0.0138764541378635,-0.0349452761023764,
0.0743287262288287));
#94109=CARTESIAN_POINT('Ctrl Pts',(0.013861551575317,-0.0346444289983475,
0.0745451297465273));
#94110=CARTESIAN_POINT('Ctrl Pts',(0.0138533048573479,-0.0345231616327822,
0.0746335812268912));
#94111=CARTESIAN_POINT('Ctrl Pts',(0.0138466393709632,-0.0344132092796975,
0.0747125546302946));
#94112=CARTESIAN_POINT('Ctrl Pts',(0.0138383407259309,-0.0343032738558973,
0.0747913860887051));
#94113=CARTESIAN_POINT('Ctrl Pts',(0.0138284221407276,-0.0341934961088741,
0.0748699748822446));
#94114=CARTESIAN_POINT('Ctrl Pts',(0.0139414394845606,-0.0345231616327822,
0.0745623532574936));
#94115=CARTESIAN_POINT('Ctrl Pts',(0.0139357557754531,-0.0344132092796975,
0.0746425414726495));
#94116=CARTESIAN_POINT('Ctrl Pts',(0.0139284137296199,-0.0343032738558973,
0.0747226079874224));
#94117=CARTESIAN_POINT('Ctrl Pts',(0.0139194253805535,-0.0341934961088741,
0.0748024504682921));
#94118=CARTESIAN_POINT('Ctrl Pts',(0.0140295741117733,-0.0345231616327822,
0.074491125288096));
#94119=CARTESIAN_POINT('Ctrl Pts',(0.014024872179943,-0.0344132092796975,
0.0745725283150044));
#94120=CARTESIAN_POINT('Ctrl Pts',(0.0140184867333089,-0.0343032738558973,
0.0746538298861396));
#94121=CARTESIAN_POINT('Ctrl Pts',(0.0140104286203793,-0.0341934961088741,
0.0747349260543396));
#94122=CARTESIAN_POINT('Ctrl Pts',(0.014117708738986,-0.0345231616327822,
0.0744198973186984));
#94123=CARTESIAN_POINT('Ctrl Pts',(0.0141139885844328,-0.0344132092796975,
0.0745025151573592));
#94124=CARTESIAN_POINT('Ctrl Pts',(0.0141085597369979,-0.0343032738558973,
0.0745850517848568));
#94125=CARTESIAN_POINT('Ctrl Pts',(0.0141014318602052,-0.0341934961088741,
0.0746674016403871));
#94126=CARTESIAN_POINT('Origin',(-0.00289323127354824,-0.034562559623145,
0.0732778028343769));
#94127=CARTESIAN_POINT('Ctrl Pts',(0.0140609037262127,-0.0346945769586885,
0.0750163647622781));
#94128=CARTESIAN_POINT('Ctrl Pts',(0.0140489647818862,-0.0345846629176052,
0.0750981812979107));
#94129=CARTESIAN_POINT('Ctrl Pts',(0.0140353318660018,-0.0344746925050311,
0.0751797649155431));
#94130=CARTESIAN_POINT('Ctrl Pts',(0.0140200228783344,-0.0343648066253259,
0.0752610111529836));
#94131=CARTESIAN_POINT('Ctrl Pts',(0.013987798456992,-0.0346945769586885,
0.0749297810386632));
#94132=CARTESIAN_POINT('Ctrl Pts',(0.0139770526801405,-0.0345846629176052,
0.075010590146735));
#94133=CARTESIAN_POINT('Ctrl Pts',(0.0139646339687153,-0.0344746925050311,
0.0750911908389489));
#94134=CARTESIAN_POINT('Ctrl Pts',(0.0139505586615112,-0.0343648066253259,
0.0751714799061253));
#94135=CARTESIAN_POINT('Ctrl Pts',(0.0139146931877713,-0.0346945769586885,
0.0748431973150483));
#94136=CARTESIAN_POINT('Ctrl Pts',(0.0139051405783948,-0.0345846629176052,
0.0749229989955593));
#94137=CARTESIAN_POINT('Ctrl Pts',(0.0138939360714287,-0.0344746925050311,
0.0750026167623547));
#94138=CARTESIAN_POINT('Ctrl Pts',(0.013881094444688,-0.0343648066253259,
0.0750819486592671));
#94139=CARTESIAN_POINT('Ctrl Pts',(0.0138415879185506,-0.0346945769586885,
0.0747566135914333));
#94140=CARTESIAN_POINT('Ctrl Pts',(0.013833228476649,-0.0345846629176052,
0.0748354078443836));
#94141=CARTESIAN_POINT('Ctrl Pts',(0.0138232381741422,-0.0344746925050311,
0.0749140426857605));
#94142=CARTESIAN_POINT('Ctrl Pts',(0.0138116302278648,-0.0343648066253259,
0.0749924174124088));
#94143=CARTESIAN_POINT('Origin',(-0.00285610491349698,-0.034562644673227,
0.0727984138314592));
#94144=CARTESIAN_POINT('Ctrl Pts',(0.0138428960169573,-0.0346945769586885,
0.0747581628645858));
#94145=CARTESIAN_POINT('Ctrl Pts',(0.0138301578022637,-0.034527515336289,
0.0748779519934327));
#94146=CARTESIAN_POINT('Ctrl Pts',(0.0138136490349714,-0.0343603235965158,
0.0749973715007565));
#94147=CARTESIAN_POINT('Ctrl Pts',(0.0137934237900075,-0.0341934961088739,
0.0751160689223409));
#94148=CARTESIAN_POINT('Ctrl Pts',(0.0138499468489827,-0.0346945769586885,
0.0746746265605078));
#94149=CARTESIAN_POINT('Ctrl Pts',(0.013838958335624,-0.034527515336289,
0.0747945633718544));
#94150=CARTESIAN_POINT('Ctrl Pts',(0.0138241950777504,-0.0343603235965158,
0.0749141856263728));
#94151=CARTESIAN_POINT('Ctrl Pts',(0.013805705996759,-0.0341934961088739,
0.0750331401834829));
#94152=CARTESIAN_POINT('Ctrl Pts',(0.013856997681008,-0.0346945769586885,
0.0745910902564298));
#94153=CARTESIAN_POINT('Ctrl Pts',(0.0138477588689843,-0.034527515336289,
0.0747111747502762));
#94154=CARTESIAN_POINT('Ctrl Pts',(0.0138347411205294,-0.0343603235965158,
0.074830999751989));
#94155=CARTESIAN_POINT('Ctrl Pts',(0.0138179882035106,-0.0341934961088739,
0.0749502114446248));
#94156=CARTESIAN_POINT('Ctrl Pts',(0.0138640485130333,-0.0346945769586885,
0.0745075539523517));
#94157=CARTESIAN_POINT('Ctrl Pts',(0.0138565594023446,-0.034527515336289,
0.0746277861286979));
#94158=CARTESIAN_POINT('Ctrl Pts',(0.0138452871633084,-0.0343603235965158,
0.0747478138776052));
#94159=CARTESIAN_POINT('Ctrl Pts',(0.0138302704102621,-0.0341934961088739,
0.0748672827057668));
#94160=CARTESIAN_POINT('Ctrl Pts',(0.0138116343000179,-0.0340223579322365,
0.0749923861169942));
#94161=CARTESIAN_POINT('Ctrl Pts',(0.0138000155984294,-0.0339125849573554,
0.0750708364320888));
#94162=CARTESIAN_POINT('Ctrl Pts',(0.0137867813219389,-0.0338030433565221,
0.0751489911409305));
#94163=CARTESIAN_POINT('Ctrl Pts',(0.0137719572548097,-0.0336938721132328,
0.0752267517970983));
#94164=CARTESIAN_POINT('Ctrl Pts',(0.0139040676016188,-0.0340223579322365,
0.0749268325924097));
#94165=CARTESIAN_POINT('Ctrl Pts',(0.0138933530541051,-0.0339125849573554,
0.0750065578038095));
#94166=CARTESIAN_POINT('Ctrl Pts',(0.0138809959089597,-0.0338030433565221,
0.07508600522699));
#94167=CARTESIAN_POINT('Ctrl Pts',(0.0138670209752888,-0.0336938721132328,
0.075165074662932));
#94168=CARTESIAN_POINT('Ctrl Pts',(0.0139965009032197,-0.0340223579322365,
0.0748612790678253));
#94169=CARTESIAN_POINT('Ctrl Pts',(0.0139866905097808,-0.0339125849573554,
0.0749422791755303));
#94170=CARTESIAN_POINT('Ctrl Pts',(0.0139752104959805,-0.0338030433565221,
0.0750230193130495));
#94171=CARTESIAN_POINT('Ctrl Pts',(0.013962084695768,-0.0336938721132328,
0.0751033975287658));
#94172=CARTESIAN_POINT('Ctrl Pts',(0.0140889342048206,-0.0340223579322365,
0.0747957255432408));
#94173=CARTESIAN_POINT('Ctrl Pts',(0.0140800279654565,-0.0339125849573554,
0.0748780005472511));
#94174=CARTESIAN_POINT('Ctrl Pts',(0.0140694250830013,-0.0338030433565221,
0.074960033399109));
#94175=CARTESIAN_POINT('Ctrl Pts',(0.0140571484162471,-0.0336938721132328,
0.0750417203945996));
#94176=CARTESIAN_POINT('Origin',(-0.00277361863472758,-0.0345589643412889,
0.0732898732429793));
#94177=CARTESIAN_POINT('Ctrl Pts',(0.0139947886795483,-0.034193496108874,
0.0753874501348942));
#94178=CARTESIAN_POINT('Ctrl Pts',(0.0139777249749769,-0.0340836138581107,
0.0754684078376702));
#94179=CARTESIAN_POINT('Ctrl Pts',(0.0139589942081052,-0.03397388966435,
0.075548973597857));
#94180=CARTESIAN_POINT('Ctrl Pts',(0.0139386272642535,-0.0338644633294062,
0.0756290459082627));
#94181=CARTESIAN_POINT('Ctrl Pts',(0.0139272642048352,-0.034193496108874,
0.0752964468131808));
#94182=CARTESIAN_POINT('Ctrl Pts',(0.0139114553821803,-0.0340836138581107,
0.075376473393437));
#94183=CARTESIAN_POINT('Ctrl Pts',(0.0138939981627359,-0.03397388966435,
0.0754561344450221));
#94184=CARTESIAN_POINT('Ctrl Pts',(0.013874921724218,-0.0338644633294062,
0.0755353295093939));
#94185=CARTESIAN_POINT('Ctrl Pts',(0.0138597397301222,-0.034193496108874,
0.0752054434914675));
#94186=CARTESIAN_POINT('Ctrl Pts',(0.0138451857893837,-0.0340836138581107,
0.0752845389492037));
#94187=CARTESIAN_POINT('Ctrl Pts',(0.0138290021173665,-0.03397388966435,
0.0753632952921872));
#94188=CARTESIAN_POINT('Ctrl Pts',(0.0138112161841826,-0.0338644633294062,
0.0754416131105251));
#94189=CARTESIAN_POINT('Ctrl Pts',(0.0137922152554091,-0.034193496108874,
0.0751144401697541));
#94190=CARTESIAN_POINT('Ctrl Pts',(0.013778916196587,-0.0340836138581107,
0.0751926045049705));
#94191=CARTESIAN_POINT('Ctrl Pts',(0.0137640060719971,-0.03397388966435,
0.0752704561393523));
#94192=CARTESIAN_POINT('Ctrl Pts',(0.0137475106441471,-0.0338644633294062,
0.0753478967116564));
#94193=CARTESIAN_POINT('Origin',(-0.00278154034885785,-0.0345610621863028,
0.072808742015884));
#94194=CARTESIAN_POINT('Ctrl Pts',(0.0137993884145856,-0.03424362768739,
0.0750803864889012));
#94195=CARTESIAN_POINT('Ctrl Pts',(0.0137642983096897,-0.033943005420186,
0.0752944455063475));
#94196=CARTESIAN_POINT('Ctrl Pts',(0.01371318408983,-0.0336441434784164,
0.0755052532740882));
#94197=CARTESIAN_POINT('Ctrl Pts',(0.0138344589599498,-0.03424362768739,
0.0748328585978508));
#94198=CARTESIAN_POINT('Ctrl Pts',(0.0138087045233651,-0.033943005420186,
0.0750482403227206));
#94199=CARTESIAN_POINT('Ctrl Pts',(0.0137667998184188,-0.0336441434784164,
0.0752610702410006));
#94200=CARTESIAN_POINT('Ctrl Pts',(0.0137475162976187,-0.0335235895815127,
0.0753478695626977));
#94201=CARTESIAN_POINT('Ctrl Pts',(0.0137310252647002,-0.0334144449262719,
0.0754252913347587));
#94202=CARTESIAN_POINT('Ctrl Pts',(0.0137129158100385,-0.0333049234473133,
0.0755024613627267));
#94203=CARTESIAN_POINT('Ctrl Pts',(0.0136932021514972,-0.0331951640388589,
0.0755792788722186));
#94204=CARTESIAN_POINT('Ctrl Pts',(0.0138438833427115,-0.0335235895815127,
0.0752882493890444));
#94205=CARTESIAN_POINT('Ctrl Pts',(0.0138282130988648,-0.0334144449262719,
0.0753669978432104));
#94206=CARTESIAN_POINT('Ctrl Pts',(0.013810897968008,-0.0333049234473133,
0.0754455130343649));
#94207=CARTESIAN_POINT('Ctrl Pts',(0.0137919509964991,-0.0331951640388589,
0.0755236925600801));
#94208=CARTESIAN_POINT('Ctrl Pts',(0.0139402503878044,-0.0335235895815127,
0.0752286292153912));
#94209=CARTESIAN_POINT('Ctrl Pts',(0.0139254009330293,-0.0334144449262719,
0.0753087043516621));
#94210=CARTESIAN_POINT('Ctrl Pts',(0.0139088801259775,-0.0333049234473133,
0.0753885647060031));
#94211=CARTESIAN_POINT('Ctrl Pts',(0.0138906998415011,-0.0331951640388589,
0.0754681062479417));
#94212=CARTESIAN_POINT('Ctrl Pts',(0.0140366174328973,-0.0335235895815127,
0.0751690090417379));
#94213=CARTESIAN_POINT('Ctrl Pts',(0.0140225887671938,-0.0334144449262719,
0.0752504108601138));
#94214=CARTESIAN_POINT('Ctrl Pts',(0.0140068622839471,-0.0333049234473133,
0.0753316163776412));
#94215=CARTESIAN_POINT('Ctrl Pts',(0.013989448686503,-0.0331951640388589,
0.0754125199358033));
#94216=CARTESIAN_POINT('Origin',(-0.00224467807951498,-0.0326434571769961,
0.07070333641904));
#94217=CARTESIAN_POINT('Ctrl Pts',(0.013906607016739,-0.0336938721132417,
0.0757553527942172));
#94218=CARTESIAN_POINT('Ctrl Pts',(0.0138972103541217,-0.0336474569764972,
0.0757892015868557));
#94219=CARTESIAN_POINT('Ctrl Pts',(0.0138874180925144,-0.033601104548885,
0.0758229380603531));
#94220=CARTESIAN_POINT('Ctrl Pts',(0.0138626263385752,-0.0334837508643185,
0.0759083510510667));
#94221=CARTESIAN_POINT('Ctrl Pts',(0.0138353145074499,-0.0333660264760452,
0.0759929919036535));
#94222=CARTESIAN_POINT('Ctrl Pts',(0.013721576077889,-0.0336938721132417,
0.0754701623474079));
#94223=CARTESIAN_POINT('Ctrl Pts',(0.0137138487295931,-0.0336474569764972,
0.0755029280925615));
#94224=CARTESIAN_POINT('Ctrl Pts',(0.0137057383463631,-0.033601104548885,
0.0755356011342169));
#94225=CARTESIAN_POINT('Ctrl Pts',(0.0136852047216034,-0.0334837508643185,
0.0756183217601209));
#94226=CARTESIAN_POINT('Ctrl Pts',(0.0136622289301495,-0.0333660264760452,
0.075700397607377));
#94227=CARTESIAN_POINT('Ctrl Pts',(0.0137215760778975,-0.0336938721132427,
0.0754701623474244));
#94228=CARTESIAN_POINT('Ctrl Pts',(0.0137138487296023,-0.0336474569765026,
0.0755029280925747));
#94229=CARTESIAN_POINT('Ctrl Pts',(0.0137057383463731,-0.0336011045488949,
0.0755356011342269));
#94230=CARTESIAN_POINT('Ctrl Pts',(0.0136853757387396,-0.0334847282606778,
0.0756176328099879));
#94231=CARTESIAN_POINT('Ctrl Pts',(0.0136626113922525,-0.0333679869945434,
0.07569903069784));
#94232=CARTESIAN_POINT('Ctrl Pts',(0.0137215760778892,-0.0336938721132429,
0.0754701623474071));
#94233=CARTESIAN_POINT('Ctrl Pts',(0.0136939396606921,-0.0335278710435085,
0.0755873471523571));
#94234=CARTESIAN_POINT('Ctrl Pts',(0.0136626380809068,-0.0333620469224321,
0.0757036240611069));
#94235=CARTESIAN_POINT('Ctrl Pts',(0.0136276364306934,-0.0331951640388602,
0.0758190456948265));
#94236=CARTESIAN_POINT('Ctrl Pts',(0.0137390411889619,-0.0336938721132429,
0.0753881684469115));
#94237=CARTESIAN_POINT('Ctrl Pts',(0.0137131212406871,-0.0335278710435085,
0.0755057188683304));
#94238=CARTESIAN_POINT('Ctrl Pts',(0.0136835240603369,-0.0333620469224321,
0.0756224150929454));
#94239=CARTESIAN_POINT('Ctrl Pts',(0.0136502155179694,-0.0331951640388602,
0.0757383102339616));
#94240=CARTESIAN_POINT('Ctrl Pts',(0.0137565063000346,-0.0336938721132429,
0.0753061745464158));
#94241=CARTESIAN_POINT('Ctrl Pts',(0.0137323028206821,-0.0335278710435085,
0.0754240905843038));
#94242=CARTESIAN_POINT('Ctrl Pts',(0.013704410039767,-0.0333620469224321,
0.0755412061247839));
#94243=CARTESIAN_POINT('Ctrl Pts',(0.0136727946052454,-0.0331951640388602,
0.0756575747730968));
#94244=CARTESIAN_POINT('Ctrl Pts',(0.0137739714111073,-0.0336938721132429,
0.0752241806459202));
#94245=CARTESIAN_POINT('Ctrl Pts',(0.0137514844006771,-0.0335278710435085,
0.0753424623002772));
#94246=CARTESIAN_POINT('Ctrl Pts',(0.0137252960191972,-0.0333620469224321,
0.0754599971566224));
#94247=CARTESIAN_POINT('Ctrl Pts',(0.0136953736925213,-0.0331951640388602,
0.0755768393122319));
#94248=CARTESIAN_POINT('Ctrl Pts',(0.0136612049649121,-0.0330240426238156,
0.0756986219119778));
#94249=CARTESIAN_POINT('Ctrl Pts',(0.0136398711893255,-0.0329142774063509,
0.0757749053055085));
#94250=CARTESIAN_POINT('Ctrl Pts',(0.0136169497872423,-0.0328043479726686,
0.0758507857003587));
#94251=CARTESIAN_POINT('Ctrl Pts',(0.0135924674455825,-0.0326943950436594,
0.0759261650794112));
#94252=CARTESIAN_POINT('Ctrl Pts',(0.0137611252827565,-0.0330240426238156,
0.0756451703819095));
#94253=CARTESIAN_POINT('Ctrl Pts',(0.0137405278540719,-0.0329142774063509,
0.0757228302751662));
#94254=CARTESIAN_POINT('Ctrl Pts',(0.013718314709892,-0.0328043479726686,
0.075800103078325));
#94255=CARTESIAN_POINT('Ctrl Pts',(0.0136945115806809,-0.0326943950436594,
0.0758768890154778));
#94256=CARTESIAN_POINT('Ctrl Pts',(0.0138610456006008,-0.0330240426238156,
0.0755917188518412));
#94257=CARTESIAN_POINT('Ctrl Pts',(0.0138411845188182,-0.0329142774063509,
0.0756707552448238));
#94258=CARTESIAN_POINT('Ctrl Pts',(0.0138196796325417,-0.0328043479726686,
0.0757494204562913));
#94259=CARTESIAN_POINT('Ctrl Pts',(0.0137965557157793,-0.0326943950436594,
0.0758276129515443));
#94260=CARTESIAN_POINT('Ctrl Pts',(0.0139609659184451,-0.0330240426238156,
0.0755382673217728));
#94261=CARTESIAN_POINT('Ctrl Pts',(0.0139418411835645,-0.0329142774063509,
0.0756186802144815));
#94262=CARTESIAN_POINT('Ctrl Pts',(0.0139210445551914,-0.0328043479726686,
0.0756987378342575));
#94263=CARTESIAN_POINT('Ctrl Pts',(0.0138985998508777,-0.0326943950436594,
0.0757783368876108));
#94264=CARTESIAN_POINT('Origin',(-0.00236288068206818,-0.0326396682854024,
0.0706669558810331));
#94265=CARTESIAN_POINT('Ctrl Pts',(0.0137934004130372,-0.0331951640388588,
0.0761135246981947));
#94266=CARTESIAN_POINT('Ctrl Pts',(0.0137663568324977,-0.0330855618255041,
0.0761916122196299));
#94267=CARTESIAN_POINT('Ctrl Pts',(0.0137376798210301,-0.0329757224427708,
0.0762691970886851));
#94268=CARTESIAN_POINT('Ctrl Pts',(0.0137074012278423,-0.0328657862078596,
0.0763461781519554));
#94269=CARTESIAN_POINT('Ctrl Pts',(0.0137378141451506,-0.0331951640388588,
0.0760147759318061));
#94270=CARTESIAN_POINT('Ctrl Pts',(0.013712130629101,-0.0330855618255041,
0.0760920978648513));
#94271=CARTESIAN_POINT('Ctrl Pts',(0.0136848304859782,-0.0329757224427708,
0.0761689447038226));
#94272=CARTESIAN_POINT('Ctrl Pts',(0.013655943848186,-0.0328657862078596,
0.076245216326894));
#94273=CARTESIAN_POINT('Ctrl Pts',(0.0136822278772641,-0.0331951640388588,
0.0759160271654175));
#94274=CARTESIAN_POINT('Ctrl Pts',(0.0136579044257043,-0.0330855618255041,
0.0759925835100727));
#94275=CARTESIAN_POINT('Ctrl Pts',(0.0136319811509262,-0.0329757224427708,
0.0760686923189602));
#94276=CARTESIAN_POINT('Ctrl Pts',(0.0136044864685298,-0.0328657862078596,
0.0761442545018326));
#94277=CARTESIAN_POINT('Ctrl Pts',(0.0136266416093775,-0.0331951640388588,
0.0758172783990289));
#94278=CARTESIAN_POINT('Ctrl Pts',(0.0136036782223076,-0.0330855618255041,
0.0758930691552941));
#94279=CARTESIAN_POINT('Ctrl Pts',(0.0135791318158743,-0.0329757224427708,
0.0759684399340977));
#94280=CARTESIAN_POINT('Ctrl Pts',(0.0135530290888735,-0.0328657862078596,
0.0760432926767712));
#94281=CARTESIAN_POINT('Origin',(-0.00217519739879767,-0.0326401908830531,
0.0702241829630992));
#94282=CARTESIAN_POINT('Ctrl Pts',(0.0136380056228228,-0.0332451089994433,
0.0757844616750446));
#94283=CARTESIAN_POINT('Ctrl Pts',(0.013576360892188,-0.0329451141710259,
0.0759924340143016));
#94284=CARTESIAN_POINT('Ctrl Pts',(0.0134992259609365,-0.0326442513127504,
0.0761951721929752));
#94285=CARTESIAN_POINT('Ctrl Pts',(0.0137038261364008,-0.0332451089994433,
0.0755432819495444));
#94286=CARTESIAN_POINT('Ctrl Pts',(0.0136512776479356,-0.0329451141710259,
0.0757537367500862));
#94287=CARTESIAN_POINT('Ctrl Pts',(0.0135830261282573,-0.0326442513127504,
0.07595963550378));
#94288=CARTESIAN_POINT('Ctrl Pts',(0.0135530395745123,-0.0325229783203384,
0.0760432628802644));
#94289=CARTESIAN_POINT('Ctrl Pts',(0.0135269409875858,-0.0324130253112079,
0.0761181050731748));
#94290=CARTESIAN_POINT('Ctrl Pts',(0.0134992981521476,-0.0323031222247694,
0.0761923960320136));
#94291=CARTESIAN_POINT('Ctrl Pts',(0.0134701498346369,-0.0321934096636184,
0.0762660418447972));
#94292=CARTESIAN_POINT('Ctrl Pts',(0.0136561189909885,-0.0325229783203384,
0.0759961908445267));
#94293=CARTESIAN_POINT('Ctrl Pts',(0.0136306692910335,-0.0324130253112079,
0.0760724539849131));
#94294=CARTESIAN_POINT('Ctrl Pts',(0.013603645850027,-0.0323031222247694,
0.0761481790987737));
#94295=CARTESIAN_POINT('Ctrl Pts',(0.0135750867058314,-0.0321934096636184,
0.0762232704090779));
#94296=CARTESIAN_POINT('Ctrl Pts',(0.0137591984074648,-0.0325229783203384,
0.0759491188087889));
#94297=CARTESIAN_POINT('Ctrl Pts',(0.0137343975944812,-0.0324130253112079,
0.0760268028966513));
#94298=CARTESIAN_POINT('Ctrl Pts',(0.0137079935479064,-0.0323031222247694,
0.0761039621655338));
#94299=CARTESIAN_POINT('Ctrl Pts',(0.013680023577026,-0.0321934096636184,
0.0761804989733586));
#94300=CARTESIAN_POINT('Ctrl Pts',(0.0138622778239411,-0.0325229783203384,
0.0759020467730511));
#94301=CARTESIAN_POINT('Ctrl Pts',(0.013838125897929,-0.0324130253112079,
0.0759811518083896));
#94302=CARTESIAN_POINT('Ctrl Pts',(0.0138123412457858,-0.0323031222247694,
0.076059745232294));
#94303=CARTESIAN_POINT('Ctrl Pts',(0.0137849604482206,-0.0321934096636184,
0.0761377275376394));
#94304=CARTESIAN_POINT('Origin',(-0.00235486772564658,-0.0326393375178655,
0.0706698685348405));
#94305=CARTESIAN_POINT('Ctrl Pts',(0.0136589219806714,-0.0326943950436593,
0.0764656484042864));
#94306=CARTESIAN_POINT('Ctrl Pts',(0.0136270080056728,-0.0325844576448127,
0.0765419330045164));
#94307=CARTESIAN_POINT('Ctrl Pts',(0.0135935140814695,-0.0324744968375319,
0.0766175629701994));
#94308=CARTESIAN_POINT('Ctrl Pts',(0.0135584844589939,-0.0323646534831895,
0.076692441991731));
#94309=CARTESIAN_POINT('Ctrl Pts',(0.0136096459328591,-0.0326943950436593,
0.0763636043025727));
#94310=CARTESIAN_POINT('Ctrl Pts',(0.0135791383168331,-0.0325844576448127,
0.0764392097865106));
#94311=CARTESIAN_POINT('Ctrl Pts',(0.013547064896371,-0.0324744968375319,
0.0765141896736488));
#94312=CARTESIAN_POINT('Ctrl Pts',(0.0135134680908844,-0.0323646534831894,
0.0765884484621976));
#94313=CARTESIAN_POINT('Ctrl Pts',(0.0135603698850467,-0.0326943950436593,
0.076261560200859));
#94314=CARTESIAN_POINT('Ctrl Pts',(0.0135312686279934,-0.0325844576448127,
0.0763364865685049));
#94315=CARTESIAN_POINT('Ctrl Pts',(0.0135006157112725,-0.0324744968375319,
0.0764108163770983));
#94316=CARTESIAN_POINT('Ctrl Pts',(0.0134684517227749,-0.0323646534831894,
0.0764844549326643));
#94317=CARTESIAN_POINT('Ctrl Pts',(0.0135110938372344,-0.0326943950436593,
0.0761595160991453));
#94318=CARTESIAN_POINT('Ctrl Pts',(0.0134833989391537,-0.0325844576448127,
0.0762337633504992));
#94319=CARTESIAN_POINT('Ctrl Pts',(0.013454166526174,-0.0324744968375319,
0.0763074430805478));
#94320=CARTESIAN_POINT('Ctrl Pts',(0.0134234353546655,-0.0323646534831894,
0.076380461403131));
#94321=CARTESIAN_POINT('Origin',(-0.00221071737745596,-0.0326395579069148,
0.07021113332839));
#94322=CARTESIAN_POINT('Ctrl Pts',(0.0135245093507114,-0.0327445246961878,
0.0761274405602016));
#94323=CARTESIAN_POINT('Ctrl Pts',(0.0134499289615361,-0.0324436878365476,
0.0763311323127379));
#94324=CARTESIAN_POINT('Ctrl Pts',(0.0133602175522251,-0.0321434074463188,
0.0765286276988619));
#94325=CARTESIAN_POINT('Ctrl Pts',(0.0136053421694281,-0.0327445246961878,
0.0758908691007685));
#94326=CARTESIAN_POINT('Ctrl Pts',(0.0135396842186145,-0.0324436878365476,
0.0760976095128697));
#94327=CARTESIAN_POINT('Ctrl Pts',(0.0134586402624646,-0.0321434074463188,
0.0762988169721559));
#94328=CARTESIAN_POINT('Ctrl Pts',(0.0133874362929384,-0.0322357242816073,
0.0764677727492884));
#94329=CARTESIAN_POINT('Ctrl Pts',(0.0133136182369147,-0.0319819883628706,
0.0766354133056589));
#94330=CARTESIAN_POINT('Ctrl Pts',(0.0132292823341623,-0.0317295851069885,
0.0767980168635604));
#94331=CARTESIAN_POINT('Ctrl Pts',(0.0134831886711788,-0.0322357242816073,
0.0762368366497688));
#94332=CARTESIAN_POINT('Ctrl Pts',(0.0134167256304116,-0.0319819883628706,
0.0764075267952));
#94333=CARTESIAN_POINT('Ctrl Pts',(0.0133395357829886,-0.0317295851069885,
0.0765736417824531));
#94334=CARTESIAN_POINT('Origin',(-0.00212228582860941,-0.0326371942647832,
0.0702466616927344));
#94335=CARTESIAN_POINT('Origin',(-0.00223934016449962,-0.0326352985530809,
0.0707113074730911));
#94336=CARTESIAN_POINT('Ctrl Pts',(0.013502598880332,-0.0321934096636183,
0.0768086333040518));
#94337=CARTESIAN_POINT('Ctrl Pts',(0.0134659342550564,-0.0320835708272303,
0.0768828113781633));
#94338=CARTESIAN_POINT('Ctrl Pts',(0.0134277557853652,-0.0319739230346346,
0.0769561876534628));
#94339=CARTESIAN_POINT('Ctrl Pts',(0.0133881195229781,-0.0318646057455575,
0.0770286719989447));
#94340=CARTESIAN_POINT('Ctrl Pts',(0.01345982740778,-0.0321934096636183,
0.0767036963424907));
#94341=CARTESIAN_POINT('Ctrl Pts',(0.0134246099449873,-0.0320835708272303,
0.0767772845646617));
#94342=CARTESIAN_POINT('Ctrl Pts',(0.0133878900053211,-0.0319739230346346,
0.076850101279111));
#94343=CARTESIAN_POINT('Ctrl Pts',(0.0133497217194684,-0.0318646057455575,
0.0769220569275356));
#94344=CARTESIAN_POINT('Ctrl Pts',(0.0134170559352281,-0.0321934096636183,
0.0765987593809296));
#94345=CARTESIAN_POINT('Ctrl Pts',(0.0133832856349181,-0.0320835708272303,
0.07667175775116));
#94346=CARTESIAN_POINT('Ctrl Pts',(0.013348024225277,-0.0319739230346346,
0.0767440149047593));
#94347=CARTESIAN_POINT('Ctrl Pts',(0.0133113239159587,-0.0318646057455575,
0.0768154418561265));
#94348=CARTESIAN_POINT('Ctrl Pts',(0.0133742844626761,-0.0321934096636183,
0.0764938224193685));
#94349=CARTESIAN_POINT('Ctrl Pts',(0.013341961324849,-0.0320835708272303,
0.0765662309376583));
#94350=CARTESIAN_POINT('Ctrl Pts',(0.0133081584452328,-0.0319739230346346,
0.0766379285304076));
#94351=CARTESIAN_POINT('Ctrl Pts',(0.013272926112449,-0.0318646057455575,
0.0767088267847174));
#94352=CARTESIAN_POINT('Ctrl Pts',(0.0134243802119738,-0.0320218834582289,
0.0763803493992706));
#94353=CARTESIAN_POINT('Ctrl Pts',(0.0134011676665627,-0.0319391099350591,
0.076435515810533));
#94354=CARTESIAN_POINT('Ctrl Pts',(0.013377107753796,-0.0318564869454879,
0.0764902863307171));
#94355=CARTESIAN_POINT('Ctrl Pts',(0.0133522217224225,-0.0317740741446479,
0.0765446227027933));
#94356=CARTESIAN_POINT('Ctrl Pts',(0.0134706728047956,-0.0320218834582289,
0.0763626343238399));
#94357=CARTESIAN_POINT('Ctrl Pts',(0.0134476446304938,-0.0319391099350591,
0.0764182825290819));
#94358=CARTESIAN_POINT('Ctrl Pts',(0.0134237614538501,-0.0318564869454879,
0.0764735374303196));
#94359=CARTESIAN_POINT('Ctrl Pts',(0.0133990444278215,-0.0317740741446479,
0.0765283604056984));
#94360=CARTESIAN_POINT('Ctrl Pts',(0.0135169653976174,-0.0320218834582289,
0.0763449192484091));
#94361=CARTESIAN_POINT('Ctrl Pts',(0.013494121594425,-0.0319391099350591,
0.0764010492476308));
#94362=CARTESIAN_POINT('Ctrl Pts',(0.0134704151539042,-0.0318564869454879,
0.0764567885299222));
#94363=CARTESIAN_POINT('Ctrl Pts',(0.0134458671332205,-0.0317740741446479,
0.0765120981086035));
#94364=CARTESIAN_POINT('Ctrl Pts',(0.0135632579904393,-0.0320218834582289,
0.0763272041729783));
#94365=CARTESIAN_POINT('Ctrl Pts',(0.0135405985583561,-0.0319391099350591,
0.0763838159661797));
#94366=CARTESIAN_POINT('Ctrl Pts',(0.0135170688539583,-0.0318564869454879,
0.0764400396295247));
#94367=CARTESIAN_POINT('Ctrl Pts',(0.0134926898386194,-0.0317740741446479,
0.0764958358115086));
#94368=CARTESIAN_POINT('Origin',(0.0195878915861359,-0.0391228853390771,
0.0779519487312299));
#94369=CARTESIAN_POINT('Ctrl Pts',(0.013822693757782,-0.0352722978779567,
0.0733711729841441));
#94370=CARTESIAN_POINT('Ctrl Pts',(0.0138249051228944,-0.0352466642097199,
0.0733899400441789));
#94371=CARTESIAN_POINT('Ctrl Pts',(0.0138271923802544,-0.0352210183808292,
0.0734086812102294));
#94372=CARTESIAN_POINT('Ctrl Pts',(0.0138295561391753,-0.0351953608940151,
0.0734273970791384));
#94373=CARTESIAN_POINT('Origin',(0.018706873236719,-0.0352456003065015,
0.0729780648421797));
#94374=CARTESIAN_POINT('Ctrl Pts',(0.0138424333923555,-0.0350241211493338,
0.0735514111580519));
#94375=CARTESIAN_POINT('Ctrl Pts',(0.0138506787078506,-0.0349144232867421,
0.0736301832300313));
#94376=CARTESIAN_POINT('Ctrl Pts',(0.0138573006836223,-0.0348045283677512,
0.0737091728874461));
#94377=CARTESIAN_POINT('Ctrl Pts',(0.0138622870727791,-0.0346945769586886,
0.0737882792702225));
#94378=CARTESIAN_POINT('Ctrl Pts',(0.0139156601524725,-0.0350241211493338,
0.0734649300421613));
#94379=CARTESIAN_POINT('Ctrl Pts',(0.0139250967098266,-0.0349144232867421,
0.0735447107826918));
#94380=CARTESIAN_POINT('Ctrl Pts',(0.0139328897905743,-0.0348045283677512,
0.0736247343362135));
#94381=CARTESIAN_POINT('Ctrl Pts',(0.0139390255985074,-0.0346945769586886,
0.0737048985741835));
#94382=CARTESIAN_POINT('Ctrl Pts',(0.0139888869125895,-0.0350241211493338,
0.0733784489262708));
#94383=CARTESIAN_POINT('Ctrl Pts',(0.0139995147118027,-0.0349144232867421,
0.0734592383353522));
#94384=CARTESIAN_POINT('Ctrl Pts',(0.0140084788975263,-0.0348045283677512,
0.073540295784981));
#94385=CARTESIAN_POINT('Ctrl Pts',(0.0140157641242358,-0.0346945769586886,
0.0736215178781444));
#94386=CARTESIAN_POINT('Ctrl Pts',(0.0140621136727065,-0.0350241211493338,
0.0732919678103802));
#94387=CARTESIAN_POINT('Ctrl Pts',(0.0140739327137787,-0.0349144232867421,
0.0733737658880126));
#94388=CARTESIAN_POINT('Ctrl Pts',(0.0140840680044782,-0.0348045283677512,
0.0734558572337484));
#94389=CARTESIAN_POINT('Ctrl Pts',(0.0140925026499641,-0.0346945769586886,
0.0735381371821054));
#94390=CARTESIAN_POINT('Origin',(-0.00290359790462051,-0.0345629067941849,
0.0746646638922539));
#94391=CARTESIAN_POINT('Ctrl Pts',(0.0140459665905722,-0.035197097365154,
0.0738286688005412));
#94392=CARTESIAN_POINT('Ctrl Pts',(0.014050418198839,-0.0350869349326852,
0.0739107126390035));
#94393=CARTESIAN_POINT('Ctrl Pts',(0.0140531678488388,-0.0349764985139983,
0.073992916988095));
#94394=CARTESIAN_POINT('Ctrl Pts',(0.0140542057092152,-0.0348659306865088,
0.0740751755593631));
#94395=CARTESIAN_POINT('Ctrl Pts',(0.0139820774768958,-0.035197097365154,
0.0737769131071014));
#94396=CARTESIAN_POINT('Ctrl Pts',(0.0139872460901505,-0.0350869349326852,
0.0738580718484829));
#94397=CARTESIAN_POINT('Ctrl Pts',(0.0139907317397745,-0.0349764985139983,
0.0739394052734259));
#94398=CARTESIAN_POINT('Ctrl Pts',(0.0139925237073211,-0.0348659306865088,
0.0740208082779145));
#94399=CARTESIAN_POINT('Ctrl Pts',(0.0139181883632194,-0.035197097365154,
0.0737251574136616));
#94400=CARTESIAN_POINT('Ctrl Pts',(0.013924073981462,-0.0350869349326852,
0.0738054310579624));
#94401=CARTESIAN_POINT('Ctrl Pts',(0.0139282956307102,-0.0349764985139983,
0.0738858935587567));
#94402=CARTESIAN_POINT('Ctrl Pts',(0.0139308417054269,-0.0348659306865088,
0.0739664409964658));
#94403=CARTESIAN_POINT('Ctrl Pts',(0.0138542992495431,-0.035197097365154,
0.0736734017202218));
#94404=CARTESIAN_POINT('Ctrl Pts',(0.0138609018727735,-0.0350869349326852,
0.0737527902674419));
#94405=CARTESIAN_POINT('Ctrl Pts',(0.0138658595216458,-0.0349764985139983,
0.0738323818440876));
#94406=CARTESIAN_POINT('Ctrl Pts',(0.0138691597035328,-0.0348659306865088,
0.0739120737150172));
#94407=CARTESIAN_POINT('Origin',(-0.00288050121975449,-0.0345637187969441,
0.0741842558375359));
#94408=CARTESIAN_POINT('Ctrl Pts',(0.0138524634841713,-0.0352450361861253,
0.0736397690077748));
#94409=CARTESIAN_POINT('Ctrl Pts',(0.013871707161322,-0.0349452761023764,
0.0738558297625003));
#94410=CARTESIAN_POINT('Ctrl Pts',(0.0138746215895376,-0.0346444289983475,
0.0740727262238615));
#94411=CARTESIAN_POINT('Ctrl Pts',(0.0138248779320376,-0.0352450361861253,
0.0733912955940793));
#94412=CARTESIAN_POINT('Ctrl Pts',(0.0138534929375211,-0.0349452761023764,
0.0736063159426606));
#94413=CARTESIAN_POINT('Ctrl Pts',(0.0138658304387593,-0.0346444289983475,
0.073822880840338));
#94414=CARTESIAN_POINT('Ctrl Pts',(0.0138687346586722,-0.0345231616327822,
0.0739116684421894));
#94415=CARTESIAN_POINT('Ctrl Pts',(0.0138720197236526,-0.0344132092796975,
0.0739908545236805));
#94416=CARTESIAN_POINT('Ctrl Pts',(0.0138736667175042,-0.0343032738558973,
0.0740701044685118));
#94417=CARTESIAN_POINT('Ctrl Pts',(0.013873676130924,-0.034193496108874,
0.0741493166942968));
#94418=CARTESIAN_POINT('Ctrl Pts',(0.0139472470862997,-0.0345231616327822,
0.0738299559287879));
#94419=CARTESIAN_POINT('Ctrl Pts',(0.0139516584432353,-0.0344132092796975,
0.0739102241935573));
#94420=CARTESIAN_POINT('Ctrl Pts',(0.0139544092868232,-0.0343032738558973,
0.0739905795622917));
#94421=CARTESIAN_POINT('Ctrl Pts',(0.0139554987298771,-0.034193496108874,
0.0740709190002049));
#94422=CARTESIAN_POINT('Ctrl Pts',(0.0140257595139273,-0.0345231616327822,
0.0737482434153864));
#94423=CARTESIAN_POINT('Ctrl Pts',(0.0140312971628181,-0.0344132092796975,
0.0738295938634339));
#94424=CARTESIAN_POINT('Ctrl Pts',(0.0140351518561422,-0.0343032738558973,
0.0739110546560716));
#94425=CARTESIAN_POINT('Ctrl Pts',(0.0140373213288301,-0.034193496108874,
0.073992521306113));
#94426=CARTESIAN_POINT('Ctrl Pts',(0.0141042719415548,-0.0345231616327822,
0.0736665309019849));
#94427=CARTESIAN_POINT('Ctrl Pts',(0.0141109358824009,-0.0344132092796975,
0.0737489635333106));
#94428=CARTESIAN_POINT('Ctrl Pts',(0.0141158944254612,-0.0343032738558973,
0.0738315297498515));
#94429=CARTESIAN_POINT('Ctrl Pts',(0.0141191439277832,-0.034193496108874,
0.0739141236120211));
#94430=CARTESIAN_POINT('Origin',(-0.00291567412291486,-0.0345625596233013,
0.0746654782917601));
#94431=CARTESIAN_POINT('Ctrl Pts',(0.0141226720466942,-0.0346945769586885,
0.0742654145775485));
#94432=CARTESIAN_POINT('Ctrl Pts',(0.0141210815754795,-0.0345846629176052,
0.074348082311858));
#94433=CARTESIAN_POINT('Ctrl Pts',(0.0141177812978126,-0.0344746925050311,
0.0744307312757282));
#94434=CARTESIAN_POINT('Ctrl Pts',(0.0141127758797389,-0.0343648066253259,
0.0745132555872463));
#94435=CARTESIAN_POINT('Ctrl Pts',(0.0140392914163022,-0.0346945769586885,
0.0741886761122377));
#94436=CARTESIAN_POINT('Ctrl Pts',(0.0140387584399268,-0.0345846629176052,
0.0742701948193158));
#94437=CARTESIAN_POINT('Ctrl Pts',(0.0140365395991332,-0.0344746925050311,
0.0743517164282569));
#94438=CARTESIAN_POINT('Ctrl Pts',(0.0140326381683396,-0.0343648066253259,
0.0744331364959228));
#94439=CARTESIAN_POINT('Ctrl Pts',(0.0139559107859102,-0.0346945769586885,
0.0741119376469268));
#94440=CARTESIAN_POINT('Ctrl Pts',(0.013956435304374,-0.0345846629176052,
0.0741923073267736));
#94441=CARTESIAN_POINT('Ctrl Pts',(0.0139552979004537,-0.0344746925050311,
0.0742727015807857));
#94442=CARTESIAN_POINT('Ctrl Pts',(0.0139525004569403,-0.0343648066253259,
0.0743530174045992));
#94443=CARTESIAN_POINT('Ctrl Pts',(0.0138725301555181,-0.0346945769586885,
0.074035199181616));
#94444=CARTESIAN_POINT('Ctrl Pts',(0.0138741121688213,-0.0345846629176052,
0.0741144198342314));
#94445=CARTESIAN_POINT('Ctrl Pts',(0.0138740562017742,-0.0344746925050311,
0.0741936867333144));
#94446=CARTESIAN_POINT('Ctrl Pts',(0.0138723627455409,-0.0343648066253259,
0.0742728983132757));
#94447=CARTESIAN_POINT('Origin',(-0.00293892388889004,-0.0345626446733475,
0.0741852162475095));
#94448=CARTESIAN_POINT('Ctrl Pts',(0.013874022114592,-0.0346945769586885,
0.0740365722900838));
#94449=CARTESIAN_POINT('Ctrl Pts',(0.0138763979033902,-0.034527515336289,
0.0741570133675078));
#94450=CARTESIAN_POINT('Ctrl Pts',(0.0138749865456624,-0.0343603235965158,
0.0742775603135345));
#94451=CARTESIAN_POINT('Ctrl Pts',(0.013869797514459,-0.0341934961088739,
0.0743978566658474));
#94452=CARTESIAN_POINT('Ctrl Pts',(0.0138705474735907,-0.0346945769586885,
0.0739528109911374));
#94453=CARTESIAN_POINT('Ctrl Pts',(0.0138746776763315,-0.034527515336289,
0.0740731792908145));
#94454=CARTESIAN_POINT('Ctrl Pts',(0.0138750234751208,-0.0343603235965158,
0.0741937086149738));
#94455=CARTESIAN_POINT('Ctrl Pts',(0.0138715891453453,-0.0341934961088739,
0.0743140424761774));
#94456=CARTESIAN_POINT('Ctrl Pts',(0.0138670728325894,-0.0346945769586885,
0.073869049692191));
#94457=CARTESIAN_POINT('Ctrl Pts',(0.0138729574492728,-0.034527515336289,
0.0739893452141212));
#94458=CARTESIAN_POINT('Ctrl Pts',(0.0138750604045792,-0.0343603235965158,
0.0741098569164131));
#94459=CARTESIAN_POINT('Ctrl Pts',(0.0138733807762316,-0.0341934961088739,
0.0742302282865074));
#94460=CARTESIAN_POINT('Ctrl Pts',(0.0138635981915882,-0.0346945769586885,
0.0737852883932446));
#94461=CARTESIAN_POINT('Ctrl Pts',(0.0138712372222141,-0.034527515336289,
0.0739055111374278));
#94462=CARTESIAN_POINT('Ctrl Pts',(0.0138750973340376,-0.0343603235965158,
0.0740260052178525));
#94463=CARTESIAN_POINT('Ctrl Pts',(0.013875172407118,-0.0341934961088739,
0.0741464140968374));
#94464=CARTESIAN_POINT('Ctrl Pts',(0.0138723628632283,-0.0340223579322365,
0.0742728667542586));
#94465=CARTESIAN_POINT('Ctrl Pts',(0.0138706682102372,-0.0339125849573554,
0.0743521546746266));
#94466=CARTESIAN_POINT('Ctrl Pts',(0.0138673336723471,-0.0338030433565221,
0.0744313518049119));
#94467=CARTESIAN_POINT('Ctrl Pts',(0.0138623724918966,-0.0336938721132327,
0.0745103572433477));
#94468=CARTESIAN_POINT('Ctrl Pts',(0.0139558512654297,-0.0340223579322365,
0.0741962451742169));
#94469=CARTESIAN_POINT('Ctrl Pts',(0.0139552134238648,-0.0339125849573554,
0.0742766846173982));
#94470=CARTESIAN_POINT('Ctrl Pts',(0.0139529111209454,-0.0338030433565221,
0.0743570543348758));
#94471=CARTESIAN_POINT('Ctrl Pts',(0.0139489564118833,-0.0336938721132327,
0.0744372518083244));
#94472=CARTESIAN_POINT('Ctrl Pts',(0.0140393396676311,-0.0340223579322365,
0.0741196235941752));
#94473=CARTESIAN_POINT('Ctrl Pts',(0.0140397586374924,-0.0339125849573554,
0.0742012145601697));
#94474=CARTESIAN_POINT('Ctrl Pts',(0.0140384885695436,-0.0338030433565221,
0.0742827568648396));
#94475=CARTESIAN_POINT('Ctrl Pts',(0.01403554033187,-0.0336938721132327,
0.074364146373301));
#94476=CARTESIAN_POINT('Ctrl Pts',(0.0141228280698325,-0.0340223579322365,
0.0740430020141335));
#94477=CARTESIAN_POINT('Ctrl Pts',(0.01412430385112,-0.0339125849573554,
0.0741257445029412));
#94478=CARTESIAN_POINT('Ctrl Pts',(0.0141240660181418,-0.0338030433565221,
0.0742084593948035));
#94479=CARTESIAN_POINT('Ctrl Pts',(0.0141221242518568,-0.0336938721132327,
0.0742910409382776));
#94480=CARTESIAN_POINT('Origin',(-0.00279549184214396,-0.0345589643412495,
0.0746624620825095));
#94481=CARTESIAN_POINT('Ctrl Pts',(0.0141035876665988,-0.034193496108874,
0.0746418602437495));
#94482=CARTESIAN_POINT('Ctrl Pts',(0.0140968052051056,-0.0340836138581107,
0.0747243182201288));
#94483=CARTESIAN_POINT('Ctrl Pts',(0.014088319703164,-0.03397388966435,
0.0748065962828118));
#94484=CARTESIAN_POINT('Ctrl Pts',(0.0140781490803299,-0.0338644633294063,
0.0748885898540643));
#94485=CARTESIAN_POINT('Ctrl Pts',(0.0140251899019621,-0.034193496108874,
0.0745600375711698));
#94486=CARTESIAN_POINT('Ctrl Pts',(0.0140195357266702,-0.0340836138581107,
0.0746414144888));
#94487=CARTESIAN_POINT('Ctrl Pts',(0.0140122003397996,-0.03397388966435,
0.0747226353589618));
#94488=CARTESIAN_POINT('Ctrl Pts',(0.0140032000981974,-0.0338644633294063,
0.074803596858321));
#94489=CARTESIAN_POINT('Ctrl Pts',(0.0139467921373253,-0.034193496108874,
0.0744782148985901));
#94490=CARTESIAN_POINT('Ctrl Pts',(0.0139422662482349,-0.0340836138581107,
0.0745585107574713));
#94491=CARTESIAN_POINT('Ctrl Pts',(0.0139360809764352,-0.0339738896643499,
0.0746386744351118));
#94492=CARTESIAN_POINT('Ctrl Pts',(0.0139282511160649,-0.0338644633294062,
0.0747186038625776));
#94493=CARTESIAN_POINT('Ctrl Pts',(0.0138683943726886,-0.034193496108874,
0.0743963922260104));
#94494=CARTESIAN_POINT('Ctrl Pts',(0.0138649967697996,-0.0340836138581107,
0.0744756070261426));
#94495=CARTESIAN_POINT('Ctrl Pts',(0.0138599616130708,-0.0339738896643499,
0.0745547135112618));
#94496=CARTESIAN_POINT('Ctrl Pts',(0.0138533021339323,-0.0338644633294062,
0.0746336108668343));
#94497=CARTESIAN_POINT('Origin',(-0.0028636528235915,-0.0345610621865684,
0.0741861175733144));
#94498=CARTESIAN_POINT('Ctrl Pts',(0.0138712429114264,-0.03424362768739,
0.0743617080333678));
#94499=CARTESIAN_POINT('Ctrl Pts',(0.0138632582113186,-0.0339430054201859,
0.074578477087838));
#94500=CARTESIAN_POINT('Ctrl Pts',(0.0138389682615409,-0.0336441434784161,
0.0747940288838211));
#94501=CARTESIAN_POINT('Ctrl Pts',(0.0138750134440826,-0.03424362768739,
0.0741117364688179));
#94502=CARTESIAN_POINT('Ctrl Pts',(0.0138764565769514,-0.0339430054201859,
0.0743286477312716));
#94503=CARTESIAN_POINT('Ctrl Pts',(0.0138615569649772,-0.0336441434784161,
0.0745450514742492));
#94504=CARTESIAN_POINT('Ctrl Pts',(0.0138533043401578,-0.0335235895815127,
0.0746335832233854));
#94505=CARTESIAN_POINT('Ctrl Pts',(0.0138466468650002,-0.0334144449262718,
0.0747124613761294));
#94506=CARTESIAN_POINT('Ctrl Pts',(0.013838352177937,-0.0333049234473133,
0.0747912926118882));
#94507=CARTESIAN_POINT('Ctrl Pts',(0.0138284217543404,-0.0331951640388588,
0.0748699751689439));
#94508=CARTESIAN_POINT('Ctrl Pts',(0.0139414391131666,-0.0335235895815127,
0.0745623551792388));
#94509=CARTESIAN_POINT('Ctrl Pts',(0.0139357622322718,-0.0334144449262718,
0.0746424466806548));
#94510=CARTESIAN_POINT('Ctrl Pts',(0.013928424199185,-0.0333049234473133,
0.0747225129174156));
#94511=CARTESIAN_POINT('Ctrl Pts',(0.013919425122962,-0.0331951640388588,
0.0748024506594249));
#94512=CARTESIAN_POINT('Ctrl Pts',(0.0140295738861754,-0.0335235895815127,
0.0744911271350923));
#94513=CARTESIAN_POINT('Ctrl Pts',(0.0140248775995434,-0.0334144449262718,
0.0745724319851801));
#94514=CARTESIAN_POINT('Ctrl Pts',(0.014018496220433,-0.0333049234473133,
0.0746537332229428));
#94515=CARTESIAN_POINT('Ctrl Pts',(0.0140104284915836,-0.0331951640388588,
0.074734926149906));
#94516=CARTESIAN_POINT('Ctrl Pts',(0.0141177086591842,-0.0335235895815127,
0.0744198990909458));
#94517=CARTESIAN_POINT('Ctrl Pts',(0.014113992966815,-0.0334144449262718,
0.0745024172897054));
#94518=CARTESIAN_POINT('Ctrl Pts',(0.0141085682416809,-0.0333049234473133,
0.0745849535284701));
#94519=CARTESIAN_POINT('Ctrl Pts',(0.0141014318602052,-0.0331951640388588,
0.074667401640387));
#94520=CARTESIAN_POINT('Origin',(-0.00259490116497956,-0.0326434571769064,
0.0720300270437704));
#94521=CARTESIAN_POINT('Ctrl Pts',(0.0140622117724693,-0.033693872113241,
0.0750179139736581));
#94522=CARTESIAN_POINT('Ctrl Pts',(0.014057131583977,-0.0336474569764968,
0.0750526735725668));
#94523=CARTESIAN_POINT('Ctrl Pts',(0.0140516448385898,-0.033601104548885,
0.0750873713197049));
#94524=CARTESIAN_POINT('Ctrl Pts',(0.0140377536613498,-0.0334837508643181,
0.0751752180341624));
#94525=CARTESIAN_POINT('Ctrl Pts',(0.0140212655039169,-0.0333660264760445,
0.0752626145484553));
#94526=CARTESIAN_POINT('Ctrl Pts',(0.013842896016958,-0.033693872113241,
0.0747581628645798));
#94527=CARTESIAN_POINT('Ctrl Pts',(0.0138393362379017,-0.0336474569764968,
0.0747916387355947));
#94528=CARTESIAN_POINT('Ctrl Pts',(0.0138353848254269,-0.033601104548885,
0.0748250706411131));
#94529=CARTESIAN_POINT('Ctrl Pts',(0.0138253807579586,-0.0334837508643181,
0.0749097125357627));
#94530=CARTESIAN_POINT('Ctrl Pts',(0.0138128729688169,-0.0333660264760445,
0.074994020820685));
#94531=CARTESIAN_POINT('Ctrl Pts',(0.0138428960169673,-0.0336938721132427,
0.0747581628645958));
#94532=CARTESIAN_POINT('Ctrl Pts',(0.0138393362379113,-0.0336474569765026,
0.0747916387356076));
#94533=CARTESIAN_POINT('Ctrl Pts',(0.0138353848254369,-0.0336011045488949,
0.0748250706411231));
#94534=CARTESIAN_POINT('Ctrl Pts',(0.0138254640782245,-0.0334847282606778,
0.0749090075840775));
#94535=CARTESIAN_POINT('Ctrl Pts',(0.0138130810958987,-0.0333679869945434,
0.0749926167544268));
#94536=CARTESIAN_POINT('Ctrl Pts',(0.0138428960169581,-0.0336938721132429,
0.0747581628645785));
#94537=CARTESIAN_POINT('Ctrl Pts',(0.0138301646716942,-0.0335278710435085,
0.0748778873938714));
#94538=CARTESIAN_POINT('Ctrl Pts',(0.0138136832751773,-0.0333620469224321,
0.0749971705526756));
#94539=CARTESIAN_POINT('Ctrl Pts',(0.0137934237900076,-0.0331951640388602,
0.0751160689223398));
#94540=CARTESIAN_POINT('Ctrl Pts',(0.0138499468497317,-0.0336938721132429,
0.0746746265516333));
#94541=CARTESIAN_POINT('Ctrl Pts',(0.0138389642624143,-0.0335278710435085,
0.0747944986837998));
#94542=CARTESIAN_POINT('Ctrl Pts',(0.0138242263798471,-0.0333620469224321,
0.0749139842341458));
#94543=CARTESIAN_POINT('Ctrl Pts',(0.0138057059980629,-0.0331951640388602,
0.0750331401746792));
#94544=CARTESIAN_POINT('Ctrl Pts',(0.0138569976825054,-0.0336938721132429,
0.0745910902386881));
#94545=CARTESIAN_POINT('Ctrl Pts',(0.0138477638531344,-0.0335278710435085,
0.0747111099737282));
#94546=CARTESIAN_POINT('Ctrl Pts',(0.013834769484517,-0.0333620469224321,
0.074830797915616));
#94547=CARTESIAN_POINT('Ctrl Pts',(0.0138179882061182,-0.0331951640388602,
0.0749502114270185));
#94548=CARTESIAN_POINT('Ctrl Pts',(0.013864048515279,-0.0336938721132429,
0.0745075539257429));
#94549=CARTESIAN_POINT('Ctrl Pts',(0.0138565634438545,-0.0335278710435085,
0.0746277212636567));
#94550=CARTESIAN_POINT('Ctrl Pts',(0.0138453125891868,-0.0333620469224321,
0.0747476115970862));
#94551=CARTESIAN_POINT('Ctrl Pts',(0.0138302704141734,-0.0331951640388602,
0.0748672826793579));
#94552=CARTESIAN_POINT('Ctrl Pts',(0.0138116345242051,-0.0330240426238155,
0.074992387464048));
#94553=CARTESIAN_POINT('Ctrl Pts',(0.0138000298161896,-0.0329142774063506,
0.0750707431713147));
#94554=CARTESIAN_POINT('Ctrl Pts',(0.0137867994914587,-0.0328043479726681,
0.0751488980400283));
#94555=CARTESIAN_POINT('Ctrl Pts',(0.0137719577416961,-0.0326943950436586,
0.0752267514812079));
#94556=CARTESIAN_POINT('Ctrl Pts',(0.0139040676873957,-0.0330240426238155,
0.0749268340787256));
#94557=CARTESIAN_POINT('Ctrl Pts',(0.0138933660411285,-0.0329142774063506,
0.0750064631428685));
#94558=CARTESIAN_POINT('Ctrl Pts',(0.0138810129045117,-0.0328043479726681,
0.075085910672082));
#94559=CARTESIAN_POINT('Ctrl Pts',(0.0138670212998796,-0.0326943950436586,
0.0751650744523387));
#94560=CARTESIAN_POINT('Ctrl Pts',(0.0139965008505862,-0.0330240426238155,
0.0748612806934032));
#94561=CARTESIAN_POINT('Ctrl Pts',(0.0139867022660674,-0.0329142774063506,
0.0749421831144223));
#94562=CARTESIAN_POINT('Ctrl Pts',(0.0139752263175646,-0.0328043479726681,
0.0750229233041358));
#94563=CARTESIAN_POINT('Ctrl Pts',(0.0139620848580632,-0.0326943950436586,
0.0751033974234695));
#94564=CARTESIAN_POINT('Ctrl Pts',(0.0140889340137767,-0.0330240426238155,
0.0747957273080808));
#94565=CARTESIAN_POINT('Ctrl Pts',(0.0140800384910063,-0.0329142774063506,
0.0748779030859761));
#94566=CARTESIAN_POINT('Ctrl Pts',(0.0140694397306175,-0.0328043479726681,
0.0749599359361896));
#94567=CARTESIAN_POINT('Ctrl Pts',(0.0140571484162467,-0.0326943950436586,
0.0750417203946003));
#94568=CARTESIAN_POINT('Origin',(-0.00271673139515919,-0.0326396682855295,
0.0720087480918698));
#94569=CARTESIAN_POINT('Ctrl Pts',(0.0139947886795482,-0.0331951640388588,
0.0753874501348943));
#94570=CARTESIAN_POINT('Ctrl Pts',(0.0139777453072813,-0.0330855618255041,
0.0754683113722955));
#94571=CARTESIAN_POINT('Ctrl Pts',(0.013959018385129,-0.0329757224427708,
0.0755488786440608));
#94572=CARTESIAN_POINT('Ctrl Pts',(0.0139386268332751,-0.0328657862078596,
0.0756290476026461));
#94573=CARTESIAN_POINT('Ctrl Pts',(0.0139272642237848,-0.0331951640388588,
0.0752964468387195));
#94574=CARTESIAN_POINT('Ctrl Pts',(0.0139114742378245,-0.0330855618255041,
0.0753763780633434));
#94575=CARTESIAN_POINT('Ctrl Pts',(0.0138940208273019,-0.0329757224427708,
0.0754560405572507));
#94576=CARTESIAN_POINT('Ctrl Pts',(0.0138749213384255,-0.0328657862078596,
0.0755353312115142));
#94577=CARTESIAN_POINT('Ctrl Pts',(0.0138597397680214,-0.0331951640388588,
0.0752054435425447));
#94578=CARTESIAN_POINT('Ctrl Pts',(0.0138452031683678,-0.0330855618255041,
0.0752844447543914));
#94579=CARTESIAN_POINT('Ctrl Pts',(0.0138290232694748,-0.0329757224427708,
0.0753632024704407));
#94580=CARTESIAN_POINT('Ctrl Pts',(0.0138112158435759,-0.0328657862078596,
0.0754416148203823));
#94581=CARTESIAN_POINT('Ctrl Pts',(0.013792215312258,-0.0331951640388588,
0.0751144402463699));
#94582=CARTESIAN_POINT('Ctrl Pts',(0.013778932098911,-0.0330855618255041,
0.0751925114454393));
#94583=CARTESIAN_POINT('Ctrl Pts',(0.0137640257116477,-0.0329757224427708,
0.0752703643836306));
#94584=CARTESIAN_POINT('Ctrl Pts',(0.0137475103487263,-0.0328657862078596,
0.0753478984292504));
#94585=CARTESIAN_POINT('Origin',(-0.00258602221238202,-0.0326401908833295,
0.0715459436180389));
#94586=CARTESIAN_POINT('Ctrl Pts',(0.0137993766909311,-0.0332451089994434,
0.0750804580035046));
#94587=CARTESIAN_POINT('Ctrl Pts',(0.0137642838931807,-0.0329451141710259,
0.0752945165521709));
#94588=CARTESIAN_POINT('Ctrl Pts',(0.0137131670254013,-0.0326442513127503,
0.0755053236501053));
#94589=CARTESIAN_POINT('Ctrl Pts',(0.0138344503552328,-0.0332451089994434,
0.0748329305543754));
#94590=CARTESIAN_POINT('Ctrl Pts',(0.0138086932079656,-0.0329451141710259,
0.0750483119279333));
#94591=CARTESIAN_POINT('Ctrl Pts',(0.013766785828493,-0.0326442513127503,
0.0752611412921123));
#94592=CARTESIAN_POINT('Ctrl Pts',(0.0137475170171901,-0.0325229783203385,
0.0753478675534991));
#94593=CARTESIAN_POINT('Ctrl Pts',(0.0137310044394613,-0.0324130253112079,
0.075425390613655));
#94594=CARTESIAN_POINT('Ctrl Pts',(0.0137128907021329,-0.0323031222247694,
0.0755025603320442));
#94595=CARTESIAN_POINT('Ctrl Pts',(0.0136932024956666,-0.0321934096636184,
0.0755792786784837));
#94596=CARTESIAN_POINT('Ctrl Pts',(0.0138438839312293,-0.0325229783203385,
0.0752882474182422));
#94597=CARTESIAN_POINT('Ctrl Pts',(0.0138281932157462,-0.0324130253112079,
0.0753670988941766));
#94598=CARTESIAN_POINT('Ctrl Pts',(0.0138108737360257,-0.0323031222247694,
0.0754456138281399));
#94599=CARTESIAN_POINT('Ctrl Pts',(0.0137919512259454,-0.0321934096636184,
0.0755236924309236));
#94600=CARTESIAN_POINT('Ctrl Pts',(0.0139402508452684,-0.0325229783203385,
0.0752286272829853));
#94601=CARTESIAN_POINT('Ctrl Pts',(0.0139253819920311,-0.0324130253112079,
0.0753088071746981));
#94602=CARTESIAN_POINT('Ctrl Pts',(0.0139088567699185,-0.0323031222247694,
0.0753886673242356));
#94603=CARTESIAN_POINT('Ctrl Pts',(0.0138906999562241,-0.0321934096636184,
0.0754681061833634));
#94604=CARTESIAN_POINT('Ctrl Pts',(0.0140366177593076,-0.0325229783203385,
0.0751690071477284));
#94605=CARTESIAN_POINT('Ctrl Pts',(0.014022570768316,-0.0324130253112079,
0.0752505154552196));
#94606=CARTESIAN_POINT('Ctrl Pts',(0.0140068398038113,-0.0323031222247694,
0.0753317208203313));
#94607=CARTESIAN_POINT('Ctrl Pts',(0.0139894486865029,-0.0321934096636184,
0.0754125199358033));
#94608=CARTESIAN_POINT('Origin',(-0.00270841657096725,-0.0326393375178475,
0.0720106334885954));
#94609=CARTESIAN_POINT('Ctrl Pts',(0.0139055034524876,-0.0326943950436594,
0.0757536518571623));
#94610=CARTESIAN_POINT('Ctrl Pts',(0.0138834021243321,-0.0325844576448127,
0.0758333348122168));
#94611=CARTESIAN_POINT('Ctrl Pts',(0.0138596512578787,-0.0324744968375319,
0.075912566314856));
#94612=CARTESIAN_POINT('Ctrl Pts',(0.0138342826843338,-0.0323646534831894,
0.0759912452687929));
#94613=CARTESIAN_POINT('Ctrl Pts',(0.0138438264437963,-0.0326943950436594,
0.0756585883300793));
#94614=CARTESIAN_POINT('Ctrl Pts',(0.013823035269212,-0.0325844576448127,
0.075737421260359));
#94615=CARTESIAN_POINT('Ctrl Pts',(0.0138006122289575,-0.0324744968375319,
0.0758158297741897));
#94616=CARTESIAN_POINT('Ctrl Pts',(0.0137765874384064,-0.0323646534831894,
0.0758937138062798));
#94617=CARTESIAN_POINT('Ctrl Pts',(0.0137821494351051,-0.0326943950436594,
0.0755635248029962));
#94618=CARTESIAN_POINT('Ctrl Pts',(0.013762668414092,-0.0325844576448127,
0.0756415077085012));
#94619=CARTESIAN_POINT('Ctrl Pts',(0.0137415732000363,-0.0324744968375319,
0.0757190932335233));
#94620=CARTESIAN_POINT('Ctrl Pts',(0.013718892192479,-0.0323646534831894,
0.0757961823437667));
#94621=CARTESIAN_POINT('Ctrl Pts',(0.0137204724264138,-0.0326943950436594,
0.0754684612759132));
#94622=CARTESIAN_POINT('Ctrl Pts',(0.013702301558972,-0.0325844576448127,
0.0755455941566433));
#94623=CARTESIAN_POINT('Ctrl Pts',(0.0136825341711151,-0.0324744968375319,
0.075622356692857));
#94624=CARTESIAN_POINT('Ctrl Pts',(0.0136611969465517,-0.0323646534831894,
0.0756986508812536));
#94625=CARTESIAN_POINT('Origin',(-0.00262289765796629,-0.0326395579068381,
0.0715374487169558));
#94626=CARTESIAN_POINT('Ctrl Pts',(0.0137297620235459,-0.0327445246961876,
0.0754349572524908));
#94627=CARTESIAN_POINT('Ctrl Pts',(0.0136812990690111,-0.0324436878365475,
0.0756463902360544));
#94628=CARTESIAN_POINT('Ctrl Pts',(0.013617047796315,-0.0321434074463186,
0.0758535721330864));
#94629=CARTESIAN_POINT('Ctrl Pts',(0.0137803071853637,-0.0327445246961876,
0.0751901201911279));
#94630=CARTESIAN_POINT('Ctrl Pts',(0.0137410784114604,-0.0324436878365475,
0.075403459516614));
#94631=CARTESIAN_POINT('Ctrl Pts',(0.013685891492601,-0.0321434074463186,
0.0756132378960711));
#94632=CARTESIAN_POINT('Ctrl Pts',(0.0136364247615194,-0.0322357242816072,
0.0757897856301795));
#94633=CARTESIAN_POINT('Ctrl Pts',(0.0135841997159223,-0.0319819883628705,
0.0759653561463479));
#94634=CARTESIAN_POINT('Ctrl Pts',(0.0135209084566539,-0.0317295851069886,
0.0761372476180256));
#94635=CARTESIAN_POINT('Ctrl Pts',(0.013702478135558,-0.0322357242816072,
0.0755486695755957));
#94636=CARTESIAN_POINT('Ctrl Pts',(0.0136579323235833,-0.0319819883628705,
0.075726343806059));
#94637=CARTESIAN_POINT('Ctrl Pts',(0.0136021708696587,-0.0317295851069886,
0.0759008233801974));
#94638=CARTESIAN_POINT('Origin',(-0.00253071053354238,-0.0326371942645646,
0.0715616135173585));
#94639=CARTESIAN_POINT('Origin',(-0.00258860630304265,-0.0326352985525967,
0.0720372662249546));
#94640=CARTESIAN_POINT('Ctrl Pts',(0.0137934004130372,-0.0321934096636183,
0.0761135246981948));
#94641=CARTESIAN_POINT('Ctrl Pts',(0.013766321877171,-0.0320835708272303,
0.0761917131520792));
#94642=CARTESIAN_POINT('Ctrl Pts',(0.0137376409419669,-0.0319739230346346,
0.0762692958645905));
#94643=CARTESIAN_POINT('Ctrl Pts',(0.0137074019207495,-0.0318646057455575,
0.0763461763902898));
#94644=CARTESIAN_POINT('Ctrl Pts',(0.0137378141176087,-0.0321934096636183,
0.076014775882878));
#94645=CARTESIAN_POINT('Ctrl Pts',(0.0137120974048659,-0.0320835708272303,
0.0760921977584271));
#94646=CARTESIAN_POINT('Ctrl Pts',(0.0136847933671711,-0.0319739230346346,
0.0761690425201084));
#94647=CARTESIAN_POINT('Ctrl Pts',(0.013655944483743,-0.0318646057455575,
0.0762452145314387));
#94648=CARTESIAN_POINT('Ctrl Pts',(0.0136822278221801,-0.0321934096636183,
0.0759160270675611));
#94649=CARTESIAN_POINT('Ctrl Pts',(0.0136578729325607,-0.0320835708272304,
0.075992682364775));
#94650=CARTESIAN_POINT('Ctrl Pts',(0.0136319457923753,-0.0319739230346346,
0.0760687891756264));
#94651=CARTESIAN_POINT('Ctrl Pts',(0.0136044870467364,-0.0318646057455575,
0.0761442526725876));
#94652=CARTESIAN_POINT('Ctrl Pts',(0.0136266415267516,-0.0321934096636183,
0.0758172782522443));
#94653=CARTESIAN_POINT('Ctrl Pts',(0.0136036484602555,-0.0320835708272304,
0.0758931669711228));
#94654=CARTESIAN_POINT('Ctrl Pts',(0.0135790982175796,-0.0319739230346346,
0.0759685358311443));
#94655=CARTESIAN_POINT('Ctrl Pts',(0.0135530296097299,-0.0318646057455575,
0.0760432908137365));
#94656=CARTESIAN_POINT('Ctrl Pts',(0.0136621203155706,-0.0320218834582286,
0.0756984213385563));
#94657=CARTESIAN_POINT('Ctrl Pts',(0.013646004992721,-0.0319391099350591,
0.0757560620495639));
#94658=CARTESIAN_POINT('Ctrl Pts',(0.0136289993659515,-0.0318564869454882,
0.0758134161945033));
#94659=CARTESIAN_POINT('Ctrl Pts',(0.0136111197215809,-0.0317740741446483,
0.0758704431548386));
#94660=CARTESIAN_POINT('Ctrl Pts',(0.0137058275897845,-0.0320218834582286,
0.0756750439514381));
#94661=CARTESIAN_POINT('Ctrl Pts',(0.0136899555690203,-0.0319391099350591,
0.0757331395495086));
#94662=CARTESIAN_POINT('Ctrl Pts',(0.0136731859938004,-0.0318564869454882,
0.0757909521051026));
#94663=CARTESIAN_POINT('Ctrl Pts',(0.0136555350096825,-0.0317740741446483,
0.0758484406497417));
#94664=CARTESIAN_POINT('Ctrl Pts',(0.0137495348639984,-0.0320218834582286,
0.0756516665643199));
#94665=CARTESIAN_POINT('Ctrl Pts',(0.0137339061453196,-0.0319391099350591,
0.0757102170494534));
#94666=CARTESIAN_POINT('Ctrl Pts',(0.0137173726216494,-0.0318564869454882,
0.0757684880157019));
#94667=CARTESIAN_POINT('Ctrl Pts',(0.0136999502977841,-0.0317740741446483,
0.0758264381446449));
#94668=CARTESIAN_POINT('Ctrl Pts',(0.0137932421382123,-0.0320218834582286,
0.0756282891772017));
#94669=CARTESIAN_POINT('Ctrl Pts',(0.013777856721619,-0.0319391099350591,
0.0756872945493981));
#94670=CARTESIAN_POINT('Ctrl Pts',(0.0137615592494983,-0.0318564869454882,
0.0757460239263013));
#94671=CARTESIAN_POINT('Ctrl Pts',(0.0137443655858856,-0.0317740741446483,
0.075804435639548));
#94672=CARTESIAN_POINT('Origin',(0.0199740041877478,-0.0391228853390816,
0.0764851353297408));
#94673=CARTESIAN_POINT('Ctrl Pts',(0.0136801432296278,-0.0352722978779561,
0.0726630512535914));
#94674=CARTESIAN_POINT('Ctrl Pts',(0.0136846892937845,-0.0352466642097194,
0.0726813931722122));
#94675=CARTESIAN_POINT('Ctrl Pts',(0.0136893074063788,-0.035221018380829,
0.0726996998892095));
#94676=CARTESIAN_POINT('Ctrl Pts',(0.0136939982467239,-0.0351953608940152,
0.0727179719203529));
#94677=CARTESIAN_POINT('Origin',(0.0184765399799541,-0.035245600306501,
0.0716608928793427));
#94678=CARTESIAN_POINT('Ctrl Pts',(0.0137223170444343,-0.0350241211493338,
0.0728393941634325));
#94679=CARTESIAN_POINT('Ctrl Pts',(0.0137403701016496,-0.034914423286742,
0.0729165116820436));
#94680=CARTESIAN_POINT('Ctrl Pts',(0.0137568398903465,-0.0348045283677512,
0.0729940485287804));
#94681=CARTESIAN_POINT('Ctrl Pts',(0.0137717016190843,-0.0346945769586886,
0.0730719061738239));
#94682=CARTESIAN_POINT('Ctrl Pts',(0.0137841274317792,-0.0350241211493338,
0.0727444172303425));
#94683=CARTESIAN_POINT('Ctrl Pts',(0.0138034887572468,-0.034914423286742,
0.0728223861616576));
#94684=CARTESIAN_POINT('Ctrl Pts',(0.0138212499979493,-0.0348045283677512,
0.0729008019735484));
#94685=CARTESIAN_POINT('Ctrl Pts',(0.0138373846663652,-0.0346945769586886,
0.0729795650719092));
#94686=CARTESIAN_POINT('Ctrl Pts',(0.0138459378191241,-0.0350241211493338,
0.0726494402972525));
#94687=CARTESIAN_POINT('Ctrl Pts',(0.013866607412844,-0.034914423286742,
0.0727282606412716));
#94688=CARTESIAN_POINT('Ctrl Pts',(0.0138856601055521,-0.0348045283677512,
0.0728075554183163));
#94689=CARTESIAN_POINT('Ctrl Pts',(0.0139030677136461,-0.0346945769586886,
0.0728872239699945));
#94690=CARTESIAN_POINT('Ctrl Pts',(0.013907748206469,-0.0350241211493338,
0.0725544633641624));
#94691=CARTESIAN_POINT('Ctrl Pts',(0.0139297260684412,-0.034914423286742,
0.0726341351208856));
#94692=CARTESIAN_POINT('Ctrl Pts',(0.013950070213155,-0.0348045283677512,
0.0727143088630843));
#94693=CARTESIAN_POINT('Ctrl Pts',(0.013968750760927,-0.0346945769586886,
0.0727948828680799));
#94694=CARTESIAN_POINT('Origin',(-0.00275213922892978,-0.0345629067943203,
0.0760427028193072));
#94695=CARTESIAN_POINT('Ctrl Pts',(0.0139589949194522,-0.0351970973651636,
0.0730889560727202));
#94696=CARTESIAN_POINT('Ctrl Pts',(0.0139736942450957,-0.0350869349321789,
0.0731697950369309));
#94697=CARTESIAN_POINT('Ctrl Pts',(0.0139867251502219,-0.0349764985129735,
0.0732510065580329));
#94698=CARTESIAN_POINT('Ctrl Pts',(0.0139980645595221,-0.0348659306849651,
0.0733324864178842));
#94699=CARTESIAN_POINT('Ctrl Pts',(0.0138891228821058,-0.0351970973651636,
0.0730456159175887));
#94700=CARTESIAN_POINT('Ctrl Pts',(0.0139044226268623,-0.0350869349321789,
0.0731254868994152));
#94701=CARTESIAN_POINT('Ctrl Pts',(0.0139180745722991,-0.0349764985129735,
0.0732057421186485));
#94702=CARTESIAN_POINT('Ctrl Pts',(0.0139300549114613,-0.0348659306849651,
0.0732862786434255));
#94703=CARTESIAN_POINT('Ctrl Pts',(0.0138192508447593,-0.0351970973651636,
0.073002275762457));
#94704=CARTESIAN_POINT('Ctrl Pts',(0.0138351510086288,-0.0350869349321789,
0.0730811787618996));
#94705=CARTESIAN_POINT('Ctrl Pts',(0.0138494239943763,-0.0349764985129735,
0.073160477679264));
#94706=CARTESIAN_POINT('Ctrl Pts',(0.0138620452634006,-0.0348659306849651,
0.0732400708689667));
#94707=CARTESIAN_POINT('Ctrl Pts',(0.0137493788074128,-0.0351970973651636,
0.0729589356073255));
#94708=CARTESIAN_POINT('Ctrl Pts',(0.0137658793903954,-0.0350869349321789,
0.0730368706243839));
#94709=CARTESIAN_POINT('Ctrl Pts',(0.0137807734164534,-0.0349764985129735,
0.0731152132398796));
#94710=CARTESIAN_POINT('Ctrl Pts',(0.0137940356153398,-0.0348659306849651,
0.073193863094508));
#94711=CARTESIAN_POINT('Origin',(-0.00278943576368031,-0.0345637187963003,
0.075563188142377));
#94712=CARTESIAN_POINT('Ctrl Pts',(0.0137433422209968,-0.0352450361861253,
0.0729257981812789));
#94713=CARTESIAN_POINT('Ctrl Pts',(0.0137895137490415,-0.0349452761023765,
0.0731377433601362));
#94714=CARTESIAN_POINT('Ctrl Pts',(0.0138195895309711,-0.0346444289983475,
0.0733525642534035));
#94715=CARTESIAN_POINT('Ctrl Pts',(0.0136848322127879,-0.0352450361861253,
0.0726827414411143));
#94716=CARTESIAN_POINT('Ctrl Pts',(0.0137401707759761,-0.0349452761023765,
0.0728924798788579));
#94717=CARTESIAN_POINT('Ctrl Pts',(0.0137795537712344,-0.0346444289983475,
0.073105790798708));
#94718=CARTESIAN_POINT('Ctrl Pts',(0.0137935631277463,-0.0345231616327822,
0.0731935142885265));
#94719=CARTESIAN_POINT('Ctrl Pts',(0.0138067469366547,-0.0344132092796975,
0.0732716642362969));
#94720=CARTESIAN_POINT('Ctrl Pts',(0.0138183135953134,-0.0343032738558974,
0.0733500828485773));
#94721=CARTESIAN_POINT('Ctrl Pts',(0.013828250858901,-0.0341934961088741,
0.0734286692824882));
#94722=CARTESIAN_POINT('Ctrl Pts',(0.0138612151679042,-0.0345231616327822,
0.07310260588627));
#94723=CARTESIAN_POINT('Ctrl Pts',(0.0138756520211489,-0.0344132092796975,
0.0731816883221675));
#94724=CARTESIAN_POINT('Ctrl Pts',(0.0138884523717112,-0.0343032738558974,
0.0732610652926967));
#94725=CARTESIAN_POINT('Ctrl Pts',(0.0138996024257176,-0.0341934961088741,
0.073340634686725));
#94726=CARTESIAN_POINT('Ctrl Pts',(0.0139288672080621,-0.0345231616327822,
0.0730116974840134));
#94727=CARTESIAN_POINT('Ctrl Pts',(0.0139445571056432,-0.0344132092796975,
0.0730917124080381));
#94728=CARTESIAN_POINT('Ctrl Pts',(0.013958591148109,-0.0343032738558974,
0.0731720477368159));
#94729=CARTESIAN_POINT('Ctrl Pts',(0.0139709539925342,-0.0341934961088741,
0.0732526000909618));
#94730=CARTESIAN_POINT('Ctrl Pts',(0.0139965192482201,-0.0345231616327822,
0.0729207890817569));
#94731=CARTESIAN_POINT('Ctrl Pts',(0.0140134621901374,-0.0344132092796975,
0.0730017364939087));
#94732=CARTESIAN_POINT('Ctrl Pts',(0.0140287299245069,-0.0343032738558974,
0.0730830301809353));
#94733=CARTESIAN_POINT('Ctrl Pts',(0.0140423055593507,-0.0341934961088741,
0.0731645654951986));
#94734=CARTESIAN_POINT('Origin',(-0.00276401815133821,-0.0345625596232808,
0.0760450243483039));
#94735=CARTESIAN_POINT('Ctrl Pts',(0.0140898342906213,-0.0346945769586885,
0.0735126442359855));
#94736=CARTESIAN_POINT('Ctrl Pts',(0.0140986173751996,-0.0345846629176052,
0.0735948594494186));
#94737=CARTESIAN_POINT('Ctrl Pts',(0.0141057017831005,-0.0344746925050311,
0.0736772703359942));
#94738=CARTESIAN_POINT('Ctrl Pts',(0.0141110788730535,-0.0343648066253259,
0.0737597712638998));
#94739=CARTESIAN_POINT('Ctrl Pts',(0.0139974932614085,-0.0346945769586885,
0.0734469612404181));
#94740=CARTESIAN_POINT('Ctrl Pts',(0.0140071814908651,-0.0345846629176052,
0.073527903947795));
#94741=CARTESIAN_POINT('Ctrl Pts',(0.0140151975131478,-0.0344746925050311,
0.0736090608289917));
#94742=CARTESIAN_POINT('Ctrl Pts',(0.0140215314866589,-0.0343648066253259,
0.073690327854042));
#94743=CARTESIAN_POINT('Ctrl Pts',(0.0139051522321957,-0.0346945769586885,
0.0733812782448507));
#94744=CARTESIAN_POINT('Ctrl Pts',(0.0139157456065305,-0.0345846629176052,
0.0734609484461715));
#94745=CARTESIAN_POINT('Ctrl Pts',(0.0139246932431951,-0.0344746925050311,
0.0735408513219892));
#94746=CARTESIAN_POINT('Ctrl Pts',(0.0139319841002643,-0.0343648066253259,
0.0736208844441842));
#94747=CARTESIAN_POINT('Ctrl Pts',(0.0138128112029828,-0.0346945769586885,
0.0733155952492833));
#94748=CARTESIAN_POINT('Ctrl Pts',(0.013824309722196,-0.0345846629176052,
0.0733939929445479));
#94749=CARTESIAN_POINT('Ctrl Pts',(0.0138341889732425,-0.0344746925050311,
0.0734726418149867));
#94750=CARTESIAN_POINT('Ctrl Pts',(0.0138424367138697,-0.0343648066253259,
0.0735514410343263));
#94751=CARTESIAN_POINT('Origin',(-0.00284727738114501,-0.0345626446731677,
0.0755714632818768));
#94752=CARTESIAN_POINT('Ctrl Pts',(0.0138144634936381,-0.0346945769586885,
0.0733167705383256));
#94753=CARTESIAN_POINT('Ctrl Pts',(0.0138319158183195,-0.0345275153362891,
0.0734359641365878));
#94754=CARTESIAN_POINT('Ctrl Pts',(0.0138456241281108,-0.0343603235965159,
0.0735557374239671));
#94755=CARTESIAN_POINT('Ctrl Pts',(0.0138555531447897,-0.034193496108874,
0.073675735561671));
#94756=CARTESIAN_POINT('Ctrl Pts',(0.0138005181767745,-0.0346945769586885,
0.0732341052102319));
#94757=CARTESIAN_POINT('Ctrl Pts',(0.0138197019598501,-0.0345275153362891,
0.0733530067182489));
#94758=CARTESIAN_POINT('Ctrl Pts',(0.0138351513618489,-0.0343603235965159,
0.0734725422926064));
#94759=CARTESIAN_POINT('Ctrl Pts',(0.0138468259447214,-0.034193496108874,
0.0735923577210283));
#94760=CARTESIAN_POINT('Ctrl Pts',(0.0137865728599108,-0.0346945769586885,
0.0731514398821381));
#94761=CARTESIAN_POINT('Ctrl Pts',(0.0138074881013808,-0.0345275153362891,
0.0732700492999101));
#94762=CARTESIAN_POINT('Ctrl Pts',(0.013824678595587,-0.0343603235965159,
0.0733893471612458));
#94763=CARTESIAN_POINT('Ctrl Pts',(0.0138380987446531,-0.034193496108874,
0.0735089798803856));
#94764=CARTESIAN_POINT('Ctrl Pts',(0.0137726275430471,-0.0346945769586885,
0.0730687745540444));
#94765=CARTESIAN_POINT('Ctrl Pts',(0.0137952742429114,-0.0345275153362891,
0.0731870918815713));
#94766=CARTESIAN_POINT('Ctrl Pts',(0.0138142058293251,-0.0343603235965159,
0.0733061520298852));
#94767=CARTESIAN_POINT('Ctrl Pts',(0.0138293715445849,-0.034193496108874,
0.0734256020397429));
#94768=CARTESIAN_POINT('Ctrl Pts',(0.0138424328752354,-0.0340223579322365,
0.0735514097094114));
#94769=CARTESIAN_POINT('Ctrl Pts',(0.0138506889965316,-0.0339125849573554,
0.0736302848171843));
#94770=CARTESIAN_POINT('Ctrl Pts',(0.0138573067848964,-0.0338030433565221,
0.0737092753828584));
#94771=CARTESIAN_POINT('Ctrl Pts',(0.0138622867319039,-0.0336938721132328,
0.0737882796406025));
#94772=CARTESIAN_POINT('Ctrl Pts',(0.0139156597160613,-0.0340223579322365,
0.073464928442001));
#94773=CARTESIAN_POINT('Ctrl Pts',(0.0139251086395876,-0.0339125849573554,
0.0735448135388925));
#94774=CARTESIAN_POINT('Ctrl Pts',(0.0139328974875865,-0.0338030433565221,
0.0736248380722121));
#94775=CARTESIAN_POINT('Ctrl Pts',(0.0139390253712576,-0.0336938721132328,
0.0737048988211032));
#94776=CARTESIAN_POINT('Ctrl Pts',(0.0139888865568871,-0.0340223579322365,
0.0733784471745906));
#94777=CARTESIAN_POINT('Ctrl Pts',(0.0139995282826436,-0.0339125849573554,
0.0734593422606007));
#94778=CARTESIAN_POINT('Ctrl Pts',(0.0140084881902765,-0.0338030433565221,
0.0735404007615657));
#94779=CARTESIAN_POINT('Ctrl Pts',(0.0140157640106112,-0.0336938721132328,
0.0736215180016039));
#94780=CARTESIAN_POINT('Ctrl Pts',(0.0140621133977129,-0.0340223579322365,
0.0732919659071803));
#94781=CARTESIAN_POINT('Ctrl Pts',(0.0140739479256997,-0.0339125849573554,
0.073373870982309));
#94782=CARTESIAN_POINT('Ctrl Pts',(0.0140840788929665,-0.0338030433565221,
0.0734559634509193));
#94783=CARTESIAN_POINT('Ctrl Pts',(0.0140925026499649,-0.0336938721132328,
0.0735381371821046));
#94784=CARTESIAN_POINT('Origin',(-0.00264516157481752,-0.0345589643414915,
0.076026969089253));
#94785=CARTESIAN_POINT('Ctrl Pts',(0.0141180815491695,-0.034193496108874,
0.0738885134227377));
#94786=CARTESIAN_POINT('Ctrl Pts',(0.0141216872942238,-0.0340836138581107,
0.0739711712611747));
#94787=CARTESIAN_POINT('Ctrl Pts',(0.014123580878647,-0.03397388966435,
0.0740538640521549));
#94788=CARTESIAN_POINT('Ctrl Pts',(0.0141237669736284,-0.0338644633294062,
0.0741364857966549));
#94789=CARTESIAN_POINT('Ctrl Pts',(0.0140300468741901,-0.034193496108874,
0.0738171617917167));
#94790=CARTESIAN_POINT('Ctrl Pts',(0.0140346365159833,-0.0340836138581107,
0.0738986056841178));
#94791=CARTESIAN_POINT('Ctrl Pts',(0.0140375386451194,-0.03397388966435,
0.0739801054712147));
#94792=CARTESIAN_POINT('Ctrl Pts',(0.0140387565396194,-0.0338644633294062,
0.0740615565943523));
#94793=CARTESIAN_POINT('Ctrl Pts',(0.0139420121992106,-0.034193496108874,
0.0737458101606958));
#94794=CARTESIAN_POINT('Ctrl Pts',(0.0139475857377429,-0.0340836138581107,
0.0738260401070609));
#94795=CARTESIAN_POINT('Ctrl Pts',(0.0139514964115919,-0.03397388966435,
0.0739063468902746));
#94796=CARTESIAN_POINT('Ctrl Pts',(0.0139537461056104,-0.0338644633294062,
0.0739866273920497));
#94797=CARTESIAN_POINT('Ctrl Pts',(0.0138539775242311,-0.034193496108874,
0.0736744585296748));
#94798=CARTESIAN_POINT('Ctrl Pts',(0.0138605349595024,-0.0340836138581107,
0.0737534745300041));
#94799=CARTESIAN_POINT('Ctrl Pts',(0.0138654541780643,-0.03397388966435,
0.0738325883093345));
#94800=CARTESIAN_POINT('Ctrl Pts',(0.0138687356716015,-0.0338644633294062,
0.0739116981897471));
#94801=CARTESIAN_POINT('Origin',(-0.00277248688440006,-0.0345610621863777,
0.075562923534416));
#94802=CARTESIAN_POINT('Ctrl Pts',(0.0138524565193727,-0.03424362768739,
0.0736396908156799));
#94803=CARTESIAN_POINT('Ctrl Pts',(0.0138717031475436,-0.033943005420186,
0.0738557513296935));
#94804=CARTESIAN_POINT('Ctrl Pts',(0.0138746205348661,-0.0336441434784161,
0.0740726477733318));
#94805=CARTESIAN_POINT('Ctrl Pts',(0.0138248675757685,-0.03424362768739,
0.0733912177785293));
#94806=CARTESIAN_POINT('Ctrl Pts',(0.0138534855190235,-0.033943005420186,
0.0736062377583814));
#94807=CARTESIAN_POINT('Ctrl Pts',(0.0138658259758028,-0.0336441434784161,
0.0738228025097566));
#94808=CARTESIAN_POINT('Ctrl Pts',(0.0138687343957871,-0.0335235895815127,
0.073911670487762));
#94809=CARTESIAN_POINT('Ctrl Pts',(0.0138720154707506,-0.0334144449262718,
0.0739907610656007));
#94810=CARTESIAN_POINT('Ctrl Pts',(0.013873666363456,-0.0333049234473132,
0.0740700102934708));
#94811=CARTESIAN_POINT('Ctrl Pts',(0.0138736757835164,-0.0331951640388588,
0.0741493170271627));
#94812=CARTESIAN_POINT('Ctrl Pts',(0.0139472469587047,-0.0335235895815127,
0.0738299578819154));
#94813=CARTESIAN_POINT('Ctrl Pts',(0.013951652968565,-0.0334144449262718,
0.0739101293397597));
#94814=CARTESIAN_POINT('Ctrl Pts',(0.0139544077584135,-0.0333049234473132,
0.0739904839297438));
#94815=CARTESIAN_POINT('Ctrl Pts',(0.0139554984982845,-0.0331951640388588,
0.0740709192221035));
#94816=CARTESIAN_POINT('Ctrl Pts',(0.0140257595216223,-0.0335235895815127,
0.0737482452760687));
#94817=CARTESIAN_POINT('Ctrl Pts',(0.0140312904663793,-0.0334144449262718,
0.0738294976139186));
#94818=CARTESIAN_POINT('Ctrl Pts',(0.0140351491533711,-0.0333049234473132,
0.0739109575660169));
#94819=CARTESIAN_POINT('Ctrl Pts',(0.0140373212130526,-0.0331951640388588,
0.0739925214170443));
#94820=CARTESIAN_POINT('Ctrl Pts',(0.0141042720845398,-0.0335235895815127,
0.0736665326702221));
#94821=CARTESIAN_POINT('Ctrl Pts',(0.0141109279641937,-0.0334144449262718,
0.0737488658880775));
#94822=CARTESIAN_POINT('Ctrl Pts',(0.0141158905483287,-0.0333049234473132,
0.0738314312022899));
#94823=CARTESIAN_POINT('Ctrl Pts',(0.0141191439278208,-0.0331951640388588,
0.0739141236119851));
#94824=CARTESIAN_POINT('Origin',(-0.00277608421101272,-0.0326434571770578,
0.0733901509087705));
#94825=CARTESIAN_POINT('Ctrl Pts',(0.0141241639462871,-0.0336938721132403,
0.0742667876312677));
#94826=CARTESIAN_POINT('Ctrl Pts',(0.014123480349527,-0.0336474569764965,
0.0743019098568073));
#94827=CARTESIAN_POINT('Ctrl Pts',(0.0141223856496123,-0.033601104548885,
0.0743370216733863));
#94828=CARTESIAN_POINT('Ctrl Pts',(0.0141196141212349,-0.0334837508643177,
0.0744259167164236));
#94829=CARTESIAN_POINT('Ctrl Pts',(0.0141142096655867,-0.0333660264760438,
0.0745146905971841));
#94830=CARTESIAN_POINT('Ctrl Pts',(0.0138740221145919,-0.0336938721132403,
0.0740365722900783));
#94831=CARTESIAN_POINT('Ctrl Pts',(0.0138746860446174,-0.0336474569764965,
0.0740702303524711));
#94832=CARTESIAN_POINT('Ctrl Pts',(0.0138749559190331,-0.033601104548885,
0.0741038938807312));
#94833=CARTESIAN_POINT('Ctrl Pts',(0.0138756391789763,-0.0334837508643177,
0.074189122190885));
#94834=CARTESIAN_POINT('Ctrl Pts',(0.0138737966474534,-0.0333660264760438,
0.0742743333214573));
#94835=CARTESIAN_POINT('Ctrl Pts',(0.0138740221146021,-0.0336938721132427,
0.0740365722900937));
#94836=CARTESIAN_POINT('Ctrl Pts',(0.0138746860446274,-0.0336474569765026,
0.0740702303524838));
#94837=CARTESIAN_POINT('Ctrl Pts',(0.0138749559190431,-0.0336011045488949,
0.0741038938807412));
#94838=CARTESIAN_POINT('Ctrl Pts',(0.0138756334883616,-0.0334847282606778,
0.0741884123551572));
#94839=CARTESIAN_POINT('Ctrl Pts',(0.0138738271572256,-0.0333679869945434,
0.0742729142414415));
#94840=CARTESIAN_POINT('Ctrl Pts',(0.0138740221145919,-0.0336938721132428,
0.0740365722900764));
#94841=CARTESIAN_POINT('Ctrl Pts',(0.0138763966221813,-0.0335278710435084,
0.0741569484163655));
#94842=CARTESIAN_POINT('Ctrl Pts',(0.0138749953304014,-0.033362046922432,
0.0742773566585535));
#94843=CARTESIAN_POINT('Ctrl Pts',(0.0138697975144591,-0.0331951640388601,
0.0743978566658464));
#94844=CARTESIAN_POINT('Ctrl Pts',(0.0138705474732217,-0.0336938721132428,
0.073952810982239));
#94845=CARTESIAN_POINT('Ctrl Pts',(0.0138746754488243,-0.0335278710435084,
0.0740731143700208));
#94846=CARTESIAN_POINT('Ctrl Pts',(0.0138750292892522,-0.033362046922432,
0.0741935048875918));
#94847=CARTESIAN_POINT('Ctrl Pts',(0.0138715891455355,-0.0331951640388601,
0.0743140424672798));
#94848=CARTESIAN_POINT('Ctrl Pts',(0.0138670728318515,-0.0336938721132428,
0.0738690496744017));
#94849=CARTESIAN_POINT('Ctrl Pts',(0.0138729542754672,-0.0335278710435084,
0.0739892803236762));
#94850=CARTESIAN_POINT('Ctrl Pts',(0.013875063248103,-0.033362046922432,
0.0741096531166301));
#94851=CARTESIAN_POINT('Ctrl Pts',(0.013873380776612,-0.0331951640388601,
0.0742302282687132));
#94852=CARTESIAN_POINT('Ctrl Pts',(0.0138635981904812,-0.0336938721132428,
0.0737852883665644));
#94853=CARTESIAN_POINT('Ctrl Pts',(0.0138712331021102,-0.0335278710435084,
0.0739054462773315));
#94854=CARTESIAN_POINT('Ctrl Pts',(0.0138750972069538,-0.033362046922432,
0.0740258013456685));
#94855=CARTESIAN_POINT('Ctrl Pts',(0.0138751724076885,-0.0331951640388601,
0.0741464140701466));
#94856=CARTESIAN_POINT('Ctrl Pts',(0.0138723632544785,-0.0330240426238155,
0.0742728680625924));
#94857=CARTESIAN_POINT('Ctrl Pts',(0.0138706706272117,-0.0329142774063509,
0.0743520603672835));
#94858=CARTESIAN_POINT('Ctrl Pts',(0.0138673400299578,-0.0328043479726686,
0.074431257160893));
#94859=CARTESIAN_POINT('Ctrl Pts',(0.0138623729353523,-0.0326943950436594,
0.0745103568689245));
#94860=CARTESIAN_POINT('Ctrl Pts',(0.0139558515368148,-0.0330240426238155,
0.0741962466380622));
#94861=CARTESIAN_POINT('Ctrl Pts',(0.0139552144443196,-0.0329142774063509,
0.0742765890751812));
#94862=CARTESIAN_POINT('Ctrl Pts',(0.0139529161316098,-0.0328043479726686,
0.0743569583954537));
#94863=CARTESIAN_POINT('Ctrl Pts',(0.0139489567075201,-0.0326943950436594,
0.074437251558709));
#94864=CARTESIAN_POINT('Ctrl Pts',(0.0140393398191512,-0.0330240426238155,
0.0741196252135321));
#94865=CARTESIAN_POINT('Ctrl Pts',(0.0140397582614275,-0.0329142774063509,
0.0742011177830789));
#94866=CARTESIAN_POINT('Ctrl Pts',(0.0140384922332618,-0.0328043479726686,
0.0742826596300145));
#94867=CARTESIAN_POINT('Ctrl Pts',(0.014035540479688,-0.0326943950436594,
0.0743641462484936));
#94868=CARTESIAN_POINT('Ctrl Pts',(0.0141228281014876,-0.0330240426238155,
0.0740430037890019));
#94869=CARTESIAN_POINT('Ctrl Pts',(0.0141243020785354,-0.0329142774063509,
0.0741256464909766));
#94870=CARTESIAN_POINT('Ctrl Pts',(0.0141240683349138,-0.0328043479726686,
0.0742083608645752));
#94871=CARTESIAN_POINT('Ctrl Pts',(0.0141221242518558,-0.0326943950436594,
0.0742910409382782));
#94872=CARTESIAN_POINT('Origin',(-0.00289962073335013,-0.0326396682857968,
0.0733843091246045));
#94873=CARTESIAN_POINT('Ctrl Pts',(0.0141035876665988,-0.0331951640388587,
0.0746418602437495));
#94874=CARTESIAN_POINT('Ctrl Pts',(0.0140968132867663,-0.0330855618255041,
0.0747242199670989));
#94875=CARTESIAN_POINT('Ctrl Pts',(0.0140883317886784,-0.0329757224427708,
0.0748064990475701));
#94876=CARTESIAN_POINT('Ctrl Pts',(0.0140781488651125,-0.0328657862078596,
0.074888591589103));
#94877=CARTESIAN_POINT('Ctrl Pts',(0.0140251899239631,-0.0331951640388587,
0.074560037594132));
#94878=CARTESIAN_POINT('Ctrl Pts',(0.0140195424856032,-0.0330855618255041,
0.0746413175471739));
#94879=CARTESIAN_POINT('Ctrl Pts',(0.0140122110583908,-0.0329757224427708,
0.0747225393709002));
#94880=CARTESIAN_POINT('Ctrl Pts',(0.0140031999287792,-0.0328657862078596,
0.0748035985953723));
#94881=CARTESIAN_POINT('Ctrl Pts',(0.0139467921813274,-0.0331951640388588,
0.0744782149445145));
#94882=CARTESIAN_POINT('Ctrl Pts',(0.0139422716844402,-0.0330855618255041,
0.0745584151272489));
#94883=CARTESIAN_POINT('Ctrl Pts',(0.0139360903281033,-0.0329757224427708,
0.0746385796942304));
#94884=CARTESIAN_POINT('Ctrl Pts',(0.013928250992446,-0.0328657862078596,
0.0747186056016415));
#94885=CARTESIAN_POINT('Ctrl Pts',(0.0138683944386917,-0.0331951640388588,
0.0743963922948969));
#94886=CARTESIAN_POINT('Ctrl Pts',(0.0138650008832771,-0.0330855618255041,
0.0744755127073239));
#94887=CARTESIAN_POINT('Ctrl Pts',(0.0138599695978157,-0.0329757224427708,
0.0745546200175605));
#94888=CARTESIAN_POINT('Ctrl Pts',(0.0138533020561127,-0.0328657862078596,
0.0746336126079108));
#94889=CARTESIAN_POINT('Origin',(-0.00282794701289518,-0.0326401908833756,
0.0729087717974273));
#94890=CARTESIAN_POINT('Ctrl Pts',(0.0138712402433729,-0.033245108999443,
0.074361780453421));
#94891=CARTESIAN_POINT('Ctrl Pts',(0.0138632528128909,-0.0329451141710257,
0.0745785493803117));
#94892=CARTESIAN_POINT('Ctrl Pts',(0.0138389601521242,-0.0326442513127504,
0.074794100843642));
#94893=CARTESIAN_POINT('Ctrl Pts',(0.0138750139257603,-0.033245108999443,
0.074111808936401));
#94894=CARTESIAN_POINT('Ctrl Pts',(0.0138764543252901,-0.0329451141710257,
0.0743287201900515));
#94895=CARTESIAN_POINT('Ctrl Pts',(0.0138615519904318,-0.0326442513127504,
0.0745451237185043));
#94896=CARTESIAN_POINT('Ctrl Pts',(0.0138533048022358,-0.0325229783203385,
0.0746335811398438));
#94897=CARTESIAN_POINT('Ctrl Pts',(0.0138466386469197,-0.0324130253112079,
0.0747125624822765));
#94898=CARTESIAN_POINT('Ctrl Pts',(0.0138383396721593,-0.0323031222247695,
0.074791393947658));
#94899=CARTESIAN_POINT('Ctrl Pts',(0.0138284220715146,-0.0321934096636184,
0.0748699749336006));
#94900=CARTESIAN_POINT('Ctrl Pts',(0.0139414394500367,-0.0325229783203385,
0.0745623531502163));
#94901=CARTESIAN_POINT('Ctrl Pts',(0.013935755170982,-0.0324130253112079,
0.0746425494268195));
#94902=CARTESIAN_POINT('Ctrl Pts',(0.0139284127910888,-0.0323031222247695,
0.0747226159534742));
#94903=CARTESIAN_POINT('Ctrl Pts',(0.0139194253344114,-0.0321934096636184,
0.0748024505025294));
#94904=CARTESIAN_POINT('Ctrl Pts',(0.0140295740978375,-0.0325229783203385,
0.0744911251605887));
#94905=CARTESIAN_POINT('Ctrl Pts',(0.0140248716950443,-0.0324130253112079,
0.0745725363713624));
#94906=CARTESIAN_POINT('Ctrl Pts',(0.0140184859100183,-0.0323031222247695,
0.0746538379592904));
#94907=CARTESIAN_POINT('Ctrl Pts',(0.0140104285973083,-0.0321934096636184,
0.0747349260714583));
#94908=CARTESIAN_POINT('Ctrl Pts',(0.0141177087456384,-0.0325229783203385,
0.0744198971709612));
#94909=CARTESIAN_POINT('Ctrl Pts',(0.0141139882191066,-0.0324130253112079,
0.0745025233159053));
#94910=CARTESIAN_POINT('Ctrl Pts',(0.0141085590289478,-0.0323031222247695,
0.0745850599651066));
#94911=CARTESIAN_POINT('Ctrl Pts',(0.0141014318602051,-0.0321934096636184,
0.0746674016403871));
#94912=CARTESIAN_POINT('Origin',(-0.00289113517097316,-0.0326393375180434,
0.0733851375305188));
#94913=CARTESIAN_POINT('Ctrl Pts',(0.0140609037262105,-0.0326943950436593,
0.0750163647622754));
#94914=CARTESIAN_POINT('Ctrl Pts',(0.0140489635960458,-0.0325844576448127,
0.075098189424353));
#94915=CARTESIAN_POINT('Ctrl Pts',(0.0140353303526944,-0.0324744968375319,
0.0751797729358211));
#94916=CARTESIAN_POINT('Ctrl Pts',(0.0140200229056394,-0.0323646534831894,
0.0752610110080593));
#94917=CARTESIAN_POINT('Ctrl Pts',(0.0139877984399115,-0.0326943950436593,
0.0749297810184334));
#94918=CARTESIAN_POINT('Ctrl Pts',(0.0139770515960121,-0.0325844576448127,
0.0750105981526519));
#94919=CARTESIAN_POINT('Ctrl Pts',(0.0139646325607048,-0.0324744968375319,
0.075091198744073));
#94920=CARTESIAN_POINT('Ctrl Pts',(0.0139505586703879,-0.0323646534831894,
0.0751714797419927));
#94921=CARTESIAN_POINT('Ctrl Pts',(0.0139146931536124,-0.0326943950436593,
0.0748431972745913));
#94922=CARTESIAN_POINT('Ctrl Pts',(0.0139051395959784,-0.0325844576448127,
0.0749230068809507));
#94923=CARTESIAN_POINT('Ctrl Pts',(0.0138939347687152,-0.0324744968375319,
0.0750026245523248));
#94924=CARTESIAN_POINT('Ctrl Pts',(0.0138810944351364,-0.0323646534831895,
0.0750819484759261));
#94925=CARTESIAN_POINT('Ctrl Pts',(0.0138415878673133,-0.0326943950436593,
0.0747566135307493));
#94926=CARTESIAN_POINT('Ctrl Pts',(0.0138332275959447,-0.0325844576448127,
0.0748354156092496));
#94927=CARTESIAN_POINT('Ctrl Pts',(0.0138232369767255,-0.0324744968375319,
0.0749140503605767));
#94928=CARTESIAN_POINT('Ctrl Pts',(0.0138116301998849,-0.0323646534831895,
0.0749924172098595));
#94929=CARTESIAN_POINT('Origin',(-0.00286559637766498,-0.0326395579068401,
0.0729049655999673));
#94930=CARTESIAN_POINT('Ctrl Pts',(0.0138466050456045,-0.0327445246961879,
0.0747222094013116));
#94931=CARTESIAN_POINT('Ctrl Pts',(0.0138250238154535,-0.0324436878365476,
0.0749380491914477));
#94932=CARTESIAN_POINT('Ctrl Pts',(0.0137872459603246,-0.0321434074463186,
0.0751516502171071));
#94933=CARTESIAN_POINT('Ctrl Pts',(0.0138660654231273,-0.0327445246961879,
0.0744729679647352));
#94934=CARTESIAN_POINT('Ctrl Pts',(0.0138538844873328,-0.0324436878365476,
0.0746895417150006));
#94935=CARTESIAN_POINT('Ctrl Pts',(0.0138254249364414,-0.0321434074463186,
0.0749045826842691));
#94936=CARTESIAN_POINT('Ctrl Pts',(0.0137984755637037,-0.0322357242816073,
0.0750859381121221));
#94937=CARTESIAN_POINT('Ctrl Pts',(0.0137686671486999,-0.0319819883628705,
0.0752666697361679));
#94938=CARTESIAN_POINT('Ctrl Pts',(0.0137274186738825,-0.0317295851069886,
0.0754451382904304));
#94939=CARTESIAN_POINT('Ctrl Pts',(0.0138337882323735,-0.0322357242816073,
0.0748384446466904));
#94940=CARTESIAN_POINT('Ctrl Pts',(0.0138118621632564,-0.0319819883628705,
0.0750203009334345));
#94941=CARTESIAN_POINT('Ctrl Pts',(0.0137784084942689,-0.0317295851069886,
0.0752003934473449));
#94942=CARTESIAN_POINT('Origin',(-0.00277110752374236,-0.0326371942649529,
0.0729173857438345));
#94943=CARTESIAN_POINT('Origin',(-0.00276893167612555,-0.0326352985533183,
0.0733965440521899));
#94944=CARTESIAN_POINT('Ctrl Pts',(0.0139947886795484,-0.0321934096636184,
0.0753874501348944));
#94945=CARTESIAN_POINT('Ctrl Pts',(0.0139777232777782,-0.0320835708272304,
0.0754684158899265));
#94946=CARTESIAN_POINT('Ctrl Pts',(0.0139589921925425,-0.0319739230346346,
0.0755489815139276));
#94947=CARTESIAN_POINT('Ctrl Pts',(0.0139386272999234,-0.0318646057455575,
0.0756290457680276));
#94948=CARTESIAN_POINT('Ctrl Pts',(0.0139272641903278,-0.0321934096636184,
0.0752964467936291));
#94949=CARTESIAN_POINT('Ctrl Pts',(0.0139114537955573,-0.0320835708272304,
0.0753764813333295));
#94950=CARTESIAN_POINT('Ctrl Pts',(0.0138939962608192,-0.0319739230346346,
0.0754561422544462));
#94951=CARTESIAN_POINT('Ctrl Pts',(0.0138749217439407,-0.0318646057455575,
0.0755353293505604));
#94952=CARTESIAN_POINT('Ctrl Pts',(0.0138597397011072,-0.0321934096636184,
0.0752054434523638));
#94953=CARTESIAN_POINT('Ctrl Pts',(0.0138451843133365,-0.0320835708272304,
0.0752845467767324));
#94954=CARTESIAN_POINT('Ctrl Pts',(0.0138290003290959,-0.0319739230346346,
0.0753633029949647));
#94955=CARTESIAN_POINT('Ctrl Pts',(0.013811216187958,-0.0318646057455575,
0.0754416129330931));
#94956=CARTESIAN_POINT('Ctrl Pts',(0.0137922152118866,-0.0321934096636184,
0.0751144401110984));
#94957=CARTESIAN_POINT('Ctrl Pts',(0.0137789148311156,-0.0320835708272304,
0.0751926122201353));
#94958=CARTESIAN_POINT('Ctrl Pts',(0.0137640043973725,-0.0319739230346346,
0.0752704637354833));
#94959=CARTESIAN_POINT('Ctrl Pts',(0.0137475106319754,-0.0318646057455575,
0.0753478965156258));
#94960=CARTESIAN_POINT('Ctrl Pts',(0.0138125175185335,-0.0320218834582285,
0.0749920737483511));
#94961=CARTESIAN_POINT('Ctrl Pts',(0.0138037535665135,-0.0319391099350593,
0.0750512797306585));
#94962=CARTESIAN_POINT('Ctrl Pts',(0.013794070414634,-0.0318564869454885,
0.0751103129912258));
#94963=CARTESIAN_POINT('Ctrl Pts',(0.0137834791299389,-0.0317740741446489,
0.0751691311905896));
#94964=CARTESIAN_POINT('Ctrl Pts',(0.0138529501843157,-0.0320218834582285,
0.0749634027249053));
#94965=CARTESIAN_POINT('Ctrl Pts',(0.013844484628338,-0.0319391099350593,
0.0750230295135182));
#94966=CARTESIAN_POINT('Ctrl Pts',(0.0138350931207608,-0.0318564869454885,
0.0750824879849312));
#94967=CARTESIAN_POINT('Ctrl Pts',(0.0138247865451173,-0.0317740741446489,
0.0751417354701397));
#94968=CARTESIAN_POINT('Ctrl Pts',(0.0138933828500979,-0.0320218834582285,
0.0749347317014596));
#94969=CARTESIAN_POINT('Ctrl Pts',(0.0138852156901625,-0.0319391099350593,
0.0749947792963779));
#94970=CARTESIAN_POINT('Ctrl Pts',(0.0138761158268876,-0.0318564869454885,
0.0750546629786365));
#94971=CARTESIAN_POINT('Ctrl Pts',(0.0138660939602956,-0.0317740741446489,
0.0751143397496899));
#94972=CARTESIAN_POINT('Ctrl Pts',(0.01393381551588,-0.0320218834582285,
0.0749060606780138));
#94973=CARTESIAN_POINT('Ctrl Pts',(0.013925946751987,-0.0319391099350593,
0.0749665290792376));
#94974=CARTESIAN_POINT('Ctrl Pts',(0.0139171385330143,-0.0318564869454885,
0.0750268379723418));
#94975=CARTESIAN_POINT('Ctrl Pts',(0.013907401375474,-0.0317740741446489,
0.0750869440292401));
#94976=CARTESIAN_POINT('Origin',(0.0201732317095217,-0.039122885339083,
0.0749814954491545));
#94977=CARTESIAN_POINT('Ctrl Pts',(0.0134499655687186,-0.0352722978779556,
0.0719783795930296));
#94978=CARTESIAN_POINT('Ctrl Pts',(0.013456774637772,-0.0352466642097192,
0.0719960071072227));
#94979=CARTESIAN_POINT('Ctrl Pts',(0.0134636507752063,-0.0352210183808287,
0.072013590667304));
#94980=CARTESIAN_POINT('Ctrl Pts',(0.0134705947196212,-0.0351953608940151,
0.0720311306998356));
#94981=CARTESIAN_POINT('Origin',(0.0180829375484461,-0.0352456003065004,
0.0703829756227244));
#94982=CARTESIAN_POINT('Ctrl Pts',(0.013513908457505,-0.0350241211493339,
0.0721480462057737));
#94983=CARTESIAN_POINT('Ctrl Pts',(0.013541484548944,-0.0349144232867421,
0.0722222929816801));
#94984=CARTESIAN_POINT('Ctrl Pts',(0.0135675424121596,-0.0348045283677512,
0.0722971542153479));
#94985=CARTESIAN_POINT('Ctrl Pts',(0.0135920451021384,-0.0346945769586886,
0.0723725352610863));
#94986=CARTESIAN_POINT('Ctrl Pts',(0.0135633276853456,-0.0350241211493339,
0.0720460712984555));
#94987=CARTESIAN_POINT('Ctrl Pts',(0.0135923084392583,-0.0349144232867421,
0.0721209988039321));
#94988=CARTESIAN_POINT('Ctrl Pts',(0.0136197577345397,-0.0348045283677512,
0.0721965702099951));
#94989=CARTESIAN_POINT('Ctrl Pts',(0.013645636810079,-0.0346945769586886,
0.072272690027635));
#94990=CARTESIAN_POINT('Ctrl Pts',(0.0136127469131863,-0.0350241211493339,
0.0719440963911372));
#94991=CARTESIAN_POINT('Ctrl Pts',(0.0136431323295726,-0.0349144232867421,
0.0720197046261839));
#94992=CARTESIAN_POINT('Ctrl Pts',(0.0136719730569197,-0.0348045283677512,
0.0720959862046423));
#94993=CARTESIAN_POINT('Ctrl Pts',(0.0136992285180197,-0.0346945769586886,
0.0721728447941837));
#94994=CARTESIAN_POINT('Ctrl Pts',(0.0136621661410269,-0.0350241211493339,
0.071842121483819));
#94995=CARTESIAN_POINT('Ctrl Pts',(0.0136939562198869,-0.0349144232867421,
0.0719184104484358));
#94996=CARTESIAN_POINT('Ctrl Pts',(0.0137241883792998,-0.0348045283677512,
0.0719954021992895));
#94997=CARTESIAN_POINT('Ctrl Pts',(0.0137528202259604,-0.0346945769586886,
0.0720729995607325));
#94998=CARTESIAN_POINT('Origin',(-0.00242916077554619,-0.0345629067942929,
0.0773908926920414));
#94999=CARTESIAN_POINT('Ctrl Pts',(0.0137799984578508,-0.035197097365164,
0.0723659766414764));
#95000=CARTESIAN_POINT('Ctrl Pts',(0.0138047136837033,-0.0350869349321807,
0.0724443358522937));
#95001=CARTESIAN_POINT('Ctrl Pts',(0.0138278203387926,-0.0349764985129768,
0.0725232737908184));
#95002=CARTESIAN_POINT('Ctrl Pts',(0.0138492824677688,-0.0348659306849698,
0.0726026899528025));
#95003=CARTESIAN_POINT('Ctrl Pts',(0.0137052454206028,-0.035197097365164,
0.0723317355247895));
#95004=CARTESIAN_POINT('Ctrl Pts',(0.013730435010722,-0.0350869349321807,
0.072409059133584));
#95005=CARTESIAN_POINT('Ctrl Pts',(0.0137540379526281,-0.0349764985129768,
0.0724869704739755));
#95006=CARTESIAN_POINT('Ctrl Pts',(0.0137760177263077,-0.0348659306849698,
0.072565370409552));
#95007=CARTESIAN_POINT('Ctrl Pts',(0.0136304923833547,-0.035197097365164,
0.0722974944081026));
#95008=CARTESIAN_POINT('Ctrl Pts',(0.0136561563377407,-0.0350869349321807,
0.0723737824148743));
#95009=CARTESIAN_POINT('Ctrl Pts',(0.0136802555664635,-0.0349764985129768,
0.0724506671571325));
#95010=CARTESIAN_POINT('Ctrl Pts',(0.0137027529848467,-0.0348659306849698,
0.0725280508663016));
#95011=CARTESIAN_POINT('Ctrl Pts',(0.0135557393461067,-0.035197097365164,
0.0722632532914156));
#95012=CARTESIAN_POINT('Ctrl Pts',(0.0135818776647594,-0.0350869349321807,
0.0723385056961646));
#95013=CARTESIAN_POINT('Ctrl Pts',(0.013606473180299,-0.0349764985129768,
0.0724143638402896));
#95014=CARTESIAN_POINT('Ctrl Pts',(0.0136294882433856,-0.0348659306849698,
0.0724907313230511));
#95015=CARTESIAN_POINT('Origin',(-0.00252626234102887,-0.034563718796407,
0.076919833627074));
#95016=CARTESIAN_POINT('Ctrl Pts',(0.01354559713922,-0.0352450361861253,
0.0722311337487669));
#95017=CARTESIAN_POINT('Ctrl Pts',(0.0136179683655798,-0.0349452761023765,
0.0724356208496755));
#95018=CARTESIAN_POINT('Ctrl Pts',(0.0136747311881761,-0.0346444289983475,
0.0726449783210342));
#95019=CARTESIAN_POINT('Ctrl Pts',(0.0134570854127176,-0.0352450361861253,
0.0719973268321208));
#95020=CARTESIAN_POINT('Ctrl Pts',(0.0135382748114113,-0.0349452761023765,
0.0721984756585717));
#95021=CARTESIAN_POINT('Ctrl Pts',(0.0136040822073283,-0.0346444289983475,
0.0724051685599627));
#95022=CARTESIAN_POINT('Ctrl Pts',(0.0136289757645181,-0.0345231616327822,
0.0724904444859104));
#95023=CARTESIAN_POINT('Ctrl Pts',(0.0136518504008124,-0.0344132092796975,
0.0725663258285993));
#95024=CARTESIAN_POINT('Ctrl Pts',(0.0136731543111615,-0.0343032738558974,
0.0726426763999681));
#95025=CARTESIAN_POINT('Ctrl Pts',(0.013692862708334,-0.0341934961088741,
0.0727193976869967));
#95026=CARTESIAN_POINT('Ctrl Pts',(0.0136847005041198,-0.0345231616327822,
0.0723917738746085));
#95027=CARTESIAN_POINT('Ctrl Pts',(0.0137089351758738,-0.0344132092796975,
0.0724684233043786));
#95028=CARTESIAN_POINT('Ctrl Pts',(0.0137315831642355,-0.0343032738558974,
0.0725455700544596));
#95029=CARTESIAN_POINT('Ctrl Pts',(0.013752617986182,-0.0341934961088741,
0.0726231145477268));
#95030=CARTESIAN_POINT('Ctrl Pts',(0.0137404252437214,-0.0345231616327822,
0.0722931032633066));
#95031=CARTESIAN_POINT('Ctrl Pts',(0.0137660199509351,-0.0344132092796975,
0.0723705207801579));
#95032=CARTESIAN_POINT('Ctrl Pts',(0.0137900120173095,-0.0343032738558974,
0.0724484637089511));
#95033=CARTESIAN_POINT('Ctrl Pts',(0.0138123732640301,-0.0341934961088741,
0.0725268314084568));
#95034=CARTESIAN_POINT('Ctrl Pts',(0.013796149983323,-0.0345231616327822,
0.0721944326520047));
#95035=CARTESIAN_POINT('Ctrl Pts',(0.0138231047259964,-0.0344132092796975,
0.0722726182559372));
#95036=CARTESIAN_POINT('Ctrl Pts',(0.0138484408703835,-0.0343032738558974,
0.0723513573634426));
#95037=CARTESIAN_POINT('Ctrl Pts',(0.0138721285418781,-0.0341934961088741,
0.0724305482691869));
#95038=CARTESIAN_POINT('Origin',(-0.00244065506430078,-0.0345625596231532,
0.0773946847386776));
#95039=CARTESIAN_POINT('Ctrl Pts',(0.0139629083290236,-0.0346945769586885,
0.072769925375559));
#95040=CARTESIAN_POINT('Ctrl Pts',(0.0139819264548934,-0.034584662917669,
0.0728503914850401));
#95041=CARTESIAN_POINT('Ctrl Pts',(0.0139992838230083,-0.0344746925051587,
0.0729312646253629));
#95042=CARTESIAN_POINT('Ctrl Pts',(0.0140149586210603,-0.0343648066255171,
0.0730124410806917));
#95043=CARTESIAN_POINT('Ctrl Pts',(0.0138630631741826,-0.0346945769586885,
0.0727163337098122));
#95044=CARTESIAN_POINT('Ctrl Pts',(0.0138828198202937,-0.034584662917669,
0.0727954239025938));
#95045=CARTESIAN_POINT('Ctrl Pts',(0.0139009442881833,-0.0344746925051587,
0.0728749361635026));
#95046=CARTESIAN_POINT('Ctrl Pts',(0.0139174137754455,-0.0343648066255171,
0.0729547685163588));
#95047=CARTESIAN_POINT('Ctrl Pts',(0.0137632180193416,-0.0346945769586885,
0.0726627420440654));
#95048=CARTESIAN_POINT('Ctrl Pts',(0.0137837131856941,-0.034584662917669,
0.0727404563201476));
#95049=CARTESIAN_POINT('Ctrl Pts',(0.0138026047533584,-0.0344746925051587,
0.0728186077016422));
#95050=CARTESIAN_POINT('Ctrl Pts',(0.0138198689298307,-0.0343648066255171,
0.072897095952026));
#95051=CARTESIAN_POINT('Ctrl Pts',(0.0136633728645006,-0.0346945769586885,
0.0726091503783186));
#95052=CARTESIAN_POINT('Ctrl Pts',(0.0136846065510945,-0.034584662917669,
0.0726854887377014));
#95053=CARTESIAN_POINT('Ctrl Pts',(0.0137042652185335,-0.0344746925051587,
0.0727622792397819));
#95054=CARTESIAN_POINT('Ctrl Pts',(0.0137223240842159,-0.0343648066255171,
0.0728394233876932));
#95055=CARTESIAN_POINT('Origin',(-0.00258261070982406,-0.0345626446731565,
0.0769352929913375));
#95056=CARTESIAN_POINT('Ctrl Pts',(0.0136651594291266,-0.0346945769586886,
0.0726101093129251));
#95057=CARTESIAN_POINT('Ctrl Pts',(0.0136974130561055,-0.0345275153362891,
0.0727261756777781));
#95058=CARTESIAN_POINT('Ctrl Pts',(0.0137260248451815,-0.0343603235965159,
0.072843286410219));
#95059=CARTESIAN_POINT('Ctrl Pts',(0.0137509153232183,-0.034193496108874,
0.072961093890999));
#95060=CARTESIAN_POINT('Ctrl Pts',(0.013640963362378,-0.0346945769586886,
0.07252984363729));
#95061=CARTESIAN_POINT('Ctrl Pts',(0.0136748981860697,-0.0345275153362891,
0.0726454032058373));
#95062=CARTESIAN_POINT('Ctrl Pts',(0.0137052075449794,-0.0343603235965159,
0.0727620598829783));
#95063=CARTESIAN_POINT('Ctrl Pts',(0.0137318069253539,-0.034193496108874,
0.072879467317738));
#95064=CARTESIAN_POINT('Ctrl Pts',(0.0136167672956295,-0.0346945769586886,
0.0724495779616548));
#95065=CARTESIAN_POINT('Ctrl Pts',(0.0136523833160339,-0.0345275153362891,
0.0725646307338965));
#95066=CARTESIAN_POINT('Ctrl Pts',(0.0136843902447773,-0.0343603235965159,
0.0726808333557376));
#95067=CARTESIAN_POINT('Ctrl Pts',(0.0137126985274895,-0.034193496108874,
0.0727978407444771));
#95068=CARTESIAN_POINT('Ctrl Pts',(0.0135925712288809,-0.0346945769586886,
0.0723693122860197));
#95069=CARTESIAN_POINT('Ctrl Pts',(0.0136298684459981,-0.0345275153362891,
0.0724838582619558));
#95070=CARTESIAN_POINT('Ctrl Pts',(0.0136635729445752,-0.0343603235965159,
0.0725996068284969));
#95071=CARTESIAN_POINT('Ctrl Pts',(0.0136935901296251,-0.034193496108874,
0.0727162141712161));
#95072=CARTESIAN_POINT('Ctrl Pts',(0.013722316349829,-0.0340223579322365,
0.0728393927910273));
#95073=CARTESIAN_POINT('Ctrl Pts',(0.0137403930414476,-0.0339125849573554,
0.0729166111786378));
#95074=CARTESIAN_POINT('Ctrl Pts',(0.0137568587895916,-0.0338030433565221,
0.0729941494512934));
#95075=CARTESIAN_POINT('Ctrl Pts',(0.0137717013273179,-0.0336938721132327,
0.0730719065840064));
#95076=CARTESIAN_POINT('Ctrl Pts',(0.0137841267982558,-0.0340223579322365,
0.0727444156974968));
#95077=CARTESIAN_POINT('Ctrl Pts',(0.0138035134717049,-0.0339125849573554,
0.0728224866123995));
#95078=CARTESIAN_POINT('Ctrl Pts',(0.0138212706358363,-0.0338030433565221,
0.0729009039268662));
#95079=CARTESIAN_POINT('Ctrl Pts',(0.0138373844718545,-0.0336938721132327,
0.0729795653453639));
#95080=CARTESIAN_POINT('Ctrl Pts',(0.0138459372466827,-0.0340223579322365,
0.0726494386039662));
#95081=CARTESIAN_POINT('Ctrl Pts',(0.0138666339019622,-0.0339125849573554,
0.0727283620461611));
#95082=CARTESIAN_POINT('Ctrl Pts',(0.013885682482081,-0.0338030433565221,
0.0728076584024389));
#95083=CARTESIAN_POINT('Ctrl Pts',(0.013903067616391,-0.0336938721132327,
0.0728872241067214));
#95084=CARTESIAN_POINT('Ctrl Pts',(0.0139077476951095,-0.0340223579322365,
0.0725544615104357));
#95085=CARTESIAN_POINT('Ctrl Pts',(0.0139297543322195,-0.0339125849573554,
0.0726342374799228));
#95086=CARTESIAN_POINT('Ctrl Pts',(0.0139500943283257,-0.0338030433565221,
0.0727144128780116));
#95087=CARTESIAN_POINT('Ctrl Pts',(0.0139687507609276,-0.0336938721132327,
0.0727948828680789));
#95088=CARTESIAN_POINT('Origin',(-0.00232499863165299,-0.0345589643413838,
0.0773618751717664));
#95089=CARTESIAN_POINT('Ctrl Pts',(0.0140380417500741,-0.034193496108874,
0.0731392904012537));
#95090=CARTESIAN_POINT('Ctrl Pts',(0.0140519788368658,-0.0340836138585568,
0.0732208445379278));
#95091=CARTESIAN_POINT('Ctrl Pts',(0.0140642216446534,-0.033973889665241,
0.07330264794216));
#95092=CARTESIAN_POINT('Ctrl Pts',(0.0140747615225922,-0.0338644633307392,
0.073384594865307));
#95093=CARTESIAN_POINT('Ctrl Pts',(0.0139417585241658,-0.034193496108874,
0.0730795350696361));
#95094=CARTESIAN_POINT('Ctrl Pts',(0.0139565196015914,-0.0340836138585568,
0.0731597615176469));
#95095=CARTESIAN_POINT('Ctrl Pts',(0.0139696134783777,-0.033973889665241,
0.0732402549210231));
#95096=CARTESIAN_POINT('Ctrl Pts',(0.0139810303020233,-0.0338644633307392,
0.0733209111347417));
#95097=CARTESIAN_POINT('Ctrl Pts',(0.0138454752982574,-0.034193496108874,
0.0730197797380186));
#95098=CARTESIAN_POINT('Ctrl Pts',(0.013861060366317,-0.0340836138585568,
0.0730986784973661));
#95099=CARTESIAN_POINT('Ctrl Pts',(0.013875005312102,-0.033973889665241,
0.0731778618998861));
#95100=CARTESIAN_POINT('Ctrl Pts',(0.0138872990814544,-0.0338644633307392,
0.0732572274041764));
#95101=CARTESIAN_POINT('Ctrl Pts',(0.0137491920723491,-0.034193496108874,
0.072960024406401));
#95102=CARTESIAN_POINT('Ctrl Pts',(0.0137656011310426,-0.0340836138585568,
0.0730375954770853));
#95103=CARTESIAN_POINT('Ctrl Pts',(0.0137803971458263,-0.033973889665241,
0.0731154688787492));
#95104=CARTESIAN_POINT('Ctrl Pts',(0.0137935678608855,-0.0338644633307392,
0.0731935436736112));
#95105=CARTESIAN_POINT('Origin',(-0.00250948027280974,-0.0345610621864204,
0.0769174468476583));
#95106=CARTESIAN_POINT('Ctrl Pts',(0.0137433255110496,-0.0342436276873901,
0.0729257214786727));
#95107=CARTESIAN_POINT('Ctrl Pts',(0.0137894999366756,-0.0339430054201861,
0.0731376660488551));
#95108=CARTESIAN_POINT('Ctrl Pts',(0.0138195786521574,-0.0336441434784163,
0.0733524865536648));
#95109=CARTESIAN_POINT('Ctrl Pts',(0.0136848121853066,-0.0342436276873901,
0.072682665537148));
#95110=CARTESIAN_POINT('Ctrl Pts',(0.013740153616887,-0.0339430054201861,
0.0728924032408694));
#95111=CARTESIAN_POINT('Ctrl Pts',(0.0137795395260446,-0.0336441434784163,
0.0731057136451434));
#95112=CARTESIAN_POINT('Ctrl Pts',(0.0137935631233125,-0.0335235895815127,
0.0731935163509172));
#95113=CARTESIAN_POINT('Ctrl Pts',(0.0138067310038849,-0.0334144449262719,
0.0732715720481918));
#95114=CARTESIAN_POINT('Ctrl Pts',(0.0138183014407946,-0.0333049234473133,
0.0733499894605085));
#95115=CARTESIAN_POINT('Ctrl Pts',(0.0138282505559521,-0.0331951640388588,
0.0734286696562709));
#95116=CARTESIAN_POINT('Ctrl Pts',(0.0138612152860968,-0.0335235895815127,
0.0731026078400021));
#95117=CARTESIAN_POINT('Ctrl Pts',(0.0138756347013044,-0.0334144449262719,
0.0731815949024922));
#95118=CARTESIAN_POINT('Ctrl Pts',(0.0138884388694064,-0.0333049234473133,
0.073260970605814));
#95119=CARTESIAN_POINT('Ctrl Pts',(0.0138996022237517,-0.0331951640388588,
0.0733406349359134));
#95120=CARTESIAN_POINT('Ctrl Pts',(0.0139288674488812,-0.0335235895815127,
0.0730116993290869));
#95121=CARTESIAN_POINT('Ctrl Pts',(0.0139445383987239,-0.0334144449262719,
0.0730916177567926));
#95122=CARTESIAN_POINT('Ctrl Pts',(0.0139585762980183,-0.0333049234473133,
0.0731719517511194));
#95123=CARTESIAN_POINT('Ctrl Pts',(0.0139709538915513,-0.0331951640388588,
0.0732526002155559));
#95124=CARTESIAN_POINT('Ctrl Pts',(0.0139965196116655,-0.0335235895815127,
0.0729207908181717));
#95125=CARTESIAN_POINT('Ctrl Pts',(0.0140134420961433,-0.0334144449262719,
0.073001640611093));
#95126=CARTESIAN_POINT('Ctrl Pts',(0.0140287137266301,-0.0333049234473133,
0.0730829328964249));
#95127=CARTESIAN_POINT('Ctrl Pts',(0.0140423055593509,-0.0331951640388588,
0.0731645654951985));
#95128=CARTESIAN_POINT('Origin',(-0.0027853698522513,-0.0326434571771509,
0.0747622580477667));
#95129=CARTESIAN_POINT('Ctrl Pts',(0.0140914865154029,-0.0336938721132395,
0.0735138194781665));
#95130=CARTESIAN_POINT('Ctrl Pts',(0.0140952102911043,-0.0336474569764961,
0.0735487504318593));
#95131=CARTESIAN_POINT('Ctrl Pts',(0.0140985249007336,-0.033601104548885,
0.0735837225835572));
#95132=CARTESIAN_POINT('Ctrl Pts',(0.0141069167297378,-0.0334837508662626,
0.0736722640257744));
#95133=CARTESIAN_POINT('Ctrl Pts',(0.0141126812073164,-0.0333660264799449,
0.073761015254398));
#95134=CARTESIAN_POINT('Ctrl Pts',(0.0138144634936374,-0.0336938721132395,
0.0733167705383206));
#95135=CARTESIAN_POINT('Ctrl Pts',(0.0138193406621715,-0.0336474569764961,
0.0733500799843411));
#95136=CARTESIAN_POINT('Ctrl Pts',(0.0138238275673968,-0.033601104548885,
0.0733834442413926));
#95137=CARTESIAN_POINT('Ctrl Pts',(0.0138351873791458,-0.0334837508662626,
0.0734679148642864));
#95138=CARTESIAN_POINT('Ctrl Pts',(0.0138440391629595,-0.0333660264799449,
0.0735526850086673));
#95139=CARTESIAN_POINT('Ctrl Pts',(0.0138144634936481,-0.0336938721132427,
0.0733167705383356));
#95140=CARTESIAN_POINT('Ctrl Pts',(0.0138193406621818,-0.0336474569765026,
0.0733500799843536));
#95141=CARTESIAN_POINT('Ctrl Pts',(0.0138238275674068,-0.0336011045488949,
0.0733834442414026));
#95142=CARTESIAN_POINT('Ctrl Pts',(0.0138350927673962,-0.0334847282626114,
0.0734672113390579));
#95143=CARTESIAN_POINT('Ctrl Pts',(0.0138438915742658,-0.0333679869984219,
0.0735512732946507));
#95144=CARTESIAN_POINT('Ctrl Pts',(0.0138144634936371,-0.0336938721132428,
0.0733167705383183));
#95145=CARTESIAN_POINT('Ctrl Pts',(0.0138319064066766,-0.0335278710435084,
0.0734358998581826));
#95146=CARTESIAN_POINT('Ctrl Pts',(0.0138456073188421,-0.0333620469224321,
0.0735555342738467));
#95147=CARTESIAN_POINT('Ctrl Pts',(0.0138555531447896,-0.0331951640388602,
0.07367573556167));
#95148=CARTESIAN_POINT('Ctrl Pts',(0.013800518175293,-0.0336938721132428,
0.07323410520145));
#95149=CARTESIAN_POINT('Ctrl Pts',(0.0138196916131744,-0.0335278710435084,
0.0733529425885558));
#95150=CARTESIAN_POINT('Ctrl Pts',(0.0138351315963226,-0.0333620469224321,
0.0734723394429718));
#95151=CARTESIAN_POINT('Ctrl Pts',(0.013846825943795,-0.0331951640388602,
0.073592357712177));
#95152=CARTESIAN_POINT('Ctrl Pts',(0.013786572856949,-0.0336938721132428,
0.0731514398645816));
#95153=CARTESIAN_POINT('Ctrl Pts',(0.0138074768196722,-0.0335278710435084,
0.0732699853189289));
#95154=CARTESIAN_POINT('Ctrl Pts',(0.013824655873803,-0.0333620469224321,
0.0733891446120969));
#95155=CARTESIAN_POINT('Ctrl Pts',(0.0138380987428003,-0.0331951640388602,
0.073508979862684));
#95156=CARTESIAN_POINT('Ctrl Pts',(0.013772627538605,-0.0336938721132428,
0.0730687745277132));
#95157=CARTESIAN_POINT('Ctrl Pts',(0.01379526202617,-0.0335278710435084,
0.0731870280493021));
#95158=CARTESIAN_POINT('Ctrl Pts',(0.0138141801512834,-0.0333620469224321,
0.073305949781222));
#95159=CARTESIAN_POINT('Ctrl Pts',(0.0138293715418057,-0.0331951640388602,
0.073425602013191));
#95160=CARTESIAN_POINT('Ctrl Pts',(0.0138424334273781,-0.0330240426238155,
0.073551410958392));
#95161=CARTESIAN_POINT('Ctrl Pts',(0.0138506795746033,-0.0329142774063509,
0.0736301909505556));
#95162=CARTESIAN_POINT('Ctrl Pts',(0.0138573012303345,-0.0328043479726686,
0.0737091806883161));
#95163=CARTESIAN_POINT('Ctrl Pts',(0.0138622871249351,-0.0326943950436594,
0.0737882792135521));
#95164=CARTESIAN_POINT('Ctrl Pts',(0.0139156601687748,-0.0330240426238155,
0.07346492986029));
#95165=CARTESIAN_POINT('Ctrl Pts',(0.0139250976773808,-0.0329142774063509,
0.0735447186221577));
#95166=CARTESIAN_POINT('Ctrl Pts',(0.0139328904343422,-0.0328043479726686,
0.0736247422612984));
#95167=CARTESIAN_POINT('Ctrl Pts',(0.0139390256332781,-0.0326943950436594,
0.0737048985364033));
#95168=CARTESIAN_POINT('Ctrl Pts',(0.0139888869101716,-0.0330240426238155,
0.0733784487621881));
#95169=CARTESIAN_POINT('Ctrl Pts',(0.0139995157801583,-0.0329142774063509,
0.0734592462937599));
#95170=CARTESIAN_POINT('Ctrl Pts',(0.01400847963835,-0.0328043479726686,
0.0735403038342808));
#95171=CARTESIAN_POINT('Ctrl Pts',(0.014015764141621,-0.0326943950436594,
0.0736215178592544));
#95172=CARTESIAN_POINT('Ctrl Pts',(0.0140621136515683,-0.0330240426238155,
0.0732919676640861));
#95173=CARTESIAN_POINT('Ctrl Pts',(0.0140739338829358,-0.0329142774063509,
0.073373773965362));
#95174=CARTESIAN_POINT('Ctrl Pts',(0.0140840688423578,-0.0328043479726686,
0.0734558654072631));
#95175=CARTESIAN_POINT('Ctrl Pts',(0.014092502649964,-0.0326943950436594,
0.0735381371821056));
#95176=CARTESIAN_POINT('Origin',(-0.00290866442199188,-0.03263966828572,
0.0747719455594014));
#95177=CARTESIAN_POINT('Ctrl Pts',(0.0141180815491696,-0.0331951640388587,
0.0738885134227377));
#95178=CARTESIAN_POINT('Ctrl Pts',(0.0141216829976228,-0.0330855618305429,
0.073971072766203));
#95179=CARTESIAN_POINT('Ctrl Pts',(0.0141235806818819,-0.0329757224528702,
0.0740537660613222));
#95180=CARTESIAN_POINT('Ctrl Pts',(0.0141237669775404,-0.0328657862230221,
0.0741364875335773));
#95181=CARTESIAN_POINT('Ctrl Pts',(0.0140300468988956,-0.0331951640388587,
0.0738171618117404));
#95182=CARTESIAN_POINT('Ctrl Pts',(0.0140346310714019,-0.0330855618305429,
0.0738985086560466));
#95183=CARTESIAN_POINT('Ctrl Pts',(0.0140375372484301,-0.0329757224528702,
0.0739800088891584));
#95184=CARTESIAN_POINT('Ctrl Pts',(0.0140387565890793,-0.0328657862230221,
0.0740615583276929));
#95185=CARTESIAN_POINT('Ctrl Pts',(0.0139420122486216,-0.0331951640388587,
0.0737458102007431));
#95186=CARTESIAN_POINT('Ctrl Pts',(0.0139475791451811,-0.0330855618305429,
0.0738259445458902));
#95187=CARTESIAN_POINT('Ctrl Pts',(0.0139514938149783,-0.0329757224528702,
0.0739062517169946));
#95188=CARTESIAN_POINT('Ctrl Pts',(0.0139537462006182,-0.0328657862230221,
0.0739866291218084));
#95189=CARTESIAN_POINT('Ctrl Pts',(0.0138539775983476,-0.0331951640388587,
0.0736744585897458));
#95190=CARTESIAN_POINT('Ctrl Pts',(0.0138605272189603,-0.0330855618305429,
0.0737533804357337));
#95191=CARTESIAN_POINT('Ctrl Pts',(0.0138654503815266,-0.0329757224528702,
0.0738324945448307));
#95192=CARTESIAN_POINT('Ctrl Pts',(0.0138687358121571,-0.0328657862230221,
0.073911699915924));
#95193=CARTESIAN_POINT('Origin',(-0.00289715649951292,-0.0326401908835659,
0.0742911748872013));
#95194=CARTESIAN_POINT('Ctrl Pts',(0.013852462948997,-0.0332451089994432,
0.0736397629990749));
#95195=CARTESIAN_POINT('Ctrl Pts',(0.0138717068523336,-0.0329451141710258,
0.0738558237287217));
#95196=CARTESIAN_POINT('Ctrl Pts',(0.0138746215083516,-0.0326442513127503,
0.0740727201821075));
#95197=CARTESIAN_POINT('Ctrl Pts',(0.0138248771362445,-0.0332451089994432,
0.0733912896143136));
#95198=CARTESIAN_POINT('Ctrl Pts',(0.0138534923666103,-0.0329451141710258,
0.0736063099280102));
#95199=CARTESIAN_POINT('Ctrl Pts',(0.0138658300950892,-0.0326442513127503,
0.0738228748078201));
#95200=CARTESIAN_POINT('Ctrl Pts',(0.0138687345930848,-0.0325229783203384,
0.0739116683627356));
#95201=CARTESIAN_POINT('Ctrl Pts',(0.0138720199894327,-0.0324130253112079,
0.073990862404494));
#95202=CARTESIAN_POINT('Ctrl Pts',(0.01387366665703,-0.0323031222247695,
0.0740701123975671));
#95203=CARTESIAN_POINT('Ctrl Pts',(0.0138736760686934,-0.0321934096636184,
0.0741493167539226));
#95204=CARTESIAN_POINT('Ctrl Pts',(0.0139472470386026,-0.0325229783203384,
0.0738299558266834));
#95205=CARTESIAN_POINT('Ctrl Pts',(0.0139516588404526,-0.0324130253112079,
0.0739102321607666));
#95206=CARTESIAN_POINT('Ctrl Pts',(0.0139544093541039,-0.0323031222247695,
0.073990587583158));
#95207=CARTESIAN_POINT('Ctrl Pts',(0.01395549868839,-0.0321934096636184,
0.0740709190399554));
#95208=CARTESIAN_POINT('Ctrl Pts',(0.0140257594841205,-0.0325229783203384,
0.0737482432906312));
#95209=CARTESIAN_POINT('Ctrl Pts',(0.0140312976914725,-0.0324130253112079,
0.0738296019170392));
#95210=CARTESIAN_POINT('Ctrl Pts',(0.0140351520511777,-0.0323031222247695,
0.0739110627687489));
#95211=CARTESIAN_POINT('Ctrl Pts',(0.0140373213080865,-0.0321934096636184,
0.0739925213259883));
#95212=CARTESIAN_POINT('Ctrl Pts',(0.0141042719296383,-0.0325229783203384,
0.073666530754579));
#95213=CARTESIAN_POINT('Ctrl Pts',(0.0141109365424923,-0.0324130253112079,
0.0737489716733118));
#95214=CARTESIAN_POINT('Ctrl Pts',(0.0141158947482515,-0.0323031222247695,
0.0738315379543398));
#95215=CARTESIAN_POINT('Ctrl Pts',(0.0141191439277831,-0.0321934096636184,
0.0739141236120212));
#95216=CARTESIAN_POINT('Origin',(-0.0029001419440751,-0.0326393375178958,
0.0747717039100236));
#95217=CARTESIAN_POINT('Ctrl Pts',(0.0141226720466918,-0.0326943950436593,
0.0742654145775462));
#95218=CARTESIAN_POINT('Ctrl Pts',(0.0141210814175033,-0.0325844576448127,
0.0743480905228462));
#95219=CARTESIAN_POINT('Ctrl Pts',(0.0141177808016456,-0.0324744968375319,
0.0744307394224318));
#95220=CARTESIAN_POINT('Ctrl Pts',(0.0141127758886649,-0.0323646534831895,
0.0745132554400428));
#95221=CARTESIAN_POINT('Ctrl Pts',(0.014039291396821,-0.0326943950436593,
0.0741886760943082));
#95222=CARTESIAN_POINT('Ctrl Pts',(0.0140387583677547,-0.0325844576448127,
0.074270202897981));
#95223=CARTESIAN_POINT('Ctrl Pts',(0.0140365391930001,-0.0324744968375319,
0.0743517244475174));
#95224=CARTESIAN_POINT('Ctrl Pts',(0.0140326381565751,-0.0323646534831895,
0.074433136331972));
#95225=CARTESIAN_POINT('Ctrl Pts',(0.0139559107469501,-0.0326943950436593,
0.0741119376110703));
#95226=CARTESIAN_POINT('Ctrl Pts',(0.0139564353180061,-0.0325844576448127,
0.0741923152731158));
#95227=CARTESIAN_POINT('Ctrl Pts',(0.0139552975843547,-0.0324744968375319,
0.0742727094726029));
#95228=CARTESIAN_POINT('Ctrl Pts',(0.0139525004244853,-0.0323646534831895,
0.0743530172239012));
#95229=CARTESIAN_POINT('Ctrl Pts',(0.0138725300970792,-0.0326943950436593,
0.0740351991278323));
#95230=CARTESIAN_POINT('Ctrl Pts',(0.0138741122682574,-0.0325844576448127,
0.0741144276482506));
#95231=CARTESIAN_POINT('Ctrl Pts',(0.0138740559757092,-0.0324744968375319,
0.0741936944976885));
#95232=CARTESIAN_POINT('Ctrl Pts',(0.0138723626923955,-0.0323646534831895,
0.0742728981158304));
#95233=CARTESIAN_POINT('Origin',(-0.00293498603248267,-0.0326395579068033,
0.0742921174191728));
#95234=CARTESIAN_POINT('Ctrl Pts',(0.0138731957326305,-0.0327445246961876,
0.0740004374660528));
#95235=CARTESIAN_POINT('Ctrl Pts',(0.0138788365757548,-0.0324436878365475,
0.0742172801403344));
#95236=CARTESIAN_POINT('Ctrl Pts',(0.0138681279175358,-0.0321434074463188,
0.0744339316788471));
#95237=CARTESIAN_POINT('Ctrl Pts',(0.0138612644240796,-0.0327445246961876,
0.0737507223406073));
#95238=CARTESIAN_POINT('Ctrl Pts',(0.0138763234270281,-0.0324436878365475,
0.0739671150182352));
#95239=CARTESIAN_POINT('Ctrl Pts',(0.0138750400682232,-0.0321434074463188,
0.0741840272527702));
#95240=CARTESIAN_POINT('Ctrl Pts',(0.0138710330615361,-0.0322357242816074,
0.0743673302909342));
#95241=CARTESIAN_POINT('Ctrl Pts',(0.0138641113736369,-0.0319819883628706,
0.0745503727771823));
#95242=CARTESIAN_POINT('Ctrl Pts',(0.013845556196359,-0.0317295851069885,
0.074732603858317));
#95243=CARTESIAN_POINT('Ctrl Pts',(0.0138750481229576,-0.0322357242816074,
0.0741173625344499));
#95244=CARTESIAN_POINT('Ctrl Pts',(0.0138760875839061,-0.0319819883628706,
0.074300532895197));
#95245=CARTESIAN_POINT('Ctrl Pts',(0.0138654692841997,-0.0317295851069885,
0.074483398182353));
#95246=CARTESIAN_POINT('Origin',(-0.00283968559452192,-0.0326371942645095,
0.0742925970323401));
#95247=CARTESIAN_POINT('Origin',(-0.00277747244381728,-0.0326352985532441,
0.0747677043288159));
#95248=CARTESIAN_POINT('Ctrl Pts',(0.0141035876665989,-0.0321934096636183,
0.0746418602437497));
#95249=CARTESIAN_POINT('Ctrl Pts',(0.0140968045305051,-0.0320835708272304,
0.074724326421606));
#95250=CARTESIAN_POINT('Ctrl Pts',(0.0140883186956413,-0.0319739230346346,
0.0748066043890788));
#95251=CARTESIAN_POINT('Ctrl Pts',(0.0140781490981425,-0.0318646057455575,
0.0748885897104643));
#95252=CARTESIAN_POINT('Ctrl Pts',(0.0140251898851185,-0.0321934096636183,
0.0745600375535904));
#95253=CARTESIAN_POINT('Ctrl Pts',(0.0140195351476907,-0.0320835708272304,
0.0746414225649406));
#95254=CARTESIAN_POINT('Ctrl Pts',(0.0140121994316605,-0.0319739230346346,
0.0747226433451796));
#95255=CARTESIAN_POINT('Ctrl Pts',(0.0140032000978575,-0.0318646057455575,
0.0748035966982679));
#95256=CARTESIAN_POINT('Ctrl Pts',(0.0139467921036381,-0.0321934096636183,
0.0744782148634312));
#95257=CARTESIAN_POINT('Ctrl Pts',(0.0139422657648763,-0.0320835708272304,
0.0745585187082753));
#95258=CARTESIAN_POINT('Ctrl Pts',(0.0139360801676797,-0.0319739230346346,
0.0746386823012803));
#95259=CARTESIAN_POINT('Ctrl Pts',(0.0139282510975725,-0.0318646057455575,
0.0747186036860715));
#95260=CARTESIAN_POINT('Ctrl Pts',(0.0138683943221577,-0.0321934096636183,
0.074396392173272));
#95261=CARTESIAN_POINT('Ctrl Pts',(0.0138649963820619,-0.0320835708272304,
0.0744756148516099));
#95262=CARTESIAN_POINT('Ctrl Pts',(0.0138599609036989,-0.0319739230346346,
0.0745547212573811));
#95263=CARTESIAN_POINT('Ctrl Pts',(0.0138533020972875,-0.0318646057455575,
0.0746336106738751));
#95264=CARTESIAN_POINT('Ctrl Pts',(0.0138731999671288,-0.0320218834582284,
0.0742724461521044));
#95265=CARTESIAN_POINT('Ctrl Pts',(0.0138719255986971,-0.0319391099350594,
0.0743322836920026));
#95266=CARTESIAN_POINT('Ctrl Pts',(0.0138697176307971,-0.0318564869454889,
0.0743920650784139));
#95267=CARTESIAN_POINT('Ctrl Pts',(0.013866581736664,-0.0317740741446495,
0.0744517469186658));
#95268=CARTESIAN_POINT('Ctrl Pts',(0.0139097203771866,-0.0320218834582284,
0.074238933651498));
#95269=CARTESIAN_POINT('Ctrl Pts',(0.0139087947928702,-0.0319391099350594,
0.0742991512805774));
#95270=CARTESIAN_POINT('Ctrl Pts',(0.0139069294626203,-0.0318564869454889,
0.0743593179721964));
#95271=CARTESIAN_POINT('Ctrl Pts',(0.013904129836306,-0.0317740741446495,
0.0744193900297399));
#95272=CARTESIAN_POINT('Ctrl Pts',(0.0139462407872444,-0.0320218834582284,
0.0742054211508916));
#95273=CARTESIAN_POINT('Ctrl Pts',(0.0139456639870434,-0.0319391099350594,
0.0742660188691522));
#95274=CARTESIAN_POINT('Ctrl Pts',(0.0139441412944436,-0.0318564869454889,
0.0743265708659789));
#95275=CARTESIAN_POINT('Ctrl Pts',(0.0139416779359479,-0.0317740741446495,
0.0743870331408141));
#95276=CARTESIAN_POINT('Ctrl Pts',(0.0139827611973022,-0.0320218834582284,
0.0741719086502852));
#95277=CARTESIAN_POINT('Ctrl Pts',(0.0139825331812165,-0.0319391099350594,
0.074232886457727));
#95278=CARTESIAN_POINT('Ctrl Pts',(0.0139813531262668,-0.0318564869454889,
0.0742938237597613));
#95279=CARTESIAN_POINT('Ctrl Pts',(0.0139792260355899,-0.0317740741446495,
0.0743546762518882));
#95280=CARTESIAN_POINT('Origin',(0.0201824322144088,-0.0391228853390779,
0.0734647423886097));
#95281=CARTESIAN_POINT('Ctrl Pts',(0.0131357908142684,-0.035272297877955,
0.0713279556835488));
#95282=CARTESIAN_POINT('Ctrl Pts',(0.0131447555051321,-0.0352466642097187,
0.0713445907968852));
#95283=CARTESIAN_POINT('Ctrl Pts',(0.0131537812266114,-0.0352210183808287,
0.0713611738968043));
#95284=CARTESIAN_POINT('Ctrl Pts',(0.0131628687649444,-0.0351953608940152,
0.071377705313933));
#95285=CARTESIAN_POINT('Origin',(0.0175322732876919,-0.0352456003065006,
0.0691644665908431));
#95286=CARTESIAN_POINT('Ctrl Pts',(0.0132204943594808,-0.035024121149334,
0.071488270255359));
#95287=CARTESIAN_POINT('Ctrl Pts',(0.0132571585937083,-0.0349144232867422,
0.0715584753725519));
#95288=CARTESIAN_POINT('Ctrl Pts',(0.0132923935833736,-0.0348045283677513,
0.0716294803867756));
#95289=CARTESIAN_POINT('Ctrl Pts',(0.0133261508125351,-0.0346945769586886,
0.071701196029087));
#95290=CARTESIAN_POINT('Ctrl Pts',(0.0132567430570725,-0.035024121149334,
0.0713809055790178));
#95291=CARTESIAN_POINT('Ctrl Pts',(0.0132948861956287,-0.0349144232867422,
0.071451610007135));
#95292=CARTESIAN_POINT('Ctrl Pts',(0.013331590653705,-0.0348045283677513,
0.0715231452011525));
#95293=CARTESIAN_POINT('Ctrl Pts',(0.0133668060078872,-0.0346945769586886,
0.0715954212830754));
#95294=CARTESIAN_POINT('Ctrl Pts',(0.0132929917546642,-0.035024121149334,
0.0712735409026767));
#95295=CARTESIAN_POINT('Ctrl Pts',(0.0133326137975491,-0.0349144232867422,
0.0713447446417181));
#95296=CARTESIAN_POINT('Ctrl Pts',(0.0133707877240365,-0.0348045283677513,
0.0714168100155294));
#95297=CARTESIAN_POINT('Ctrl Pts',(0.0134074612032392,-0.0346945769586886,
0.0714896465370638));
#95298=CARTESIAN_POINT('Ctrl Pts',(0.0133292404522559,-0.035024121149334,
0.0711661762263355));
#95299=CARTESIAN_POINT('Ctrl Pts',(0.0133703413994695,-0.0349144232867422,
0.0712378792763012));
#95300=CARTESIAN_POINT('Ctrl Pts',(0.0134099847943679,-0.0348045283677513,
0.0713104748299062));
#95301=CARTESIAN_POINT('Ctrl Pts',(0.0134481163985913,-0.0346945769586886,
0.0713838717910522));
#95302=CARTESIAN_POINT('Origin',(-0.00193975610763966,-0.0345629067941104,
0.0786879717508215));
#95303=CARTESIAN_POINT('Ctrl Pts',(0.0135118000868944,-0.0351970973651643,
0.0716711323243206));
#95304=CARTESIAN_POINT('Ctrl Pts',(0.0135461414390807,-0.0350869349321794,
0.0717457760101826));
#95305=CARTESIAN_POINT('Ctrl Pts',(0.0135789594383797,-0.0349764985129738,
0.0718211954676863));
#95306=CARTESIAN_POINT('Ctrl Pts',(0.0136102058164377,-0.0348659306849652,
0.0718972954914902));
#95307=CARTESIAN_POINT('Ctrl Pts',(0.0134333449497974,-0.0351970973651643,
0.0716465302489431));
#95308=CARTESIAN_POINT('Ctrl Pts',(0.0134680271303964,-0.0350869349321794,
0.0717200870452061));
#95309=CARTESIAN_POINT('Ctrl Pts',(0.0135012088362788,-0.0349764985129738,
0.071794425798378));
#95310=CARTESIAN_POINT('Ctrl Pts',(0.0135328414103154,-0.0348659306849652,
0.0718694527309385));
#95311=CARTESIAN_POINT('Ctrl Pts',(0.0133548898127005,-0.0351970973651643,
0.0716219281735656));
#95312=CARTESIAN_POINT('Ctrl Pts',(0.0133899128217121,-0.0350869349321794,
0.0716943980802297));
#95313=CARTESIAN_POINT('Ctrl Pts',(0.0134234582341778,-0.0349764985129738,
0.0717676561290697));
#95314=CARTESIAN_POINT('Ctrl Pts',(0.0134554770041932,-0.0348659306849652,
0.0718416099703869));
#95315=CARTESIAN_POINT('Ctrl Pts',(0.0132764346756035,-0.0351970973651643,
0.0715973260981881));
#95316=CARTESIAN_POINT('Ctrl Pts',(0.0133117985130278,-0.0350869349321794,
0.0716687091152532));
#95317=CARTESIAN_POINT('Ctrl Pts',(0.0133457076320769,-0.0349764985129738,
0.0717408864597614));
#95318=CARTESIAN_POINT('Ctrl Pts',(0.0133781125980709,-0.0348659306849652,
0.0718137672098353));
#95319=CARTESIAN_POINT('Origin',(-0.00209513135373274,-0.0345637187965986,
0.0782327971808723));
#95320=CARTESIAN_POINT('Ctrl Pts',(0.0132623467969079,-0.0352450361861252,
0.071566730983312));
#95321=CARTESIAN_POINT('Ctrl Pts',(0.0133597763841107,-0.0349452761023764,
0.071760535122536));
#95322=CARTESIAN_POINT('Ctrl Pts',(0.0134423310637528,-0.0346444289983474,
0.0719611274795987));
#95323=CARTESIAN_POINT('Ctrl Pts',(0.0131452292349131,-0.0352450361861252,
0.0713458611649293));
#95324=CARTESIAN_POINT('Ctrl Pts',(0.0132509890637948,-0.0349452761023764,
0.0715352481429339));
#95325=CARTESIAN_POINT('Ctrl Pts',(0.0133421830384254,-0.0346444289983474,
0.0717320633553387));
#95326=CARTESIAN_POINT('Ctrl Pts',(0.0133775682100256,-0.0345231616327823,
0.0718135468651221));
#95327=CARTESIAN_POINT('Ctrl Pts',(0.0134097729270268,-0.0344132092796976,
0.0718859629086258));
#95328=CARTESIAN_POINT('Ctrl Pts',(0.0134404781136738,-0.0343032738558974,
0.071959041344963));
#95329=CARTESIAN_POINT('Ctrl Pts',(0.0134696468312344,-0.0341934961088741,
0.0720326875445818));
#95330=CARTESIAN_POINT('Ctrl Pts',(0.0134204868366391,-0.0345231616327823,
0.0717086701392579));
#95331=CARTESIAN_POINT('Ctrl Pts',(0.0134541371316517,-0.0344132092796976,
0.0717816777556049));
#95332=CARTESIAN_POINT('Ctrl Pts',(0.0134862755855073,-0.0343032738558974,
0.0718553776349038));
#95333=CARTESIAN_POINT('Ctrl Pts',(0.0135168634436862,-0.0341934961088741,
0.0719296743044281));
#95334=CARTESIAN_POINT('Ctrl Pts',(0.0134634054632526,-0.0345231616327823,
0.0716037934133937));
#95335=CARTESIAN_POINT('Ctrl Pts',(0.0134985013362766,-0.0344132092796976,
0.0716773926025839));
#95336=CARTESIAN_POINT('Ctrl Pts',(0.0135320730573408,-0.0343032738558974,
0.0717517139248446));
#95337=CARTESIAN_POINT('Ctrl Pts',(0.013564080056138,-0.0341934961088741,
0.0718266610642744));
#95338=CARTESIAN_POINT('Ctrl Pts',(0.0135063240898661,-0.0345231616327823,
0.0714989166875295));
#95339=CARTESIAN_POINT('Ctrl Pts',(0.0135428655409015,-0.0344132092796976,
0.071573107449563));
#95340=CARTESIAN_POINT('Ctrl Pts',(0.0135778705291742,-0.0343032738558974,
0.0716480502147854));
#95341=CARTESIAN_POINT('Ctrl Pts',(0.0136112966685897,-0.0341934961088741,
0.0717236478241207));
#95342=CARTESIAN_POINT('Origin',(-0.00195068449090722,-0.0345625596231814,
0.0786931745126852));
#95343=CARTESIAN_POINT('Ctrl Pts',(0.0137438958601374,-0.0346945769586885,
0.0720489711163765));
#95344=CARTESIAN_POINT('Ctrl Pts',(0.0137728491000978,-0.034584662917669,
0.0721264191233387));
#95345=CARTESIAN_POINT('Ctrl Pts',(0.0138002056923659,-0.0344746925051587,
0.0722044790997225));
#95346=CARTESIAN_POINT('Ctrl Pts',(0.0138259309975891,-0.0343648066255171,
0.0722830508813294));
#95347=CARTESIAN_POINT('Ctrl Pts',(0.0136381211974047,-0.0346945769586885,
0.0720083159530333));
#95348=CARTESIAN_POINT('Ctrl Pts',(0.0136676346860648,-0.034584662917669,
0.0720843063316803));
#95349=CARTESIAN_POINT('Ctrl Pts',(0.0136955817658793,-0.0344746925051587,
0.0721609200164953));
#95350=CARTESIAN_POINT('Ctrl Pts',(0.0137219270332417,-0.0343648066255171,
0.0722380586933108));
#95351=CARTESIAN_POINT('Ctrl Pts',(0.0135323465346721,-0.0346945769586885,
0.07196766078969));
#95352=CARTESIAN_POINT('Ctrl Pts',(0.0135624202720318,-0.034584662917669,
0.0720421935400218));
#95353=CARTESIAN_POINT('Ctrl Pts',(0.0135909578393927,-0.0344746925051587,
0.0721173609332682));
#95354=CARTESIAN_POINT('Ctrl Pts',(0.0136179230688944,-0.0343648066255171,
0.0721930665052923));
#95355=CARTESIAN_POINT('Ctrl Pts',(0.0134265718719395,-0.0346945769586885,
0.0719270056263468));
#95356=CARTESIAN_POINT('Ctrl Pts',(0.0134572058579988,-0.034584662917669,
0.0720000807483634));
#95357=CARTESIAN_POINT('Ctrl Pts',(0.0134863339129061,-0.0344746925051587,
0.072073801850041));
#95358=CARTESIAN_POINT('Ctrl Pts',(0.013513919104547,-0.0343648066255171,
0.0721480743172738));
#95359=CARTESIAN_POINT('Origin',(-0.00214909782709286,-0.0345626446731185,
0.0782551969665255));
#95360=CARTESIAN_POINT('Ctrl Pts',(0.0134284645353448,-0.0346945769586885,
0.071927733083546));
#95361=CARTESIAN_POINT('Ctrl Pts',(0.0134750108056564,-0.034527515336289,
0.0720388417790813));
#95362=CARTESIAN_POINT('Ctrl Pts',(0.0135180748490115,-0.0343603235965158,
0.0721514430503747));
#95363=CARTESIAN_POINT('Ctrl Pts',(0.0135575342506988,-0.034193496108874,
0.072265201979884));
#95364=CARTESIAN_POINT('Ctrl Pts',(0.013394399305138,-0.0346945769586885,
0.0718511328980226));
#95365=CARTESIAN_POINT('Ctrl Pts',(0.0134425499970044,-0.034527515336289,
0.0719615280836723));
#95366=CARTESIAN_POINT('Ctrl Pts',(0.013487241316129,-0.0343603235965158,
0.0720734661181109));
#95367=CARTESIAN_POINT('Ctrl Pts',(0.0135283460058874,-0.034193496108874,
0.0721866139738265));
#95368=CARTESIAN_POINT('Ctrl Pts',(0.0133603340749312,-0.0346945769586885,
0.0717745327124992));
#95369=CARTESIAN_POINT('Ctrl Pts',(0.0134100891883523,-0.034527515336289,
0.0718842143882632));
#95370=CARTESIAN_POINT('Ctrl Pts',(0.0134564077832466,-0.0343603235965158,
0.0719954891858471));
#95371=CARTESIAN_POINT('Ctrl Pts',(0.013499157761076,-0.034193496108874,
0.0721080259677689));
#95372=CARTESIAN_POINT('Ctrl Pts',(0.0133262688447244,-0.0346945769586885,
0.0716979325269758));
#95373=CARTESIAN_POINT('Ctrl Pts',(0.0133776283797003,-0.034527515336289,
0.0718069006928541));
#95374=CARTESIAN_POINT('Ctrl Pts',(0.0134255742503641,-0.0343603235965158,
0.0719175122535833));
#95375=CARTESIAN_POINT('Ctrl Pts',(0.0134699695162646,-0.034193496108874,
0.0720294379617114));
#95376=CARTESIAN_POINT('Ctrl Pts',(0.0135139075963689,-0.0340223579322365,
0.0721480449312474));
#95377=CARTESIAN_POINT('Ctrl Pts',(0.0135415197780848,-0.0339125849573554,
0.0722223888185949));
#95378=CARTESIAN_POINT('Ctrl Pts',(0.0135675738113235,-0.0338030433565221,
0.0722972519733532));
#95379=CARTESIAN_POINT('Ctrl Pts',(0.0135920448640821,-0.0336938721132328,
0.0723725357046022));
#95380=CARTESIAN_POINT('Ctrl Pts',(0.0135633268647013,-0.0340223579322365,
0.0720460698570982));
#95381=CARTESIAN_POINT('Ctrl Pts',(0.0135923455486518,-0.0339125849573554,
0.0721210953650469));
#95382=CARTESIAN_POINT('Ctrl Pts',(0.0136197909878298,-0.0338030433565221,
0.0721966687727674));
#95383=CARTESIAN_POINT('Ctrl Pts',(0.013645636651375,-0.0336938721132328,
0.072272690323312));
#95384=CARTESIAN_POINT('Ctrl Pts',(0.0136127461330337,-0.0340223579322365,
0.0719440947829491));
#95385=CARTESIAN_POINT('Ctrl Pts',(0.0136431713192189,-0.0339125849573554,
0.0720198019114989));
#95386=CARTESIAN_POINT('Ctrl Pts',(0.0136720081643361,-0.0338030433565221,
0.0720960855721816));
#95387=CARTESIAN_POINT('Ctrl Pts',(0.013699228438668,-0.0336938721132328,
0.0721728449420217));
#95388=CARTESIAN_POINT('Ctrl Pts',(0.0136621654013662,-0.0340223579322365,
0.0718421197087999));
#95389=CARTESIAN_POINT('Ctrl Pts',(0.013693997089786,-0.0339125849573554,
0.0719185084579508));
#95390=CARTESIAN_POINT('Ctrl Pts',(0.0137242253408424,-0.0338030433565221,
0.0719955023715958));
#95391=CARTESIAN_POINT('Ctrl Pts',(0.0137528202259609,-0.0336938721132328,
0.0720729995607315));
#95392=CARTESIAN_POINT('Origin',(-0.00184005217284519,-0.0345589643414554,
0.0786461280643633));
#95393=CARTESIAN_POINT('Ctrl Pts',(0.0138647305447576,-0.034193496108874,
0.0724060068739107));
#95394=CARTESIAN_POINT('Ctrl Pts',(0.0138887791772146,-0.0340836138581107,
0.0724851711520253));
#95395=CARTESIAN_POINT('Ctrl Pts',(0.0139111781320594,-0.0339738896643499,
0.0725647950816189));
#95396=CARTESIAN_POINT('Ctrl Pts',(0.0139319055728418,-0.0338644633294062,
0.0726447748321448));
#95397=CARTESIAN_POINT('Ctrl Pts',(0.0137617172119098,-0.034193496108874,
0.0723587902189722));
#95398=CARTESIAN_POINT('Ctrl Pts',(0.0137864169340779,-0.0340836138581107,
0.0724365340042289));
#95399=CARTESIAN_POINT('Ctrl Pts',(0.0138094960603477,-0.0339738896643499,
0.0725147515954792));
#95400=CARTESIAN_POINT('Ctrl Pts',(0.0138309317630749,-0.0338644633294062,
0.0725933409037595));
#95401=CARTESIAN_POINT('Ctrl Pts',(0.0136587038790621,-0.034193496108874,
0.0723115735640337));
#95402=CARTESIAN_POINT('Ctrl Pts',(0.0136840546909412,-0.0340836138581107,
0.0723878968564325));
#95403=CARTESIAN_POINT('Ctrl Pts',(0.013707813988636,-0.0339738896643499,
0.0724647081093394));
#95404=CARTESIAN_POINT('Ctrl Pts',(0.0137299579533081,-0.0338644633294062,
0.0725419069753741));
#95405=CARTESIAN_POINT('Ctrl Pts',(0.0135556905462144,-0.034193496108874,
0.0722643569090952));
#95406=CARTESIAN_POINT('Ctrl Pts',(0.0135816924478045,-0.0340836138581107,
0.0723392597086361));
#95407=CARTESIAN_POINT('Ctrl Pts',(0.0136061319169243,-0.0339738896643499,
0.0724146646231997));
#95408=CARTESIAN_POINT('Ctrl Pts',(0.0136289841435412,-0.0338644633294062,
0.0724904730469888));
#95409=CARTESIAN_POINT('Origin',(-0.00207878075995784,-0.0345610621865069,
0.0782283258709278));
#95410=CARTESIAN_POINT('Ctrl Pts',(0.0135455709476501,-0.03424362768739,
0.0722310597452954));
#95411=CARTESIAN_POINT('Ctrl Pts',(0.0136179449724558,-0.033943005420186,
0.0724355458791655));
#95412=CARTESIAN_POINT('Ctrl Pts',(0.0136747106567857,-0.0336441434784162,
0.0726449025974582));
#95413=CARTESIAN_POINT('Ctrl Pts',(0.0134570560298694,-0.03424362768739,
0.0719972540367888));
#95414=CARTESIAN_POINT('Ctrl Pts',(0.0135382481823398,-0.033943005420186,
0.0721984017755008));
#95415=CARTESIAN_POINT('Ctrl Pts',(0.0136040584045603,-0.0336441434784162,
0.0724050938001729));
#95416=CARTESIAN_POINT('Ctrl Pts',(0.0136289760186054,-0.0335235895815127,
0.0724904465325943));
#95417=CARTESIAN_POINT('Ctrl Pts',(0.013651823039444,-0.0334144449262719,
0.0725662363643304));
#95418=CARTESIAN_POINT('Ctrl Pts',(0.0136731305478561,-0.0333049234473133,
0.0726425852716573));
#95419=CARTESIAN_POINT('Ctrl Pts',(0.0136928624546213,-0.0331951640388588,
0.0727193980958017));
#95420=CARTESIAN_POINT('Ctrl Pts',(0.013684700866248,-0.0335235895815127,
0.0723917757981214));
#95421=CARTESIAN_POINT('Ctrl Pts',(0.0137089062840114,-0.0334144449262719,
0.0724683327920974));
#95422=CARTESIAN_POINT('Ctrl Pts',(0.0137315579009873,-0.0333049234473133,
0.0725454778064989));
#95423=CARTESIAN_POINT('Ctrl Pts',(0.0137526178170403,-0.0331951640388588,
0.0726231148202633));
#95424=CARTESIAN_POINT('Ctrl Pts',(0.0137404257138906,-0.0335235895815127,
0.0722931050636484));
#95425=CARTESIAN_POINT('Ctrl Pts',(0.0137659895285788,-0.0334144449262719,
0.0723704292198644));
#95426=CARTESIAN_POINT('Ctrl Pts',(0.0137899852541185,-0.0333049234473133,
0.0724483703413403));
#95427=CARTESIAN_POINT('Ctrl Pts',(0.0138123731794593,-0.0331951640388588,
0.0725268315447249));
#95428=CARTESIAN_POINT('Ctrl Pts',(0.0137961505615332,-0.0335235895815127,
0.0721944343291755));
#95429=CARTESIAN_POINT('Ctrl Pts',(0.0138230727731462,-0.0334144449262719,
0.0722725256476314));
#95430=CARTESIAN_POINT('Ctrl Pts',(0.0138484126072496,-0.0333049234473133,
0.0723512628761819));
#95431=CARTESIAN_POINT('Ctrl Pts',(0.0138721285418783,-0.0331951640388588,
0.0724305482691866));
#95432=CARTESIAN_POINT('Origin',(-0.00262261164918678,-0.0326434571770125,
0.0761247095113126));
#95433=CARTESIAN_POINT('Ctrl Pts',(0.0139646948224223,-0.0336938721132388,
0.0727708842719304));
#95434=CARTESIAN_POINT('Ctrl Pts',(0.0139727672444178,-0.0336474569764957,
0.07280507307177));
#95435=CARTESIAN_POINT('Ctrl Pts',(0.013980438890217,-0.033601104548885,
0.0728393540268629));
#95436=CARTESIAN_POINT('Ctrl Pts',(0.0139998617318712,-0.0334837508694609,
0.0729261455159323));
#95437=CARTESIAN_POINT('Ctrl Pts',(0.0140167042329001,-0.0333660264863603,
0.073013474431601));
#95438=CARTESIAN_POINT('Ctrl Pts',(0.0136651594291254,-0.0336938721132388,
0.0726101093129208));
#95439=CARTESIAN_POINT('Ctrl Pts',(0.0136741729203068,-0.0336474569764957,
0.072642544832707));
#95440=CARTESIAN_POINT('Ctrl Pts',(0.0136828060951659,-0.033601104548885,
0.0726750836442855));
#95441=CARTESIAN_POINT('Ctrl Pts',(0.013704663307119,-0.0334837508694609,
0.0727574644269033));
#95442=CARTESIAN_POINT('Ctrl Pts',(0.0137240698078166,-0.0333660264863603,
0.0728404567084104));
#95443=CARTESIAN_POINT('Ctrl Pts',(0.0136651594291366,-0.0336938721132427,
0.0726101093129352));
#95444=CARTESIAN_POINT('Ctrl Pts',(0.0136741729203174,-0.0336474569765026,
0.0726425448327193));
#95445=CARTESIAN_POINT('Ctrl Pts',(0.0136828060951759,-0.0336011045488949,
0.0726750836442955));
#95446=CARTESIAN_POINT('Ctrl Pts',(0.0137044812663218,-0.033484728265791,
0.0727567783071924));
#95447=CARTESIAN_POINT('Ctrl Pts',(0.0137237464482251,-0.0333679870047996,
0.0728390746239767));
#95448=CARTESIAN_POINT('Ctrl Pts',(0.0136651594291247,-0.0336938721132428,
0.0726101093129181));
#95449=CARTESIAN_POINT('Ctrl Pts',(0.0136973956624559,-0.0335278710435084,
0.072726113085819));
#95450=CARTESIAN_POINT('Ctrl Pts',(0.0137259827069975,-0.033362046922432,
0.072843086968758));
#95451=CARTESIAN_POINT('Ctrl Pts',(0.0137509153232181,-0.0331951640388601,
0.072961093890998));
#95452=CARTESIAN_POINT('Ctrl Pts',(0.0136409633598077,-0.0336938721132428,
0.072529843628763));
#95453=CARTESIAN_POINT('Ctrl Pts',(0.0136748798833989,-0.0335278710435084,
0.0726453408786083));
#95454=CARTESIAN_POINT('Ctrl Pts',(0.0137051625115095,-0.033362046922432,
0.072761861110151));
#95455=CARTESIAN_POINT('Ctrl Pts',(0.0137318069233254,-0.0331951640388601,
0.0728794673090727));
#95456=CARTESIAN_POINT('Ctrl Pts',(0.0136167672904907,-0.0336938721132428,
0.0724495779446079));
#95457=CARTESIAN_POINT('Ctrl Pts',(0.0136523641043418,-0.0335278710435084,
0.0725645686713976));
#95458=CARTESIAN_POINT('Ctrl Pts',(0.0136843423160216,-0.033362046922432,
0.0726806352515439));
#95459=CARTESIAN_POINT('Ctrl Pts',(0.0137126985234327,-0.0331951640388601,
0.0727978407271474));
#95460=CARTESIAN_POINT('Ctrl Pts',(0.0135925712211737,-0.0336938721132428,
0.0723693122604529));
#95461=CARTESIAN_POINT('Ctrl Pts',(0.0136298483252848,-0.0335278710435084,
0.0724837964641869));
#95462=CARTESIAN_POINT('Ctrl Pts',(0.0136635221205336,-0.033362046922432,
0.0725994093929369));
#95463=CARTESIAN_POINT('Ctrl Pts',(0.01369359012354,-0.0331951640388601,
0.072716214145222));
#95464=CARTESIAN_POINT('Ctrl Pts',(0.0137223170541567,-0.0330240426238156,
0.0728393939609575));
#95465=CARTESIAN_POINT('Ctrl Pts',(0.013740371929206,-0.0329142774063509,
0.0729165192330562));
#95466=CARTESIAN_POINT('Ctrl Pts',(0.0137568414104559,-0.0328043479726686,
0.072994056199617));
#95467=CARTESIAN_POINT('Ctrl Pts',(0.0137717016637264,-0.0326943950436594,
0.0730719061110635));
#95468=CARTESIAN_POINT('Ctrl Pts',(0.0137841274251584,-0.0330240426238156,
0.072744417047862));
#95469=CARTESIAN_POINT('Ctrl Pts',(0.0138034906997171,-0.0329142774063509,
0.0728223938180403));
#95470=CARTESIAN_POINT('Ctrl Pts',(0.0138212516299175,-0.0328043479726686,
0.0729008097554561));
#95471=CARTESIAN_POINT('Ctrl Pts',(0.0138373846961265,-0.0326943950436594,
0.072979565030069));
#95472=CARTESIAN_POINT('Ctrl Pts',(0.0138459377961602,-0.0330240426238156,
0.0726494401347666));
#95473=CARTESIAN_POINT('Ctrl Pts',(0.0138666094702283,-0.0329142774063509,
0.0727282684030243));
#95474=CARTESIAN_POINT('Ctrl Pts',(0.0138856618493791,-0.0328043479726686,
0.0728075633112951));
#95475=CARTESIAN_POINT('Ctrl Pts',(0.0139030677285267,-0.0326943950436594,
0.0728872239490745));
#95476=CARTESIAN_POINT('Ctrl Pts',(0.0139077481671619,-0.0330240426238156,
0.0725544632216711));
#95477=CARTESIAN_POINT('Ctrl Pts',(0.0139297282407395,-0.0329142774063509,
0.0726341429880084));
#95478=CARTESIAN_POINT('Ctrl Pts',(0.0139500720688406,-0.0328043479726686,
0.0727143168671342));
#95479=CARTESIAN_POINT('Ctrl Pts',(0.0139687507609269,-0.0326943950436594,
0.07279488286808));
#95480=CARTESIAN_POINT('Origin',(-0.00274371983696767,-0.0326396682861129,
0.0761497735418175));
#95481=CARTESIAN_POINT('Ctrl Pts',(0.0140380417500741,-0.0331951640388588,
0.0731392904012537));
#95482=CARTESIAN_POINT('Ctrl Pts',(0.0140519622301479,-0.0330855618255041,
0.0732207473622013));
#95483=CARTESIAN_POINT('Ctrl Pts',(0.0140642091691572,-0.0329757224427708,
0.0733025507568613));
#95484=CARTESIAN_POINT('Ctrl Pts',(0.0140747617457512,-0.0328657862078596,
0.0733845966003569));
#95485=CARTESIAN_POINT('Ctrl Pts',(0.013941758551186,-0.0331951640388588,
0.0730795350864055));
#95486=CARTESIAN_POINT('Ctrl Pts',(0.0139565020398379,-0.0330855618255041,
0.0731596659410677));
#95487=CARTESIAN_POINT('Ctrl Pts',(0.0139695999890708,-0.0329757224427708,
0.0732401592836514));
#95488=CARTESIAN_POINT('Ctrl Pts',(0.0139810305700538,-0.0328657862078596,
0.0733209128603354));
#95489=CARTESIAN_POINT('Ctrl Pts',(0.013845475352298,-0.0331951640388588,
0.0730197797715573));
#95490=CARTESIAN_POINT('Ctrl Pts',(0.0138610418495279,-0.0330855618255041,
0.0730985845199341));
#95491=CARTESIAN_POINT('Ctrl Pts',(0.0138749908089843,-0.0329757224427708,
0.0731777678104415));
#95492=CARTESIAN_POINT('Ctrl Pts',(0.0138872993943565,-0.0328657862078596,
0.073257229120314));
#95493=CARTESIAN_POINT('Ctrl Pts',(0.0137491921534099,-0.0331951640388588,
0.072960024456709));
#95494=CARTESIAN_POINT('Ctrl Pts',(0.0137655816592178,-0.0330855618255041,
0.0730375030988005));
#95495=CARTESIAN_POINT('Ctrl Pts',(0.0137803816288978,-0.0329757224427708,
0.0731153763372315));
#95496=CARTESIAN_POINT('Ctrl Pts',(0.0137935682186592,-0.0328657862078596,
0.0731935453802926));
#95497=CARTESIAN_POINT('Origin',(-0.00279255920260905,-0.0326401908835072,
0.0756713515645391));
#95498=CARTESIAN_POINT('Ctrl Pts',(0.0137433409369527,-0.0332451089994432,
0.0729257922870346));
#95499=CARTESIAN_POINT('Ctrl Pts',(0.0137895126862565,-0.0329451141710257,
0.0731377374126622));
#95500=CARTESIAN_POINT('Ctrl Pts',(0.0138195886931928,-0.0326442513127503,
0.0733525582694659));
#95501=CARTESIAN_POINT('Ctrl Pts',(0.0136848306738065,-0.0332451089994432,
0.0726827356082403));
#95502=CARTESIAN_POINT('Ctrl Pts',(0.0137401694557315,-0.0329451141710257,
0.0728924739831889));
#95503=CARTESIAN_POINT('Ctrl Pts',(0.0137795526741993,-0.0326442513127503,
0.0731057848568316));
#95504=CARTESIAN_POINT('Ctrl Pts',(0.0137935630527179,-0.0325229783203385,
0.0731935142179197));
#95505=CARTESIAN_POINT('Ctrl Pts',(0.0138067481880669,-0.032413025311208,
0.0732716720216568));
#95506=CARTESIAN_POINT('Ctrl Pts',(0.0138183145290902,-0.0323031222247695,
0.0733500907226891));
#95507=CARTESIAN_POINT('Ctrl Pts',(0.0138282508046342,-0.0321934096636184,
0.0734286693494433));
#95508=CARTESIAN_POINT('Ctrl Pts',(0.0138612151077861,-0.0325229783203385,
0.0731026057909487));
#95509=CARTESIAN_POINT('Ctrl Pts',(0.0138756534137901,-0.032413025311208,
0.0731816961767686));
#95510=CARTESIAN_POINT('Ctrl Pts',(0.0138884534437424,-0.0323031222247695,
0.0732610732418835));
#95511=CARTESIAN_POINT('Ctrl Pts',(0.0138996023895397,-0.0321934096636184,
0.0733406347313618));
#95512=CARTESIAN_POINT('Ctrl Pts',(0.0139288671628544,-0.0325229783203385,
0.0730116973639778));
#95513=CARTESIAN_POINT('Ctrl Pts',(0.0139445586395133,-0.032413025311208,
0.0730917203318803));
#95514=CARTESIAN_POINT('Ctrl Pts',(0.0139585923583947,-0.0323031222247695,
0.073172055761078));
#95515=CARTESIAN_POINT('Ctrl Pts',(0.0139709539744452,-0.0321934096636184,
0.0732526001132802));
#95516=CARTESIAN_POINT('Ctrl Pts',(0.0139965192179226,-0.0325229783203385,
0.0729207889370068));
#95517=CARTESIAN_POINT('Ctrl Pts',(0.0140134638652365,-0.032413025311208,
0.0730017444869921));
#95518=CARTESIAN_POINT('Ctrl Pts',(0.0140287312730469,-0.0323031222247695,
0.0730830382802724));
#95519=CARTESIAN_POINT('Ctrl Pts',(0.0140423055593507,-0.0321934096636184,
0.0731645654951987));
#95520=CARTESIAN_POINT('Origin',(-0.00273529484821876,-0.0326393375179589,
0.076148465647772));
#95521=CARTESIAN_POINT('Ctrl Pts',(0.0140898342906189,-0.0326943950436593,
0.0735126442359838));
#95522=CARTESIAN_POINT('Ctrl Pts',(0.014098618247579,-0.0325844576448127,
0.0735948676154605));
#95523=CARTESIAN_POINT('Ctrl Pts',(0.0141057023118987,-0.0324744968375319,
0.0736772784806451));
#95524=CARTESIAN_POINT('Ctrl Pts',(0.0141110788634599,-0.0323646534831894,
0.0737597711167384));
#95525=CARTESIAN_POINT('Ctrl Pts',(0.0139974932398338,-0.0326943950436593,
0.0734469612250719));
#95526=CARTESIAN_POINT('Ctrl Pts',(0.0140071824317874,-0.0325844576448127,
0.0735279119718032));
#95527=CARTESIAN_POINT('Ctrl Pts',(0.0140151981152972,-0.0324744968375319,
0.07360906883592));
#95528=CARTESIAN_POINT('Ctrl Pts',(0.0140215314544389,-0.0323646534831894,
0.0736903276928586));
#95529=CARTESIAN_POINT('Ctrl Pts',(0.0139051521890488,-0.0326943950436593,
0.07338127821416));
#95530=CARTESIAN_POINT('Ctrl Pts',(0.0139157466159958,-0.0325844576448127,
0.0734609563281459));
#95531=CARTESIAN_POINT('Ctrl Pts',(0.0139246939186956,-0.0324744968375319,
0.0735408591911949));
#95532=CARTESIAN_POINT('Ctrl Pts',(0.0139319840454179,-0.0323646534831894,
0.0736208842689787));
#95533=CARTESIAN_POINT('Ctrl Pts',(0.0138128111382638,-0.0326943950436593,
0.0733155952032481));
#95534=CARTESIAN_POINT('Ctrl Pts',(0.0138243108002043,-0.0325844576448127,
0.0733940006844886));
#95535=CARTESIAN_POINT('Ctrl Pts',(0.0138341897220941,-0.0324744968375319,
0.0734726495464699));
#95536=CARTESIAN_POINT('Ctrl Pts',(0.0138424366363968,-0.0323646534831894,
0.0735514408450988));
#95537=CARTESIAN_POINT('Origin',(-0.00282997230623912,-0.0326395579068746,
0.075677027961926));
#95538=CARTESIAN_POINT('Ctrl Pts',(0.0138091147336051,-0.0327445246961876,
0.0732810242212984));
#95539=CARTESIAN_POINT('Ctrl Pts',(0.0138418886905391,-0.0324436878365474,
0.0734954500412169));
#95540=CARTESIAN_POINT('Ctrl Pts',(0.0138584181111671,-0.0321434074463185,
0.0737117353683997));
#95541=CARTESIAN_POINT('Ctrl Pts',(0.0137659799028439,-0.0327445246961876,
0.0730347735636847));
#95542=CARTESIAN_POINT('Ctrl Pts',(0.013808041355063,-0.0324436878365474,
0.0732475725268825));
#95543=CARTESIAN_POINT('Ctrl Pts',(0.0138339544276795,-0.0321434074463185,
0.0734629351911686));
#95544=CARTESIAN_POINT('Ctrl Pts',(0.0138529529799322,-0.0322357242816071,
0.0736452950412317));
#95545=CARTESIAN_POINT('Ctrl Pts',(0.0138690271782907,-0.0319819883628704,
0.0738277617003296));
#95546=CARTESIAN_POINT('Ctrl Pts',(0.0138734579247823,-0.0317295851069886,
0.0740108814153272));
#95547=CARTESIAN_POINT('Ctrl Pts',(0.0138256071141881,-0.0322357242816071,
0.0733967951345381));
#95548=CARTESIAN_POINT('Ctrl Pts',(0.0138495957122821,-0.0319819883628704,
0.0735783908632785));
#95549=CARTESIAN_POINT('Ctrl Pts',(0.0138619802387864,-0.0317295851069886,
0.0737611450288631));
#95550=CARTESIAN_POINT('Origin',(-0.00273536322915428,-0.0326371942643931,
0.0756655594808861));
#95551=CARTESIAN_POINT('Origin',(-0.00261409391399649,-0.0326352985534603,
0.0761291230395348));
#95552=CARTESIAN_POINT('Ctrl Pts',(0.0141180815491696,-0.0321934096636184,
0.0738885134227378));
#95553=CARTESIAN_POINT('Ctrl Pts',(0.0141216876528603,-0.0320835708272304,
0.0739711794825305));
#95554=CARTESIAN_POINT('Ctrl Pts',(0.0141235808950535,-0.0319739230346346,
0.0740538722207776));
#95555=CARTESIAN_POINT('Ctrl Pts',(0.0141237669733025,-0.0318646057455575,
0.0741364856519547));
#95556=CARTESIAN_POINT('Ctrl Pts',(0.014030046855276,-0.0321934096636184,
0.073817161776387));
#95557=CARTESIAN_POINT('Ctrl Pts',(0.0140346369537779,-0.0320835708272304,
0.0738986137691409));
#95558=CARTESIAN_POINT('Ctrl Pts',(0.0140375387450797,-0.0319739230346346,
0.0739801135082788));
#95559=CARTESIAN_POINT('Ctrl Pts',(0.0140387565192221,-0.0318646057455575,
0.0740615564356039));
#95560=CARTESIAN_POINT('Ctrl Pts',(0.0139420121613824,-0.0321934096636184,
0.0737458101300362));
#95561=CARTESIAN_POINT('Ctrl Pts',(0.0139475862546956,-0.0320835708272304,
0.0738260480557513));
#95562=CARTESIAN_POINT('Ctrl Pts',(0.0139514965951059,-0.0319739230346346,
0.07390635479578));
#95563=CARTESIAN_POINT('Ctrl Pts',(0.0139537460651417,-0.0318646057455575,
0.073986627219253));
#95564=CARTESIAN_POINT('Ctrl Pts',(0.0138539774674888,-0.0321934096636184,
0.0736744584836855));
#95565=CARTESIAN_POINT('Ctrl Pts',(0.0138605355556133,-0.0320835708272304,
0.0737534823423617));
#95566=CARTESIAN_POINT('Ctrl Pts',(0.0138654544451321,-0.0319739230346346,
0.0738325960832812));
#95567=CARTESIAN_POINT('Ctrl Pts',(0.0138687356110613,-0.0318646057455575,
0.0739116980029022));
#95568=CARTESIAN_POINT('Ctrl Pts',(0.0138432106628924,-0.0320218834582284,
0.0735508875068933));
#95569=CARTESIAN_POINT('Ctrl Pts',(0.0138494459756004,-0.0319391099350596,
0.0736104129306331));
#95570=CARTESIAN_POINT('Ctrl Pts',(0.0138547480126527,-0.0318564869454893,
0.0736699996547131));
#95571=CARTESIAN_POINT('Ctrl Pts',(0.0138591169640053,-0.0317740741446501,
0.0737296039175802));
#95572=CARTESIAN_POINT('Ctrl Pts',(0.013875242868543,-0.0320218834582284,
0.0735130620412803));
#95573=CARTESIAN_POINT('Ctrl Pts',(0.0138818718529055,-0.0319391099350596,
0.0735729208428435));
#95574=CARTESIAN_POINT('Ctrl Pts',(0.0138875621173552,-0.0318564869454893,
0.0736328468899999));
#95575=CARTESIAN_POINT('Ctrl Pts',(0.0138923135921493,-0.0317740741446501,
0.0736927961476457));
#95576=CARTESIAN_POINT('Ctrl Pts',(0.0139072750741935,-0.0320218834582284,
0.0734752365756672));
#95577=CARTESIAN_POINT('Ctrl Pts',(0.0139142977302106,-0.0319391099350596,
0.0735354287550539));
#95578=CARTESIAN_POINT('Ctrl Pts',(0.0139203762220577,-0.0318564869454893,
0.0735956941252867));
#95579=CARTESIAN_POINT('Ctrl Pts',(0.0139255102202933,-0.0317740741446501,
0.0736559883777112));
#95580=CARTESIAN_POINT('Ctrl Pts',(0.0139393072798441,-0.0320218834582284,
0.0734374111100542));
#95581=CARTESIAN_POINT('Ctrl Pts',(0.0139467236075157,-0.0319391099350596,
0.0734979366672643));
#95582=CARTESIAN_POINT('Ctrl Pts',(0.0139531903267603,-0.0318564869454893,
0.0735585413605735));
#95583=CARTESIAN_POINT('Ctrl Pts',(0.0139587068484374,-0.0317740741446501,
0.0736191806077768));
#95584=CARTESIAN_POINT('Origin',(0.0200014606049758,-0.0391228853390726,
0.0719587962499599));
#95585=CARTESIAN_POINT('Ctrl Pts',(0.0127425736898337,-0.0352722978779547,
0.0707220370987458));
#95586=CARTESIAN_POINT('Ctrl Pts',(0.0127535526239773,-0.0352466642097185,
0.070737417465551));
#95587=CARTESIAN_POINT('Ctrl Pts',(0.0127645855884823,-0.0352210183808286,
0.0707527385799157));
#95588=CARTESIAN_POINT('Ctrl Pts',(0.0127756734048254,-0.0351953608940152,
0.0707680006713182));
#95589=CARTESIAN_POINT('Origin',(0.0168332315020225,-0.0352456003065004,
0.0680245823990329));
#95590=CARTESIAN_POINT('Ctrl Pts',(0.0128467020659647,-0.035024121149334,
0.0708704713730577));
#95591=CARTESIAN_POINT('Ctrl Pts',(0.0128918762261048,-0.0349144232867421,
0.0709355276549003));
#95592=CARTESIAN_POINT('Ctrl Pts',(0.0129357326653843,-0.0348045283677512,
0.0710015566581894));
#95593=CARTESIAN_POINT('Ctrl Pts',(0.0129782120620591,-0.0346945769586886,
0.0710684758985538));
#95594=CARTESIAN_POINT('Ctrl Pts',(0.0128692085696925,-0.035024121149334,
0.070759410132776));
#95595=CARTESIAN_POINT('Ctrl Pts',(0.0129159125528116,-0.0349144232867421,
0.0708247764324656));
#95596=CARTESIAN_POINT('Ctrl Pts',(0.0129612933224528,-0.0348045283677512,
0.0708911472616948));
#95597=CARTESIAN_POINT('Ctrl Pts',(0.0130052895881056,-0.0346945769586886,
0.0709584397709131));
#95598=CARTESIAN_POINT('Ctrl Pts',(0.0128917150734203,-0.035024121149334,
0.0706483488924945));
#95599=CARTESIAN_POINT('Ctrl Pts',(0.0129399488795185,-0.0349144232867421,
0.0707140252100308));
#95600=CARTESIAN_POINT('Ctrl Pts',(0.0129868539795212,-0.0348045283677512,
0.0707807378652002));
#95601=CARTESIAN_POINT('Ctrl Pts',(0.0130323671141522,-0.0346945769586886,
0.0708484036432725));
#95602=CARTESIAN_POINT('Ctrl Pts',(0.0129142215771481,-0.035024121149334,
0.0705372876522129));
#95603=CARTESIAN_POINT('Ctrl Pts',(0.0129639852062253,-0.0349144232867421,
0.0706032739875961));
#95604=CARTESIAN_POINT('Ctrl Pts',(0.0130124146365897,-0.0348045283677512,
0.0706703284687056));
#95605=CARTESIAN_POINT('Ctrl Pts',(0.0130594446401987,-0.0346945769586886,
0.0707383675156319));
#95606=CARTESIAN_POINT('Origin',(-0.00129164342851129,-0.0345629067944392,
0.0799134842847298));
#95607=CARTESIAN_POINT('Ctrl Pts',(0.0131586294551069,-0.0351970973651647,
0.0710153812312143));
#95608=CARTESIAN_POINT('Ctrl Pts',(0.0132020553499877,-0.0350869349321812,
0.0710851322166028));
#95609=CARTESIAN_POINT('Ctrl Pts',(0.013244067134042,-0.034976498512977,
0.0711558437831852));
#95610=CARTESIAN_POINT('Ctrl Pts',(0.0132846049871334,-0.0348659306849697,
0.0712274275259713));
#95611=CARTESIAN_POINT('Ctrl Pts',(0.0130777095025398,-0.0351970973651647,
0.0710008061865715));
#95612=CARTESIAN_POINT('Ctrl Pts',(0.0131213373149115,-0.0350869349321812,
0.0710694361356832));
#95613=CARTESIAN_POINT('Ctrl Pts',(0.0131635744894457,-0.034976498512977,
0.0711390299350881));
#95614=CARTESIAN_POINT('Ctrl Pts',(0.0132043609992496,-0.0348659306849697,
0.071209500645085));
#95615=CARTESIAN_POINT('Ctrl Pts',(0.0129967895499728,-0.0351970973651647,
0.0709862311419287));
#95616=CARTESIAN_POINT('Ctrl Pts',(0.0130406192798352,-0.0350869349321812,
0.0710537400547635));
#95617=CARTESIAN_POINT('Ctrl Pts',(0.0130830818448493,-0.034976498512977,
0.0711222160869908));
#95618=CARTESIAN_POINT('Ctrl Pts',(0.0131241170113659,-0.0348659306849697,
0.0711915737641986));
#95619=CARTESIAN_POINT('Ctrl Pts',(0.0129158695974057,-0.0351970973651647,
0.0709716560972859));
#95620=CARTESIAN_POINT('Ctrl Pts',(0.0129599012447589,-0.0350869349321812,
0.0710380439738438));
#95621=CARTESIAN_POINT('Ctrl Pts',(0.013002589200253,-0.034976498512977,
0.0711054022388937));
#95622=CARTESIAN_POINT('Ctrl Pts',(0.0130438730234821,-0.0348659306849697,
0.0711736468833122));
#95623=CARTESIAN_POINT('Origin',(-0.00150284199576083,-0.0345637187964519,
0.0794813725838939));
#95624=CARTESIAN_POINT('Ctrl Pts',(0.0128980582211641,-0.0352450361861252,
0.0709430679134204));
#95625=CARTESIAN_POINT('Ctrl Pts',(0.0130190096464181,-0.0349452761023764,
0.0711231326839111));
#95626=CARTESIAN_POINT('Ctrl Pts',(0.0131260542464923,-0.0346444289983474,
0.0713117964653789));
#95627=CARTESIAN_POINT('Ctrl Pts',(0.0127541818375923,-0.0352450361861252,
0.0707386184422782));
#95628=CARTESIAN_POINT('Ctrl Pts',(0.0128828442009826,-0.0349452761023764,
0.0709132568260592));
#95629=CARTESIAN_POINT('Ctrl Pts',(0.0129979865708702,-0.0346444289983474,
0.0710970904560062));
#95630=CARTESIAN_POINT('Ctrl Pts',(0.0130433053115867,-0.0345231616327822,
0.0711734965060001));
#95631=CARTESIAN_POINT('Ctrl Pts',(0.0130843322216695,-0.0344132092796975,
0.0712413052060534));
#95632=CARTESIAN_POINT('Ctrl Pts',(0.0131239544454785,-0.0343032738558974,
0.0713099590167629));
#95633=CARTESIAN_POINT('Ctrl Pts',(0.0131621234753269,-0.0341934961088741,
0.0713793686844099));
#95634=CARTESIAN_POINT('Ctrl Pts',(0.013072740972832,-0.0345231616327822,
0.0710640676341909));
#95635=CARTESIAN_POINT('Ctrl Pts',(0.0131152762058492,-0.0344132092796975,
0.0711322820633924));
#95636=CARTESIAN_POINT('Ctrl Pts',(0.0131563982825826,-0.0343032738558974,
0.0712013727807864));
#95637=CARTESIAN_POINT('Ctrl Pts',(0.0131960567881982,-0.0341934961088741,
0.0712712499237069));
#95638=CARTESIAN_POINT('Ctrl Pts',(0.0131021766340773,-0.0345231616327822,
0.0709546387623816));
#95639=CARTESIAN_POINT('Ctrl Pts',(0.0131462201900288,-0.0344132092796975,
0.0710232589207312));
#95640=CARTESIAN_POINT('Ctrl Pts',(0.0131888421196867,-0.0343032738558974,
0.0710927865448099));
#95641=CARTESIAN_POINT('Ctrl Pts',(0.0132299901010695,-0.0341934961088741,
0.0711631311630038));
#95642=CARTESIAN_POINT('Ctrl Pts',(0.0131316122953226,-0.0345231616327822,
0.0708452098905724));
#95643=CARTESIAN_POINT('Ctrl Pts',(0.0131771641742084,-0.0344132092796975,
0.0709142357780702));
#95644=CARTESIAN_POINT('Ctrl Pts',(0.0132212859567907,-0.0343032738558974,
0.0709842003088334));
#95645=CARTESIAN_POINT('Ctrl Pts',(0.0132639234139408,-0.0341934961088741,
0.0710550124023007));
#95646=CARTESIAN_POINT('Origin',(-0.00130183356012355,-0.0345625596229081,
0.0799200157104307));
#95647=CARTESIAN_POINT('Ctrl Pts',(0.0134362508414286,-0.0346945769586885,
0.0713611513377829));
#95648=CARTESIAN_POINT('Ctrl Pts',(0.0134746825855898,-0.034584662917669,
0.0714343598408911));
#95649=CARTESIAN_POINT('Ctrl Pts',(0.0135116069722089,-0.0344746925051587,
0.0715083756008774));
#95650=CARTESIAN_POINT('Ctrl Pts',(0.0135469770811724,-0.0343648066255171,
0.0715831035848301));
#95651=CARTESIAN_POINT('Ctrl Pts',(0.0133262148004225,-0.0346945769586885,
0.0713340738330552));
#95652=CARTESIAN_POINT('Ctrl Pts',(0.0133650196862848,-0.034584662917669,
0.0714057659839018));
#95653=CARTESIAN_POINT('Ctrl Pts',(0.0134023486358807,-0.0344746925051587,
0.0714782728490469));
#95654=CARTESIAN_POINT('Ctrl Pts',(0.0134381542027392,-0.0343648066255171,
0.0715515013268078));
#95655=CARTESIAN_POINT('Ctrl Pts',(0.0132161787594164,-0.0346945769586885,
0.0713069963283276));
#95656=CARTESIAN_POINT('Ctrl Pts',(0.0132553567869799,-0.034584662917669,
0.0713771721269125));
#95657=CARTESIAN_POINT('Ctrl Pts',(0.0132930902995526,-0.0344746925051587,
0.0714481700972163));
#95658=CARTESIAN_POINT('Ctrl Pts',(0.0133293313243061,-0.0343648066255171,
0.0715198990687856));
#95659=CARTESIAN_POINT('Ctrl Pts',(0.0131061427184102,-0.0346945769586885,
0.0712799188235999));
#95660=CARTESIAN_POINT('Ctrl Pts',(0.013145693887675,-0.034584662917669,
0.0713485782699231));
#95661=CARTESIAN_POINT('Ctrl Pts',(0.0131838319632244,-0.0344746925051587,
0.0714180673453858));
#95662=CARTESIAN_POINT('Ctrl Pts',(0.0132205084458729,-0.0343648066255171,
0.0714882968107634));
#95663=CARTESIAN_POINT('Origin',(-0.00155357548898538,-0.0345626446734559,
0.079510359533461));
#95664=CARTESIAN_POINT('Ctrl Pts',(0.0131081116321624,-0.0346945769586884,
0.0712804033309573));
#95665=CARTESIAN_POINT('Ctrl Pts',(0.0131682164833183,-0.0345275153362889,
0.0713848021066732));
#95666=CARTESIAN_POINT('Ctrl Pts',(0.0132250536352637,-0.0343603235965158,
0.0714911181275061));
#95667=CARTESIAN_POINT('Ctrl Pts',(0.0132784596622649,-0.0341934961088739,
0.0715990344594701));
#95668=CARTESIAN_POINT('Ctrl Pts',(0.0130647144675272,-0.0346945769586884,
0.07120867666623));
#95669=CARTESIAN_POINT('Ctrl Pts',(0.0131263216623937,-0.0345275153362889,
0.0713121664709574));
#95670=CARTESIAN_POINT('Ctrl Pts',(0.0131846901329335,-0.0343603235965158,
0.0714176205330221));
#95671=CARTESIAN_POINT('Ctrl Pts',(0.0132396518865634,-0.0341934961088739,
0.0715247244004177));
#95672=CARTESIAN_POINT('Ctrl Pts',(0.0130213173028921,-0.0346945769586884,
0.0711369500015027));
#95673=CARTESIAN_POINT('Ctrl Pts',(0.0130844268414691,-0.0345275153362889,
0.0712395308352416));
#95674=CARTESIAN_POINT('Ctrl Pts',(0.0131443266306033,-0.0343603235965158,
0.0713441229385381));
#95675=CARTESIAN_POINT('Ctrl Pts',(0.0132008441108619,-0.0341934961088739,
0.0714504143413653));
#95676=CARTESIAN_POINT('Ctrl Pts',(0.012977920138257,-0.0346945769586884,
0.0710652233367754));
#95677=CARTESIAN_POINT('Ctrl Pts',(0.0130425320205444,-0.0345275153362889,
0.0711668951995257));
#95678=CARTESIAN_POINT('Ctrl Pts',(0.0131039631282731,-0.0343603235965158,
0.0712706253440542));
#95679=CARTESIAN_POINT('Ctrl Pts',(0.0131620363351604,-0.0341934961088739,
0.0713761042823129));
#95680=CARTESIAN_POINT('Ctrl Pts',(0.0132204933453946,-0.0340223579322365,
0.0714882690988118));
#95681=CARTESIAN_POINT('Ctrl Pts',(0.0132572055566073,-0.0339125849573552,
0.071558566038382));
#95682=CARTESIAN_POINT('Ctrl Pts',(0.0132924369872727,-0.0338030433565217,
0.0716295734385714));
#95683=CARTESIAN_POINT('Ctrl Pts',(0.0133261506319435,-0.033693872113232,
0.0717011964989426));
#95684=CARTESIAN_POINT('Ctrl Pts',(0.0132567420622493,-0.0340223579322365,
0.0713809042518803));
#95685=CARTESIAN_POINT('Ctrl Pts',(0.0132949351147205,-0.0339125849573552,
0.0714517011557965));
#95686=CARTESIAN_POINT('Ctrl Pts',(0.0133316359979741,-0.0338030433565217,
0.0715232388189858));
#95687=CARTESIAN_POINT('Ctrl Pts',(0.013366805887493,-0.033693872113232,
0.0715954215963123));
#95688=CARTESIAN_POINT('Ctrl Pts',(0.013292990779104,-0.0340223579322365,
0.0712735394049487));
#95689=CARTESIAN_POINT('Ctrl Pts',(0.0133326646728337,-0.0339125849573552,
0.071344836273211));
#95690=CARTESIAN_POINT('Ctrl Pts',(0.0133708350086756,-0.0338030433565217,
0.0714169041994003));
#95691=CARTESIAN_POINT('Ctrl Pts',(0.0134074611430425,-0.033693872113232,
0.071489646693682));
#95692=CARTESIAN_POINT('Ctrl Pts',(0.0133292394959588,-0.0340223579322365,
0.0711661745580171));
#95693=CARTESIAN_POINT('Ctrl Pts',(0.0133703942309469,-0.0339125849573552,
0.0712379713906255));
#95694=CARTESIAN_POINT('Ctrl Pts',(0.013410034019377,-0.0338030433565217,
0.0713105695798147));
#95695=CARTESIAN_POINT('Ctrl Pts',(0.013448116398592,-0.033693872113232,
0.0713838717910516));
#95696=CARTESIAN_POINT('Origin',(-0.00119797009390548,-0.0345589643415581,
0.0798594743315512));
#95697=CARTESIAN_POINT('Ctrl Pts',(0.0136008811544589,-0.034193496108874,
0.0717002271599773));
#95698=CARTESIAN_POINT('Ctrl Pts',(0.0136346620707946,-0.0340836138595105,
0.071775753110283));
#95699=CARTESIAN_POINT('Ctrl Pts',(0.0136668639273651,-0.0339738896671456,
0.0718519418469909));
#95700=CARTESIAN_POINT('Ctrl Pts',(0.0136974520464904,-0.0338644633335883,
0.0719286930951262));
#95701=CARTESIAN_POINT('Ctrl Pts',(0.0134927622964681,-0.034193496108874,
0.0716662938165721));
#95702=CARTESIAN_POINT('Ctrl Pts',(0.0135270111335089,-0.0340836138595105,
0.0717403288718705));
#95703=CARTESIAN_POINT('Ctrl Pts',(0.0135597115372108,-0.0339738896671456,
0.0718150371115677));
#95704=CARTESIAN_POINT('Ctrl Pts',(0.0135908280647937,-0.0338644633335883,
0.0718903201127684));
#95705=CARTESIAN_POINT('Ctrl Pts',(0.0133846434384773,-0.034193496108874,
0.0716323604731668));
#95706=CARTESIAN_POINT('Ctrl Pts',(0.0134193601962231,-0.0340836138595105,
0.071704904633458));
#95707=CARTESIAN_POINT('Ctrl Pts',(0.0134525591470564,-0.0339738896671456,
0.0717781323761444));
#95708=CARTESIAN_POINT('Ctrl Pts',(0.013484204083097,-0.0338644633335883,
0.0718519471304106));
#95709=CARTESIAN_POINT('Ctrl Pts',(0.0132765245804865,-0.034193496108874,
0.0715984271297616));
#95710=CARTESIAN_POINT('Ctrl Pts',(0.0133117092589374,-0.0340836138595105,
0.0716694803950455));
#95711=CARTESIAN_POINT('Ctrl Pts',(0.0133454067569021,-0.0339738896671456,
0.0717412276407211));
#95712=CARTESIAN_POINT('Ctrl Pts',(0.0133775801014003,-0.0338644633335883,
0.0718135741480528));
#95713=CARTESIAN_POINT('Origin',(-0.00148718073547668,-0.0345610621864637,
0.0794748872591137));
#95714=CARTESIAN_POINT('Ctrl Pts',(0.013262311536772,-0.0342436276873899,
0.0715666608460542));
#95715=CARTESIAN_POINT('Ctrl Pts',(0.0133597437791519,-0.033943005420186,
0.0717604636751267));
#95716=CARTESIAN_POINT('Ctrl Pts',(0.0134423012035778,-0.0336441434784164,
0.0719610549263912));
#95717=CARTESIAN_POINT('Ctrl Pts',(0.0131451909600831,-0.0342436276873899,
0.0713457926262577));
#95718=CARTESIAN_POINT('Ctrl Pts',(0.0132509533846973,-0.033943005420186,
0.0715351781799608));
#95719=CARTESIAN_POINT('Ctrl Pts',(0.0133421500534631,-0.0336441434784164,
0.0717319921683297));
#95720=CARTESIAN_POINT('Ctrl Pts',(0.0133775687186269,-0.0335235895815127,
0.0718135488638217));
#95721=CARTESIAN_POINT('Ctrl Pts',(0.0134097345685649,-0.0334144449262719,
0.0718858775790982));
#95722=CARTESIAN_POINT('Ctrl Pts',(0.0134404431163433,-0.0333049234473133,
0.071958953913558));
#95723=CARTESIAN_POINT('Ctrl Pts',(0.0134696466307592,-0.0331951640388588,
0.0720326879819619));
#95724=CARTESIAN_POINT('Ctrl Pts',(0.0134204874369919,-0.0335235895815127,
0.0717086720022167));
#95725=CARTESIAN_POINT('Ctrl Pts',(0.0134540971234135,-0.0334144449262719,
0.0717815915781507));
#95726=CARTESIAN_POINT('Ctrl Pts',(0.0134862389597321,-0.0333049234473133,
0.0718552892806703));
#95727=CARTESIAN_POINT('Ctrl Pts',(0.0135168633100361,-0.0331951640388588,
0.0719296745960148));
#95728=CARTESIAN_POINT('Ctrl Pts',(0.013463406155357,-0.0335235895815127,
0.0716037951406117));
#95729=CARTESIAN_POINT('Ctrl Pts',(0.013498459678262,-0.0334144449262719,
0.0716773055772031));
#95730=CARTESIAN_POINT('Ctrl Pts',(0.0135320348031209,-0.0333049234473133,
0.0717516246477827));
#95731=CARTESIAN_POINT('Ctrl Pts',(0.0135640799893129,-0.0331951640388588,
0.0718266612100676));
#95732=CARTESIAN_POINT('Ctrl Pts',(0.0135063248737221,-0.0335235895815127,
0.0714989182790066));
#95733=CARTESIAN_POINT('Ctrl Pts',(0.0135428222331106,-0.0334144449262719,
0.0715730195762555));
#95734=CARTESIAN_POINT('Ctrl Pts',(0.0135778306465096,-0.0333049234473133,
0.071647960014895));
#95735=CARTESIAN_POINT('Ctrl Pts',(0.0136112966685898,-0.0331951640388588,
0.0717236478241205));
#95736=CARTESIAN_POINT('Origin',(-0.00229037639583367,-0.0326434571767497,
0.0774560186261367));
#95737=CARTESIAN_POINT('Ctrl Pts',(0.013745788448085,-0.0336938721132382,
0.0720496985445698));
#95738=CARTESIAN_POINT('Ctrl Pts',(0.0137580822094575,-0.0336474569764954,
0.0720826060127594));
#95739=CARTESIAN_POINT('Ctrl Pts',(0.0137699899049895,-0.033601104548885,
0.0721156551401071));
#95740=CARTESIAN_POINT('Ctrl Pts',(0.0138001374510285,-0.0334837508643167,
0.07219932792848));
#95741=CARTESIAN_POINT('Ctrl Pts',(0.013827792360393,-0.0333660264760416,
0.0722838573081909));
#95742=CARTESIAN_POINT('Ctrl Pts',(0.0134284645353433,-0.0336938721132382,
0.0719277330835424));
#95743=CARTESIAN_POINT('Ctrl Pts',(0.0134414722010316,-0.0336474569764954,
0.0719587831495714));
#95744=CARTESIAN_POINT('Ctrl Pts',(0.0134541154951997,-0.033601104548885,
0.0719899833591804));
#95745=CARTESIAN_POINT('Ctrl Pts',(0.0134861254077803,-0.0334837508643167,
0.0720689751131332));
#95746=CARTESIAN_POINT('Ctrl Pts',(0.0135157805746217,-0.0333660264760416,
0.0721488806997686));
#95747=CARTESIAN_POINT('Ctrl Pts',(0.0134284645353548,-0.0336938721132426,
0.071927733083556));
#95748=CARTESIAN_POINT('Ctrl Pts',(0.0134414722010423,-0.0336474569765026,
0.0719587831495832));
#95749=CARTESIAN_POINT('Ctrl Pts',(0.0134541154952097,-0.0336011045488949,
0.0719899833591904));
#95750=CARTESIAN_POINT('Ctrl Pts',(0.0134858588088175,-0.0334847282606778,
0.0720683172194232));
#95751=CARTESIAN_POINT('Ctrl Pts',(0.013515286543691,-0.0333679869945434,
0.0721475500411451));
#95752=CARTESIAN_POINT('Ctrl Pts',(0.013428464535342,-0.0336938721132427,
0.0719277330835393));
#95753=CARTESIAN_POINT('Ctrl Pts',(0.0134749857043083,-0.0335278710435083,
0.0720387818606809));
#95754=CARTESIAN_POINT('Ctrl Pts',(0.0135180080464564,-0.033362046922432,
0.0721512504628841));
#95755=CARTESIAN_POINT('Ctrl Pts',(0.0135575342506985,-0.0331951640388601,
0.0722652019798831));
#95756=CARTESIAN_POINT('Ctrl Pts',(0.0133943993015192,-0.0336938721132427,
0.071851132889885));
#95757=CARTESIAN_POINT('Ctrl Pts',(0.0134425240269824,-0.0335278710435083,
0.0719614685418449));
#95758=CARTESIAN_POINT('Ctrl Pts',(0.0134871717249203,-0.033362046922432,
0.0720732745568571));
#95759=CARTESIAN_POINT('Ctrl Pts',(0.0135283460027888,-0.0331951640388601,
0.0721866139654837));
#95760=CARTESIAN_POINT('Ctrl Pts',(0.0133603340676964,-0.0336938721132427,
0.0717745326962308));
#95761=CARTESIAN_POINT('Ctrl Pts',(0.0134100623496565,-0.0335278710435083,
0.0718841552230089));
#95762=CARTESIAN_POINT('Ctrl Pts',(0.0134563354033842,-0.033362046922432,
0.0719952986508301));
#95763=CARTESIAN_POINT('Ctrl Pts',(0.0134991577548792,-0.0331951640388601,
0.0721080259510843));
#95764=CARTESIAN_POINT('Ctrl Pts',(0.0133262688338736,-0.0336938721132427,
0.0716979325025765));
#95765=CARTESIAN_POINT('Ctrl Pts',(0.0133776006723306,-0.0335278710435083,
0.0718068419041729));
#95766=CARTESIAN_POINT('Ctrl Pts',(0.0134254990818481,-0.033362046922432,
0.0719173227448031));
#95767=CARTESIAN_POINT('Ctrl Pts',(0.0134699695069695,-0.0331951640388601,
0.0720294379366849));
#95768=CARTESIAN_POINT('Ctrl Pts',(0.0135139084417739,-0.0330240426238156,
0.0721480460036767));
#95769=CARTESIAN_POINT('Ctrl Pts',(0.0135414873084824,-0.0329142774063509,
0.0722223002440972));
#95770=CARTESIAN_POINT('Ctrl Pts',(0.0135675448816933,-0.0328043479726686,
0.0722971616351774));
#95771=CARTESIAN_POINT('Ctrl Pts',(0.0135920451385624,-0.0326943950436594,
0.0723725351932255));
#95772=CARTESIAN_POINT('Ctrl Pts',(0.0135633276559063,-0.0330240426238156,
0.0720460711182437));
#95773=CARTESIAN_POINT('Ctrl Pts',(0.0135923113260109,-0.0329142774063509,
0.0721210061564858));
#95774=CARTESIAN_POINT('Ctrl Pts',(0.0136197603289709,-0.0328043479726686,
0.0721965777260002));
#95775=CARTESIAN_POINT('Ctrl Pts',(0.0136456368343617,-0.0326943950436594,
0.0722726899823945));
#95776=CARTESIAN_POINT('Ctrl Pts',(0.0136127468700386,-0.0330240426238156,
0.0719440962328108));
#95777=CARTESIAN_POINT('Ctrl Pts',(0.0136431353435394,-0.0329142774063509,
0.0720197120688743));
#95778=CARTESIAN_POINT('Ctrl Pts',(0.0136719757762486,-0.0328043479726686,
0.0720959938168231));
#95779=CARTESIAN_POINT('Ctrl Pts',(0.013699228530161,-0.0326943950436594,
0.0721728447715636));
#95780=CARTESIAN_POINT('Ctrl Pts',(0.0136621660841709,-0.0330240426238156,
0.0718421213473778));
#95781=CARTESIAN_POINT('Ctrl Pts',(0.0136939593610679,-0.0329142774063509,
0.0719184179812629));
#95782=CARTESIAN_POINT('Ctrl Pts',(0.0137241912235263,-0.0328043479726686,
0.071995409907646));
#95783=CARTESIAN_POINT('Ctrl Pts',(0.0137528202259603,-0.0326943950436594,
0.0720729995607326));
#95784=CARTESIAN_POINT('Origin',(-0.00240738825288042,-0.0326396682861535,
0.0774960639003165));
#95785=CARTESIAN_POINT('Ctrl Pts',(0.0138647305447576,-0.0331951640388587,
0.0724060068739108));
#95786=CARTESIAN_POINT('Ctrl Pts',(0.0138887505220001,-0.0330855618255041,
0.0724850768236108));
#95787=CARTESIAN_POINT('Ctrl Pts',(0.0139111535742066,-0.0329757224427708,
0.0725647002256031));
#95788=CARTESIAN_POINT('Ctrl Pts',(0.013931906011448,-0.0328657862078596,
0.0726447765245699));
#95789=CARTESIAN_POINT('Ctrl Pts',(0.0137617172408188,-0.0331951640388587,
0.0723587902322228));
#95790=CARTESIAN_POINT('Ctrl Pts',(0.0137863875317821,-0.0330855618255041,
0.0724364413820553));
#95791=CARTESIAN_POINT('Ctrl Pts',(0.0138094706906795,-0.0329757224427708,
0.0725146584022601));
#95792=CARTESIAN_POINT('Ctrl Pts',(0.0138309322450051,-0.0328657862078596,
0.072593342581196));
#95793=CARTESIAN_POINT('Ctrl Pts',(0.0136587039368801,-0.0331951640388587,
0.0723115735905349));
#95794=CARTESIAN_POINT('Ctrl Pts',(0.0136840245415641,-0.0330855618255041,
0.0723878059404998));
#95795=CARTESIAN_POINT('Ctrl Pts',(0.0137077878071524,-0.0329757224427708,
0.0724646165789171));
#95796=CARTESIAN_POINT('Ctrl Pts',(0.0137299584785622,-0.0328657862078596,
0.072541908637822));
#95797=CARTESIAN_POINT('Ctrl Pts',(0.0135556906329414,-0.0331951640388587,
0.072264356948847));
#95798=CARTESIAN_POINT('Ctrl Pts',(0.0135816615513462,-0.0330855618255041,
0.0723391704989444));
#95799=CARTESIAN_POINT('Ctrl Pts',(0.0136061049236253,-0.0329757224427708,
0.0724145747555741));
#95800=CARTESIAN_POINT('Ctrl Pts',(0.0136289847121193,-0.0328657862078596,
0.0724904746944481));
#95801=CARTESIAN_POINT('Origin',(-0.00251580467905608,-0.0326401908832323,
0.0770275356184265));
#95802=CARTESIAN_POINT('Ctrl Pts',(0.0135455951265563,-0.0332451089994432,
0.0722311280619339));
#95803=CARTESIAN_POINT('Ctrl Pts',(0.0136179665657591,-0.0329451141710257,
0.0724356150823013));
#95804=CARTESIAN_POINT('Ctrl Pts',(0.0136747296070177,-0.0326442513127503,
0.0726449724892832));
#95805=CARTESIAN_POINT('Ctrl Pts',(0.0134570831548185,-0.0332451089994432,
0.0719973212381261));
#95806=CARTESIAN_POINT('Ctrl Pts',(0.013538272762654,-0.0329451141710257,
0.0721984699748624));
#95807=CARTESIAN_POINT('Ctrl Pts',(0.013604080374229,-0.0326442513127503,
0.0724051628024348));
#95808=CARTESIAN_POINT('Ctrl Pts',(0.013628975681232,-0.0325229783203385,
0.072490444425264));
#95809=CARTESIAN_POINT('Ctrl Pts',(0.0136518526181212,-0.032413025311208,
0.0725663333957258));
#95810=CARTESIAN_POINT('Ctrl Pts',(0.0136731562244631,-0.0323031222247695,
0.0726426840949569));
#95811=CARTESIAN_POINT('Ctrl Pts',(0.0136928626628868,-0.0321934096636184,
0.0727193977602254));
#95812=CARTESIAN_POINT('Ctrl Pts',(0.0136847004325288,-0.0325229783203385,
0.0723917737875737));
#95813=CARTESIAN_POINT('Ctrl Pts',(0.0137089375419761,-0.032413025311208,
0.0724684309224996));
#95814=CARTESIAN_POINT('Ctrl Pts',(0.0137315852241107,-0.0323031222247695,
0.0725455778066037));
#95815=CARTESIAN_POINT('Ctrl Pts',(0.0137526179558839,-0.0321934096636184,
0.0726231145965459));
#95816=CARTESIAN_POINT('Ctrl Pts',(0.0137404251838257,-0.0325229783203385,
0.0722931031498835));
#95817=CARTESIAN_POINT('Ctrl Pts',(0.0137660224658309,-0.032413025311208,
0.0723705284492734));
#95818=CARTESIAN_POINT('Ctrl Pts',(0.0137900142237584,-0.0323031222247695,
0.0724484715182504));
#95819=CARTESIAN_POINT('Ctrl Pts',(0.013812373248881,-0.0321934096636184,
0.0725268314328665));
#95820=CARTESIAN_POINT('Ctrl Pts',(0.0137961499351225,-0.0325229783203385,
0.0721944325121933));
#95821=CARTESIAN_POINT('Ctrl Pts',(0.0138231073896858,-0.032413025311208,
0.0722726259760472));
#95822=CARTESIAN_POINT('Ctrl Pts',(0.013848443223406,-0.0323031222247695,
0.0723513652298972));
#95823=CARTESIAN_POINT('Ctrl Pts',(0.013872128541878,-0.0321934096636184,
0.072430548269187));
#95824=CARTESIAN_POINT('Origin',(-0.00239919362031183,-0.0326393375181522,
0.0774937103885663));
#95825=CARTESIAN_POINT('Ctrl Pts',(0.0139629083290213,-0.0326943950436593,
0.0727699253755577));
#95826=CARTESIAN_POINT('Ctrl Pts',(0.0139819283438816,-0.0325844576448127,
0.0728503994773991));
#95827=CARTESIAN_POINT('Ctrl Pts',(0.0139992853684527,-0.0324744968375319,
0.0729312726396087));
#95828=CARTESIAN_POINT('Ctrl Pts',(0.0140149585931257,-0.0323646534831894,
0.0730124409360345));
#95829=CARTESIAN_POINT('Ctrl Pts',(0.0138630631508549,-0.0326943950436593,
0.0727163336972911));
#95830=CARTESIAN_POINT('Ctrl Pts',(0.0138828217594832,-0.0325844576448127,
0.0727954317454475));
#95831=CARTESIAN_POINT('Ctrl Pts',(0.01390094588914,-0.0324744968375319,
0.0728749440319168));
#95832=CARTESIAN_POINT('Ctrl Pts',(0.0139174137233068,-0.0323646534831894,
0.0729547683606236));
#95833=CARTESIAN_POINT('Ctrl Pts',(0.0137632179726886,-0.0326943950436593,
0.0726627420190245));
#95834=CARTESIAN_POINT('Ctrl Pts',(0.0137837151750849,-0.0325844576448127,
0.0727404640134959));
#95835=CARTESIAN_POINT('Ctrl Pts',(0.0138026064098274,-0.0324744968375319,
0.0728186154242249));
#95836=CARTESIAN_POINT('Ctrl Pts',(0.0138198688534879,-0.0323646534831894,
0.0728970957852128));
#95837=CARTESIAN_POINT('Ctrl Pts',(0.0136633727945222,-0.0326943950436593,
0.0726091503407578));
#95838=CARTESIAN_POINT('Ctrl Pts',(0.0136846085906865,-0.0325844576448127,
0.0726854962815443));
#95839=CARTESIAN_POINT('Ctrl Pts',(0.0137042669305148,-0.0324744968375319,
0.072762286816533));
#95840=CARTESIAN_POINT('Ctrl Pts',(0.013722323983669,-0.0323646534831894,
0.0728394232098019));
#95841=CARTESIAN_POINT('Origin',(-0.00255221132791817,-0.0326395579070405,
0.0770378563616196));
#95842=CARTESIAN_POINT('Ctrl Pts',(0.0136553726441631,-0.0327445246961876,
0.0725753152436751));
#95843=CARTESIAN_POINT('Ctrl Pts',(0.0137147628500275,-0.0324436878365474,
0.0727839425859584));
#95844=CARTESIAN_POINT('Ctrl Pts',(0.0137582696706652,-0.0321434074463186,
0.0729964507529987));
#95845=CARTESIAN_POINT('Ctrl Pts',(0.0135817145532401,-0.0327445246961876,
0.0723364125738667));
#95846=CARTESIAN_POINT('Ctrl Pts',(0.013650115120502,-0.0324436878365474,
0.0725422618558647));
#95847=CARTESIAN_POINT('Ctrl Pts',(0.013702815959905,-0.0321434074463186,
0.0727526785520346));
#95848=CARTESIAN_POINT('Ctrl Pts',(0.0137445204525794,-0.0322357242816072,
0.0729312192902247));
#95849=CARTESIAN_POINT('Ctrl Pts',(0.013783337037485,-0.0319819883628705,
0.0731102325139584));
#95850=CARTESIAN_POINT('Ctrl Pts',(0.0138106838322272,-0.0317295851069886,
0.0732913529555231));
#95851=CARTESIAN_POINT('Ctrl Pts',(0.0136862449203081,-0.0322357242816072,
0.0726881062252971));
#95852=CARTESIAN_POINT('Ctrl Pts',(0.0137328043410256,-0.0319819883628705,
0.0728652634489086));
#95853=CARTESIAN_POINT('Ctrl Pts',(0.0137679963823594,-0.0317295851069886,
0.0730450243505586));
#95854=CARTESIAN_POINT('Origin',(-0.00245978565393022,-0.0326371942644254,
0.077014620651325));
#95855=CARTESIAN_POINT('Origin',(-0.00228137266389705,-0.0326352985527658,
0.0774593297964607));
#95856=CARTESIAN_POINT('Ctrl Pts',(0.0140380417500742,-0.0321934096636183,
0.0731392904012538));
#95857=CARTESIAN_POINT('Ctrl Pts',(0.0140519802231401,-0.0320835708272303,
0.0732208526498378));
#95858=CARTESIAN_POINT('Ctrl Pts',(0.0140642226848299,-0.0319739230346346,
0.0733026560449787));
#95859=CARTESIAN_POINT('Ctrl Pts',(0.0140747615042616,-0.0318646057455575,
0.073384594722787));
#95860=CARTESIAN_POINT('Ctrl Pts',(0.0139417585034795,-0.0321934096636183,
0.0730795350567979));
#95861=CARTESIAN_POINT('Ctrl Pts',(0.0139565210493159,-0.0320835708272303,
0.0731597694843727));
#95862=CARTESIAN_POINT('Ctrl Pts',(0.0139696145849673,-0.0319739230346346,
0.0732402628828378));
#95863=CARTESIAN_POINT('Ctrl Pts',(0.0139810302620295,-0.0318646057455575,
0.0733209109807841));
#95864=CARTESIAN_POINT('Ctrl Pts',(0.0138454752568849,-0.0321934096636183,
0.0730197797123419));
#95865=CARTESIAN_POINT('Ctrl Pts',(0.0138610618754918,-0.0320835708272303,
0.0730986863189077));
#95866=CARTESIAN_POINT('Ctrl Pts',(0.0138750064851048,-0.0319739230346346,
0.0731778697206968));
#95867=CARTESIAN_POINT('Ctrl Pts',(0.0138872990197974,-0.0318646057455575,
0.0732572272387812));
#95868=CARTESIAN_POINT('Ctrl Pts',(0.0137491920102902,-0.0321934096636183,
0.072960024367886));
#95869=CARTESIAN_POINT('Ctrl Pts',(0.0137656027016676,-0.0320835708272303,
0.0730376031534426));
#95870=CARTESIAN_POINT('Ctrl Pts',(0.0137803983852423,-0.0319739230346346,
0.0731154765585559));
#95871=CARTESIAN_POINT('Ctrl Pts',(0.0137935677775653,-0.0318646057455575,
0.0731935434967783));
#95872=CARTESIAN_POINT('Ctrl Pts',(0.0137230225550669,-0.0320218834582285,
0.0728387772235915));
#95873=CARTESIAN_POINT('Ctrl Pts',(0.0137366692143082,-0.0319391099350598,
0.0728970517796814));
#95874=CARTESIAN_POINT('Ctrl Pts',(0.0137493976400211,-0.0318564869454897,
0.072955504123196));
#95875=CARTESIAN_POINT('Ctrl Pts',(0.0137612025358867,-0.0317740741446507,
0.073014090813847));
#95876=CARTESIAN_POINT('Ctrl Pts',(0.0137500613892921,-0.0320218834582285,
0.0727972353231601));
#95877=CARTESIAN_POINT('Ctrl Pts',(0.01376414039929,-0.0319391099350598,
0.0728557912881484));
#95878=CARTESIAN_POINT('Ctrl Pts',(0.0137772965195698,-0.0318564869454897,
0.0729145316212805));
#95879=CARTESIAN_POINT('Ctrl Pts',(0.0137895241618764,-0.0317740741446507,
0.0729734126434235));
#95880=CARTESIAN_POINT('Ctrl Pts',(0.0137771002235173,-0.0320218834582285,
0.0727556934227288));
#95881=CARTESIAN_POINT('Ctrl Pts',(0.0137916115842718,-0.0319391099350598,
0.0728145307966154));
#95882=CARTESIAN_POINT('Ctrl Pts',(0.0138051953991184,-0.0318564869454897,
0.072873559119365));
#95883=CARTESIAN_POINT('Ctrl Pts',(0.0138178457878661,-0.0317740741446507,
0.072932734473));
#95884=CARTESIAN_POINT('Ctrl Pts',(0.0138041390577425,-0.0320218834582285,
0.0727141515222974));
#95885=CARTESIAN_POINT('Ctrl Pts',(0.0138190827692536,-0.0319391099350598,
0.0727732703050823));
#95886=CARTESIAN_POINT('Ctrl Pts',(0.013833094278667,-0.0318564869454897,
0.0728325866174495));
#95887=CARTESIAN_POINT('Ctrl Pts',(0.0138461674138558,-0.0317740741446507,
0.0728920563025765));
#95888=CARTESIAN_POINT('Origin',(0.0196331709116167,-0.039122885339073,
0.0704874067034132));
#95889=CARTESIAN_POINT('Ctrl Pts',(0.0122765154643634,-0.0352722978779544,
0.0701701795366615));
#95890=CARTESIAN_POINT('Ctrl Pts',(0.0122893354974371,-0.0352466642097183,
0.0701840625993632));
#95891=CARTESIAN_POINT('Ctrl Pts',(0.0123022017085266,-0.0352210183808285,
0.0701978801050475));
#95892=CARTESIAN_POINT('Ctrl Pts',(0.0123151149413924,-0.0351953608940152,
0.0702116321784253));
#95893=CARTESIAN_POINT('Origin',(0.0159968364979673,-0.0352456003065005,
0.0669812997019457));
#95894=CARTESIAN_POINT('Ctrl Pts',(0.012398426504718,-0.035024121149334,
0.0703043926162986));
#95895=CARTESIAN_POINT('Ctrl Pts',(0.0124513981672796,-0.0349144232867422,
0.0703632740863637));
#95896=CARTESIAN_POINT('Ctrl Pts',(0.0125031844139273,-0.0348045283677513,
0.0704232857618924));
#95897=CARTESIAN_POINT('Ctrl Pts',(0.0125537160526539,-0.0346945769586886,
0.0704843532439135));
#95898=CARTESIAN_POINT('Ctrl Pts',(0.0124068358735734,-0.035024121149334,
0.0701913863141805));
#95899=CARTESIAN_POINT('Ctrl Pts',(0.0124613641515421,-0.0349144232867422,
0.0702503836198484));
#95900=CARTESIAN_POINT('Ctrl Pts',(0.0125147055509017,-0.0348045283677513,
0.0703105433766643));
#95901=CARTESIAN_POINT('Ctrl Pts',(0.0125667888806338,-0.0346945769586886,
0.0703717910701092));
#95902=CARTESIAN_POINT('Ctrl Pts',(0.0124152452424289,-0.035024121149334,
0.0700783800120624));
#95903=CARTESIAN_POINT('Ctrl Pts',(0.0124713301358046,-0.0349144232867422,
0.070137493153333));
#95904=CARTESIAN_POINT('Ctrl Pts',(0.012526226687876,-0.0348045283677513,
0.0701978009914363));
#95905=CARTESIAN_POINT('Ctrl Pts',(0.0125798617086137,-0.0346945769586886,
0.0702592288963048));
#95906=CARTESIAN_POINT('Ctrl Pts',(0.0124236546112843,-0.035024121149334,
0.0699653737099443));
#95907=CARTESIAN_POINT('Ctrl Pts',(0.0124812961200671,-0.0349144232867422,
0.0700246026868177));
#95908=CARTESIAN_POINT('Ctrl Pts',(0.0125377478248504,-0.0348045283677513,
0.0700850586062083));
#95909=CARTESIAN_POINT('Ctrl Pts',(0.0125929345365936,-0.0346945769586886,
0.0701466667225005));
#95910=CARTESIAN_POINT('Origin',(-0.000495043863386638,-0.0345629067943128,
0.0810481032281225));
#95911=CARTESIAN_POINT('Ctrl Pts',(0.0127260562743256,-0.035197097365165,
0.0704090649486225));
#95912=CARTESIAN_POINT('Ctrl Pts',(0.0127778818595984,-0.0350869349321799,
0.0704728232188328));
#95913=CARTESIAN_POINT('Ctrl Pts',(0.0128284248774781,-0.034976498512974,
0.0705377117308498));
#95914=CARTESIAN_POINT('Ctrl Pts',(0.0128776148994444,-0.0348659306849651,
0.0706036502742342));
#95915=CARTESIAN_POINT('Ctrl Pts',(0.0126439476622796,-0.035197097365165,
0.0704047467918752));
#95916=CARTESIAN_POINT('Ctrl Pts',(0.012695833069762,-0.0350869349321799,
0.0704673675585424));
#95917=CARTESIAN_POINT('Ctrl Pts',(0.0127464596074756,-0.034976498512974,
0.0705311188683923));
#95918=CARTESIAN_POINT('Ctrl Pts',(0.0127957568254235,-0.0348659306849652,
0.0705959219906337));
#95919=CARTESIAN_POINT('Ctrl Pts',(0.0125618390502336,-0.035197097365165,
0.0704004286351279));
#95920=CARTESIAN_POINT('Ctrl Pts',(0.0126137842799256,-0.0350869349321799,
0.070461911898252));
#95921=CARTESIAN_POINT('Ctrl Pts',(0.0126644943374731,-0.0349764985129741,
0.0705245260059347));
#95922=CARTESIAN_POINT('Ctrl Pts',(0.0127138987514027,-0.0348659306849652,
0.0705881937070332));
#95923=CARTESIAN_POINT('Ctrl Pts',(0.0124797304381876,-0.035197097365165,
0.0703961104783805));
#95924=CARTESIAN_POINT('Ctrl Pts',(0.0125317354900891,-0.0350869349321799,
0.0704564562379617));
#95925=CARTESIAN_POINT('Ctrl Pts',(0.0125825290674705,-0.0349764985129741,
0.0705179331434772));
#95926=CARTESIAN_POINT('Ctrl Pts',(0.0126320406773818,-0.0348659306849652,
0.0705804654234326));
#95927=CARTESIAN_POINT('Origin',(-0.000758735023101335,-0.0345637187965591,
0.0806458690564938));
#95928=CARTESIAN_POINT('Ctrl Pts',(0.0124584764604435,-0.0352450361861253,
0.0703699800782624));
#95929=CARTESIAN_POINT('Ctrl Pts',(0.0126010422475195,-0.0349452761023765,
0.0705334657510238));
#95930=CARTESIAN_POINT('Ctrl Pts',(0.0127308886107374,-0.0346444289983474,
0.0707072256163607));
#95931=CARTESIAN_POINT('Ctrl Pts',(0.0122901102718113,-0.0352450361861253,
0.0701851752446529));
#95932=CARTESIAN_POINT('Ctrl Pts',(0.0124396460873804,-0.0349452761023765,
0.0703423108825742));
#95933=CARTESIAN_POINT('Ctrl Pts',(0.0125769209885692,-0.0346444289983474,
0.0705102637639023));
#95934=CARTESIAN_POINT('Ctrl Pts',(0.0126314585947887,-0.0345231616327823,
0.0705803873850557));
#95935=CARTESIAN_POINT('Ctrl Pts',(0.0126806606790728,-0.0344132092796976,
0.0706425193579517));
#95936=CARTESIAN_POINT('Ctrl Pts',(0.0127285750739053,-0.0343032738558974,
0.0707056658314269));
#95937=CARTESIAN_POINT('Ctrl Pts',(0.0127751424676396,-0.0341934961088741,
0.0707697443351799));
#95938=CARTESIAN_POINT('Ctrl Pts',(0.0126469470727039,-0.0345231616327823,
0.0704681321259795));
#95939=CARTESIAN_POINT('Ctrl Pts',(0.0126976964376916,-0.0344132092796976,
0.0705304775857376));
#95940=CARTESIAN_POINT('Ctrl Pts',(0.0127471536175878,-0.0343032738558974,
0.0705938695393407));
#95941=CARTESIAN_POINT('Ctrl Pts',(0.0127952573323156,-0.0341934961088741,
0.0706582251513707));
#95942=CARTESIAN_POINT('Ctrl Pts',(0.0126624355506191,-0.0345231616327823,
0.0703558768669033));
#95943=CARTESIAN_POINT('Ctrl Pts',(0.0127147321963105,-0.0344132092796976,
0.0704184358135234));
#95944=CARTESIAN_POINT('Ctrl Pts',(0.0127657321612702,-0.0343032738558974,
0.0704820732472545));
#95945=CARTESIAN_POINT('Ctrl Pts',(0.0128153721969916,-0.0341934961088741,
0.0705467059675616));
#95946=CARTESIAN_POINT('Ctrl Pts',(0.0126779240285344,-0.0345231616327823,
0.0702436216078271));
#95947=CARTESIAN_POINT('Ctrl Pts',(0.0127317679549293,-0.0344132092796976,
0.0703063940413092));
#95948=CARTESIAN_POINT('Ctrl Pts',(0.0127843107049527,-0.0343032738558974,
0.0703702769551683));
#95949=CARTESIAN_POINT('Ctrl Pts',(0.0128354870616676,-0.0341934961088741,
0.0704351867837524));
#95950=CARTESIAN_POINT('Origin',(-0.000504335037640546,-0.0345625596231234,
0.0810558603139963));
#95951=CARTESIAN_POINT('Ctrl Pts',(0.0130448250186207,-0.0346945769586885,
0.0707173133685701));
#95952=CARTESIAN_POINT('Ctrl Pts',(0.0130921291754465,-0.0345846629176052,
0.0707851278260371));
#95953=CARTESIAN_POINT('Ctrl Pts',(0.013138039036808,-0.0344746925050311,
0.0708539320969166));
#95954=CARTESIAN_POINT('Ctrl Pts',(0.0131824961417883,-0.0343648066253259,
0.0709236377783091));
#95955=CARTESIAN_POINT('Ctrl Pts',(0.0129322629334401,-0.0346945769586885,
0.0707042405508829));
#95956=CARTESIAN_POINT('Ctrl Pts',(0.0129797472403013,-0.0345846629176052,
0.0707705038459218));
#95957=CARTESIAN_POINT('Ctrl Pts',(0.0130258693598702,-0.0344746925050311,
0.0708377604148596));
#95958=CARTESIAN_POINT('Ctrl Pts',(0.0130705705510705,-0.0343648066253259,
0.0709059238367677));
#95959=CARTESIAN_POINT('Ctrl Pts',(0.0128197008482596,-0.0346945769586885,
0.0706911677331956));
#95960=CARTESIAN_POINT('Ctrl Pts',(0.0128673653051561,-0.0345846629176052,
0.0707558798658065));
#95961=CARTESIAN_POINT('Ctrl Pts',(0.0129136996829324,-0.0344746925050311,
0.0708215887328026));
#95962=CARTESIAN_POINT('Ctrl Pts',(0.0129586449603526,-0.0343648066253259,
0.0708882098952263));
#95963=CARTESIAN_POINT('Ctrl Pts',(0.012707138763079,-0.0346945769586885,
0.0706780949155084));
#95964=CARTESIAN_POINT('Ctrl Pts',(0.0127549833700109,-0.0345846629176052,
0.0707412558856912));
#95965=CARTESIAN_POINT('Ctrl Pts',(0.0128015300059947,-0.0344746925050311,
0.0708054170507456));
#95966=CARTESIAN_POINT('Ctrl Pts',(0.0128467193696347,-0.0343648066253259,
0.0708704959536849));
#95967=CARTESIAN_POINT('Origin',(-0.000805435439944113,-0.0345626446733757,
0.08068098602812));
#95968=CARTESIAN_POINT('Ctrl Pts',(0.0127091528762319,-0.0346945769586885,
0.0706783288320533));
#95969=CARTESIAN_POINT('Ctrl Pts',(0.0127818684188246,-0.034527515336289,
0.070774371256892));
#95970=CARTESIAN_POINT('Ctrl Pts',(0.0128515823235211,-0.0343603235965159,
0.0708727253601056));
#95971=CARTESIAN_POINT('Ctrl Pts',(0.0129180927308873,-0.034193496108874,
0.0709730971895031));
#95972=CARTESIAN_POINT('Ctrl Pts',(0.0126571081763789,-0.0346945769586885,
0.0706126068604723));
#95973=CARTESIAN_POINT('Ctrl Pts',(0.0127312002919801,-0.034527515336289,
0.0707075591882351));
#95974=CARTESIAN_POINT('Ctrl Pts',(0.0128023254082869,-0.0343603235965159,
0.0708048662043718));
#95975=CARTESIAN_POINT('Ctrl Pts',(0.0128702774461011,-0.034193496108874,
0.0709042369914778));
#95976=CARTESIAN_POINT('Ctrl Pts',(0.012605063476526,-0.0346945769586885,
0.0705468848888913));
#95977=CARTESIAN_POINT('Ctrl Pts',(0.0126805321651355,-0.034527515336289,
0.0706407471195782));
#95978=CARTESIAN_POINT('Ctrl Pts',(0.0127530684930527,-0.0343603235965159,
0.0707370070486381));
#95979=CARTESIAN_POINT('Ctrl Pts',(0.0128224621613149,-0.034193496108874,
0.0708353767934525));
#95980=CARTESIAN_POINT('Ctrl Pts',(0.0125530187766731,-0.0346945769586885,
0.0704811629173104));
#95981=CARTESIAN_POINT('Ctrl Pts',(0.012629864038291,-0.034527515336289,
0.0705739350509212));
#95982=CARTESIAN_POINT('Ctrl Pts',(0.0127038115778185,-0.0343603235965159,
0.0706691478929043));
#95983=CARTESIAN_POINT('Ctrl Pts',(0.0127746468765287,-0.034193496108874,
0.0707665165954272));
#95984=CARTESIAN_POINT('Ctrl Pts',(0.012846700914921,-0.0340223579322366,
0.0708704703527289));
#95985=CARTESIAN_POINT('Ctrl Pts',(0.0128919341821289,-0.0339125849573554,
0.0709356117197912));
#95986=CARTESIAN_POINT('Ctrl Pts',(0.012935787389513,-0.0338030433565221,
0.0710016435362927));
#95987=CARTESIAN_POINT('Ctrl Pts',(0.0129782119417798,-0.0336938721132327,
0.0710684763873381));
#95988=CARTESIAN_POINT('Ctrl Pts',(0.0128692074163793,-0.0340223579322366,
0.0707594089407877));
#95989=CARTESIAN_POINT('Ctrl Pts',(0.0129159725101181,-0.0339125849573554,
0.0708248607312046));
#95990=CARTESIAN_POINT('Ctrl Pts',(0.0129613500425943,-0.0338030433565221,
0.0708912344581794));
#95991=CARTESIAN_POINT('Ctrl Pts',(0.0130052895079195,-0.0336938721132327,
0.070958440096769));
#95992=CARTESIAN_POINT('Ctrl Pts',(0.0128917139178376,-0.0340223579322366,
0.0706483475288465));
#95993=CARTESIAN_POINT('Ctrl Pts',(0.0129400108381074,-0.0339125849573554,
0.0707141097426179));
#95994=CARTESIAN_POINT('Ctrl Pts',(0.0129869126956757,-0.0338030433565221,
0.0707808253800661));
#95995=CARTESIAN_POINT('Ctrl Pts',(0.0130323670740592,-0.0336938721132327,
0.0708484038061999));
#95996=CARTESIAN_POINT('Ctrl Pts',(0.0129142204192959,-0.0340223579322366,
0.0705372861169054));
#95997=CARTESIAN_POINT('Ctrl Pts',(0.0129640491660967,-0.0339125849573554,
0.0706033587540312));
#95998=CARTESIAN_POINT('Ctrl Pts',(0.0130124753487571,-0.0338030433565221,
0.0706704163019528));
#95999=CARTESIAN_POINT('Ctrl Pts',(0.013059444640199,-0.0336938721132327,
0.0707383675156308));
#96000=CARTESIAN_POINT('Origin',(-0.000408878412918008,-0.0345589643414788,
0.0809827787775909));
#96001=CARTESIAN_POINT('Ctrl Pts',(0.0132506546416793,-0.034193496108874,
0.0710330818271546));
#96002=CARTESIAN_POINT('Ctrl Pts',(0.0132936350975172,-0.0340836138581107,
0.0711037783622071));
#96003=CARTESIAN_POINT('Ctrl Pts',(0.0133351320140729,-0.03397388966435,
0.0711753303660813));
#96004=CARTESIAN_POINT('Ctrl Pts',(0.0133750984193218,-0.0338644633294062,
0.0712476427007624));
#96005=CARTESIAN_POINT('Ctrl Pts',(0.013139135357523,-0.034193496108874,
0.0710129669443788));
#96006=CARTESIAN_POINT('Ctrl Pts',(0.0131823931856828,-0.0340836138581107,
0.0710821256945419));
#96007=CARTESIAN_POINT('Ctrl Pts',(0.0132241991627036,-0.03397388966435,
0.071152146391023));
#96008=CARTESIAN_POINT('Ctrl Pts',(0.0132645057896207,-0.0338644633294062,
0.0712229358291754));
#96009=CARTESIAN_POINT('Ctrl Pts',(0.0130276160733668,-0.034193496108874,
0.070992852061603));
#96010=CARTESIAN_POINT('Ctrl Pts',(0.0130711512738485,-0.0340836138581107,
0.0710604730268767));
#96011=CARTESIAN_POINT('Ctrl Pts',(0.0131132663113343,-0.03397388966435,
0.0711289624159647));
#96012=CARTESIAN_POINT('Ctrl Pts',(0.0131539131599197,-0.0338644633294062,
0.0711982289575884));
#96013=CARTESIAN_POINT('Ctrl Pts',(0.0129160967892105,-0.034193496108874,
0.0709727371788273));
#96014=CARTESIAN_POINT('Ctrl Pts',(0.0129599093620141,-0.0340836138581107,
0.0710388203592115));
#96015=CARTESIAN_POINT('Ctrl Pts',(0.013002333459965,-0.03397388966435,
0.0711057784409064));
#96016=CARTESIAN_POINT('Ctrl Pts',(0.0130433205302187,-0.0338644633294062,
0.0711735220860013));
#96017=CARTESIAN_POINT('Origin',(-0.000744010083504203,-0.0345610621862648,
0.0806374719937393));
#96018=CARTESIAN_POINT('Ctrl Pts',(0.0128980144485355,-0.03424362768739,
0.0709430027484825));
#96019=CARTESIAN_POINT('Ctrl Pts',(0.0130189683438243,-0.033943005420186,
0.0711230658863709));
#96020=CARTESIAN_POINT('Ctrl Pts',(0.0131260155284456,-0.0336441434784162,
0.0713117282267475));
#96021=CARTESIAN_POINT('Ctrl Pts',(0.0127541352743974,-0.03424362768739,
0.0707385552411627));
#96022=CARTESIAN_POINT('Ctrl Pts',(0.0128828000345398,-0.033943005420186,
0.0709131918865416));
#96023=CARTESIAN_POINT('Ctrl Pts',(0.0129979449239063,-0.0336441434784162,
0.0710970239644403));
#96024=CARTESIAN_POINT('Ctrl Pts',(0.0130433060666809,-0.0335235895815128,
0.0711734984251947));
#96025=CARTESIAN_POINT('Ctrl Pts',(0.0130842834710499,-0.0334144449262719,
0.0712412253569647));
#96026=CARTESIAN_POINT('Ctrl Pts',(0.0131239087660518,-0.0333049234473133,
0.0713098766611093));
#96027=CARTESIAN_POINT('Ctrl Pts',(0.0131621233312507,-0.0331951640388588,
0.0713793691434673));
#96028=CARTESIAN_POINT('Ctrl Pts',(0.0130727418019415,-0.0335235895815128,
0.0710640694072154));
#96029=CARTESIAN_POINT('Ctrl Pts',(0.0131152257121888,-0.0334144449262719,
0.0711322015798349));
#96030=CARTESIAN_POINT('Ctrl Pts',(0.0131563508718908,-0.0333049234473133,
0.0712012897136793));
#96031=CARTESIAN_POINT('Ctrl Pts',(0.0131960566921474,-0.0331951640388588,
0.071271250229745));
#96032=CARTESIAN_POINT('Ctrl Pts',(0.013102177537202,-0.0335235895815128,
0.0709546403892362));
#96033=CARTESIAN_POINT('Ctrl Pts',(0.0131461679533277,-0.0334144449262719,
0.0710231778027052));
#96034=CARTESIAN_POINT('Ctrl Pts',(0.0131887929777299,-0.0333049234473133,
0.0710927027662494));
#96035=CARTESIAN_POINT('Ctrl Pts',(0.0132299900530441,-0.0331951640388588,
0.0711631313160227));
#96036=CARTESIAN_POINT('Ctrl Pts',(0.0131316132724625,-0.0335235895815128,
0.0708452113712569));
#96037=CARTESIAN_POINT('Ctrl Pts',(0.0131771101944666,-0.0334144449262719,
0.0709141540255754));
#96038=CARTESIAN_POINT('Ctrl Pts',(0.0132212350835689,-0.0333049234473133,
0.0709841158188194));
#96039=CARTESIAN_POINT('Ctrl Pts',(0.0132639234139408,-0.0331951640388588,
0.0710550124023004));
#96040=CARTESIAN_POINT('Origin',(-0.00179390363966221,-0.0326434571770524,
0.0787351898528119));
#96041=CARTESIAN_POINT('Ctrl Pts',(0.013438219676683,-0.0336938721132375,
0.0713616358258208));
#96042=CARTESIAN_POINT('Ctrl Pts',(0.0134545408974716,-0.033647456976495,
0.071392742991929));
#96043=CARTESIAN_POINT('Ctrl Pts',(0.0134704968512645,-0.033601104548885,
0.0714240390870506));
#96044=CARTESIAN_POINT('Ctrl Pts',(0.0135108936560266,-0.0334837508643164,
0.0715032736010666));
#96045=CARTESIAN_POINT('Ctrl Pts',(0.0135489248386611,-0.033366026476041,
0.0715836703621564));
#96046=CARTESIAN_POINT('Ctrl Pts',(0.0131081116321606,-0.0336938721132375,
0.0712804033309542));
#96047=CARTESIAN_POINT('Ctrl Pts',(0.0131249083336974,-0.0336474569764951,
0.0713095782651363));
#96048=CARTESIAN_POINT('Ctrl Pts',(0.0131413623548727,-0.033601104548885,
0.0713389478268323));
#96049=CARTESIAN_POINT('Ctrl Pts',(0.0131830201516796,-0.0334837508643164,
0.0714133048013619));
#96050=CARTESIAN_POINT('Ctrl Pts',(0.0132224563042259,-0.033366026476041,
0.0714888635306281));
#96051=CARTESIAN_POINT('Ctrl Pts',(0.0131081116321723,-0.0336938721132427,
0.0712804033309673));
#96052=CARTESIAN_POINT('Ctrl Pts',(0.0131249083337082,-0.0336474569765026,
0.0713095782651479));
#96053=CARTESIAN_POINT('Ctrl Pts',(0.0131413623548827,-0.0336011045488949,
0.0713389478268423));
#96054=CARTESIAN_POINT('Ctrl Pts',(0.013182673198982,-0.0334847282606778,
0.0714126855090515));
#96055=CARTESIAN_POINT('Ctrl Pts',(0.0132217993931271,-0.0333679869945434,
0.0714876052831402));
#96056=CARTESIAN_POINT('Ctrl Pts',(0.0131081116321587,-0.0336938721132427,
0.0712804033309509));
#96057=CARTESIAN_POINT('Ctrl Pts',(0.0131681840701349,-0.0335278710435084,
0.0713847458067803));
#96058=CARTESIAN_POINT('Ctrl Pts',(0.0132249632218537,-0.0333620469224321,
0.0714909354312055));
#96059=CARTESIAN_POINT('Ctrl Pts',(0.0132784596622644,-0.0331951640388602,
0.071599034459469));
#96060=CARTESIAN_POINT('Ctrl Pts',(0.013064714462917,-0.0336938721132427,
0.0712086766586101));
#96061=CARTESIAN_POINT('Ctrl Pts',(0.0131262884345833,-0.0335278710435084,
0.071312110653542));
#96062=CARTESIAN_POINT('Ctrl Pts',(0.0131845970814808,-0.0333620469224321,
0.0714174392043771));
#96063=CARTESIAN_POINT('Ctrl Pts',(0.0132396518824436,-0.0331951640388602,
0.0715247243925289));
#96064=CARTESIAN_POINT('Ctrl Pts',(0.0130213172936753,-0.0336938721132427,
0.0711369499862693));
#96065=CARTESIAN_POINT('Ctrl Pts',(0.0130843927990317,-0.0335278710435084,
0.0712394755003036));
#96066=CARTESIAN_POINT('Ctrl Pts',(0.0131442309411079,-0.0333620469224321,
0.0713439429775488));
#96067=CARTESIAN_POINT('Ctrl Pts',(0.0132008441026227,-0.0331951640388602,
0.0714504143255888));
#96068=CARTESIAN_POINT('Ctrl Pts',(0.0129779201244336,-0.0336938721132427,
0.0710652233139285));
#96069=CARTESIAN_POINT('Ctrl Pts',(0.01304249716348,-0.0335278710435084,
0.0711668403470652));
#96070=CARTESIAN_POINT('Ctrl Pts',(0.013103864800735,-0.0333620469224321,
0.0712704467507205));
#96071=CARTESIAN_POINT('Ctrl Pts',(0.0131620363228018,-0.0331951640388602,
0.0713761042586486));
#96072=CARTESIAN_POINT('Ctrl Pts',(0.0132204943185443,-0.0330240426238155,
0.0714882700568273));
#96073=CARTESIAN_POINT('Ctrl Pts',(0.0132571622417092,-0.0329142774063509,
0.0715584822318409));
#96074=CARTESIAN_POINT('Ctrl Pts',(0.0132923969633854,-0.0328043479726686,
0.071629487438583));
#96075=CARTESIAN_POINT('Ctrl Pts',(0.0133261508401667,-0.0326943950436594,
0.0717011959571964));
#96076=CARTESIAN_POINT('Ctrl Pts',(0.0132567430052788,-0.0330240426238156,
0.071380905403917));
#96077=CARTESIAN_POINT('Ctrl Pts',(0.0132948899811378,-0.0329142774063509,
0.0714516169399057));
#96078=CARTESIAN_POINT('Ctrl Pts',(0.0133315941696836,-0.0328043479726686,
0.0715231523327233));
#96079=CARTESIAN_POINT('Ctrl Pts',(0.0133668060263082,-0.0326943950436594,
0.0715954212351484));
#96080=CARTESIAN_POINT('Ctrl Pts',(0.0132929916920132,-0.0330240426238156,
0.0712735407510067));
#96081=CARTESIAN_POINT('Ctrl Pts',(0.0133326177205664,-0.0329142774063509,
0.0713447516479706));
#96082=CARTESIAN_POINT('Ctrl Pts',(0.0133707913759818,-0.0328043479726686,
0.0714168172268637));
#96083=CARTESIAN_POINT('Ctrl Pts',(0.0134074612124497,-0.0326943950436594,
0.0714896465131004));
#96084=CARTESIAN_POINT('Ctrl Pts',(0.0133292403787477,-0.0330240426238156,
0.0711661760980964));
#96085=CARTESIAN_POINT('Ctrl Pts',(0.013370345459995,-0.0329142774063509,
0.0712378863560354));
#96086=CARTESIAN_POINT('Ctrl Pts',(0.01340998858228,-0.0328043479726686,
0.071310482121004));
#96087=CARTESIAN_POINT('Ctrl Pts',(0.0134481163985912,-0.0326943950436594,
0.0713838717910524));
#96088=CARTESIAN_POINT('Origin',(-0.00190497382074644,-0.0326396682857095,
0.0787895848319035));
#96089=CARTESIAN_POINT('Ctrl Pts',(0.013600881154459,-0.0331951640388587,
0.0717002271599773));
#96090=CARTESIAN_POINT('Ctrl Pts',(0.0136346218194802,-0.0330855618255041,
0.0717756631180889));
#96091=CARTESIAN_POINT('Ctrl Pts',(0.0136668276753677,-0.0329757224427708,
0.0718518508187994));
#96092=CARTESIAN_POINT('Ctrl Pts',(0.0136974526949243,-0.0328657862078596,
0.0719286947221673));
#96093=CARTESIAN_POINT('Ctrl Pts',(0.0134927623268099,-0.0331951640388587,
0.0716662938260949));
#96094=CARTESIAN_POINT('Ctrl Pts',(0.0135269703548588,-0.0330855618255041,
0.0717402406660782));
#96095=CARTESIAN_POINT('Ctrl Pts',(0.0135596746882157,-0.0329757224427708,
0.0718149478347709));
#96096=CARTESIAN_POINT('Ctrl Pts',(0.0135908287543516,-0.0328657862078596,
0.0718903217194531));
#96097=CARTESIAN_POINT('Ctrl Pts',(0.0133846434991609,-0.0331951640388587,
0.0716323604922125));
#96098=CARTESIAN_POINT('Ctrl Pts',(0.0134193188902374,-0.0330855618255041,
0.0717048182140676));
#96099=CARTESIAN_POINT('Ctrl Pts',(0.0134525217010637,-0.0329757224427708,
0.0717780448507424));
#96100=CARTESIAN_POINT('Ctrl Pts',(0.0134842048137788,-0.0328657862078596,
0.0718519487167388));
#96101=CARTESIAN_POINT('Ctrl Pts',(0.0132765246715118,-0.0331951640388587,
0.0715984271583301));
#96102=CARTESIAN_POINT('Ctrl Pts',(0.013311667425616,-0.0330855618255041,
0.0716693957620569));
#96103=CARTESIAN_POINT('Ctrl Pts',(0.0133453687139117,-0.0329757224427708,
0.071741141866714));
#96104=CARTESIAN_POINT('Ctrl Pts',(0.013377580873206,-0.0328657862078596,
0.0718135757140245));
#96105=CARTESIAN_POINT('Origin',(-0.00207125751478917,-0.0326401908834337,
0.0783383392173187));
#96106=CARTESIAN_POINT('Ctrl Pts',(0.0132623440873654,-0.0332451089994434,
0.0715667255935749));
#96107=CARTESIAN_POINT('Ctrl Pts',(0.0133597738756384,-0.0329451141710259,
0.0717605296262166));
#96108=CARTESIAN_POINT('Ctrl Pts',(0.01344232876415,-0.0326442513127503,
0.0719611218920045));
#96109=CARTESIAN_POINT('Ctrl Pts',(0.0131452262937048,-0.0332451089994434,
0.0713458558980347));
#96110=CARTESIAN_POINT('Ctrl Pts',(0.0132509863188348,-0.0329451141710259,
0.0715352427608197));
#96111=CARTESIAN_POINT('Ctrl Pts',(0.013342180498171,-0.0326442513127503,
0.0717320578729588));
#96112=CARTESIAN_POINT('Ctrl Pts',(0.0133775681197952,-0.0325229783203385,
0.0718135468153923));
#96113=CARTESIAN_POINT('Ctrl Pts',(0.0134097760752639,-0.032413025311208,
0.0718859701381807));
#96114=CARTESIAN_POINT('Ctrl Pts',(0.0134404809763262,-0.0323031222247695,
0.0719590487394742));
#96115=CARTESIAN_POINT('Ctrl Pts',(0.0134696467953236,-0.0321934096636184,
0.0720326876229291));
#96116=CARTESIAN_POINT('Ctrl Pts',(0.0134204867547043,-0.0325229783203385,
0.0717086700618821));
#96117=CARTESIAN_POINT('Ctrl Pts',(0.0134541404339004,-0.032413025311208,
0.0717816850171034));
#96118=CARTESIAN_POINT('Ctrl Pts',(0.013486278600741,-0.0323031222247695,
0.0718553850677491));
#96119=CARTESIAN_POINT('Ctrl Pts',(0.0135168634197456,-0.0321934096636184,
0.0719296743566597));
#96120=CARTESIAN_POINT('Ctrl Pts',(0.0134634053896135,-0.0325229783203385,
0.071603793308372));
#96121=CARTESIAN_POINT('Ctrl Pts',(0.0134985047925368,-0.032413025311208,
0.0716773998960262));
#96122=CARTESIAN_POINT('Ctrl Pts',(0.0135320762251558,-0.0323031222247695,
0.0717517213960239));
#96123=CARTESIAN_POINT('Ctrl Pts',(0.0135640800441676,-0.0321934096636184,
0.0718266610903903));
#96124=CARTESIAN_POINT('Ctrl Pts',(0.0135063240245226,-0.0325229783203385,
0.0714989165548618));
#96125=CARTESIAN_POINT('Ctrl Pts',(0.0135428691511733,-0.032413025311208,
0.0715731147749489));
#96126=CARTESIAN_POINT('Ctrl Pts',(0.0135778738495706,-0.0323031222247695,
0.0716480577242988));
#96127=CARTESIAN_POINT('Ctrl Pts',(0.0136112966685897,-0.0321934096636184,
0.0717236478241209));
#96128=CARTESIAN_POINT('Origin',(-0.00189713877787275,-0.0326393375179539,
0.0787862228185586));
#96129=CARTESIAN_POINT('Ctrl Pts',(0.0137438958601353,-0.0326943950436594,
0.0720489711163758));
#96130=CARTESIAN_POINT('Ctrl Pts',(0.0137728519758994,-0.0325844576448127,
0.0721264268159228));
#96131=CARTESIAN_POINT('Ctrl Pts',(0.0138002082300757,-0.0324744968375319,
0.0722044868570782));
#96132=CARTESIAN_POINT('Ctrl Pts',(0.0138259309517448,-0.0323646534831894,
0.0722830507413142));
#96133=CARTESIAN_POINT('Ctrl Pts',(0.0136381211726919,-0.0326943950436594,
0.0720083159435348));
#96134=CARTESIAN_POINT('Ctrl Pts',(0.0136676375929337,-0.0325844576448127,
0.0720843138696459));
#96135=CARTESIAN_POINT('Ctrl Pts',(0.013695584340386,-0.0324744968375319,
0.0721609276222118));
#96136=CARTESIAN_POINT('Ctrl Pts',(0.0137219269619956,-0.0323646534831894,
0.0722380585453385));
#96137=CARTESIAN_POINT('Ctrl Pts',(0.0135323464852486,-0.0326943950436594,
0.0719676607706938));
#96138=CARTESIAN_POINT('Ctrl Pts',(0.013562423209968,-0.0325844576448127,
0.0720422009233691));
#96139=CARTESIAN_POINT('Ctrl Pts',(0.0135909604506963,-0.0324744968375319,
0.0721173683873454));
#96140=CARTESIAN_POINT('Ctrl Pts',(0.0136179229722464,-0.0323646534831894,
0.0721930663493628));
#96141=CARTESIAN_POINT('Ctrl Pts',(0.0134265717978053,-0.0326943950436594,
0.0719270055978528));
#96142=CARTESIAN_POINT('Ctrl Pts',(0.0134572088270023,-0.0325844576448127,
0.0720000879770922));
#96143=CARTESIAN_POINT('Ctrl Pts',(0.0134863365610066,-0.0324744968375319,
0.0720738091524791));
#96144=CARTESIAN_POINT('Ctrl Pts',(0.0135139189824972,-0.0323646534831894,
0.0721480741533871));
#96145=CARTESIAN_POINT('Origin',(-0.0021060835547087,-0.0326395579068067,
0.0783531415409322));
#96146=CARTESIAN_POINT('Ctrl Pts',(0.0134143940688959,-0.0327445246961877,
0.0718944399853301));
#96147=CARTESIAN_POINT('Ctrl Pts',(0.0134994639046664,-0.0324436878365475,
0.0720939786721626));
#96148=CARTESIAN_POINT('Ctrl Pts',(0.0135692619967624,-0.0321434074463186,
0.07229935829832));
#96149=CARTESIAN_POINT('Ctrl Pts',(0.0133113743499062,-0.0327445246961877,
0.0716666529411436));
#96150=CARTESIAN_POINT('Ctrl Pts',(0.0134050353144047,-0.0324436878365475,
0.0718623061757962));
#96151=CARTESIAN_POINT('Ctrl Pts',(0.0134836927968749,-0.0321434074463186,
0.0720644585068544));
#96152=CARTESIAN_POINT('Ctrl Pts',(0.0135474455252084,-0.0322357242816072,
0.0722363644390754));
#96153=CARTESIAN_POINT('Ctrl Pts',(0.0136083923359294,-0.0319819883628705,
0.0724091010819691));
#96154=CARTESIAN_POINT('Ctrl Pts',(0.0136582239036328,-0.0317295851069886,
0.0725853658725414));
#96155=CARTESIAN_POINT('Ctrl Pts',(0.013459159366366,-0.0322357242816072,
0.0720024722541764));
#96156=CARTESIAN_POINT('Ctrl Pts',(0.0135275553398291,-0.0319819883628705,
0.0721723970974139));
#96157=CARTESIAN_POINT('Ctrl Pts',(0.0135849998964778,-0.0317295851069886,
0.0723463297983264));
#96158=CARTESIAN_POINT('Origin',(-0.00201729889068405,-0.0326371942646779,
0.0783185050430045));
#96159=CARTESIAN_POINT('Origin',(-0.00178455590506462,-0.0326352985531359,
0.0787373464468648));
#96160=CARTESIAN_POINT('Ctrl Pts',(0.0138647305447577,-0.0321934096636183,
0.0724060068739108));
#96161=CARTESIAN_POINT('Ctrl Pts',(0.013888781569152,-0.0320835708272303,
0.072485179025903));
#96162=CARTESIAN_POINT('Ctrl Pts',(0.0139111801794043,-0.0319739230346346,
0.0725648029895292));
#96163=CARTESIAN_POINT('Ctrl Pts',(0.0139319055365407,-0.0318646057455575,
0.0726447746920718));
#96164=CARTESIAN_POINT('Ctrl Pts',(0.0137617171897777,-0.0321934096636183,
0.0723587902088279));
#96165=CARTESIAN_POINT('Ctrl Pts',(0.0137864193687819,-0.0320835708272303,
0.0724365417263711));
#96166=CARTESIAN_POINT('Ctrl Pts',(0.0138094981559041,-0.0319739230346346,
0.072514759355185));
#96167=CARTESIAN_POINT('Ctrl Pts',(0.0138309317038393,-0.0318646057455575,
0.0725933407550711));
#96168=CARTESIAN_POINT('Ctrl Pts',(0.0136587038347977,-0.0321934096636183,
0.0723115735437449));
#96169=CARTESIAN_POINT('Ctrl Pts',(0.0136840571684119,-0.0320835708272303,
0.0723879044268393));
#96170=CARTESIAN_POINT('Ctrl Pts',(0.0137078161324039,-0.0319739230346346,
0.0724647157208408));
#96171=CARTESIAN_POINT('Ctrl Pts',(0.013729957871138,-0.0318646057455575,
0.0725419068180704));
#96172=CARTESIAN_POINT('Ctrl Pts',(0.0135556904798177,-0.0321934096636183,
0.072264356878662));
#96173=CARTESIAN_POINT('Ctrl Pts',(0.0135816949680418,-0.0320835708272303,
0.0723392671273075));
#96174=CARTESIAN_POINT('Ctrl Pts',(0.0136061341089037,-0.0319739230346346,
0.0724146720864966));
#96175=CARTESIAN_POINT('Ctrl Pts',(0.0136289840384366,-0.0318646057455575,
0.0724904728810697));
#96176=CARTESIAN_POINT('Ctrl Pts',(0.0135145310819095,-0.0320218834582287,
0.0721473457067602));
#96177=CARTESIAN_POINT('Ctrl Pts',(0.0135353738717159,-0.0319391099350602,
0.0722034503706395));
#96178=CARTESIAN_POINT('Ctrl Pts',(0.0135553279512123,-0.0318564869454902,
0.0722598465052138));
#96179=CARTESIAN_POINT('Ctrl Pts',(0.0135743826213311,-0.0317740741446512,
0.0723164916765391));
#96180=CARTESIAN_POINT('Ctrl Pts',(0.0135361501261414,-0.0320218834582287,
0.0721027425120963));
#96181=CARTESIAN_POINT('Ctrl Pts',(0.0135574571273767,-0.0319391099350602,
0.0721590721779623));
#96182=CARTESIAN_POINT('Ctrl Pts',(0.0135778716236106,-0.0318564869454902,
0.0722157004269268));
#96183=CARTESIAN_POINT('Ctrl Pts',(0.0135973825962061,-0.0317740741446512,
0.072272584624674));
#96184=CARTESIAN_POINT('Ctrl Pts',(0.0135577691703733,-0.0320218834582287,
0.0720581393174323));
#96185=CARTESIAN_POINT('Ctrl Pts',(0.0135795403830375,-0.0319391099350602,
0.072114693985285));
#96186=CARTESIAN_POINT('Ctrl Pts',(0.0136004152960088,-0.0318564869454902,
0.0721715543486399));
#96187=CARTESIAN_POINT('Ctrl Pts',(0.0136203825710811,-0.0317740741446512,
0.0722286775728089));
#96188=CARTESIAN_POINT('Ctrl Pts',(0.0135793882146052,-0.0320218834582287,
0.0720135361227683));
#96189=CARTESIAN_POINT('Ctrl Pts',(0.0136016236386984,-0.0319391099350602,
0.0720703157926078));
#96190=CARTESIAN_POINT('Ctrl Pts',(0.013622958968407,-0.0318564869454902,
0.0721274082703529));
#96191=CARTESIAN_POINT('Ctrl Pts',(0.0136433825459561,-0.0317740741446512,
0.0721847705209438));
#96192=CARTESIAN_POINT('Origin',(0.0190833712827904,-0.0391228853390731,
0.0690737784410806));
#96193=CARTESIAN_POINT('Ctrl Pts',(0.0117449661544827,-0.0352722978779542,
0.0696810861207133));
#96194=CARTESIAN_POINT('Ctrl Pts',(0.0117594251069067,-0.0352466642097181,
0.0696932529351193));
#96195=CARTESIAN_POINT('Ctrl Pts',(0.011773921656746,-0.0352210183808283,
0.0697053489218047));
#96196=CARTESIAN_POINT('Ctrl Pts',(0.0117884566567382,-0.0351953608940152,
0.0697173740987455));
#96197=CARTESIAN_POINT('Origin',(0.0150362787244069,-0.0352456003065003,
0.0660510716909158));
#96198=CARTESIAN_POINT('Ctrl Pts',(0.0118827372491286,-0.035024121149334,
0.0697989613852351));
#96199=CARTESIAN_POINT('Ctrl Pts',(0.0119426710193492,-0.0349144232867421,
0.0698507394475655));
#96200=CARTESIAN_POINT('Ctrl Pts',(0.0120015703733199,-0.0348045283677512,
0.0699037873753614));
#96201=CARTESIAN_POINT('Ctrl Pts',(0.0120593573399695,-0.0346945769586886,
0.069958040028368));
#96202=CARTESIAN_POINT('Ctrl Pts',(0.0118769168623412,-0.035024121149334,
0.0696857921981716));
#96203=CARTESIAN_POINT('Ctrl Pts',(0.0119384094916422,-0.0349144232867421,
0.0697374900870641));
#96204=CARTESIAN_POINT('Ctrl Pts',(0.0119988702949877,-0.0348045283677512,
0.0697904900161641));
#96205=CARTESIAN_POINT('Ctrl Pts',(0.0120582193035762,-0.0346945769586886,
0.0698447269811222));
#96206=CARTESIAN_POINT('Ctrl Pts',(0.0118710964755538,-0.035024121149334,
0.0695726230111081));
#96207=CARTESIAN_POINT('Ctrl Pts',(0.0119341479639352,-0.0349144232867422,
0.0696242407265627));
#96208=CARTESIAN_POINT('Ctrl Pts',(0.0119961702166554,-0.0348045283677512,
0.0696771926569668));
#96209=CARTESIAN_POINT('Ctrl Pts',(0.0120570812671828,-0.0346945769586886,
0.0697314139338764));
#96210=CARTESIAN_POINT('Ctrl Pts',(0.0118652760887664,-0.035024121149334,
0.0694594538240447));
#96211=CARTESIAN_POINT('Ctrl Pts',(0.0119298864362281,-0.0349144232867422,
0.0695109913660613));
#96212=CARTESIAN_POINT('Ctrl Pts',(0.0119934701383231,-0.0348045283677512,
0.0695638952977694));
#96213=CARTESIAN_POINT('Ctrl Pts',(0.0120559432307895,-0.0346945769586886,
0.0696181008866307));
#96214=CARTESIAN_POINT('Origin',(0.000437479737908236,-0.0345629067945187,
0.0820739349628899));
#96215=CARTESIAN_POINT('Ctrl Pts',(0.0122209024820182,-0.0351970973651652,
0.0698617454465175));
#96216=CARTESIAN_POINT('Ctrl Pts',(0.0122803104372427,-0.0350869349321816,
0.0699185054955392));
#96217=CARTESIAN_POINT('Ctrl Pts',(0.0123385875953615,-0.0349764985129772,
0.0699765476223919));
#96218=CARTESIAN_POINT('Ctrl Pts',(0.0123956540301704,-0.0348659306849697,
0.070035801076154));
#96219=CARTESIAN_POINT('Ctrl Pts',(0.0121389001123545,-0.0351970973651652,
0.0698677522775772));
#96220=CARTESIAN_POINT('Ctrl Pts',(0.0121982248510754,-0.0350869349321816,
0.0699233762949));
#96221=CARTESIAN_POINT('Ctrl Pts',(0.0122564423412243,-0.0349764985129772,
0.0699802797189535));
#96222=CARTESIAN_POINT('Ctrl Pts',(0.0123134728207393,-0.0348659306849697,
0.0700383932694884));
#96223=CARTESIAN_POINT('Ctrl Pts',(0.0120568977426908,-0.0351970973651652,
0.0698737591086368));
#96224=CARTESIAN_POINT('Ctrl Pts',(0.012116139264908,-0.0350869349321816,
0.0699282470942608));
#96225=CARTESIAN_POINT('Ctrl Pts',(0.0121742970870872,-0.0349764985129772,
0.0699840118155151));
#96226=CARTESIAN_POINT('Ctrl Pts',(0.0122312916113082,-0.0348659306849698,
0.0700409854628228));
#96227=CARTESIAN_POINT('Ctrl Pts',(0.0119748953730271,-0.0351970973651652,
0.0698797659396964));
#96228=CARTESIAN_POINT('Ctrl Pts',(0.0120340536787406,-0.0350869349321816,
0.0699331178936216));
#96229=CARTESIAN_POINT('Ctrl Pts',(0.0120921518329501,-0.0349764985129772,
0.0699877439120767));
#96230=CARTESIAN_POINT('Ctrl Pts',(0.0121491104018771,-0.0348659306849698,
0.0700435776561572));
#96231=CARTESIAN_POINT('Origin',(0.000125454551840935,-0.0345637187966511,
0.0817079217938938));
#96232=CARTESIAN_POINT('Ctrl Pts',(0.0119505339817063,-0.0352450361861253,
0.0698565054153448));
#96233=CARTESIAN_POINT('Ctrl Pts',(0.0121124657829775,-0.0349452761023765,
0.0700008337236558));
#96234=CARTESIAN_POINT('Ctrl Pts',(0.0122630661546245,-0.0346444289983475,
0.0701569493759862));
#96235=CARTESIAN_POINT('Ctrl Pts',(0.0117603332233854,-0.0352450361861253,
0.0696942597018911));
#96236=CARTESIAN_POINT('Ctrl Pts',(0.0119283842219934,-0.0349452761023765,
0.0698314144710741));
#96237=CARTESIAN_POINT('Ctrl Pts',(0.0120856267472876,-0.0346444289983475,
0.0699808378865146));
#96238=CARTESIAN_POINT('Ctrl Pts',(0.0121485231283809,-0.0345231616327822,
0.0700435731874319));
#96239=CARTESIAN_POINT('Ctrl Pts',(0.0122051244406053,-0.0344132092796975,
0.0700990485748423));
#96240=CARTESIAN_POINT('Ctrl Pts',(0.0122605753678319,-0.0343032738558974,
0.0701556918534746));
#96241=CARTESIAN_POINT('Ctrl Pts',(0.012314806729835,-0.034193496108874,
0.0702134286370508));
#96242=CARTESIAN_POINT('Ctrl Pts',(0.012149820160417,-0.0345231616327822,
0.0699302618735825));
#96243=CARTESIAN_POINT('Ctrl Pts',(0.0122079833095732,-0.0344132092796975,
0.0699857551387534));
#96244=CARTESIAN_POINT('Ctrl Pts',(0.0122649956233607,-0.0343032738558974,
0.0700424485995888));
#96245=CARTESIAN_POINT('Ctrl Pts',(0.0123207859228837,-0.034193496108874,
0.0701002677542826));
#96246=CARTESIAN_POINT('Ctrl Pts',(0.012151117192453,-0.0345231616327822,
0.069816950559733));
#96247=CARTESIAN_POINT('Ctrl Pts',(0.0122108421785411,-0.0344132092796975,
0.0698724617026645));
#96248=CARTESIAN_POINT('Ctrl Pts',(0.0122694158788894,-0.0343032738558974,
0.069929205345703));
#96249=CARTESIAN_POINT('Ctrl Pts',(0.0123267651159325,-0.034193496108874,
0.0699871068715144));
#96250=CARTESIAN_POINT('Ctrl Pts',(0.0121524142244891,-0.0345231616327822,
0.0697036392458835));
#96251=CARTESIAN_POINT('Ctrl Pts',(0.012213701047509,-0.0344132092796975,
0.0697591682665756));
#96252=CARTESIAN_POINT('Ctrl Pts',(0.0122738361344182,-0.0343032738558974,
0.0698159620918172));
#96253=CARTESIAN_POINT('Ctrl Pts',(0.0123327443089813,-0.034193496108874,
0.0698739459887462));
#96254=CARTESIAN_POINT('Origin',(0.000429234047500226,-0.0345625596230095,
0.0820827953746281));
#96255=CARTESIAN_POINT('Ctrl Pts',(0.0125757914107657,-0.0346945769586885,
0.0701276109181229));
#96256=CARTESIAN_POINT('Ctrl Pts',(0.0126312219653004,-0.0345846629178476,
0.0701889618552662));
#96257=CARTESIAN_POINT('Ctrl Pts',(0.0126853932753282,-0.034474692505516,
0.0702514695524017));
#96258=CARTESIAN_POINT('Ctrl Pts',(0.0127382362610932,-0.0343648066260528,
0.0703150536308093));
#96259=CARTESIAN_POINT('Ctrl Pts',(0.0124624784527354,-0.0346945769586885,
0.0701287489536201));
#96260=CARTESIAN_POINT('Ctrl Pts',(0.0125178933245658,-0.0345846629178476,
0.0701885383809315));
#96261=CARTESIAN_POINT('Ctrl Pts',(0.0125720812405926,-0.034474692505516,
0.0702494839772133));
#96262=CARTESIAN_POINT('Ctrl Pts',(0.0126249730915163,-0.0343648066260528,
0.0703115073652014));
#96263=CARTESIAN_POINT('Ctrl Pts',(0.0123491654947052,-0.0346945769586885,
0.0701298869891174));
#96264=CARTESIAN_POINT('Ctrl Pts',(0.0124045646838312,-0.0345846629178476,
0.0701881149065968));
#96265=CARTESIAN_POINT('Ctrl Pts',(0.012458769205857,-0.034474692505516,
0.0702474984020249));
#96266=CARTESIAN_POINT('Ctrl Pts',(0.0125117099219394,-0.0343648066260528,
0.0703079610995936));
#96267=CARTESIAN_POINT('Ctrl Pts',(0.0122358525366749,-0.0346945769586885,
0.0701310250246147));
#96268=CARTESIAN_POINT('Ctrl Pts',(0.0122912360430966,-0.0345846629178476,
0.070187691432262));
#96269=CARTESIAN_POINT('Ctrl Pts',(0.0123454571711213,-0.034474692505516,
0.0702455128268366));
#96270=CARTESIAN_POINT('Ctrl Pts',(0.0123984467523625,-0.0343648066260528,
0.0703044148339857));
#96271=CARTESIAN_POINT('Origin',(8.35237049665021E-5,-0.0345626446730908,
0.0817486149715776));
#96272=CARTESIAN_POINT('Ctrl Pts',(0.0122378800854608,-0.0346945769586887,
0.0701310046613435));
#96273=CARTESIAN_POINT('Ctrl Pts',(0.0123220595519455,-0.0345275153362892,
0.0702171760888924));
#96274=CARTESIAN_POINT('Ctrl Pts',(0.012403550779471,-0.034360323596516,
0.0703060171715252));
#96275=CARTESIAN_POINT('Ctrl Pts',(0.0124821166583466,-0.0341934961088741,
0.0703972615746474));
#96276=CARTESIAN_POINT('Ctrl Pts',(0.0121780086263968,-0.0346945769586887,
0.0700723238576612));
#96277=CARTESIAN_POINT('Ctrl Pts',(0.0122634171858091,-0.0345275153362892,
0.0701572412535287));
#96278=CARTESIAN_POINT('Ctrl Pts',(0.0123461772623108,-0.034360323596516,
0.0702448666339647));
#96279=CARTESIAN_POINT('Ctrl Pts',(0.0124260479400804,-0.0341934961088741,
0.0703349372041072));
#96280=CARTESIAN_POINT('Ctrl Pts',(0.0121181371673327,-0.0346945769586887,
0.0700136430539788));
#96281=CARTESIAN_POINT('Ctrl Pts',(0.0122047748196728,-0.0345275153362892,
0.070097306418165));
#96282=CARTESIAN_POINT('Ctrl Pts',(0.0122888037451505,-0.034360323596516,
0.0701837160964042));
#96283=CARTESIAN_POINT('Ctrl Pts',(0.0123699792218141,-0.0341934961088741,
0.070272612833567));
#96284=CARTESIAN_POINT('Ctrl Pts',(0.0120582657082687,-0.0346945769586887,
0.0699549622502964));
#96285=CARTESIAN_POINT('Ctrl Pts',(0.0121461324535364,-0.0345275153362892,
0.0700373715828014));
#96286=CARTESIAN_POINT('Ctrl Pts',(0.0122314302279902,-0.034360323596516,
0.0701225655588437));
#96287=CARTESIAN_POINT('Ctrl Pts',(0.0123139105035478,-0.0341934961088741,
0.0702102884630267));
#96288=CARTESIAN_POINT('Ctrl Pts',(0.0123984252348696,-0.0340223579322365,
0.0703043917482794));
#96289=CARTESIAN_POINT('Ctrl Pts',(0.0124514662024277,-0.0339125849573554,
0.0703633502245619));
#96290=CARTESIAN_POINT('Ctrl Pts',(0.0125032495952535,-0.0338030433565221,
0.0704233650961839));
#96291=CARTESIAN_POINT('Ctrl Pts',(0.0125537159945839,-0.0336938721132327,
0.0704843537439186));
#96292=CARTESIAN_POINT('Ctrl Pts',(0.0124068345799588,-0.0340223579322365,
0.0701913852761399));
#96293=CARTESIAN_POINT('Ctrl Pts',(0.0124614342015009,-0.0339125849573554,
0.0702504597392235));
#96294=CARTESIAN_POINT('Ctrl Pts',(0.0125147727524054,-0.0338030433565221,
0.0703106227766599));
#96295=CARTESIAN_POINT('Ctrl Pts',(0.0125667888419205,-0.0336938721132327,
0.0703717914034456));
#96296=CARTESIAN_POINT('Ctrl Pts',(0.0124152439250479,-0.0340223579322365,
0.0700783788040003));
#96297=CARTESIAN_POINT('Ctrl Pts',(0.012471402200574,-0.0339125849573554,
0.0701375692538852));
#96298=CARTESIAN_POINT('Ctrl Pts',(0.0125262959095572,-0.0338030433565221,
0.0701978804571359));
#96299=CARTESIAN_POINT('Ctrl Pts',(0.0125798616892571,-0.0336938721132327,
0.0702592290629725));
#96300=CARTESIAN_POINT('Ctrl Pts',(0.012423653270137,-0.0340223579322365,
0.0699653723318607));
#96301=CARTESIAN_POINT('Ctrl Pts',(0.0124813701996472,-0.0339125849573554,
0.0700246787685469));
#96302=CARTESIAN_POINT('Ctrl Pts',(0.012537819066709,-0.0338030433565221,
0.0700851381376119));
#96303=CARTESIAN_POINT('Ctrl Pts',(0.0125929345365937,-0.0336938721132327,
0.0701466667224994));
#96304=CARTESIAN_POINT('Origin',(0.000514778422947674,-0.0345589643415595,
0.0819983262209085));
#96305=CARTESIAN_POINT('Ctrl Pts',(0.0128195742877403,-0.034193496108874,
0.0704150921558745));
#96306=CARTESIAN_POINT('Ctrl Pts',(0.0128710764551861,-0.0340836138581106,
0.0704798443481219));
#96307=CARTESIAN_POINT('Ctrl Pts',(0.0129212140001739,-0.0339738896643499,
0.0705456312003391));
#96308=CARTESIAN_POINT('Ctrl Pts',(0.0129699283971121,-0.0338644633294062,
0.0706123642118589));
#96309=CARTESIAN_POINT('Ctrl Pts',(0.0127064133031482,-0.034193496108874,
0.0704091129574456));
#96310=CARTESIAN_POINT('Ctrl Pts',(0.0127579979201997,-0.0340836138581106,
0.0704723047267267));
#96311=CARTESIAN_POINT('Ctrl Pts',(0.0128082501649112,-0.0339738896643499,
0.0705365336108195));
#96312=CARTESIAN_POINT('Ctrl Pts',(0.0128571112312219,-0.0338644633294062,
0.0706017130932228));
#96313=CARTESIAN_POINT('Ctrl Pts',(0.0125932523185562,-0.034193496108874,
0.0704031337590166));
#96314=CARTESIAN_POINT('Ctrl Pts',(0.0126449193852132,-0.0340836138581106,
0.0704647651053315));
#96315=CARTESIAN_POINT('Ctrl Pts',(0.0126952863296485,-0.0339738896643499,
0.0705274360212999));
#96316=CARTESIAN_POINT('Ctrl Pts',(0.0127442940653318,-0.0338644633294062,
0.0705910619745866));
#96317=CARTESIAN_POINT('Ctrl Pts',(0.0124800913339641,-0.034193496108874,
0.0703971545605877));
#96318=CARTESIAN_POINT('Ctrl Pts',(0.0125318408502268,-0.0340836138581106,
0.0704572254839363));
#96319=CARTESIAN_POINT('Ctrl Pts',(0.0125823224943859,-0.0339738896643499,
0.0705183384317803));
#96320=CARTESIAN_POINT('Ctrl Pts',(0.0126314768994416,-0.0338644633294062,
0.0705804108559505));
#96321=CARTESIAN_POINT('Origin',(0.000139010950174352,-0.0345610621862704,
0.081697745419754));
#96322=CARTESIAN_POINT('Ctrl Pts',(0.0124584248656429,-0.0342436276873901,
0.0703699209133347));
#96323=CARTESIAN_POINT('Ctrl Pts',(0.0126009928986574,-0.0339430054201861,
0.0705334046567898));
#96324=CARTESIAN_POINT('Ctrl Pts',(0.0127308416454257,-0.0336441434784164,
0.0707071627684692));
#96325=CARTESIAN_POINT('Ctrl Pts',(0.0122900561545809,-0.0342436276873901,
0.0701851183778129));
#96326=CARTESIAN_POINT('Ctrl Pts',(0.0124395941301235,-0.0339430054201861,
0.0703422519906471));
#96327=CARTESIAN_POINT('Ctrl Pts',(0.0125768713364009,-0.0336441434784164,
0.0705102030163908));
#96328=CARTESIAN_POINT('Ctrl Pts',(0.0126314595844677,-0.0335235895815127,
0.0705803891944784));
#96329=CARTESIAN_POINT('Ctrl Pts',(0.0126806023051219,-0.0334144449262719,
0.0706424462485696));
#96330=CARTESIAN_POINT('Ctrl Pts',(0.0127285194327741,-0.0333049234473133,
0.0707055898503223));
#96331=CARTESIAN_POINT('Ctrl Pts',(0.0127751423822346,-0.0331951640388588,
0.0707697448086749));
#96332=CARTESIAN_POINT('Ctrl Pts',(0.0126469481174946,-0.0335235895815127,
0.0704681337811082));
#96333=CARTESIAN_POINT('Ctrl Pts',(0.0126976362549244,-0.0334144449262719,
0.0705304040653507));
#96334=CARTESIAN_POINT('Ctrl Pts',(0.0127470961696743,-0.0333049234473133,
0.0705937930693777));
#96335=CARTESIAN_POINT('Ctrl Pts',(0.012795257275379,-0.0331951640388588,
0.0706582254670339));
#96336=CARTESIAN_POINT('Ctrl Pts',(0.0126624366505214,-0.0335235895815127,
0.070355878367738));
#96337=CARTESIAN_POINT('Ctrl Pts',(0.0127146702047269,-0.0334144449262719,
0.0704183618821317));
#96338=CARTESIAN_POINT('Ctrl Pts',(0.0127656729065746,-0.0333049234473133,
0.0704819962884332));
#96339=CARTESIAN_POINT('Ctrl Pts',(0.0128153721685233,-0.0331951640388588,
0.0705467061253931));
#96340=CARTESIAN_POINT('Ctrl Pts',(0.0126779251835483,-0.0335235895815127,
0.0702436229543678));
#96341=CARTESIAN_POINT('Ctrl Pts',(0.0127317041545293,-0.0334144449262719,
0.0703063196989127));
#96342=CARTESIAN_POINT('Ctrl Pts',(0.0127842496434748,-0.0333049234473133,
0.0703701995074886));
#96343=CARTESIAN_POINT('Ctrl Pts',(0.0128354870616677,-0.0331951640388588,
0.0704351867837521));
#96344=CARTESIAN_POINT('Origin',(-0.00114102305421436,-0.0326434571769475,
0.0799420498962871));
#96345=CARTESIAN_POINT('Ctrl Pts',(0.0130468390514737,-0.0336938721132369,
0.0707175472757866));
#96346=CARTESIAN_POINT('Ctrl Pts',(0.0130669303362767,-0.0336474569764948,
0.0707463635612215));
#96347=CARTESIAN_POINT('Ctrl Pts',(0.0130866829134076,-0.033601104548885,
0.0707754130660018));
#96348=CARTESIAN_POINT('Ctrl Pts',(0.0131366918951498,-0.033483750864316,
0.0708489597300422));
#96349=CARTESIAN_POINT('Ctrl Pts',(0.0131844995765855,-0.0333660264760404,
0.0709239559675618));
#96350=CARTESIAN_POINT('Ctrl Pts',(0.01270915287623,-0.0336938721132369,
0.0706783288320508));
#96351=CARTESIAN_POINT('Ctrl Pts',(0.0127294737195982,-0.0336474569764948,
0.0707051685282458));
#96352=CARTESIAN_POINT('Ctrl Pts',(0.0127494789780375,-0.033601104548885,
0.0707322442664963));
#96353=CARTESIAN_POINT('Ctrl Pts',(0.0128001276907301,-0.033483750864316,
0.0708007938076956));
#96354=CARTESIAN_POINT('Ctrl Pts',(0.0128487228972976,-0.0333660264760404,
0.0708708140732955));
#96355=CARTESIAN_POINT('Ctrl Pts',(0.0127091528762419,-0.0336938721132426,
0.0706783288320632));
#96356=CARTESIAN_POINT('Ctrl Pts',(0.0127294737196091,-0.0336474569765026,
0.070705168528257));
#96357=CARTESIAN_POINT('Ctrl Pts',(0.0127494789780475,-0.0336011045488949,
0.0707322442665063));
#96358=CARTESIAN_POINT('Ctrl Pts',(0.012799705855949,-0.0334847282606778,
0.0708002228833947));
#96359=CARTESIAN_POINT('Ctrl Pts',(0.0128479134659113,-0.0333679869945434,
0.070869648080258));
#96360=CARTESIAN_POINT('Ctrl Pts',(0.0127091528762275,-0.0336938721132427,
0.0706783288320474));
#96361=CARTESIAN_POINT('Ctrl Pts',(0.0127818292049813,-0.0335278710435083,
0.0707743194633896));
#96362=CARTESIAN_POINT('Ctrl Pts',(0.0128514697251298,-0.033362046922432,
0.070872555436225));
#96363=CARTESIAN_POINT('Ctrl Pts',(0.0129180927308868,-0.0331951640388602,
0.0709730971895022));
#96364=CARTESIAN_POINT('Ctrl Pts',(0.0126571081708501,-0.0336938721132427,
0.0706126068534904));
#96365=CARTESIAN_POINT('Ctrl Pts',(0.0127311603304038,-0.0335278710435083,
0.0707075079755056));
#96366=CARTESIAN_POINT('Ctrl Pts',(0.0128022103640674,-0.033362046922432,
0.0708046979679969));
#96367=CARTESIAN_POINT('Ctrl Pts',(0.0128702774410251,-0.0331951640388602,
0.0709042369841676));
#96368=CARTESIAN_POINT('Ctrl Pts',(0.0126050634654727,-0.0336938721132427,
0.0705468848749333));
#96369=CARTESIAN_POINT('Ctrl Pts',(0.0126804914558263,-0.0335278710435083,
0.0706406964876216));
#96370=CARTESIAN_POINT('Ctrl Pts',(0.0127529510030049,-0.033362046922432,
0.0707368404997688));
#96371=CARTESIAN_POINT('Ctrl Pts',(0.0128224621511635,-0.0331951640388602,
0.070835376778833));
#96372=CARTESIAN_POINT('Ctrl Pts',(0.0125530187600953,-0.0336938721132427,
0.0704811628963763));
#96373=CARTESIAN_POINT('Ctrl Pts',(0.0126298225812489,-0.0335278710435083,
0.0705738849997375));
#96374=CARTESIAN_POINT('Ctrl Pts',(0.0127036916419425,-0.033362046922432,
0.0706689830315406));
#96375=CARTESIAN_POINT('Ctrl Pts',(0.0127746468613019,-0.0331951640388602,
0.0707665165734984));
#96376=CARTESIAN_POINT('Ctrl Pts',(0.0128467020004684,-0.0330240426238155,
0.0708704711812222));
#96377=CARTESIAN_POINT('Ctrl Pts',(0.0128918807050369,-0.0329142774063509,
0.070935534002886));
#96378=CARTESIAN_POINT('Ctrl Pts',(0.0129357369025695,-0.0328043479726686,
0.0710015632307633));
#96379=CARTESIAN_POINT('Ctrl Pts',(0.0129782120804626,-0.0326943950436594,
0.0710684758237667));
#96380=CARTESIAN_POINT('Ctrl Pts',(0.0128692084963612,-0.0330240426238155,
0.0707594099655474));
#96381=CARTESIAN_POINT('Ctrl Pts',(0.0129159171773774,-0.0329142774063509,
0.0708247828361192));
#96382=CARTESIAN_POINT('Ctrl Pts',(0.0129612977045297,-0.0328043479726686,
0.070891153896362));
#96383=CARTESIAN_POINT('Ctrl Pts',(0.0130052896003746,-0.0326943950436594,
0.0709584397210552));
#96384=CARTESIAN_POINT('Ctrl Pts',(0.0128917149922541,-0.0330240426238155,
0.0706483487498726));
#96385=CARTESIAN_POINT('Ctrl Pts',(0.0129399536497178,-0.0329142774063509,
0.0707140316693524));
#96386=CARTESIAN_POINT('Ctrl Pts',(0.0129868585064898,-0.0328043479726686,
0.0707807445619608));
#96387=CARTESIAN_POINT('Ctrl Pts',(0.0130323671202866,-0.0326943950436594,
0.0708484036183436));
#96388=CARTESIAN_POINT('Ctrl Pts',(0.0129142214881469,-0.0330240426238155,
0.0705372875341979));
#96389=CARTESIAN_POINT('Ctrl Pts',(0.0129639901220583,-0.0329142774063509,
0.0706032805025856));
#96390=CARTESIAN_POINT('Ctrl Pts',(0.0130124193084499,-0.0328043479726686,
0.0706703352275596));
#96391=CARTESIAN_POINT('Ctrl Pts',(0.0130594446401986,-0.0326943950436594,
0.0707383675156321));
#96392=CARTESIAN_POINT('Origin',(-0.0012443999145456,-0.0326396682858909,
0.0800099367397309));
#96393=CARTESIAN_POINT('Ctrl Pts',(0.0132506546416792,-0.0331951640388587,
0.0710330818271546));
#96394=CARTESIAN_POINT('Ctrl Pts',(0.0132935838840361,-0.0330855618255041,
0.0711036941235551));
#96395=CARTESIAN_POINT('Ctrl Pts',(0.0133350846380184,-0.0329757224427708,
0.0711752445974313));
#96396=CARTESIAN_POINT('Ctrl Pts',(0.0133750992650374,-0.0328657862078596,
0.07124764423094));
#96397=CARTESIAN_POINT('Ctrl Pts',(0.0131391353888191,-0.0331951640388587,
0.0710129669500237));
#96398=CARTESIAN_POINT('Ctrl Pts',(0.0131823416729163,-0.0330855618255041,
0.0710820432943177));
#96399=CARTESIAN_POINT('Ctrl Pts',(0.0132241514138591,-0.0329757224427708,
0.0711520624348202));
#96400=CARTESIAN_POINT('Ctrl Pts',(0.0132645066735717,-0.0328657862078596,
0.071222937334061));
#96401=CARTESIAN_POINT('Ctrl Pts',(0.0130276161359589,-0.0331951640388587,
0.0709928520728929));
#96402=CARTESIAN_POINT('Ctrl Pts',(0.0130710994617965,-0.0330855618255041,
0.0710603924650804));
#96403=CARTESIAN_POINT('Ctrl Pts',(0.0131132181896998,-0.0329757224427708,
0.0711288802722091));
#96404=CARTESIAN_POINT('Ctrl Pts',(0.013153914082106,-0.0328657862078596,
0.0711982304371821));
#96405=CARTESIAN_POINT('Ctrl Pts',(0.0129160968830987,-0.0331951640388587,
0.070972737195762));
#96406=CARTESIAN_POINT('Ctrl Pts',(0.0129598572506768,-0.0330855618255041,
0.071038741635843));
#96407=CARTESIAN_POINT('Ctrl Pts',(0.0130022849655405,-0.0329757224427708,
0.071105698109598));
#96408=CARTESIAN_POINT('Ctrl Pts',(0.0130433214906403,-0.0328657862078596,
0.0711735235403031));
#96409=CARTESIAN_POINT('Origin',(-0.00146592848484389,-0.0326401908829356,
0.0795830902040864));
#96410=CARTESIAN_POINT('Ctrl Pts',(0.012898054857474,-0.0332451089994433,
0.0709430629057787));
#96411=CARTESIAN_POINT('Ctrl Pts',(0.0130190064688544,-0.0329451141710259,
0.0711231275453268));
#96412=CARTESIAN_POINT('Ctrl Pts',(0.0131260512647113,-0.0326442513127504,
0.0713117912100612));
#96413=CARTESIAN_POINT('Ctrl Pts',(0.0127541782594593,-0.0332451089994433,
0.0707386135855457));
#96414=CARTESIAN_POINT('Ctrl Pts',(0.0128828408031097,-0.0329451141710259,
0.0709132518304192));
#96415=CARTESIAN_POINT('Ctrl Pts',(0.0129979833635221,-0.0326442513127504,
0.0710970853352348));
#96416=CARTESIAN_POINT('Ctrl Pts',(0.013043305215835,-0.0325229783203385,
0.0711734964679713));
#96417=CARTESIAN_POINT('Ctrl Pts',(0.0130843362511853,-0.0324130253112079,
0.0712413119840224));
#96418=CARTESIAN_POINT('Ctrl Pts',(0.0131239582123361,-0.0323031222247695,
0.0713099659941807));
#96419=CARTESIAN_POINT('Ctrl Pts',(0.0131621234495188,-0.0321934096636184,
0.0713793687666401));
#96420=CARTESIAN_POINT('Ctrl Pts',(0.0130727408818455,-0.0325229783203385,
0.0710640675676944));
#96421=CARTESIAN_POINT('Ctrl Pts',(0.0131152803921657,-0.0324130253112079,
0.0711322888537504));
#96422=CARTESIAN_POINT('Ctrl Pts',(0.0131564022056229,-0.0323031222247695,
0.0712013797771125));
#96423=CARTESIAN_POINT('Ctrl Pts',(0.0131960567709927,-0.0321934096636184,
0.0712712499785271));
#96424=CARTESIAN_POINT('Ctrl Pts',(0.0131021765478561,-0.0325229783203385,
0.0709546386674175));
#96425=CARTESIAN_POINT('Ctrl Pts',(0.013146224533146,-0.0324130253112079,
0.0710232657234783));
#96426=CARTESIAN_POINT('Ctrl Pts',(0.0131888461989096,-0.0323031222247695,
0.0710927935600443));
#96427=CARTESIAN_POINT('Ctrl Pts',(0.0132299900924667,-0.0321934096636184,
0.071163131190414));
#96428=CARTESIAN_POINT('Ctrl Pts',(0.0131316122138666,-0.0325229783203385,
0.0708452097671406));
#96429=CARTESIAN_POINT('Ctrl Pts',(0.0131771686741264,-0.0324130253112079,
0.0709142425932062));
#96430=CARTESIAN_POINT('Ctrl Pts',(0.0132212901921964,-0.0323031222247695,
0.0709842073429761));
#96431=CARTESIAN_POINT('Ctrl Pts',(0.0132639234139407,-0.0321934096636184,
0.0710550124023009));
#96432=CARTESIAN_POINT('Origin',(-0.00123704802509541,-0.0326393375182704,
0.0800056192456978));
#96433=CARTESIAN_POINT('Ctrl Pts',(0.0134362508414271,-0.0326943950436593,
0.0713611513377825));
#96434=CARTESIAN_POINT('Ctrl Pts',(0.0134746864028517,-0.0325844576448127,
0.0714343671123835));
#96435=CARTESIAN_POINT('Ctrl Pts',(0.0135116104621632,-0.0324744968375319,
0.0715083829790049));
#96436=CARTESIAN_POINT('Ctrl Pts',(0.0135469770181415,-0.0323646534831895,
0.071583103451665));
#96437=CARTESIAN_POINT('Ctrl Pts',(0.0133262147747145,-0.0326943950436593,
0.0713340738267291));
#96438=CARTESIAN_POINT('Ctrl Pts',(0.0133650235149901,-0.0325844576448127,
0.0714057730981012));
#96439=CARTESIAN_POINT('Ctrl Pts',(0.0134023521433361,-0.0324744968375319,
0.0714782800721189));
#96440=CARTESIAN_POINT('Ctrl Pts',(0.0134381541135094,-0.0323646534831895,
0.071551501188932));
#96441=CARTESIAN_POINT('Ctrl Pts',(0.0132161787080019,-0.0326943950436593,
0.0713069963156756));
#96442=CARTESIAN_POINT('Ctrl Pts',(0.0132553606271285,-0.0325844576448127,
0.0713771790838189));
#96443=CARTESIAN_POINT('Ctrl Pts',(0.0132930938245091,-0.0324744968375319,
0.0714481771652329));
#96444=CARTESIAN_POINT('Ctrl Pts',(0.0133293312088772,-0.0323646534831895,
0.071519898926199));
#96445=CARTESIAN_POINT('Ctrl Pts',(0.0131061426412893,-0.0326943950436593,
0.0712799188046222));
#96446=CARTESIAN_POINT('Ctrl Pts',(0.0131456977392669,-0.0325844576448127,
0.0713485850695366));
#96447=CARTESIAN_POINT('Ctrl Pts',(0.013183835505682,-0.0324744968375319,
0.0714180742583469));
#96448=CARTESIAN_POINT('Ctrl Pts',(0.0132205083042451,-0.0323646534831895,
0.071488296663466));
#96449=CARTESIAN_POINT('Origin',(-0.00149862468699762,-0.0326395579068937,
0.0796021406675311));
#96450=CARTESIAN_POINT('Ctrl Pts',(0.0130899793838892,-0.0327445246961878,
0.0712491362558227));
#96451=CARTESIAN_POINT('Ctrl Pts',(0.0131993872474374,-0.0324436878365475,
0.0714364394429143));
#96452=CARTESIAN_POINT('Ctrl Pts',(0.0132943758533842,-0.0321434074463186,
0.0716314515687966));
#96453=CARTESIAN_POINT('Ctrl Pts',(0.0129592227193422,-0.0327445246961878,
0.0710360571750181));
#96454=CARTESIAN_POINT('Ctrl Pts',(0.0130766669917168,-0.0324436878365475,
0.0712184287939373));
#96455=CARTESIAN_POINT('Ctrl Pts',(0.0131800406417681,-0.0321434074463186,
0.0714091286968632));
#96456=CARTESIAN_POINT('Ctrl Pts',(0.0132648361871507,-0.0322357242816073,
0.0715716887638722));
#96457=CARTESIAN_POINT('Ctrl Pts',(0.0133469520560742,-0.0319819883628706,
0.0717354246658798));
#96458=CARTESIAN_POINT('Ctrl Pts',(0.0134184825231483,-0.0317295851069886,
0.0719040540044168));
#96459=CARTESIAN_POINT('Ctrl Pts',(0.0131479317272018,-0.0322357242816073,
0.0713507060784779));
#96460=CARTESIAN_POINT('Ctrl Pts',(0.0132370856080511,-0.0319819883628706,
0.0715107187250557));
#96461=CARTESIAN_POINT('Ctrl Pts',(0.0133158767450407,-0.0317295851069886,
0.0716760802026348));
#96462=CARTESIAN_POINT('Origin',(-0.00141488122122914,-0.0326371942647059,
0.0795566496198092));
#96463=CARTESIAN_POINT('Origin',(-0.00113147873671373,-0.0326352985528954,
0.0799430179030252));
#96464=CARTESIAN_POINT('Ctrl Pts',(0.0136008811544591,-0.0321934096636183,
0.0717002271599773));
#96465=CARTESIAN_POINT('Ctrl Pts',(0.0136346654311598,-0.0320835708272304,
0.0717757606232456));
#96466=CARTESIAN_POINT('Ctrl Pts',(0.0136668669505106,-0.0319739230346346,
0.0718519494378859));
#96467=CARTESIAN_POINT('Ctrl Pts',(0.0136974519940889,-0.0318646057455575,
0.0719286929636407));
#96468=CARTESIAN_POINT('Ctrl Pts',(0.013492762273239,-0.0321934096636183,
0.0716662938092816));
#96469=CARTESIAN_POINT('Ctrl Pts',(0.0135270145172919,-0.0320835708272304,
0.0717403362289151));
#96470=CARTESIAN_POINT('Ctrl Pts',(0.0135597145896253,-0.0319739230346346,
0.0718150445493465));
#96471=CARTESIAN_POINT('Ctrl Pts',(0.0135908279885789,-0.0318646057455575,
0.0718903199755538));
#96472=CARTESIAN_POINT('Ctrl Pts',(0.013384643392019,-0.0321934096636183,
0.0716323604585858));
#96473=CARTESIAN_POINT('Ctrl Pts',(0.013419363603424,-0.0320835708272304,
0.0717049118345846));
#96474=CARTESIAN_POINT('Ctrl Pts',(0.0134525622287399,-0.0319739230346346,
0.0717781396608072));
#96475=CARTESIAN_POINT('Ctrl Pts',(0.0134842039830689,-0.0318646057455575,
0.0718519469874669));
#96476=CARTESIAN_POINT('Ctrl Pts',(0.013276524510799,-0.0321934096636183,
0.07159842710789));
#96477=CARTESIAN_POINT('Ctrl Pts',(0.0133117126895561,-0.0320835708272304,
0.071669487440254));
#96478=CARTESIAN_POINT('Ctrl Pts',(0.0133454098678546,-0.0319739230346346,
0.0717412347722678));
#96479=CARTESIAN_POINT('Ctrl Pts',(0.0133775799775589,-0.0318646057455575,
0.07181357399938));
#96480=CARTESIAN_POINT('Ctrl Pts',(0.0132210242785011,-0.0320218834582289,
0.0714874972444543));
#96481=CARTESIAN_POINT('Ctrl Pts',(0.0132487344956265,-0.0319391099350605,
0.0715405472120583));
#96482=CARTESIAN_POINT('Ctrl Pts',(0.0132755995411529,-0.0318564869454907,
0.0715939977369605));
#96483=CARTESIAN_POINT('Ctrl Pts',(0.0133016034819944,-0.0317740741446519,
0.0716478080607704));
#96484=CARTESIAN_POINT('Ctrl Pts',(0.0132368825874967,-0.0320218834582289,
0.0714405361745845));
#96485=CARTESIAN_POINT('Ctrl Pts',(0.0132650815558318,-0.0319391099350605,
0.0714937511888478));
#96486=CARTESIAN_POINT('Ctrl Pts',(0.0132924324792191,-0.0318564869454907,
0.0715473742923306));
#96487=CARTESIAN_POINT('Ctrl Pts',(0.0133189190824105,-0.0317740741446519,
0.0716013645679027));
#96488=CARTESIAN_POINT('Ctrl Pts',(0.0132527408964923,-0.0320218834582289,
0.0713935751047146));
#96489=CARTESIAN_POINT('Ctrl Pts',(0.0132814286160371,-0.0319391099350606,
0.0714469551656374));
#96490=CARTESIAN_POINT('Ctrl Pts',(0.0133092654172854,-0.0318564869454907,
0.0715007508477007));
#96491=CARTESIAN_POINT('Ctrl Pts',(0.0133362346828265,-0.0317740741446519,
0.071554921075035));
#96492=CARTESIAN_POINT('Ctrl Pts',(0.0132685992054879,-0.0320218834582289,
0.0713466140348448));
#96493=CARTESIAN_POINT('Ctrl Pts',(0.0132977756762424,-0.0319391099350606,
0.071400159142427));
#96494=CARTESIAN_POINT('Ctrl Pts',(0.0133260983553517,-0.0318564869454907,
0.0714541274030708));
#96495=CARTESIAN_POINT('Ctrl Pts',(0.0133535502832426,-0.0317740741446519,
0.0715084775821673));
#96496=CARTESIAN_POINT('Origin',(0.0183607323870741,-0.0391228853390707,
0.067740205225121));
#96497=CARTESIAN_POINT('Ctrl Pts',(0.0111563086103407,-0.035272297877954,
0.0692624701462411));
#96498=CARTESIAN_POINT('Ctrl Pts',(0.0111721784557977,-0.0352466642097181,
0.0692727288344202));
#96499=CARTESIAN_POINT('Ctrl Pts',(0.0111880767251362,-0.0352210183808283,
0.0692829125411708));
#96500=CARTESIAN_POINT('Ctrl Pts',(0.0112040042666222,-0.0351953608940152,
0.0692930211774508));
#96501=CARTESIAN_POINT('Origin',(0.0139667067512102,-0.0352456003065003,
0.0652485686174006));
#96502=CARTESIAN_POINT('Ctrl Pts',(0.0113077670268148,-0.035024121149334,
0.0693621486323109));
#96503=CARTESIAN_POINT('Ctrl Pts',(0.0113737177133355,-0.0349144232867422,
0.069406006715933));
#96504=CARTESIAN_POINT('Ctrl Pts',(0.0114388012966323,-0.0348045283677512,
0.0694512542984857));
#96505=CARTESIAN_POINT('Ctrl Pts',(0.0115029322562204,-0.0346945769586886,
0.0694978365257308));
#96506=CARTESIAN_POINT('Ctrl Pts',(0.0112878086753612,-0.035024121149334,
0.069250601305986));
#96507=CARTESIAN_POINT('Ctrl Pts',(0.0113552958804965,-0.0349144232867422,
0.0692941844715125));
#96508=CARTESIAN_POINT('Ctrl Pts',(0.0114219225848416,-0.0348045283677512,
0.0693391887323541));
#96509=CARTESIAN_POINT('Ctrl Pts',(0.0114876013029676,-0.0346945769586886,
0.0693855596194885));
#96510=CARTESIAN_POINT('Ctrl Pts',(0.0112678503239075,-0.035024121149334,
0.0691390539796612));
#96511=CARTESIAN_POINT('Ctrl Pts',(0.0113368740476575,-0.0349144232867422,
0.069182362227092));
#96512=CARTESIAN_POINT('Ctrl Pts',(0.011405043873051,-0.0348045283677512,
0.0692271231662225));
#96513=CARTESIAN_POINT('Ctrl Pts',(0.0114722703497148,-0.0346945769586886,
0.0692732827132463));
#96514=CARTESIAN_POINT('Ctrl Pts',(0.0112478919724539,-0.035024121149334,
0.0690275066533363));
#96515=CARTESIAN_POINT('Ctrl Pts',(0.0113184522148186,-0.0349144232867422,
0.0690705399826715));
#96516=CARTESIAN_POINT('Ctrl Pts',(0.0113881651612603,-0.0348045283677512,
0.0691150576000909));
#96517=CARTESIAN_POINT('Ctrl Pts',(0.011456939396462,-0.0346945769586886,
0.069161005807004));
#96518=CARTESIAN_POINT('Origin',(0.00149122091931901,-0.0345629067941437,
0.0829748015098817));
#96519=CARTESIAN_POINT('Ctrl Pts',(0.0116511346552536,-0.0351970973651656,
0.0693820542804004));
#96520=CARTESIAN_POINT('Ctrl Pts',(0.011717188081489,-0.0350869349321803,
0.0694309209683551));
#96521=CARTESIAN_POINT('Ctrl Pts',(0.0117822803142518,-0.0349764985129742,
0.069481201351032));
#96522=CARTESIAN_POINT('Ctrl Pts',(0.0118463231901381,-0.0348659306849652,
0.0695328352528112));
#96523=CARTESIAN_POINT('Ctrl Pts',(0.0115705317543276,-0.0351970973651656,
0.0693982913679529));
#96524=CARTESIAN_POINT('Ctrl Pts',(0.0116363602377201,-0.0350869349321803,
0.0694460414119515));
#96525=CARTESIAN_POINT('Ctrl Pts',(0.011701250555709,-0.0349764985129742,
0.0694951995492205));
#96526=CARTESIAN_POINT('Ctrl Pts',(0.0117651148920621,-0.0348659306849652,
0.0695457070426431));
#96527=CARTESIAN_POINT('Ctrl Pts',(0.0114899288534016,-0.0351970973651656,
0.0694145284555054));
#96528=CARTESIAN_POINT('Ctrl Pts',(0.0115555323939512,-0.0350869349321803,
0.0694611618555479));
#96529=CARTESIAN_POINT('Ctrl Pts',(0.0116202207971662,-0.0349764985129742,
0.0695091977474089));
#96530=CARTESIAN_POINT('Ctrl Pts',(0.0116839065939862,-0.0348659306849652,
0.0695585788324751));
#96531=CARTESIAN_POINT('Ctrl Pts',(0.0114093259524756,-0.0351970973651656,
0.0694307655430578));
#96532=CARTESIAN_POINT('Ctrl Pts',(0.0114747045501823,-0.0350869349321803,
0.0694762822991443));
#96533=CARTESIAN_POINT('Ctrl Pts',(0.0115391910386234,-0.0349764985129742,
0.0695231959455974));
#96534=CARTESIAN_POINT('Ctrl Pts',(0.0116026982959102,-0.0348659306849652,
0.069571450622307));
#96535=CARTESIAN_POINT('Origin',(0.00113578253201136,-0.0345637187967305,
0.0826507815892884));
#96536=CARTESIAN_POINT('Ctrl Pts',(0.0113822413412722,-0.0352450361861253,
0.0694107417268366));
#96537=CARTESIAN_POINT('Ctrl Pts',(0.0115609853954992,-0.0349452761023765,
0.0695336365270574));
#96538=CARTESIAN_POINT('Ctrl Pts',(0.0117299647177502,-0.0346444289983475,
0.0696696459292855));
#96539=CARTESIAN_POINT('Ctrl Pts',(0.0111732055928418,-0.0352450361861253,
0.0692736138453606));
#96540=CARTESIAN_POINT('Ctrl Pts',(0.0113571215098518,-0.0349452761023765,
0.0693886247331633));
#96541=CARTESIAN_POINT('Ctrl Pts',(0.0115318518506954,-0.0346444289983475,
0.0695171621861935));
#96542=CARTESIAN_POINT('Ctrl Pts',(0.0116021150931601,-0.0345231616327823,
0.069571519793703));
#96543=CARTESIAN_POINT('Ctrl Pts',(0.011665222996819,-0.0344132092796976,
0.0696194637156289));
#96544=CARTESIAN_POINT('Ctrl Pts',(0.0117273359621928,-0.0343032738558974,
0.0696687105010772));
#96545=CARTESIAN_POINT('Ctrl Pts',(0.0117883760314895,-0.0341934961088741,
0.0697191950209093));
#96546=CARTESIAN_POINT('Ctrl Pts',(0.011589200224347,-0.0345231616327823,
0.0694589394121885));
#96547=CARTESIAN_POINT('Ctrl Pts',(0.0116538598900645,-0.0344132092796976,
0.0695067053208305));
#96548=CARTESIAN_POINT('Ctrl Pts',(0.0117175282194975,-0.0343032738558974,
0.0695558061991537));
#96549=CARTESIAN_POINT('Ctrl Pts',(0.0117801252574648,-0.0341934961088741,
0.0696061770539023));
#96550=CARTESIAN_POINT('Ctrl Pts',(0.0115762853555338,-0.0345231616327823,
0.069346359030674));
#96551=CARTESIAN_POINT('Ctrl Pts',(0.0116424967833101,-0.0344132092796976,
0.0693939469260321));
#96552=CARTESIAN_POINT('Ctrl Pts',(0.0117077204768023,-0.0343032738558974,
0.0694429018972302));
#96553=CARTESIAN_POINT('Ctrl Pts',(0.0117718744834402,-0.0341934961088741,
0.0694931590868952));
#96554=CARTESIAN_POINT('Ctrl Pts',(0.0115633704867207,-0.0345231616327823,
0.0692337786491595));
#96555=CARTESIAN_POINT('Ctrl Pts',(0.0116311336765556,-0.0344132092796976,
0.0692811885312336));
#96556=CARTESIAN_POINT('Ctrl Pts',(0.0116979127341071,-0.0343032738558974,
0.0693299975953067));
#96557=CARTESIAN_POINT('Ctrl Pts',(0.0117636237094155,-0.0341934961088741,
0.0693801411198881));
#96558=CARTESIAN_POINT('Origin',(0.00148415075349963,-0.0345625596230733,
0.082984625513595));
#96559=CARTESIAN_POINT('Ctrl Pts',(0.0120365469580469,-0.0346945769586885,
0.069601343946356));
#96560=CARTESIAN_POINT('Ctrl Pts',(0.0120992297375753,-0.0345846629176052,
0.0696552638225161));
#96561=CARTESIAN_POINT('Ctrl Pts',(0.0121608081825813,-0.0344746925050311,
0.0697104891624619));
#96562=CARTESIAN_POINT('Ctrl Pts',(0.0122212036838981,-0.0343648066253259,
0.0697669488792724));
#96563=CARTESIAN_POINT('Ctrl Pts',(0.0119242701402049,-0.0346945769586885,
0.0696166748875381));
#96564=CARTESIAN_POINT('Ctrl Pts',(0.0119867416516149,-0.0345846629176052,
0.0696690475323982));
#96565=CARTESIAN_POINT('Ctrl Pts',(0.0120481407885251,-0.0344746925050311,
0.0697227210078353));
#96566=CARTESIAN_POINT('Ctrl Pts',(0.0121083891633072,-0.0343648066253259,
0.0697776262163046));
#96567=CARTESIAN_POINT('Ctrl Pts',(0.0118119933223629,-0.0346945769586885,
0.0696320058287201));
#96568=CARTESIAN_POINT('Ctrl Pts',(0.0118742535656544,-0.0345846629176052,
0.0696828312422803));
#96569=CARTESIAN_POINT('Ctrl Pts',(0.0119354733944689,-0.0344746925050311,
0.0697349528532086));
#96570=CARTESIAN_POINT('Ctrl Pts',(0.0119955746427163,-0.0343648066253259,
0.0697883035533368));
#96571=CARTESIAN_POINT('Ctrl Pts',(0.0116997165045209,-0.0346945769586885,
0.0696473367699022));
#96572=CARTESIAN_POINT('Ctrl Pts',(0.011761765479694,-0.0345846629176052,
0.0696966149521625));
#96573=CARTESIAN_POINT('Ctrl Pts',(0.0118228060004128,-0.0344746925050311,
0.0697471846985819));
#96574=CARTESIAN_POINT('Ctrl Pts',(0.0118827601221254,-0.0343648066253259,
0.069798980890369));
#96575=CARTESIAN_POINT('Origin',(0.00109928252967554,-0.0345626446731628,
0.0826964092180731));
#96576=CARTESIAN_POINT('Ctrl Pts',(0.0117017255132845,-0.0346945769586885,
0.069647062447956));
#96577=CARTESIAN_POINT('Ctrl Pts',(0.0117960413431884,-0.0345275153362891,
0.0697220039033263));
#96578=CARTESIAN_POINT('Ctrl Pts',(0.0118880247282043,-0.0343603235965159,
0.0697999308884341));
#96579=CARTESIAN_POINT('Ctrl Pts',(0.0119774070477464,-0.034193496108874,
0.069880608886537));
#96580=CARTESIAN_POINT('Ctrl Pts',(0.0116349715036842,-0.0346945769586885,
0.0695963482435004));
#96581=CARTESIAN_POINT('Ctrl Pts',(0.0117303495629053,-0.0345275153362891,
0.0696698915094128));
#96582=CARTESIAN_POINT('Ctrl Pts',(0.0118234394237568,-0.0343603235965159,
0.0697464533495536));
#96583=CARTESIAN_POINT('Ctrl Pts',(0.0119139691331808,-0.034193496108874,
0.0698258032360359));
#96584=CARTESIAN_POINT('Ctrl Pts',(0.0115682174940839,-0.0346945769586885,
0.0695456340390449));
#96585=CARTESIAN_POINT('Ctrl Pts',(0.0116646577826221,-0.0345275153362891,
0.0696177791154993));
#96586=CARTESIAN_POINT('Ctrl Pts',(0.0117588541193092,-0.0343603235965159,
0.0696929758106731));
#96587=CARTESIAN_POINT('Ctrl Pts',(0.0118505312186153,-0.034193496108874,
0.0697709975855348));
#96588=CARTESIAN_POINT('Ctrl Pts',(0.0115014634844837,-0.0346945769586885,
0.0694949198345893));
#96589=CARTESIAN_POINT('Ctrl Pts',(0.011598966002339,-0.0345275153362891,
0.0695656667215859));
#96590=CARTESIAN_POINT('Ctrl Pts',(0.0116942688148617,-0.0343603235965159,
0.0696394982717926));
#96591=CARTESIAN_POINT('Ctrl Pts',(0.0117870933040497,-0.034193496108874,
0.0697161919350337));
#96592=CARTESIAN_POINT('Ctrl Pts',(0.0118827358805017,-0.0340223579322365,
0.0697989606832147));
#96593=CARTESIAN_POINT('Ctrl Pts',(0.0119427480606665,-0.0339125849573554,
0.0698508064583261));
#96594=CARTESIAN_POINT('Ctrl Pts',(0.0120016449838952,-0.0338030433565221,
0.069903857914692));
#96595=CARTESIAN_POINT('Ctrl Pts',(0.0120593573450247,-0.0336938721132328,
0.0699580405317086));
#96596=CARTESIAN_POINT('Ctrl Pts',(0.011876915448826,-0.0340223579322365,
0.0696857913304491));
#96597=CARTESIAN_POINT('Ctrl Pts',(0.0119384885295235,-0.0339125849573554,
0.0697375568266274));
#96598=CARTESIAN_POINT('Ctrl Pts',(0.0119989469180457,-0.0338030433565221,
0.0697905603674852));
#96599=CARTESIAN_POINT('Ctrl Pts',(0.0120582193069463,-0.0336938721132328,
0.0698447273166822));
#96600=CARTESIAN_POINT('Ctrl Pts',(0.0118710950171504,-0.0340223579322365,
0.0695726219776836));
#96601=CARTESIAN_POINT('Ctrl Pts',(0.0119342289983806,-0.0339125849573554,
0.0696243071949287));
#96602=CARTESIAN_POINT('Ctrl Pts',(0.0119962488521961,-0.0338030433565221,
0.0696772628202785));
#96603=CARTESIAN_POINT('Ctrl Pts',(0.0120570812688679,-0.0336938721132328,
0.0697314141016559));
#96604=CARTESIAN_POINT('Ctrl Pts',(0.0118652745854748,-0.0340223579322365,
0.069459452624918));
#96605=CARTESIAN_POINT('Ctrl Pts',(0.0119299694672377,-0.0339125849573554,
0.06951105756323));
#96606=CARTESIAN_POINT('Ctrl Pts',(0.0119935507863465,-0.0338030433565221,
0.0695639652730717));
#96607=CARTESIAN_POINT('Ctrl Pts',(0.0120559432307895,-0.0336938721132328,
0.0696181008866296));
#96608=CARTESIAN_POINT('Origin',(0.00155843379365339,-0.0345589643415022,
0.0828901008711272));
#96609=CARTESIAN_POINT('Ctrl Pts',(0.0123144384873385,-0.034193496108874,
0.0698560042124226));
#96610=CARTESIAN_POINT('Ctrl Pts',(0.0123736501464459,-0.0340836138581106,
0.0699137908811119));
#96611=CARTESIAN_POINT('Ctrl Pts',(0.0124316376208305,-0.0339738896643499,
0.0699727750837136));
#96612=CARTESIAN_POINT('Ctrl Pts',(0.0124883317543179,-0.0338644633294062,
0.0700328763526159));
#96613=CARTESIAN_POINT('Ctrl Pts',(0.0122014204186368,-0.034193496108874,
0.0698642549938713));
#96614=CARTESIAN_POINT('Ctrl Pts',(0.0122605183043539,-0.0340836138581106,
0.0699204832103199));
#96615=CARTESIAN_POINT('Ctrl Pts',(0.0123184243088379,-0.0339738896643499,
0.0699779073541539));
#96616=CARTESIAN_POINT('Ctrl Pts',(0.0123750692463383,-0.0338644633294062,
0.0700364489614341));
#96617=CARTESIAN_POINT('Ctrl Pts',(0.0120884023499351,-0.034193496108874,
0.0698725057753202));
#96618=CARTESIAN_POINT('Ctrl Pts',(0.0121473864622619,-0.0340836138581106,
0.069927175539528));
#96619=CARTESIAN_POINT('Ctrl Pts',(0.0122052109968453,-0.0339738896643499,
0.0699830396245943));
#96620=CARTESIAN_POINT('Ctrl Pts',(0.0122618067383588,-0.0338644633294062,
0.0700400215702524));
#96621=CARTESIAN_POINT('Ctrl Pts',(0.0119753842812334,-0.034193496108874,
0.069880756556769));
#96622=CARTESIAN_POINT('Ctrl Pts',(0.0120342546201699,-0.0340836138581106,
0.069933867868736));
#96623=CARTESIAN_POINT('Ctrl Pts',(0.0120919976848527,-0.0339738896643499,
0.0699881718950347));
#96624=CARTESIAN_POINT('Ctrl Pts',(0.0121485442303792,-0.0338644633294062,
0.0700435941790706));
#96625=CARTESIAN_POINT('Origin',(0.00114795659634253,-0.0345610621864789,
0.0826389863918568));
#96626=CARTESIAN_POINT('Ctrl Pts',(0.0119504753784144,-0.0342436276873901,
0.0698564531834935));
#96627=CARTESIAN_POINT('Ctrl Pts',(0.012112409166108,-0.0339430054201861,
0.0700007792962205));
#96628=CARTESIAN_POINT('Ctrl Pts',(0.012263011682719,-0.0336441434784162,
0.0701568929099836));
#96629=CARTESIAN_POINT('Ctrl Pts',(0.0117602724055806,-0.0342436276873901,
0.0696942100661505));
#96630=CARTESIAN_POINT('Ctrl Pts',(0.0119283252933194,-0.0339430054201861,
0.0698313625554986));
#96631=CARTESIAN_POINT('Ctrl Pts',(0.0120855698729596,-0.0336441434784162,
0.0699807838410823));
#96632=CARTESIAN_POINT('Ctrl Pts',(0.0121485243370367,-0.0335235895815128,
0.0700435748585472));
#96633=CARTESIAN_POINT('Ctrl Pts',(0.0122050573639151,-0.0334144449262719,
0.0700989833581458));
#96634=CARTESIAN_POINT('Ctrl Pts',(0.0122605106424901,-0.0333049234473133,
0.0701556234451868));
#96635=CARTESIAN_POINT('Ctrl Pts',(0.0123148067044481,-0.0331951640388588,
0.0702134291175165));
#96636=CARTESIAN_POINT('Ctrl Pts',(0.0121498214044117,-0.0335235895815128,
0.0699302633847131));
#96637=CARTESIAN_POINT('Ctrl Pts',(0.0122079143868172,-0.0334144449262719,
0.0699856897409977));
#96638=CARTESIAN_POINT('Ctrl Pts',(0.0122649290442134,-0.0333049234473133,
0.0700423799327472));
#96639=CARTESIAN_POINT('Ctrl Pts',(0.0123207859059592,-0.0331951640388588,
0.0701002680745929));
#96640=CARTESIAN_POINT('Ctrl Pts',(0.0121511184717866,-0.0335235895815128,
0.0698169519108789));
#96641=CARTESIAN_POINT('Ctrl Pts',(0.0122107714097192,-0.0334144449262719,
0.0698723961238496));
#96642=CARTESIAN_POINT('Ctrl Pts',(0.0122693474459368,-0.0333049234473133,
0.0699291364203076));
#96643=CARTESIAN_POINT('Ctrl Pts',(0.0123267651074702,-0.0331951640388588,
0.0699871070316694));
#96644=CARTESIAN_POINT('Ctrl Pts',(0.0121524155391616,-0.0335235895815128,
0.0697036404370447));
#96645=CARTESIAN_POINT('Ctrl Pts',(0.0122136284326212,-0.0334144449262719,
0.0697591025067015));
#96646=CARTESIAN_POINT('Ctrl Pts',(0.0122737658476601,-0.0333049234473133,
0.069815892907868));
#96647=CARTESIAN_POINT('Ctrl Pts',(0.0123327443089813,-0.0331951640388588,
0.0698739459887459));
#96648=CARTESIAN_POINT('Origin',(-0.00034203095527586,-0.0326434571768189,
0.0810575658527565));
#96649=CARTESIAN_POINT('Ctrl Pts',(0.0125778188787164,-0.0336938721132364,
0.0701275905556615));
#96650=CARTESIAN_POINT('Ctrl Pts',(0.0126013633759704,-0.0336474569764945,
0.0701536615103876));
#96651=CARTESIAN_POINT('Ctrl Pts',(0.0126246010664983,-0.033601104548885,
0.0701800062967829));
#96652=CARTESIAN_POINT('Ctrl Pts',(0.0126834335537046,-0.0334837508643158,
0.0702467052360211));
#96653=CARTESIAN_POINT('Ctrl Pts',(0.0127402637782464,-0.0333660264760398,
0.0703151182145042));
#96654=CARTESIAN_POINT('Ctrl Pts',(0.012237880085459,-0.0336938721132364,
0.0701310046613417));
#96655=CARTESIAN_POINT('Ctrl Pts',(0.0122614045988195,-0.0336474569764945,
0.0701550858415074));
#96656=CARTESIAN_POINT('Ctrl Pts',(0.0122846455996468,-0.033601104548885,
0.070179440755746));
#96657=CARTESIAN_POINT('Ctrl Pts',(0.0123434864677696,-0.0334837508643158,
0.0702411017964006));
#96658=CARTESIAN_POINT('Ctrl Pts',(0.0124004743529215,-0.0333660264760398,
0.0703044793369176));
#96659=CARTESIAN_POINT('Ctrl Pts',(0.0122378800854708,-0.0336938721132427,
0.0701310046613536));
#96660=CARTESIAN_POINT('Ctrl Pts',(0.0122614045988304,-0.0336474569765026,
0.0701550858415182));
#96661=CARTESIAN_POINT('Ctrl Pts',(0.0122846455996568,-0.0336011045488949,
0.070179440755756));
#96662=CARTESIAN_POINT('Ctrl Pts',(0.0123429964034918,-0.0334847282606778,
0.0702405882439267));
#96663=CARTESIAN_POINT('Ctrl Pts',(0.0123995251664643,-0.0333679869945434,
0.0703034239867374));
#96664=CARTESIAN_POINT('Ctrl Pts',(0.0122378800854558,-0.0336938721132427,
0.0701310046613385));
#96665=CARTESIAN_POINT('Ctrl Pts',(0.0123220141558681,-0.0335278710435083,
0.0702171296185953));
#96666=CARTESIAN_POINT('Ctrl Pts',(0.0124034177718423,-0.033362046922432,
0.0703058626998658));
#96667=CARTESIAN_POINT('Ctrl Pts',(0.012482116658346,-0.0331951640388602,
0.0703972615746468));
#96668=CARTESIAN_POINT('Ctrl Pts',(0.0121780086200365,-0.0336938721132427,
0.0700723238514274));
#96669=CARTESIAN_POINT('Ctrl Pts',(0.0122633711206849,-0.0335278710435083,
0.0701571954531406));
#96670=CARTESIAN_POINT('Ctrl Pts',(0.0123460420396404,-0.033362046922432,
0.0702447141430479));
#96671=CARTESIAN_POINT('Ctrl Pts',(0.0124260479341282,-0.0331951640388602,
0.070334937197491));
#96672=CARTESIAN_POINT('Ctrl Pts',(0.0121181371546173,-0.0336938721132427,
0.0700136430415162));
#96673=CARTESIAN_POINT('Ctrl Pts',(0.0122047280855018,-0.0335278710435083,
0.070097261287686));
#96674=CARTESIAN_POINT('Ctrl Pts',(0.0122886663074385,-0.033362046922432,
0.0701835655862302));
#96675=CARTESIAN_POINT('Ctrl Pts',(0.0123699792099104,-0.0331951640388602,
0.0702726128203351));
#96676=CARTESIAN_POINT('Ctrl Pts',(0.012058265689198,-0.0336938721132427,
0.0699549622316051));
#96677=CARTESIAN_POINT('Ctrl Pts',(0.0121460850503186,-0.0335278710435083,
0.0700373271222313));
#96678=CARTESIAN_POINT('Ctrl Pts',(0.0122312905752366,-0.033362046922432,
0.0701224170294123));
#96679=CARTESIAN_POINT('Ctrl Pts',(0.0123139104856925,-0.0331951640388602,
0.0702102884431793));
#96680=CARTESIAN_POINT('Ctrl Pts',(0.0123984264156948,-0.0330240426238156,
0.0703043924341847));
#96681=CARTESIAN_POINT('Ctrl Pts',(0.0124514034065075,-0.0329142774063509,
0.0703632798229346));
#96682=CARTESIAN_POINT('Ctrl Pts',(0.012503189441463,-0.0328043479726686,
0.0704232917515795));
#96683=CARTESIAN_POINT('Ctrl Pts',(0.0125537160615389,-0.0326943950436594,
0.0704843531674097));
#96684=CARTESIAN_POINT('Ctrl Pts',(0.012406835779861,-0.0330240426238156,
0.0701913861574614));
#96685=CARTESIAN_POINT('Ctrl Pts',(0.0124613695422323,-0.0329142774063509,
0.0702503893933956));
#96686=CARTESIAN_POINT('Ctrl Pts',(0.0125147107299688,-0.0328043479726686,
0.0703105494097955));
#96687=CARTESIAN_POINT('Ctrl Pts',(0.0125667888865571,-0.0326943950436594,
0.0703717910191067));
#96688=CARTESIAN_POINT('Ctrl Pts',(0.0124152451440273,-0.0330240426238156,
0.0700783798807381));
#96689=CARTESIAN_POINT('Ctrl Pts',(0.0124713356779571,-0.0329142774063509,
0.0701374989638565));
#96690=CARTESIAN_POINT('Ctrl Pts',(0.0125262320184747,-0.0328043479726686,
0.0701978070680114));
#96691=CARTESIAN_POINT('Ctrl Pts',(0.0125798617115753,-0.0326943950436594,
0.0702592288708037));
#96692=CARTESIAN_POINT('Ctrl Pts',(0.0124236545081936,-0.0330240426238156,
0.0699653736040149));
#96693=CARTESIAN_POINT('Ctrl Pts',(0.0124813018136819,-0.0329142774063509,
0.0700246085343175));
#96694=CARTESIAN_POINT('Ctrl Pts',(0.0125377533069805,-0.0328043479726686,
0.0700850647262274));
#96695=CARTESIAN_POINT('Ctrl Pts',(0.0125929345365935,-0.0326943950436594,
0.0701466667225008));
#96696=CARTESIAN_POINT('Origin',(-0.000436084180803091,-0.0326396682856425,
0.0811378739443185));
#96697=CARTESIAN_POINT('Ctrl Pts',(0.0128195742877403,-0.0331951640388587,
0.0704150921558746));
#96698=CARTESIAN_POINT('Ctrl Pts',(0.0128710150876361,-0.0330855618255041,
0.0704797671924681));
#96699=CARTESIAN_POINT('Ctrl Pts',(0.0129211562480315,-0.0329757224427708,
0.0705455520457946));
#96700=CARTESIAN_POINT('Ctrl Pts',(0.0129699294279412,-0.0328657862078596,
0.0706123656239742));
#96701=CARTESIAN_POINT('Ctrl Pts',(0.012706413334905,-0.0331951640388587,
0.0704091129591236));
#96702=CARTESIAN_POINT('Ctrl Pts',(0.0127579364861402,-0.0330855618255041,
0.0704722294325145));
#96703=CARTESIAN_POINT('Ctrl Pts',(0.0128081922700783,-0.0329757224427708,
0.0705364563011535));
#96704=CARTESIAN_POINT('Ctrl Pts',(0.0128571122968149,-0.0328657862078596,
0.0706017144754535));
#96705=CARTESIAN_POINT('Ctrl Pts',(0.0125932523820697,-0.0331951640388587,
0.0704031337623726));
#96706=CARTESIAN_POINT('Ctrl Pts',(0.0126448578846443,-0.0330855618255041,
0.070464691672561));
#96707=CARTESIAN_POINT('Ctrl Pts',(0.012695228292125,-0.0329757224427708,
0.0705273605565124));
#96708=CARTESIAN_POINT('Ctrl Pts',(0.0127442951656886,-0.0328657862078596,
0.0705910633269327));
#96709=CARTESIAN_POINT('Ctrl Pts',(0.0124800914292343,-0.0331951640388587,
0.0703971545656216));
#96710=CARTESIAN_POINT('Ctrl Pts',(0.0125317792831484,-0.0330855618255041,
0.0704571539126075));
#96711=CARTESIAN_POINT('Ctrl Pts',(0.0125822643141717,-0.0329757224427708,
0.0705182648118713));
#96712=CARTESIAN_POINT('Ctrl Pts',(0.0126314780345623,-0.0328657862078596,
0.0705804121784119));
#96713=CARTESIAN_POINT('Origin',(-0.000709363987007214,-0.0326401908837922,
0.0807421581137135));
#96714=CARTESIAN_POINT('Ctrl Pts',(0.0124584724956533,-0.0332451089994433,
0.0703699755316898));
#96715=CARTESIAN_POINT('Ctrl Pts',(0.0126010384509766,-0.0329451141710258,
0.0705334610512132));
#96716=CARTESIAN_POINT('Ctrl Pts',(0.0127308849938027,-0.0326442513127503,
0.0707072207761991));
#96717=CARTESIAN_POINT('Ctrl Pts',(0.012290106113183,-0.0332451089994433,
0.0701851708746763));
#96718=CARTESIAN_POINT('Ctrl Pts',(0.0124396420901811,-0.0329451141710258,
0.0703423063521926));
#96719=CARTESIAN_POINT('Ctrl Pts',(0.0125769171647092,-0.0326442513127503,
0.070510259085497));
#96720=CARTESIAN_POINT('Ctrl Pts',(0.0126314584950257,-0.0325229783203385,
0.0705803873593277));
#96721=CARTESIAN_POINT('Ctrl Pts',(0.0126806655263194,-0.0324130253112079,
0.0706425255774421));
#96722=CARTESIAN_POINT('Ctrl Pts',(0.0127285796855624,-0.0323031222247695,
0.0707056722817132));
#96723=CARTESIAN_POINT('Ctrl Pts',(0.0127751424523411,-0.0321934096636184,
0.0707697444199963));
#96724=CARTESIAN_POINT('Ctrl Pts',(0.0126469469741007,-0.0325229783203385,
0.070468132071411));
#96725=CARTESIAN_POINT('Ctrl Pts',(0.0126977014420553,-0.0324130253112079,
0.0705304837978669));
#96726=CARTESIAN_POINT('Ctrl Pts',(0.0127471583865658,-0.0323031222247695,
0.0705938759888112));
#96727=CARTESIAN_POINT('Ctrl Pts',(0.0127952573221166,-0.0321934096636184,
0.070658225207915));
#96728=CARTESIAN_POINT('Ctrl Pts',(0.0126624354531757,-0.0325229783203385,
0.0703558767834943));
#96729=CARTESIAN_POINT('Ctrl Pts',(0.0127147373577912,-0.0324130253112079,
0.0704184420182917));
#96730=CARTESIAN_POINT('Ctrl Pts',(0.0127657370875693,-0.0323031222247695,
0.0704820796959093));
#96731=CARTESIAN_POINT('Ctrl Pts',(0.0128153721918921,-0.0321934096636184,
0.0705467059958338));
#96732=CARTESIAN_POINT('Ctrl Pts',(0.0126779239322506,-0.0325229783203385,
0.0702436214955776));
#96733=CARTESIAN_POINT('Ctrl Pts',(0.0127317732735271,-0.0324130253112079,
0.0703064002387165));
#96734=CARTESIAN_POINT('Ctrl Pts',(0.0127843157885728,-0.0323031222247695,
0.0703702834030074));
#96735=CARTESIAN_POINT('Ctrl Pts',(0.0128354870616676,-0.0321934096636184,
0.0704351867837525));
#96736=CARTESIAN_POINT('Origin',(-0.000429331389440062,-0.0326393375175697,
0.081132669058702));
#96737=CARTESIAN_POINT('Ctrl Pts',(0.0130448250186197,-0.0326943950436594,
0.07071731336857));
#96738=CARTESIAN_POINT('Ctrl Pts',(0.0130921338739411,-0.0325844576448127,
0.0707851345617225));
#96739=CARTESIAN_POINT('Ctrl Pts',(0.0131380434239149,-0.0324744968375319,
0.0708539389793783));
#96740=CARTESIAN_POINT('Ctrl Pts',(0.0131824960624879,-0.0323646534831894,
0.0709236376539727));
#96741=CARTESIAN_POINT('Ctrl Pts',(0.0129322629071423,-0.0326943950436594,
0.0707042405478287));
#96742=CARTESIAN_POINT('Ctrl Pts',(0.0129797519304346,-0.0325844576448127,
0.0707705104241212));
#96743=CARTESIAN_POINT('Ctrl Pts',(0.0130258737449062,-0.0324744968375319,
0.0708377671412968));
#96744=CARTESIAN_POINT('Ctrl Pts',(0.0130705704451865,-0.0323646534831894,
0.0709059237110439));
#96745=CARTESIAN_POINT('Ctrl Pts',(0.012819700795665,-0.0326943950436594,
0.0706911677270873));
#96746=CARTESIAN_POINT('Ctrl Pts',(0.0128673699869281,-0.0325844576448127,
0.0707558862865198));
#96747=CARTESIAN_POINT('Ctrl Pts',(0.0129137040658974,-0.0324744968375319,
0.0708215953032153));
#96748=CARTESIAN_POINT('Ctrl Pts',(0.0129586448278851,-0.0323646534831894,
0.0708882097681151));
#96749=CARTESIAN_POINT('Ctrl Pts',(0.0127071386841876,-0.0326943950436594,
0.070678094906346));
#96750=CARTESIAN_POINT('Ctrl Pts',(0.0127549880434217,-0.0325844576448127,
0.0707412621489184));
#96751=CARTESIAN_POINT('Ctrl Pts',(0.0128015343868887,-0.0324744968375319,
0.0708054234651338));
#96752=CARTESIAN_POINT('Ctrl Pts',(0.0128467192105837,-0.0323646534831894,
0.0708704958251864));
#96753=CARTESIAN_POINT('Origin',(-0.000739414714879376,-0.0326395579070081,
0.0807651562789755));
#96754=CARTESIAN_POINT('Ctrl Pts',(0.0126872448025215,-0.0327445246961876,
0.0706495808804532));
#96755=CARTESIAN_POINT('Ctrl Pts',(0.0128192652664822,-0.0324436878365475,
0.0708216946846538));
#96756=CARTESIAN_POINT('Ctrl Pts',(0.0129379463592203,-0.0321434074463188,
0.071003263852541));
#96757=CARTESIAN_POINT('Ctrl Pts',(0.0125308133031275,-0.0327445246961876,
0.070454570147422));
#96758=CARTESIAN_POINT('Ctrl Pts',(0.012670188717045,-0.0324436878365475,
0.070620784041234));
#96759=CARTESIAN_POINT('Ctrl Pts',(0.0127966482704634,-0.0321434074463188,
0.0707970240646397));
#96760=CARTESIAN_POINT('Ctrl Pts',(0.0129011493564902,-0.0322357242816073,
0.0709476745970712));
#96761=CARTESIAN_POINT('Ctrl Pts',(0.0130031392673096,-0.0319819883628706,
0.0710998275452069));
#96762=CARTESIAN_POINT('Ctrl Pts',(0.0130952405555584,-0.0317295851069886,
0.0712581620463056));
#96763=CARTESIAN_POINT('Ctrl Pts',(0.0127574702486035,-0.0322357242816073,
0.0707430864401392));
#96764=CARTESIAN_POINT('Ctrl Pts',(0.01286597602688,-0.0319819883628706,
0.0708906633950335));
#96765=CARTESIAN_POINT('Ctrl Pts',(0.0129648711609127,-0.0317295851069886,
0.0710448457999957));
#96766=CARTESIAN_POINT('Origin',(-0.000662033131781533,-0.0326371942646385,
0.0807095281023099));
#96767=CARTESIAN_POINT('Origin',(-0.000332440573460987,-0.0326352985530457,
0.0810573300062842));
#96768=CARTESIAN_POINT('Ctrl Pts',(0.0132506546416794,-0.0321934096636184,
0.0710330818271546));
#96769=CARTESIAN_POINT('Ctrl Pts',(0.0132936393724612,-0.0320835708272304,
0.0711037853938617));
#96770=CARTESIAN_POINT('Ctrl Pts',(0.0133351359637141,-0.0319739230346346,
0.0711753375163961));
#96771=CARTESIAN_POINT('Ctrl Pts',(0.0133750983493265,-0.0318646057455575,
0.0712476425741178));
#96772=CARTESIAN_POINT('Ctrl Pts',(0.0131391353335633,-0.0321934096636184,
0.0710129669400572));
#96773=CARTESIAN_POINT('Ctrl Pts',(0.0131823974643148,-0.0320835708272304,
0.0710821325685925));
#96774=CARTESIAN_POINT('Ctrl Pts',(0.0132242031221846,-0.0319739230346346,
0.0711521533857997));
#96775=CARTESIAN_POINT('Ctrl Pts',(0.0132645056952689,-0.0318646057455575,
0.0712229356998896));
#96776=CARTESIAN_POINT('Ctrl Pts',(0.0130276160254473,-0.0321934096636184,
0.0709928520529598));
#96777=CARTESIAN_POINT('Ctrl Pts',(0.0130711555561684,-0.0320835708272304,
0.0710604797433233));
#96778=CARTESIAN_POINT('Ctrl Pts',(0.0131132702806552,-0.0319739230346346,
0.0711289692552033));
#96779=CARTESIAN_POINT('Ctrl Pts',(0.0131539130412113,-0.0318646057455575,
0.0711982288256615));
#96780=CARTESIAN_POINT('Ctrl Pts',(0.0129160967173313,-0.0321934096636184,
0.0709727371658623));
#96781=CARTESIAN_POINT('Ctrl Pts',(0.012959913648022,-0.0320835708272304,
0.0710388269180541));
#96782=CARTESIAN_POINT('Ctrl Pts',(0.0130023374391257,-0.0319739230346346,
0.0711057851246069));
#96783=CARTESIAN_POINT('Ctrl Pts',(0.0130433203871538,-0.0318646057455575,
0.0711735219514334));
#96784=CARTESIAN_POINT('Ctrl Pts',(0.0128471309224587,-0.0320218834582295,
0.0708696380411101));
#96785=CARTESIAN_POINT('Ctrl Pts',(0.0128812715602258,-0.0319391099350611,
0.0709187966827591));
#96786=CARTESIAN_POINT('Ctrl Pts',(0.0129146238939656,-0.0318564869454912,
0.070968458651282));
#96787=CARTESIAN_POINT('Ctrl Pts',(0.0129471670078489,-0.0317740741446524,
0.0710185855066251));
#96788=CARTESIAN_POINT('Ctrl Pts',(0.0128569784012128,-0.0320218834582295,
0.0708210597001579));
#96789=CARTESIAN_POINT('Ctrl Pts',(0.0128916246220717,-0.0319391099350611,
0.0708703208302546));
#96790=CARTESIAN_POINT('Ctrl Pts',(0.012925480632212,-0.0318564869454912,
0.0709200931198808));
#96791=CARTESIAN_POINT('Ctrl Pts',(0.0129585251564445,-0.0317740741446524,
0.0709703380143798));
#96792=CARTESIAN_POINT('Ctrl Pts',(0.0128668258799668,-0.0320218834582295,
0.0707724813592056));
#96793=CARTESIAN_POINT('Ctrl Pts',(0.0129019776839176,-0.0319391099350611,
0.07082184497775));
#96794=CARTESIAN_POINT('Ctrl Pts',(0.0129363373704585,-0.0318564869454912,
0.0708717275884797));
#96795=CARTESIAN_POINT('Ctrl Pts',(0.0129698833050402,-0.0317740741446524,
0.0709220905221345));
#96796=CARTESIAN_POINT('Ctrl Pts',(0.0128766733587208,-0.0320218834582295,
0.0707239030182534));
#96797=CARTESIAN_POINT('Ctrl Pts',(0.0129123307457636,-0.0319391099350611,
0.0707733691252455));
#96798=CARTESIAN_POINT('Ctrl Pts',(0.0129471941087049,-0.0318564869454912,
0.0708233620570786));
#96799=CARTESIAN_POINT('Ctrl Pts',(0.0129812414536358,-0.0317740741446524,
0.0708738430298891));
#96800=CARTESIAN_POINT('Origin',(0.0174766506715612,-0.0391228853390799,
0.0665077183017818));
#96801=CARTESIAN_POINT('Ctrl Pts',(0.0105198263130554,-0.0352722978779541,
0.0689209334372314));
#96802=CARTESIAN_POINT('Ctrl Pts',(0.0105368567746026,-0.0352466642097181,
0.0689291222135428));
#96803=CARTESIAN_POINT('Ctrl Pts',(0.0105539060382353,-0.0352210183808284,
0.0689372330372197));
#96804=CARTESIAN_POINT('Ctrl Pts',(0.0105709749343713,-0.0351953608940152,
0.0689452657136062));
#96805=CARTESIAN_POINT('Origin',(0.0128049883673411,-0.0352456003065,0.0645864464342393));
#96806=CARTESIAN_POINT('Ctrl Pts',(0.010682583461653,-0.035024121149334,
0.0690008431555788));
#96807=CARTESIAN_POINT('Ctrl Pts',(0.0107535109827503,-0.0349144232867422,
0.0690360895923144));
#96808=CARTESIAN_POINT('Ctrl Pts',(0.0108237523883856,-0.0348045283677512,
0.0690728232482173));
#96809=CARTESIAN_POINT('Ctrl Pts',(0.0108932159573696,-0.0346945769586886,
0.0691110004201504));
#96810=CARTESIAN_POINT('Ctrl Pts',(0.0106488019006581,-0.035024121149334,
0.0688926768579639));
#96811=CARTESIAN_POINT('Ctrl Pts',(0.0107212193680879,-0.0349144232867422,
0.0689274579675687));
#96812=CARTESIAN_POINT('Ctrl Pts',(0.0107929612305043,-0.0348045283677512,
0.0689637568160742));
#96813=CARTESIAN_POINT('Ctrl Pts',(0.0108639338655484,-0.0346945769586886,
0.0690015303287941));
#96814=CARTESIAN_POINT('Ctrl Pts',(0.0106150203396632,-0.035024121149334,
0.0687845105603489));
#96815=CARTESIAN_POINT('Ctrl Pts',(0.0106889277534256,-0.0349144232867422,
0.068818826342823));
#96816=CARTESIAN_POINT('Ctrl Pts',(0.0107621700726231,-0.0348045283677512,
0.068854690383931));
#96817=CARTESIAN_POINT('Ctrl Pts',(0.0108346517737272,-0.0346945769586886,
0.0688920602374378));
#96818=CARTESIAN_POINT('Ctrl Pts',(0.0105812387786684,-0.035024121149334,
0.0686763442627339));
#96819=CARTESIAN_POINT('Ctrl Pts',(0.0106566361387633,-0.0349144232867422,
0.0687101947180773));
#96820=CARTESIAN_POINT('Ctrl Pts',(0.0107313789147418,-0.0348045283677512,
0.0687456239517878));
#96821=CARTESIAN_POINT('Ctrl Pts',(0.010805369681906,-0.0346945769586886,
0.0687825901460815));
#96822=CARTESIAN_POINT('Origin',(0.00264956155499517,-0.0345629067942747,
0.083736495665415));
#96823=CARTESIAN_POINT('Ctrl Pts',(0.0110257383730229,-0.0351970973651658,
0.0689775564665144));
#96824=CARTESIAN_POINT('Ctrl Pts',(0.0110973955682782,-0.0350869349321804,
0.0690177591365407));
#96825=CARTESIAN_POINT('Ctrl Pts',(0.0111682763322893,-0.0349764985129743,
0.0690594848233701));
#96826=CARTESIAN_POINT('Ctrl Pts',(0.0112382856548422,-0.0348659306849651,
0.0691026848756899));
#96827=CARTESIAN_POINT('Ctrl Pts',(0.010947806096732,-0.0351970973651658,
0.0690037677419895));
#96828=CARTESIAN_POINT('Ctrl Pts',(0.0110191001702881,-0.0350869349321804,
0.0690428907659447));
#96829=CARTESIAN_POINT('Ctrl Pts',(0.0110896399570378,-0.0349764985129743,
0.069083528363238));
#96830=CARTESIAN_POINT('Ctrl Pts',(0.0111593309714934,-0.0348659306849651,
0.0691256332662046));
#96831=CARTESIAN_POINT('Ctrl Pts',(0.0108698738204411,-0.0351970973651658,
0.0690299790174647));
#96832=CARTESIAN_POINT('Ctrl Pts',(0.0109408047722981,-0.0350869349321804,
0.0690680223953488));
#96833=CARTESIAN_POINT('Ctrl Pts',(0.0110110035817863,-0.0349764985129743,
0.0691075719031058));
#96834=CARTESIAN_POINT('Ctrl Pts',(0.0110803762881446,-0.0348659306849651,
0.0691485816567192));
#96835=CARTESIAN_POINT('Ctrl Pts',(0.0107919415441502,-0.0351970973651658,
0.0690561902929398));
#96836=CARTESIAN_POINT('Ctrl Pts',(0.010862509374308,-0.0350869349321804,
0.0690931540247529));
#96837=CARTESIAN_POINT('Ctrl Pts',(0.0109323672065349,-0.0349764985129743,
0.0691316154429736));
#96838=CARTESIAN_POINT('Ctrl Pts',(0.0110014216047959,-0.0348659306849651,
0.0691715300472339));
#96839=CARTESIAN_POINT('Origin',(0.00225631544113613,-0.0345637187968448,
0.0834595789810976));
#96840=CARTESIAN_POINT('Ctrl Pts',(0.0107625608535624,-0.0352450361861253,
0.0690397189723917));
#96841=CARTESIAN_POINT('Ctrl Pts',(0.0109552982602334,-0.0349452761023765,
0.0691392421401093));
#96842=CARTESIAN_POINT('Ctrl Pts',(0.0111399916282332,-0.0346444289983475,
0.0692530003427135));
#96843=CARTESIAN_POINT('Ctrl Pts',(0.010537986733647,-0.0352450361861253,
0.0689298715115006));
#96844=CARTESIAN_POINT('Ctrl Pts',(0.0107348671051819,-0.0349452761023765,
0.0690209247275181));
#96845=CARTESIAN_POINT('Ctrl Pts',(0.0109243296597209,-0.0346444289983475,
0.0691265491057191));
#96846=CARTESIAN_POINT('Ctrl Pts',(0.0110008516702502,-0.0345231616327822,
0.0691716717678788));
#96847=CARTESIAN_POINT('Ctrl Pts',(0.011069470916004,-0.0344132092796975,
0.0692113281200311));
#96848=CARTESIAN_POINT('Ctrl Pts',(0.0111372663609564,-0.0343032738558973,
0.0692524017610703));
#96849=CARTESIAN_POINT('Ctrl Pts',(0.0112041524991905,-0.0341934961088741,
0.0692948378461226));
#96850=CARTESIAN_POINT('Ctrl Pts',(0.010973928575784,-0.0345231616327822,
0.0690615977785681));
#96851=CARTESIAN_POINT('Ctrl Pts',(0.0110440650365087,-0.0344132092796975,
0.0691008830337679));
#96852=CARTESIAN_POINT('Ctrl Pts',(0.0111133852939984,-0.0343032738558973,
0.0691416169793963));
#96853=CARTESIAN_POINT('Ctrl Pts',(0.0111818018777275,-0.0341934961088741,
0.0691837451557301));
#96854=CARTESIAN_POINT('Ctrl Pts',(0.0109470054813178,-0.0345231616327822,
0.0689515237892573));
#96855=CARTESIAN_POINT('Ctrl Pts',(0.0110186591570133,-0.0344132092796975,
0.0689904379475046));
#96856=CARTESIAN_POINT('Ctrl Pts',(0.0110895042270403,-0.0343032738558973,
0.0690308321977223));
#96857=CARTESIAN_POINT('Ctrl Pts',(0.0111594512562646,-0.0341934961088741,
0.0690726524653377));
#96858=CARTESIAN_POINT('Ctrl Pts',(0.0109200823868516,-0.0345231616327822,
0.0688414497999466));
#96859=CARTESIAN_POINT('Ctrl Pts',(0.010993253277518,-0.0344132092796975,
0.0688799928612413));
#96860=CARTESIAN_POINT('Ctrl Pts',(0.0110656231600823,-0.0343032738558973,
0.0689200474160483));
#96861=CARTESIAN_POINT('Ctrl Pts',(0.0111371006348017,-0.0341934961088741,
0.0689615597749452));
#96862=CARTESIAN_POINT('Origin',(0.00264377841353288,-0.0345625596230839,
0.083747128330629));
#96863=CARTESIAN_POINT('Ctrl Pts',(0.0114355958676125,-0.0346945769586885,
0.0691468119977909));
#96864=CARTESIAN_POINT('Ctrl Pts',(0.0115045423269825,-0.0345846629178476,
0.0691924504640746));
#96865=CARTESIAN_POINT('Ctrl Pts',(0.0115725567778391,-0.0344746925055161,
0.0692395225099826));
#96866=CARTESIAN_POINT('Ctrl Pts',(0.0116395523213195,-0.0343648066260528,
0.0692879674614766));
#96867=CARTESIAN_POINT('Ctrl Pts',(0.0113261258624471,-0.0346945769586885,
0.0691760940665569));
#96868=CARTESIAN_POINT('Ctrl Pts',(0.0113946688001098,-0.0345846629178476,
0.0692202239808414));
#96869=CARTESIAN_POINT('Ctrl Pts',(0.0114623108565725,-0.0344746925055161,
0.0692657788724225));
#96870=CARTESIAN_POINT('Ctrl Pts',(0.0115289656020984,-0.0343648066260528,
0.0693127000131858));
#96871=CARTESIAN_POINT('Ctrl Pts',(0.0112166558572818,-0.0346945769586885,
0.069205376135323));
#96872=CARTESIAN_POINT('Ctrl Pts',(0.0112847952732372,-0.0345846629178476,
0.0692479974976082));
#96873=CARTESIAN_POINT('Ctrl Pts',(0.0113520649353058,-0.0344746925055161,
0.0692920352348625));
#96874=CARTESIAN_POINT('Ctrl Pts',(0.0114183788828774,-0.0343648066260528,
0.0693374325648949));
#96875=CARTESIAN_POINT('Ctrl Pts',(0.0111071858521164,-0.0346945769586885,
0.069234658204089));
#96876=CARTESIAN_POINT('Ctrl Pts',(0.0111749217463646,-0.0345846629178476,
0.069275771014375));
#96877=CARTESIAN_POINT('Ctrl Pts',(0.0112418190140392,-0.0344746925055161,
0.0693182915973025));
#96878=CARTESIAN_POINT('Ctrl Pts',(0.0113077921636563,-0.0343648066260528,
0.069362165116604));
#96879=CARTESIAN_POINT('Origin',(0.00222582190978953,-0.0345626446729341,
0.0835094214858947));
#96880=CARTESIAN_POINT('Ctrl Pts',(0.0111091446375892,-0.0346945769586886,
0.0692341342496886));
#96881=CARTESIAN_POINT('Ctrl Pts',(0.0112121094139331,-0.0345275153362891,
0.0692966638613612));
#96882=CARTESIAN_POINT('Ctrl Pts',(0.0113131343235095,-0.0343603235965159,
0.0693624477938375));
#96883=CARTESIAN_POINT('Ctrl Pts',(0.0114119234711446,-0.034193496108874,
0.0694312870466963));
#96884=CARTESIAN_POINT('Ctrl Pts',(0.011036560828061,-0.0346945769586886,
0.0691921864377594));
#96885=CARTESIAN_POINT('Ctrl Pts',(0.0111404042181207,-0.0345275153362891,
0.0692531957524804));
#96886=CARTESIAN_POINT('Ctrl Pts',(0.0112423557806073,-0.0343603235965159,
0.0693174866263712));
#96887=CARTESIAN_POINT('Ctrl Pts',(0.0113421168140885,-0.034193496108874,
0.0693848644340822));
#96888=CARTESIAN_POINT('Ctrl Pts',(0.0109639770185329,-0.0346945769586886,
0.0691502386258302));
#96889=CARTESIAN_POINT('Ctrl Pts',(0.0110686990223084,-0.0345275153362891,
0.0692097276435997));
#96890=CARTESIAN_POINT('Ctrl Pts',(0.0111715772377051,-0.0343603235965159,
0.069272525458905));
#96891=CARTESIAN_POINT('Ctrl Pts',(0.0112723101570324,-0.034193496108874,
0.0693384418214681));
#96892=CARTESIAN_POINT('Ctrl Pts',(0.0108913932090047,-0.0346945769586886,
0.0691082908139009));
#96893=CARTESIAN_POINT('Ctrl Pts',(0.0109969938264961,-0.0345275153362891,
0.0691662595347189));
#96894=CARTESIAN_POINT('Ctrl Pts',(0.0111007986948029,-0.0343603235965159,
0.0692275642914387));
#96895=CARTESIAN_POINT('Ctrl Pts',(0.0112025034999763,-0.034193496108874,
0.0692920192088539));
#96896=CARTESIAN_POINT('Ctrl Pts',(0.0113077655809934,-0.0340223579322365,
0.0693621481073606));
#96897=CARTESIAN_POINT('Ctrl Pts',(0.0113738025458342,-0.0339125849573554,
0.0694060635424564));
#96898=CARTESIAN_POINT('Ctrl Pts',(0.0114388841598033,-0.0338030433565221,
0.0694513149304079));
#96899=CARTESIAN_POINT('Ctrl Pts',(0.011502932324321,-0.0336938721132328,
0.0694978370244687));
#96900=CARTESIAN_POINT('Ctrl Pts',(0.0112878071642375,-0.0340223579322365,
0.0692506006222662));
#96901=CARTESIAN_POINT('Ctrl Pts',(0.0113553826598258,-0.0339125849573554,
0.0692942407787412));
#96902=CARTESIAN_POINT('Ctrl Pts',(0.0114220074210625,-0.0338030433565221,
0.0693392489255184));
#96903=CARTESIAN_POINT('Ctrl Pts',(0.011487601348368,-0.0336938721132328,
0.0693855599519801));
#96904=CARTESIAN_POINT('Ctrl Pts',(0.0112678487474817,-0.0340223579322365,
0.0691390531371719));
#96905=CARTESIAN_POINT('Ctrl Pts',(0.0113369627738175,-0.0339125849573554,
0.069182418015026));
#96906=CARTESIAN_POINT('Ctrl Pts',(0.0114051306823216,-0.0338030433565221,
0.069227182920629));
#96907=CARTESIAN_POINT('Ctrl Pts',(0.0114722703724149,-0.0336938721132328,
0.0692732828794915));
#96908=CARTESIAN_POINT('Ctrl Pts',(0.0112478903307258,-0.0340223579322365,
0.0690275056520775));
#96909=CARTESIAN_POINT('Ctrl Pts',(0.0113185428878091,-0.0339125849573554,
0.0690705952513109));
#96910=CARTESIAN_POINT('Ctrl Pts',(0.0113882539435808,-0.0338030433565221,
0.0691151169157396));
#96911=CARTESIAN_POINT('Ctrl Pts',(0.0114569393964619,-0.0336938721132328,
0.0691610058070029));
#96912=CARTESIAN_POINT('Origin',(0.00270562863037882,-0.034558964341501,
0.0836440389099324));
#96913=CARTESIAN_POINT('Ctrl Pts',(0.0117432135338,-0.034193496108874,0.0693646351476499));
#96914=CARTESIAN_POINT('Ctrl Pts',(0.0118092008813334,-0.0340836138581107,
0.0694145449624959));
#96915=CARTESIAN_POINT('Ctrl Pts',(0.0118741237880036,-0.03397388966435,
0.0694657962993714));
#96916=CARTESIAN_POINT('Ctrl Pts',(0.0119379035576876,-0.0338644633294062,
0.069518317992743));
#96917=CARTESIAN_POINT('Ctrl Pts',(0.0116321207434458,-0.034193496108874,
0.069386985789224));
#96918=CARTESIAN_POINT('Ctrl Pts',(0.0116977998888674,-0.0340836138581107,
0.0694353637002776));
#96919=CARTESIAN_POINT('Ctrl Pts',(0.0117624464408417,-0.03397388966435,
0.0694850774908009));
#96920=CARTESIAN_POINT('Ctrl Pts',(0.0118259819250294,-0.0338644633294062,
0.0695360579868402));
#96921=CARTESIAN_POINT('Ctrl Pts',(0.0115210279530916,-0.034193496108874,
0.0694093364307981));
#96922=CARTESIAN_POINT('Ctrl Pts',(0.0115863988964014,-0.0340836138581107,
0.0694561824380593));
#96923=CARTESIAN_POINT('Ctrl Pts',(0.0116507690936797,-0.03397388966435,
0.0695043586822304));
#96924=CARTESIAN_POINT('Ctrl Pts',(0.0117140602923711,-0.0338644633294062,
0.0695537979809374));
#96925=CARTESIAN_POINT('Ctrl Pts',(0.0114099351627374,-0.034193496108874,
0.0694316870723723));
#96926=CARTESIAN_POINT('Ctrl Pts',(0.0114749979039354,-0.0340836138581107,
0.069477001175841));
#96927=CARTESIAN_POINT('Ctrl Pts',(0.0115390917465177,-0.03397388966435,
0.0695236398736599));
#96928=CARTESIAN_POINT('Ctrl Pts',(0.0116021386597128,-0.0338644633294062,
0.0695715379750346));
#96929=CARTESIAN_POINT('Origin',(0.00226691517884985,-0.0345610621863834,
0.0834463509773151));
#96930=CARTESIAN_POINT('Ctrl Pts',(0.0113821766536979,-0.0342436276873901,
0.069410697251789));
#96931=CARTESIAN_POINT('Ctrl Pts',(0.0115609224035041,-0.0339430054201861,
0.0695335896247741));
#96932=CARTESIAN_POINT('Ctrl Pts',(0.0117299035983051,-0.0336441434784164,
0.069669596735674));
#96933=CARTESIAN_POINT('Ctrl Pts',(0.0111731390335956,-0.0342436276873901,
0.0692735722235048));
#96934=CARTESIAN_POINT('Ctrl Pts',(0.0113570565391009,-0.0339430054201861,
0.0693885806126787));
#96935=CARTESIAN_POINT('Ctrl Pts',(0.0115317886511495,-0.0336441434784164,
0.0695171156951689));
#96936=CARTESIAN_POINT('Ctrl Pts',(0.0116021165017316,-0.0335235895815127,
0.0695715213001562));
#96937=CARTESIAN_POINT('Ctrl Pts',(0.0116651482752291,-0.0334144449262719,
0.0696194074201238));
#96938=CARTESIAN_POINT('Ctrl Pts',(0.0117272631733977,-0.0333049234473133,
0.0696686507444454));
#96939=CARTESIAN_POINT('Ctrl Pts',(0.0117883760665211,-0.0331951640388588,
0.069719195500768));
#96940=CARTESIAN_POINT('Ctrl Pts',(0.0115892016479273,-0.0335235895815127,
0.0694589407554894));
#96941=CARTESIAN_POINT('Ctrl Pts',(0.0116537833142729,-0.0334144449262719,
0.0695066490770674));
#96942=CARTESIAN_POINT('Ctrl Pts',(0.0117174535591095,-0.0333049234473133,
0.0695557464183504));
#96943=CARTESIAN_POINT('Ctrl Pts',(0.0117801252808193,-0.0331951640388588,
0.069606177373808));
#96944=CARTESIAN_POINT('Ctrl Pts',(0.0115762867941231,-0.0335235895815127,
0.0693463602108227));
#96945=CARTESIAN_POINT('Ctrl Pts',(0.0116424183533166,-0.0334144449262719,
0.069393890734011));
#96946=CARTESIAN_POINT('Ctrl Pts',(0.0117076439448212,-0.0333049234473133,
0.0694428420922554));
#96947=CARTESIAN_POINT('Ctrl Pts',(0.0117718744951174,-0.0331951640388588,
0.069493159246848));
#96948=CARTESIAN_POINT('Ctrl Pts',(0.0115633719403188,-0.0335235895815127,
0.0692337796661559));
#96949=CARTESIAN_POINT('Ctrl Pts',(0.0116310533923603,-0.0334144449262719,
0.0692811323909546));
#96950=CARTESIAN_POINT('Ctrl Pts',(0.011697834330533,-0.0333049234473133,
0.0693299377661604));
#96951=CARTESIAN_POINT('Ctrl Pts',(0.0117636237094155,-0.0331951640388588,
0.0693801411198879));
#96952=CARTESIAN_POINT('Origin',(0.00059047207459251,-0.0326434571769134,
0.0820641453694175));
#96953=CARTESIAN_POINT('Ctrl Pts',(0.0120385558867142,-0.0336938721132359,
0.0696010696353447));
#96954=CARTESIAN_POINT('Ctrl Pts',(0.0120651822856328,-0.0336474569764943,
0.0696239841048323));
#96955=CARTESIAN_POINT('Ctrl Pts',(0.0120915386172965,-0.033601104548885,
0.0696472086998235));
#96956=CARTESIAN_POINT('Ctrl Pts',(0.0121582667864989,-0.0334837508643155,
0.0697060080321436));
#96957=CARTESIAN_POINT('Ctrl Pts',(0.012223223307557,-0.0333660264760393,
0.0697667588380515));
#96958=CARTESIAN_POINT('Ctrl Pts',(0.0117017255132827,-0.0336938721132359,
0.0696470624479546));
#96959=CARTESIAN_POINT('Ctrl Pts',(0.011728082701007,-0.0336474569764943,
0.0696680053374943));
#96960=CARTESIAN_POINT('Ctrl Pts',(0.0117541929197555,-0.033601104548885,
0.0696892553361747));
#96961=CARTESIAN_POINT('Ctrl Pts',(0.0118202979876687,-0.0334837508643155,
0.069743055444839));
#96962=CARTESIAN_POINT('Ctrl Pts',(0.0118847798184132,-0.0333660264760393,
0.0697987907585992));
#96963=CARTESIAN_POINT('Ctrl Pts',(0.0117017255132945,-0.0336938721132427,
0.069647062447966));
#96964=CARTESIAN_POINT('Ctrl Pts',(0.0117280827010179,-0.0336474569765026,
0.069668005337505));
#96965=CARTESIAN_POINT('Ctrl Pts',(0.0117541929197655,-0.0336011045488949,
0.0696892553361847));
#96966=CARTESIAN_POINT('Ctrl Pts',(0.0118197474225006,-0.0334847282606778,
0.0697426073632216));
#96967=CARTESIAN_POINT('Ctrl Pts',(0.0118837058461226,-0.0333679869945434,
0.0697978626947793));
#96968=CARTESIAN_POINT('Ctrl Pts',(0.0117017255132788,-0.0336938721132427,
0.0696470624479515));
#96969=CARTESIAN_POINT('Ctrl Pts',(0.0117959904807998,-0.0335278710435083,
0.0697219634890984));
#96970=CARTESIAN_POINT('Ctrl Pts',(0.0118878734089479,-0.033362046922432,
0.069799794305106));
#96971=CARTESIAN_POINT('Ctrl Pts',(0.0119774070477457,-0.0331951640388602,
0.0698806088865364));
#96972=CARTESIAN_POINT('Ctrl Pts',(0.0116349714965928,-0.0336938721132427,
0.0695963482381129));
#96973=CARTESIAN_POINT('Ctrl Pts',(0.0117302981207075,-0.0335278710435083,
0.0696698518436653));
#96974=CARTESIAN_POINT('Ctrl Pts',(0.0118232861551779,-0.033362046922432,
0.0697463190089678));
#96975=CARTESIAN_POINT('Ctrl Pts',(0.0119139691264464,-0.0331951640388602,
0.0698258032302179));
#96976=CARTESIAN_POINT('Ctrl Pts',(0.0115682174799067,-0.0336938721132427,
0.0695456340282742));
#96977=CARTESIAN_POINT('Ctrl Pts',(0.0116646057606152,-0.0335278710435083,
0.0696177401982322));
#96978=CARTESIAN_POINT('Ctrl Pts',(0.0117586989014079,-0.033362046922432,
0.0696928437128296));
#96979=CARTESIAN_POINT('Ctrl Pts',(0.0118505312051471,-0.0331951640388602,
0.0697709975738993));
#96980=CARTESIAN_POINT('Ctrl Pts',(0.0115014634632207,-0.0336938721132427,
0.0694949198184356));
#96981=CARTESIAN_POINT('Ctrl Pts',(0.0115989134005229,-0.0335278710435083,
0.0695656285527992));
#96982=CARTESIAN_POINT('Ctrl Pts',(0.0116941116476378,-0.033362046922432,
0.0696393684166914));
#96983=CARTESIAN_POINT('Ctrl Pts',(0.0117870932838478,-0.0331951640388602,
0.0697161919175808));
#96984=CARTESIAN_POINT('Ctrl Pts',(0.0118827371379824,-0.0330240426238156,
0.0697989612157147));
#96985=CARTESIAN_POINT('Ctrl Pts',(0.0119426769362473,-0.0329142774063509,
0.0698507444822524));
#96986=CARTESIAN_POINT('Ctrl Pts',(0.0120015761119189,-0.0328043479726686,
0.0699037926877008));
#96987=CARTESIAN_POINT('Ctrl Pts',(0.0120593573391959,-0.0326943950436595,
0.0699580399513539));
#96988=CARTESIAN_POINT('Ctrl Pts',(0.0118769167497257,-0.0330240426238156,
0.0696857920544335));
#96989=CARTESIAN_POINT('Ctrl Pts',(0.0119384155634426,-0.0329142774063509,
0.0697374951394524));
#96990=CARTESIAN_POINT('Ctrl Pts',(0.0119988761893682,-0.0328043479726686,
0.0697904953526129));
#96991=CARTESIAN_POINT('Ctrl Pts',(0.0120582193030605,-0.0326943950436595,
0.0698447269297796));
#96992=CARTESIAN_POINT('Ctrl Pts',(0.0118710963614689,-0.0330240426238156,
0.0695726228931522));
#96993=CARTESIAN_POINT('Ctrl Pts',(0.0119341541906378,-0.0329142774063509,
0.0696242457966524));
#96994=CARTESIAN_POINT('Ctrl Pts',(0.0119961762668175,-0.0328043479726686,
0.069677198017525));
#96995=CARTESIAN_POINT('Ctrl Pts',(0.012057081266925,-0.0326943950436595,
0.0697314139082052));
#96996=CARTESIAN_POINT('Ctrl Pts',(0.0118652759732122,-0.0330240426238156,
0.069459453731871));
#96997=CARTESIAN_POINT('Ctrl Pts',(0.0119298928178331,-0.0329142774063509,
0.0695109964538524));
#96998=CARTESIAN_POINT('Ctrl Pts',(0.0119934763442668,-0.0328043479726686,
0.0695639006824371));
#96999=CARTESIAN_POINT('Ctrl Pts',(0.0120559432307895,-0.0326943950436595,
0.0696181008866309));
#97000=CARTESIAN_POINT('Origin',(0.000507225759736011,-0.0326396682857532,
0.0821556082025202));
#97001=CARTESIAN_POINT('Ctrl Pts',(0.0123144384873385,-0.0331951640388588,
0.0698560042124226));
#97002=CARTESIAN_POINT('Ctrl Pts',(0.0123735795995155,-0.0330855618127431,
0.0699137220319671));
#97003=CARTESIAN_POINT('Ctrl Pts',(0.0124315704168896,-0.0329757224171935,
0.0699727038053237));
#97004=CARTESIAN_POINT('Ctrl Pts',(0.0124883329738301,-0.0328657861694598,
0.0700328776454173));
#97005=CARTESIAN_POINT('Ctrl Pts',(0.0122014204503534,-0.0331951640388588,
0.0698642549915559));
#97006=CARTESIAN_POINT('Ctrl Pts',(0.0122604479247258,-0.0330855618127431,
0.0699204162160933));
#97007=CARTESIAN_POINT('Ctrl Pts',(0.0123183571945371,-0.0329757224171935,
0.0699778379236157));
#97008=CARTESIAN_POINT('Ctrl Pts',(0.0123750704965776,-0.0328657861694598,
0.070036450219684));
#97009=CARTESIAN_POINT('Ctrl Pts',(0.0120884024133683,-0.0331951640388588,
0.0698725057706893));
#97010=CARTESIAN_POINT('Ctrl Pts',(0.012147316249936,-0.0330855618127431,
0.0699271104002196));
#97011=CARTESIAN_POINT('Ctrl Pts',(0.0122051439721847,-0.0329757224171935,
0.0699829720419077));
#97012=CARTESIAN_POINT('Ctrl Pts',(0.012261808019325,-0.0328657861694598,
0.0700400227939507));
#97013=CARTESIAN_POINT('Ctrl Pts',(0.0119753843763832,-0.0331951640388588,
0.0698807565498226));
#97014=CARTESIAN_POINT('Ctrl Pts',(0.0120341845751463,-0.0330855618127431,
0.0699338045843459));
#97015=CARTESIAN_POINT('Ctrl Pts',(0.0120919307498322,-0.0329757224171935,
0.0699881061601998));
#97016=CARTESIAN_POINT('Ctrl Pts',(0.0121485455420724,-0.0328657861694598,
0.0700435953682174));
#97017=CARTESIAN_POINT('Origin',(0.000186504498140234,-0.0326401908833285,
0.0817972637539969));
#97018=CARTESIAN_POINT('Ctrl Pts',(0.011950529478343,-0.0332451089994433,
0.0698565014015431));
#97019=CARTESIAN_POINT('Ctrl Pts',(0.0121124614273289,-0.0329451141710259,
0.0700008295367375));
#97020=CARTESIAN_POINT('Ctrl Pts',(0.0122630619595774,-0.0326442513127503,
0.0701569450273128));
#97021=CARTESIAN_POINT('Ctrl Pts',(0.0117603285498458,-0.0332451089994433,
0.0696942558875872));
#97022=CARTESIAN_POINT('Ctrl Pts',(0.0119283796885058,-0.0329451141710259,
0.0698314104773981));
#97023=CARTESIAN_POINT('Ctrl Pts',(0.0120856223672202,-0.0326442513127503,
0.0699808337242568));
#97024=CARTESIAN_POINT('Ctrl Pts',(0.0121485230261799,-0.0325229783203385,
0.0700435731744104));
#97025=CARTESIAN_POINT('Ctrl Pts',(0.0122051300291387,-0.0324130253112079,
0.0700990541377692));
#97026=CARTESIAN_POINT('Ctrl Pts',(0.01226058075156,-0.0323031222247695,
0.0701556976749047));
#97027=CARTESIAN_POINT('Ctrl Pts',(0.0123148067252875,-0.0321934096636184,
0.070213428723116));
#97028=CARTESIAN_POINT('Ctrl Pts',(0.0121498200557519,-0.0325229783203385,
0.0699302618318026));
#97029=CARTESIAN_POINT('Ctrl Pts',(0.0122079890530622,-0.0324130253112079,
0.0699857606746853));
#97030=CARTESIAN_POINT('Ctrl Pts',(0.012265001163067,-0.0323031222247695,
0.070042454400492));
#97031=CARTESIAN_POINT('Ctrl Pts',(0.0123207859198521,-0.0321934096636184,
0.0701002678116594));
#97032=CARTESIAN_POINT('Ctrl Pts',(0.0121511170853239,-0.0325229783203385,
0.0698169504891947));
#97033=CARTESIAN_POINT('Ctrl Pts',(0.0122108480769856,-0.0324130253112079,
0.0698724672116013));
#97034=CARTESIAN_POINT('Ctrl Pts',(0.0122694215745739,-0.0323031222247695,
0.0699292111260794));
#97035=CARTESIAN_POINT('Ctrl Pts',(0.0123267651144167,-0.0321934096636184,
0.0699871069002029));
#97036=CARTESIAN_POINT('Ctrl Pts',(0.0121524141148959,-0.0325229783203385,
0.0697036391465868));
#97037=CARTESIAN_POINT('Ctrl Pts',(0.0122137071009091,-0.0324130253112079,
0.0697591737485174));
#97038=CARTESIAN_POINT('Ctrl Pts',(0.0122738419860809,-0.0323031222247695,
0.0698159678516667));
#97039=CARTESIAN_POINT('Ctrl Pts',(0.0123327443089813,-0.0321934096636184,
0.0698739459887464));
#97040=CARTESIAN_POINT('Origin',(0.000513272958069437,-0.0326393375177826,
0.0821495980101279));
#97041=CARTESIAN_POINT('Ctrl Pts',(0.0125757914107655,-0.0326943950436593,
0.0701276109181228));
#97042=CARTESIAN_POINT('Ctrl Pts',(0.0126312274710742,-0.0325844576448127,
0.0701889679490965));
#97043=CARTESIAN_POINT('Ctrl Pts',(0.0126853984906822,-0.0324744968375319,
0.0702514758310184));
#97044=CARTESIAN_POINT('Ctrl Pts',(0.0127382361671847,-0.0323646534831894,
0.0703150535178129));
#97045=CARTESIAN_POINT('Ctrl Pts',(0.0124624784262628,-0.0326943950436593,
0.070128748953886));
#97046=CARTESIAN_POINT('Ctrl Pts',(0.0125178988023057,-0.0325844576448127,
0.0701885443195621));
#97047=CARTESIAN_POINT('Ctrl Pts',(0.0125720864343368,-0.0324744968375319,
0.0702494901012886));
#97048=CARTESIAN_POINT('Ctrl Pts',(0.0126249729710602,-0.0323646534831894,
0.0703115072541501));
#97049=CARTESIAN_POINT('Ctrl Pts',(0.01234916544176,-0.0326943950436593,
0.0701298869896492));
#97050=CARTESIAN_POINT('Ctrl Pts',(0.0124045701335372,-0.0325844576448127,
0.0701881206900276));
#97051=CARTESIAN_POINT('Ctrl Pts',(0.0124587743779913,-0.0324744968375319,
0.0702475043715587));
#97052=CARTESIAN_POINT('Ctrl Pts',(0.0125117097749356,-0.0323646534831894,
0.0703079609904873));
#97053=CARTESIAN_POINT('Ctrl Pts',(0.0122358524572572,-0.0326943950436593,
0.0701310250254124));
#97054=CARTESIAN_POINT('Ctrl Pts',(0.0122912414647688,-0.0325844576448127,
0.0701876970604932));
#97055=CARTESIAN_POINT('Ctrl Pts',(0.0123454623216459,-0.0324744968375319,
0.0702455186418289));
#97056=CARTESIAN_POINT('Ctrl Pts',(0.012398446578811,-0.0323646534831894,
0.0703044147268244));
#97057=CARTESIAN_POINT('Origin',(0.000159573167040383,-0.0326395579069251,
0.081823846923887));
#97058=CARTESIAN_POINT('Ctrl Pts',(0.0122125416897229,-0.0327445246961877,
0.0701052292056477));
#97059=CARTESIAN_POINT('Ctrl Pts',(0.0123650927125142,-0.0324436878365474,
0.0702594392894495));
#97060=CARTESIAN_POINT('Ctrl Pts',(0.0125055946203147,-0.0321434074463186,
0.0704247020451001));
#97061=CARTESIAN_POINT('Ctrl Pts',(0.0120329023736749,-0.0327445246961877,
0.0699313622561437));
#97062=CARTESIAN_POINT('Ctrl Pts',(0.0121920108955991,-0.0324436878365474,
0.0700787971324517));
#97063=CARTESIAN_POINT('Ctrl Pts',(0.0123395620096841,-0.0321434074463186,
0.0702377978658875));
#97064=CARTESIAN_POINT('Ctrl Pts',(0.0124621205918024,-0.0322357242816072,
0.0703741630148512));
#97065=CARTESIAN_POINT('Ctrl Pts',(0.0125823761026982,-0.0319819883628705,
0.0705123334662308));
#97066=CARTESIAN_POINT('Ctrl Pts',(0.0126935957197873,-0.0317295851069886,
0.0706578761002245));
#97067=CARTESIAN_POINT('Ctrl Pts',(0.012293932741339,-0.0322357242816072,
0.0701891958638311));
#97068=CARTESIAN_POINT('Ctrl Pts',(0.0124200792161012,-0.0319819883628705,
0.070322009750305));
#97069=CARTESIAN_POINT('Ctrl Pts',(0.0125375187118361,-0.0317295851069886,
0.0704625815340199));
#97070=CARTESIAN_POINT('Origin',(0.000229372514003324,-0.0326371942646295,
0.0817589589081086));
#97071=CARTESIAN_POINT('Origin',(0.000599957274254053,-0.0326352985531905,
0.0820627093890013));
#97072=CARTESIAN_POINT('Ctrl Pts',(0.0128195742877404,-0.0321934096636183,
0.0704150921558745));
#97073=CARTESIAN_POINT('Ctrl Pts',(0.012871081577721,-0.0320835708272303,
0.0704798507885373));
#97074=CARTESIAN_POINT('Ctrl Pts',(0.0129212188148431,-0.0319739230346346,
0.0705456377992503));
#97075=CARTESIAN_POINT('Ctrl Pts',(0.0129699283117961,-0.0318646057455575,
0.0706123640949856));
#97076=CARTESIAN_POINT('Ctrl Pts',(0.0127064132788358,-0.0321934096636183,
0.070409112956161));
#97077=CARTESIAN_POINT('Ctrl Pts',(0.0127580030266404,-0.0320835708272303,
0.0704723110103186));
#97078=CARTESIAN_POINT('Ctrl Pts',(0.0128082549698485,-0.0319739230346346,
0.0705365400541858));
#97079=CARTESIAN_POINT('Ctrl Pts',(0.0128571111214103,-0.0318646057455575,
0.0706017129767819));
#97080=CARTESIAN_POINT('Ctrl Pts',(0.0125932522699313,-0.0321934096636183,
0.0704031337564475));
#97081=CARTESIAN_POINT('Ctrl Pts',(0.0126449244755597,-0.0320835708272303,
0.0704647712320999));
#97082=CARTESIAN_POINT('Ctrl Pts',(0.012695291124854,-0.0319739230346346,
0.0705274423091213));
#97083=CARTESIAN_POINT('Ctrl Pts',(0.0127442939310246,-0.0318646057455575,
0.0705910618585781));
#97084=CARTESIAN_POINT('Ctrl Pts',(0.0124800912610267,-0.0321934096636183,
0.0703971545567339));
#97085=CARTESIAN_POINT('Ctrl Pts',(0.0125318459244791,-0.0320835708272303,
0.0704572314538812));
#97086=CARTESIAN_POINT('Ctrl Pts',(0.0125823272798595,-0.0319739230346346,
0.0705183445640569));
#97087=CARTESIAN_POINT('Ctrl Pts',(0.0126314767406389,-0.0318646057455575,
0.0705804107403744));
#97088=CARTESIAN_POINT('Ctrl Pts',(0.0123987475353627,-0.03202188345823,
0.070303512105451));
#97089=CARTESIAN_POINT('Ctrl Pts',(0.0124387801755191,-0.0319391099350616,
0.0703480041600004));
#97090=CARTESIAN_POINT('Ctrl Pts',(0.0124780938112457,-0.0318564869454917,
0.0703930943732335));
#97091=CARTESIAN_POINT('Ctrl Pts',(0.0125166628738244,-0.0317740741446529,
0.0704387472296568));
#97092=CARTESIAN_POINT('Ctrl Pts',(0.0124024288832527,-0.03202188345823,
0.0702540826028725));
#97093=CARTESIAN_POINT('Ctrl Pts',(0.0124429759650359,-0.0319391099350616,
0.0702986129713538));
#97094=CARTESIAN_POINT('Ctrl Pts',(0.0124828031324247,-0.0318564869454917,
0.0703437495083835));
#97095=CARTESIAN_POINT('Ctrl Pts',(0.0125218844458113,-0.0317740741446529,
0.0703894566298082));
#97096=CARTESIAN_POINT('Ctrl Pts',(0.0124061102311427,-0.03202188345823,
0.070204653100294));
#97097=CARTESIAN_POINT('Ctrl Pts',(0.0124471717545526,-0.0319391099350616,
0.0702492217827072));
#97098=CARTESIAN_POINT('Ctrl Pts',(0.0124875124536037,-0.0318564869454917,
0.0702944046435336));
#97099=CARTESIAN_POINT('Ctrl Pts',(0.0125271060177983,-0.0317740741446529,
0.0703401660299596));
#97100=CARTESIAN_POINT('Ctrl Pts',(0.0124097915790327,-0.03202188345823,
0.0701552235977154));
#97101=CARTESIAN_POINT('Ctrl Pts',(0.0124513675440694,-0.0319391099350616,
0.0701998305940606));
#97102=CARTESIAN_POINT('Ctrl Pts',(0.0124922217747827,-0.0318564869454917,
0.0702450597786836));
#97103=CARTESIAN_POINT('Ctrl Pts',(0.0125323275897852,-0.0317740741446529,
0.0702908754301111));
#97104=CARTESIAN_POINT('Origin',(0.0164450686329765,-0.0391228853390699,
0.0653957547261134));
#97105=CARTESIAN_POINT('Ctrl Pts',(0.00984555696867123,-0.0352722978779542,
0.0686618622316097));
#97106=CARTESIAN_POINT('Ctrl Pts',(0.00986347946575636,-0.0352466642097182,
0.0686678519541593));
#97107=CARTESIAN_POINT('Ctrl Pts',(0.00988141084661135,-0.0352210183808283,
0.0686737619822279));
#97108=CARTESIAN_POINT('Ctrl Pts',(0.00989935191070874,-0.0351953608940152,
0.0686795920186157));
#97109=CARTESIAN_POINT('Origin',(0.0115694445656761,-0.0352456003065,0.064075147203832));
#97110=CARTESIAN_POINT('Ctrl Pts',(0.0100170460719326,-0.035024121149334,
0.0687207429582405));
#97111=CARTESIAN_POINT('Ctrl Pts',(0.0100918318582287,-0.0349144232867422,
0.0687468218907271));
#97112=CARTESIAN_POINT('Ctrl Pts',(0.0101661233372754,-0.0348045283677513,
0.068774462308283));
#97113=CARTESIAN_POINT('Ctrl Pts',(0.0102398240336769,-0.0346945769586886,
0.0688036323480967));
#97114=CARTESIAN_POINT('Ctrl Pts',(0.00996997405679344,-0.035024121149334,
0.0686176635364643));
#97115=CARTESIAN_POINT('Ctrl Pts',(0.0100461797197962,-0.0349144232867422,
0.0686430940712718));
#97116=CARTESIAN_POINT('Ctrl Pts',(0.0101219053282571,-0.0348045283677513,
0.0686701150529163));
#97117=CARTESIAN_POINT('Ctrl Pts',(0.0101970525993676,-0.0346945769586886,
0.0686986954803613));
#97118=CARTESIAN_POINT('Ctrl Pts',(0.0099229020416543,-0.035024121149334,
0.0685145841146881));
#97119=CARTESIAN_POINT('Ctrl Pts',(0.0100005275813638,-0.0349144232867422,
0.0685393662518166));
#97120=CARTESIAN_POINT('Ctrl Pts',(0.0100776873192388,-0.0348045283677513,
0.0685657677975495));
#97121=CARTESIAN_POINT('Ctrl Pts',(0.0101542811650583,-0.0346945769586886,
0.068593758612626));
#97122=CARTESIAN_POINT('Ctrl Pts',(0.00987583002651516,-0.035024121149334,
0.0684115046929119));
#97123=CARTESIAN_POINT('Ctrl Pts',(0.00995487544293143,-0.0349144232867422,
0.0684356384323613));
#97124=CARTESIAN_POINT('Ctrl Pts',(0.0100334693102204,-0.0348045283677513,
0.0684614205421828));
#97125=CARTESIAN_POINT('Ctrl Pts',(0.010111509730749,-0.0346945769586886,
0.0684888217448907));
#97126=CARTESIAN_POINT('Origin',(0.00389423392027531,-0.0345629067943679,
0.0843470050574501));
#97127=CARTESIAN_POINT('Ctrl Pts',(0.0103545765082903,-0.035197097365166,
0.0686546311770197));
#97128=CARTESIAN_POINT('Ctrl Pts',(0.0104307073957904,-0.0350869349321805,
0.0686855358089954));
#97129=CARTESIAN_POINT('Ctrl Pts',(0.0105062588590593,-0.0349764985129744,
0.0687180487609703));
#97130=CARTESIAN_POINT('Ctrl Pts',(0.0105811305394404,-0.0348659306849652,
0.0687521336731991));
#97131=CARTESIAN_POINT('Ctrl Pts',(0.0102805438951862,-0.035197097365166,
0.0686904032729455));
#97132=CARTESIAN_POINT('Ctrl Pts',(0.0103561792087769,-0.0350869349321805,
0.0687202822833985));
#97133=CARTESIAN_POINT('Ctrl Pts',(0.010431256009712,-0.0349764985129744,
0.068751758461531));
#97134=CARTESIAN_POINT('Ctrl Pts',(0.0105056746333406,-0.0348659306849652,
0.0687847967545695));
#97135=CARTESIAN_POINT('Ctrl Pts',(0.010206511282082,-0.0351970973651659,
0.0687261753688713));
#97136=CARTESIAN_POINT('Ctrl Pts',(0.0102816510217635,-0.0350869349321805,
0.0687550287578017));
#97137=CARTESIAN_POINT('Ctrl Pts',(0.0103562531603647,-0.0349764985129744,
0.0687854681620917));
#97138=CARTESIAN_POINT('Ctrl Pts',(0.0104302187272408,-0.0348659306849652,
0.0688174598359399));
#97139=CARTESIAN_POINT('Ctrl Pts',(0.0101324786689779,-0.0351970973651659,
0.0687619474647971));
#97140=CARTESIAN_POINT('Ctrl Pts',(0.0102071228347501,-0.0350869349321805,
0.0687897752322049));
#97141=CARTESIAN_POINT('Ctrl Pts',(0.0102812503110174,-0.0349764985129744,
0.0688191778626523));
#97142=CARTESIAN_POINT('Ctrl Pts',(0.010354762821141,-0.0348659306849652,
0.0688501229173102));
#97143=CARTESIAN_POINT('Origin',(0.00346938180570812,-0.0345637187967836,
0.0841215587510999));
#97144=CARTESIAN_POINT('Ctrl Pts',(0.0101012652500473,-0.0352450361861253,
0.0687492884024862));
#97145=CARTESIAN_POINT('Ctrl Pts',(0.0103049564251235,-0.0349452761023765,
0.0688238703978933));
#97146=CARTESIAN_POINT('Ctrl Pts',(0.0105024511141282,-0.0346444289983475,
0.0689135833660627));
#97147=CARTESIAN_POINT('Ctrl Pts',(0.0098646944266722,-0.0352450361861253,
0.0686684537222579));
#97148=CARTESIAN_POINT('Ctrl Pts',(0.010071434331662,-0.0349452761023765,
0.068734113302881));
#97149=CARTESIAN_POINT('Ctrl Pts',(0.010272641162232,-0.0346444289983475,
0.0688151588467118));
#97150=CARTESIAN_POINT('Ctrl Pts',(0.0103542151430076,-0.0345231616327823,
0.0688503349521842));
#97151=CARTESIAN_POINT('Ctrl Pts',(0.0104272635643597,-0.0344132092796976,
0.0688810783302));
#97152=CARTESIAN_POINT('Ctrl Pts',(0.0104996723142249,-0.0343032738558974,
0.0689133310709747));
#97153=CARTESIAN_POINT('Ctrl Pts',(0.0105713496870405,-0.0341934961088741,
0.0689470494788358));
#97154=CARTESIAN_POINT('Ctrl Pts',(0.0103137084161712,-0.0345231616327823,
0.0687445032876437));
#97155=CARTESIAN_POINT('Ctrl Pts',(0.0103882155780199,-0.0344132092796976,
0.068774688337459));
#97156=CARTESIAN_POINT('Ctrl Pts',(0.0104620945416958,-0.0343032738558974,
0.0688064129517368));
#97157=CARTESIAN_POINT('Ctrl Pts',(0.0105352517007913,-0.0341934961088741,
0.068839634063149));
#97158=CARTESIAN_POINT('Ctrl Pts',(0.0102732016893348,-0.0345231616327823,
0.0686386716231032));
#97159=CARTESIAN_POINT('Ctrl Pts',(0.0103491675916801,-0.0344132092796976,
0.0686682983447179));
#97160=CARTESIAN_POINT('Ctrl Pts',(0.0104245167691668,-0.0343032738558974,
0.0686994948324989));
#97161=CARTESIAN_POINT('Ctrl Pts',(0.0104991537145422,-0.0341934961088741,
0.0687322186474621));
#97162=CARTESIAN_POINT('Ctrl Pts',(0.0102326949624984,-0.0345231616327823,
0.0685328399585627));
#97163=CARTESIAN_POINT('Ctrl Pts',(0.0103101196053404,-0.0344132092796976,
0.0685619083519769));
#97164=CARTESIAN_POINT('Ctrl Pts',(0.0103869389966377,-0.0343032738558974,
0.0685925767132611));
#97165=CARTESIAN_POINT('Ctrl Pts',(0.010463055728293,-0.0341934961088741,
0.0686248032317753));
#97166=CARTESIAN_POINT('Origin',(0.00388982900676628,-0.0345625596231603,
0.084358278701058));
#97167=CARTESIAN_POINT('Ctrl Pts',(0.0107824154971496,-0.0346945769586886,
0.0687711833127807));
#97168=CARTESIAN_POINT('Ctrl Pts',(0.0108565383098119,-0.0345846629176053,
0.0688078206235114));
#97169=CARTESIAN_POINT('Ctrl Pts',(0.0109299161382929,-0.0344746925050311,
0.0688459970213101));
#97170=CARTESIAN_POINT('Ctrl Pts',(0.0110024551644792,-0.0343648066253259,
0.0688856632018872));
#97171=CARTESIAN_POINT('Ctrl Pts',(0.0106774787120365,-0.0346945769586886,
0.0688139547134139));
#97172=CARTESIAN_POINT('Ctrl Pts',(0.0107510121131793,-0.0345846629176053,
0.0688491459422056));
#97173=CARTESIAN_POINT('Ctrl Pts',(0.0108238303338486,-0.0344746925050311,
0.0688858638222829));
#97174=CARTESIAN_POINT('Ctrl Pts',(0.0108958402652469,-0.0343648066253259,
0.0689240609211381));
#97175=CARTESIAN_POINT('Ctrl Pts',(0.0105725419269234,-0.0346945769586886,
0.068856726114047));
#97176=CARTESIAN_POINT('Ctrl Pts',(0.0106454859165468,-0.0345846629176053,
0.0688904712608998));
#97177=CARTESIAN_POINT('Ctrl Pts',(0.0107177445294043,-0.0344746925050311,
0.0689257306232556));
#97178=CARTESIAN_POINT('Ctrl Pts',(0.0107892253660145,-0.0343648066253259,
0.0689624586403891));
#97179=CARTESIAN_POINT('Ctrl Pts',(0.0104676051418103,-0.0346945769586886,
0.0688994975146802));
#97180=CARTESIAN_POINT('Ctrl Pts',(0.0105399597199142,-0.0345846629176053,
0.068931796579594));
#97181=CARTESIAN_POINT('Ctrl Pts',(0.01061165872496,-0.0344746925050311,
0.0689655974242283));
#97182=CARTESIAN_POINT('Ctrl Pts',(0.0106826104667822,-0.0343648066253259,
0.06900085635964));
#97183=CARTESIAN_POINT('Origin',(0.00344537564772737,-0.0345626446730476,
0.084174830085337));
#97184=CARTESIAN_POINT('Ctrl Pts',(0.0104694828127754,-0.0346945769586885,
0.0688987321908996));
#97185=CARTESIAN_POINT('Ctrl Pts',(0.0105794727195282,-0.0345275153362891,
0.068947863829545));
#97186=CARTESIAN_POINT('Ctrl Pts',(0.0106879459304918,-0.0343603235965159,
0.0690004672574773));
#97187=CARTESIAN_POINT('Ctrl Pts',(0.0107945839423478,-0.034193496108874,
0.0690563821289519));
#97188=CARTESIAN_POINT('Ctrl Pts',(0.0103922138933551,-0.0346945769586885,
0.0688662123135492));
#97189=CARTESIAN_POINT('Ctrl Pts',(0.0105028849419592,-0.0345275153362891,
0.0689137255237406));
#97190=CARTESIAN_POINT('Ctrl Pts',(0.0106120903690375,-0.0343603235965159,
0.0689647315258947));
#97191=CARTESIAN_POINT('Ctrl Pts',(0.0107195094354834,-0.034193496108874,
0.0690190746665572));
#97192=CARTESIAN_POINT('Ctrl Pts',(0.0103149449739347,-0.0346945769586885,
0.0688336924361988));
#97193=CARTESIAN_POINT('Ctrl Pts',(0.0104262971643902,-0.0345275153362891,
0.0688795872179362));
#97194=CARTESIAN_POINT('Ctrl Pts',(0.0105362348075832,-0.0343603235965159,
0.068928995794312));
#97195=CARTESIAN_POINT('Ctrl Pts',(0.010644434928619,-0.034193496108874,
0.0689817672041624));
#97196=CARTESIAN_POINT('Ctrl Pts',(0.0102376760545144,-0.0346945769586885,
0.0688011725588484));
#97197=CARTESIAN_POINT('Ctrl Pts',(0.0103497093868212,-0.0345275153362891,
0.0688454489121318));
#97198=CARTESIAN_POINT('Ctrl Pts',(0.010460379246129,-0.0343603235965159,
0.0688932600627293));
#97199=CARTESIAN_POINT('Ctrl Pts',(0.0105693604217546,-0.034193496108874,
0.0689444597417676));
#97200=CARTESIAN_POINT('Ctrl Pts',(0.0106825819614387,-0.0340223579322365,
0.0690008428159775));
#97201=CARTESIAN_POINT('Ctrl Pts',(0.0107536022685714,-0.0339125849573554,
0.0690361353384123));
#97202=CARTESIAN_POINT('Ctrl Pts',(0.0108238421973506,-0.0338030433565221,
0.0690728730165295));
#97203=CARTESIAN_POINT('Ctrl Pts',(0.0108932160874417,-0.0336938721132328,
0.0691110009064204));
#97204=CARTESIAN_POINT('Ctrl Pts',(0.0106488003157574,-0.0340223579322365,
0.0688926763690295));
#97205=CARTESIAN_POINT('Ctrl Pts',(0.0107213125203034,-0.0339125849573554,
0.0689275029544642));
#97206=CARTESIAN_POINT('Ctrl Pts',(0.0107930529419702,-0.0338030433565221,
0.0689638059017995));
#97207=CARTESIAN_POINT('Ctrl Pts',(0.0108639339522631,-0.0336938721132328,
0.0690015306529737));
#97208=CARTESIAN_POINT('Ctrl Pts',(0.0106150186700761,-0.0340223579322365,
0.0687845099220815));
#97209=CARTESIAN_POINT('Ctrl Pts',(0.0106890227720354,-0.0339125849573554,
0.068818870570516));
#97210=CARTESIAN_POINT('Ctrl Pts',(0.0107622636865897,-0.0338030433565221,
0.0688547387870695));
#97211=CARTESIAN_POINT('Ctrl Pts',(0.0108346518170844,-0.0336938721132328,
0.0688920603995271));
#97212=CARTESIAN_POINT('Ctrl Pts',(0.0105812370243948,-0.0340223579322365,
0.0686763434751334));
#97213=CARTESIAN_POINT('Ctrl Pts',(0.0106567330237674,-0.0339125849573554,
0.0687102381865678));
#97214=CARTESIAN_POINT('Ctrl Pts',(0.0107314744312092,-0.0338030433565221,
0.0687456716723394));
#97215=CARTESIAN_POINT('Ctrl Pts',(0.0108053696819057,-0.0336938721132328,
0.0687825901460804));
#97216=CARTESIAN_POINT('Origin',(0.00393827098599277,-0.0345589643415482,
0.0842482502829731));
#97217=CARTESIAN_POINT('Ctrl Pts',(0.0111149079858753,-0.034193496108874,
0.0689487341452375));
#97218=CARTESIAN_POINT('Ctrl Pts',(0.0111866303619451,-0.0340836138581107,
0.0689899799986454));
#97219=CARTESIAN_POINT('Ctrl Pts',(0.0112574648278799,-0.03397388966435,
0.0690326902055963));
#97220=CARTESIAN_POINT('Ctrl Pts',(0.0113273243886923,-0.0338644633294062,
0.0690768040249576));
#97221=CARTESIAN_POINT('Ctrl Pts',(0.0110074924735361,-0.034193496108874,
0.0689848321639676));
#97222=CARTESIAN_POINT('Ctrl Pts',(0.011078717079304,-0.0340836138581107,
0.0690245968210693));
#97223=CARTESIAN_POINT('Ctrl Pts',(0.011149084664026,-0.03397388966435,
0.0690658162421078));
#97224=CARTESIAN_POINT('Ctrl Pts',(0.0112185087023611,-0.0338644633294062,
0.0691084316340294));
#97225=CARTESIAN_POINT('Ctrl Pts',(0.0109000769611969,-0.034193496108874,
0.0690209301826978));
#97226=CARTESIAN_POINT('Ctrl Pts',(0.010970803796663,-0.0340836138581107,
0.0690592136434932));
#97227=CARTESIAN_POINT('Ctrl Pts',(0.0110407045001722,-0.03397388966435,
0.0690989422786194));
#97228=CARTESIAN_POINT('Ctrl Pts',(0.0111096930160299,-0.0338644633294062,
0.0691400592431011));
#97229=CARTESIAN_POINT('Ctrl Pts',(0.0107926614488577,-0.034193496108874,
0.0690570282014279));
#97230=CARTESIAN_POINT('Ctrl Pts',(0.0108628905140219,-0.0340836138581107,
0.0690938304659171));
#97231=CARTESIAN_POINT('Ctrl Pts',(0.0109323243363184,-0.03397388966435,
0.069132068315131));
#97232=CARTESIAN_POINT('Ctrl Pts',(0.0110008773296986,-0.0338644633294062,
0.0691716868521729));
#97233=CARTESIAN_POINT('Origin',(0.00347824005280992,-0.0345610621863455,
0.0841071065547872));
#97234=CARTESIAN_POINT('Ctrl Pts',(0.0107624911018675,-0.03424362768739,
0.0690396829555461));
#97235=CARTESIAN_POINT('Ctrl Pts',(0.0109552298865343,-0.033943005420186,
0.0691392035026549));
#97236=CARTESIAN_POINT('Ctrl Pts',(0.0111399248251389,-0.0336441434784162,
0.0692529591973061));
#97237=CARTESIAN_POINT('Ctrl Pts',(0.0105379154826387,-0.03424362768739,
0.068929838559931));
#97238=CARTESIAN_POINT('Ctrl Pts',(0.0107347971169819,-0.033943005420186,
0.069020889097931));
#97239=CARTESIAN_POINT('Ctrl Pts',(0.010924261131652,-0.0336441434784162,
0.0691265109022937));
#97240=CARTESIAN_POINT('Ctrl Pts',(0.0110008532565233,-0.0335235895815128,
0.0691716730859124));
#97241=CARTESIAN_POINT('Ctrl Pts',(0.0110693897279185,-0.0334144449262719,
0.0692112816335314));
#97242=CARTESIAN_POINT('Ctrl Pts',(0.0111371866566308,-0.0333049234473133,
0.0692523515984925));
#97243=CARTESIAN_POINT('Ctrl Pts',(0.0112041525940881,-0.0331951640388588,
0.0692948383178068));
#97244=CARTESIAN_POINT('Ctrl Pts',(0.0109739301564992,-0.0335235895815128,
0.0690615989328548));
#97245=CARTESIAN_POINT('Ctrl Pts',(0.0110439820153273,-0.0334144449262719,
0.0691008368309952));
#97246=CARTESIAN_POINT('Ctrl Pts',(0.0111133037298084,-0.0333049234473133,
0.0691415670274103));
#97247=CARTESIAN_POINT('Ctrl Pts',(0.0111818019409926,-0.0331951640388588,
0.0691837454701862));
#97248=CARTESIAN_POINT('Ctrl Pts',(0.0109470070564751,-0.0335235895815128,
0.0689515247797971));
#97249=CARTESIAN_POINT('Ctrl Pts',(0.0110185743027361,-0.0334144449262719,
0.0689903920284591));
#97250=CARTESIAN_POINT('Ctrl Pts',(0.0110894208029859,-0.0333049234473133,
0.0690307824563282));
#97251=CARTESIAN_POINT('Ctrl Pts',(0.011159451287897,-0.0331951640388588,
0.0690726526225656));
#97252=CARTESIAN_POINT('Ctrl Pts',(0.0109200839564511,-0.0335235895815128,
0.0688414506267395));
#97253=CARTESIAN_POINT('Ctrl Pts',(0.0109931665901449,-0.0334144449262719,
0.0688799472259229));
#97254=CARTESIAN_POINT('Ctrl Pts',(0.0110655378761634,-0.0333049234473133,
0.0689199978852461));
#97255=CARTESIAN_POINT('Ctrl Pts',(0.0111371006348015,-0.0331951640388588,
0.0689615597749449));
#97256=CARTESIAN_POINT('Origin',(0.00164177990531128,-0.0326434571770353,
0.0829459140857844));
#97257=CARTESIAN_POINT('Ctrl Pts',(0.0114375545749916,-0.0336938721132355,
0.0691462880642782));
#97258=CARTESIAN_POINT('Ctrl Pts',(0.011466842961358,-0.0336474569764941,
0.0691656846736549));
#97259=CARTESIAN_POINT('Ctrl Pts',(0.0114959022790625,-0.033601104548885,
0.0691854228115053));
#97260=CARTESIAN_POINT('Ctrl Pts',(0.0115694737871713,-0.0334837508643153,
0.0692353952363117));
#97261=CARTESIAN_POINT('Ctrl Pts',(0.0116415322016055,-0.0333660264760389,
0.0692875257931444));
#97262=CARTESIAN_POINT('Ctrl Pts',(0.0111091446375875,-0.0336938721132355,
0.0692341342496876));
#97263=CARTESIAN_POINT('Ctrl Pts',(0.0111379188310802,-0.0336474569764941,
0.0692516085667228));
#97264=CARTESIAN_POINT('Ctrl Pts',(0.0111664864940029,-0.033601104548885,
0.0692694185246716));
#97265=CARTESIAN_POINT('Ctrl Pts',(0.011238813245296,-0.0334837508643153,
0.0693145092414934));
#97266=CARTESIAN_POINT('Ctrl Pts',(0.0113097721046427,-0.0333660264760389,
0.0693617233493038));
#97267=CARTESIAN_POINT('Ctrl Pts',(0.0111091446375992,-0.0336938721132427,
0.0692341342496987));
#97268=CARTESIAN_POINT('Ctrl Pts',(0.011137918831091,-0.0336474569765026,
0.0692516085667332));
#97269=CARTESIAN_POINT('Ctrl Pts',(0.0111664864940129,-0.0336011045488949,
0.0692694185246816));
#97270=CARTESIAN_POINT('Ctrl Pts',(0.0112382108619794,-0.0334847282606778,
0.0693141336972473));
#97271=CARTESIAN_POINT('Ctrl Pts',(0.0113085902837036,-0.0333679869945434,
0.0693609372079656));
#97272=CARTESIAN_POINT('Ctrl Pts',(0.0111091446375831,-0.0336938721132426,
0.0692341342496849));
#97273=CARTESIAN_POINT('Ctrl Pts',(0.0112120538873638,-0.0335278710435083,
0.0692966301405592));
#97274=CARTESIAN_POINT('Ctrl Pts',(0.0113129670790205,-0.033362046922432,
0.0693623312528415));
#97275=CARTESIAN_POINT('Ctrl Pts',(0.0114119234711438,-0.0331951640388602,
0.0694312870466959));
#97276=CARTESIAN_POINT('Ctrl Pts',(0.0110365608203503,-0.0336938721132426,
0.0691921864333031));
#97277=CARTESIAN_POINT('Ctrl Pts',(0.0111403482101237,-0.0335278710435083,
0.0692531628469262));
#97278=CARTESIAN_POINT('Ctrl Pts',(0.011242186883257,-0.033362046922432,
0.0693173725547477));
#97279=CARTESIAN_POINT('Ctrl Pts',(0.0113421168066779,-0.0331951640388602,
0.0693848644291541));
#97280=CARTESIAN_POINT('Ctrl Pts',(0.0109639770031176,-0.0336938721132426,
0.0691502386169214));
#97281=CARTESIAN_POINT('Ctrl Pts',(0.0110686425328836,-0.0335278710435083,
0.0692096955532933));
#97282=CARTESIAN_POINT('Ctrl Pts',(0.0111714066874934,-0.033362046922432,
0.0692724138566539));
#97283=CARTESIAN_POINT('Ctrl Pts',(0.0112723101422121,-0.0331951640388602,
0.0693384418116124));
#97284=CARTESIAN_POINT('Ctrl Pts',(0.0108913931858848,-0.0336938721132426,
0.0691082908005396));
#97285=CARTESIAN_POINT('Ctrl Pts',(0.0109969368556435,-0.0335278710435083,
0.0691662282596603));
#97286=CARTESIAN_POINT('Ctrl Pts',(0.0111006264917299,-0.033362046922432,
0.0692274551585602));
#97287=CARTESIAN_POINT('Ctrl Pts',(0.0112025034777462,-0.0331951640388602,
0.0692920191940707));
#97288=CARTESIAN_POINT('Ctrl Pts',(0.0113077668952985,-0.0330240426238156,
0.0693621484780575));
#97289=CARTESIAN_POINT('Ctrl Pts',(0.0113737242145906,-0.0329142774063509,
0.069406010969336));
#97290=CARTESIAN_POINT('Ctrl Pts',(0.0114388076557933,-0.0328043479726686,
0.0694512588496985));
#97291=CARTESIAN_POINT('Ctrl Pts',(0.0115029322458005,-0.0326943950436594,
0.0694978364494208));
#97292=CARTESIAN_POINT('Ctrl Pts',(0.0112878085456185,-0.0330240426238156,
0.0692506011774958));
#97293=CARTESIAN_POINT('Ctrl Pts',(0.0113553025376511,-0.0329142774063509,
0.069294188723063));
#97294=CARTESIAN_POINT('Ctrl Pts',(0.0114219291015776,-0.0328043479726686,
0.0693391932879617));
#97295=CARTESIAN_POINT('Ctrl Pts',(0.011487601296021,-0.0326943950436594,
0.0693855595686153));
#97296=CARTESIAN_POINT('Ctrl Pts',(0.0112678501959385,-0.0330240426238156,
0.0691390538769341));
#97297=CARTESIAN_POINT('Ctrl Pts',(0.0113368808607116,-0.0329142774063509,
0.0691823664767899));
#97298=CARTESIAN_POINT('Ctrl Pts',(0.0114050505473619,-0.0328043479726686,
0.0692271277262249));
#97299=CARTESIAN_POINT('Ctrl Pts',(0.0114722703462415,-0.0326943950436594,
0.0692732826878098));
#97300=CARTESIAN_POINT('Ctrl Pts',(0.0112478918462585,-0.0330240426238156,
0.0690275065763724));
#97301=CARTESIAN_POINT('Ctrl Pts',(0.0113184591837721,-0.0329142774063509,
0.0690705442305169));
#97302=CARTESIAN_POINT('Ctrl Pts',(0.0113881719931461,-0.0328043479726686,
0.0691150621644881));
#97303=CARTESIAN_POINT('Ctrl Pts',(0.011456939396462,-0.0326943950436594,
0.0691610058070043));
#97304=CARTESIAN_POINT('Origin',(0.00157065334461952,-0.0326396682857218,
0.0830470892373371));
#97305=CARTESIAN_POINT('Ctrl Pts',(0.0117432135338,-0.0331951640388588,
0.0693646351476499));
#97306=CARTESIAN_POINT('Ctrl Pts',(0.0118091222539269,-0.0330855618255041,
0.0694144854923179));
#97307=CARTESIAN_POINT('Ctrl Pts',(0.0118740481653163,-0.0329757224427708,
0.0694657339939863));
#97308=CARTESIAN_POINT('Ctrl Pts',(0.0119379049073101,-0.0328657862078597,
0.0695183191041373));
#97309=CARTESIAN_POINT('Ctrl Pts',(0.0116321207746222,-0.0331951640388588,
0.0693869857829517));
#97310=CARTESIAN_POINT('Ctrl Pts',(0.0116977216599627,-0.0330855618255041,
0.0694353060496009));
#97311=CARTESIAN_POINT('Ctrl Pts',(0.0117623711387492,-0.0329757224427708,
0.0694850170078197));
#97312=CARTESIAN_POINT('Ctrl Pts',(0.0118259833008915,-0.0328657862078597,
0.0695360590606433));
#97313=CARTESIAN_POINT('Ctrl Pts',(0.0115210280154443,-0.0331951640388588,
0.0694093364182535));
#97314=CARTESIAN_POINT('Ctrl Pts',(0.0115863210659985,-0.0330855618255041,
0.0694561266068838));
#97315=CARTESIAN_POINT('Ctrl Pts',(0.0116506941121821,-0.0329757224427708,
0.0695043000216531));
#97316=CARTESIAN_POINT('Ctrl Pts',(0.011714061694473,-0.0328657862078597,
0.0695537990171493));
#97317=CARTESIAN_POINT('Ctrl Pts',(0.0114099352562665,-0.0331951640388588,
0.0694316870535553));
#97318=CARTESIAN_POINT('Ctrl Pts',(0.0114749204720344,-0.0330855618255041,
0.0694769471641668));
#97319=CARTESIAN_POINT('Ctrl Pts',(0.011539017085615,-0.0329757224427708,
0.0695235830354865));
#97320=CARTESIAN_POINT('Ctrl Pts',(0.0116021400880544,-0.0328657862078597,
0.0695715389736553));
#97321=CARTESIAN_POINT('Origin',(0.0012075486003039,-0.0326401908836129,
0.0827317674714501));
#97322=CARTESIAN_POINT('Ctrl Pts',(0.0113822363703565,-0.0332451089994432,
0.0694107383091061));
#97323=CARTESIAN_POINT('Ctrl Pts',(0.0115609805494362,-0.0329451141710258,
0.0695336329190619));
#97324=CARTESIAN_POINT('Ctrl Pts',(0.0117299600107489,-0.0326442513127503,
0.0696696421406814));
#97325=CARTESIAN_POINT('Ctrl Pts',(0.0111732004780954,-0.0332451089994432,
0.0692736106468835));
#97326=CARTESIAN_POINT('Ctrl Pts',(0.0113571165115718,-0.0329451141710258,
0.0693886213391751));
#97327=CARTESIAN_POINT('Ctrl Pts',(0.0115318469834969,-0.0326442513127503,
0.0695171586057243));
#97328=CARTESIAN_POINT('Ctrl Pts',(0.011602114990133,-0.0325229783203385,
0.0695715197935932));
#97329=CARTESIAN_POINT('Ctrl Pts',(0.0116652292385048,-0.032413025311208,
0.0696194685342614));
#97330=CARTESIAN_POINT('Ctrl Pts',(0.0117273420330872,-0.0323031222247695,
0.0696687156018434));
#97331=CARTESIAN_POINT('Ctrl Pts',(0.0117883760377646,-0.0321934096636184,
0.0697191951068656));
#97332=CARTESIAN_POINT('Ctrl Pts',(0.0115892001152709,-0.0325229783203385,
0.069458939383856));
#97333=CARTESIAN_POINT('Ctrl Pts',(0.0116538662821006,-0.032413025311208,
0.0695067100932598));
#97334=CARTESIAN_POINT('Ctrl Pts',(0.0117175344425675,-0.0323031222247695,
0.0695558112600057));
#97335=CARTESIAN_POINT('Ctrl Pts',(0.0117801252616482,-0.0321934096636184,
0.0696061771112066));
#97336=CARTESIAN_POINT('Ctrl Pts',(0.0115762852404087,-0.0325229783203385,
0.0693463589741187));
#97337=CARTESIAN_POINT('Ctrl Pts',(0.0116425033256965,-0.032413025311208,
0.0693939516522582));
#97338=CARTESIAN_POINT('Ctrl Pts',(0.0117077268520479,-0.0323031222247695,
0.069442906918168));
#97339=CARTESIAN_POINT('Ctrl Pts',(0.0117718744855319,-0.0321934096636184,
0.0694931591155475));
#97340=CARTESIAN_POINT('Ctrl Pts',(0.0115633703655466,-0.0325229783203385,
0.0692337785643814));
#97341=CARTESIAN_POINT('Ctrl Pts',(0.0116311403692924,-0.032413025311208,
0.0692811932112566));
#97342=CARTESIAN_POINT('Ctrl Pts',(0.0116979192615282,-0.0323031222247695,
0.0693300025763304));
#97343=CARTESIAN_POINT('Ctrl Pts',(0.0117636237094155,-0.0321934096636184,
0.0693801411198884));
#97344=CARTESIAN_POINT('Origin',(0.00157589958277574,-0.0326393375179485,
0.0830403685218024));
#97345=CARTESIAN_POINT('Ctrl Pts',(0.0120365469580468,-0.0326943950436594,
0.0696013439463559));
#97346=CARTESIAN_POINT('Ctrl Pts',(0.0120992359635559,-0.0325844576448127,
0.0696552691781193));
#97347=CARTESIAN_POINT('Ctrl Pts',(0.0121608141434588,-0.0324744968375319,
0.0697104947376692));
#97348=CARTESIAN_POINT('Ctrl Pts',(0.0122212035761687,-0.0323646534831895,
0.0697669487785634));
#97349=CARTESIAN_POINT('Ctrl Pts',(0.0119242701139744,-0.0326943950436594,
0.0696166748911197));
#97350=CARTESIAN_POINT('Ctrl Pts',(0.0119867478303313,-0.0325844576448127,
0.0696690527375426));
#97351=CARTESIAN_POINT('Ctrl Pts',(0.0120481467085947,-0.0324744968375319,
0.0697227264324349));
#97352=CARTESIAN_POINT('Ctrl Pts',(0.0121083890294841,-0.0323646534831895,
0.0697776261208629));
#97353=CARTESIAN_POINT('Ctrl Pts',(0.0118119932699019,-0.0326943950436594,
0.0696320058358835));
#97354=CARTESIAN_POINT('Ctrl Pts',(0.0118742596971068,-0.0325844576448127,
0.0696828362969658));
#97355=CARTESIAN_POINT('Ctrl Pts',(0.0119354792737306,-0.0324744968375319,
0.0697349581272007));
#97356=CARTESIAN_POINT('Ctrl Pts',(0.0119955744827996,-0.0323646534831895,
0.0697883034631624));
#97357=CARTESIAN_POINT('Ctrl Pts',(0.0116997164258294,-0.0326943950436594,
0.0696473367806473));
#97358=CARTESIAN_POINT('Ctrl Pts',(0.0117617715638822,-0.0325844576448127,
0.0696966198563891));
#97359=CARTESIAN_POINT('Ctrl Pts',(0.0118228118388665,-0.0324744968375319,
0.0697471898219664));
#97360=CARTESIAN_POINT('Ctrl Pts',(0.011882759936115,-0.0323646534831895,
0.0697989808054619));
#97361=CARTESIAN_POINT('Origin',(0.00118416138267592,-0.0326395579069507,
0.0827615164191161));
#97362=CARTESIAN_POINT('Ctrl Pts',(0.0116733563971562,-0.0327445246961877,
0.0696246659824982));
#97363=CARTESIAN_POINT('Ctrl Pts',(0.0118440321580191,-0.0324436878365475,
0.069758540360759));
#97364=CARTESIAN_POINT('Ctrl Pts',(0.0120041390818642,-0.0321434074463186,
0.0699048904117932));
#97365=CARTESIAN_POINT('Ctrl Pts',(0.0114733422837796,-0.0327445246961877,
0.0694746848021782));
#97366=CARTESIAN_POINT('Ctrl Pts',(0.0116496746772728,-0.0324436878365475,
0.0696010155249095));
#97367=CARTESIAN_POINT('Ctrl Pts',(0.0118159903828125,-0.0321434074463186,
0.0697402694318267));
#97368=CARTESIAN_POINT('Ctrl Pts',(0.0119546736389694,-0.0322357242816072,
0.0698601986374625));
#97369=CARTESIAN_POINT('Ctrl Pts',(0.0120912982486977,-0.0319819883628705,
0.0699822075615288));
#97370=CARTESIAN_POINT('Ctrl Pts',(0.0122198821948262,-0.0317295851069886,
0.0701126630341365));
#97371=CARTESIAN_POINT('Ctrl Pts',(0.0117646294688016,-0.0322357242816072,
0.0696977695348199));
#97372=CARTESIAN_POINT('Ctrl Pts',(0.0119064272347863,-0.0319819883628705,
0.0698137257985448));
#97373=CARTESIAN_POINT('Ctrl Pts',(0.0120405590012207,-0.0317295851069886,
0.0699384700600097));
#97374=CARTESIAN_POINT('Origin',(0.00124527771626521,-0.0326371942645812,
0.0826883918865079));
#97375=CARTESIAN_POINT('Origin',(0.00165101033500555,-0.032635298553037,
0.0829433006175441));
#97376=CARTESIAN_POINT('Ctrl Pts',(0.0123144384873387,-0.0321934096636184,
0.0698560042124227));
#97377=CARTESIAN_POINT('Ctrl Pts',(0.0123736560357861,-0.0320835708272304,
0.0699137966287189));
#97378=CARTESIAN_POINT('Ctrl Pts',(0.0124316432245973,-0.0319739230346346,
0.0699727810271523));
#97379=CARTESIAN_POINT('Ctrl Pts',(0.0124883316550263,-0.0318646057455575,
0.0700328762473571));
#97380=CARTESIAN_POINT('Ctrl Pts',(0.0122014203943551,-0.0321934096636184,
0.0698642549956441));
#97381=CARTESIAN_POINT('Ctrl Pts',(0.0122605241580717,-0.0320835708272304,
0.0699204888043572));
#97382=CARTESIAN_POINT('Ctrl Pts',(0.0123184298834547,-0.0319739230346346,
0.069977913144494));
#97383=CARTESIAN_POINT('Ctrl Pts',(0.0123750691227986,-0.0318646057455575,
0.0700364488596744));
#97384=CARTESIAN_POINT('Ctrl Pts',(0.0120884023013716,-0.0321934096636184,
0.0698725057788655));
#97385=CARTESIAN_POINT('Ctrl Pts',(0.0121473922803572,-0.0320835708272304,
0.0699271809799954));
#97386=CARTESIAN_POINT('Ctrl Pts',(0.0122052165423121,-0.0319739230346346,
0.0699830452618357));
#97387=CARTESIAN_POINT('Ctrl Pts',(0.0122618065905709,-0.0318646057455575,
0.0700400214719917));
#97388=CARTESIAN_POINT('Ctrl Pts',(0.0119753842083881,-0.0321934096636184,
0.069880756562087));
#97389=CARTESIAN_POINT('Ctrl Pts',(0.0120342604026428,-0.0320835708272304,
0.0699338731556337));
#97390=CARTESIAN_POINT('Ctrl Pts',(0.0120920032011695,-0.0319739230346346,
0.0699881773791775));
#97391=CARTESIAN_POINT('Ctrl Pts',(0.0121485440583432,-0.0318646057455575,
0.070043594084309));
#97392=CARTESIAN_POINT('Ctrl Pts',(0.0118829453910787,-0.0320218834582305,
0.0697980475816695));
#97393=CARTESIAN_POINT('Ctrl Pts',(0.0119282386949749,-0.0319391099350621,
0.0698371713828407));
#97394=CARTESIAN_POINT('Ctrl Pts',(0.011972893633168,-0.0318564869454922,
0.0698769787411859));
#97395=CARTESIAN_POINT('Ctrl Pts',(0.0120168803872852,-0.0317740741446535,
0.069917437625872));
#97396=CARTESIAN_POINT('Ctrl Pts',(0.0118804025510494,-0.0320218834582305,
0.0697485464502481));
#97397=CARTESIAN_POINT('Ctrl Pts',(0.0119262110420555,-0.0319391099350621,
0.0697876437866018));
#97398=CARTESIAN_POINT('Ctrl Pts',(0.0119713812684715,-0.0318564869454922,
0.069827432740883));
#97399=CARTESIAN_POINT('Ctrl Pts',(0.0120158830353541,-0.0317740741446535,
0.0698678812606245));
#97400=CARTESIAN_POINT('Ctrl Pts',(0.0118778597110201,-0.0320218834582305,
0.0696990453188266));
#97401=CARTESIAN_POINT('Ctrl Pts',(0.011924183389136,-0.0319391099350621,
0.069738116190363));
#97402=CARTESIAN_POINT('Ctrl Pts',(0.011969868903775,-0.0318564869454922,
0.06977788674058));
#97403=CARTESIAN_POINT('Ctrl Pts',(0.012014885683423,-0.0317740741446535,
0.069818324895377));
#97404=CARTESIAN_POINT('Ctrl Pts',(0.0118753168709907,-0.0320218834582305,
0.0696495441874052));
#97405=CARTESIAN_POINT('Ctrl Pts',(0.0119221557362166,-0.0319391099350621,
0.0696885885941241));
#97406=CARTESIAN_POINT('Ctrl Pts',(0.0119683565390784,-0.0318564869454922,
0.069728340740277));
#97407=CARTESIAN_POINT('Ctrl Pts',(0.0120138883314918,-0.0317740741446535,
0.0697687685301295));
#97408=CARTESIAN_POINT('Origin',(0.0152822549363563,-0.0391228853390692,
0.0644218508279418));
#97409=CARTESIAN_POINT('Ctrl Pts',(0.00914413420753776,-0.0352722978779543,
0.06848934223705));
#97410=CARTESIAN_POINT('Ctrl Pts',(0.00916266609167554,-0.0352466642097183,
0.068493038444335));
#97411=CARTESIAN_POINT('Ctrl Pts',(0.00918119680116501,-0.0352210183808283,
0.0684966544721222));
#97412=CARTESIAN_POINT('Ctrl Pts',(0.00919972709192561,-0.0351953608940152,
0.0685001899253548));
#97413=CARTESIAN_POINT('Origin',(0.010279560610078,-0.0352456003065005,
0.0637227344203754));
#97414=CARTESIAN_POINT('Ctrl Pts',(0.0093216507798621,-0.0350241211493339,
0.0685262653877318));
#97415=CARTESIAN_POINT('Ctrl Pts',(0.00939911541483222,-0.0349144232867421,
0.0685427655356251));
#97416=CARTESIAN_POINT('Ctrl Pts',(0.00947628534628622,-0.0348045283677512,
0.0685608768089376));
#97417=CARTESIAN_POINT('Ctrl Pts',(0.00955306086609633,-0.0346945769586886,
0.0685805796876788));
#97418=CARTESIAN_POINT('Ctrl Pts',(0.0092620306643769,-0.0350241211493339,
0.0684298984658524));
#97419=CARTESIAN_POINT('Ctrl Pts',(0.00934082271412408,-0.0349144232867421,
0.0684455773711371));
#97420=CARTESIAN_POINT('Ctrl Pts',(0.00941933783054762,-0.0348045283677512,
0.0684628943488985));
#97421=CARTESIAN_POINT('Ctrl Pts',(0.00949747462036837,-0.0346945769586886,
0.0684818309606548));
#97422=CARTESIAN_POINT('Ctrl Pts',(0.00920241054889171,-0.0350241211493339,
0.068333531543973));
#97423=CARTESIAN_POINT('Ctrl Pts',(0.00928253001341594,-0.0349144232867421,
0.0683483892066491));
#97424=CARTESIAN_POINT('Ctrl Pts',(0.00936239031480901,-0.0348045283677512,
0.0683649118888594));
#97425=CARTESIAN_POINT('Ctrl Pts',(0.00944188837464041,-0.0346945769586886,
0.0683830822336308));
#97426=CARTESIAN_POINT('Ctrl Pts',(0.00914279043340651,-0.0350241211493339,
0.0682371646220936));
#97427=CARTESIAN_POINT('Ctrl Pts',(0.00922423731270781,-0.0349144232867421,
0.0682512010421611));
#97428=CARTESIAN_POINT('Ctrl Pts',(0.0093054427990704,-0.0348045283677512,
0.0682669294288202));
#97429=CARTESIAN_POINT('Ctrl Pts',(0.00938630212891245,-0.0346945769586886,
0.0682843335066068));
#97430=CARTESIAN_POINT('Origin',(0.0052056087878164,-0.0345629067941657,
0.0847967015889882));
#97431=CARTESIAN_POINT('Ctrl Pts',(0.00964823368459569,-0.035197097365166,
0.0684183711366379));
#97432=CARTESIAN_POINT('Ctrl Pts',(0.00972763763476626,-0.0350869349321805,
0.0684394903460552));
#97433=CARTESIAN_POINT('Ctrl Pts',(0.00980666830558493,-0.0349764985129744,
0.0684622778145007));
#97434=CARTESIAN_POINT('Ctrl Pts',(0.00988522157266863,-0.0348659306849651,
0.0684867100472114));
#97435=CARTESIAN_POINT('Ctrl Pts',(0.00957926827321185,-0.035197097365166,
0.0684631399056924));
#97436=CARTESIAN_POINT('Ctrl Pts',(0.00965805201275959,-0.0350869349321805,
0.0684833036927996));
#97437=CARTESIAN_POINT('Ctrl Pts',(0.00973648182188052,-0.0349764985129744,
0.0685051220536392));
#97438=CARTESIAN_POINT('Ctrl Pts',(0.00981445442853207,-0.0348659306849651,
0.0685285727031323));
#97439=CARTESIAN_POINT('Ctrl Pts',(0.009510302861828,-0.035197097365166,
0.0685079086747469));
#97440=CARTESIAN_POINT('Ctrl Pts',(0.00958846639075291,-0.0350869349321805,
0.0685271170395441));
#97441=CARTESIAN_POINT('Ctrl Pts',(0.00966629533817611,-0.0349764985129744,
0.0685479662927777));
#97442=CARTESIAN_POINT('Ctrl Pts',(0.0097436872843955,-0.0348659306849652,
0.0685704353590531));
#97443=CARTESIAN_POINT('Ctrl Pts',(0.00944133745044416,-0.035197097365166,
0.0685526774438014));
#97444=CARTESIAN_POINT('Ctrl Pts',(0.00951888076874623,-0.0350869349321805,
0.0685709303862885));
#97445=CARTESIAN_POINT('Ctrl Pts',(0.0095961088544717,-0.0349764985129744,
0.0685908105319162));
#97446=CARTESIAN_POINT('Ctrl Pts',(0.00967292014025894,-0.0348659306849652,
0.068612298014974));
#97447=CARTESIAN_POINT('Origin',(0.0047558508444338,-0.0345637187965071,
0.0846262810831878));
#97448=CARTESIAN_POINT('Ctrl Pts',(0.00940878355743313,-0.0352450361861253,
0.0685440302807021));
#97449=CARTESIAN_POINT('Ctrl Pts',(0.00962021616940426,-0.0349452761023765,
0.0685924949011781));
#97450=CARTESIAN_POINT('Ctrl Pts',(0.00982739757019066,-0.0346444289983475,
0.0686567478078128));
#97451=CARTESIAN_POINT('Ctrl Pts',(0.00916394689380343,-0.0352450361861253,
0.0684934831923322));
#97452=CARTESIAN_POINT('Ctrl Pts',(0.00937728592044621,-0.0349452761023765,
0.0685327136467514));
#97453=CARTESIAN_POINT('Ctrl Pts',(0.0095870638751338,-0.0346444289983475,
0.0685879022195713));
#97454=CARTESIAN_POINT('Ctrl Pts',(0.00967240335574919,-0.0345231616327822,
0.0686125770201603));
#97455=CARTESIAN_POINT('Ctrl Pts',(0.00974872893545784,-0.0344132092796975,
0.068633922582603));
#97456=CARTESIAN_POINT('Ctrl Pts',(0.00982460906099546,-0.0343032738558974,
0.0686568457781242));
#97457=CARTESIAN_POINT('Ctrl Pts',(0.00989994727340524,-0.034193496108874,
0.0686813147493598));
#97458=CARTESIAN_POINT('Ctrl Pts',(0.00961895181182228,-0.0345231616327822,
0.0685126567089605));
#97459=CARTESIAN_POINT('Ctrl Pts',(0.00969665465234427,-0.0344132092796975,
0.0685332655171239));
#97460=CARTESIAN_POINT('Ctrl Pts',(0.00977392720681601,-0.0343032738558974,
0.0685554804839326));
#97461=CARTESIAN_POINT('Ctrl Pts',(0.00985067120917691,-0.034193496108874,
0.0685792706136508));
#97462=CARTESIAN_POINT('Ctrl Pts',(0.00956550026789536,-0.0345231616327822,
0.0684127363977608));
#97463=CARTESIAN_POINT('Ctrl Pts',(0.00964458036923068,-0.0344132092796975,
0.0684326084516449));
#97464=CARTESIAN_POINT('Ctrl Pts',(0.00972324535263657,-0.0343032738558974,
0.068454115189741));
#97465=CARTESIAN_POINT('Ctrl Pts',(0.00980139514494859,-0.034193496108874,
0.0684772264779418));
#97466=CARTESIAN_POINT('Ctrl Pts',(0.00951204872396846,-0.0345231616327822,
0.068312816086561));
#97467=CARTESIAN_POINT('Ctrl Pts',(0.00959250608611711,-0.0344132092796975,
0.0683319513861659));
#97468=CARTESIAN_POINT('Ctrl Pts',(0.00967256349845712,-0.0343032738558974,
0.0683527498955494));
#97469=CARTESIAN_POINT('Ctrl Pts',(0.00975211908072027,-0.034193496108874,
0.0683751823422328));
#97470=CARTESIAN_POINT('Origin',(0.00520265157077387,-0.0345625596229807,
0.0848084384179098));
#97471=CARTESIAN_POINT('Ctrl Pts',(0.0100873068912915,-0.0346945769586886,
0.0684803817800777));
#97472=CARTESIAN_POINT('Ctrl Pts',(0.0101654370960595,-0.0345846629176053,
0.0685074401428784));
#97473=CARTESIAN_POINT('Ctrl Pts',(0.010243021089828,-0.0344746925050311,
0.0685361188278624));
#97474=CARTESIAN_POINT('Ctrl Pts',(0.0103199596148012,-0.034364806625326,
0.0685663806780462));
#97475=CARTESIAN_POINT('Ctrl Pts',(0.00998855824201811,-0.0346945769586886,
0.0685359679820395));
#97476=CARTESIAN_POINT('Ctrl Pts',(0.0100659224408271,-0.0345846629176053,
0.0685616655385408));
#97477=CARTESIAN_POINT('Ctrl Pts',(0.0101427684387163,-0.0344746925050311,
0.0685889673441078));
#97478=CARTESIAN_POINT('Ctrl Pts',(0.0102189979162095,-0.034364806625326,
0.0686178380098787));
#97479=CARTESIAN_POINT('Ctrl Pts',(0.00988980959274471,-0.0346945769586886,
0.0685915541840012));
#97480=CARTESIAN_POINT('Ctrl Pts',(0.00996640778559471,-0.0345846629176053,
0.0686158909342032));
#97481=CARTESIAN_POINT('Ctrl Pts',(0.0100425157876047,-0.0344746925050311,
0.0686418158603531));
#97482=CARTESIAN_POINT('Ctrl Pts',(0.0101180362176177,-0.034364806625326,
0.0686692953417112));
#97483=CARTESIAN_POINT('Ctrl Pts',(0.00979106094347131,-0.0346945769586886,
0.0686471403859629));
#97484=CARTESIAN_POINT('Ctrl Pts',(0.00986689313036234,-0.0345846629176053,
0.0686701163298657));
#97485=CARTESIAN_POINT('Ctrl Pts',(0.00994226313649308,-0.0344746925050311,
0.0686946643765985));
#97486=CARTESIAN_POINT('Ctrl Pts',(0.010017074519026,-0.034364806625326,
0.0687207526735436));
#97487=CARTESIAN_POINT('Origin',(0.00473871065156685,-0.0345626446731966,
0.0846821411257449));
#97488=CARTESIAN_POINT('Ctrl Pts',(0.00979282788793581,-0.0346945769586886,
0.0686461457624153));
#97489=CARTESIAN_POINT('Ctrl Pts',(0.00990810831856319,-0.0345275153362891,
0.0686811045927423));
#97490=CARTESIAN_POINT('Ctrl Pts',(0.0100223191435783,-0.0343603235965159,
0.0687196979286484));
#97491=CARTESIAN_POINT('Ctrl Pts',(0.0101351242745059,-0.034193496108874,
0.0687618066078137));
#97492=CARTESIAN_POINT('Ctrl Pts',(0.00971209243564077,-0.0346945769586886,
0.068623566677536));
#97493=CARTESIAN_POINT('Ctrl Pts',(0.00982784579424111,-0.0345275153362891,
0.0686568344714901));
#97494=CARTESIAN_POINT('Ctrl Pts',(0.00994258285109001,-0.0343603235965159,
0.0686937512067839));
#97495=CARTESIAN_POINT('Ctrl Pts',(0.0100559658876537,-0.034193496108874,
0.0687342026566066));
#97496=CARTESIAN_POINT('Ctrl Pts',(0.00963135698334572,-0.0346945769586886,
0.0686009875926567));
#97497=CARTESIAN_POINT('Ctrl Pts',(0.00974758326991903,-0.0345275153362891,
0.0686325643502378));
#97498=CARTESIAN_POINT('Ctrl Pts',(0.00986284655860173,-0.0343603235965159,
0.0686678044849194));
#97499=CARTESIAN_POINT('Ctrl Pts',(0.0099768075008016,-0.034193496108874,
0.0687065987053996));
#97500=CARTESIAN_POINT('Ctrl Pts',(0.00955062153105068,-0.0346945769586886,
0.0685784085077774));
#97501=CARTESIAN_POINT('Ctrl Pts',(0.00966732074559696,-0.0345275153362891,
0.0686082942289855));
#97502=CARTESIAN_POINT('Ctrl Pts',(0.00978311026611345,-0.0343603235965159,
0.068641857763055));
#97503=CARTESIAN_POINT('Ctrl Pts',(0.00989764911394947,-0.034193496108874,
0.0686789947541926));
#97504=CARTESIAN_POINT('Ctrl Pts',(0.0100170445409845,-0.0340223579322365,
0.0687207428093437));
#97505=CARTESIAN_POINT('Ctrl Pts',(0.0100919281577402,-0.0339125849573554,
0.0687468558349562));
#97506=CARTESIAN_POINT('Ctrl Pts',(0.0101662186756934,-0.0338030433565221,
0.0687745004281092));
#97507=CARTESIAN_POINT('Ctrl Pts',(0.0102398242236691,-0.0336938721132327,
0.06880363281423));
#97508=CARTESIAN_POINT('Ctrl Pts',(0.00996997242311036,-0.0340223579322365,
0.068617663250026));
#97509=CARTESIAN_POINT('Ctrl Pts',(0.0100462777758317,-0.0339125849573554,
0.0686431270283638));
#97510=CARTESIAN_POINT('Ctrl Pts',(0.0101220024686233,-0.0338030433565221,
0.0686701522570915));
#97511=CARTESIAN_POINT('Ctrl Pts',(0.0101970527260289,-0.0336938721132327,
0.0686986957911165));
#97512=CARTESIAN_POINT('Ctrl Pts',(0.00992290030523617,-0.0340223579322365,
0.0685145836907083));
#97513=CARTESIAN_POINT('Ctrl Pts',(0.0100006273939233,-0.0339125849573554,
0.0685393982217713));
#97514=CARTESIAN_POINT('Ctrl Pts',(0.0100777862615531,-0.0338030433565221,
0.0685658040860737));
#97515=CARTESIAN_POINT('Ctrl Pts',(0.0101542812283887,-0.0336938721132327,
0.0685937587680031));
#97516=CARTESIAN_POINT('Ctrl Pts',(0.00987582818736198,-0.0340223579322365,
0.0684115041313906));
#97517=CARTESIAN_POINT('Ctrl Pts',(0.00995497701201486,-0.0339125849573554,
0.0684356694151789));
#97518=CARTESIAN_POINT('Ctrl Pts',(0.010033570054483,-0.0338030433565221,
0.0684614559150559));
#97519=CARTESIAN_POINT('Ctrl Pts',(0.0101115097307485,-0.0336938721132327,
0.0684888217448896));
#97520=CARTESIAN_POINT('Origin',(0.0052369213529601,-0.0345589643414132,
0.0846932062174358));
#97521=CARTESIAN_POINT('Ctrl Pts',(0.0104394305973868,-0.034193496108874,
0.0686148602124408));
#97522=CARTESIAN_POINT('Ctrl Pts',(0.0105157568963052,-0.0340836138595105,
0.0686467916322565));
#97523=CARTESIAN_POINT('Ctrl Pts',(0.0105913858187076,-0.0339738896671456,
0.0686802871433586));
#97524=CARTESIAN_POINT('Ctrl Pts',(0.0106662234427092,-0.0338644633335883,
0.0687152973869414));
#97525=CARTESIAN_POINT('Ctrl Pts',(0.0103373863698591,-0.034193496108874,
0.0686641363210075));
#97526=CARTESIAN_POINT('Ctrl Pts',(0.0104130331804292,-0.0340836138595105,
0.0686946606113717));
#97527=CARTESIAN_POINT('Ctrl Pts',(0.0104880120581056,-0.0339738896671456,
0.068726735607604));
#97528=CARTESIAN_POINT('Ctrl Pts',(0.0105622297911055,-0.0338644633335883,
0.0687603138247538));
#97529=CARTESIAN_POINT('Ctrl Pts',(0.0102353421423314,-0.034193496108874,
0.0687134124295741));
#97530=CARTESIAN_POINT('Ctrl Pts',(0.0103103094645532,-0.0340836138595105,
0.0687425295904869));
#97531=CARTESIAN_POINT('Ctrl Pts',(0.0103846382975036,-0.0339738896671456,
0.0687731840718493));
#97532=CARTESIAN_POINT('Ctrl Pts',(0.0104582361395018,-0.0338644633335883,
0.0688053302625662));
#97533=CARTESIAN_POINT('Ctrl Pts',(0.0101332979148037,-0.034193496108874,
0.0687626885381408));
#97534=CARTESIAN_POINT('Ctrl Pts',(0.0102075857486772,-0.0340836138595105,
0.068790398569602));
#97535=CARTESIAN_POINT('Ctrl Pts',(0.0102812645369016,-0.0339738896671456,
0.0688196325360947));
#97536=CARTESIAN_POINT('Ctrl Pts',(0.010354242487898,-0.0338644633335883,
0.0688503467003786));
#97537=CARTESIAN_POINT('Origin',(0.00476282790100567,-0.0345610621862272,
0.0846108326147277));
#97538=CARTESIAN_POINT('Ctrl Pts',(0.0101011915342575,-0.03424362768739,
0.0687492614118496));
#97539=CARTESIAN_POINT('Ctrl Pts',(0.0103048837480143,-0.033943005420186,
0.0688238406346036));
#97540=CARTESIAN_POINT('Ctrl Pts',(0.0105023796809093,-0.0336441434784162,
0.068913550917747));
#97541=CARTESIAN_POINT('Ctrl Pts',(0.00986461960757254,-0.03424362768739,
0.0686684299606406));
#97542=CARTESIAN_POINT('Ctrl Pts',(0.0100713604297685,-0.033943005420186,
0.0687340867260913));
#97543=CARTESIAN_POINT('Ctrl Pts',(0.0102725683863685,-0.0336441434784162,
0.0688151295333762));
#97544=CARTESIAN_POINT('Ctrl Pts',(0.010354216881966,-0.0335235895815127,
0.0688503360610121));
#97545=CARTESIAN_POINT('Ctrl Pts',(0.0104271771901633,-0.0334144449262719,
0.0688810423858256));
#97546=CARTESIAN_POINT('Ctrl Pts',(0.0104995869513537,-0.0333049234473133,
0.0689132912935447));
#97547=CARTESIAN_POINT('Ctrl Pts',(0.0105713498403076,-0.0331951640388588,
0.068947049934907));
#97548=CARTESIAN_POINT('Ctrl Pts',(0.0103137101290925,-0.0335235895815127,
0.0687445042347124));
#97549=CARTESIAN_POINT('Ctrl Pts',(0.0103881274207425,-0.0334144449262719,
0.0687746529043221));
#97550=CARTESIAN_POINT('Ctrl Pts',(0.01046200736002,-0.0333049234473133,
0.0688063736163409));
#97551=CARTESIAN_POINT('Ctrl Pts',(0.0105352518029693,-0.0331951640388588,
0.0688396343671963));
#97552=CARTESIAN_POINT('Ctrl Pts',(0.0102732033762191,-0.0335235895815127,
0.0686386724084127));
#97553=CARTESIAN_POINT('Ctrl Pts',(0.0103490776513218,-0.0334144449262719,
0.0686682634228187));
#97554=CARTESIAN_POINT('Ctrl Pts',(0.0104244277686862,-0.0333049234473133,
0.0686994559391371));
#97555=CARTESIAN_POINT('Ctrl Pts',(0.0104991537656311,-0.0331951640388588,
0.0687322187994857));
#97556=CARTESIAN_POINT('Ctrl Pts',(0.0102326966233457,-0.0335235895815127,
0.068532840582113));
#97557=CARTESIAN_POINT('Ctrl Pts',(0.010310027881901,-0.0334144449262719,
0.0685618739413153));
#97558=CARTESIAN_POINT('Ctrl Pts',(0.0103868481773524,-0.0333049234473133,
0.0685925382619333));
#97559=CARTESIAN_POINT('Ctrl Pts',(0.0104630557282929,-0.0331951640388588,
0.068624803231775));
#97560=CARTESIAN_POINT('Origin',(0.00279531278370614,-0.0326434571769497,
0.0836889659829717));
#97561=CARTESIAN_POINT('Ctrl Pts',(0.010784293093255,-0.0336938721132351,
0.0687704180195108));
#97562=CARTESIAN_POINT('Ctrl Pts',(0.01081578157172,-0.0336474569764939,
0.0687859908726599));
#97563=CARTESIAN_POINT('Ctrl Pts',(0.0108470855926661,-0.033601104548885,
0.0688019312711447));
#97564=CARTESIAN_POINT('Ctrl Pts',(0.0109263401730489,-0.0334837508643151,
0.068842288693446));
#97565=CARTESIAN_POINT('Ctrl Pts',(0.0110043640766178,-0.0333660264760385,
0.068884976871181));
#97566=CARTESIAN_POINT('Ctrl Pts',(0.0104694828127738,-0.0336938721132351,
0.0688987321908988));
#97567=CARTESIAN_POINT('Ctrl Pts',(0.0105002202258146,-0.0336474569764939,
0.0689124623550111));
#97568=CARTESIAN_POINT('Ctrl Pts',(0.0105307948038016,-0.033601104548885,
0.0689265513985524));
#97569=CARTESIAN_POINT('Ctrl Pts',(0.010608202602401,-0.0334837508643151,
0.0689622216159913));
#97570=CARTESIAN_POINT('Ctrl Pts',(0.0106845194267492,-0.0333660264760385,
0.0690001699231677));
#97571=CARTESIAN_POINT('Ctrl Pts',(0.0104694828127854,-0.0336938721132426,
0.0688987321909096));
#97572=CARTESIAN_POINT('Ctrl Pts',(0.0105002202258254,-0.0336474569765026,
0.0689124623550215));
#97573=CARTESIAN_POINT('Ctrl Pts',(0.0105307948038116,-0.0336011045488949,
0.0689265513985624));
#97574=CARTESIAN_POINT('Ctrl Pts',(0.0106075579008808,-0.0334847282606778,
0.0689619245316742));
#97575=CARTESIAN_POINT('Ctrl Pts',(0.0106832483951838,-0.0333679869945434,
0.0689995381022298));
#97576=CARTESIAN_POINT('Ctrl Pts',(0.0104694828127689,-0.0336938721132426,
0.0688987321908966));
#97577=CARTESIAN_POINT('Ctrl Pts',(0.0105794134044654,-0.0335278710435082,
0.0689478373339662));
#97578=CARTESIAN_POINT('Ctrl Pts',(0.0106877653983156,-0.033362046922432,
0.0690003725967344));
#97579=CARTESIAN_POINT('Ctrl Pts',(0.0107945839423469,-0.0331951640388602,
0.0690563821289514));
#97580=CARTESIAN_POINT('Ctrl Pts',(0.0103922138851466,-0.0336938721132426,
0.0688662123100945));
#97581=CARTESIAN_POINT('Ctrl Pts',(0.0105028252514424,-0.0335278710435082,
0.0689136998973199));
#97582=CARTESIAN_POINT('Ctrl Pts',(0.0106119085065277,-0.033362046922432,
0.0689646395222109));
#97583=CARTESIAN_POINT('Ctrl Pts',(0.0107195094275136,-0.0331951640388602,
0.0690190746625966));
#97584=CARTESIAN_POINT('Ctrl Pts',(0.0103149449575244,-0.0336938721132426,
0.0688336924292923));
#97585=CARTESIAN_POINT('Ctrl Pts',(0.0104262370984195,-0.0335278710435082,
0.0688795624606737));
#97586=CARTESIAN_POINT('Ctrl Pts',(0.0105360516147399,-0.033362046922432,
0.0689289064476875));
#97587=CARTESIAN_POINT('Ctrl Pts',(0.0106444349126802,-0.0331951640388602,
0.0689817671962418));
#97588=CARTESIAN_POINT('Ctrl Pts',(0.0102376760299022,-0.0336938721132426,
0.0688011725484902));
#97589=CARTESIAN_POINT('Ctrl Pts',(0.0103496489453966,-0.0335278710435082,
0.0688454250240274));
#97590=CARTESIAN_POINT('Ctrl Pts',(0.010460194722952,-0.033362046922432,
0.0688931733731641));
#97591=CARTESIAN_POINT('Ctrl Pts',(0.0105693603978469,-0.0331951640388602,
0.068944459729887));
#97592=CARTESIAN_POINT('Ctrl Pts',(0.0106825833118407,-0.0330240426238155,
0.0690008430190253));
#97593=CARTESIAN_POINT('Ctrl Pts',(0.0107535179658339,-0.0329142774063509,
0.0690360929973547));
#97594=CARTESIAN_POINT('Ctrl Pts',(0.010823759267821,-0.0328043479726686,
0.0690728269665282));
#97595=CARTESIAN_POINT('Ctrl Pts',(0.0108932159374678,-0.0326943950436594,
0.069111000345748));
#97596=CARTESIAN_POINT('Ctrl Pts',(0.0106488017558345,-0.0330240426238155,
0.068892676746748));
#97597=CARTESIAN_POINT('Ctrl Pts',(0.0107212265056095,-0.0329142774063509,
0.0689274613512317));
#97598=CARTESIAN_POINT('Ctrl Pts',(0.0107929682668229,-0.0328043479726686,
0.0689637605189958));
#97599=CARTESIAN_POINT('Ctrl Pts',(0.0108639338522805,-0.0326943950436594,
0.0690015302791926));
#97600=CARTESIAN_POINT('Ctrl Pts',(0.0106150201998282,-0.0330240426238155,
0.0687845104744708));
#97601=CARTESIAN_POINT('Ctrl Pts',(0.0106889350453851,-0.0329142774063509,
0.0688188297051087));
#97602=CARTESIAN_POINT('Ctrl Pts',(0.0107621772658249,-0.0328043479726686,
0.0688546940714634));
#97603=CARTESIAN_POINT('Ctrl Pts',(0.0108346517670933,-0.0326943950436594,
0.0688920602126372));
#97604=CARTESIAN_POINT('Ctrl Pts',(0.0105812386438219,-0.0330240426238155,
0.0686763442021935));
#97605=CARTESIAN_POINT('Ctrl Pts',(0.0106566435851607,-0.0329142774063509,
0.0687101980589857));
#97606=CARTESIAN_POINT('Ctrl Pts',(0.0107313862648268,-0.0328043479726686,
0.068745627623931));
#97607=CARTESIAN_POINT('Ctrl Pts',(0.010805369681906,-0.0326943950436594,
0.0687825901460818));
#97608=CARTESIAN_POINT('Origin',(0.00273742768633797,-0.0326396682856775,
0.0837982578597));
#97609=CARTESIAN_POINT('Ctrl Pts',(0.0111149079858753,-0.0331951640388587,
0.0689487341452376));
#97610=CARTESIAN_POINT('Ctrl Pts',(0.0111865449009495,-0.0330855618255041,
0.0689899308520347));
#97611=CARTESIAN_POINT('Ctrl Pts',(0.0112573819925646,-0.0329757224427708,
0.0690326378695436));
#97612=CARTESIAN_POINT('Ctrl Pts',(0.0113273258669672,-0.0328657862078596,
0.0690768049584357));
#97613=CARTESIAN_POINT('Ctrl Pts',(0.0110074925036805,-0.0331951640388587,
0.0689848321538374));
#97614=CARTESIAN_POINT('Ctrl Pts',(0.0110786322417119,-0.0330855618255041,
0.069024549429667));
#97615=CARTESIAN_POINT('Ctrl Pts',(0.0111490023751854,-0.0329757224427708,
0.0690657656739077));
#97616=CARTESIAN_POINT('Ctrl Pts',(0.0112185102019574,-0.0328657862078596,
0.069108432526924));
#97617=CARTESIAN_POINT('Ctrl Pts',(0.0109000770214857,-0.0331951640388587,
0.0690209301624372));
#97618=CARTESIAN_POINT('Ctrl Pts',(0.0109707195824743,-0.0330855618255041,
0.0690591680072993));
#97619=CARTESIAN_POINT('Ctrl Pts',(0.0110406227578063,-0.0329757224427708,
0.0690988934782718));
#97620=CARTESIAN_POINT('Ctrl Pts',(0.0111096945369476,-0.0328657862078596,
0.0691400600954123));
#97621=CARTESIAN_POINT('Ctrl Pts',(0.0107926615392909,-0.0331951640388587,
0.069057028171037));
#97622=CARTESIAN_POINT('Ctrl Pts',(0.0108628069232368,-0.0330855618255041,
0.0690937865849316));
#97623=CARTESIAN_POINT('Ctrl Pts',(0.0109322431404272,-0.0329757224427708,
0.069132021282636));
#97624=CARTESIAN_POINT('Ctrl Pts',(0.0110008788719377,-0.0328657862078596,
0.0691716876639005));
#97625=CARTESIAN_POINT('Origin',(0.00233766583397968,-0.0326401908830995,
0.0835309315920745));
#97626=CARTESIAN_POINT('Ctrl Pts',(0.0107625554934886,-0.0332451089994432,
0.069039716204632));
#97627=CARTESIAN_POINT('Ctrl Pts',(0.0109552930001814,-0.0329451141710258,
0.0691392391679365));
#97628=CARTESIAN_POINT('Ctrl Pts',(0.0111399864835101,-0.0326442513127503,
0.0692529971739274));
#97629=CARTESIAN_POINT('Ctrl Pts',(0.0105379812583565,-0.0332451089994432,
0.0689298689792922));
#97630=CARTESIAN_POINT('Ctrl Pts',(0.0107348617209353,-0.0329451141710258,
0.0690209219867431));
#97631=CARTESIAN_POINT('Ctrl Pts',(0.0109243243821499,-0.0326442513127503,
0.0691265461635047));
#97632=CARTESIAN_POINT('Ctrl Pts',(0.0110008515680218,-0.0325229783203385,
0.0691716717806828));
#97633=CARTESIAN_POINT('Ctrl Pts',(0.011069477712407,-0.0324130253112079,
0.0692113321183767));
#97634=CARTESIAN_POINT('Ctrl Pts',(0.0111372730232755,-0.0323031222247694,
0.0692524060607307));
#97635=CARTESIAN_POINT('Ctrl Pts',(0.0112041525161893,-0.0321934096636184,
0.0692948379306147));
#97636=CARTESIAN_POINT('Ctrl Pts',(0.010973928464017,-0.0325229783203385,
0.0690615977641299));
#97637=CARTESIAN_POINT('Ctrl Pts',(0.0110440719762857,-0.0324130253112079,
0.0691008869674306));
#97638=CARTESIAN_POINT('Ctrl Pts',(0.0111133921022906,-0.0323031222247694,
0.0691416212203845));
#97639=CARTESIAN_POINT('Ctrl Pts',(0.0111818018890601,-0.0321934096636184,
0.0691837452120583));
#97640=CARTESIAN_POINT('Ctrl Pts',(0.0109470053600122,-0.0325229783203385,
0.068951523747577));
#97641=CARTESIAN_POINT('Ctrl Pts',(0.0110186662401643,-0.0324130253112079,
0.0689904418164846));
#97642=CARTESIAN_POINT('Ctrl Pts',(0.0110895111813056,-0.0323031222247694,
0.0690308363800384));
#97643=CARTESIAN_POINT('Ctrl Pts',(0.0111594512619309,-0.0321934096636184,
0.0690726524935018));
#97644=CARTESIAN_POINT('Ctrl Pts',(0.0109200822560075,-0.0325229783203385,
0.0688414497310241));
#97645=CARTESIAN_POINT('Ctrl Pts',(0.010993260504043,-0.0324130253112079,
0.0688799966655385));
#97646=CARTESIAN_POINT('Ctrl Pts',(0.0110656302603206,-0.0323031222247694,
0.0689200515396923));
#97647=CARTESIAN_POINT('Ctrl Pts',(0.0111371006348016,-0.0321934096636184,
0.0689615597749454));
#97648=CARTESIAN_POINT('Origin',(0.00274179022720111,-0.0326393375178865,
0.0837909326111887));
#97649=CARTESIAN_POINT('Ctrl Pts',(0.0114355958676124,-0.0326943950436593,
0.0691468119977909));
#97650=CARTESIAN_POINT('Ctrl Pts',(0.0115045491752563,-0.0325844576448126,
0.0691924549972257));
#97651=CARTESIAN_POINT('Ctrl Pts',(0.0115725633907719,-0.0324744968375318,
0.0692395272943391));
#97652=CARTESIAN_POINT('Ctrl Pts',(0.0116395522022605,-0.0323646534831894,
0.0692879673753842));
#97653=CARTESIAN_POINT('Ctrl Pts',(0.0113261258368723,-0.0326943950436593,
0.0691760940733979));
#97654=CARTESIAN_POINT('Ctrl Pts',(0.0113946755826339,-0.0325844576448126,
0.0692202283706404));
#97655=CARTESIAN_POINT('Ctrl Pts',(0.0114623174101414,-0.0324744968375318,
0.069265783512467));
#97656=CARTESIAN_POINT('Ctrl Pts',(0.0115289654578094,-0.0323646534831894,
0.0693126999355795));
#97657=CARTESIAN_POINT('Ctrl Pts',(0.0112166558061322,-0.0326943950436593,
0.0692053761490049));
#97658=CARTESIAN_POINT('Ctrl Pts',(0.0112848019900115,-0.0325844576448126,
0.0692480017440551));
#97659=CARTESIAN_POINT('Ctrl Pts',(0.0113520714295108,-0.0324744968375318,
0.0692920397305948));
#97660=CARTESIAN_POINT('Ctrl Pts',(0.0114183787133584,-0.0323646534831894,
0.0693374324957747));
#97661=CARTESIAN_POINT('Ctrl Pts',(0.0111071857753921,-0.0326943950436593,
0.0692346582246119));
#97662=CARTESIAN_POINT('Ctrl Pts',(0.0111749283973891,-0.0325844576448126,
0.0692757751174699));
#97663=CARTESIAN_POINT('Ctrl Pts',(0.0112418254488803,-0.0324744968375318,
0.0693182959487227));
#97664=CARTESIAN_POINT('Ctrl Pts',(0.0113077919689073,-0.0323646534831894,
0.0693621650559699));
#97665=CARTESIAN_POINT('Origin',(0.00231819156432896,-0.0326395579069474,
0.0835633771557399));
#97666=CARTESIAN_POINT('Ctrl Pts',(0.0110781921989789,-0.0327445246961876,
0.0692154699801082));
#97667=CARTESIAN_POINT('Ctrl Pts',(0.0112643010392078,-0.0324436878365474,
0.0693268973739101));
#97668=CARTESIAN_POINT('Ctrl Pts',(0.0114414879972651,-0.0321434074463186,
0.0694520266925976));
#97669=CARTESIAN_POINT('Ctrl Pts',(0.0108609576303243,-0.0327445246961876,
0.0690917398617802));
#97670=CARTESIAN_POINT('Ctrl Pts',(0.0110517330282052,-0.0324436878365474,
0.069194974119971));
#97671=CARTESIAN_POINT('Ctrl Pts',(0.011234190427171,-0.0321434074463186,
0.0693122850830711));
#97672=CARTESIAN_POINT('Ctrl Pts',(0.0113868112395716,-0.0322357242816072,
0.069413886990164));
#97673=CARTESIAN_POINT('Ctrl Pts',(0.0115376502964213,-0.0319819883628705,
0.0695178102333001));
#97674=CARTESIAN_POINT('Ctrl Pts',(0.0116815707259465,-0.0317295851069886,
0.0696311211837884));
#97675=CARTESIAN_POINT('Ctrl Pts',(0.0111779078597899,-0.0322357242816072,
0.0692765575398782));
#97676=CARTESIAN_POINT('Ctrl Pts',(0.0113331206815214,-0.0319819883628705,
0.0693738274813061));
#97677=CARTESIAN_POINT('Ctrl Pts',(0.0114818293805723,-0.0317295851069886,
0.0694807769289991));
#97678=CARTESIAN_POINT('Origin',(0.00236966104337161,-0.0326371942646938,
0.0834831693243248));
#97679=CARTESIAN_POINT('Origin',(0.00280414287347799,-0.0326352985528283,
0.083685216243867));
#97680=CARTESIAN_POINT('Ctrl Pts',(0.0117432135338001,-0.0321934096636183,
0.0693646351476498));
#97681=CARTESIAN_POINT('Ctrl Pts',(0.0118092074446005,-0.0320835708272304,
0.0694145499266512));
#97682=CARTESIAN_POINT('Ctrl Pts',(0.0118741300924936,-0.0319739230346346,
0.0694658014936061));
#97683=CARTESIAN_POINT('Ctrl Pts',(0.0119379034459866,-0.0318646057455575,
0.0695183179007587));
#97684=CARTESIAN_POINT('Ctrl Pts',(0.0116321207195778,-0.0321934096636183,
0.069386985794026));
#97685=CARTESIAN_POINT('Ctrl Pts',(0.0116978063975456,-0.0320835708272304,
0.0694353685165387));
#97686=CARTESIAN_POINT('Ctrl Pts',(0.0117624526972231,-0.0319739230346346,
0.0694850825367976));
#97687=CARTESIAN_POINT('Ctrl Pts',(0.01182598178971,-0.0318646057455575,
0.0695360579013665));
#97688=CARTESIAN_POINT('Ctrl Pts',(0.0115210279053554,-0.0321934096636183,
0.0694093364404021));
#97689=CARTESIAN_POINT('Ctrl Pts',(0.0115864053504907,-0.0320835708272304,
0.0694561871064263));
#97690=CARTESIAN_POINT('Ctrl Pts',(0.0116507753019525,-0.0319739230346346,
0.0695043635799891));
#97691=CARTESIAN_POINT('Ctrl Pts',(0.0117140601334333,-0.0318646057455575,
0.0695537979019742));
#97692=CARTESIAN_POINT('Ctrl Pts',(0.011409935091133,-0.0321934096636183,
0.0694316870867783));
#97693=CARTESIAN_POINT('Ctrl Pts',(0.0114750043034357,-0.0320835708272304,
0.0694770056963138));
#97694=CARTESIAN_POINT('Ctrl Pts',(0.011539097906682,-0.0319739230346346,
0.0695236446231807));
#97695=CARTESIAN_POINT('Ctrl Pts',(0.0116021384771566,-0.0318646057455575,
0.069571537902582));
#97696=CARTESIAN_POINT('Ctrl Pts',(0.0113078589975475,-0.0320218834582309,
0.0693612159472554));
#97697=CARTESIAN_POINT('Ctrl Pts',(0.0113576986627241,-0.0319391099350625,
0.0693943544893326));
#97698=CARTESIAN_POINT('Ctrl Pts',(0.0114069906683328,-0.0318564869454927,
0.069428251206969));
#97699=CARTESIAN_POINT('Ctrl Pts',(0.0114557014165997,-0.031774074144654,
0.0694628780591373));
#97700=CARTESIAN_POINT('Ctrl Pts',(0.0112991320717052,-0.0320218834582309,
0.0693124238494042));
#97701=CARTESIAN_POINT('Ctrl Pts',(0.0113494795446663,-0.0319391099350625,
0.0693454715652805));
#97702=CARTESIAN_POINT('Ctrl Pts',(0.0113992804686555,-0.0318564869454927,
0.0693792854412352));
#97703=CARTESIAN_POINT('Ctrl Pts',(0.0114485008695863,-0.031774074144654,
0.0694138374619745));
#97704=CARTESIAN_POINT('Ctrl Pts',(0.0112904051458629,-0.0320218834582309,
0.069263631751553));
#97705=CARTESIAN_POINT('Ctrl Pts',(0.0113412604266085,-0.0319391099350625,
0.0692965886412284));
#97706=CARTESIAN_POINT('Ctrl Pts',(0.0113915702689782,-0.0318564869454927,
0.0693303196755014));
#97707=CARTESIAN_POINT('Ctrl Pts',(0.0114413003225729,-0.031774074144654,
0.0693647968648116));
#97708=CARTESIAN_POINT('Ctrl Pts',(0.0112816782200206,-0.0320218834582309,
0.0692148396537017));
#97709=CARTESIAN_POINT('Ctrl Pts',(0.0113330413085507,-0.0319391099350625,
0.0692477057171764));
#97710=CARTESIAN_POINT('Ctrl Pts',(0.0113838600693009,-0.0318564869454927,
0.0692813539097676));
#97711=CARTESIAN_POINT('Ctrl Pts',(0.0114340997755596,-0.031774074144654,
0.0693157562676487));
#97712=CARTESIAN_POINT('Origin',(0.0140065478483093,-0.0391228853390673,
0.0636013656535299));
#97713=CARTESIAN_POINT('Ctrl Pts',(0.00842661988560802,-0.0352722978779546,
0.0684060941969251));
#97714=CARTESIAN_POINT('Ctrl Pts',(0.00844546889791518,-0.0352466642097184,
0.0684074385975486));
#97715=CARTESIAN_POINT('Ctrl Pts',(0.00846430669568076,-0.0352210183808285,
0.0684087035981362));
#97716=CARTESIAN_POINT('Ctrl Pts',(0.00848313397934979,-0.0351953608940152,
0.0684098887120041));
#97717=CARTESIAN_POINT('Origin',(0.00895567874103067,-0.0352456003065015,
0.0635347658441051));
#97718=CARTESIAN_POINT('Ctrl Pts',(0.00860736438460647,-0.035024121149334,
0.0684204774715147));
#97719=CARTESIAN_POINT('Ctrl Pts',(0.00868628620468203,-0.0349144232867422,
0.0684271386176258));
#97720=CARTESIAN_POINT('Ctrl Pts',(0.00876511757262519,-0.0348045283677512,
0.0684354351210956));
#97721=CARTESIAN_POINT('Ctrl Pts',(0.008843757120033,-0.0346945769586886,
0.0684453601125965));
#97722=CARTESIAN_POINT('Ctrl Pts',(0.00853613641361172,-0.035024121149334,
0.0683323428134569));
#97723=CARTESIAN_POINT('Ctrl Pts',(0.00861627225241067,-0.0349144232867422,
0.0683380228235164));
#97724=CARTESIAN_POINT('Ctrl Pts',(0.00869633864650826,-0.0348045283677512,
0.0683453626983107));
#97725=CARTESIAN_POINT('Ctrl Pts',(0.00877623269118711,-0.0346945769586886,
0.0683543568526987));
#97726=CARTESIAN_POINT('Ctrl Pts',(0.00846490844261696,-0.035024121149334,
0.0682442081553991));
#97727=CARTESIAN_POINT('Ctrl Pts',(0.0085462583001393,-0.0349144232867422,
0.068248907029407));
#97728=CARTESIAN_POINT('Ctrl Pts',(0.00862755972039133,-0.0348045283677512,
0.0682552902755259));
#97729=CARTESIAN_POINT('Ctrl Pts',(0.00870870826234121,-0.0346945769586886,
0.0682633535928009));
#97730=CARTESIAN_POINT('Ctrl Pts',(0.00839368047162221,-0.035024121149334,
0.0681560734973413));
#97731=CARTESIAN_POINT('Ctrl Pts',(0.00847624434786794,-0.0349144232867422,
0.0681597912352976));
#97732=CARTESIAN_POINT('Ctrl Pts',(0.0085587807942744,-0.0348045283677512,
0.0681652178527411));
#97733=CARTESIAN_POINT('Ctrl Pts',(0.00864118383349532,-0.0346945769586886,
0.0681723503329031));
#97734=CARTESIAN_POINT('Origin',(0.0065630049941059,-0.034562906794416,
0.0850784932751654));
#97735=CARTESIAN_POINT('Ctrl Pts',(0.00891784935021737,-0.0351970973651661,
0.0682725023073406));
#97736=CARTESIAN_POINT('Ctrl Pts',(0.00899927411533065,-0.0350869349321806,
0.068283503031651));
#97737=CARTESIAN_POINT('Ctrl Pts',(0.00908053763280962,-0.0349764985129744,
0.068296205644577));
#97738=CARTESIAN_POINT('Ctrl Pts',(0.00916153365464846,-0.0348659306849652,
0.0683105998868645));
#97739=CARTESIAN_POINT('Ctrl Pts',(0.00885503876628931,-0.0351970973651661,
0.0683255617192924));
#97740=CARTESIAN_POINT('Ctrl Pts',(0.00893572846515821,-0.0350869349321806,
0.0683356922880859));
#97741=CARTESIAN_POINT('Ctrl Pts',(0.00901627439752347,-0.0349764985129744,
0.0683475087430483));
#97742=CARTESIAN_POINT('Ctrl Pts',(0.00909657131261243,-0.0348659306849652,
0.0683610019182447));
#97743=CARTESIAN_POINT('Ctrl Pts',(0.00879222818236124,-0.0351970973651661,
0.0683786211312442));
#97744=CARTESIAN_POINT('Ctrl Pts',(0.00887218281498578,-0.0350869349321806,
0.0683878815445207));
#97745=CARTESIAN_POINT('Ctrl Pts',(0.00895201116223733,-0.0349764985129744,
0.0683988118415197));
#97746=CARTESIAN_POINT('Ctrl Pts',(0.0090316089705764,-0.0348659306849652,
0.0684114039496248));
#97747=CARTESIAN_POINT('Ctrl Pts',(0.00872941759843317,-0.0351970973651661,
0.0684316805431959));
#97748=CARTESIAN_POINT('Ctrl Pts',(0.00880863716481334,-0.0350869349321806,
0.0684400708009555));
#97749=CARTESIAN_POINT('Ctrl Pts',(0.00888774792695119,-0.0349764985129744,
0.068450114939991));
#97750=CARTESIAN_POINT('Ctrl Pts',(0.00896664662854037,-0.0348659306849652,
0.068461805981005));
#97751=CARTESIAN_POINT('Origin',(0.00609543417322961,-0.034563718796662,
0.084965786203636));
#97752=CARTESIAN_POINT('Ctrl Pts',(0.00869603662568097,-0.0352450361861253,
0.0684271816502354));
#97753=CARTESIAN_POINT('Ctrl Pts',(0.00891187625595256,-0.0349452761023765,
0.0684487645797641));
#97754=CARTESIAN_POINT('Ctrl Pts',(0.0091254769940661,-0.0346444289983475,
0.0684865441181435));
#97755=CARTESIAN_POINT('Ctrl Pts',(0.00844679534224049,-0.0352450361861253,
0.0684077193115027));
#97756=CARTESIAN_POINT('Ctrl Pts',(0.00866336900664345,-0.0349452761023765,
0.0684199019520167));
#97757=CARTESIAN_POINT('Ctrl Pts',(0.00887840976178802,-0.0346444289983475,
0.0684483631970645));
#97758=CARTESIAN_POINT('Ctrl Pts',(0.00896616888765449,-0.0345231616327822,
0.0684621475564246));
#97759=CARTESIAN_POINT('Ctrl Pts',(0.00904456792573297,-0.0344132092796975,
0.0684737586710232));
#97760=CARTESIAN_POINT('Ctrl Pts',(0.00912272275203471,-0.0343032738558974,
0.068486990808804));
#97761=CARTESIAN_POINT('Ctrl Pts',(0.00920053367542413,-0.0341934961088741,
0.0685018244531206));
#97762=CARTESIAN_POINT('Ctrl Pts',(0.0089006154894152,-0.0345231616327822,
0.0683697144015627));
#97763=CARTESIAN_POINT('Ctrl Pts',(0.00898028858839797,-0.0344132092796975,
0.0683804219548584));
#97764=CARTESIAN_POINT('Ctrl Pts',(0.00905973609932115,-0.0343032738558974,
0.0683927769309008));
#97765=CARTESIAN_POINT('Ctrl Pts',(0.00913885664618559,-0.0341934961088741,
0.0684067608943678));
#97766=CARTESIAN_POINT('Ctrl Pts',(0.00883506209117591,-0.0345231616327822,
0.0682772812467008));
#97767=CARTESIAN_POINT('Ctrl Pts',(0.00891600925106296,-0.0344132092796975,
0.0682870852386936));
#97768=CARTESIAN_POINT('Ctrl Pts',(0.00899674944660758,-0.0343032738558974,
0.0682985630529975));
#97769=CARTESIAN_POINT('Ctrl Pts',(0.00907717961694704,-0.0341934961088741,
0.068311697335615));
#97770=CARTESIAN_POINT('Ctrl Pts',(0.00876950869293662,-0.0345231616327822,
0.0681848480918389));
#97771=CARTESIAN_POINT('Ctrl Pts',(0.00885172991372796,-0.0344132092796975,
0.0681937485225288));
#97772=CARTESIAN_POINT('Ctrl Pts',(0.00893376279389401,-0.0343032738558974,
0.0682043491750943));
#97773=CARTESIAN_POINT('Ctrl Pts',(0.0090155025877085,-0.0341934961088741,
0.0682166337768622));
#97774=CARTESIAN_POINT('Origin',(0.00656154210998243,-0.0345625596230191,
0.0850905081937899));
#97775=CARTESIAN_POINT('Ctrl Pts',(0.00936123232799057,-0.0346945769586885,
0.0682789935135691));
#97776=CARTESIAN_POINT('Ctrl Pts',(0.0094421377648623,-0.0345846629176052,
0.0682960462018945));
#97777=CARTESIAN_POINT('Ctrl Pts',(0.0095227043779901,-0.0344746925050311,
0.0683147748940696));
#97778=CARTESIAN_POINT('Ctrl Pts',(0.00960282903525073,-0.034364806625326,
0.0683351551664054));
#97779=CARTESIAN_POINT('Ctrl Pts',(0.00927022913974539,-0.0346945769586885,
0.0683465178892488));
#97780=CARTESIAN_POINT('Ctrl Pts',(0.00935020405659018,-0.0345846629176052,
0.0683623165076428));
#97781=CARTESIAN_POINT('Ctrl Pts',(0.00942986592440711,-0.0344746925050311,
0.0683797716729162));
#97782=CARTESIAN_POINT('Ctrl Pts',(0.00950911276359782,-0.034364806625326,
0.0683988605979571));
#97783=CARTESIAN_POINT('Ctrl Pts',(0.00917922595150019,-0.0346945769586885,
0.0684140422649284));
#97784=CARTESIAN_POINT('Ctrl Pts',(0.00925827034831806,-0.0345846629176052,
0.068428586813391));
#97785=CARTESIAN_POINT('Ctrl Pts',(0.00933702747082412,-0.0344746925050311,
0.0684447684517628));
#97786=CARTESIAN_POINT('Ctrl Pts',(0.00941539649194491,-0.034364806625326,
0.0684625660295089));
#97787=CARTESIAN_POINT('Ctrl Pts',(0.00908822276325501,-0.0346945769586885,
0.068481566640608));
#97788=CARTESIAN_POINT('Ctrl Pts',(0.00916633664004595,-0.0345846629176052,
0.0684948571191392));
#97789=CARTESIAN_POINT('Ctrl Pts',(0.00924418901724114,-0.0344746925050311,
0.0685097652306094));
#97790=CARTESIAN_POINT('Ctrl Pts',(0.009321680220292,-0.034364806625326,
0.0685262714610606));
#97791=CARTESIAN_POINT('Origin',(0.00608543025515759,-0.0345626446730496,
0.0850233540094552));
#97792=CARTESIAN_POINT('Ctrl Pts',(0.00908985111544923,-0.0346945769586886,
0.068480358403101));
#97793=CARTESIAN_POINT('Ctrl Pts',(0.00920860402869501,-0.0345275153362891,
0.068500593103472));
#97794=CARTESIAN_POINT('Ctrl Pts',(0.00932675129482487,-0.0343603235965159,
0.0685245677073899));
#97795=CARTESIAN_POINT('Ctrl Pts',(0.0094439445405227,-0.034193496108874,
0.0685522061152209));
#97796=CARTESIAN_POINT('Ctrl Pts',(0.00900692237659121,-0.0346945769586886,
0.0684680761963494));
#97797=CARTESIAN_POINT('Ctrl Pts',(0.00912593254557493,-0.0345275153362891,
0.0684865739210822));
#97798=CARTESIAN_POINT('Ctrl Pts',(0.00924439176026727,-0.0343603235965159,
0.0685088191905472));
#97799=CARTESIAN_POINT('Ctrl Pts',(0.00936195064873045,-0.034193496108874,
0.068534741006002));
#97800=CARTESIAN_POINT('Ctrl Pts',(0.00892399363773319,-0.0346945769586886,
0.0684557939895979));
#97801=CARTESIAN_POINT('Ctrl Pts',(0.00904326106245485,-0.0345275153362891,
0.0684725547386924));
#97802=CARTESIAN_POINT('Ctrl Pts',(0.00916203222570968,-0.0343603235965159,
0.0684930706737045));
#97803=CARTESIAN_POINT('Ctrl Pts',(0.0092799567569382,-0.034193496108874,
0.068517275896783));
#97804=CARTESIAN_POINT('Ctrl Pts',(0.00884106489887517,-0.0346945769586886,
0.0684435117828463));
#97805=CARTESIAN_POINT('Ctrl Pts',(0.00896058957933477,-0.0345275153362891,
0.0684585355563027));
#97806=CARTESIAN_POINT('Ctrl Pts',(0.00907967269115209,-0.0343603235965159,
0.0684773221568619));
#97807=CARTESIAN_POINT('Ctrl Pts',(0.00919796286514594,-0.034193496108874,
0.0684998107875641));
#97808=CARTESIAN_POINT('Ctrl Pts',(0.00932164924232423,-0.0340223579322365,
0.0685262654318876));
#97809=CARTESIAN_POINT('Ctrl Pts',(0.00939921520933324,-0.0339125849573555,
0.0685427871426646));
#97810=CARTESIAN_POINT('Ctrl Pts',(0.00947638471061337,-0.0338030433565222,
0.0685609026791053));
#97811=CARTESIAN_POINT('Ctrl Pts',(0.00955306111301236,-0.0336938721132328,
0.068580580126324));
#97812=CARTESIAN_POINT('Ctrl Pts',(0.00926202900767557,-0.0340223579322365,
0.0684298983864274));
#97813=CARTESIAN_POINT('Ctrl Pts',(0.00934092412757726,-0.0339125849573555,
0.0684455977786725));
#97814=CARTESIAN_POINT('Ctrl Pts',(0.00941943886785254,-0.0338030433565222,
0.0684629190847914));
#97815=CARTESIAN_POINT('Ctrl Pts',(0.00949747478497886,-0.0336938721132328,
0.0684818312530846));
#97816=CARTESIAN_POINT('Ctrl Pts',(0.00920240877302691,-0.0340223579322365,
0.0683335313409672));
#97817=CARTESIAN_POINT('Ctrl Pts',(0.00928263304582129,-0.0339125849573555,
0.0683484084146803));
#97818=CARTESIAN_POINT('Ctrl Pts',(0.00936249302509171,-0.0338030433565222,
0.0683649354904774));
#97819=CARTESIAN_POINT('Ctrl Pts',(0.00944188845694536,-0.0336938721132328,
0.0683830823798452));
#97820=CARTESIAN_POINT('Ctrl Pts',(0.00914278853837825,-0.0340223579322365,
0.068237164295507));
#97821=CARTESIAN_POINT('Ctrl Pts',(0.00922434196406532,-0.0339125849573555,
0.0682512190506882));
#97822=CARTESIAN_POINT('Ctrl Pts',(0.00930554718233089,-0.0338030433565222,
0.0682669518961634));
#97823=CARTESIAN_POINT('Ctrl Pts',(0.00938630212891187,-0.0336938721132328,
0.0682843335066058));
#97824=CARTESIAN_POINT('Origin',(0.00658109924038061,-0.0345589643414756,
0.0849718894913104));
#97825=CARTESIAN_POINT('Ctrl Pts',(0.00972743405026164,-0.034193496108874,
0.0683682787406266));
#97826=CARTESIAN_POINT('Ctrl Pts',(0.00980716056262902,-0.0340836138581107,
0.0683903921500919));
#97827=CARTESIAN_POINT('Ctrl Pts',(0.00988639123010831,-0.03397388966435,
0.068414144722012));
#97828=CARTESIAN_POINT('Ctrl Pts',(0.00996502668511442,-0.0338644633294063,
0.0684394992583226));
#97829=CARTESIAN_POINT('Ctrl Pts',(0.00963237040597177,-0.034193496108874,
0.0684299558253615));
#97830=CARTESIAN_POINT('Ctrl Pts',(0.00971124642786439,-0.0340836138581107,
0.0684507583634664));
#97831=CARTESIAN_POINT('Ctrl Pts',(0.00978965413868244,-0.03397388966435,
0.0684731830938911));
#97832=CARTESIAN_POINT('Ctrl Pts',(0.00986749511019974,-0.0338644633294063,
0.0684971945886511));
#97833=CARTESIAN_POINT('Ctrl Pts',(0.00953730676168191,-0.034193496108874,
0.0684916329100963));
#97834=CARTESIAN_POINT('Ctrl Pts',(0.00961533229309976,-0.0340836138581107,
0.0685111245768409));
#97835=CARTESIAN_POINT('Ctrl Pts',(0.00969291704725657,-0.03397388966435,
0.0685322214657703));
#97836=CARTESIAN_POINT('Ctrl Pts',(0.00976996353528506,-0.0338644633294063,
0.0685548899189796));
#97837=CARTESIAN_POINT('Ctrl Pts',(0.00944224311739205,-0.034193496108874,
0.0685533099948311));
#97838=CARTESIAN_POINT('Ctrl Pts',(0.00951941815833512,-0.0340836138581107,
0.0685714907902154));
#97839=CARTESIAN_POINT('Ctrl Pts',(0.0095961799558307,-0.03397388966435,
0.0685912598376494));
#97840=CARTESIAN_POINT('Ctrl Pts',(0.00967243196037038,-0.0338644633294063,
0.0686125852493082));
#97841=CARTESIAN_POINT('Origin',(0.00610042000738715,-0.0345610621863924,
0.0849495850931085));
#97842=CARTESIAN_POINT('Ctrl Pts',(0.00940870704009062,-0.0342436276873901,
0.0685440127419332));
#97843=CARTESIAN_POINT('Ctrl Pts',(0.00962014033504646,-0.0339430054201861,
0.068592474481438));
#97844=CARTESIAN_POINT('Ctrl Pts',(0.0098273226333917,-0.0336441434784162,
0.0686567245683181));
#97845=CARTESIAN_POINT('Ctrl Pts',(0.00916386968655442,-0.0342436276873901,
0.068493468995402));
#97846=CARTESIAN_POINT('Ctrl Pts',(0.00937720927033622,-0.0339430054201861,
0.0685326965418909));
#97847=CARTESIAN_POINT('Ctrl Pts',(0.00958698799919459,-0.0336441434784162,
0.0685878822586144));
#97848=CARTESIAN_POINT('Ctrl Pts',(0.00967240521996829,-0.0335235895815128,
0.0686125779022954));
#97849=CARTESIAN_POINT('Ctrl Pts',(0.00974863873732299,-0.0334144449262719,
0.0686338977472179));
#97850=CARTESIAN_POINT('Ctrl Pts',(0.00982451938580206,-0.0333049234473133,
0.0686568170131558));
#97851=CARTESIAN_POINT('Ctrl Pts',(0.00989994748262462,-0.0331951640388588,
0.0686813151826251));
#97852=CARTESIAN_POINT('Ctrl Pts',(0.00961895362993591,-0.0335235895815128,
0.0685126574338753));
#97853=CARTESIAN_POINT('Ctrl Pts',(0.00969656274926369,-0.0334144449262719,
0.0685332414124246));
#97854=CARTESIAN_POINT('Ctrl Pts',(0.00977383578256132,-0.0333049234473133,
0.0685554523854694));
#97855=CARTESIAN_POINT('Ctrl Pts',(0.00985067134865647,-0.0331951640388588,
0.0685792709024943));
#97856=CARTESIAN_POINT('Ctrl Pts',(0.00956550203990353,-0.0335235895815128,
0.0684127369654553));
#97857=CARTESIAN_POINT('Ctrl Pts',(0.00964448676120439,-0.0334144449262719,
0.0684325850776313));
#97858=CARTESIAN_POINT('Ctrl Pts',(0.00972315217932059,-0.0333049234473133,
0.068454087757783));
#97859=CARTESIAN_POINT('Ctrl Pts',(0.00980139521468832,-0.0331951640388588,
0.0684772266223635));
#97860=CARTESIAN_POINT('Ctrl Pts',(0.00951205044987115,-0.0335235895815128,
0.0683128164970353));
#97861=CARTESIAN_POINT('Ctrl Pts',(0.0095924107731451,-0.0334144449262719,
0.068331928742838));
#97862=CARTESIAN_POINT('Ctrl Pts',(0.00967246857607985,-0.0333049234473133,
0.0683527231300966));
#97863=CARTESIAN_POINT('Ctrl Pts',(0.00975211908072016,-0.0331951640388588,
0.0683751823422326));
#97864=CARTESIAN_POINT('Origin',(0.00403287880815687,-0.0326434571769683,
0.0842815826877775));
#97865=CARTESIAN_POINT('Ctrl Pts',(0.0100890737653109,-0.033693872113235,
0.0684793871961827));
#97866=CARTESIAN_POINT('Ctrl Pts',(0.010122265743759,-0.0336474569764938,
0.0684908906999072));
#97867=CARTESIAN_POINT('Ctrl Pts',(0.0101553207848362,-0.033601104548885,
0.06850278196942));
#97868=CARTESIAN_POINT('Ctrl Pts',(0.010239008545416,-0.033483750864315,
0.0685328879285582));
#97869=CARTESIAN_POINT('Ctrl Pts',(0.0103217674545512,-0.0333660264760382,
0.0685654605091318));
#97870=CARTESIAN_POINT('Ctrl Pts',(0.00979282788793425,-0.033693872113235,
0.0686461457624149));
#97871=CARTESIAN_POINT('Ctrl Pts',(0.00982504377315792,-0.0336474569764938,
0.0686559152407143));
#97872=CARTESIAN_POINT('Ctrl Pts',(0.00985714308685013,-0.033601104548885,
0.0686660611772151));
#97873=CARTESIAN_POINT('Ctrl Pts',(0.00993841116553064,-0.033483750864315,
0.0686917483546339));
#97874=CARTESIAN_POINT('Ctrl Pts',(0.0100188823929709,-0.0333660264760383,
0.0687198323937026));
#97875=CARTESIAN_POINT('Ctrl Pts',(0.00979282788794581,-0.0336938721132427,
0.0686461457624253));
#97876=CARTESIAN_POINT('Ctrl Pts',(0.00982504377316868,-0.0336474569765026,
0.0686559152407246));
#97877=CARTESIAN_POINT('Ctrl Pts',(0.00985714308686013,-0.0336011045488949,
0.0686660611772251));
#97878=CARTESIAN_POINT('Ctrl Pts',(0.00993773431313503,-0.0334847282606778,
0.0686915344154427));
#97879=CARTESIAN_POINT('Ctrl Pts',(0.0100175421957065,-0.0333679869945434,
0.0687193648573588));
#97880=CARTESIAN_POINT('Ctrl Pts',(0.00979282788792897,-0.0336938721132426,
0.0686461457624133));
#97881=CARTESIAN_POINT('Ctrl Pts',(0.00990804615044084,-0.0335278710435082,
0.0686810857402377));
#97882=CARTESIAN_POINT('Ctrl Pts',(0.0100221281708153,-0.033362046922432,
0.0687196266410151));
#97883=CARTESIAN_POINT('Ctrl Pts',(0.0101351242745049,-0.0331951640388601,
0.0687618066078133));
#97884=CARTESIAN_POINT('Ctrl Pts',(0.0097120924270641,-0.0336938721132426,
0.0686235666751374));
#97885=CARTESIAN_POINT('Ctrl Pts',(0.00982778336255979,-0.0335278710435082,
0.0686568165283469));
#97886=CARTESIAN_POINT('Ctrl Pts',(0.00994239089150128,-0.033362046922432,
0.0686936827219932));
#97887=CARTESIAN_POINT('Ctrl Pts',(0.0100559658792504,-0.0331951640388601,
0.0687342026536762));
#97888=CARTESIAN_POINT('Ctrl Pts',(0.00963135696619923,-0.0336938721132426,
0.0686009875878615));
#97889=CARTESIAN_POINT('Ctrl Pts',(0.00974752057467875,-0.0335278710435082,
0.0686325473164561));
#97890=CARTESIAN_POINT('Ctrl Pts',(0.0098626536121873,-0.033362046922432,
0.0686677388029712));
#97891=CARTESIAN_POINT('Ctrl Pts',(0.00997680748399584,-0.0331951640388601,
0.0687065986995392));
#97892=CARTESIAN_POINT('Ctrl Pts',(0.00955062150533435,-0.0336938721132426,
0.0685784085005856));
#97893=CARTESIAN_POINT('Ctrl Pts',(0.00966725778679771,-0.0335278710435082,
0.0686082781045653));
#97894=CARTESIAN_POINT('Ctrl Pts',(0.00978291633287332,-0.033362046922432,
0.0686417948839492));
#97895=CARTESIAN_POINT('Ctrl Pts',(0.00989764908874131,-0.0331951640388601,
0.0686789947454021));
#97896=CARTESIAN_POINT('Ctrl Pts',(0.0100170459061869,-0.0330240426238155,
0.0687207428415402));
#97897=CARTESIAN_POINT('Ctrl Pts',(0.0100918392130133,-0.0329142774063509,
0.0687468243937052));
#97898=CARTESIAN_POINT('Ctrl Pts',(0.0101661306284923,-0.0328043479726686,
0.068774465135052));
#97899=CARTESIAN_POINT('Ctrl Pts',(0.0102398240046069,-0.0326943950436594,
0.0688036322767755));
#97900=CARTESIAN_POINT('Ctrl Pts',(0.00996997389917268,-0.0330240426238155,
0.0686176634442766));
#97901=CARTESIAN_POINT('Ctrl Pts',(0.0100461872251217,-0.0329142774063509,
0.0686430965336849));
#97902=CARTESIAN_POINT('Ctrl Pts',(0.0101219127731913,-0.0328043479726686,
0.0686701178447547));
#97903=CARTESIAN_POINT('Ctrl Pts',(0.0101970525799876,-0.0326943950436594,
0.068698695432814));
#97904=CARTESIAN_POINT('Ctrl Pts',(0.00992290189215845,-0.0330240426238155,
0.068514584047013));
#97905=CARTESIAN_POINT('Ctrl Pts',(0.0100005352372302,-0.0329142774063509,
0.0685393686736647));
#97906=CARTESIAN_POINT('Ctrl Pts',(0.0100776949178904,-0.0328043479726686,
0.0685657705544574));
#97907=CARTESIAN_POINT('Ctrl Pts',(0.0101542811553683,-0.0326943950436594,
0.0685937585888524));
#97908=CARTESIAN_POINT('Ctrl Pts',(0.00987582988514422,-0.0330240426238155,
0.0684115046497494));
#97909=CARTESIAN_POINT('Ctrl Pts',(0.00995488324933863,-0.0329142774063509,
0.0684356408136444));
#97910=CARTESIAN_POINT('Ctrl Pts',(0.0100334770625894,-0.0328043479726686,
0.06846142326416));
#97911=CARTESIAN_POINT('Ctrl Pts',(0.0101115097307491,-0.0326943950436594,
0.0684888217448909));
#97912=CARTESIAN_POINT('Origin',(0.00398914805644169,-0.032639668285777,
0.0843972676920441));
#97913=CARTESIAN_POINT('Ctrl Pts',(0.0104394305973869,-0.0331951640388587,
0.0686148602124409));
#97914=CARTESIAN_POINT('Ctrl Pts',(0.0105156659504639,-0.0330855618255041,
0.0686467535846912));
#97915=CARTESIAN_POINT('Ctrl Pts',(0.0105912970790538,-0.0329757224427708,
0.0686802456028626));
#97916=CARTESIAN_POINT('Ctrl Pts',(0.0106662250291835,-0.0328657862078596,
0.0687152981291199));
#97917=CARTESIAN_POINT('Ctrl Pts',(0.0103373863984962,-0.0331951640388587,
0.068664136307179));
#97918=CARTESIAN_POINT('Ctrl Pts',(0.0104129430730529,-0.0330855618255041,
0.0686946242270234));
#97919=CARTESIAN_POINT('Ctrl Pts',(0.0104879240821715,-0.0329757224427708,
0.0687266957524929));
#97920=CARTESIAN_POINT('Ctrl Pts',(0.0105622313936229,-0.0328657862078596,
0.0687603145239418));
#97921=CARTESIAN_POINT('Ctrl Pts',(0.0102353421996055,-0.0331951640388587,
0.0687134124019171));
#97922=CARTESIAN_POINT('Ctrl Pts',(0.0103102201956419,-0.0330855618255041,
0.0687424948693555));
#97923=CARTESIAN_POINT('Ctrl Pts',(0.0103845510852892,-0.0329757224427708,
0.0687731459021232));
#97924=CARTESIAN_POINT('Ctrl Pts',(0.0104582377580623,-0.0328657862078596,
0.0688053309187638));
#97925=CARTESIAN_POINT('Ctrl Pts',(0.0101332980007148,-0.0331951640388587,
0.0687626884966553));
#97926=CARTESIAN_POINT('Ctrl Pts',(0.010207497318231,-0.0330855618255041,
0.0687903655116877));
#97927=CARTESIAN_POINT('Ctrl Pts',(0.0102811780884069,-0.0329757224427708,
0.0688195960517534));
#97928=CARTESIAN_POINT('Ctrl Pts',(0.0103542441225017,-0.0328657862078596,
0.0688503473135857));
#97929=CARTESIAN_POINT('Origin',(0.00355903358096729,-0.0326401908835644,
0.0841821528168722));
#97930=CARTESIAN_POINT('Ctrl Pts',(0.010101259585347,-0.0332451089994432,
0.0687492863283464));
#97931=CARTESIAN_POINT('Ctrl Pts',(0.0103049508340365,-0.0329451141710258,
0.0688238681084164));
#97932=CARTESIAN_POINT('Ctrl Pts',(0.0105024456128185,-0.0326442513127503,
0.0689135808670683));
#97933=CARTESIAN_POINT('Ctrl Pts',(0.00986468867718615,-0.0332451089994432,
0.0686684518962526));
#97934=CARTESIAN_POINT('Ctrl Pts',(0.0100714286463617,-0.0329451141710258,
0.0687341112585429));
#97935=CARTESIAN_POINT('Ctrl Pts',(0.0102726355575189,-0.0326442513127503,
0.0688151565891526));
#97936=CARTESIAN_POINT('Ctrl Pts',(0.0103542150431901,-0.0325229783203385,
0.0688503349776998));
#97937=CARTESIAN_POINT('Ctrl Pts',(0.0104272708082967,-0.0324130253112079,
0.0688810814452022));
#97938=CARTESIAN_POINT('Ctrl Pts',(0.0104996794629,-0.0323031222247695,
0.0689133345017209));
#97939=CARTESIAN_POINT('Ctrl Pts',(0.010571349714495,-0.0321934096636184,
0.0689470495605312));
#97940=CARTESIAN_POINT('Ctrl Pts',(0.0103137083034759,-0.0325229783203385,
0.0687445032873275));
#97941=CARTESIAN_POINT('Ctrl Pts',(0.0103882229560934,-0.0324130253112079,
0.0687746913703189));
#97942=CARTESIAN_POINT('Ctrl Pts',(0.0104621018278394,-0.0323031222247695,
0.0688064163059783));
#97943=CARTESIAN_POINT('Ctrl Pts',(0.0105352517190943,-0.0321934096636184,
0.0688396341176126));
#97944=CARTESIAN_POINT('Ctrl Pts',(0.0102732015637618,-0.0325229783203385,
0.0686386715969551));
#97945=CARTESIAN_POINT('Ctrl Pts',(0.0103491751038901,-0.0324130253112079,
0.0686683012954356));
#97946=CARTESIAN_POINT('Ctrl Pts',(0.0104245241927788,-0.0323031222247695,
0.0686994981102356));
#97947=CARTESIAN_POINT('Ctrl Pts',(0.0104991537236937,-0.0321934096636184,
0.068732218674694));
#97948=CARTESIAN_POINT('Ctrl Pts',(0.0102326948240477,-0.0325229783203385,
0.0685328399065827));
#97949=CARTESIAN_POINT('Ctrl Pts',(0.0103101272516868,-0.0324130253112079,
0.0685619112205522));
#97950=CARTESIAN_POINT('Ctrl Pts',(0.0103869465577181,-0.0323031222247695,
0.0685925799144929));
#97951=CARTESIAN_POINT('Ctrl Pts',(0.0104630557282931,-0.0321934096636184,
0.0686248032317755));
#97952=CARTESIAN_POINT('Origin',(0.0039925581003947,-0.0326393375180069,
0.0843894534338173));
#97953=CARTESIAN_POINT('Ctrl Pts',(0.0107824154971495,-0.0326943950436593,
0.0687711833127807));
#97954=CARTESIAN_POINT('Ctrl Pts',(0.010856545672076,-0.0325844576448127,
0.0688078242625201));
#97955=CARTESIAN_POINT('Ctrl Pts',(0.0109299232983959,-0.0324744968375319,
0.0688460009389521));
#97956=CARTESIAN_POINT('Ctrl Pts',(0.0110024550350888,-0.0323646534831895,
0.0688856631311333));
#97957=CARTESIAN_POINT('Ctrl Pts',(0.0106774786875208,-0.0326943950436593,
0.0688139547234062));
#97958=CARTESIAN_POINT('Ctrl Pts',(0.0107510193922467,-0.0325844576448127,
0.0688491494472364));
#97959=CARTESIAN_POINT('Ctrl Pts',(0.0108238374169712,-0.0324744968375319,
0.0688858676041973));
#97960=CARTESIAN_POINT('Ctrl Pts',(0.0108958401118926,-0.0323646534831895,
0.0689240608619753));
#97961=CARTESIAN_POINT('Ctrl Pts',(0.010572541877892,-0.0326943950436593,
0.0688567261340318));
#97962=CARTESIAN_POINT('Ctrl Pts',(0.0106454931124174,-0.0325844576448127,
0.0688904746319527));
#97963=CARTESIAN_POINT('Ctrl Pts',(0.0107177515355465,-0.0324744968375319,
0.0689257342694425));
#97964=CARTESIAN_POINT('Ctrl Pts',(0.0107892251886963,-0.0323646534831895,
0.0689624585928173));
#97965=CARTESIAN_POINT('Ctrl Pts',(0.0104676050682633,-0.0326943950436593,
0.0688994975446573));
#97966=CARTESIAN_POINT('Ctrl Pts',(0.0105399668325881,-0.0325844576448127,
0.068931799816669));
#97967=CARTESIAN_POINT('Ctrl Pts',(0.0106116656541218,-0.0324744968375319,
0.0689656009346878));
#97968=CARTESIAN_POINT('Ctrl Pts',(0.0106826102655001,-0.0323646534831895,
0.0690008563236593));
#97969=CARTESIAN_POINT('Origin',(0.00354377937801091,-0.0326395579068536,
0.0842167833115162));
#97970=CARTESIAN_POINT('Ctrl Pts',(0.0104364351901299,-0.0327445246961876,
0.0688840944638773));
#97971=CARTESIAN_POINT('Ctrl Pts',(0.0106350420621385,-0.0324436878365475,
0.0689713175966564));
#97972=CARTESIAN_POINT('Ctrl Pts',(0.0108265147102331,-0.0321434074463186,
0.0690732528188931));
#97973=CARTESIAN_POINT('Ctrl Pts',(0.0102054060851146,-0.0327445246961876,
0.0687885667054201));
#97974=CARTESIAN_POINT('Ctrl Pts',(0.0104076158453951,-0.0324436878365475,
0.0688670764331495));
#97975=CARTESIAN_POINT('Ctrl Pts',(0.0106033374756105,-0.0321434074463186,
0.0689605943884664));
#97976=CARTESIAN_POINT('Ctrl Pts',(0.010767488922872,-0.0322357242816072,
0.0690422666742474));
#97977=CARTESIAN_POINT('Ctrl Pts',(0.0109301636048097,-0.0319819883628705,
0.0691264653048283));
#97978=CARTESIAN_POINT('Ctrl Pts',(0.0110871508065841,-0.0317295851069886,
0.0692208447518193));
#97979=CARTESIAN_POINT('Ctrl Pts',(0.0105430208645683,-0.0322357242816072,
0.0689322026437861));
#97980=CARTESIAN_POINT('Ctrl Pts',(0.0107092009431285,-0.0319819883628705,
0.0690092522578344));
#97981=CARTESIAN_POINT('Ctrl Pts',(0.0108701413497775,-0.0317295851069886,
0.069096720235077));
#97982=CARTESIAN_POINT('Origin',(0.00358479029800732,-0.0326371942645875,
0.0841307571064515));
#97983=CARTESIAN_POINT('Origin',(0.00404116930378793,-0.0326352985530836,
0.0842767558123109));
#97984=CARTESIAN_POINT('Ctrl Pts',(0.0111149079858754,-0.0321934096636184,
0.0689487341452376));
#97985=CARTESIAN_POINT('Ctrl Pts',(0.0111866374956326,-0.0320835708272304,
0.0689899841010614));
#97986=CARTESIAN_POINT('Ctrl Pts',(0.0112574717336673,-0.0319739230346346,
0.0690326945687108));
#97987=CARTESIAN_POINT('Ctrl Pts',(0.0113273242663435,-0.0318646057455575,
0.0690768039476986));
#97988=CARTESIAN_POINT('Ctrl Pts',(0.0110074924504581,-0.0321934096636184,
0.0689848321717232));
#97989=CARTESIAN_POINT('Ctrl Pts',(0.011078724140297,-0.0320835708272304,
0.0690246007835992));
#97990=CARTESIAN_POINT('Ctrl Pts',(0.0111490915035051,-0.0319739230346346,
0.0690658204641829));
#97991=CARTESIAN_POINT('Ctrl Pts',(0.0112185085573961,-0.0318646057455575,
0.0691084315661897));
#97992=CARTESIAN_POINT('Ctrl Pts',(0.0109000769150408,-0.0321934096636184,
0.0690209301982089));
#97993=CARTESIAN_POINT('Ctrl Pts',(0.0109708107849613,-0.0320835708272304,
0.0690592174661369));
#97994=CARTESIAN_POINT('Ctrl Pts',(0.0110407112733429,-0.0319739230346346,
0.069098946359655));
#97995=CARTESIAN_POINT('Ctrl Pts',(0.0111096928484487,-0.0318646057455575,
0.0691400591846809));
#97996=CARTESIAN_POINT('Ctrl Pts',(0.0107926613796235,-0.0321934096636184,
0.0690570282246946));
#97997=CARTESIAN_POINT('Ctrl Pts',(0.0108628974296257,-0.0320835708272304,
0.0690938341486746));
#97998=CARTESIAN_POINT('Ctrl Pts',(0.0109323310431808,-0.0319739230346346,
0.0691320722551271));
#97999=CARTESIAN_POINT('Ctrl Pts',(0.0110008771395012,-0.0318646057455575,
0.0691716868031721));
#98000=CARTESIAN_POINT('Ctrl Pts',(0.0106825578107348,-0.0320218834582315,
0.0689999062980342));
#98001=CARTESIAN_POINT('Ctrl Pts',(0.0107361578358993,-0.0319391099350631,
0.0690265369664127));
#98002=CARTESIAN_POINT('Ctrl Pts',(0.0107893095445496,-0.0318564869454932,
0.0690539884718543));
#98003=CARTESIAN_POINT('Ctrl Pts',(0.0108419760893676,-0.0317740741446544,
0.0690822372053611));
#98004=CARTESIAN_POINT('Ctrl Pts',(0.0106677844279134,-0.0320218834582315,
0.0689525927142832));
#98005=CARTESIAN_POINT('Ctrl Pts',(0.0107218768731049,-0.0319391099350631,
0.0689790696274609));
#98006=CARTESIAN_POINT('Ctrl Pts',(0.0107755231043464,-0.0318564869454932,
0.069006375160066));
#98007=CARTESIAN_POINT('Ctrl Pts',(0.0108286859041999,-0.0317740741446544,
0.0690344857757955));
#98008=CARTESIAN_POINT('Ctrl Pts',(0.010653011045092,-0.0320218834582315,
0.0689052791305322));
#98009=CARTESIAN_POINT('Ctrl Pts',(0.0107075959103105,-0.0319391099350631,
0.0689316022885092));
#98010=CARTESIAN_POINT('Ctrl Pts',(0.0107617366641432,-0.0318564869454932,
0.0689587618482776));
#98011=CARTESIAN_POINT('Ctrl Pts',(0.0108153957190322,-0.0317740741446544,
0.06898673434623));
#98012=CARTESIAN_POINT('Ctrl Pts',(0.0106382376622707,-0.0320218834582315,
0.0688579655467812));
#98013=CARTESIAN_POINT('Ctrl Pts',(0.0106933149475161,-0.0319391099350631,
0.0688841349495575));
#98014=CARTESIAN_POINT('Ctrl Pts',(0.0107479502239401,-0.0318564869454932,
0.0689111485364893));
#98015=CARTESIAN_POINT('Ctrl Pts',(0.0108021055338645,-0.0317740741446544,
0.0689389829166644));
#98016=CARTESIAN_POINT('Origin',(0.0126380660316932,-0.0391228853390702,
0.0629472387442048));
#98017=CARTESIAN_POINT('Ctrl Pts',(0.00770432963236102,-0.0352722978779549,
0.0684134309825576));
#98018=CARTESIAN_POINT('Ctrl Pts',(0.00772319851265365,-0.0352466642097187,
0.0684124023745188));
#98019=CARTESIAN_POINT('Ctrl Pts',(0.00774204631537146,-0.0352210183808286,
0.0684112963980917));
#98020=CARTESIAN_POINT('Ctrl Pts',(0.00776087367443863,-0.0351953608940152,
0.0684101124826413));
#98021=CARTESIAN_POINT('Origin',(0.00761867736647191,-0.0352456003065027,
0.0635142058516324));
#98022=CARTESIAN_POINT('Ctrl Pts',(0.007885451609313,-0.0350241211493338,
0.0684050475482226));
#98023=CARTESIAN_POINT('Ctrl Pts',(0.00796458597024578,-0.034914423286742,
0.0684017646422982));
#98024=CARTESIAN_POINT('Ctrl Pts',(0.00804383555691403,-0.0348045283677512,
0.0684001155351095));
#98025=CARTESIAN_POINT('Ctrl Pts',(0.00812309893927992,-0.0346945769586886,
0.0684001061163253));
#98026=CARTESIAN_POINT('Ctrl Pts',(0.00780373909046085,-0.0350241211493338,
0.0683265350901932));
#98027=CARTESIAN_POINT('Ctrl Pts',(0.00788395492826286,-0.034914423286742,
0.0683221266278758));
#98028=CARTESIAN_POINT('Ctrl Pts',(0.00796430990517022,-0.0348045283677512,
0.068319373645493));
#98029=CARTESIAN_POINT('Ctrl Pts',(0.00804470122789617,-0.0346945769586886,
0.068318283499325));
#98030=CARTESIAN_POINT('Ctrl Pts',(0.0077220265716087,-0.0350241211493338,
0.0682480226321637));
#98031=CARTESIAN_POINT('Ctrl Pts',(0.00780332388627993,-0.034914423286742,
0.0682424886134533));
#98032=CARTESIAN_POINT('Ctrl Pts',(0.0078847842534264,-0.0348045283677512,
0.0682386317558764));
#98033=CARTESIAN_POINT('Ctrl Pts',(0.00796630351651241,-0.0346945769586886,
0.0682364608823247));
#98034=CARTESIAN_POINT('Ctrl Pts',(0.00764031405275655,-0.0350241211493338,
0.0681695101741343));
#98035=CARTESIAN_POINT('Ctrl Pts',(0.00772269284429701,-0.034914423286742,
0.0681628505990308));
#98036=CARTESIAN_POINT('Ctrl Pts',(0.00780525860168259,-0.0348045283677512,
0.0681578898662599));
#98037=CARTESIAN_POINT('Ctrl Pts',(0.00788790580512866,-0.0346945769586886,
0.0681546382653243));
#98038=CARTESIAN_POINT('Origin',(0.00794501558844048,-0.0345629067942562,
0.0851879360948764));
#98039=CARTESIAN_POINT('Ctrl Pts',(0.00817494210242489,-0.0351970973651569,
0.0682193251277047));
#98040=CARTESIAN_POINT('Ctrl Pts',(0.00825710356490954,-0.0350869349326871,
0.068220033878911));
#98041=CARTESIAN_POINT('Ctrl Pts',(0.0083393183544485,-0.0349764985139992,
0.0682224513085043));
#98042=CARTESIAN_POINT('Ctrl Pts',(0.00842147977500923,-0.0348659306865088,
0.0682265805545339));
#98043=CARTESIAN_POINT('Ctrl Pts',(0.00811927690638267,-0.0351970973651569,
0.0682798384039308));
#98044=CARTESIAN_POINT('Ctrl Pts',(0.00820060003943912,-0.0350869349326871,
0.0682797759892892));
#98045=CARTESIAN_POINT('Ctrl Pts',(0.0082819918371981,-0.0349764985139992,
0.0682814041858056));
#98046=CARTESIAN_POINT('Ctrl Pts',(0.00836334673002591,-0.0348659306865088,
0.0682847270912407));
#98047=CARTESIAN_POINT('Ctrl Pts',(0.00806361171034044,-0.0351970973651569,
0.0683403516801568));
#98048=CARTESIAN_POINT('Ctrl Pts',(0.00814409651396871,-0.0350869349326871,
0.0683395180996673));
#98049=CARTESIAN_POINT('Ctrl Pts',(0.0082246653199477,-0.0349764985139992,
0.068340357063107));
#98050=CARTESIAN_POINT('Ctrl Pts',(0.00830521368504259,-0.0348659306865088,
0.0683428736279475));
#98051=CARTESIAN_POINT('Ctrl Pts',(0.00800794651429821,-0.0351970973651569,
0.0684008649563829));
#98052=CARTESIAN_POINT('Ctrl Pts',(0.00808759298849829,-0.0350869349326871,
0.0683992602100455));
#98053=CARTESIAN_POINT('Ctrl Pts',(0.00816733880269731,-0.0349764985139992,
0.0683993099404083));
#98054=CARTESIAN_POINT('Ctrl Pts',(0.00824708064005927,-0.0348659306865088,
0.0684010201646543));
#98055=CARTESIAN_POINT('Origin',(0.00746700576144667,-0.0345637187965205,
0.0851347199151462));
#98056=CARTESIAN_POINT('Ctrl Pts',(0.00797426489967894,-0.0352450361861252,
0.0684005852837905));
#98057=CARTESIAN_POINT('Ctrl Pts',(0.00819110762834526,-0.0349452761023764,
0.06839494614668));
#98058=CARTESIAN_POINT('Ctrl Pts',(0.00840775909254698,-0.0346444289983475,
0.0684056565109156));
#98059=CARTESIAN_POINT('Ctrl Pts',(0.00772454968035705,-0.0352450361861252,
0.0684125146274031));
#98060=CARTESIAN_POINT('Ctrl Pts',(0.00794094248645773,-0.0349452761023764,
0.0683974573264934));
#98061=CARTESIAN_POINT('Ctrl Pts',(0.0081578547208915,-0.0346444289983475,
0.0683987423929325));
#98062=CARTESIAN_POINT('Ctrl Pts',(0.00824664947816935,-0.0345231616327822,
0.0684014189234823));
#98063=CARTESIAN_POINT('Ctrl Pts',(0.00832588557495387,-0.0344132092796975,
0.0684031124760236));
#98064=CARTESIAN_POINT('Ctrl Pts',(0.00840508255372156,-0.0343032738558974,
0.0684064448773467));
#98065=CARTESIAN_POINT('Ctrl Pts',(0.00848413906334682,-0.034193496108874,
0.0684114092593122));
#98066=CARTESIAN_POINT('Ctrl Pts',(0.00817002804186763,-0.0345231616327822,
0.0683179306510274));
#98067=CARTESIAN_POINT('Ctrl Pts',(0.00825041490694585,-0.0344132092796975,
0.0683185680849436));
#98068=CARTESIAN_POINT('Ctrl Pts',(0.00833078443961359,-0.0343032738558974,
0.068320868224867));
#98069=CARTESIAN_POINT('Ctrl Pts',(0.00841103375269323,-0.034193496108874,
0.0683248254866254));
#98070=CARTESIAN_POINT('Ctrl Pts',(0.00809340660556591,-0.0345231616327822,
0.0682344423785725));
#98071=CARTESIAN_POINT('Ctrl Pts',(0.00817494423893782,-0.0344132092796975,
0.0682340236938637));
#98072=CARTESIAN_POINT('Ctrl Pts',(0.00825648632550562,-0.0343032738558974,
0.0682352915723873));
#98073=CARTESIAN_POINT('Ctrl Pts',(0.00833792844203965,-0.034193496108874,
0.0682382417139386));
#98074=CARTESIAN_POINT('Ctrl Pts',(0.00801678516926419,-0.0345231616327822,
0.0681509541061177));
#98075=CARTESIAN_POINT('Ctrl Pts',(0.0080994735709298,-0.0344132092796975,
0.0681494793027837));
#98076=CARTESIAN_POINT('Ctrl Pts',(0.00818218821139765,-0.0343032738558974,
0.0681497149199076));
#98077=CARTESIAN_POINT('Ctrl Pts',(0.00826482313138606,-0.034193496108874,
0.0681516579412518));
#98078=CARTESIAN_POINT('Origin',(0.00794507010844505,-0.0345625596230578,
0.0852000396209644));
#98079=CARTESIAN_POINT('Ctrl Pts',(0.00861564243684595,-0.0346945769586885,
0.0681701945265211));
#98080=CARTESIAN_POINT('Ctrl Pts',(0.00869804717875144,-0.0345846629176052,
0.0681769726092896));
#98081=CARTESIAN_POINT('Ctrl Pts',(0.00878032582762136,-0.0344746925050311,
0.0681854559459922));
#98082=CARTESIAN_POINT('Ctrl Pts',(0.00886237300346016,-0.034364806625326,
0.0681956332314106));
#98083=CARTESIAN_POINT('Ctrl Pts',(0.00853381988427018,-0.0346945769586885,
0.068248592176177));
#98084=CARTESIAN_POINT('Ctrl Pts',(0.00861514426693746,-0.0345846629176052,
0.0682542427028139));
#98085=CARTESIAN_POINT('Ctrl Pts',(0.00869636568943892,-0.0344746925050311,
0.0682615759494103));
#98086=CARTESIAN_POINT('Ctrl Pts',(0.00877738012033336,-0.034364806625326,
0.0682705820899701));
#98087=CARTESIAN_POINT('Ctrl Pts',(0.0084519973316944,-0.0346945769586885,
0.0683269898258329));
#98088=CARTESIAN_POINT('Ctrl Pts',(0.00853224135512349,-0.0345846629176052,
0.0683315127963383));
#98089=CARTESIAN_POINT('Ctrl Pts',(0.00861240555125647,-0.0344746925050311,
0.0683376959528283));
#98090=CARTESIAN_POINT('Ctrl Pts',(0.00869238723720655,-0.034364806625326,
0.0683455309485296));
#98091=CARTESIAN_POINT('Ctrl Pts',(0.00837017477911863,-0.0346945769586885,
0.0684053874754887));
#98092=CARTESIAN_POINT('Ctrl Pts',(0.00844933844330952,-0.0345846629176052,
0.0684087828898626));
#98093=CARTESIAN_POINT('Ctrl Pts',(0.00852844541307403,-0.0344746925050311,
0.0684138159562464));
#98094=CARTESIAN_POINT('Ctrl Pts',(0.00860739435407974,-0.034364806625326,
0.0684204798070892));
#98095=CARTESIAN_POINT('Origin',(0.00746429588693701,-0.0345626446732229,
0.0851930876050632));
#98096=CARTESIAN_POINT('Ctrl Pts',(0.00837163885895575,-0.0346945769586886,
0.0684039846786495));
#98097=CARTESIAN_POINT('Ctrl Pts',(0.00849199145043852,-0.0345275153362891,
0.068409176135752));
#98098=CARTESIAN_POINT('Ctrl Pts',(0.00861221190471851,-0.0343603235965159,
0.0684181539138563));
#98099=CARTESIAN_POINT('Ctrl Pts',(0.00873194505769413,-0.034193496108874,
0.0684308861761511));
#98100=CARTESIAN_POINT('Ctrl Pts',(0.00828782466928575,-0.0346945769586886,
0.0684021930477631));
#98101=CARTESIAN_POINT('Ctrl Pts',(0.00840821478719476,-0.0345275153362891,
0.0684056289831056));
#98102=CARTESIAN_POINT('Ctrl Pts',(0.00852852798715076,-0.0343603235965159,
0.0684128519655537));
#98103=CARTESIAN_POINT('Ctrl Pts',(0.00864840875361607,-0.034193496108874,
0.0684238353441258));
#98104=CARTESIAN_POINT('Ctrl Pts',(0.00820401047961575,-0.0346945769586886,
0.0684004014168768));
#98105=CARTESIAN_POINT('Ctrl Pts',(0.00832443812395101,-0.0345275153362891,
0.0684020818304593));
#98106=CARTESIAN_POINT('Ctrl Pts',(0.00844484406958301,-0.0343603235965159,
0.0684075500172511));
#98107=CARTESIAN_POINT('Ctrl Pts',(0.00856487244953801,-0.034193496108874,
0.0684167845121004));
#98108=CARTESIAN_POINT('Ctrl Pts',(0.00812019628994575,-0.0346945769586886,
0.0683986097859904));
#98109=CARTESIAN_POINT('Ctrl Pts',(0.00824066146070725,-0.0345275153362891,
0.068398534677813));
#98110=CARTESIAN_POINT('Ctrl Pts',(0.00836116015201525,-0.0343603235965159,
0.0684022480689486));
#98111=CARTESIAN_POINT('Ctrl Pts',(0.00848133614545995,-0.034193496108874,
0.0684097336800751));
#98112=CARTESIAN_POINT('Ctrl Pts',(0.00860736286472677,-0.0340223579322365,
0.0684204777080269));
#98113=CARTESIAN_POINT('Ctrl Pts',(0.00868638792035394,-0.0339125849573552,
0.0684271475467199));
#98114=CARTESIAN_POINT('Ctrl Pts',(0.00876521939582711,-0.0338030433565217,
0.0684354483336169));
#98115=CARTESIAN_POINT('Ctrl Pts',(0.00884375741997943,-0.0336938721132321,
0.0684453605168362));
#98116=CARTESIAN_POINT('Ctrl Pts',(0.0085361347600194,-0.0340223579322365,
0.0683323429422979));
#98117=CARTESIAN_POINT('Ctrl Pts',(0.00861637542393109,-0.0339125849573552,
0.0683380303596563));
#98118=CARTESIAN_POINT('Ctrl Pts',(0.0086964419873337,-0.0338030433565217,
0.0683453745758217));
#98119=CARTESIAN_POINT('Ctrl Pts',(0.00877623289115136,-0.0336938721132321,
0.0683543571221916));
#98120=CARTESIAN_POINT('Ctrl Pts',(0.00846490665531203,-0.0340223579322365,
0.0682442081765689));
#98121=CARTESIAN_POINT('Ctrl Pts',(0.00854636292750823,-0.0339125849573552,
0.0682489131725927));
#98122=CARTESIAN_POINT('Ctrl Pts',(0.00862766457884028,-0.0338030433565217,
0.0682553008180264));
#98123=CARTESIAN_POINT('Ctrl Pts',(0.00870870836232328,-0.0336938721132321,
0.0682633537275469));
#98124=CARTESIAN_POINT('Ctrl Pts',(0.00839367855060466,-0.0340223579322365,
0.0681560734108399));
#98125=CARTESIAN_POINT('Ctrl Pts',(0.00847635043108537,-0.0339125849573552,
0.0681597959855291));
#98126=CARTESIAN_POINT('Ctrl Pts',(0.00855888717034687,-0.0338030433565217,
0.0681652270602311));
#98127=CARTESIAN_POINT('Ctrl Pts',(0.00864118383349521,-0.0336938721132321,
0.0681723503329022));
#98128=CARTESIAN_POINT('Origin',(0.00794960615951678,-0.0345589643415262,
0.0850799051032651));
#98129=CARTESIAN_POINT('Ctrl Pts',(0.0089901469553743,-0.034193496108874,
0.0682128784669059));
#98130=CARTESIAN_POINT('Ctrl Pts',(0.00907201634549192,-0.0340836138581107,
0.0682248251239368));
#98131=CARTESIAN_POINT('Ctrl Pts',(0.00915359924213727,-0.03397388966435,
0.0682384601639801));
#98132=CARTESIAN_POINT('Ctrl Pts',(0.00923479239911469,-0.0338644633294063,
0.0682537591363501));
#98133=CARTESIAN_POINT('Ctrl Pts',(0.00890356310478089,-0.034193496108874,
0.0682859838433384));
#98134=CARTESIAN_POINT('Ctrl Pts',(0.00898442441504878,-0.0340836138581107,
0.0682967365603425));
#98135=CARTESIAN_POINT('Ctrl Pts',(0.00906502442162371,-0.03397388966435,
0.0683091573731367));
#98136=CARTESIAN_POINT('Ctrl Pts',(0.00914526103211158,-0.0338644633294063,
0.0683232234694246));
#98137=CARTESIAN_POINT('Ctrl Pts',(0.00881697925418748,-0.034193496108874,
0.0683590892197709));
#98138=CARTESIAN_POINT('Ctrl Pts',(0.00889683248460565,-0.0340836138581107,
0.0683686479967483));
#98139=CARTESIAN_POINT('Ctrl Pts',(0.00897644960111015,-0.03397388966435,
0.0683798545822933));
#98140=CARTESIAN_POINT('Ctrl Pts',(0.00905572966510848,-0.0338644633294063,
0.068392687802499));
#98141=CARTESIAN_POINT('Ctrl Pts',(0.00873039540359407,-0.034193496108874,
0.0684321945962035));
#98142=CARTESIAN_POINT('Ctrl Pts',(0.00880924055416252,-0.0340836138581107,
0.068440559433154));
#98143=CARTESIAN_POINT('Ctrl Pts',(0.00888787478059659,-0.03397388966435,
0.0684505517914499));
#98144=CARTESIAN_POINT('Ctrl Pts',(0.00896619829810537,-0.0338644633294063,
0.0684621521355734));
#98145=CARTESIAN_POINT('Origin',(0.00746992174341197,-0.034561062186391,
0.0851180216646338));
#98146=CARTESIAN_POINT('Ctrl Pts',(0.0086959585135099,-0.0342436276873901,
0.0684271738399308));
#98147=CARTESIAN_POINT('Ctrl Pts',(0.00891179846029925,-0.0339430054201861,
0.0684487538256049));
#98148=CARTESIAN_POINT('Ctrl Pts',(0.00912539973548516,-0.0336441434784162,
0.0684865304539705));
#98149=CARTESIAN_POINT('Ctrl Pts',(0.00844671696444653,-0.0342436276873901,
0.0684077149031538));
#98150=CARTESIAN_POINT('Ctrl Pts',(0.008663290817135,-0.0339430054201861,
0.0684198945888393));
#98151=CARTESIAN_POINT('Ctrl Pts',(0.00887833198238197,-0.0336441434784162,
0.0684483529032824));
#98152=CARTESIAN_POINT('Ctrl Pts',(0.00896617084773448,-0.0335235895815127,
0.068462148197955));
#98153=CARTESIAN_POINT('Ctrl Pts',(0.00904447532613822,-0.0334144449262719,
0.0684737453362964));
#98154=CARTESIAN_POINT('Ctrl Pts',(0.00912263017875049,-0.0333049234473133,
0.0684869735099379));
#98155=CARTESIAN_POINT('Ctrl Pts',(0.00920053393729631,-0.0331951640388588,
0.0685018248567473));
#98156=CARTESIAN_POINT('Ctrl Pts',(0.00890061738404836,-0.0335235895815127,
0.0683697148928912));
#98157=CARTESIAN_POINT('Ctrl Pts',(0.00898019438888071,-0.0334144449262719,
0.0683804095587421));
#98158=CARTESIAN_POINT('Ctrl Pts',(0.00905964187430276,-0.0333049234473133,
0.0683927605124998));
#98159=CARTESIAN_POINT('Ctrl Pts',(0.009138856820767,-0.0331951640388588,
0.0684067611634522));
#98160=CARTESIAN_POINT('Ctrl Pts',(0.00883506392036223,-0.0335235895815127,
0.0682772815878273));
#98161=CARTESIAN_POINT('Ctrl Pts',(0.00891591345162321,-0.0334144449262719,
0.0682870737811877));
#98162=CARTESIAN_POINT('Ctrl Pts',(0.00899665356985503,-0.0333049234473133,
0.0682985475150617));
#98163=CARTESIAN_POINT('Ctrl Pts',(0.00907717970423769,-0.0331951640388588,
0.0683116974701572));
#98164=CARTESIAN_POINT('Ctrl Pts',(0.00876951045667611,-0.0335235895815127,
0.0681848482827635));
#98165=CARTESIAN_POINT('Ctrl Pts',(0.0088516325143657,-0.0334144449262719,
0.0681937380036333));
#98166=CARTESIAN_POINT('Ctrl Pts',(0.0089336652654073,-0.0333049234473133,
0.0682043345176235));
#98167=CARTESIAN_POINT('Ctrl Pts',(0.00901550258770838,-0.0331951640388588,
0.0682166337768621));
#98168=CARTESIAN_POINT('Origin',(0.00533496082260069,-0.0326434571769664,
0.0847144182816732));
#98169=CARTESIAN_POINT('Ctrl Pts',(0.00936286061526512,-0.0336938721132348,
0.068277785324231));
#98170=CARTESIAN_POINT('Ctrl Pts',(0.00939723263636825,-0.0336474569764937,
0.0682850380614053));
#98171=CARTESIAN_POINT('Ctrl Pts',(0.00943151739983263,-0.033601104548885,
0.0682926926695225));
#98172=CARTESIAN_POINT('Ctrl Pts',(0.00951831853082757,-0.0334837508694588,
0.068312072375688));
#98173=CARTESIAN_POINT('Ctrl Pts',(0.00960450728434494,-0.0333660264863561,
0.0683340156689728));
#98174=CARTESIAN_POINT('Ctrl Pts',(0.00908985111544777,-0.0336938721132348,
0.0684803584031007));
#98175=CARTESIAN_POINT('Ctrl Pts',(0.00912303740909947,-0.0336474569764937,
0.0684860131250785));
#98176=CARTESIAN_POINT('Ctrl Pts',(0.00915615523314472,-0.033601104548885,
0.0684920559470593));
#98177=CARTESIAN_POINT('Ctrl Pts',(0.00924000194208312,-0.0334837508694588,
0.0685073549816545));
#98178=CARTESIAN_POINT('Ctrl Pts',(0.00932335848965693,-0.0333660264863561,
0.0685251318496555));
#98179=CARTESIAN_POINT('Ctrl Pts',(0.00908985111545924,-0.0336938721132427,
0.068480358403111));
#98180=CARTESIAN_POINT('Ctrl Pts',(0.0091230374091102,-0.0336474569765026,
0.0684860131250887));
#98181=CARTESIAN_POINT('Ctrl Pts',(0.00915615523315472,-0.0336011045488949,
0.0684920559470693));
#98182=CARTESIAN_POINT('Ctrl Pts',(0.00923930361320096,-0.033484728265791,
0.0685072275615425));
#98183=CARTESIAN_POINT('Ctrl Pts',(0.00932197026244842,-0.0333679870047996,
0.0685248359712446));
#98184=CARTESIAN_POINT('Ctrl Pts',(0.0090898511154422,-0.0336938721132426,
0.0684803584030998));
#98185=CARTESIAN_POINT('Ctrl Pts',(0.00920853998794152,-0.0335278710435082,
0.0685005821913567));
#98186=CARTESIAN_POINT('Ctrl Pts',(0.00932655289322954,-0.033362046922432,
0.0685245209171148));
#98187=CARTESIAN_POINT('Ctrl Pts',(0.00944394454052174,-0.0331951640388602,
0.0685522061152207));
#98188=CARTESIAN_POINT('Ctrl Pts',(0.00900692236778153,-0.0336938721132426,
0.0684680761950446));
#98189=CARTESIAN_POINT('Ctrl Pts',(0.00912586835731391,-0.0335278710435082,
0.0684865639441905));
#98190=CARTESIAN_POINT('Ctrl Pts',(0.00924419273091696,-0.033362046922432,
0.0685087753046955));
#98191=CARTESIAN_POINT('Ctrl Pts',(0.00936195064002609,-0.0331951640388602,
0.0685347410041479));
#98192=CARTESIAN_POINT('Ctrl Pts',(0.00892399362012087,-0.0336938721132426,
0.0684557939869894));
#98193=CARTESIAN_POINT('Ctrl Pts',(0.0090431967266863,-0.0335278710435082,
0.0684725456970244));
#98194=CARTESIAN_POINT('Ctrl Pts',(0.00916183256860439,-0.033362046922432,
0.0684930296922761));
#98195=CARTESIAN_POINT('Ctrl Pts',(0.00927995673953043,-0.0331951640388602,
0.0685172758930751));
#98196=CARTESIAN_POINT('Ctrl Pts',(0.00884106487246021,-0.0336938721132426,
0.0684435117789343));
#98197=CARTESIAN_POINT('Ctrl Pts',(0.0089605250960587,-0.0335278710435082,
0.0684585274498582));
#98198=CARTESIAN_POINT('Ctrl Pts',(0.00907947240629182,-0.033362046922432,
0.0684772840798568));
#98199=CARTESIAN_POINT('Ctrl Pts',(0.00919796283903478,-0.0331951640388602,
0.0684998107820023));
#98200=CARTESIAN_POINT('Ctrl Pts',(0.00932165060079693,-0.0330240426238155,
0.068526265292725));
#98201=CARTESIAN_POINT('Ctrl Pts',(0.00939912302532848,-0.0329142774063509,
0.0685427670970675));
#98202=CARTESIAN_POINT('Ctrl Pts',(0.00947629293429782,-0.0328043479726686,
0.0685608786995848));
#98203=CARTESIAN_POINT('Ctrl Pts',(0.00955306082831667,-0.0326943950436594,
0.0685805796205633));
#98204=CARTESIAN_POINT('Ctrl Pts',(0.0092620304964448,-0.0330240426238155,
0.0684298983941466));
#98205=CARTESIAN_POINT('Ctrl Pts',(0.00934083046888998,-0.0329142774063509,
0.0684455788734666));
#98206=CARTESIAN_POINT('Ctrl Pts',(0.00941934556668648,-0.0328043479726686,
0.0684628961856246));
#98207=CARTESIAN_POINT('Ctrl Pts',(0.00949747459518195,-0.0326943950436594,
0.0684818309159112));
#98208=CARTESIAN_POINT('Ctrl Pts',(0.00920241039209268,-0.0330240426238155,
0.0683335314955683));
#98209=CARTESIAN_POINT('Ctrl Pts',(0.00928253791245148,-0.0329142774063509,
0.0683483906498657));
#98210=CARTESIAN_POINT('Ctrl Pts',(0.00936239819907514,-0.0328043479726686,
0.0683649136716645));
#98211=CARTESIAN_POINT('Ctrl Pts',(0.00944188836204723,-0.0326943950436594,
0.0683830822112591));
#98212=CARTESIAN_POINT('Ctrl Pts',(0.00914279028774055,-0.0330240426238155,
0.0682371645969899));
#98213=CARTESIAN_POINT('Ctrl Pts',(0.00922424535601299,-0.0329142774063509,
0.0682512024262648));
#98214=CARTESIAN_POINT('Ctrl Pts',(0.0093054508314638,-0.0328043479726686,
0.0682669311577043));
#98215=CARTESIAN_POINT('Ctrl Pts',(0.00938630212891251,-0.0326943950436594,
0.068284333506607));
#98216=CARTESIAN_POINT('Origin',(0.00530607407682471,-0.0326396682858201,
0.0848346719908854));
#98217=CARTESIAN_POINT('Ctrl Pts',(0.00972743405026172,-0.0331951640388587,
0.0683682787406266));
#98218=CARTESIAN_POINT('Ctrl Pts',(0.00980706556428271,-0.0330855618255041,
0.0683903658007976));
#98219=CARTESIAN_POINT('Ctrl Pts',(0.00988629798176981,-0.0329757224427708,
0.0684141146304979));
#98220=CARTESIAN_POINT('Ctrl Pts',(0.00996502834909326,-0.0328657862078596,
0.0684394997948417));
#98221=CARTESIAN_POINT('Ctrl Pts',(0.00963237043264987,-0.0331951640388587,
0.0684299558080528));
#98222=CARTESIAN_POINT('Ctrl Pts',(0.00971115246983876,-0.0330855618255041,
0.0684507335592033));
#98223=CARTESIAN_POINT('Ctrl Pts',(0.00978956185929717,-0.0329757224427708,
0.0684731545787865));
#98224=CARTESIAN_POINT('Ctrl Pts',(0.00986749678473739,-0.0328657862078596,
0.0684971950805594));
#98225=CARTESIAN_POINT('Ctrl Pts',(0.00953730681503803,-0.0331951640388587,
0.0684916328754789));
#98226=CARTESIAN_POINT('Ctrl Pts',(0.00961523937539481,-0.0330855618255041,
0.068511101317609));
#98227=CARTESIAN_POINT('Ctrl Pts',(0.00969282573682452,-0.0329757224427708,
0.0685321945270751));
#98228=CARTESIAN_POINT('Ctrl Pts',(0.00976996522038151,-0.0328657862078596,
0.068554890366277));
#98229=CARTESIAN_POINT('Ctrl Pts',(0.00944224319742619,-0.0331951640388587,
0.0685533099429051));
#98230=CARTESIAN_POINT('Ctrl Pts',(0.00951932628095086,-0.0330855618255041,
0.0685714690760147));
#98231=CARTESIAN_POINT('Ctrl Pts',(0.00959608961435188,-0.0329757224427708,
0.0685912344753637));
#98232=CARTESIAN_POINT('Ctrl Pts',(0.00967243365602564,-0.0328657862078596,
0.0686125856519946));
#98233=CARTESIAN_POINT('Origin',(0.00485239013941621,-0.0326401908836119,
0.0846751609994067));
#98234=CARTESIAN_POINT('Ctrl Pts',(0.00940877767744207,-0.0332451089994432,
0.0685440289328928));
#98235=CARTESIAN_POINT('Ctrl Pts',(0.00962021033545713,-0.0329451141710258,
0.0685924933305034));
#98236=CARTESIAN_POINT('Ctrl Pts',(0.00982739179905341,-0.0326442513127503,
0.0686567460180206));
#98237=CARTESIAN_POINT('Ctrl Pts',(0.00916394096079468,-0.0332451089994432,
0.0684934821013271));
#98238=CARTESIAN_POINT('Ctrl Pts',(0.00937728002375266,-0.0329451141710258,
0.0685327123310906));
#98239=CARTESIAN_POINT('Ctrl Pts',(0.00958705803166844,-0.0326442513127503,
0.0685879006822705));
#98240=CARTESIAN_POINT('Ctrl Pts',(0.00967240325991672,-0.0325229783203384,
0.0686125770579851));
#98241=CARTESIAN_POINT('Ctrl Pts',(0.00974873651268751,-0.0324130253112079,
0.0686339247651364));
#98242=CARTESIAN_POINT('Ctrl Pts',(0.00982461658328766,-0.0323031222247694,
0.0686568482858514));
#98243=CARTESIAN_POINT('Ctrl Pts',(0.00989994731088243,-0.0321934096636184,
0.06868131482697));
#98244=CARTESIAN_POINT('Ctrl Pts',(0.00961895169997607,-0.0325229783203384,
0.0685126567227713));
#98245=CARTESIAN_POINT('Ctrl Pts',(0.0096966623523576,-0.0324130253112079,
0.0685332676013511));
#98246=CARTESIAN_POINT('Ctrl Pts',(0.00977393485590409,-0.0323031222247694,
0.068555482898529));
#98247=CARTESIAN_POINT('Ctrl Pts',(0.00985067123416174,-0.0321934096636184,
0.068579270665391));
#98248=CARTESIAN_POINT('Ctrl Pts',(0.00956550014003542,-0.0325229783203384,
0.0684127363875574));
#98249=CARTESIAN_POINT('Ctrl Pts',(0.00964458819202769,-0.0324130253112079,
0.0684326104375657));
#98250=CARTESIAN_POINT('Ctrl Pts',(0.00972325312852053,-0.0323031222247694,
0.0684541175112065));
#98251=CARTESIAN_POINT('Ctrl Pts',(0.00980139515744106,-0.0321934096636184,
0.068477226503812));
#98252=CARTESIAN_POINT('Ctrl Pts',(0.00951204858009477,-0.0325229783203384,
0.0683128160523436));
#98253=CARTESIAN_POINT('Ctrl Pts',(0.00959251403169778,-0.0324130253112079,
0.0683319532737804));
#98254=CARTESIAN_POINT('Ctrl Pts',(0.00967257140113696,-0.0323031222247694,
0.068352752123884));
#98255=CARTESIAN_POINT('Ctrl Pts',(0.00975211908072037,-0.0321934096636184,
0.068375182342233));
#98256=CARTESIAN_POINT('Origin',(0.00530847784489562,-0.0326393375179126,
0.0848264919594345));
#98257=CARTESIAN_POINT('Ctrl Pts',(0.0100873068912915,-0.0326943950436593,
0.0684803817800777));
#98258=CARTESIAN_POINT('Ctrl Pts',(0.0101654448563588,-0.0325844576448127,
0.0685074428304561));
#98259=CARTESIAN_POINT('Ctrl Pts',(0.0102430286844823,-0.0324744968375319,
0.0685361218172136));
#98260=CARTESIAN_POINT('Ctrl Pts',(0.0103199594775635,-0.0323646534831894,
0.0685663806240671));
#98261=CARTESIAN_POINT('Ctrl Pts',(0.00998855821894807,-0.0326943950436593,
0.0685359679950257));
#98262=CARTESIAN_POINT('Ctrl Pts',(0.0100659301017937,-0.0325844576448127,
0.0685616681036245));
#98263=CARTESIAN_POINT('Ctrl Pts',(0.0101427759399861,-0.0324744968375319,
0.06858897020845));
#98264=CARTESIAN_POINT('Ctrl Pts',(0.0102189977566495,-0.0323646534831894,
0.0686178379704027));
#98265=CARTESIAN_POINT('Ctrl Pts',(0.00988980954660469,-0.0326943950436593,
0.0685915542099737));
#98266=CARTESIAN_POINT('Ctrl Pts',(0.00996641534722872,-0.0325844576448127,
0.0686158933767928));
#98267=CARTESIAN_POINT('Ctrl Pts',(0.0100425231954899,-0.0324744968375319,
0.0686418185996864));
#98268=CARTESIAN_POINT('Ctrl Pts',(0.0101180360357355,-0.0323646534831894,
0.0686692953167383));
#98269=CARTESIAN_POINT('Ctrl Pts',(0.00979106087426132,-0.0326943950436593,
0.0686471404249216));
#98270=CARTESIAN_POINT('Ctrl Pts',(0.0098669005926637,-0.0325844576448127,
0.0686701186499611));
#98271=CARTESIAN_POINT('Ctrl Pts',(0.00994227045099364,-0.0324744968375319,
0.0686946669909228));
#98272=CARTESIAN_POINT('Ctrl Pts',(0.0100170743148215,-0.0323646534831894,
0.068720752663074));
#98273=CARTESIAN_POINT('Origin',(0.00484159657221721,-0.0326395579068595,
0.0847114302808474));
#98274=CARTESIAN_POINT('Ctrl Pts',(0.00975820626200597,-0.0327445246961877,
0.0686357654236504));
#98275=CARTESIAN_POINT('Ctrl Pts',(0.00996617901678053,-0.0324436878365475,
0.0686974087344984));
#98276=CARTESIAN_POINT('Ctrl Pts',(0.0101689177168719,-0.0321434074463188,
0.0687745422809362));
#98277=CARTESIAN_POINT('Ctrl Pts',(0.00951702608762621,-0.0327445246961877,
0.0685699465548805));
#98278=CARTESIAN_POINT('Ctrl Pts',(0.00972748124159231,-0.0324436878365475,
0.0686224936068429));
#98279=CARTESIAN_POINT('Ctrl Pts',(0.00993338045603041,-0.0321434074463188,
0.0686907437203563));
#98280=CARTESIAN_POINT('Ctrl Pts',(0.0101064737717701,-0.0322357242816073,
0.0687511983640899));
#98281=CARTESIAN_POINT('Ctrl Pts',(0.0102784186018846,-0.0319819883628706,
0.0688143445194136));
#98282=CARTESIAN_POINT('Ctrl Pts',(0.0104459967939566,-0.0317295851069886,
0.0688883040426486));
#98283=CARTESIAN_POINT('Ctrl Pts',(0.00986998103031469,-0.0322357242816073,
0.0686701355289624));
#98284=CARTESIAN_POINT('Ctrl Pts',(0.0100445076065934,-0.0319819883628706,
0.0687257496971906));
#98285=CARTESIAN_POINT('Ctrl Pts',(0.0102151415944866,-0.0317295851069886,
0.0687923567817306));
#98286=CARTESIAN_POINT('Origin',(0.00487150216666944,-0.0326371942646915,
0.0846209423866145));
#98287=CARTESIAN_POINT('Origin',(0.00534258097687683,-0.0326352985530559,
0.0847085903938754));
#98288=CARTESIAN_POINT('Ctrl Pts',(0.0104394305973869,-0.0321934096636184,
0.0686148602124408));
#98289=CARTESIAN_POINT('Ctrl Pts',(0.0105157644888829,-0.0320835708272304,
0.0686467948086424));
#98290=CARTESIAN_POINT('Ctrl Pts',(0.010591393218811,-0.0319739230346346,
0.0686802906073974));
#98291=CARTESIAN_POINT('Ctrl Pts',(0.0106662233145021,-0.0318646057455575,
0.068715297326964));
#98292=CARTESIAN_POINT('Ctrl Pts',(0.0103373863479351,-0.0321934096636184,
0.0686641363315943));
#98293=CARTESIAN_POINT('Ctrl Pts',(0.0104130406833445,-0.0320835708272304,
0.0686946636580675));
#98294=CARTESIAN_POINT('Ctrl Pts',(0.01048801937473,-0.0319739230346346,
0.0687267389399899));
#98295=CARTESIAN_POINT('Ctrl Pts',(0.0105622296416174,-0.0318646057455575,
0.0687603137769014));
#98296=CARTESIAN_POINT('Ctrl Pts',(0.0102353420984833,-0.0321934096636184,
0.0687134124507479));
#98297=CARTESIAN_POINT('Ctrl Pts',(0.0103103168778061,-0.0320835708272304,
0.0687425325074927));
#98298=CARTESIAN_POINT('Ctrl Pts',(0.0103846455306491,-0.0319739230346346,
0.0687731872725824));
#98299=CARTESIAN_POINT('Ctrl Pts',(0.0104582359687327,-0.0318646057455575,
0.0688053302268388));
#98300=CARTESIAN_POINT('Ctrl Pts',(0.0101332978490316,-0.0321934096636184,
0.0687626885699015));
#98301=CARTESIAN_POINT('Ctrl Pts',(0.0102075930722677,-0.0320835708272304,
0.0687904013569179));
#98302=CARTESIAN_POINT('Ctrl Pts',(0.0102812716865681,-0.0319739230346346,
0.0688196356051749));
#98303=CARTESIAN_POINT('Ctrl Pts',(0.0103542422958481,-0.0318646057455575,
0.0688503466767762));
#98304=CARTESIAN_POINT('Ctrl Pts',(0.0100169032038936,-0.0320218834582322,
0.0687198167030099));
#98305=CARTESIAN_POINT('Ctrl Pts',(0.01007341828463,-0.0319391099350637,
0.068739519516141));
#98306=CARTESIAN_POINT('Ctrl Pts',(0.0101295914621253,-0.0318564869454936,
0.0687600928827483));
#98307=CARTESIAN_POINT('Ctrl Pts',(0.0101853832206213,-0.0317740741446547,
0.0687815179981912));
#98308=CARTESIAN_POINT('Ctrl Pts',(0.00999631634916544,-0.0320218834582322,
0.0686747277968386));
#98309=CARTESIAN_POINT('Ctrl Pts',(0.0100533006964134,-0.0319391099350637,
0.0686942163505805));
#98310=CARTESIAN_POINT('Ctrl Pts',(0.0101099462017939,-0.0318564869454936,
0.0687145829152751));
#98311=CARTESIAN_POINT('Ctrl Pts',(0.0101662129914586,-0.0317740741446547,
0.0687358088047925));
#98312=CARTESIAN_POINT('Ctrl Pts',(0.0099757294944373,-0.0320218834582322,
0.0686296388906674));
#98313=CARTESIAN_POINT('Ctrl Pts',(0.0100331831081968,-0.0319391099350637,
0.0686489131850199));
#98314=CARTESIAN_POINT('Ctrl Pts',(0.0100903009414625,-0.0318564869454936,
0.0686690729478019));
#98315=CARTESIAN_POINT('Ctrl Pts',(0.0101470427622958,-0.0317740741446547,
0.0686900996113937));
#98316=CARTESIAN_POINT('Ctrl Pts',(0.00995514263970917,-0.0320218834582322,
0.0685845499844961));
#98317=CARTESIAN_POINT('Ctrl Pts',(0.0100130655199801,-0.0319391099350637,
0.0686036100194593));
#98318=CARTESIAN_POINT('Ctrl Pts',(0.0100706556811311,-0.0318564869454936,
0.0686235629803287));
#98319=CARTESIAN_POINT('Ctrl Pts',(0.0101278725331331,-0.0317740741446547,
0.068644390417995));
#98320=CARTESIAN_POINT('Origin',(0.0111983912622235,-0.0391228853390594,
0.0624697860721113));
#98321=CARTESIAN_POINT('Ctrl Pts',(0.0069886543965657,-0.0352722978779554,
0.0685112368884557));
#98322=CARTESIAN_POINT('Ctrl Pts',(0.0070072455713299,-0.035246664209719,
0.0685078514935177));
#98323=CARTESIAN_POINT('Ctrl Pts',(0.00702580613789197,-0.0352210183808288,
0.0685043919819847));
#98324=CARTESIAN_POINT('Ctrl Pts',(0.00704433665365789,-0.0351953608940152,
0.0685008577082699));
#98325=CARTESIAN_POINT('Origin',(0.00628964179675846,-0.0352456003065018,
0.0636613786864799));
#98326=CARTESIAN_POINT('Ctrl Pts',(0.0071672974496976,-0.0350241211493339,
0.0684802189569634));
#98327=CARTESIAN_POINT('Ctrl Pts',(0.00724539635534315,-0.0349144232867421,
0.068467043772391));
#98328=CARTESIAN_POINT('Ctrl Pts',(0.00732381434741339,-0.0348045283677512,
0.0684554750619493));
#98329=CARTESIAN_POINT('Ctrl Pts',(0.00740245153384783,-0.0346945769586886,
0.0684455313814199));
#98330=CARTESIAN_POINT('Ctrl Pts',(0.00707638903822302,-0.0350241211493339,
0.0684125668873264));
#98331=CARTESIAN_POINT('Ctrl Pts',(0.00715541982334738,-0.0349144232867421,
0.0683981394767163));
#98332=CARTESIAN_POINT('Ctrl Pts',(0.007234796137077,-0.0348045283677512,
0.0683853370533331));
#98333=CARTESIAN_POINT('Ctrl Pts',(0.00731441691866725,-0.0346945769586886,
0.0683741797988656));
#98334=CARTESIAN_POINT('Ctrl Pts',(0.00698548062674844,-0.0350241211493339,
0.0683449148176895));
#98335=CARTESIAN_POINT('Ctrl Pts',(0.0070654432913516,-0.0349144232867421,
0.0683292351810417));
#98336=CARTESIAN_POINT('Ctrl Pts',(0.00714577792674061,-0.0348045283677512,
0.068315199044717));
#98337=CARTESIAN_POINT('Ctrl Pts',(0.00722638230348667,-0.0346945769586886,
0.0683028282163112));
#98338=CARTESIAN_POINT('Ctrl Pts',(0.00689457221527386,-0.0350241211493339,
0.0682772627480525));
#98339=CARTESIAN_POINT('Ctrl Pts',(0.00697546675935583,-0.0349144232867421,
0.068260330885367));
#98340=CARTESIAN_POINT('Ctrl Pts',(0.00705675971640422,-0.0348045283677512,
0.0682450610361009));
#98341=CARTESIAN_POINT('Ctrl Pts',(0.0071383476883061,-0.0346945769586886,
0.0682314766337569));
#98342=CARTESIAN_POINT('Origin',(0.00932984543910564,-0.0345629067942411,
0.0851233040683128));
#98343=CARTESIAN_POINT('Ctrl Pts',(0.00743122803229611,-0.0351970973651569,
0.0682596782336155));
#98344=CARTESIAN_POINT('Ctrl Pts',(0.0075128304571892,-0.035086934932687,
0.0682500838343393));
#98345=CARTESIAN_POINT('Ctrl Pts',(0.00759469994282422,-0.034976498513999,
0.0682421779563585));
#98346=CARTESIAN_POINT('Ctrl Pts',(0.00767673102780055,-0.0348659306865085,
0.0682359770855367));
#98347=CARTESIAN_POINT('Ctrl Pts',(0.00738358609753361,-0.0351970973651569,
0.0683266910436016));
#98348=CARTESIAN_POINT('Ctrl Pts',(0.00746426015076711,-0.035086934932687,
0.0683164366298886));
#98349=CARTESIAN_POINT('Ctrl Pts',(0.00754521421702457,-0.034976498513999,
0.0683078508903905));
#98350=CARTESIAN_POINT('Ctrl Pts',(0.00762634407270598,-0.0348659306865085,
0.0683009511219393));
#98351=CARTESIAN_POINT('Ctrl Pts',(0.00733594416277111,-0.0351970973651569,
0.0683937038535878));
#98352=CARTESIAN_POINT('Ctrl Pts',(0.00741568984434501,-0.035086934932687,
0.068382789425438));
#98353=CARTESIAN_POINT('Ctrl Pts',(0.00749572849122493,-0.034976498513999,
0.0683735238244226));
#98354=CARTESIAN_POINT('Ctrl Pts',(0.00757595711761141,-0.0348659306865085,
0.0683659251583419));
#98355=CARTESIAN_POINT('Ctrl Pts',(0.0072883022280086,-0.0351970973651569,
0.068460716663574));
#98356=CARTESIAN_POINT('Ctrl Pts',(0.00736711953792292,-0.0350869349326871,
0.0684491422209874));
#98357=CARTESIAN_POINT('Ctrl Pts',(0.00744624276542529,-0.0349764985139991,
0.0684391967584546));
#98358=CARTESIAN_POINT('Ctrl Pts',(0.00752557016251684,-0.0348659306865085,
0.0684308991947446));
#98359=CARTESIAN_POINT('Origin',(0.0088489351065516,-0.0345637187965151,
0.085130418031708));
#98360=CARTESIAN_POINT('Ctrl Pts',(0.00725485115071148,-0.0352450361861253,
0.068464660621954));
#98361=CARTESIAN_POINT('Ctrl Pts',(0.00746927723840594,-0.0349452761023765,
0.0684318883507653));
#98362=CARTESIAN_POINT('Ctrl Pts',(0.00768556270568411,-0.0346444289983475,
0.068415360632015));
#98363=CARTESIAN_POINT('Ctrl Pts',(0.00700860015368956,-0.0352450361861253,
0.0685077935150371));
#98364=CARTESIAN_POINT('Ctrl Pts',(0.00722139945766898,-0.0349452761023765,
0.0684657337353337));
#98365=CARTESIAN_POINT('Ctrl Pts',(0.0074367623358779,-0.0346444289983475,
0.0684398223568989));
#98366=CARTESIAN_POINT('Ctrl Pts',(0.00752519237820144,-0.0345231616327822,
0.0684313488481526));
#98367=CARTESIAN_POINT('Ctrl Pts',(0.00760401593311234,-0.0344132092796975,
0.0684230981303012));
#98368=CARTESIAN_POINT('Ctrl Pts',(0.00768300608068082,-0.0343032738558973,
0.0684164782412072));
#98369=CARTESIAN_POINT('Ctrl Pts',(0.00776206140815902,-0.034193496108874,
0.0684114950695524));
#98370=CARTESIAN_POINT('Ctrl Pts',(0.00743871126965919,-0.0345231616327822,
0.0683581221180348));
#98371=CARTESIAN_POINT('Ctrl Pts',(0.00751854415194977,-0.0344132092796975,
0.0683486793798578));
#98372=CARTESIAN_POINT('Ctrl Pts',(0.00759856823082146,-0.0343032738558973,
0.0683408884090816));
#98373=CARTESIAN_POINT('Ctrl Pts',(0.00767868073051039,-0.034193496108874,
0.0683347565607495));
#98374=CARTESIAN_POINT('Ctrl Pts',(0.00735223016111695,-0.0345231616327822,
0.068284895387917));
#98375=CARTESIAN_POINT('Ctrl Pts',(0.0074330723707872,-0.0344132092796975,
0.0682742606294144));
#98376=CARTESIAN_POINT('Ctrl Pts',(0.0075141303809621,-0.0343032738558973,
0.0682652985769561));
#98377=CARTESIAN_POINT('Ctrl Pts',(0.00759530005286176,-0.034193496108874,
0.0682580180519466));
#98378=CARTESIAN_POINT('Ctrl Pts',(0.00726574905257471,-0.0345231616327822,
0.0682116686577992));
#98379=CARTESIAN_POINT('Ctrl Pts',(0.00734760058962464,-0.0344132092796975,
0.068199841878971));
#98380=CARTESIAN_POINT('Ctrl Pts',(0.00742969253110274,-0.0343032738558973,
0.0681897087448306));
#98381=CARTESIAN_POINT('Ctrl Pts',(0.00751191937521313,-0.034193496108874,
0.0681812795431436));
#98382=CARTESIAN_POINT('Origin',(0.0093314165033207,-0.0345625596231041,
0.0851353053208476));
#98383=CARTESIAN_POINT('Ctrl Pts',(0.00786229561583597,-0.0346945769586885,
0.0681557006439514));
#98384=CARTESIAN_POINT('Ctrl Pts',(0.00794490009058703,-0.0345846629178475,
0.0681520972267567));
#98385=CARTESIAN_POINT('Ctrl Pts',(0.00802759319157298,-0.034474692505516,
0.0681502014206997));
#98386=CARTESIAN_POINT('Ctrl Pts',(0.00811026895283217,-0.0343648066260528,
0.068150015217323));
#98387=CARTESIAN_POINT('Ctrl Pts',(0.00779094408946165,-0.0346945769586885,
0.0682437351898163));
#98388=CARTESIAN_POINT('Ctrl Pts',(0.00787233540367648,-0.0345846629178475,
0.0682391485125258));
#98389=CARTESIAN_POINT('Ctrl Pts',(0.00795383547033033,-0.034474692505516,
0.0682362441907683));
#98390=CARTESIAN_POINT('Ctrl Pts',(0.0080353398467779,-0.0343648066260528,
0.0682350255146257));
#98391=CARTESIAN_POINT('Ctrl Pts',(0.00771959256308734,-0.0346945769586885,
0.0683317697356813));
#98392=CARTESIAN_POINT('Ctrl Pts',(0.00779977071676592,-0.0345846629178475,
0.068326199798295));
#98393=CARTESIAN_POINT('Ctrl Pts',(0.00788007774908768,-0.034474692505516,
0.0683222869608369));
#98394=CARTESIAN_POINT('Ctrl Pts',(0.00796041074072362,-0.0343648066260528,
0.0683200358119284));
#98395=CARTESIAN_POINT('Ctrl Pts',(0.00764824103671302,-0.0346945769586885,
0.0684198042815462));
#98396=CARTESIAN_POINT('Ctrl Pts',(0.00772720602985537,-0.0345846629178475,
0.0684132510840642));
#98397=CARTESIAN_POINT('Ctrl Pts',(0.00780632002784502,-0.034474692505516,
0.0684083297309054));
#98398=CARTESIAN_POINT('Ctrl Pts',(0.00788548163466935,-0.0343648066260528,
0.0684050461092312));
#98399=CARTESIAN_POINT('Origin',(0.00885356201123892,-0.0345626446730313,
0.085188665111889));
#98400=CARTESIAN_POINT('Ctrl Pts',(0.00764951775477944,-0.0346945769586885,
0.0684182290483187));
#98401=CARTESIAN_POINT('Ctrl Pts',(0.00776957199223636,-0.034527515336289,
0.0684082953897729));
#98402=CARTESIAN_POINT('Ctrl Pts',(0.00788996968628629,-0.0343603235965159,
0.0684021347571399));
#98403=CARTESIAN_POINT('Ctrl Pts',(0.00801035448319214,-0.034193496108874,
0.0683997600785163));
#98404=CARTESIAN_POINT('Ctrl Pts',(0.00756613991413675,-0.0346945769586885,
0.068426956248387));
#98405=CARTESIAN_POINT('Ctrl Pts',(0.00768601135689406,-0.034527515336289,
0.0684152762075863));
#98406=CARTESIAN_POINT('Ctrl Pts',(0.00780628113107879,-0.0343603235965159,
0.0684073629922694));
#98407=CARTESIAN_POINT('Ctrl Pts',(0.00792659318424578,-0.034193496108874,
0.0684032347195176));
#98408=CARTESIAN_POINT('Ctrl Pts',(0.00748276207349405,-0.0346945769586885,
0.0684356834484552));
#98409=CARTESIAN_POINT('Ctrl Pts',(0.00760245072155176,-0.034527515336289,
0.0684222570253997));
#98410=CARTESIAN_POINT('Ctrl Pts',(0.0077225925758713,-0.0343603235965159,
0.068412591227399));
#98411=CARTESIAN_POINT('Ctrl Pts',(0.00784283188529941,-0.034193496108874,
0.0684067093605189));
#98412=CARTESIAN_POINT('Ctrl Pts',(0.00739938423285136,-0.0346945769586885,
0.0684444106485235));
#98413=CARTESIAN_POINT('Ctrl Pts',(0.00751889008620946,-0.034527515336289,
0.0684292378432131));
#98414=CARTESIAN_POINT('Ctrl Pts',(0.00763890402066379,-0.0343603235965159,
0.0684178194625285));
#98415=CARTESIAN_POINT('Ctrl Pts',(0.00775907058635305,-0.034193496108874,
0.0684101840015202));
#98416=CARTESIAN_POINT('Ctrl Pts',(0.00788545013106071,-0.0340223579322365,
0.0684050479733614));
#98417=CARTESIAN_POINT('Ctrl Pts',(0.00796468800297119,-0.0339125849573554,
0.0684017607526297));
#98418=CARTESIAN_POINT('Ctrl Pts',(0.0080439382331772,-0.0338030433565221,
0.0684001158816151));
#98419=CARTESIAN_POINT('Ctrl Pts',(0.0081230992875253,-0.0336938721132327,
0.0684001064797843));
#98420=CARTESIAN_POINT('Ctrl Pts',(0.00780373746605553,-0.0340223579322365,
0.0683265354252684));
#98421=CARTESIAN_POINT('Ctrl Pts',(0.00788405823077352,-0.0339125849573554,
0.0683221211737707));
#98422=CARTESIAN_POINT('Ctrl Pts',(0.00796441391976881,-0.0338030433565221,
0.0683193724773064));
#98423=CARTESIAN_POINT('Ctrl Pts',(0.00804470146005949,-0.0336938721132327,
0.0683182837416307));
#98424=CARTESIAN_POINT('Ctrl Pts',(0.00772202480105035,-0.0340223579322365,
0.0682480228771754));
#98425=CARTESIAN_POINT('Ctrl Pts',(0.00780342845857586,-0.0339125849573554,
0.0682424815949117));
#98426=CARTESIAN_POINT('Ctrl Pts',(0.00788488960636042,-0.0338030433565221,
0.0682386290729977));
#98427=CARTESIAN_POINT('Ctrl Pts',(0.00796630363259369,-0.0336938721132327,
0.0682364610034771));
#98428=CARTESIAN_POINT('Ctrl Pts',(0.00764031213604517,-0.0340223579322365,
0.0681695103290823));
#98429=CARTESIAN_POINT('Ctrl Pts',(0.0077227986863782,-0.0339125849573554,
0.0681628420160527));
#98430=CARTESIAN_POINT('Ctrl Pts',(0.00780536529295203,-0.0338030433565221,
0.068157885668689));
#98431=CARTESIAN_POINT('Ctrl Pts',(0.00788790580512789,-0.0336938721132327,
0.0681546382653236));
#98432=CARTESIAN_POINT('Origin',(0.00932085993867162,-0.0345589643415153,
0.0850155495813615));
#98433=CARTESIAN_POINT('Ctrl Pts',(0.0082391967706457,-0.034193496108874,
0.0681511101464263));
#98434=CARTESIAN_POINT('Ctrl Pts',(0.00832191790932497,-0.0340836138581106,
0.0681527016451047));
#98435=CARTESIAN_POINT('Ctrl Pts',(0.00840456642412107,-0.0339738896643499,
0.0681560041205447));
#98436=CARTESIAN_POINT('Ctrl Pts',(0.00848703681848185,-0.0338644633294062,
0.0681610062550407));
#98437=CARTESIAN_POINT('Ctrl Pts',(0.00816245819279496,-0.034193496108874,
0.0682344908990992));
#98438=CARTESIAN_POINT('Ctrl Pts',(0.008244029560271,-0.0340836138581106,
0.0682350242182319));
#98439=CARTESIAN_POINT('Ctrl Pts',(0.00832555075235104,-0.0339738896643499,
0.068237245229758));
#98440=CARTESIAN_POINT('Ctrl Pts',(0.00840691762253109,-0.0338644633294062,
0.0682411440968326));
#98441=CARTESIAN_POINT('Ctrl Pts',(0.00808571961494423,-0.034193496108874,
0.0683178716517722));
#98442=CARTESIAN_POINT('Ctrl Pts',(0.00816614121121704,-0.0340836138581106,
0.068317346791359));
#98443=CARTESIAN_POINT('Ctrl Pts',(0.00824653508058101,-0.0339738896643499,
0.0683184863389713));
#98444=CARTESIAN_POINT('Ctrl Pts',(0.00832679842658033,-0.0338644633294062,
0.0683212819386244));
#98445=CARTESIAN_POINT('Ctrl Pts',(0.0080089810370935,-0.034193496108874,
0.0684012524044451));
#98446=CARTESIAN_POINT('Ctrl Pts',(0.00808825286216307,-0.0340836138581106,
0.0683996693644862));
#98447=CARTESIAN_POINT('Ctrl Pts',(0.00816751940881098,-0.0339738896643499,
0.0683997274481846));
#98448=CARTESIAN_POINT('Ctrl Pts',(0.00824667923062957,-0.0338644633294062,
0.0684014197804163));
#98449=CARTESIAN_POINT('Origin',(0.00884973524919201,-0.0345610621862526,
0.0851134859820757));
#98450=CARTESIAN_POINT('Ctrl Pts',(0.0079741864245549,-0.03424362768739,
0.0684005873251233));
#98451=CARTESIAN_POINT('Ctrl Pts',(0.00819102909828033,-0.033943005420186,
0.0683949452277013));
#98452=CARTESIAN_POINT('Ctrl Pts',(0.00840768073059799,-0.0336441434784162,
0.0684056526375564));
#98453=CARTESIAN_POINT('Ctrl Pts',(0.00772447136808276,-0.03424362768739,
0.0684125200771577));
#98454=CARTESIAN_POINT('Ctrl Pts',(0.00794086399064604,-0.033943005420186,
0.0683974598211207));
#98455=CARTESIAN_POINT('Ctrl Pts',(0.00815777626464629,-0.0336441434784162,
0.0683987419286646));
#98456=CARTESIAN_POINT('Ctrl Pts',(0.0082466515031986,-0.0335235895815127,
0.068401419314291));
#98457=CARTESIAN_POINT('Ctrl Pts',(0.00832579203425014,-0.0334144449262719,
0.0684031108522518));
#98458=CARTESIAN_POINT('Ctrl Pts',(0.00840498854228248,-0.0333049234473133,
0.0684064393173964));
#98459=CARTESIAN_POINT('Ctrl Pts',(0.00848413937374187,-0.0331951640388588,
0.068411409626935));
#98460=CARTESIAN_POINT('Ctrl Pts',(0.00817002998314079,-0.0335235895815127,
0.0683179309010212));
#98461=CARTESIAN_POINT('Ctrl Pts',(0.00825031989657454,-0.0334144449262719,
0.0683185675929045));
#98462=CARTESIAN_POINT('Ctrl Pts',(0.00833068889981629,-0.0333049234473133,
0.0683208637454563));
#98463=CARTESIAN_POINT('Ctrl Pts',(0.00841103395962319,-0.0331951640388588,
0.0683248257317072));
#98464=CARTESIAN_POINT('Ctrl Pts',(0.00809340846308299,-0.0335235895815127,
0.0682344424877513));
#98465=CARTESIAN_POINT('Ctrl Pts',(0.00817484775889894,-0.0334144449262719,
0.0682340243335572));
#98466=CARTESIAN_POINT('Ctrl Pts',(0.00825638925735009,-0.0333049234473133,
0.0682352881735162));
#98467=CARTESIAN_POINT('Ctrl Pts',(0.00833792854550451,-0.0331951640388588,
0.0682382418364794));
#98468=CARTESIAN_POINT('Ctrl Pts',(0.00801678694302518,-0.0335235895815127,
0.0681509540744815));
#98469=CARTESIAN_POINT('Ctrl Pts',(0.00809937562122333,-0.0334144449262719,
0.0681494810742099));
#98470=CARTESIAN_POINT('Ctrl Pts',(0.0081820896148839,-0.0333049234473133,
0.068149712601576));
#98471=CARTESIAN_POINT('Ctrl Pts',(0.00826482313138583,-0.0331951640388588,
0.0681516579412516));
#98472=CARTESIAN_POINT('Origin',(0.00668102421589752,-0.03264345717686,
0.0849806466885375));
#98473=CARTESIAN_POINT('Ctrl Pts',(0.00861710645831259,-0.0336938721132347,
0.0681687917856074));
#98474=CARTESIAN_POINT('Ctrl Pts',(0.00865211645476513,-0.0336474569764937,
0.0681716793762339));
#98475=CARTESIAN_POINT('Ctrl Pts',(0.00868709024941617,-0.033601104548885,
0.0681749766052127));
#98476=CARTESIAN_POINT('Ctrl Pts',(0.0087756358526874,-0.0334837508643148,
0.0681833244305479));
#98477=CARTESIAN_POINT('Ctrl Pts',(0.00886389520989677,-0.033366026476038,
0.0681942923798312));
#98478=CARTESIAN_POINT('Ctrl Pts',(0.00837163885895429,-0.0336938721132347,
0.0684039846786493));
#98479=CARTESIAN_POINT('Ctrl Pts',(0.00840527219335863,-0.0336474569764937,
0.068405435465962));
#98480=CARTESIAN_POINT('Ctrl Pts',(0.00843888623988815,-0.033601104548885,
0.0684072798745103));
#98481=CARTESIAN_POINT('Ctrl Pts',(0.00852398927368931,-0.0334837508643148,
0.0684119494926978));
#98482=CARTESIAN_POINT('Ctrl Pts',(0.00860891656605055,-0.033366026476038,
0.0684191388395642));
#98483=CARTESIAN_POINT('Ctrl Pts',(0.00837163885896573,-0.0336938721132426,
0.0684039846786594));
#98484=CARTESIAN_POINT('Ctrl Pts',(0.00840527219336936,-0.0336474569765026,
0.0684054354659721));
#98485=CARTESIAN_POINT('Ctrl Pts',(0.00843888623989815,-0.0336011045488949,
0.0684072798745204));
#98486=CARTESIAN_POINT('Ctrl Pts',(0.00852328048134079,-0.0334847282606778,
0.0684119106011486));
#98487=CARTESIAN_POINT('Ctrl Pts',(0.00860750220198468,-0.0333679869945434,
0.0684190192852437));
#98488=CARTESIAN_POINT('Ctrl Pts',(0.00837163885894863,-0.0336938721132425,
0.068403984678649));
#98489=CARTESIAN_POINT('Ctrl Pts',(0.0084919265470148,-0.0335278710435082,
0.0684091733361166));
#98490=CARTESIAN_POINT('Ctrl Pts',(0.00861200920320254,-0.0333620469224319,
0.0684181323588499));
#98491=CARTESIAN_POINT('Ctrl Pts',(0.00873194505769313,-0.0331951640388602,
0.068430886176151));
#98492=CARTESIAN_POINT('Ctrl Pts',(0.00828782466038203,-0.0336938721132425,
0.0684021930475727));
#98493=CARTESIAN_POINT('Ctrl Pts',(0.00840814985464127,-0.0335278710435082,
0.068405627129807));
#98494=CARTESIAN_POINT('Ctrl Pts',(0.00852832502685063,-0.0333620469224319,
0.068412833370747));
#98495=CARTESIAN_POINT('Ctrl Pts',(0.00864840874474797,-0.0331951640388602,
0.0684238353433773));
#98496=CARTESIAN_POINT('Ctrl Pts',(0.00820401046181543,-0.0336938721132425,
0.0684004014164963));
#98497=CARTESIAN_POINT('Ctrl Pts',(0.00832437316226774,-0.0335278710435082,
0.0684020809234974));
#98498=CARTESIAN_POINT('Ctrl Pts',(0.00844464085049871,-0.0333620469224319,
0.0684075343826441));
#98499=CARTESIAN_POINT('Ctrl Pts',(0.0085648724318028,-0.0331951640388602,
0.0684167845106035));
#98500=CARTESIAN_POINT('Ctrl Pts',(0.00812019626324883,-0.0336938721132425,
0.0683986097854199));
#98501=CARTESIAN_POINT('Ctrl Pts',(0.00824059646989421,-0.0335278710435082,
0.0683985347171878));
#98502=CARTESIAN_POINT('Ctrl Pts',(0.0083609566741468,-0.0333620469224319,
0.0684022353945412));
#98503=CARTESIAN_POINT('Ctrl Pts',(0.00848133611885764,-0.0331951640388602,
0.0684097336778298));
#98504=CARTESIAN_POINT('Ctrl Pts',(0.00860736419504573,-0.0330240426238155,
0.0684204773996999));
#98505=CARTESIAN_POINT('Ctrl Pts',(0.00868629395086783,-0.0329142774063509,
0.0684271392129077));
#98506=CARTESIAN_POINT('Ctrl Pts',(0.00876512533776395,-0.0328043479726686,
0.0684354360458046));
#98507=CARTESIAN_POINT('Ctrl Pts',(0.00884375707413942,-0.0326943950436594,
0.0684453600507454));
#98508=CARTESIAN_POINT('Ctrl Pts',(0.00853613623801668,-0.0330240426238155,
0.0683323427633641));
#98509=CARTESIAN_POINT('Ctrl Pts',(0.00861628013431971,-0.0329142774063509,
0.0683380233420697));
#98510=CARTESIAN_POINT('Ctrl Pts',(0.00869634655184818,-0.0328043479726686,
0.0683453635509586));
#98511=CARTESIAN_POINT('Ctrl Pts',(0.00877623266059143,-0.0326943950436594,
0.0683543568114647));
#98512=CARTESIAN_POINT('Ctrl Pts',(0.00846490828098764,-0.0330240426238155,
0.0682442081270282));
#98513=CARTESIAN_POINT('Ctrl Pts',(0.00854626631777161,-0.0329142774063509,
0.0682489074712318));
#98514=CARTESIAN_POINT('Ctrl Pts',(0.00862756776593242,-0.0328043479726686,
0.0682552910561126));
#98515=CARTESIAN_POINT('Ctrl Pts',(0.00870870824704343,-0.0326943950436594,
0.068263353572184));
#98516=CARTESIAN_POINT('Ctrl Pts',(0.00839368032395859,-0.0330240426238155,
0.0681560734906924));
#98517=CARTESIAN_POINT('Ctrl Pts',(0.00847625250122349,-0.0329142774063509,
0.0681597916003938));
#98518=CARTESIAN_POINT('Ctrl Pts',(0.00855878898001665,-0.0328043479726686,
0.0681652185612667));
#98519=CARTESIAN_POINT('Ctrl Pts',(0.00864118383349544,-0.0326943950436594,
0.0681723503329033));
#98520=CARTESIAN_POINT('Origin',(0.00666743703714251,-0.0326396682858257,
0.0851035726301499));
#98521=CARTESIAN_POINT('Ctrl Pts',(0.00899014695537431,-0.0331951640388587,
0.0682128784669059));
#98522=CARTESIAN_POINT('Ctrl Pts',(0.00907191879379361,-0.0330855618255041,
0.0682248108888645));
#98523=CARTESIAN_POINT('Ctrl Pts',(0.00915350295762293,-0.0329757224427708,
0.0682384419968624));
#98524=CARTESIAN_POINT('Ctrl Pts',(0.00923479411721618,-0.0328657862078596,
0.0682537594600869));
#98525=CARTESIAN_POINT('Ctrl Pts',(0.00890356312907921,-0.0331951640388587,
0.0682859838228226));
#98526=CARTESIAN_POINT('Ctrl Pts',(0.00898432808911168,-0.0330855618255041,
0.0682967237277317));
#98527=CARTESIAN_POINT('Ctrl Pts',(0.00906492929599861,-0.0329757224427708,
0.0683091406485559));
#98528=CARTESIAN_POINT('Ctrl Pts',(0.0091452627550974,-0.0328657862078596,
0.0683232237475788));
#98529=CARTESIAN_POINT('Ctrl Pts',(0.0088169793027841,-0.0331951640388587,
0.0683590891787393));
#98530=CARTESIAN_POINT('Ctrl Pts',(0.00889673738442976,-0.0330855618255041,
0.0683686365665988));
#98531=CARTESIAN_POINT('Ctrl Pts',(0.0089763556343743,-0.0329757224427708,
0.0683798393002495));
#98532=CARTESIAN_POINT('Ctrl Pts',(0.00905573139297862,-0.0328657862078596,
0.0683926880350707));
#98533=CARTESIAN_POINT('Ctrl Pts',(0.008730395476489,-0.0331951640388587,
0.068432194534656));
#98534=CARTESIAN_POINT('Ctrl Pts',(0.00880914667974784,-0.0330855618255041,
0.0684405494054659));
#98535=CARTESIAN_POINT('Ctrl Pts',(0.00888778197274998,-0.0329757224427708,
0.0684505379519431));
#98536=CARTESIAN_POINT('Ctrl Pts',(0.00896620003085984,-0.0328657862078596,
0.0684621523225627));
#98537=CARTESIAN_POINT('Origin',(0.00619733850441799,-0.0326401908834255,
0.0850021811058405));
#98538=CARTESIAN_POINT('Ctrl Pts',(0.00869603062313004,-0.0332451089994432,
0.0684271810500122));
#98539=CARTESIAN_POINT('Ctrl Pts',(0.00891187027115007,-0.0329451141710258,
0.068448763752662));
#98540=CARTESIAN_POINT('Ctrl Pts',(0.00912547104411551,-0.0326442513127503,
0.0684865430657797));
#98541=CARTESIAN_POINT('Ctrl Pts',(0.00844678931927606,-0.0332451089994432,
0.0684077189727038));
#98542=CARTESIAN_POINT('Ctrl Pts',(0.00866336299155103,-0.0329451141710258,
0.0684199013857819));
#98543=CARTESIAN_POINT('Ctrl Pts',(0.00887840377172522,-0.0326442513127503,
0.0684483624042661));
#98544=CARTESIAN_POINT('Ctrl Pts',(0.00896616879731833,-0.0325229783203384,
0.0684621476059621));
#98545=CARTESIAN_POINT('Ctrl Pts',(0.00904457571675786,-0.0324130253112079,
0.068473759886668));
#98546=CARTESIAN_POINT('Ctrl Pts',(0.00912273052931295,-0.0323031222247694,
0.0684869923539639));
#98547=CARTESIAN_POINT('Ctrl Pts',(0.00920053372233297,-0.0321934096636184,
0.0685018245254217));
#98548=CARTESIAN_POINT('Ctrl Pts',(0.00890061538018178,-0.0325229783203384,
0.0683697144292825));
#98549=CARTESIAN_POINT('Ctrl Pts',(0.00898029648891727,-0.0324130253112079,
0.0683804230575832));
#98550=CARTESIAN_POINT('Ctrl Pts',(0.00905974399072303,-0.0323031222247694,
0.0683927783677724));
#98551=CARTESIAN_POINT('Ctrl Pts',(0.00913885667745818,-0.0321934096636184,
0.0684067609425686));
#98552=CARTESIAN_POINT('Ctrl Pts',(0.00883506196304524,-0.0325229783203384,
0.0682772812526029));
#98553=CARTESIAN_POINT('Ctrl Pts',(0.00891601726107668,-0.0324130253112079,
0.0682870862284984));
#98554=CARTESIAN_POINT('Ctrl Pts',(0.00899675745213311,-0.0323031222247694,
0.0682985643815809));
#98555=CARTESIAN_POINT('Ctrl Pts',(0.00907717963258339,-0.0321934096636184,
0.0683116973597155));
#98556=CARTESIAN_POINT('Ctrl Pts',(0.00876950854590869,-0.0325229783203384,
0.0681848480759233));
#98557=CARTESIAN_POINT('Ctrl Pts',(0.00885173803323609,-0.0324130253112079,
0.0681937493994136));
#98558=CARTESIAN_POINT('Ctrl Pts',(0.0089337709135432,-0.0323031222247694,
0.0682043503953893));
#98559=CARTESIAN_POINT('Ctrl Pts',(0.0090155025877086,-0.0321934096636184,
0.0682166337768624));
#98560=CARTESIAN_POINT('Origin',(0.00666879662080091,-0.0326393375178324,
0.0850951558291911));
#98561=CARTESIAN_POINT('Ctrl Pts',(0.00936123232799051,-0.0326943950436594,
0.0682789935135691));
#98562=CARTESIAN_POINT('Ctrl Pts',(0.00944214580081217,-0.0325844576448127,
0.0682960478956564));
#98563=CARTESIAN_POINT('Ctrl Pts',(0.0095227122874234,-0.0324744968375319,
0.0683147769079863));
#98564=CARTESIAN_POINT('Ctrl Pts',(0.00960282889232979,-0.0323646534831894,
0.0683351551300524));
#98565=CARTESIAN_POINT('Ctrl Pts',(0.00927022911848484,-0.0326943950436594,
0.0683465179050241));
#98566=CARTESIAN_POINT('Ctrl Pts',(0.00935021197863805,-0.0325844576448127,
0.0683623180923262));
#98567=CARTESIAN_POINT('Ctrl Pts',(0.00942987372552438,-0.0324744968375319,
0.0683797735745138));
#98568=CARTESIAN_POINT('Ctrl Pts',(0.00950911260034835,-0.0323646534831894,
0.0683988605787906));
#98569=CARTESIAN_POINT('Ctrl Pts',(0.00917922590897917,-0.0326943950436594,
0.0684140422964789));
#98570=CARTESIAN_POINT('Ctrl Pts',(0.00925827815646394,-0.0325844576448127,
0.0684285882889959));
#98571=CARTESIAN_POINT('Ctrl Pts',(0.00933703516362535,-0.0324744968375319,
0.0684447702410413));
#98572=CARTESIAN_POINT('Ctrl Pts',(0.0094153963083669,-0.0323646534831894,
0.0684625660275288));
#98573=CARTESIAN_POINT('Ctrl Pts',(0.00908822269947349,-0.0326943950436594,
0.0684815666879339));
#98574=CARTESIAN_POINT('Ctrl Pts',(0.00916634433428982,-0.0325844576448127,
0.0684948584856657));
#98575=CARTESIAN_POINT('Ctrl Pts',(0.00924419660172632,-0.0324744968375319,
0.0685097669075688));
#98576=CARTESIAN_POINT('Ctrl Pts',(0.00932168001638546,-0.0323646534831894,
0.0685262714762671));
#98577=CARTESIAN_POINT('Origin',(0.0061911757942771,-0.0326395579067402,
0.0850395171850295));
#98578=CARTESIAN_POINT('Ctrl Pts',(0.0090542014899579,-0.0327445246961877,
0.0684743991567367));
#98579=CARTESIAN_POINT('Ctrl Pts',(0.00926826027291881,-0.0324436878365475,
0.0685094904938175));
#98580=CARTESIAN_POINT('Ctrl Pts',(0.00947906771459618,-0.0321434074463187,
0.0685606059223521));
#98581=CARTESIAN_POINT('Ctrl Pts',(0.00880667380163768,-0.0327445246961877,
0.0684393271805328));
#98582=CARTESIAN_POINT('Ctrl Pts',(0.00902205534579157,-0.0324436878365475,
0.0684650828583286));
#98583=CARTESIAN_POINT('Ctrl Pts',(0.0092348849908425,-0.0321434074463187,
0.0685069887849776));
#98584=CARTESIAN_POINT('Ctrl Pts',(0.00941419039007019,-0.0322357242816072,
0.0685452723808186));
#98585=CARTESIAN_POINT('Ctrl Pts',(0.0095926936956757,-0.0319819883628706,
0.0685863702082937));
#98586=CARTESIAN_POINT('Ctrl Pts',(0.00976822006984993,-0.0317295851069886,
0.0686387434219101));
#98587=CARTESIAN_POINT('Ctrl Pts',(0.00916940259726973,-0.0322357242816072,
0.0684944891503594));
#98588=CARTESIAN_POINT('Ctrl Pts',(0.00934952328290193,-0.0319819883628706,
0.0685277908041121));
#98589=CARTESIAN_POINT('Ctrl Pts',(0.00952715985211837,-0.0317295851069886,
0.0685724865624373));
#98590=CARTESIAN_POINT('Origin',(0.00620950443384443,-0.032637194264687,
0.0849459946505887));
#98591=CARTESIAN_POINT('Origin',(0.00668785385502022,-0.0326352985529741,
0.0849739096964743));
#98592=CARTESIAN_POINT('Ctrl Pts',(0.00972743405026177,-0.0321934096636183,
0.0683682787406266));
#98593=CARTESIAN_POINT('Ctrl Pts',(0.00980716849242794,-0.0320835708272304,
0.0683903943495469));
#98594=CARTESIAN_POINT('Ctrl Pts',(0.00988639900400012,-0.0319739230346346,
0.0684141472306517));
#98595=CARTESIAN_POINT('Ctrl Pts',(0.00996502654739581,-0.0318646057455575,
0.0684394992139177));
#98596=CARTESIAN_POINT('Ctrl Pts',(0.00963237038554758,-0.0321934096636183,
0.0684299558386126));
#98597=CARTESIAN_POINT('Ctrl Pts',(0.00971125425246431,-0.0320835708272304,
0.0684507604455085));
#98598=CARTESIAN_POINT('Ctrl Pts',(0.00978966181327403,-0.0319739230346346,
0.0684731854824126));
#98599=CARTESIAN_POINT('Ctrl Pts',(0.009867494952918,-0.0318646057455575,
0.0684971945589941));
#98600=CARTESIAN_POINT('Ctrl Pts',(0.00953730672083339,-0.0321934096636183,
0.0684916329365987));
#98601=CARTESIAN_POINT('Ctrl Pts',(0.00961534001250069,-0.0320835708272304,
0.06851112654147));
#98602=CARTESIAN_POINT('Ctrl Pts',(0.00969292462254795,-0.0319739230346346,
0.0685322237341735));
#98603=CARTESIAN_POINT('Ctrl Pts',(0.00976996335844018,-0.0318646057455575,
0.0685548899040705));
#98604=CARTESIAN_POINT('Ctrl Pts',(0.0094422430561192,-0.0321934096636183,
0.0685533100345848));
#98605=CARTESIAN_POINT('Ctrl Pts',(0.00951942577253707,-0.0320835708272304,
0.0685714926374316));
#98606=CARTESIAN_POINT('Ctrl Pts',(0.00959618743182186,-0.0319739230346346,
0.0685912619859344));
#98607=CARTESIAN_POINT('Ctrl Pts',(0.00967243176396236,-0.0318646057455575,
0.068612585249147));
#98608=CARTESIAN_POINT('Ctrl Pts',(0.00932139294781656,-0.0320218834582328,
0.0685253643424135));
#98609=CARTESIAN_POINT('Ctrl Pts',(0.00937993180754131,-0.0319391099350642,
0.0685378285751643));
#98610=CARTESIAN_POINT('Ctrl Pts',(0.00943824056931616,-0.031856486945494,
0.0685511993486559));
#98611=CARTESIAN_POINT('Ctrl Pts',(0.00949627767213026,-0.031774074144655,
0.0685654629591656));
#98612=CARTESIAN_POINT('Ctrl Pts',(0.00929531728817879,-0.0320218834582328,
0.068483211192807));
#98613=CARTESIAN_POINT('Ctrl Pts',(0.00935429486028635,-0.0319391099350642,
0.0684954040409785));
#98614=CARTESIAN_POINT('Ctrl Pts',(0.00941304630634758,-0.031856486945494,
0.0685085104448712));
#98615=CARTESIAN_POINT('Ctrl Pts',(0.0094715297249382,-0.031774074144655,
0.0685225168632189));
#98616=CARTESIAN_POINT('Ctrl Pts',(0.00926924162854101,-0.0320218834582328,
0.0684410580432006));
#98617=CARTESIAN_POINT('Ctrl Pts',(0.00932865791303139,-0.0319391099350642,
0.0684529795067928));
#98618=CARTESIAN_POINT('Ctrl Pts',(0.009387852043379,-0.031856486945494,
0.0684658215410865));
#98619=CARTESIAN_POINT('Ctrl Pts',(0.00944678177774615,-0.031774074144655,
0.0684795707672721));
#98620=CARTESIAN_POINT('Ctrl Pts',(0.00924316596890324,-0.0320218834582328,
0.0683989048935941));
#98621=CARTESIAN_POINT('Ctrl Pts',(0.00930302096577642,-0.0319391099350642,
0.068410554972607));
#98622=CARTESIAN_POINT('Ctrl Pts',(0.00936265778041042,-0.031856486945494,
0.0684231326373018));
#98623=CARTESIAN_POINT('Ctrl Pts',(0.0094220338305541,-0.031774074144655,
0.0684366246713254));
#98624=CARTESIAN_POINT('Origin',(0.00971022807106882,-0.0391228853390632,
0.0621765373510591));
#98625=CARTESIAN_POINT('Ctrl Pts',(0.00629088080421439,-0.0352722978779559,
0.0686979694570567));
#98626=CARTESIAN_POINT('Ctrl Pts',(0.00630890107951828,-0.0352466642097193,
0.0686922806649198));
#98627=CARTESIAN_POINT('Ctrl Pts',(0.00632688169870236,-0.035221018380829,
0.0686865221768446));
#98628=CARTESIAN_POINT('Ctrl Pts',(0.00634482313386381,-0.0351953608940152,
0.0686806932824731));
#98629=CARTESIAN_POINT('Origin',(0.00498953171674852,-0.0352456003065034,
0.0639739633449897));
#98630=CARTESIAN_POINT('Ctrl Pts',(0.00646422762586219,-0.0350241211493339,
0.0686448061997158));
#98631=CARTESIAN_POINT('Ctrl Pts',(0.00654005940982445,-0.0349144232867421,
0.0686219465170266));
#98632=CARTESIAN_POINT('Ctrl Pts',(0.00661640910871704,-0.0348045283677512,
0.0686006406488063));
#98633=CARTESIAN_POINT('Ctrl Pts',(0.00669317994381437,-0.0346945769586886,
0.0685809195243136));
#98634=CARTESIAN_POINT('Ctrl Pts',(0.00636555700172017,-0.0350241211493339,
0.0685890814320229));
#98635=CARTESIAN_POINT('Ctrl Pts',(0.00644215637147474,-0.0349144232867421,
0.068564862602004));
#98636=CARTESIAN_POINT('Ctrl Pts',(0.00651930221014196,-0.0348045283677512,
0.0685422126394849));
#98637=CARTESIAN_POINT('Ctrl Pts',(0.00659689678330767,-0.0346945769586886,
0.0685211642332857));
#98638=CARTESIAN_POINT('Ctrl Pts',(0.00626688637757816,-0.0350241211493339,
0.06853335666433));
#98639=CARTESIAN_POINT('Ctrl Pts',(0.00634425333312504,-0.0349144232867421,
0.0685077786869814));
#98640=CARTESIAN_POINT('Ctrl Pts',(0.00642219531156688,-0.0348045283677512,
0.0684837846301635));
#98641=CARTESIAN_POINT('Ctrl Pts',(0.00650061362280097,-0.0346945769586886,
0.0684614089422577));
#98642=CARTESIAN_POINT('Ctrl Pts',(0.00616821575343614,-0.0350241211493339,
0.0684776318966372));
#98643=CARTESIAN_POINT('Ctrl Pts',(0.00624635029477534,-0.0349144232867421,
0.0684506947719588));
#98644=CARTESIAN_POINT('Ctrl Pts',(0.0063250884129918,-0.0348045283677512,
0.0684253566208421));
#98645=CARTESIAN_POINT('Ctrl Pts',(0.00640433046229427,-0.0346945769586886,
0.0684016536512297));
#98646=CARTESIAN_POINT('Origin',(0.0106956549522073,-0.0345629067943476,
0.0848856164820718));
#98647=CARTESIAN_POINT('Ctrl Pts',(0.0066984359549881,-0.035197097365166,
0.0683929252324924));
#98648=CARTESIAN_POINT('Ctrl Pts',(0.00677819242367436,-0.0350869349321818,
0.0683731789920494));
#98649=CARTESIAN_POINT('Ctrl Pts',(0.00685842547508718,-0.0349764985129769,
0.0683550744868359));
#98650=CARTESIAN_POINT('Ctrl Pts',(0.00693903254564575,-0.034865930684969,
0.0683386412905385));
#98651=CARTESIAN_POINT('Ctrl Pts',(0.00665956862327684,-0.035197097365166,
0.0684653807441935));
#98652=CARTESIAN_POINT('Ctrl Pts',(0.00673832131904309,-0.0350869349321818,
0.0684450960495441));
#98653=CARTESIAN_POINT('Ctrl Pts',(0.00681756096018664,-0.0349764985129769,
0.0684264317761925));
#98654=CARTESIAN_POINT('Ctrl Pts',(0.00689718631280816,-0.034865930684969,
0.0684094181472611));
#98655=CARTESIAN_POINT('Ctrl Pts',(0.00662070129156558,-0.035197097365166,
0.0685378362558945));
#98656=CARTESIAN_POINT('Ctrl Pts',(0.00669845021441181,-0.0350869349321818,
0.0685170131070389));
#98657=CARTESIAN_POINT('Ctrl Pts',(0.0067766964452861,-0.0349764985129769,
0.068497789065549));
#98658=CARTESIAN_POINT('Ctrl Pts',(0.00685534007997056,-0.034865930684969,
0.0684801950039836));
#98659=CARTESIAN_POINT('Ctrl Pts',(0.00658183395985432,-0.035197097365166,
0.0686102917675956));
#98660=CARTESIAN_POINT('Ctrl Pts',(0.00665857910978054,-0.0350869349321818,
0.0685889301645337));
#98661=CARTESIAN_POINT('Ctrl Pts',(0.00673583193038556,-0.0349764985129769,
0.0685691463549055));
#98662=CARTESIAN_POINT('Ctrl Pts',(0.00681349384713296,-0.034865930684969,
0.0685509718607061));
#98663=CARTESIAN_POINT('Origin',(0.0102194283572242,-0.0345637187966277,
0.0849529483964491));
#98664=CARTESIAN_POINT('Ctrl Pts',(0.00654914096335699,-0.0352450361861253,
0.0686183971583664));
#98665=CARTESIAN_POINT('Ctrl Pts',(0.00675776878258464,-0.0349452761023765,
0.0685590085913934));
#98666=CARTESIAN_POINT('Ctrl Pts',(0.00697027730191754,-0.0346444289983475,
0.0685155034416551));
#98667=CARTESIAN_POINT('Ctrl Pts',(0.00631023771396125,-0.0352450361861253,
0.0686920533694295));
#98668=CARTESIAN_POINT('Ctrl Pts',(0.00651608754367545,-0.0349452761023765,
0.0686236544187838));
#98669=CARTESIAN_POINT('Ctrl Pts',(0.00672650466441856,-0.0346444289983475,
0.0685709552333918));
#98670=CARTESIAN_POINT('Ctrl Pts',(0.00681317539719488,-0.0345231616327822,
0.0685514653176442));
#98671=CARTESIAN_POINT('Ctrl Pts',(0.00689034331568431,-0.0344132092796975,
0.0685334004481495));
#98672=CARTESIAN_POINT('Ctrl Pts',(0.00696788091024001,-0.0343032738558974,
0.0685169326682436));
#98673=CARTESIAN_POINT('Ctrl Pts',(0.00704568830583149,-0.0341934961088741,
0.0685020805305624));
#98674=CARTESIAN_POINT('Ctrl Pts',(0.00671819847515509,-0.0345231616327822,
0.068489654959141));
#98675=CARTESIAN_POINT('Ctrl Pts',(0.00679621836241447,-0.0344132092796975,
0.0684702809664927));
#98676=CARTESIAN_POINT('Ctrl Pts',(0.00687463495996224,-0.0343032738558974,
0.0684525217532801));
#98677=CARTESIAN_POINT('Ctrl Pts',(0.0069533472242835,-0.0341934961088741,
0.0684363974977686));
#98678=CARTESIAN_POINT('Ctrl Pts',(0.00662322155311531,-0.0345231616327822,
0.0684278446006377));
#98679=CARTESIAN_POINT('Ctrl Pts',(0.00670209340914463,-0.0344132092796975,
0.0684071614848359));
#98680=CARTESIAN_POINT('Ctrl Pts',(0.00678138900968448,-0.0343032738558974,
0.0683881108383165));
#98681=CARTESIAN_POINT('Ctrl Pts',(0.00686100614273552,-0.0341934961088741,
0.0683707144649747));
#98682=CARTESIAN_POINT('Ctrl Pts',(0.00652824463107553,-0.0345231616327822,
0.0683660342421344));
#98683=CARTESIAN_POINT('Ctrl Pts',(0.00660796845587478,-0.0344132092796975,
0.0683440420031791));
#98684=CARTESIAN_POINT('Ctrl Pts',(0.0066881430594067,-0.0343032738558974,
0.068323699923353));
#98685=CARTESIAN_POINT('Ctrl Pts',(0.00676866506118753,-0.0341934961088741,
0.0683050314321808));
#98686=CARTESIAN_POINT('Origin',(0.0106987177838239,-0.034562559623147,
0.0848973261947764));
#98687=CARTESIAN_POINT('Ctrl Pts',(0.00711307259435406,-0.0346945769586886,
0.0682357404430474));
#98688=CARTESIAN_POINT('Ctrl Pts',(0.00719457408035251,-0.034584662917669,
0.0682218123539234));
#98689=CARTESIAN_POINT('Ctrl Pts',(0.00727637751416807,-0.0344746925051587,
0.0682095673031063));
#98690=CARTESIAN_POINT('Ctrl Pts',(0.00735837801501828,-0.0343648066255171,
0.0681990205474912));
#98691=CARTESIAN_POINT('Ctrl Pts',(0.00705331735037547,-0.0346945769586886,
0.0683320235277438));
#98692=CARTESIAN_POINT('Ctrl Pts',(0.00713349200680147,-0.034584662917669,
0.0683172719811551));
#98693=CARTESIAN_POINT('Ctrl Pts',(0.00721398541318103,-0.0344746925051587,
0.0683041758939341));
#98694=CARTESIAN_POINT('Ctrl Pts',(0.00729469436278638,-0.0343648066255171,
0.068292751620354));
#98695=CARTESIAN_POINT('Ctrl Pts',(0.00699356210639688,-0.0346945769586886,
0.0684283066124402));
#98696=CARTESIAN_POINT('Ctrl Pts',(0.00707240993325044,-0.034584662917669,
0.0684127316083868));
#98697=CARTESIAN_POINT('Ctrl Pts',(0.00715159331219398,-0.0344746925051587,
0.0683987844847619));
#98698=CARTESIAN_POINT('Ctrl Pts',(0.00723101071055449,-0.0343648066255171,
0.0683864826932167));
#98699=CARTESIAN_POINT('Ctrl Pts',(0.00693380686241829,-0.0346945769586886,
0.0685245896971366));
#98700=CARTESIAN_POINT('Ctrl Pts',(0.0070113278596994,-0.034584662917669,
0.0685081912356185));
#98701=CARTESIAN_POINT('Ctrl Pts',(0.00708920121120694,-0.0344746925051587,
0.0684933930755897));
#98702=CARTESIAN_POINT('Ctrl Pts',(0.00716732705832259,-0.0343648066255171,
0.0684802137660795));
#98703=CARTESIAN_POINT('Origin',(0.0102313190724556,-0.0345626446731875,
0.0850101562767245));
#98704=CARTESIAN_POINT('Ctrl Pts',(0.0069348760841074,-0.0346945769586886,
0.0685228668698901));
#98705=CARTESIAN_POINT('Ctrl Pts',(0.00705273864049687,-0.0345275153362891,
0.0684979647554254));
#98706=CARTESIAN_POINT('Ctrl Pts',(0.0071714148307595,-0.0343603235965159,
0.0684767628689118));
#98707=CARTESIAN_POINT('Ctrl Pts',(0.00729055273143401,-0.034193496108874,
0.0684593186994703));
#98708=CARTESIAN_POINT('Ctrl Pts',(0.00685324951084643,-0.0346945769586886,
0.0685419752677544));
#98709=CARTESIAN_POINT('Ctrl Pts',(0.00697071183419206,-0.0345275153362891,
0.0685153634520314));
#98710=CARTESIAN_POINT('Ctrl Pts',(0.00708904145642097,-0.0343603235965159,
0.0684924388350822));
#98711=CARTESIAN_POINT('Ctrl Pts',(0.00720788740334028,-0.034193496108874,
0.0684732640163339));
#98712=CARTESIAN_POINT('Ctrl Pts',(0.00677162293758547,-0.0346945769586886,
0.0685610836656189));
#98713=CARTESIAN_POINT('Ctrl Pts',(0.00688868502788724,-0.0345275153362891,
0.0685327621486373));
#98714=CARTESIAN_POINT('Ctrl Pts',(0.00700666808208244,-0.0343603235965159,
0.0685081148012525));
#98715=CARTESIAN_POINT('Ctrl Pts',(0.00712522207524654,-0.034193496108874,
0.0684872093331976));
#98716=CARTESIAN_POINT('Ctrl Pts',(0.0066899963643245,-0.0346945769586886,
0.0685801920634833));
#98717=CARTESIAN_POINT('Ctrl Pts',(0.00680665822158242,-0.0345275153362891,
0.0685501608452433));
#98718=CARTESIAN_POINT('Ctrl Pts',(0.00692429470774392,-0.0343603235965159,
0.068523790767423));
#98719=CARTESIAN_POINT('Ctrl Pts',(0.00704255674715281,-0.034193496108874,
0.0685011546500612));
#98720=CARTESIAN_POINT('Ctrl Pts',(0.00716729603638599,-0.0340223579322365,
0.0684802195640239));
#98721=CARTESIAN_POINT('Ctrl Pts',(0.0072454970960055,-0.0339125849573554,
0.0684670271253022));
#98722=CARTESIAN_POINT('Ctrl Pts',(0.00732391625747238,-0.0338030433565221,
0.0684554625369745));
#98723=CARTESIAN_POINT('Ctrl Pts',(0.00740245192490082,-0.0336938721132328,
0.0684455316983661));
#98724=CARTESIAN_POINT('Ctrl Pts',(0.00707638746862284,-0.0340223579322365,
0.0684125674233514));
#98725=CARTESIAN_POINT('Ctrl Pts',(0.0071555216277064,-0.0339125849573554,
0.0683981211183808));
#98726=CARTESIAN_POINT('Ctrl Pts',(0.00723489918507691,-0.0338030433565221,
0.068385322857872));
#98727=CARTESIAN_POINT('Ctrl Pts',(0.00731441717936894,-0.0336938721132328,
0.0683741800101628));
#98728=CARTESIAN_POINT('Ctrl Pts',(0.00698547890085968,-0.0340223579322365,
0.0683449152826789));
#98729=CARTESIAN_POINT('Ctrl Pts',(0.00706554615940729,-0.0339125849573554,
0.0683292151114593));
#98730=CARTESIAN_POINT('Ctrl Pts',(0.00714588211268144,-0.0338030433565221,
0.0683151831787696));
#98731=CARTESIAN_POINT('Ctrl Pts',(0.00722638243383706,-0.0336938721132328,
0.0683028283219595));
#98732=CARTESIAN_POINT('Ctrl Pts',(0.00689457033309653,-0.0340223579322365,
0.0682772631420064));
#98733=CARTESIAN_POINT('Ctrl Pts',(0.00697557069110819,-0.0339125849573554,
0.0682603091045379));
#98734=CARTESIAN_POINT('Ctrl Pts',(0.00705686504028598,-0.0338030433565221,
0.0682450434996672));
#98735=CARTESIAN_POINT('Ctrl Pts',(0.00713834768830519,-0.0336938721132328,
0.0682314766337562));
#98736=CARTESIAN_POINT('Origin',(0.0106732350869064,-0.0345589643416464,
0.0847798378537598));
#98737=CARTESIAN_POINT('Ctrl Pts',(0.00748642642908477,-0.034193496108874,
0.0681839479025));
#98738=CARTESIAN_POINT('Ctrl Pts',(0.00756869475421948,-0.0340836138585569,
0.068175159143977));
#98739=CARTESIAN_POINT('Ctrl Pts',(0.00765110547038093,-0.033973889665241,
0.0681680769728248));
#98740=CARTESIAN_POINT('Ctrl Pts',(0.00773355249440548,-0.0338644633307392,
0.0681627033828056));
#98741=CARTESIAN_POINT('Ctrl Pts',(0.00742074333719059,-0.034193496108874,
0.0682762890671347));
#98742=CARTESIAN_POINT('Ctrl Pts',(0.00750173833235243,-0.0340836138585569,
0.068266594577674));
#98743=CARTESIAN_POINT('Ctrl Pts',(0.00758289507170985,-0.033973889665241,
0.0682585807612792));
#98744=CARTESIAN_POINT('Ctrl Pts',(0.00766410899710287,-0.0338644633307392,
0.0682522509116897));
#98745=CARTESIAN_POINT('Ctrl Pts',(0.00735506024529641,-0.034193496108874,
0.0683686302317693));
#98746=CARTESIAN_POINT('Ctrl Pts',(0.00743478191048538,-0.0340836138585569,
0.0683580300113712));
#98747=CARTESIAN_POINT('Ctrl Pts',(0.00751468467303877,-0.033973889665241,
0.0683490845497336));
#98748=CARTESIAN_POINT('Ctrl Pts',(0.00759466549980026,-0.0338644633307392,
0.0683417984405737));
#98749=CARTESIAN_POINT('Ctrl Pts',(0.00728937715340224,-0.034193496108874,
0.068460971396404));
#98750=CARTESIAN_POINT('Ctrl Pts',(0.00736782548861832,-0.0340836138585569,
0.0684494654450682));
#98751=CARTESIAN_POINT('Ctrl Pts',(0.0074464742743677,-0.033973889665241,
0.068439588338188));
#98752=CARTESIAN_POINT('Ctrl Pts',(0.00752522200249765,-0.0338644633307392,
0.0684313459694578));
#98753=CARTESIAN_POINT('Origin',(0.0102181000419078,-0.0345610621862964,
0.0849360495769488));
#98754=CARTESIAN_POINT('Ctrl Pts',(0.00725477355023421,-0.03424362768739,
0.0684646724827314));
#98755=CARTESIAN_POINT('Ctrl Pts',(0.00746919921239556,-0.033943005420186,
0.06843189728146));
#98756=CARTESIAN_POINT('Ctrl Pts',(0.00768548447618193,-0.0336441434784162,
0.068415366610555));
#98757=CARTESIAN_POINT('Ctrl Pts',(0.0070085231419664,-0.03424362768739,
0.0685078087369492));
#98758=CARTESIAN_POINT('Ctrl Pts',(0.00722132189348,-0.033943005420186,
0.0684657460484239));
#98759=CARTESIAN_POINT('Ctrl Pts',(0.00743668444009545,-0.0336441434784162,
0.0684398317294667));
#98760=CARTESIAN_POINT('Ctrl Pts',(0.0075251944362441,-0.0335235895815127,
0.0684313489820763));
#98761=CARTESIAN_POINT('Ctrl Pts',(0.00760392292649248,-0.0334144449262719,
0.0684231082430923));
#98762=CARTESIAN_POINT('Ctrl Pts',(0.0076829121137035,-0.0333049234473132,
0.0684164845078563));
#98763=CARTESIAN_POINT('Ctrl Pts',(0.0077620617621819,-0.0331951640388588,
0.0684114953953736));
#98764=CARTESIAN_POINT('Ctrl Pts',(0.00743871322695743,-0.0335235895815127,
0.0683581221227513));
#98765=CARTESIAN_POINT('Ctrl Pts',(0.00751844982909482,-0.0334144449262719,
0.0683486907996557));
#98766=CARTESIAN_POINT('Ctrl Pts',(0.00759847288296501,-0.0333049234473132,
0.0683408959393041));
#98767=CARTESIAN_POINT('Ctrl Pts',(0.00767868096652558,-0.0331951640388588,
0.0683347567779636));
#98768=CARTESIAN_POINT('Ctrl Pts',(0.00735223201767076,-0.0335235895815127,
0.0682848952634263));
#98769=CARTESIAN_POINT('Ctrl Pts',(0.00743297673169716,-0.0334144449262719,
0.068274273356219));
#98770=CARTESIAN_POINT('Ctrl Pts',(0.00751403365222652,-0.0333049234473132,
0.0682653073707518));
#98771=CARTESIAN_POINT('Ctrl Pts',(0.00759530017086926,-0.0331951640388588,
0.0682580181605535));
#98772=CARTESIAN_POINT('Ctrl Pts',(0.00726575080838409,-0.0335235895815127,
0.0682116684041013));
#98773=CARTESIAN_POINT('Ctrl Pts',(0.00734750363429951,-0.0334144449262719,
0.0681998559127824));
#98774=CARTESIAN_POINT('Ctrl Pts',(0.00742959442148803,-0.0333049234473132,
0.0681897188021996));
#98775=CARTESIAN_POINT('Ctrl Pts',(0.00751191937521294,-0.0331951640388588,
0.0681812795431434));
#98776=CARTESIAN_POINT('Origin',(0.00804984076466302,-0.0326434571769387,
0.0850760693271538));
#98777=CARTESIAN_POINT('Ctrl Pts',(0.00786357228300075,-0.0336938721132348,
0.0681541254735253));
#98778=CARTESIAN_POINT('Ctrl Pts',(0.00789866812624473,-0.0336474569764937,
0.0681526023785747));
#98779=CARTESIAN_POINT('Ctrl Pts',(0.00793377939444855,-0.033601104548885,
0.0681514902291446));
#98780=CARTESIAN_POINT('Ctrl Pts',(0.00802267304765969,-0.0334837508662601,
0.0681486745226544));
#98781=CARTESIAN_POINT('Ctrl Pts',(0.00811161110055061,-0.0333660264799399,
0.0681484941557096));
#98782=CARTESIAN_POINT('Ctrl Pts',(0.00764951775477796,-0.0336938721132348,
0.0684182290483189));
#98783=CARTESIAN_POINT('Ctrl Pts',(0.00768306771215988,-0.0336474569764937,
0.0684154530211838));
#98784=CARTESIAN_POINT('Ctrl Pts',(0.0077166478675799,-0.033601104548885,
0.0684130699288751));
#98785=CARTESIAN_POINT('Ctrl Pts',(0.00780166509547823,-0.0334837508662601,
0.0684070364874161));
#98786=CARTESIAN_POINT('Ctrl Pts',(0.00788682377344934,-0.0333660264799399,
0.0684035249319819));
#98787=CARTESIAN_POINT('Ctrl Pts',(0.00764951775478944,-0.0336938721132427,
0.0684182290483287));
#98788=CARTESIAN_POINT('Ctrl Pts',(0.00768306771217062,-0.0336474569765026,
0.0684154530211937));
#98789=CARTESIAN_POINT('Ctrl Pts',(0.0077166478675899,-0.0336011045488949,
0.0684130699288851));
#98790=CARTESIAN_POINT('Ctrl Pts',(0.0078009570177727,-0.0334847282626114,
0.0684070867377759));
#98791=CARTESIAN_POINT('Ctrl Pts',(0.00788540557795273,-0.0333679869984219,
0.068403583587206));
#98792=CARTESIAN_POINT('Ctrl Pts',(0.00764951775477237,-0.0336938721132425,
0.0684182290483193));
#98793=CARTESIAN_POINT('Ctrl Pts',(0.00776950724970819,-0.0335278710435082,
0.0684083007467696));
#98794=CARTESIAN_POINT('Ctrl Pts',(0.00788976588157369,-0.033362046922432,
0.0684021387773378));
#98795=CARTESIAN_POINT('Ctrl Pts',(0.00801035448319115,-0.0331951640388602,
0.0683997600785164));
#98796=CARTESIAN_POINT('Ctrl Pts',(0.0075661399052794,-0.0336938721132425,
0.068426956249314));
#98797=CARTESIAN_POINT('Ctrl Pts',(0.00768594670407325,-0.0335278710435082,
0.0684152825071084));
#98798=CARTESIAN_POINT('Ctrl Pts',(0.007806077440634,-0.033362046922432,
0.0684073699817591));
#98799=CARTESIAN_POINT('Ctrl Pts',(0.00792659317535379,-0.0331951640388602,
0.0684032347198865));
#98800=CARTESIAN_POINT('Ctrl Pts',(0.00748276205578642,-0.0336938721132425,
0.0684356834503088));
#98801=CARTESIAN_POINT('Ctrl Pts',(0.0076023861584383,-0.0335278710435082,
0.0684222642674473));
#98802=CARTESIAN_POINT('Ctrl Pts',(0.00772238899969432,-0.033362046922432,
0.0684126011861805));
#98803=CARTESIAN_POINT('Ctrl Pts',(0.00784283186751643,-0.0331951640388602,
0.0684067093612567));
#98804=CARTESIAN_POINT('Ctrl Pts',(0.00739938420629345,-0.0336938721132425,
0.0684444106513035));
#98805=CARTESIAN_POINT('Ctrl Pts',(0.00751882561280336,-0.0335278710435082,
0.0684292460277861));
#98806=CARTESIAN_POINT('Ctrl Pts',(0.00763870055875463,-0.033362046922432,
0.0684178323906018));
#98807=CARTESIAN_POINT('Ctrl Pts',(0.00775907055967907,-0.0331951640388602,
0.0684101840026268));
#98808=CARTESIAN_POINT('Ctrl Pts',(0.00788545141224616,-0.0330240426238155,
0.0684050475007324));
#98809=CARTESIAN_POINT('Ctrl Pts',(0.00796459372995917,-0.0329142774063509,
0.0684017642620316));
#98810=CARTESIAN_POINT('Ctrl Pts',(0.00804384337671913,-0.0328043479726686,
0.0684001154792969));
#98811=CARTESIAN_POINT('Ctrl Pts',(0.00812309888599626,-0.0326943950436594,
0.0684001060607139));
#98812=CARTESIAN_POINT('Ctrl Pts',(0.00780373890997204,-0.0330240426238155,
0.0683265350625032));
#98813=CARTESIAN_POINT('Ctrl Pts',(0.00788396281301261,-0.0329142774063509,
0.0683221261544749));
#98814=CARTESIAN_POINT('Ctrl Pts',(0.00796431785503927,-0.0328043479726686,
0.0683193735006156));
#98815=CARTESIAN_POINT('Ctrl Pts',(0.00804470119237377,-0.0326943950436594,
0.0683182834622508));
#98816=CARTESIAN_POINT('Ctrl Pts',(0.00772202640769792,-0.0330240426238155,
0.068248022624274));
#98817=CARTESIAN_POINT('Ctrl Pts',(0.00780333189606606,-0.0329142774063509,
0.0682424880469183));
#98818=CARTESIAN_POINT('Ctrl Pts',(0.00788479233335941,-0.0328043479726686,
0.0682386315219343));
#98819=CARTESIAN_POINT('Ctrl Pts',(0.00796630349875127,-0.0326943950436594,
0.0682364608637877));
#98820=CARTESIAN_POINT('Ctrl Pts',(0.0076403139054238,-0.0330240426238155,
0.0681695101860449));
#98821=CARTESIAN_POINT('Ctrl Pts',(0.0077227009791195,-0.0329142774063509,
0.0681628499393617));
#98822=CARTESIAN_POINT('Ctrl Pts',(0.00780526681167955,-0.0328043479726686,
0.0681578895432529));
#98823=CARTESIAN_POINT('Ctrl Pts',(0.00788790580512878,-0.0326943950436594,
0.0681546382653245));
#98824=CARTESIAN_POINT('Origin',(0.00805176743042016,-0.0326396682857536,
0.085199728886723));
#98825=CARTESIAN_POINT('Ctrl Pts',(0.00823919677064576,-0.0331951640388588,
0.0681511101464263));
#98826=CARTESIAN_POINT('Ctrl Pts',(0.00832181933892492,-0.033085561830543,
0.068152699748677));
#98827=CARTESIAN_POINT('Ctrl Pts',(0.00840446861429596,-0.0329757224528702,
0.0681559981640262));
#98828=CARTESIAN_POINT('Ctrl Pts',(0.0084870385522225,-0.0328657862230221,
0.0681610063601986));
#98829=CARTESIAN_POINT('Ctrl Pts',(0.00816245821433043,-0.0331951640388588,
0.0682344908756998));
#98830=CARTESIAN_POINT('Ctrl Pts',(0.00824393238179449,-0.033085561830543,
0.0682350235596266));
#98831=CARTESIAN_POINT('Ctrl Pts',(0.00832545427317847,-0.0329757224528702,
0.0682372405592537));
#98832=CARTESIAN_POINT('Ctrl Pts',(0.00840691935555694,-0.0328657862230221,
0.0682411441563076));
#98833=CARTESIAN_POINT('Ctrl Pts',(0.00808571965801511,-0.0331951640388588,
0.0683178716049733));
#98834=CARTESIAN_POINT('Ctrl Pts',(0.00816604542466406,-0.033085561830543,
0.0683173473705764));
#98835=CARTESIAN_POINT('Ctrl Pts',(0.00824643993206098,-0.0329757224528702,
0.0683184829544813));
#98836=CARTESIAN_POINT('Ctrl Pts',(0.00832680015889138,-0.0328657862230221,
0.0683212819524166));
#98837=CARTESIAN_POINT('Ctrl Pts',(0.00800898110169978,-0.0331951640388588,
0.0684012523342468));
#98838=CARTESIAN_POINT('Ctrl Pts',(0.00808815846753363,-0.033085561830543,
0.0683996711815261));
#98839=CARTESIAN_POINT('Ctrl Pts',(0.00816742559094349,-0.0329757224528702,
0.0683997253497088));
#98840=CARTESIAN_POINT('Ctrl Pts',(0.00824668096222582,-0.0328657862230221,
0.0684014197485256));
#98841=CARTESIAN_POINT('Origin',(0.0075726680375036,-0.0326401908834165,
0.0851580558324018));
#98842=CARTESIAN_POINT('Ctrl Pts',(0.00797425886923198,-0.0332451089994433,
0.0684005854406194));
#98843=CARTESIAN_POINT('Ctrl Pts',(0.00819110158707134,-0.0329451141710259,
0.0683949460761945));
#98844=CARTESIAN_POINT('Ctrl Pts',(0.00840775305761736,-0.0326442513127504,
0.0684056562125766));
#98845=CARTESIAN_POINT('Ctrl Pts',(0.0077245436624227,-0.0332451089994433,
0.0684125150461534));
#98846=CARTESIAN_POINT('Ctrl Pts',(0.00794093644782806,-0.0329451141710259,
0.0683974575186145));
#98847=CARTESIAN_POINT('Ctrl Pts',(0.00815784867869816,-0.0326442513127504,
0.0683987423571396));
#98848=CARTESIAN_POINT('Ctrl Pts',(0.00824664939475422,-0.0325229783203384,
0.0684014189839514));
#98849=CARTESIAN_POINT('Ctrl Pts',(0.00832589345690486,-0.0324130253112079,
0.0684031127056083));
#98850=CARTESIAN_POINT('Ctrl Pts',(0.00840509046333346,-0.0323031222247695,
0.068406445435571));
#98851=CARTESIAN_POINT('Ctrl Pts',(0.00848413911894741,-0.0321934096636184,
0.0684114093251639));
#98852=CARTESIAN_POINT('Ctrl Pts',(0.00817002793696981,-0.0325229783203384,
0.0683179306922193));
#98853=CARTESIAN_POINT('Ctrl Pts',(0.00825042288337526,-0.0324130253112079,
0.0683185681887754));
#98854=CARTESIAN_POINT('Ctrl Pts',(0.00833079244887716,-0.0323031222247695,
0.0683208686613535));
#98855=CARTESIAN_POINT('Ctrl Pts',(0.00841103378976034,-0.0321934096636184,
0.0683248255305266));
#98856=CARTESIAN_POINT('Ctrl Pts',(0.00809340647918541,-0.0325229783203384,
0.0682344424004872));
#98857=CARTESIAN_POINT('Ctrl Pts',(0.00817495230984567,-0.0324130253112079,
0.0682340236719426));
#98858=CARTESIAN_POINT('Ctrl Pts',(0.00825649443442085,-0.0323031222247695,
0.068235291887136));
#98859=CARTESIAN_POINT('Ctrl Pts',(0.00833792846057326,-0.0321934096636184,
0.0682382417358893));
#98860=CARTESIAN_POINT('Ctrl Pts',(0.008016785021401,-0.0325229783203384,
0.0681509541087551));
#98861=CARTESIAN_POINT('Ctrl Pts',(0.00809948173631607,-0.0324130253112079,
0.0681494791551098));
#98862=CARTESIAN_POINT('Ctrl Pts',(0.00818219641996455,-0.0323031222247695,
0.0681497151129185));
#98863=CARTESIAN_POINT('Ctrl Pts',(0.00826482313138619,-0.0321934096636184,
0.068151657941252));
#98864=CARTESIAN_POINT('Origin',(0.00805206138852261,-0.0326393375177959,
0.0851912080523513));
#98865=CARTESIAN_POINT('Ctrl Pts',(0.00861564243684593,-0.0326943950436593,
0.0681701945265211));
#98866=CARTESIAN_POINT('Ctrl Pts',(0.00869805536362011,-0.0325844576448127,
0.0681769732825241));
#98867=CARTESIAN_POINT('Ctrl Pts',(0.0087803339270971,-0.0324744968375319,
0.0681854569527138));
#98868=CARTESIAN_POINT('Ctrl Pts',(0.00886237285710993,-0.0323646534831895,
0.0681956332132571));
#98869=CARTESIAN_POINT('Ctrl Pts',(0.0085338198651545,-0.0326943950436593,
0.0682485921944925));
#98870=CARTESIAN_POINT('Ctrl Pts',(0.00861515232513115,-0.0325844576448127,
0.0682542432821058));
#98871=CARTESIAN_POINT('Ctrl Pts',(0.00869637366737543,-0.0324744968375319,
0.068261576858274));
#98872=CARTESIAN_POINT('Ctrl Pts',(0.00877737995596894,-0.0323646534831895,
0.0682705820914154));
#98873=CARTESIAN_POINT('Ctrl Pts',(0.00845199729346307,-0.0326943950436593,
0.0683269898624639));
#98874=CARTESIAN_POINT('Ctrl Pts',(0.00853224928664219,-0.0325844576448127,
0.0683315132816874));
#98875=CARTESIAN_POINT('Ctrl Pts',(0.00861241340765376,-0.0324744968375319,
0.0683376967638342));
#98876=CARTESIAN_POINT('Ctrl Pts',(0.00869238705482796,-0.0323646534831895,
0.0683455309695737));
#98877=CARTESIAN_POINT('Ctrl Pts',(0.00837017472177164,-0.0326943950436593,
0.0684053875304353));
#98878=CARTESIAN_POINT('Ctrl Pts',(0.00844934624815322,-0.0325844576448127,
0.0684087832812691));
#98879=CARTESIAN_POINT('Ctrl Pts',(0.00852845314793209,-0.0324744968375319,
0.0684138166693945));
#98880=CARTESIAN_POINT('Ctrl Pts',(0.00860739415368697,-0.0323646534831895,
0.068420479847732));
#98881=CARTESIAN_POINT('Origin',(0.00757123337387066,-0.0326395579068887,
0.0851958698995984));
#98882=CARTESIAN_POINT('Ctrl Pts',(0.00833552344979301,-0.0327445246961877,
0.0684025405055608));
#98883=CARTESIAN_POINT('Ctrl Pts',(0.00855229242606044,-0.0324436878365475,
0.0684105264575262));
#98884=CARTESIAN_POINT('Ctrl Pts',(0.00876784405003831,-0.0321434074463187,
0.0684348176473144));
#98885=CARTESIAN_POINT('Ctrl Pts',(0.008085551907043,-0.0327445246961877,
0.0683987685279387));
#98886=CARTESIAN_POINT('Ctrl Pts',(0.00830246314577066,-0.0324436878365475,
0.0683973266491432));
#98887=CARTESIAN_POINT('Ctrl Pts',(0.00851886677079367,-0.0321434074463187,
0.0684122275074315));
#98888=CARTESIAN_POINT('Ctrl Pts',(0.00870155650025176,-0.0322357242816073,
0.0684277363002037));
#98889=CARTESIAN_POINT('Ctrl Pts',(0.00888380317758615,-0.0319819883628706,
0.0684461376625405));
#98890=CARTESIAN_POINT('Ctrl Pts',(0.00906450957808754,-0.0317295851069886,
0.0684760986096733));
#98891=CARTESIAN_POINT('Ctrl Pts',(0.00845233410582779,-0.0322357242816073,
0.0684080335562937));
#98892=CARTESIAN_POINT('Ctrl Pts',(0.00863520829000221,-0.0319819883628706,
0.0684184975085977));
#98893=CARTESIAN_POINT('Ctrl Pts',(0.00881704600573044,-0.0317295851069886,
0.0684405770618994));
#98894=CARTESIAN_POINT('Origin',(0.00757769600471676,-0.0326371942646347,
0.0851007876301448));
#98895=CARTESIAN_POINT('Origin',(0.00805577218063784,-0.0326352985527098,
0.0850685294765079));
#98896=CARTESIAN_POINT('Ctrl Pts',(0.00899014695537443,-0.0321934096636184,
0.0682128784669059));
#98897=CARTESIAN_POINT('Ctrl Pts',(0.00907202448842683,-0.0320835708272304,
0.0682248263121812));
#98898=CARTESIAN_POINT('Ctrl Pts',(0.00915360726914559,-0.0319739230346346,
0.0682384616785115));
#98899=CARTESIAN_POINT('Ctrl Pts',(0.00923479225691667,-0.0318646057455575,
0.0682537591095561));
#98900=CARTESIAN_POINT('Ctrl Pts',(0.00890356308617857,-0.0321934096636184,
0.068285983859045));
#98901=CARTESIAN_POINT('Ctrl Pts',(0.00898443243889849,-0.0320835708272304,
0.0682967376452847));
#98902=CARTESIAN_POINT('Ctrl Pts',(0.00906503233506001,-0.0319739230346346,
0.0683091587809427));
#98903=CARTESIAN_POINT('Ctrl Pts',(0.00914526087235309,-0.0318646057455575,
0.0683232234597141));
#98904=CARTESIAN_POINT('Ctrl Pts',(0.0088169792169827,-0.0321934096636184,
0.0683590892511841));
#98905=CARTESIAN_POINT('Ctrl Pts',(0.00889684038937014,-0.0320835708272304,
0.0683686489783883));
#98906=CARTESIAN_POINT('Ctrl Pts',(0.00897645740097444,-0.0319739230346346,
0.0683798558833738));
#98907=CARTESIAN_POINT('Ctrl Pts',(0.00905572948778951,-0.0318646057455575,
0.068392687809872));
#98908=CARTESIAN_POINT('Ctrl Pts',(0.00873039534778683,-0.0321934096636184,
0.0684321946433232));
#98909=CARTESIAN_POINT('Ctrl Pts',(0.0088092483398418,-0.0320835708272304,
0.0684405603114918));
#98910=CARTESIAN_POINT('Ctrl Pts',(0.00888788246688886,-0.0319739230346346,
0.068450552985805));
#98911=CARTESIAN_POINT('Ctrl Pts',(0.00896619810322593,-0.0318646057455575,
0.06846215216003));
#98912=CARTESIAN_POINT('Ctrl Pts',(0.00860699565471972,-0.0320218834582337,
0.0684196158461317));
#98913=CARTESIAN_POINT('Ctrl Pts',(0.00866663510064553,-0.0319391099350648,
0.0684246449301059));
#98914=CARTESIAN_POINT('Ctrl Pts',(0.00872615988269489,-0.0318564869454945,
0.0684306022453965));
#98915=CARTESIAN_POINT('Ctrl Pts',(0.00878552705004609,-0.0317740741446553,
0.0684374794053147));
#98916=CARTESIAN_POINT('Ctrl Pts',(0.00857584241890168,-0.0320218834582337,
0.0683810632334404));
#98917=CARTESIAN_POINT('Ctrl Pts',(0.00863588310432525,-0.0319391099350648,
0.0683857680875422));
#98918=CARTESIAN_POINT('Ctrl Pts',(0.00869581394566648,-0.0318564869454945,
0.068391407634814));
#98919=CARTESIAN_POINT('Ctrl Pts',(0.00875559167473568,-0.0317740741446553,
0.0683979736924077));
#98920=CARTESIAN_POINT('Ctrl Pts',(0.00854468918308364,-0.0320218834582337,
0.0683425106207491));
#98921=CARTESIAN_POINT('Ctrl Pts',(0.00860513110800498,-0.0319391099350648,
0.0683468912449785));
#98922=CARTESIAN_POINT('Ctrl Pts',(0.00866546800863808,-0.0318564869454945,
0.0683522130242316));
#98923=CARTESIAN_POINT('Ctrl Pts',(0.00872565629942528,-0.0317740741446553,
0.0683584679795008));
#98924=CARTESIAN_POINT('Ctrl Pts',(0.00851353594726561,-0.0320218834582337,
0.0683039580080578));
#98925=CARTESIAN_POINT('Ctrl Pts',(0.00857437911168471,-0.0319391099350648,
0.0683080144024148));
#98926=CARTESIAN_POINT('Ctrl Pts',(0.00863512207160967,-0.0318564869454945,
0.0683130184136491));
#98927=CARTESIAN_POINT('Ctrl Pts',(0.00869572092411487,-0.0317740741446553,
0.0683189622665938));
#98928=CARTESIAN_POINT('Origin',(0.00819704568072141,-0.0391228853390677,
0.0620721172885788));
#98929=CARTESIAN_POINT('Ctrl Pts',(0.00562201316168811,-0.0352722978779565,
0.0689706838042051));
#98930=CARTESIAN_POINT('Ctrl Pts',(0.00563917834702537,-0.0352466642097198,
0.0689627813305198));
#98931=CARTESIAN_POINT('Ctrl Pts',(0.00565629545372585,-0.0352210183808291,
0.0689548146806992));
#98932=CARTESIAN_POINT('Ctrl Pts',(0.00567336486113266,-0.0351953608940152,
0.0689467830908172));
#98933=CARTESIAN_POINT('Origin',(0.00373885063905858,-0.0352456003065043,
0.0644470301804282));
#98934=CARTESIAN_POINT('Ctrl Pts',(0.00578732996892189,-0.035024121149334,
0.0688962136373421));
#98935=CARTESIAN_POINT('Ctrl Pts',(0.0058596987186681,-0.0349144232867421,
0.0688640299673878));
#98936=CARTESIAN_POINT('Ctrl Pts',(0.00593277604402248,-0.0348045283677512,
0.0688333229476583));
#98937=CARTESIAN_POINT('Ctrl Pts',(0.00600646980585258,-0.0346945769586886,
0.0688041353931166));
#98938=CARTESIAN_POINT('Ctrl Pts',(0.00568245322679813,-0.035024121149334,
0.0688532949844682));
#98939=CARTESIAN_POINT('Ctrl Pts',(0.00575541316336368,-0.0349144232867421,
0.0688196666804574));
#98940=CARTESIAN_POINT('Ctrl Pts',(0.00582911189100808,-0.0348045283677512,
0.0687875263822418));
#98941=CARTESIAN_POINT('Ctrl Pts',(0.00590345654297772,-0.0346945769586886,
0.0687569187702505));
#98942=CARTESIAN_POINT('Ctrl Pts',(0.00557757648467437,-0.035024121149334,
0.0688103763315943));
#98943=CARTESIAN_POINT('Ctrl Pts',(0.00565112760805927,-0.0349144232867421,
0.0687753033935271));
#98944=CARTESIAN_POINT('Ctrl Pts',(0.00572544773799369,-0.0348045283677512,
0.0687417298168253));
#98945=CARTESIAN_POINT('Ctrl Pts',(0.00580044328010287,-0.0346945769586886,
0.0687097021473843));
#98946=CARTESIAN_POINT('Ctrl Pts',(0.0054726997425506,-0.035024121149334,
0.0687674576787204));
#98947=CARTESIAN_POINT('Ctrl Pts',(0.00554684205275485,-0.0349144232867421,
0.0687309401065967));
#98948=CARTESIAN_POINT('Ctrl Pts',(0.00562178358497929,-0.0348045283677512,
0.0686959332514088));
#98949=CARTESIAN_POINT('Ctrl Pts',(0.00569743001722801,-0.0346945769586886,
0.0686624855245182));
#98950=CARTESIAN_POINT('Origin',(0.0120209044952922,-0.0345629067943303,
0.0844786218103012));
#98951=CARTESIAN_POINT('Ctrl Pts',(0.00598812243932284,-0.0351970973651659,
0.0686169647395614));
#98952=CARTESIAN_POINT('Ctrl Pts',(0.00606477514426711,-0.03508693493218,
0.0685873780680036));
#98953=CARTESIAN_POINT('Ctrl Pts',(0.0061421064379258,-0.0349764985129734,
0.0685593604544486));
#98954=CARTESIAN_POINT('Ctrl Pts',(0.0062200182720283,-0.0348659306849638,
0.0685329540940108));
#98955=CARTESIAN_POINT('Ctrl Pts',(0.00595864267170211,-0.0351970973651659,
0.0686937202862751));
#98956=CARTESIAN_POINT('Ctrl Pts',(0.00603423203256883,-0.03508693493218,
0.0686637252124891));
#98957=CARTESIAN_POINT('Ctrl Pts',(0.00611050759174411,-0.0349764985129734,
0.0686352767520561));
#98958=CARTESIAN_POINT('Ctrl Pts',(0.0061873727015498,-0.0348659306849638,
0.0686084175777525));
#98959=CARTESIAN_POINT('Ctrl Pts',(0.00592916290408138,-0.0351970973651659,
0.0687704758329889));
#98960=CARTESIAN_POINT('Ctrl Pts',(0.00600368892087055,-0.03508693493218,
0.0687400723569746));
#98961=CARTESIAN_POINT('Ctrl Pts',(0.00607890874556241,-0.0349764985129734,
0.0687111930496637));
#98962=CARTESIAN_POINT('Ctrl Pts',(0.00615472713107129,-0.0348659306849638,
0.0686838810614941));
#98963=CARTESIAN_POINT('Ctrl Pts',(0.00589968313646066,-0.0351970973651659,
0.0688472313797026));
#98964=CARTESIAN_POINT('Ctrl Pts',(0.00597314580917227,-0.03508693493218,
0.0688164195014601));
#98965=CARTESIAN_POINT('Ctrl Pts',(0.00604730989938071,-0.0349764985129734,
0.0687871093472712));
#98966=CARTESIAN_POINT('Ctrl Pts',(0.00612208156059279,-0.0348659306849638,
0.0687593445452358));
#98967=CARTESIAN_POINT('Origin',(0.0115568720158949,-0.034563718796663,
0.0846051098115322));
#98968=CARTESIAN_POINT('Ctrl Pts',(0.00586826380884067,-0.0352450361861252,
0.0688593703760109));
#98969=CARTESIAN_POINT('Ctrl Pts',(0.00606780317426413,-0.0349452761023764,
0.0687743021064317));
#98970=CARTESIAN_POINT('Ctrl Pts',(0.0062731833593555,-0.0346444289983475,
0.0687045056279055));
#98971=CARTESIAN_POINT('Ctrl Pts',(0.005640475954028,-0.0352450361861252,
0.0689623883026054));
#98972=CARTESIAN_POINT('Ctrl Pts',(0.00583612993469371,-0.0349452761023764,
0.0688687288733285));
#98973=CARTESIAN_POINT('Ctrl Pts',(0.00603828289427984,-0.0346444289983475,
0.0687900729786137));
#98974=CARTESIAN_POINT('Ctrl Pts',(0.00612182746827824,-0.0345231616327822,
0.068759874023479));
#98975=CARTESIAN_POINT('Ctrl Pts',(0.00619612276617375,-0.0344132092796975,
0.0687322798961242));
#98976=CARTESIAN_POINT('Ctrl Pts',(0.00627098499353181,-0.0343032738558974,
0.0687062239321332));
#98977=CARTESIAN_POINT('Ctrl Pts',(0.00634631738812818,-0.0341934961088741,
0.0686817370555091));
#98978=CARTESIAN_POINT('Ctrl Pts',(0.00601985257553799,-0.0345231616327822,
0.0687104548228676));
#98979=CARTESIAN_POINT('Ctrl Pts',(0.00609482904753725,-0.0344132092796975,
0.0686814551151856));
#98980=CARTESIAN_POINT('Ctrl Pts',(0.00617040148717397,-0.0343032738558974,
0.0686540077329378));
#98981=CARTESIAN_POINT('Ctrl Pts',(0.00624647217669877,-0.0341934961088741,
0.0686281453593886));
#98982=CARTESIAN_POINT('Ctrl Pts',(0.00591787768279773,-0.0345231616327822,
0.0686610356222562));
#98983=CARTESIAN_POINT('Ctrl Pts',(0.00599353532890075,-0.0344132092796975,
0.0686306303342469));
#98984=CARTESIAN_POINT('Ctrl Pts',(0.00606981798081613,-0.0343032738558974,
0.0686017915337425));
#98985=CARTESIAN_POINT('Ctrl Pts',(0.00614662696526936,-0.0341934961088741,
0.0685745536632681));
#98986=CARTESIAN_POINT('Ctrl Pts',(0.00581590279005748,-0.0345231616327822,
0.0686116164216449));
#98987=CARTESIAN_POINT('Ctrl Pts',(0.00589224161026425,-0.0344132092796975,
0.0685798055533083));
#98988=CARTESIAN_POINT('Ctrl Pts',(0.0059692344744583,-0.0343032738558974,
0.0685495753345471));
#98989=CARTESIAN_POINT('Ctrl Pts',(0.00604678175383996,-0.0341934961088741,
0.0685209619671476));
#98990=CARTESIAN_POINT('Origin',(0.0120254107912183,-0.0345625596229832,
0.0844898553130019));
#98991=CARTESIAN_POINT('Ctrl Pts',(0.00637978906701317,-0.0346945769586885,
0.0684090516483639));
#98992=CARTESIAN_POINT('Ctrl Pts',(0.00645890223700392,-0.0345846629176689,
0.0683850185416024));
#98993=CARTESIAN_POINT('Ctrl Pts',(0.00653852591449628,-0.0344746925051586,
0.0683626173577916));
#98994=CARTESIAN_POINT('Ctrl Pts',(0.00661855795792006,-0.0343648066255171,
0.0683418763785691));
#98995=CARTESIAN_POINT('Ctrl Pts',(0.0063325724813239,-0.0346945769586885,
0.0685120648301294));
#98996=CARTESIAN_POINT('Ctrl Pts',(0.00641026607760293,-0.0345846629176689,
0.0684873810549519));
#98997=CARTESIAN_POINT('Ctrl Pts',(0.00648848339447251,-0.0344746925051586,
0.0684642997353881));
#98998=CARTESIAN_POINT('Ctrl Pts',(0.00656712408875471,-0.0343648066255171,
0.0684428500319857));
#98999=CARTESIAN_POINT('Ctrl Pts',(0.00628535589563463,-0.0346945769586885,
0.068615078011895));
#99000=CARTESIAN_POINT('Ctrl Pts',(0.00636162991820194,-0.034584662917669,
0.0685897435683015));
#99001=CARTESIAN_POINT('Ctrl Pts',(0.00643844087444875,-0.0344746925051586,
0.0685659821129846));
#99002=CARTESIAN_POINT('Ctrl Pts',(0.00651569021958936,-0.0343648066255171,
0.0685438236854023));
#99003=CARTESIAN_POINT('Ctrl Pts',(0.00623813930994536,-0.0346945769586885,
0.0687180911936605));
#99004=CARTESIAN_POINT('Ctrl Pts',(0.00631299375880095,-0.034584662917669,
0.068692106081651));
#99005=CARTESIAN_POINT('Ctrl Pts',(0.00638839835442498,-0.0344746925051586,
0.0686676644905811));
#99006=CARTESIAN_POINT('Ctrl Pts',(0.00646425635042401,-0.0343648066255171,
0.0686447973388189));
#99007=CARTESIAN_POINT('Origin',(0.0115758390175073,-0.0345626446731051,
0.0846603762881038));
#99008=CARTESIAN_POINT('Ctrl Pts',(0.00623898417299243,-0.0346945769586885,
0.0687162479424096));
#99009=CARTESIAN_POINT('Ctrl Pts',(0.00635279628539246,-0.034527515336289,
0.068676770093247));
#99010=CARTESIAN_POINT('Ctrl Pts',(0.00646787937745356,-0.0343603235965159,
0.0686408613192686));
#99011=CARTESIAN_POINT('Ctrl Pts',(0.00658389150603351,-0.034193496108874,
0.0686086227639818));
#99012=CARTESIAN_POINT('Ctrl Pts',(0.00616039616693489,-0.0346945769586885,
0.0687454361872211));
#99013=CARTESIAN_POINT('Ctrl Pts',(0.00627359691986101,-0.034527515336289,
0.0687043122808066));
#99014=CARTESIAN_POINT('Ctrl Pts',(0.00638812026130482,-0.0343603235965159,
0.068666737797129));
#99015=CARTESIAN_POINT('Ctrl Pts',(0.00650362583039834,-0.034193496108874,
0.0686328188307304));
#99016=CARTESIAN_POINT('Ctrl Pts',(0.00608180816087734,-0.0346945769586885,
0.0687746244320324));
#99017=CARTESIAN_POINT('Ctrl Pts',(0.00619439755432957,-0.034527515336289,
0.0687318544683663));
#99018=CARTESIAN_POINT('Ctrl Pts',(0.00630836114515607,-0.0343603235965159,
0.0686926142749894));
#99019=CARTESIAN_POINT('Ctrl Pts',(0.00642336015476317,-0.034193496108874,
0.0686570148974789));
#99020=CARTESIAN_POINT('Ctrl Pts',(0.0060032201548198,-0.0346945769586885,
0.0688038126768439));
#99021=CARTESIAN_POINT('Ctrl Pts',(0.00611519818879812,-0.034527515336289,
0.0687593966559259));
#99022=CARTESIAN_POINT('Ctrl Pts',(0.00622860202900733,-0.0343603235965159,
0.0687184907528498));
#99023=CARTESIAN_POINT('Ctrl Pts',(0.006343094479128,-0.034193496108874,
0.0686812109642275));
#99024=CARTESIAN_POINT('Ctrl Pts',(0.00646422629977976,-0.0340223579322365,
0.0686448069791245));
#99025=CARTESIAN_POINT('Ctrl Pts',(0.00654015726968307,-0.0339125849573554,
0.0686219173750522));
#99026=CARTESIAN_POINT('Ctrl Pts',(0.00661650864538917,-0.0338030433565221,
0.0686006154498775));
#99027=CARTESIAN_POINT('Ctrl Pts',(0.0066931803715077,-0.0336938721132327,
0.0685809197897488));
#99028=CARTESIAN_POINT('Ctrl Pts',(0.00636555551167844,-0.0340223579322365,
0.0685890821605443));
#99029=CARTESIAN_POINT('Ctrl Pts',(0.00644225507216639,-0.0339125849573554,
0.0685648316289599));
#99030=CARTESIAN_POINT('Ctrl Pts',(0.00651940266641457,-0.0338030433565221,
0.0685421856406203));
#99031=CARTESIAN_POINT('Ctrl Pts',(0.00659689706843624,-0.0336938721132327,
0.0685211644102423));
#99032=CARTESIAN_POINT('Ctrl Pts',(0.00626688472357712,-0.0340223579322365,
0.0685333573419642));
#99033=CARTESIAN_POINT('Ctrl Pts',(0.00634435287464971,-0.0339125849573554,
0.0685077458828677));
#99034=CARTESIAN_POINT('Ctrl Pts',(0.00642229668743997,-0.0338030433565221,
0.068483755831363));
#99035=CARTESIAN_POINT('Ctrl Pts',(0.00650061376536478,-0.0336938721132327,
0.0684614090307357));
#99036=CARTESIAN_POINT('Ctrl Pts',(0.0061682139354758,-0.0340223579322365,
0.0684776325233841));
#99037=CARTESIAN_POINT('Ctrl Pts',(0.00624645067713303,-0.0339125849573554,
0.0684506601367754));
#99038=CARTESIAN_POINT('Ctrl Pts',(0.00632519070846537,-0.0338030433565221,
0.0684253260221058));
#99039=CARTESIAN_POINT('Ctrl Pts',(0.00640433046229332,-0.0336938721132327,
0.0684016536512291));
#99040=CARTESIAN_POINT('Origin',(0.0119854038397793,-0.0345589643416696,
0.0843764872320283));
#99041=CARTESIAN_POINT('Ctrl Pts',(0.00674370756866029,-0.0341934961088739,
0.0683108738640981));
#99042=CARTESIAN_POINT('Ctrl Pts',(0.00682422565995426,-0.0340836138585568,
0.0682918434523519));
#99043=CARTESIAN_POINT('Ctrl Pts',(0.00690509891159273,-0.033973889665241,
0.0682744883246977));
#99044=CARTESIAN_POINT('Ctrl Pts',(0.00698622232679418,-0.0338644633307392,
0.0682588237549221));
#99045=CARTESIAN_POINT('Ctrl Pts',(0.00669011582431903,-0.0341934961088739,
0.0684107191653662));
#99046=CARTESIAN_POINT('Ctrl Pts',(0.00676925710804014,-0.0340836138585568,
0.0683909497552044));
#99047=CARTESIAN_POINT('Ctrl Pts',(0.00684876950474543,-0.033973889665241,
0.0683728274935761));
#99048=CARTESIAN_POINT('Ctrl Pts',(0.00692854969356229,-0.0338644633307392,
0.0683563687528613));
#99049=CARTESIAN_POINT('Ctrl Pts',(0.00663652407997777,-0.0341934961088739,
0.0685105644666344));
#99050=CARTESIAN_POINT('Ctrl Pts',(0.00671428855612601,-0.0340836138585568,
0.0684900560580568));
#99051=CARTESIAN_POINT('Ctrl Pts',(0.00679244009789812,-0.033973889665241,
0.0684711666624546));
#99052=CARTESIAN_POINT('Ctrl Pts',(0.0068708770603304,-0.0338644633307392,
0.0684539137508006));
#99053=CARTESIAN_POINT('Ctrl Pts',(0.00658293233563651,-0.0341934961088739,
0.0686104097679026));
#99054=CARTESIAN_POINT('Ctrl Pts',(0.00665932000421189,-0.0340836138585568,
0.0685891623609093));
#99055=CARTESIAN_POINT('Ctrl Pts',(0.00673611069105082,-0.033973889665241,
0.068569505831333));
#99056=CARTESIAN_POINT('Ctrl Pts',(0.00681320442709851,-0.0338644633307392,
0.0685514587487399));
#99057=CARTESIAN_POINT('Origin',(0.0115534361909259,-0.0345610621862693,
0.0845885107262112));
#99058=CARTESIAN_POINT('Ctrl Pts',(0.00654906546133213,-0.03424362768739,
0.0686184186515369));
#99059=CARTESIAN_POINT('Ctrl Pts',(0.00675769249114546,-0.033943005420186,
0.0685590272309192));
#99060=CARTESIAN_POINT('Ctrl Pts',(0.00697020043858811,-0.0336441434784161,
0.068515519177809));
#99061=CARTESIAN_POINT('Ctrl Pts',(0.00631016321730991,-0.03424362768739,
0.0686920781234407));
#99062=CARTESIAN_POINT('Ctrl Pts',(0.00651601213434268,-0.033943005420186,
0.0686236763561524));
#99063=CARTESIAN_POINT('Ctrl Pts',(0.0067264285575619,-0.0336441434784161,
0.0685709742949843));
#99064=CARTESIAN_POINT('Ctrl Pts',(0.00681317745579414,-0.0335235895815127,
0.0685514651925706));
#99065=CARTESIAN_POINT('Ctrl Pts',(0.00689025230991804,-0.0334144449262719,
0.0685334221380184));
#99066=CARTESIAN_POINT('Ctrl Pts',(0.00696778846963959,-0.0333049234473133,
0.0685169506626634));
#99067=CARTESIAN_POINT('Ctrl Pts',(0.00704568869789882,-0.0331951640388588,
0.0685020808094435));
#99068=CARTESIAN_POINT('Ctrl Pts',(0.00671820041761043,-0.0335235895815127,
0.0684896547185057));
#99069=CARTESIAN_POINT('Ctrl Pts',(0.00679612621460344,-0.0334144449262719,
0.0684703041180303));
#99070=CARTESIAN_POINT('Ctrl Pts',(0.0068745413077391,-0.0333049234473133,
0.0684525411743796));
#99071=CARTESIAN_POINT('Ctrl Pts',(0.00695334748566163,-0.0331951640388588,
0.0684363976836892));
#99072=CARTESIAN_POINT('Ctrl Pts',(0.00662322337942671,-0.0335235895815127,
0.0684278442444407));
#99073=CARTESIAN_POINT('Ctrl Pts',(0.00670200011928885,-0.0334144449262719,
0.0684071860980422));
#99074=CARTESIAN_POINT('Ctrl Pts',(0.00678129414583862,-0.0333049234473133,
0.0683881316860958));
#99075=CARTESIAN_POINT('Ctrl Pts',(0.00686100627342445,-0.0331951640388588,
0.068370714557935));
#99076=CARTESIAN_POINT('Ctrl Pts',(0.006528246341243,-0.0335235895815127,
0.0683660337703758));
#99077=CARTESIAN_POINT('Ctrl Pts',(0.00660787402397425,-0.0334144449262719,
0.0683440680780541));
#99078=CARTESIAN_POINT('Ctrl Pts',(0.00668804698393813,-0.0333049234473133,
0.0683237221978119));
#99079=CARTESIAN_POINT('Ctrl Pts',(0.00676866506118727,-0.0331951640388588,
0.0683050314321807));
#99080=CARTESIAN_POINT('Origin',(0.00941982341379305,-0.0326434571770007,
0.0849991813247499));
#99081=CARTESIAN_POINT('Ctrl Pts',(0.00711414177341354,-0.0336938721132353,
0.0682340176844868));
#99082=CARTESIAN_POINT('Ctrl Pts',(0.00714876998103594,-0.033647456976494,
0.0682281079240763));
#99083=CARTESIAN_POINT('Ctrl Pts',(0.00718346499711866,-0.033601104548885,
0.068222603935498));
#99084=CARTESIAN_POINT('Ctrl Pts',(0.00727130479332956,-0.0334837508694588,
0.0682086691030741));
#99085=CARTESIAN_POINT('Ctrl Pts',(0.0073595189347229,-0.0333660264863561,
0.0681973432648582));
#99086=CARTESIAN_POINT('Ctrl Pts',(0.00693487608410553,-0.0336938721132353,
0.0685228668698905));
#99087=CARTESIAN_POINT('Ctrl Pts',(0.00696781356159551,-0.033647456976494,
0.0685159078079139));
#99088=CARTESIAN_POINT('Ctrl Pts',(0.00700083024679538,-0.033601104548885,
0.0685093347975374));
#99089=CARTESIAN_POINT('Ctrl Pts',(0.00708442089545231,-0.0334837508694588,
0.0684926934479388));
#99090=CARTESIAN_POINT('Ctrl Pts',(0.00716846795491225,-0.0333660264863561,
0.0684785363700099));
#99091=CARTESIAN_POINT('Ctrl Pts',(0.00693487608411741,-0.0336938721132426,
0.0685228668699001));
#99092=CARTESIAN_POINT('Ctrl Pts',(0.00696781356160645,-0.0336474569765026,
0.0685159078079236));
#99093=CARTESIAN_POINT('Ctrl Pts',(0.00700083024680538,-0.0336011045488949,
0.0685093347975474));
#99094=CARTESIAN_POINT('Ctrl Pts',(0.00708372469920354,-0.033484728265791,
0.0684928320477266));
#99095=CARTESIAN_POINT('Ctrl Pts',(0.00716706829378607,-0.0333679870047996,
0.0684787723097453));
#99096=CARTESIAN_POINT('Ctrl Pts',(0.00693487608410046,-0.0336938721132425,
0.0685228668698915));
#99097=CARTESIAN_POINT('Ctrl Pts',(0.00705267507989257,-0.0335278710435082,
0.068497978184571));
#99098=CARTESIAN_POINT('Ctrl Pts',(0.00717121313697226,-0.0333620469224319,
0.0684767924009128));
#99099=CARTESIAN_POINT('Ctrl Pts',(0.00729055273143295,-0.0331951640388601,
0.0684593186994704));
#99100=CARTESIAN_POINT('Ctrl Pts',(0.00685324950217514,-0.0336938721132425,
0.0685419752697843));
#99101=CARTESIAN_POINT('Ctrl Pts',(0.00697064848071752,-0.0335278710435082,
0.068515377805027));
#99102=CARTESIAN_POINT('Ctrl Pts',(0.00708884024815148,-0.0333620469224319,
0.0684924712986398));
#99103=CARTESIAN_POINT('Ctrl Pts',(0.00720788739456458,-0.0331951640388601,
0.0684732640178144));
#99104=CARTESIAN_POINT('Ctrl Pts',(0.00677162292024982,-0.0336938721132425,
0.0685610836696771));
#99105=CARTESIAN_POINT('Ctrl Pts',(0.00688862188154248,-0.0335278710435082,
0.068532777425483));
#99106=CARTESIAN_POINT('Ctrl Pts',(0.0070064673593307,-0.0333620469224319,
0.0685081501963667));
#99107=CARTESIAN_POINT('Ctrl Pts',(0.00712522205769621,-0.0331951640388601,
0.0684872093361583));
#99108=CARTESIAN_POINT('Ctrl Pts',(0.0066899963383245,-0.0336938721132425,
0.0685801920695698));
#99109=CARTESIAN_POINT('Ctrl Pts',(0.00680659528236743,-0.0335278710435082,
0.068550177045939));
#99110=CARTESIAN_POINT('Ctrl Pts',(0.00692409447050992,-0.0333620469224319,
0.0685238290940936));
#99111=CARTESIAN_POINT('Ctrl Pts',(0.00704255672082784,-0.0331951640388601,
0.0685011546545022));
#99112=CARTESIAN_POINT('Ctrl Pts',(0.0071672972482326,-0.0330240426238155,
0.0684802189345466));
#99113=CARTESIAN_POINT('Ctrl Pts',(0.00724540400620885,-0.0329142774063509,
0.0684670424225728));
#99114=CARTESIAN_POINT('Ctrl Pts',(0.00732382209856182,-0.0328043479726686,
0.0684554740264952));
#99115=CARTESIAN_POINT('Ctrl Pts',(0.00740245147401439,-0.0326943950436593,
0.0684455313329251));
#99116=CARTESIAN_POINT('Ctrl Pts',(0.00707638885568696,-0.0330240426238155,
0.068412566882476));
#99117=CARTESIAN_POINT('Ctrl Pts',(0.00715542758659068,-0.0329142774063509,
0.0683981380188272));
#99118=CARTESIAN_POINT('Ctrl Pts',(0.007234804006101,-0.0328043479726686,
0.0683853359132153));
#99119=CARTESIAN_POINT('Ctrl Pts',(0.00731441687877833,-0.0326943950436594,
0.0683741797665357));
#99120=CARTESIAN_POINT('Ctrl Pts',(0.00698548046314132,-0.0330240426238155,
0.0683449148304054));
#99121=CARTESIAN_POINT('Ctrl Pts',(0.0070654511669725,-0.0329142774063509,
0.0683292336150816));
#99122=CARTESIAN_POINT('Ctrl Pts',(0.00714578591364018,-0.0328043479726686,
0.0683151977999353));
#99123=CARTESIAN_POINT('Ctrl Pts',(0.00722638228354226,-0.0326943950436594,
0.0683028282001464));
#99124=CARTESIAN_POINT('Ctrl Pts',(0.00689457207059568,-0.0330240426238155,
0.0682772627783349));
#99125=CARTESIAN_POINT('Ctrl Pts',(0.00697547474735433,-0.0329142774063509,
0.0682603292113359));
#99126=CARTESIAN_POINT('Ctrl Pts',(0.00705676782117937,-0.0328043479726686,
0.0682450596866554));
#99127=CARTESIAN_POINT('Ctrl Pts',(0.0071383476883062,-0.0326943950436594,
0.068231476633757));
#99128=CARTESIAN_POINT('Origin',(0.00943723353963632,-0.0326396682857081,
0.0851216243169898));
#99129=CARTESIAN_POINT('Ctrl Pts',(0.00748642642908473,-0.0331951640388588,
0.0681839479025));
#99130=CARTESIAN_POINT('Ctrl Pts',(0.00756859672750268,-0.0330855618255041,
0.0681751696162108));
#99131=CARTESIAN_POINT('Ctrl Pts',(0.00765100769351245,-0.0329757224427708,
0.0681680833213879));
#99132=CARTESIAN_POINT('Ctrl Pts',(0.00773355424004404,-0.0328657862078596,
0.0681627032690316));
#99133=CARTESIAN_POINT('Ctrl Pts',(0.00742074335562341,-0.0331951640388588,
0.0682762890412207));
#99134=CARTESIAN_POINT('Ctrl Pts',(0.00750164184166008,-0.0330855618255041,
0.0682666061034703));
#99135=CARTESIAN_POINT('Ctrl Pts',(0.00758279877605615,-0.0329757224427708,
0.0682585882188477));
#99136=CARTESIAN_POINT('Ctrl Pts',(0.00766411073612138,-0.0328657862078596,
0.0682522507525389));
#99137=CARTESIAN_POINT('Ctrl Pts',(0.00735506028216208,-0.0331951640388588,
0.0683686301799413));
#99138=CARTESIAN_POINT('Ctrl Pts',(0.00743468695581749,-0.0330855618255041,
0.0683580425907298));
#99139=CARTESIAN_POINT('Ctrl Pts',(0.00751458985859985,-0.0329757224427708,
0.0683490931163075));
#99140=CARTESIAN_POINT('Ctrl Pts',(0.00759466723219872,-0.0328657862078596,
0.0683417982360462));
#99141=CARTESIAN_POINT('Ctrl Pts',(0.00728937720870076,-0.0331951640388588,
0.068460971318662));
#99142=CARTESIAN_POINT('Ctrl Pts',(0.00736773206997489,-0.0330855618255041,
0.0684494790779893));
#99143=CARTESIAN_POINT('Ctrl Pts',(0.00744638094114354,-0.0329757224427708,
0.0684395980137673));
#99144=CARTESIAN_POINT('Ctrl Pts',(0.00752522372827606,-0.0328657862078596,
0.0684313457195535));
#99145=CARTESIAN_POINT('Origin',(0.00895668896995906,-0.0326401908832491,
0.0851403269451843));
#99146=CARTESIAN_POINT('Ctrl Pts',(0.00725484518747234,-0.0332451089994432,
0.0684646615333617));
#99147=CARTESIAN_POINT('Ctrl Pts',(0.00746927123593514,-0.0329451141710258,
0.0684318890380081));
#99148=CARTESIAN_POINT('Ctrl Pts',(0.00768555668094991,-0.0326442513127503,
0.0684153610924057));
#99149=CARTESIAN_POINT('Ctrl Pts',(0.0070085942356918,-0.0332451089994432,
0.0685077946847324));
#99150=CARTESIAN_POINT('Ctrl Pts',(0.00722139349073491,-0.0329451141710258,
0.0684657346827808));
#99151=CARTESIAN_POINT('Ctrl Pts',(0.007436756336843,-0.0326442513127503,
0.0684398230786758));
#99152=CARTESIAN_POINT('Ctrl Pts',(0.00752519230302276,-0.0325229783203385,
0.0684313489185996));
#99153=CARTESIAN_POINT('Ctrl Pts',(0.00760402378168633,-0.0324130253112079,
0.0684230973702052));
#99154=CARTESIAN_POINT('Ctrl Pts',(0.00768301399788709,-0.0323031222247695,
0.0684164778036925));
#99155=CARTESIAN_POINT('Ctrl Pts',(0.00776206147157459,-0.0321934096636184,
0.0684114951279163));
#99156=CARTESIAN_POINT('Ctrl Pts',(0.00743871117075113,-0.0325229783203385,
0.068358122172049));
#99157=CARTESIAN_POINT('Ctrl Pts',(0.00751855207849617,-0.0324130253112079,
0.0683486784831592));
#99158=CARTESIAN_POINT('Ctrl Pts',(0.00759857623163581,-0.0323031222247695,
0.0683408878382994));
#99159=CARTESIAN_POINT('Ctrl Pts',(0.00767868077278747,-0.0321934096636184,
0.0683347565996588));
#99160=CARTESIAN_POINT('Ctrl Pts',(0.00735223003847951,-0.0325229783203385,
0.0682848954254985));
#99161=CARTESIAN_POINT('Ctrl Pts',(0.00743308037530601,-0.0324130253112079,
0.0682742595961133));
#99162=CARTESIAN_POINT('Ctrl Pts',(0.00751413846538452,-0.0323031222247695,
0.0682652978729063));
#99163=CARTESIAN_POINT('Ctrl Pts',(0.00759530007400035,-0.0321934096636184,
0.0682580180714012));
#99164=CARTESIAN_POINT('Ctrl Pts',(0.00726574890620788,-0.0325229783203385,
0.0682116686789479));
#99165=CARTESIAN_POINT('Ctrl Pts',(0.00734760867211584,-0.0324130253112079,
0.0681998407090673));
#99166=CARTESIAN_POINT('Ctrl Pts',(0.00742970069913324,-0.0323031222247695,
0.0681897079075132));
#99167=CARTESIAN_POINT('Ctrl Pts',(0.00751191937521324,-0.0321934096636184,
0.0681812795431437));
#99168=CARTESIAN_POINT('Origin',(0.00943645723634511,-0.0326393375179207,
0.0851131338295842));
#99169=CARTESIAN_POINT('Ctrl Pts',(0.00786229561583585,-0.0326943950436593,
0.0681557006439515));
#99170=CARTESIAN_POINT('Ctrl Pts',(0.00794490829547628,-0.0325844576448126,
0.0681520968688386));
#99171=CARTESIAN_POINT('Ctrl Pts',(0.00802760135372221,-0.0324744968375318,
0.0681502014043413));
#99172=CARTESIAN_POINT('Ctrl Pts',(0.00811026880590754,-0.0323646534831894,
0.068150015217654));
#99173=CARTESIAN_POINT('Ctrl Pts',(0.00779094407279218,-0.0326943950436593,
0.0682437352103833));
#99174=CARTESIAN_POINT('Ctrl Pts',(0.00787234347111283,-0.0325844576448126,
0.0682391480772802));
#99175=CARTESIAN_POINT('Ctrl Pts',(0.00795384349962864,-0.0324744968375318,
0.0682362440925521));
#99176=CARTESIAN_POINT('Ctrl Pts',(0.0080353396844298,-0.0323646534831894,
0.0682350255366519));
#99177=CARTESIAN_POINT('Ctrl Pts',(0.00771959252974852,-0.0326943950436593,
0.0683317697768151));
#99178=CARTESIAN_POINT('Ctrl Pts',(0.00779977864674937,-0.0325844576448126,
0.0683261992857219));
#99179=CARTESIAN_POINT('Ctrl Pts',(0.00788008564553506,-0.0324744968375318,
0.0683222867807628));
#99180=CARTESIAN_POINT('Ctrl Pts',(0.00796041056295206,-0.0323646534831894,
0.0683200358556498));
#99181=CARTESIAN_POINT('Ctrl Pts',(0.00764824098670485,-0.0326943950436593,
0.0684198043432469));
#99182=CARTESIAN_POINT('Ctrl Pts',(0.00772721382238591,-0.0325844576448126,
0.0684132504941635));
#99183=CARTESIAN_POINT('Ctrl Pts',(0.00780632779144149,-0.0324744968375318,
0.0684083294689736));
#99184=CARTESIAN_POINT('Ctrl Pts',(0.00788548144147433,-0.0323646534831894,
0.0684050461746477));
#99185=CARTESIAN_POINT('Origin',(0.00896000497826417,-0.0326395579068352,
0.0851780226454139));
#99186=CARTESIAN_POINT('Ctrl Pts',(0.00761350612352206,-0.0327445246961877,
0.0684213227239782));
#99187=CARTESIAN_POINT('Ctrl Pts',(0.00782956671684877,-0.0324436878365475,
0.0684020773475949));
#99188=CARTESIAN_POINT('Ctrl Pts',(0.00804646314525272,-0.0321434074463187,
0.0683991612120631));
#99189=CARTESIAN_POINT('Ctrl Pts',(0.00736503292689721,-0.0327445246961877,
0.0684489102312782));
#99190=CARTESIAN_POINT('Ctrl Pts',(0.0075800530403874,-0.0324436878365475,
0.0684202935351815));
#99191=CARTESIAN_POINT('Ctrl Pts',(0.00779661783094262,-0.0321434074463187,
0.0684079543296724));
#99192=CARTESIAN_POINT('Ctrl Pts',(0.00797981580823882,-0.0322357172926635,
0.0684004436101531));
#99193=CARTESIAN_POINT('Ctrl Pts',(0.00816290150188186,-0.0319820232604284,
0.06839585922422));
#99194=CARTESIAN_POINT('Ctrl Pts',(0.00834590794153078,-0.0317296613809579,
0.0684029324736967));
#99195=CARTESIAN_POINT('Ctrl Pts',(0.00773008918797611,-0.0322357172926635,
0.0684121318577619));
#99196=CARTESIAN_POINT('Ctrl Pts',(0.00791280268752697,-0.0319820232604284,
0.0683995953154551));
#99197=CARTESIAN_POINT('Ctrl Pts',(0.00809594362225033,-0.0317296613809579,
0.068398708839402));
#99198=CARTESIAN_POINT('Origin',(0.00895449968112472,-0.0326371942645948,
0.0850828801466654));
#99199=CARTESIAN_POINT('Origin',(0.00942476306524877,-0.0326352985529246,
0.0849909575247938));
#99200=CARTESIAN_POINT('Ctrl Pts',(0.00823919677064608,-0.0321934096636183,
0.0681511101464259));
#99201=CARTESIAN_POINT('Ctrl Pts',(0.00832192613697718,-0.0320835708272303,
0.0681527018033987));
#99202=CARTESIAN_POINT('Ctrl Pts',(0.00840457457765538,-0.0319739230346346,
0.0681560046170822));
#99203=CARTESIAN_POINT('Ctrl Pts',(0.00848703667404713,-0.0318646057455575,
0.0681610062462797));
#99204=CARTESIAN_POINT('Ctrl Pts',(0.00816245817630805,-0.0321934096636183,
0.0682344909170132));
#99205=CARTESIAN_POINT('Ctrl Pts',(0.00824403765682973,-0.0320835708272303,
0.0682350242889637));
#99206=CARTESIAN_POINT('Ctrl Pts',(0.00832555877983254,-0.0319739230346346,
0.0682372456346461));
#99207=CARTESIAN_POINT('Ctrl Pts',(0.00840691746281541,-0.0318646057455575,
0.0682411441072214));
#99208=CARTESIAN_POINT('Ctrl Pts',(0.00808571958197001,-0.0321934096636183,
0.0683178716876005));
#99209=CARTESIAN_POINT('Ctrl Pts',(0.00816614917668227,-0.0320835708272303,
0.0683173467745287));
#99210=CARTESIAN_POINT('Ctrl Pts',(0.0082465429820097,-0.0319739230346346,
0.06831848665221));
#99211=CARTESIAN_POINT('Ctrl Pts',(0.00832679825158368,-0.0318646057455575,
0.0683212819681631));
#99212=CARTESIAN_POINT('Ctrl Pts',(0.00800898098763197,-0.0321934096636183,
0.0684012524581878));
#99213=CARTESIAN_POINT('Ctrl Pts',(0.00808826069653482,-0.0320835708272303,
0.0683996692600936));
#99214=CARTESIAN_POINT('Ctrl Pts',(0.00816752718418686,-0.0319739230346346,
0.0683997276697739));
#99215=CARTESIAN_POINT('Ctrl Pts',(0.00824667904035195,-0.0318646057455575,
0.0684014198291049));
#99216=CARTESIAN_POINT('Ctrl Pts',(0.00788497779667553,-0.0320218834582343,
0.0684042389311222));
#99217=CARTESIAN_POINT('Ctrl Pts',(0.00794477727911326,-0.0319391099350653,
0.0684017535546613));
#99218=CARTESIAN_POINT('Ctrl Pts',(0.00800457934006583,-0.0318564869454948,
0.06840020346133));
#99219=CARTESIAN_POINT('Ctrl Pts',(0.00806434031626076,-0.0317740741446554,
0.0683995857137364));
#99220=CARTESIAN_POINT('Ctrl Pts',(0.00784923828981616,-0.0320218834582343,
0.0683698948530783));
#99221=CARTESIAN_POINT('Ctrl Pts',(0.00790939521108004,-0.0319391099350653,
0.0683670375147507));
#99222=CARTESIAN_POINT('Ctrl Pts',(0.00796956030253236,-0.0318564869454948,
0.0683651212663723));
#99223=CARTESIAN_POINT('Ctrl Pts',(0.00802968961158322,-0.0317740741446554,
0.0683641434125613));
#99224=CARTESIAN_POINT('Ctrl Pts',(0.00781349878295678,-0.0320218834582343,
0.0683355507750344));
#99225=CARTESIAN_POINT('Ctrl Pts',(0.00787401314304682,-0.0319391099350653,
0.0683323214748401));
#99226=CARTESIAN_POINT('Ctrl Pts',(0.00793454126499889,-0.0318564869454948,
0.0683300390714146));
#99227=CARTESIAN_POINT('Ctrl Pts',(0.00799503890690568,-0.0317740741446554,
0.0683287011113862));
#99228=CARTESIAN_POINT('Ctrl Pts',(0.00777775927609741,-0.0320218834582343,
0.0683012066969905));
#99229=CARTESIAN_POINT('Ctrl Pts',(0.0078386310750136,-0.0319391099350653,
0.0682976054349295));
#99230=CARTESIAN_POINT('Ctrl Pts',(0.00789952222746543,-0.0318564869454948,
0.068294956876457));
#99231=CARTESIAN_POINT('Ctrl Pts',(0.00796038820222814,-0.0317740741446554,
0.0682932588102111));
#99232=CARTESIAN_POINT('Origin',(0.00668270788140655,-0.0391228853390711,
0.0621581726514373));
#99233=CARTESIAN_POINT('Ctrl Pts',(0.00499259991127169,-0.0352722978779572,
0.0693250790617349));
#99234=CARTESIAN_POINT('Ctrl Pts',(0.00500863930141557,-0.0352466642097202,
0.0693150875332319));
#99235=CARTESIAN_POINT('Ctrl Pts',(0.00502462294863455,-0.0352210183808294,
0.0693050383604924));
#99236=CARTESIAN_POINT('Ctrl Pts',(0.00504055113353512,-0.0351953608940153,
0.0692949307380702));
#99237=CARTESIAN_POINT('Origin',(0.00255732255140221,-0.0352456003065054,
0.0650731186462026));
#99238=CARTESIAN_POINT('Ctrl Pts',(0.00514727955928602,-0.035024121149334,
0.0692304764243673));
#99239=CARTESIAN_POINT('Ctrl Pts',(0.00521504397640165,-0.0349144232867422,
0.0691894763228488));
#99240=CARTESIAN_POINT('Ctrl Pts',(0.00528369645514265,-0.0348045283677512,
0.0691498524196547));
#99241=CARTESIAN_POINT('Ctrl Pts',(0.00535315094905891,-0.0346945769586886,
0.0691116587402347));
#99242=CARTESIAN_POINT('Ctrl Pts',(0.00503785066805416,-0.035024121149334,
0.0692010407391066));
#99243=CARTESIAN_POINT('Ctrl Pts',(0.00510602054964687,-0.0349144232867422,
0.0691585332995469));
#99244=CARTESIAN_POINT('Ctrl Pts',(0.00517510989330797,-0.0348045283677512,
0.0691174095373373));
#99245=CARTESIAN_POINT('Ctrl Pts',(0.0052450321645086,-0.0346945769586886,
0.0690777254198789));
#99246=CARTESIAN_POINT('Ctrl Pts',(0.0049284217768223,-0.035024121149334,
0.0691716050538458));
#99247=CARTESIAN_POINT('Ctrl Pts',(0.0049969971228921,-0.0349144232867422,
0.0691275902762449));
#99248=CARTESIAN_POINT('Ctrl Pts',(0.00506652333147329,-0.0348045283677512,
0.0690849666550198));
#99249=CARTESIAN_POINT('Ctrl Pts',(0.00513691337995829,-0.0346945769586886,
0.0690437920995231));
#99250=CARTESIAN_POINT('Ctrl Pts',(0.00481899288559044,-0.035024121149334,
0.069142169368585));
#99251=CARTESIAN_POINT('Ctrl Pts',(0.00488797369613732,-0.0349144232867422,
0.069096647252943));
#99252=CARTESIAN_POINT('Ctrl Pts',(0.00495793676963861,-0.0348045283677512,
0.0690525237727024));
#99253=CARTESIAN_POINT('Ctrl Pts',(0.00502879459540797,-0.0346945769586886,
0.0690098587791673));
#99254=CARTESIAN_POINT('Origin',(0.0132846940916072,-0.0345629067942152,
0.0839087386028029));
#99255=CARTESIAN_POINT('Ctrl Pts',(0.00531148955375613,-0.0351970973651657,
0.0689282635179625));
#99256=CARTESIAN_POINT('Ctrl Pts',(0.0053838296360102,-0.0350869349321797,
0.0688893030147748));
#99257=CARTESIAN_POINT('Ctrl Pts',(0.00545703961121713,-0.0349764985129731,
0.0688518141473813));
#99258=CARTESIAN_POINT('Ctrl Pts',(0.00553102749269634,-0.0348659306849633,
0.0688158510668816));
#99259=CARTESIAN_POINT('Ctrl Pts',(0.00529186226377177,-0.0351970973651657,
0.0690081086188657));
#99260=CARTESIAN_POINT('Ctrl Pts',(0.00536309620036208,-0.0350869349321797,
0.0689688762061751));
#99261=CARTESIAN_POINT('Ctrl Pts',(0.00543520476643493,-0.0349764985129731,
0.0689310922078764));
#99262=CARTESIAN_POINT('Ctrl Pts',(0.00550809742472504,-0.0348659306849633,
0.0688948110734243));
#99263=CARTESIAN_POINT('Ctrl Pts',(0.00527223497378742,-0.0351970973651657,
0.069087953719769));
#99264=CARTESIAN_POINT('Ctrl Pts',(0.00534236276471396,-0.0350869349321797,
0.0690484493975753));
#99265=CARTESIAN_POINT('Ctrl Pts',(0.00541336992165274,-0.034976498512973,
0.0690103702683716));
#99266=CARTESIAN_POINT('Ctrl Pts',(0.00548516735675374,-0.0348659306849633,
0.068973771079967));
#99267=CARTESIAN_POINT('Ctrl Pts',(0.00525260768380306,-0.0351970973651657,
0.0691677988206723));
#99268=CARTESIAN_POINT('Ctrl Pts',(0.00532162932906583,-0.0350869349321797,
0.0691280225889755));
#99269=CARTESIAN_POINT('Ctrl Pts',(0.00539153507687054,-0.034976498512973,
0.0690896483288667));
#99270=CARTESIAN_POINT('Ctrl Pts',(0.00546223728878244,-0.0348659306849633,
0.0690527310865096));
#99271=CARTESIAN_POINT('Origin',(0.0128401737970739,-0.0345637187966152,
0.0840923878992216));
#99272=CARTESIAN_POINT('Ctrl Pts',(0.00522295752662561,-0.0352450361861253,
0.0691837799832946));
#99273=CARTESIAN_POINT('Ctrl Pts',(0.00541026158325311,-0.0349452761023765,
0.0690743735885377));
#99274=CARTESIAN_POINT('Ctrl Pts',(0.00560527446589586,-0.0346444289983475,
0.0689793865133844));
#99275=CARTESIAN_POINT('Ctrl Pts',(0.00500987741694025,-0.0352450361861253,
0.0693145349711782));
#99276=CARTESIAN_POINT('Ctrl Pts',(0.00519224996840435,-0.0349452761023765,
0.0691970921284193));
#99277=CARTESIAN_POINT('Ctrl Pts',(0.00538295069390048,-0.0346444289983475,
0.0690937199748283));
#99278=CARTESIAN_POINT('Ctrl Pts',(0.00546205156128212,-0.0345231616327823,
0.0690532882358687));
#99279=CARTESIAN_POINT('Ctrl Pts',(0.00553230255735404,-0.0344132092796976,
0.0690166000265262));
#99280=CARTESIAN_POINT('Ctrl Pts',(0.00560330879546848,-0.0343032738558974,
0.0689813667965672));
#99281=CARTESIAN_POINT('Ctrl Pts',(0.00567497815220558,-0.034193496108874,
0.0689476313536723));
#99282=CARTESIAN_POINT('Ctrl Pts',(0.00535468690281672,-0.0345231616327823,
0.0690170395634645));
#99283=CARTESIAN_POINT('Ctrl Pts',(0.00542543753580368,-0.0344132092796976,
0.0689788714834624));
#99284=CARTESIAN_POINT('Ctrl Pts',(0.00549697399501148,-0.0343032738558974,
0.0689421687937938));
#99285=CARTESIAN_POINT('Ctrl Pts',(0.0055692034295236,-0.034193496108874,
0.0689069761672871));
#99286=CARTESIAN_POINT('Ctrl Pts',(0.00524732224435132,-0.0345231616327823,
0.0689807908910602));
#99287=CARTESIAN_POINT('Ctrl Pts',(0.00531857251425332,-0.0344132092796976,
0.0689411429403985));
#99288=CARTESIAN_POINT('Ctrl Pts',(0.00539063919455449,-0.0343032738558974,
0.0689029707910203));
#99289=CARTESIAN_POINT('Ctrl Pts',(0.00546342870684162,-0.034193496108874,
0.0688663209809019));
#99290=CARTESIAN_POINT('Ctrl Pts',(0.00513995758588592,-0.0345231616327823,
0.0689445422186559));
#99291=CARTESIAN_POINT('Ctrl Pts',(0.00521170749270296,-0.0344132092796976,
0.0689034143973347));
#99292=CARTESIAN_POINT('Ctrl Pts',(0.00528430439409749,-0.0343032738558974,
0.0688637727882469));
#99293=CARTESIAN_POINT('Ctrl Pts',(0.00535765398415964,-0.034193496108874,
0.0688256657945168));
#99294=CARTESIAN_POINT('Origin',(0.0132905727852292,-0.0345625596229409,
0.0839193187370609));
#99295=CARTESIAN_POINT('Ctrl Pts',(0.00567400935308173,-0.0346945769586885,
0.0686729010386621));
#99296=CARTESIAN_POINT('Ctrl Pts',(0.00574948654511411,-0.0345846629176689,
0.0686391419307133));
#99297=CARTESIAN_POINT('Ctrl Pts',(0.00582567475332433,-0.0344746925051586,
0.0686069378939594));
#99298=CARTESIAN_POINT('Ctrl Pts',(0.00590247618618805,-0.0343648066255171,
0.0685763297887621));
#99299=CARTESIAN_POINT('Ctrl Pts',(0.00564007605944396,-0.0346945769586885,
0.0687810197380832));
#99300=CARTESIAN_POINT('Ctrl Pts',(0.0057140633211508,-0.0345846629176689,
0.0687467930121968));
#99301=CARTESIAN_POINT('Ctrl Pts',(0.00578877101469861,-0.0344746925051586,
0.0687140904664878));
#99302=CARTESIAN_POINT('Ctrl Pts',(0.00586410324293113,-0.0343648066255171,
0.0686829536078994));
#99303=CARTESIAN_POINT('Ctrl Pts',(0.00560614276580618,-0.0346945769586885,
0.0688891384375043));
#99304=CARTESIAN_POINT('Ctrl Pts',(0.00567864009718748,-0.0345846629176689,
0.0688544440936803));
#99305=CARTESIAN_POINT('Ctrl Pts',(0.00575186727607289,-0.0344746925051586,
0.0688212430390162));
#99306=CARTESIAN_POINT('Ctrl Pts',(0.00582573029967421,-0.0343648066255171,
0.0687895774270366));
#99307=CARTESIAN_POINT('Ctrl Pts',(0.0055722094721684,-0.0346945769586885,
0.0689972571369253));
#99308=CARTESIAN_POINT('Ctrl Pts',(0.00564321687322416,-0.0345846629176689,
0.0689620951751638));
#99309=CARTESIAN_POINT('Ctrl Pts',(0.00571496353744717,-0.0344746925051586,
0.0689283956115446));
#99310=CARTESIAN_POINT('Ctrl Pts',(0.00578735735641729,-0.0343648066255171,
0.0688962012461739));
#99311=CARTESIAN_POINT('Origin',(0.0128659179646129,-0.0345626446730797,
0.084144841387769));
#99312=CARTESIAN_POINT('Ctrl Pts',(0.00557281665257836,-0.0346945769586886,
0.0689953225308436));
#99313=CARTESIAN_POINT('Ctrl Pts',(0.00568078343598838,-0.0345275153362891,
0.0689418915362472));
#99314=CARTESIAN_POINT('Ctrl Pts',(0.00579045850073889,-0.0343603235965159,
0.0688918421776204));
#99315=CARTESIAN_POINT('Ctrl Pts',(0.00590151527665433,-0.0341934961088741,
0.0688453176577636));
#99316=CARTESIAN_POINT('Ctrl Pts',(0.00549850659352597,-0.0346945769586886,
0.0690341303065451));
#99317=CARTESIAN_POINT('Ctrl Pts',(0.00560566053253615,-0.0345275153362891,
0.0689791428580097));
#99318=CARTESIAN_POINT('Ctrl Pts',(0.00571457149168738,-0.0343603235965159,
0.068927511079657));
#99319=CARTESIAN_POINT('Ctrl Pts',(0.00582491509113088,-0.0341934961088741,
0.0688793828879704));
#99320=CARTESIAN_POINT('Ctrl Pts',(0.00542419653447358,-0.0346945769586886,
0.0690729380822466));
#99321=CARTESIAN_POINT('Ctrl Pts',(0.00553053762908392,-0.0345275153362891,
0.0690163941797723));
#99322=CARTESIAN_POINT('Ctrl Pts',(0.00563868448263588,-0.0343603235965159,
0.0689631799816938));
#99323=CARTESIAN_POINT('Ctrl Pts',(0.00574831490560744,-0.0341934961088741,
0.0689134481181772));
#99324=CARTESIAN_POINT('Ctrl Pts',(0.00534988647542119,-0.0346945769586886,
0.0691117458579481));
#99325=CARTESIAN_POINT('Ctrl Pts',(0.00545541472563169,-0.0345275153362891,
0.0690536455015349));
#99326=CARTESIAN_POINT('Ctrl Pts',(0.00556279747358437,-0.0343603235965159,
0.0689988488837304));
#99327=CARTESIAN_POINT('Ctrl Pts',(0.005671714720084,-0.0341934961088741,
0.068947513348384));
#99328=CARTESIAN_POINT('Ctrl Pts',(0.00578732875098196,-0.0340223579322365,
0.0688962145768071));
#99329=CARTESIAN_POINT('Ctrl Pts',(0.0058597921544147,-0.0339125849573554,
0.0688639887901141));
#99330=CARTESIAN_POINT('Ctrl Pts',(0.005932871637555,-0.0338030433565221,
0.0688332854721777));
#99331=CARTESIAN_POINT('Ctrl Pts',(0.00600647026344122,-0.0336938721132328,
0.0688041356028545));
#99332=CARTESIAN_POINT('Ctrl Pts',(0.00568245183981392,-0.0340223579322365,
0.0688532958939967));
#99333=CARTESIAN_POINT('Ctrl Pts',(0.00575550720381924,-0.0339125849573554,
0.0688196235811683));
#99334=CARTESIAN_POINT('Ctrl Pts',(0.00582920817129801,-0.0338030433565221,
0.0687874870057619));
#99335=CARTESIAN_POINT('Ctrl Pts',(0.00590345684803649,-0.0336938721132328,
0.0687569189100756));
#99336=CARTESIAN_POINT('Ctrl Pts',(0.00557757492864589,-0.0340223579322365,
0.0688103772111864));
#99337=CARTESIAN_POINT('Ctrl Pts',(0.00565122225322378,-0.0339125849573554,
0.0687752583722225));
#99338=CARTESIAN_POINT('Ctrl Pts',(0.00572554470504103,-0.0338030433565221,
0.068741688539346));
#99339=CARTESIAN_POINT('Ctrl Pts',(0.00580044343263177,-0.0336938721132328,
0.0687097022172967));
#99340=CARTESIAN_POINT('Ctrl Pts',(0.00547269801747785,-0.0340223579322365,
0.068767458528376));
#99341=CARTESIAN_POINT('Ctrl Pts',(0.00554693730262832,-0.0339125849573554,
0.0687308931632766));
#99342=CARTESIAN_POINT('Ctrl Pts',(0.00562188123878404,-0.0338030433565221,
0.0686958900729302));
#99343=CARTESIAN_POINT('Ctrl Pts',(0.00569743001722704,-0.0336938721132328,
0.0686624855245177));
#99344=CARTESIAN_POINT('Origin',(0.013236672512422,-0.03455896434161,0.0838118587980092));
#99345=CARTESIAN_POINT('Ctrl Pts',(0.00602275330947995,-0.0341934961088739,
0.0685298863329841));
#99346=CARTESIAN_POINT('Ctrl Pts',(0.00610025134884894,-0.0340836138581106,
0.0685009143888588));
#99347=CARTESIAN_POINT('Ctrl Pts',(0.006178311716794,-0.0339738896643499,
0.0684735600053287));
#99348=CARTESIAN_POINT('Ctrl Pts',(0.00625683215877638,-0.0338644633294062,
0.0684478514953285));
#99349=CARTESIAN_POINT('Ctrl Pts',(0.00598209808651405,-0.0341934961088739,
0.0686356611508401));
#99350=CARTESIAN_POINT('Ctrl Pts',(0.00605813755378216,-0.0340836138581106,
0.0686061285952651));
#99351=CARTESIAN_POINT('Ctrl Pts',(0.00613475165015428,-0.0339738896643499,
0.0685781836871882));
#99352=CARTESIAN_POINT('Ctrl Pts',(0.00621183992147581,-0.0338644633294062,
0.0685518556194274));
#99353=CARTESIAN_POINT('Ctrl Pts',(0.00594144286354814,-0.0341934961088739,
0.0687414359686961));
#99354=CARTESIAN_POINT('Ctrl Pts',(0.00601602375871537,-0.0340836138581106,
0.0687113428016715));
#99355=CARTESIAN_POINT('Ctrl Pts',(0.00609119158351456,-0.0339738896643499,
0.0686828073690477));
#99356=CARTESIAN_POINT('Ctrl Pts',(0.00616684768417524,-0.0338644633294062,
0.0686558597435262));
#99357=CARTESIAN_POINT('Ctrl Pts',(0.00590078764058223,-0.0341934961088739,
0.0688472107865521));
#99358=CARTESIAN_POINT('Ctrl Pts',(0.00597390996364859,-0.0340836138581106,
0.0688165570080778));
#99359=CARTESIAN_POINT('Ctrl Pts',(0.00604763151687485,-0.0339738896643499,
0.0687874310509072));
#99360=CARTESIAN_POINT('Ctrl Pts',(0.00612185544687467,-0.0338644633294062,
0.068759863867625));
#99361=CARTESIAN_POINT('Origin',(0.0128346846475394,-0.0345610621862508,
0.0840763503254826));
#99362=CARTESIAN_POINT('Ctrl Pts',(0.00586819159598038,-0.0342436276873901,
0.0688594011626142));
#99363=CARTESIAN_POINT('Ctrl Pts',(0.00606772982055773,-0.0339430054201861,
0.068774330160832));
#99364=CARTESIAN_POINT('Ctrl Pts',(0.00627310907437932,-0.0336441434784163,
0.0687045308735047));
#99365=CARTESIAN_POINT('Ctrl Pts',(0.00564040514730526,-0.0342436276873901,
0.06896242219833));
#99366=CARTESIAN_POINT('Ctrl Pts',(0.00583605786946734,-0.0339430054201861,
0.06886876008901));
#99367=CARTESIAN_POINT('Ctrl Pts',(0.00603820977659939,-0.0336441434784163,
0.0687901014286185));
#99368=CARTESIAN_POINT('Ctrl Pts',(0.00612182949496901,-0.0335235895815127,
0.0687598736413807));
#99369=CARTESIAN_POINT('Ctrl Pts',(0.00619603519647663,-0.0334144449262719,
0.0687323128210091));
#99370=CARTESIAN_POINT('Ctrl Pts',(0.00627089553715207,-0.0333049234473132,
0.068706253370541));
#99371=CARTESIAN_POINT('Ctrl Pts',(0.00634631781205715,-0.0331951640388588,
0.068681737283052));
#99372=CARTESIAN_POINT('Ctrl Pts',(0.0060198544725169,-0.0335235895815127,
0.0687104543406756));
#99373=CARTESIAN_POINT('Ctrl Pts',(0.00609474052799637,-0.0334144449262719,
0.0686814896333496));
#99374=CARTESIAN_POINT('Ctrl Pts',(0.00617031100753587,-0.0333049234473132,
0.0686540387386321));
#99375=CARTESIAN_POINT('Ctrl Pts',(0.00624647245931801,-0.0331951640388588,
0.0686281455110838));
#99376=CARTESIAN_POINT('Ctrl Pts',(0.00591787945006479,-0.0335235895815127,
0.0686610350399705));
#99377=CARTESIAN_POINT('Ctrl Pts',(0.00599344585951611,-0.0334144449262719,
0.06863066644569));
#99378=CARTESIAN_POINT('Ctrl Pts',(0.00606972647791968,-0.0333049234473132,
0.0686018241067232));
#99379=CARTESIAN_POINT('Ctrl Pts',(0.00614662710657887,-0.0331951640388588,
0.0685745537391156));
#99380=CARTESIAN_POINT('Ctrl Pts',(0.00581590442761268,-0.0335235895815127,
0.0686116157392653));
#99381=CARTESIAN_POINT('Ctrl Pts',(0.00589215119103584,-0.0334144449262719,
0.0685798432580305));
#99382=CARTESIAN_POINT('Ctrl Pts',(0.00596914194830348,-0.0333049234473132,
0.0685496094748143));
#99383=CARTESIAN_POINT('Ctrl Pts',(0.00604678175383973,-0.0331951640388588,
0.0685209619671475));
#99384=CARTESIAN_POINT('Origin',(0.0107693667188908,-0.032643457177125,
0.0847511952527698));
#99385=CARTESIAN_POINT('Ctrl Pts',(0.00638063389637515,-0.0336938721132356,
0.0684072084706003));
#99386=CARTESIAN_POINT('Ctrl Pts',(0.00641424836085578,-0.0336474569764941,
0.068397005245182));
#99387=CARTESIAN_POINT('Ctrl Pts',(0.00644797996368787,-0.033601104548885,
0.0683871962186434));
#99388=CARTESIAN_POINT('Ctrl Pts',(0.00653338061926225,-0.0334837508694588,
0.0683623620208405));
#99389=CARTESIAN_POINT('Ctrl Pts',(0.00661947966187594,-0.0333660264863562,
0.0683400693266549));
#99390=CARTESIAN_POINT('Ctrl Pts',(0.00623898417299042,-0.0336938721132356,
0.0687162479424104));
#99391=CARTESIAN_POINT('Ctrl Pts',(0.00627078972689244,-0.0336474569764941,
0.0687052155941567));
#99392=CARTESIAN_POINT('Ctrl Pts',(0.00630272224902327,-0.033601104548885,
0.0686945563260126));
#99393=CARTESIAN_POINT('Ctrl Pts',(0.00638356804629211,-0.0334837508694588,
0.0686675695121342));
#99394=CARTESIAN_POINT('Ctrl Pts',(0.00646517801722987,-0.0333660264863562,
0.0686429901772596));
#99395=CARTESIAN_POINT('Ctrl Pts',(0.00623898417300239,-0.0336938721132427,
0.0687162479424196));
#99396=CARTESIAN_POINT('Ctrl Pts',(0.00627078972690343,-0.0336474569765026,
0.0687052155941663));
#99397=CARTESIAN_POINT('Ctrl Pts',(0.00630272224903327,-0.0336011045488949,
0.0686945563260226));
#99398=CARTESIAN_POINT('Ctrl Pts',(0.00638289471091717,-0.033484728265791,
0.0686677942755497));
#99399=CARTESIAN_POINT('Ctrl Pts',(0.00646381896393862,-0.0333679870047995,
0.0686433996805959));
#99400=CARTESIAN_POINT('Ctrl Pts',(0.0062389841729857,-0.0336938721132425,
0.068716247942412));
#99401=CARTESIAN_POINT('Ctrl Pts',(0.00635273490910074,-0.0335278710435083,
0.0686767913827558));
#99402=CARTESIAN_POINT('Ctrl Pts',(0.00646768297542329,-0.033362046922432,
0.0686409158973354));
#99403=CARTESIAN_POINT('Ctrl Pts',(0.00658389150603253,-0.0331951640388601,
0.0686086227639821));
#99404=CARTESIAN_POINT('Ctrl Pts',(0.00616039615858634,-0.0336938721132425,
0.0687454361903217));
#99405=CARTESIAN_POINT('Ctrl Pts',(0.00627353586485489,-0.0335278710435083,
0.0687043344609204));
#99406=CARTESIAN_POINT('Ctrl Pts',(0.00638792470838529,-0.033362046922432,
0.0686667952227847));
#99407=CARTESIAN_POINT('Ctrl Pts',(0.00650362582187743,-0.0331951640388601,
0.068632818833299));
#99408=CARTESIAN_POINT('Ctrl Pts',(0.00608180814418698,-0.0336938721132425,
0.0687746244382315));
#99409=CARTESIAN_POINT('Ctrl Pts',(0.00619433682060903,-0.0335278710435083,
0.0687318775390851));
#99410=CARTESIAN_POINT('Ctrl Pts',(0.00630816644134729,-0.033362046922432,
0.0686926745482339));
#99411=CARTESIAN_POINT('Ctrl Pts',(0.00642336013772234,-0.0331951640388601,
0.0686570149026159));
#99412=CARTESIAN_POINT('Ctrl Pts',(0.00600322012978762,-0.0336938721132425,
0.0688038126861412));
#99413=CARTESIAN_POINT('Ctrl Pts',(0.00611513777636318,-0.0335278710435083,
0.0687594206172497));
#99414=CARTESIAN_POINT('Ctrl Pts',(0.00622840817430929,-0.033362046922432,
0.0687185538736831));
#99415=CARTESIAN_POINT('Ctrl Pts',(0.00634309445356724,-0.0331951640388601,
0.0686812109719328));
#99416=CARTESIAN_POINT('Ctrl Pts',(0.00646422742317616,-0.0330240426238155,
0.068644806202726));
#99417=CARTESIAN_POINT('Ctrl Pts',(0.00654006683118363,-0.0329142774063509,
0.0686219442189445));
#99418=CARTESIAN_POINT('Ctrl Pts',(0.00661641666896846,-0.0328043479726686,
0.0686006386500407));
#99419=CARTESIAN_POINT('Ctrl Pts',(0.00669317987837464,-0.0326943950436594,
0.0685809194837004));
#99420=CARTESIAN_POINT('Ctrl Pts',(0.00636555682001553,-0.0330240426238155,
0.0685890814500886));
#99421=CARTESIAN_POINT('Ctrl Pts',(0.00644216389078057,-0.0329142774063509,
0.0685648601826184));
#99422=CARTESIAN_POINT('Ctrl Pts',(0.00651930987422167,-0.0328043479726686,
0.068542210522107));
#99423=CARTESIAN_POINT('Ctrl Pts',(0.00659689673968124,-0.0326943950436594,
0.0685211642062102));
#99424=CARTESIAN_POINT('Ctrl Pts',(0.00626688621685489,-0.0330240426238155,
0.0685333566974512));
#99425=CARTESIAN_POINT('Ctrl Pts',(0.00634426095037751,-0.0329142774063509,
0.0685077761462924));
#99426=CARTESIAN_POINT('Ctrl Pts',(0.00642220307947488,-0.0328043479726686,
0.0684837823941734));
#99427=CARTESIAN_POINT('Ctrl Pts',(0.00650061360098785,-0.0326943950436594,
0.06846140892872));
#99428=CARTESIAN_POINT('Ctrl Pts',(0.00616821561369426,-0.0330240426238155,
0.0684776319448138));
#99429=CARTESIAN_POINT('Ctrl Pts',(0.00624635800997445,-0.0329142774063509,
0.0684506921099663));
#99430=CARTESIAN_POINT('Ctrl Pts',(0.00632509628472809,-0.0328043479726686,
0.0684253542662398));
#99431=CARTESIAN_POINT('Ctrl Pts',(0.00640433046229446,-0.0326943950436594,
0.0684016536512298));
#99432=CARTESIAN_POINT('Origin',(0.0108019857363915,-0.0326396682856121,
0.0848704906776846));
#99433=CARTESIAN_POINT('Ctrl Pts',(0.00674370756866024,-0.0331951640388587,
0.0683108738640981));
#99434=CARTESIAN_POINT('Ctrl Pts',(0.00682412971872628,-0.0330855618255041,
0.0682918661280146));
#99435=CARTESIAN_POINT('Ctrl Pts',(0.00690500270140994,-0.0329757224427708,
0.0682745068778918));
#99436=CARTESIAN_POINT('Ctrl Pts',(0.00698622404440808,-0.0328657862078596,
0.0682588234232589));
#99437=CARTESIAN_POINT('Ctrl Pts',(0.00669011583935863,-0.0331951640388587,
0.0684107191373463));
#99438=CARTESIAN_POINT('Ctrl Pts',(0.00676916282277103,-0.0330855618255041,
0.0683909732836069));
#99439=CARTESIAN_POINT('Ctrl Pts',(0.00684867490309286,-0.0329757224427708,
0.0683728469613853));
#99440=CARTESIAN_POINT('Ctrl Pts',(0.00692855139892115,-0.0328657862078596,
0.0683563683770089));
#99441=CARTESIAN_POINT('Ctrl Pts',(0.00663652411005703,-0.0331951640388587,
0.0685105644105946));
#99442=CARTESIAN_POINT('Ctrl Pts',(0.00671419592681577,-0.0330855618255041,
0.0684900804391991));
#99443=CARTESIAN_POINT('Ctrl Pts',(0.00679234710477578,-0.0329757224427708,
0.0684711870448789));
#99444=CARTESIAN_POINT('Ctrl Pts',(0.00687087875343423,-0.0328657862078596,
0.0684539133307588));
#99445=CARTESIAN_POINT('Ctrl Pts',(0.00658293238075542,-0.0331951640388587,
0.0686104096838428));
#99446=CARTESIAN_POINT('Ctrl Pts',(0.00665922903086051,-0.0330855618255041,
0.0685891875947914));
#99447=CARTESIAN_POINT('Ctrl Pts',(0.00673601930645869,-0.0329757224427708,
0.0685695271283724));
#99448=CARTESIAN_POINT('Ctrl Pts',(0.00681320610794731,-0.0328657862078596,
0.0685514582845088));
#99449=CARTESIAN_POINT('Origin',(0.0103275744650057,-0.0326401908832347,
0.0849492740342608));
#99450=CARTESIAN_POINT('Ctrl Pts',(0.00654913516136936,-0.0332451089994432,
0.0686183988099795));
#99451=CARTESIAN_POINT('Ctrl Pts',(0.00675776291357944,-0.0329451141710258,
0.0685590100255262));
#99452=CARTESIAN_POINT('Ctrl Pts',(0.00697027138239242,-0.0326442513127503,
0.0685155046535149));
#99453=CARTESIAN_POINT('Ctrl Pts',(0.0063102319892303,-0.0332451089994432,
0.0686920552716233));
#99454=CARTESIAN_POINT('Ctrl Pts',(0.00651608174253904,-0.0329451141710258,
0.0686236561066152));
#99455=CARTESIAN_POINT('Ctrl Pts',(0.00672649880315049,-0.0326442513127503,
0.0685709567013557));
#99456=CARTESIAN_POINT('Ctrl Pts',(0.00681317533143831,-0.0325229783203385,
0.068551465396958));
#99457=CARTESIAN_POINT('Ctrl Pts',(0.00689035100710463,-0.0324130253112079,
0.0685333987103598));
#99458=CARTESIAN_POINT('Ctrl Pts',(0.00696788871018158,-0.0323031222247695,
0.0685169312418898));
#99459=CARTESIAN_POINT('Ctrl Pts',(0.00704568837606189,-0.0321934096636184,
0.0685020805805181));
#99460=CARTESIAN_POINT('Ctrl Pts',(0.00671819838379667,-0.0325229783203385,
0.0684896550251256));
#99461=CARTESIAN_POINT('Ctrl Pts',(0.00679622611407149,-0.0324130253112079,
0.068470279083405));
#99462=CARTESIAN_POINT('Ctrl Pts',(0.00687464282614974,-0.0323031222247695,
0.0684525201842307));
#99463=CARTESIAN_POINT('Ctrl Pts',(0.00695334727110378,-0.0321934096636184,
0.0684363975310723));
#99464=CARTESIAN_POINT('Ctrl Pts',(0.00662322143615504,-0.0325229783203385,
0.0684278446532933));
#99465=CARTESIAN_POINT('Ctrl Pts',(0.00670210122103835,-0.0324130253112079,
0.0684071594564503));
#99466=CARTESIAN_POINT('Ctrl Pts',(0.0067813969421179,-0.0323031222247695,
0.0683881091265715));
#99467=CARTESIAN_POINT('Ctrl Pts',(0.00686100616614567,-0.0321934096636184,
0.0683707144816266));
#99468=CARTESIAN_POINT('Ctrl Pts',(0.00652824448851341,-0.0325229783203385,
0.068366034281461));
#99469=CARTESIAN_POINT('Ctrl Pts',(0.00660797632800521,-0.0324130253112079,
0.0683440398294956));
#99470=CARTESIAN_POINT('Ctrl Pts',(0.00668815105808605,-0.0323031222247695,
0.0683236980689124));
#99471=CARTESIAN_POINT('Ctrl Pts',(0.00676866506118755,-0.0321934096636184,
0.0683050314321809));
#99472=CARTESIAN_POINT('Origin',(0.0108001514141797,-0.0326393375178216,
0.0848621644365802));
#99473=CARTESIAN_POINT('Ctrl Pts',(0.00711307259435396,-0.0326943950436593,
0.0682357404430475));
#99474=CARTESIAN_POINT('Ctrl Pts',(0.00719458217555229,-0.0325844576448127,
0.068221810970505));
#99475=CARTESIAN_POINT('Ctrl Pts',(0.00727638560964018,-0.0324744968375319,
0.0682095662639281));
#99476=CARTESIAN_POINT('Ctrl Pts',(0.00735837786889389,-0.0323646534831894,
0.0681990205662855));
#99477=CARTESIAN_POINT('Ctrl Pts',(0.00705331733641517,-0.0326943950436593,
0.0683320235502378));
#99478=CARTESIAN_POINT('Ctrl Pts',(0.00713349995594264,-0.0325844576448127,
0.0683172705382477));
#99479=CARTESIAN_POINT('Ctrl Pts',(0.00721399336659453,-0.0324744968375319,
0.068304174790197));
#99480=CARTESIAN_POINT('Ctrl Pts',(0.00729469420408556,-0.0323646534831894,
0.0682927516626098));
#99481=CARTESIAN_POINT('Ctrl Pts',(0.00699356207847638,-0.0326943950436593,
0.0684283066574282));
#99482=CARTESIAN_POINT('Ctrl Pts',(0.007072417736333,-0.0325844576448127,
0.0684127301059904));
#99483=CARTESIAN_POINT('Ctrl Pts',(0.00715160112354887,-0.0324744968375319,
0.0683987833164659));
#99484=CARTESIAN_POINT('Ctrl Pts',(0.00723101053927724,-0.0323646534831894,
0.068386482758934));
#99485=CARTESIAN_POINT('Ctrl Pts',(0.00693380682053759,-0.0326943950436593,
0.0685245897646186));
#99486=CARTESIAN_POINT('Ctrl Pts',(0.00701133551672335,-0.0325844576448127,
0.0685081896737331));
#99487=CARTESIAN_POINT('Ctrl Pts',(0.00708920888050322,-0.0324744968375319,
0.0684933918427348));
#99488=CARTESIAN_POINT('Ctrl Pts',(0.00716732687446891,-0.0323646534831894,
0.0684802138552583));
#99489=CARTESIAN_POINT('Origin',(0.0103355888499022,-0.0326395579068055,
0.0849862568880412));
#99490=CARTESIAN_POINT('Ctrl Pts',(0.00689953615569267,-0.0327445246961877,
0.0685304496051844));
#99491=CARTESIAN_POINT('Ctrl Pts',(0.00711148096145355,-0.0324436878365475,
0.0684842764115347));
#99492=CARTESIAN_POINT('Ctrl Pts',(0.00732630160803998,-0.0321434074463187,
0.0684541989398822));
#99493=CARTESIAN_POINT('Ctrl Pts',(0.00665647987593443,-0.0327445246961877,
0.0685889615259362));
#99494=CARTESIAN_POINT('Ctrl Pts',(0.00686621786855063,-0.0324436878365475,
0.0685336213149307));
#99495=CARTESIAN_POINT('Ctrl Pts',(0.00707952846852147,-0.0321434074463187,
0.068494236642266));
#99496=CARTESIAN_POINT('Ctrl Pts',(0.00726033554411033,-0.0322357242816072,
0.0684638251095895));
#99497=CARTESIAN_POINT('Ctrl Pts',(0.00744143283967124,-0.0319819883628706,
0.0684363254536683));
#99498=CARTESIAN_POINT('Ctrl Pts',(0.00762391300086686,-0.0317295851069886,
0.0684204052682019));
#99499=CARTESIAN_POINT('Ctrl Pts',(0.00701404305633529,-0.0322357242816072,
0.0685067204527584));
#99500=CARTESIAN_POINT('Ctrl Pts',(0.00719377419084949,-0.0319819883628706,
0.0684713767005311));
#99501=CARTESIAN_POINT('Ctrl Pts',(0.00737539010198121,-0.0317295851069886,
0.0684475413830576));
#99502=CARTESIAN_POINT('Origin',(0.0103182024466775,-0.0326371942646543,
0.0848925546125099));
#99503=CARTESIAN_POINT('Origin',(0.0107732367041174,-0.0326352985529337,
0.0847424171978103));
#99504=CARTESIAN_POINT('Ctrl Pts',(0.00748642642908508,-0.0321934096636183,
0.0681839479024995));
#99505=CARTESIAN_POINT('Ctrl Pts',(0.00756870293716775,-0.0320835708272304,
0.0681751582697888));
#99506=CARTESIAN_POINT('Ctrl Pts',(0.00765111362252414,-0.0319739230346346,
0.0681680764434806));
#99507=CARTESIAN_POINT('Ctrl Pts',(0.00773355235101604,-0.0318646057455575,
0.0681627033921506));
#99508=CARTESIAN_POINT('Ctrl Pts',(0.00742074332307886,-0.0321934096636183,
0.0682762890869737));
#99509=CARTESIAN_POINT('Ctrl Pts',(0.00750174637426129,-0.0320835708272304,
0.0682665936330409));
#99510=CARTESIAN_POINT('Ctrl Pts',(0.00758290308729731,-0.0319739230346346,
0.0682585801567993));
#99511=CARTESIAN_POINT('Ctrl Pts',(0.00766410884093803,-0.0318646057455575,
0.0682522509419371));
#99512=CARTESIAN_POINT('Ctrl Pts',(0.00735506021707264,-0.0321934096636183,
0.0683686302714479));
#99513=CARTESIAN_POINT('Ctrl Pts',(0.00743478981135483,-0.0320835708272304,
0.0683580289962929));
#99514=CARTESIAN_POINT('Ctrl Pts',(0.00751469255207047,-0.0319739230346346,
0.0683490838701181));
#99515=CARTESIAN_POINT('Ctrl Pts',(0.00759466533086003,-0.0318646057455575,
0.0683417984917237));
#99516=CARTESIAN_POINT('Ctrl Pts',(0.00728937711106641,-0.0321934096636183,
0.0684609714559222));
#99517=CARTESIAN_POINT('Ctrl Pts',(0.00736783324844837,-0.0320835708272304,
0.068449464359545));
#99518=CARTESIAN_POINT('Ctrl Pts',(0.00744648201684363,-0.0319739230346346,
0.0684395875834368));
#99519=CARTESIAN_POINT('Ctrl Pts',(0.00752522182078202,-0.0318646057455575,
0.0684313460415102));
#99520=CARTESIAN_POINT('Ctrl Pts',(0.007166726026618,-0.032021883458235,
0.0684794761005202));
#99521=CARTESIAN_POINT('Ctrl Pts',(0.00722574247200713,-0.0319391099350658,
0.0684695154594957));
#99522=CARTESIAN_POINT('Ctrl Pts',(0.00728487869763767,-0.0318564869454951,
0.0684604824034403));
#99523=CARTESIAN_POINT('Ctrl Pts',(0.00734409101638228,-0.0317740741446555,
0.0684523794905836));
#99524=CARTESIAN_POINT('Ctrl Pts',(0.00712696388209023,-0.032021883458235,
0.0684498821837506));
#99525=CARTESIAN_POINT('Ctrl Pts',(0.00718628832861009,-0.0319391099350658,
0.0684395077149259));
#99526=CARTESIAN_POINT('Ctrl Pts',(0.00724573883074043,-0.0318564869454951,
0.0684300658912789));
#99527=CARTESIAN_POINT('Ctrl Pts',(0.00730527144464972,-0.0317740741446555,
0.068421559547402));
#99528=CARTESIAN_POINT('Ctrl Pts',(0.00708720173756246,-0.032021883458235,
0.068420288266981));
#99529=CARTESIAN_POINT('Ctrl Pts',(0.00714683418521306,-0.0319391099350658,
0.0684094999703561));
#99530=CARTESIAN_POINT('Ctrl Pts',(0.00720659896384319,-0.0318564869454951,
0.0683996493791175));
#99531=CARTESIAN_POINT('Ctrl Pts',(0.00726645187291716,-0.0317740741446555,
0.0683907396042204));
#99532=CARTESIAN_POINT('Ctrl Pts',(0.00704743959303469,-0.032021883458235,
0.0683906943502114));
#99533=CARTESIAN_POINT('Ctrl Pts',(0.00710738004181602,-0.0319391099350658,
0.0683794922257863));
#99534=CARTESIAN_POINT('Ctrl Pts',(0.00716745909694595,-0.0318564869454951,
0.0683692328669562));
#99535=CARTESIAN_POINT('Ctrl Pts',(0.0072276323011846,-0.0317740741446555,
0.0683599196610388));
#99536=CARTESIAN_POINT('Origin',(0.00519109668483847,-0.0391228853390555,
0.0624333462951897));
#99537=CARTESIAN_POINT('Ctrl Pts',(0.0044125672759175,-0.0352722978779579,
0.0697555662047294));
#99538=CARTESIAN_POINT('Ctrl Pts',(0.00442722792010397,-0.0352466642097207,
0.0697436431937817));
#99539=CARTESIAN_POINT('Ctrl Pts',(0.00444182603617658,-0.0352210183808296,
0.0697316699795806));
#99540=CARTESIAN_POINT('Ctrl Pts',(0.00445636180158001,-0.0351953608940152,
0.0697196457278616));
#99541=CARTESIAN_POINT('Origin',(0.0014635808575311,-0.0352456003065056,
0.0658423549531952));
#99542=CARTESIAN_POINT('Ctrl Pts',(0.00455417037426209,-0.035024121149334,
0.0696423230369613));
#99543=CARTESIAN_POINT('Ctrl Pts',(0.00461626177340869,-0.0349144232867422,
0.0695931530999717));
#99544=CARTESIAN_POINT('Ctrl Pts',(0.00467940671493554,-0.0348045283677513,
0.0695452372059366));
#99545=CARTESIAN_POINT('Ctrl Pts',(0.00474352660207877,-0.0346945769586887,
0.0694986397387786));
#99546=CARTESIAN_POINT('Ctrl Pts',(0.00444191509290649,-0.035024121149334,
0.0696268345376543));
#99547=CARTESIAN_POINT('Ctrl Pts',(0.00450421983977089,-0.0349144232867422,
0.0695761183302601));
#99548=CARTESIAN_POINT('Ctrl Pts',(0.00456761021922716,-0.0348045283677513,
0.0695266596503528));
#99549=CARTESIAN_POINT('Ctrl Pts',(0.00463200739367237,-0.0346945769586887,
0.0694785248696659));
#99550=CARTESIAN_POINT('Ctrl Pts',(0.00432965981155089,-0.035024121149334,
0.0696113460383472));
#99551=CARTESIAN_POINT('Ctrl Pts',(0.00439217790613309,-0.0349144232867422,
0.0695590835605486));
#99552=CARTESIAN_POINT('Ctrl Pts',(0.00445581372351877,-0.0348045283677513,
0.069508082094769));
#99553=CARTESIAN_POINT('Ctrl Pts',(0.00452048818526597,-0.0346945769586887,
0.0694584100005532));
#99554=CARTESIAN_POINT('Ctrl Pts',(0.00421740453019528,-0.035024121149334,
0.0695958575390402));
#99555=CARTESIAN_POINT('Ctrl Pts',(0.00428013597249529,-0.0349144232867422,
0.069542048790837));
#99556=CARTESIAN_POINT('Ctrl Pts',(0.00434401722781038,-0.0348045283677513,
0.0694895045391852));
#99557=CARTESIAN_POINT('Ctrl Pts',(0.00440896897685957,-0.0346945769586887,
0.0694382951314405));
#99558=CARTESIAN_POINT('Origin',(0.0144670930243381,-0.0345629067941596,
0.0831849542577961));
#99559=CARTESIAN_POINT('Ctrl Pts',(0.00467920820309421,-0.0351970973651654,
0.0693219121999994));
#99560=CARTESIAN_POINT('Ctrl Pts',(0.00474609481634698,-0.0350869349321794,
0.0692741922955912));
#99561=CARTESIAN_POINT('Ctrl Pts',(0.00481402890805956,-0.0349764985129727,
0.0692278233961926));
#99562=CARTESIAN_POINT('Ctrl Pts',(0.00488292600382625,-0.034865930684963,
0.069182870754894));
#99563=CARTESIAN_POINT('Ctrl Pts',(0.00466974292483447,-0.0351970973651654,
0.0694035876501514));
#99564=CARTESIAN_POINT('Ctrl Pts',(0.0047354980354152,-0.0350869349321794,
0.0693557366171406));
#99565=CARTESIAN_POINT('Ctrl Pts',(0.00480230241322307,-0.0349764985129727,
0.0693092129572004));
#99566=CARTESIAN_POINT('Ctrl Pts',(0.00487007305923235,-0.034865930684963,
0.0692640820377635));
#99567=CARTESIAN_POINT('Ctrl Pts',(0.00466027764657473,-0.0351970973651654,
0.0694852631003033));
#99568=CARTESIAN_POINT('Ctrl Pts',(0.00472490125448342,-0.0350869349321794,
0.06943728093869));
#99569=CARTESIAN_POINT('Ctrl Pts',(0.00479057591838658,-0.0349764985129727,
0.0693906025182083));
#99570=CARTESIAN_POINT('Ctrl Pts',(0.00485722011463844,-0.034865930684963,
0.0693452933206331));
#99571=CARTESIAN_POINT('Ctrl Pts',(0.00465081236831499,-0.0351970973651654,
0.0695669385504553));
#99572=CARTESIAN_POINT('Ctrl Pts',(0.00471430447355164,-0.0350869349321794,
0.0695188252602393));
#99573=CARTESIAN_POINT('Ctrl Pts',(0.0047788494235501,-0.0349764985129727,
0.0694719920792162));
#99574=CARTESIAN_POINT('Ctrl Pts',(0.00484436717004454,-0.034865930684963,
0.0694265046035027));
#99575=CARTESIAN_POINT('Origin',(0.0140490952653582,-0.0345637187966762,
0.0834228685904193));
#99576=CARTESIAN_POINT('Ctrl Pts',(0.00462339898226972,-0.0352450361861252,
0.0695865098469176));
#99577=CARTESIAN_POINT('Ctrl Pts',(0.0047955138332382,-0.0349452761023765,
0.0694544907311847));
#99578=CARTESIAN_POINT('Ctrl Pts',(0.00497708394377801,-0.0346444289983475,
0.069335811062322));
#99579=CARTESIAN_POINT('Ctrl Pts',(0.0044283870183293,-0.0352450361861252,
0.0697429398118224));
#99580=CARTESIAN_POINT('Ctrl Pts',(0.0045946020165111,-0.0349452761023765,
0.0696035656993688));
#99581=CARTESIAN_POINT('Ctrl Pts',(0.00477084304355708,-0.0346444289983475,
0.069477107527515));
#99582=CARTESIAN_POINT('Ctrl Pts',(0.00484425273639071,-0.0345231616327822,
0.0694270806374069));
#99583=CARTESIAN_POINT('Ctrl Pts',(0.00490935153046505,-0.0344132092796975,
0.0693818769410545));
#99584=CARTESIAN_POINT('Ctrl Pts',(0.00497538196854374,-0.0343032738558974,
0.0693380220942112));
#99585=CARTESIAN_POINT('Ctrl Pts',(0.00504225801885261,-0.0341934961088741,
0.0692955701131324));
#99586=CARTESIAN_POINT('Ctrl Pts',(0.00473319151700071,-0.0345231616327822,
0.0694045741564275));
#99587=CARTESIAN_POINT('Ctrl Pts',(0.00479860053122876,-0.0344132092796975,
0.0693578396375275));
#99588=CARTESIAN_POINT('Ctrl Pts',(0.00486497283731212,-0.0343032738558974,
0.0693124604637792));
#99589=CARTESIAN_POINT('Ctrl Pts',(0.00493222191548151,-0.0341934961088741,
0.0692684925930581));
#99590=CARTESIAN_POINT('Ctrl Pts',(0.00462213029761071,-0.0345231616327822,
0.0693820676754481));
#99591=CARTESIAN_POINT('Ctrl Pts',(0.00468784953199247,-0.0344132092796975,
0.0693338023340005));
#99592=CARTESIAN_POINT('Ctrl Pts',(0.00475456370608051,-0.0343032738558974,
0.0692868988333472));
#99593=CARTESIAN_POINT('Ctrl Pts',(0.00482218581211042,-0.0341934961088741,
0.0692414150729838));
#99594=CARTESIAN_POINT('Ctrl Pts',(0.00451106907822071,-0.0345231616327822,
0.0693595611944686));
#99595=CARTESIAN_POINT('Ctrl Pts',(0.00457709853275618,-0.0344132092796975,
0.0693097650304734));
#99596=CARTESIAN_POINT('Ctrl Pts',(0.00464415457484889,-0.0343032738558974,
0.0692613372029152));
#99597=CARTESIAN_POINT('Ctrl Pts',(0.00471214970873932,-0.0341934961088741,
0.0692143375529095));
#99598=CARTESIAN_POINT('Origin',(0.0144742514056604,-0.034562559623074,
0.0831947141691753));
#99599=CARTESIAN_POINT('Ctrl Pts',(0.00500686402026084,-0.0346945769586885,
0.0690231275514409));
#99600=CARTESIAN_POINT('Ctrl Pts',(0.00507751491392863,-0.034584662917669,
0.0689801748436039));
#99601=CARTESIAN_POINT('Ctrl Pts',(0.0051490661193006,-0.0344746925051586,
0.0689386758308042));
#99602=CARTESIAN_POINT('Ctrl Pts',(0.00522142573712908,-0.0343648066255171,
0.0688986833077355));
#99603=CARTESIAN_POINT('Ctrl Pts',(0.00498674916698599,-0.0346945769586885,
0.0691346466720407));
#99604=CARTESIAN_POINT('Ctrl Pts',(0.00505586327080568,-0.034584662917669,
0.0690914167713586));
#99605=CARTESIAN_POINT('Ctrl Pts',(0.00512588315607627,-0.0344746925051586,
0.0690496087381858));
#99606=CARTESIAN_POINT('Ctrl Pts',(0.00519671888401862,-0.0343648066255171,
0.0690092757712716));
#99607=CARTESIAN_POINT('Ctrl Pts',(0.00496663431371114,-0.0346945769586885,
0.0692461657926404));
#99608=CARTESIAN_POINT('Ctrl Pts',(0.00503421162768274,-0.034584662917669,
0.0692026586991134));
#99609=CARTESIAN_POINT('Ctrl Pts',(0.00510270019285194,-0.0344746925051586,
0.0691605416455675));
#99610=CARTESIAN_POINT('Ctrl Pts',(0.00517201203090817,-0.0343648066255171,
0.0691198682348077));
#99611=CARTESIAN_POINT('Ctrl Pts',(0.00494651946043629,-0.0346945769586885,
0.0693576849132402));
#99612=CARTESIAN_POINT('Ctrl Pts',(0.0050125599845598,-0.034584662917669,
0.0693139006268682));
#99613=CARTESIAN_POINT('Ctrl Pts',(0.00507951722962762,-0.0344746925051586,
0.0692714745529491));
#99614=CARTESIAN_POINT('Ctrl Pts',(0.00514730517779772,-0.0343648066255171,
0.0692304606983438));
#99615=CARTESIAN_POINT('Origin',(0.0140812105975753,-0.0345626446730884,
0.083471681867596));
#99616=CARTESIAN_POINT('Ctrl Pts',(0.00494687938261152,-0.0346945769586885,
0.069355689462221));
#99617=CARTESIAN_POINT('Ctrl Pts',(0.00504729813636091,-0.0345275153362891,
0.0692891479608938));
#99618=CARTESIAN_POINT('Ctrl Pts',(0.00514983553251299,-0.0343603235965159,
0.0692257473259022));
#99619=CARTESIAN_POINT('Ctrl Pts',(0.00525418552406562,-0.034193496108874,
0.0691656705609461));
#99620=CARTESIAN_POINT('Ctrl Pts',(0.0048780191845862,-0.0346945769586885,
0.0694035047470073));
#99621=CARTESIAN_POINT('Ctrl Pts',(0.00497743642805156,-0.0345275153362891,
0.0693355209412622));
#99622=CARTESIAN_POINT('Ctrl Pts',(0.00507901741402414,-0.0343603235965159,
0.0692706461322225));
#99623=CARTESIAN_POINT('Ctrl Pts',(0.00518245885933831,-0.034193496108874,
0.0692090677255812));
#99624=CARTESIAN_POINT('Ctrl Pts',(0.00480915898656087,-0.0346945769586885,
0.0694513200317935));
#99625=CARTESIAN_POINT('Ctrl Pts',(0.00490757471974221,-0.0345275153362891,
0.0693818939216307));
#99626=CARTESIAN_POINT('Ctrl Pts',(0.0050081992955353,-0.0343603235965159,
0.0693155449385429));
#99627=CARTESIAN_POINT('Ctrl Pts',(0.00511073219461101,-0.034193496108874,
0.0692524648902163));
#99628=CARTESIAN_POINT('Ctrl Pts',(0.00474029878853555,-0.0346945769586885,
0.0694991353165797));
#99629=CARTESIAN_POINT('Ctrl Pts',(0.00483771301143286,-0.0345275153362891,
0.0694282669019992));
#99630=CARTESIAN_POINT('Ctrl Pts',(0.00493738117704646,-0.0343603235965159,
0.0693604437448632));
#99631=CARTESIAN_POINT('Ctrl Pts',(0.00503900552988371,-0.034193496108874,
0.0692958620548515));
#99632=CARTESIAN_POINT('Ctrl Pts',(0.00514727846869623,-0.0340223579322365,
0.0692304775090728));
#99633=CARTESIAN_POINT('Ctrl Pts',(0.00521513151449874,-0.0339125849573554,
0.0691894237596659));
#99634=CARTESIAN_POINT('Ctrl Pts',(0.00528378659796856,-0.0338030433565221,
0.0691498032586328));
#99635=CARTESIAN_POINT('Ctrl Pts',(0.00535315142932657,-0.0336938721132328,
0.0691116588909678));
#99636=CARTESIAN_POINT('Ctrl Pts',(0.00503784940600099,-0.0340223579322365,
0.0692010418152985));
#99637=CARTESIAN_POINT('Ctrl Pts',(0.00510610844679215,-0.0339125849573554,
0.0691584787537141));
#99638=CARTESIAN_POINT('Ctrl Pts',(0.00517520047921756,-0.0338030433565221,
0.0691173584042325));
#99639=CARTESIAN_POINT('Ctrl Pts',(0.00524503248468668,-0.0336938721132328,
0.0690777255203675));
#99640=CARTESIAN_POINT('Ctrl Pts',(0.00492842034330574,-0.0340223579322365,
0.0691716061215241));
#99641=CARTESIAN_POINT('Ctrl Pts',(0.00499708537908556,-0.0339125849573554,
0.0691275337477622));
#99642=CARTESIAN_POINT('Ctrl Pts',(0.00506661436046656,-0.0338030433565221,
0.0690849135498322));
#99643=CARTESIAN_POINT('Ctrl Pts',(0.0051369135400468,-0.0336938721132328,
0.0690437921497672));
#99644=CARTESIAN_POINT('Ctrl Pts',(0.00481899128061049,-0.0340223579322365,
0.0691421704277498));
#99645=CARTESIAN_POINT('Ctrl Pts',(0.00488806231137896,-0.0339125849573554,
0.0690965887418104));
#99646=CARTESIAN_POINT('Ctrl Pts',(0.00495802824171557,-0.0338030433565221,
0.0690524686954319));
#99647=CARTESIAN_POINT('Ctrl Pts',(0.00502879459540692,-0.0336938721132328,
0.069009858779167));
#99648=CARTESIAN_POINT('Origin',(0.01440730785072,-0.0345589643417286,0.0830948570790016));
#99649=CARTESIAN_POINT('Ctrl Pts',(0.00533493353088826,-0.034193496108874,
0.0688375313516922));
#99650=CARTESIAN_POINT('Ctrl Pts',(0.00540818932669617,-0.0340836138595105,
0.0687990747806207));
#99651=CARTESIAN_POINT('Ctrl Pts',(0.00548220575103187,-0.0339738896671456,
0.0687621525366981));
#99652=CARTESIAN_POINT('Ctrl Pts',(0.00555688490421961,-0.0338644633335883,
0.0687268055254937));
#99653=CARTESIAN_POINT('Ctrl Pts',(0.00530785598645012,-0.034193496108874,
0.0689475675540716));
#99654=CARTESIAN_POINT('Ctrl Pts',(0.0053795944482074,-0.0340836138595105,
0.0689087375997018));
#99655=CARTESIAN_POINT('Ctrl Pts',(0.00545210199292166,-0.0339738896671456,
0.0688714107535931));
#99656=CARTESIAN_POINT('Ctrl Pts',(0.00552528261738328,-0.0338644633335883,
0.0688356285686123));
#99657=CARTESIAN_POINT('Ctrl Pts',(0.00528077844201199,-0.034193496108874,
0.069057603756451));
#99658=CARTESIAN_POINT('Ctrl Pts',(0.00535099956971864,-0.0340836138595105,
0.0690184004187828));
#99659=CARTESIAN_POINT('Ctrl Pts',(0.00542199823481146,-0.0339738896671456,
0.0689806689704882));
#99660=CARTESIAN_POINT('Ctrl Pts',(0.00549368033054695,-0.0338644633335883,
0.0689444516117309));
#99661=CARTESIAN_POINT('Ctrl Pts',(0.00525370089757385,-0.034193496108874,
0.0691676399588304));
#99662=CARTESIAN_POINT('Ctrl Pts',(0.00532240469122988,-0.0340836138595105,
0.0691280632378638));
#99663=CARTESIAN_POINT('Ctrl Pts',(0.00539189447670125,-0.0339738896671456,
0.0690899271873832));
#99664=CARTESIAN_POINT('Ctrl Pts',(0.00546207804371062,-0.0338644633335883,
0.0690532746548495));
#99665=CARTESIAN_POINT('Origin',(0.0140416393589376,-0.0345610621863313,
0.0834076454514424));
#99666=CARTESIAN_POINT('Ctrl Pts',(0.0052228897417699,-0.03424362768739,
0.0691838195778075));
#99667=CARTESIAN_POINT('Ctrl Pts',(0.00541019232411137,-0.033943005420186,
0.0690744106153777));
#99668=CARTESIAN_POINT('Ctrl Pts',(0.00560520393079155,-0.0336441434784162,
0.0689794208702906));
#99669=CARTESIAN_POINT('Ctrl Pts',(0.00500981141681051,-0.03424362768739,
0.0693145774740604));
#99670=CARTESIAN_POINT('Ctrl Pts',(0.00519218238379618,-0.033943005420186,
0.0691971321301237));
#99671=CARTESIAN_POINT('Ctrl Pts',(0.00538288171850594,-0.0336441434784162,
0.0690937573645715));
#99672=CARTESIAN_POINT('Ctrl Pts',(0.00546205352410219,-0.0335235895815127,
0.0690532876027717));
#99673=CARTESIAN_POINT('Ctrl Pts',(0.00553221980475236,-0.0334144449262719,
0.0690166436671819));
#99674=CARTESIAN_POINT('Ctrl Pts',(0.00560322373408977,-0.0333049234473132,
0.0689814072147018));
#99675=CARTESIAN_POINT('Ctrl Pts',(0.00567497860131031,-0.0331951640388588,
0.0689476315262886));
#99676=CARTESIAN_POINT('Ctrl Pts',(0.00535468872440273,-0.0335235895815127,
0.0690170388473202));
#99677=CARTESIAN_POINT('Ctrl Pts',(0.00542535404053891,-0.0334144449262719,
0.0689789168238806));
#99678=CARTESIAN_POINT('Ctrl Pts',(0.00549688811487624,-0.0333049234473132,
0.0689422108951045));
#99679=CARTESIAN_POINT('Ctrl Pts',(0.00556920372892668,-0.0331951640388588,
0.0689069762823646));
#99680=CARTESIAN_POINT('Ctrl Pts',(0.00524732392470326,-0.0335235895815127,
0.0689807900918687));
#99681=CARTESIAN_POINT('Ctrl Pts',(0.00531848827632547,-0.0334144449262719,
0.0689411899805794));
#99682=CARTESIAN_POINT('Ctrl Pts',(0.00539055249566271,-0.0333049234473132,
0.0689030145755074));
#99683=CARTESIAN_POINT('Ctrl Pts',(0.00546342885654305,-0.0331951640388588,
0.0688663210384406));
#99684=CARTESIAN_POINT('Ctrl Pts',(0.0051399591250038,-0.0335235895815127,
0.0689445413364172));
#99685=CARTESIAN_POINT('Ctrl Pts',(0.00521162251211202,-0.0334144449262719,
0.0689034631372782));
#99686=CARTESIAN_POINT('Ctrl Pts',(0.00528421687644918,-0.0333049234473132,
0.0688638182559102));
#99687=CARTESIAN_POINT('Ctrl Pts',(0.00535765398415942,-0.0331951640388588,
0.0688256657945166));
#99688=CARTESIAN_POINT('Origin',(0.0120771875754346,-0.0326434571770968,
0.0843360219986812));
#99689=CARTESIAN_POINT('Ctrl Pts',(0.00567461650928284,-0.0336938721132354,
0.0686709665097099));
#99690=CARTESIAN_POINT('Ctrl Pts',(0.00570668711043635,-0.033647456976494,
0.0686566307302437));
#99691=CARTESIAN_POINT('Ctrl Pts',(0.00573892333249069,-0.033601104548885,
0.0686426713599529));
#99692=CARTESIAN_POINT('Ctrl Pts',(0.00582053802807421,-0.033483750869459,
0.0686073294469058));
#99693=CARTESIAN_POINT('Ctrl Pts',(0.00590316413857309,-0.0333660264863565,
0.0685744214658548));
#99694=CARTESIAN_POINT('Ctrl Pts',(0.00557281665257666,-0.0336938721132354,
0.0689953225308444));
#99695=CARTESIAN_POINT('Ctrl Pts',(0.0056029886903058,-0.033647456976494,
0.0689803908830361));
#99696=CARTESIAN_POINT('Ctrl Pts',(0.00563333345441785,-0.033601104548885,
0.0689658134601506));
#99697=CARTESIAN_POINT('Ctrl Pts',(0.00571015941378067,-0.033483750869459,
0.0689289067801685));
#99698=CARTESIAN_POINT('Ctrl Pts',(0.00578804525820308,-0.0333660264863565,
0.0688942928191422));
#99699=CARTESIAN_POINT('Ctrl Pts',(0.00557281665258841,-0.0336938721132427,
0.0689953225308535));
#99700=CARTESIAN_POINT('Ctrl Pts',(0.00560298869031667,-0.0336474569765026,
0.0689803908830456));
#99701=CARTESIAN_POINT('Ctrl Pts',(0.00563333345442785,-0.0336011045488949,
0.0689658134601606));
#99702=CARTESIAN_POINT('Ctrl Pts',(0.00570951955818085,-0.033484728265791,
0.0689292141625584));
#99703=CARTESIAN_POINT('Ctrl Pts',(0.00578674824582927,-0.0333679870047996,
0.0688948694279671));
#99704=CARTESIAN_POINT('Ctrl Pts',(0.00557281665257206,-0.0336938721132425,
0.0689953225308467));
#99705=CARTESIAN_POINT('Ctrl Pts',(0.00568072521195011,-0.0335278710435082,
0.0689419203503709));
#99706=CARTESIAN_POINT('Ctrl Pts',(0.00579027048784295,-0.0333620469224319,
0.0688919209410244));
#99707=CARTESIAN_POINT('Ctrl Pts',(0.00590151527665343,-0.0331951640388602,
0.068845317657764));
#99708=CARTESIAN_POINT('Ctrl Pts',(0.00549850658563194,-0.0336938721132425,
0.0690341303106676));
#99709=CARTESIAN_POINT('Ctrl Pts',(0.00560560273887242,-0.0335278710435082,
0.068979172515448));
#99710=CARTESIAN_POINT('Ctrl Pts',(0.0057143846781042,-0.0333620469224319,
0.068927592561774));
#99711=CARTESIAN_POINT('Ctrl Pts',(0.00582491508299913,-0.0331951640388602,
0.0688793828915867));
#99712=CARTESIAN_POINT('Ctrl Pts',(0.00542419651869182,-0.0336938721132425,
0.0690729380904886));
#99713=CARTESIAN_POINT('Ctrl Pts',(0.00553048026579473,-0.0335278710435082,
0.069016424680525));
#99714=CARTESIAN_POINT('Ctrl Pts',(0.00563849886836544,-0.0333620469224319,
0.0689632641825236));
#99715=CARTESIAN_POINT('Ctrl Pts',(0.00574831488934483,-0.0331951640388602,
0.0689134481254095));
#99716=CARTESIAN_POINT('Ctrl Pts',(0.0053498864517517,-0.0336938721132425,
0.0691117458703095));
#99717=CARTESIAN_POINT('Ctrl Pts',(0.00545535779271704,-0.0335278710435082,
0.069053676845602));
#99718=CARTESIAN_POINT('Ctrl Pts',(0.00556261305862668,-0.0333620469224319,
0.0689989358032733));
#99719=CARTESIAN_POINT('Ctrl Pts',(0.00567171469569052,-0.0331951640388602,
0.0689475133592322));
#99720=CARTESIAN_POINT('Ctrl Pts',(0.00578732976821152,-0.0330240426238155,
0.0688962136657319));
#99721=CARTESIAN_POINT('Ctrl Pts',(0.00585970579348169,-0.0329142774063509,
0.0688640267572839));
#99722=CARTESIAN_POINT('Ctrl Pts',(0.00593278329414736,-0.0328043479726686,
0.0688333200171028));
#99723=CARTESIAN_POINT('Ctrl Pts',(0.00600646973583871,-0.0326943950436594,
0.0688041353610254));
#99724=CARTESIAN_POINT('Ctrl Pts',(0.00568245304879065,-0.0330240426238155,
0.0688532950251651));
#99725=CARTESIAN_POINT('Ctrl Pts',(0.00575542032014823,-0.0329142774063509,
0.0688196633377306));
#99726=CARTESIAN_POINT('Ctrl Pts',(0.00582911922927649,-0.0328043479726686,
0.0687875233209962));
#99727=CARTESIAN_POINT('Ctrl Pts',(0.00590345649630189,-0.0326943950436594,
0.0687569187488564));
#99728=CARTESIAN_POINT('Ctrl Pts',(0.00557757632936978,-0.0330240426238155,
0.0688103763845982));
#99729=CARTESIAN_POINT('Ctrl Pts',(0.00565113484681477,-0.0329142774063509,
0.0687752999181773));
#99730=CARTESIAN_POINT('Ctrl Pts',(0.00572545516440562,-0.0328043479726686,
0.0687417266248897));
#99731=CARTESIAN_POINT('Ctrl Pts',(0.00580044325676507,-0.0326943950436594,
0.0687097021366873));
#99732=CARTESIAN_POINT('Ctrl Pts',(0.0054726996099489,-0.0330240426238155,
0.0687674577440314));
#99733=CARTESIAN_POINT('Ctrl Pts',(0.00554684937348131,-0.0329142774063509,
0.068730936498624));
#99734=CARTESIAN_POINT('Ctrl Pts',(0.00562179109953475,-0.0328043479726686,
0.0686959299287831));
#99735=CARTESIAN_POINT('Ctrl Pts',(0.00569743001722824,-0.0326943950436594,
0.0686624855245183));
#99736=CARTESIAN_POINT('Origin',(0.0121245010631098,-0.0326396682854783,
0.0844502884958673));
#99737=CARTESIAN_POINT('Ctrl Pts',(0.00602275330947993,-0.0331951640388587,
0.0685298863329841));
#99738=CARTESIAN_POINT('Ctrl Pts',(0.00610015901485808,-0.0330855618127431,
0.0685009489070897));
#99739=CARTESIAN_POINT('Ctrl Pts',(0.00617821860813228,-0.0329757224171935,
0.0684735904644101));
#99740=CARTESIAN_POINT('Ctrl Pts',(0.00625683384778119,-0.0328657861694598,
0.0684478509423289));
#99741=CARTESIAN_POINT('Ctrl Pts',(0.00598209809792321,-0.0331951640388587,
0.0686356611211562));
#99742=CARTESIAN_POINT('Ctrl Pts',(0.00605804696940533,-0.0330855618127431,
0.0686061637519023));
#99743=CARTESIAN_POINT('Ctrl Pts',(0.00613466025164563,-0.0329757224171935,
0.0685782148519377));
#99744=CARTESIAN_POINT('Ctrl Pts',(0.00621184159230039,-0.0328657861694598,
0.0685518550239138));
#99745=CARTESIAN_POINT('Ctrl Pts',(0.00594144288636649,-0.0331951640388587,
0.0687414359093283));
#99746=CARTESIAN_POINT('Ctrl Pts',(0.00601593492395257,-0.0330855618127431,
0.0687113785967148));
#99747=CARTESIAN_POINT('Ctrl Pts',(0.00609110189515898,-0.0329757224171935,
0.0686828392394654));
#99748=CARTESIAN_POINT('Ctrl Pts',(0.00616684933681959,-0.0328657861694598,
0.0686558591054987));
#99749=CARTESIAN_POINT('Ctrl Pts',(0.00590078767480977,-0.0331951640388587,
0.0688472106975004));
#99750=CARTESIAN_POINT('Ctrl Pts',(0.00597382287849982,-0.0330855618127431,
0.0688165934415273));
#99751=CARTESIAN_POINT('Ctrl Pts',(0.00604754353867233,-0.0329757224171935,
0.0687874636269931));
#99752=CARTESIAN_POINT('Ctrl Pts',(0.0061218570813388,-0.0328657861694598,
0.0687598631870836));
#99753=CARTESIAN_POINT('Origin',(0.0116637048409317,-0.0326401908832987,
0.084587910124528));
#99754=CARTESIAN_POINT('Ctrl Pts',(0.00586825825960548,-0.0332451089994432,
0.0688593727417823));
#99755=CARTESIAN_POINT('Ctrl Pts',(0.00606779753128231,-0.0329451141710258,
0.0687743042648371));
#99756=CARTESIAN_POINT('Ctrl Pts',(0.00627317763839391,-0.0326442513127503,
0.0687045075721225));
#99757=CARTESIAN_POINT('Ctrl Pts',(0.00564047051284638,-0.0332451089994432,
0.0689623909072989));
#99758=CARTESIAN_POINT('Ctrl Pts',(0.00583612439084238,-0.0329451141710258,
0.0688687312749261));
#99759=CARTESIAN_POINT('Ctrl Pts',(0.00603827726321428,-0.0326442513127503,
0.068790075169614));
#99760=CARTESIAN_POINT('Ctrl Pts',(0.00612182741298092,-0.0325229783203384,
0.0687598741104088));
#99761=CARTESIAN_POINT('Ctrl Pts',(0.0061961301791422,-0.0324130253112079,
0.068732277208047));
#99762=CARTESIAN_POINT('Ctrl Pts',(0.00627099255319903,-0.0323031222247695,
0.0687062215394347));
#99763=CARTESIAN_POINT('Ctrl Pts',(0.00634631746406593,-0.0321934096636184,
0.0686817370962685));
#99764=CARTESIAN_POINT('Ctrl Pts',(0.00601985249317014,-0.0325229783203384,
0.0687104548997822));
#99765=CARTESIAN_POINT('Ctrl Pts',(0.00609483650205677,-0.0324130253112079,
0.0686814522754064));
#99766=CARTESIAN_POINT('Ctrl Pts',(0.00617040909468027,-0.0323031222247695,
0.0686540051903661));
#99767=CARTESIAN_POINT('Ctrl Pts',(0.00624647222732398,-0.0321934096636184,
0.0686281453865616));
#99768=CARTESIAN_POINT('Ctrl Pts',(0.00591787757335935,-0.0325229783203384,
0.0686610356891557));
#99769=CARTESIAN_POINT('Ctrl Pts',(0.00599354282497134,-0.0324130253112079,
0.0686306273427659));
#99770=CARTESIAN_POINT('Ctrl Pts',(0.0060698256361615,-0.0323031222247695,
0.0686017888412976));
#99771=CARTESIAN_POINT('Ctrl Pts',(0.00614662699058202,-0.0321934096636184,
0.0685745536768546));
#99772=CARTESIAN_POINT('Ctrl Pts',(0.00581590265354856,-0.0325229783203384,
0.0686116164785291));
#99773=CARTESIAN_POINT('Ctrl Pts',(0.00589224914788592,-0.0324130253112079,
0.0685798024101254));
#99774=CARTESIAN_POINT('Ctrl Pts',(0.00596924217764273,-0.0323031222247695,
0.068549572492229));
#99775=CARTESIAN_POINT('Ctrl Pts',(0.00604678175384007,-0.0321934096636184,
0.0685209619671477));
#99776=CARTESIAN_POINT('Origin',(0.0121216376506533,-0.0326393375177596,
0.0844422578116633));
#99777=CARTESIAN_POINT('Ctrl Pts',(0.00637978906701306,-0.0326943950436593,
0.0684090516483641));
#99778=CARTESIAN_POINT('Ctrl Pts',(0.00645891009498231,-0.0325844576448126,
0.0683850161544951));
#99779=CARTESIAN_POINT('Ctrl Pts',(0.00653853381588957,-0.0324744968375319,
0.068362615312176));
#99780=CARTESIAN_POINT('Ctrl Pts',(0.00661855781530343,-0.0323646534831894,
0.0683418764155297));
#99781=CARTESIAN_POINT('Ctrl Pts',(0.00633257247029293,-0.0326943950436593,
0.0685120648541959));
#99782=CARTESIAN_POINT('Ctrl Pts',(0.00641027378321849,-0.0325844576448126,
0.0684873786271307));
#99783=CARTESIAN_POINT('Ctrl Pts',(0.00648849114683602,-0.0324744968375319,
0.0684642976435273));
#99784=CARTESIAN_POINT('Ctrl Pts',(0.00656712393660134,-0.0323646534831894,
0.0684428500937989));
#99785=CARTESIAN_POINT('Ctrl Pts',(0.0062853558735728,-0.0326943950436593,
0.0686150780600276));
#99786=CARTESIAN_POINT('Ctrl Pts',(0.00636163747145468,-0.0325844576448126,
0.0685897410997663));
#99787=CARTESIAN_POINT('Ctrl Pts',(0.00643844847778248,-0.0324744968375319,
0.0685659799748785));
#99788=CARTESIAN_POINT('Ctrl Pts',(0.00651569005789925,-0.0323646534831894,
0.0685438237720681));
#99789=CARTESIAN_POINT('Ctrl Pts',(0.00623813927685267,-0.0326943950436593,
0.0687180912658593));
#99790=CARTESIAN_POINT('Ctrl Pts',(0.00631300115969087,-0.0325844576448126,
0.0686921035724019));
#99791=CARTESIAN_POINT('Ctrl Pts',(0.00638840580872893,-0.0324744968375319,
0.0686676623062299));
#99792=CARTESIAN_POINT('Ctrl Pts',(0.00646425617919717,-0.0323646534831894,
0.0686447974503374));
#99793=CARTESIAN_POINT('Origin',(0.0116762912092995,-0.032639557906863,
0.0846235968853021));
#99794=CARTESIAN_POINT('Ctrl Pts',(0.00620487327920245,-0.0327445246961877,
0.0687282001530734));
#99795=CARTESIAN_POINT('Ctrl Pts',(0.00640935980120099,-0.0324436878365475,
0.0686558273210038));
#99796=CARTESIAN_POINT('Ctrl Pts',(0.00661871681604563,-0.0321434074463186,
0.0685990628529258));
#99797=CARTESIAN_POINT('Ctrl Pts',(0.00597106705903739,-0.0327445246961877,
0.0688167137193337));
#99798=CARTESIAN_POINT('Ctrl Pts',(0.00617221523734467,-0.0324436878365475,
0.0687355227416054));
#99799=CARTESIAN_POINT('Ctrl Pts',(0.00637890761114403,-0.0321434074463186,
0.0686697137216004));
#99800=CARTESIAN_POINT('Ctrl Pts',(0.00655447739320943,-0.0322357242816072,
0.0686168808575076));
#99801=CARTESIAN_POINT('Ctrl Pts',(0.00673070006170515,-0.0319819883628706,
0.0685669005349447));
#99802=CARTESIAN_POINT('Ctrl Pts',(0.0069097459840021,-0.0317295851069887,
0.068528235056232));
#99803=CARTESIAN_POINT('Ctrl Pts',(0.00631550320732872,-0.0322357242816072,
0.0686903065919789));
#99804=CARTESIAN_POINT('Ctrl Pts',(0.00648938736141121,-0.0319819883628706,
0.0686327152515338));
#99805=CARTESIAN_POINT('Ctrl Pts',(0.00666658381942561,-0.0317295851069887,
0.0685863053732491));
#99806=CARTESIAN_POINT('Origin',(0.0116472978938751,-0.0326371942647044,
0.0845328125743387));
#99807=CARTESIAN_POINT('Origin',(0.0120799268622383,-0.032635298552708,
0.0843268281231969));
#99808=CARTESIAN_POINT('Ctrl Pts',(0.00674370756866054,-0.0321934096636183,
0.0683108738640975));
#99809=CARTESIAN_POINT('Ctrl Pts',(0.0068242336688127,-0.0320835708272303,
0.0682918415594616));
#99810=CARTESIAN_POINT('Ctrl Pts',(0.00690510693310943,-0.0319739230346346,
0.0682744867777932));
#99811=CARTESIAN_POINT('Ctrl Pts',(0.00698622218570662,-0.0318646057455575,
0.0682588237821651));
#99812=CARTESIAN_POINT('Ctrl Pts',(0.00669011581280508,-0.0321934096636183,
0.0684107191868175));
#99813=CARTESIAN_POINT('Ctrl Pts',(0.00676926496814222,-0.0320835708272303,
0.0683909478101015));
#99814=CARTESIAN_POINT('Ctrl Pts',(0.00684877738136617,-0.0319739230346346,
0.0683728258892434));
#99815=CARTESIAN_POINT('Ctrl Pts',(0.00692854954241986,-0.0318646057455575,
0.0683563688024431));
#99816=CARTESIAN_POINT('Ctrl Pts',(0.00663652405694963,-0.0321934096636183,
0.0685105645095375));
#99817=CARTESIAN_POINT('Ctrl Pts',(0.00671429626747175,-0.0320835708272303,
0.0684900540607413));
#99818=CARTESIAN_POINT('Ctrl Pts',(0.00679244782962291,-0.0319739230346346,
0.0684711650006936));
#99819=CARTESIAN_POINT('Ctrl Pts',(0.00687087689913309,-0.0318646057455575,
0.0684539138227211));
#99820=CARTESIAN_POINT('Ctrl Pts',(0.00658293230109417,-0.0321934096636183,
0.0686104098322574));
#99821=CARTESIAN_POINT('Ctrl Pts',(0.00665932756680127,-0.0320835708272303,
0.0685891603113812));
#99822=CARTESIAN_POINT('Ctrl Pts',(0.00673611827787965,-0.0319739230346346,
0.0685695041121437));
#99823=CARTESIAN_POINT('Ctrl Pts',(0.00681320425584633,-0.0318646057455575,
0.0685514588429991));
#99824=CARTESIAN_POINT('Ctrl Pts',(0.0064635676040236,-0.0320218834582358,
0.0686441408192202));
#99825=CARTESIAN_POINT('Ctrl Pts',(0.00652087028776568,-0.0319391099350663,
0.0686268619988911));
#99826=CARTESIAN_POINT('Ctrl Pts',(0.00657840806446979,-0.0318564869454954,
0.0686104884368015));
#99827=CARTESIAN_POINT('Ctrl Pts',(0.0066361379121258,-0.0317740741446555,
0.0685950281464577));
#99828=CARTESIAN_POINT('Ctrl Pts',(0.00642040989459936,-0.0320218834582358,
0.0686197637774708));
#99829=CARTESIAN_POINT('Ctrl Pts',(0.00647796628441493,-0.0319391099350663,
0.0686020357897196));
#99830=CARTESIAN_POINT('Ctrl Pts',(0.00653576462729074,-0.0318564869454954,
0.0685852172940031));
#99831=CARTESIAN_POINT('Ctrl Pts',(0.00659376168117411,-0.0317740741446555,
0.0685693166101845));
#99832=CARTESIAN_POINT('Ctrl Pts',(0.00637725218517513,-0.0320218834582358,
0.0685953867357213));
#99833=CARTESIAN_POINT('Ctrl Pts',(0.00643506228106419,-0.0319391099350663,
0.0685772095805482));
#99834=CARTESIAN_POINT('Ctrl Pts',(0.00649312119011169,-0.0318564869454954,
0.0685599461512047));
#99835=CARTESIAN_POINT('Ctrl Pts',(0.00655138545022241,-0.0317740741446555,
0.0685436050739113));
#99836=CARTESIAN_POINT('Ctrl Pts',(0.00633409447575089,-0.0320218834582358,
0.0685710096939719));
#99837=CARTESIAN_POINT('Ctrl Pts',(0.00639215827771344,-0.0319391099350663,
0.0685523833713767));
#99838=CARTESIAN_POINT('Ctrl Pts',(0.00645047775293264,-0.0318564869454954,
0.0685346750084063));
#99839=CARTESIAN_POINT('Ctrl Pts',(0.00650900921927072,-0.0317740741446555,
0.0685178935376381));
#99840=CARTESIAN_POINT('Origin',(0.00374573569064397,-0.0391228853390723,
0.0628932985669952));
#99841=CARTESIAN_POINT('Ctrl Pts',(0.00389106271677981,-0.0352722978779586,
0.0702553561937829));
#99842=CARTESIAN_POINT('Ctrl Pts',(0.00390411340789216,-0.0352466642097211,
0.0702416897333956));
#99843=CARTESIAN_POINT('Ctrl Pts',(0.00391709577180745,-0.0352210183808299,
0.0702279813024733));
#99844=CARTESIAN_POINT('Ctrl Pts',(0.00393000988001004,-0.0351953608940152,
0.0702142300510901));
#99845=CARTESIAN_POINT('Origin',(0.000474874517336402,-0.0352456003065064,
0.066742607785333));
#99846=CARTESIAN_POINT('Ctrl Pts',(0.00401735610000403,-0.035024121149334,
0.0701252584080182));
#99847=CARTESIAN_POINT('Ctrl Pts',(0.00407279526272551,-0.0349144232867422,
0.0700686940748364));
#99848=CARTESIAN_POINT('Ctrl Pts',(0.0041294368335894,-0.0348045283677512,
0.0700132418522327));
#99849=CARTESIAN_POINT('Ctrl Pts',(0.00418721090503603,-0.0346945769586886,
0.0699589754672298));
#99850=CARTESIAN_POINT('Ctrl Pts',(0.00390404476136973,-0.035024121149334,
0.0701239613575513));
#99851=CARTESIAN_POINT('Ctrl Pts',(0.00395950179042877,-0.0349144232867422,
0.0700658362072097));
#99852=CARTESIAN_POINT('Ctrl Pts',(0.00401619350152863,-0.0348045283677512,
0.0700088226025319));
#99853=CARTESIAN_POINT('Ctrl Pts',(0.00407404999730846,-0.0346945769586886,
0.0699529962728622));
#99854=CARTESIAN_POINT('Ctrl Pts',(0.00379073342273543,-0.035024121149334,
0.0701226643070845));
#99855=CARTESIAN_POINT('Ctrl Pts',(0.00384620831813203,-0.0349144232867422,
0.070062978339583));
#99856=CARTESIAN_POINT('Ctrl Pts',(0.00390295016946786,-0.0348045283677512,
0.070004403352831));
#99857=CARTESIAN_POINT('Ctrl Pts',(0.0039608890895809,-0.0346945769586886,
0.0699470170784946));
#99858=CARTESIAN_POINT('Ctrl Pts',(0.00367742208410113,-0.035024121149334,
0.0701213672566176));
#99859=CARTESIAN_POINT('Ctrl Pts',(0.00373291484583529,-0.0349144232867422,
0.0700601204719563));
#99860=CARTESIAN_POINT('Ctrl Pts',(0.00378970683740709,-0.0348045283677512,
0.0699999841031302));
#99861=CARTESIAN_POINT('Ctrl Pts',(0.00384772818185334,-0.0346945769586886,
0.0699410378841271));
#99862=CARTESIAN_POINT('Origin',(0.0155494541559422,-0.0345629067942227,
0.0823186832866856));
#99863=CARTESIAN_POINT('Ctrl Pts',(0.00410124984194354,-0.0351970973651652,
0.0697917027108022));
#99864=CARTESIAN_POINT('Ctrl Pts',(0.00416162814434792,-0.0350869349321791,
0.0697359759765723));
#99865=CARTESIAN_POINT('Ctrl Pts',(0.004223214991358,-0.0349764985129724,
0.0696814583104115));
#99866=CARTESIAN_POINT('Ctrl Pts',(0.00428593475305483,-0.0348659306849626,
0.0696282250383206));
#99867=CARTESIAN_POINT('Ctrl Pts',(0.00410209584850038,-0.0351970973651652,
0.0698739204395653));
#99868=CARTESIAN_POINT('Ctrl Pts',(0.00416133513569748,-0.0350869349321791,
0.0698182054256097));
#99869=CARTESIAN_POINT('Ctrl Pts',(0.00422178178029532,-0.0349764985129724,
0.0697636758099372));
#99870=CARTESIAN_POINT('Ctrl Pts',(0.00428336163045199,-0.0348659306849626,
0.0697104068470749));
#99871=CARTESIAN_POINT('Ctrl Pts',(0.00410294185505723,-0.0351970973651652,
0.0699561381683284));
#99872=CARTESIAN_POINT('Ctrl Pts',(0.00416104212704704,-0.0350869349321791,
0.0699004348746471));
#99873=CARTESIAN_POINT('Ctrl Pts',(0.00422034856923265,-0.0349764985129724,
0.0698458933094629));
#99874=CARTESIAN_POINT('Ctrl Pts',(0.00428078850784914,-0.0348659306849626,
0.0697925886558292));
#99875=CARTESIAN_POINT('Ctrl Pts',(0.00410378786161407,-0.0351970973651652,
0.0700383558970915));
#99876=CARTESIAN_POINT('Ctrl Pts',(0.0041607491183966,-0.0350869349321791,
0.0699826643236845));
#99877=CARTESIAN_POINT('Ctrl Pts',(0.00421891535816998,-0.0349764985129724,
0.0699281108089885));
#99878=CARTESIAN_POINT('Ctrl Pts',(0.00427821538524629,-0.0348659306849626,
0.0698747704645834));
#99879=CARTESIAN_POINT('Origin',(0.0151645710067182,-0.0345637187965536,
0.0826071106048243));
#99880=CARTESIAN_POINT('Ctrl Pts',(0.00407904357217628,-0.0352450361861253,
0.0700612086763518));
#99881=CARTESIAN_POINT('Ctrl Pts',(0.00423325486346955,-0.0349452761023765,
0.0699086588599623));
#99882=CARTESIAN_POINT('Ctrl Pts',(0.0043985187327985,-0.0346444289983475,
0.0697681582466638));
#99883=CARTESIAN_POINT('Ctrl Pts',(0.00390517520914662,-0.0352450361861253,
0.0702408466242843));
#99884=CARTESIAN_POINT('Ctrl Pts',(0.00405261134423279,-0.0349452761023765,
0.0700817392551474));
#99885=CARTESIAN_POINT('Ctrl Pts',(0.00421161324655083,-0.0346444289983475,
0.0699341893859435));
#99886=CARTESIAN_POINT('Ctrl Pts',(0.00427817405012767,-0.0345231616327821,
0.0698753562986284));
#99887=CARTESIAN_POINT('Ctrl Pts',(0.00433709399533374,-0.0344132092796975,
0.069822350004561));
#99888=CARTESIAN_POINT('Ctrl Pts',(0.00439710729392348,-0.0343032738558973,
0.0697705651579658));
#99889=CARTESIAN_POINT('Ctrl Pts',(0.00445813536254092,-0.034193496108874,
0.0697200661318044));
#99890=CARTESIAN_POINT('Ctrl Pts',(0.00416516777158763,-0.0345231616327821,
0.0698669469497236));
#99891=CARTESIAN_POINT('Ctrl Pts',(0.00422420362782893,-0.0344132092796975,
0.0698123830232066));
#99892=CARTESIAN_POINT('Ctrl Pts',(0.004284365049872,-0.0343032738558973,
0.0697590430220569));
#99893=CARTESIAN_POINT('Ctrl Pts',(0.00434557321356326,-0.034193496108874,
0.0697069933067079));
#99894=CARTESIAN_POINT('Ctrl Pts',(0.00405216149304758,-0.0345231616327821,
0.0698585376008188));
#99895=CARTESIAN_POINT('Ctrl Pts',(0.00411131326032411,-0.0344132092796975,
0.0698024160418523));
#99896=CARTESIAN_POINT('Ctrl Pts',(0.00417162280582052,-0.0343032738558973,
0.069747520886148));
#99897=CARTESIAN_POINT('Ctrl Pts',(0.0042330110645856,-0.034193496108874,
0.0696939204816113));
#99898=CARTESIAN_POINT('Ctrl Pts',(0.00393915521450753,-0.0345231616327821,
0.069850128251914));
#99899=CARTESIAN_POINT('Ctrl Pts',(0.0039984228928193,-0.0344132092796975,
0.0697924490604979));
#99900=CARTESIAN_POINT('Ctrl Pts',(0.00405888056176904,-0.0343032738558973,
0.0697359987502391));
#99901=CARTESIAN_POINT('Ctrl Pts',(0.00412044891560794,-0.034193496108874,
0.0696808476565147));
#99902=CARTESIAN_POINT('Origin',(0.0155577793327288,-0.0345625596230697,
0.0823274690555088));
#99903=CARTESIAN_POINT('Ctrl Pts',(0.00438887434898244,-0.0346945769586885,
0.0694542079053786));
#99904=CARTESIAN_POINT('Ctrl Pts',(0.00445358473752521,-0.0345846629176052,
0.0694027389874847));
#99905=CARTESIAN_POINT('Ctrl Pts',(0.00451937053484638,-0.0344746925050311,
0.0693525994628331));
#99906=CARTESIAN_POINT('Ctrl Pts',(0.00458614718328078,-0.0343648066253259,
0.0693038532278454));
#99907=CARTESIAN_POINT('Ctrl Pts',(0.00438289515932269,-0.0346945769586885,
0.0695673687240069));
#99908=CARTESIAN_POINT('Ctrl Pts',(0.00444604613458785,-0.0345846629176052,
0.0695158174098574));
#99909=CARTESIAN_POINT('Ctrl Pts',(0.00451027395620052,-0.0344746925050311,
0.0694655632268504));
#99910=CARTESIAN_POINT('Ctrl Pts',(0.0045754960621468,-0.0343648066253259,
0.0694166702265655));
#99911=CARTESIAN_POINT('Ctrl Pts',(0.00437691596966294,-0.0346945769586885,
0.0696805295426352));
#99912=CARTESIAN_POINT('Ctrl Pts',(0.00443850753165049,-0.0345846629176052,
0.0696288958322299));
#99913=CARTESIAN_POINT('Ctrl Pts',(0.00450117737755465,-0.0344746925050311,
0.0695785269908678));
#99914=CARTESIAN_POINT('Ctrl Pts',(0.00456484494101283,-0.0343648066253259,
0.0695294872252856));
#99915=CARTESIAN_POINT('Ctrl Pts',(0.00437093678000319,-0.0346945769586885,
0.0697936903612635));
#99916=CARTESIAN_POINT('Ctrl Pts',(0.00443096892871313,-0.0345846629176052,
0.0697419742546026));
#99917=CARTESIAN_POINT('Ctrl Pts',(0.00449208079890879,-0.0344746925050311,
0.0696914907548851));
#99918=CARTESIAN_POINT('Ctrl Pts',(0.00455419381987885,-0.0343648066253259,
0.0696423042240056));
#99919=CARTESIAN_POINT('Origin',(0.0152025510260162,-0.0345626446730064,
0.0826515138564479));
#99920=CARTESIAN_POINT('Ctrl Pts',(0.00437104376775593,-0.0346945769586885,
0.0697916655347617));
#99921=CARTESIAN_POINT('Ctrl Pts',(0.00446233082811079,-0.034527515336289,
0.0697130629259295));
#99922=CARTESIAN_POINT('Ctrl Pts',(0.00455611347967425,-0.0343603235965158,
0.0696373108804606));
#99923=CARTESIAN_POINT('Ctrl Pts',(0.0046521110251616,-0.034193496108874,
0.0695646293168765));
#99924=CARTESIAN_POINT('Ctrl Pts',(0.00430871939721564,-0.0346945769586885,
0.069847734253028));
#99925=CARTESIAN_POINT('Ctrl Pts',(0.00439883207581774,-0.034527515336289,
0.0697678262353015));
#99926=CARTESIAN_POINT('Ctrl Pts',(0.00449148109578134,-0.0343603235965158,
0.0696907315100676));
#99927=CARTESIAN_POINT('Ctrl Pts',(0.00458638905358064,-0.034193496108874,
0.0696166740167295));
#99928=CARTESIAN_POINT('Ctrl Pts',(0.00424639502667535,-0.0346945769586885,
0.0699038029712944));
#99929=CARTESIAN_POINT('Ctrl Pts',(0.00433533332352469,-0.034527515336289,
0.0698225895446736));
#99930=CARTESIAN_POINT('Ctrl Pts',(0.00442684871188844,-0.0343603235965158,
0.0697441521396747));
#99931=CARTESIAN_POINT('Ctrl Pts',(0.00452066708199968,-0.034193496108874,
0.0696687187165824));
#99932=CARTESIAN_POINT('Ctrl Pts',(0.00418407065613505,-0.0346945769586885,
0.0699598716895607));
#99933=CARTESIAN_POINT('Ctrl Pts',(0.00427183457123164,-0.034527515336289,
0.0698773528540456));
#99934=CARTESIAN_POINT('Ctrl Pts',(0.00436221632799553,-0.0343603235965158,
0.0697975727692817));
#99935=CARTESIAN_POINT('Ctrl Pts',(0.00445494511041871,-0.034193496108874,
0.0697207634164353));
#99936=CARTESIAN_POINT('Ctrl Pts',(0.0045541694282215,-0.0340223579322365,
0.0696423242498007));
#99937=CARTESIAN_POINT('Ctrl Pts',(0.00461634203332804,-0.0339125849573554,
0.0695930899798324));
#99938=CARTESIAN_POINT('Ctrl Pts',(0.00467948998544851,-0.0338030433565221,
0.0695451771346721));
#99939=CARTESIAN_POINT('Ctrl Pts',(0.00474352709745127,-0.0336938721132327,
0.0694986398281295));
#99940=CARTESIAN_POINT('Ctrl Pts',(0.00444191397568752,-0.0340223579322365,
0.0696268357635373));
#99941=CARTESIAN_POINT('Ctrl Pts',(0.0045043002074153,-0.0339125849573554,
0.0695760531981041));
#99942=CARTESIAN_POINT('Ctrl Pts',(0.00456769368216244,-0.0338030433565221,
0.0695265975670228));
#99943=CARTESIAN_POINT('Ctrl Pts',(0.00463200772392035,-0.0336938721132327,
0.0694785249292331));
#99944=CARTESIAN_POINT('Ctrl Pts',(0.00432965852315354,-0.0340223579322365,
0.0696113472772738));
#99945=CARTESIAN_POINT('Ctrl Pts',(0.00439225838150255,-0.0339125849573554,
0.0695590164163757));
#99946=CARTESIAN_POINT('Ctrl Pts',(0.00445589737887636,-0.0338030433565221,
0.0695080179993735));
#99947=CARTESIAN_POINT('Ctrl Pts',(0.00452048835038944,-0.0336938721132327,
0.0694584100303368));
#99948=CARTESIAN_POINT('Ctrl Pts',(0.00421740307061956,-0.0340223579322365,
0.0695958587910104));
#99949=CARTESIAN_POINT('Ctrl Pts',(0.00428021655558981,-0.0339125849573554,
0.0695419796346474));
#99950=CARTESIAN_POINT('Ctrl Pts',(0.00434410107559029,-0.0338030433565221,
0.0694894384317242));
#99951=CARTESIAN_POINT('Ctrl Pts',(0.00440896897685852,-0.0336938721132327,
0.0694382951314404));
#99952=CARTESIAN_POINT('Origin',(0.015478848235124,-0.0345589643415136,
0.0822367896202505));
#99953=CARTESIAN_POINT('Ctrl Pts',(0.00469109556167717,-0.034193496108874,
0.069228957174499));
#99954=CARTESIAN_POINT('Ctrl Pts',(0.00475895382725051,-0.0340836138595105,
0.0691816224592109));
#99955=CARTESIAN_POINT('Ctrl Pts',(0.00482775902575142,-0.0339738896671456,
0.0691357146404109));
#99956=CARTESIAN_POINT('Ctrl Pts',(0.00489741915629962,-0.0338644633335883,
0.0690912865711986));
#99957=CARTESIAN_POINT('Ctrl Pts',(0.00467802272481794,-0.034193496108874,
0.0693415194247579));
#99958=CARTESIAN_POINT('Ctrl Pts',(0.0047443288236367,-0.0340836138595105,
0.0692940044427933));
#99959=CARTESIAN_POINT('Ctrl Pts',(0.00481158633038239,-0.0339738896671456,
0.0692478843249783));
#99960=CARTESIAN_POINT('Ctrl Pts',(0.00487970520681449,-0.0338644633335883,
0.0692032123289156));
#99961=CARTESIAN_POINT('Ctrl Pts',(0.00466494988795871,-0.034193496108874,
0.0694540816750168));
#99962=CARTESIAN_POINT('Ctrl Pts',(0.00472970382002289,-0.0340836138595105,
0.0694063864263755));
#99963=CARTESIAN_POINT('Ctrl Pts',(0.00479541363501335,-0.0339738896671456,
0.0693600540095457));
#99964=CARTESIAN_POINT('Ctrl Pts',(0.00486199125732937,-0.0338644633335883,
0.0693151380866326));
#99965=CARTESIAN_POINT('Ctrl Pts',(0.00465187705109948,-0.034193496108874,
0.0695666439252757));
#99966=CARTESIAN_POINT('Ctrl Pts',(0.00471507881640908,-0.0340836138595105,
0.0695187684099579));
#99967=CARTESIAN_POINT('Ctrl Pts',(0.00477924093964432,-0.0339738896671456,
0.0694722236941131));
#99968=CARTESIAN_POINT('Ctrl Pts',(0.00484427730784424,-0.0338644633335883,
0.0694270638443497));
#99969=CARTESIAN_POINT('Origin',(0.0151552659273055,-0.0345610621863334,
0.0825929419776828));
#99970=CARTESIAN_POINT('Ctrl Pts',(0.00462333669442617,-0.03424362768739,
0.0695865576249111));
#99971=CARTESIAN_POINT('Ctrl Pts',(0.00479544976091908,-0.033943005420186,
0.0694545361465294));
#99972=CARTESIAN_POINT('Ctrl Pts',(0.00497701827092622,-0.0336441434784162,
0.0693358539887064));
#99973=CARTESIAN_POINT('Ctrl Pts',(0.00442832686565394,-0.03424362768739,
0.0697429902515664));
#99974=CARTESIAN_POINT('Ctrl Pts',(0.00459453997837069,-0.033943005420186,
0.0696036138562452));
#99975=CARTESIAN_POINT('Ctrl Pts',(0.00477077929823152,-0.0336441434784162,
0.0694771532673382));
#99976=CARTESIAN_POINT('Ctrl Pts',(0.00484425460438518,-0.0335235895815127,
0.0694270797632955));
#99977=CARTESIAN_POINT('Ctrl Pts',(0.00490927490001677,-0.0334144449262719,
0.0693819306092417));
#99978=CARTESIAN_POINT('Ctrl Pts',(0.00497530264363483,-0.0333049234473133,
0.0693380728546543));
#99979=CARTESIAN_POINT('Ctrl Pts',(0.00504225848605051,-0.0331951640388588,
0.0692955702280998));
#99980=CARTESIAN_POINT('Ctrl Pts',(0.00473319323446622,-0.0335235895815127,
0.069404573217625));
#99981=CARTESIAN_POINT('Ctrl Pts',(0.00479852337701027,-0.0334144449262719,
0.0693578950851545));
#99982=CARTESIAN_POINT('Ctrl Pts',(0.00486489291106075,-0.0333049234473133,
0.0693125129967436));
#99983=CARTESIAN_POINT('Ctrl Pts',(0.00493222222694669,-0.0331951640388588,
0.069268492669703));
#99984=CARTESIAN_POINT('Ctrl Pts',(0.00462213186454726,-0.0335235895815127,
0.0693820666719544));
#99985=CARTESIAN_POINT('Ctrl Pts',(0.00468777185400377,-0.0334144449262719,
0.0693338595610674));
#99986=CARTESIAN_POINT('Ctrl Pts',(0.00475448317848668,-0.0333049234473133,
0.0692869531388329));
#99987=CARTESIAN_POINT('Ctrl Pts',(0.00482218596784287,-0.0331951640388588,
0.0692414151113062));
#99988=CARTESIAN_POINT('Ctrl Pts',(0.0045110704946283,-0.0335235895815127,
0.0693595601262839));
#99989=CARTESIAN_POINT('Ctrl Pts',(0.00457702033099727,-0.0334144449262719,
0.0693098240369803));
#99990=CARTESIAN_POINT('Ctrl Pts',(0.00464407344591261,-0.0333049234473133,
0.0692613932809222));
#99991=CARTESIAN_POINT('Ctrl Pts',(0.00471214970873905,-0.0331951640388588,
0.0692143375529094));
#99992=CARTESIAN_POINT('Origin',(0.013322660867038,-0.032643457176965,0.0837602090924077));
#99993=CARTESIAN_POINT('Ctrl Pts',(0.00500722392808472,-0.0336938721132358,
0.0690211321799775));
#99994=CARTESIAN_POINT('Ctrl Pts',(0.00503724489337306,-0.0336474569764942,
0.0690028899302693));
#99995=CARTESIAN_POINT('Ctrl Pts',(0.00506747735017109,-0.033601104548885,
0.0689850003638347));
#99996=CARTESIAN_POINT('Ctrl Pts',(0.00514401897661511,-0.0334837508643153,
0.068939708096639));
#99997=CARTESIAN_POINT('Ctrl Pts',(0.00522186909534638,-0.0333660264760389,
0.0688967038054583));
#99998=CARTESIAN_POINT('Ctrl Pts',(0.00494687938260966,-0.0336938721132358,
0.0693556894622223));
#99999=CARTESIAN_POINT('Ctrl Pts',(0.00497494207310721,-0.0336474569764942,
0.0693370939958649));
#100000=CARTESIAN_POINT('Ctrl Pts',(0.00500322052414354,-0.033601104548885,
0.069318828312905));
#100001=CARTESIAN_POINT('Ctrl Pts',(0.00507481505746574,-0.0334837508643153,
0.0692725838051825));
#100002=CARTESIAN_POINT('Ctrl Pts',(0.00514774847233361,-0.0333660264760389,
0.0692284810990089));
#100003=CARTESIAN_POINT('Ctrl Pts',(0.00494687938262152,-0.0336938721132427,
0.0693556894622311));
#100004=CARTESIAN_POINT('Ctrl Pts',(0.00497494207311814,-0.0336474569765026,
0.0693370939958744));
#100005=CARTESIAN_POINT('Ctrl Pts',(0.00500322052415354,-0.0336011045488949,
0.069318828312915));
#100006=CARTESIAN_POINT('Ctrl Pts',(0.00507421877252747,-0.0334847282606778,
0.0692729689589552));
#100007=CARTESIAN_POINT('Ctrl Pts',(0.00514653395549822,-0.0333679869945434,
0.0692292157198786));
#100008=CARTESIAN_POINT('Ctrl Pts',(0.0049468793826056,-0.0336938721132425,
0.069355689462225));
#100009=CARTESIAN_POINT('Ctrl Pts',(0.00504724398280381,-0.0335278710435082,
0.0692891838452165));
#100010=CARTESIAN_POINT('Ctrl Pts',(0.00514965887382696,-0.0333620469224319,
0.0692258490324976));
#100011=CARTESIAN_POINT('Ctrl Pts',(0.00525418552406473,-0.0331951640388601,
0.0691656705609466));
#100012=CARTESIAN_POINT('Ctrl Pts',(0.00487801917727106,-0.0336938721132425,
0.0694035047520867));
#100013=CARTESIAN_POINT('Ctrl Pts',(0.00497738280717072,-0.0335278710435082,
0.0693355576083095));
#100014=CARTESIAN_POINT('Ctrl Pts',(0.00507884228593903,-0.0333620469224319,
0.0692707503857792));
#100015=CARTESIAN_POINT('Ctrl Pts',(0.00518245885172389,-0.0331951640388601,
0.0692090677301882));
#100016=CARTESIAN_POINT('Ctrl Pts',(0.00480915897193652,-0.0336938721132425,
0.0694513200419484));
#100017=CARTESIAN_POINT('Ctrl Pts',(0.00490752163153764,-0.0335278710435082,
0.0693819313714024));
#100018=CARTESIAN_POINT('Ctrl Pts',(0.00500802569805109,-0.0333620469224319,
0.0693156517390608));
#100019=CARTESIAN_POINT('Ctrl Pts',(0.00511073217938306,-0.0331951640388601,
0.0692524648994298));
#100020=CARTESIAN_POINT('Ctrl Pts',(0.00474029876660199,-0.0336938721132425,
0.0694991353318102));
#100021=CARTESIAN_POINT('Ctrl Pts',(0.00483766045590456,-0.0335278710435082,
0.0694283051344953));
#100022=CARTESIAN_POINT('Ctrl Pts',(0.00493720911016316,-0.0333620469224319,
0.0693605530923424));
#100023=CARTESIAN_POINT('Ctrl Pts',(0.00503900550704223,-0.0331951640388601,
0.0692958620686714));
#100024=CARTESIAN_POINT('Ctrl Pts',(0.00514727936371654,-0.0330240426238155,
0.069230476477689));
#100025=CARTESIAN_POINT('Ctrl Pts',(0.00521505059309556,-0.0329142774063509,
0.0691894722513481));
#100026=CARTESIAN_POINT('Ctrl Pts',(0.00528370328080219,-0.0328043479726686,
0.0691498486035259));
#100027=CARTESIAN_POINT('Ctrl Pts',(0.00535315087557508,-0.0326943950436594,
0.0691116587171717));
#100028=CARTESIAN_POINT('Ctrl Pts',(0.005037850496551,-0.0330240426238155,
0.0692010408017928));
#100029=CARTESIAN_POINT('Ctrl Pts',(0.00510602723104327,-0.0329142774063509,
0.0691585290861954));
#100030=CARTESIAN_POINT('Ctrl Pts',(0.00517511679003615,-0.0328043479726686,
0.0691174055805016));
#100031=CARTESIAN_POINT('Ctrl Pts',(0.00524503211551944,-0.0326943950436594,
0.0690777254045036));
#100032=CARTESIAN_POINT('Ctrl Pts',(0.00492842162938546,-0.0330240426238155,
0.0691716051258966));
#100033=CARTESIAN_POINT('Ctrl Pts',(0.00499700386899099,-0.0329142774063509,
0.0691275859210426));
#100034=CARTESIAN_POINT('Ctrl Pts',(0.00506653029927011,-0.0328043479726686,
0.0690849625574773));
#100035=CARTESIAN_POINT('Ctrl Pts',(0.00513691335546381,-0.0326943950436594,
0.0690437920918355));
#100036=CARTESIAN_POINT('Ctrl Pts',(0.00481899276221992,-0.0330240426238155,
0.0691421694500005));
#100037=CARTESIAN_POINT('Ctrl Pts',(0.00488798050693871,-0.0329142774063509,
0.0690966427558899));
#100038=CARTESIAN_POINT('Ctrl Pts',(0.00495794380850407,-0.0328043479726686,
0.069052519534453));
#100039=CARTESIAN_POINT('Ctrl Pts',(0.00502879459540817,-0.0326943950436594,
0.0690098587791674));
#100040=CARTESIAN_POINT('Origin',(0.0133839226643085,-0.0326396682856107,
0.0838676446126732));
#100041=CARTESIAN_POINT('Ctrl Pts',(0.00533493353088823,-0.0331951640388587,
0.0688375313516922));
#100042=CARTESIAN_POINT('Ctrl Pts',(0.00540810203948209,-0.0330855618255041,
0.0687991206031651));
#100043=CARTESIAN_POINT('Ctrl Pts',(0.00548211717874542,-0.0329757224427708,
0.068762194432868));
#100044=CARTESIAN_POINT('Ctrl Pts',(0.00555688648733464,-0.0328657862078596,
0.0687268047761767));
#100045=CARTESIAN_POINT('Ctrl Pts',(0.00530785599404896,-0.0331951640388587,
0.0689475675231918));
#100046=CARTESIAN_POINT('Ctrl Pts',(0.00537950897698177,-0.0330855618255041,
0.0689087838363721));
#100047=CARTESIAN_POINT('Ctrl Pts',(0.00545201520605982,-0.0329757224427708,
0.0688714531356117));
#100048=CARTESIAN_POINT('Ctrl Pts',(0.00552528417759984,-0.0328657862078596,
0.0688356277795307));
#100049=CARTESIAN_POINT('Ctrl Pts',(0.00528077845720969,-0.0331951640388587,
0.0690576036946913));
#100050=CARTESIAN_POINT('Ctrl Pts',(0.00535091591448146,-0.0330855618255041,
0.0690184470695791));
#100051=CARTESIAN_POINT('Ctrl Pts',(0.00542191323337422,-0.0329757224427708,
0.0689807118383553));
#100052=CARTESIAN_POINT('Ctrl Pts',(0.00549368186786503,-0.0328657862078596,
0.0689444507828847));
#100053=CARTESIAN_POINT('Ctrl Pts',(0.00525370092037042,-0.0331951640388587,
0.0691676398661909));
#100054=CARTESIAN_POINT('Ctrl Pts',(0.00532232285198114,-0.0330855618255041,
0.0691281103027861));
#100055=CARTESIAN_POINT('Ctrl Pts',(0.00539181126068862,-0.0329757224427708,
0.0690899705410989));
#100056=CARTESIAN_POINT('Ctrl Pts',(0.00546207955813023,-0.0328657862078596,
0.0690532737862387));
#100057=CARTESIAN_POINT('Origin',(0.0129440085191781,-0.0326401908833561,
0.0840619341299403));
#100058=CARTESIAN_POINT('Ctrl Pts',(0.00522295231765763,-0.0332451089994432,
0.0691837830259146));
#100059=CARTESIAN_POINT('Ctrl Pts',(0.00541025625528785,-0.0329451141710258,
0.0690743764371766));
#100060=CARTESIAN_POINT('Ctrl Pts',(0.00560526903372078,-0.0326442513127503,
0.0689793891592973));
#100061=CARTESIAN_POINT('Ctrl Pts',(0.00500987234511869,-0.0332451089994432,
0.0693145382372938));
#100062=CARTESIAN_POINT('Ctrl Pts',(0.00519224476926797,-0.0329451141710258,
0.0691970952059085));
#100063=CARTESIAN_POINT('Ctrl Pts',(0.00538294538184271,-0.0326442513127503,
0.0690937228543116));
#100064=CARTESIAN_POINT('Ctrl Pts',(0.00546205151731605,-0.0325229783203385,
0.0690532883290438));
#100065=CARTESIAN_POINT('Ctrl Pts',(0.00553230957496362,-0.0324130253112079,
0.0690165964305541));
#100066=CARTESIAN_POINT('Ctrl Pts',(0.00560331599564085,-0.0323031222247694,
0.0689813634752584));
#100067=CARTESIAN_POINT('Ctrl Pts',(0.00567497823265307,-0.0321934096636184,
0.0689476313845928));
#100068=CARTESIAN_POINT('Ctrl Pts',(0.00535468683073835,-0.0325229783203385,
0.0690170396500961));
#100069=CARTESIAN_POINT('Ctrl Pts',(0.0054254445756234,-0.0324130253112079,
0.0689788677317768));
#100070=CARTESIAN_POINT('Ctrl Pts',(0.00549698122386161,-0.0323031222247694,
0.0689421653177977));
#100071=CARTESIAN_POINT('Ctrl Pts',(0.00556920348315531,-0.0321934096636184,
0.0689069761879008));
#100072=CARTESIAN_POINT('Ctrl Pts',(0.00524732214416064,-0.0325229783203385,
0.0689807909711484));
#100073=CARTESIAN_POINT('Ctrl Pts',(0.00531857957628318,-0.0324130253112079,
0.0689411390329995));
#100074=CARTESIAN_POINT('Ctrl Pts',(0.00539064645208236,-0.0323031222247694,
0.068902967160337));
#100075=CARTESIAN_POINT('Ctrl Pts',(0.00546342873365755,-0.0321934096636184,
0.0688663209912088));
#100076=CARTESIAN_POINT('Ctrl Pts',(0.00513995745758293,-0.0325229783203385,
0.0689445422922008));
#100077=CARTESIAN_POINT('Ctrl Pts',(0.00521171457694297,-0.0324130253112079,
0.0689034103342222));
#100078=CARTESIAN_POINT('Ctrl Pts',(0.00528431168030312,-0.0323031222247694,
0.0688637690028764));
#100079=CARTESIAN_POINT('Ctrl Pts',(0.00535765398415979,-0.0321934096636184,
0.0688256657945168));
#100080=CARTESIAN_POINT('Origin',(0.0133800753187604,-0.0326393375177818,
0.0838600361333332));
#100081=CARTESIAN_POINT('Ctrl Pts',(0.00567400935308162,-0.0326943950436593,
0.0686729010386623));
#100082=CARTESIAN_POINT('Ctrl Pts',(0.00574949404194613,-0.0325844576448127,
0.0686391385775631));
#100083=CARTESIAN_POINT('Ctrl Pts',(0.00582568233602918,-0.0324744968375319,
0.0686069348741667));
#100084=CARTESIAN_POINT('Ctrl Pts',(0.00590247604932843,-0.0323646534831894,
0.0685763298433056));
#100085=CARTESIAN_POINT('Ctrl Pts',(0.00564007605151625,-0.0326943950436593,
0.0687810197633423));
#100086=CARTESIAN_POINT('Ctrl Pts',(0.00571407066171858,-0.0325844576448127,
0.0687467896377499));
#100087=CARTESIAN_POINT('Ctrl Pts',(0.00578877844375275,-0.0324744968375319,
0.068714087419493));
#100088=CARTESIAN_POINT('Ctrl Pts',(0.00586410309972482,-0.0323646534831894,
0.0686829536882949));
#100089=CARTESIAN_POINT('Ctrl Pts',(0.00560614274995088,-0.0326943950436593,
0.0688891384880224));
#100090=CARTESIAN_POINT('Ctrl Pts',(0.00567864728149104,-0.0325844576448127,
0.0688544406979365));
#100091=CARTESIAN_POINT('Ctrl Pts',(0.00575187455147631,-0.0324744968375319,
0.0688212399648193));
#100092=CARTESIAN_POINT('Ctrl Pts',(0.00582573015012121,-0.0323646534831894,
0.0687895775332841));
#100093=CARTESIAN_POINT('Ctrl Pts',(0.00557220944838551,-0.0326943950436593,
0.0689972572127024));
#100094=CARTESIAN_POINT('Ctrl Pts',(0.00564322390126349,-0.0325844576448127,
0.0689620917581233));
#100095=CARTESIAN_POINT('Ctrl Pts',(0.00571497065919988,-0.0324744968375319,
0.0689283925101456));
#100096=CARTESIAN_POINT('Ctrl Pts',(0.0057873572005176,-0.0323646534831894,
0.0688962013782734));
#100097=CARTESIAN_POINT('Origin',(0.0129609683792565,-0.0326395579068092,
0.0840957620033715));
#100098=CARTESIAN_POINT('Ctrl Pts',(0.00554047274258514,-0.0327445246961877,
0.0690114557233747));
#100099=CARTESIAN_POINT('Ctrl Pts',(0.00573427610621507,-0.0324436878365475,
0.0689140246156803));
#100100=CARTESIAN_POINT('Ctrl Pts',(0.00593486780412998,-0.0321434074463186,
0.068831468360748));
#100101=CARTESIAN_POINT('Ctrl Pts',(0.00531960384577433,-0.0327445246961877,
0.0691285750233282));
#100102=CARTESIAN_POINT('Ctrl Pts',(0.00550898998284065,-0.0324436878365475,
0.0690228137090968));
#100103=CARTESIAN_POINT('Ctrl Pts',(0.00570580446826165,-0.0321434074463186,
0.0689316181893094));
#100104=CARTESIAN_POINT('Ctrl Pts',(0.00587336811646014,-0.0322357242816072,
0.0688571971996282));
#100105=CARTESIAN_POINT('Ctrl Pts',(0.0060419370211382,-0.0319819883628705,
0.068785524429967));
#100106=CARTESIAN_POINT('Ctrl Pts',(0.00621472504338505,-0.0317295851069887,
0.0687247234357048));
#100107=CARTESIAN_POINT('Ctrl Pts',(0.00564548099814133,-0.0322357242816072,
0.0689599953577067));
#100108=CARTESIAN_POINT('Ctrl Pts',(0.00581077591480891,-0.0319819883628705,
0.0688810646788859));
#100109=CARTESIAN_POINT('Ctrl Pts',(0.0059807584257111,-0.0317295851069887,
0.0688128121512944));
#100110=CARTESIAN_POINT('Origin',(0.0129208253933554,-0.0326371942645984,
0.0840093273795378));
#100111=CARTESIAN_POINT('Origin',(0.0133242262562021,-0.0326352985528889,
0.0837507443898176));
#100112=CARTESIAN_POINT('Ctrl Pts',(0.00602275330948016,-0.0321934096636183,
0.0685298863329836));
#100113=CARTESIAN_POINT('Ctrl Pts',(0.00610025905699843,-0.0320835708272303,
0.068500911507236));
#100114=CARTESIAN_POINT('Ctrl Pts',(0.00617831948054618,-0.0319739230346346,
0.0684735574654815));
#100115=CARTESIAN_POINT('Ctrl Pts',(0.00625683202125929,-0.0318646057455576,
0.0684478515403528));
#100116=CARTESIAN_POINT('Ctrl Pts',(0.00598209807777947,-0.0321934096636183,
0.0686356611735653));
#100117=CARTESIAN_POINT('Ctrl Pts',(0.00605814510781022,-0.0320835708272303,
0.0686061256804878));
#100118=CARTESIAN_POINT('Ctrl Pts',(0.00613475926296713,-0.0319739230346346,
0.0685781811085306));
#100119=CARTESIAN_POINT('Ctrl Pts',(0.00621183977680037,-0.0318646057455576,
0.068551855687882));
#100120=CARTESIAN_POINT('Ctrl Pts',(0.00594144284607878,-0.0321934096636183,
0.068741436014147));
#100121=CARTESIAN_POINT('Ctrl Pts',(0.00601603115862201,-0.0320835708272303,
0.0687113398537396));
#100122=CARTESIAN_POINT('Ctrl Pts',(0.00609119904538808,-0.0319739230346346,
0.0686828047515797));
#100123=CARTESIAN_POINT('Ctrl Pts',(0.00616684753234146,-0.0318646057455576,
0.0686558598354111));
#100124=CARTESIAN_POINT('Ctrl Pts',(0.00590078761437809,-0.0321934096636183,
0.0688472108547287));
#100125=CARTESIAN_POINT('Ctrl Pts',(0.0059739172094338,-0.0320835708272303,
0.0688165540269914));
#100126=CARTESIAN_POINT('Ctrl Pts',(0.00604763882780903,-0.0319739230346346,
0.0687874283946289));
#100127=CARTESIAN_POINT('Ctrl Pts',(0.00612185528788254,-0.0318646057455576,
0.0687598639829403));
#100128=CARTESIAN_POINT('Ctrl Pts',(0.0057865917572633,-0.0320218834582364,
0.0688956362262419));
#100129=CARTESIAN_POINT('Ctrl Pts',(0.0058412769818047,-0.0319391099350667,
0.0688713117239265));
#100130=CARTESIAN_POINT('Ctrl Pts',(0.00589630890447229,-0.0318564869454955,
0.0688478558766581));
#100131=CARTESIAN_POINT('Ctrl Pts',(0.00595164584685598,-0.0317740741446555,
0.0688252820268415));
#100132=CARTESIAN_POINT('Ctrl Pts',(0.0057407191058014,-0.0320218834582364,
0.0688768605000231));
#100133=CARTESIAN_POINT('Ctrl Pts',(0.00579559974026271,-0.0319391099350667,
0.0688520585743025));
#100134=CARTESIAN_POINT('Ctrl Pts',(0.00585083440948972,-0.0318564869454955,
0.0688281286442408));
#100135=CARTESIAN_POINT('Ctrl Pts',(0.00590638125516161,-0.0317740741446555,
0.0688050843837629));
#100136=CARTESIAN_POINT('Ctrl Pts',(0.00569484645433949,-0.0320218834582364,
0.0688580847738044));
#100137=CARTESIAN_POINT('Ctrl Pts',(0.00574992249872072,-0.0319391099350667,
0.0688328054246785));
#100138=CARTESIAN_POINT('Ctrl Pts',(0.00580535991450715,-0.0318564869454955,
0.0688084014118235));
#100139=CARTESIAN_POINT('Ctrl Pts',(0.00586111666346724,-0.0317740741446555,
0.0687848867406844));
#100140=CARTESIAN_POINT('Ctrl Pts',(0.00564897380287759,-0.0320218834582364,
0.0688393090475856));
#100141=CARTESIAN_POINT('Ctrl Pts',(0.00570424525717873,-0.0319391099350667,
0.0688135522750544));
#100142=CARTESIAN_POINT('Ctrl Pts',(0.00575988541952458,-0.0318564869454955,
0.0687886741794062));
#100143=CARTESIAN_POINT('Ctrl Pts',(0.00581585207177287,-0.0317740741446555,
0.0687646890976059));
#100144=CARTESIAN_POINT('Origin',(0.00236941910510931,-0.0391228853390649,
0.0635307757448714));
#100145=CARTESIAN_POINT('Ctrl Pts',(0.00343631067228798,-0.0352722978779595,
0.070816567042208));
#100146=CARTESIAN_POINT('Ctrl Pts',(0.00344754559313125,-0.0352466642097217,
0.0708013726606252));
#100147=CARTESIAN_POINT('Ctrl Pts',(0.00345870746525495,-0.0352210183808301,
0.0707861452031262));
#100148=CARTESIAN_POINT('Ctrl Pts',(0.00346979625305581,-0.0351953608940152,
0.0707708838175277));
#100149=CARTESIAN_POINT('Origin',(-0.000393203979565928,-0.0352456003065074,
0.0677596796176656));
#100150=CARTESIAN_POINT('Ctrl Pts',(0.00354530261829435,-0.0350241211493339,
0.0706716663582445));
#100151=CARTESIAN_POINT('Ctrl Pts',(0.00359321523587681,-0.0349144232867421,
0.0706085996821949));
#100152=CARTESIAN_POINT('Ctrl Pts',(0.00364246016466918,-0.0348045283677512,
0.0705464856456987));
#100153=CARTESIAN_POINT('Ctrl Pts',(0.00369297728879991,-0.0346945769586886,
0.0704854061561595));
#100154=CARTESIAN_POINT('Ctrl Pts',(0.0034327222098805,-0.0350241211493339,
0.0706845812118786));
#100155=CARTESIAN_POINT('Ctrl Pts',(0.00348045693065747,-0.0349144232867421,
0.0706199637869327));
#100156=CARTESIAN_POINT('Ctrl Pts',(0.00352955591125088,-0.0348045283677512,
0.0705562943960884));
#100157=CARTESIAN_POINT('Ctrl Pts',(0.00357995929686508,-0.0346945769586886,
0.070493656932004));
#100158=CARTESIAN_POINT('Ctrl Pts',(0.00332014180146665,-0.0350241211493339,
0.0706974960655126));
#100159=CARTESIAN_POINT('Ctrl Pts',(0.00336769862543812,-0.0349144232867421,
0.0706313278916705));
#100160=CARTESIAN_POINT('Ctrl Pts',(0.00341665165783259,-0.0348045283677512,
0.0705661031464782));
#100161=CARTESIAN_POINT('Ctrl Pts',(0.00346694130493024,-0.0346945769586886,
0.0705019077078485));
#100162=CARTESIAN_POINT('Ctrl Pts',(0.00320756139305279,-0.0350241211493339,
0.0707104109191467));
#100163=CARTESIAN_POINT('Ctrl Pts',(0.00325494032021878,-0.0349144232867421,
0.0706426919964084));
#100164=CARTESIAN_POINT('Ctrl Pts',(0.00330374740441429,-0.0348045283677512,
0.070575911896868));
#100165=CARTESIAN_POINT('Ctrl Pts',(0.00335392331299541,-0.0346945769586886,
0.070510158483693));
#100166=CARTESIAN_POINT('Origin',(0.0165147080052373,-0.0345629067943449,
0.0813235873006996));
#100167=CARTESIAN_POINT('Ctrl Pts',(0.00358672921891514,-0.0351970973651648,
0.0703302261733762));
#100168=CARTESIAN_POINT('Ctrl Pts',(0.00363964700857392,-0.0350869349321788,
0.070267371453213));
#100169=CARTESIAN_POINT('Ctrl Pts',(0.00369391534951389,-0.0349764985129721,
0.0702055647964528));
#100170=CARTESIAN_POINT('Ctrl Pts',(0.00374946864903189,-0.0348659306849623,
0.0701448904140705));
#100171=CARTESIAN_POINT('Ctrl Pts',(0.00359787316825978,-0.0351970973651648,
0.0704116895580534));
#100172=CARTESIAN_POINT('Ctrl Pts',(0.00364966239312627,-0.0350869349321788,
0.0703489892222056));
#100173=CARTESIAN_POINT('Ctrl Pts',(0.00370279802481965,-0.0349764985129721,
0.0702873136154144));
#100174=CARTESIAN_POINT('Ctrl Pts',(0.00375721592810065,-0.0348659306849623,
0.0702267466924924));
#100175=CARTESIAN_POINT('Ctrl Pts',(0.00360901711760441,-0.0351970973651648,
0.0704931529427305));
#100176=CARTESIAN_POINT('Ctrl Pts',(0.00365967777767861,-0.0350869349321788,
0.0704306069911982));
#100177=CARTESIAN_POINT('Ctrl Pts',(0.0037116807001254,-0.0349764985129721,
0.0703690624343759));
#100178=CARTESIAN_POINT('Ctrl Pts',(0.00376496320716942,-0.0348659306849623,
0.0703086029709142));
#100179=CARTESIAN_POINT('Ctrl Pts',(0.00362016106694905,-0.0351970973651648,
0.0705746163274077));
#100180=CARTESIAN_POINT('Ctrl Pts',(0.00366969316223096,-0.0350869349321788,
0.0705122247601908));
#100181=CARTESIAN_POINT('Ctrl Pts',(0.00372056337543116,-0.0349764985129721,
0.0704508112533375));
#100182=CARTESIAN_POINT('Ctrl Pts',(0.00377271048623818,-0.0348659306849623,
0.0703904592493361));
#100183=CARTESIAN_POINT('Origin',(0.0161690093029537,-0.0345637187966485,
0.0816579789329045));
#100184=CARTESIAN_POINT('Ctrl Pts',(0.00359847610634473,-0.0352450361861253,
0.0706003901874853));
#100185=CARTESIAN_POINT('Ctrl Pts',(0.00373235183377771,-0.0349452761023764,
0.0704297154721725));
#100186=CARTESIAN_POINT('Ctrl Pts',(0.00387870315195259,-0.0346444289983475,
0.0702696096930411));
#100187=CARTESIAN_POINT('Ctrl Pts',(0.00344849335217477,-0.0352450361861253,
0.0708004031206961));
#100188=CARTESIAN_POINT('Ctrl Pts',(0.00357482546824089,-0.0349452761023764,
0.0706240717131334));
#100189=CARTESIAN_POINT('Ctrl Pts',(0.00371408069084825,-0.0346444289983475,
0.0704577570961589));
#100190=CARTESIAN_POINT('Ctrl Pts',(0.00377274290153435,-0.0345231616327822,
0.0703910456445689));
#100191=CARTESIAN_POINT('Ctrl Pts',(0.00382455479513922,-0.0344132092796975,
0.0703310726937082));
#100192=CARTESIAN_POINT('Ctrl Pts',(0.00387760450867109,-0.0343032738558974,
0.0702721745253267));
#100193=CARTESIAN_POINT('Ctrl Pts',(0.00393182214649865,-0.0341934961088741,
0.0702144248538919));
#100194=CARTESIAN_POINT('Ctrl Pts',(0.00365957374036347,-0.0345231616327822,
0.0703968660481945));
#100195=CARTESIAN_POINT('Ctrl Pts',(0.00371130540789883,-0.0344132092796975,
0.0703353332197765));
#100196=CARTESIAN_POINT('Ctrl Pts',(0.00376430716433736,-0.0343032738558974,
0.0702748735949072));
#100197=CARTESIAN_POINT('Ctrl Pts',(0.00381850912424515,-0.0341934961088741,
0.0702155628900342));
#100198=CARTESIAN_POINT('Ctrl Pts',(0.00354640457919259,-0.0345231616327822,
0.07040268645182));
#100199=CARTESIAN_POINT('Ctrl Pts',(0.00359805602065845,-0.0344132092796975,
0.0703395937458448));
#100200=CARTESIAN_POINT('Ctrl Pts',(0.00365100982000363,-0.0343032738558974,
0.0702775726644878));
#100201=CARTESIAN_POINT('Ctrl Pts',(0.00370519610199164,-0.0341934961088741,
0.0702167009261765));
#100202=CARTESIAN_POINT('Ctrl Pts',(0.00343323541802172,-0.0345231616327822,
0.0704085068554456));
#100203=CARTESIAN_POINT('Ctrl Pts',(0.00348480663341807,-0.0344132092796975,
0.0703438542719131));
#100204=CARTESIAN_POINT('Ctrl Pts',(0.00353771247566989,-0.0343032738558974,
0.0702802717340683));
#100205=CARTESIAN_POINT('Ctrl Pts',(0.00359188307973814,-0.0341934961088741,
0.0702178389623189));
#100206=CARTESIAN_POINT('Origin',(0.0165240686837907,-0.0345625596230435,
0.0813312603696003));
#100207=CARTESIAN_POINT('Ctrl Pts',(0.00382978640553166,-0.0346945769586885,
0.0699593437057787));
#100208=CARTESIAN_POINT('Ctrl Pts',(0.00388753576742504,-0.0345846629176052,
0.0699001702734341));
#100209=CARTESIAN_POINT('Ctrl Pts',(0.00394651867533112,-0.0344746925050311,
0.0698421809672095));
#100210=CARTESIAN_POINT('Ctrl Pts',(0.00400665924669232,-0.0343648066253259,
0.0697854497775696));
#100211=CARTESIAN_POINT('Ctrl Pts',(0.00383803717487975,-0.0346945769586885,
0.0700723616087268));
#100212=CARTESIAN_POINT('Ctrl Pts',(0.00389422909294583,-0.0345846629176052,
0.0700133018761542));
#100213=CARTESIAN_POINT('Ctrl Pts',(0.00395165193974478,-0.0344746925050311,
0.069955394081823));
#100214=CARTESIAN_POINT('Ctrl Pts',(0.00401023183208043,-0.0343648066253259,
0.0698987121200108));
#100215=CARTESIAN_POINT('Ctrl Pts',(0.00384628794422784,-0.0346945769586885,
0.070185379511675));
#100216=CARTESIAN_POINT('Ctrl Pts',(0.00390092241846661,-0.0345846629176052,
0.0701264334788743));
#100217=CARTESIAN_POINT('Ctrl Pts',(0.00395678520415844,-0.0344746925050311,
0.0700686071964365));
#100218=CARTESIAN_POINT('Ctrl Pts',(0.00401380441746853,-0.0343648066253259,
0.070011974462452));
#100219=CARTESIAN_POINT('Ctrl Pts',(0.00385453871357593,-0.0346945769586885,
0.0702983974146231));
#100220=CARTESIAN_POINT('Ctrl Pts',(0.0039076157439874,-0.0345846629176052,
0.0702395650815944));
#100221=CARTESIAN_POINT('Ctrl Pts',(0.0039619184685721,-0.0344746925050311,
0.07018182031105));
#100222=CARTESIAN_POINT('Ctrl Pts',(0.00401737700285664,-0.0343648066253259,
0.0701252368048932));
#100223=CARTESIAN_POINT('Origin',(0.0162122550414581,-0.0345626446731979,
0.0816972718927456));
#100224=CARTESIAN_POINT('Ctrl Pts',(0.00385439107964542,-0.0346945769586885,
0.070296375145362));
#100225=CARTESIAN_POINT('Ctrl Pts',(0.00393510679513173,-0.034527515336289,
0.070206951039121));
#100226=CARTESIAN_POINT('Ctrl Pts',(0.00401865569366838,-0.0343603235965158,
0.0701200422381841));
#100227=CARTESIAN_POINT('Ctrl Pts',(0.004104786854452,-0.0341934961088739,
0.0700359021076476));
#100228=CARTESIAN_POINT('Ctrl Pts',(0.00379958542914434,-0.0346945769586885,
0.0703598130599275));
#100229=CARTESIAN_POINT('Ctrl Pts',(0.00387897241211095,-0.034527515336289,
0.0702692410273938));
#100230=CARTESIAN_POINT('Ctrl Pts',(0.00396122833567491,-0.0343603235965158,
0.0701811422158369));
#100231=CARTESIAN_POINT('Ctrl Pts',(0.0040461060507696,-0.0341934961088739,
0.0700957735667116));
#100232=CARTESIAN_POINT('Ctrl Pts',(0.00374477977864326,-0.0346945769586885,
0.070423250974493));
#100233=CARTESIAN_POINT('Ctrl Pts',(0.00382283802909016,-0.034527515336289,
0.0703315310156666));
#100234=CARTESIAN_POINT('Ctrl Pts',(0.00390380097768144,-0.0343603235965158,
0.0702422421934897));
#100235=CARTESIAN_POINT('Ctrl Pts',(0.0039874252470872,-0.0341934961088739,
0.0701556450257756));
#100236=CARTESIAN_POINT('Ctrl Pts',(0.00368997412814219,-0.0346945769586885,
0.0704866888890586));
#100237=CARTESIAN_POINT('Ctrl Pts',(0.00376670364606938,-0.034527515336289,
0.0703938210039394));
#100238=CARTESIAN_POINT('Ctrl Pts',(0.00384637361968797,-0.0343603235965158,
0.0703033421711425));
#100239=CARTESIAN_POINT('Ctrl Pts',(0.0039287444434048,-0.0341934961088739,
0.0702155164848397));
#100240=CARTESIAN_POINT('Ctrl Pts',(0.00401735531343243,-0.0340223579322365,
0.0701252597298641));
#100241=CARTESIAN_POINT('Ctrl Pts',(0.00407286697872035,-0.0339125849573554,
0.0700686213931831));
#100242=CARTESIAN_POINT('Ctrl Pts',(0.00412951191856377,-0.0338030433565221,
0.0700131718180855));
#100243=CARTESIAN_POINT('Ctrl Pts',(0.00418721140770106,-0.0336938721132328,
0.0699589754937896));
#100244=CARTESIAN_POINT('Ctrl Pts',(0.00390404380660431,-0.0340223579322365,
0.0701239627137924));
#100245=CARTESIAN_POINT('Ctrl Pts',(0.00395957336112662,-0.0339125849573554,
0.0700657615159034));
#100246=CARTESIAN_POINT('Ctrl Pts',(0.00401626852522929,-0.0338030433565221,
0.070008750548068));
#100247=CARTESIAN_POINT('Ctrl Pts',(0.00407405033241811,-0.0336938721132328,
0.0699529962905688));
#100248=CARTESIAN_POINT('Ctrl Pts',(0.00379073229977619,-0.0340223579322365,
0.0701226656977207));
#100249=CARTESIAN_POINT('Ctrl Pts',(0.00384627974353289,-0.0339125849573554,
0.0700629016386237));
#100250=CARTESIAN_POINT('Ctrl Pts',(0.0039030251318948,-0.0338030433565221,
0.0700043292780504));
#100251=CARTESIAN_POINT('Ctrl Pts',(0.00396088925713516,-0.0336938721132328,
0.0699470170873479));
#100252=CARTESIAN_POINT('Ctrl Pts',(0.00367742079294807,-0.0340223579322365,
0.070121368681649));
#100253=CARTESIAN_POINT('Ctrl Pts',(0.00373298612593915,-0.0339125849573554,
0.0700600417613441));
#100254=CARTESIAN_POINT('Ctrl Pts',(0.00378978173856031,-0.0338030433565221,
0.0699999080080329));
#100255=CARTESIAN_POINT('Ctrl Pts',(0.00384772818185221,-0.0336938721132328,
0.069941037884127));
#100256=CARTESIAN_POINT('Origin',(0.0164343948347533,-0.0345589643415299,
0.0812511886584912));
#100257=CARTESIAN_POINT('Ctrl Pts',(0.00410139311123136,-0.034193496108874,
0.0696979907823524));
#100258=CARTESIAN_POINT('Ctrl Pts',(0.00416278368118548,-0.0340836138595105,
0.0696425244195842));
#100259=CARTESIAN_POINT('Ctrl Pts',(0.00422529255476902,-0.0339738896671456,
0.0695883550196333));
#100260=CARTESIAN_POINT('Ctrl Pts',(0.00428883508080599,-0.0338644633335883,
0.0695355465496046));
#100261=CARTESIAN_POINT('Ctrl Pts',(0.00410253114839765,-0.034193496108874,
0.0698113039065627));
#100262=CARTESIAN_POINT('Ctrl Pts',(0.00416235919749018,-0.0340836138595105,
0.0697558532366529));
#100263=CARTESIAN_POINT('Ctrl Pts',(0.00422330597520824,-0.0339738896671456,
0.0697016671889405));
#100264=CARTESIAN_POINT('Ctrl Pts',(0.00428528882823726,-0.0338644633335883,
0.0696488098858596));
#100265=CARTESIAN_POINT('Ctrl Pts',(0.00410366918556394,-0.034193496108874,
0.069924617030773));
#100266=CARTESIAN_POINT('Ctrl Pts',(0.00416193471379489,-0.0340836138595105,
0.0698691820537216));
#100267=CARTESIAN_POINT('Ctrl Pts',(0.00422131939564746,-0.0339738896671456,
0.0698149793582477));
#100268=CARTESIAN_POINT('Ctrl Pts',(0.00428174257566853,-0.0338644633335883,
0.0697620732221146));
#100269=CARTESIAN_POINT('Ctrl Pts',(0.00410480722273024,-0.034193496108874,
0.0700379301549834));
#100270=CARTESIAN_POINT('Ctrl Pts',(0.00416151023009959,-0.0340836138595105,
0.0699825108707904));
#100271=CARTESIAN_POINT('Ctrl Pts',(0.00421933281608668,-0.0339738896671456,
0.0699282915275549));
#100272=CARTESIAN_POINT('Ctrl Pts',(0.00427819632309979,-0.0338644633335883,
0.0698753365583697));
#100273=CARTESIAN_POINT('Origin',(0.0161580017964341,-0.0345610621862345,
0.0816450882651416));
#100274=CARTESIAN_POINT('Ctrl Pts',(0.00407898776366144,-0.03424362768739,
0.0700612638843384));
#100275=CARTESIAN_POINT('Ctrl Pts',(0.00423319698843185,-0.0339430054201859,
0.0699087119475842));
#100276=CARTESIAN_POINT('Ctrl Pts',(0.00439845895789937,-0.0336441434784161,
0.0697682090655518));
#100277=CARTESIAN_POINT('Ctrl Pts',(0.00390512185256935,-0.03424362768739,
0.0702409042054249));
#100278=CARTESIAN_POINT('Ctrl Pts',(0.00405255583093875,-0.0339430054201859,
0.070081794807733));
#100279=CARTESIAN_POINT('Ctrl Pts',(0.0042115557365962,-0.0336441434784161,
0.0699342427545023));
#100280=CARTESIAN_POINT('Ctrl Pts',(0.00427817579383718,-0.0335235895815127,
0.0698753551972878));
#100281=CARTESIAN_POINT('Ctrl Pts',(0.00433702469554684,-0.0334144449262719,
0.0698224128539003));
#100282=CARTESIAN_POINT('Ctrl Pts',(0.00439703495648564,-0.0333049234473133,
0.0697706254601949));
#100283=CARTESIAN_POINT('Ctrl Pts',(0.00445813584046408,-0.0331951640388588,
0.0697200661873098));
#100284=CARTESIAN_POINT('Ctrl Pts',(0.00416516935784719,-0.0335235895815127,
0.0698669458030683));
#100285=CARTESIAN_POINT('Ctrl Pts',(0.00422413403142485,-0.0334144449262719,
0.0698124477036002));
#100286=CARTESIAN_POINT('Ctrl Pts',(0.0042842923379893,-0.0333049234473133,
0.0697591051581987));
#100287=CARTESIAN_POINT('Ctrl Pts',(0.00434557353217863,-0.0331951640388588,
0.0697069933437114));
#100288=CARTESIAN_POINT('Ctrl Pts',(0.0040521629218572,-0.0335235895815127,
0.0698585364088488));
#100289=CARTESIAN_POINT('Ctrl Pts',(0.00411124336730287,-0.0334144449262719,
0.0698024825533001));
#100290=CARTESIAN_POINT('Ctrl Pts',(0.00417154971949296,-0.0333049234473133,
0.0697475848562025));
#100291=CARTESIAN_POINT('Ctrl Pts',(0.00423301122389317,-0.0331951640388588,
0.069693920500113));
#100292=CARTESIAN_POINT('Ctrl Pts',(0.00393915648586722,-0.0335235895815127,
0.0698501270146293));
#100293=CARTESIAN_POINT('Ctrl Pts',(0.00399835270318089,-0.0334144449262719,
0.0697925174030001));
#100294=CARTESIAN_POINT('Ctrl Pts',(0.00405880710099661,-0.0333049234473133,
0.0697360645542062));
#100295=CARTESIAN_POINT('Ctrl Pts',(0.00412044891560771,-0.0331951640388588,
0.0696808476565146));
#100296=CARTESIAN_POINT('Origin',(0.014486144736754,-0.0326434571770401,
0.0830328374481446));
#100297=CARTESIAN_POINT('Ctrl Pts',(0.0043889813324677,-0.0336938721132362,
0.0694521831596041));
#100298=CARTESIAN_POINT('Ctrl Pts',(0.00441647921333464,-0.0336474569764944,
0.069430322130829));
#100299=CARTESIAN_POINT('Ctrl Pts',(0.00444423112097265,-0.033601104548885,
0.0694087844974));
#100300=CARTESIAN_POINT('Ctrl Pts',(0.00451449256752707,-0.0334837508643155,
0.0693542561637148));
#100301=CARTESIAN_POINT('Ctrl Pts',(0.00458633894794849,-0.0333660264760393,
0.0693018337671009));
#100302=CARTESIAN_POINT('Ctrl Pts',(0.00437104376775398,-0.0336938721132362,
0.0697916655347634));
#100303=CARTESIAN_POINT('Ctrl Pts',(0.00439655454562698,-0.0336474569764944,
0.0697696995114698));
#100304=CARTESIAN_POINT('Ctrl Pts',(0.00442232071552202,-0.033601104548885,
0.069748033629167));
#100305=CARTESIAN_POINT('Ctrl Pts',(0.00448755473087715,-0.0334837508643155,
0.0696931805988338));
#100306=CARTESIAN_POINT('Ctrl Pts',(0.00455438550921085,-0.0333660264760393,
0.069640284674951));
#100307=CARTESIAN_POINT('Ctrl Pts',(0.00437104376776591,-0.0336938721132427,
0.0697916655347717));
#100308=CARTESIAN_POINT('Ctrl Pts',(0.00439655454563795,-0.0336474569765026,
0.0697696995114789));
#100309=CARTESIAN_POINT('Ctrl Pts',(0.00442232071553202,-0.0336011045488949,
0.069748033629177));
#100310=CARTESIAN_POINT('Ctrl Pts',(0.00448701142039042,-0.0334847282606778,
0.0696936374498745));
#100311=CARTESIAN_POINT('Ctrl Pts',(0.00455327264161155,-0.0333679869945434,
0.069641165722439));
#100312=CARTESIAN_POINT('Ctrl Pts',(0.00437104376775055,-0.0336938721132425,
0.0697916655347663));
#100313=CARTESIAN_POINT('Ctrl Pts',(0.0044622815990689,-0.0335278710435082,
0.0697131053145341));
#100314=CARTESIAN_POINT('Ctrl Pts',(0.00455595096121121,-0.0333620469224319,
0.0696374339262735));
#100315=CARTESIAN_POINT('Ctrl Pts',(0.00465211102516082,-0.0331951640388601,
0.0695646293168772));
#100316=CARTESIAN_POINT('Ctrl Pts',(0.0043087193905948,-0.0336938721132425,
0.0698477342589842));
#100317=CARTESIAN_POINT('Ctrl Pts',(0.00439878347335318,-0.0335278710435082,
0.0697678693336966));
#100318=CARTESIAN_POINT('Ctrl Pts',(0.00449132041506886,-0.0333620469224319,
0.0696908568909231));
#100319=CARTESIAN_POINT('Ctrl Pts',(0.0045863890466037,-0.0331951640388601,
0.0696166740222545));
#100320=CARTESIAN_POINT('Ctrl Pts',(0.00424639501343906,-0.0336938721132425,
0.0699038029832021));
#100321=CARTESIAN_POINT('Ctrl Pts',(0.00433528534763747,-0.0335278710435082,
0.0698226333528591));
#100322=CARTESIAN_POINT('Ctrl Pts',(0.00442668986892651,-0.0333620469224319,
0.0697442798555727));
#100323=CARTESIAN_POINT('Ctrl Pts',(0.00452066706804658,-0.0331951640388601,
0.0696687187276318));
#100324=CARTESIAN_POINT('Ctrl Pts',(0.00418407063628331,-0.0336938721132425,
0.0699598717074199));
#100325=CARTESIAN_POINT('Ctrl Pts',(0.00427178722192175,-0.0335278710435082,
0.0698773973720216));
#100326=CARTESIAN_POINT('Ctrl Pts',(0.00436205932278417,-0.0333620469224319,
0.0697977028202223));
#100327=CARTESIAN_POINT('Ctrl Pts',(0.00445494508948946,-0.0331951640388601,
0.0697207634330091));
#100328=CARTESIAN_POINT('Ctrl Pts',(0.00455417018691768,-0.0330240426238155,
0.0696423231143738));
#100329=CARTESIAN_POINT('Ctrl Pts',(0.00461626782763365,-0.0329142774063509,
0.0695931482312844));
#100330=CARTESIAN_POINT('Ctrl Pts',(0.00467941300848498,-0.0328043479726686,
0.069545232564417));
#100331=CARTESIAN_POINT('Ctrl Pts',(0.00474352652628386,-0.0326943950436594,
0.0694986397251073));
#100332=CARTESIAN_POINT('Ctrl Pts',(0.00444191493061234,-0.0330240426238155,
0.0696268346213412));
#100333=CARTESIAN_POINT('Ctrl Pts',(0.00450422594040955,-0.0329142774063509,
0.0695761133127312));
#100334=CARTESIAN_POINT('Ctrl Pts',(0.00456761656564961,-0.0328043479726686,
0.0695266548603287));
#100335=CARTESIAN_POINT('Ctrl Pts',(0.00463200734314253,-0.0326943950436594,
0.0694785248605517));
#100336=CARTESIAN_POINT('Ctrl Pts',(0.004329659674307,-0.0330240426238155,
0.0696113461283087));
#100337=CARTESIAN_POINT('Ctrl Pts',(0.00439218405318544,-0.0329142774063509,
0.069559078394178));
#100338=CARTESIAN_POINT('Ctrl Pts',(0.00445582012281424,-0.0328043479726686,
0.0695080771562403));
#100339=CARTESIAN_POINT('Ctrl Pts',(0.0045204881600012,-0.0326943950436594,
0.0694584099959962));
#100340=CARTESIAN_POINT('Ctrl Pts',(0.00421740441800167,-0.0330240426238155,
0.0695958576352761));
#100341=CARTESIAN_POINT('Ctrl Pts',(0.00428014216596133,-0.0329142774063509,
0.0695420434756248));
#100342=CARTESIAN_POINT('Ctrl Pts',(0.00434402367997886,-0.0328043479726686,
0.0694894994521519));
#100343=CARTESIAN_POINT('Ctrl Pts',(0.00440896897685988,-0.0326943950436594,
0.0694382951314406));
#100344=CARTESIAN_POINT('Origin',(0.0145603887075589,-0.0326396682856945,
0.0831317476680125));
#100345=CARTESIAN_POINT('Ctrl Pts',(0.00469109556167719,-0.0331951640388588,
0.069228957174499));
#100346=CARTESIAN_POINT('Ctrl Pts',(0.00475887297930124,-0.0330855618127431,
0.0691816788549149));
#100347=CARTESIAN_POINT('Ctrl Pts',(0.00482767641888813,-0.0329757224171935,
0.0691357672965771));
#100348=CARTESIAN_POINT('Ctrl Pts',(0.0048974206573781,-0.0328657861694599,
0.0690912856138361));
#100349=CARTESIAN_POINT('Ctrl Pts',(0.00467802272848662,-0.0331951640388588,
0.0693415193931692));
#100350=CARTESIAN_POINT('Ctrl Pts',(0.0047442498290795,-0.0330855618127431,
0.0692940610217331));
#100351=CARTESIAN_POINT('Ctrl Pts',(0.00481150555539766,-0.0329757224171935,
0.0692479372393397));
#100352=CARTESIAN_POINT('Ctrl Pts',(0.00487970667965222,-0.0328657861694599,
0.0692032113348868));
#100353=CARTESIAN_POINT('Ctrl Pts',(0.00466494989529606,-0.0331951640388588,
0.0694540816118394));
#100354=CARTESIAN_POINT('Ctrl Pts',(0.00472962667885776,-0.0330855618127431,
0.0694064431885513));
#100355=CARTESIAN_POINT('Ctrl Pts',(0.00479533469190719,-0.0329757224171935,
0.0693601071821022));
#100356=CARTESIAN_POINT('Ctrl Pts',(0.00486199270192635,-0.0328657861694599,
0.0693151370559375));
#100357=CARTESIAN_POINT('Ctrl Pts',(0.00465187706210549,-0.0331951640388588,
0.0695666438305097));
#100358=CARTESIAN_POINT('Ctrl Pts',(0.00471500352863602,-0.0330855618127431,
0.0695188253553695));
#100359=CARTESIAN_POINT('Ctrl Pts',(0.00477916382841672,-0.0329757224171935,
0.0694722771248648));
#100360=CARTESIAN_POINT('Ctrl Pts',(0.00484427872420048,-0.0328657861694599,
0.0694270627769882));
#100361=CARTESIAN_POINT('Origin',(0.0141482943526272,-0.0326401908832812,
0.0833796410202241));
#100362=CARTESIAN_POINT('Ctrl Pts',(0.00462339419571742,-0.0332451089994432,
0.0695865135184027));
#100363=CARTESIAN_POINT('Ctrl Pts',(0.0047955089043147,-0.0329451141710257,
0.0694544942251325));
#100364=CARTESIAN_POINT('Ctrl Pts',(0.00497707888605812,-0.0326442513127503,
0.0693358143682031));
#100365=CARTESIAN_POINT('Ctrl Pts',(0.00442838239585338,-0.0332451089994432,
0.0697429436878515));
#100366=CARTESIAN_POINT('Ctrl Pts',(0.00459459724408313,-0.0329451141710257,
0.0696035694042155));
#100367=CARTESIAN_POINT('Ctrl Pts',(0.00477083813428145,-0.0326442513127503,
0.06947711105007));
#100368=CARTESIAN_POINT('Ctrl Pts',(0.00484425270444921,-0.0325229783203385,
0.0694270807353576));
#100369=CARTESIAN_POINT('Ctrl Pts',(0.00490935804204383,-0.032413025311208,
0.0693818724938979));
#100370=CARTESIAN_POINT('Ctrl Pts',(0.00497538869567019,-0.0323031222247695,
0.069338017896671));
#100371=CARTESIAN_POINT('Ctrl Pts',(0.00504225810254109,-0.0321934096636185,
0.0692955701337264));
#100372=CARTESIAN_POINT('Ctrl Pts',(0.00473319145634849,-0.0325229783203385,
0.0694045742514098));
#100373=CARTESIAN_POINT('Ctrl Pts',(0.00479860704532649,-0.032413025311208,
0.0693578350331017));
#100374=CARTESIAN_POINT('Ctrl Pts',(0.00486497957350275,-0.0323031222247695,
0.0693124561091772));
#100375=CARTESIAN_POINT('Ctrl Pts',(0.00493222197127388,-0.0321934096636185,
0.0692684926067874));
#100376=CARTESIAN_POINT('Ctrl Pts',(0.00462213020824776,-0.0325229783203385,
0.069382067767462));
#100377=CARTESIAN_POINT('Ctrl Pts',(0.00468785604860915,-0.032413025311208,
0.0693337975723054));
#100378=CARTESIAN_POINT('Ctrl Pts',(0.00475457045133531,-0.0323031222247695,
0.0692868943216834));
#100379=CARTESIAN_POINT('Ctrl Pts',(0.00482218584000668,-0.0321934096636185,
0.0692414150798485));
#100380=CARTESIAN_POINT('Ctrl Pts',(0.00451106896014703,-0.0325229783203385,
0.0693595612835142));
#100381=CARTESIAN_POINT('Ctrl Pts',(0.00457710505189181,-0.032413025311208,
0.0693097601115091));
#100382=CARTESIAN_POINT('Ctrl Pts',(0.00464416132916788,-0.0323031222247695,
0.0692613325341897));
#100383=CARTESIAN_POINT('Ctrl Pts',(0.00471214970873947,-0.0321934096636185,
0.0692143375529095));
#100384=CARTESIAN_POINT('Origin',(0.0145556181039783,-0.0326393375177737,
0.0831246813840125));
#100385=CARTESIAN_POINT('Ctrl Pts',(0.00500686402026082,-0.0326943950436593,
0.069023127551441));
#100386=CARTESIAN_POINT('Ctrl Pts',(0.0050775219313848,-0.0325844576448127,
0.0689801705772921));
#100387=CARTESIAN_POINT('Ctrl Pts',(0.00514907326373325,-0.0324744968375319,
0.0689386718844586));
#100388=CARTESIAN_POINT('Ctrl Pts',(0.0052214256081848,-0.0323646534831894,
0.0688986833790018));
#100389=CARTESIAN_POINT('Ctrl Pts',(0.00498674916228668,-0.0326943950436593,
0.0691346466980942));
#100390=CARTESIAN_POINT('Ctrl Pts',(0.00505587013056062,-0.0325844576448127,
0.0690914125035031));
#100391=CARTESIAN_POINT('Ctrl Pts',(0.00512589014466045,-0.0324744968375319,
0.0690496047841102));
#100392=CARTESIAN_POINT('Ctrl Pts',(0.00519671875201782,-0.0323646534831894,
0.0690092758689816));
#100393=CARTESIAN_POINT('Ctrl Pts',(0.00496663430431253,-0.0326943950436593,
0.0692461658447474));
#100394=CARTESIAN_POINT('Ctrl Pts',(0.00503421832973644,-0.0325844576448127,
0.0692026544297142));
#100395=CARTESIAN_POINT('Ctrl Pts',(0.00510270702558766,-0.0324744968375319,
0.0691605376837617));
#100396=CARTESIAN_POINT('Ctrl Pts',(0.00517201189585083,-0.0323646534831894,
0.0691198683589613));
#100397=CARTESIAN_POINT('Ctrl Pts',(0.00494651944633839,-0.0326943950436593,
0.0693576849914006));
#100398=CARTESIAN_POINT('Ctrl Pts',(0.00501256652891226,-0.0325844576448127,
0.0693138963559252));
#100399=CARTESIAN_POINT('Ctrl Pts',(0.00507952390651487,-0.0324744968375319,
0.0692714705834133));
#100400=CARTESIAN_POINT('Ctrl Pts',(0.00514730503968384,-0.0323646534831894,
0.0692304608489411));
#100401=CARTESIAN_POINT('Origin',(0.0141693602333143,-0.0326395579067716,
0.083411076513016));
#100402=CARTESIAN_POINT('Ctrl Pts',(0.00491681253919695,-0.0327445246961876,
0.069375749206536));
#100403=CARTESIAN_POINT('Ctrl Pts',(0.00509687634964127,-0.0324436878365474,
0.0692547963699877));
#100404=CARTESIAN_POINT('Ctrl Pts',(0.00528553927972262,-0.0321434074463186,
0.069147750289658));
#100405=CARTESIAN_POINT('Ctrl Pts',(0.00471236420018378,-0.0327445246961876,
0.0695196271988585));
#100406=CARTESIAN_POINT('Ctrl Pts',(0.00488700156349379,-0.0324436878365474,
0.0693909634672285));
#100407=CARTESIAN_POINT('Ctrl Pts',(0.00507083427853004,-0.0321434074463186,
0.0692758196554833));
#100408=CARTESIAN_POINT('Ctrl Pts',(0.00522774921403184,-0.0322357242816072,
0.0691809842036775));
#100409=CARTESIAN_POINT('Ctrl Pts',(0.00538600592256728,-0.0319819883628705,
0.0690887493093111));
#100410=CARTESIAN_POINT('Ctrl Pts',(0.00554981107443461,-0.0317295851069887,
0.0690067716674996));
#100411=CARTESIAN_POINT('Ctrl Pts',(0.005014543079264,-0.0322357242816072,
0.069311533597002));
#100412=CARTESIAN_POINT('Ctrl Pts',(0.00516864195893842,-0.0319819883628705,
0.0692125083637614));
#100413=CARTESIAN_POINT('Ctrl Pts',(0.00532872979698884,-0.0317295851069887,
0.0691234895699953));
#100414=CARTESIAN_POINT('Origin',(0.0141187006564011,-0.0326371942646127,
0.0833303547028761));
#100415=CARTESIAN_POINT('Origin',(0.0144865115407432,-0.0326352985529064,
0.0830232511827497));
#100416=CARTESIAN_POINT('Ctrl Pts',(0.0053349335308884,-0.0321934096636184,
0.0688375313516916));
#100417=CARTESIAN_POINT('Ctrl Pts',(0.00540819661383477,-0.0320835708272304,
0.0687990709551432));
#100418=CARTESIAN_POINT('Ctrl Pts',(0.0054822131371232,-0.0319739230346346,
0.0687621490428815));
#100419=CARTESIAN_POINT('Ctrl Pts',(0.00555688477628411,-0.0318646057455575,
0.0687268055860474));
#100420=CARTESIAN_POINT('Ctrl Pts',(0.00530785598063264,-0.0321934096636184,
0.0689475675777124));
#100421=CARTESIAN_POINT('Ctrl Pts',(0.00537960157826516,-0.0320835708272304,
0.0689087337606429));
#100422=CARTESIAN_POINT('Ctrl Pts',(0.00545210922436118,-0.0319739230346346,
0.0688714072401796));
#100423=CARTESIAN_POINT('Ctrl Pts',(0.00552528248522519,-0.0318646057455575,
0.0688356286532922));
#100424=CARTESIAN_POINT('Ctrl Pts',(0.00528077843037688,-0.0321934096636184,
0.0690576038037331));
#100425=CARTESIAN_POINT('Ctrl Pts',(0.00535100654269556,-0.0320835708272304,
0.0690183965661427));
#100426=CARTESIAN_POINT('Ctrl Pts',(0.00542200531159916,-0.0319739230346346,
0.0689806654374777));
#100427=CARTESIAN_POINT('Ctrl Pts',(0.00549368019416628,-0.0318646057455575,
0.068944451720537));
#100428=CARTESIAN_POINT('Ctrl Pts',(0.00525370088012111,-0.0321934096636184,
0.0691676400297538));
#100429=CARTESIAN_POINT('Ctrl Pts',(0.00532241150712595,-0.0320835708272304,
0.0691280593716424));
#100430=CARTESIAN_POINT('Ctrl Pts',(0.00539190139883713,-0.0319739230346346,
0.0690899236347759));
#100431=CARTESIAN_POINT('Ctrl Pts',(0.00546207790310737,-0.0318646057455575,
0.0690532747877818));
#100432=CARTESIAN_POINT('Ctrl Pts',(0.00514647479984622,-0.0320218834582372,
0.0692299960887807));
#100433=CARTESIAN_POINT('Ctrl Pts',(0.00519768014652859,-0.0319391099350671,
0.0691990095164114));
#100434=CARTESIAN_POINT('Ctrl Pts',(0.00524933832886476,-0.0318564869454956,
0.0691688412966873));
#100435=CARTESIAN_POINT('Ctrl Pts',(0.00530140966933807,-0.0317740741446553,
0.0691395098904944));
#100436=CARTESIAN_POINT('Ctrl Pts',(0.00509861064546314,-0.0320218834582372,
0.0692171177825111));
#100437=CARTESIAN_POINT('Ctrl Pts',(0.00514995002418067,-0.0319391099350671,
0.0691856330600055));
#100438=CARTESIAN_POINT('Ctrl Pts',(0.00520174993602962,-0.0318564869454956,
0.0691549690848907));
#100439=CARTESIAN_POINT('Ctrl Pts',(0.00525397056655174,-0.0317740741446553,
0.0691251446695073));
#100440=CARTESIAN_POINT('Ctrl Pts',(0.00505074649108006,-0.0320218834582372,
0.0692042394762415));
#100441=CARTESIAN_POINT('Ctrl Pts',(0.00510221990183275,-0.0319391099350671,
0.0691722566035997));
#100442=CARTESIAN_POINT('Ctrl Pts',(0.00515416154319448,-0.0318564869454956,
0.0691410968730942));
#100443=CARTESIAN_POINT('Ctrl Pts',(0.0052065314637654,-0.0317740741446553,
0.0691107794485202));
#100444=CARTESIAN_POINT('Ctrl Pts',(0.00500288233669698,-0.0320218834582372,
0.0691913611699719));
#100445=CARTESIAN_POINT('Ctrl Pts',(0.00505448977948483,-0.0319391099350671,
0.0691588801471938));
#100446=CARTESIAN_POINT('Ctrl Pts',(0.00510657315035933,-0.0318564869454956,
0.0691272246612976));
#100447=CARTESIAN_POINT('Ctrl Pts',(0.00515909236097907,-0.0317740741446553,
0.0690964142275331));
#100448=CARTESIAN_POINT('Origin',(0.00108385226297125,-0.0391228853390487,
0.0643357244328841));
#100449=CARTESIAN_POINT('Ctrl Pts',(0.00305548285383934,-0.0352722978779602,
0.0714303481196738));
#100450=CARTESIAN_POINT('Ctrl Pts',(0.00306472482300037,-0.0352466642097222,
0.0714138654413699));
#100451=CARTESIAN_POINT('Ctrl Pts',(0.00307389017394128,-0.0352210183808304,
0.0713973591033955));
#100452=CARTESIAN_POINT('Ctrl Pts',(0.00308297876453264,-0.0351953608940152,
0.0713808282647492));
#100453=CARTESIAN_POINT('Origin',(-0.00112696451673218,-0.035245600306509,
0.0688775306198176));
#100454=CARTESIAN_POINT('Ctrl Pts',(0.00314545449453057,-0.0350241211493339,
0.0712729297078573));
#100455=CARTESIAN_POINT('Ctrl Pts',(0.00318508495637312,-0.0349144232867421,
0.0712043552880952));
#100456=CARTESIAN_POINT('Ctrl Pts',(0.00322615662114941,-0.0348045283677512,
0.0711365590131672));
#100457=CARTESIAN_POINT('Ctrl Pts',(0.00326862011273923,-0.0346945769586887,
0.071069629679129));
#100458=CARTESIAN_POINT('Ctrl Pts',(0.00303538047663015,-0.0350241211493339,
0.0712998527906354));
#100459=CARTESIAN_POINT('Ctrl Pts',(0.00307464008406305,-0.0349144232867421,
0.0712297621464773));
#100460=CARTESIAN_POINT('Ctrl Pts',(0.00311537201389575,-0.0348045283677512,
0.0711604410737945));
#100461=CARTESIAN_POINT('Ctrl Pts',(0.00315752739784363,-0.0346945769586887,
0.0710919803055216));
#100462=CARTESIAN_POINT('Ctrl Pts',(0.00292530645872974,-0.0350241211493339,
0.0713267758734136));
#100463=CARTESIAN_POINT('Ctrl Pts',(0.00296419521175299,-0.0349144232867421,
0.0712551690048593));
#100464=CARTESIAN_POINT('Ctrl Pts',(0.00300458740664209,-0.0348045283677512,
0.0711843231344218));
#100465=CARTESIAN_POINT('Ctrl Pts',(0.00304643468294803,-0.0346945769586887,
0.0711143309319143));
#100466=CARTESIAN_POINT('Ctrl Pts',(0.00281523244082933,-0.0350241211493339,
0.0713536989561917));
#100467=CARTESIAN_POINT('Ctrl Pts',(0.00285375033944292,-0.0349144232867421,
0.0712805758632414));
#100468=CARTESIAN_POINT('Ctrl Pts',(0.00289380279938843,-0.0348045283677512,
0.0712082051950491));
#100469=CARTESIAN_POINT('Ctrl Pts',(0.00293534196805244,-0.0346945769586887,
0.071136681558307));
#100470=CARTESIAN_POINT('Origin',(0.0173476319408053,-0.0345629067939361,
0.0802153595577315));
#100471=CARTESIAN_POINT('Ctrl Pts',(0.00314376063159375,-0.0351970973651645,
0.0709289897510182));
#100472=CARTESIAN_POINT('Ctrl Pts',(0.00318838336335184,-0.03508693493218,
0.0708599983014073));
#100473=CARTESIAN_POINT('Ctrl Pts',(0.00323447735406611,-0.0349764985129749,
0.0707918773819471));
#100474=CARTESIAN_POINT('Ctrl Pts',(0.00328198808268525,-0.0348659306849666,
0.0707247187605296));
#100475=CARTESIAN_POINT('Ctrl Pts',(0.00316502677698795,-0.0351970973651645,
0.0710084140653692));
#100476=CARTESIAN_POINT('Ctrl Pts',(0.00320854919250971,-0.03508693493218,
0.070939717229382));
#100477=CARTESIAN_POINT('Ctrl Pts',(0.0032535358306445,-0.0349764985129748,
0.0708718682926352));
#100478=CARTESIAN_POINT('Ctrl Pts',(0.00329993358420676,-0.0348659306849666,
0.0708049585862098));
#100479=CARTESIAN_POINT('Ctrl Pts',(0.00318629292238215,-0.0351970973651645,
0.0710878383797203));
#100480=CARTESIAN_POINT('Ctrl Pts',(0.00322871502166757,-0.03508693493218,
0.0710194361573567));
#100481=CARTESIAN_POINT('Ctrl Pts',(0.0032725943072229,-0.0349764985129748,
0.0709518592033234));
#100482=CARTESIAN_POINT('Ctrl Pts',(0.00331787908572827,-0.0348659306849666,
0.0708851984118901));
#100483=CARTESIAN_POINT('Ctrl Pts',(0.00320755906777635,-0.0351970973651645,
0.0711672626940713));
#100484=CARTESIAN_POINT('Ctrl Pts',(0.00324888085082544,-0.03508693493218,
0.0710991550853315));
#100485=CARTESIAN_POINT('Ctrl Pts',(0.00329165278380129,-0.0349764985129748,
0.0710318501140115));
#100486=CARTESIAN_POINT('Ctrl Pts',(0.00333582458724978,-0.0348659306849666,
0.0709654382375704));
#100487=CARTESIAN_POINT('Origin',(0.0170465695611525,-0.0345637187966549,
0.0805904419479017));
#100488=CARTESIAN_POINT('Ctrl Pts',(0.00318927542078819,-0.0352450361861253,
0.0711955511657964));
#100489=CARTESIAN_POINT('Ctrl Pts',(0.00330070428416582,-0.0349452761023765,
0.071009443193777));
#100490=CARTESIAN_POINT('Ctrl Pts',(0.00342583500347301,-0.0346444289983475,
0.070832257212592));
#100491=CARTESIAN_POINT('Ctrl Pts',(0.00306554359310653,-0.0352450361861253,
0.0714127847608469));
#100492=CARTESIAN_POINT('Ctrl Pts',(0.00316877935721512,-0.0349452761023765,
0.0712220101664909));
#100493=CARTESIAN_POINT('Ctrl Pts',(0.0032860917620643,-0.0346444289983475,
0.0710395536826068));
#100494=CARTESIAN_POINT('Ctrl Pts',(0.00333593024175403,-0.0345231616327822,
0.0709660159461851));
#100495=CARTESIAN_POINT('Ctrl Pts',(0.0033798169792446,-0.0344132092796975,
0.0709000221477925));
#100496=CARTESIAN_POINT('Ctrl Pts',(0.00342506648204582,-0.0343032738558974,
0.070834939516924));
#100497=CARTESIAN_POINT('Ctrl Pts',(0.00347161864454688,-0.0341934961088741,
0.0707708499470323));
#100498=CARTESIAN_POINT('Ctrl Pts',(0.003224382943228,-0.0345231616327822,
0.0709859743110989));
#100499=CARTESIAN_POINT('Ctrl Pts',(0.00326799458275737,-0.0344132092796975,
0.0709184429902421));
#100500=CARTESIAN_POINT('Ctrl Pts',(0.00331300080423056,-0.0343032738558974,
0.0708518172260543));
#100501=CARTESIAN_POINT('Ctrl Pts',(0.00335934176306841,-0.0341934961088741,
0.0707861808969037));
#100502=CARTESIAN_POINT('Ctrl Pts',(0.00311283564470197,-0.0345231616327822,
0.0710059326760127));
#100503=CARTESIAN_POINT('Ctrl Pts',(0.00315617218627013,-0.0344132092796975,
0.0709368638326918));
#100504=CARTESIAN_POINT('Ctrl Pts',(0.0032009351264153,-0.0343032738558974,
0.0708686949351846));
#100505=CARTESIAN_POINT('Ctrl Pts',(0.00324706488158994,-0.0341934961088741,
0.0708015118467751));
#100506=CARTESIAN_POINT('Ctrl Pts',(0.00300128834617593,-0.0345231616327822,
0.0710258910409265));
#100507=CARTESIAN_POINT('Ctrl Pts',(0.00304434978978289,-0.0344132092796975,
0.0709552846751415));
#100508=CARTESIAN_POINT('Ctrl Pts',(0.00308886944860003,-0.0343032738558974,
0.0708855726443149));
#100509=CARTESIAN_POINT('Ctrl Pts',(0.00313478800011147,-0.0341934961088741,
0.0708168427966465));
#100510=CARTESIAN_POINT('Origin',(0.0173578804990277,-0.0345625596230697,
0.0802217989179083));
#100511=CARTESIAN_POINT('Ctrl Pts',(0.00333841734075968,-0.0346945769586886,
0.0705305686593154));
#100512=CARTESIAN_POINT('Ctrl Pts',(0.00338829493406878,-0.0345846629176052,
0.0704646239128968));
#100513=CARTESIAN_POINT('Ctrl Pts',(0.0034395447568674,-0.0344746925050311,
0.0703996993510994));
#100514=CARTESIAN_POINT('Ctrl Pts',(0.00349210079841876,-0.0343648066253259,
0.0703358778915575));
#100515=CARTESIAN_POINT('Ctrl Pts',(0.00336076794955423,-0.0346945769586886,
0.0706416612867402));
#100516=CARTESIAN_POINT('Ctrl Pts',(0.00340911463030587,-0.0345846629176052,
0.0705760245430078));
#100517=CARTESIAN_POINT('Ctrl Pts',(0.00345882690969433,-0.0344746925050311,
0.0705113763778614));
#100518=CARTESIAN_POINT('Ctrl Pts',(0.00350984074852324,-0.0343648066253259,
0.0704477993629199));
#100519=CARTESIAN_POINT('Ctrl Pts',(0.00338311855834878,-0.0346945769586886,
0.0707527539141651));
#100520=CARTESIAN_POINT('Ctrl Pts',(0.00342993432654296,-0.0345846629176052,
0.070687425173119));
#100521=CARTESIAN_POINT('Ctrl Pts',(0.00347810906252126,-0.0344746925050311,
0.0706230534046234));
#100522=CARTESIAN_POINT('Ctrl Pts',(0.00352758069862772,-0.0343648066253259,
0.0705597208342823));
#100523=CARTESIAN_POINT('Ctrl Pts',(0.00340546916714334,-0.0346945769586886,
0.0708638465415899));
#100524=CARTESIAN_POINT('Ctrl Pts',(0.00345075402278005,-0.0345846629176052,
0.07079882580323));
#100525=CARTESIAN_POINT('Ctrl Pts',(0.00349739121534819,-0.0344746925050311,
0.0707347304313854));
#100526=CARTESIAN_POINT('Ctrl Pts',(0.0035453206487322,-0.0343648066253259,
0.0706716423056448));
#100527=CARTESIAN_POINT('Origin',(0.0170943990081613,-0.0345626446732366,
0.080624004942947));
#100528=CARTESIAN_POINT('Ctrl Pts',(0.00340506923980482,-0.0346945769586885,
0.0708618587219638));
#100529=CARTESIAN_POINT('Ctrl Pts',(0.00347394067537212,-0.034527515336289,
0.0707630233898889));
#100530=CARTESIAN_POINT('Ctrl Pts',(0.00354593820484234,-0.0343603235965158,
0.0706663284371914));
#100531=CARTESIAN_POINT('Ctrl Pts',(0.00362084464106438,-0.0341934961088739,
0.0705720566798239));
#100532=CARTESIAN_POINT('Ctrl Pts',(0.00335864662719066,-0.0346945769586885,
0.0709316653790199));
#100533=CARTESIAN_POINT('Ctrl Pts',(0.00342605593437689,-0.034527515336289,
0.0708318577067372));
#100534=CARTESIAN_POINT('Ctrl Pts',(0.00349662153648929,-0.0343603235965158,
0.0707341441797431));
#100535=CARTESIAN_POINT('Ctrl Pts',(0.00357013043660882,-0.0341934961088739,
0.0706388106894242));
#100536=CARTESIAN_POINT('Ctrl Pts',(0.0033122240145765,-0.0346945769586885,
0.071001472036076));
#100537=CARTESIAN_POINT('Ctrl Pts',(0.00337817119338165,-0.034527515336289,
0.0709006920235855));
#100538=CARTESIAN_POINT('Ctrl Pts',(0.00344730486813625,-0.0343603235965158,
0.0708019599222949));
#100539=CARTESIAN_POINT('Ctrl Pts',(0.00351941623215327,-0.0341934961088739,
0.0707055646990244));
#100540=CARTESIAN_POINT('Ctrl Pts',(0.00326580140196235,-0.0346945769586885,
0.0710712786931321));
#100541=CARTESIAN_POINT('Ctrl Pts',(0.00333028645238642,-0.034527515336289,
0.0709695263404338));
#100542=CARTESIAN_POINT('Ctrl Pts',(0.0033979881997832,-0.0343603235965158,
0.0708697756648466));
#100543=CARTESIAN_POINT('Ctrl Pts',(0.00346870202769771,-0.0341934961088739,
0.0707723187086247));
#100544=CARTESIAN_POINT('Ctrl Pts',(0.00354530200359632,-0.0340223579322366,
0.070671667768251));
#100545=CARTESIAN_POINT('Ctrl Pts',(0.00359327727694297,-0.0339125849573554,
0.0706085185852605));
#100546=CARTESIAN_POINT('Ctrl Pts',(0.00364252587996998,-0.0338030433565221,
0.070546406753149));
#100547=CARTESIAN_POINT('Ctrl Pts',(0.00369297779083012,-0.0336938721132328,
0.0704854061195093));
#100548=CARTESIAN_POINT('Ctrl Pts',(0.00343272143262576,-0.0340223579322366,
0.0706845826770892));
#100549=CARTESIAN_POINT('Ctrl Pts',(0.00348051857569604,-0.0339125849573554,
0.0706198807144027));
#100550=CARTESIAN_POINT('Ctrl Pts',(0.0035296213125483,-0.0338030433565221,
0.0705562135068326));
#100551=CARTESIAN_POINT('Ctrl Pts',(0.00357995963155151,-0.0336938721132328,
0.0704936569075705));
#100552=CARTESIAN_POINT('Ctrl Pts',(0.0033201408616552,-0.0340223579322366,
0.0706974975859275));
#100553=CARTESIAN_POINT('Ctrl Pts',(0.00336775987444911,-0.0339125849573554,
0.0706312428435448));
#100554=CARTESIAN_POINT('Ctrl Pts',(0.00341671674512663,-0.0338030433565221,
0.070566020260516));
#100555=CARTESIAN_POINT('Ctrl Pts',(0.0034669414722729,-0.0336938721132328,
0.0705019076956318));
#100556=CARTESIAN_POINT('Ctrl Pts',(0.00320756029068464,-0.0340223579322366,
0.0707104124947657));
#100557=CARTESIAN_POINT('Ctrl Pts',(0.00325500117320218,-0.0339125849573554,
0.0706426049726869));
#100558=CARTESIAN_POINT('Ctrl Pts',(0.00330381217770495,-0.0338030433565221,
0.0705758270141996));
#100559=CARTESIAN_POINT('Ctrl Pts',(0.0033539233129943,-0.0336938721132328,
0.0705101584836931));
#100560=CARTESIAN_POINT('Origin',(0.0172588781084155,-0.0345589643413925,
0.0801535977097717));
#100561=CARTESIAN_POINT('Ctrl Pts',(0.00357512613946545,-0.034193496108874,
0.0702372352350696));
#100562=CARTESIAN_POINT('Ctrl Pts',(0.00362908084852657,-0.0340836138581106,
0.0701745119616971));
#100563=CARTESIAN_POINT('Ctrl Pts',(0.00368430759563511,-0.0339738896643499,
0.0701129352636219));
#100564=CARTESIAN_POINT('Ctrl Pts',(0.00374073041431604,-0.0338644633294062,
0.0700525792131577));
#100565=CARTESIAN_POINT('Ctrl Pts',(0.00359045710313133,-0.034193496108874,
0.0703495122175726));
#100566=CARTESIAN_POINT('Ctrl Pts',(0.00364286357909152,-0.0340836138581106,
0.0702870003491104));
#100567=CARTESIAN_POINT('Ctrl Pts',(0.00369653846138944,-0.0339738896643499,
0.070225602917074));
#100568=CARTESIAN_POINT('Ctrl Pts',(0.00375140778512577,-0.0338644633294062,
0.0701653938974833));
#100569=CARTESIAN_POINT('Ctrl Pts',(0.0036057880667972,-0.034193496108874,
0.0704617892000756));
#100570=CARTESIAN_POINT('Ctrl Pts',(0.00365664630965646,-0.0340836138581106,
0.0703994887365236));
#100571=CARTESIAN_POINT('Ctrl Pts',(0.00370876932714378,-0.0339738896643499,
0.0703382705705262));
#100572=CARTESIAN_POINT('Ctrl Pts',(0.00376208515593551,-0.0338644633294062,
0.0702782085818089));
#100573=CARTESIAN_POINT('Ctrl Pts',(0.00362111903046307,-0.034193496108874,
0.0705740661825786));
#100574=CARTESIAN_POINT('Ctrl Pts',(0.00367042904022141,-0.0340836138581106,
0.0705119771239369));
#100575=CARTESIAN_POINT('Ctrl Pts',(0.00372100019289811,-0.0339738896643499,
0.0704509382239784));
#100576=CARTESIAN_POINT('Ctrl Pts',(0.00377276252674524,-0.0338644633294062,
0.0703910232661346));
#100577=CARTESIAN_POINT('Origin',(0.0170340332225967,-0.0345610621861625,
0.0805790325330161));
#100578=CARTESIAN_POINT('Ctrl Pts',(0.00359842765729212,-0.03424362768739,
0.0706004519548022));
#100579=CARTESIAN_POINT('Ctrl Pts',(0.00373230106874527,-0.0339430054201859,
0.0704297753948485));
#100580=CARTESIAN_POINT('Ctrl Pts',(0.00387865021769195,-0.0336441434784161,
0.0702696676029884));
#100581=CARTESIAN_POINT('Ctrl Pts',(0.00344844763316054,-0.03424362768739,
0.0708004669351448));
#100582=CARTESIAN_POINT('Ctrl Pts',(0.00357477735527091,-0.0339430054201859,
0.0706241337853311));
#100583=CARTESIAN_POINT('Ctrl Pts',(0.00371403032323082,-0.0336441434784161,
0.0704578172517991));
#100584=CARTESIAN_POINT('Ctrl Pts',(0.00377274449345952,-0.0335235895815127,
0.0703910443333679));
#100585=CARTESIAN_POINT('Ctrl Pts',(0.00382449391891267,-0.0334144449262719,
0.0703311437330281));
#100586=CARTESIAN_POINT('Ctrl Pts',(0.00387754029950884,-0.0333049234473133,
0.0702722434183398));
#100587=CARTESIAN_POINT('Ctrl Pts',(0.00393182262760982,-0.0331951640388588,
0.07021442484906));
#100588=CARTESIAN_POINT('Ctrl Pts',(0.00365957517040082,-0.0335235895815127,
0.0703968647117698));
#100589=CARTESIAN_POINT('Ctrl Pts',(0.003711244466886,-0.0334144449262719,
0.0703354061128883));
#100590=CARTESIAN_POINT('Ctrl Pts',(0.00376424281353307,-0.0333049234473133,
0.0702749443543024));
#100591=CARTESIAN_POINT('Ctrl Pts',(0.00381850944498583,-0.0331951640388588,
0.070215562886813));
#100592=CARTESIAN_POINT('Ctrl Pts',(0.00354640584734212,-0.0335235895815127,
0.0704026850901717));
#100593=CARTESIAN_POINT('Ctrl Pts',(0.00359799501485933,-0.0334144449262719,
0.0703396684927484));
#100594=CARTESIAN_POINT('Ctrl Pts',(0.0036509453275573,-0.0333049234473133,
0.070277645290265));
#100595=CARTESIAN_POINT('Ctrl Pts',(0.00370519626236183,-0.0331951640388588,
0.0702167009245659));
#100596=CARTESIAN_POINT('Ctrl Pts',(0.00343323652428342,-0.0335235895815127,
0.0704085054685736));
#100597=CARTESIAN_POINT('Ctrl Pts',(0.00348474556283266,-0.0334144449262719,
0.0703439308726085));
#100598=CARTESIAN_POINT('Ctrl Pts',(0.00353764784158153,-0.0333049234473133,
0.0702803462262276));
#100599=CARTESIAN_POINT('Ctrl Pts',(0.00359188307973784,-0.0331951640388588,
0.0702178389623189));
#100600=CARTESIAN_POINT('Origin',(0.0155492903479003,-0.0326434571768441,
0.0821653781509418));
#100601=CARTESIAN_POINT('Ctrl Pts',(0.00382963877748485,-0.0336938721132367,
0.0699573215171435));
#100602=CARTESIAN_POINT('Ctrl Pts',(0.00385417991592264,-0.0336474569764946,
0.0699321864707846));
#100603=CARTESIAN_POINT('Ctrl Pts',(0.00387901361023897,-0.033601104548885,
0.0699073404317061));
#100604=CARTESIAN_POINT('Ctrl Pts',(0.00394188680916358,-0.0334837508694597,
0.0698444359786847));
#100605=CARTESIAN_POINT('Ctrl Pts',(0.00400659638802133,-0.0333660264863578,
0.0697834222117383));
#100606=CARTESIAN_POINT('Ctrl Pts',(0.00385439107964342,-0.0336938721132367,
0.0702963751453641));
#100607=CARTESIAN_POINT('Ctrl Pts',(0.00387694762468536,-0.0336474569764946,
0.0702713849824435));
#100608=CARTESIAN_POINT('Ctrl Pts',(0.00389979516554788,-0.033601104548885,
0.0702466605847043));
#100609=CARTESIAN_POINT('Ctrl Pts',(0.00395763988100942,-0.0334837508694597,
0.0701840640995601));
#100610=CARTESIAN_POINT('Ctrl Pts',(0.00401731405881714,-0.0333660264863578,
0.0701232091608762));
#100611=CARTESIAN_POINT('Ctrl Pts',(0.00385439107965538,-0.0336938721132426,
0.070296375145372));
#100612=CARTESIAN_POINT('Ctrl Pts',(0.00387694762469635,-0.0336474569765026,
0.0702713849824524));
#100613=CARTESIAN_POINT('Ctrl Pts',(0.00389979516555788,-0.0336011045488949,
0.0702466605847143));
#100614=CARTESIAN_POINT('Ctrl Pts',(0.00395715811332046,-0.033484728265791,
0.0701845854430388));
#100615=CARTESIAN_POINT('Ctrl Pts',(0.00401632039107351,-0.0333679870047996,
0.0701242227403068));
#100616=CARTESIAN_POINT('Ctrl Pts',(0.00385439107964064,-0.0336938721132424,
0.0702963751453673));
#100617=CARTESIAN_POINT('Ctrl Pts',(0.00393506326697639,-0.0335278710435081,
0.0702069992635138));
#100618=CARTESIAN_POINT('Ctrl Pts',(0.00401850987844153,-0.0333620469224319,
0.0701201846827083));
#100619=CARTESIAN_POINT('Ctrl Pts',(0.00410478685445126,-0.0331951640388601,
0.0700359021076483));
#100620=CARTESIAN_POINT('Ctrl Pts',(0.0037995854233222,-0.0336938721132424,
0.0703598130666666));
#100621=CARTESIAN_POINT('Ctrl Pts',(0.00387892959455252,-0.0335278710435081,
0.0702692898774492));
#100622=CARTESIAN_POINT('Ctrl Pts',(0.00396108463636584,-0.0333620469224319,
0.07018128674666));
#100623=CARTESIAN_POINT('Ctrl Pts',(0.00404610604454009,-0.0331951640388601,
0.0700957735730675));
#100624=CARTESIAN_POINT('Ctrl Pts',(0.00374477976700376,-0.0336938721132424,
0.0704232509879659));
#100625=CARTESIAN_POINT('Ctrl Pts',(0.00382279592212864,-0.0335278710435081,
0.0703315804913845));
#100626=CARTESIAN_POINT('Ctrl Pts',(0.00390365939429015,-0.0333620469224319,
0.0702423888106118));
#100627=CARTESIAN_POINT('Ctrl Pts',(0.00398742523462892,-0.0331951640388601,
0.0701556450384867));
#100628=CARTESIAN_POINT('Ctrl Pts',(0.00368997411068532,-0.0336938721132424,
0.0704866889092652));
#100629=CARTESIAN_POINT('Ctrl Pts',(0.00376666224970477,-0.0335278710435081,
0.0703938711053199));
#100630=CARTESIAN_POINT('Ctrl Pts',(0.00384623415221446,-0.0333620469224319,
0.0703034908745635));
#100631=CARTESIAN_POINT('Ctrl Pts',(0.00392874442471776,-0.0331951640388601,
0.0702155165039059));
#100632=CARTESIAN_POINT('Ctrl Pts',(0.00401735592383927,-0.0330240426238156,
0.0701252585083006));
#100633=CARTESIAN_POINT('Ctrl Pts',(0.00407280065900278,-0.0329142774063509,
0.0700686884857445));
#100634=CARTESIAN_POINT('Ctrl Pts',(0.00412944249577568,-0.0328043479726686,
0.0700132364585221));
#100635=CARTESIAN_POINT('Ctrl Pts',(0.00418721082812532,-0.0326943950436594,
0.069958975463166));
#100636=CARTESIAN_POINT('Ctrl Pts',(0.00390404461084407,-0.0330240426238156,
0.0701239614609192));
#100637=CARTESIAN_POINT('Ctrl Pts',(0.00395950721409892,-0.0329142774063509,
0.0700658304646327));
#100638=CARTESIAN_POINT('Ctrl Pts',(0.00401619919755841,-0.0328043479726686,
0.0700088170548609));
#100639=CARTESIAN_POINT('Ctrl Pts',(0.00407404994603473,-0.0326943950436594,
0.069952996270153));
#100640=CARTESIAN_POINT('Ctrl Pts',(0.00379073329784888,-0.0330240426238156,
0.0701226644135377));
#100641=CARTESIAN_POINT('Ctrl Pts',(0.00384621376919505,-0.0329142774063509,
0.0700629724435208));
#100642=CARTESIAN_POINT('Ctrl Pts',(0.00390295589934115,-0.0328043479726686,
0.0700043976511997));
#100643=CARTESIAN_POINT('Ctrl Pts',(0.00396088906394415,-0.0326943950436594,
0.0699470170771401));
#100644=CARTESIAN_POINT('Ctrl Pts',(0.00367742198485368,-0.0330240426238156,
0.0701213673661562));
#100645=CARTESIAN_POINT('Ctrl Pts',(0.00373292032429119,-0.0329142774063509,
0.070060114422409));
#100646=CARTESIAN_POINT('Ctrl Pts',(0.00378971260112388,-0.0328043479726686,
0.0699999782475385));
#100647=CARTESIAN_POINT('Ctrl Pts',(0.00384772818185357,-0.0326943950436594,
0.0699410378841271));
#100648=CARTESIAN_POINT('Origin',(0.0156353456212262,-0.0326396682857831,
0.08225420319739));
#100649=CARTESIAN_POINT('Ctrl Pts',(0.00410139311123134,-0.0331951640388587,
0.0696979907823525));
#100650=CARTESIAN_POINT('Ctrl Pts',(0.00416271053186312,-0.0330855618255041,
0.0696425905099765));
#100651=CARTESIAN_POINT('Ctrl Pts',(0.00422521718429758,-0.0329757224427708,
0.0695884176265899));
#100652=CARTESIAN_POINT('Ctrl Pts',(0.00428883642783697,-0.0328657862078596,
0.0695355454301241));
#100653=CARTESIAN_POINT('Ctrl Pts',(0.00410253114807826,-0.0331951640388587,
0.0698113038747634));
#100654=CARTESIAN_POINT('Ctrl Pts',(0.0041622879100926,-0.0330855618255041,
0.0697559192765427));
#100655=CARTESIAN_POINT('Ctrl Pts',(0.00422323245489464,-0.0329757224427708,
0.0697017298224648));
#100656=CARTESIAN_POINT('Ctrl Pts',(0.00428529014320011,-0.0328657862078596,
0.0696488087335584));
#100657=CARTESIAN_POINT('Ctrl Pts',(0.00410366918492518,-0.0331951640388587,
0.0699246169671742));
#100658=CARTESIAN_POINT('Ctrl Pts',(0.00416186528832207,-0.0330855618255041,
0.0698692480431089));
#100659=CARTESIAN_POINT('Ctrl Pts',(0.0042212477254917,-0.0329757224427708,
0.0698150420183397));
#100660=CARTESIAN_POINT('Ctrl Pts',(0.00428174385856326,-0.0328657862078596,
0.0697620720369927));
#100661=CARTESIAN_POINT('Ctrl Pts',(0.00410480722177209,-0.0331951640388587,
0.0700379300595851));
#100662=CARTESIAN_POINT('Ctrl Pts',(0.00416144266655155,-0.0330855618255041,
0.0699825768096751));
#100663=CARTESIAN_POINT('Ctrl Pts',(0.00421926299608876,-0.0329757224427708,
0.0699283542142146));
#100664=CARTESIAN_POINT('Ctrl Pts',(0.0042781975739264,-0.0328657862078596,
0.0698753353404269));
#100665=CARTESIAN_POINT('Origin',(0.0152575700259859,-0.0326401908832753,
0.0825517909517735));
#100666=CARTESIAN_POINT('Ctrl Pts',(0.0040790392835265,-0.0332451089994432,
0.0700612129188001));
#100667=CARTESIAN_POINT('Ctrl Pts',(0.00423325041131986,-0.0329451141710257,
0.0699086629441171));
#100668=CARTESIAN_POINT('Ctrl Pts',(0.00439851412929696,-0.0326442513127503,
0.0697681621603776));
#100669=CARTESIAN_POINT('Ctrl Pts',(0.00390517110891562,-0.0332451089994432,
0.0702408510490995));
#100670=CARTESIAN_POINT('Ctrl Pts',(0.00405260707377728,-0.0329451141710257,
0.070081743528924));
#100671=CARTESIAN_POINT('Ctrl Pts',(0.00421160881747946,-0.0326442513127503,
0.0699341934960175));
#100672=CARTESIAN_POINT('Ctrl Pts',(0.00427817403071446,-0.0325229783203385,
0.0698753563998101));
#100673=CARTESIAN_POINT('Ctrl Pts',(0.00433709989819023,-0.0324130253112079,
0.0698223447763543));
#100674=CARTESIAN_POINT('Ctrl Pts',(0.00439711344191326,-0.0323031222247695,
0.0697705601503919));
#100675=CARTESIAN_POINT('Ctrl Pts',(0.00445813544815066,-0.0321934096636184,
0.069720066141747));
#100676=CARTESIAN_POINT('Ctrl Pts',(0.00416516772331802,-0.0325229783203385,
0.0698669470515587));
#100677=CARTESIAN_POINT('Ctrl Pts',(0.00422420951347343,-0.0324130253112079,
0.0698123776386551));
#100678=CARTESIAN_POINT('Ctrl Pts',(0.00428437118716941,-0.0323031222247695,
0.0697590378575237));
#100679=CARTESIAN_POINT('Ctrl Pts',(0.00434557327063648,-0.0321934096636184,
0.0697069933133363));
#100680=CARTESIAN_POINT('Ctrl Pts',(0.00405216141592158,-0.0325229783203385,
0.0698585377033074));
#100681=CARTESIAN_POINT('Ctrl Pts',(0.00411131912875662,-0.0324130253112079,
0.0698024105009559));
#100682=CARTESIAN_POINT('Ctrl Pts',(0.00417162893242555,-0.0323031222247695,
0.0697475155646555));
#100683=CARTESIAN_POINT('Ctrl Pts',(0.00423301109312229,-0.0321934096636184,
0.0696939204849255));
#100684=CARTESIAN_POINT('Ctrl Pts',(0.00393915510852514,-0.0325229783203385,
0.069850128355056));
#100685=CARTESIAN_POINT('Ctrl Pts',(0.00399842874403982,-0.0324130253112079,
0.0697924433632568));
#100686=CARTESIAN_POINT('Ctrl Pts',(0.0040588866776817,-0.0323031222247695,
0.0697359932717873));
#100687=CARTESIAN_POINT('Ctrl Pts',(0.00412044891560811,-0.0321934096636184,
0.0696808476565148));
#100688=CARTESIAN_POINT('Origin',(0.0156297269948085,-0.0326393375177989,
0.0822477905481969));
#100689=CARTESIAN_POINT('Ctrl Pts',(0.0043888743489824,-0.0326943950436593,
0.0694542079053788));
#100690=CARTESIAN_POINT('Ctrl Pts',(0.00445359116489844,-0.0325844576448127,
0.0694027338753235));
#100691=CARTESIAN_POINT('Ctrl Pts',(0.00451937712825846,-0.0324744968375319,
0.069352594652229));
#100692=CARTESIAN_POINT('Ctrl Pts',(0.00458614706416913,-0.0323646534831894,
0.0693038533147957));
#100693=CARTESIAN_POINT('Ctrl Pts',(0.00438289515792577,-0.0326943950436593,
0.0695673687504441));
#100694=CARTESIAN_POINT('Ctrl Pts',(0.00444605240531079,-0.0325844576448127,
0.0695158123159298));
#100695=CARTESIAN_POINT('Ctrl Pts',(0.00451028039402602,-0.0324744968375319,
0.0694655584281103));
#100696=CARTESIAN_POINT('Ctrl Pts',(0.00457549594331969,-0.0323646534831894,
0.0694166703401343));
#100697=CARTESIAN_POINT('Ctrl Pts',(0.00437691596686915,-0.0326943950436594,
0.0696805295955094));
#100698=CARTESIAN_POINT('Ctrl Pts',(0.00443851364572314,-0.0325844576448127,
0.0696288907565362));
#100699=CARTESIAN_POINT('Ctrl Pts',(0.00450118365979357,-0.0324744968375319,
0.0695785222039916));
#100700=CARTESIAN_POINT('Ctrl Pts',(0.00456484482247025,-0.0323646534831894,
0.0695294873654728));
#100701=CARTESIAN_POINT('Ctrl Pts',(0.00437093677581252,-0.0326943950436594,
0.0697936904405747));
#100702=CARTESIAN_POINT('Ctrl Pts',(0.0044309748861355,-0.0325844576448127,
0.0697419691971425));
#100703=CARTESIAN_POINT('Ctrl Pts',(0.00449208692556113,-0.0324744968375319,
0.0696914859798729));
#100704=CARTESIAN_POINT('Ctrl Pts',(0.00455419370162081,-0.0323646534831894,
0.0696423043908113));
#100705=CARTESIAN_POINT('Origin',(0.0152824097106913,-0.0326395579068753,
0.0825803383141517));
#100706=CARTESIAN_POINT('Ctrl Pts',(0.00434372816300158,-0.0327445246961877,
0.0698153354767094));
#100707=CARTESIAN_POINT('Ctrl Pts',(0.00450721270640475,-0.0324436878365475,
0.0696727684097933));
#100708=CARTESIAN_POINT('Ctrl Pts',(0.00468097154154346,-0.0321434074463186,
0.0695429206846993));
#100709=CARTESIAN_POINT('Ctrl Pts',(0.00415892465422382,-0.0327445246961877,
0.0699837031195135));
#100710=CARTESIAN_POINT('Ctrl Pts',(0.00431605910823487,-0.0324436878365475,
0.0698341660743927));
#100711=CARTESIAN_POINT('Ctrl Pts',(0.00448401090115397,-0.0321434074463186,
0.0696968898573845));
#100712=CARTESIAN_POINT('Ctrl Pts',(0.00462780248168976,-0.0322357242816072,
0.0695831355551812));
#100713=CARTESIAN_POINT('Ctrl Pts',(0.00477325119125102,-0.0319819883628705,
0.069471793135492));
#100714=CARTESIAN_POINT('Ctrl Pts',(0.00492549016764143,-0.0317295851069887,
0.0693699316825138));
#100715=CARTESIAN_POINT('Ctrl Pts',(0.00443263971858135,-0.0322357242816072,
0.0697393773418322));
#100716=CARTESIAN_POINT('Ctrl Pts',(0.00457311232987594,-0.0319819883628705,
0.069621819241255));
#100717=CARTESIAN_POINT('Ctrl Pts',(0.0047207808142367,-0.0317295851069887,
0.069513438060869));
#100718=CARTESIAN_POINT('Origin',(0.0152220324737634,-0.0326371942646248,
0.08250660234782));
#100719=CARTESIAN_POINT('Origin',(0.0155484527814898,-0.0326352985525135,
0.0821558215032046));
#100720=CARTESIAN_POINT('Ctrl Pts',(0.00469109556167726,-0.0321934096636183,
0.0692289571744985));
#100721=CARTESIAN_POINT('Ctrl Pts',(0.00475896057746837,-0.0320835708272304,
0.0691816177505778));
#100722=CARTESIAN_POINT('Ctrl Pts',(0.00482776591570985,-0.0319739230346346,
0.0691357102484214));
#100723=CARTESIAN_POINT('Ctrl Pts',(0.00489741903696226,-0.0318646057455575,
0.0690912866473095));
#100724=CARTESIAN_POINT('Ctrl Pts',(0.00467802272200933,-0.0321934096636183,
0.0693415194489414));
#100725=CARTESIAN_POINT('Ctrl Pts',(0.00474433541631017,-0.0320835708272304,
0.0692939997403734));
#100726=CARTESIAN_POINT('Ctrl Pts',(0.00481159306445234,-0.0319739230346346,
0.0692478799329295));
#100727=CARTESIAN_POINT('Ctrl Pts',(0.00487970508631167,-0.0318646057455575,
0.0692032124294917));
#100728=CARTESIAN_POINT('Ctrl Pts',(0.00466494988234139,-0.0321934096636183,
0.0694540817233843));
#100729=CARTESIAN_POINT('Ctrl Pts',(0.00472971025515197,-0.0320835708272304,
0.069406381730169));
#100730=CARTESIAN_POINT('Ctrl Pts',(0.00479542021319483,-0.0319739230346346,
0.0693600496174375));
#100731=CARTESIAN_POINT('Ctrl Pts',(0.00486199113566107,-0.0318646057455575,
0.0693151382116739));
#100732=CARTESIAN_POINT('Ctrl Pts',(0.00465187704267346,-0.0321934096636183,
0.0695666439978272));
#100733=CARTESIAN_POINT('Ctrl Pts',(0.00471508509399377,-0.0320835708272304,
0.0695187637199645));
#100734=CARTESIAN_POINT('Ctrl Pts',(0.00477924736193731,-0.0319739230346346,
0.0694722193019455));
#100735=CARTESIAN_POINT('Ctrl Pts',(0.00484427718501048,-0.0318646057455575,
0.069427063993856));
#100736=CARTESIAN_POINT('Ctrl Pts',(0.00455331175857821,-0.0320218834582377,
0.0696419473520672));
#100737=CARTESIAN_POINT('Ctrl Pts',(0.00460022968849572,-0.0319391099350675,
0.0696047873864008));
#100738=CARTESIAN_POINT('Ctrl Pts',(0.00464769945010586,-0.0318564869454957,
0.0695683825650677));
#100739=CARTESIAN_POINT('Ctrl Pts',(0.00469568399252358,-0.0317740741446551,
0.0695327561762958));
#100740=CARTESIAN_POINT('Ctrl Pts',(0.0045042109475812,-0.0320218834582377,
0.0696351695643298));
#100741=CARTESIAN_POINT('Ctrl Pts',(0.00455119941788386,-0.0319391099350675,
0.0695974985779213));
#100742=CARTESIAN_POINT('Ctrl Pts',(0.00459874765680106,-0.0318564869454957,
0.0695605841469588));
#100743=CARTESIAN_POINT('Ctrl Pts',(0.00464681852163494,-0.0317740741446551,
0.0695244499255165));
#100744=CARTESIAN_POINT('Ctrl Pts',(0.00445511013658419,-0.0320218834582377,
0.0696283917765924));
#100745=CARTESIAN_POINT('Ctrl Pts',(0.004502169147272,-0.0319391099350675,
0.0695902097694419));
#100746=CARTESIAN_POINT('Ctrl Pts',(0.00454979586349626,-0.0318564869454957,
0.0695527857288498));
#100747=CARTESIAN_POINT('Ctrl Pts',(0.00459795305074629,-0.0317740741446551,
0.0695161436747372));
#100748=CARTESIAN_POINT('Ctrl Pts',(0.00440600932558717,-0.0320218834582377,
0.069621613988855));
#100749=CARTESIAN_POINT('Ctrl Pts',(0.00445313887666013,-0.0319391099350675,
0.0695829209609625));
#100750=CARTESIAN_POINT('Ctrl Pts',(0.00450084407019146,-0.0318564869454957,
0.0695449873107408));
#100751=CARTESIAN_POINT('Ctrl Pts',(0.00454908757985765,-0.0317740741446551,
0.0695078374239579));
#100752=CARTESIAN_POINT('Origin',(-9.06906787348535E-5,-0.0391228853390656,
0.0652954501092941));
#100753=CARTESIAN_POINT('Ctrl Pts',(0.00275458514362636,-0.0352722978779612,
0.0720870197319338));
#100754=CARTESIAN_POINT('Ctrl Pts',(0.00276168840973056,-0.0352466642097229,
0.0720695086985918));
#100755=CARTESIAN_POINT('Ctrl Pts',(0.00276871269642917,-0.0352210183808307,
0.0720519837949522));
#100756=CARTESIAN_POINT('Ctrl Pts',(0.00277565775730809,-0.0351953608940152,
0.0720344442044586));
#100757=CARTESIAN_POINT('Origin',(-0.00171483525212223,-0.03524560030651,
0.0700785316137319));
#100758=CARTESIAN_POINT('Ctrl Pts',(0.00282411757248214,-0.035024121149334,
0.0719195661746556));
#100759=CARTESIAN_POINT('Ctrl Pts',(0.00285484088252747,-0.0349144232867422,
0.0718465654707452));
#100760=CARTESIAN_POINT('Ctrl Pts',(0.00288709155859916,-0.0348045283677512,
0.0717741561451404));
#100761=CARTESIAN_POINT('Ctrl Pts',(0.00292083174301926,-0.0346945769586886,
0.0717024324821825));
#100762=CARTESIAN_POINT('Ctrl Pts',(0.00271828587811248,-0.035024121149334,
0.0719600728934794));
#100763=CARTESIAN_POINT('Ctrl Pts',(0.00274845122473957,-0.0349144232867422,
0.0718856144014375));
#100764=CARTESIAN_POINT('Ctrl Pts',(0.00278017373694604,-0.0348045283677512,
0.0718117348816427));
#100765=CARTESIAN_POINT('Ctrl Pts',(0.00281341630364038,-0.0346945769586886,
0.0717385304763935));
#100766=CARTESIAN_POINT('Ctrl Pts',(0.00261245418374283,-0.035024121149334,
0.0720005796123032));
#100767=CARTESIAN_POINT('Ctrl Pts',(0.00264206156695168,-0.0349144232867422,
0.0719246633321297));
#100768=CARTESIAN_POINT('Ctrl Pts',(0.00267325591529292,-0.0348045283677512,
0.0718493136181449));
#100769=CARTESIAN_POINT('Ctrl Pts',(0.00270600086426149,-0.0346945769586886,
0.0717746284706046));
#100770=CARTESIAN_POINT('Ctrl Pts',(0.00250662248937317,-0.035024121149334,
0.072041086331127));
#100771=CARTESIAN_POINT('Ctrl Pts',(0.00253567190916378,-0.0349144232867422,
0.071963712262822));
#100772=CARTESIAN_POINT('Ctrl Pts',(0.00256633809363979,-0.0348045283677512,
0.0718868923546472));
#100773=CARTESIAN_POINT('Ctrl Pts',(0.0025985854248826,-0.0346945769586886,
0.0718107264648157));
#100774=CARTESIAN_POINT('Origin',(0.0180350902565986,-0.0345629067939025,
0.0790114774712389));
#100775=CARTESIAN_POINT('Ctrl Pts',(0.00277932995921813,-0.0351970973651641,
0.071578550584425));
#100776=CARTESIAN_POINT('Ctrl Pts',(0.00281495390594009,-0.0350869349321797,
0.0715045104417393));
#100777=CARTESIAN_POINT('Ctrl Pts',(0.00285214661666063,-0.0349764985129746,
0.0714311495671717));
#100778=CARTESIAN_POINT('Ctrl Pts',(0.00289086550180983,-0.0348659306849665,
0.0713585658382966));
#100779=CARTESIAN_POINT('Ctrl Pts',(0.00281038292084524,-0.0351970973651641,
0.0716546832595667));
#100780=CARTESIAN_POINT('Ctrl Pts',(0.00284495215253115,-0.0350869349321797,
0.0715810733135801));
#100781=CARTESIAN_POINT('Ctrl Pts',(0.002881080330951,-0.0349764985129746,
0.0715081210651405));
#100782=CARTESIAN_POINT('Ctrl Pts',(0.00291872621450492,-0.0348659306849665,
0.0714359237812513));
#100783=CARTESIAN_POINT('Ctrl Pts',(0.00284143588247235,-0.0351970973651641,
0.0717308159347085));
#100784=CARTESIAN_POINT('Ctrl Pts',(0.00287495039912221,-0.0350869349321797,
0.071657636185421));
#100785=CARTESIAN_POINT('Ctrl Pts',(0.00291001404524137,-0.0349764985129746,
0.0715850925631094));
#100786=CARTESIAN_POINT('Ctrl Pts',(0.00294658692720001,-0.0348659306849664,
0.0715132817242059));
#100787=CARTESIAN_POINT('Ctrl Pts',(0.00287248884409946,-0.0351970973651641,
0.0718069486098502));
#100788=CARTESIAN_POINT('Ctrl Pts',(0.00290494864571327,-0.0350869349321797,
0.0717341990572619));
#100789=CARTESIAN_POINT('Ctrl Pts',(0.00293894775953174,-0.0349764985129746,
0.0716620640610782));
#100790=CARTESIAN_POINT('Ctrl Pts',(0.0029744476398951,-0.0348659306849664,
0.0715906396671606));
#100791=CARTESIAN_POINT('Origin',(0.0177834121327603,-0.0345637187967461,
0.0794213353461847));
#100792=CARTESIAN_POINT('Ctrl Pts',(0.00285789485476266,-0.0352450361861253,
0.0718373055671251));
#100793=CARTESIAN_POINT('Ctrl Pts',(0.00294511955434506,-0.0349452761023765,
0.0716386993722933));
#100794=CARTESIAN_POINT('Ctrl Pts',(0.00304705628859159,-0.0346444289983475,
0.0714472275178238));
#100795=CARTESIAN_POINT('Ctrl Pts',(0.00276236527840564,-0.0352450361861253,
0.0720683339204522));
#100796=CARTESIAN_POINT('Ctrl Pts',(0.00284087660088663,-0.0349452761023765,
0.0718661247686191));
#100797=CARTESIAN_POINT('Ctrl Pts',(0.00293439610127408,-0.0346444289983475,
0.0716704038655705));
#100798=CARTESIAN_POINT('Ctrl Pts',(0.00297462486737071,-0.0345231616327822,
0.0715911995783497));
#100799=CARTESIAN_POINT('Ctrl Pts',(0.0030098943286801,-0.0344132092796975,
0.0715202256940485));
#100800=CARTESIAN_POINT('Ctrl Pts',(0.00304663000906076,-0.0343032738558974,
0.0714499849926605));
#100801=CARTESIAN_POINT('Ctrl Pts',(0.00308478254082378,-0.0341934961088741,
0.0713805662551144));
#100802=CARTESIAN_POINT('Ctrl Pts',(0.00286645859902239,-0.0345231616327822,
0.0716249811492146));
#100803=CARTESIAN_POINT('Ctrl Pts',(0.00290126242893806,-0.0344132092796975,
0.0715525163451901));
#100804=CARTESIAN_POINT('Ctrl Pts',(0.00293756334044789,-0.0343032738558974,
0.0714807751697854));
#100805=CARTESIAN_POINT('Ctrl Pts',(0.00297531247361221,-0.0341934961088741,
0.0714098483404771));
#100806=CARTESIAN_POINT('Ctrl Pts',(0.00275829233067407,-0.0345231616327822,
0.0716587627200794));
#100807=CARTESIAN_POINT('Ctrl Pts',(0.00279263052919602,-0.0344132092796975,
0.0715848069963317));
#100808=CARTESIAN_POINT('Ctrl Pts',(0.00282849667183502,-0.0343032738558974,
0.0715115653469102));
#100809=CARTESIAN_POINT('Ctrl Pts',(0.00286584240640064,-0.0341934961088741,
0.0714391304258398));
#100810=CARTESIAN_POINT('Ctrl Pts',(0.00265012606232575,-0.0345231616327822,
0.0716925442909443));
#100811=CARTESIAN_POINT('Ctrl Pts',(0.00268399862945398,-0.0344132092796975,
0.0716170976474733));
#100812=CARTESIAN_POINT('Ctrl Pts',(0.00271943000322216,-0.0343032738558974,
0.0715423555240351));
#100813=CARTESIAN_POINT('Ctrl Pts',(0.00275637233918907,-0.0341934961088741,
0.0714684125112026));
#100814=CARTESIAN_POINT('Origin',(0.0180460650678999,-0.0345625596232997,
0.0790165815698863));
#100815=CARTESIAN_POINT('Ctrl Pts',(0.00292251633834766,-0.0346945769586886,
0.0711588742072382));
#100816=CARTESIAN_POINT('Ctrl Pts',(0.00296373556363058,-0.0345846629176052,
0.07108719813479));
#100817=CARTESIAN_POINT('Ctrl Pts',(0.00300644406100104,-0.0344746925050311,
0.0710163622165435));
#100818=CARTESIAN_POINT('Ctrl Pts',(0.00305058673257186,-0.0343648066253259,
0.0709464569896416));
#100819=CARTESIAN_POINT('Ctrl Pts',(0.00295861430413636,-0.0346945769586886,
0.0712662895620416));
#100820=CARTESIAN_POINT('Ctrl Pts',(0.00299835329153721,-0.0345846629176052,
0.0711951109378076));
#100821=CARTESIAN_POINT('Ctrl Pts',(0.00303957101117255,-0.0344746925050311,
0.0711247419420293));
#100822=CARTESIAN_POINT('Ctrl Pts',(0.00308221427778222,-0.0343648066253259,
0.0710552725214632));
#100823=CARTESIAN_POINT('Ctrl Pts',(0.00299471226992506,-0.0346945769586886,
0.0713737049168451));
#100824=CARTESIAN_POINT('Ctrl Pts',(0.00303297101944384,-0.0345846629176052,
0.0713030237408253));
#100825=CARTESIAN_POINT('Ctrl Pts',(0.00307269796134406,-0.0344746925050311,
0.071233121667515));
#100826=CARTESIAN_POINT('Ctrl Pts',(0.00311384182299258,-0.0343648066253259,
0.0711640880532847));
#100827=CARTESIAN_POINT('Ctrl Pts',(0.00303081023571377,-0.0346945769586886,
0.0714811202716486));
#100828=CARTESIAN_POINT('Ctrl Pts',(0.00306758874735047,-0.0345846629176052,
0.071410936543843));
#100829=CARTESIAN_POINT('Ctrl Pts',(0.00310582491151557,-0.0344746925050311,
0.0713415013930008));
#100830=CARTESIAN_POINT('Ctrl Pts',(0.00314546936820293,-0.0343648066253259,
0.0712729035851062));
#100831=CARTESIAN_POINT('Origin',(0.0178350709883733,-0.0345626446729731,
0.0794486390679691));
#100832=CARTESIAN_POINT('Ctrl Pts',(0.00303016432206027,-0.0346945769586886,
0.0714791982507607));
#100833=CARTESIAN_POINT('Ctrl Pts',(0.00308610533402788,-0.0345275153362891,
0.0713725103850799));
#100834=CARTESIAN_POINT('Ctrl Pts',(0.00314541605038269,-0.0343603235965159,
0.0712675542177887));
#100835=CARTESIAN_POINT('Ctrl Pts',(0.003207916442797,-0.034193496108874,
0.0711646375555192));
#100836=CARTESIAN_POINT('Ctrl Pts',(0.0029928568596655,-0.0346945769586886,
0.0715542727576251));
#100837=CARTESIAN_POINT('Ctrl Pts',(0.00304722540602866,-0.0345275153362891,
0.0714468034722074));
#100838=CARTESIAN_POINT('Ctrl Pts',(0.00310498782499035,-0.0343603235965159,
0.0713410162304682));
#100839=CARTESIAN_POINT('Ctrl Pts',(0.00316596863086776,-0.034193496108874,
0.0712372213650474));
#100840=CARTESIAN_POINT('Ctrl Pts',(0.00295554939727072,-0.0346945769586886,
0.0716293472644895));
#100841=CARTESIAN_POINT('Ctrl Pts',(0.00300834547802944,-0.0345275153362891,
0.0715210965593349));
#100842=CARTESIAN_POINT('Ctrl Pts',(0.00306455959959802,-0.0343603235965159,
0.0714144782431476));
#100843=CARTESIAN_POINT('Ctrl Pts',(0.00312402081893851,-0.034193496108874,
0.0713098051745756));
#100844=CARTESIAN_POINT('Ctrl Pts',(0.00291824193487594,-0.0346945769586886,
0.071704421771354));
#100845=CARTESIAN_POINT('Ctrl Pts',(0.00296946555003022,-0.0345275153362891,
0.0715953896464624));
#100846=CARTESIAN_POINT('Ctrl Pts',(0.00302413137420568,-0.0343603235965159,
0.0714879402558271));
#100847=CARTESIAN_POINT('Ctrl Pts',(0.00308207300700927,-0.034193496108874,
0.0713823889841038));
#100848=CARTESIAN_POINT('Ctrl Pts',(0.00314545406140031,-0.0340223579322365,
0.0712729311837875));
#100849=CARTESIAN_POINT('Ctrl Pts',(0.00318513634408598,-0.0339125849573554,
0.071204267054827));
#100850=CARTESIAN_POINT('Ctrl Pts',(0.00322621193040712,-0.0338030433565221,
0.0711364725063977));
#100851=CARTESIAN_POINT('Ctrl Pts',(0.00326862060621732,-0.0336938721132328,
0.0710696295798466));
#100852=CARTESIAN_POINT('Ctrl Pts',(0.0030353798891439,-0.0340223579322365,
0.0712998543417083));
#100853=CARTESIAN_POINT('Ctrl Pts',(0.00307469083126329,-0.0339125849573554,
0.071229672002827));
#100854=CARTESIAN_POINT('Ctrl Pts',(0.00311542676137242,-0.0338030433565221,
0.0711603526254184));
#100855=CARTESIAN_POINT('Ctrl Pts',(0.00315752772682866,-0.0336938721132328,
0.0710919802393335));
#100856=CARTESIAN_POINT('Ctrl Pts',(0.00292530571688748,-0.0340223579322365,
0.0713267774996291));
#100857=CARTESIAN_POINT('Ctrl Pts',(0.00296424531844061,-0.0339125849573554,
0.0712550769508269));
#100858=CARTESIAN_POINT('Ctrl Pts',(0.00300464159233771,-0.0338030433565221,
0.0711842327444392));
#100859=CARTESIAN_POINT('Ctrl Pts',(0.00304643484743999,-0.0336938721132328,
0.0711143308988204));
#100860=CARTESIAN_POINT('Ctrl Pts',(0.00281523154463107,-0.0340223579322365,
0.0713537006575499));
#100861=CARTESIAN_POINT('Ctrl Pts',(0.00285379980561793,-0.0339125849573554,
0.0712804818988268));
#100862=CARTESIAN_POINT('Ctrl Pts',(0.00289385642330301,-0.0338030433565221,
0.0712081128634599));
#100863=CARTESIAN_POINT('Ctrl Pts',(0.00293534196805132,-0.0336938721132328,
0.0711366815583073));
#100864=CARTESIAN_POINT('Origin',(0.0179392954629266,-0.0345589643417464,
0.078961326438295));
#100865=CARTESIAN_POINT('Ctrl Pts',(0.00312059419090093,-0.034193496108874,
0.0708381863255022));
#100866=CARTESIAN_POINT('Ctrl Pts',(0.00316626214029408,-0.0340836138581107,
0.070769195325722));
#100867=CARTESIAN_POINT('Ctrl Pts',(0.00321333580132424,-0.0339738896643499,
0.0707011824315089));
#100868=CARTESIAN_POINT('Ctrl Pts',(0.00326174909025732,-0.0338644633294062,
0.070634230652218));
#100869=CARTESIAN_POINT('Ctrl Pts',(0.00314987630261111,-0.034193496108874,
0.0709476564912127));
#100870=CARTESIAN_POINT('Ctrl Pts',(0.00319403472324476,-0.0340836138581107,
0.0708790692744129));
#100871=CARTESIAN_POINT('Ctrl Pts',(0.00323959122437419,-0.0339738896643499,
0.0708114287329071));
#100872=CARTESIAN_POINT('Ctrl Pts',(0.00328648169598912,-0.0338644633294062,
0.070744817529652));
#100873=CARTESIAN_POINT('Ctrl Pts',(0.00317915841432129,-0.034193496108874,
0.0710571266569233));
#100874=CARTESIAN_POINT('Ctrl Pts',(0.00322180730619545,-0.0340836138581107,
0.0709889432231037));
#100875=CARTESIAN_POINT('Ctrl Pts',(0.00326584664742414,-0.0339738896643499,
0.0709216750343054));
#100876=CARTESIAN_POINT('Ctrl Pts',(0.00331121430172092,-0.0338644633294062,
0.0708554044070861));
#100877=CARTESIAN_POINT('Ctrl Pts',(0.00320844052603147,-0.034193496108874,
0.0711665968226338));
#100878=CARTESIAN_POINT('Ctrl Pts',(0.00324957988914614,-0.0340836138581107,
0.0710988171717946));
#100879=CARTESIAN_POINT('Ctrl Pts',(0.00329210207047409,-0.0339738896643499,
0.0710319213357036));
#100880=CARTESIAN_POINT('Ctrl Pts',(0.00333594690745272,-0.0338644633294062,
0.0709659912845202));
#100881=CARTESIAN_POINT('Origin',(0.0177695446677903,-0.0345610621860672,
0.0794115871179137));
#100882=CARTESIAN_POINT('Ctrl Pts',(0.00318923509526838,-0.0342436276873901,
0.0711956185183359));
#100883=CARTESIAN_POINT('Ctrl Pts',(0.00330066142973354,-0.0339430054201861,
0.0710095090064905));
#100884=CARTESIAN_POINT('Ctrl Pts',(0.00342578974465575,-0.0336441434784162,
0.0708323213003242));
#100885=CARTESIAN_POINT('Ctrl Pts',(0.0030655062326716,-0.0342436276873901,
0.0714128538022115));
#100886=CARTESIAN_POINT('Ctrl Pts',(0.00316873940333953,-0.0339430054201861,
0.0712220777793848));
#100887=CARTESIAN_POINT('Ctrl Pts',(0.00328604933111146,-0.0336441434784162,
0.0710396196766382));
#100888=CARTESIAN_POINT('Ctrl Pts',(0.00333593165678936,-0.0335235895815127,
0.0709660144458022));
#100889=CARTESIAN_POINT('Ctrl Pts',(0.00337976548663298,-0.0334144449262719,
0.0709001002567604));
#100890=CARTESIAN_POINT('Ctrl Pts',(0.0034250114137761,-0.0333049234473133,
0.070835015914237));
#100891=CARTESIAN_POINT('Ctrl Pts',(0.00347161912125876,-0.0331951640388588,
0.0707708498819393));
#100892=CARTESIAN_POINT('Ctrl Pts',(0.00322438419449067,-0.0335235895815127,
0.0709859728059811));
#100893=CARTESIAN_POINT('Ctrl Pts',(0.00326794325821204,-0.0334144449262719,
0.0709185229465041));
#100894=CARTESIAN_POINT('Ctrl Pts',(0.0033129458293554,-0.0333049234473133,
0.0708518954927849));
#100895=CARTESIAN_POINT('Ctrl Pts',(0.00335934208087624,-0.0331951640388588,
0.0707861808535084));
#100896=CARTESIAN_POINT('Ctrl Pts',(0.00311283673219199,-0.0335235895815127,
0.0710059311661601));
#100897=CARTESIAN_POINT('Ctrl Pts',(0.0031561210297911,-0.0334144449262719,
0.0709369456362478));
#100898=CARTESIAN_POINT('Ctrl Pts',(0.00320088024493469,-0.0333049234473133,
0.0708687750713328));
#100899=CARTESIAN_POINT('Ctrl Pts',(0.00324706504049372,-0.0331951640388588,
0.0708015118250775));
#100900=CARTESIAN_POINT('Ctrl Pts',(0.00300128926989331,-0.0335235895815127,
0.0710258895263391));
#100901=CARTESIAN_POINT('Ctrl Pts',(0.00304429880137016,-0.0334144449262719,
0.0709553683259915));
#100902=CARTESIAN_POINT('Ctrl Pts',(0.00308881466051398,-0.0333049234473133,
0.0708856546498806));
#100903=CARTESIAN_POINT('Ctrl Pts',(0.00313478800011121,-0.0331951640388588,
0.0708168427966466));
#100904=CARTESIAN_POINT('Origin',(0.0164953312605408,-0.0326434571770201,
0.0811715115522585));
#100905=CARTESIAN_POINT('Ctrl Pts',(0.00333801742936333,-0.0336938721132373,
0.0705285809189424));
#100906=CARTESIAN_POINT('Ctrl Pts',(0.00335921479695864,-0.033647456976495,
0.0705005682496956));
#100907=CARTESIAN_POINT('Ctrl Pts',(0.00338073863575899,-0.033601104548885,
0.0704728056418462));
#100908=CARTESIAN_POINT('Ctrl Pts',(0.00343523204461644,-0.033483750864316,
0.070402517104819));
#100909=CARTESIAN_POINT('Ctrl Pts',(0.0034917843189816,-0.0333660264760404,
0.0703338741859529));
#100910=CARTESIAN_POINT('Ctrl Pts',(0.00340506923980288,-0.0336938721132373,
0.0708618587219665));
#100911=CARTESIAN_POINT('Ctrl Pts',(0.00342431582182383,-0.033647456976495,
0.0708342385292164));
#100912=CARTESIAN_POINT('Ctrl Pts',(0.00344388441428595,-0.033601104548885,
0.0708068455345627));
#100913=CARTESIAN_POINT('Ctrl Pts',(0.00349342758916729,-0.033483750864316,
0.0707374927731274));
#100914=CARTESIAN_POINT('Ctrl Pts',(0.00354500407436432,-0.0333660264760404,
0.0706696385332396));
#100915=CARTESIAN_POINT('Ctrl Pts',(0.0034050692398148,-0.0336938721132427,
0.0708618587219738));
#100916=CARTESIAN_POINT('Ctrl Pts',(0.0034243158218348,-0.0336474569765026,
0.070834238529225));
#100917=CARTESIAN_POINT('Ctrl Pts',(0.00344388441429596,-0.0336011045488949,
0.0708068455345727));
#100918=CARTESIAN_POINT('Ctrl Pts',(0.00349301496201041,-0.0334847282606778,
0.0707380703871787));
#100919=CARTESIAN_POINT('Ctrl Pts',(0.00354414527714575,-0.0333679869945434,
0.0706707686599204));
#100920=CARTESIAN_POINT('Ctrl Pts',(0.00340506923980075,-0.0336938721132425,
0.0708618587219697));
#100921=CARTESIAN_POINT('Ctrl Pts',(0.00347390353456838,-0.0335278710435082,
0.0707630766895424));
#100922=CARTESIAN_POINT('Ctrl Pts',(0.00354581139244494,-0.0333620469224319,
0.0706664880339919));
#100923=CARTESIAN_POINT('Ctrl Pts',(0.00362084464106375,-0.0331951640388601,
0.0705720566798247));
#100924=CARTESIAN_POINT('Ctrl Pts',(0.00335864662225908,-0.0336938721132425,
0.0709316653864356));
#100925=CARTESIAN_POINT('Ctrl Pts',(0.00342601957698312,-0.0335278710435082,
0.0708319115380583));
#100926=CARTESIAN_POINT('Ctrl Pts',(0.00349649708480763,-0.0333620469224319,
0.0707343055811966));
#100927=CARTESIAN_POINT('Ctrl Pts',(0.00357013043122506,-0.0331951640388601,
0.0706388106965107));
#100928=CARTESIAN_POINT('Ctrl Pts',(0.00331222400471741,-0.0336938721132425,
0.0710014720509014));
#100929=CARTESIAN_POINT('Ctrl Pts',(0.00337813561939785,-0.0335278710435082,
0.0709007463865742));
#100930=CARTESIAN_POINT('Ctrl Pts',(0.00344718277717032,-0.0333620469224319,
0.0708021231284014));
#100931=CARTESIAN_POINT('Ctrl Pts',(0.00351941622138638,-0.0331951640388601,
0.0707055647131967));
#100932=CARTESIAN_POINT('Ctrl Pts',(0.00326580138717574,-0.0336938721132425,
0.0710712787153673));
#100933=CARTESIAN_POINT('Ctrl Pts',(0.00333025166181258,-0.0335278710435082,
0.0709695812350901));
#100934=CARTESIAN_POINT('Ctrl Pts',(0.00339786846953301,-0.0333620469224319,
0.0708699406756061));
#100935=CARTESIAN_POINT('Ctrl Pts',(0.00346870201154769,-0.0331951640388601,
0.0707723187298827));
#100936=CARTESIAN_POINT('Ctrl Pts',(0.0035453024560874,-0.0330240426238156,
0.0706716664798157));
#100937=CARTESIAN_POINT('Ctrl Pts',(0.00359321988910383,-0.0329142774063509,
0.0706085934608418));
#100938=CARTESIAN_POINT('Ctrl Pts',(0.00364246510619618,-0.0328043479726686,
0.070546479584859));
#100939=CARTESIAN_POINT('Ctrl Pts',(0.00369297721198627,-0.0326943950436594,
0.0704854061617673));
#100940=CARTESIAN_POINT('Ctrl Pts',(0.0034327220734972,-0.0330240426238156,
0.0706845813332973));
#100941=CARTESIAN_POINT('Ctrl Pts',(0.00348046159182459,-0.0329142774063509,
0.0706199574098715));
#100942=CARTESIAN_POINT('Ctrl Pts',(0.0035295608670582,-0.0328043479726686,
0.0705562881782607));
#100943=CARTESIAN_POINT('Ctrl Pts',(0.00357995924565606,-0.0326943950436594,
0.0704936569357425));
#100944=CARTESIAN_POINT('Ctrl Pts',(0.003320141690907,-0.0330240426238156,
0.0706974961867789));
#100945=CARTESIAN_POINT('Ctrl Pts',(0.00336770329454535,-0.0329142774063509,
0.0706313213589012));
#100946=CARTESIAN_POINT('Ctrl Pts',(0.00341665662792022,-0.0328043479726686,
0.0705660967716625));
#100947=CARTESIAN_POINT('Ctrl Pts',(0.00346694127932585,-0.0326943950436594,
0.0705019077097177));
#100948=CARTESIAN_POINT('Ctrl Pts',(0.0032075613083168,-0.0330240426238156,
0.0707104110402606));
#100949=CARTESIAN_POINT('Ctrl Pts',(0.00325494499726611,-0.0329142774063509,
0.0706426853079309));
#100950=CARTESIAN_POINT('Ctrl Pts',(0.00330375238878223,-0.0328043479726686,
0.0705759053650642));
#100951=CARTESIAN_POINT('Ctrl Pts',(0.00335392331299563,-0.0326943950436594,
0.070510158483693));
#100952=CARTESIAN_POINT('Origin',(0.0165918406917995,-0.0326396682856393,
0.0812488506009495));
#100953=CARTESIAN_POINT('Ctrl Pts',(0.00357512613946548,-0.0331951640388587,
0.0702372352350697));
#100954=CARTESIAN_POINT('Ctrl Pts',(0.00362901655864372,-0.0330855618255041,
0.070174586699787));
#100955=CARTESIAN_POINT('Ctrl Pts',(0.00368424066480755,-0.0329757224427708,
0.0701130068248977));
#100956=CARTESIAN_POINT('Ctrl Pts',(0.00374073160826077,-0.0328657862078596,
0.0700525779359834));
#100957=CARTESIAN_POINT('Ctrl Pts',(0.00359045709882897,-0.0331951640388587,
0.070349512186064));
#100958=CARTESIAN_POINT('Ctrl Pts',(0.00364280113014169,-0.0330855618255041,
0.0702870748037323));
#100959=CARTESIAN_POINT('Ctrl Pts',(0.00369647336950004,-0.0329757224427708,
0.0702256742728173));
#100960=CARTESIAN_POINT('Ctrl Pts',(0.0037514089432011,-0.0328657862078596,
0.0701653925917607));
#100961=CARTESIAN_POINT('Ctrl Pts',(0.00360578805819247,-0.0331951640388587,
0.0704617891370583));
#100962=CARTESIAN_POINT('Ctrl Pts',(0.00365658570163966,-0.0330855618255041,
0.0703995629076776));
#100963=CARTESIAN_POINT('Ctrl Pts',(0.00370870607419253,-0.0329757224427708,
0.0703383417207369));
#100964=CARTESIAN_POINT('Ctrl Pts',(0.00376208627814143,-0.0328657862078596,
0.0702782072475381));
#100965=CARTESIAN_POINT('Ctrl Pts',(0.00362111901755597,-0.0331951640388587,
0.0705740660880526));
#100966=CARTESIAN_POINT('Ctrl Pts',(0.00367037027313763,-0.0330855618255041,
0.0705120510116229));
#100967=CARTESIAN_POINT('Ctrl Pts',(0.00372093877888502,-0.0329757224427708,
0.0704510091686565));
#100968=CARTESIAN_POINT('Ctrl Pts',(0.00377276361308176,-0.0328657862078596,
0.0703910219033155));
#100969=CARTESIAN_POINT('Origin',(0.016254341606255,-0.032640190883445,
0.0815914396239748));
#100970=CARTESIAN_POINT('Ctrl Pts',(0.00359847238323193,-0.0332451089994432,
0.0706003949339911));
#100971=CARTESIAN_POINT('Ctrl Pts',(0.00373234792861486,-0.0329451141710257,
0.070429720082125));
#100972=CARTESIAN_POINT('Ctrl Pts',(0.00387869907526945,-0.0326442513127503,
0.0702696141528658));
#100973=CARTESIAN_POINT('Ctrl Pts',(0.00344848983885165,-0.0332451089994432,
0.0708004080245157));
#100974=CARTESIAN_POINT('Ctrl Pts',(0.00357482176710542,-0.0329451141710257,
0.0706240764884401));
#100975=CARTESIAN_POINT('Ctrl Pts',(0.00371407681183032,-0.0326442513127503,
0.0704577617289336));
#100976=CARTESIAN_POINT('Ctrl Pts',(0.00377274289495567,-0.0325229783203385,
0.0703910457473858));
#100977=CARTESIAN_POINT('Ctrl Pts',(0.00382455999618189,-0.032413025311208,
0.0703310667669035));
#100978=CARTESIAN_POINT('Ctrl Pts',(0.0038776099805667,-0.0323031222247695,
0.0702721687866917));
#100979=CARTESIAN_POINT('Ctrl Pts',(0.00393182223267944,-0.0321934096636184,
0.0702144248530265));
#100980=CARTESIAN_POINT('Ctrl Pts',(0.00365957370523785,-0.0325229783203385,
0.0703968661552763));
#100981=CARTESIAN_POINT('Ctrl Pts',(0.00371131057227004,-0.032413025311208,
0.070335327140017));
#100982=CARTESIAN_POINT('Ctrl Pts',(0.00376431260595269,-0.0323031222247695,
0.0702748677018907));
#100983=CARTESIAN_POINT('Ctrl Pts',(0.00381850918169905,-0.0321934096636184,
0.0702155628894573));
#100984=CARTESIAN_POINT('Ctrl Pts',(0.00354640451552002,-0.0325229783203385,
0.0704026865631669));
#100985=CARTESIAN_POINT('Ctrl Pts',(0.00359806114835818,-0.032413025311208,
0.0703395875131305));
#100986=CARTESIAN_POINT('Ctrl Pts',(0.00365101523133868,-0.0323031222247695,
0.0702775666170897));
#100987=CARTESIAN_POINT('Ctrl Pts',(0.00370519613071867,-0.0321934096636184,
0.0702167009258881));
#100988=CARTESIAN_POINT('Ctrl Pts',(0.00343323532580219,-0.0325229783203385,
0.0704085069710574));
#100989=CARTESIAN_POINT('Ctrl Pts',(0.00348481172444633,-0.032413025311208,
0.070343847886244));
#100990=CARTESIAN_POINT('Ctrl Pts',(0.00353771785672467,-0.0323031222247695,
0.0702802655322886));
#100991=CARTESIAN_POINT('Ctrl Pts',(0.00359188307973828,-0.0321934096636184,
0.070217838962319));
#100992=CARTESIAN_POINT('Origin',(0.0165854626521562,-0.0326393375177015,
0.0812431927181626));
#100993=CARTESIAN_POINT('Ctrl Pts',(0.00382978640553164,-0.0326943950436593,
0.0699593437057789));
#100994=CARTESIAN_POINT('Ctrl Pts',(0.0038875415033928,-0.0325844576448127,
0.0699001643960204));
#100995=CARTESIAN_POINT('Ctrl Pts',(0.00394652461382358,-0.0324744968375319,
0.0698421753681648));
#100996=CARTESIAN_POINT('Ctrl Pts',(0.00400665913941762,-0.0323646534831894,
0.069785449878763));
#100997=CARTESIAN_POINT('Ctrl Pts',(0.0038380371768073,-0.0326943950436593,
0.0700723616351306));
#100998=CARTESIAN_POINT('Ctrl Pts',(0.00389423467578382,-0.0325844576448127,
0.0700132960364639));
#100999=CARTESIAN_POINT('Ctrl Pts',(0.00395165772536446,-0.0324744968375319,
0.0699553885140489));
#101000=CARTESIAN_POINT('Ctrl Pts',(0.00401023172842419,-0.0323646534831894,
0.0698987122475771));
#101001=CARTESIAN_POINT('Ctrl Pts',(0.00384628794808296,-0.0326943950436593,
0.0701853795644822));
#101002=CARTESIAN_POINT('Ctrl Pts',(0.00390092784817484,-0.0325844576448127,
0.0701264276769074));
#101003=CARTESIAN_POINT('Ctrl Pts',(0.00395679083690534,-0.0324744968375319,
0.070068601659933));
#101004=CARTESIAN_POINT('Ctrl Pts',(0.00401380431743077,-0.0323646534831894,
0.0700119746163912));
#101005=CARTESIAN_POINT('Ctrl Pts',(0.00385453871935861,-0.0326943950436593,
0.0702983974938339));
#101006=CARTESIAN_POINT('Ctrl Pts',(0.00390762102056586,-0.0325844576448127,
0.0702395593173508));
#101007=CARTESIAN_POINT('Ctrl Pts',(0.00396192394844622,-0.0324744968375319,
0.0701818148058171));
#101008=CARTESIAN_POINT('Ctrl Pts',(0.00401737690643735,-0.0323646534831894,
0.0701252369852052));
#101009=CARTESIAN_POINT('Origin',(0.0162825633549792,-0.032639557906579,
0.0816166486439388));
#101010=CARTESIAN_POINT('Ctrl Pts',(0.00383025749695593,-0.0327445246961876,
0.0703232819958182));
#101011=CARTESIAN_POINT('Ctrl Pts',(0.00397458452440749,-0.0324436878365475,
0.0701613490663448));
#101012=CARTESIAN_POINT('Ctrl Pts',(0.00413069898397488,-0.0321434074463186,
0.0700107474726786));
#101013=CARTESIAN_POINT('Ctrl Pts',(0.00366801328014326,-0.0327445246961876,
0.070513484030799));
#101014=CARTESIAN_POINT('Ctrl Pts',(0.00380516672064799,-0.0324436878365475,
0.0703454319607179));
#101015=CARTESIAN_POINT('Ctrl Pts',(0.00395458889134602,-0.0321434074463186,
0.0701881882663937));
#101016=CARTESIAN_POINT('Ctrl Pts',(0.00408298943779383,-0.0322357242816072,
0.0700573090870923));
#101017=CARTESIAN_POINT('Ctrl Pts',(0.00421333633534426,-0.0319819883628705,
0.0699286150785516));
#101018=CARTESIAN_POINT('Ctrl Pts',(0.00435160823665694,-0.0317295851069887,
0.0698084762303691));
#101019=CARTESIAN_POINT('Ctrl Pts',(0.00390894787970366,-0.0322357242816072,
0.07023677924076));
#101020=CARTESIAN_POINT('Ctrl Pts',(0.00403357888562404,-0.0319819883628705,
0.0701025422343179));
#101021=CARTESIAN_POINT('Ctrl Pts',(0.00416649919608388,-0.0317295851069887,
0.0699765079032707));
#101022=CARTESIAN_POINT('Origin',(0.0162134206443787,-0.0326371942647745,
0.0815510613820758));
#101023=CARTESIAN_POINT('Origin',(0.0164933025329328,-0.0326352985527776,
0.0811621352362565));
#101024=CARTESIAN_POINT('Ctrl Pts',(0.00410139311123134,-0.0321934096636183,
0.0696979907823519));
#101025=CARTESIAN_POINT('Ctrl Pts',(0.0041627897880276,-0.0320835708272304,
0.0696425189020534));
#101026=CARTESIAN_POINT('Ctrl Pts',(0.00422529883993577,-0.0319739230346346,
0.0695883497987352));
#101027=CARTESIAN_POINT('Ctrl Pts',(0.00428883497194882,-0.0318646057455575,
0.0695355466400723));
#101028=CARTESIAN_POINT('Ctrl Pts',(0.00410253114864214,-0.0321934096636183,
0.0698113039309076));
#101029=CARTESIAN_POINT('Ctrl Pts',(0.00416236514880892,-0.0320835708272304,
0.069755847745032));
#101030=CARTESIAN_POINT('Ctrl Pts',(0.0042233121057083,-0.0319739230346346,
0.0697016619875215));
#101031=CARTESIAN_POINT('Ctrl Pts',(0.00428528872129011,-0.0318646057455575,
0.0696488100007457));
#101032=CARTESIAN_POINT('Ctrl Pts',(0.00410366918605294,-0.0321934096636184,
0.0699246170794633));
#101033=CARTESIAN_POINT('Ctrl Pts',(0.00416194050959024,-0.0320835708272304,
0.0698691765880105));
#101034=CARTESIAN_POINT('Ctrl Pts',(0.00422132537148083,-0.0319739230346346,
0.0698149741763078));
#101035=CARTESIAN_POINT('Ctrl Pts',(0.0042817424706314,-0.0318646057455575,
0.069762073361419));
#101036=CARTESIAN_POINT('Ctrl Pts',(0.00410480722346373,-0.0321934096636184,
0.0700379302280189));
#101037=CARTESIAN_POINT('Ctrl Pts',(0.00416151587037156,-0.0320835708272304,
0.0699825054309891));
#101038=CARTESIAN_POINT('Ctrl Pts',(0.00421933863725336,-0.0319739230346346,
0.0699282863650941));
#101039=CARTESIAN_POINT('Ctrl Pts',(0.00427819621997269,-0.0318646057455575,
0.0698753367220923));
#101040=CARTESIAN_POINT('Ctrl Pts',(0.00401645716895846,-0.0320218834582383,
0.070124993298592));
#101041=CARTESIAN_POINT('Ctrl Pts',(0.0040583477583289,-0.0319391099350678,
0.070082245974485));
#101042=CARTESIAN_POINT('Ctrl Pts',(0.00410088047271536,-0.0318564869454957,
0.0700401786773225));
#101043=CARTESIAN_POINT('Ctrl Pts',(0.00414402147217898,-0.0317740741446548,
0.0699988191554047));
#101044=CARTESIAN_POINT('Ctrl Pts',(0.00396689405046831,-0.0320218834582383,
0.0701244229191482));
#101045=CARTESIAN_POINT('Ctrl Pts',(0.00400879057610988,-0.0319391099350678,
0.0700811597627959));
#101046=CARTESIAN_POINT('Ctrl Pts',(0.00405133727796367,-0.0318564869454957,
0.0700385770386133));
#101047=CARTESIAN_POINT('Ctrl Pts',(0.00409450027085473,-0.0317740741446548,
0.0699967028693698));
#101048=CARTESIAN_POINT('Ctrl Pts',(0.00391733093197817,-0.0320218834582383,
0.0701238525397044));
#101049=CARTESIAN_POINT('Ctrl Pts',(0.00395923339389086,-0.0319391099350678,
0.0700800735511067));
#101050=CARTESIAN_POINT('Ctrl Pts',(0.00400179408321198,-0.0318564869454957,
0.0700369753999041));
#101051=CARTESIAN_POINT('Ctrl Pts',(0.00404497906953048,-0.0317740741446548,
0.069994586583335));
#101052=CARTESIAN_POINT('Ctrl Pts',(0.00386776781348802,-0.0320218834582383,
0.0701232821602607));
#101053=CARTESIAN_POINT('Ctrl Pts',(0.00390967621167184,-0.0319391099350678,
0.0700789873394175));
#101054=CARTESIAN_POINT('Ctrl Pts',(0.00395225088846029,-0.0318564869454957,
0.0700353737611948));
#101055=CARTESIAN_POINT('Ctrl Pts',(0.00399545786820623,-0.0317740741446548,
0.0699924702973002));
#101056=CARTESIAN_POINT('Origin',(-0.00113568647615043,-0.0391228853390614,
0.0663948173269696));
#101057=CARTESIAN_POINT('Ctrl Pts',(0.00253836287828677,-0.0352722978779618,
0.0727762257753859));
#101058=CARTESIAN_POINT('Ctrl Pts',(0.00254321541858433,-0.0352466642097233,
0.0727579625464622));
#101059=CARTESIAN_POINT('Ctrl Pts',(0.00254798786384325,-0.0352210183808309,
0.0727396954553567));
#101060=CARTESIAN_POINT('Ctrl Pts',(0.00255267986725082,-0.0351953608940152,
0.0727214237228355));
#101061=CARTESIAN_POINT('Origin',(-0.00214754511313579,-0.0352456003065105,
0.071343742096256));
#101062=CARTESIAN_POINT('Ctrl Pts',(0.00258635952736725,-0.035024121149334,
0.0726013779152761));
#101063=CARTESIAN_POINT('Ctrl Pts',(0.0026076911606627,-0.0349144232867421,
0.0725251021919265));
#101064=CARTESIAN_POINT('Ctrl Pts',(0.00263061223560249,-0.0348045283677512,
0.072449221753965));
#101065=CARTESIAN_POINT('Ctrl Pts',(0.00265509700998915,-0.0346945769586886,
0.072373834887098));
#101066=CARTESIAN_POINT('Ctrl Pts',(0.00248643918556934,-0.035024121149334,
0.0726548294549921));
#101067=CARTESIAN_POINT('Ctrl Pts',(0.00250703454585438,-0.0349144232867421,
0.0725771773699653));
#101068=CARTESIAN_POINT('Ctrl Pts',(0.00252924735746698,-0.0348045283677512,
0.0724999045272192));
#101069=CARTESIAN_POINT('Ctrl Pts',(0.00255305285177284,-0.0346945769586886,
0.0724231109621948));
#101070=CARTESIAN_POINT('Ctrl Pts',(0.00238651884377143,-0.035024121149334,
0.0727082809947082));
#101071=CARTESIAN_POINT('Ctrl Pts',(0.00240637793104606,-0.0349144232867421,
0.0726292525480041));
#101072=CARTESIAN_POINT('Ctrl Pts',(0.00242788247933147,-0.0348045283677512,
0.0725505873004734));
#101073=CARTESIAN_POINT('Ctrl Pts',(0.00245100869355653,-0.0346945769586886,
0.0724723870372917));
#101074=CARTESIAN_POINT('Ctrl Pts',(0.00228659850197351,-0.035024121149334,
0.0727617325344242));
#101075=CARTESIAN_POINT('Ctrl Pts',(0.00230572131623774,-0.0349144232867421,
0.0726813277260428));
#101076=CARTESIAN_POINT('Ctrl Pts',(0.00232651760119597,-0.0348045283677512,
0.0726012700737276));
#101077=CARTESIAN_POINT('Ctrl Pts',(0.00234896453534022,-0.0346945769586886,
0.0725216631123886));
#101078=CARTESIAN_POINT('Origin',(0.0185662413236461,-0.0345629067939343,
0.0777309269808658));
#101079=CARTESIAN_POINT('Ctrl Pts',(0.00249918449119187,-0.0351970973651637,
0.0722686647112246));
#101080=CARTESIAN_POINT('Ctrl Pts',(0.00252524784195756,-0.0350869349321779,
0.0721907435327427));
#101081=CARTESIAN_POINT('Ctrl Pts',(0.00255295272141885,-0.0349764985129713,
0.0721132996478823));
#101082=CARTESIAN_POINT('Ctrl Pts',(0.00258226914315024,-0.0348659306849617,
0.0720364355003123));
#101083=CARTESIAN_POINT('Ctrl Pts',(0.0025395345452969,-0.0351970973651637,
0.0723403050893907));
#101084=CARTESIAN_POINT('Ctrl Pts',(0.00256460541571298,-0.0350869349321779,
0.0722629429062244));
#101085=CARTESIAN_POINT('Ctrl Pts',(0.00259130537146266,-0.0349764985129713,
0.0721860378466283));
#101086=CARTESIAN_POINT('Ctrl Pts',(0.00261960568693649,-0.0348659306849617,
0.0721096915795697));
#101087=CARTESIAN_POINT('Ctrl Pts',(0.00257988459940193,-0.0351970973651637,
0.0724119454675567));
#101088=CARTESIAN_POINT('Ctrl Pts',(0.0026039629894684,-0.0350869349321779,
0.0723351422797061));
#101089=CARTESIAN_POINT('Ctrl Pts',(0.00262965802150647,-0.0349764985129713,
0.0722587760453744));
#101090=CARTESIAN_POINT('Ctrl Pts',(0.00265694223072274,-0.0348659306849617,
0.072182947658827));
#101091=CARTESIAN_POINT('Ctrl Pts',(0.00262023465350695,-0.0351970973651637,
0.0724835858457228));
#101092=CARTESIAN_POINT('Ctrl Pts',(0.00264332056322382,-0.0350869349321779,
0.0724073416531878));
#101093=CARTESIAN_POINT('Ctrl Pts',(0.00266801067155029,-0.0349764985129713,
0.0723315142441205));
#101094=CARTESIAN_POINT('Ctrl Pts',(0.00269427877450898,-0.0348659306849617,
0.0722562037380843));
#101095=CARTESIAN_POINT('Origin',(0.0183679165695076,-0.0345637187966988,
0.0781690966371691));
#101096=CARTESIAN_POINT('Ctrl Pts',(0.00260956047775145,-0.0352450361861253,
0.0725155325411968));
#101097=CARTESIAN_POINT('Ctrl Pts',(0.00267120542792072,-0.0349452761023765,
0.0723075602618868));
#101098=CARTESIAN_POINT('Ctrl Pts',(0.00274834057391347,-0.0346444289983475,
0.0721048221596576));
#101099=CARTESIAN_POINT('Ctrl Pts',(0.00254373971120484,-0.0352450361861253,
0.072756712197659));
#101100=CARTESIAN_POINT('Ctrl Pts',(0.00259628842160232,-0.0349452761023765,
0.0725462574474671));
#101101=CARTESIAN_POINT('Ctrl Pts',(0.0026645401591411,-0.0346444289983475,
0.0723403587608132));
#101102=CARTESIAN_POINT('Ctrl Pts',(0.00269452477997173,-0.0345231616327823,
0.0722567370217171));
#101103=CARTESIAN_POINT('Ctrl Pts',(0.00272062074462613,-0.0344132092796976,
0.0721819023520605));
#101104=CARTESIAN_POINT('Ctrl Pts',(0.00274826325896179,-0.0343032738558974,
0.0721076113179735));
#101105=CARTESIAN_POINT('Ctrl Pts',(0.00277741447176964,-0.0341934961088741,
0.0720339581877328));
#101106=CARTESIAN_POINT('Ctrl Pts',(0.00259144538846841,-0.0345231616327823,
0.0723038090429803));
#101107=CARTESIAN_POINT('Ctrl Pts',(0.0026168925315818,-0.0344132092796976,
0.072227553569036));
#101108=CARTESIAN_POINT('Ctrl Pts',(0.00264391564606864,-0.0343032738558974,
0.0721518283836065));
#101109=CARTESIAN_POINT('Ctrl Pts',(0.00267247762717917,-0.0341934961088741,
0.0720767296126085));
#101110=CARTESIAN_POINT('Ctrl Pts',(0.00248836599696508,-0.0345231616327823,
0.0723508810642435));
#101111=CARTESIAN_POINT('Ctrl Pts',(0.00251316431853747,-0.0344132092796976,
0.0722732047860115));
#101112=CARTESIAN_POINT('Ctrl Pts',(0.00253956803317549,-0.0343032738558974,
0.0721960454492395));
#101113=CARTESIAN_POINT('Ctrl Pts',(0.0025675407825887,-0.0341934961088741,
0.0721195010374841));
#101114=CARTESIAN_POINT('Ctrl Pts',(0.00238528660546176,-0.0345231616327823,
0.0723979530855067));
#101115=CARTESIAN_POINT('Ctrl Pts',(0.00240943610549314,-0.0344132092796976,
0.072318856002987));
#101116=CARTESIAN_POINT('Ctrl Pts',(0.00243522042028234,-0.0343032738558974,
0.0722402625148725));
#101117=CARTESIAN_POINT('Ctrl Pts',(0.00246260393799823,-0.0341934961088741,
0.0721622724623598));
#101118=CARTESIAN_POINT('Origin',(0.0185777693083837,-0.0345625596232488,
0.07773461532368));
#101119=CARTESIAN_POINT('Ctrl Pts',(0.00258864240555079,-0.0346945769586886,
0.0718343515957248));
#101120=CARTESIAN_POINT('Ctrl Pts',(0.00262055321100165,-0.0345846629176052,
0.0717580745717267));
#101121=CARTESIAN_POINT('Ctrl Pts',(0.0026540468444276,-0.0344746925050311,
0.0716824444217771));
#101122=CARTESIAN_POINT('Ctrl Pts',(0.00268907998971765,-0.0343648066253259,
0.0716075578747029));
#101123=CARTESIAN_POINT('Ctrl Pts',(0.00263791844184932,-0.0346945769586886,
0.0719363956735949));
#101124=CARTESIAN_POINT('Ctrl Pts',(0.00266842302832914,-0.0345846629176052,
0.0718607976982835));
#101125=CARTESIAN_POINT('Ctrl Pts',(0.00270049616015044,-0.0344746925050311,
0.0717858176329729));
#101126=CARTESIAN_POINT('Ctrl Pts',(0.00273409634475257,-0.0343648066253259,
0.0717115513810435));
#101127=CARTESIAN_POINT('Ctrl Pts',(0.00268719447814784,-0.0346945769586886,
0.072038439751465));
#101128=CARTESIAN_POINT('Ctrl Pts',(0.00271629284565663,-0.0345846629176052,
0.0719635208248402));
#101129=CARTESIAN_POINT('Ctrl Pts',(0.00274694547587327,-0.0344746925050311,
0.0718891908441687));
#101130=CARTESIAN_POINT('Ctrl Pts',(0.00277911269978749,-0.0343648066253259,
0.0718155448873842));
#101131=CARTESIAN_POINT('Ctrl Pts',(0.00273647051444636,-0.0346945769586886,
0.0721404838293351));
#101132=CARTESIAN_POINT('Ctrl Pts',(0.00276416266298413,-0.0345846629176052,
0.072066243951397));
#101133=CARTESIAN_POINT('Ctrl Pts',(0.00279339479159611,-0.0344746925050311,
0.0719925640553645));
#101134=CARTESIAN_POINT('Ctrl Pts',(0.00282412905482241,-0.0343648066253259,
0.0719195383937248));
#101135=CARTESIAN_POINT('Origin',(0.0184225901435341,-0.0345626446730962,
0.0781897104893465));
#101136=CARTESIAN_POINT('Ctrl Pts',(0.00273558880092203,-0.0346945769586887,
0.0721386579186026));
#101137=CARTESIAN_POINT('Ctrl Pts',(0.00277771716611366,-0.0345275153362892,
0.0720258000506902));
#101138=CARTESIAN_POINT('Ctrl Pts',(0.00282340570392564,-0.034360323596516,
0.0719142378902611));
#101139=CARTESIAN_POINT('Ctrl Pts',(0.00287251438400793,-0.0341934961088741,
0.071804299380333));
#101140=CARTESIAN_POINT('Ctrl Pts',(0.002707984849715,-0.0346945769586887,
0.0722178163054548));
#101141=CARTESIAN_POINT('Ctrl Pts',(0.00274845521080075,-0.0345275153362892,
0.0721043802617323));
#101142=CARTESIAN_POINT('Ctrl Pts',(0.00279250349875911,-0.034360323596516,
0.0719921876332443));
#101143=CARTESIAN_POINT('Ctrl Pts',(0.00283999450665753,-0.0341934961088741,
0.0718815682997534));
#101144=CARTESIAN_POINT('Ctrl Pts',(0.00268038089850797,-0.0346945769586887,
0.0722969746923069));
#101145=CARTESIAN_POINT('Ctrl Pts',(0.00271919325548784,-0.0345275153362892,
0.0721829604727744));
#101146=CARTESIAN_POINT('Ctrl Pts',(0.00276160129359259,-0.034360323596516,
0.0720701373762274));
#101147=CARTESIAN_POINT('Ctrl Pts',(0.00280747462930714,-0.0341934961088741,
0.0719588372191737));
#101148=CARTESIAN_POINT('Ctrl Pts',(0.00265277694730095,-0.0346945769586887,
0.0723761330791591));
#101149=CARTESIAN_POINT('Ctrl Pts',(0.00268993130017493,-0.0345275153362892,
0.0722615406838164));
#101150=CARTESIAN_POINT('Ctrl Pts',(0.00273069908842606,-0.034360323596516,
0.0721480871192105));
#101151=CARTESIAN_POINT('Ctrl Pts',(0.00277495475195675,-0.0341934961088741,
0.0720361061385941));
#101152=CARTESIAN_POINT('Ctrl Pts',(0.00282411732775041,-0.0340223579322365,
0.0719195676932332));
#101153=CARTESIAN_POINT('Ctrl Pts',(0.00285488080647209,-0.0339125849573554,
0.0718464714926344));
#101154=CARTESIAN_POINT('Ctrl Pts',(0.00288713558955374,-0.0338030433565221,
0.0717740633884145));
#101155=CARTESIAN_POINT('Ctrl Pts',(0.00292083222016277,-0.0336938721132328,
0.0717024323218338));
#101156=CARTESIAN_POINT('Ctrl Pts',(0.00271828548965978,-0.0340223579322365,
0.071960074505953));
#101157=CARTESIAN_POINT('Ctrl Pts',(0.00274849027378785,-0.0339125849573554,
0.071885518608286));
#101158=CARTESIAN_POINT('Ctrl Pts',(0.00278021696720156,-0.0338030433565221,
0.0718116402690302));
#101159=CARTESIAN_POINT('Ctrl Pts',(0.00281341662173569,-0.0336938721132328,
0.0717385303694945));
#101160=CARTESIAN_POINT('Ctrl Pts',(0.00261245365156914,-0.0340223579322365,
0.0720005813186729));
#101161=CARTESIAN_POINT('Ctrl Pts',(0.00264209974110361,-0.0339125849573554,
0.0719245657239375));
#101162=CARTESIAN_POINT('Ctrl Pts',(0.00267329834484938,-0.0338030433565221,
0.0718492171496458));
#101163=CARTESIAN_POINT('Ctrl Pts',(0.00270600102330862,-0.0336938721132328,
0.0717746284171553));
#101164=CARTESIAN_POINT('Ctrl Pts',(0.0025066218134785,-0.0340223579322365,
0.0720410881313928));
#101165=CARTESIAN_POINT('Ctrl Pts',(0.00253570920841937,-0.0339125849573554,
0.0719636128395891));
#101166=CARTESIAN_POINT('Ctrl Pts',(0.00256637972249721,-0.0338030433565221,
0.0718867940302615));
#101167=CARTESIAN_POINT('Ctrl Pts',(0.00259858542488155,-0.0336938721132328,
0.071810726464816));
#101168=CARTESIAN_POINT('Origin',(0.0184649163094403,-0.0345589643418681,
0.0776931776749366));
#101169=CARTESIAN_POINT('Ctrl Pts',(0.00274496550589085,-0.034193496108874,
0.0714913666959631));
#101170=CARTESIAN_POINT('Ctrl Pts',(0.0027816264847734,-0.0340836138581107,
0.0714171959990552));
#101171=CARTESIAN_POINT('Ctrl Pts',(0.00281980467997033,-0.03397388966435,
0.0713438195126748));
#101172=CARTESIAN_POINT('Ctrl Pts',(0.0028594449326684,-0.0338644633294062,
0.0712713278741116));
#101173=CARTESIAN_POINT('Ctrl Pts',(0.00278773696925139,-0.034193496108874,
0.0715963036349737));
#101174=CARTESIAN_POINT('Ctrl Pts',(0.00282295092988617,-0.0340836138581107,
0.0715227227312173));
#101175=CARTESIAN_POINT('Ctrl Pts',(0.00285967059661017,-0.03397388966435,
0.0714499058119881));
#101176=CARTESIAN_POINT('Ctrl Pts',(0.00289784272535534,-0.0338644633294062,
0.0713779429235356));
#101177=CARTESIAN_POINT('Ctrl Pts',(0.00283050843261193,-0.034193496108874,
0.0717012405739843));
#101178=CARTESIAN_POINT('Ctrl Pts',(0.00286427537499894,-0.0340836138581107,
0.0716282494633793));
#101179=CARTESIAN_POINT('Ctrl Pts',(0.00289953651325002,-0.03397388966435,
0.0715559921113014));
#101180=CARTESIAN_POINT('Ctrl Pts',(0.00293624051804228,-0.0338644633294062,
0.0714845579729596));
#101181=CARTESIAN_POINT('Ctrl Pts',(0.00287327989597247,-0.034193496108874,
0.0718061775129949));
#101182=CARTESIAN_POINT('Ctrl Pts',(0.00290559982011171,-0.0340836138581107,
0.0717337761955414));
#101183=CARTESIAN_POINT('Ctrl Pts',(0.00293940242988986,-0.03397388966435,
0.0716620784106148));
#101184=CARTESIAN_POINT('Ctrl Pts',(0.00297463831072922,-0.0338644633294062,
0.0715911730223836));
#101185=CARTESIAN_POINT('Origin',(0.0183529366772285,-0.0345610621863404,
0.0781611633305691));
#101186=CARTESIAN_POINT('Ctrl Pts',(0.00285786328873317,-0.0342436276873901,
0.0718373774426975));
#101187=CARTESIAN_POINT('Ctrl Pts',(0.00294508528635293,-0.0339430054201862,
0.0716387700371384));
#101188=CARTESIAN_POINT('Ctrl Pts',(0.00304701941897627,-0.0336441434784164,
0.0714472967726391));
#101189=CARTESIAN_POINT('Ctrl Pts',(0.00276233686574636,-0.0342436276873901,
0.0720684070999092));
#101190=CARTESIAN_POINT('Ctrl Pts',(0.00284084543620189,-0.0339430054201862,
0.0718661968559136));
#101191=CARTESIAN_POINT('Ctrl Pts',(0.0029343622761473,-0.0336441434784164,
0.071670474657228));
#101192=CARTESIAN_POINT('Ctrl Pts',(0.00297462608320018,-0.0335235895815127,
0.0715911979124468));
#101193=CARTESIAN_POINT('Ctrl Pts',(0.00300985303175257,-0.0334144449262719,
0.0715203096408395));
#101194=CARTESIAN_POINT('Ctrl Pts',(0.00304658495014301,-0.0333049234473133,
0.0714500676894422));
#101195=CARTESIAN_POINT('Ctrl Pts',(0.00308478300561825,-0.0331951640388588,
0.0713805661307868));
#101196=CARTESIAN_POINT('Ctrl Pts',(0.00286645965177719,-0.0335235895815127,
0.0716249794991403));
#101197=CARTESIAN_POINT('Ctrl Pts',(0.00290122153027892,-0.0334144449262719,
0.0715526021036443));
#101198=CARTESIAN_POINT('Ctrl Pts',(0.00293751860848841,-0.0333049234473133,
0.0714808597095383));
#101199=CARTESIAN_POINT('Ctrl Pts',(0.00297531278347509,-0.0331951640388588,
0.0714098482575921));
#101200=CARTESIAN_POINT('Ctrl Pts',(0.00275829322035419,-0.0335235895815127,
0.0716587610858338));
#101201=CARTESIAN_POINT('Ctrl Pts',(0.00279259002880527,-0.0334144449262719,
0.0715848945664492));
#101202=CARTESIAN_POINT('Ctrl Pts',(0.00282845226683381,-0.0333049234473133,
0.0715116517296343));
#101203=CARTESIAN_POINT('Ctrl Pts',(0.00286584256133193,-0.0331951640388588,
0.0714391303843974));
#101204=CARTESIAN_POINT('Ctrl Pts',(0.00265012678893119,-0.0335235895815127,
0.0716925426725273));
#101205=CARTESIAN_POINT('Ctrl Pts',(0.00268395852733162,-0.0334144449262719,
0.071617187029254));
#101206=CARTESIAN_POINT('Ctrl Pts',(0.00271938592517922,-0.0333049234473133,
0.0715424437497303));
#101207=CARTESIAN_POINT('Ctrl Pts',(0.00275637233918876,-0.0331951640388588,
0.0714684125112027));
#101208=CARTESIAN_POINT('Origin',(0.017309347843454,-0.0326434571772312,
0.0800669115217672));
#101209=CARTESIAN_POINT('Ctrl Pts',(0.00292187045044344,-0.0336938721132379,
0.0711569522629806));
#101210=CARTESIAN_POINT('Ctrl Pts',(0.00293938975204655,-0.0336474569764953,
0.0711265037473738));
#101211=CARTESIAN_POINT('Ctrl Pts',(0.00295726429153528,-0.033601104548885,
0.0710962624036639));
#101212=CARTESIAN_POINT('Ctrl Pts',(0.00300251851395925,-0.0334837508643164,
0.0710196982776055));
#101213=CARTESIAN_POINT('Ctrl Pts',(0.00305002161776679,-0.033366026476041,
0.0709445087492458));
#101214=CARTESIAN_POINT('Ctrl Pts',(0.00303016432205854,-0.0336938721132379,
0.0714791982507639));
#101215=CARTESIAN_POINT('Ctrl Pts',(0.00304579741096262,-0.0336474569764953,
0.0714493836151234));
#101216=CARTESIAN_POINT('Ctrl Pts',(0.00306177844663147,-0.033601104548885,
0.0714197540274447));
#101217=CARTESIAN_POINT('Ctrl Pts',(0.00310223875293364,-0.0334837508643164,
0.0713447387269392));
#101218=CARTESIAN_POINT('Ctrl Pts',(0.00314490415084343,-0.033366026476041,
0.0712709552903345));
#101219=CARTESIAN_POINT('Ctrl Pts',(0.00303016432207031,-0.0336938721132426,
0.0714791982507706));
#101220=CARTESIAN_POINT('Ctrl Pts',(0.00304579741097352,-0.0336474569765026,
0.0714493836151318));
#101221=CARTESIAN_POINT('Ctrl Pts',(0.00306177844664147,-0.0336011045488949,
0.0714197540274547));
#101222=CARTESIAN_POINT('Ctrl Pts',(0.00310190177370088,-0.0334847282606778,
0.0713453635022282));
#101223=CARTESIAN_POINT('Ctrl Pts',(0.00314419376792775,-0.0333679869945434,
0.0712721841414624));
#101224=CARTESIAN_POINT('Ctrl Pts',(0.00303016432205703,-0.0336938721132424,
0.0714791982507669));
#101225=CARTESIAN_POINT('Ctrl Pts',(0.00308607516630843,-0.0335278710435082,
0.0713725679194267));
#101226=CARTESIAN_POINT('Ctrl Pts',(0.00314531024072201,-0.033362046922432,
0.0712677284499286));
#101227=CARTESIAN_POINT('Ctrl Pts',(0.00320791644279647,-0.0331951640388603,
0.0711646375555202));
#101228=CARTESIAN_POINT('Ctrl Pts',(0.00299285685570229,-0.0336938721132424,
0.0715542727656003));
#101229=CARTESIAN_POINT('Ctrl Pts',(0.00304719608217738,-0.0335278710435082,
0.0714468614358421));
#101230=CARTESIAN_POINT('Ctrl Pts',(0.00310488458361347,-0.033362046922432,
0.0713411919571547));
#101231=CARTESIAN_POINT('Ctrl Pts',(0.00316596862641463,-0.0331951640388603,
0.0712372213727529));
#101232=CARTESIAN_POINT('Ctrl Pts',(0.00295554938934755,-0.0336938721132424,
0.0716293472804336));
#101233=CARTESIAN_POINT('Ctrl Pts',(0.00300831699804633,-0.0335278710435082,
0.0715211549522575));
#101234=CARTESIAN_POINT('Ctrl Pts',(0.00306445892650492,-0.033362046922432,
0.0714146554643807));
#101235=CARTESIAN_POINT('Ctrl Pts',(0.00312402081003279,-0.0331951640388603,
0.0713098051899855));
#101236=CARTESIAN_POINT('Ctrl Pts',(0.00291824192299281,-0.0336938721132424,
0.071704421795267));
#101237=CARTESIAN_POINT('Ctrl Pts',(0.00296943791391528,-0.0335278710435082,
0.0715954484686729));
#101238=CARTESIAN_POINT('Ctrl Pts',(0.00302403326939637,-0.033362046922432,
0.0714881189716068));
#101239=CARTESIAN_POINT('Ctrl Pts',(0.00308207299365095,-0.0331951640388603,
0.0713823890072182));
#101240=CARTESIAN_POINT('Ctrl Pts',(0.00314545434883956,-0.0330240426238156,
0.0712729298487996));
#101241=CARTESIAN_POINT('Ctrl Pts',(0.00318508879316578,-0.0329142774063509,
0.0712043485325954));
#101242=CARTESIAN_POINT('Ctrl Pts',(0.00322616076408639,-0.0328043479726686,
0.0711365523807815));
#101243=CARTESIAN_POINT('Ctrl Pts',(0.00326862003723418,-0.0326943950436594,
0.0710696296943197));
#101244=CARTESIAN_POINT('Ctrl Pts',(0.00303538035654005,-0.0330240426238156,
0.07129985292819));
#101245=CARTESIAN_POINT('Ctrl Pts',(0.00307464390921778,-0.0329142774063509,
0.071229755235502));
#101246=CARTESIAN_POINT('Ctrl Pts',(0.00311537615132461,-0.0328043479726686,
0.0711604342838688));
#101247=CARTESIAN_POINT('Ctrl Pts',(0.00315752734750701,-0.0326943950436594,
0.0710919803156488));
#101248=CARTESIAN_POINT('Ctrl Pts',(0.00292530636424054,-0.0330240426238156,
0.0713267760075804));
#101249=CARTESIAN_POINT('Ctrl Pts',(0.00296419902526979,-0.0329142774063509,
0.0712551619384086));
#101250=CARTESIAN_POINT('Ctrl Pts',(0.00300459153856282,-0.0328043479726686,
0.0711843161869562));
#101251=CARTESIAN_POINT('Ctrl Pts',(0.00304643465777984,-0.0326943950436594,
0.0711143309369779));
#101252=CARTESIAN_POINT('Ctrl Pts',(0.00281523237194103,-0.0330240426238156,
0.0713536990869708));
#101253=CARTESIAN_POINT('Ctrl Pts',(0.00285375414132179,-0.0329142774063509,
0.0712805686413151));
#101254=CARTESIAN_POINT('Ctrl Pts',(0.00289380692580104,-0.0328043479726686,
0.0712081980900436));
#101255=CARTESIAN_POINT('Ctrl Pts',(0.00293534196805267,-0.0326943950436594,
0.071136681558307));
#101256=CARTESIAN_POINT('Origin',(0.0174147894217676,-0.0326396682856539,
0.0801315448900268));
#101257=CARTESIAN_POINT('Ctrl Pts',(0.00312059419090093,-0.0331951640388587,
0.0708381863255022));
#101258=CARTESIAN_POINT('Ctrl Pts',(0.00316620772452263,-0.0330855618255041,
0.0707692775321387));
#101259=CARTESIAN_POINT('Ctrl Pts',(0.00321327836727237,-0.0329757224427708,
0.0707012618171597));
#101260=CARTESIAN_POINT('Ctrl Pts',(0.00326175011471513,-0.0328657862078596,
0.0706342292354737));
#101261=CARTESIAN_POINT('Ctrl Pts',(0.00314987629439357,-0.0331951640388587,
0.0709476564604918));
#101262=CARTESIAN_POINT('Ctrl Pts',(0.00319398209836207,-0.0330855618255041,
0.0708791509688667));
#101263=CARTESIAN_POINT('Ctrl Pts',(0.00323953558899983,-0.0329757224427708,
0.0708115076841659));
#101264=CARTESIAN_POINT('Ctrl Pts',(0.00328648268128231,-0.0328657862078596,
0.0707448160890802));
#101265=CARTESIAN_POINT('Ctrl Pts',(0.00317915839788622,-0.0331951640388588,
0.0710571265954814));
#101266=CARTESIAN_POINT('Ctrl Pts',(0.00322175647220151,-0.0330855618255041,
0.0709890244055947));
#101267=CARTESIAN_POINT('Ctrl Pts',(0.0032657928107273,-0.0329757224427708,
0.0709217535511722));
#101268=CARTESIAN_POINT('Ctrl Pts',(0.00331121524784949,-0.0328657862078596,
0.0708554029426867));
#101269=CARTESIAN_POINT('Ctrl Pts',(0.00320844050137886,-0.0331951640388588,
0.071166596730471));
#101270=CARTESIAN_POINT('Ctrl Pts',(0.00324953084604096,-0.0330855618255041,
0.0710988978423227));
#101271=CARTESIAN_POINT('Ctrl Pts',(0.00329205003245476,-0.0329757224427708,
0.0710319994181785));
#101272=CARTESIAN_POINT('Ctrl Pts',(0.00333594781441668,-0.0328657862078596,
0.0709659897962932));
#101273=CARTESIAN_POINT('Origin',(0.0171228894063379,-0.0326401908830065,
0.0805137323480971));
#101274=CARTESIAN_POINT('Ctrl Pts',(0.0031892723219281,-0.0332451089994434,
0.0711955563415044));
#101275=CARTESIAN_POINT('Ctrl Pts',(0.00330070098757655,-0.0329451141710259,
0.0710094482568253));
#101276=CARTESIAN_POINT('Ctrl Pts',(0.00342583151789996,-0.0326442513127504,
0.0708322621481936));
#101277=CARTESIAN_POINT('Ctrl Pts',(0.00306554072209852,-0.0332451089994434,
0.0714127900663346));
#101278=CARTESIAN_POINT('Ctrl Pts',(0.00316877628376881,-0.0329451141710259,
0.0712220153680182));
#101279=CARTESIAN_POINT('Ctrl Pts',(0.00328608849427418,-0.0326442513127504,
0.0710395587650206));
#101280=CARTESIAN_POINT('Ctrl Pts',(0.00333593024811363,-0.0325229783203385,
0.0709660160490157));
#101281=CARTESIAN_POINT('Ctrl Pts',(0.00337982139644991,-0.032413025311208,
0.0709000156158587));
#101282=CARTESIAN_POINT('Ctrl Pts',(0.00342507119155223,-0.0323031222247695,
0.0708349331377294));
#101283=CARTESIAN_POINT('Ctrl Pts',(0.00347161872993966,-0.0321934096636184,
0.0707708499353724));
#101284=CARTESIAN_POINT('Ctrl Pts',(0.00322438292180028,-0.0325229783203385,
0.0709859744217387));
#101285=CARTESIAN_POINT('Ctrl Pts',(0.00326799894441005,-0.032413025311208,
0.0709184363111559));
#101286=CARTESIAN_POINT('Ctrl Pts',(0.00331300546434632,-0.0323031222247695,
0.0708518106974906));
#101287=CARTESIAN_POINT('Ctrl Pts',(0.00335934181999699,-0.0321934096636184,
0.0707861808891304));
#101288=CARTESIAN_POINT('Ctrl Pts',(0.00311283559548694,-0.0325229783203385,
0.0710059327944618));
#101289=CARTESIAN_POINT('Ctrl Pts',(0.00315617649237019,-0.032413025311208,
0.0709368570064531));
#101290=CARTESIAN_POINT('Ctrl Pts',(0.0032009397371404,-0.0323031222247695,
0.0708686882572519));
#101291=CARTESIAN_POINT('Ctrl Pts',(0.00324706491005432,-0.0321934096636184,
0.0708015118428885));
#101292=CARTESIAN_POINT('Ctrl Pts',(0.00300128826917359,-0.0325229783203385,
0.0710258911671848));
#101293=CARTESIAN_POINT('Ctrl Pts',(0.00304435404033032,-0.032413025311208,
0.0709552777017503));
#101294=CARTESIAN_POINT('Ctrl Pts',(0.00308887400993449,-0.0323031222247695,
0.0708855658170131));
#101295=CARTESIAN_POINT('Ctrl Pts',(0.00313478800011164,-0.0321934096636184,
0.0708168427966465));
#101296=CARTESIAN_POINT('Origin',(0.0174077525540327,-0.0326393375176799,
0.0801267310016776));
#101297=CARTESIAN_POINT('Ctrl Pts',(0.00333841734075972,-0.0326943950436593,
0.0705305686593156));
#101298=CARTESIAN_POINT('Ctrl Pts',(0.0033882998881715,-0.0325844576448126,
0.0704646173629209));
#101299=CARTESIAN_POINT('Ctrl Pts',(0.00343954994678673,-0.0324744968375318,
0.0703996930519144));
#101300=CARTESIAN_POINT('Ctrl Pts',(0.0034921007046729,-0.0323646534831894,
0.070335878005398));
#101301=CARTESIAN_POINT('Ctrl Pts',(0.00336076795477588,-0.0326943950436593,
0.0706416613126942));
#101302=CARTESIAN_POINT('Ctrl Pts',(0.00340911943721428,-0.0325844576448126,
0.0705760180496501));
#101303=CARTESIAN_POINT('Ctrl Pts',(0.00345883195186557,-0.0324744968375318,
0.0705113701288604));
#101304=CARTESIAN_POINT('Ctrl Pts',(0.0035098406616727,-0.0323646534831894,
0.0704477995024718));
#101305=CARTESIAN_POINT('Ctrl Pts',(0.00338311856879204,-0.0326943950436593,
0.0707527539660728));
#101306=CARTESIAN_POINT('Ctrl Pts',(0.00342993898625707,-0.0325844576448126,
0.0706874187363793));
#101307=CARTESIAN_POINT('Ctrl Pts',(0.00347811395694441,-0.0324744968375318,
0.0706230472058065));
#101308=CARTESIAN_POINT('Ctrl Pts',(0.00352758061867251,-0.0323646534831894,
0.0705597209995456));
#101309=CARTESIAN_POINT('Ctrl Pts',(0.0034054691828082,-0.0326943950436593,
0.0708638466194514));
#101310=CARTESIAN_POINT('Ctrl Pts',(0.00345075853529985,-0.0325844576448126,
0.0707988194231086));
#101311=CARTESIAN_POINT('Ctrl Pts',(0.00349739596202326,-0.0324744968375318,
0.0707347242827525));
#101312=CARTESIAN_POINT('Ctrl Pts',(0.00354532057567232,-0.0323646534831894,
0.0706716424966194));
#101313=CARTESIAN_POINT('Origin',(0.0171540481476118,-0.0326395579068999,
0.0805352054641116));
#101314=CARTESIAN_POINT('Ctrl Pts',(0.00338449828019584,-0.0327445246961878,
0.0708915781438235));
#101315=CARTESIAN_POINT('Ctrl Pts',(0.00350739166825613,-0.0324436878365476,
0.0707128331308248));
#101316=CARTESIAN_POINT('Ctrl Pts',(0.0036433997339666,-0.0321434074463187,
0.0705438527456834));
#101317=CARTESIAN_POINT('Ctrl Pts',(0.00324737204356741,-0.0327445246961878,
0.0711006149712681));
#101318=CARTESIAN_POINT('Ctrl Pts',(0.00336238147887758,-0.0324436878365476,
0.0709166981577614));
#101319=CARTESIAN_POINT('Ctrl Pts',(0.0034909175504622,-0.0321434074463187,
0.0707419668131136));
#101320=CARTESIAN_POINT('Ctrl Pts',(0.00360190210950176,-0.0322357242816073,
0.0705960267995549));
#101321=CARTESIAN_POINT('Ctrl Pts',(0.00371509154660157,-0.0319819883628706,
0.0704520107835557));
#101322=CARTESIAN_POINT('Ctrl Pts',(0.0038372157423532,-0.0317295851069886,
0.070315489201572));
#101323=CARTESIAN_POINT('Ctrl Pts',(0.00345172649576831,-0.0322357242816073,
0.0707958949687059));
#101324=CARTESIAN_POINT('Ctrl Pts',(0.00355855039090018,-0.0319819883628706,
0.0706470960541798));
#101325=CARTESIAN_POINT('Ctrl Pts',(0.00367462629476046,-0.0317295851069886,
0.0705053962091613));
#101326=CARTESIAN_POINT('Origin',(0.0170772303833248,-0.0326371942646307,
0.0804788012569333));
#101327=CARTESIAN_POINT('Origin',(0.0173061599489961,-0.0326352985530895,
0.0800578634077293));
#101328=CARTESIAN_POINT('Ctrl Pts',(0.00357512613946539,-0.0321934096636183,
0.0702372352350691));
#101329=CARTESIAN_POINT('Ctrl Pts',(0.00362908621499712,-0.0320835708272304,
0.0701745057230825));
#101330=CARTESIAN_POINT('Ctrl Pts',(0.00368431317548228,-0.0319739230346346,
0.0701129292977206));
#101331=CARTESIAN_POINT('Ctrl Pts',(0.00374073031549945,-0.0318646057455575,
0.070052579318862));
#101332=CARTESIAN_POINT('Ctrl Pts',(0.00359045710642513,-0.0321934096636183,
0.0703495122416948));
#101333=CARTESIAN_POINT('Ctrl Pts',(0.00364286879453211,-0.0320835708272304,
0.0702869941556908));
#101334=CARTESIAN_POINT('Ctrl Pts',(0.00369654389027044,-0.0319739230346346,
0.0702255969898787));
#101335=CARTESIAN_POINT('Ctrl Pts',(0.00375140769132395,-0.0318646057455575,
0.0701653940271684));
#101336=CARTESIAN_POINT('Ctrl Pts',(0.00360578807338487,-0.0321934096636183,
0.0704617892483205));
#101337=CARTESIAN_POINT('Ctrl Pts',(0.00365665137406711,-0.0320835708272304,
0.0703994825882991));
#101338=CARTESIAN_POINT('Ctrl Pts',(0.00370877460505861,-0.0319739230346346,
0.0703382646820367));
#101339=CARTESIAN_POINT('Ctrl Pts',(0.00376208506714845,-0.0318646057455575,
0.0702782087354748));
#101340=CARTESIAN_POINT('Ctrl Pts',(0.00362111904034461,-0.0321934096636183,
0.0705740662549463));
#101341=CARTESIAN_POINT('Ctrl Pts',(0.00367043395360211,-0.0320835708272304,
0.0705119710209075));
#101342=CARTESIAN_POINT('Ctrl Pts',(0.00372100531984677,-0.0319739230346346,
0.0704509323741947));
#101343=CARTESIAN_POINT('Ctrl Pts',(0.00377276244297296,-0.0318646057455575,
0.0703910234437812));
#101344=CARTESIAN_POINT('Ctrl Pts',(0.00354437754856675,-0.0320218834582388,
0.0706715160052204));
#101345=CARTESIAN_POINT('Ctrl Pts',(0.00358058015777147,-0.031939109935068,
0.0706238554735102));
#101346=CARTESIAN_POINT('Ctrl Pts',(0.00361750505862053,-0.0318564869454956,
0.0705767891269242));
#101347=CARTESIAN_POINT('Ctrl Pts',(0.00365512215579729,-0.0317740741446545,
0.070530348736228));
#101348=CARTESIAN_POINT('Ctrl Pts',(0.00349513376256958,-0.0320218834582388,
0.0706771620292948));
#101349=CARTESIAN_POINT('Ctrl Pts',(0.00353127761031287,-0.031939109935068,
0.0706289889888185));
#101350=CARTESIAN_POINT('Ctrl Pts',(0.00356815178819881,-0.0318564869454956,
0.0705814095264139));
#101351=CARTESIAN_POINT('Ctrl Pts',(0.0036057262029648,-0.0317740741446545,
0.0705344557900326));
#101352=CARTESIAN_POINT('Ctrl Pts',(0.00344588997657241,-0.0320218834582388,
0.0706828080533692));
#101353=CARTESIAN_POINT('Ctrl Pts',(0.00348197506285426,-0.031939109935068,
0.0706341225041267));
#101354=CARTESIAN_POINT('Ctrl Pts',(0.00351879851777708,-0.0318564869454956,
0.0705860299259036));
#101355=CARTESIAN_POINT('Ctrl Pts',(0.0035563302501323,-0.0317740741446545,
0.0705385628438372));
#101356=CARTESIAN_POINT('Ctrl Pts',(0.00339664619057525,-0.0320218834582388,
0.0706884540774437));
#101357=CARTESIAN_POINT('Ctrl Pts',(0.00343267251539565,-0.031939109935068,
0.070639256019435));
#101358=CARTESIAN_POINT('Ctrl Pts',(0.00346944524735535,-0.0318564869454956,
0.0705906503253933));
#101359=CARTESIAN_POINT('Ctrl Pts',(0.00350693429729981,-0.0317740741446545,
0.0705426698976418));
#101360=CARTESIAN_POINT('Origin',(-0.00203465492131801,-0.0391228853390622,
0.067616488408112));
#101361=CARTESIAN_POINT('Ctrl Pts',(0.00241022601210972,-0.0352722978779625,
0.0734870970590132));
#101362=CARTESIAN_POINT('Ctrl Pts',(0.00241275129914135,-0.0352466642097238,
0.0734683696565378));
#101363=CARTESIAN_POINT('Ctrl Pts',(0.00241519663864789,-0.0352210183808312,
0.0734496484609053));
#101364=CARTESIAN_POINT('Ctrl Pts',(0.00241756158888749,-0.0351953608940153,
0.0734309327424934));
#101365=CARTESIAN_POINT('Origin',(-0.00241827000673056,-0.0352456003065117,
0.072653208942305));
#101366=CARTESIAN_POINT('Ctrl Pts',(0.002435929945587,-0.035024121149334,
0.0733076123512748));
#101367=CARTESIAN_POINT('Ctrl Pts',(0.00244753348953259,-0.0349144232867422,
0.0732292645222082));
#101368=CARTESIAN_POINT('Ctrl Pts',(0.00246076348429631,-0.0348045283677513,
0.0731511096517255));
#101369=CARTESIAN_POINT('Ctrl Pts',(0.00247560670913094,-0.0346945769586887,
0.0730732484768736));
#101370=CARTESIAN_POINT('Ctrl Pts',(0.00234349675984053,-0.035024121149334,
0.0733731657491714));
#101371=CARTESIAN_POINT('Ctrl Pts',(0.00235419733264876,-0.0349144232867422,
0.0732935446909276));
#101372=CARTESIAN_POINT('Ctrl Pts',(0.00236655013435908,-0.0348045283677513,
0.0732140971641209));
#101373=CARTESIAN_POINT('Ctrl Pts',(0.00238054312941053,-0.0346945769586887,
0.0731349255197159));
#101374=CARTESIAN_POINT('Ctrl Pts',(0.00225106357409406,-0.035024121149334,
0.073438719147068));
#101375=CARTESIAN_POINT('Ctrl Pts',(0.00226086117576492,-0.0349144232867422,
0.073357824859647));
#101376=CARTESIAN_POINT('Ctrl Pts',(0.00227233678442185,-0.0348045283677513,
0.0732770846765164));
#101377=CARTESIAN_POINT('Ctrl Pts',(0.00228547954969013,-0.0346945769586887,
0.0731966025625582));
#101378=CARTESIAN_POINT('Ctrl Pts',(0.0021586303883476,-0.035024121149334,
0.0735042725449646));
#101379=CARTESIAN_POINT('Ctrl Pts',(0.00216752501888108,-0.0349144232867422,
0.0734221050283664));
#101380=CARTESIAN_POINT('Ctrl Pts',(0.00217812343448462,-0.0348045283677513,
0.0733400721889119));
#101381=CARTESIAN_POINT('Ctrl Pts',(0.00219041596996972,-0.0346945769586887,
0.0732582796054005));
#101382=CARTESIAN_POINT('Origin',(0.0189327085722657,-0.0345629067940946,
0.0763939031326696));
#101383=CARTESIAN_POINT('Ctrl Pts',(0.00230774228889657,-0.0351970973651633,
0.0729884486193835));
#101384=CARTESIAN_POINT('Ctrl Pts',(0.00232383400909443,-0.0350869349321776,
0.072907875268639));
#101385=CARTESIAN_POINT('Ctrl Pts',(0.00234161413479677,-0.0349764985129712,
0.0728275697098138));
#101386=CARTESIAN_POINT('Ctrl Pts',(0.00236106575562629,-0.0348659306849618,
0.0727476373370736));
#101387=CARTESIAN_POINT('Ctrl Pts',(0.00235675309102232,-0.0351970973651633,
0.0730544668890143));
#101388=CARTESIAN_POINT('Ctrl Pts',(0.00237193021756503,-0.0350869349321776,
0.0729745725165119));
#101389=CARTESIAN_POINT('Ctrl Pts',(0.00238878087639209,-0.0349764985129712,
0.0728949274844911));
#101390=CARTESIAN_POINT('Ctrl Pts',(0.00240728931090446,-0.0348659306849618,
0.0728156362605026));
#101391=CARTESIAN_POINT('Ctrl Pts',(0.00240576389314807,-0.0351970973651633,
0.0731204851586451));
#101392=CARTESIAN_POINT('Ctrl Pts',(0.00242002642603563,-0.0350869349321776,
0.0730412697643848));
#101393=CARTESIAN_POINT('Ctrl Pts',(0.00243594761798742,-0.0349764985129712,
0.0729622852591685));
#101394=CARTESIAN_POINT('Ctrl Pts',(0.00245351286618263,-0.0348659306849618,
0.0728836351839316));
#101395=CARTESIAN_POINT('Ctrl Pts',(0.00245477469527383,-0.0351970973651633,
0.0731865034282759));
#101396=CARTESIAN_POINT('Ctrl Pts',(0.00246812263450623,-0.0350869349321776,
0.0731079670122576));
#101397=CARTESIAN_POINT('Ctrl Pts',(0.00248311435958274,-0.0349764985129712,
0.0730296430338458));
#101398=CARTESIAN_POINT('Ctrl Pts',(0.0024997364214608,-0.0348659306849618,
0.0729516341073605));
#101399=CARTESIAN_POINT('Origin',(0.0187908648875428,-0.0345637187965049,
0.0768534743735188));
#101400=CARTESIAN_POINT('Ctrl Pts',(0.00244818867122777,-0.0352450361861252,
0.0732195360434774));
#101401=CARTESIAN_POINT('Ctrl Pts',(0.00248328169429483,-0.0349452761023764,
0.0730054775267704));
#101402=CARTESIAN_POINT('Ctrl Pts',(0.00253439878470322,-0.0346444289983475,
0.0727946704777635));
#101403=CARTESIAN_POINT('Ctrl Pts',(0.00241311474729942,-0.0352450361861252,
0.0734670634558184));
#101404=CARTESIAN_POINT('Ctrl Pts',(0.00243887212105936,-0.0349452761023764,
0.0732516821043978));
#101405=CARTESIAN_POINT('Ctrl Pts',(0.00248077972507688,-0.0346444289983475,
0.0730388527794252));
#101406=CARTESIAN_POINT('Ctrl Pts',(0.00250004732525913,-0.0345231616327821,
0.0729521323532325));
#101407=CARTESIAN_POINT('Ctrl Pts',(0.00251655824430696,-0.0344132092796975,
0.072874617085665));
#101408=CARTESIAN_POINT('Ctrl Pts',(0.0025346716536337,-0.0343032738558973,
0.0727974473328659));
#101409=CARTESIAN_POINT('Ctrl Pts',(0.0025543618154463,-0.0341934961088741,
0.0727207213637928));
#101410=CARTESIAN_POINT('Ctrl Pts',(0.00240368043418143,-0.0345231616327821,
0.0730117524709993));
#101411=CARTESIAN_POINT('Ctrl Pts',(0.00241936957384426,-0.0344132092796975,
0.072932908921512));
#101412=CARTESIAN_POINT('Ctrl Pts',(0.00243668872064982,-0.0343032738558973,
0.0728543939574681));
#101413=CARTESIAN_POINT('Ctrl Pts',(0.00245561311020234,-0.0341934961088741,
0.0727763075972607));
#101414=CARTESIAN_POINT('Ctrl Pts',(0.00230731354310373,-0.0345231616327821,
0.073071372588766));
#101415=CARTESIAN_POINT('Ctrl Pts',(0.00232218090338157,-0.0344132092796975,
0.072991200757359));
#101416=CARTESIAN_POINT('Ctrl Pts',(0.00233870578766594,-0.0343032738558973,
0.0729113405820702));
#101417=CARTESIAN_POINT('Ctrl Pts',(0.00235686440495838,-0.0341934961088741,
0.0728318938307285));
#101418=CARTESIAN_POINT('Ctrl Pts',(0.00221094665202603,-0.0345231616327821,
0.0731309927065328));
#101419=CARTESIAN_POINT('Ctrl Pts',(0.00222499223291887,-0.0344132092796975,
0.073049492593206));
#101420=CARTESIAN_POINT('Ctrl Pts',(0.00224072285468207,-0.0343032738558973,
0.0729682872066723));
#101421=CARTESIAN_POINT('Ctrl Pts',(0.00225811569971443,-0.0341934961088741,
0.0728874800641964));
#101422=CARTESIAN_POINT('Origin',(0.0189446079269458,-0.0345625596231005,
0.0763961175525524));
#101423=CARTESIAN_POINT('Ctrl Pts',(0.0023420609337359,-0.0346945769586885,
0.0725463481428481));
#101424=CARTESIAN_POINT('Ctrl Pts',(0.00236416006689013,-0.0345846629176052,
0.0724666731015343));
#101425=CARTESIAN_POINT('Ctrl Pts',(0.00238791062176432,-0.0344746925050311,
0.0723874414525256));
#101426=CARTESIAN_POINT('Ctrl Pts',(0.00241328174714459,-0.0343648066253259,
0.0723087545908615));
#101427=CARTESIAN_POINT('Ctrl Pts',(0.00240373792801572,-0.0346945769586885,
0.0726414116477186));
#101428=CARTESIAN_POINT('Ctrl Pts',(0.00242452703802318,-0.0345846629176052,
0.0725625865465605));
#101429=CARTESIAN_POINT('Ctrl Pts',(0.00244694976958205,-0.0344746925050311,
0.0724841778921387));
#101430=CARTESIAN_POINT('Ctrl Pts',(0.0024709769771937,-0.0343648066253259,
0.0724062860320035));
#101431=CARTESIAN_POINT('Ctrl Pts',(0.00246541492229555,-0.0346945769586885,
0.0727364751525891));
#101432=CARTESIAN_POINT('Ctrl Pts',(0.00248489400915623,-0.0345846629176052,
0.0726584999915867));
#101433=CARTESIAN_POINT('Ctrl Pts',(0.00250598891739978,-0.0344746925050311,
0.0725809143317517));
#101434=CARTESIAN_POINT('Ctrl Pts',(0.00252867220724281,-0.0343648066253259,
0.0725038174731455));
#101435=CARTESIAN_POINT('Ctrl Pts',(0.00252709191657538,-0.0346945769586885,
0.0728315386574596));
#101436=CARTESIAN_POINT('Ctrl Pts',(0.00254526098028928,-0.0345846629176052,
0.0727544134366129));
#101437=CARTESIAN_POINT('Ctrl Pts',(0.00256502806521751,-0.0344746925050311,
0.0726776507713648));
#101438=CARTESIAN_POINT('Ctrl Pts',(0.00258636743729192,-0.0343648066253259,
0.0726013489142874));
#101439=CARTESIAN_POINT('Origin',(0.0188476909451964,-0.0345626446731571,
0.0768670732632059));
#101440=CARTESIAN_POINT('Ctrl Pts',(0.00252598830832928,-0.0346945769586886,
0.0728298376525857));
#101441=CARTESIAN_POINT('Ctrl Pts',(0.00255363963725959,-0.0345275153362891,
0.0727125896184365));
#101442=CARTESIAN_POINT('Ctrl Pts',(0.00258498546099442,-0.0343603235965159,
0.0725961808667837));
#101443=CARTESIAN_POINT('Ctrl Pts',(0.00261992795552367,-0.0341934961088741,
0.0724809543051727));
#101444=CARTESIAN_POINT('Ctrl Pts',(0.00250852319911034,-0.0346945769586886,
0.0729118315443779));
#101445=CARTESIAN_POINT('Ctrl Pts',(0.00253445713314853,-0.0345275153362891,
0.0727942176965235));
#101446=CARTESIAN_POINT('Ctrl Pts',(0.00256409662228927,-0.0343603235965159,
0.0726773890260587));
#101447=CARTESIAN_POINT('Ctrl Pts',(0.00259734887064439,-0.0341934961088741,
0.0725616897574677));
#101448=CARTESIAN_POINT('Ctrl Pts',(0.0024910580898914,-0.0346945769586886,
0.0729938254361702));
#101449=CARTESIAN_POINT('Ctrl Pts',(0.00251527462903747,-0.0345275153362891,
0.0728758457746105));
#101450=CARTESIAN_POINT('Ctrl Pts',(0.00254320778358412,-0.0343603235965159,
0.0727585971853337));
#101451=CARTESIAN_POINT('Ctrl Pts',(0.0025747697857651,-0.0341934961088741,
0.0726424252097627));
#101452=CARTESIAN_POINT('Ctrl Pts',(0.00247359298067246,-0.0346945769586886,
0.0730758193279624));
#101453=CARTESIAN_POINT('Ctrl Pts',(0.0024960921249264,-0.0345275153362891,
0.0729574738526975));
#101454=CARTESIAN_POINT('Ctrl Pts',(0.00252231894487896,-0.0343603235965159,
0.0728398053446087));
#101455=CARTESIAN_POINT('Ctrl Pts',(0.00255219070088582,-0.0341934961088741,
0.0727231606620577));
#101456=CARTESIAN_POINT('Ctrl Pts',(0.00258635947489357,-0.0340223579322365,
0.0726013794525524));
#101457=CARTESIAN_POINT('Ctrl Pts',(0.00260771899121465,-0.0339125849573551,
0.0725250039510641));
#101458=CARTESIAN_POINT('Ctrl Pts',(0.00263064429385958,-0.0338030433565216,
0.0724491242101115));
#101459=CARTESIAN_POINT('Ctrl Pts',(0.00265509746327339,-0.033693872113232,
0.0723738346682113));
#101460=CARTESIAN_POINT('Ctrl Pts',(0.00248643900227624,-0.0340223579322365,
0.0726548311034371));
#101461=CARTESIAN_POINT('Ctrl Pts',(0.00250706128092387,-0.0339125849573551,
0.0725770774380279));
#101462=CARTESIAN_POINT('Ctrl Pts',(0.00252927838873448,-0.0338030433565216,
0.0724998052424675));
#101463=CARTESIAN_POINT('Ctrl Pts',(0.00255305315396205,-0.033693872113232,
0.0724231108162704));
#101464=CARTESIAN_POINT('Ctrl Pts',(0.00238651852965892,-0.0340223579322365,
0.0727082827543218));
#101465=CARTESIAN_POINT('Ctrl Pts',(0.0024064035706331,-0.0339125849573551,
0.0726291509249917));
#101466=CARTESIAN_POINT('Ctrl Pts',(0.00242791248360938,-0.0338030433565216,
0.0725504862748235));
#101467=CARTESIAN_POINT('Ctrl Pts',(0.0024510088446507,-0.033693872113232,
0.0724723869643295));
#101468=CARTESIAN_POINT('Ctrl Pts',(0.00228659805704159,-0.0340223579322365,
0.0727617344052066));
#101469=CARTESIAN_POINT('Ctrl Pts',(0.00230574586034232,-0.0339125849573551,
0.0726812244119555));
#101470=CARTESIAN_POINT('Ctrl Pts',(0.00232654657848428,-0.0338030433565216,
0.0726011673071795));
#101471=CARTESIAN_POINT('Ctrl Pts',(0.00234896453533936,-0.033693872113232,
0.0725216631123886));
#101472=CARTESIAN_POINT('Origin',(0.0188274512928389,-0.0345589643414767,
0.0763691508835896));
#101473=CARTESIAN_POINT('Ctrl Pts',(0.0024541639731875,-0.034193496108874,
0.0721864753018193));
#101474=CARTESIAN_POINT('Ctrl Pts',(0.00248123981602225,-0.0340836138581107,
0.0721082946239812));
#101475=CARTESIAN_POINT('Ctrl Pts',(0.00250992045244113,-0.0339738896643499,
0.0720307117364567));
#101476=CARTESIAN_POINT('Ctrl Pts',(0.00254016251843922,-0.0338644633294062,
0.0719538234750659));
#101477=CARTESIAN_POINT('Ctrl Pts',(0.00250975025667077,-0.034193496108874,
0.0722852240959154));
#101478=CARTESIAN_POINT('Ctrl Pts',(0.00253546441211166,-0.0340836138581107,
0.0722078099200096));
#101479=CARTESIAN_POINT('Ctrl Pts',(0.00256276815335073,-0.0339738896643499,
0.072130964989372));
#101480=CARTESIAN_POINT('Ctrl Pts',(0.0025916199419529,-0.0338644633294062,
0.0720547853134616));
#101481=CARTESIAN_POINT('Ctrl Pts',(0.00256533654015405,-0.034193496108874,
0.0723839728900115));
#101482=CARTESIAN_POINT('Ctrl Pts',(0.00258968900820107,-0.0340836138581107,
0.0723073252160381));
#101483=CARTESIAN_POINT('Ctrl Pts',(0.00261561585426032,-0.0339738896643499,
0.0722312182422874));
#101484=CARTESIAN_POINT('Ctrl Pts',(0.00264307736546658,-0.0338644633294062,
0.0721557471518574));
#101485=CARTESIAN_POINT('Ctrl Pts',(0.00262092282363733,-0.034193496108874,
0.0724827216841076));
#101486=CARTESIAN_POINT('Ctrl Pts',(0.00264391360429047,-0.0340836138581107,
0.0724068405120665));
#101487=CARTESIAN_POINT('Ctrl Pts',(0.00266846355516991,-0.03397388966435,
0.0723314714952027));
#101488=CARTESIAN_POINT('Ctrl Pts',(0.00269453478898026,-0.0338644633294063,
0.0722567089902531));
#101489=CARTESIAN_POINT('Origin',(0.0187750088091898,-0.0345610621861796,
0.076847481101678));
#101490=CARTESIAN_POINT('Ctrl Pts',(0.00260953816902741,-0.0342436276873901,
0.0725156078062815));
#101491=CARTESIAN_POINT('Ctrl Pts',(0.00267118028679546,-0.0339430054201861,
0.0723076346644367));
#101492=CARTESIAN_POINT('Ctrl Pts',(0.00274831267495602,-0.0336441434784164,
0.072104895489366));
#101493=CARTESIAN_POINT('Ctrl Pts',(0.0025437206944058,-0.0342436276873901,
0.0727567883611246));
#101494=CARTESIAN_POINT('Ctrl Pts',(0.00259626653759414,-0.0339430054201861,
0.0725463328723026));
#101495=CARTESIAN_POINT('Ctrl Pts',(0.00266451547328288,-0.0336441434784164,
0.0723404332336699));
#101496=CARTESIAN_POINT('Ctrl Pts',(0.00269452577742099,-0.0335235895815127,
0.0722567352165666));
#101497=CARTESIAN_POINT('Ctrl Pts',(0.00272059029465993,-0.0334144449262719,
0.0721819908127834));
#101498=CARTESIAN_POINT('Ctrl Pts',(0.00274822892000209,-0.0333049234473133,
0.0721076990100463));
#101499=CARTESIAN_POINT('Ctrl Pts',(0.00277741491731665,-0.0331951640388588,
0.0720339580061314));
#101500=CARTESIAN_POINT('Ctrl Pts',(0.00259144622611276,-0.0335235895815127,
0.0723038072739723));
#101501=CARTESIAN_POINT('Ctrl Pts',(0.00261686270380516,-0.0334144449262719,
0.0722276437772204));
#101502=CARTESIAN_POINT('Ctrl Pts',(0.0026438818624746,-0.0333049234473133,
0.0721519178631394));
#101503=CARTESIAN_POINT('Ctrl Pts',(0.00267247792421042,-0.0331951640388588,
0.0720767294915409));
#101504=CARTESIAN_POINT('Ctrl Pts',(0.00248836667480452,-0.0335235895815127,
0.072350879331378));
#101505=CARTESIAN_POINT('Ctrl Pts',(0.00251313511295039,-0.0334144449262719,
0.0722732967416574));
#101506=CARTESIAN_POINT('Ctrl Pts',(0.00253953480494712,-0.0333049234473133,
0.0721961367162324));
#101507=CARTESIAN_POINT('Ctrl Pts',(0.00256754093110419,-0.0331951640388588,
0.0721195009769504));
#101508=CARTESIAN_POINT('Ctrl Pts',(0.00238528712349628,-0.0335235895815127,
0.0723979513887837));
#101509=CARTESIAN_POINT('Ctrl Pts',(0.00240940752209562,-0.0334144449262719,
0.0723189497060944));
#101510=CARTESIAN_POINT('Ctrl Pts',(0.00243518774741963,-0.0333049234473133,
0.0722403555693255));
#101511=CARTESIAN_POINT('Ctrl Pts',(0.00246260393799796,-0.0331951640388588,
0.0721622724623599));
#101512=CARTESIAN_POINT('Origin',(0.0179785025681745,-0.0326434571770922,
0.0788689982621595));
#101513=CARTESIAN_POINT('Ctrl Pts',(0.00258776072717685,-0.0336938721132386,
0.0718325257577917));
#101514=CARTESIAN_POINT('Ctrl Pts',(0.00260132567293593,-0.0336474569764956,
0.0718001215871051));
#101515=CARTESIAN_POINT('Ctrl Pts',(0.00261526902094752,-0.033601104548885,
0.0717678784315901));
#101516=CARTESIAN_POINT('Ctrl Pts',(0.00265057036926952,-0.0334837508694606,
0.0716862461820837));
#101517=CARTESIAN_POINT('Ctrl Pts',(0.00268827514843814,-0.0333660264863597,
0.0716056958314907));
#101518=CARTESIAN_POINT('Ctrl Pts',(0.00273558880092054,-0.0336938721132386,
0.0721386579186066));
#101519=CARTESIAN_POINT('Ctrl Pts',(0.00274736185355695,-0.0336474569764956,
0.0721071190346901));
#101520=CARTESIAN_POINT('Ctrl Pts',(0.00275950330195339,-0.033601104548885,
0.0720757201302838));
#101521=CARTESIAN_POINT('Ctrl Pts',(0.00279024265512883,-0.0334837508694606,
0.0719962253302936));
#101522=CARTESIAN_POINT('Ctrl Pts',(0.00282332410538725,-0.0333660264863597,
0.0719176763092435));
#101523=CARTESIAN_POINT('Ctrl Pts',(0.00273558880093204,-0.0336938721132426,
0.0721386579186126));
#101524=CARTESIAN_POINT('Ctrl Pts',(0.00274736185356772,-0.0336474569765026,
0.0721071190346981));
#101525=CARTESIAN_POINT('Ctrl Pts',(0.00275950330196339,-0.0336011045488949,
0.0720757201302938));
#101526=CARTESIAN_POINT('Ctrl Pts',(0.00278998663819216,-0.033484728265791,
0.07199688741372));
#101527=CARTESIAN_POINT('Ctrl Pts',(0.00282277333995648,-0.0333679870047996,
0.0719189845050616));
#101528=CARTESIAN_POINT('Ctrl Pts',(0.00273558880091956,-0.0336938721132425,
0.0721386579186092));
#101529=CARTESIAN_POINT('Ctrl Pts',(0.00277769444724139,-0.0335278710435082,
0.0720258609123792));
#101530=CARTESIAN_POINT('Ctrl Pts',(0.00282332256568321,-0.033362046922432,
0.0719144240099955));
#101531=CARTESIAN_POINT('Ctrl Pts',(0.0028725143840075,-0.0331951640388602,
0.071804299380334));
#101532=CARTESIAN_POINT('Ctrl Pts',(0.00270798484678257,-0.0336938721132425,
0.0722178163138638));
#101533=CARTESIAN_POINT('Ctrl Pts',(0.00274843338294655,-0.0335278710435082,
0.0721044414435594));
#101534=CARTESIAN_POINT('Ctrl Pts',(0.00279242309586514,-0.033362046922432,
0.071992374913849));
#101535=CARTESIAN_POINT('Ctrl Pts',(0.00283999450320525,-0.0331951640388602,
0.0718815683079562));
#101536=CARTESIAN_POINT('Ctrl Pts',(0.00268038089264557,-0.0336938721132425,
0.0722969747091183));
#101537=CARTESIAN_POINT('Ctrl Pts',(0.0027191723186517,-0.0335278710435082,
0.0721830219747397));
#101538=CARTESIAN_POINT('Ctrl Pts',(0.00276152362604707,-0.033362046922432,
0.0720703258177025));
#101539=CARTESIAN_POINT('Ctrl Pts',(0.00280747462240301,-0.0331951640388602,
0.0719588372355784));
#101540=CARTESIAN_POINT('Ctrl Pts',(0.00265277693850858,-0.0336938721132425,
0.0723761331043729));
#101541=CARTESIAN_POINT('Ctrl Pts',(0.00268991125435685,-0.0335278710435082,
0.07226160250592));
#101542=CARTESIAN_POINT('Ctrl Pts',(0.002730624156229,-0.033362046922432,
0.0721482767215559));
#101543=CARTESIAN_POINT('Ctrl Pts',(0.00277495474160076,-0.0331951640388602,
0.0720361061632006));
#101544=CARTESIAN_POINT('Ctrl Pts',(0.00282411744560475,-0.0330240426238155,
0.0719195663327465));
#101545=CARTESIAN_POINT('Ctrl Pts',(0.00285484384237725,-0.0329142774063509,
0.0718465582876369));
#101546=CARTESIAN_POINT('Ctrl Pts',(0.00288709483760948,-0.0328043479726686,
0.0717741490458054));
#101547=CARTESIAN_POINT('Ctrl Pts',(0.00292083167001347,-0.0326943950436594,
0.0717024325067168));
#101548=CARTESIAN_POINT('Ctrl Pts',(0.00271828577620953,-0.0330240426238155,
0.0719600730450006));
#101549=CARTESIAN_POINT('Ctrl Pts',(0.00274845415355695,-0.0329142774063509,
0.0718856070655383));
#101550=CARTESIAN_POINT('Ctrl Pts',(0.00278017699074669,-0.0328043479726686,
0.0718117276267003));
#101551=CARTESIAN_POINT('Ctrl Pts',(0.00281341625496992,-0.0326943950436594,
0.0717385304927498));
#101552=CARTESIAN_POINT('Ctrl Pts',(0.00261245410681431,-0.0330240426238155,
0.0720005797572547));
#101553=CARTESIAN_POINT('Ctrl Pts',(0.00264206446473666,-0.0329142774063509,
0.0719246558434397));
#101554=CARTESIAN_POINT('Ctrl Pts',(0.00267325914388389,-0.0328043479726686,
0.0718493062075953));
#101555=CARTESIAN_POINT('Ctrl Pts',(0.00270600083992636,-0.0326943950436594,
0.0717746284787828));
#101556=CARTESIAN_POINT('Ctrl Pts',(0.00250662243741909,-0.0330240426238155,
0.0720410864695089));
#101557=CARTESIAN_POINT('Ctrl Pts',(0.00253567477591636,-0.0329142774063509,
0.0719637046213411));
#101558=CARTESIAN_POINT('Ctrl Pts',(0.0025663412970211,-0.0328043479726686,
0.0718868847884903));
#101559=CARTESIAN_POINT('Ctrl Pts',(0.00259858542488281,-0.0326943950436594,
0.0718107264648157));
#101560=CARTESIAN_POINT('Origin',(0.0180912134173041,-0.0326396682855438,
0.0789199066430371));
#101561=CARTESIAN_POINT('Ctrl Pts',(0.00274496550589082,-0.0331951640388587,
0.0714913666959631));
#101562=CARTESIAN_POINT('Ctrl Pts',(0.00278158280128254,-0.0330855618255041,
0.0714172843773542));
#101563=CARTESIAN_POINT('Ctrl Pts',(0.00281975764846336,-0.0329757224427708,
0.0713439054707414));
#101564=CARTESIAN_POINT('Ctrl Pts',(0.00285944577148284,-0.0328657862078596,
0.0712713263401401));
#101565=CARTESIAN_POINT('Ctrl Pts',(0.00278773695724827,-0.0331951640388587,
0.0715963036055249));
#101566=CARTESIAN_POINT('Ctrl Pts',(0.00282290895899642,-0.0330855618255041,
0.0715228103771325));
#101567=CARTESIAN_POINT('Ctrl Pts',(0.00285962529515387,-0.0329757224427708,
0.071449991113654));
#101568=CARTESIAN_POINT('Ctrl Pts',(0.00289784352232761,-0.0328657862078596,
0.0713779413708331));
#101569=CARTESIAN_POINT('Ctrl Pts',(0.00283050840860572,-0.0331951640388587,
0.0717012405150867));
#101570=CARTESIAN_POINT('Ctrl Pts',(0.0028642351167103,-0.0330855618255041,
0.0716283363769108));
#101571=CARTESIAN_POINT('Ctrl Pts',(0.00289949294184438,-0.0329757224427708,
0.0715560767565666));
#101572=CARTESIAN_POINT('Ctrl Pts',(0.00293624127317238,-0.0328657862078596,
0.0714845564015261));
#101573=CARTESIAN_POINT('Ctrl Pts',(0.00287327985996318,-0.0331951640388587,
0.0718061774246485));
#101574=CARTESIAN_POINT('Ctrl Pts',(0.00290556127442418,-0.0330855618255041,
0.0717338623766891));
#101575=CARTESIAN_POINT('Ctrl Pts',(0.00293936058853489,-0.0329757224427708,
0.0716621623994793));
#101576=CARTESIAN_POINT('Ctrl Pts',(0.00297463902401715,-0.0328657862078596,
0.0715911714322191));
#101577=CARTESIAN_POINT('Origin',(0.0178495159115153,-0.0326401908833634,
0.079335665211352));
#101578=CARTESIAN_POINT('Ctrl Pts',(0.00285789242902623,-0.0332451089994433,
0.0718373110904111));
#101579=CARTESIAN_POINT('Ctrl Pts',(0.00294511691831862,-0.0329451141710259,
0.07163870480859));
#101580=CARTESIAN_POINT('Ctrl Pts',(0.00304705344909823,-0.0326442513127503,
0.0714472328513648));
#101581=CARTESIAN_POINT('Ctrl Pts',(0.00276236309499031,-0.0332451089994433,
0.0720683395439372));
#101582=CARTESIAN_POINT('Ctrl Pts',(0.00284087420359961,-0.0329451141710259,
0.0718661303143357));
#101583=CARTESIAN_POINT('Ctrl Pts',(0.00293439349624683,-0.0326442513127503,
0.0716704093174707));
#101584=CARTESIAN_POINT('Ctrl Pts',(0.00297462488656823,-0.0325229783203385,
0.0715911996795726));
#101585=CARTESIAN_POINT('Ctrl Pts',(0.00300989789238602,-0.0324130253112079,
0.0715202186599985));
#101586=CARTESIAN_POINT('Ctrl Pts',(0.00304663388190617,-0.0323031222247694,
0.0714499780735101));
#101587=CARTESIAN_POINT('Ctrl Pts',(0.00308478262408177,-0.0321934096636184,
0.0713805662328438));
#101588=CARTESIAN_POINT('Ctrl Pts',(0.00286645859163048,-0.0325229783203385,
0.0716249812616677));
#101589=CARTESIAN_POINT('Ctrl Pts',(0.00290126591908632,-0.0324130253112079,
0.0715525091721105));
#101590=CARTESIAN_POINT('Ctrl Pts',(0.00293756714557121,-0.0323031222247694,
0.071480768108634));
#101591=CARTESIAN_POINT('Ctrl Pts',(0.00297531252911759,-0.0321934096636184,
0.0714098483256301));
#101592=CARTESIAN_POINT('Ctrl Pts',(0.00275829229669273,-0.0325229783203385,
0.0716587628437628));
#101593=CARTESIAN_POINT('Ctrl Pts',(0.00279263394578661,-0.0324130253112079,
0.0715847996842225));
#101594=CARTESIAN_POINT('Ctrl Pts',(0.00282850040923626,-0.0323031222247694,
0.0715115581437579));
#101595=CARTESIAN_POINT('Ctrl Pts',(0.0028658424341534,-0.0321934096636184,
0.0714391304184163));
#101596=CARTESIAN_POINT('Ctrl Pts',(0.00265012600175497,-0.0325229783203385,
0.0716925444258579));
#101597=CARTESIAN_POINT('Ctrl Pts',(0.00268400197248691,-0.0324130253112079,
0.0716170901963345));
#101598=CARTESIAN_POINT('Ctrl Pts',(0.00271943367290131,-0.0323031222247694,
0.0715423481788817));
#101599=CARTESIAN_POINT('Ctrl Pts',(0.00275637233918922,-0.0321934096636184,
0.0714684125112026));
#101600=CARTESIAN_POINT('Origin',(0.0180836286971742,-0.0326393375175912,
0.0789160126669681));
#101601=CARTESIAN_POINT('Ctrl Pts',(0.0029225163383477,-0.0326943950436593,
0.0711588742072384));
#101602=CARTESIAN_POINT('Ctrl Pts',(0.00296373965773903,-0.0325844576448127,
0.0710871910155488));
#101603=CARTESIAN_POINT('Ctrl Pts',(0.00300644842049906,-0.0324744968375319,
0.07101635531656));
#101604=CARTESIAN_POINT('Ctrl Pts',(0.00305058665383319,-0.0323646534831894,
0.070946457114334));
#101605=CARTESIAN_POINT('Ctrl Pts',(0.00295861431256972,-0.0326943950436593,
0.0712662895871365));
#101606=CARTESIAN_POINT('Ctrl Pts',(0.00299835724670818,-0.0325844576448127,
0.0711951038931866));
#101607=CARTESIAN_POINT('Ctrl Pts',(0.00303957523037726,-0.0324744968375319,
0.0711247351103519));
#101608=CARTESIAN_POINT('Ctrl Pts',(0.003082214209107,-0.0323646534831894,
0.0710552726708));
#101609=CARTESIAN_POINT('Ctrl Pts',(0.00299471228679173,-0.0326943950436593,
0.0713737049670347));
#101610=CARTESIAN_POINT('Ctrl Pts',(0.00303297483567733,-0.0325844576448127,
0.0713030167708243));
#101611=CARTESIAN_POINT('Ctrl Pts',(0.00307270204025546,-0.0324744968375319,
0.0712331149041438));
#101612=CARTESIAN_POINT('Ctrl Pts',(0.00311384176438082,-0.0323646534831894,
0.0711640882272659));
#101613=CARTESIAN_POINT('Ctrl Pts',(0.00303081026101375,-0.0326943950436593,
0.0714811203469328));
#101614=CARTESIAN_POINT('Ctrl Pts',(0.00306759242464647,-0.0325844576448127,
0.0714109296484621));
#101615=CARTESIAN_POINT('Ctrl Pts',(0.00310582885013366,-0.0324744968375319,
0.0713414946979357));
#101616=CARTESIAN_POINT('Ctrl Pts',(0.00314546931965463,-0.0323646534831894,
0.0712729037837319));
#101617=CARTESIAN_POINT('Origin',(0.0178831202510714,-0.0326395579068478,
0.0793530637798792));
#101618=CARTESIAN_POINT('Ctrl Pts',(0.00301348040185345,-0.0327445246961877,
0.0715112615509875));
#101619=CARTESIAN_POINT('Ctrl Pts',(0.00311300204837979,-0.0324436878365475,
0.0713185233700955));
#101620=CARTESIAN_POINT('Ctrl Pts',(0.00322675879178978,-0.0321434074463186,
0.0711338291150967));
#101621=CARTESIAN_POINT('Ctrl Pts',(0.0029036347080761,-0.0327445246961877,
0.0717358365352546));
#101622=CARTESIAN_POINT('Ctrl Pts',(0.00299468637069356,-0.0324436878365475,
0.0715389554563378));
#101623=CARTESIAN_POINT('Ctrl Pts',(0.00310030925253212,-0.0321434074463186,
0.0713494920790509));
#101624=CARTESIAN_POINT('Ctrl Pts',(0.00319212753136846,-0.0322357242816072,
0.0711907927924291));
#101625=CARTESIAN_POINT('Ctrl Pts',(0.00328637444297842,-0.0319819883628705,
0.0710337259875744));
#101626=CARTESIAN_POINT('Ctrl Pts',(0.00339042496164847,-0.0317295851069887,
0.0708829746986919));
#101627=CARTESIAN_POINT('Ctrl Pts',(0.00306818622113084,-0.0322357242816072,
0.0714079069366403));
#101628=CARTESIAN_POINT('Ctrl Pts',(0.00315551832883441,-0.0319819883628705,
0.0712468927618007));
#101629=CARTESIAN_POINT('Ctrl Pts',(0.00325291923975078,-0.0317295851069887,
0.0710917620940142));
#101630=CARTESIAN_POINT('Origin',(0.0177998388959256,-0.0326371942644636,
0.0793067321555741));
#101631=CARTESIAN_POINT('Origin',(0.0179742057822713,-0.0326352985531313,
0.078860421044255));
#101632=CARTESIAN_POINT('Ctrl Pts',(0.00312059419090078,-0.0321934096636183,
0.0708381863255016));
#101633=CARTESIAN_POINT('Ctrl Pts',(0.00316626668254265,-0.0320835708272303,
0.0707691884637037));
#101634=CARTESIAN_POINT('Ctrl Pts',(0.00321334058944697,-0.0319739230346346,
0.0707011758133103));
#101635=CARTESIAN_POINT('Ctrl Pts',(0.00326174900546822,-0.0318646057455576,
0.0706342307694738));
#101636=CARTESIAN_POINT('Ctrl Pts',(0.00314987630890223,-0.0321934096636183,
0.0709476565147319));
#101637=CARTESIAN_POINT('Ctrl Pts',(0.00319403912131875,-0.0320835708272303,
0.0708790624761623));
#101638=CARTESIAN_POINT('Ctrl Pts',(0.00323959586757229,-0.0319739230346346,
0.0708114221720302));
#101639=CARTESIAN_POINT('Ctrl Pts',(0.00328648161918083,-0.0318646057455576,
0.070744817670071));
#101640=CARTESIAN_POINT('Ctrl Pts',(0.00317915842690369,-0.0321934096636183,
0.0710571267039621));
#101641=CARTESIAN_POINT('Ctrl Pts',(0.00322181156009484,-0.0320835708272303,
0.0709889364886208));
#101642=CARTESIAN_POINT('Ctrl Pts',(0.0032658511456976,-0.0319739230346346,
0.0709216685307502));
#101643=CARTESIAN_POINT('Ctrl Pts',(0.00331121423289344,-0.0318646057455576,
0.0708554045706683));
#101644=CARTESIAN_POINT('Ctrl Pts',(0.00320844054490514,-0.0321934096636183,
0.0711665968931924));
#101645=CARTESIAN_POINT('Ctrl Pts',(0.00324958399887094,-0.0320835708272303,
0.0710988105010794));
#101646=CARTESIAN_POINT('Ctrl Pts',(0.00329210642382292,-0.0319739230346346,
0.0710319148894701));
#101647=CARTESIAN_POINT('Ctrl Pts',(0.00333594684660605,-0.0318646057455575,
0.0709659914712655));
#101648=CARTESIAN_POINT('Ctrl Pts',(0.00314451787502327,-0.0320218834582391,
0.071272896482392));
#101649=CARTESIAN_POINT('Ctrl Pts',(0.00317446156728867,-0.0319391099350681,
0.0712210743781347));
#101650=CARTESIAN_POINT('Ctrl Pts',(0.003205196326856,-0.0318564869454955,
0.071169751246527));
#101651=CARTESIAN_POINT('Ctrl Pts',(0.00323669627765198,-0.0317740741446541,
0.0711189623797559));
#101652=CARTESIAN_POINT('Ctrl Pts',(0.00309637002544079,-0.0320218834582391,
0.0712846698688123));
#101653=CARTESIAN_POINT('Ctrl Pts',(0.00312619118521553,-0.0319391099350681,
0.0712323466618374));
#101654=CARTESIAN_POINT('Ctrl Pts',(0.00315681131132073,-0.0318564869454955,
0.0711805208177556));
#101655=CARTESIAN_POINT('Ctrl Pts',(0.00318820457699485,-0.0317740741446541,
0.0711292280027081));
#101656=CARTESIAN_POINT('Ctrl Pts',(0.00304822217585832,-0.0320218834582391,
0.0712964432552326));
#101657=CARTESIAN_POINT('Ctrl Pts',(0.0030779208031424,-0.0319391099350681,
0.0712436189455402));
#101658=CARTESIAN_POINT('Ctrl Pts',(0.00310842629578546,-0.0318564869454955,
0.0711912903889843));
#101659=CARTESIAN_POINT('Ctrl Pts',(0.00313971287633772,-0.0317740741446541,
0.0711394936256603));
#101660=CARTESIAN_POINT('Ctrl Pts',(0.00300007432627584,-0.0320218834582391,
0.0713082166416528));
#101661=CARTESIAN_POINT('Ctrl Pts',(0.00302965042106927,-0.0319391099350681,
0.071254891229243));
#101662=CARTESIAN_POINT('Ctrl Pts',(0.00306004128025019,-0.0318564869454955,
0.071202059960213));
#101663=CARTESIAN_POINT('Ctrl Pts',(0.00309122117568059,-0.0317740741446541,
0.0711497592486124));
#101664=CARTESIAN_POINT('Origin',(-0.00277341874484063,-0.0391228853390644,
0.068941196869976));
#101665=CARTESIAN_POINT('Ctrl Pts',(0.00237219534002025,-0.0352722978779633,
0.0742084227180186));
#101666=CARTESIAN_POINT('Ctrl Pts',(0.00237235354850088,-0.0352466642097243,
0.0741895264843159));
#101667=CARTESIAN_POINT('Ctrl Pts',(0.0023724332177902,-0.0352210183808314,
0.074170646428595));
#101668=CARTESIAN_POINT('Ctrl Pts',(0.00237243381818375,-0.0351953608940152,
0.074151781882352));
#101669=CARTESIAN_POINT('Origin',(-0.00252274043965582,-0.0352456003065124,
0.0739862810774749));
#101670=CARTESIAN_POINT('Ctrl Pts',(0.00237520119150846,-0.0350241211493339,
0.0740271317437118));
#101671=CARTESIAN_POINT('Ctrl Pts',(0.00237689365128457,-0.0349144232867421,
0.0739479474009952));
#101672=CARTESIAN_POINT('Ctrl Pts',(0.00238022392095156,-0.0348045283677512,
0.0738687506469863));
#101673=CARTESIAN_POINT('Ctrl Pts',(0.00238519150971162,-0.0346945769586886,
0.0737896430813891));
#101674=CARTESIAN_POINT('Ctrl Pts',(0.00229171288836954,-0.0350241211493339,
0.0741037531835444));
#101675=CARTESIAN_POINT('Ctrl Pts',(0.00229234991927556,-0.0349144232867421,
0.0740234188237355));
#101676=CARTESIAN_POINT('Ctrl Pts',(0.00229464790002142,-0.0348045283677512,
0.0739430495478256));
#101677=CARTESIAN_POINT('Ctrl Pts',(0.00229860771792751,-0.0346945769586886,
0.0738627484081671));
#101678=CARTESIAN_POINT('Ctrl Pts',(0.00220822458523062,-0.0350241211493339,
0.074180374623377));
#101679=CARTESIAN_POINT('Ctrl Pts',(0.00220780618726655,-0.0349144232867421,
0.0740988902464757));
#101680=CARTESIAN_POINT('Ctrl Pts',(0.00220907187909128,-0.0348045283677512,
0.0740173484486649));
#101681=CARTESIAN_POINT('Ctrl Pts',(0.0022120239261434,-0.0346945769586886,
0.0739358537349451));
#101682=CARTESIAN_POINT('Ctrl Pts',(0.0021247362820917,-0.0350241211493339,
0.0742569960632096));
#101683=CARTESIAN_POINT('Ctrl Pts',(0.00212326245525754,-0.0349144232867421,
0.074174361669216));
#101684=CARTESIAN_POINT('Ctrl Pts',(0.00212349585816114,-0.0348045283677512,
0.0740916473495043));
#101685=CARTESIAN_POINT('Ctrl Pts',(0.00212544013435929,-0.0346945769586886,
0.0740089590617232));
#101686=CARTESIAN_POINT('Origin',(0.0191287125947155,-0.0345629067942066,
0.0750214915916345));
#101687=CARTESIAN_POINT('Ctrl Pts',(0.00220802251022496,-0.0351970973651537,
0.073726550886685));
#101688=CARTESIAN_POINT('Ctrl Pts',(0.00221388882378741,-0.0350869349326839,
0.073644596053935));
#101689=CARTESIAN_POINT('Ctrl Pts',(0.00222146379248379,-0.0349764985139959,
0.073562695288163));
#101690=CARTESIAN_POINT('Ctrl Pts',(0.00223074384867184,-0.0348659306865055,
0.0734809552719012));
#101691=CARTESIAN_POINT('Ctrl Pts',(0.00226492113074422,-0.0351970973651537,
0.0737859059002311));
#101692=CARTESIAN_POINT('Ctrl Pts',(0.00226996516103811,-0.0350869349326839,
0.0737047393207534));
#101693=CARTESIAN_POINT('Ctrl Pts',(0.00227670077794741,-0.0349764985139959,
0.0736236103664203));
#101694=CARTESIAN_POINT('Ctrl Pts',(0.00228512544237453,-0.0348659306865055,
0.0735426246558483));
#101695=CARTESIAN_POINT('Ctrl Pts',(0.00232181975126347,-0.0351970973651537,
0.0738452609137773));
#101696=CARTESIAN_POINT('Ctrl Pts',(0.0023260414982888,-0.0350869349326839,
0.0737648825875719));
#101697=CARTESIAN_POINT('Ctrl Pts',(0.00233193776341103,-0.0349764985139959,
0.0736845254446775));
#101698=CARTESIAN_POINT('Ctrl Pts',(0.00233950703607721,-0.0348659306865055,
0.0736042940397953));
#101699=CARTESIAN_POINT('Ctrl Pts',(0.00237871837178273,-0.0351970973651537,
0.0739046159273234));
#101700=CARTESIAN_POINT('Ctrl Pts',(0.0023821178355395,-0.0350869349326839,
0.0738250258543903));
#101701=CARTESIAN_POINT('Ctrl Pts',(0.00238717474887465,-0.0349764985139959,
0.0737454405229347));
#101702=CARTESIAN_POINT('Ctrl Pts',(0.0023938886297799,-0.0348659306865055,
0.0736659634237424));
#101703=CARTESIAN_POINT('Origin',(0.0190455869393428,-0.0345637187965369,
0.0754952167037528));
#101704=CARTESIAN_POINT('Ctrl Pts',(0.00237632436497943,-0.0352450361861252,
0.0739382135181846));
#101705=CARTESIAN_POINT('Ctrl Pts',(0.00238431202300694,-0.0349452761023764,
0.0737214445947614));
#101706=CARTESIAN_POINT('Ctrl Pts',(0.00240860491077934,-0.0346444289983475,
0.0735058931520697));
#101707=CARTESIAN_POINT('Ctrl Pts',(0.00237255042040183,-0.0352450361861252,
0.0741881850312462));
#101708=CARTESIAN_POINT('Ctrl Pts',(0.00237111024835331,-0.0349452761023764,
0.0739712737711714));
#101709=CARTESIAN_POINT('Ctrl Pts',(0.00238601281089983,-0.0346444289983475,
0.0737548702534727));
#101710=CARTESIAN_POINT('Ctrl Pts',(0.00239425952886891,-0.0345231616327822,
0.0736664187731089));
#101711=CARTESIAN_POINT('Ctrl Pts',(0.00240092501525366,-0.0344132092796975,
0.0735874453697055));
#101712=CARTESIAN_POINT('Ctrl Pts',(0.00240922366028598,-0.0343032738558973,
0.0735086139112949));
#101713=CARTESIAN_POINT('Ctrl Pts',(0.00241914224548923,-0.034193496108874,
0.0734300251177555));
#101714=CARTESIAN_POINT('Ctrl Pts',(0.00230612490165591,-0.0345231616327822,
0.0737376467425067));
#101715=CARTESIAN_POINT('Ctrl Pts',(0.00231180861076347,-0.0344132092796975,
0.0736574585273509));
#101716=CARTESIAN_POINT('Ctrl Pts',(0.00231915065659668,-0.0343032738558973,
0.0735773920125779));
#101717=CARTESIAN_POINT('Ctrl Pts',(0.00232813900566308,-0.034193496108874,
0.0734975495317082));
#101718=CARTESIAN_POINT('Ctrl Pts',(0.00221799027444291,-0.0345231616327822,
0.0738088747119046));
#101719=CARTESIAN_POINT('Ctrl Pts',(0.00222269220627329,-0.0344132092796975,
0.0737274716849962));
#101720=CARTESIAN_POINT('Ctrl Pts',(0.00222907765290738,-0.0343032738558973,
0.0736461701138609));
#101721=CARTESIAN_POINT('Ctrl Pts',(0.00223713576583693,-0.034193496108874,
0.0735650739456609));
#101722=CARTESIAN_POINT('Ctrl Pts',(0.00212985564722991,-0.0345231616327822,
0.0738801026813024));
#101723=CARTESIAN_POINT('Ctrl Pts',(0.00213357580178311,-0.0344132092796975,
0.0737974848426416));
#101724=CARTESIAN_POINT('Ctrl Pts',(0.00213900464921807,-0.0343032738558973,
0.0737149482151439));
#101725=CARTESIAN_POINT('Ctrl Pts',(0.00214613252601077,-0.034193496108874,
0.0736325983596136));
#101726=CARTESIAN_POINT('Origin',(0.0191407956598087,-0.0345625596230709,
0.0750221971657493));
#101727=CARTESIAN_POINT('Ctrl Pts',(0.00218666066001417,-0.0346945769586885,
0.0732836352377339));
#101728=CARTESIAN_POINT('Ctrl Pts',(0.00219859960434057,-0.0345846629176052,
0.0732018187021015));
#101729=CARTESIAN_POINT('Ctrl Pts',(0.00221223252022474,-0.0344746925050311,
0.0731202350844692));
#101730=CARTESIAN_POINT('Ctrl Pts',(0.002227541507892,-0.0343648066253259,
0.0730389888470288));
#101731=CARTESIAN_POINT('Ctrl Pts',(0.00225976592923148,-0.0346945769586885,
0.0733702189613448));
#101732=CARTESIAN_POINT('Ctrl Pts',(0.00227051170608294,-0.0345846629176052,
0.0732894098532731));
#101733=CARTESIAN_POINT('Ctrl Pts',(0.00228293041750801,-0.0344746925050311,
0.0732088091610593));
#101734=CARTESIAN_POINT('Ctrl Pts',(0.00229700572471198,-0.0343648066253259,
0.0731285200938829));
#101735=CARTESIAN_POINT('Ctrl Pts',(0.00233287119844878,-0.0346945769586885,
0.0734568026849557));
#101736=CARTESIAN_POINT('Ctrl Pts',(0.00234242380782531,-0.0345846629176052,
0.0733770010044447));
#101737=CARTESIAN_POINT('Ctrl Pts',(0.00235362831479128,-0.0344746925050311,
0.0732973832376494));
#101738=CARTESIAN_POINT('Ctrl Pts',(0.00236646994153196,-0.0343648066253259,
0.073218051340737));
#101739=CARTESIAN_POINT('Ctrl Pts',(0.00240597646766608,-0.0346945769586885,
0.0735433864085666));
#101740=CARTESIAN_POINT('Ctrl Pts',(0.00241433590956768,-0.0345846629176052,
0.0734645921556163));
#101741=CARTESIAN_POINT('Ctrl Pts',(0.00242432621207455,-0.0344746925050311,
0.0733859573142394));
#101742=CARTESIAN_POINT('Ctrl Pts',(0.00243593415835193,-0.0343648066253259,
0.0733075825875911));
#101743=CARTESIAN_POINT('Origin',(0.0191036692995611,-0.0345626446731572,
0.0755015861686337));
#101744=CARTESIAN_POINT('Ctrl Pts',(0.0024046683692595,-0.0346945769586885,
0.0735418371354142));
#101745=CARTESIAN_POINT('Ctrl Pts',(0.00241740658395317,-0.034527515336289,
0.0734220480065674));
#101746=CARTESIAN_POINT('Ctrl Pts',(0.00243391535124547,-0.0343603235965158,
0.0733026284992435));
#101747=CARTESIAN_POINT('Ctrl Pts',(0.00245414059620935,-0.0341934961088739,
0.0731839310776591));
#101748=CARTESIAN_POINT('Ctrl Pts',(0.00239761753723417,-0.0346945769586885,
0.0736253734394922));
#101749=CARTESIAN_POINT('Ctrl Pts',(0.00240860605059284,-0.034527515336289,
0.0735054366281457));
#101750=CARTESIAN_POINT('Ctrl Pts',(0.00242336930846644,-0.0343603235965158,
0.0733858143736273));
#101751=CARTESIAN_POINT('Ctrl Pts',(0.00244185838945779,-0.0341934961088739,
0.0732668598165172));
#101752=CARTESIAN_POINT('Ctrl Pts',(0.00239056670520884,-0.0346945769586885,
0.0737089097435703));
#101753=CARTESIAN_POINT('Ctrl Pts',(0.00239980551723251,-0.034527515336289,
0.0735888252497239));
#101754=CARTESIAN_POINT('Ctrl Pts',(0.00241282326568742,-0.0343603235965158,
0.0734690002480111));
#101755=CARTESIAN_POINT('Ctrl Pts',(0.00242957618270623,-0.0341934961088739,
0.0733497885553752));
#101756=CARTESIAN_POINT('Ctrl Pts',(0.0023835158731835,-0.0346945769586885,
0.0737924460476483));
#101757=CARTESIAN_POINT('Ctrl Pts',(0.00239100498387218,-0.034527515336289,
0.0736722138713022));
#101758=CARTESIAN_POINT('Ctrl Pts',(0.00240227722290839,-0.0343603235965158,
0.0735521861223949));
#101759=CARTESIAN_POINT('Ctrl Pts',(0.00241729397595467,-0.0341934961088739,
0.0734327172942333));
#101760=CARTESIAN_POINT('Ctrl Pts',(0.00243593008619894,-0.0340223579322365,
0.0733076138830058));
#101761=CARTESIAN_POINT('Ctrl Pts',(0.00244754878778742,-0.0339125849573552,
0.0732291635679111));
#101762=CARTESIAN_POINT('Ctrl Pts',(0.00246078306427793,-0.0338030433565216,
0.0731510088590692));
#101763=CARTESIAN_POINT('Ctrl Pts',(0.00247560713140719,-0.033693872113232,
0.0730732482029013));
#101764=CARTESIAN_POINT('Ctrl Pts',(0.00234349678459771,-0.0340223579322365,
0.0733731674075905));
#101765=CARTESIAN_POINT('Ctrl Pts',(0.00235421133211141,-0.0339125849573552,
0.0732934421961905));
#101766=CARTESIAN_POINT('Ctrl Pts',(0.00236656847725681,-0.0338030433565216,
0.0732139947730099));
#101767=CARTESIAN_POINT('Ctrl Pts',(0.00238054341092774,-0.033693872113232,
0.0731349253370677));
#101768=CARTESIAN_POINT('Ctrl Pts',(0.00225106348299649,-0.0340223579322365,
0.0734387209321752));
#101769=CARTESIAN_POINT('Ctrl Pts',(0.0022608738764354,-0.0339125849573552,
0.07335772082447));
#101770=CARTESIAN_POINT('Ctrl Pts',(0.00227235389023568,-0.0338030433565216,
0.0732769806869506));
#101771=CARTESIAN_POINT('Ctrl Pts',(0.00228547969044829,-0.033693872113232,
0.0731966024712341));
#101772=CARTESIAN_POINT('Ctrl Pts',(0.00215863018139526,-0.0340223579322365,
0.0735042744567599));
#101773=CARTESIAN_POINT('Ctrl Pts',(0.00216753642075939,-0.0339125849573552,
0.0734219994527494));
#101774=CARTESIAN_POINT('Ctrl Pts',(0.00217813930321455,-0.0338030433565216,
0.0733399666008913));
#101775=CARTESIAN_POINT('Ctrl Pts',(0.00219041596996884,-0.033693872113232,
0.0732582796054005));
#101776=CARTESIAN_POINT('Origin',(0.0190211830209275,-0.0345589643412385,
0.0750101267571015));
#101777=CARTESIAN_POINT('Ctrl Pts',(0.00225277570667803,-0.034193496108874,
0.0729125498651185));
#101778=CARTESIAN_POINT('Ctrl Pts',(0.00226983941103179,-0.0340836138595105,
0.072831592163374));
#101779=CARTESIAN_POINT('Ctrl Pts',(0.00228857017764344,-0.0339738896671456,
0.0727510264042088));
#101780=CARTESIAN_POINT('Ctrl Pts',(0.00230893712119388,-0.0338644633335883,
0.0726709540948107));
#101781=CARTESIAN_POINT('Ctrl Pts',(0.00232030018138788,-0.034193496108874,
0.0730035531868276));
#101782=CARTESIAN_POINT('Ctrl Pts',(0.00233610900384129,-0.0340836138595105,
0.072923526607591));
#101783=CARTESIAN_POINT('Ctrl Pts',(0.0023535662230422,-0.0339738896671456,
0.0728438655570162));
#101784=CARTESIAN_POINT('Ctrl Pts',(0.00237264266127564,-0.0338644633335883,
0.0727646704936415));
#101785=CARTESIAN_POINT('Ctrl Pts',(0.00238782465609773,-0.0341934961088739,
0.0730945565085366));
#101786=CARTESIAN_POINT('Ctrl Pts',(0.00240237859665078,-0.0340836138595105,
0.0730154610518081));
#101787=CARTESIAN_POINT('Ctrl Pts',(0.00241856226844097,-0.0339738896671456,
0.0729367047098237));
#101788=CARTESIAN_POINT('Ctrl Pts',(0.0024363482013574,-0.0338644633335883,
0.0728583868924724));
#101789=CARTESIAN_POINT('Ctrl Pts',(0.00245534913080758,-0.0341934961088739,
0.0731855598302457));
#101790=CARTESIAN_POINT('Ctrl Pts',(0.00246864818946028,-0.0340836138595105,
0.0731073954960251));
#101791=CARTESIAN_POINT('Ctrl Pts',(0.00248355831383973,-0.0339738896671456,
0.0730295438626311));
#101792=CARTESIAN_POINT('Ctrl Pts',(0.00250005374143916,-0.0338644633335883,
0.0729521032913032));
#101793=CARTESIAN_POINT('Origin',(0.0190291047356391,-0.0345610621861485,
0.0754912579844561));
#101794=CARTESIAN_POINT('Ctrl Pts',(0.00244817597163118,-0.03424362768739,
0.0732196135110987));
#101795=CARTESIAN_POINT('Ctrl Pts',(0.00248326607652709,-0.033943005420186,
0.0730055544936525));
#101796=CARTESIAN_POINT('Ctrl Pts',(0.00253438029638688,-0.0336441434784164,
0.0727947467259119));
#101797=CARTESIAN_POINT('Ctrl Pts',(0.002413105426267,-0.03424362768739,
0.0734671414021492));
#101798=CARTESIAN_POINT('Ctrl Pts',(0.00243885986285169,-0.033943005420186,
0.0732517596772794));
#101799=CARTESIAN_POINT('Ctrl Pts',(0.002480764567798,-0.0336441434784164,
0.0730389297589995));
#101800=CARTESIAN_POINT('Ctrl Pts',(0.00250004808859784,-0.0335235895815127,
0.0729521304373025));
#101801=CARTESIAN_POINT('Ctrl Pts',(0.00251653912151628,-0.0334144449262719,
0.0728747086652415));
#101802=CARTESIAN_POINT('Ctrl Pts',(0.002534648576178,-0.0333049234473132,
0.0727975386372734));
#101803=CARTESIAN_POINT('Ctrl Pts',(0.00255436223471938,-0.0331951640388588,
0.0727207211277815));
#101804=CARTESIAN_POINT('Ctrl Pts',(0.0024036810435052,-0.0335235895815127,
0.0730117506109557));
#101805=CARTESIAN_POINT('Ctrl Pts',(0.002419351287352,-0.0334144449262719,
0.0729330021567897));
#101806=CARTESIAN_POINT('Ctrl Pts',(0.00243666641820872,-0.0333049234473132,
0.0728544869656352));
#101807=CARTESIAN_POINT('Ctrl Pts',(0.00245561338971766,-0.0331951640388588,
0.0727763074399199));
#101808=CARTESIAN_POINT('Ctrl Pts',(0.00230731399841256,-0.0335235895815127,
0.0730713707846088));
#101809=CARTESIAN_POINT('Ctrl Pts',(0.00232216345318771,-0.0334144449262719,
0.0729912956483379));
#101810=CARTESIAN_POINT('Ctrl Pts',(0.00233868426023943,-0.0333049234473132,
0.0729114352939969));
#101811=CARTESIAN_POINT('Ctrl Pts',(0.00235686454471594,-0.0331951640388588,
0.0728318937520582));
#101812=CARTESIAN_POINT('Ctrl Pts',(0.00221094695331992,-0.0335235895815127,
0.0731309909582619));
#101813=CARTESIAN_POINT('Ctrl Pts',(0.00222497561902343,-0.0334144449262719,
0.0730495891398861));
#101814=CARTESIAN_POINT('Ctrl Pts',(0.00224070210227015,-0.0333049234473132,
0.0729683836223587));
#101815=CARTESIAN_POINT('Ctrl Pts',(0.00225811569971422,-0.0331951640388588,
0.0728874800641966));
#101816=CARTESIAN_POINT('Origin',(0.0184922424657708,-0.0326434571769605,
0.0775966635810342));
#101817=CARTESIAN_POINT('Ctrl Pts',(0.00234095736948707,-0.0336938721132393,
0.0725446472057946));
#101818=CARTESIAN_POINT('Ctrl Pts',(0.00235035403210412,-0.033647456976496,
0.0725107984131571));
#101819=CARTESIAN_POINT('Ctrl Pts',(0.00236014629371103,-0.033601104548885,
0.0724770619396607));
#101820=CARTESIAN_POINT('Ctrl Pts',(0.00238493804765038,-0.033483750864317,
0.0723916489489461));
#101821=CARTESIAN_POINT('Ctrl Pts',(0.00241224987877581,-0.0333660264760423,
0.0723070080963583));
#101822=CARTESIAN_POINT('Ctrl Pts',(0.0025259883083282,-0.0336938721132393,
0.0728298376525904));
#101823=CARTESIAN_POINT('Ctrl Pts',(0.00253371565662393,-0.033647456976496,
0.0727970719074377));
#101824=CARTESIAN_POINT('Ctrl Pts',(0.00254182603985373,-0.033601104548885,
0.0727643988657831));
#101825=CARTESIAN_POINT('Ctrl Pts',(0.00256235966461365,-0.033483750864317,
0.0726816782398781));
#101826=CARTESIAN_POINT('Ctrl Pts',(0.00258533545606793,-0.0333660264760423,
0.072599602392621));
#101827=CARTESIAN_POINT('Ctrl Pts',(0.0025259883083393,-0.0336938721132427,
0.0728298376525957));
#101828=CARTESIAN_POINT('Ctrl Pts',(0.0025337156566345,-0.0336474569765026,
0.0727970719074453));
#101829=CARTESIAN_POINT('Ctrl Pts',(0.00254182603986373,-0.0336011045488949,
0.0727643988657931));
#101830=CARTESIAN_POINT('Ctrl Pts',(0.00256218864749723,-0.0334847282606778,
0.0726823671900321));
#101831=CARTESIAN_POINT('Ctrl Pts',(0.00258495299398426,-0.0333679869945434,
0.0726009693021799));
#101832=CARTESIAN_POINT('Ctrl Pts',(0.00252598830832766,-0.0336938721132425,
0.0728298376525926));
#101833=CARTESIAN_POINT('Ctrl Pts',(0.00255362472552474,-0.0335278710435082,
0.0727126528476428));
#101834=CARTESIAN_POINT('Ctrl Pts',(0.00258492630531003,-0.033362046922432,
0.0725963759388932));
#101835=CARTESIAN_POINT('Ctrl Pts',(0.00261992795552341,-0.0331951640388602,
0.0724809543051736));
#101836=CARTESIAN_POINT('Ctrl Pts',(0.00250852319725496,-0.0336938721132425,
0.0729118315530883));
#101837=CARTESIAN_POINT('Ctrl Pts',(0.00253444314552974,-0.0335278710435082,
0.0727942811316695));
#101838=CARTESIAN_POINT('Ctrl Pts',(0.00256404032587993,-0.033362046922432,
0.0726775849070547));
#101839=CARTESIAN_POINT('Ctrl Pts',(0.00259734886824744,-0.0331951640388602,
0.0725616897660385));
#101840=CARTESIAN_POINT('Ctrl Pts',(0.00249105808618226,-0.0336938721132425,
0.0729938254535839));
#101841=CARTESIAN_POINT('Ctrl Pts',(0.00251526156553474,-0.0335278710435082,
0.0728759094156961));
#101842=CARTESIAN_POINT('Ctrl Pts',(0.00254315434644982,-0.033362046922432,
0.0727587938752161));
#101843=CARTESIAN_POINT('Ctrl Pts',(0.00257476978097148,-0.0331951640388602,
0.0726424252269033));
#101844=CARTESIAN_POINT('Ctrl Pts',(0.00247359297510956,-0.0336938721132425,
0.0730758193540796));
#101845=CARTESIAN_POINT('Ctrl Pts',(0.00249607998553974,-0.0335278710435082,
0.0729575376997227));
#101846=CARTESIAN_POINT('Ctrl Pts',(0.00252226836701971,-0.033362046922432,
0.0728400028433776));
#101847=CARTESIAN_POINT('Ctrl Pts',(0.00255219069369551,-0.0331951640388602,
0.0727231606877681));
#101848=CARTESIAN_POINT('Ctrl Pts',(0.00258635942130437,-0.0330240426238155,
0.0726013780880225));
#101849=CARTESIAN_POINT('Ctrl Pts',(0.00260769319689097,-0.0329142774063509,
0.0725250946944917));
#101850=CARTESIAN_POINT('Ctrl Pts',(0.0026306145989742,-0.0328043479726686,
0.0724492142996415));
#101851=CARTESIAN_POINT('Ctrl Pts',(0.00265509694063396,-0.0326943950436594,
0.072373834920589));
#101852=CARTESIAN_POINT('Ctrl Pts',(0.00248643910346057,-0.0330240426238155,
0.0726548296180905));
#101853=CARTESIAN_POINT('Ctrl Pts',(0.00250703653214519,-0.0329142774063509,
0.0725771697248338));
#101854=CARTESIAN_POINT('Ctrl Pts',(0.00252924967632504,-0.0328043479726686,
0.072499896921675));
#101855=CARTESIAN_POINT('Ctrl Pts',(0.00255305280553612,-0.0326943950436594,
0.0724231109845222));
#101856=CARTESIAN_POINT('Ctrl Pts',(0.00238651878561677,-0.0330240426238155,
0.0727082811481585));
#101857=CARTESIAN_POINT('Ctrl Pts',(0.00240637986739941,-0.0329142774063509,
0.0726292447551759));
#101858=CARTESIAN_POINT('Ctrl Pts',(0.00242788475367589,-0.0328043479726686,
0.0725505795437084));
#101859=CARTESIAN_POINT('Ctrl Pts',(0.00245100867043827,-0.0326943950436594,
0.0724723870484554));
#101860=CARTESIAN_POINT('Ctrl Pts',(0.00228659846777298,-0.0330240426238155,
0.0727617326782265));
#101861=CARTESIAN_POINT('Ctrl Pts',(0.00230572320265362,-0.0329142774063509,
0.0726813197855179));
#101862=CARTESIAN_POINT('Ctrl Pts',(0.00232651983102673,-0.0328043479726686,
0.0726012621657419));
#101863=CARTESIAN_POINT('Ctrl Pts',(0.00234896453534043,-0.0326943950436594,
0.0725216631123886));
#101864=CARTESIAN_POINT('Origin',(0.0186104450682804,-0.0326396682854751,
0.0776330441188748));
#101865=CARTESIAN_POINT('Ctrl Pts',(0.00245416397318748,-0.0331951640388587,
0.0721864753018193));
#101866=CARTESIAN_POINT('Ctrl Pts',(0.00248120755687549,-0.0330855618127431,
0.0721083877712924));
#101867=CARTESIAN_POINT('Ctrl Pts',(0.00250988457187204,-0.0329757224171935,
0.0720308028932627));
#101868=CARTESIAN_POINT('Ctrl Pts',(0.00254016316895784,-0.0328657861694598,
0.07195382182117));
#101869=CARTESIAN_POINT('Ctrl Pts',(0.00250975024107142,-0.0331951640388587,
0.0722852240682033));
#101870=CARTESIAN_POINT('Ctrl Pts',(0.00253543376011127,-0.0330855618127431,
0.0722079021261555));
#101871=CARTESIAN_POINT('Ctrl Pts',(0.0025627339066009,-0.0329757224171935,
0.0721310552782923));
#101872=CARTESIAN_POINT('Ctrl Pts',(0.00259162054812548,-0.0328657861694598,
0.0720547836464745));
#101873=CARTESIAN_POINT('Ctrl Pts',(0.00256533650895536,-0.0331951640388587,
0.0723839728345872));
#101874=CARTESIAN_POINT('Ctrl Pts',(0.00258965996334704,-0.0330855618127431,
0.0723074164810186));
#101875=CARTESIAN_POINT('Ctrl Pts',(0.00261558324132976,-0.0329757224171935,
0.0722313076633219));
#101876=CARTESIAN_POINT('Ctrl Pts',(0.00264307792729312,-0.0328657861694598,
0.072155745471779));
#101877=CARTESIAN_POINT('Ctrl Pts',(0.00262092277683929,-0.0331951640388587,
0.0724827216009712));
#101878=CARTESIAN_POINT('Ctrl Pts',(0.00264388616658281,-0.0330855618127431,
0.0724069308358816));
#101879=CARTESIAN_POINT('Ctrl Pts',(0.00266843257605861,-0.0329757224171935,
0.0723315600483515));
#101880=CARTESIAN_POINT('Ctrl Pts',(0.00269453530646077,-0.0328657861694598,
0.0722567072970835));
#101881=CARTESIAN_POINT('Origin',(0.0184227617885679,-0.032640190883161,
0.0780758170378834));
#101882=CARTESIAN_POINT('Ctrl Pts',(0.00260955876339398,-0.0332451089994433,
0.0725155383249555));
#101883=CARTESIAN_POINT('Ctrl Pts',(0.0026712034940288,-0.0329451141710258,
0.0723075659856985));
#101884=CARTESIAN_POINT('Ctrl Pts',(0.00274833842528032,-0.0326442513127503,
0.0721048278070249));
#101885=CARTESIAN_POINT('Ctrl Pts',(0.00254373824981596,-0.0332451089994433,
0.0727567180504557));
#101886=CARTESIAN_POINT('Ctrl Pts',(0.00259628673828125,-0.0329451141710258,
0.0725462632499138));
#101887=CARTESIAN_POINT('Ctrl Pts',(0.00266453825795956,-0.0326442513127503,
0.07234036449622));
#101888=CARTESIAN_POINT('Ctrl Pts',(0.00269452481170455,-0.0325229783203384,
0.0722567371197357));
#101889=CARTESIAN_POINT('Ctrl Pts',(0.00272062339863101,-0.0324130253112079,
0.0721818949268253));
#101890=CARTESIAN_POINT('Ctrl Pts',(0.00274826623406922,-0.0323031222247695,
0.0721076039679865));
#101891=CARTESIAN_POINT('Ctrl Pts',(0.00277741455157991,-0.0321934096636185,
0.0720339581552029));
#101892=CARTESIAN_POINT('Ctrl Pts',(0.00259144539522894,-0.0325229783203384,
0.0723038091554731));
#101893=CARTESIAN_POINT('Ctrl Pts',(0.00261689509518397,-0.0324130253112079,
0.0722275460150867));
#101894=CARTESIAN_POINT('Ctrl Pts',(0.00264391853619052,-0.0323031222247695,
0.0721518209012261));
#101895=CARTESIAN_POINT('Ctrl Pts',(0.00267247768038604,-0.0321934096636185,
0.0720767295909218));
#101896=CARTESIAN_POINT('Ctrl Pts',(0.00248836597875334,-0.0325229783203384,
0.0723508811912106));
#101897=CARTESIAN_POINT('Ctrl Pts',(0.00251316679173693,-0.0324130253112079,
0.0722731971033481));
#101898=CARTESIAN_POINT('Ctrl Pts',(0.00253957083831181,-0.0323031222247695,
0.0721960378344656));
#101899=CARTESIAN_POINT('Ctrl Pts',(0.00256754080919217,-0.0321934096636184,
0.0721195010266408));
#101900=CARTESIAN_POINT('Ctrl Pts',(0.00238528656227773,-0.0325229783203384,
0.072397953226948));
#101901=CARTESIAN_POINT('Ctrl Pts',(0.0024094384882899,-0.0324130253112079,
0.0723188481916095));
#101902=CARTESIAN_POINT('Ctrl Pts',(0.0024352231404331,-0.0323031222247695,
0.0722402547677052));
#101903=CARTESIAN_POINT('Ctrl Pts',(0.0024626039379983,-0.0321934096636184,
0.0721622724623597));
#101904=CARTESIAN_POINT('Origin',(0.0186024321118089,-0.0326393375178981,
0.0776301314651015));
#101905=CARTESIAN_POINT('Ctrl Pts',(0.00258864240555086,-0.0326943950436594,
0.071834351595725));
#101906=CARTESIAN_POINT('Ctrl Pts',(0.00262055638054933,-0.0325844576448127,
0.0717580669954951));
#101907=CARTESIAN_POINT('Ctrl Pts',(0.00265405030475245,-0.0324744968375319,
0.0716824370298121));
#101908=CARTESIAN_POINT('Ctrl Pts',(0.00268907992722798,-0.0323646534831894,
0.0716075580082806));
#101909=CARTESIAN_POINT('Ctrl Pts',(0.00263791845336137,-0.0326943950436594,
0.0719363956974349));
#101910=CARTESIAN_POINT('Ctrl Pts',(0.00266842606938725,-0.0325844576448127,
0.0718607902134969));
#101911=CARTESIAN_POINT('Ctrl Pts',(0.00270049948984924,-0.0324744968375319,
0.0717858103263588));
#101912=CARTESIAN_POINT('Ctrl Pts',(0.00273409629533575,-0.0323646534831894,
0.0717115515378101));
#101913=CARTESIAN_POINT('Ctrl Pts',(0.00268719450117189,-0.0326943950436594,
0.0720384397991448));
#101914=CARTESIAN_POINT('Ctrl Pts',(0.00271629575822518,-0.0325844576448127,
0.0719635134314988));
#101915=CARTESIAN_POINT('Ctrl Pts',(0.00274694867494603,-0.0324744968375319,
0.0718891836229055));
#101916=CARTESIAN_POINT('Ctrl Pts',(0.00277911266344352,-0.0323646534831894,
0.0718155450673395));
#101917=CARTESIAN_POINT('Ctrl Pts',(0.00273647054898241,-0.0326943950436594,
0.0721404839008547));
#101918=CARTESIAN_POINT('Ctrl Pts',(0.00276416544706311,-0.0325844576448127,
0.0720662366495007));
#101919=CARTESIAN_POINT('Ctrl Pts',(0.00279339786004281,-0.0324744968375319,
0.0719925569194521));
#101920=CARTESIAN_POINT('Ctrl Pts',(0.0028241290315513,-0.0323646534831894,
0.0719195385968689));
#101921=CARTESIAN_POINT('Origin',(0.0184582817635514,-0.0326395579068394,
0.0780888666716867));
#101922=CARTESIAN_POINT('Ctrl Pts',(0.00272305503550547,-0.0327445246961876,
0.0721725594397983));
#101923=CARTESIAN_POINT('Ctrl Pts',(0.00279763542468079,-0.0324436878365475,
0.071968867687262));
#101924=CARTESIAN_POINT('Ctrl Pts',(0.00288734683399173,-0.0321434074463186,
0.0717713723011381));
#101925=CARTESIAN_POINT('Ctrl Pts',(0.00264222221678873,-0.0327445246961876,
0.0724091308992313));
#101926=CARTESIAN_POINT('Ctrl Pts',(0.00270788016760237,-0.0324436878365475,
0.0722023904871302));
#101927=CARTESIAN_POINT('Ctrl Pts',(0.00278892412375222,-0.0321434074463186,
0.072001183027844));
#101928=CARTESIAN_POINT('Ctrl Pts',(0.00286012809327848,-0.0322357242816072,
0.0718322272507116));
#101929=CARTESIAN_POINT('Ctrl Pts',(0.00293394614930217,-0.0319819883628705,
0.0716645866943412));
#101930=CARTESIAN_POINT('Ctrl Pts',(0.00301828205205449,-0.0317295851069887,
0.0715019831364399));
#101931=CARTESIAN_POINT('Ctrl Pts',(0.00276437571503811,-0.0322357242816072,
0.0720631633502311));
#101932=CARTESIAN_POINT('Ctrl Pts',(0.00283083875580525,-0.0319819883628705,
0.0718924732048001));
#101933=CARTESIAN_POINT('Ctrl Pts',(0.00290802860322813,-0.0317295851069887,
0.0717263582175471));
#101934=CARTESIAN_POINT('Origin',(0.0183698502145489,-0.0326371942646075,
0.078053338307413));
#101935=CARTESIAN_POINT('Origin',(0.0184869045507201,-0.032635298552719,
0.077588692527467));
#101936=CARTESIAN_POINT('Ctrl Pts',(0.00274496550589063,-0.0321934096636183,
0.0714913666959626));
#101937=CARTESIAN_POINT('Ctrl Pts',(0.00278163013116605,-0.0320835708272303,
0.0714171886218511));
#101938=CARTESIAN_POINT('Ctrl Pts',(0.00281980860085707,-0.0319739230346346,
0.0713438123465517));
#101939=CARTESIAN_POINT('Ctrl Pts',(0.00285944486324399,-0.0318646057455575,
0.0712713280010697));
#101940=CARTESIAN_POINT('Ctrl Pts',(0.00278773697844063,-0.0321934096636183,
0.0715963036575189));
#101941=CARTESIAN_POINT('Ctrl Pts',(0.0028229544412333,-0.0320835708272303,
0.071522715435348));
#101942=CARTESIAN_POINT('Ctrl Pts',(0.00285967438089936,-0.0319739230346346,
0.0714498987208986));
#101943=CARTESIAN_POINT('Ctrl Pts',(0.00289784266675191,-0.0318646057455575,
0.071377943072474));
#101944=CARTESIAN_POINT('Ctrl Pts',(0.00283050845099063,-0.0321934096636183,
0.0717012406190752));
#101945=CARTESIAN_POINT('Ctrl Pts',(0.00286427875130054,-0.0320835708272303,
0.0716282422488448));
#101946=CARTESIAN_POINT('Ctrl Pts',(0.00289954016094165,-0.0319739230346346,
0.0715559850952455));
#101947=CARTESIAN_POINT('Ctrl Pts',(0.00293624047025983,-0.0318646057455575,
0.0714845581438782));
#101948=CARTESIAN_POINT('Ctrl Pts',(0.00287327992354062,-0.0321934096636183,
0.0718061775806315));
#101949=CARTESIAN_POINT('Ctrl Pts',(0.00290560306136778,-0.0320835708272303,
0.0717337690623416));
#101950=CARTESIAN_POINT('Ctrl Pts',(0.00293940594098394,-0.0319739230346346,
0.0716620714695923));
#101951=CARTESIAN_POINT('Ctrl Pts',(0.00297463827376775,-0.0318646057455575,
0.0715911732152825));
#101952=CARTESIAN_POINT('Ctrl Pts',(0.00282318417424442,-0.0320218834582395,
0.0719196506007348));
#101953=CARTESIAN_POINT('Ctrl Pts',(0.00284639671965595,-0.0319391099350682,
0.0718644841894713));
#101954=CARTESIAN_POINT('Ctrl Pts',(0.00287045663242311,-0.0318564869454953,
0.0718097136692862));
#101955=CARTESIAN_POINT('Ctrl Pts',(0.00289534266379709,-0.0317740741446536,
0.0717553772972089));
#101956=CARTESIAN_POINT('Ctrl Pts',(0.00277689158142658,-0.0320218834582395,
0.0719373656761641));
#101957=CARTESIAN_POINT('Ctrl Pts',(0.00279991975572881,-0.0319391099350682,
0.071881717470921));
#101958=CARTESIAN_POINT('Ctrl Pts',(0.00282380293237298,-0.0318564869454953,
0.0718264625696823));
#101959=CARTESIAN_POINT('Ctrl Pts',(0.00284851995840211,-0.0317740741446536,
0.0717716395943025));
#101960=CARTESIAN_POINT('Ctrl Pts',(0.00273059898860874,-0.0320218834582395,
0.0719550807515934));
#101961=CARTESIAN_POINT('Ctrl Pts',(0.00275344279180167,-0.0319391099350682,
0.0718989507523707));
#101962=CARTESIAN_POINT('Ctrl Pts',(0.00277714923232285,-0.0318564869454953,
0.0718432114700783));
#101963=CARTESIAN_POINT('Ctrl Pts',(0.00280169725300713,-0.0317740741446536,
0.071787901891396));
#101964=CARTESIAN_POINT('Ctrl Pts',(0.0026843063957909,-0.0320218834582395,
0.0719727958270227));
#101965=CARTESIAN_POINT('Ctrl Pts',(0.00270696582787452,-0.0319391099350682,
0.0719161840338204));
#101966=CARTESIAN_POINT('Ctrl Pts',(0.00273049553227273,-0.0318564869454953,
0.0718599603704744));
#101967=CARTESIAN_POINT('Ctrl Pts',(0.00275487454761215,-0.0317740741446536,
0.0718041641884896));
#101968=CARTESIAN_POINT('Origin',(-0.00334032719988602,-0.0391228853390595,
0.0703480512688116));
#101969=CARTESIAN_POINT('Ctrl Pts',(0.00242487062843551,-0.035272297877964,
0.0749288270158611));
#101970=CARTESIAN_POINT('Ctrl Pts',(0.00242265926332284,-0.0352466642097247,
0.0749100599558245));
#101971=CARTESIAN_POINT('Ctrl Pts',(0.00242037200596261,-0.0352210183808316,
0.0748913187897723));
#101972=CARTESIAN_POINT('Ctrl Pts',(0.00241800824704151,-0.0351953608940153,
0.0748726029208616));
#101973=CARTESIAN_POINT('Origin',(-0.00245930885073002,-0.0352456003065141,
0.0753219351578665));
#101974=CARTESIAN_POINT('Ctrl Pts',(0.00240513099386094,-0.0350241211493338,
0.0747485888419485));
#101975=CARTESIAN_POINT('Ctrl Pts',(0.00239688567836588,-0.034914423286742,
0.074669816769969));
#101976=CARTESIAN_POINT('Ctrl Pts',(0.00239026370259411,-0.0348045283677512,
0.0745908271125543));
#101977=CARTESIAN_POINT('Ctrl Pts',(0.00238527731343735,-0.0346945769586886,
0.0745117207297779));
#101978=CARTESIAN_POINT('Ctrl Pts',(0.00233190423374359,-0.0350241211493338,
0.0748350699578395));
#101979=CARTESIAN_POINT('Ctrl Pts',(0.00232246767638947,-0.034914423286742,
0.074755289217309));
#101980=CARTESIAN_POINT('Ctrl Pts',(0.00231467459564178,-0.0348045283677512,
0.0746752656637873));
#101981=CARTESIAN_POINT('Ctrl Pts',(0.00230853878770864,-0.0346945769586886,
0.0745951014258173));
#101982=CARTESIAN_POINT('Ctrl Pts',(0.00225867747362623,-0.0350241211493338,
0.0749215510737304));
#101983=CARTESIAN_POINT('Ctrl Pts',(0.00224804967441307,-0.034914423286742,
0.074840761664649));
#101984=CARTESIAN_POINT('Ctrl Pts',(0.00223908548868946,-0.0348045283677512,
0.0747597042150202));
#101985=CARTESIAN_POINT('Ctrl Pts',(0.00223180026197993,-0.0346945769586886,
0.0746784821218568));
#101986=CARTESIAN_POINT('Ctrl Pts',(0.00218545071350887,-0.0350241211493338,
0.0750080321896214));
#101987=CARTESIAN_POINT('Ctrl Pts',(0.00217363167243667,-0.034914423286742,
0.074926234111989));
#101988=CARTESIAN_POINT('Ctrl Pts',(0.00216349638173713,-0.0348045283677512,
0.0748441427662532));
#101989=CARTESIAN_POINT('Ctrl Pts',(0.00215506173625123,-0.0346945769586886,
0.0747618628178962));
#101990=CARTESIAN_POINT('Origin',(0.0191511622908026,-0.0345629067940586,
0.0736353361079466));
#101991=CARTESIAN_POINT('Ctrl Pts',(0.00220159779565417,-0.0351970973651532,
0.0744713311994661));
#101992=CARTESIAN_POINT('Ctrl Pts',(0.00219714618738722,-0.0350869349326836,
0.0743892873610033));
#101993=CARTESIAN_POINT('Ctrl Pts',(0.00219439653738732,-0.0349764985139958,
0.0743070830119113));
#101994=CARTESIAN_POINT('Ctrl Pts',(0.00219335867701082,-0.0348659306865056,
0.0742248244406427));
#101995=CARTESIAN_POINT('Ctrl Pts',(0.00226548690933194,-0.0351970973651532,
0.074523086892907));
#101996=CARTESIAN_POINT('Ctrl Pts',(0.0022603182960771,-0.0350869349326836,
0.074441928151525));
#101997=CARTESIAN_POINT('Ctrl Pts',(0.00225683264645299,-0.0349764985139958,
0.0743605947265817));
#101998=CARTESIAN_POINT('Ctrl Pts',(0.00225504067890629,-0.0348659306865056,
0.0742791917220926));
#101999=CARTESIAN_POINT('Ctrl Pts',(0.00232937602300971,-0.0351970973651532,
0.0745748425863479));
#102000=CARTESIAN_POINT('Ctrl Pts',(0.00232349040476698,-0.0350869349326836,
0.0744945689420467));
#102001=CARTESIAN_POINT('Ctrl Pts',(0.00231926875551866,-0.0349764985139958,
0.074414106441252));
#102002=CARTESIAN_POINT('Ctrl Pts',(0.00231672268080175,-0.0348659306865056,
0.0743335590035424));
#102003=CARTESIAN_POINT('Ctrl Pts',(0.00239326513668748,-0.0351970973651532,
0.0746265982797888));
#102004=CARTESIAN_POINT('Ctrl Pts',(0.00238666251345686,-0.0350869349326836,
0.0745472097325684));
#102005=CARTESIAN_POINT('Ctrl Pts',(0.00238170486458433,-0.0349764985139958,
0.0744676181559223));
#102006=CARTESIAN_POINT('Ctrl Pts',(0.00237840468269722,-0.0348659306865056,
0.0743879262849923));
#102007=CARTESIAN_POINT('Origin',(0.0191280656060807,-0.0345637187964347,
0.0741157441631858));
#102008=CARTESIAN_POINT('Ctrl Pts',(0.00239510090204551,-0.0352450361861253,
0.0746602309922252));
#102009=CARTESIAN_POINT('Ctrl Pts',(0.0023758572248948,-0.0349452761023765,
0.0744441702374998));
#102010=CARTESIAN_POINT('Ctrl Pts',(0.00237294279667918,-0.0346444289983475,
0.0742272737761386));
#102011=CARTESIAN_POINT('Ctrl Pts',(0.00242268645417911,-0.0352450361861253,
0.0749087044059207));
#102012=CARTESIAN_POINT('Ctrl Pts',(0.00239407144869566,-0.0349452761023765,
0.0746936840573395));
#102013=CARTESIAN_POINT('Ctrl Pts',(0.00238173394745746,-0.0346444289983475,
0.0744771191596621));
#102014=CARTESIAN_POINT('Ctrl Pts',(0.0023788297275446,-0.0345231616327822,
0.0743883315578107));
#102015=CARTESIAN_POINT('Ctrl Pts',(0.0023755446625642,-0.0344132092796975,
0.0743091454763196));
#102016=CARTESIAN_POINT('Ctrl Pts',(0.00237389766871257,-0.0343032738558974,
0.0742298955314883));
#102017=CARTESIAN_POINT('Ctrl Pts',(0.00237388825529274,-0.0341934961088741,
0.0741506833057032));
#102018=CARTESIAN_POINT('Ctrl Pts',(0.00230031729991655,-0.0345231616327822,
0.0744700440712127));
#102019=CARTESIAN_POINT('Ctrl Pts',(0.00229590594298092,-0.0344132092796975,
0.0743897758064433));
#102020=CARTESIAN_POINT('Ctrl Pts',(0.00229315509939306,-0.0343032738558974,
0.0743094204377089));
#102021=CARTESIAN_POINT('Ctrl Pts',(0.00229206565633918,-0.0341934961088741,
0.0742290809997956));
#102022=CARTESIAN_POINT('Ctrl Pts',(0.0022218048722885,-0.0345231616327822,
0.0745517565846147));
#102023=CARTESIAN_POINT('Ctrl Pts',(0.00221626722339765,-0.0344132092796975,
0.0744704061365671));
#102024=CARTESIAN_POINT('Ctrl Pts',(0.00221241253007354,-0.0343032738558974,
0.0743889453439295));
#102025=CARTESIAN_POINT('Ctrl Pts',(0.00221024305738562,-0.0341934961088741,
0.074307478693888));
#102026=CARTESIAN_POINT('Ctrl Pts',(0.00214329244466045,-0.0345231616327822,
0.0746334690980167));
#102027=CARTESIAN_POINT('Ctrl Pts',(0.00213662850381438,-0.0344132092796975,
0.0745510364666909));
#102028=CARTESIAN_POINT('Ctrl Pts',(0.00213166996075403,-0.0343032738558974,
0.07446847025015));
#102029=CARTESIAN_POINT('Ctrl Pts',(0.00212842045843206,-0.0341934961088741,
0.0743858763879804));
#102030=CARTESIAN_POINT('Origin',(0.0191632385091167,-0.0345625596229836,
0.0736345217087045));
#102031=CARTESIAN_POINT('Ctrl Pts',(0.00212489233953381,-0.0346945769586885,
0.0740345854224619));
#102032=CARTESIAN_POINT('Ctrl Pts',(0.00212648281074835,-0.0345846629176052,
0.0739519176881526));
#102033=CARTESIAN_POINT('Ctrl Pts',(0.00212978308841509,-0.0344746925050311,
0.0738692687242825));
#102034=CARTESIAN_POINT('Ctrl Pts',(0.00213478850648869,-0.034364806625326,
0.0737867444127645));
#102035=CARTESIAN_POINT('Ctrl Pts',(0.00220827296992208,-0.0346945769586885,
0.0741113238877693));
#102036=CARTESIAN_POINT('Ctrl Pts',(0.00220880594629738,-0.0345846629176052,
0.0740298051806913));
#102037=CARTESIAN_POINT('Ctrl Pts',(0.0022110247870909,-0.0344746925050311,
0.0739482835717502));
#102038=CARTESIAN_POINT('Ctrl Pts',(0.0022149262178844,-0.034364806625326,
0.0738668635040844));
#102039=CARTESIAN_POINT('Ctrl Pts',(0.00229165360031035,-0.0346945769586885,
0.0741880623530767));
#102040=CARTESIAN_POINT('Ctrl Pts',(0.00229112908184641,-0.0345846629176052,
0.0741076926732299));
#102041=CARTESIAN_POINT('Ctrl Pts',(0.0022922664857667,-0.0344746925050311,
0.0740272984192179));
#102042=CARTESIAN_POINT('Ctrl Pts',(0.0022950639292801,-0.034364806625326,
0.0739469825954044));
#102043=CARTESIAN_POINT('Ctrl Pts',(0.00237503423069861,-0.0346945769586885,
0.074264800818384));
#102044=CARTESIAN_POINT('Ctrl Pts',(0.00237345221739543,-0.0345846629176052,
0.0741855801657686));
#102045=CARTESIAN_POINT('Ctrl Pts',(0.0023735081844425,-0.0344746925050311,
0.0741063132666856));
#102046=CARTESIAN_POINT('Ctrl Pts',(0.0023752016406758,-0.034364806625326,
0.0740271016867243));
#102047=CARTESIAN_POINT('Origin',(0.0191864882751684,-0.0345626446732421,
0.0741147837526571));
#102048=CARTESIAN_POINT('Ctrl Pts',(0.00237354227162475,-0.0346945769586885,
0.0742634277099163));
#102049=CARTESIAN_POINT('Ctrl Pts',(0.00237116648282662,-0.034527515336289,
0.0741429866324923));
#102050=CARTESIAN_POINT('Ctrl Pts',(0.00237257784055434,-0.0343603235965158,
0.0740224396864657));
#102051=CARTESIAN_POINT('Ctrl Pts',(0.00237776687175778,-0.0341934961088739,
0.0739021433341527));
#102052=CARTESIAN_POINT('Ctrl Pts',(0.00237701691262604,-0.0346945769586885,
0.0743471890088627));
#102053=CARTESIAN_POINT('Ctrl Pts',(0.0023728867098853,-0.034527515336289,
0.0742268207091856));
#102054=CARTESIAN_POINT('Ctrl Pts',(0.00237254091109597,-0.0343603235965158,
0.0741062913850263));
#102055=CARTESIAN_POINT('Ctrl Pts',(0.00237597524087146,-0.0341934961088739,
0.0739859575238226));
#102056=CARTESIAN_POINT('Ctrl Pts',(0.00238049155362732,-0.0346945769586885,
0.074430950307809));
#102057=CARTESIAN_POINT('Ctrl Pts',(0.00237460693694399,-0.034527515336289,
0.0743106547858789));
#102058=CARTESIAN_POINT('Ctrl Pts',(0.00237250398163759,-0.0343603235965158,
0.0741901430835869));
#102059=CARTESIAN_POINT('Ctrl Pts',(0.00237418360998514,-0.0341934961088739,
0.0740697717134926));
#102060=CARTESIAN_POINT('Ctrl Pts',(0.0023839661946286,-0.0346945769586885,
0.0745147116067554));
#102061=CARTESIAN_POINT('Ctrl Pts',(0.00237632716400267,-0.034527515336289,
0.0743944888625722));
#102062=CARTESIAN_POINT('Ctrl Pts',(0.00237246705217922,-0.0343603235965158,
0.0742739947821475));
#102063=CARTESIAN_POINT('Ctrl Pts',(0.00237239197909882,-0.0341934961088739,
0.0741535859031625));
#102064=CARTESIAN_POINT('Ctrl Pts',(0.00237520152298843,-0.0340223579322365,
0.0740271332457414));
#102065=CARTESIAN_POINT('Ctrl Pts',(0.00237689617597959,-0.0339125849573554,
0.0739478453253734));
#102066=CARTESIAN_POINT('Ctrl Pts',(0.00238023071386964,-0.0338030433565221,
0.0738686481950882));
#102067=CARTESIAN_POINT('Ctrl Pts',(0.00238519189432022,-0.0336938721132328,
0.0737896427566524));
#102068=CARTESIAN_POINT('Ctrl Pts',(0.00229171312078655,-0.0340223579322365,
0.0741037548257835));
#102069=CARTESIAN_POINT('Ctrl Pts',(0.00229235096235146,-0.0339125849573554,
0.0740233153826023));
#102070=CARTESIAN_POINT('Ctrl Pts',(0.00229465326527089,-0.0338030433565221,
0.0739429456651248));
#102071=CARTESIAN_POINT('Ctrl Pts',(0.00229860797433296,-0.0336938721132328,
0.0738627481916762));
#102072=CARTESIAN_POINT('Ctrl Pts',(0.00220822471858466,-0.0340223579322365,
0.0741803764058257));
#102073=CARTESIAN_POINT('Ctrl Pts',(0.00220780574872334,-0.0339125849573554,
0.0740987854398313));
#102074=CARTESIAN_POINT('Ctrl Pts',(0.00220907581667214,-0.0338030433565221,
0.0740172431351613));
#102075=CARTESIAN_POINT('Ctrl Pts',(0.0022120240543457,-0.0336938721132328,
0.0739358536267));
#102076=CARTESIAN_POINT('Ctrl Pts',(0.00212473631638278,-0.0340223579322365,
0.0742569979858679));
#102077=CARTESIAN_POINT('Ctrl Pts',(0.00212326053509521,-0.0339125849573554,
0.0741742554970602));
#102078=CARTESIAN_POINT('Ctrl Pts',(0.00212349836807339,-0.0338030433565221,
0.0740915406051979));
#102079=CARTESIAN_POINT('Ctrl Pts',(0.00212544013435845,-0.0336938721132328,
0.0740089590617238));
#102080=CARTESIAN_POINT('Origin',(0.019043056228323,-0.0345589643414795,
0.073637537917189));
#102081=CARTESIAN_POINT('Ctrl Pts',(0.00214397671962884,-0.034193496108874,
0.0736581397562618));
#102082=CARTESIAN_POINT('Ctrl Pts',(0.00215075918112192,-0.0340836138581107,
0.0735756817798827));
#102083=CARTESIAN_POINT('Ctrl Pts',(0.00215924468306331,-0.0339738896643499,
0.0734934037171999));
#102084=CARTESIAN_POINT('Ctrl Pts',(0.00216941530589721,-0.0338644633294062,
0.0734114101459476));
#102085=CARTESIAN_POINT('Ctrl Pts',(0.00222237448426191,-0.034193496108874,
0.0737399624288377));
#102086=CARTESIAN_POINT('Ctrl Pts',(0.00222802865955363,-0.0340836138581107,
0.0736585855112076));
#102087=CARTESIAN_POINT('Ctrl Pts',(0.00223536404642415,-0.0339738896643499,
0.073577364641046));
#102088=CARTESIAN_POINT('Ctrl Pts',(0.00224436428802624,-0.0338644633294062,
0.0734964031416869));
#102089=CARTESIAN_POINT('Ctrl Pts',(0.00230077224889499,-0.034193496108874,
0.0738217851014136));
#102090=CARTESIAN_POINT('Ctrl Pts',(0.00230529813798535,-0.0340836138581107,
0.0737414892425325));
#102091=CARTESIAN_POINT('Ctrl Pts',(0.002311483409785,-0.0339738896643499,
0.0736613255648921));
#102092=CARTESIAN_POINT('Ctrl Pts',(0.00231931327015528,-0.0338644633294062,
0.0735813961374263));
#102093=CARTESIAN_POINT('Ctrl Pts',(0.00237917001352806,-0.034193496108874,
0.0739036077739895));
#102094=CARTESIAN_POINT('Ctrl Pts',(0.00238256761641706,-0.0340836138581106,
0.0738243929738574));
#102095=CARTESIAN_POINT('Ctrl Pts',(0.00238760277314584,-0.0339738896643499,
0.0737452864887382));
#102096=CARTESIAN_POINT('Ctrl Pts',(0.00239426225228432,-0.0338644633294062,
0.0736663891331656));
#102097=CARTESIAN_POINT('Origin',(0.0191112172097644,-0.0345610621863715,
0.0741138824269738));
#102098=CARTESIAN_POINT('Ctrl Pts',(0.00237632147479038,-0.0342436276873899,
0.0739382919666322));
#102099=CARTESIAN_POINT('Ctrl Pts',(0.00238430617489815,-0.0339430054201859,
0.073721522912162));
#102100=CARTESIAN_POINT('Ctrl Pts',(0.00240859612467587,-0.0336441434784161,
0.073505971116179));
#102101=CARTESIAN_POINT('Ctrl Pts',(0.00237255094213417,-0.0342436276873899,
0.074188263531182));
#102102=CARTESIAN_POINT('Ctrl Pts',(0.00237110780926533,-0.0339430054201859,
0.0739713522687283));
#102103=CARTESIAN_POINT('Ctrl Pts',(0.00238600742123956,-0.0336441434784161,
0.0737549485257507));
#102104=CARTESIAN_POINT('Ctrl Pts',(0.0023942600460587,-0.0335235895815127,
0.0736664167766149));
#102105=CARTESIAN_POINT('Ctrl Pts',(0.00240091752121627,-0.0334144449262716,
0.0735875386238706));
#102106=CARTESIAN_POINT('Ctrl Pts',(0.00240921220827948,-0.0333049234473127,
0.0735087073881116));
#102107=CARTESIAN_POINT('Ctrl Pts',(0.00241914263187613,-0.033195164038858,
0.0734300248310558));
#102108=CARTESIAN_POINT('Ctrl Pts',(0.00230612527304964,-0.0335235895815127,
0.0737376448207616));
#102109=CARTESIAN_POINT('Ctrl Pts',(0.00231180215394443,-0.0334144449262716,
0.0736575533193455));
#102110=CARTESIAN_POINT('Ctrl Pts',(0.00231914018703127,-0.0333049234473127,
0.0735774870825845));
#102111=CARTESIAN_POINT('Ctrl Pts',(0.00232813926325428,-0.033195164038858,
0.0734975493405749));
#102112=CARTESIAN_POINT('Ctrl Pts',(0.00221799050004059,-0.0335235895815127,
0.0738088728649083));
#102113=CARTESIAN_POINT('Ctrl Pts',(0.0022226867866726,-0.0334144449262716,
0.0737275680148203));
#102114=CARTESIAN_POINT('Ctrl Pts',(0.00222906816578306,-0.0333049234473127,
0.0736462667770574));
#102115=CARTESIAN_POINT('Ctrl Pts',(0.00223713589463243,-0.033195164038858,
0.0735650738500941));
#102116=CARTESIAN_POINT('Ctrl Pts',(0.00212985572703154,-0.0335235895815127,
0.073880100909055));
#102117=CARTESIAN_POINT('Ctrl Pts',(0.00213357141940076,-0.0334144449262716,
0.0737975827102952));
#102118=CARTESIAN_POINT('Ctrl Pts',(0.00213899614453485,-0.0333049234473127,
0.0737150464715303));
#102119=CARTESIAN_POINT('Ctrl Pts',(0.00214613252601059,-0.033195164038858,
0.0736325983596132));
#102120=CARTESIAN_POINT('Origin',(0.0188424655511459,-0.0326434571768116,
0.0762699729563738));
#102121=CARTESIAN_POINT('Ctrl Pts',(0.00218535261375798,-0.03369387211324,
0.0732820860263534));
#102122=CARTESIAN_POINT('Ctrl Pts',(0.00219043280225018,-0.0336474569764963,
0.0732473264274453));
#102123=CARTESIAN_POINT('Ctrl Pts',(0.00219591954763718,-0.033601104548885,
0.0732126286803076));
#102124=CARTESIAN_POINT('Ctrl Pts',(0.00220981072487708,-0.0334837508643174,
0.0731247819658497));
#102125=CARTESIAN_POINT('Ctrl Pts',(0.00222629888230992,-0.0333660264760431,
0.0730373854515563));
#102126=CARTESIAN_POINT('Ctrl Pts',(0.00240466836925891,-0.03369387211324,
0.0735418371354195));
#102127=CARTESIAN_POINT('Ctrl Pts',(0.00240822814831518,-0.0336474569764963,
0.073508361264405));
#102128=CARTESIAN_POINT('Ctrl Pts',(0.00241217956078985,-0.033601104548885,
0.073474929358887));
#102129=CARTESIAN_POINT('Ctrl Pts',(0.00242218362825825,-0.0334837508643174,
0.073390287464237));
#102130=CARTESIAN_POINT('Ctrl Pts',(0.00243469141740008,-0.0333660264760431,
0.073305979179314));
#102131=CARTESIAN_POINT('Ctrl Pts',(0.00240466836926948,-0.0336938721132426,
0.0735418371354243));
#102132=CARTESIAN_POINT('Ctrl Pts',(0.00240822814832549,-0.0336474569765026,
0.0735083612644123));
#102133=CARTESIAN_POINT('Ctrl Pts',(0.00241217956079984,-0.0336011045488949,
0.073474929358897));
#102134=CARTESIAN_POINT('Ctrl Pts',(0.00242210030801232,-0.0334847282606778,
0.0733909924159425));
#102135=CARTESIAN_POINT('Ctrl Pts',(0.00243448329033809,-0.0333679869945434,
0.0733073832455932));
#102136=CARTESIAN_POINT('Ctrl Pts',(0.00240466836925872,-0.0336938721132425,
0.0735418371354214));
#102137=CARTESIAN_POINT('Ctrl Pts',(0.00241739971452264,-0.0335278710435082,
0.0734221126061285));
#102138=CARTESIAN_POINT('Ctrl Pts',(0.00243388111103953,-0.0333620469224319,
0.0733028294473244));
#102139=CARTESIAN_POINT('Ctrl Pts',(0.00245414059620915,-0.0331951640388601,
0.0731839310776603));
#102140=CARTESIAN_POINT('Ctrl Pts',(0.00239761753648507,-0.0336938721132425,
0.0736253734483665));
#102141=CARTESIAN_POINT('Ctrl Pts',(0.00240860012380252,-0.0335278710435082,
0.0735055013162));
#102142=CARTESIAN_POINT('Ctrl Pts',(0.00242333800636967,-0.0333620469224319,
0.0733860157658541));
#102143=CARTESIAN_POINT('Ctrl Pts',(0.00244185838815389,-0.0331951640388601,
0.0732668598253209));
#102144=CARTESIAN_POINT('Ctrl Pts',(0.00239056670371142,-0.0336938721132425,
0.0737089097613116));
#102145=CARTESIAN_POINT('Ctrl Pts',(0.0023998005330824,-0.0335278710435082,
0.0735888900262716));
#102146=CARTESIAN_POINT('Ctrl Pts',(0.00241279490169981,-0.0333620469224319,
0.0734692020843839));
#102147=CARTESIAN_POINT('Ctrl Pts',(0.00242957618009863,-0.0331951640388601,
0.0733497885729815));
#102148=CARTESIAN_POINT('Ctrl Pts',(0.00238351587093777,-0.0336938721132425,
0.0737924460742568));
#102149=CARTESIAN_POINT('Ctrl Pts',(0.00239100094236228,-0.0335278710435082,
0.0736722787363431));
#102150=CARTESIAN_POINT('Ctrl Pts',(0.00240225179702995,-0.0333620469224319,
0.0735523884029136));
#102151=CARTESIAN_POINT('Ctrl Pts',(0.00241729397204338,-0.0331951640388601,
0.0734327173206421));
#102152=CARTESIAN_POINT('Ctrl Pts',(0.00243592986201132,-0.0330240426238155,
0.0733076125359522));
#102153=CARTESIAN_POINT('Ctrl Pts',(0.00244753457002689,-0.0329142774063506,
0.0732292568286855));
#102154=CARTESIAN_POINT('Ctrl Pts',(0.00246076489475772,-0.032804347972668,
0.0731511019599719));
#102155=CARTESIAN_POINT('Ctrl Pts',(0.0024756066445203,-0.0326943950436586,
0.0730732485187923));
#102156=CARTESIAN_POINT('Ctrl Pts',(0.00234349669882086,-0.0330240426238155,
0.0733731659212745));
#102157=CARTESIAN_POINT('Ctrl Pts',(0.00235419834508804,-0.0329142774063506,
0.0732935368571316));
#102158=CARTESIAN_POINT('Ctrl Pts',(0.00236655148170485,-0.032804347972668,
0.0732140893279181));
#102159=CARTESIAN_POINT('Ctrl Pts',(0.00238054308633687,-0.0326943950436586,
0.0731349255476614));
#102160=CARTESIAN_POINT('Ctrl Pts',(0.0022510635356304,-0.0330240426238155,
0.0734387193065969));
#102161=CARTESIAN_POINT('Ctrl Pts',(0.0022608621201492,-0.0329142774063506,
0.0733578168855778));
#102162=CARTESIAN_POINT('Ctrl Pts',(0.00227233806865199,-0.032804347972668,
0.0732770766958643));
#102163=CARTESIAN_POINT('Ctrl Pts',(0.00228547952815344,-0.0326943950436586,
0.0731966025765306));
#102164=CARTESIAN_POINT('Ctrl Pts',(0.00215863037243994,-0.0330240426238155,
0.0735042726919192));
#102165=CARTESIAN_POINT('Ctrl Pts',(0.00216752589521035,-0.0329142774063506,
0.0734220969140239));
#102166=CARTESIAN_POINT('Ctrl Pts',(0.00217812465559913,-0.032804347972668,
0.0733400640638104));
#102167=CARTESIAN_POINT('Ctrl Pts',(0.00219041596997002,-0.0326943950436586,
0.0732582796053997));
#102168=CARTESIAN_POINT('Origin',(0.0189642957816681,-0.0326396682857656,
0.0762912519078639));
#102169=CARTESIAN_POINT('Ctrl Pts',(0.00225277570667803,-0.0331951640388587,
0.0729125498651186));
#102170=CARTESIAN_POINT('Ctrl Pts',(0.00226981907894478,-0.0330855618255041,
0.0728316886277174));
#102171=CARTESIAN_POINT('Ctrl Pts',(0.00228854600109696,-0.0329757224427708,
0.0727511213559523));
#102172=CARTESIAN_POINT('Ctrl Pts',(0.00230893755295068,-0.0328657862078596,
0.072670952397367));
#102173=CARTESIAN_POINT('Ctrl Pts',(0.00232030016243826,-0.0331951640388587,
0.0730035531612891));
#102174=CARTESIAN_POINT('Ctrl Pts',(0.00233609014839843,-0.0330855618255041,
0.0729236219366652));
#102175=CARTESIAN_POINT('Ctrl Pts',(0.00235354355892097,-0.0329757224427708,
0.072843959442758));
#102176=CARTESIAN_POINT('Ctrl Pts',(0.00237264304779727,-0.0328657862078596,
0.0727646687884945));
#102177=CARTESIAN_POINT('Ctrl Pts',(0.00238782461819848,-0.0331951640388587,
0.0730945564574596));
#102178=CARTESIAN_POINT('Ctrl Pts',(0.00240236121785207,-0.0330855618255041,
0.0730155552456129));
#102179=CARTESIAN_POINT('Ctrl Pts',(0.00241854111674499,-0.0329757224427708,
0.0729367975295637));
#102180=CARTESIAN_POINT('Ctrl Pts',(0.00243634854264385,-0.0328657862078596,
0.072858385179622));
#102181=CARTESIAN_POINT('Ctrl Pts',(0.0024553490739587,-0.0331951640388587,
0.0731855597536301));
#102182=CARTESIAN_POINT('Ctrl Pts',(0.00246863228730572,-0.0330855618255041,
0.0731074885545606));
#102183=CARTESIAN_POINT('Ctrl Pts',(0.002483538674569,-0.0329757224427708,
0.0730296356163694));
#102184=CARTESIAN_POINT('Ctrl Pts',(0.00250005403749043,-0.0328657862078596,
0.0729521015707495));
#102185=CARTESIAN_POINT('Origin',(0.0188335865984539,-0.0326401908830343,
0.0767540563823664));
#102186=CARTESIAN_POINT('Ctrl Pts',(0.00244818769528571,-0.0332451089994432,
0.0732195419964954));
#102187=CARTESIAN_POINT('Ctrl Pts',(0.00248328049303606,-0.0329451141710258,
0.073005483447829));
#102188=CARTESIAN_POINT('Ctrl Pts',(0.00253439736081545,-0.0326442513127503,
0.0727946763498947));
#102189=CARTESIAN_POINT('Ctrl Pts',(0.00241311403098397,-0.0332451089994432,
0.0734670694456246));
#102190=CARTESIAN_POINT('Ctrl Pts',(0.00243887117825119,-0.0329451141710258,
0.0732516880720666));
#102191=CARTESIAN_POINT('Ctrl Pts',(0.00248077855772377,-0.0326442513127503,
0.0730388587078877));
#102192=CARTESIAN_POINT('Ctrl Pts',(0.00250004736902662,-0.0325229783203384,
0.0729521324465009));
#102193=CARTESIAN_POINT('Ctrl Pts',(0.0025165599467554,-0.0324130253112079,
0.0728746093863449));
#102194=CARTESIAN_POINT('Ctrl Pts',(0.00253467368408381,-0.0323031222247695,
0.0727974396679559));
#102195=CARTESIAN_POINT('Ctrl Pts',(0.00255436189055012,-0.0321934096636184,
0.0727207213215165));
#102196=CARTESIAN_POINT('Ctrl Pts',(0.0024036804549877,-0.0325229783203384,
0.0730117525817576));
#102197=CARTESIAN_POINT('Ctrl Pts',(0.00241937117047073,-0.0324130253112079,
0.0729329011058233));
#102198=CARTESIAN_POINT('Ctrl Pts',(0.00243669065019125,-0.0323031222247695,
0.07285438617186));
#102199=CARTESIAN_POINT('Ctrl Pts',(0.0024556131602716,-0.0321934096636184,
0.0727763075690764));
#102200=CARTESIAN_POINT('Ctrl Pts',(0.00230731354094878,-0.0325229783203384,
0.0730713727170144));
#102201=CARTESIAN_POINT('Ctrl Pts',(0.00232218239418606,-0.0324130253112079,
0.0729911928253016));
#102202=CARTESIAN_POINT('Ctrl Pts',(0.00233870761629869,-0.0323031222247695,
0.0729113326757642));
#102203=CARTESIAN_POINT('Ctrl Pts',(0.00235686442999307,-0.0321934096636184,
0.0728318938166364));
#102204=CARTESIAN_POINT('Ctrl Pts',(0.00221094662690986,-0.0325229783203384,
0.0731309928522712));
#102205=CARTESIAN_POINT('Ctrl Pts',(0.0022249936179014,-0.0324130253112079,
0.07304948454478));
#102206=CARTESIAN_POINT('Ctrl Pts',(0.00224072458240613,-0.0323031222247695,
0.0729682791796684));
#102207=CARTESIAN_POINT('Ctrl Pts',(0.00225811569971455,-0.0321934096636184,
0.0728874800641964));
#102208=CARTESIAN_POINT('Origin',(0.0189559809570794,-0.0326393375178101,
0.0762893665114488));
#102209=CARTESIAN_POINT('Ctrl Pts',(0.00234206093373601,-0.0326943950436593,
0.0725463481428483));
#102210=CARTESIAN_POINT('Ctrl Pts',(0.0023641622618914,-0.0325844576448127,
0.0724666651877939));
#102211=CARTESIAN_POINT('Ctrl Pts',(0.00238791312834463,-0.0324744968375319,
0.0723874336851549));
#102212=CARTESIAN_POINT('Ctrl Pts',(0.0024132817018894,-0.0323646534831894,
0.072308754731218));
#102213=CARTESIAN_POINT('Ctrl Pts',(0.00240373794242499,-0.0326943950436593,
0.0726414116699278));
#102214=CARTESIAN_POINT('Ctrl Pts',(0.00242452911700918,-0.0325844576448127,
0.0725625787396482));
#102215=CARTESIAN_POINT('Ctrl Pts',(0.00244695215726364,-0.0324744968375319,
0.0724841702258176));
#102216=CARTESIAN_POINT('Ctrl Pts',(0.00247097694781462,-0.0323646534831894,
0.0724062861937275));
#102217=CARTESIAN_POINT('Ctrl Pts',(0.00246541495111396,-0.0326943950436593,
0.0727364751970073));
#102218=CARTESIAN_POINT('Ctrl Pts',(0.00248489597212697,-0.0325844576448127,
0.0726584922915024));
#102219=CARTESIAN_POINT('Ctrl Pts',(0.00250599118618266,-0.0324744968375319,
0.0725809067664803));
#102220=CARTESIAN_POINT('Ctrl Pts',(0.00252867219373984,-0.0323646534831894,
0.0725038176562369));
#102221=CARTESIAN_POINT('Ctrl Pts',(0.00252709195980294,-0.0326943950436593,
0.0728315387240867));
#102222=CARTESIAN_POINT('Ctrl Pts',(0.00254526282724476,-0.0325844576448127,
0.0727544058433566));
#102223=CARTESIAN_POINT('Ctrl Pts',(0.00256503021510168,-0.0324744968375319,
0.072677643307143));
#102224=CARTESIAN_POINT('Ctrl Pts',(0.00258636743966506,-0.0323646534831894,
0.0726013491187464));
#102225=CARTESIAN_POINT('Origin',(0.0188704620442487,-0.0326395579068987,
0.0767625512829897));
#102226=CARTESIAN_POINT('Ctrl Pts',(0.00251780236267085,-0.0327445246961877,
0.0728650427475093));
#102227=CARTESIAN_POINT('Ctrl Pts',(0.00256626531720569,-0.0324436878365475,
0.0726536097639458));
#102228=CARTESIAN_POINT('Ctrl Pts',(0.00263051658990176,-0.0321434074463187,
0.0724464278669139));
#102229=CARTESIAN_POINT('Ctrl Pts',(0.00246725720085306,-0.0327445246961877,
0.0731098798088722));
#102230=CARTESIAN_POINT('Ctrl Pts',(0.00250648597475639,-0.0324436878365475,
0.0728965404833861));
#102231=CARTESIAN_POINT('Ctrl Pts',(0.00256167289361573,-0.0321434074463187,
0.072686762103929));
#102232=CARTESIAN_POINT('Ctrl Pts',(0.0026111396246973,-0.0322357242816073,
0.0725102143698205));
#102233=CARTESIAN_POINT('Ctrl Pts',(0.00266336467029447,-0.0319819883628706,
0.0723346438536521));
#102234=CARTESIAN_POINT('Ctrl Pts',(0.00272665592956285,-0.0317295851069887,
0.0721627523819745));
#102235=CARTESIAN_POINT('Ctrl Pts',(0.00254508625065872,-0.0322357242816073,
0.0727513304244044));
#102236=CARTESIAN_POINT('Ctrl Pts',(0.00258963206263345,-0.0319819883628706,
0.072573656193941));
#102237=CARTESIAN_POINT('Ctrl Pts',(0.002645393516558,-0.0317295851069887,
0.0723991766198027));
#102238=CARTESIAN_POINT('Origin',(0.0187782749196005,-0.0326371942644775,
0.0767383864827326));
#102239=CARTESIAN_POINT('Origin',(0.0188361706893204,-0.0326352985529264,
0.0762627337746027));
#102240=CARTESIAN_POINT('Ctrl Pts',(0.00245416397318719,-0.0321934096636183,
0.0721864753018188));
#102241=CARTESIAN_POINT('Ctrl Pts',(0.00248124250905315,-0.0320835708272303,
0.0721082868479344));
#102242=CARTESIAN_POINT('Ctrl Pts',(0.00250992344425711,-0.0319739230346346,
0.0720307041354232));
#102243=CARTESIAN_POINT('Ctrl Pts',(0.00254016246547428,-0.0318646057455575,
0.071953823609724));
#102244=CARTESIAN_POINT('Ctrl Pts',(0.00250975026861318,-0.0321934096636183,
0.0722852241171311));
#102245=CARTESIAN_POINT('Ctrl Pts',(0.00253546698135585,-0.0320835708272303,
0.072207802241582));
#102246=CARTESIAN_POINT('Ctrl Pts',(0.00256277101905045,-0.0319739230346346,
0.0721309574799007));
#102247=CARTESIAN_POINT('Ctrl Pts',(0.00259161990247846,-0.0318646057455575,
0.0720547854685705));
#102248=CARTESIAN_POINT('Ctrl Pts',(0.00256533656403917,-0.0321934096636183,
0.0723839729324434));
#102249=CARTESIAN_POINT('Ctrl Pts',(0.00258969145365854,-0.0320835708272303,
0.0723073176352295));
#102250=CARTESIAN_POINT('Ctrl Pts',(0.00261561859384379,-0.0319739230346346,
0.0722312108243781));
#102251=CARTESIAN_POINT('Ctrl Pts',(0.00264307733948264,-0.0318646057455575,
0.0721557473274169));
#102252=CARTESIAN_POINT('Ctrl Pts',(0.00262092285946516,-0.0321934096636183,
0.0724827217477557));
#102253=CARTESIAN_POINT('Ctrl Pts',(0.00264391592596123,-0.0320835708272303,
0.0724068330288771));
#102254=CARTESIAN_POINT('Ctrl Pts',(0.00266846616863713,-0.0319739230346346,
0.0723314641688556));
#102255=CARTESIAN_POINT('Ctrl Pts',(0.00269453477648683,-0.0318646057455575,
0.0722567091862634));
#102256=CARTESIAN_POINT('Ctrl Pts',(0.00258544407064685,-0.0320218834582398,
0.07260157866145));
#102257=CARTESIAN_POINT('Ctrl Pts',(0.00260155939349681,-0.0319391099350682,
0.0725439379504409));
#102258=CARTESIAN_POINT('Ctrl Pts',(0.00261856502026669,-0.0318564869454951,
0.0724865838055));
#102259=CARTESIAN_POINT('Ctrl Pts',(0.00263644466463766,-0.0317740741446532,
0.0724295568451632));
#102260=CARTESIAN_POINT('Ctrl Pts',(0.00254173679643626,-0.0320218834582398,
0.0726249560485665));
#102261=CARTESIAN_POINT('Ctrl Pts',(0.00255760881720081,-0.0319391099350682,
0.0725668604504945));
#102262=CARTESIAN_POINT('Ctrl Pts',(0.0025743783924211,-0.0318564869454951,
0.0725090478948991));
#102263=CARTESIAN_POINT('Ctrl Pts',(0.00259202937653946,-0.0317740741446532,
0.0724515593502585));
#102264=CARTESIAN_POINT('Ctrl Pts',(0.00249802952222568,-0.0320218834582398,
0.0726483334356829));
#102265=CARTESIAN_POINT('Ctrl Pts',(0.00251365824090481,-0.0319391099350682,
0.0725897829505481));
#102266=CARTESIAN_POINT('Ctrl Pts',(0.0025301917645755,-0.0318564869454951,
0.0725315119842981));
#102267=CARTESIAN_POINT('Ctrl Pts',(0.00254761408844127,-0.0317740741446532,
0.0724735618553538));
#102268=CARTESIAN_POINT('Ctrl Pts',(0.00245432224801509,-0.0320218834582398,
0.0726717108227994));
#102269=CARTESIAN_POINT('Ctrl Pts',(0.00246970766460881,-0.0319391099350682,
0.0726127054506017));
#102270=CARTESIAN_POINT('Ctrl Pts',(0.00248600513672991,-0.0318564869454951,
0.0725539760736971));
#102271=CARTESIAN_POINT('Ctrl Pts',(0.00250319880034307,-0.0317740741446532,
0.072495564360449));
#102272=CARTESIAN_POINT('Origin',(-0.00372643980148012,-0.039122885339058,
0.071814864670307));
#102273=CARTESIAN_POINT('Ctrl Pts',(0.00256742115659057,-0.0352722978779646,
0.0756369487464146));
#102274=CARTESIAN_POINT('Ctrl Pts',(0.0025628750924334,-0.0352466642097251,
0.0756186068277919));
#102275=CARTESIAN_POINT('Ctrl Pts',(0.00255825697983851,-0.0352210183808318,
0.0756003001107925));
#102276=CARTESIAN_POINT('Ctrl Pts',(0.00255356613949293,-0.0351953608940152,
0.0755820280796471));
#102277=CARTESIAN_POINT('Origin',(-0.00222897559393711,-0.0352456003065129,
0.0766391071207262));
#102278=CARTESIAN_POINT('Ctrl Pts',(0.00252524734178226,-0.0350241211493339,
0.0754606058365681));
#102279=CARTESIAN_POINT('Ctrl Pts',(0.00250719428456688,-0.0349144232867421,
0.075383488317957));
#102280=CARTESIAN_POINT('Ctrl Pts',(0.00249072449587003,-0.0348045283677512,
0.0753059514712201));
#102281=CARTESIAN_POINT('Ctrl Pts',(0.00247586276713219,-0.0346945769586886,
0.0752280938261766));
#102282=CARTESIAN_POINT('Ctrl Pts',(0.00246343695443706,-0.0350241211493339,
0.0755555827696585));
#102283=CARTESIAN_POINT('Ctrl Pts',(0.0024440756289694,-0.0349144232867421,
0.0754776138383434));
#102284=CARTESIAN_POINT('Ctrl Pts',(0.0024263143882669,-0.0348045283677512,
0.0753991980264526));
#102285=CARTESIAN_POINT('Ctrl Pts',(0.00241017971985099,-0.0346945769586886,
0.0753204349280917));
#102286=CARTESIAN_POINT('Ctrl Pts',(0.00240162656709186,-0.0350241211493339,
0.075650559702749));
#102287=CARTESIAN_POINT('Ctrl Pts',(0.00238095697337193,-0.0349144232867421,
0.0755717393587299));
#102288=CARTESIAN_POINT('Ctrl Pts',(0.00236190428066376,-0.0348045283677512,
0.0754924445816851));
#102289=CARTESIAN_POINT('Ctrl Pts',(0.00234449667256979,-0.0346945769586886,
0.0754127760300068));
#102290=CARTESIAN_POINT('Ctrl Pts',(0.00233981617974666,-0.0350241211493339,
0.0757455366358395));
#102291=CARTESIAN_POINT('Ctrl Pts',(0.00231783831777446,-0.0349144232867421,
0.0756658648791163));
#102292=CARTESIAN_POINT('Ctrl Pts',(0.00229749417306063,-0.0348045283677512,
0.0755856911369176));
#102293=CARTESIAN_POINT('Ctrl Pts',(0.0022788136252886,-0.0346945769586886,
0.0755051171319219));
#102294=CARTESIAN_POINT('Origin',(0.0189997036149989,-0.0345629067943529,
0.0722572971807028));
#102295=CARTESIAN_POINT('Ctrl Pts',(0.00228856946677351,-0.035197097365162,
0.0752110439272844));
#102296=CARTESIAN_POINT('Ctrl Pts',(0.00227387014112994,-0.0350869349321768,
0.0751302049630735));
#102297=CARTESIAN_POINT('Ctrl Pts',(0.00226083923600357,-0.034976498512971,
0.0750489934419713));
#102298=CARTESIAN_POINT('Ctrl Pts',(0.00224949982670333,-0.034865930684962,
0.0749675135821197));
#102299=CARTESIAN_POINT('Ctrl Pts',(0.00235844150412178,-0.035197097365162,
0.0752543840824171));
#102300=CARTESIAN_POINT('Ctrl Pts',(0.00234314175936515,-0.0350869349321768,
0.0751745131005903));
#102301=CARTESIAN_POINT('Ctrl Pts',(0.00232948981392817,-0.034976498512971,
0.0750942578813569));
#102302=CARTESIAN_POINT('Ctrl Pts',(0.00231750947476583,-0.034865930684962,
0.0750137213565797));
#102303=CARTESIAN_POINT('Ctrl Pts',(0.00242831354147005,-0.035197097365162,
0.0752977242375498));
#102304=CARTESIAN_POINT('Ctrl Pts',(0.00241241337760036,-0.0350869349321768,
0.0752188212381071));
#102305=CARTESIAN_POINT('Ctrl Pts',(0.00239814039185277,-0.034976498512971,
0.0751395223207425));
#102306=CARTESIAN_POINT('Ctrl Pts',(0.00238551912282833,-0.034865930684962,
0.0750599291310396));
#102307=CARTESIAN_POINT('Ctrl Pts',(0.00249818557881832,-0.035197097365162,
0.0753410643926826));
#102308=CARTESIAN_POINT('Ctrl Pts',(0.00248168499583556,-0.0350869349321768,
0.075263129375624));
#102309=CARTESIAN_POINT('Ctrl Pts',(0.00246679096977737,-0.034976498512971,
0.0751847867601281));
#102310=CARTESIAN_POINT('Ctrl Pts',(0.00245352877089082,-0.034865930684962,
0.0751061369054996));
#102311=CARTESIAN_POINT('Origin',(0.019037000149744,-0.0345637187967391,
0.0727368118570569));
#102312=CARTESIAN_POINT('Ctrl Pts',(0.00250422216522004,-0.0352450361861252,
0.0753742018187211));
#102313=CARTESIAN_POINT('Ctrl Pts',(0.0024580506371754,-0.0349452761023765,
0.0751622566398639));
#102314=CARTESIAN_POINT('Ctrl Pts',(0.0024279748552457,-0.0346444289983475,
0.0749474357465967));
#102315=CARTESIAN_POINT('Ctrl Pts',(0.00256273217342888,-0.0352450361861252,
0.0756172585588856));
#102316=CARTESIAN_POINT('Ctrl Pts',(0.00250739361024074,-0.0349452761023765,
0.0754075201211421));
#102317=CARTESIAN_POINT('Ctrl Pts',(0.00246801061498241,-0.0346444289983475,
0.0751942092012921));
#102318=CARTESIAN_POINT('Ctrl Pts',(0.00245400125847058,-0.0345231616327822,
0.0751064857114735));
#102319=CARTESIAN_POINT('Ctrl Pts',(0.00244081744956218,-0.0344132092796975,
0.0750283357637031));
#102320=CARTESIAN_POINT('Ctrl Pts',(0.00242925079090351,-0.0343032738558974,
0.0749499171514227));
#102321=CARTESIAN_POINT('Ctrl Pts',(0.00241931352731584,-0.0341934961088741,
0.0748713307175119));
#102322=CARTESIAN_POINT('Ctrl Pts',(0.00238634921831221,-0.0345231616327822,
0.0751973941137306));
#102323=CARTESIAN_POINT('Ctrl Pts',(0.00237191236506749,-0.0344132092796975,
0.0751183116778331));
#102324=CARTESIAN_POINT('Ctrl Pts',(0.00235911201450521,-0.0343032738558974,
0.075038934707304));
#102325=CARTESIAN_POINT('Ctrl Pts',(0.00234796196049881,-0.0341934961088741,
0.0749593653132757));
#102326=CARTESIAN_POINT('Ctrl Pts',(0.00231869717815384,-0.0345231616327822,
0.0752883025159877));
#102327=CARTESIAN_POINT('Ctrl Pts',(0.0023030072805728,-0.0344132092796975,
0.0752082875919631));
#102328=CARTESIAN_POINT('Ctrl Pts',(0.00228897323810691,-0.0343032738558974,
0.0751279522631852));
#102329=CARTESIAN_POINT('Ctrl Pts',(0.00227661039368177,-0.0341934961088741,
0.0750473999090394));
#102330=CARTESIAN_POINT('Ctrl Pts',(0.00225104513799546,-0.0345231616327822,
0.0753792109182449));
#102331=CARTESIAN_POINT('Ctrl Pts',(0.00223410219607811,-0.0344132092796975,
0.0752982635060931));
#102332=CARTESIAN_POINT('Ctrl Pts',(0.00221883446170861,-0.0343032738558974,
0.0752169698190665));
#102333=CARTESIAN_POINT('Ctrl Pts',(0.00220525882686474,-0.0341934961088741,
0.0751354345048032));
#102334=CARTESIAN_POINT('Origin',(0.0190115825377258,-0.0345625596229667,
0.0722549756521341));
#102335=CARTESIAN_POINT('Ctrl Pts',(0.00215773009560743,-0.0346945769586885,
0.074787355764023));
#102336=CARTESIAN_POINT('Ctrl Pts',(0.00214894701102897,-0.0345846629176052,
0.0747051405505901));
#102337=CARTESIAN_POINT('Ctrl Pts',(0.002141862603128,-0.0344746925050311,
0.0746227296640146));
#102338=CARTESIAN_POINT('Ctrl Pts',(0.00213648551317482,-0.0343648066253259,
0.0745402287361092));
#102339=CARTESIAN_POINT('Ctrl Pts',(0.00225007112481624,-0.0346945769586885,
0.0748530387595875));
#102340=CARTESIAN_POINT('Ctrl Pts',(0.00224038289535956,-0.0345846629176052,
0.0747720960522108));
#102341=CARTESIAN_POINT('Ctrl Pts',(0.00223236687307674,-0.0344746925050311,
0.0746909391710142));
#102342=CARTESIAN_POINT('Ctrl Pts',(0.00222603289956556,-0.0343648066253259,
0.074609672145964));
#102343=CARTESIAN_POINT('Ctrl Pts',(0.00234241215402504,-0.0346945769586885,
0.0749187217551521));
#102344=CARTESIAN_POINT('Ctrl Pts',(0.00233181877969015,-0.0345846629176052,
0.0748390515538314));
#102345=CARTESIAN_POINT('Ctrl Pts',(0.00232287114302549,-0.0344746925050311,
0.0747591486780137));
#102346=CARTESIAN_POINT('Ctrl Pts',(0.0023155802859563,-0.0343648066253259,
0.0746791155558189));
#102347=CARTESIAN_POINT('Ctrl Pts',(0.00243475318323385,-0.0346945769586885,
0.0749844047507166));
#102348=CARTESIAN_POINT('Ctrl Pts',(0.00242325466402074,-0.0345846629176052,
0.074906007055452));
#102349=CARTESIAN_POINT('Ctrl Pts',(0.00241337541297424,-0.0344746925050311,
0.0748273581850132));
#102350=CARTESIAN_POINT('Ctrl Pts',(0.00240512767234704,-0.0343648066253259,
0.0747485589656737));
#102351=CARTESIAN_POINT('Origin',(0.0190948417673933,-0.0345626446727627,
0.0727285367187088));
#102352=CARTESIAN_POINT('Ctrl Pts',(0.0024331008925787,-0.0346945769586885,
0.0749832294616745));
#102353=CARTESIAN_POINT('Ctrl Pts',(0.00241564856789733,-0.034527515336289,
0.0748640358634123));
#102354=CARTESIAN_POINT('Ctrl Pts',(0.002401940258106,-0.0343603235965158,
0.0747442625760329));
#102355=CARTESIAN_POINT('Ctrl Pts',(0.00239201124142713,-0.0341934961088739,
0.074624264438329));
#102356=CARTESIAN_POINT('Ctrl Pts',(0.00244704620944235,-0.0346945769586885,
0.0750658947897682));
#102357=CARTESIAN_POINT('Ctrl Pts',(0.0024278624263667,-0.034527515336289,
0.0749469932817511));
#102358=CARTESIAN_POINT('Ctrl Pts',(0.00241241302436789,-0.0343603235965158,
0.0748274577073935));
#102359=CARTESIAN_POINT('Ctrl Pts',(0.00240073844149539,-0.0341934961088739,
0.0747076422789716));
#102360=CARTESIAN_POINT('Ctrl Pts',(0.002460991526306,-0.0346945769586885,
0.0751485601178619));
#102361=CARTESIAN_POINT('Ctrl Pts',(0.00244007628483606,-0.034527515336289,
0.0750299507000899));
#102362=CARTESIAN_POINT('Ctrl Pts',(0.00242288579062979,-0.0343603235965158,
0.0749106528387541));
#102363=CARTESIAN_POINT('Ctrl Pts',(0.00240946564156365,-0.0341934961088739,
0.0747910201196143));
#102364=CARTESIAN_POINT('Ctrl Pts',(0.00247493684316965,-0.0346945769586885,
0.0752312254459556));
#102365=CARTESIAN_POINT('Ctrl Pts',(0.00245229014330543,-0.034527515336289,
0.0751129081184287));
#102366=CARTESIAN_POINT('Ctrl Pts',(0.00243335855689168,-0.0343603235965158,
0.0749938479701148));
#102367=CARTESIAN_POINT('Ctrl Pts',(0.00241819284163192,-0.0341934961088739,
0.074874397960257));
#102368=CARTESIAN_POINT('Ctrl Pts',(0.00240513151098137,-0.0340223579322366,
0.0747485902905886));
#102369=CARTESIAN_POINT('Ctrl Pts',(0.00239687538968521,-0.0339125849573555,
0.0746697151828158));
#102370=CARTESIAN_POINT('Ctrl Pts',(0.00239025760132036,-0.0338030433565222,
0.0745907246171416));
#102371=CARTESIAN_POINT('Ctrl Pts',(0.00238527765431292,-0.0336938721132328,
0.0745117203593975));
#102372=CARTESIAN_POINT('Ctrl Pts',(0.0023319046701551,-0.0340223579322366,
0.0748350715579995));
#102373=CARTESIAN_POINT('Ctrl Pts',(0.00232245574662875,-0.0339125849573555,
0.0747551864611081));
#102374=CARTESIAN_POINT('Ctrl Pts',(0.00231466689862988,-0.0338030433565222,
0.0746751619277885));
#102375=CARTESIAN_POINT('Ctrl Pts',(0.00230853901495878,-0.0336938721132328,
0.0745951011788974));
#102376=CARTESIAN_POINT('Ctrl Pts',(0.00225867782932883,-0.0340223579322366,
0.0749215528254104));
#102377=CARTESIAN_POINT('Ctrl Pts',(0.00224803610357228,-0.0339125849573555,
0.0748406577394004));
#102378=CARTESIAN_POINT('Ctrl Pts',(0.00223907619593939,-0.0338030433565222,
0.0747595992384354));
#102379=CARTESIAN_POINT('Ctrl Pts',(0.00223180037560463,-0.0336938721132328,
0.0746784819983972));
#102380=CARTESIAN_POINT('Ctrl Pts',(0.00218545098850257,-0.0340223579322366,
0.0750080340928213));
#102381=CARTESIAN_POINT('Ctrl Pts',(0.00217361646051582,-0.0339125849573555,
0.0749261290176926));
#102382=CARTESIAN_POINT('Ctrl Pts',(0.00216348549324891,-0.0338030433565222,
0.0748440365490823));
#102383=CARTESIAN_POINT('Ctrl Pts',(0.00215506173625048,-0.0336938721132328,
0.074761862817897));
#102384=CARTESIAN_POINT('Origin',(0.018892725961209,-0.0345589643414346,
0.0722730309108332));
#102385=CARTESIAN_POINT('Ctrl Pts',(0.00212948283705902,-0.034193496108874,
0.0744114865772719));
#102386=CARTESIAN_POINT('Ctrl Pts',(0.00212587709205058,-0.0340836138595105,
0.0743288287398881));
#102387=CARTESIAN_POINT('Ctrl Pts',(0.00212398350762951,-0.0339738896671456,
0.074246135949962));
#102388=CARTESIAN_POINT('Ctrl Pts',(0.0021237974126069,-0.0338644633335883,
0.0741635142065129));
#102389=CARTESIAN_POINT('Ctrl Pts',(0.00221751751203453,-0.034193496108874,
0.0744828382082896));
#102390=CARTESIAN_POINT('Ctrl Pts',(0.00221292787029965,-0.0340836138595105,
0.0744013943169262));
#102391=CARTESIAN_POINT('Ctrl Pts',(0.00221002574117891,-0.0339738896671456,
0.0743198945308684));
#102392=CARTESIAN_POINT('Ctrl Pts',(0.00220880784665147,-0.0338644633335883,
0.0742384434087674));
#102393=CARTESIAN_POINT('Ctrl Pts',(0.00230555218701004,-0.034193496108874,
0.0745541898393074));
#102394=CARTESIAN_POINT('Ctrl Pts',(0.00229997864854872,-0.0340836138595105,
0.0744739598939644));
#102395=CARTESIAN_POINT('Ctrl Pts',(0.00229606797472831,-0.0339738896671456,
0.0743936531117748));
#102396=CARTESIAN_POINT('Ctrl Pts',(0.00229381828069604,-0.0338644633335883,
0.0743133726110218));
#102397=CARTESIAN_POINT('Ctrl Pts',(0.00239358686198556,-0.034193496108874,
0.0746255414703251));
#102398=CARTESIAN_POINT('Ctrl Pts',(0.00238702942679779,-0.0340836138595105,
0.0745465254710025));
#102399=CARTESIAN_POINT('Ctrl Pts',(0.00238211020827771,-0.0339738896671456,
0.0744674116926812));
#102400=CARTESIAN_POINT('Ctrl Pts',(0.00237882871474061,-0.0338644633335883,
0.0743883018132763));
#102401=CARTESIAN_POINT('Origin',(0.0190200512712865,-0.0345610621861553,
0.0727370764658675));
#102402=CARTESIAN_POINT('Ctrl Pts',(0.00239510786684413,-0.03424362768739,
0.07466030918432));
#102403=CARTESIAN_POINT('Ctrl Pts',(0.00237586123867319,-0.0339430054201859,
0.0744442486703066));
#102404=CARTESIAN_POINT('Ctrl Pts',(0.00237294385135072,-0.033644143478416,
0.0742273522266683));
#102405=CARTESIAN_POINT('Ctrl Pts',(0.00242269681044828,-0.03424362768739,
0.0749087822214706));
#102406=CARTESIAN_POINT('Ctrl Pts',(0.00239407886719331,-0.0339430054201859,
0.0746937622416185));
#102407=CARTESIAN_POINT('Ctrl Pts',(0.00238173841041401,-0.033644143478416,
0.0744771974902433));
#102408=CARTESIAN_POINT('Ctrl Pts',(0.00237882999042919,-0.0335235895815127,
0.0743883295122386));
#102409=CARTESIAN_POINT('Ctrl Pts',(0.00237554891546564,-0.0334144449262719,
0.0743092389343998));
#102410=CARTESIAN_POINT('Ctrl Pts',(0.00237389802276031,-0.0333049234473133,
0.0742299897065297));
#102411=CARTESIAN_POINT('Ctrl Pts',(0.0023738886026999,-0.0331951640388588,
0.0741506829728378));
#102412=CARTESIAN_POINT('Ctrl Pts',(0.00230031742752324,-0.0335235895815127,
0.0744700421180732));
#102413=CARTESIAN_POINT('Ctrl Pts',(0.00229591141766308,-0.0334144449262719,
0.074389870660229));
#102414=CARTESIAN_POINT('Ctrl Pts',(0.00229315662781468,-0.0333049234473133,
0.0743095160702449));
#102415=CARTESIAN_POINT('Ctrl Pts',(0.00229206588794388,-0.0331951640388588,
0.0742290807778854));
#102416=CARTESIAN_POINT('Ctrl Pts',(0.00222180486461729,-0.0335235895815127,
0.0745517547239077));
#102417=CARTESIAN_POINT('Ctrl Pts',(0.00221627391986051,-0.0334144449262719,
0.0744705023860581));
#102418=CARTESIAN_POINT('Ctrl Pts',(0.00221241523286906,-0.0333049234473133,
0.0743890424339601));
#102419=CARTESIAN_POINT('Ctrl Pts',(0.00221024317318787,-0.0331951640388588,
0.074307478582933));
#102420=CARTESIAN_POINT('Ctrl Pts',(0.00214329230171133,-0.0335235895815127,
0.0746334673297422));
#102421=CARTESIAN_POINT('Ctrl Pts',(0.00213663642205794,-0.0334144449262719,
0.0745511341118873));
#102422=CARTESIAN_POINT('Ctrl Pts',(0.00213167383792343,-0.0333049234473133,
0.0744685687976754));
#102423=CARTESIAN_POINT('Ctrl Pts',(0.00212842045843185,-0.0331951640388588,
0.0743858763879806));
#102424=CARTESIAN_POINT('Origin',(0.0190236485971153,-0.0326434571770372,
0.0749098490912811));
#102425=CARTESIAN_POINT('Ctrl Pts',(0.00212340043994126,-0.0336938721132408,
0.0740332123687434));
#102426=CARTESIAN_POINT('Ctrl Pts',(0.00212408403670126,-0.0336474569764967,
0.0739980901432037));
#102427=CARTESIAN_POINT('Ctrl Pts',(0.00212517873661592,-0.033601104548885,
0.0739629783266245));
#102428=CARTESIAN_POINT('Ctrl Pts',(0.00212795026487169,-0.0334837508694616,
0.0738740832874839));
#102429=CARTESIAN_POINT('Ctrl Pts',(0.00213335472016756,-0.0333660264863617,
0.0737853094106077));
#102430=CARTESIAN_POINT('Ctrl Pts',(0.00237354227162489,-0.0336938721132408,
0.0742634277099222));
#102431=CARTESIAN_POINT('Ctrl Pts',(0.0023728783415994,-0.0336474569764967,
0.0742297696475292));
#102432=CARTESIAN_POINT('Ctrl Pts',(0.00237260846718368,-0.033601104548885,
0.0741961061192689));
#102433=CARTESIAN_POINT('Ctrl Pts',(0.00237192520727048,-0.0334837508694616,
0.0741108778128509));
#102434=CARTESIAN_POINT('Ctrl Pts',(0.00237376773860192,-0.0333660264863617,
0.0740256666860111));
#102435=CARTESIAN_POINT('Ctrl Pts',(0.00237354227163478,-0.0336938721132427,
0.0742634277099263));
#102436=CARTESIAN_POINT('Ctrl Pts',(0.00237287834160937,-0.0336474569765026,
0.0742297696475362));
#102437=CARTESIAN_POINT('Ctrl Pts',(0.00237260846719368,-0.0336011045488949,
0.0741961061192789));
#102438=CARTESIAN_POINT('Ctrl Pts',(0.00237193089790498,-0.033484728265791,
0.0741115876485763));
#102439=CARTESIAN_POINT('Ctrl Pts',(0.00237373722885253,-0.0333679870047995,
0.0740270857660023));
#102440=CARTESIAN_POINT('Ctrl Pts',(0.00237354227162492,-0.0336938721132425,
0.0742634277099235));
#102441=CARTESIAN_POINT('Ctrl Pts',(0.00237116776403552,-0.0335278710435082,
0.0741430515836346));
#102442=CARTESIAN_POINT('Ctrl Pts',(0.00237256905581545,-0.0333620469224319,
0.0740226433414466));
#102443=CARTESIAN_POINT('Ctrl Pts',(0.00237776687175776,-0.0331951640388601,
0.0739021433341537));
#102444=CARTESIAN_POINT('Ctrl Pts',(0.00237701691299514,-0.0336938721132425,
0.0743471890177609));
#102445=CARTESIAN_POINT('Ctrl Pts',(0.00237288893739257,-0.0335278710435082,
0.0742268856299792));
#102446=CARTESIAN_POINT('Ctrl Pts',(0.00237253509696462,-0.0333620469224319,
0.0741064951124082));
#102447=CARTESIAN_POINT('Ctrl Pts',(0.00237597524068128,-0.0331951640388601,
0.0739859575327203));
#102448=CARTESIAN_POINT('Ctrl Pts',(0.00238049155436535,-0.0336938721132425,
0.0744309503255982));
#102449=CARTESIAN_POINT('Ctrl Pts',(0.00237461011074962,-0.0335278710435082,
0.0743107196763237));
#102450=CARTESIAN_POINT('Ctrl Pts',(0.0023725011381138,-0.0333620469224319,
0.0741903468833699));
#102451=CARTESIAN_POINT('Ctrl Pts',(0.0023741836096048,-0.0331951640388601,
0.0740697717312869));
#102452=CARTESIAN_POINT('Ctrl Pts',(0.00238396619573556,-0.0336938721132425,
0.0745147116334355));
#102453=CARTESIAN_POINT('Ctrl Pts',(0.00237633128410666,-0.0335278710435082,
0.0743945537226684));
#102454=CARTESIAN_POINT('Ctrl Pts',(0.00237246717926298,-0.0333620469224319,
0.0742741986543316));
#102455=CARTESIAN_POINT('Ctrl Pts',(0.00237239197852832,-0.0331951640388601,
0.0741535859298535));
#102456=CARTESIAN_POINT('Ctrl Pts',(0.00237520113173803,-0.0330240426238155,
0.0740271319374078));
#102457=CARTESIAN_POINT('Ctrl Pts',(0.00237689375900478,-0.0329142774063508,
0.0739479396327167));
#102458=CARTESIAN_POINT('Ctrl Pts',(0.00238022435625873,-0.0328043479726686,
0.0738687428391072));
#102459=CARTESIAN_POINT('Ctrl Pts',(0.00238519145086425,-0.0326943950436594,
0.0737896431310757));
#102460=CARTESIAN_POINT('Ctrl Pts',(0.00229171284940129,-0.0330240426238155,
0.0741037533619383));
#102461=CARTESIAN_POINT('Ctrl Pts',(0.0022923499418965,-0.0329142774063508,
0.0740234109248193));
#102462=CARTESIAN_POINT('Ctrl Pts',(0.00229464825460635,-0.0328043479726686,
0.0739430416045468));
#102463=CARTESIAN_POINT('Ctrl Pts',(0.00229860767869599,-0.0326943950436594,
0.0738627484412915));
#102464=CARTESIAN_POINT('Ctrl Pts',(0.00220822456706454,-0.0330240426238155,
0.0741803747864688));
#102465=CARTESIAN_POINT('Ctrl Pts',(0.00220780612478822,-0.0329142774063508,
0.074098882216922));
#102466=CARTESIAN_POINT('Ctrl Pts',(0.00220907215295397,-0.0328043479726686,
0.0740173403699864));
#102467=CARTESIAN_POINT('Ctrl Pts',(0.00221202390652774,-0.0326943950436594,
0.0739358537515073));
#102468=CARTESIAN_POINT('Ctrl Pts',(0.0021247362847278,-0.0330240426238155,
0.0742569962109993));
#102469=CARTESIAN_POINT('Ctrl Pts',(0.00212326230767993,-0.0329142774063508,
0.0741743535090246));
#102470=CARTESIAN_POINT('Ctrl Pts',(0.00212349605130159,-0.0328043479726686,
0.074091639135426));
#102471=CARTESIAN_POINT('Ctrl Pts',(0.00212544013435949,-0.0326943950436594,
0.0740089590617231));
#102472=CARTESIAN_POINT('Origin',(0.0191471851194885,-0.0326396682855343,
0.0749156908757754));
#102473=CARTESIAN_POINT('Ctrl Pts',(0.00214397671962881,-0.0331951640388587,
0.0736581397562618));
#102474=CARTESIAN_POINT('Ctrl Pts',(0.00215075109946113,-0.0330855618255041,
0.0735757800329126));
#102475=CARTESIAN_POINT('Ctrl Pts',(0.00215923259754889,-0.0329757224427708,
0.0734935009524415));
#102476=CARTESIAN_POINT('Ctrl Pts',(0.00216941552111462,-0.0328657862078596,
0.0734114084109088));
#102477=CARTESIAN_POINT('Ctrl Pts',(0.00222237446226089,-0.0331951640388587,
0.0737399624058756));
#102478=CARTESIAN_POINT('Ctrl Pts',(0.00222802190062066,-0.0330855618255041,
0.0736586824528338));
#102479=CARTESIAN_POINT('Ctrl Pts',(0.00223535332783296,-0.0329757224427708,
0.0735774606291075));
#102480=CARTESIAN_POINT('Ctrl Pts',(0.00224436445744446,-0.0328657862078596,
0.0734964014046356));
#102481=CARTESIAN_POINT('Ctrl Pts',(0.00230077220489298,-0.0331951640388587,
0.0738217850554894));
#102482=CARTESIAN_POINT('Ctrl Pts',(0.00230529270178019,-0.0330855618255041,
0.073741584872755));
#102483=CARTESIAN_POINT('Ctrl Pts',(0.00231147405811704,-0.0329757224427708,
0.0736614203057736));
#102484=CARTESIAN_POINT('Ctrl Pts',(0.0023193133937743,-0.0328657862078596,
0.0735813943983625));
#102485=CARTESIAN_POINT('Ctrl Pts',(0.00237916994752506,-0.0331951640388587,
0.0739036077051031));
#102486=CARTESIAN_POINT('Ctrl Pts',(0.00238256350293971,-0.0330855618255041,
0.0738244872926761));
#102487=CARTESIAN_POINT('Ctrl Pts',(0.00238759478840111,-0.0329757224427708,
0.0737453799824396));
#102488=CARTESIAN_POINT('Ctrl Pts',(0.00239426233010414,-0.0328657862078596,
0.0736663873920893));
#102489=CARTESIAN_POINT('Origin',(0.0190755113989164,-0.0326401908835166,
0.0753912282023842));
#102490=CARTESIAN_POINT('Ctrl Pts',(0.00237632414284395,-0.0332451089994431,
0.0739382195465792));
#102491=CARTESIAN_POINT('Ctrl Pts',(0.00238431157332591,-0.0329451141710257,
0.0737214506196884));
#102492=CARTESIAN_POINT('Ctrl Pts',(0.00240860423409257,-0.0326442513127503,
0.073505899156358));
#102493=CARTESIAN_POINT('Ctrl Pts',(0.00237255046045652,-0.0332451089994431,
0.0741881910635991));
#102494=CARTESIAN_POINT('Ctrl Pts',(0.00237111006092671,-0.0329451141710257,
0.0739712798099484));
#102495=CARTESIAN_POINT('Ctrl Pts',(0.00238601239578505,-0.0326442513127503,
0.0737548762814957));
#102496=CARTESIAN_POINT('Ctrl Pts',(0.00239425958398091,-0.0325229783203385,
0.0736664188601564));
#102497=CARTESIAN_POINT('Ctrl Pts',(0.0024009257392971,-0.0324130253112079,
0.0735874375177236));
#102498=CARTESIAN_POINT('Ctrl Pts',(0.00240922471405741,-0.0323031222247695,
0.0735086060523421));
#102499=CARTESIAN_POINT('Ctrl Pts',(0.00241914231470219,-0.0321934096636184,
0.0734300250663995));
#102500=CARTESIAN_POINT('Ctrl Pts',(0.00230612493617983,-0.0325229783203385,
0.0737376468497841));
#102501=CARTESIAN_POINT('Ctrl Pts',(0.00231180921523453,-0.0324130253112079,
0.0736574505731809));
#102502=CARTESIAN_POINT('Ctrl Pts',(0.00231915159512767,-0.0323031222247695,
0.0735773840465261));
#102503=CARTESIAN_POINT('Ctrl Pts',(0.0023281390518051,-0.0321934096636184,
0.0734975494974708));
#102504=CARTESIAN_POINT('Ctrl Pts',(0.00221799028837875,-0.0325229783203385,
0.0738088748394118));
#102505=CARTESIAN_POINT('Ctrl Pts',(0.00222269269117196,-0.0324130253112079,
0.0737274636286381));
#102506=CARTESIAN_POINT('Ctrl Pts',(0.00222907847619793,-0.0323031222247695,
0.0736461620407101));
#102507=CARTESIAN_POINT('Ctrl Pts',(0.002237135788908,-0.0321934096636184,
0.0735650739285422));
#102508=CARTESIAN_POINT('Ctrl Pts',(0.00212985564057767,-0.0325229783203385,
0.0738801028290395));
#102509=CARTESIAN_POINT('Ctrl Pts',(0.00213357616710938,-0.0324130253112079,
0.0737974766840954));
#102510=CARTESIAN_POINT('Ctrl Pts',(0.00213900535726818,-0.0323031222247695,
0.0737149400348941));
#102511=CARTESIAN_POINT('Ctrl Pts',(0.00214613252601091,-0.0321934096636184,
0.0736325983596135));
#102512=CARTESIAN_POINT('Origin',(0.0191386995571209,-0.0326393375178722,
0.0749148624697292));
#102513=CARTESIAN_POINT('Ctrl Pts',(0.00218666066001428,-0.0326943950436593,
0.0732836352377341));
#102514=CARTESIAN_POINT('Ctrl Pts',(0.00219860079017889,-0.0325844576448126,
0.0732018105756567));
#102515=CARTESIAN_POINT('Ctrl Pts',(0.00221223403353018,-0.0324744968375319,
0.0731202270641886));
#102516=CARTESIAN_POINT('Ctrl Pts',(0.00222754148058497,-0.0323646534831895,
0.0730389889919505));
#102517=CARTESIAN_POINT('Ctrl Pts',(0.00225976594631064,-0.0326943950436593,
0.0733702189815729));
#102518=CARTESIAN_POINT('Ctrl Pts',(0.00227051279020992,-0.0325844576448126,
0.0732894018473545));
#102519=CARTESIAN_POINT('Ctrl Pts',(0.00228293182551718,-0.0324744968375319,
0.0732088012559335));
#102520=CARTESIAN_POINT('Ctrl Pts',(0.00229700571583393,-0.0323646534831895,
0.0731285202580138));
#102521=CARTESIAN_POINT('Ctrl Pts',(0.002332871232607,-0.0326943950436593,
0.0734568027254117));
#102522=CARTESIAN_POINT('Ctrl Pts',(0.00234242479024096,-0.0325844576448126,
0.0733769931190524));
#102523=CARTESIAN_POINT('Ctrl Pts',(0.00235362961750417,-0.0324744968375319,
0.0732973754476784));
#102524=CARTESIAN_POINT('Ctrl Pts',(0.00236646995108289,-0.0323646534831894,
0.0732180515240771));
#102525=CARTESIAN_POINT('Ctrl Pts',(0.00240597651890337,-0.0326943950436593,
0.0735433864692505));
#102526=CARTESIAN_POINT('Ctrl Pts',(0.00241433679027199,-0.0325844576448126,
0.0734645843907503));
#102527=CARTESIAN_POINT('Ctrl Pts',(0.00242432740949117,-0.0324744968375319,
0.0733859496394233));
#102528=CARTESIAN_POINT('Ctrl Pts',(0.00243593418633185,-0.0323646534831894,
0.0733075827901404));
#102529=CARTESIAN_POINT('Origin',(0.0191131607638069,-0.0326395579068891,
0.0753950343999735));
#102530=CARTESIAN_POINT('Ctrl Pts',(0.00240095934061233,-0.0327445246961877,
0.0735777905986883));
#102531=CARTESIAN_POINT('Ctrl Pts',(0.00242254057076331,-0.0324436878365475,
0.0733619508085522));
#102532=CARTESIAN_POINT('Ctrl Pts',(0.00246031842589224,-0.0321434074463188,
0.073148349782893));
#102533=CARTESIAN_POINT('Ctrl Pts',(0.00238149896308957,-0.0327445246961877,
0.0738270320352647));
#102534=CARTESIAN_POINT('Ctrl Pts',(0.00239367989888399,-0.0324436878365475,
0.0736104582849994));
#102535=CARTESIAN_POINT('Ctrl Pts',(0.00242213944977537,-0.0321434074463188,
0.073395417315731));
#102536=CARTESIAN_POINT('Ctrl Pts',(0.0024490888225131,-0.0322357242816073,
0.0732140618878779));
#102537=CARTESIAN_POINT('Ctrl Pts',(0.00247889723751693,-0.0319819883628706,
0.0730333302638323));
#102538=CARTESIAN_POINT('Ctrl Pts',(0.00252014571233431,-0.0317295851069887,
0.0728548617095699));
#102539=CARTESIAN_POINT('Ctrl Pts',(0.00241377615384327,-0.0322357242816073,
0.0734615553533096));
#102540=CARTESIAN_POINT('Ctrl Pts',(0.00243570222296037,-0.0319819883628706,
0.0732796990665657));
#102541=CARTESIAN_POINT('Ctrl Pts',(0.00246915589194791,-0.0317295851069887,
0.0730996065526553));
#102542=CARTESIAN_POINT('Origin',(0.019018671909538,-0.032637194264179,
0.0753826142571921));
#102543=CARTESIAN_POINT('Origin',(0.0190164960621664,-0.0326352985532318,
0.0749034559479179));
#102544=CARTESIAN_POINT('Ctrl Pts',(0.00225277570667768,-0.0321934096636183,
0.0729125498651181));
#102545=CARTESIAN_POINT('Ctrl Pts',(0.00226984110844767,-0.0320835708272303,
0.0728315841100861));
#102546=CARTESIAN_POINT('Ctrl Pts',(0.00228857219368324,-0.0319739230346346,
0.0727510184860852));
#102547=CARTESIAN_POINT('Ctrl Pts',(0.00230893708630216,-0.0318646057455575,
0.0726709542319852));
#102548=CARTESIAN_POINT('Ctrl Pts',(0.00232030019589517,-0.0321934096636183,
0.0730035532063792));
#102549=CARTESIAN_POINT('Ctrl Pts',(0.00233611059066547,-0.0320835708272303,
0.072923518666679));
#102550=CARTESIAN_POINT('Ctrl Pts',(0.00235356812540354,-0.0319739230346346,
0.0728438577455623));
#102551=CARTESIAN_POINT('Ctrl Pts',(0.00237264264228187,-0.0318646057455575,
0.0727646706494482));
#102552=CARTESIAN_POINT('Ctrl Pts',(0.00238782468511265,-0.0321934096636183,
0.0730945565476404));
#102553=CARTESIAN_POINT('Ctrl Pts',(0.00240238007288327,-0.0320835708272303,
0.0730154532232718));
#102554=CARTESIAN_POINT('Ctrl Pts',(0.00241856405712383,-0.0319739230346346,
0.0729366970050395));
#102555=CARTESIAN_POINT('Ctrl Pts',(0.00243634819826157,-0.0318646057455575,
0.0728583870669111));
#102556=CARTESIAN_POINT('Ctrl Pts',(0.00245534917433013,-0.0321934096636183,
0.0731855598889015));
#102557=CARTESIAN_POINT('Ctrl Pts',(0.00246864955510107,-0.0320835708272303,
0.0731073877798646));
#102558=CARTESIAN_POINT('Ctrl Pts',(0.00248355998884413,-0.0319739230346346,
0.0730295362645166));
#102559=CARTESIAN_POINT('Ctrl Pts',(0.00250005375424128,-0.0318646057455575,
0.0729521034843741));
#102560=CARTESIAN_POINT('Ctrl Pts',(0.00243504686768346,-0.0320218834582399,
0.0733079262516562));
#102561=CARTESIAN_POINT('Ctrl Pts',(0.00244381081970364,-0.0319391099350681,
0.073248720269347));
#102562=CARTESIAN_POINT('Ctrl Pts',(0.00245349397158339,-0.0318564869454948,
0.0731896870087778));
#102563=CARTESIAN_POINT('Ctrl Pts',(0.00246408525627879,-0.0317740741446526,
0.0731308688094123));
#102564=CARTESIAN_POINT('Ctrl Pts',(0.00239461420190388,-0.0320218834582399,
0.0733365972751002));
#102565=CARTESIAN_POINT('Ctrl Pts',(0.00240307975788176,-0.0319391099350681,
0.0732769704864855));
#102566=CARTESIAN_POINT('Ctrl Pts',(0.00241247126545925,-0.0318564869454948,
0.0732175120150707));
#102567=CARTESIAN_POINT('Ctrl Pts',(0.00242277784110307,-0.0317740741446526,
0.0731582645298604));
#102568=CARTESIAN_POINT('Ctrl Pts',(0.00235418153612429,-0.0320218834582399,
0.0733652682985442));
#102569=CARTESIAN_POINT('Ctrl Pts',(0.00236234869605987,-0.0319391099350681,
0.0733052207036241));
#102570=CARTESIAN_POINT('Ctrl Pts',(0.0023714485593351,-0.0318564869454947,
0.0732453370213637));
#102571=CARTESIAN_POINT('Ctrl Pts',(0.00238147042592736,-0.0317740741446526,
0.0731856602503085));
#102572=CARTESIAN_POINT('Ctrl Pts',(0.00231374887034471,-0.0320218834582399,
0.0733939393219882));
#102573=CARTESIAN_POINT('Ctrl Pts',(0.00232161763423799,-0.0319391099350681,
0.0733334709207627));
#102574=CARTESIAN_POINT('Ctrl Pts',(0.00233042585321096,-0.0318564869454947,
0.0732731620276566));
#102575=CARTESIAN_POINT('Ctrl Pts',(0.00234016301075164,-0.0317740741446526,
0.0732130559707566));
#102576=CARTESIAN_POINT('Origin',(-0.00392566732324075,-0.039122885339057,
0.0733185045508921));
#102577=CARTESIAN_POINT('Ctrl Pts',(0.00279759881750081,-0.0352722978779652,
0.0763216204069769));
#102578=CARTESIAN_POINT('Ctrl Pts',(0.00279078974844655,-0.0352466642097256,
0.0763039928927817));
#102579=CARTESIAN_POINT('Ctrl Pts',(0.00278391361101129,-0.035221018380832,
0.0762864093326981));
#102580=CARTESIAN_POINT('Ctrl Pts',(0.00277696966659563,-0.0351953608940152,
0.0762688693001644));
#102581=CARTESIAN_POINT('Origin',(-0.00183537316245779,-0.0352456003065139,
0.0779170243773864));
#102582=CARTESIAN_POINT('Ctrl Pts',(0.00273365592871159,-0.0350241211493339,
0.0761519537942269));
#102583=CARTESIAN_POINT('Ctrl Pts',(0.00270607983727255,-0.0349144232867421,
0.0760777070183204));
#102584=CARTESIAN_POINT('Ctrl Pts',(0.00268002197405695,-0.0348045283677512,
0.0760028457846527));
#102585=CARTESIAN_POINT('Ctrl Pts',(0.00265551928407819,-0.0346945769586886,
0.0759274647389144));
#102586=CARTESIAN_POINT('Ctrl Pts',(0.00268423670087071,-0.0350241211493339,
0.0762539287015456));
#102587=CARTESIAN_POINT('Ctrl Pts',(0.00265525594695804,-0.0349144232867421,
0.076179001196069));
#102588=CARTESIAN_POINT('Ctrl Pts',(0.00262780665167665,-0.0348045283677512,
0.0761034297900059));
#102589=CARTESIAN_POINT('Ctrl Pts',(0.00260192757613728,-0.0346945769586886,
0.0760273099723661));
#102590=CARTESIAN_POINT('Ctrl Pts',(0.00263481747302984,-0.0350241211493339,
0.0763559036088642));
#102591=CARTESIAN_POINT('Ctrl Pts',(0.00260443205664353,-0.0349144232867421,
0.0762802953738175));
#102592=CARTESIAN_POINT('Ctrl Pts',(0.00257559132929634,-0.0348045283677512,
0.0762040137953592));
#102593=CARTESIAN_POINT('Ctrl Pts',(0.00254833586819637,-0.0346945769586886,
0.0761271552058178));
#102594=CARTESIAN_POINT('Ctrl Pts',(0.00258539824518897,-0.0350241211493339,
0.0764578785161829));
#102595=CARTESIAN_POINT('Ctrl Pts',(0.00255360816632902,-0.0349144232867421,
0.0763815895515661));
#102596=CARTESIAN_POINT('Ctrl Pts',(0.00252337600691604,-0.0348045283677512,
0.0763045978007125));
#102597=CARTESIAN_POINT('Ctrl Pts',(0.00249474416025546,-0.0346945769586886,
0.0762270004392695));
#102598=CARTESIAN_POINT('Origin',(0.018676725161843,-0.03456290679408,0.0709091073082728));
#102599=CARTESIAN_POINT('Ctrl Pts',(0.00246756592837366,-0.0351970973651616,
0.0759340233585258));
#102600=CARTESIAN_POINT('Ctrl Pts',(0.00244285070252079,-0.0350869349321767,
0.0758556641477074));
#102601=CARTESIAN_POINT('Ctrl Pts',(0.00241974404743112,-0.034976498512971,
0.0757767262091816));
#102602=CARTESIAN_POINT('Ctrl Pts',(0.00239828191845461,-0.0348659306849624,
0.0756973100471963));
#102603=CARTESIAN_POINT('Ctrl Pts',(0.0025423189656239,-0.0351970973651616,
0.0759682644752137));
#102604=CARTESIAN_POINT('Ctrl Pts',(0.00251712937550424,-0.0350869349321767,
0.0758909408664182));
#102605=CARTESIAN_POINT('Ctrl Pts',(0.00249352643359778,-0.034976498512971,
0.0758130295260256));
#102606=CARTESIAN_POINT('Ctrl Pts',(0.00247154665991777,-0.0348659306849624,
0.0757346295904479));
#102607=CARTESIAN_POINT('Ctrl Pts',(0.00261707200287414,-0.0351970973651616,
0.0760025055919017));
#102608=CARTESIAN_POINT('Ctrl Pts',(0.00259140804848769,-0.0350869349321767,
0.0759262175851289));
#102609=CARTESIAN_POINT('Ctrl Pts',(0.00256730881976445,-0.034976498512971,
0.0758493328428697));
#102610=CARTESIAN_POINT('Ctrl Pts',(0.00254481140138094,-0.0348659306849624,
0.0757719491336996));
#102611=CARTESIAN_POINT('Ctrl Pts',(0.00269182504012437,-0.0351970973651616,
0.0760367467085896));
#102612=CARTESIAN_POINT('Ctrl Pts',(0.00266568672147114,-0.0350869349321767,
0.0759614943038397));
#102613=CARTESIAN_POINT('Ctrl Pts',(0.00264109120593112,-0.034976498512971,
0.0758856361597137));
#102614=CARTESIAN_POINT('Ctrl Pts',(0.0026180761428441,-0.0348659306849624,
0.0758092686769512));
#102615=CARTESIAN_POINT('Origin',(0.0187738267269148,-0.0345637187967918,
0.0713801663725021));
#102616=CARTESIAN_POINT('Ctrl Pts',(0.00270196724699681,-0.0352450361861254,
0.0760688662512332));
#102617=CARTESIAN_POINT('Ctrl Pts',(0.002629596020637,-0.0349452761023765,
0.0758643791503246));
#102618=CARTESIAN_POINT('Ctrl Pts',(0.00257283319804065,-0.0346444289983475,
0.0756550216789658));
#102619=CARTESIAN_POINT('Ctrl Pts',(0.00279047897349925,-0.0352450361861254,
0.0763026731678793));
#102620=CARTESIAN_POINT('Ctrl Pts',(0.00270928957480554,-0.0349452761023765,
0.0761015243414284));
#102621=CARTESIAN_POINT('Ctrl Pts',(0.00264348217888855,-0.0346444289983475,
0.0758948314400373));
#102622=CARTESIAN_POINT('Ctrl Pts',(0.00261858862169873,-0.0345231616327822,
0.0758095555140895));
#102623=CARTESIAN_POINT('Ctrl Pts',(0.00259571398540442,-0.0344132092796975,
0.0757336741714007));
#102624=CARTESIAN_POINT('Ctrl Pts',(0.00257441007505534,-0.0343032738558974,
0.0756573236000318));
#102625=CARTESIAN_POINT('Ctrl Pts',(0.00255470167788285,-0.0341934961088741,
0.0755806023130033));
#102626=CARTESIAN_POINT('Ctrl Pts',(0.00256286388209672,-0.0345231616327822,
0.0759082261253921));
#102627=CARTESIAN_POINT('Ctrl Pts',(0.00253862921034272,-0.0344132092796975,
0.075831576695622));
#102628=CARTESIAN_POINT('Ctrl Pts',(0.00251598122198095,-0.0343032738558974,
0.075754429945541));
#102629=CARTESIAN_POINT('Ctrl Pts',(0.00249494640003443,-0.0341934961088741,
0.0756768854522739));
#102630=CARTESIAN_POINT('Ctrl Pts',(0.00250713914249471,-0.0345231616327822,
0.0760068967366947));
#102631=CARTESIAN_POINT('Ctrl Pts',(0.00248154443528103,-0.0344132092796975,
0.0759294792198434));
#102632=CARTESIAN_POINT('Ctrl Pts',(0.00245755236890656,-0.0343032738558974,
0.0758515362910501));
#102633=CARTESIAN_POINT('Ctrl Pts',(0.002435191122186,-0.0341934961088741,
0.0757731685915444));
#102634=CARTESIAN_POINT('Ctrl Pts',(0.0024514144028927,-0.0345231616327822,
0.0761055673479973));
#102635=CARTESIAN_POINT('Ctrl Pts',(0.00242445966021933,-0.0344132092796975,
0.0760273817440647));
#102636=CARTESIAN_POINT('Ctrl Pts',(0.00239912351583217,-0.0343032738558974,
0.0759486426365593));
#102637=CARTESIAN_POINT('Ctrl Pts',(0.00237543584433758,-0.0341934961088741,
0.075869451730815));
#102638=CARTESIAN_POINT('Origin',(0.018688219451002,-0.0345625596227404,
0.0709053152618022));
#102639=CARTESIAN_POINT('Ctrl Pts',(0.00228465605720541,-0.0346945769586885,
0.0755300746244476));
#102640=CARTESIAN_POINT('Ctrl Pts',(0.00226563793133554,-0.034584662917669,
0.0754496085149667));
#102641=CARTESIAN_POINT('Ctrl Pts',(0.00224828056322056,-0.0344746925051587,
0.075368735374644));
#102642=CARTESIAN_POINT('Ctrl Pts',(0.00223260576516843,-0.0343648066255171,
0.0752875589193154));
#102643=CARTESIAN_POINT('Ctrl Pts',(0.00238450121204229,-0.0346945769586885,
0.0755836662901922));
#102644=CARTESIAN_POINT('Ctrl Pts',(0.00236474456593109,-0.034584662917669,
0.0755045760974107));
#102645=CARTESIAN_POINT('Ctrl Pts',(0.00234662009804143,-0.0344746925051587,
0.075425063836502));
#102646=CARTESIAN_POINT('Ctrl Pts',(0.0023301506107792,-0.0343648066255171,
0.0753452314836459));
#102647=CARTESIAN_POINT('Ctrl Pts',(0.00248434636687917,-0.0346945769586885,
0.0756372579559368));
#102648=CARTESIAN_POINT('Ctrl Pts',(0.00246385120052663,-0.034584662917669,
0.0755595436798546));
#102649=CARTESIAN_POINT('Ctrl Pts',(0.0024449596328623,-0.0344746925051587,
0.07548139229836));
#102650=CARTESIAN_POINT('Ctrl Pts',(0.00242769545638997,-0.0343648066255171,
0.0754029040479763));
#102651=CARTESIAN_POINT('Ctrl Pts',(0.00258419152171605,-0.0346945769586885,
0.0756908496216814));
#102652=CARTESIAN_POINT('Ctrl Pts',(0.00256295783512218,-0.034584662917669,
0.0756145112622986));
#102653=CARTESIAN_POINT('Ctrl Pts',(0.00254329916768317,-0.0344746925051587,
0.0755377207602181));
#102654=CARTESIAN_POINT('Ctrl Pts',(0.00252524030200075,-0.0343648066255171,
0.0754605766123068));
#102655=CARTESIAN_POINT('Origin',(0.0188301750962575,-0.0345626446730578,
0.071364707008772));
#102656=CARTESIAN_POINT('Ctrl Pts',(0.00258240495709019,-0.0346945769586885,
0.0756898906870749));
#102657=CARTESIAN_POINT('Ctrl Pts',(0.00255015133011134,-0.0345275153362891,
0.075573824322222));
#102658=CARTESIAN_POINT('Ctrl Pts',(0.00252153954103531,-0.0343603235965159,
0.0754567135897811));
#102659=CARTESIAN_POINT('Ctrl Pts',(0.00249664906299847,-0.034193496108874,
0.0753389061090011));
#102660=CARTESIAN_POINT('Ctrl Pts',(0.00260660102383874,-0.0346945769586885,
0.07577015636271));
#102661=CARTESIAN_POINT('Ctrl Pts',(0.00257266620014711,-0.0345275153362891,
0.0756545967941627));
#102662=CARTESIAN_POINT('Ctrl Pts',(0.00254235684123739,-0.0343603235965159,
0.0755379401170217));
#102663=CARTESIAN_POINT('Ctrl Pts',(0.00251575746086286,-0.034193496108874,
0.075420532682262));
#102664=CARTESIAN_POINT('Ctrl Pts',(0.00263079709058728,-0.0346945769586885,
0.0758504220383451));
#102665=CARTESIAN_POINT('Ctrl Pts',(0.00259518107018288,-0.0345275153362891,
0.0757353692661034));
#102666=CARTESIAN_POINT('Ctrl Pts',(0.00256317414143947,-0.0343603235965159,
0.0756191666442624));
#102667=CARTESIAN_POINT('Ctrl Pts',(0.00253486585872724,-0.034193496108874,
0.0755021592555229));
#102668=CARTESIAN_POINT('Ctrl Pts',(0.00265499315733583,-0.0346945769586885,
0.0759306877139802));
#102669=CARTESIAN_POINT('Ctrl Pts',(0.00261769594021865,-0.0345275153362891,
0.0758161417380442));
#102670=CARTESIAN_POINT('Ctrl Pts',(0.00258399144164155,-0.0343603235965159,
0.075700393171503));
#102671=CARTESIAN_POINT('Ctrl Pts',(0.00255397425659163,-0.034193496108874,
0.0755837858287838));
#102672=CARTESIAN_POINT('Ctrl Pts',(0.00252524803638778,-0.0340223579322365,
0.0754606072089728));
#102673=CARTESIAN_POINT('Ctrl Pts',(0.00250717134476912,-0.0339125849573554,
0.0753833888213624));
#102674=CARTESIAN_POINT('Ctrl Pts',(0.00249070559662516,-0.0338030433565221,
0.0753058505487067));
#102675=CARTESIAN_POINT('Ctrl Pts',(0.0024758630588989,-0.0336938721132328,
0.0752280934159937));
#102676=CARTESIAN_POINT('Ctrl Pts',(0.00246343758796055,-0.0340223579322365,
0.0755555843025039));
#102677=CARTESIAN_POINT('Ctrl Pts',(0.00244405091451146,-0.0339125849573554,
0.0754775133876013));
#102678=CARTESIAN_POINT('Ctrl Pts',(0.00242629375038006,-0.0338030433565221,
0.0753990960731345));
#102679=CARTESIAN_POINT('Ctrl Pts',(0.00241017991436192,-0.0336938721132328,
0.0753204346546368));
#102680=CARTESIAN_POINT('Ctrl Pts',(0.00240162713953332,-0.0340223579322365,
0.075650561396035));
#102681=CARTESIAN_POINT('Ctrl Pts',(0.00238093048425379,-0.0339125849573554,
0.0755716379538401));
#102682=CARTESIAN_POINT('Ctrl Pts',(0.00236188190413497,-0.0338030433565221,
0.0754923415975624));
#102683=CARTESIAN_POINT('Ctrl Pts',(0.00234449676982493,-0.0336938721132328,
0.0754127758932798));
#102684=CARTESIAN_POINT('Ctrl Pts',(0.0023398166911061,-0.0340223579322365,
0.0757455384895661));
#102685=CARTESIAN_POINT('Ctrl Pts',(0.00231781005399612,-0.0339125849573554,
0.075665762520079));
#102686=CARTESIAN_POINT('Ctrl Pts',(0.00229747005788988,-0.0338030433565221,
0.0755855871219902));
#102687=CARTESIAN_POINT('Ctrl Pts',(0.00227881362528795,-0.0336938721132328,
0.0755051171319228));
#102688=CARTESIAN_POINT('Origin',(0.018572563017671,-0.0345589643416638,
0.0709381248279057));
#102689=CARTESIAN_POINT('Ctrl Pts',(0.00220952263615494,-0.034193496108874,
0.0751607095987538));
#102690=CARTESIAN_POINT('Ctrl Pts',(0.00219558554936318,-0.0340836138585569,
0.07507915546208));
#102691=CARTESIAN_POINT('Ctrl Pts',(0.00218334274157543,-0.033973889665241,
0.074997352057848));
#102692=CARTESIAN_POINT('Ctrl Pts',(0.00217280286363653,-0.0338644633307392,
0.0749154051347012));
#102693=CARTESIAN_POINT('Ctrl Pts',(0.00230580586205917,-0.034193496108874,
0.0752204649303689));
#102694=CARTESIAN_POINT('Ctrl Pts',(0.00229104478463349,-0.0340836138585569,
0.0751402384823583));
#102695=CARTESIAN_POINT('Ctrl Pts',(0.00227795090784711,-0.033973889665241,
0.0750597450789823));
#102696=CARTESIAN_POINT('Ctrl Pts',(0.00226653408420143,-0.0338644633307392,
0.0749790888652637));
#102697=CARTESIAN_POINT('Ctrl Pts',(0.0024020890879634,-0.034193496108874,
0.0752802202619839));
#102698=CARTESIAN_POINT('Ctrl Pts',(0.00238650401990379,-0.0340836138585569,
0.0752013215026364));
#102699=CARTESIAN_POINT('Ctrl Pts',(0.00237255907411878,-0.033973889665241,
0.0751221381001166));
#102700=CARTESIAN_POINT('Ctrl Pts',(0.00236026530476633,-0.0338644633307392,
0.0750427725958263));
#102701=CARTESIAN_POINT('Ctrl Pts',(0.00249837231386763,-0.034193496108874,
0.075339975593599));
#102702=CARTESIAN_POINT('Ctrl Pts',(0.0024819632551741,-0.0340836138585569,
0.0752624045229147));
#102703=CARTESIAN_POINT('Ctrl Pts',(0.00246716724039046,-0.033973889665241,
0.0751845311212508));
#102704=CARTESIAN_POINT('Ctrl Pts',(0.00245399652533122,-0.0338644633307392,
0.0751064563263888));
#102705=CARTESIAN_POINT('Origin',(0.0187570446595347,-0.0345610621860694,
0.0713825531527638));
#102706=CARTESIAN_POINT('Ctrl Pts',(0.00250423887516722,-0.0342436276873901,
0.0753742785213273));
#102707=CARTESIAN_POINT('Ctrl Pts',(0.00245806444954122,-0.0339430054201861,
0.0751623339511449));
#102708=CARTESIAN_POINT('Ctrl Pts',(0.00242798573405938,-0.0336441434784162,
0.0749475134463352));
#102709=CARTESIAN_POINT('Ctrl Pts',(0.00256275220091025,-0.0342436276873901,
0.0756173344628521));
#102710=CARTESIAN_POINT('Ctrl Pts',(0.00250741076932982,-0.0339430054201861,
0.0754075967591307));
#102711=CARTESIAN_POINT('Ctrl Pts',(0.00246802486017225,-0.0336441434784162,
0.0751942863548567));
#102712=CARTESIAN_POINT('Ctrl Pts',(0.00245400126290403,-0.0335235895815127,
0.0751064836490833));
#102713=CARTESIAN_POINT('Ctrl Pts',(0.00244083338233157,-0.0334144449262719,
0.0750284279518087));
#102714=CARTESIAN_POINT('Ctrl Pts',(0.00242926294542188,-0.0333049234473133,
0.074950010539492));
#102715=CARTESIAN_POINT('Ctrl Pts',(0.00241931383026442,-0.0331951640388588,
0.0748713303437296));
#102716=CARTESIAN_POINT('Ctrl Pts',(0.00238634910011936,-0.0335235895815127,
0.0751973921599989));
#102717=CARTESIAN_POINT('Ctrl Pts',(0.00237192968491178,-0.0334144449262719,
0.0751184050975087));
#102718=CARTESIAN_POINT('Ctrl Pts',(0.00235912551680972,-0.0333049234473133,
0.0750390293941869));
#102719=CARTESIAN_POINT('Ctrl Pts',(0.00234796216246448,-0.0331951640388588,
0.0749593650640875));
#102720=CARTESIAN_POINT('Ctrl Pts',(0.00231869693733469,-0.0335235895815127,
0.0752883006709144));
#102721=CARTESIAN_POINT('Ctrl Pts',(0.00230302598749199,-0.0334144449262719,
0.0752083822432087));
#102722=CARTESIAN_POINT('Ctrl Pts',(0.00228898808819756,-0.0333049234473133,
0.0751280482488818));
#102723=CARTESIAN_POINT('Ctrl Pts',(0.00227661049466454,-0.0331951640388588,
0.0750473997844454));
#102724=CARTESIAN_POINT('Ctrl Pts',(0.00225104477455003,-0.0335235895815127,
0.07537920918183));
#102725=CARTESIAN_POINT('Ctrl Pts',(0.0022341222900722,-0.0334144449262719,
0.0752983593889087));
#102726=CARTESIAN_POINT('Ctrl Pts',(0.00221885065958541,-0.0333049234473133,
0.0752170671035768));
#102727=CARTESIAN_POINT('Ctrl Pts',(0.0022052588268646,-0.0331951640388588,
0.0751354345048033));
#102728=CARTESIAN_POINT('Origin',(0.0190329342385817,-0.0326434571769145,
0.0735377419525711));
#102729=CARTESIAN_POINT('Ctrl Pts',(0.00215607787082645,-0.0336938721132415,
0.0747861805218438));
#102730=CARTESIAN_POINT('Ctrl Pts',(0.00215235409512492,-0.0336474569764971,
0.0747512495681503));
#102731=CARTESIAN_POINT('Ctrl Pts',(0.00214903948549557,-0.033601104548885,
0.0747162774164519));
#102732=CARTESIAN_POINT('Ctrl Pts',(0.00214064765649121,-0.0334837508662633,
0.0746277359742353));
#102733=CARTESIAN_POINT('Ctrl Pts',(0.00213488317891247,-0.0333660264799464,
0.0745389847456124));
#102734=CARTESIAN_POINT('Ctrl Pts',(0.00243310089257962,-0.0336938721132415,
0.0749832294616808));
#102735=CARTESIAN_POINT('Ctrl Pts',(0.00242822372404542,-0.0336474569764971,
0.0749499200156596));
#102736=CARTESIAN_POINT('Ctrl Pts',(0.00242373681882,-0.033601104548885,
0.0749165557586074));
#102737=CARTESIAN_POINT('Ctrl Pts',(0.00241237700707111,-0.0334837508662633,
0.0748320851357141));
#102738=CARTESIAN_POINT('Ctrl Pts',(0.00240352522325742,-0.0333660264799464,
0.0747473149913337));
#102739=CARTESIAN_POINT('Ctrl Pts',(0.0024331008925887,-0.0336938721132427,
0.0749832294616845));
#102740=CARTESIAN_POINT('Ctrl Pts',(0.00242822372405499,-0.0336474569765026,
0.0749499200156664));
#102741=CARTESIAN_POINT('Ctrl Pts',(0.00242373681883,-0.0336011045488949,
0.0749165557586174));
#102742=CARTESIAN_POINT('Ctrl Pts',(0.00241247161884069,-0.0334847282626114,
0.0748327886609622));
#102743=CARTESIAN_POINT('Ctrl Pts',(0.00240367281197103,-0.0333679869984219,
0.0747487267053694));
#102744=CARTESIAN_POINT('Ctrl Pts',(0.00243310089257973,-0.0336938721132426,
0.0749832294616816));
#102745=CARTESIAN_POINT('Ctrl Pts',(0.00241565797954017,-0.0335278710435082,
0.0748641001418174));
#102746=CARTESIAN_POINT('Ctrl Pts',(0.00240195706737466,-0.033362046922432,
0.0747444657261533));
#102747=CARTESIAN_POINT('Ctrl Pts',(0.00239201124142721,-0.0331951640388601,
0.07462426443833));
#102748=CARTESIAN_POINT('Ctrl Pts',(0.00244704621092374,-0.0336938721132426,
0.0750658947985499));
#102749=CARTESIAN_POINT('Ctrl Pts',(0.00242787277304235,-0.0335278710435082,
0.0749470574114441));
#102750=CARTESIAN_POINT('Ctrl Pts',(0.00241243278989423,-0.033362046922432,
0.0748276605570282));
#102751=CARTESIAN_POINT('Ctrl Pts',(0.00240073844242185,-0.0331951640388601,
0.074707642287823));
#102752=CARTESIAN_POINT('Ctrl Pts',(0.00246099152926775,-0.0336938721132426,
0.0751485601354182));
#102753=CARTESIAN_POINT('Ctrl Pts',(0.00244008756654453,-0.0335278710435082,
0.0750300146810709));
#102754=CARTESIAN_POINT('Ctrl Pts',(0.0024229085124138,-0.033362046922432,
0.0749108553879031));
#102755=CARTESIAN_POINT('Ctrl Pts',(0.0024094656434165,-0.0331951640388601,
0.074791020137316));
#102756=CARTESIAN_POINT('Ctrl Pts',(0.00247493684761175,-0.0336938721132426,
0.0752312254722866));
#102757=CARTESIAN_POINT('Ctrl Pts',(0.00245230236004672,-0.0335278710435082,
0.0751129719506977));
#102758=CARTESIAN_POINT('Ctrl Pts',(0.00243338423493337,-0.033362046922432,
0.074994050218778));
#102759=CARTESIAN_POINT('Ctrl Pts',(0.00241819284441114,-0.0331951640388601,
0.0748743979868089));
#102760=CARTESIAN_POINT('Ctrl Pts',(0.00240513095883838,-0.0330240426238155,
0.0747485890416084));
#102761=CARTESIAN_POINT('Ctrl Pts',(0.00239688481161322,-0.0329142774063509,
0.0746698090494448));
#102762=CARTESIAN_POINT('Ctrl Pts',(0.00239026315588202,-0.0328043479726686,
0.0745908193116843));
#102763=CARTESIAN_POINT('Ctrl Pts',(0.00238527726128139,-0.0326943950436594,
0.0745117207864483));
#102764=CARTESIAN_POINT('Ctrl Pts',(0.00233190421744132,-0.0330240426238155,
0.0748350701397107));
#102765=CARTESIAN_POINT('Ctrl Pts',(0.00232246670883535,-0.0329142774063509,
0.0747552813778431));
#102766=CARTESIAN_POINT('Ctrl Pts',(0.00231467395187389,-0.0328043479726686,
0.0746752577387024));
#102767=CARTESIAN_POINT('Ctrl Pts',(0.00230853875293807,-0.0326943950436594,
0.0745951014635975));
#102768=CARTESIAN_POINT('Ctrl Pts',(0.00225867747604425,-0.0330240426238155,
0.0749215512378131));
#102769=CARTESIAN_POINT('Ctrl Pts',(0.00224804860605748,-0.0329142774063509,
0.0748407537062414));
#102770=CARTESIAN_POINT('Ctrl Pts',(0.00223908474786576,-0.0328043479726686,
0.0747596961657204));
#102771=CARTESIAN_POINT('Ctrl Pts',(0.00223180024459474,-0.0326943950436594,
0.0746784821407468));
#102772=CARTESIAN_POINT('Ctrl Pts',(0.00218545073464719,-0.0330240426238155,
0.0750080323359155));
#102773=CARTESIAN_POINT('Ctrl Pts',(0.00217363050327962,-0.0329142774063509,
0.0749262260346396));
#102774=CARTESIAN_POINT('Ctrl Pts',(0.00216349554385763,-0.0328043479726686,
0.0748441345927385));
#102775=CARTESIAN_POINT('Ctrl Pts',(0.00215506173625141,-0.0326943950436594,
0.074761862817896));
#102776=CARTESIAN_POINT('Origin',(0.0191562288082617,-0.0326396682858259,
0.0735280544404682));
#102777=CARTESIAN_POINT('Ctrl Pts',(0.00212948283705904,-0.0331951640388587,
0.0744114865772719));
#102778=CARTESIAN_POINT('Ctrl Pts',(0.00212588138860573,-0.0330855618305429,
0.0743289272338067));
#102779=CARTESIAN_POINT('Ctrl Pts',(0.00212398370434648,-0.0329757224528702,
0.0742462339386878));
#102780=CARTESIAN_POINT('Ctrl Pts',(0.00212379740868786,-0.0328657862230221,
0.0741635124664328));
#102781=CARTESIAN_POINT('Ctrl Pts',(0.00221751748732908,-0.0331951640388587,
0.074482838188266));
#102782=CARTESIAN_POINT('Ctrl Pts',(0.00221293331482264,-0.0330855618305429,
0.0744014913439599));
#102783=CARTESIAN_POINT('Ctrl Pts',(0.00221002713779438,-0.0329757224528702,
0.0743199911108482));
#102784=CARTESIAN_POINT('Ctrl Pts',(0.00220880779714513,-0.0328657862230221,
0.0742384416723138));
#102785=CARTESIAN_POINT('Ctrl Pts',(0.00230555213759912,-0.0331951640388587,
0.0745541897992601));
#102786=CARTESIAN_POINT('Ctrl Pts',(0.00229998524103954,-0.0330855618305429,
0.0744740554541131));
#102787=CARTESIAN_POINT('Ctrl Pts',(0.00229607057124228,-0.0329757224528702,
0.0743937482830087));
#102788=CARTESIAN_POINT('Ctrl Pts',(0.00229381818560241,-0.0328657862230221,
0.0743133708781948));
#102789=CARTESIAN_POINT('Ctrl Pts',(0.00239358678786915,-0.0331951640388587,
0.0746255414102542));
#102790=CARTESIAN_POINT('Ctrl Pts',(0.00238703716725645,-0.0330855618305429,
0.0745466195642662));
#102791=CARTESIAN_POINT('Ctrl Pts',(0.00238211400469018,-0.0329757224528702,
0.0744675054551692));
#102792=CARTESIAN_POINT('Ctrl Pts',(0.00237882857405968,-0.0328657862230221,
0.0743883000840759));
#102793=CARTESIAN_POINT('Origin',(0.0191447208858007,-0.0326401908832289,
0.0740088251132834));
#102794=CARTESIAN_POINT('Ctrl Pts',(0.00239510143721985,-0.0332451089994432,
0.0746602370009251));
#102795=CARTESIAN_POINT('Ctrl Pts',(0.00237585753388324,-0.0329451141710258,
0.0744441762712784));
#102796=CARTESIAN_POINT('Ctrl Pts',(0.00237294287786516,-0.0326442513127503,
0.0742272798178925));
#102797=CARTESIAN_POINT('Ctrl Pts',(0.00242268724997227,-0.0332451089994432,
0.0749087103856865));
#102798=CARTESIAN_POINT('Ctrl Pts',(0.00239407201960647,-0.0329451141710258,
0.0746936900719898));
#102799=CARTESIAN_POINT('Ctrl Pts',(0.00238173429112761,-0.0326442513127503,
0.07447712519218));
#102800=CARTESIAN_POINT('Ctrl Pts',(0.00237882979313201,-0.0325229783203384,
0.0743883316372644));
#102801=CARTESIAN_POINT('Ctrl Pts',(0.00237554439678409,-0.0324130253112079,
0.0743091375955061));
#102802=CARTESIAN_POINT('Ctrl Pts',(0.00237389772918677,-0.0323031222247694,
0.074229887602433));
#102803=CARTESIAN_POINT('Ctrl Pts',(0.00237388831752336,-0.0321934096636184,
0.0741506832460775));
#102804=CARTESIAN_POINT('Ctrl Pts',(0.00230031734761368,-0.0325229783203384,
0.0744700441733171));
#102805=CARTESIAN_POINT('Ctrl Pts',(0.00229590554576372,-0.0324130253112079,
0.074389767839234));
#102806=CARTESIAN_POINT('Ctrl Pts',(0.00229315503211244,-0.0323031222247694,
0.0743094124168426));
#102807=CARTESIAN_POINT('Ctrl Pts',(0.0022920656978263,-0.0321934096636184,
0.0742290809600451));
#102808=CARTESIAN_POINT('Ctrl Pts',(0.00222180490209536,-0.0325229783203384,
0.0745517567093699));
#102809=CARTESIAN_POINT('Ctrl Pts',(0.00221626669474334,-0.0324130253112079,
0.0744703980829619));
#102810=CARTESIAN_POINT('Ctrl Pts',(0.00221241233503811,-0.0323031222247694,
0.0743889372312521));
#102811=CARTESIAN_POINT('Ctrl Pts',(0.00221024307812924,-0.0321934096636184,
0.0743074786740127));
#102812=CARTESIAN_POINT('Ctrl Pts',(0.00214329245657703,-0.0325229783203384,
0.0746334692454226));
#102813=CARTESIAN_POINT('Ctrl Pts',(0.00213662784372297,-0.0324130253112079,
0.0745510283266898));
#102814=CARTESIAN_POINT('Ctrl Pts',(0.00213166963796378,-0.0323031222247694,
0.0744684620456617));
#102815=CARTESIAN_POINT('Ctrl Pts',(0.00212842045843218,-0.0321934096636184,
0.0743858763879803));
#102816=CARTESIAN_POINT('Origin',(0.0191477063303145,-0.0326393375175144,
0.0735282960905243));
#102817=CARTESIAN_POINT('Ctrl Pts',(0.00212489233953397,-0.0326943950436593,
0.074034585422462));
#102818=CARTESIAN_POINT('Ctrl Pts',(0.00212648296872241,-0.0325844576448127,
0.0739519094771622));
#102819=CARTESIAN_POINT('Ctrl Pts',(0.00212978358458001,-0.0324744968375319,
0.0738692605775767));
#102820=CARTESIAN_POINT('Ctrl Pts',(0.00213478849756053,-0.0323646534831895,
0.0737867445599659));
#102821=CARTESIAN_POINT('Ctrl Pts',(0.00220827298940184,-0.0326943950436593,
0.0741113239056972));
#102822=CARTESIAN_POINT('Ctrl Pts',(0.00220880601846805,-0.0325844576448127,
0.0740297971020245));
#102823=CARTESIAN_POINT('Ctrl Pts',(0.00221102519322253,-0.0324744968375319,
0.0739482755524883));
#102824=CARTESIAN_POINT('Ctrl Pts',(0.00221492622964742,-0.0323646534831895,
0.0738668636680338));
#102825=CARTESIAN_POINT('Ctrl Pts',(0.0022916536392697,-0.0326943950436593,
0.0741880623889324));
#102826=CARTESIAN_POINT('Ctrl Pts',(0.00229112906821369,-0.0325844576448127,
0.0741076847268869));
#102827=CARTESIAN_POINT('Ctrl Pts',(0.00229226680186505,-0.0324744968375319,
0.0740272905273999));
#102828=CARTESIAN_POINT('Ctrl Pts',(0.00229506396173432,-0.0323646534831895,
0.0739469827761017));
#102829=CARTESIAN_POINT('Ctrl Pts',(0.00237503428913756,-0.0326943950436593,
0.0742648008721676));
#102830=CARTESIAN_POINT('Ctrl Pts',(0.00237345211795933,-0.0325844576448127,
0.0741855723517493));
#102831=CARTESIAN_POINT('Ctrl Pts',(0.00237350841050757,-0.0324744968375319,
0.0741063055023115));
#102832=CARTESIAN_POINT('Ctrl Pts',(0.00237520169382122,-0.0323646534831895,
0.0740271018841696));
#102833=CARTESIAN_POINT('Origin',(0.0191825504187299,-0.032639557906713,
0.0740078825809728));
#102834=CARTESIAN_POINT('Ctrl Pts',(0.0023743686535863,-0.0327445246961876,
0.0742995625339472));
#102835=CARTESIAN_POINT('Ctrl Pts',(0.00236872781046194,-0.0324436878365474,
0.0740827198596655));
#102836=CARTESIAN_POINT('Ctrl Pts',(0.00237943646868096,-0.0321434074463187,
0.0738660683211528));
#102837=CARTESIAN_POINT('Ctrl Pts',(0.00238629996213717,-0.0327445246961876,
0.0745492776593927));
#102838=CARTESIAN_POINT('Ctrl Pts',(0.00237124095918869,-0.0324436878365474,
0.0743328849817647));
#102839=CARTESIAN_POINT('Ctrl Pts',(0.00237252431799363,-0.0321434074463187,
0.0741159727472298));
#102840=CARTESIAN_POINT('Ctrl Pts',(0.00237653132468067,-0.0322357242816072,
0.0739326697090658));
#102841=CARTESIAN_POINT('Ctrl Pts',(0.00238345301257987,-0.0319819883628706,
0.0737496272228177));
#102842=CARTESIAN_POINT('Ctrl Pts',(0.00240200818985774,-0.0317295851069886,
0.0735673961416831));
#102843=CARTESIAN_POINT('Ctrl Pts',(0.00237251626325928,-0.0322357242816072,
0.07418263746555));
#102844=CARTESIAN_POINT('Ctrl Pts',(0.00237147680231076,-0.0319819883628706,
0.073999467104803));
#102845=CARTESIAN_POINT('Ctrl Pts',(0.0023820951020171,-0.0317295851069886,
0.0738166018176471));
#102846=CARTESIAN_POINT('Origin',(0.0190872499807766,-0.0326371942644308,
0.0740074029677877));
#102847=CARTESIAN_POINT('Origin',(0.0190250368299907,-0.0326352985529686,
0.0735322956715836));
#102848=CARTESIAN_POINT('Ctrl Pts',(0.00214397671962844,-0.0321934096636184,
0.0736581397562614));
#102849=CARTESIAN_POINT('Ctrl Pts',(0.00215075985572215,-0.0320835708272304,
0.0735756735784052));
#102850=CARTESIAN_POINT('Ctrl Pts',(0.00215924569058578,-0.0319739230346346,
0.0734933956109326));
#102851=CARTESIAN_POINT('Ctrl Pts',(0.00216941528808444,-0.0318646057455575,
0.0734114102895471));
#102852=CARTESIAN_POINT('Ctrl Pts',(0.0022223745011053,-0.0321934096636184,
0.0737399624464169));
#102853=CARTESIAN_POINT('Ctrl Pts',(0.00222802923853304,-0.0320835708272304,
0.0736585774350668));
#102854=CARTESIAN_POINT('Ctrl Pts',(0.00223536495456313,-0.0319739230346346,
0.073577356654828));
#102855=CARTESIAN_POINT('Ctrl Pts',(0.00224436428836604,-0.0318646057455575,
0.0734964033017397));
#102856=CARTESIAN_POINT('Ctrl Pts',(0.00230077228258216,-0.0321934096636184,
0.0738217851365724));
#102857=CARTESIAN_POINT('Ctrl Pts',(0.00230529862134393,-0.0320835708272304,
0.0737414812917285));
#102858=CARTESIAN_POINT('Ctrl Pts',(0.00231148421854049,-0.0319739230346346,
0.0736613176987234));
#102859=CARTESIAN_POINT('Ctrl Pts',(0.00231931328864765,-0.0318646057455575,
0.0735813963139323));
#102860=CARTESIAN_POINT('Ctrl Pts',(0.00237917006405902,-0.0321934096636184,
0.073903607826728));
#102861=CARTESIAN_POINT('Ctrl Pts',(0.00238256800415482,-0.0320835708272304,
0.0738243851483901));
#102862=CARTESIAN_POINT('Ctrl Pts',(0.00238760348251784,-0.0319739230346346,
0.0737452787426189));
#102863=CARTESIAN_POINT('Ctrl Pts',(0.00239426228892925,-0.0318646057455575,
0.0736663893261249));
#102864=CARTESIAN_POINT('Ctrl Pts',(0.00237436441908778,-0.03202188345824,
0.0740275538479042));
#102865=CARTESIAN_POINT('Ctrl Pts',(0.00237563878751945,-0.031939109935068,
0.0739677163080037));
#102866=CARTESIAN_POINT('Ctrl Pts',(0.00237784675541944,-0.0318564869454944,
0.0739079349215902));
#102867=CARTESIAN_POINT('Ctrl Pts',(0.00238098264955265,-0.031774074144652,
0.0738482530813361));
#102868=CARTESIAN_POINT('Ctrl Pts',(0.00233784400903193,-0.03202188345824,
0.0740610663485089));
#102869=CARTESIAN_POINT('Ctrl Pts',(0.00233876959334825,-0.031939109935068,
0.0740008487194273));
#102870=CARTESIAN_POINT('Ctrl Pts',(0.00234063492359818,-0.0318564869454944,
0.0739406820278061));
#102871=CARTESIAN_POINT('Ctrl Pts',(0.00234343454991267,-0.031774074144652,
0.0738806099702603));
#102872=CARTESIAN_POINT('Ctrl Pts',(0.00230132359897608,-0.03202188345824,
0.0740945788491135));
#102873=CARTESIAN_POINT('Ctrl Pts',(0.00230190039917705,-0.031939109935068,
0.0740339811308508));
#102874=CARTESIAN_POINT('Ctrl Pts',(0.00230342309177692,-0.0318564869454944,
0.0739734291340219));
#102875=CARTESIAN_POINT('Ctrl Pts',(0.00230588645027268,-0.031774074144652,
0.0739129668591845));
#102876=CARTESIAN_POINT('Ctrl Pts',(0.00226480318892024,-0.03202188345824,
0.0741280913497182));
#102877=CARTESIAN_POINT('Ctrl Pts',(0.00226503120500585,-0.031939109935068,
0.0740671135422743));
#102878=CARTESIAN_POINT('Ctrl Pts',(0.00226621125995567,-0.0318564869454944,
0.0740061762402378));
#102879=CARTESIAN_POINT('Ctrl Pts',(0.0022683383506327,-0.031774074144652,
0.0739453237481087));
#102880=CARTESIAN_POINT('Origin',(-0.00393486782814988,-0.039122885339064,
0.0748352576114155));
#102881=CARTESIAN_POINT('Ctrl Pts',(0.00311177357195213,-0.0352722978779657,
0.076972044316458));
#102882=CARTESIAN_POINT('Ctrl Pts',(0.00310280888108729,-0.0352466642097258,
0.0769554092031193));
#102883=CARTESIAN_POINT('Ctrl Pts',(0.00309378315960661,-0.0352210183808322,
0.076938826103198));
#102884=CARTESIAN_POINT('Ctrl Pts',(0.00308469562127239,-0.0351953608940152,
0.076922294686067));
#102885=CARTESIAN_POINT('Origin',(-0.00128470890169918,-0.0352456003065134,
0.0791355334093028));
#102886=CARTESIAN_POINT('Ctrl Pts',(0.00302707002673582,-0.035024121149334,
0.0768117297446416));
#102887=CARTESIAN_POINT('Ctrl Pts',(0.00299040579250827,-0.0349144232867421,
0.0767415246274487));
#102888=CARTESIAN_POINT('Ctrl Pts',(0.00295517080284304,-0.0348045283677512,
0.076670519613225));
#102889=CARTESIAN_POINT('Ctrl Pts',(0.0029214135736815,-0.0346945769586886,
0.0765988039709136));
#102890=CARTESIAN_POINT('Ctrl Pts',(0.00299082132914393,-0.0350241211493339,
0.0769190944209832));
#102891=CARTESIAN_POINT('Ctrl Pts',(0.00295267819058769,-0.0349144232867421,
0.0768483899928661));
#102892=CARTESIAN_POINT('Ctrl Pts',(0.00291597373251141,-0.0348045283677512,
0.0767768547988486));
#102893=CARTESIAN_POINT('Ctrl Pts',(0.00288075837832923,-0.0346945769586886,
0.0767045787169257));
#102894=CARTESIAN_POINT('Ctrl Pts',(0.00295457263155204,-0.0350241211493339,
0.0770264590973249));
#102895=CARTESIAN_POINT('Ctrl Pts',(0.00291495058866711,-0.0349144232867421,
0.0769552553582835));
#102896=CARTESIAN_POINT('Ctrl Pts',(0.00287677666217978,-0.0348045283677512,
0.0768831899844722));
#102897=CARTESIAN_POINT('Ctrl Pts',(0.00284010318297697,-0.0346945769586886,
0.0768103534629378));
#102898=CARTESIAN_POINT('Ctrl Pts',(0.00291832393396015,-0.0350241211493339,
0.0771338237736666));
#102899=CARTESIAN_POINT('Ctrl Pts',(0.00287722298674654,-0.0349144232867421,
0.0770621207237008));
#102900=CARTESIAN_POINT('Ctrl Pts',(0.00283757959184816,-0.0348045283677512,
0.0769895251700958));
#102901=CARTESIAN_POINT('Ctrl Pts',(0.0027994479876247,-0.0346945769586886,
0.0769161282089499));
#102902=CARTESIAN_POINT('Origin',(0.0181873204939195,-0.0345629067940851,
0.0696120282492125));
#102903=CARTESIAN_POINT('Ctrl Pts',(0.0027357642993283,-0.0351970973651613,
0.0766288676756795));
#102904=CARTESIAN_POINT('Ctrl Pts',(0.00270142294714201,-0.0350869349321765,
0.0765542239898177));
#102905=CARTESIAN_POINT('Ctrl Pts',(0.00266860494784307,-0.0349764985129711,
0.0764788045323143));
#102906=CARTESIAN_POINT('Ctrl Pts',(0.00263735856978515,-0.0348659306849626,
0.0764027045085106));
#102907=CARTESIAN_POINT('Ctrl Pts',(0.00281421943642782,-0.0351970973651613,
0.0766534697510578));
#102908=CARTESIAN_POINT('Ctrl Pts',(0.00277953725582888,-0.0350869349321765,
0.0765799129547951));
#102909=CARTESIAN_POINT('Ctrl Pts',(0.00274635554994655,-0.0349764985129711,
0.0765055742016235));
#102910=CARTESIAN_POINT('Ctrl Pts',(0.00271472297590992,-0.0348659306849626,
0.0764305472690632));
#102911=CARTESIAN_POINT('Ctrl Pts',(0.00289267457352733,-0.0351970973651613,
0.0766780718264362));
#102912=CARTESIAN_POINT('Ctrl Pts',(0.00285765156451574,-0.0350869349321765,
0.0766056019197724));
#102913=CARTESIAN_POINT('Ctrl Pts',(0.00282410615205003,-0.0349764985129711,
0.0765323438709326));
#102914=CARTESIAN_POINT('Ctrl Pts',(0.00279208738203469,-0.0348659306849626,
0.0764583900296157));
#102915=CARTESIAN_POINT('Ctrl Pts',(0.00297112971062685,-0.0351970973651613,
0.0767026739018145));
#102916=CARTESIAN_POINT('Ctrl Pts',(0.00293576587320261,-0.0350869349321765,
0.0766312908847497));
#102917=CARTESIAN_POINT('Ctrl Pts',(0.00290185675415351,-0.0349764985129711,
0.0765591135402418));
#102918=CARTESIAN_POINT('Ctrl Pts',(0.00286945178815946,-0.0348659306849626,
0.0764862327901682));
#102919=CARTESIAN_POINT('Origin',(0.0183426957394639,-0.0345637187969653,
0.070067202818824));
#102920=CARTESIAN_POINT('Ctrl Pts',(0.00298521758930896,-0.0352450361861253,
0.076733269016688));
#102921=CARTESIAN_POINT('Ctrl Pts',(0.00288778800210619,-0.0349452761023765,
0.0765394648774642));
#102922=CARTESIAN_POINT('Ctrl Pts',(0.00280523332246403,-0.0346444289983475,
0.0763388725204015));
#102923=CARTESIAN_POINT('Ctrl Pts',(0.00310233515130371,-0.0352450361861253,
0.0769541388350707));
#102924=CARTESIAN_POINT('Ctrl Pts',(0.00299657532242206,-0.0349452761023765,
0.0767647518570661));
#102925=CARTESIAN_POINT('Ctrl Pts',(0.00290538134779148,-0.0346444289983475,
0.0765679366446615));
#102926=CARTESIAN_POINT('Ctrl Pts',(0.00286999617619118,-0.0345231616327822,
0.0764864531348779));
#102927=CARTESIAN_POINT('Ctrl Pts',(0.00283779145918998,-0.0344132092796975,
0.0764140370913742));
#102928=CARTESIAN_POINT('Ctrl Pts',(0.00280708627254303,-0.0343032738558974,
0.0763409586550371));
#102929=CARTESIAN_POINT('Ctrl Pts',(0.00277791755498236,-0.0341934961088741,
0.0762673124554182));
#102930=CARTESIAN_POINT('Ctrl Pts',(0.00282707754957742,-0.0345231616327822,
0.0765913298607428));
#102931=CARTESIAN_POINT('Ctrl Pts',(0.00279342725456481,-0.0344132092796975,
0.0765183222443958));
#102932=CARTESIAN_POINT('Ctrl Pts',(0.00276128880070926,-0.0343032738558974,
0.0764446223650969));
#102933=CARTESIAN_POINT('Ctrl Pts',(0.0027307009425303,-0.0341934961088741,
0.0763703256955726));
#102934=CARTESIAN_POINT('Ctrl Pts',(0.00278415892296366,-0.0345231616327822,
0.0766962065866076));
#102935=CARTESIAN_POINT('Ctrl Pts',(0.00274906304993963,-0.0344132092796975,
0.0766226073974174));
#102936=CARTESIAN_POINT('Ctrl Pts',(0.00271549132887548,-0.0343032738558974,
0.0765482860751567));
#102937=CARTESIAN_POINT('Ctrl Pts',(0.00268348433007824,-0.0341934961088741,
0.0764733389357269));
#102938=CARTESIAN_POINT('Ctrl Pts',(0.00274124029634991,-0.0345231616327822,
0.0768010833124725));
#102939=CARTESIAN_POINT('Ctrl Pts',(0.00270469884531446,-0.0344132092796975,
0.076726892550439));
#102940=CARTESIAN_POINT('Ctrl Pts',(0.0026696938570417,-0.0343032738558974,
0.0766519497852166));
#102941=CARTESIAN_POINT('Ctrl Pts',(0.00263626771762619,-0.0341934961088741,
0.0765763521758813));
#102942=CARTESIAN_POINT('Origin',(0.0181982488773147,-0.0345625596229882,
0.0696068254875496));
#102943=CARTESIAN_POINT('Ctrl Pts',(0.00250366852609144,-0.0346945769586886,
0.0762510288836281));
#102944=CARTESIAN_POINT('Ctrl Pts',(0.00247471528617795,-0.0345846629178476,
0.0761735808767919));
#102945=CARTESIAN_POINT('Ctrl Pts',(0.00244735869395167,-0.034474692505516,
0.0760955209005362));
#102946=CARTESIAN_POINT('Ctrl Pts',(0.00242163338876489,-0.0343648066260528,
0.0760169491190588));
#102947=CARTESIAN_POINT('Ctrl Pts',(0.00260944318882002,-0.0346945769586886,
0.0762916840469698));
#102948=CARTESIAN_POINT('Ctrl Pts',(0.00257992970020784,-0.0345846629178476,
0.0762156936684464));
#102949=CARTESIAN_POINT('Ctrl Pts',(0.00255198262043619,-0.034474692505516,
0.076139079983757));
#102950=CARTESIAN_POINT('Ctrl Pts',(0.00252563735311132,-0.0343648066260528,
0.0760619413070686));
#102951=CARTESIAN_POINT('Ctrl Pts',(0.00271521785154859,-0.0346945769586886,
0.0763323392103115));
#102952=CARTESIAN_POINT('Ctrl Pts',(0.00268514411423773,-0.0345846629178476,
0.0762578064601009));
#102953=CARTESIAN_POINT('Ctrl Pts',(0.00265660654692071,-0.034474692505516,
0.0761826390669778));
#102954=CARTESIAN_POINT('Ctrl Pts',(0.00262964131745774,-0.0343648066260528,
0.0761069334950785));
#102955=CARTESIAN_POINT('Ctrl Pts',(0.00282099251427717,-0.0346945769586886,
0.0763729943736532));
#102956=CARTESIAN_POINT('Ctrl Pts',(0.00279035852826763,-0.0345846629178476,
0.0762999192517554));
#102957=CARTESIAN_POINT('Ctrl Pts',(0.00276123047340524,-0.034474692505516,
0.0762261981501985));
#102958=CARTESIAN_POINT('Ctrl Pts',(0.00273364528180416,-0.0343648066260528,
0.0761519256830883));
#102959=CARTESIAN_POINT('Origin',(0.0183966622133401,-0.0345626446730873,
0.070044803033538));
#102960=CARTESIAN_POINT('Ctrl Pts',(0.00281909985087201,-0.0346945769586886,
0.0763722669164541));
#102961=CARTESIAN_POINT('Ctrl Pts',(0.00277255358056049,-0.0345275153362891,
0.0762611582209188));
#102962=CARTESIAN_POINT('Ctrl Pts',(0.00272948953720534,-0.0343603235965159,
0.0761485569496254));
#102963=CARTESIAN_POINT('Ctrl Pts',(0.00269003013551802,-0.034193496108874,
0.076034798020116));
#102964=CARTESIAN_POINT('Ctrl Pts',(0.00285316508107882,-0.0346945769586886,
0.0764488671019775));
#102965=CARTESIAN_POINT('Ctrl Pts',(0.00280501438921249,-0.0345275153362891,
0.0763384719163279));
#102966=CARTESIAN_POINT('Ctrl Pts',(0.00276032307008778,-0.0343603235965159,
0.0762265338818892));
#102967=CARTESIAN_POINT('Ctrl Pts',(0.00271921838032941,-0.034193496108874,
0.0761133860261735));
#102968=CARTESIAN_POINT('Ctrl Pts',(0.00288723031128562,-0.0346945769586886,
0.0765254672875009));
#102969=CARTESIAN_POINT('Ctrl Pts',(0.00283747519786449,-0.0345275153362891,
0.0764157856117369));
#102970=CARTESIAN_POINT('Ctrl Pts',(0.00279115660297022,-0.0343603235965159,
0.0763045108141529));
#102971=CARTESIAN_POINT('Ctrl Pts',(0.00274840662514081,-0.034193496108874,
0.076191974032231));
#102972=CARTESIAN_POINT('Ctrl Pts',(0.00292129554149242,-0.0346945769586886,
0.0766020674730243));
#102973=CARTESIAN_POINT('Ctrl Pts',(0.00286993600651649,-0.0345275153362891,
0.076493099307146));
#102974=CARTESIAN_POINT('Ctrl Pts',(0.00282199013585266,-0.0343603235965159,
0.0763824877464167));
#102975=CARTESIAN_POINT('Ctrl Pts',(0.0027775948699522,-0.034193496108874,
0.0762705620382886));
#102976=CARTESIAN_POINT('Ctrl Pts',(0.00273365678984782,-0.0340223579322365,
0.0761519550687527));
#102977=CARTESIAN_POINT('Ctrl Pts',(0.00270604460813198,-0.0339125849573554,
0.0760776111814053));
#102978=CARTESIAN_POINT('Ctrl Pts',(0.00267999057489329,-0.0338030433565222,
0.076002748026647));
#102979=CARTESIAN_POINT('Ctrl Pts',(0.00265551952213465,-0.0336938721132328,
0.075927464295398));
#102980=CARTESIAN_POINT('Ctrl Pts',(0.00268423752151511,-0.0340223579322365,
0.0762539301429025));
#102981=CARTESIAN_POINT('Ctrl Pts',(0.00265521883756461,-0.0339125849573554,
0.0761789046349539));
#102982=CARTESIAN_POINT('Ctrl Pts',(0.00262777339838666,-0.0338030433565222,
0.0761033312272334));
#102983=CARTESIAN_POINT('Ctrl Pts',(0.0026019277348414,-0.0336938721132328,
0.0760273096766888));
#102984=CARTESIAN_POINT('Ctrl Pts',(0.00263481825318241,-0.0340223579322365,
0.0763559052170523));
#102985=CARTESIAN_POINT('Ctrl Pts',(0.00260439306699723,-0.0339125849573554,
0.0762801980885026));
#102986=CARTESIAN_POINT('Ctrl Pts',(0.00257555622188002,-0.0338030433565222,
0.0762039144278198));
#102987=CARTESIAN_POINT('Ctrl Pts',(0.00254833594754816,-0.0336938721132328,
0.0761271550579797));
#102988=CARTESIAN_POINT('Ctrl Pts',(0.00258539898484971,-0.0340223579322365,
0.0764578802912021));
#102989=CARTESIAN_POINT('Ctrl Pts',(0.00255356729642986,-0.0339125849573554,
0.0763814915420512));
#102990=CARTESIAN_POINT('Ctrl Pts',(0.00252333904537339,-0.0338030433565222,
0.0763044976284062));
#102991=CARTESIAN_POINT('Ctrl Pts',(0.00249474416025491,-0.0336938721132328,
0.0762270004392705));
#102992=CARTESIAN_POINT('Origin',(0.0180876165588606,-0.0345589643416277,
0.0696538719354821));
#102993=CARTESIAN_POINT('Ctrl Pts',(0.00238283384147149,-0.034193496108874,
0.0758939931260948));
#102994=CARTESIAN_POINT('Ctrl Pts',(0.00235878520901436,-0.0340836138581107,
0.0758148288479804));
#102995=CARTESIAN_POINT('Ctrl Pts',(0.00233638625416955,-0.03397388966435,
0.075735204918387));
#102996=CARTESIAN_POINT('Ctrl Pts',(0.00231565881338707,-0.0338644633294063,
0.0756552251678614));
#102997=CARTESIAN_POINT('Ctrl Pts',(0.0024858471743151,-0.034193496108874,
0.0759412097810315));
#102998=CARTESIAN_POINT('Ctrl Pts',(0.00246114745214699,-0.0340836138581107,
0.0758634659957749));
#102999=CARTESIAN_POINT('Ctrl Pts',(0.00243806832587719,-0.03397388966435,
0.0757852484045248));
#103000=CARTESIAN_POINT('Ctrl Pts',(0.0024166326231499,-0.0338644633294063,
0.0757066590962446));
#103001=CARTESIAN_POINT('Ctrl Pts',(0.00258886050715872,-0.034193496108874,
0.0759884264359681));
#103002=CARTESIAN_POINT('Ctrl Pts',(0.00256350969527962,-0.0340836138581107,
0.0759121031435693));
#103003=CARTESIAN_POINT('Ctrl Pts',(0.00253975039758483,-0.03397388966435,
0.0758352918906625));
#103004=CARTESIAN_POINT('Ctrl Pts',(0.00251760643291272,-0.0338644633294063,
0.0757580930246279));
#103005=CARTESIAN_POINT('Ctrl Pts',(0.00269187384000233,-0.034193496108874,
0.0760356430909048));
#103006=CARTESIAN_POINT('Ctrl Pts',(0.00266587193841225,-0.0340836138581107,
0.0759607402913638));
#103007=CARTESIAN_POINT('Ctrl Pts',(0.00264143246929247,-0.03397388966435,
0.0758853353768002));
#103008=CARTESIAN_POINT('Ctrl Pts',(0.00261858024267554,-0.0338644633294063,
0.0758095269530112));
#103009=CARTESIAN_POINT('Origin',(0.0183263451466634,-0.0345610621861401,
0.0700716741294723));
#103010=CARTESIAN_POINT('Ctrl Pts',(0.00270199343856667,-0.03424362768739,
0.0760689402547046));
#103011=CARTESIAN_POINT('Ctrl Pts',(0.00262961941376101,-0.033943005420186,
0.0758644541208345));
#103012=CARTESIAN_POINT('Ctrl Pts',(0.00257285372943111,-0.0336441434784162,
0.0756550974025419));
#103013=CARTESIAN_POINT('Ctrl Pts',(0.00279050835634744,-0.03424362768739,
0.0763027459632112));
#103014=CARTESIAN_POINT('Ctrl Pts',(0.00270931620387696,-0.033943005420186,
0.0761015982244992));
#103015=CARTESIAN_POINT('Ctrl Pts',(0.00264350598165653,-0.0336441434784162,
0.0758949061998273));
#103016=CARTESIAN_POINT('Ctrl Pts',(0.00261858836761115,-0.0335235895815127,
0.0758095534674062));
#103017=CARTESIAN_POINT('Ctrl Pts',(0.00259574134677251,-0.0334144449262719,
0.0757337636356701));
#103018=CARTESIAN_POINT('Ctrl Pts',(0.00257443383836038,-0.0333049234473133,
0.0756574147283433));
#103019=CARTESIAN_POINT('Ctrl Pts',(0.00255470193159522,-0.0331951640388589,
0.0755806019041989));
#103020=CARTESIAN_POINT('Ctrl Pts',(0.0025628635199683,-0.0335235895815127,
0.0759082242018796));
#103021=CARTESIAN_POINT('Ctrl Pts',(0.00253865810220486,-0.0334144449262719,
0.0758316672079036));
#103022=CARTESIAN_POINT('Ctrl Pts',(0.00251600648522894,-0.0333049234473133,
0.0757545221935022));
#103023=CARTESIAN_POINT('Ctrl Pts',(0.00249494656917595,-0.0331951640388589,
0.0756768851797377));
#103024=CARTESIAN_POINT('Ctrl Pts',(0.00250713867232545,-0.0335235895815127,
0.076006894936353));
#103025=CARTESIAN_POINT('Ctrl Pts',(0.0024815748576372,-0.0334144449262719,
0.0759295707801371));
#103026=CARTESIAN_POINT('Ctrl Pts',(0.00245757913209751,-0.0333049234473133,
0.0758516296586612));
#103027=CARTESIAN_POINT('Ctrl Pts',(0.00243519120675668,-0.0331951640388589,
0.0757731684552765));
#103028=CARTESIAN_POINT('Ctrl Pts',(0.0024514138246826,-0.0335235895815127,
0.0761055656708264));
#103029=CARTESIAN_POINT('Ctrl Pts',(0.00242449161306955,-0.0334144449262719,
0.0760274743523705));
#103030=CARTESIAN_POINT('Ctrl Pts',(0.00239915177896608,-0.0333049234473133,
0.0759487371238201));
#103031=CARTESIAN_POINT('Ctrl Pts',(0.00237543584433741,-0.0331951640388589,
0.0758694517308153));
#103032=CARTESIAN_POINT('Origin',(0.0188701760354181,-0.0326434571770769,
0.0721752904886176));
#103033=CARTESIAN_POINT('Ctrl Pts',(0.00228286956380782,-0.0336938721132422,
0.0755291157280789));
#103034=CARTESIAN_POINT('Ctrl Pts',(0.00227479714181198,-0.0336474569764974,
0.0754949269282381));
#103035=CARTESIAN_POINT('Ctrl Pts',(0.00226712549601245,-0.033601104548885,
0.0754606459731441));
#103036=CARTESIAN_POINT('Ctrl Pts',(0.00224770265350699,-0.0334837508643185,
0.0753738544802717));
#103037=CARTESIAN_POINT('Ctrl Pts',(0.00223086015185338,-0.0333660264760453,
0.0752865255607544));
#103038=CARTESIAN_POINT('Ctrl Pts',(0.00258240495709203,-0.0336938721132422,
0.0756898906870816));
#103039=CARTESIAN_POINT('Ctrl Pts',(0.00257339146591032,-0.0336474569764974,
0.0756574551672941));
#103040=CARTESIAN_POINT('Ctrl Pts',(0.00256475829105089,-0.033601104548885,
0.0756249163557145));
#103041=CARTESIAN_POINT('Ctrl Pts',(0.00254290107814002,-0.0334837508643185,
0.0755425355694867));
#103042=CARTESIAN_POINT('Ctrl Pts',(0.00252349457669983,-0.0333660264760453,
0.0754595432843177));
#103043=CARTESIAN_POINT('Ctrl Pts',(0.00258240495710018,-0.0336938721132426,
0.0756898906870849));
#103044=CARTESIAN_POINT('Ctrl Pts',(0.00257339146591944,-0.0336474569765026,
0.0756574551673007));
#103045=CARTESIAN_POINT('Ctrl Pts',(0.00256475829106089,-0.0336011045488949,
0.0756249163557245));
#103046=CARTESIAN_POINT('Ctrl Pts',(0.00254308311896268,-0.0334847282606778,
0.0755432216892383));
#103047=CARTESIAN_POINT('Ctrl Pts',(0.00252381793631918,-0.0333679869945435,
0.0754609253688133));
#103048=CARTESIAN_POINT('Ctrl Pts',(0.00258240495709209,-0.0336938721132425,
0.0756898906870818));
#103049=CARTESIAN_POINT('Ctrl Pts',(0.00255016872376089,-0.0335278710435082,
0.0755738869141809));
#103050=CARTESIAN_POINT('Ctrl Pts',(0.00252158167921933,-0.033362046922432,
0.075456913031242));
#103051=CARTESIAN_POINT('Ctrl Pts',(0.00249664906299867,-0.0331951640388602,
0.0753389061090021));
#103052=CARTESIAN_POINT('Ctrl Pts',(0.00260660102640909,-0.0336938721132425,
0.0757701563712369));
#103053=CARTESIAN_POINT('Ctrl Pts',(0.00257268450281793,-0.0335278710435082,
0.0756546591213917));
#103054=CARTESIAN_POINT('Ctrl Pts',(0.00254240187470728,-0.033362046922432,
0.0755381388898491));
#103055=CARTESIAN_POINT('Ctrl Pts',(0.00251575746289138,-0.0331951640388602,
0.0754205326909275));
#103056=CARTESIAN_POINT('Ctrl Pts',(0.00263079709572609,-0.0336938721132425,
0.075850422055392));
#103057=CARTESIAN_POINT('Ctrl Pts',(0.00259520028187497,-0.0335278710435082,
0.0757354313286024));
#103058=CARTESIAN_POINT('Ctrl Pts',(0.00256322207019523,-0.033362046922432,
0.0756193647484562));
#103059=CARTESIAN_POINT('Ctrl Pts',(0.00253486586278409,-0.0331951640388602,
0.0755021592728528));
#103060=CARTESIAN_POINT('Ctrl Pts',(0.00265499316504309,-0.0336938721132425,
0.075930687739547));
#103061=CARTESIAN_POINT('Ctrl Pts',(0.00261771606093201,-0.0335278710435082,
0.0758162035358132));
#103062=CARTESIAN_POINT('Ctrl Pts',(0.00258404226568318,-0.033362046922432,
0.0757005906070632));
#103063=CARTESIAN_POINT('Ctrl Pts',(0.0025539742626768,-0.0331951640388602,
0.0755837858547782));
#103064=CARTESIAN_POINT('Ctrl Pts',(0.00252524733205986,-0.0330240426238155,
0.075460606039043));
#103065=CARTESIAN_POINT('Ctrl Pts',(0.00250719245701054,-0.0329142774063509,
0.0753834807669443));
#103066=CARTESIAN_POINT('Ctrl Pts',(0.00249072297576066,-0.0328043479726686,
0.0753059438003835));
#103067=CARTESIAN_POINT('Ctrl Pts',(0.00247586272249016,-0.0326943950436594,
0.075228093888937));
#103068=CARTESIAN_POINT('Ctrl Pts',(0.00246343696105782,-0.0330240426238155,
0.0755555829521389));
#103069=CARTESIAN_POINT('Ctrl Pts',(0.00244407368649909,-0.0329142774063509,
0.0754776061819607));
#103070=CARTESIAN_POINT('Ctrl Pts',(0.00242631275629876,-0.0328043479726686,
0.0753991902445449));
#103071=CARTESIAN_POINT('Ctrl Pts',(0.00241017969008967,-0.0326943950436594,
0.0753204349699319));
#103072=CARTESIAN_POINT('Ctrl Pts',(0.00240162659005577,-0.0330240426238155,
0.0756505598652348));
#103073=CARTESIAN_POINT('Ctrl Pts',(0.00238095491598763,-0.0329142774063509,
0.0755717315969771));
#103074=CARTESIAN_POINT('Ctrl Pts',(0.00236190253683687,-0.0328043479726686,
0.0754924366887063));
#103075=CARTESIAN_POINT('Ctrl Pts',(0.00234449665768919,-0.0326943950436594,
0.0754127760509268));
#103076=CARTESIAN_POINT('Ctrl Pts',(0.00233981621905373,-0.0330240426238155,
0.0757455367783307));
#103077=CARTESIAN_POINT('Ctrl Pts',(0.00231783614547617,-0.0329142774063509,
0.0756658570119935));
#103078=CARTESIAN_POINT('Ctrl Pts',(0.00229749231737497,-0.0328043479726686,
0.0755856831328677));
#103079=CARTESIAN_POINT('Ctrl Pts',(0.0022788136252887,-0.0326943950436594,
0.0755051171319217));
#103080=CARTESIAN_POINT('Origin',(0.0189912842235296,-0.0326396682855742,
0.0721502264588975));
#103081=CARTESIAN_POINT('Ctrl Pts',(0.00220952263615499,-0.0331951640388587,
0.0751607095987539));
#103082=CARTESIAN_POINT('Ctrl Pts',(0.00219560215608103,-0.0330855618255041,
0.0750792526378066));
#103083=CARTESIAN_POINT('Ctrl Pts',(0.0021833552170716,-0.0329757224427708,
0.0749974492431467));
#103084=CARTESIAN_POINT('Ctrl Pts',(0.00217280264047757,-0.0328657862078596,
0.0749154033996513));
#103085=CARTESIAN_POINT('Ctrl Pts',(0.00230580583503894,-0.0331951640388587,
0.0752204649135996));
#103086=CARTESIAN_POINT('Ctrl Pts',(0.00229106234638699,-0.0330855618255041,
0.0751403340589375));
#103087=CARTESIAN_POINT('Ctrl Pts',(0.00227796439715407,-0.0329757224427708,
0.075059840716354));
#103088=CARTESIAN_POINT('Ctrl Pts',(0.00226653381617092,-0.0328657862078596,
0.07497908713967));
#103089=CARTESIAN_POINT('Ctrl Pts',(0.00240208903392289,-0.0331951640388587,
0.0752802202284453));
#103090=CARTESIAN_POINT('Ctrl Pts',(0.00238652253669296,-0.0330855618255041,
0.0752014154800685));
#103091=CARTESIAN_POINT('Ctrl Pts',(0.00237257357723654,-0.0329757224427708,
0.0751222321895612));
#103092=CARTESIAN_POINT('Ctrl Pts',(0.00236026499186427,-0.0328657862078596,
0.0750427708796888));
#103093=CARTESIAN_POINT('Ctrl Pts',(0.00249837223280683,-0.0331951640388587,
0.075339975543291));
#103094=CARTESIAN_POINT('Ctrl Pts',(0.00248198272699892,-0.0330855618255041,
0.0752624969011995));
#103095=CARTESIAN_POINT('Ctrl Pts',(0.00246718275731901,-0.0329757224427708,
0.0751846236627685));
#103096=CARTESIAN_POINT('Ctrl Pts',(0.00245399616755762,-0.0328657862078596,
0.0751064546197075));
#103097=CARTESIAN_POINT('Origin',(0.0190401235886673,-0.0326401908834989,
0.0726286484355253));
#103098=CARTESIAN_POINT('Ctrl Pts',(0.00250422344926411,-0.0332451089994432,
0.0753742077129654));
#103099=CARTESIAN_POINT('Ctrl Pts',(0.00245805169996031,-0.0329451141710258,
0.0751622625873378));
#103100=CARTESIAN_POINT('Ctrl Pts',(0.00242797569302402,-0.0326442513127503,
0.0749474417305342));
#103101=CARTESIAN_POINT('Ctrl Pts',(0.00256273371241031,-0.0332451089994432,
0.0756172643917598));
#103102=CARTESIAN_POINT('Ctrl Pts',(0.00250739493048529,-0.0329451141710258,
0.0754075260168111));
#103103=CARTESIAN_POINT('Ctrl Pts',(0.00246801171201756,-0.0326442513127503,
0.0751942151431685));
#103104=CARTESIAN_POINT('Ctrl Pts',(0.00245400133349894,-0.0325229783203385,
0.0751064857820804));
#103105=CARTESIAN_POINT('Ctrl Pts',(0.00244081619814992,-0.032413025311208,
0.0750283279783433));
#103106=CARTESIAN_POINT('Ctrl Pts',(0.00242924985712664,-0.0323031222247695,
0.074949909277311));
#103107=CARTESIAN_POINT('Ctrl Pts',(0.00241931358158259,-0.0321934096636184,
0.0748713306505568));
#103108=CARTESIAN_POINT('Ctrl Pts',(0.00238634927843028,-0.0325229783203385,
0.0751973942090519));
#103109=CARTESIAN_POINT('Ctrl Pts',(0.0023719109724263,-0.032413025311208,
0.0751183038232321));
#103110=CARTESIAN_POINT('Ctrl Pts',(0.00235911094247396,-0.0323031222247695,
0.0750389267581171));
#103111=CARTESIAN_POINT('Ctrl Pts',(0.00234796199667667,-0.0321934096636184,
0.0749593652686388));
#103112=CARTESIAN_POINT('Ctrl Pts',(0.00231869722336161,-0.0325229783203385,
0.0752883026360234));
#103113=CARTESIAN_POINT('Ctrl Pts',(0.00230300574670268,-0.032413025311208,
0.0752082796681209));
#103114=CARTESIAN_POINT('Ctrl Pts',(0.00228897202782127,-0.0323031222247695,
0.0751279442389232));
#103115=CARTESIAN_POINT('Ctrl Pts',(0.00227661041177075,-0.0321934096636184,
0.0750473998867209));
#103116=CARTESIAN_POINT('Ctrl Pts',(0.00225104516829294,-0.0325229783203385,
0.0753792110629949));
#103117=CARTESIAN_POINT('Ctrl Pts',(0.00223410052097905,-0.032413025311208,
0.0752982555130097));
#103118=CARTESIAN_POINT('Ctrl Pts',(0.00221883311316859,-0.0323031222247695,
0.0752169617197293));
#103119=CARTESIAN_POINT('Ctrl Pts',(0.00220525882686484,-0.0321934096636184,
0.075135434504803));
#103120=CARTESIAN_POINT('Origin',(0.0189828592343901,-0.032639337517782,
0.0721515343525047));
#103121=CARTESIAN_POINT('Ctrl Pts',(0.00215773009560759,-0.0326943950436594,
0.0747873557640232));
#103122=CARTESIAN_POINT('Ctrl Pts',(0.00214894613864736,-0.0325844576448127,
0.0747051323845465));
#103123=CARTESIAN_POINT('Ctrl Pts',(0.00214186207432751,-0.0324744968375319,
0.0746227215193621));
#103124=CARTESIAN_POINT('Ctrl Pts',(0.00213648552276626,-0.0323646534831895,
0.0745402288832689));
#103125=CARTESIAN_POINT('Ctrl Pts',(0.00225007114638938,-0.0326943950436594,
0.0748530387749328));
#103126=CARTESIAN_POINT('Ctrl Pts',(0.00224038195443574,-0.0325844576448127,
0.0747720880282014));
#103127=CARTESIAN_POINT('Ctrl Pts',(0.00223236627092589,-0.0324744968375319,
0.0746909311640848));
#103128=CARTESIAN_POINT('Ctrl Pts',(0.00222603293178415,-0.0323646534831895,
0.0746096723071463));
#103129=CARTESIAN_POINT('Ctrl Pts',(0.00234241219717117,-0.0326943950436594,
0.0749187217858424));
#103130=CARTESIAN_POINT('Ctrl Pts',(0.00233181777022411,-0.0325844576448127,
0.0748390436718564));
#103131=CARTESIAN_POINT('Ctrl Pts',(0.00232287046752428,-0.0324744968375319,
0.0747591408088074));
#103132=CARTESIAN_POINT('Ctrl Pts',(0.00231558034080203,-0.0323646534831895,
0.0746791157310237));
#103133=CARTESIAN_POINT('Ctrl Pts',(0.00243475324795296,-0.0326943950436594,
0.074984404796752));
#103134=CARTESIAN_POINT('Ctrl Pts',(0.00242325358601249,-0.0325844576448127,
0.0749059993155113));
#103135=CARTESIAN_POINT('Ctrl Pts',(0.00241337466412267,-0.0324744968375319,
0.0748273504535301));
#103136=CARTESIAN_POINT('Ctrl Pts',(0.00240512774981991,-0.0323646534831895,
0.0747485591549012));
#103137=CARTESIAN_POINT('Origin',(0.0190775366925626,-0.0326395579068863,
0.0726229720380674));
#103138=CARTESIAN_POINT('Ctrl Pts',(0.0024384496526117,-0.0327445246961877,
0.0750189757787017));
#103139=CARTESIAN_POINT('Ctrl Pts',(0.00240567569567775,-0.0324436878365475,
0.0748045499587832));
#103140=CARTESIAN_POINT('Ctrl Pts',(0.0023891462750497,-0.0321434074463187,
0.0745882646316005));
#103141=CARTESIAN_POINT('Ctrl Pts',(0.00248158448337294,-0.0327445246961877,
0.0752652264363154));
#103142=CARTESIAN_POINT('Ctrl Pts',(0.00243952303115385,-0.0324436878365475,
0.0750524274731176));
#103143=CARTESIAN_POINT('Ctrl Pts',(0.00241360995853735,-0.0321434074463187,
0.0748370648088316));
#103144=CARTESIAN_POINT('Ctrl Pts',(0.00239461140628459,-0.0322357242816073,
0.0746547049587685));
#103145=CARTESIAN_POINT('Ctrl Pts',(0.00237853720792616,-0.0319819883628706,
0.0744722382996705));
#103146=CARTESIAN_POINT('Ctrl Pts',(0.00237410646143453,-0.0317295851069886,
0.0742891185846729));
#103147=CARTESIAN_POINT('Ctrl Pts',(0.00242195727202873,-0.0322357242816073,
0.074903204865462));
#103148=CARTESIAN_POINT('Ctrl Pts',(0.00239796867393468,-0.0319819883628706,
0.0747216091367218));
#103149=CARTESIAN_POINT('Ctrl Pts',(0.00238558414743039,-0.0317295851069886,
0.074538854971137));
#103150=CARTESIAN_POINT('Origin',(0.0189829276155652,-0.0326371942643099,
0.0726344405192385));
#103151=CARTESIAN_POINT('Origin',(0.0188616583006038,-0.0326352985525182,
0.0721708769617584));
#103152=CARTESIAN_POINT('Ctrl Pts',(0.00212948283705859,-0.0321934096636183,
0.0744114865772715));
#103153=CARTESIAN_POINT('Ctrl Pts',(0.00212587673336777,-0.0320835708272303,
0.0743288205174788));
#103154=CARTESIAN_POINT('Ctrl Pts',(0.00212398349117446,-0.0319739230346346,
0.0742461277792319));
#103155=CARTESIAN_POINT('Ctrl Pts',(0.00212379741292528,-0.0318646057455575,
0.0741635143480549));
#103156=CARTESIAN_POINT('Ctrl Pts',(0.00221751753094838,-0.0321934096636183,
0.0744828382236192));
#103157=CARTESIAN_POINT('Ctrl Pts',(0.00221292743244634,-0.0320835708272303,
0.0744013862308653));
#103158=CARTESIAN_POINT('Ctrl Pts',(0.00221002564114451,-0.0319739230346346,
0.0743198864917275));
#103159=CARTESIAN_POINT('Ctrl Pts',(0.00220880786700199,-0.0318646057455575,
0.0742384435644025));
#103160=CARTESIAN_POINT('Ctrl Pts',(0.00230555222483818,-0.0321934096636183,
0.0745541898699668));
#103161=CARTESIAN_POINT('Ctrl Pts',(0.00229997813152491,-0.0320835708272303,
0.0744739519442518));
#103162=CARTESIAN_POINT('Ctrl Pts',(0.00229606779111457,-0.0319739230346346,
0.0743936452042231));
#103163=CARTESIAN_POINT('Ctrl Pts',(0.0022938183210787,-0.0318646057455575,
0.0743133727807501));
#103164=CARTESIAN_POINT('Ctrl Pts',(0.00239358691872797,-0.0321934096636183,
0.0746255415163145));
#103165=CARTESIAN_POINT('Ctrl Pts',(0.00238702883060348,-0.0320835708272303,
0.0745465176576383));
#103166=CARTESIAN_POINT('Ctrl Pts',(0.00238210994108463,-0.0319739230346346,
0.0744674039167187));
#103167=CARTESIAN_POINT('Ctrl Pts',(0.00237882877515541,-0.0318646057455575,
0.0743883019970977));
#103168=CARTESIAN_POINT('Ctrl Pts',(0.00240435372332806,-0.03202188345824,
0.0747491124931118));
#103169=CARTESIAN_POINT('Ctrl Pts',(0.00239811841061979,-0.0319391099350678,
0.0746895870693697));
#103170=CARTESIAN_POINT('Ctrl Pts',(0.00239281637356727,-0.031856486945494,
0.0746300003452872));
#103171=CARTESIAN_POINT('Ctrl Pts',(0.00238844742221453,-0.0317740741446515,
0.0745703960824178));
#103172=CARTESIAN_POINT('Ctrl Pts',(0.00237232151767753,-0.03202188345824,
0.0747869379587249));
#103173=CARTESIAN_POINT('Ctrl Pts',(0.0023656925333147,-0.0319391099350678,
0.0747270791571593));
#103174=CARTESIAN_POINT('Ctrl Pts',(0.00236000226886473,-0.031856486945494,
0.0746671531100005));
#103175=CARTESIAN_POINT('Ctrl Pts',(0.00235525079407047,-0.0317740741446515,
0.0746072038523523));
#103176=CARTESIAN_POINT('Ctrl Pts',(0.002340289312027,-0.03202188345824,
0.074824763424338));
#103177=CARTESIAN_POINT('Ctrl Pts',(0.00233326665600961,-0.0319391099350678,
0.074764571244949));
#103178=CARTESIAN_POINT('Ctrl Pts',(0.00232718816416218,-0.031856486945494,
0.0747043058747137));
#103179=CARTESIAN_POINT('Ctrl Pts',(0.00232205416592641,-0.0317740741446515,
0.0746440116222868));
#103180=CARTESIAN_POINT('Ctrl Pts',(0.00230825710637647,-0.03202188345824,
0.0748625888899511));
#103181=CARTESIAN_POINT('Ctrl Pts',(0.00230084077870451,-0.0319391099350678,
0.0748020633327386));
#103182=CARTESIAN_POINT('Ctrl Pts',(0.00229437405945963,-0.031856486945494,
0.074741458639427));
#103183=CARTESIAN_POINT('Ctrl Pts',(0.00228885753778234,-0.0317740741446515,
0.0746808193922213));
#103184=CARTESIAN_POINT('Origin',(-0.00375389621872825,-0.0391228853390656,
0.0763412037500568));
#103185=CARTESIAN_POINT('Ctrl Pts',(0.00350499069638799,-0.0352722978779661,
0.0775779629012608));
#103186=CARTESIAN_POINT('Ctrl Pts',(0.00349401176224274,-0.0352466642097261,
0.0775625825344534));
#103187=CARTESIAN_POINT('Ctrl Pts',(0.00348297879773608,-0.0352210183808323,
0.0775472614200865));
#103188=CARTESIAN_POINT('Ctrl Pts',(0.00347189098139146,-0.0351953608940152,
0.0775319993286817));
#103189=CARTESIAN_POINT('Origin',(-0.000585667115997817,-0.0352456003065141,
0.0802754176011314));
#103190=CARTESIAN_POINT('Ctrl Pts',(0.00340086232025206,-0.035024121149334,
0.0774295286269429));
#103191=CARTESIAN_POINT('Ctrl Pts',(0.00335568816011192,-0.0349144232867422,
0.0773644723451003));
#103192=CARTESIAN_POINT('Ctrl Pts',(0.00331183172083244,-0.0348045283677513,
0.0772984433418113));
#103193=CARTESIAN_POINT('Ctrl Pts',(0.0032693523241576,-0.0346945769586886,
0.0772315241014469));
#103194=CARTESIAN_POINT('Ctrl Pts',(0.00337835581652413,-0.035024121149334,
0.0775405898672251));
#103195=CARTESIAN_POINT('Ctrl Pts',(0.00333165183340497,-0.0349144232867422,
0.0774752235675356));
#103196=CARTESIAN_POINT('Ctrl Pts',(0.00328627106376384,-0.0348045283677513,
0.0774088527383064));
#103197=CARTESIAN_POINT('Ctrl Pts',(0.00324227479811095,-0.0346945769586886,
0.077341560229088));
#103198=CARTESIAN_POINT('Ctrl Pts',(0.0033558493127962,-0.035024121149334,
0.0776516511075072));
#103199=CARTESIAN_POINT('Ctrl Pts',(0.00330761550669801,-0.0349144232867422,
0.0775859747899709));
#103200=CARTESIAN_POINT('Ctrl Pts',(0.00326071040669524,-0.0348045283677513,
0.0775192621348016));
#103201=CARTESIAN_POINT('Ctrl Pts',(0.00321519727206429,-0.0346945769586886,
0.0774515963567292));
#103202=CARTESIAN_POINT('Ctrl Pts',(0.00333334280906827,-0.035024121149334,
0.0777627123477894));
#103203=CARTESIAN_POINT('Ctrl Pts',(0.00328357917999106,-0.0349144232867422,
0.0776967260124062));
#103204=CARTESIAN_POINT('Ctrl Pts',(0.00323514974962664,-0.0348045283677513,
0.0776296715312967));
#103205=CARTESIAN_POINT('Ctrl Pts',(0.00318811974601763,-0.0346945769586886,
0.0775616324843703));
#103206=CARTESIAN_POINT('Origin',(0.0175392078150369,-0.0345629067942413,
0.0683865157154276));
#103207=CARTESIAN_POINT('Ctrl Pts',(0.00308893493111351,-0.0351970973651609,
0.0772846187687842));
#103208=CARTESIAN_POINT('Ctrl Pts',(0.00304550903623238,-0.0350869349321765,
0.0772148677833951));
#103209=CARTESIAN_POINT('Ctrl Pts',(0.00300349725217769,-0.0349764985129713,
0.0771441562168122));
#103210=CARTESIAN_POINT('Ctrl Pts',(0.00296295939908606,-0.034865930684963,
0.0770725724740255));
#103211=CARTESIAN_POINT('Ctrl Pts',(0.00316985488368547,-0.0351970973651609,
0.0772991938134279));
#103212=CARTESIAN_POINT('Ctrl Pts',(0.00312622707131348,-0.0350869349321765,
0.0772305638643158));
#103213=CARTESIAN_POINT('Ctrl Pts',(0.00308398989677888,-0.0349764985129713,
0.0771609700649104));
#103214=CARTESIAN_POINT('Ctrl Pts',(0.00304320338697462,-0.034865930684963,
0.077090499354913));
#103215=CARTESIAN_POINT('Ctrl Pts',(0.00325077483625743,-0.0351970973651609,
0.0773137688580717));
#103216=CARTESIAN_POINT('Ctrl Pts',(0.00320694510639458,-0.0350869349321765,
0.0772462599452364));
#103217=CARTESIAN_POINT('Ctrl Pts',(0.00316448254138008,-0.0349764985129713,
0.0771777839130087));
#103218=CARTESIAN_POINT('Ctrl Pts',(0.00312344737486319,-0.034865930684963,
0.0771084262358005));
#103219=CARTESIAN_POINT('Ctrl Pts',(0.00333169478882939,-0.0351970973651609,
0.0773283439027154));
#103220=CARTESIAN_POINT('Ctrl Pts',(0.00328766314147569,-0.0350869349321765,
0.0772619560261571));
#103221=CARTESIAN_POINT('Ctrl Pts',(0.00324497518598127,-0.0349764985129713,
0.0771945977611069));
#103222=CARTESIAN_POINT('Ctrl Pts',(0.00320369136275175,-0.034865930684963,
0.077126353116688));
#103223=CARTESIAN_POINT('Origin',(0.0177504063812929,-0.0345637187967915,
0.0688186274160212));
#103224=CARTESIAN_POINT('Ctrl Pts',(0.0033495061650528,-0.0352450361861253,
0.0773569320865797));
#103225=CARTESIAN_POINT('Ctrl Pts',(0.00322855473979882,-0.0349452761023765,
0.077176867316089));
#103226=CARTESIAN_POINT('Ctrl Pts',(0.00312151013972454,-0.0346444289983474,
0.0769882035346211));
#103227=CARTESIAN_POINT('Ctrl Pts',(0.00349338254862458,-0.0352450361861253,
0.0775613815577218));
#103228=CARTESIAN_POINT('Ctrl Pts',(0.00336472018523426,-0.0349452761023765,
0.0773867431739409));
#103229=CARTESIAN_POINT('Ctrl Pts',(0.00324957781534661,-0.0346444289983474,
0.0772029095439938));
#103230=CARTESIAN_POINT('Ctrl Pts',(0.0032042590746301,-0.0345231616327822,
0.0771265034939999));
#103231=CARTESIAN_POINT('Ctrl Pts',(0.0031632321645473,-0.0344132092796975,
0.0770586947939467));
#103232=CARTESIAN_POINT('Ctrl Pts',(0.00312360994073829,-0.0343032738558974,
0.0769900409832371));
#103233=CARTESIAN_POINT('Ctrl Pts',(0.00308544091088991,-0.0341934961088741,
0.0769206313155901));
#103234=CARTESIAN_POINT('Ctrl Pts',(0.00317482341338464,-0.0345231616327822,
0.0772359323658098));
#103235=CARTESIAN_POINT('Ctrl Pts',(0.00313228818036747,-0.0344132092796975,
0.0771677179366084));
#103236=CARTESIAN_POINT('Ctrl Pts',(0.00309116610363403,-0.0343032738558974,
0.0770986272192143));
#103237=CARTESIAN_POINT('Ctrl Pts',(0.00305150759801842,-0.0341934961088741,
0.0770287500762939));
#103238=CARTESIAN_POINT('Ctrl Pts',(0.00314538775213918,-0.0345231616327822,
0.0773453612376198));
#103239=CARTESIAN_POINT('Ctrl Pts',(0.00310134419618765,-0.0344132092796975,
0.0772767410792702));
#103240=CARTESIAN_POINT('Ctrl Pts',(0.00305872226652977,-0.0343032738558974,
0.0772072134551915));
#103241=CARTESIAN_POINT('Ctrl Pts',(0.00301757428514694,-0.034193496108874,
0.0771368688369976));
#103242=CARTESIAN_POINT('Ctrl Pts',(0.00311595209089371,-0.0345231616327822,
0.0774547901094297));
#103243=CARTESIAN_POINT('Ctrl Pts',(0.00307040021200782,-0.0344132092796975,
0.0773857642219319));
#103244=CARTESIAN_POINT('Ctrl Pts',(0.0030262784294255,-0.0343032738558974,
0.0773157996911687));
#103245=CARTESIAN_POINT('Ctrl Pts',(0.00298364097227546,-0.034193496108874,
0.0772449875977014));
#103246=CARTESIAN_POINT('Origin',(0.0175493979460578,-0.0345625596230862,
0.0683799842894739));
#103247=CARTESIAN_POINT('Ctrl Pts',(0.00281131354479945,-0.0346945769586885,
0.0769388486622199));
#103248=CARTESIAN_POINT('Ctrl Pts',(0.00277288180063825,-0.0345846629176689,
0.0768656401591118));
#103249=CARTESIAN_POINT('Ctrl Pts',(0.00273595741401905,-0.0344746925051586,
0.0767916243991256));
#103250=CARTESIAN_POINT('Ctrl Pts',(0.00270058730505555,-0.034364806625517,
0.0767168964151731));
#103251=CARTESIAN_POINT('Ctrl Pts',(0.00292134958580179,-0.0346945769586885,
0.0769659261669466));
#103252=CARTESIAN_POINT('Ctrl Pts',(0.00288254469993941,-0.0345846629176689,
0.0768942340161001));
#103253=CARTESIAN_POINT('Ctrl Pts',(0.00284521575034348,-0.0344746925051586,
0.0768217271509552));
#103254=CARTESIAN_POINT('Ctrl Pts',(0.00280941018348495,-0.034364806625517,
0.0767484986731943));
#103255=CARTESIAN_POINT('Ctrl Pts',(0.00303138562680414,-0.0346945769586885,
0.0769930036716733));
#103256=CARTESIAN_POINT('Ctrl Pts',(0.00299220759924057,-0.0345846629176689,
0.0769228278730884));
#103257=CARTESIAN_POINT('Ctrl Pts',(0.0029544740866679,-0.0344746925051586,
0.0768518299027847));
#103258=CARTESIAN_POINT('Ctrl Pts',(0.00291823306191435,-0.034364806625517,
0.0767801009312154));
#103259=CARTESIAN_POINT('Ctrl Pts',(0.00314142166780648,-0.0346945769586885,
0.0770200811764));
#103260=CARTESIAN_POINT('Ctrl Pts',(0.00310187049854172,-0.0345846629176689,
0.0769514217300768));
#103261=CARTESIAN_POINT('Ctrl Pts',(0.00306373242299233,-0.0344746925051586,
0.0768819326546142));
#103262=CARTESIAN_POINT('Ctrl Pts',(0.00302705594034375,-0.034364806625517,
0.0768117031892366));
#103263=CARTESIAN_POINT('Origin',(0.0178011398758306,-0.0345626446730454,
0.0687896404668735));
#103264=CARTESIAN_POINT('Ctrl Pts',(0.00313945275405448,-0.0346945769586885,
0.0770195966690427));
#103265=CARTESIAN_POINT('Ctrl Pts',(0.00307934790289853,-0.034527515336289,
0.0769151978933269));
#103266=CARTESIAN_POINT('Ctrl Pts',(0.00302251075095321,-0.0343603235965158,
0.0768088818724941));
#103267=CARTESIAN_POINT('Ctrl Pts',(0.00296910472395195,-0.034193496108874,
0.0767009655405301));
#103268=CARTESIAN_POINT('Ctrl Pts',(0.00318284991868958,-0.0346945769586885,
0.07709132333377));
#103269=CARTESIAN_POINT('Ctrl Pts',(0.00312124272382316,-0.034527515336289,
0.0769878335290427));
#103270=CARTESIAN_POINT('Ctrl Pts',(0.00306287425328339,-0.0343603235965158,
0.076882379466978));
#103271=CARTESIAN_POINT('Ctrl Pts',(0.00300791249965346,-0.034193496108874,
0.0767752755995824));
#103272=CARTESIAN_POINT('Ctrl Pts',(0.00322624708332469,-0.0346945769586885,
0.0771630499984973));
#103273=CARTESIAN_POINT('Ctrl Pts',(0.00316313754474779,-0.034527515336289,
0.0770604691647585));
#103274=CARTESIAN_POINT('Ctrl Pts',(0.00310323775561356,-0.0343603235965158,
0.0769558770614619));
#103275=CARTESIAN_POINT('Ctrl Pts',(0.00304672027535497,-0.034193496108874,
0.0768495856586347));
#103276=CARTESIAN_POINT('Ctrl Pts',(0.0032696442479598,-0.0346945769586885,
0.0772347766632246));
#103277=CARTESIAN_POINT('Ctrl Pts',(0.00320503236567241,-0.034527515336289,
0.0771331048004743));
#103278=CARTESIAN_POINT('Ctrl Pts',(0.00314360125794374,-0.0343603235965158,
0.0770293746559459));
#103279=CARTESIAN_POINT('Ctrl Pts',(0.00308552805105648,-0.034193496108874,
0.0769238957176871));
#103280=CARTESIAN_POINT('Ctrl Pts',(0.00302707104082222,-0.0340223579322365,
0.0768117309011883));
#103281=CARTESIAN_POINT('Ctrl Pts',(0.00299035882960958,-0.0339125849573554,
0.0767414339616182));
#103282=CARTESIAN_POINT('Ctrl Pts',(0.00295512739894426,-0.0338030433565221,
0.076670426561429));
#103283=CARTESIAN_POINT('Ctrl Pts',(0.00292141375427354,-0.0336938721132328,
0.0765988035010579));
#103284=CARTESIAN_POINT('Ctrl Pts',(0.00299082232396728,-0.0340223579322365,
0.0769190957481205));
#103285=CARTESIAN_POINT('Ctrl Pts',(0.00295262927149617,-0.0339125849573554,
0.0768482988442044));
#103286=CARTESIAN_POINT('Ctrl Pts',(0.00291592838824261,-0.0338030433565221,
0.0767767611810152));
#103287=CARTESIAN_POINT('Ctrl Pts',(0.0028807584987238,-0.0336938721132328,
0.0767045784036889));
#103288=CARTESIAN_POINT('Ctrl Pts',(0.00295457360711233,-0.0340223579322365,
0.0770264605950527));
#103289=CARTESIAN_POINT('Ctrl Pts',(0.00291489971338277,-0.0339125849573554,
0.0769551637267906));
#103290=CARTESIAN_POINT('Ctrl Pts',(0.00287672937754096,-0.0338030433565221,
0.0768830958006015));
#103291=CARTESIAN_POINT('Ctrl Pts',(0.00284010324317407,-0.0336938721132328,
0.0768103533063199));
#103292=CARTESIAN_POINT('Ctrl Pts',(0.00291832489025738,-0.0340223579322365,
0.077133825441985));
#103293=CARTESIAN_POINT('Ctrl Pts',(0.00287717015526936,-0.0339125849573554,
0.0770620286093768));
#103294=CARTESIAN_POINT('Ctrl Pts',(0.00283753036683931,-0.0338030433565221,
0.0769894304201877));
#103295=CARTESIAN_POINT('Ctrl Pts',(0.00279944798762434,-0.0336938721132328,
0.0769161282089509));
#103296=CARTESIAN_POINT('Origin',(0.0174455344802189,-0.0345589643414732,
0.0684405256685634));
#103297=CARTESIAN_POINT('Ctrl Pts',(0.00264668323176961,-0.034193496108874,
0.0765997728400264));
#103298=CARTESIAN_POINT('Ctrl Pts',(0.00261290231500352,-0.0340836138581107,
0.0765242468887588));
#103299=CARTESIAN_POINT('Ctrl Pts',(0.00258070045804288,-0.03397388966435,
0.0764480581510719));
#103300=CARTESIAN_POINT('Ctrl Pts',(0.00255011233856891,-0.0338644633294062,
0.0763713069019447));
#103301=CARTESIAN_POINT('Ctrl Pts',(0.00275480208975648,-0.034193496108874,
0.0766337061834304));
#103302=CARTESIAN_POINT('Ctrl Pts',(0.00272055325227938,-0.0340836138581107,
0.0765596711271889));
#103303=CARTESIAN_POINT('Ctrl Pts',(0.00268785284818063,-0.03397388966435,
0.0764849628865316));
#103304=CARTESIAN_POINT('Ctrl Pts',(0.00265673632024154,-0.0338644633294062,
0.0764096798843573));
#103305=CARTESIAN_POINT('Ctrl Pts',(0.00286292094774335,-0.034193496108874,
0.0766676395268344));
#103306=CARTESIAN_POINT('Ctrl Pts',(0.00282820418955523,-0.0340836138581107,
0.0765950953656192));
#103307=CARTESIAN_POINT('Ctrl Pts',(0.00279500523831838,-0.03397388966435,
0.0765218676219912));
#103308=CARTESIAN_POINT('Ctrl Pts',(0.00276336030191417,-0.0338644633294062,
0.0764480528667698));
#103309=CARTESIAN_POINT('Ctrl Pts',(0.00297103980573021,-0.034193496108874,
0.0767015728702384));
#103310=CARTESIAN_POINT('Ctrl Pts',(0.00293585512683108,-0.0340836138581107,
0.0766305196040494));
#103311=CARTESIAN_POINT('Ctrl Pts',(0.00290215762845613,-0.03397388966435,
0.0765587723574509));
#103312=CARTESIAN_POINT('Ctrl Pts',(0.00286998428358681,-0.0338644633294062,
0.0764864258491823));
#103313=CARTESIAN_POINT('Origin',(0.0177347451211335,-0.0345610621863674,
0.0688251127413223));
#103314=CARTESIAN_POINT('Ctrl Pts',(0.00298525284944489,-0.03424362768739,
0.0767333391539459));
#103315=CARTESIAN_POINT('Ctrl Pts',(0.00288782060706489,-0.033943005420186,
0.0765395363248733));
#103316=CARTESIAN_POINT('Ctrl Pts',(0.00280526318263899,-0.0336441434784162,
0.0763389450736088));
#103317=CARTESIAN_POINT('Ctrl Pts',(0.00310237342613376,-0.03424362768739,
0.0769542073737423));
#103318=CARTESIAN_POINT('Ctrl Pts',(0.00299661100151951,-0.033943005420186,
0.0767648218200392));
#103319=CARTESIAN_POINT('Ctrl Pts',(0.00290541433275375,-0.0336441434784162,
0.0765680078316702));
#103320=CARTESIAN_POINT('Ctrl Pts',(0.00286999566758987,-0.0335235895815127,
0.0764864511361787));
#103321=CARTESIAN_POINT('Ctrl Pts',(0.00283782981765183,-0.0334144449262719,
0.0764141224209021));
#103322=CARTESIAN_POINT('Ctrl Pts',(0.00280712126987339,-0.0333049234473133,
0.0763410460864424));
#103323=CARTESIAN_POINT('Ctrl Pts',(0.0027779177554575,-0.0331951640388588,
0.0762673120180385));
#103324=CARTESIAN_POINT('Ctrl Pts',(0.00282707694921841,-0.0335235895815127,
0.0765913279977993));
#103325=CARTESIAN_POINT('Ctrl Pts',(0.00279346726279665,-0.0334144449262719,
0.0765184084218652));
#103326=CARTESIAN_POINT('Ctrl Pts',(0.0027613254264778,-0.0333049234473133,
0.0764447107193454));
#103327=CARTESIAN_POINT('Ctrl Pts',(0.0027307010761736,-0.0331951640388588,
0.0763703254040009));
#103328=CARTESIAN_POINT('Ctrl Pts',(0.00278415823084696,-0.0335235895815127,
0.0766962048594199));
#103329=CARTESIAN_POINT('Ctrl Pts',(0.00274910470794147,-0.0334144449262719,
0.0766226944228283));
#103330=CARTESIAN_POINT('Ctrl Pts',(0.00271552958308222,-0.0333049234473133,
0.0765483753522485));
#103331=CARTESIAN_POINT('Ctrl Pts',(0.00268348439688969,-0.0331951640388588,
0.0764733387899634));
#103332=CARTESIAN_POINT('Ctrl Pts',(0.00274123951247551,-0.0335235895815127,
0.0768010817210406));
#103333=CARTESIAN_POINT('Ctrl Pts',(0.00270474215308629,-0.0334144449262719,
0.0767269804237914));
#103334=CARTESIAN_POINT('Ctrl Pts',(0.00266973373968662,-0.0333049234473133,
0.0766520399851516));
#103335=CARTESIAN_POINT('Ctrl Pts',(0.00263626771760579,-0.0331951640388588,
0.0765763521759258));
#103336=CARTESIAN_POINT('Origin',(0.0185379407817257,-0.032643457177078,
0.0708439813735357));
#103337=CARTESIAN_POINT('Ctrl Pts',(0.00250177593814554,-0.0336938721132429,
0.0762503014554384));
#103338=CARTESIAN_POINT('Ctrl Pts',(0.00248948217677242,-0.0336474569764978,
0.0762173939872473));
#103339=CARTESIAN_POINT('Ctrl Pts',(0.00247757448123973,-0.033601104548885,
0.0761843448598979));
#103340=CARTESIAN_POINT('Ctrl Pts',(0.00244742693520127,-0.0334837508643188,
0.0761006720715267));
#103341=CARTESIAN_POINT('Ctrl Pts',(0.0024197720258371,-0.033366026476046,
0.0760161426918175));
#103342=CARTESIAN_POINT('Ctrl Pts',(0.00281909985087487,-0.0336938721132429,
0.0763722669164609));
#103343=CARTESIAN_POINT('Ctrl Pts',(0.00280609218518593,-0.0336474569764978,
0.0763412168504303));
#103344=CARTESIAN_POINT('Ctrl Pts',(0.00279344889101716,-0.033601104548885,
0.0763100166408197));
#103345=CARTESIAN_POINT('Ctrl Pts',(0.00276143897843713,-0.0334837508643188,
0.0762310248868684));
#103346=CARTESIAN_POINT('Ctrl Pts',(0.00273178381159619,-0.033366026476046,
0.0761511193002344));
#103347=CARTESIAN_POINT('Ctrl Pts',(0.00281909985088202,-0.0336938721132427,
0.0763722669164641));
#103348=CARTESIAN_POINT('Ctrl Pts',(0.00280609218519454,-0.0336474569765026,
0.0763412168504368));
#103349=CARTESIAN_POINT('Ctrl Pts',(0.00279344889102716,-0.0336011045488949,
0.0763100166408297));
#103350=CARTESIAN_POINT('Ctrl Pts',(0.00276170557741933,-0.0334847282606778,
0.0762316827805968));
#103351=CARTESIAN_POINT('Ctrl Pts',(0.00273227784254589,-0.0333679869945435,
0.076152449958875));
#103352=CARTESIAN_POINT('Ctrl Pts',(0.00281909985087479,-0.0336938721132426,
0.0763722669164607));
#103353=CARTESIAN_POINT('Ctrl Pts',(0.00277257868190858,-0.0335278710435083,
0.0762612181393193));
#103354=CARTESIAN_POINT('Ctrl Pts',(0.00272955633976043,-0.033362046922432,
0.076148749537116));
#103355=CARTESIAN_POINT('Ctrl Pts',(0.00269003013551838,-0.0331951640388602,
0.076034798020117));
#103356=CARTESIAN_POINT('Ctrl Pts',(0.00285316508469761,-0.0336938721132426,
0.076448867110115));
#103357=CARTESIAN_POINT('Ctrl Pts',(0.00280504035923445,-0.0335278710435083,
0.0763385314581551));
#103358=CARTESIAN_POINT('Ctrl Pts',(0.00276039266129652,-0.033362046922432,
0.076226725443143));
#103359=CARTESIAN_POINT('Ctrl Pts',(0.00271921838342804,-0.0331951640388602,
0.0761133860345164));
#103360=CARTESIAN_POINT('Ctrl Pts',(0.00288723031852043,-0.0336938721132426,
0.0765254673037692));
#103361=CARTESIAN_POINT('Ctrl Pts',(0.00283750203656033,-0.0335278710435083,
0.076415844776991));
#103362=CARTESIAN_POINT('Ctrl Pts',(0.00279122898283262,-0.033362046922432,
0.07630470134917));
#103363=CARTESIAN_POINT('Ctrl Pts',(0.00274840663133769,-0.0331951640388602,
0.0761919740489158));
#103364=CARTESIAN_POINT('Ctrl Pts',(0.00292129555234325,-0.0336938721132426,
0.0766020674974234));
#103365=CARTESIAN_POINT('Ctrl Pts',(0.0028699637138862,-0.0335278710435083,
0.0764931580958269));
#103366=CARTESIAN_POINT('Ctrl Pts',(0.00282206530436872,-0.033362046922432,
0.076382677255197));
#103367=CARTESIAN_POINT('Ctrl Pts',(0.00277759487924734,-0.0331951640388602,
0.0762705620633152));
#103368=CARTESIAN_POINT('Ctrl Pts',(0.00273365594444268,-0.0330240426238155,
0.0761519539963238));
#103369=CARTESIAN_POINT('Ctrl Pts',(0.0027060770777342,-0.0329142774063509,
0.0760776997559033));
#103370=CARTESIAN_POINT('Ctrl Pts',(0.00268001950452334,-0.0328043479726686,
0.0760028383648232));
#103371=CARTESIAN_POINT('Ctrl Pts',(0.00265551924765414,-0.0326943950436594,
0.0759274648067751));
#103372=CARTESIAN_POINT('Ctrl Pts',(0.00268423673031011,-0.0330240426238155,
0.0762539288817572));
#103373=CARTESIAN_POINT('Ctrl Pts',(0.00265525306020547,-0.0329142774063509,
0.0761789938435152));
#103374=CARTESIAN_POINT('Ctrl Pts',(0.00262780405724542,-0.0328043479726686,
0.0761034222740008));
#103375=CARTESIAN_POINT('Ctrl Pts',(0.00260192755185462,-0.0326943950436594,
0.0760273100176065));
#103376=CARTESIAN_POINT('Ctrl Pts',(0.00263481751617755,-0.0330240426238155,
0.0763559037671906));
#103377=CARTESIAN_POINT('Ctrl Pts',(0.00260442904267675,-0.0329142774063509,
0.0762802879311271));
#103378=CARTESIAN_POINT('Ctrl Pts',(0.0025755886099675,-0.0328043479726686,
0.0762040061831784));
#103379=CARTESIAN_POINT('Ctrl Pts',(0.00254833585605509,-0.0326943950436594,
0.0761271552284379));
#103380=CARTESIAN_POINT('Ctrl Pts',(0.00258539830204498,-0.0330240426238155,
0.076457878652624));
#103381=CARTESIAN_POINT('Ctrl Pts',(0.00255360502514803,-0.0329142774063509,
0.076381582018739));
#103382=CARTESIAN_POINT('Ctrl Pts',(0.00252337316268958,-0.0328043479726686,
0.0763045900923559));
#103383=CARTESIAN_POINT('Ctrl Pts',(0.00249474416025557,-0.0326943950436594,
0.0762270004392693));
#103384=CARTESIAN_POINT('Origin',(0.0186549526395914,-0.0326396682857451,
0.0708039361001382));
#103385=CARTESIAN_POINT('Ctrl Pts',(0.00238283384147148,-0.0331951640388587,
0.0758939931260949));
#103386=CARTESIAN_POINT('Ctrl Pts',(0.00235881386422889,-0.0330855618255041,
0.0758149231763951));
#103387=CARTESIAN_POINT('Ctrl Pts',(0.00233641081202227,-0.0329757224427708,
0.0757352997744029));
#103388=CARTESIAN_POINT('Ctrl Pts',(0.0023156583747808,-0.0328657862078596,
0.0756552234754363));
#103389=CARTESIAN_POINT('Ctrl Pts',(0.00248584714540612,-0.0331951640388587,
0.075941209767781));
#103390=CARTESIAN_POINT('Ctrl Pts',(0.00246117685444279,-0.0330855618255041,
0.0758635586179486));
#103391=CARTESIAN_POINT('Ctrl Pts',(0.00243809369554534,-0.0329757224427708,
0.0757853415977439));
#103392=CARTESIAN_POINT('Ctrl Pts',(0.00241663214121971,-0.0328657862078596,
0.0757066574188082));
#103393=CARTESIAN_POINT('Ctrl Pts',(0.00258886044934076,-0.0331951640388587,
0.075988426409467));
#103394=CARTESIAN_POINT('Ctrl Pts',(0.0025635398446567,-0.0330855618255041,
0.0759121940595022));
#103395=CARTESIAN_POINT('Ctrl Pts',(0.00253977657906841,-0.0329757224427708,
0.075835383421085));
#103396=CARTESIAN_POINT('Ctrl Pts',(0.00251760590765862,-0.0328657862078596,
0.0757580913621801));
#103397=CARTESIAN_POINT('Ctrl Pts',(0.0026918737532754,-0.0331951640388587,
0.0760356430511531));
#103398=CARTESIAN_POINT('Ctrl Pts',(0.0026659028348706,-0.0330855618255041,
0.0759608295010557));
#103399=CARTESIAN_POINT('Ctrl Pts',(0.00264145946259147,-0.0329757224427708,
0.075885425244426));
#103400=CARTESIAN_POINT('Ctrl Pts',(0.00261857967409753,-0.0328657862078596,
0.075809525305552));
#103401=CARTESIAN_POINT('Origin',(0.0187633690656965,-0.0326401908828985,
0.0712724643819485));
#103402=CARTESIAN_POINT('Ctrl Pts',(0.00270196925966051,-0.0332451089994433,
0.0760688719380663));
#103403=CARTESIAN_POINT('Ctrl Pts',(0.00262959782045771,-0.0329451141710259,
0.0758643849176987));
#103404=CARTESIAN_POINT('Ctrl Pts',(0.00257283477919912,-0.0326442513127504,
0.0756550275107169));
#103405=CARTESIAN_POINT('Ctrl Pts',(0.00279048123139834,-0.0332451089994433,
0.076302678761874));
#103406=CARTESIAN_POINT('Ctrl Pts',(0.00270929162356284,-0.0329451141710259,
0.0761015300251378));
#103407=CARTESIAN_POINT('Ctrl Pts',(0.00264348401198786,-0.0326442513127504,
0.0758948371975654));
#103408=CARTESIAN_POINT('Ctrl Pts',(0.00261858870498485,-0.0325229783203385,
0.0758095555747362));
#103409=CARTESIAN_POINT('Ctrl Pts',(0.0025957117680956,-0.032413025311208,
0.0757336666042744));
#103410=CARTESIAN_POINT('Ctrl Pts',(0.0025744081617537,-0.0323031222247695,
0.0756573159050432));
#103411=CARTESIAN_POINT('Ctrl Pts',(0.00255470172332999,-0.0321934096636184,
0.0755806022397748));
#103412=CARTESIAN_POINT('Ctrl Pts',(0.00256286395368766,-0.0325229783203385,
0.075908226212427));
#103413=CARTESIAN_POINT('Ctrl Pts',(0.00253862684424039,-0.032413025311208,
0.0758315690775011));
#103414=CARTESIAN_POINT('Ctrl Pts',(0.0025159791621057,-0.0323031222247695,
0.075754422193397));
#103415=CARTESIAN_POINT('Ctrl Pts',(0.00249494643033256,-0.0321934096636184,
0.0756768854034548));
#103416=CARTESIAN_POINT('Ctrl Pts',(0.00250713920239047,-0.0325229783203385,
0.0760068968501178));
#103417=CARTESIAN_POINT('Ctrl Pts',(0.00248154192038518,-0.032413025311208,
0.0759294715507279));
#103418=CARTESIAN_POINT('Ctrl Pts',(0.0024575501624577,-0.0323031222247695,
0.0758515284817508));
#103419=CARTESIAN_POINT('Ctrl Pts',(0.00243519113733513,-0.0321934096636184,
0.0757731685671348));
#103420=CARTESIAN_POINT('Ctrl Pts',(0.00245141445109328,-0.0325229783203385,
0.0761055674878086));
#103421=CARTESIAN_POINT('Ctrl Pts',(0.00242445699652996,-0.032413025311208,
0.0760273740239547));
#103422=CARTESIAN_POINT('Ctrl Pts',(0.00239912116280971,-0.0323031222247695,
0.0759486347701046));
#103423=CARTESIAN_POINT('Ctrl Pts',(0.00237543584433769,-0.0321934096636184,
0.0758694517308149));
#103424=CARTESIAN_POINT('Origin',(0.0186467580066177,-0.0326393375179189,
0.070806289611769));
#103425=CARTESIAN_POINT('Ctrl Pts',(0.0022846560572056,-0.0326943950436593,
0.0755300746244477));
#103426=CARTESIAN_POINT('Ctrl Pts',(0.00226563604234525,-0.0325844576448127,
0.0754496005226064));
#103427=CARTESIAN_POINT('Ctrl Pts',(0.00224827901777408,-0.0324744968375319,
0.0753687273603969));
#103428=CARTESIAN_POINT('Ctrl Pts',(0.00223260579310099,-0.0323646534831894,
0.0752875590639713));
#103429=CARTESIAN_POINT('Ctrl Pts',(0.00238450123536857,-0.0326943950436593,
0.0755836663027125));
#103430=CARTESIAN_POINT('Ctrl Pts',(0.00236474262674023,-0.0325844576448127,
0.0755045682545562));
#103431=CARTESIAN_POINT('Ctrl Pts',(0.00234661849708335,-0.0324744968375319,
0.0754250559680869));
#103432=CARTESIAN_POINT('Ctrl Pts',(0.00233015066291658,-0.0323646534831894,
0.0753452316393802));
#103433=CARTESIAN_POINT('Ctrl Pts',(0.00248434641353155,-0.0326943950436593,
0.0756372579809774));
#103434=CARTESIAN_POINT('Ctrl Pts',(0.00246384921113521,-0.0325844576448127,
0.0755595359865059));
#103435=CARTESIAN_POINT('Ctrl Pts',(0.00244495797639263,-0.0324744968375319,
0.075481384575777));
#103436=CARTESIAN_POINT('Ctrl Pts',(0.00242769553273217,-0.0323646534831894,
0.0754029042147891));
#103437=CARTESIAN_POINT('Ctrl Pts',(0.00258419159169452,-0.0326943950436593,
0.0756908496592422));
#103438=CARTESIAN_POINT('Ctrl Pts',(0.00256295579553019,-0.0325844576448127,
0.0756145037184556));
#103439=CARTESIAN_POINT('Ctrl Pts',(0.00254329745570191,-0.0324744968375319,
0.075537713183467));
#103440=CARTESIAN_POINT('Ctrl Pts',(0.00252524040254776,-0.0323646534831894,
0.075460576790198));
#103441=CARTESIAN_POINT('Origin',(0.0187997757146061,-0.0326395579065083,
0.0712621436390492));
#103442=CARTESIAN_POINT('Ctrl Pts',(0.0025921917420538,-0.0327445246961877,
0.075724684756325));
#103443=CARTESIAN_POINT('Ctrl Pts',(0.00253280153618932,-0.0324436878365475,
0.0755160574140417));
#103444=CARTESIAN_POINT('Ctrl Pts',(0.0024892947155517,-0.0321434074463187,
0.0753035492470014));
#103445=CARTESIAN_POINT('Ctrl Pts',(0.0026658498329768,-0.0327445246961877,
0.0759635874261334));
#103446=CARTESIAN_POINT('Ctrl Pts',(0.0025974492657149,-0.0324436878365475,
0.0757577381441354));
#103447=CARTESIAN_POINT('Ctrl Pts',(0.00254474842631184,-0.0321434074463187,
0.0755473214479656));
#103448=CARTESIAN_POINT('Ctrl Pts',(0.00250304393363748,-0.0322357242816073,
0.0753687807097753));
#103449=CARTESIAN_POINT('Ctrl Pts',(0.0024642273487318,-0.0319819883628706,
0.0751897674860417));
#103450=CARTESIAN_POINT('Ctrl Pts',(0.00243688055398963,-0.0317295851069886,
0.0750086470444769));
#103451=CARTESIAN_POINT('Ctrl Pts',(0.00256131946590874,-0.0322357242816073,
0.0756118937747029));
#103452=CARTESIAN_POINT('Ctrl Pts',(0.00251476004519121,-0.0319819883628706,
0.0754347365510916));
#103453=CARTESIAN_POINT('Ctrl Pts',(0.00247956800385742,-0.0317295851069886,
0.0752549756494414));
#103454=CARTESIAN_POINT('Origin',(0.0187073500398116,-0.0326371942646192,
0.0712853793484881));
#103455=CARTESIAN_POINT('Origin',(0.0185289370504553,-0.0326352985523298,
0.0708406702041081));
#103456=CARTESIAN_POINT('Ctrl Pts',(0.00220952263615451,-0.0321934096636184,
0.0751607095987536));
#103457=CARTESIAN_POINT('Ctrl Pts',(0.00219558416308856,-0.0320835708272304,
0.0750791473501697));
#103458=CARTESIAN_POINT('Ctrl Pts',(0.00218334170139865,-0.0319739230346346,
0.074997343955029));
#103459=CARTESIAN_POINT('Ctrl Pts',(0.0021728028819668,-0.0318646057455576,
0.0749154052772209));
#103460=CARTESIAN_POINT('Ctrl Pts',(0.0023058058827452,-0.0321934096636184,
0.0752204649432071));
#103461=CARTESIAN_POINT('Ctrl Pts',(0.00229104333690875,-0.0320835708272304,
0.0751402305156323));
#103462=CARTESIAN_POINT('Ctrl Pts',(0.00227794980125727,-0.0319739230346346,
0.0750597371171674));
#103463=CARTESIAN_POINT('Ctrl Pts',(0.00226653412419501,-0.0318646057455576,
0.0749790890192212));
#103464=CARTESIAN_POINT('Ctrl Pts',(0.00240208912933588,-0.0321934096636184,
0.0752802202876605));
#103465=CARTESIAN_POINT('Ctrl Pts',(0.00238650251072894,-0.0320835708272304,
0.0752013136810948));
#103466=CARTESIAN_POINT('Ctrl Pts',(0.0023725579011159,-0.0319739230346346,
0.0751221302793057));
#103467=CARTESIAN_POINT('Ctrl Pts',(0.00236026536642323,-0.0318646057455576,
0.0750427727612214));
#103468=CARTESIAN_POINT('Ctrl Pts',(0.00249837237592657,-0.0321934096636184,
0.075339975632114));
#103469=CARTESIAN_POINT('Ctrl Pts',(0.00248196168454913,-0.0320835708272304,
0.0752623968465574));
#103470=CARTESIAN_POINT('Ctrl Pts',(0.00246716600097452,-0.0319739230346346,
0.0751845234414441));
#103471=CARTESIAN_POINT('Ctrl Pts',(0.00245399660865145,-0.0318646057455576,
0.0751064565032216));
#103472=CARTESIAN_POINT('Ctrl Pts',(0.00252454183115225,-0.03202188345824,
0.0754612227764161));
#103473=CARTESIAN_POINT('Ctrl Pts',(0.00251089517191015,-0.0319391099350675,
0.0754029482203234));
#103474=CARTESIAN_POINT('Ctrl Pts',(0.00249816674619664,-0.0318564869454936,
0.0753444958768062));
#103475=CARTESIAN_POINT('Ctrl Pts',(0.00248636185033058,-0.0317740741446509,
0.0752859091861526));
#103476=CARTESIAN_POINT('Ctrl Pts',(0.00249750299692719,-0.03202188345824,
0.0755027646768473));
#103477=CARTESIAN_POINT('Ctrl Pts',(0.0024834239869285,-0.0319391099350675,
0.0754442087118564));
#103478=CARTESIAN_POINT('Ctrl Pts',(0.00247026786664812,-0.0318564869454936,
0.0753854683787216));
#103479=CARTESIAN_POINT('Ctrl Pts',(0.00245804022434095,-0.0317740741446509,
0.075326587356576));
#103480=CARTESIAN_POINT('Ctrl Pts',(0.00247046416270213,-0.03202188345824,
0.0755443065772786));
#103481=CARTESIAN_POINT('Ctrl Pts',(0.00245595280194684,-0.0319391099350675,
0.0754854692033893));
#103482=CARTESIAN_POINT('Ctrl Pts',(0.00244236898709961,-0.0318564869454936,
0.075426440880637));
#103483=CARTESIAN_POINT('Ctrl Pts',(0.00242971859835133,-0.0317740741446509,
0.0753672655269994));
#103484=CARTESIAN_POINT('Ctrl Pts',(0.00244342532847707,-0.03202188345824,
0.0755858484777098));
#103485=CARTESIAN_POINT('Ctrl Pts',(0.00242848161696518,-0.0319391099350675,
0.0755267296949222));
#103486=CARTESIAN_POINT('Ctrl Pts',(0.0024144701075511,-0.0318564869454936,
0.0754674133825524));
#103487=CARTESIAN_POINT('Ctrl Pts',(0.00240139697236171,-0.0317740741446509,
0.0754079436974228));
#103488=CARTESIAN_POINT('Origin',(-0.00338560652537836,-0.0391228853390713,
0.0778125932965984));
#103489=CARTESIAN_POINT('Ctrl Pts',(0.0039710489218594,-0.0352722978779663,
0.078129820463345));
#103490=CARTESIAN_POINT('Ctrl Pts',(0.00395822888878371,-0.0352466642097263,
0.0781159374006412));
#103491=CARTESIAN_POINT('Ctrl Pts',(0.00394536267769211,-0.0352210183808324,
0.0781021198949546));
#103492=CARTESIAN_POINT('Ctrl Pts',(0.00393244944482438,-0.0351953608940153,
0.0780883678215747));
#103493=CARTESIAN_POINT('Origin',(0.000250727888052832,-0.0352456003065144,
0.0813187002982664));
#103494=CARTESIAN_POINT('Ctrl Pts',(0.00384913788149874,-0.035024121149334,
0.077995607383702));
#103495=CARTESIAN_POINT('Ctrl Pts',(0.00379616621893717,-0.0349144232867421,
0.0779367259136369));
#103496=CARTESIAN_POINT('Ctrl Pts',(0.00374437997228945,-0.0348045283677512,
0.0778767142381083));
#103497=CARTESIAN_POINT('Ctrl Pts',(0.00369384833356284,-0.0346945769586886,
0.0778156467560871));
#103498=CARTESIAN_POINT('Ctrl Pts',(0.00384072851264329,-0.035024121149334,
0.0781086136858207));
#103499=CARTESIAN_POINT('Ctrl Pts',(0.00378620023467461,-0.0349144232867421,
0.0780496163801528));
#103500=CARTESIAN_POINT('Ctrl Pts',(0.00373285883531504,-0.0348045283677512,
0.0779894566233369));
#103501=CARTESIAN_POINT('Ctrl Pts',(0.00368077550558287,-0.0346945769586886,
0.077928208929892));
#103502=CARTESIAN_POINT('Ctrl Pts',(0.00383231914378784,-0.035024121149334,
0.0782216199879394));
#103503=CARTESIAN_POINT('Ctrl Pts',(0.00377623425041205,-0.0349144232867421,
0.0781625068466687));
#103504=CARTESIAN_POINT('Ctrl Pts',(0.00372133769834064,-0.0348045283677512,
0.0781021990085655));
#103505=CARTESIAN_POINT('Ctrl Pts',(0.0036677026776029,-0.0346945769586886,
0.0780407711036969));
#103506=CARTESIAN_POINT('Ctrl Pts',(0.00382390977493239,-0.035024121149334,
0.078334626290058));
#103507=CARTESIAN_POINT('Ctrl Pts',(0.00376626826614949,-0.0349144232867421,
0.0782753973131846));
#103508=CARTESIAN_POINT('Ctrl Pts',(0.00370981656136623,-0.0348045283677512,
0.0782149413937941));
#103509=CARTESIAN_POINT('Ctrl Pts',(0.00365462984962294,-0.0346945769586886,
0.0781533332775019));
#103510=CARTESIAN_POINT('Origin',(0.0167426082500215,-0.0345629067941904,
0.0672518967717792));
#103511=CARTESIAN_POINT('Ctrl Pts',(0.00352150811189216,-0.0351970973651605,
0.0778909350513752));
#103512=CARTESIAN_POINT('Ctrl Pts',(0.00346968252661987,-0.0350869349321763,
0.0778271767811655));
#103513=CARTESIAN_POINT('Ctrl Pts',(0.00341913950874065,-0.0349764985129714,
0.077762288269149));
#103514=CARTESIAN_POINT('Ctrl Pts',(0.00336994948677475,-0.0348659306849635,
0.0776963497257651));
#103515=CARTESIAN_POINT('Ctrl Pts',(0.00360361672394291,-0.0351970973651605,
0.0778952532081228));
#103516=CARTESIAN_POINT('Ctrl Pts',(0.00355173131646102,-0.0350869349321763,
0.0778326324414562));
#103517=CARTESIAN_POINT('Ctrl Pts',(0.00350110477874789,-0.0349764985129714,
0.077768881131607));
#103518=CARTESIAN_POINT('Ctrl Pts',(0.00345180756080035,-0.0348659306849635,
0.0777040780093661));
#103519=CARTESIAN_POINT('Ctrl Pts',(0.00368572533599366,-0.0351970973651605,
0.0778995713648704));
#103520=CARTESIAN_POINT('Ctrl Pts',(0.00363378010630217,-0.0350869349321763,
0.0778380881017469));
#103521=CARTESIAN_POINT('Ctrl Pts',(0.00358307004875512,-0.0349764985129715,
0.0777754739940649));
#103522=CARTESIAN_POINT('Ctrl Pts',(0.00353366563482594,-0.0348659306849635,
0.0777118062929671));
#103523=CARTESIAN_POINT('Ctrl Pts',(0.00376783394804441,-0.0351970973651605,
0.077903889521618));
#103524=CARTESIAN_POINT('Ctrl Pts',(0.00371582889614332,-0.0350869349321763,
0.0778435437620376));
#103525=CARTESIAN_POINT('Ctrl Pts',(0.00366503531876236,-0.0349764985129715,
0.0777820668565228));
#103526=CARTESIAN_POINT('Ctrl Pts',(0.00361552370885153,-0.0348659306849635,
0.0777195345765681));
#103527=CARTESIAN_POINT('Origin',(0.0170062994093576,-0.0345637187965744,
0.0676541309434874));
#103528=CARTESIAN_POINT('Ctrl Pts',(0.00378908792577322,-0.0352450361861252,
0.0779300199217376));
#103529=CARTESIAN_POINT('Ctrl Pts',(0.00364652213869726,-0.0349452761023764,
0.0777665342489764));
#103530=CARTESIAN_POINT('Ctrl Pts',(0.00351667577547945,-0.0346444289983475,
0.0775927743836394));
#103531=CARTESIAN_POINT('Ctrl Pts',(0.00395745411440549,-0.0352450361861252,
0.0781148247553471));
#103532=CARTESIAN_POINT('Ctrl Pts',(0.00380791829883643,-0.0349452761023764,
0.077957689117426));
#103533=CARTESIAN_POINT('Ctrl Pts',(0.00367064339764764,-0.0346444289983475,
0.0777897362360978));
#103534=CARTESIAN_POINT('Ctrl Pts',(0.00361610579142808,-0.0345231616327822,
0.0777196126149445));
#103535=CARTESIAN_POINT('Ctrl Pts',(0.00356690370714396,-0.0344132092796975,
0.0776574806420485));
#103536=CARTESIAN_POINT('Ctrl Pts',(0.00351898931231153,-0.0343032738558974,
0.0775943341685733));
#103537=CARTESIAN_POINT('Ctrl Pts',(0.00347242191857722,-0.0341934961088741,
0.0775302556648203));
#103538=CARTESIAN_POINT('Ctrl Pts',(0.00360061731351277,-0.0345231616327822,
0.0778318678740214));
#103539=CARTESIAN_POINT('Ctrl Pts',(0.00354986794852505,-0.0344132092796975,
0.0777695224142633));
#103540=CARTESIAN_POINT('Ctrl Pts',(0.00350041076862894,-0.0343032738558974,
0.0777061304606602));
#103541=CARTESIAN_POINT('Ctrl Pts',(0.00345230705390109,-0.0341934961088741,
0.0776417748486301));
#103542=CARTESIAN_POINT('Ctrl Pts',(0.00358512883559746,-0.0345231616327822,
0.0779441231330983));
#103543=CARTESIAN_POINT('Ctrl Pts',(0.00353283218990613,-0.0344132092796975,
0.0778815641864782));
#103544=CARTESIAN_POINT('Ctrl Pts',(0.00348183222494634,-0.0343032738558974,
0.0778179267527471));
#103545=CARTESIAN_POINT('Ctrl Pts',(0.00343219218922495,-0.0341934961088741,
0.07775329403244));
#103546=CARTESIAN_POINT('Ctrl Pts',(0.00356964035768215,-0.0345231616327822,
0.0780563783921752));
#103547=CARTESIAN_POINT('Ctrl Pts',(0.00351579643128722,-0.0344132092796975,
0.077993605958693));
#103548=CARTESIAN_POINT('Ctrl Pts',(0.00346325368126374,-0.0343032738558974,
0.077929723044834));
#103549=CARTESIAN_POINT('Ctrl Pts',(0.00341207732454881,-0.0341934961088741,
0.0778648132162498));
#103550=CARTESIAN_POINT('Origin',(0.0167518994234811,-0.0345625596231696,
0.0672441396862457));
#103551=CARTESIAN_POINT('Ctrl Pts',(0.00320273936760623,-0.0346945769586885,
0.0775826866314311));
#103552=CARTESIAN_POINT('Ctrl Pts',(0.0031554352107804,-0.0345846629176052,
0.0775148721739643));
#103553=CARTESIAN_POINT('Ctrl Pts',(0.00310952534941888,-0.0344746925050311,
0.0774460679030849));
#103554=CARTESIAN_POINT('Ctrl Pts',(0.00306506824443851,-0.0343648066253259,
0.0773763622216925));
#103555=CARTESIAN_POINT('Ctrl Pts',(0.00331530145278338,-0.0346945769586885,
0.077595759449118));
#103556=CARTESIAN_POINT('Ctrl Pts',(0.00326781714592219,-0.0345846629176052,
0.0775294961540791));
#103557=CARTESIAN_POINT('Ctrl Pts',(0.00322169502635326,-0.0344746925050311,
0.0774622395851415));
#103558=CARTESIAN_POINT('Ctrl Pts',(0.00317699383515299,-0.0343648066253259,
0.0773940761632334));
#103559=CARTESIAN_POINT('Ctrl Pts',(0.00342786353796052,-0.0346945769586885,
0.0776088322668048));
#103560=CARTESIAN_POINT('Ctrl Pts',(0.00338019908106397,-0.0345846629176052,
0.077544120134194));
#103561=CARTESIAN_POINT('Ctrl Pts',(0.00333386470328764,-0.0344746925050311,
0.077478411267198));
#103562=CARTESIAN_POINT('Ctrl Pts',(0.00328891942586748,-0.0343648066253259,
0.0774117901047743));
#103563=CARTESIAN_POINT('Ctrl Pts',(0.00354042562313766,-0.0346945769586885,
0.0776219050844916));
#103564=CARTESIAN_POINT('Ctrl Pts',(0.00349258101620576,-0.0345846629176052,
0.0775587441143089));
#103565=CARTESIAN_POINT('Ctrl Pts',(0.00344603438022202,-0.0344746925050311,
0.0774945829492545));
#103566=CARTESIAN_POINT('Ctrl Pts',(0.00340084501658196,-0.0343648066253259,
0.0774295040463152));
#103567=CARTESIAN_POINT('Origin',(0.0170529998266576,-0.0345626446730515,
0.0676190139721156));
#103568=CARTESIAN_POINT('Ctrl Pts',(0.00353841150998499,-0.0346945769586886,
0.0776216711679469));
#103569=CARTESIAN_POINT('Ctrl Pts',(0.00346569596739218,-0.034527515336289,
0.0775256287431082));
#103570=CARTESIAN_POINT('Ctrl Pts',(0.00339598206269568,-0.0343603235965158,
0.0774272746398945));
#103571=CARTESIAN_POINT('Ctrl Pts',(0.00332947165532945,-0.0341934961088738,
0.0773269028104969));
#103572=CARTESIAN_POINT('Ctrl Pts',(0.00359045620983789,-0.0346945769586886,
0.0776873931395278));
#103573=CARTESIAN_POINT('Ctrl Pts',(0.0035163640942367,-0.034527515336289,
0.077592440811765));
#103574=CARTESIAN_POINT('Ctrl Pts',(0.00344523897792986,-0.0343603235965158,
0.0774951337956282));
#103575=CARTESIAN_POINT('Ctrl Pts',(0.00337728694011562,-0.0341934961088738,
0.0773957630085222));
#103576=CARTESIAN_POINT('Ctrl Pts',(0.0036425009096908,-0.0346945769586886,
0.0777531151111088));
#103577=CARTESIAN_POINT('Ctrl Pts',(0.00356703222108122,-0.034527515336289,
0.0776592528804219));
#103578=CARTESIAN_POINT('Ctrl Pts',(0.00349449589316403,-0.0343603235965158,
0.0775629929513619));
#103579=CARTESIAN_POINT('Ctrl Pts',(0.00342510222490178,-0.0341934961088738,
0.0774646232065475));
#103580=CARTESIAN_POINT('Ctrl Pts',(0.0036945456095437,-0.0346945769586886,
0.0778188370826897));
#103581=CARTESIAN_POINT('Ctrl Pts',(0.00361770034792574,-0.034527515336289,
0.0777260649490788));
#103582=CARTESIAN_POINT('Ctrl Pts',(0.00354375280839821,-0.0343603235965158,
0.0776308521070957));
#103583=CARTESIAN_POINT('Ctrl Pts',(0.00347291750968795,-0.0341934961088738,
0.0775334834045728));
#103584=CARTESIAN_POINT('Ctrl Pts',(0.00340086347129577,-0.0340223579322365,
0.0774295296472712));
#103585=CARTESIAN_POINT('Ctrl Pts',(0.00335563020408784,-0.0339125849573552,
0.0773643882802087));
#103586=CARTESIAN_POINT('Ctrl Pts',(0.00331177699670363,-0.0338030433565216,
0.0772983564637071));
#103587=CARTESIAN_POINT('Ctrl Pts',(0.00326935244443675,-0.033693872113232,
0.0772315236126616));
#103588=CARTESIAN_POINT('Ctrl Pts',(0.00337835696983735,-0.0340223579322365,
0.0775405910592131));
#103589=CARTESIAN_POINT('Ctrl Pts',(0.00333159187609843,-0.0339125849573552,
0.0774751392687961));
#103590=CARTESIAN_POINT('Ctrl Pts',(0.00328621434362211,-0.0338030433565216,
0.0774087655418211));
#103591=CARTESIAN_POINT('Ctrl Pts',(0.00324227487829685,-0.033693872113232,
0.0773415599032314));
#103592=CARTESIAN_POINT('Ctrl Pts',(0.00335585046837892,-0.0340223579322365,
0.0776516524711549));
#103593=CARTESIAN_POINT('Ctrl Pts',(0.00330755354810902,-0.0339125849573552,
0.0775858902573834));
#103594=CARTESIAN_POINT('Ctrl Pts',(0.00326065169054059,-0.0338030433565216,
0.077519174619935));
#103595=CARTESIAN_POINT('Ctrl Pts',(0.00321519731215695,-0.033693872113232,
0.0774515961938011));
#103596=CARTESIAN_POINT('Ctrl Pts',(0.0033333439669205,-0.0340223579322365,
0.0777627138830968));
#103597=CARTESIAN_POINT('Ctrl Pts',(0.00328351522011961,-0.0339125849573552,
0.0776966412459707));
#103598=CARTESIAN_POINT('Ctrl Pts',(0.00323508903745907,-0.0338030433565216,
0.077629583698049));
#103599=CARTESIAN_POINT('Ctrl Pts',(0.00318811974601705,-0.033693872113232,
0.0775616324843709));
#103600=CARTESIAN_POINT('Origin',(0.0166564427992684,-0.0345589643414914,
0.0673172212223324));
#103601=CARTESIAN_POINT('Ctrl Pts',(0.00299690974454832,-0.0341934961088739,
0.0772669181728474));
#103602=CARTESIAN_POINT('Ctrl Pts',(0.0029539292887104,-0.0340836138581106,
0.0771962216377951));
#103603=CARTESIAN_POINT('Ctrl Pts',(0.00291243237215464,-0.0339738896643499,
0.077124669633921));
#103604=CARTESIAN_POINT('Ctrl Pts',(0.00287246596690574,-0.0338644633294062,
0.07705235729924));
#103605=CARTESIAN_POINT('Ctrl Pts',(0.00310842902870093,-0.0341934961088739,
0.0772870330556225));
#103606=CARTESIAN_POINT('Ctrl Pts',(0.0030651712005411,-0.0340836138581106,
0.0772178743054596));
#103607=CARTESIAN_POINT('Ctrl Pts',(0.00302336522352032,-0.0339738896643499,
0.0771478536089786));
#103608=CARTESIAN_POINT('Ctrl Pts',(0.00298305859660315,-0.0338644633294062,
0.0770770641708263));
#103609=CARTESIAN_POINT('Ctrl Pts',(0.00321994831285354,-0.0341934961088739,
0.0773071479383976));
#103610=CARTESIAN_POINT('Ctrl Pts',(0.00317641311237181,-0.0340836138581106,
0.077239526973124));
#103611=CARTESIAN_POINT('Ctrl Pts',(0.003134298074886,-0.0339738896643499,
0.0771710375840361));
#103612=CARTESIAN_POINT('Ctrl Pts',(0.00309365122630057,-0.0338644633294062,
0.0771017710424124));
#103613=CARTESIAN_POINT('Ctrl Pts',(0.00333146759700616,-0.0341934961088739,
0.0773272628211727));
#103614=CARTESIAN_POINT('Ctrl Pts',(0.00328765502420252,-0.0340836138581106,
0.0772611796407885));
#103615=CARTESIAN_POINT('Ctrl Pts',(0.00324523092625167,-0.0339738896643499,
0.0771942215590936));
#103616=CARTESIAN_POINT('Ctrl Pts',(0.00320424385599798,-0.0338644633294062,
0.0771264779139987));
#103617=CARTESIAN_POINT('Origin',(0.0169915744700192,-0.0345610621860186,
0.0676625280065053));
#103618=CARTESIAN_POINT('Ctrl Pts',(0.00334954993768123,-0.0342436276873899,
0.0773569972515174));
#103619=CARTESIAN_POINT('Ctrl Pts',(0.00322859604239246,-0.0339430054201859,
0.0771769341136292));
#103620=CARTESIAN_POINT('Ctrl Pts',(0.00312154885777119,-0.0336441434784162,
0.0769882717732526));
#103621=CARTESIAN_POINT('Ctrl Pts',(0.00349342911181937,-0.0342436276873899,
0.0775614447588372));
#103622=CARTESIAN_POINT('Ctrl Pts',(0.00336476435167696,-0.0339430054201859,
0.0773868081134584));
#103623=CARTESIAN_POINT('Ctrl Pts',(0.00324961946231059,-0.0336441434784162,
0.0772029760355599));
#103624=CARTESIAN_POINT('Ctrl Pts',(0.00320425831953572,-0.0335235895815127,
0.0771265015748059));
#103625=CARTESIAN_POINT('Ctrl Pts',(0.00316328091516676,-0.0334144449262719,
0.0770587746430359));
#103626=CARTESIAN_POINT('Ctrl Pts',(0.00312365562016488,-0.0333049234473133,
0.0769901233388914));
#103627=CARTESIAN_POINT('Ctrl Pts',(0.00308544105496591,-0.0331951640388588,
0.0769206308565334));
#103628=CARTESIAN_POINT('Ctrl Pts',(0.00317482258427507,-0.0335235895815127,
0.0772359305927856));
#103629=CARTESIAN_POINT('Ctrl Pts',(0.00313233867402772,-0.0334144449262719,
0.0771677984201661));
#103630=CARTESIAN_POINT('Ctrl Pts',(0.0030912135143257,-0.0333049234473133,
0.0770987102863218));
#103631=CARTESIAN_POINT('Ctrl Pts',(0.00305150769406908,-0.0331951640388588,
0.0770287497702561));
#103632=CARTESIAN_POINT('Ctrl Pts',(0.00314538684901441,-0.0335235895815127,
0.0773453596107654));
#103633=CARTESIAN_POINT('Ctrl Pts',(0.00310139643288869,-0.0334144449262719,
0.0772768221972964));
#103634=CARTESIAN_POINT('Ctrl Pts',(0.00305877140848652,-0.0333049234473133,
0.0772072972337522));
#103635=CARTESIAN_POINT('Ctrl Pts',(0.00301757433317225,-0.0331951640388588,
0.0771368686839789));
#103636=CARTESIAN_POINT('Ctrl Pts',(0.00311595111375375,-0.0335235895815127,
0.0774547886287451));
#103637=CARTESIAN_POINT('Ctrl Pts',(0.00307045419174965,-0.0334144449262719,
0.0773858459744266));
#103638=CARTESIAN_POINT('Ctrl Pts',(0.00302632930264734,-0.0333049234473133,
0.0773158841811827));
#103639=CARTESIAN_POINT('Ctrl Pts',(0.00298364097227541,-0.0331951640388588,
0.0772449875977016));
#103640=CARTESIAN_POINT('Origin',(0.0180414680259711,-0.0326434571770575,
0.0695648101471628));
#103641=CARTESIAN_POINT('Ctrl Pts',(0.00280934470954787,-0.0336938721132435,
0.0769383641741863));
#103642=CARTESIAN_POINT('Ctrl Pts',(0.00279302348875822,-0.0336474569764981,
0.0769072570080762));
#103643=CARTESIAN_POINT('Ctrl Pts',(0.00277706753496419,-0.033601104548885,
0.0768759609129525));
#103644=CARTESIAN_POINT('Ctrl Pts',(0.00273667073020307,-0.0334837508643192,
0.0767967263989386));
#103645=CARTESIAN_POINT('Ctrl Pts',(0.00269863954756933,-0.0333660264760466,
0.0767163296378509));
#103646=CARTESIAN_POINT('Ctrl Pts',(0.00313945275405843,-0.0336938721132435,
0.0770195966690497));
#103647=CARTESIAN_POINT('Ctrl Pts',(0.00312265605252052,-0.0336474569764981,
0.0769904217348656));
#103648=CARTESIAN_POINT('Ctrl Pts',(0.00310620203134415,-0.033601104548885,
0.0769610521731677));
#103649=CARTESIAN_POINT('Ctrl Pts',(0.00306454423453818,-0.0334837508643192,
0.0768866951986399));
#103650=CARTESIAN_POINT('Ctrl Pts',(0.00302510808199276,-0.0333660264760466,
0.0768111364693754));
#103651=CARTESIAN_POINT('Ctrl Pts',(0.00313945275406449,-0.0336938721132426,
0.0770195966690529));
#103652=CARTESIAN_POINT('Ctrl Pts',(0.00312265605252859,-0.0336474569765026,
0.0769904217348721));
#103653=CARTESIAN_POINT('Ctrl Pts',(0.00310620203135415,-0.0336011045488949,
0.0769610521731777));
#103654=CARTESIAN_POINT('Ctrl Pts',(0.00306489118725482,-0.0334847282606778,
0.0768873144909686));
#103655=CARTESIAN_POINT('Ctrl Pts',(0.00302576499310969,-0.0333679869945434,
0.0768123947168798));
#103656=CARTESIAN_POINT('Ctrl Pts',(0.00313945275405809,-0.0336938721132426,
0.077019596669049));
#103657=CARTESIAN_POINT('Ctrl Pts',(0.00307938031608184,-0.0335278710435082,
0.0769152541932195));
#103658=CARTESIAN_POINT('Ctrl Pts',(0.00302260116436309,-0.033362046922432,
0.0768090645687945));
#103659=CARTESIAN_POINT('Ctrl Pts',(0.00296910472395236,-0.0331951640388601,
0.0767009655405309));
#103660=CARTESIAN_POINT('Ctrl Pts',(0.00318284992329977,-0.0336938721132426,
0.0770913233413898));
#103661=CARTESIAN_POINT('Ctrl Pts',(0.00312127595163347,-0.0335278710435082,
0.0769878893464579));
#103662=CARTESIAN_POINT('Ctrl Pts',(0.00306296730473599,-0.033362046922432,
0.0768825607956229));
#103663=CARTESIAN_POINT('Ctrl Pts',(0.00300791250377322,-0.0331951640388601,
0.0767752756074711));
#103664=CARTESIAN_POINT('Ctrl Pts',(0.00322624709254146,-0.0336938721132426,
0.0771630500137307));
#103665=CARTESIAN_POINT('Ctrl Pts',(0.0031631715871851,-0.0335278710435082,
0.0770605244996964));
#103666=CARTESIAN_POINT('Ctrl Pts',(0.00310333344510889,-0.033362046922432,
0.0769560570224513));
#103667=CARTESIAN_POINT('Ctrl Pts',(0.00304672028359408,-0.0331951640388601,
0.0768495856744113));
#103668=CARTESIAN_POINT('Ctrl Pts',(0.00326964426178314,-0.0336938721132426,
0.0772347766860715));
#103669=CARTESIAN_POINT('Ctrl Pts',(0.00320506722273674,-0.0335278710435082,
0.0771331596529348));
#103670=CARTESIAN_POINT('Ctrl Pts',(0.00314369958548179,-0.033362046922432,
0.0770295532492797));
#103671=CARTESIAN_POINT('Ctrl Pts',(0.00308552806341493,-0.0331951640388601,
0.0769238957413515));
#103672=CARTESIAN_POINT('Ctrl Pts',(0.00302707006767231,-0.0330240426238155,
0.0768117299431733));
#103673=CARTESIAN_POINT('Ctrl Pts',(0.00299040214450746,-0.0329142774063509,
0.0767415177681598));
#103674=CARTESIAN_POINT('Ctrl Pts',(0.0029551674228312,-0.0328043479726686,
0.0766705125614177));
#103675=CARTESIAN_POINT('Ctrl Pts',(0.00292141354604987,-0.0326943950436594,
0.0765988040428044));
#103676=CARTESIAN_POINT('Ctrl Pts',(0.0029908213809377,-0.0330240426238155,
0.0769190945960841));
#103677=CARTESIAN_POINT('Ctrl Pts',(0.0029526744050787,-0.0329142774063509,
0.0768483830600954));
#103678=CARTESIAN_POINT('Ctrl Pts',(0.00291597021653283,-0.0328043479726686,
0.0767768476672778));
#103679=CARTESIAN_POINT('Ctrl Pts',(0.0028807583599082,-0.0326943950436594,
0.0767045787648528));
#103680=CARTESIAN_POINT('Ctrl Pts',(0.00295457269420309,-0.0330240426238155,
0.0770264592489949));
#103681=CARTESIAN_POINT('Ctrl Pts',(0.00291494666564993,-0.0329142774063509,
0.076955248352031));
#103682=CARTESIAN_POINT('Ctrl Pts',(0.00287677301023446,-0.0328043479726686,
0.0768831827731379));
#103683=CARTESIAN_POINT('Ctrl Pts',(0.00284010317376653,-0.0326943950436594,
0.0768103534869012));
#103684=CARTESIAN_POINT('Ctrl Pts',(0.00291832400746847,-0.0330240426238155,
0.0771338239019057));
#103685=CARTESIAN_POINT('Ctrl Pts',(0.00287721892622117,-0.0329142774063509,
0.0770621136439667));
#103686=CARTESIAN_POINT('Ctrl Pts',(0.00283757580393609,-0.0328043479726686,
0.076989517878998));
#103687=CARTESIAN_POINT('Ctrl Pts',(0.00279944798762485,-0.0326943950436594,
0.0769161282089497));
#103688=CARTESIAN_POINT('Origin',(0.0181525382067224,-0.0326396682858048,
0.069510415168098));
#103689=CARTESIAN_POINT('Ctrl Pts',(0.00264668323176962,-0.0331951640388587,
0.0765997728400265));
#103690=CARTESIAN_POINT('Ctrl Pts',(0.00261294256674836,-0.0330855618255041,
0.076524336881915));
#103691=CARTESIAN_POINT('Ctrl Pts',(0.00258073671086079,-0.0329757224427708,
0.0764481491812047));
#103692=CARTESIAN_POINT('Ctrl Pts',(0.00255011169130408,-0.0328657862078596,
0.0763713052778369));
#103693=CARTESIAN_POINT('Ctrl Pts',(0.00275480205941473,-0.0331951640388587,
0.0766337061739077));
#103694=CARTESIAN_POINT('Ctrl Pts',(0.00272059403136584,-0.0330855618255041,
0.0765597593339244));
#103695=CARTESIAN_POINT('Ctrl Pts',(0.00268788969800888,-0.0329757224427708,
0.0764850521652318));
#103696=CARTESIAN_POINT('Ctrl Pts',(0.002656735631873,-0.0328657862078596,
0.0764096782805498));
#103697=CARTESIAN_POINT('Ctrl Pts',(0.00286292088705985,-0.0331951640388587,
0.0766676395077888));
#103698=CARTESIAN_POINT('Ctrl Pts',(0.00282824549598332,-0.0330855618255041,
0.0765951817859338));
#103699=CARTESIAN_POINT('Ctrl Pts',(0.00279504268515697,-0.0329757224427708,
0.076521955149259));
#103700=CARTESIAN_POINT('Ctrl Pts',(0.00276335957244192,-0.0328657862078596,
0.0764480512832627));
#103701=CARTESIAN_POINT('Ctrl Pts',(0.00297103971470497,-0.0331951640388587,
0.07670157284167));
#103702=CARTESIAN_POINT('Ctrl Pts',(0.0029358969606008,-0.0330855618255041,
0.0766306042379432));
#103703=CARTESIAN_POINT('Ctrl Pts',(0.00290219567230506,-0.0329757224427708,
0.0765588581332861));
#103704=CARTESIAN_POINT('Ctrl Pts',(0.00286998351301083,-0.0328657862078596,
0.0764864242859755));
#103705=CARTESIAN_POINT('Origin',(0.0183188219012972,-0.0326401908832583,
0.0699616607828441));
#103706=CARTESIAN_POINT('Ctrl Pts',(0.00298522029885135,-0.0332451089994432,
0.076733274406425));
#103707=CARTESIAN_POINT('Ctrl Pts',(0.00288779051057838,-0.0329451141710257,
0.0765394703737833));
#103708=CARTESIAN_POINT('Ctrl Pts',(0.00280523562206676,-0.0326442513127503,
0.0763388781079957));
#103709=CARTESIAN_POINT('Ctrl Pts',(0.00310233809251201,-0.0332451089994432,
0.0769541441019654));
#103710=CARTESIAN_POINT('Ctrl Pts',(0.00299657806738194,-0.0329451141710257,
0.0767647572391802));
#103711=CARTESIAN_POINT('Ctrl Pts',(0.00290538388804582,-0.0326442513127503,
0.0765679421270413));
#103712=CARTESIAN_POINT('Ctrl Pts',(0.00286999626642163,-0.0325229783203385,
0.0764864531846078));
#103713=CARTESIAN_POINT('Ctrl Pts',(0.00283778831095292,-0.032413025311208,
0.0764140298618194));
#103714=CARTESIAN_POINT('Ctrl Pts',(0.00280708340989057,-0.0323031222247695,
0.076340951260526));
#103715=CARTESIAN_POINT('Ctrl Pts',(0.00277791759089321,-0.0321934096636184,
0.0762673123770711));
#103716=CARTESIAN_POINT('Ctrl Pts',(0.00282707763151222,-0.0325229783203385,
0.0765913299381186));
#103717=CARTESIAN_POINT('Ctrl Pts',(0.00279342395231619,-0.032413025311208,
0.0765183149828973));
#103718=CARTESIAN_POINT('Ctrl Pts',(0.0027612857854755,-0.0323031222247695,
0.0764446149322517));
#103719=CARTESIAN_POINT('Ctrl Pts',(0.00273070096647091,-0.0321934096636184,
0.0763703256433411));
#103720=CARTESIAN_POINT('Ctrl Pts',(0.00278415899660282,-0.0325229783203385,
0.0766962066916294));
#103721=CARTESIAN_POINT('Ctrl Pts',(0.00274905959367946,-0.032413025311208,
0.0766226001039753));
#103722=CARTESIAN_POINT('Ctrl Pts',(0.00271548816106042,-0.0323031222247695,
0.0765482786039775));
#103723=CARTESIAN_POINT('Ctrl Pts',(0.00268348434204861,-0.0321934096636184,
0.0764733389096111));
#103724=CARTESIAN_POINT('Ctrl Pts',(0.00274124036169342,-0.0325229783203385,
0.0768010834451402));
#103725=CARTESIAN_POINT('Ctrl Pts',(0.00270469523504273,-0.032413025311208,
0.0767268852250532));
#103726=CARTESIAN_POINT('Ctrl Pts',(0.00266969053664535,-0.0323031222247695,
0.0766519422757033));
#103727=CARTESIAN_POINT('Ctrl Pts',(0.00263626771762631,-0.0321934096636184,
0.0765763521758811));
#103728=CARTESIAN_POINT('Origin',(0.0181447031648636,-0.0326393375174202,
0.069513777181946));
#103729=CARTESIAN_POINT('Ctrl Pts',(0.00250366852609156,-0.0326943950436593,
0.0762510288836282));
#103730=CARTESIAN_POINT('Ctrl Pts',(0.00247471241032746,-0.0325844576448126,
0.0761735731840813));
#103731=CARTESIAN_POINT('Ctrl Pts',(0.00244735615615104,-0.0324744968375319,
0.0760955131429261));
#103732=CARTESIAN_POINT('Ctrl Pts',(0.00242163343448193,-0.0323646534831895,
0.0760169492586902));
#103733=CARTESIAN_POINT('Ctrl Pts',(0.00260944321353152,-0.0326943950436593,
0.0762916840564678));
#103734=CARTESIAN_POINT('Ctrl Pts',(0.00257992679328977,-0.0325844576448126,
0.0762156861303568));
#103735=CARTESIAN_POINT('Ctrl Pts',(0.00255198004583739,-0.0324744968375319,
0.076139072377791));
#103736=CARTESIAN_POINT('Ctrl Pts',(0.00252563742422781,-0.0323646534831895,
0.0760619414546645));
#103737=CARTESIAN_POINT('Ctrl Pts',(0.00271521790097148,-0.0326943950436593,
0.0763323392293075));
#103738=CARTESIAN_POINT('Ctrl Pts',(0.00268514117625209,-0.0325844576448126,
0.0762577990766323));
#103739=CARTESIAN_POINT('Ctrl Pts',(0.00265660393552373,-0.0324744968375319,
0.076182631612656));
#103740=CARTESIAN_POINT('Ctrl Pts',(0.00262964141397369,-0.0323646534831895,
0.0761069336506387));
#103741=CARTESIAN_POINT('Ctrl Pts',(0.00282099258841144,-0.0326943950436593,
0.0763729944021472));
#103742=CARTESIAN_POINT('Ctrl Pts',(0.0027903555592144,-0.0325844576448126,
0.0762999120229078));
#103743=CARTESIAN_POINT('Ctrl Pts',(0.00276122782521008,-0.0324744968375319,
0.0762261908475209));
#103744=CARTESIAN_POINT('Ctrl Pts',(0.00273364540371956,-0.0323646534831895,
0.0761519258466129));
#103745=CARTESIAN_POINT('Origin',(0.0183536479408555,-0.0326395579067962,
0.0699468584591393));
#103746=CARTESIAN_POINT('Ctrl Pts',(0.0028331703173209,-0.0327445246961875,
0.0764055600146698));
#103747=CARTESIAN_POINT('Ctrl Pts',(0.00274810048155036,-0.0324436878365473,
0.0762060213278374));
#103748=CARTESIAN_POINT('Ctrl Pts',(0.00267830238945435,-0.0321434074463185,
0.07600064170168));
#103749=CARTESIAN_POINT('Ctrl Pts',(0.0029361900363106,-0.0327445246961875,
0.0766333470588565));
#103750=CARTESIAN_POINT('Ctrl Pts',(0.00284252907181213,-0.0324436878365473,
0.0764376938242037));
#103751=CARTESIAN_POINT('Ctrl Pts',(0.00276387158934186,-0.0321434074463185,
0.0762355414931456));
#103752=CARTESIAN_POINT('Ctrl Pts',(0.00270011886100842,-0.0322357242816071,
0.0760636355609245));
#103753=CARTESIAN_POINT('Ctrl Pts',(0.00263917205028739,-0.0319819883628705,
0.0758908989180309));
#103754=CARTESIAN_POINT('Ctrl Pts',(0.00258934048258397,-0.0317295851069886,
0.0757146341274587));
#103755=CARTESIAN_POINT('Ctrl Pts',(0.00278840501985078,-0.0322357242816071,
0.0762975277458236));
#103756=CARTESIAN_POINT('Ctrl Pts',(0.00272000904638777,-0.0319819883628705,
0.0761276029025862));
#103757=CARTESIAN_POINT('Ctrl Pts',(0.00266256448973903,-0.0317295851069886,
0.0759536702016737));
#103758=CARTESIAN_POINT('Origin',(0.0182648632769585,-0.0326371942646736,
0.0699814949570038));
#103759=CARTESIAN_POINT('Origin',(0.0180321202916383,-0.0326352985529878,
0.0695626535532545));
#103760=CARTESIAN_POINT('Ctrl Pts',(0.00238283384147098,-0.0321934096636183,
0.0758939931260947));
#103761=CARTESIAN_POINT('Ctrl Pts',(0.00235878281707659,-0.0320835708272304,
0.0758148209741027));
#103762=CARTESIAN_POINT('Ctrl Pts',(0.00233638420682424,-0.0319739230346346,
0.0757351970104766));
#103763=CARTESIAN_POINT('Ctrl Pts',(0.00231565884968773,-0.0318646057455575,
0.0756552253079342));
#103764=CARTESIAN_POINT('Ctrl Pts',(0.002485847196447,-0.0321934096636183,
0.0759412097911758));
#103765=CARTESIAN_POINT('Ctrl Pts',(0.00246114501744271,-0.0320835708272304,
0.0758634582736327));
#103766=CARTESIAN_POINT('Ctrl Pts',(0.00243806623032052,-0.0319739230346346,
0.0757852406448189));
#103767=CARTESIAN_POINT('Ctrl Pts',(0.00241663268238519,-0.0318646057455575,
0.0757066592449329));
#103768=CARTESIAN_POINT('Ctrl Pts',(0.00258886055142302,-0.0321934096636183,
0.075988426456257));
#103769=CARTESIAN_POINT('Ctrl Pts',(0.00256350721780883,-0.0320835708272304,
0.0759120955731626));
#103770=CARTESIAN_POINT('Ctrl Pts',(0.0025397482538168,-0.0319739230346346,
0.0758352842791612));
#103771=CARTESIAN_POINT('Ctrl Pts',(0.00251760651508264,-0.0318646057455575,
0.0757580931819316));
#103772=CARTESIAN_POINT('Ctrl Pts',(0.00269187390639904,-0.0321934096636183,
0.0760356431213381));
#103773=CARTESIAN_POINT('Ctrl Pts',(0.00266586941817495,-0.0320835708272304,
0.0759607328726926));
#103774=CARTESIAN_POINT('Ctrl Pts',(0.00264143027731307,-0.0319739230346346,
0.0758853279135035));
#103775=CARTESIAN_POINT('Ctrl Pts',(0.00261858034778009,-0.0318646057455575,
0.0758095271189303));
#103776=CARTESIAN_POINT('Ctrl Pts',(0.00273303330430885,-0.0320218834582397,
0.07615265429325));
#103777=CARTESIAN_POINT('Ctrl Pts',(0.00271219051450128,-0.0319391099350671,
0.0760965496293679));
#103778=CARTESIAN_POINT('Ctrl Pts',(0.00269223643500384,-0.0318564869454931,
0.076040153494791));
#103779=CARTESIAN_POINT('Ctrl Pts',(0.00267318176488415,-0.0317740741446503,
0.0759835083234629));
#103780=CARTESIAN_POINT('Ctrl Pts',(0.00271141426007721,-0.0320218834582397,
0.0761972574879136));
#103781=CARTESIAN_POINT('Ctrl Pts',(0.00269010725884071,-0.0319391099350671,
0.0761409278220448));
#103782=CARTESIAN_POINT('Ctrl Pts',(0.00266969276260582,-0.0318564869454931,
0.0760842995730776));
#103783=CARTESIAN_POINT('Ctrl Pts',(0.00265018179000934,-0.0317740741446503,
0.0760274153753276));
#103784=CARTESIAN_POINT('Ctrl Pts',(0.00268979521584557,-0.0320218834582397,
0.0762418606825772));
#103785=CARTESIAN_POINT('Ctrl Pts',(0.00266802400318014,-0.0319391099350671,
0.0761853060147217));
#103786=CARTESIAN_POINT('Ctrl Pts',(0.00264714909020781,-0.0318564869454931,
0.0761284456513641));
#103787=CARTESIAN_POINT('Ctrl Pts',(0.00262718181513453,-0.0317740741446503,
0.0760713224271923));
#103788=CARTESIAN_POINT('Ctrl Pts',(0.00266817617161393,-0.0320218834582397,
0.0762864638772409));
#103789=CARTESIAN_POINT('Ctrl Pts',(0.00264594074751957,-0.0319391099350671,
0.0762296842073986));
#103790=CARTESIAN_POINT('Ctrl Pts',(0.00262460541780979,-0.0318564869454931,
0.0761725917296507));
#103791=CARTESIAN_POINT('Ctrl Pts',(0.00260418184025973,-0.0317740741446503,
0.076115229479057));
#103792=CARTESIAN_POINT('Origin',(-0.00283580689655155,-0.0391228853390708,
0.0792262215589275));
#103793=CARTESIAN_POINT('Ctrl Pts',(0.00450259823174105,-0.0352722978779665,
0.0786189138792926));
#103794=CARTESIAN_POINT('Ctrl Pts',(0.00448813927931483,-0.0352466642097264,
0.0786067470648846));
#103795=CARTESIAN_POINT('Ctrl Pts',(0.00447364272947313,-0.0352210183808325,
0.0785946510781973));
#103796=CARTESIAN_POINT('Ctrl Pts',(0.00445910772947859,-0.0351953608940152,
0.0785826259012546));
#103797=CARTESIAN_POINT('Origin',(0.00121128566165112,-0.0352456003065142,
0.082248928309305));
#103798=CARTESIAN_POINT('Ctrl Pts',(0.00436482713708829,-0.035024121149334,
0.0785010386147655));
#103799=CARTESIAN_POINT('Ctrl Pts',(0.00430489336686762,-0.0349144232867421,
0.0784492605524351));
#103800=CARTESIAN_POINT('Ctrl Pts',(0.0042459940128969,-0.0348045283677512,
0.0783962126246391));
#103801=CARTESIAN_POINT('Ctrl Pts',(0.00418820704624738,-0.0346945769586886,
0.0783419599716325));
#103802=CARTESIAN_POINT('Ctrl Pts',(0.00437064752387573,-0.035024121149334,
0.0786142078018301));
#103803=CARTESIAN_POINT('Ctrl Pts',(0.00430915489457471,-0.0349144232867421,
0.0785625099129376));
#103804=CARTESIAN_POINT('Ctrl Pts',(0.0042486940912292,-0.0348045283677512,
0.0785095099838376));
#103805=CARTESIAN_POINT('Ctrl Pts',(0.0041893450826407,-0.0346945769586886,
0.0784552730188794));
#103806=CARTESIAN_POINT('Ctrl Pts',(0.00437646791066317,-0.035024121149334,
0.0787273769888946));
#103807=CARTESIAN_POINT('Ctrl Pts',(0.00431341642228179,-0.0349144232867421,
0.0786757592734401));
#103808=CARTESIAN_POINT('Ctrl Pts',(0.0042513941695615,-0.0348045283677512,
0.078622807343036));
#103809=CARTESIAN_POINT('Ctrl Pts',(0.00419048311903402,-0.0346945769586886,
0.0785685860661263));
#103810=CARTESIAN_POINT('Ctrl Pts',(0.00438228829745061,-0.035024121149334,
0.0788405461759592));
#103811=CARTESIAN_POINT('Ctrl Pts',(0.00431767794998888,-0.0349144232867421,
0.0787890086339426));
#103812=CARTESIAN_POINT('Ctrl Pts',(0.00425409424789381,-0.0348045283677512,
0.0787361047022345));
#103813=CARTESIAN_POINT('Ctrl Pts',(0.00419162115542735,-0.0346945769586886,
0.0786818991133732));
#103814=CARTESIAN_POINT('Origin',(0.0158100846488341,-0.0345629067942937,
0.0662260650370403));
#103815=CARTESIAN_POINT('Ctrl Pts',(0.00402666190419685,-0.0351970973651602,
0.0784382545534798));
#103816=CARTESIAN_POINT('Ctrl Pts',(0.00396725394897228,-0.0350869349321763,
0.078381494504458));
#103817=CARTESIAN_POINT('Ctrl Pts',(0.00390897679085345,-0.0349764985129717,
0.0783234523776052));
#103818=CARTESIAN_POINT('Ctrl Pts',(0.0038519103560444,-0.034865930684964,
0.078264198923843));
#103819=CARTESIAN_POINT('Ctrl Pts',(0.00410866427386499,-0.0351970973651602,
0.0784322477224199));
#103820=CARTESIAN_POINT('Ctrl Pts',(0.00404933953514405,-0.0350869349321763,
0.078376623705097));
#103821=CARTESIAN_POINT('Ctrl Pts',(0.00399112204499497,-0.0349764985129717,
0.0783197202810434));
#103822=CARTESIAN_POINT('Ctrl Pts',(0.00393409156547994,-0.034865930684964,
0.0782616067305085));
#103823=CARTESIAN_POINT('Ctrl Pts',(0.00419066664353313,-0.0351970973651602,
0.07842624089136));
#103824=CARTESIAN_POINT('Ctrl Pts',(0.00413142512131583,-0.0350869349321763,
0.078371752905736));
#103825=CARTESIAN_POINT('Ctrl Pts',(0.0040732672991365,-0.0349764985129717,
0.0783159881844817));
#103826=CARTESIAN_POINT('Ctrl Pts',(0.00401627277491548,-0.034865930684964,
0.078259014537174));
#103827=CARTESIAN_POINT('Ctrl Pts',(0.00427266901320127,-0.0351970973651602,
0.0784202340603001));
#103828=CARTESIAN_POINT('Ctrl Pts',(0.0042135107074876,-0.0350869349321763,
0.0783668821063749));
#103829=CARTESIAN_POINT('Ctrl Pts',(0.00415541255327803,-0.0349764985129717,
0.07831225608792));
#103830=CARTESIAN_POINT('Ctrl Pts',(0.00409845398435102,-0.034865930684964,
0.0782564223438395));
#103831=CARTESIAN_POINT('Origin',(0.0161221098346002,-0.0345637187964946,
0.0665920782062245));
#103832=CARTESIAN_POINT('Ctrl Pts',(0.00429703040451049,-0.0352450361861253,
0.0784434945846552));
#103833=CARTESIAN_POINT('Ctrl Pts',(0.00413509860323931,-0.0349452761023764,
0.0782991662763443));
#103834=CARTESIAN_POINT('Ctrl Pts',(0.00398449823159228,-0.0346444289983474,
0.0781430506240137));
#103835=CARTESIAN_POINT('Ctrl Pts',(0.00448723116283145,-0.0352450361861253,
0.078605740298109));
#103836=CARTESIAN_POINT('Ctrl Pts',(0.00431918016422343,-0.0349452761023764,
0.0784685855289259));
#103837=CARTESIAN_POINT('Ctrl Pts',(0.00416193763892921,-0.0346444289983474,
0.0783191621134853));
#103838=CARTESIAN_POINT('Ctrl Pts',(0.00409904125783595,-0.0345231616327822,
0.0782564268125681));
#103839=CARTESIAN_POINT('Ctrl Pts',(0.00404243994561156,-0.0344132092796975,
0.0782009514251577));
#103840=CARTESIAN_POINT('Ctrl Pts',(0.0039869890183849,-0.0343032738558974,
0.0781443081465254));
#103841=CARTESIAN_POINT('Ctrl Pts',(0.00393275765638187,-0.034193496108874,
0.0780865713629492));
#103842=CARTESIAN_POINT('Ctrl Pts',(0.00409774422579989,-0.0345231616327822,
0.0783697381264187));
#103843=CARTESIAN_POINT('Ctrl Pts',(0.00403958107664365,-0.0344132092796975,
0.0783142448612478));
#103844=CARTESIAN_POINT('Ctrl Pts',(0.00398256876285612,-0.0343032738558974,
0.0782575514004124));
#103845=CARTESIAN_POINT('Ctrl Pts',(0.00392677846333303,-0.034193496108874,
0.0781997322457186));
#103846=CARTESIAN_POINT('Ctrl Pts',(0.00409644719376382,-0.0345231616327822,
0.0784830494402693));
#103847=CARTESIAN_POINT('Ctrl Pts',(0.00403672220767573,-0.0344132092796975,
0.0784275382973378));
#103848=CARTESIAN_POINT('Ctrl Pts',(0.00397814850732733,-0.0343032738558974,
0.0783707946542993));
#103849=CARTESIAN_POINT('Ctrl Pts',(0.0039207992702842,-0.034193496108874,
0.0783128931284879));
#103850=CARTESIAN_POINT('Ctrl Pts',(0.00409515016172776,-0.0345231616327822,
0.0785963607541199));
#103851=CARTESIAN_POINT('Ctrl Pts',(0.00403386333870782,-0.0344132092796975,
0.0785408317334278));
#103852=CARTESIAN_POINT('Ctrl Pts',(0.00397372825179854,-0.0343032738558974,
0.0784840379081863));
#103853=CARTESIAN_POINT('Ctrl Pts',(0.00391482007723537,-0.034193496108874,
0.0784260540112573));
#103854=CARTESIAN_POINT('Origin',(0.0158183303387263,-0.0345625596230808,
0.0662172046252609));
#103855=CARTESIAN_POINT('Ctrl Pts',(0.00367177297545972,-0.0346945769586886,
0.0781723890818771));
#103856=CARTESIAN_POINT('Ctrl Pts',(0.0036163424208028,-0.0345846629176053,
0.0781110381445986));
#103857=CARTESIAN_POINT('Ctrl Pts',(0.00356217111065839,-0.0344746925050312,
0.0780485304473229));
#103858=CARTESIAN_POINT('Ctrl Pts',(0.00350932812478276,-0.034364806625326,
0.0779849463687704));
#103859=CARTESIAN_POINT('Ctrl Pts',(0.0037850859334871,-0.0346945769586886,
0.0781712510463798));
#103860=CARTESIAN_POINT('Ctrl Pts',(0.00372967106153454,-0.0345846629176053,
0.0781114616189367));
#103861=CARTESIAN_POINT('Ctrl Pts',(0.00367548314539103,-0.0344746925050311,
0.0780505160225181));
#103862=CARTESIAN_POINT('Ctrl Pts',(0.00362259129435643,-0.034364806625326,
0.0779884926343885));
#103863=CARTESIAN_POINT('Ctrl Pts',(0.00389839889151448,-0.0346945769586885,
0.0781701130108826));
#103864=CARTESIAN_POINT('Ctrl Pts',(0.00384299970226629,-0.0345846629176052,
0.0781118850932749));
#103865=CARTESIAN_POINT('Ctrl Pts',(0.00378879518012367,-0.0344746925050311,
0.0780525015977133));
#103866=CARTESIAN_POINT('Ctrl Pts',(0.0037358544639301,-0.034364806625326,
0.0779920389000066));
#103867=CARTESIAN_POINT('Ctrl Pts',(0.00401171184954186,-0.0346945769586885,
0.0781689749753853));
#103868=CARTESIAN_POINT('Ctrl Pts',(0.00395632834299804,-0.0345846629176052,
0.078112308567613));
#103869=CARTESIAN_POINT('Ctrl Pts',(0.00390210721485631,-0.0344746925050311,
0.0780544871729085));
#103870=CARTESIAN_POINT('Ctrl Pts',(0.00384911763350376,-0.034364806625326,
0.0779955851656247));
#103871=CARTESIAN_POINT('Origin',(0.0161640406813811,-0.0345626446730904,
0.0665513850283427));
#103872=CARTESIAN_POINT('Ctrl Pts',(0.00400968430075594,-0.0346945769586885,
0.0781689953386564));
#103873=CARTESIAN_POINT('Ctrl Pts',(0.00392550483427121,-0.034527515336289,
0.0780828239111076));
#103874=CARTESIAN_POINT('Ctrl Pts',(0.00384401360674573,-0.0343603235965158,
0.0779939828284748));
#103875=CARTESIAN_POINT('Ctrl Pts',(0.00376544772787016,-0.034193496108874,
0.0779027384253525));
#103876=CARTESIAN_POINT('Ctrl Pts',(0.00406955575982,-0.0346945769586885,
0.0782276761423388));
#103877=CARTESIAN_POINT('Ctrl Pts',(0.00398414720040764,-0.034527515336289,
0.0781427587464713));
#103878=CARTESIAN_POINT('Ctrl Pts',(0.00390138712390605,-0.0343603235965158,
0.0780551333660354));
#103879=CARTESIAN_POINT('Ctrl Pts',(0.00382151644613647,-0.034193496108874,
0.0779650627958928));
#103880=CARTESIAN_POINT('Ctrl Pts',(0.00412942721888406,-0.0346945769586885,
0.0782863569460212));
#103881=CARTESIAN_POINT('Ctrl Pts',(0.00404278956654408,-0.034527515336289,
0.078202693581835));
#103882=CARTESIAN_POINT('Ctrl Pts',(0.00395876064106636,-0.0343603235965158,
0.0781162839035959));
#103883=CARTESIAN_POINT('Ctrl Pts',(0.00387758516440278,-0.034193496108874,
0.0780273871664331));
#103884=CARTESIAN_POINT('Ctrl Pts',(0.00418929867794812,-0.0346945769586885,
0.0783450377497036));
#103885=CARTESIAN_POINT('Ctrl Pts',(0.00410143193268052,-0.034527515336289,
0.0782626284171987));
#103886=CARTESIAN_POINT('Ctrl Pts',(0.00401613415822667,-0.0343603235965158,
0.0781774344411565));
#103887=CARTESIAN_POINT('Ctrl Pts',(0.0039336538826691,-0.034193496108874,
0.0780897115369734));
#103888=CARTESIAN_POINT('Ctrl Pts',(0.00384913915134722,-0.0340223579322365,
0.0779956082517206));
#103889=CARTESIAN_POINT('Ctrl Pts',(0.00379609818378914,-0.0339125849573554,
0.0779366497754382));
#103890=CARTESIAN_POINT('Ctrl Pts',(0.00374431479096331,-0.0338030433565221,
0.0778766349038162));
#103891=CARTESIAN_POINT('Ctrl Pts',(0.0036938483916329,-0.0336938721132328,
0.0778156462560814));
#103892=CARTESIAN_POINT('Ctrl Pts',(0.00384072980625804,-0.0340223579322365,
0.0781086147238609));
#103893=CARTESIAN_POINT('Ctrl Pts',(0.00378613018471591,-0.0339125849573554,
0.0780495402607772));
#103894=CARTESIAN_POINT('Ctrl Pts',(0.0037327916338114,-0.0338030433565221,
0.0779893772233409));
#103895=CARTESIAN_POINT('Ctrl Pts',(0.00368077554429622,-0.0336938721132328,
0.0779282085965552));
#103896=CARTESIAN_POINT('Ctrl Pts',(0.00383232046116886,-0.0340223579322365,
0.0782216211960012));
#103897=CARTESIAN_POINT('Ctrl Pts',(0.00377616218564268,-0.0339125849573554,
0.0781624307461163));
#103898=CARTESIAN_POINT('Ctrl Pts',(0.0037212684766595,-0.0338030433565221,
0.0781021195428656));
#103899=CARTESIAN_POINT('Ctrl Pts',(0.00366770269695954,-0.0336938721132328,
0.078040770937029));
#103900=CARTESIAN_POINT('Ctrl Pts',(0.00382391111607968,-0.0340223579322365,
0.0783346276681416));
#103901=CARTESIAN_POINT('Ctrl Pts',(0.00376619418656945,-0.0339125849573554,
0.0782753212314553));
#103902=CARTESIAN_POINT('Ctrl Pts',(0.0037097453195076,-0.0338030433565221,
0.0782148618623903));
#103903=CARTESIAN_POINT('Ctrl Pts',(0.00365462984962285,-0.0336938721132328,
0.0781533332775029));
#103904=CARTESIAN_POINT('Origin',(0.0157327859634578,-0.0345589643414735,
0.0663016737791342));
#103905=CARTESIAN_POINT('Ctrl Pts',(0.00342799009848604,-0.034193496108874,
0.0778849078441259));
#103906=CARTESIAN_POINT('Ctrl Pts',(0.00337648793104013,-0.0340836138581107,
0.0778201556518787));
#103907=CARTESIAN_POINT('Ctrl Pts',(0.00332635038605239,-0.0339738896643499,
0.0777543687996616));
#103908=CARTESIAN_POINT('Ctrl Pts',(0.0032776359891141,-0.0338644633294062,
0.077687635788142));
#103909=CARTESIAN_POINT('Ctrl Pts',(0.00354115108307491,-0.034193496108874,
0.0778908870425547));
#103910=CARTESIAN_POINT('Ctrl Pts',(0.00348956646602342,-0.0340836138581107,
0.0778276952732737));
#103911=CARTESIAN_POINT('Ctrl Pts',(0.00343931422131188,-0.0339738896643499,
0.077763466389181));
#103912=CARTESIAN_POINT('Ctrl Pts',(0.00339045315500113,-0.0338644633294062,
0.0776982869067778));
#103913=CARTESIAN_POINT('Ctrl Pts',(0.00365431206766379,-0.034193496108874,
0.0778968662409835));
#103914=CARTESIAN_POINT('Ctrl Pts',(0.0036026450010067,-0.0340836138581107,
0.0778352348946687));
#103915=CARTESIAN_POINT('Ctrl Pts',(0.00355227805657137,-0.0339738896643499,
0.0777725639787003));
#103916=CARTESIAN_POINT('Ctrl Pts',(0.00350327032088815,-0.0338644633294062,
0.0777089380254137));
#103917=CARTESIAN_POINT('Ctrl Pts',(0.00376747305225267,-0.034193496108874,
0.0779028454394122));
#103918=CARTESIAN_POINT('Ctrl Pts',(0.00371572353598999,-0.0340836138581107,
0.0778427745160637));
#103919=CARTESIAN_POINT('Ctrl Pts',(0.00366524189183086,-0.0339738896643499,
0.0777816615682196));
#103920=CARTESIAN_POINT('Ctrl Pts',(0.00361608748677517,-0.0338644633294062,
0.0777195891440495));
#103921=CARTESIAN_POINT('Origin',(0.0161085534363768,-0.0345610621861926,
0.0666022545801441));
#103922=CARTESIAN_POINT('Ctrl Pts',(0.00378913952057393,-0.03424362768739,
0.0779300790866652));
#103923=CARTESIAN_POINT('Ctrl Pts',(0.00364657148755933,-0.0339430054201859,
0.0777665953432102));
#103924=CARTESIAN_POINT('Ctrl Pts',(0.00351672274079097,-0.033644143478416,
0.0775928372315306));
#103925=CARTESIAN_POINT('Ctrl Pts',(0.00395750823163594,-0.03424362768739,
0.0781148816221871));
#103926=CARTESIAN_POINT('Ctrl Pts',(0.0038079702560933,-0.0339430054201859,
0.0779577480093528));
#103927=CARTESIAN_POINT('Ctrl Pts',(0.00367069304981574,-0.033644143478416,
0.0777897969836091));
#103928=CARTESIAN_POINT('Ctrl Pts',(0.00361610480174909,-0.0335235895815128,
0.0777196108055224));
#103929=CARTESIAN_POINT('Ctrl Pts',(0.00356696208109481,-0.0334144449262719,
0.077657553751431));
#103930=CARTESIAN_POINT('Ctrl Pts',(0.00351904495344267,-0.0333049234473133,
0.0775944101496783));
#103931=CARTESIAN_POINT('Ctrl Pts',(0.0034724220039821,-0.0331951640388588,
0.0775302551913258));
#103932=CARTESIAN_POINT('Ctrl Pts',(0.00360061626872215,-0.0335235895815128,
0.0778318662188931));
#103933=CARTESIAN_POINT('Ctrl Pts',(0.00354992813129227,-0.0334144449262719,
0.0777695959346505));
#103934=CARTESIAN_POINT('Ctrl Pts',(0.00350046821654235,-0.0333049234473133,
0.0777062069306234));
#103935=CARTESIAN_POINT('Ctrl Pts',(0.00345230711083766,-0.0331951640388588,
0.0776417745329672));
#103936=CARTESIAN_POINT('Ctrl Pts',(0.00358512773569521,-0.0335235895815128,
0.0779441216322637));
#103937=CARTESIAN_POINT('Ctrl Pts',(0.00353289418148973,-0.0334144449262719,
0.07788163811787));
#103938=CARTESIAN_POINT('Ctrl Pts',(0.00348189147964202,-0.0333049234473133,
0.0778180037115685));
#103939=CARTESIAN_POINT('Ctrl Pts',(0.00343219221769322,-0.0331951640388588,
0.0777532938746086));
#103940=CARTESIAN_POINT('Ctrl Pts',(0.00356963920266827,-0.0335235895815128,
0.0780563770456345));
#103941=CARTESIAN_POINT('Ctrl Pts',(0.00351586023168719,-0.0334144449262719,
0.0779936803010894));
#103942=CARTESIAN_POINT('Ctrl Pts',(0.00346331474274169,-0.0333049234473133,
0.0779298004925136));
#103943=CARTESIAN_POINT('Ctrl Pts',(0.00341207732454878,-0.0331951640388588,
0.07786481321625));
#103944=CARTESIAN_POINT('Origin',(0.0173885874402498,-0.0326434571769693,
0.0683579501038521));
#103945=CARTESIAN_POINT('Ctrl Pts',(0.00320072533475701,-0.0336938721132442,
0.0775824527242192));
#103946=CARTESIAN_POINT('Ctrl Pts',(0.00318063404995246,-0.0336474569764984,
0.0775536364387821));
#103947=CARTESIAN_POINT('Ctrl Pts',(0.00316088147281998,-0.033601104548885,
0.0775245869339996));
#103948=CARTESIAN_POINT('Ctrl Pts',(0.00311087249107923,-0.0334837508643194,
0.0774510402699615));
#103949=CARTESIAN_POINT('Ctrl Pts',(0.00306306480964481,-0.0333660264760472,
0.0773760440324443));
#103950=CARTESIAN_POINT('Ctrl Pts',(0.00353841150999001,-0.0336938721132442,
0.0776216711679534));
#103951=CARTESIAN_POINT('Ctrl Pts',(0.00351809066662021,-0.0336474569764984,
0.0775948314717563));
#103952=CARTESIAN_POINT('Ctrl Pts',(0.0034980854081793,-0.033601104548885,
0.0775677557335037));
#103953=CARTESIAN_POINT('Ctrl Pts',(0.00344743669548824,-0.0334837508643194,
0.0774992061923065));
#103954=CARTESIAN_POINT('Ctrl Pts',(0.00339884148892204,-0.0333660264760472,
0.0774291859267086));
#103955=CARTESIAN_POINT('Ctrl Pts',(0.003538411509995,-0.0336938721132427,
0.0776216711679568));
#103956=CARTESIAN_POINT('Ctrl Pts',(0.00351809066662774,-0.0336474569765026,
0.0775948314717629));
#103957=CARTESIAN_POINT('Ctrl Pts',(0.0034980854081893,-0.0336011045488949,
0.0775677557335137));
#103958=CARTESIAN_POINT('Ctrl Pts',(0.00344785853028782,-0.0334847282606778,
0.0774997771166254));
#103959=CARTESIAN_POINT('Ctrl Pts',(0.0033996509203255,-0.0333679869945434,
0.0774303519197621));
#103960=CARTESIAN_POINT('Ctrl Pts',(0.00353841150998937,-0.0336938721132427,
0.0776216711679526));
#103961=CARTESIAN_POINT('Ctrl Pts',(0.00346573518123552,-0.0335278710435083,
0.0775256805366102));
#103962=CARTESIAN_POINT('Ctrl Pts',(0.003396094661087,-0.033362046922432,
0.0774274445637751));
#103963=CARTESIAN_POINT('Ctrl Pts',(0.00332947165533008,-0.0331951640388601,
0.0773269028104978));
#103964=CARTESIAN_POINT('Ctrl Pts',(0.00359045621536674,-0.0336938721132427,
0.0776873931465096));
#103965=CARTESIAN_POINT('Ctrl Pts',(0.003516404055813,-0.0335278710435083,
0.0775924920244943));
#103966=CARTESIAN_POINT('Ctrl Pts',(0.00344535402214944,-0.033362046922432,
0.0774953020320032));
#103967=CARTESIAN_POINT('Ctrl Pts',(0.00337728694519171,-0.0331951640388601,
0.0773957630158324));
#103968=CARTESIAN_POINT('Ctrl Pts',(0.00364250092074412,-0.0336938721132427,
0.0777531151250667));
#103969=CARTESIAN_POINT('Ctrl Pts',(0.00356707293039049,-0.0335278710435083,
0.0776593035123785));
#103970=CARTESIAN_POINT('Ctrl Pts',(0.00349461338321189,-0.033362046922432,
0.0775631595002313));
#103971=CARTESIAN_POINT('Ctrl Pts',(0.00342510223505334,-0.0331951640388601,
0.0774646232211669));
#103972=CARTESIAN_POINT('Ctrl Pts',(0.0036945456261215,-0.0336938721132427,
0.0778188371036238));
#103973=CARTESIAN_POINT('Ctrl Pts',(0.00361774180496797,-0.0335278710435083,
0.0777261150002626));
#103974=CARTESIAN_POINT('Ctrl Pts',(0.00354387274427434,-0.033362046922432,
0.0776310169684594));
#103975=CARTESIAN_POINT('Ctrl Pts',(0.00347291752491498,-0.0331951640388601,
0.0775334834265015));
#103976=CARTESIAN_POINT('Ctrl Pts',(0.00340086238574835,-0.0330240426238156,
0.0774295288187784));
#103977=CARTESIAN_POINT('Ctrl Pts',(0.00335568368117981,-0.0329142774063509,
0.0773644659971146));
#103978=CARTESIAN_POINT('Ctrl Pts',(0.00331182748364718,-0.0328043479726686,
0.0772984367692373));
#103979=CARTESIAN_POINT('Ctrl Pts',(0.00326935230575415,-0.0326943950436594,
0.0772315241762339));
#103980=CARTESIAN_POINT('Ctrl Pts',(0.0033783558898554,-0.0330240426238156,
0.0775405900344537));
#103981=CARTESIAN_POINT('Ctrl Pts',(0.00333164720883924,-0.0329142774063509,
0.0774752171638819));
#103982=CARTESIAN_POINT('Ctrl Pts',(0.00328626668168694,-0.0328043479726686,
0.0774088461036391));
#103983=CARTESIAN_POINT('Ctrl Pts',(0.003242274785842,-0.0326943950436594,
0.0773415602789459));
#103984=CARTESIAN_POINT('Ctrl Pts',(0.00335584939396246,-0.0330240426238156,
0.077651651250129));
#103985=CARTESIAN_POINT('Ctrl Pts',(0.00330761073649868,-0.0329142774063509,
0.0775859683306493));
#103986=CARTESIAN_POINT('Ctrl Pts',(0.00326070587972671,-0.0328043479726686,
0.0775192554380409));
#103987=CARTESIAN_POINT('Ctrl Pts',(0.00321519726592985,-0.0326943950436594,
0.077451596381658));
#103988=CARTESIAN_POINT('Ctrl Pts',(0.00333334289806951,-0.0330240426238156,
0.0777627124658043));
#103989=CARTESIAN_POINT('Ctrl Pts',(0.00328357426415811,-0.0329142774063509,
0.0776967194974166));
#103990=CARTESIAN_POINT('Ctrl Pts',(0.00323514507776647,-0.0328043479726686,
0.0776296647724427));
#103991=CARTESIAN_POINT('Ctrl Pts',(0.0031881197460177,-0.0326943950436594,
0.0775616324843701));
#103992=CARTESIAN_POINT('Origin',(0.0174919643009571,-0.032639668285648,
0.0682900632605691));
#103993=CARTESIAN_POINT('Ctrl Pts',(0.00299690974454837,-0.0331951640388587,
0.0772669181728474));
#103994=CARTESIAN_POINT('Ctrl Pts',(0.00295398050219153,-0.0330855618255041,
0.077196305876447));
#103995=CARTESIAN_POINT('Ctrl Pts',(0.0029124797482092,-0.0329757224427708,
0.077124755402571));
#103996=CARTESIAN_POINT('Ctrl Pts',(0.00287246512119015,-0.0328657862078597,
0.0770523557690625));
#103997=CARTESIAN_POINT('Ctrl Pts',(0.00310842899740496,-0.0331951640388587,
0.0772870330499777));
#103998=CARTESIAN_POINT('Ctrl Pts',(0.00306522271330771,-0.0330855618255041,
0.0772179567056837));
#103999=CARTESIAN_POINT('Ctrl Pts',(0.00302341297236491,-0.0329757224427708,
0.0771479375651814));
#104000=CARTESIAN_POINT('Ctrl Pts',(0.00298305771265227,-0.0328657862078597,
0.0770770626659407));
#104001=CARTESIAN_POINT('Ctrl Pts',(0.00321994825026155,-0.0331951640388587,
0.0773071479271078));
#104002=CARTESIAN_POINT('Ctrl Pts',(0.0031764649244239,-0.0330855618255041,
0.0772396075349204));
#104003=CARTESIAN_POINT('Ctrl Pts',(0.00313434619652062,-0.0329757224427708,
0.0771711197277918));
#104004=CARTESIAN_POINT('Ctrl Pts',(0.00309365030411439,-0.0328657862078597,
0.0771017695628188));
#104005=CARTESIAN_POINT('Ctrl Pts',(0.00333146750311814,-0.0331951640388587,
0.077327262804238));
#104006=CARTESIAN_POINT('Ctrl Pts',(0.00328770713554008,-0.0330855618255041,
0.0772612583641571));
#104007=CARTESIAN_POINT('Ctrl Pts',(0.00324527942067632,-0.0329757224427708,
0.0771943018904021));
#104008=CARTESIAN_POINT('Ctrl Pts',(0.0032042428955765,-0.0328657862078597,
0.077126476459697));
#104009=CARTESIAN_POINT('Origin',(0.0177134928710351,-0.0326401908830748,
0.0687169097957367));
#104010=CARTESIAN_POINT('Ctrl Pts',(0.0033495095287428,-0.0332451089994432,
0.0773569370942212));
#104011=CARTESIAN_POINT('Ctrl Pts',(0.00322855791736245,-0.0329451141710257,
0.0771768724546732));
#104012=CARTESIAN_POINT('Ctrl Pts',(0.00312151312150551,-0.0326442513127503,
0.0769882087899389));
#104013=CARTESIAN_POINT('Ctrl Pts',(0.00349338612675748,-0.0332451089994432,
0.0775613864144542));
#104014=CARTESIAN_POINT('Ctrl Pts',(0.0033647235831071,-0.0329451141710257,
0.0773867481695808));
#104015=CARTESIAN_POINT('Ctrl Pts',(0.00324958102269472,-0.0326442513127503,
0.0772029146647653));
#104016=CARTESIAN_POINT('Ctrl Pts',(0.0032042591703819,-0.0325229783203385,
0.0771265035320287));
#104017=CARTESIAN_POINT('Ctrl Pts',(0.00316322813503157,-0.0324130253112079,
0.0770586880159776));
#104018=CARTESIAN_POINT('Ctrl Pts',(0.00312360617388073,-0.0323031222247694,
0.0769900340058193));
#104019=CARTESIAN_POINT('Ctrl Pts',(0.0030854409366981,-0.0321934096636184,
0.0769206312333599));
#104020=CARTESIAN_POINT('Ctrl Pts',(0.00317482350437116,-0.0325229783203385,
0.0772359324323063));
#104021=CARTESIAN_POINT('Ctrl Pts',(0.00313228399405101,-0.0324130253112079,
0.0771677111462504));
#104022=CARTESIAN_POINT('Ctrl Pts',(0.00309116218059378,-0.0323031222247694,
0.0770986202228882));
#104023=CARTESIAN_POINT('Ctrl Pts',(0.00305150761522392,-0.0321934096636184,
0.0770287500214736));
#104024=CARTESIAN_POINT('Ctrl Pts',(0.00314538783836041,-0.0325229783203385,
0.0773453613325839));
#104025=CARTESIAN_POINT('Ctrl Pts',(0.00310133985307044,-0.0324130253112079,
0.0772767342765231));
#104026=CARTESIAN_POINT('Ctrl Pts',(0.00305871818730682,-0.0323031222247694,
0.0772072064399572));
#104027=CARTESIAN_POINT('Ctrl Pts',(0.00301757429374974,-0.0321934096636184,
0.0771368688095874));
#104028=CARTESIAN_POINT('Ctrl Pts',(0.00311595217234966,-0.0325229783203385,
0.0774547902328616));
#104029=CARTESIAN_POINT('Ctrl Pts',(0.00307039571208988,-0.0324130253112079,
0.0773857574067959));
#104030=CARTESIAN_POINT('Ctrl Pts',(0.00302627419401987,-0.0323031222247694,
0.0773157926570261));
#104031=CARTESIAN_POINT('Ctrl Pts',(0.00298364097227555,-0.0321934096636184,
0.0772449875977012));
#104032=CARTESIAN_POINT('Origin',(0.0174846124122548,-0.0326393375177375,
0.0682943807546413));
#104033=CARTESIAN_POINT('Ctrl Pts',(0.00281131354479966,-0.0326943950436594,
0.07693884866222));
#104034=CARTESIAN_POINT('Ctrl Pts',(0.00277287798337493,-0.0325844576448127,
0.0768656328876191));
#104035=CARTESIAN_POINT('Ctrl Pts',(0.00273595392406345,-0.0324744968375319,
0.0767916170209979));
#104036=CARTESIAN_POINT('Ctrl Pts',(0.00270058736808504,-0.0323646534831895,
0.076716896548338));
#104037=CARTESIAN_POINT('Ctrl Pts',(0.00292134961150893,-0.0326943950436594,
0.0769659261732727));
#104038=CARTESIAN_POINT('Ctrl Pts',(0.00288254087123323,-0.0325844576448127,
0.0768942269019006));
#104039=CARTESIAN_POINT('Ctrl Pts',(0.00284521224288721,-0.0324744968375319,
0.076821719927883));
#104040=CARTESIAN_POINT('Ctrl Pts',(0.00280941027271392,-0.0323646534831895,
0.07674849881107));
#104041=CARTESIAN_POINT('Ctrl Pts',(0.00303138567821819,-0.0326943950436594,
0.0769930036843253));
#104042=CARTESIAN_POINT('Ctrl Pts',(0.00299220375909152,-0.0325844576448127,
0.0769228209161821));
#104043=CARTESIAN_POINT('Ctrl Pts',(0.00295447056171098,-0.0324744968375319,
0.0768518228347681));
#104044=CARTESIAN_POINT('Ctrl Pts',(0.0029182331773428,-0.0323646534831895,
0.0767801010738021));
#104045=CARTESIAN_POINT('Ctrl Pts',(0.00314142174492745,-0.0326943950436594,
0.077020081195378));
#104046=CARTESIAN_POINT('Ctrl Pts',(0.00310186664694981,-0.0325844576448127,
0.0769514149304635));
#104047=CARTESIAN_POINT('Ctrl Pts',(0.00306372888053474,-0.0324744968375319,
0.0768819257416532));
#104048=CARTESIAN_POINT('Ctrl Pts',(0.00302705608197167,-0.0323646534831895,
0.0768117033365341));
#104049=CARTESIAN_POINT('Origin',(0.0177461890740257,-0.0326395579065289,
0.0686978593326361));
#104050=CARTESIAN_POINT('Ctrl Pts',(0.00315758500232762,-0.0327445246961876,
0.0770508637441773));
#104051=CARTESIAN_POINT('Ctrl Pts',(0.0030481771387794,-0.0324436878365475,
0.0768635605570858));
#104052=CARTESIAN_POINT('Ctrl Pts',(0.00295318853283271,-0.0321434074463186,
0.0766685484312035));
#104053=CARTESIAN_POINT('Ctrl Pts',(0.00328834166687456,-0.0327445246961876,
0.0772639428249819));
#104054=CARTESIAN_POINT('Ctrl Pts',(0.00317089739450002,-0.0324436878365475,
0.0770815712060626));
#104055=CARTESIAN_POINT('Ctrl Pts',(0.0030675237444488,-0.0321434074463186,
0.0768908713031368));
#104056=CARTESIAN_POINT('Ctrl Pts',(0.00298272819906614,-0.0322357242816072,
0.0767283112361278));
#104057=CARTESIAN_POINT('Ctrl Pts',(0.00290061233014264,-0.0319819883628705,
0.0765645753341203));
#104058=CARTESIAN_POINT('Ctrl Pts',(0.00282908186306855,-0.0317295851069886,
0.0763959459955833));
#104059=CARTESIAN_POINT('Ctrl Pts',(0.00309963265901505,-0.0322357242816072,
0.076949293921522));
#104060=CARTESIAN_POINT('Ctrl Pts',(0.00301047877816578,-0.0319819883628705,
0.0767892812749444));
#104061=CARTESIAN_POINT('Ctrl Pts',(0.00293168764117612,-0.0317295851069886,
0.0766239197973653));
#104062=CARTESIAN_POINT('Origin',(0.0176624456079492,-0.0326371942643908,
0.0687433503804637));
#104063=CARTESIAN_POINT('Origin',(0.0173790431228128,-0.0326352985527103,
0.0683569820973483));
#104064=CARTESIAN_POINT('Ctrl Pts',(0.00264668323176902,-0.0321934096636183,
0.0765997728400263));
#104065=CARTESIAN_POINT('Ctrl Pts',(0.00261289895506826,-0.0320835708272303,
0.0765242393767581));
#104066=CARTESIAN_POINT('Ctrl Pts',(0.00258069743571743,-0.0319739230346346,
0.076448050562118));
#104067=CARTESIAN_POINT('Ctrl Pts',(0.00255011239213904,-0.0318646057455575,
0.0763713070363633));
#104068=CARTESIAN_POINT('Ctrl Pts',(0.00275480211298525,-0.0321934096636183,
0.0766337061907208));
#104069=CARTESIAN_POINT('Ctrl Pts',(0.00272054986893237,-0.0320835708272303,
0.0765596637710874));
#104070=CARTESIAN_POINT('Ctrl Pts',(0.00268784979659898,-0.0319739230346346,
0.0764849554506561));
#104071=CARTESIAN_POINT('Ctrl Pts',(0.00265673639764529,-0.0318646057455575,
0.0764096800244489));
#104072=CARTESIAN_POINT('Ctrl Pts',(0.00286292099420148,-0.0321934096636183,
0.0766676395414154));
#104073=CARTESIAN_POINT('Ctrl Pts',(0.00282820078279648,-0.0320835708272303,
0.0765950881654167));
#104074=CARTESIAN_POINT('Ctrl Pts',(0.00279500215748052,-0.0319739230346346,
0.0765218603391941));
#104075=CARTESIAN_POINT('Ctrl Pts',(0.00276336040315155,-0.0318646057455575,
0.0764480530125344));
#104076=CARTESIAN_POINT('Ctrl Pts',(0.00297103987541771,-0.0321934096636183,
0.07670157289211));
#104077=CARTESIAN_POINT('Ctrl Pts',(0.00293585169666059,-0.0320835708272303,
0.076630512559746));
#104078=CARTESIAN_POINT('Ctrl Pts',(0.00290215451836207,-0.0319739230346346,
0.0765587652277322));
#104079=CARTESIAN_POINT('Ctrl Pts',(0.00286998440865781,-0.0318646057455575,
0.07648642600062));
#104080=CARTESIAN_POINT('Ctrl Pts',(0.00302654010771948,-0.0320218834582394,
0.0768125027555518));
#104081=CARTESIAN_POINT('Ctrl Pts',(0.00299882989059256,-0.0319391099350668,
0.0767594527879451));
#104082=CARTESIAN_POINT('Ctrl Pts',(0.00297196484506484,-0.0318564869454926,
0.0767060022630402));
#104083=CARTESIAN_POINT('Ctrl Pts',(0.00294596090422198,-0.0317740741446496,
0.0766521919392276));
#104084=CARTESIAN_POINT('Ctrl Pts',(0.0030106817987234,-0.0320218834582394,
0.0768594638254233));
#104085=CARTESIAN_POINT('Ctrl Pts',(0.00298248283038676,-0.0319391099350668,
0.0768062488111572));
#104086=CARTESIAN_POINT('Ctrl Pts',(0.00295513190699799,-0.0318564869454926,
0.0767526257076716));
#104087=CARTESIAN_POINT('Ctrl Pts',(0.00292864530380531,-0.0317740741446496,
0.0766986354320969));
#104088=CARTESIAN_POINT('Ctrl Pts',(0.00299482348972731,-0.0320218834582394,
0.0769064248952948));
#104089=CARTESIAN_POINT('Ctrl Pts',(0.00296613577018095,-0.0319391099350668,
0.0768530448343692));
#104090=CARTESIAN_POINT('Ctrl Pts',(0.00293829896893114,-0.0318564869454926,
0.0767992491523032));
#104091=CARTESIAN_POINT('Ctrl Pts',(0.00291132970338863,-0.0317740741446496,
0.0767450789249662));
#104092=CARTESIAN_POINT('Ctrl Pts',(0.00297896518073123,-0.0320218834582394,
0.0769533859651663));
#104093=CARTESIAN_POINT('Ctrl Pts',(0.00294978870997515,-0.0319391099350668,
0.0768998408575813));
#104094=CARTESIAN_POINT('Ctrl Pts',(0.00292146603086429,-0.0318564869454926,
0.0768458725969347));
#104095=CARTESIAN_POINT('Ctrl Pts',(0.00289401410297195,-0.0317740741446496,
0.0767915224178355));
#104096=CARTESIAN_POINT('Ctrl Pts',(0.00493979735941889,-0.0350241211493618,
0.0789378513677008));
#104097=CARTESIAN_POINT('Ctrl Pts',(0.00487384667289248,-0.0349144232867607,
0.0788939932840753));
#104098=CARTESIAN_POINT('Ctrl Pts',(0.00480876308959006,-0.0348045283677605,
0.0788487457015188));
#104099=CARTESIAN_POINT('Ctrl Pts',(0.00474463212999654,-0.0346945769586886,
0.0788021634742698));
#104100=CARTESIAN_POINT('Ctrl Pts',(0.00495975571087317,-0.0350241211493618,
0.0790493986940272));
#104101=CARTESIAN_POINT('Ctrl Pts',(0.00489226850573195,-0.0349144232867607,
0.0790058155284973));
#104102=CARTESIAN_POINT('Ctrl Pts',(0.00482564180138109,-0.0348045283677605,
0.0789608112676519));
#104103=CARTESIAN_POINT('Ctrl Pts',(0.00475996308324953,-0.0346945769586886,
0.0789144403805136));
#104104=CARTESIAN_POINT('Ctrl Pts',(0.00497971406232745,-0.0350241211493618,
0.0791609460203535));
#104105=CARTESIAN_POINT('Ctrl Pts',(0.00491069033857141,-0.0349144232867607,
0.0791176377729192));
#104106=CARTESIAN_POINT('Ctrl Pts',(0.00484252051317211,-0.0348045283677605,
0.079072876833785));
#104107=CARTESIAN_POINT('Ctrl Pts',(0.00477529403650252,-0.0346945769586886,
0.0790267172867574));
#104108=CARTESIAN_POINT('Ctrl Pts',(0.00499967241378172,-0.0350241211493618,
0.0792724933466798));
#104109=CARTESIAN_POINT('Ctrl Pts',(0.00492911217141088,-0.0349144232867607,
0.0792294600173412));
#104110=CARTESIAN_POINT('Ctrl Pts',(0.00485939922496313,-0.0348045283677605,
0.0791849423999181));
#104111=CARTESIAN_POINT('Ctrl Pts',(0.00479062498975552,-0.0346945769586886,
0.0791389941930012));
#104112=CARTESIAN_POINT('Origin',(0.014756343467682,-0.034562906794184,
0.0653251984889228));
#104113=CARTESIAN_POINT('Ctrl Pts',(0.00459642973095872,-0.03519709736516,
0.0789179457195974));
#104114=CARTESIAN_POINT('Ctrl Pts',(0.00453037630472438,-0.0350869349321763,
0.0788690790316434));
#104115=CARTESIAN_POINT('Ctrl Pts',(0.00446528407196257,-0.034976498512972,
0.0788187986489671));
#104116=CARTESIAN_POINT('Ctrl Pts',(0.00440124119607719,-0.0348659306849645,
0.0787671647471887));
#104117=CARTESIAN_POINT('Ctrl Pts',(0.00467703263188872,-0.03519709736516,
0.0789017086320442));
#104118=CARTESIAN_POINT('Ctrl Pts',(0.00461120414849727,-0.0350869349321763,
0.0788539585880463));
#104119=CARTESIAN_POINT('Ctrl Pts',(0.00454631383050936,-0.034976498512972,
0.078804800450778));
#104120=CARTESIAN_POINT('Ctrl Pts',(0.00448244949415718,-0.0348659306849645,
0.0787542929573562));
#104121=CARTESIAN_POINT('Ctrl Pts',(0.00475763553281871,-0.03519709736516,
0.078885471544491));
#104122=CARTESIAN_POINT('Ctrl Pts',(0.00469203199227016,-0.0350869349321763,
0.0788388381444492));
#104123=CARTESIAN_POINT('Ctrl Pts',(0.00462734358905615,-0.034976498512972,
0.0787908022525889));
#104124=CARTESIAN_POINT('Ctrl Pts',(0.00456365779223717,-0.0348659306849645,
0.0787414211675236));
#104125=CARTESIAN_POINT('Ctrl Pts',(0.0048382384337487,-0.03519709736516,
0.0788692344569377));
#104126=CARTESIAN_POINT('Ctrl Pts',(0.00477285983604305,-0.0350869349321763,
0.078823717700852));
#104127=CARTESIAN_POINT('Ctrl Pts',(0.00470837334760294,-0.034976498512972,
0.0787768040543999));
#104128=CARTESIAN_POINT('Ctrl Pts',(0.00464486609031715,-0.0348659306849645,
0.0787285493776911));
#104129=CARTESIAN_POINT('Origin',(0.0151117818539896,-0.0345637187967143,
0.0656492184110888));
#104130=CARTESIAN_POINT('Ctrl Pts',(0.00486532304494461,-0.0352450361861253,
0.0788892582731634));
#104131=CARTESIAN_POINT('Ctrl Pts',(0.00468657899071769,-0.0349452761023765,
0.0787663634729426));
#104132=CARTESIAN_POINT('Ctrl Pts',(0.00451759966846667,-0.0346444289983475,
0.0786303540707146));
#104133=CARTESIAN_POINT('Ctrl Pts',(0.00507435879337509,-0.0352450361861253,
0.0790263861546395));
#104134=CARTESIAN_POINT('Ctrl Pts',(0.00489044287636505,-0.0349452761023765,
0.0789113752668368));
#104135=CARTESIAN_POINT('Ctrl Pts',(0.00471571253552146,-0.0346444289983475,
0.0787828378138066));
#104136=CARTESIAN_POINT('Origin',(-0.00211316800085609,-0.0391228853390801,
0.0805597947748885));
#104137=CARTESIAN_POINT('Ctrl Pts',(0.00509125577588388,-0.0352722978779667,
0.0790375298537638));
#104138=CARTESIAN_POINT('Ctrl Pts',(0.00507538593042427,-0.0352466642097266,
0.0790272711655831));
#104139=CARTESIAN_POINT('Ctrl Pts',(0.00505948766108327,-0.0352210183808325,
0.0790170874588308));
#104140=CARTESIAN_POINT('Ctrl Pts',(0.00504356011959463,-0.0351953608940153,
0.0790069788225492));
#104141=CARTESIAN_POINT('Origin',(0.00228085763488299,-0.0352456003065148,
0.0830514313828313));
#104142=CARTESIAN_POINT('Ctrl Pts',(0.00464544929305672,-0.0345231616327822,
0.0787284802062971));
#104143=CARTESIAN_POINT('Ctrl Pts',(0.00458234138939785,-0.0344132092796975,
0.0786805362843711));
#104144=CARTESIAN_POINT('Ctrl Pts',(0.00452022842402409,-0.0343032738558974,
0.0786312894989229));
#104145=CARTESIAN_POINT('Ctrl Pts',(0.00445918835472738,-0.0341934961088741,
0.0785808049790908));
#104146=CARTESIAN_POINT('Ctrl Pts',(0.00465836416187004,-0.0345231616327822,
0.0788410605878131));
#104147=CARTESIAN_POINT('Ctrl Pts',(0.00459370449615248,-0.0344132092796975,
0.0787932946791711));
#104148=CARTESIAN_POINT('Ctrl Pts',(0.00453003616671946,-0.0343032738558974,
0.0787441938008479));
#104149=CARTESIAN_POINT('Ctrl Pts',(0.00446743912875214,-0.0341934961088741,
0.0786938229460994));
#104150=CARTESIAN_POINT('Ctrl Pts',(0.00467127903068336,-0.0345231616327822,
0.0789536409693292));
#104151=CARTESIAN_POINT('Ctrl Pts',(0.0046050676029071,-0.0344132092796975,
0.0789060530739711));
#104152=CARTESIAN_POINT('Ctrl Pts',(0.00453984390941482,-0.0343032738558974,
0.078857098102773));
#104153=CARTESIAN_POINT('Ctrl Pts',(0.00447568990277691,-0.0341934961088741,
0.078806840913108));
#104154=CARTESIAN_POINT('Ctrl Pts',(0.00468419389949668,-0.0345231616327822,
0.0790662213508453));
#104155=CARTESIAN_POINT('Ctrl Pts',(0.00461643070966173,-0.0344132092796975,
0.0790188114687711));
#104156=CARTESIAN_POINT('Ctrl Pts',(0.00454965165211019,-0.0343032738558974,
0.078970002404698));
#104157=CARTESIAN_POINT('Ctrl Pts',(0.00448394067680167,-0.0341934961088741,
0.0789198588801166));
#104158=CARTESIAN_POINT('Origin',(0.0147634136330329,-0.0345625596229466,
0.0653153744863288));
#104159=CARTESIAN_POINT('Ctrl Pts',(0.0042110174281769,-0.0346945769586885,
0.0786986560536431));
#104160=CARTESIAN_POINT('Ctrl Pts',(0.00414833464864841,-0.0345846629176052,
0.0786447361774831));
#104161=CARTESIAN_POINT('Ctrl Pts',(0.00408675620364244,-0.034474692505031,
0.0785895108375374));
#104162=CARTESIAN_POINT('Ctrl Pts',(0.00402636070232569,-0.0343648066253259,
0.0785330511207269));
#104163=CARTESIAN_POINT('Ctrl Pts',(0.00432329424601654,-0.0346945769586885,
0.0786833251124613));
#104164=CARTESIAN_POINT('Ctrl Pts',(0.00426082273460653,-0.0345846629176052,
0.0786309524676012));
#104165=CARTESIAN_POINT('Ctrl Pts',(0.00419942359769629,-0.034474692505031,
0.0785772789921643));
#104166=CARTESIAN_POINT('Ctrl Pts',(0.00413917522291422,-0.0343648066253259,
0.078522373783695));
#104167=CARTESIAN_POINT('Ctrl Pts',(0.00443557106385618,-0.0346945769586885,
0.0786679941712795));
#104168=CARTESIAN_POINT('Ctrl Pts',(0.00437331082056465,-0.0345846629176052,
0.0786171687577194));
#104169=CARTESIAN_POINT('Ctrl Pts',(0.00431209099175013,-0.034474692505031,
0.0785650471467912));
#104170=CARTESIAN_POINT('Ctrl Pts',(0.00425198974350276,-0.0343648066253259,
0.078511696446663));
#104171=CARTESIAN_POINT('Ctrl Pts',(0.00454784788169582,-0.0346945769586885,
0.0786526632300978));
#104172=CARTESIAN_POINT('Ctrl Pts',(0.00448579890652278,-0.0345846629176052,
0.0786033850478375));
#104173=CARTESIAN_POINT('Ctrl Pts',(0.00442475838580397,-0.034474692505031,
0.0785528153014181));
#104174=CARTESIAN_POINT('Ctrl Pts',(0.0043648042640913,-0.0343648066253259,
0.0785010191096311));
#104175=CARTESIAN_POINT('Origin',(0.0151482818569298,-0.0345626446729742,
0.0656035907819192));
#104176=CARTESIAN_POINT('Ctrl Pts',(0.0045458388729324,-0.0346945769586886,
0.0786529375520441));
#104177=CARTESIAN_POINT('Ctrl Pts',(0.00445152304302849,-0.0345275153362891,
0.0785779960966738));
#104178=CARTESIAN_POINT('Ctrl Pts',(0.00435953965801255,-0.0343603235965159,
0.078500069111566));
#104179=CARTESIAN_POINT('Ctrl Pts',(0.00427015733847041,-0.034193496108874,
0.078419391113463));
#104180=CARTESIAN_POINT('Ctrl Pts',(0.00461259288253264,-0.0346945769586886,
0.0787036517564996));
#104181=CARTESIAN_POINT('Ctrl Pts',(0.00451721482331157,-0.0345275153362891,
0.0786301084905873));
#104182=CARTESIAN_POINT('Ctrl Pts',(0.00442412496246005,-0.0343603235965159,
0.0785535466504464));
#104183=CARTESIAN_POINT('Ctrl Pts',(0.00433359525303593,-0.034193496108874,
0.0784741967639641));
#104184=CARTESIAN_POINT('Ctrl Pts',(0.00467934689213288,-0.0346945769586886,
0.0787543659609552));
#104185=CARTESIAN_POINT('Ctrl Pts',(0.00458290660359465,-0.0345275153362891,
0.0786822208845007));
#104186=CARTESIAN_POINT('Ctrl Pts',(0.00448871026690755,-0.0343603235965159,
0.0786070241893269));
#104187=CARTESIAN_POINT('Ctrl Pts',(0.00439703316760146,-0.034193496108874,
0.0785290024144652));
#104188=CARTESIAN_POINT('Ctrl Pts',(0.00474610090173312,-0.0346945769586886,
0.0788050801654107));
#104189=CARTESIAN_POINT('Ctrl Pts',(0.00464859838387773,-0.0345275153362891,
0.0787343332784142));
#104190=CARTESIAN_POINT('Ctrl Pts',(0.00455329557135505,-0.0343603235965159,
0.0786605017282073));
#104191=CARTESIAN_POINT('Ctrl Pts',(0.00446047108216698,-0.034193496108874,
0.0785838080649662));
#104192=CARTESIAN_POINT('Ctrl Pts',(0.0043648285057152,-0.0340223579322365,
0.0785010393167854));
#104193=CARTESIAN_POINT('Ctrl Pts',(0.00430481632555026,-0.0339125849573552,
0.0784491935416738));
#104194=CARTESIAN_POINT('Ctrl Pts',(0.00424591940232135,-0.0338030433565217,
0.0783961420853078));
#104195=CARTESIAN_POINT('Ctrl Pts',(0.00418820704119181,-0.0336938721132321,
0.0783419594682911));
#104196=CARTESIAN_POINT('Ctrl Pts',(0.00437064893739086,-0.0340223579322365,
0.078614208669552));
#104197=CARTESIAN_POINT('Ctrl Pts',(0.00430907585669322,-0.0339125849573552,
0.0785624431733736));
#104198=CARTESIAN_POINT('Ctrl Pts',(0.00424861746817096,-0.0338030433565217,
0.0785094396325156));
#104199=CARTESIAN_POINT('Ctrl Pts',(0.00418934507927019,-0.0336938721132321,
0.0784552726833185));
#104200=CARTESIAN_POINT('Ctrl Pts',(0.00437646936906652,-0.0340223579322365,
0.0787273780223186));
#104201=CARTESIAN_POINT('Ctrl Pts',(0.00431333538783617,-0.0339125849573552,
0.0786756928050733));
#104202=CARTESIAN_POINT('Ctrl Pts',(0.00425131553402058,-0.0338030433565217,
0.0786227371797234));
#104203=CARTESIAN_POINT('Ctrl Pts',(0.00419048311734857,-0.0336938721132321,
0.0785685858983459));
#104204=CARTESIAN_POINT('Ctrl Pts',(0.00438228980074218,-0.0340223579322365,
0.0788405473750853));
#104205=CARTESIAN_POINT('Ctrl Pts',(0.00431759491897913,-0.0339125849573552,
0.0787889424367731));
#104206=CARTESIAN_POINT('Ctrl Pts',(0.00425401359987019,-0.0338030433565217,
0.0787360347269312));
#104207=CARTESIAN_POINT('Ctrl Pts',(0.00419162115542696,-0.0336938721132321,
0.0786818991133732));
#104208=CARTESIAN_POINT('Origin',(0.0146891305925633,-0.0345589643415143,
0.0654098991288901));
#104209=CARTESIAN_POINT('Ctrl Pts',(0.00393312589888617,-0.034193496108874,
0.0784439957875769));
#104210=CARTESIAN_POINT('Ctrl Pts',(0.00387391423977879,-0.0340836138581107,
0.0783862091188876));
#104211=CARTESIAN_POINT('Ctrl Pts',(0.00381592676539424,-0.0339738896643499,
0.0783272249162861));
#104212=CARTESIAN_POINT('Ctrl Pts',(0.00375923263190683,-0.0338644633294062,
0.0782671236473839));
#104213=CARTESIAN_POINT('Ctrl Pts',(0.00404614396758526,-0.034193496108874,
0.0784357450061283));
#104214=CARTESIAN_POINT('Ctrl Pts',(0.00398704608186814,-0.0340836138581107,
0.0783795167896797));
#104215=CARTESIAN_POINT('Ctrl Pts',(0.00392914007738418,-0.0339738896643499,
0.0783220926458458));
#104216=CARTESIAN_POINT('Ctrl Pts',(0.00387249513988373,-0.0338644633294062,
0.0782635510385658));
#104217=CARTESIAN_POINT('Ctrl Pts',(0.00415916203628435,-0.034193496108874,
0.0784274942246797));
#104218=CARTESIAN_POINT('Ctrl Pts',(0.00410017792395748,-0.0340836138581107,
0.0783728244604719));
#104219=CARTESIAN_POINT('Ctrl Pts',(0.00404235338937413,-0.0339738896643499,
0.0783169603754056));
#104220=CARTESIAN_POINT('Ctrl Pts',(0.00398575764786062,-0.0338644633294062,
0.0782599784297477));
#104221=CARTESIAN_POINT('Ctrl Pts',(0.00427218010498344,-0.034193496108874,
0.0784192434432311));
#104222=CARTESIAN_POINT('Ctrl Pts',(0.00421330976604683,-0.0340836138581107,
0.078366132131264));
#104223=CARTESIAN_POINT('Ctrl Pts',(0.00415556670136407,-0.0339738896643499,
0.0783118281049653));
#104224=CARTESIAN_POINT('Ctrl Pts',(0.00409902015583752,-0.0338644633294062,
0.0782564058209295));
#104225=CARTESIAN_POINT('Origin',(0.0150996077902769,-0.0345610621862833,
0.0656610136081441));
#104226=CARTESIAN_POINT('Ctrl Pts',(0.00429708900780242,-0.03424362768739,
0.0784435468165065));
#104227=CARTESIAN_POINT('Ctrl Pts',(0.00413515522010882,-0.0339430054201861,
0.0782992207037796));
#104228=CARTESIAN_POINT('Ctrl Pts',(0.00398455270349793,-0.0336441434784164,
0.0781431070900165));
#104229=CARTESIAN_POINT('Ctrl Pts',(0.00448729198063623,-0.03424362768739,
0.0786057899338495));
#104230=CARTESIAN_POINT('Ctrl Pts',(0.00431923909289752,-0.0339430054201861,
0.0784686374445015));
#104231=CARTESIAN_POINT('Ctrl Pts',(0.00416199451325736,-0.0336441434784164,
0.0783192161589178));
#104232=CARTESIAN_POINT('Ctrl Pts',(0.00409904004918011,-0.0335235895815127,
0.0782564251414534));
#104233=CARTESIAN_POINT('Ctrl Pts',(0.00404250702230167,-0.0334144449262719,
0.0782010166418549));
#104234=CARTESIAN_POINT('Ctrl Pts',(0.00398705374372666,-0.0333049234473133,
0.0781443765548139));
#104235=CARTESIAN_POINT('Ctrl Pts',(0.00393275768176867,-0.0331951640388588,
0.0780865708824843));
#104236=CARTESIAN_POINT('Ctrl Pts',(0.00409774298180513,-0.0335235895815127,
0.0783697366152884));
#104237=CARTESIAN_POINT('Ctrl Pts',(0.00403964999939961,-0.0334144449262719,
0.0783143102590038));
#104238=CARTESIAN_POINT('Ctrl Pts',(0.00398263534200331,-0.0333049234473133,
0.0782576200672543));
#104239=CARTESIAN_POINT('Ctrl Pts',(0.00392677848025757,-0.0331951640388588,
0.0781997319254086));
#104240=CARTESIAN_POINT('Ctrl Pts',(0.00409644591443015,-0.0335235895815127,
0.0784830480891234));
#104241=CARTESIAN_POINT('Ctrl Pts',(0.00403679297649755,-0.0334144449262719,
0.0784276038761527));
#104242=CARTESIAN_POINT('Ctrl Pts',(0.00397821694027996,-0.0333049234473133,
0.0783708635796947));
#104243=CARTESIAN_POINT('Ctrl Pts',(0.00392079927874647,-0.0331951640388588,
0.0783128929683329));
#104244=CARTESIAN_POINT('Ctrl Pts',(0.00409514884705517,-0.0335235895815127,
0.0785963595629584));
#104245=CARTESIAN_POINT('Ctrl Pts',(0.0040339359535955,-0.0334144449262719,
0.0785408974933015));
#104246=CARTESIAN_POINT('Ctrl Pts',(0.00397379853855662,-0.0333049234473133,
0.0784841070921351));
#104247=CARTESIAN_POINT('Ctrl Pts',(0.00391482007723537,-0.0331951640388588,
0.0784260540112573));
#104248=CARTESIAN_POINT('Origin',(0.0165895953408375,-0.0326434571771486,
0.0672424341472882));
#104249=CARTESIAN_POINT('Ctrl Pts',(0.00366974550751436,-0.0336938721132452,
0.0781724094443434));
#104250=CARTESIAN_POINT('Ctrl Pts',(0.00364620101025808,-0.0336474569764989,
0.0781463384896148));
#104251=CARTESIAN_POINT('Ctrl Pts',(0.00362296331972801,-0.033601104548885,
0.0781199937032171));
#104252=CARTESIAN_POINT('Ctrl Pts',(0.00356413083252362,-0.0334837508643197,
0.0780532947639813));
#104253=CARTESIAN_POINT('Ctrl Pts',(0.00350730060798373,-0.0333660264760478,
0.0779848817855008));
#104254=CARTESIAN_POINT('Ctrl Pts',(0.00400968430076233,-0.0336938721132452,
0.078168995338663));
#104255=CARTESIAN_POINT('Ctrl Pts',(0.00398615978739951,-0.0336474569764989,
0.0781449141584951));
#104256=CARTESIAN_POINT('Ctrl Pts',(0.00396291878657009,-0.033601104548885,
0.0781205592442541));
#104257=CARTESIAN_POINT('Ctrl Pts',(0.00390407791844918,-0.0334837508643197,
0.0780588982036015));
#104258=CARTESIAN_POINT('Ctrl Pts',(0.00384709003329916,-0.0333660264760478,
0.0779955206630868));
#104259=CARTESIAN_POINT('Ctrl Pts',(0.00400968430076601,-0.0336938721132427,
0.0781689953386665));
#104260=CARTESIAN_POINT('Ctrl Pts',(0.00398615978740639,-0.0336474569765026,
0.0781449141585017));
#104261=CARTESIAN_POINT('Ctrl Pts',(0.00396291878658009,-0.0336011045488949,
0.0781205592442641));
#104262=CARTESIAN_POINT('Ctrl Pts',(0.00390456798274507,-0.0334847282606778,
0.0780594117560933));
#104263=CARTESIAN_POINT('Ctrl Pts',(0.00384803921977251,-0.0333679869945434,
0.0779965760132826));
#104264=CARTESIAN_POINT('Ctrl Pts',(0.00400968430076107,-0.0336938721132427,
0.0781689953386617));
#104265=CARTESIAN_POINT('Ctrl Pts',(0.00392555023034879,-0.0335278710435083,
0.0780828703814048));
#104266=CARTESIAN_POINT('Ctrl Pts',(0.00384414661437448,-0.033362046922432,
0.0779941373001344));
#104267=CARTESIAN_POINT('Ctrl Pts',(0.00376544772787081,-0.0331951640388601,
0.0779027384253533));
#104268=CARTESIAN_POINT('Ctrl Pts',(0.00406955576618036,-0.0336938721132427,
0.0782276761485728));
#104269=CARTESIAN_POINT('Ctrl Pts',(0.00398419326553195,-0.0335278710435083,
0.0781428045468594));
#104270=CARTESIAN_POINT('Ctrl Pts',(0.00390152234657642,-0.033362046922432,
0.0780552858569522));
#104271=CARTESIAN_POINT('Ctrl Pts',(0.00382151645208865,-0.0331951640388601,
0.0779650628025091));
#104272=CARTESIAN_POINT('Ctrl Pts',(0.00412942723159965,-0.0336938721132427,
0.0782863569584839));
#104273=CARTESIAN_POINT('Ctrl Pts',(0.0040428363007151,-0.0335278710435083,
0.0782027387123141));
#104274=CARTESIAN_POINT('Ctrl Pts',(0.00395889807877836,-0.033362046922432,
0.07811643441377));
#104275=CARTESIAN_POINT('Ctrl Pts',(0.00387758517630648,-0.0331951640388601,
0.078027387179665));
#104276=CARTESIAN_POINT('Ctrl Pts',(0.00418929869701894,-0.0336938721132427,
0.078345037768395));
#104277=CARTESIAN_POINT('Ctrl Pts',(0.00410147933589826,-0.0335278710435083,
0.0782626728777687));
#104278=CARTESIAN_POINT('Ctrl Pts',(0.0040162738109803,-0.033362046922432,
0.0781775829705879));
#104279=CARTESIAN_POINT('Ctrl Pts',(0.00393365390052432,-0.0331951640388601,
0.0780897115568208));
#104280=CARTESIAN_POINT('Ctrl Pts',(0.00384913797052196,-0.0330240426238156,
0.0779956075658159));
#104281=CARTESIAN_POINT('Ctrl Pts',(0.00379616097970921,-0.0329142774063509,
0.077936720177066));
#104282=CARTESIAN_POINT('Ctrl Pts',(0.00374437494475373,-0.0328043479726686,
0.0778767082484212));
#104283=CARTESIAN_POINT('Ctrl Pts',(0.00369384832467781,-0.0326943950436594,
0.077815646832591));
#104284=CARTESIAN_POINT('Ctrl Pts',(0.00384072860635565,-0.0330240426238156,
0.0781086138425399));
#104285=CARTESIAN_POINT('Ctrl Pts',(0.00378619484398436,-0.0329142774063509,
0.0780496106066058));
#104286=CARTESIAN_POINT('Ctrl Pts',(0.00373285365624783,-0.0328043479726686,
0.0779894505902059));
#104287=CARTESIAN_POINT('Ctrl Pts',(0.00368077549965953,-0.0326943950436594,
0.0779282089808946));
#104288=CARTESIAN_POINT('Ctrl Pts',(0.00383231924218934,-0.0330240426238156,
0.0782216201192638));
#104289=CARTESIAN_POINT('Ctrl Pts',(0.0037762287082595,-0.0329142774063509,
0.0781625010361455));
#104290=CARTESIAN_POINT('Ctrl Pts',(0.00372133236774193,-0.0328043479726686,
0.0781021929319906));
#104291=CARTESIAN_POINT('Ctrl Pts',(0.00366770267464125,-0.0326943950436594,
0.0780407711291983));
#104292=CARTESIAN_POINT('Ctrl Pts',(0.00382390987802303,-0.0330240426238156,
0.0783346263959878));
#104293=CARTESIAN_POINT('Ctrl Pts',(0.00376626257253464,-0.0329142774063509,
0.0782753914656852));
#104294=CARTESIAN_POINT('Ctrl Pts',(0.00370981107923603,-0.0328043479726686,
0.0782149352737753));
#104295=CARTESIAN_POINT('Ctrl Pts',(0.00365462984962296,-0.0326943950436594,
0.078153333277502));
#104296=CARTESIAN_POINT('Origin',(0.0166836485668985,-0.0326396682856619,
0.0671621260557949));
#104297=CARTESIAN_POINT('Ctrl Pts',(0.00342799009848604,-0.0331951640388587,
0.077884907844126));
#104298=CARTESIAN_POINT('Ctrl Pts',(0.00337654929859024,-0.0330855618255041,
0.0778202328075326));
#104299=CARTESIAN_POINT('Ctrl Pts',(0.00332640813819479,-0.0329757224427707,
0.0777544479542062));
#104300=CARTESIAN_POINT('Ctrl Pts',(0.00327763495828507,-0.0328657862078596,
0.0776876343760267));
#104301=CARTESIAN_POINT('Ctrl Pts',(0.0035411510513182,-0.0331951640388587,
0.0778908870408769));
#104302=CARTESIAN_POINT('Ctrl Pts',(0.00348962790008298,-0.0330855618255041,
0.077827770567486));
#104303=CARTESIAN_POINT('Ctrl Pts',(0.00343937211614491,-0.0329757224427707,
0.077763543698847));
#104304=CARTESIAN_POINT('Ctrl Pts',(0.00339045208940823,-0.0328657862078596,
0.0776982855245472));
#104305=CARTESIAN_POINT('Ctrl Pts',(0.00365431200415035,-0.0331951640388587,
0.0778968662376277));
#104306=CARTESIAN_POINT('Ctrl Pts',(0.0036027065015757,-0.0330855618255041,
0.0778353083274393));
#104307=CARTESIAN_POINT('Ctrl Pts',(0.00355233609409502,-0.0329757224427707,
0.0777726394434879));
#104308=CARTESIAN_POINT('Ctrl Pts',(0.0035032692205314,-0.0328657862078596,
0.0777089366730677));
#104309=CARTESIAN_POINT('Ctrl Pts',(0.00376747295698251,-0.0331951640388587,
0.0779028454343785));
#104310=CARTESIAN_POINT('Ctrl Pts',(0.00371578510306843,-0.0330855618255041,
0.0778428460873926));
#104311=CARTESIAN_POINT('Ctrl Pts',(0.00366530007204514,-0.0329757224427707,
0.0777817351881287));
#104312=CARTESIAN_POINT('Ctrl Pts',(0.00361608635165456,-0.0328657862078596,
0.0777195878215882));
#104313=CARTESIAN_POINT('Origin',(0.0169569283738614,-0.0326401908834453,
0.0675578418864235));
#104314=CARTESIAN_POINT('Ctrl Pts',(0.00378909189056348,-0.0332451089994431,
0.0779300244683103));
#104315=CARTESIAN_POINT('Ctrl Pts',(0.00364652593524024,-0.0329451141710258,
0.0777665389487869));
#104316=CARTESIAN_POINT('Ctrl Pts',(0.00351667939241414,-0.0326442513127504,
0.077592779223801));
#104317=CARTESIAN_POINT('Ctrl Pts',(0.00395745827303377,-0.0332451089994431,
0.0781148291253237));
#104318=CARTESIAN_POINT('Ctrl Pts',(0.00380792229603575,-0.0329451141710258,
0.0779576936478073));
#104319=CARTESIAN_POINT('Ctrl Pts',(0.00367064722150769,-0.0326442513127504,
0.0777897409145031));
#104320=CARTESIAN_POINT('Ctrl Pts',(0.00361610589119112,-0.0325229783203385,
0.0777196126406724));
#104321=CARTESIAN_POINT('Ctrl Pts',(0.00356689885989739,-0.0324130253112079,
0.077657474422558));
#104322=CARTESIAN_POINT('Ctrl Pts',(0.00351898470065442,-0.0323031222247694,
0.0775943277182869));
#104323=CARTESIAN_POINT('Ctrl Pts',(0.00347242193387571,-0.0321934096636184,
0.0775302555800038));
#104324=CARTESIAN_POINT('Ctrl Pts',(0.00360061741211605,-0.0325229783203385,
0.0778318679285898));
#104325=CARTESIAN_POINT('Ctrl Pts',(0.0035498629441614,-0.0324130253112079,
0.0777695162021339));
#104326=CARTESIAN_POINT('Ctrl Pts',(0.00350040599965085,-0.0323031222247694,
0.0777061240111895));
#104327=CARTESIAN_POINT('Ctrl Pts',(0.00345230706410009,-0.0321934096636184,
0.0776417747920857));
#104328=CARTESIAN_POINT('Ctrl Pts',(0.00358512893304098,-0.0325229783203385,
0.0779441232165072));
#104329=CARTESIAN_POINT('Ctrl Pts',(0.00353282702842542,-0.0324130253112079,
0.0778815579817098));
#104330=CARTESIAN_POINT('Ctrl Pts',(0.00348182729864727,-0.0323031222247694,
0.0778179203040921));
#104331=CARTESIAN_POINT('Ctrl Pts',(0.00343219219432447,-0.0321934096636184,
0.0777532940041677));
#104332=CARTESIAN_POINT('Ctrl Pts',(0.00356964045396591,-0.0325229783203385,
0.0780563785044246));
#104333=CARTESIAN_POINT('Ctrl Pts',(0.00351579111268944,-0.0324130253112079,
0.0779935997612857));
#104334=CARTESIAN_POINT('Ctrl Pts',(0.00346324859764369,-0.0323031222247694,
0.0779297165969947));
#104335=CARTESIAN_POINT('Ctrl Pts',(0.00341207732454886,-0.0321934096636184,
0.0778648132162496));
#104336=CARTESIAN_POINT('Origin',(0.016676895775367,-0.0326393375177862,
0.0671673309411812));
#104337=CARTESIAN_POINT('Ctrl Pts',(0.00320273936760646,-0.0326943950436593,
0.0775826866314311));
#104338=CARTESIAN_POINT('Ctrl Pts',(0.00315543051228508,-0.0325844576448126,
0.0775148654382787));
#104339=CARTESIAN_POINT('Ctrl Pts',(0.00310952096231126,-0.0324744968375318,
0.0774460610206231));
#104340=CARTESIAN_POINT('Ctrl Pts',(0.00306506832373831,-0.0323646534831894,
0.0773763623460288));
#104341=CARTESIAN_POINT('Ctrl Pts',(0.00331530147908066,-0.0326943950436593,
0.0775957594521721));
#104342=CARTESIAN_POINT('Ctrl Pts',(0.00326781245578839,-0.0325844576448126,
0.0775294895758797));
#104343=CARTESIAN_POINT('Ctrl Pts',(0.00322169064131683,-0.0324744968375318,
0.0774622328587041));
#104344=CARTESIAN_POINT('Ctrl Pts',(0.00317699394103653,-0.0323646534831894,
0.0773940762889571));
#104345=CARTESIAN_POINT('Ctrl Pts',(0.00342786359055486,-0.0326943950436593,
0.0776088322729131));
#104346=CARTESIAN_POINT('Ctrl Pts',(0.0033801943992917,-0.0325844576448126,
0.0775441137134806));
#104347=CARTESIAN_POINT('Ctrl Pts',(0.0033338603203224,-0.0324744968375318,
0.0774784046967851));
#104348=CARTESIAN_POINT('Ctrl Pts',(0.00328891955833475,-0.0323646534831894,
0.0774117902318853));
#104349=CARTESIAN_POINT('Ctrl Pts',(0.00354042570202905,-0.0326943950436593,
0.077621905093654));
#104350=CARTESIAN_POINT('Ctrl Pts',(0.00349257634279501,-0.0325844576448126,
0.0775587378510816));
#104351=CARTESIAN_POINT('Ctrl Pts',(0.00344602999932797,-0.0324744968375318,
0.0774945765348661));
#104352=CARTESIAN_POINT('Ctrl Pts',(0.00340084517563298,-0.0323646534831894,
0.0774295041748136));
#104353=CARTESIAN_POINT('Origin',(0.0169869791008811,-0.0326395579070497,
0.0675348437211409));
#104354=CARTESIAN_POINT('Ctrl Pts',(0.00356031958369538,-0.0327445246961878,
0.0776504191195471));
#104355=CARTESIAN_POINT('Ctrl Pts',(0.00342829911973467,-0.0324436878365476,
0.0774783053153463));
#104356=CARTESIAN_POINT('Ctrl Pts',(0.0033096180269965,-0.0321434074463187,
0.077296736147459));
#104357=CARTESIAN_POINT('Ctrl Pts',(0.0037167510830894,-0.0327445246961878,
0.0778454298525781));
#104358=CARTESIAN_POINT('Ctrl Pts',(0.00357737566917189,-0.0324436878365476,
0.0776792159587661));
#104359=CARTESIAN_POINT('Ctrl Pts',(0.00345091611575342,-0.0321434074463187,
0.0775029759353604));
#104360=CARTESIAN_POINT('Ctrl Pts',(0.00334641502972665,-0.0322357242816073,
0.0773523254029287));
#104361=CARTESIAN_POINT('Ctrl Pts',(0.00324442511890726,-0.0319819883628706,
0.0772001724547932));
#104362=CARTESIAN_POINT('Ctrl Pts',(0.0031523238306585,-0.0317295851069886,
0.0770418379536945));
#104363=CARTESIAN_POINT('Ctrl Pts',(0.00349009413761337,-0.0322357242816073,
0.0775569135598608));
#104364=CARTESIAN_POINT('Ctrl Pts',(0.0033815883593368,-0.0319819883628706,
0.0774093366049665));
#104365=CARTESIAN_POINT('Ctrl Pts',(0.00328269322530411,-0.0317295851069886,
0.0772551542000042));
#104366=CARTESIAN_POINT('Origin',(0.0169095975179532,-0.0326371942645834,
0.0675904718978414));
#104367=CARTESIAN_POINT('Origin',(0.0165800049600085,-0.0326352985529742,
0.0672426699936465));
#104368=CARTESIAN_POINT('Ctrl Pts',(0.00299690974454782,-0.0321934096636183,
0.0772669181728473));
#104369=CARTESIAN_POINT('Ctrl Pts',(0.00295392501376602,-0.0320835708272303,
0.0771962146061403));
#104370=CARTESIAN_POINT('Ctrl Pts',(0.00291242842251313,-0.0319739230346346,
0.0771246624836061));
#104371=CARTESIAN_POINT('Ctrl Pts',(0.00287246603690069,-0.0318646057455575,
0.0770523574258845));
#104372=CARTESIAN_POINT('Ctrl Pts',(0.00310842905266035,-0.0321934096636183,
0.0772870330599441));
#104373=CARTESIAN_POINT('Ctrl Pts',(0.0030651669219089,-0.0320835708272303,
0.0772178674314088));
#104374=CARTESIAN_POINT('Ctrl Pts',(0.00302336126403907,-0.0319739230346346,
0.0771478466142018));
#104375=CARTESIAN_POINT('Ctrl Pts',(0.00298305869095478,-0.0318646057455575,
0.0770770643001119));
#104376=CARTESIAN_POINT('Ctrl Pts',(0.00321994836077288,-0.0321934096636183,
0.0773071479470409));
#104377=CARTESIAN_POINT('Ctrl Pts',(0.00317640883005177,-0.0320835708272303,
0.0772395202566774));
#104378=CARTESIAN_POINT('Ctrl Pts',(0.00313429410556502,-0.0319739230346346,
0.0771710307447974));
#104379=CARTESIAN_POINT('Ctrl Pts',(0.00309365134500887,-0.0318646057455575,
0.0771017711743393));
#104380=CARTESIAN_POINT('Ctrl Pts',(0.0033314676688854,-0.0321934096636183,
0.0773272628341376));
#104381=CARTESIAN_POINT('Ctrl Pts',(0.00328765073819465,-0.0320835708272303,
0.0772611730819459));
#104382=CARTESIAN_POINT('Ctrl Pts',(0.00324522694709097,-0.0319739230346346,
0.077194214875393));
#104383=CARTESIAN_POINT('Ctrl Pts',(0.00320424399906295,-0.0318646057455575,
0.0771264780485666));
#104384=CARTESIAN_POINT('Ctrl Pts',(0.00340043346376184,-0.0320218834582391,
0.0774303619588967));
#104385=CARTESIAN_POINT('Ctrl Pts',(0.00336629282599294,-0.0319391099350663,
0.0773812033172451));
#104386=CARTESIAN_POINT('Ctrl Pts',(0.00333294049225132,-0.0318564869454921,
0.0773315413487196));
#104387=CARTESIAN_POINT('Ctrl Pts',(0.0033003973783664,-0.0317740741446491,
0.0772814144933739));
#104388=CARTESIAN_POINT('Ctrl Pts',(0.00339058598500747,-0.0320218834582391,
0.077478940299851));
#104389=CARTESIAN_POINT('Ctrl Pts',(0.00335593976414661,-0.0319391099350663,
0.0774296791697517));
#104390=CARTESIAN_POINT('Ctrl Pts',(0.00332208375400445,-0.0318564869454921,
0.0773799068801228));
#104391=CARTESIAN_POINT('Ctrl Pts',(0.00328903922977025,-0.0317740741446491,
0.0773296619856212));
#104392=CARTESIAN_POINT('Ctrl Pts',(0.00338073850625309,-0.0320218834582391,
0.0775275186408052));
#104393=CARTESIAN_POINT('Ctrl Pts',(0.00334558670230027,-0.0319391099350663,
0.0774781550222582));
#104394=CARTESIAN_POINT('Ctrl Pts',(0.00331122701575758,-0.0318564869454921,
0.077428272411526));
#104395=CARTESIAN_POINT('Ctrl Pts',(0.0032776810811741,-0.0317740741446491,
0.0773779094778686));
#104396=CARTESIAN_POINT('Ctrl Pts',(0.00337089102749872,-0.0320218834582391,
0.0775760969817595));
#104397=CARTESIAN_POINT('Ctrl Pts',(0.00333523364045393,-0.0319391099350663,
0.0775266308747648));
#104398=CARTESIAN_POINT('Ctrl Pts',(0.00330037027751072,-0.0318564869454921,
0.0774766379429291));
#104399=CARTESIAN_POINT('Ctrl Pts',(0.00326632293257795,-0.0317740741446491,
0.0774261569701159));
#104400=CARTESIAN_POINT('Origin',(-0.00122908628533505,-0.039122885339083,
0.0817922816982227));
#104401=CARTESIAN_POINT('Ctrl Pts',(0.00572773807316979,-0.0352722978779668,
0.0793790665627724));
#104402=CARTESIAN_POINT('Ctrl Pts',(0.00571070761161987,-0.0352466642097266,
0.0793708777864596));
#104403=CARTESIAN_POINT('Ctrl Pts',(0.00569365834798426,-0.0352210183808326,
0.0793627669627815));
#104404=CARTESIAN_POINT('Ctrl Pts',(0.00567658945184547,-0.0351953608940152,
0.0793547342863937));
#104405=CARTESIAN_POINT('Origin',(0.00344257601878882,-0.035245600306513,
0.0837135535659921));
#104406=CARTESIAN_POINT('Ctrl Pts',(0.00556498092456399,-0.035024121149334,
0.0792991568444217));
#104407=CARTESIAN_POINT('Ctrl Pts',(0.00549405340346672,-0.0349144232867422,
0.0792639104076861));
#104408=CARTESIAN_POINT('Ctrl Pts',(0.00542381199783139,-0.0348045283677512,
0.0792271767517832));
#104409=CARTESIAN_POINT('Ctrl Pts',(0.00535434842884735,-0.0346945769586886,
0.0791889995798501));
#104410=CARTESIAN_POINT('Ctrl Pts',(0.00559876248555947,-0.035024121149334,
0.0794073231420385));
#104411=CARTESIAN_POINT('Ctrl Pts',(0.00552634501812962,-0.0349144232867422,
0.0793725420324337));
#104412=CARTESIAN_POINT('Ctrl Pts',(0.00545460315571319,-0.0348045283677512,
0.0793362431839283));
#104413=CARTESIAN_POINT('Ctrl Pts',(0.00538363052066906,-0.0346945769586886,
0.0792984696712083));
#104414=CARTESIAN_POINT('Ctrl Pts',(0.00563254404655495,-0.035024121149334,
0.0795154894396554));
#104415=CARTESIAN_POINT('Ctrl Pts',(0.00555863663279252,-0.0349144232867422,
0.0794811736571813));
#104416=CARTESIAN_POINT('Ctrl Pts',(0.00548539431359499,-0.0348045283677512,
0.0794453096160734));
#104417=CARTESIAN_POINT('Ctrl Pts',(0.00541291261249077,-0.0346945769586886,
0.0794079397625665));
#104418=CARTESIAN_POINT('Ctrl Pts',(0.00566632560755044,-0.035024121149334,
0.0796236557372722));
#104419=CARTESIAN_POINT('Ctrl Pts',(0.00559092824745542,-0.0349144232867422,
0.0795898052819289));
#104420=CARTESIAN_POINT('Ctrl Pts',(0.00551618547147678,-0.0348045283677512,
0.0795543760482185));
#104421=CARTESIAN_POINT('Ctrl Pts',(0.00544219470431248,-0.0346945769586886,
0.0795174098539247));
#104422=CARTESIAN_POINT('Origin',(0.0135980028313961,-0.0345629067942075,
0.0645635043344994));
#104423=CARTESIAN_POINT('Ctrl Pts',(0.00522182601318706,-0.0351970973651599,
0.0793224435334846));
#104424=CARTESIAN_POINT('Ctrl Pts',(0.00515016881793308,-0.0350869349321764,
0.0792822408634588));
#104425=CARTESIAN_POINT('Ctrl Pts',(0.0050792880539232,-0.0349764985129723,
0.07924051517663));
#104426=CARTESIAN_POINT('Ctrl Pts',(0.00500927873137156,-0.0348659306849651,
0.079197315124311));
#104427=CARTESIAN_POINT('Ctrl Pts',(0.00529975828948135,-0.0351970973651599,
0.0792962322580083));
#104428=CARTESIAN_POINT('Ctrl Pts',(0.00522846421592652,-0.0350869349321764,
0.0792571092340537));
#104429=CARTESIAN_POINT('Ctrl Pts',(0.00515792442917808,-0.0349764985129723,
0.0792164716367612));
#104430=CARTESIAN_POINT('Ctrl Pts',(0.00508823341472374,-0.0348659306849651,
0.0791743667337953));
#104431=CARTESIAN_POINT('Ctrl Pts',(0.00537769056577565,-0.0351970973651599,
0.0792700209825321));
#104432=CARTESIAN_POINT('Ctrl Pts',(0.00530675961391997,-0.0350869349321764,
0.0792319776046486));
#104433=CARTESIAN_POINT('Ctrl Pts',(0.00523656080443296,-0.0349764985129723,
0.0791924280968924));
#104434=CARTESIAN_POINT('Ctrl Pts',(0.00516718809807591,-0.0348659306849651,
0.0791514183432797));
#104435=CARTESIAN_POINT('Ctrl Pts',(0.00545562284206994,-0.0351970973651599,
0.0792438097070558));
#104436=CARTESIAN_POINT('Ctrl Pts',(0.00538505501191342,-0.0350869349321764,
0.0792068459752435));
#104437=CARTESIAN_POINT('Ctrl Pts',(0.00531519717968783,-0.0349764985129723,
0.0791683845570235));
#104438=CARTESIAN_POINT('Ctrl Pts',(0.00524614278142808,-0.0348659306849651,
0.079128469952764));
#104439=CARTESIAN_POINT('Origin',(0.0139912489451564,-0.0345637187967834,
0.0648404210190056));
#104440=CARTESIAN_POINT('Ctrl Pts',(0.00548500353265436,-0.0352450361861252,
0.0792602810276083));
#104441=CARTESIAN_POINT('Ctrl Pts',(0.00529226612598336,-0.0349452761023764,
0.0791607578598907));
#104442=CARTESIAN_POINT('Ctrl Pts',(0.00510757275798361,-0.0346444289983475,
0.0790469996572866));
#104443=CARTESIAN_POINT('Ctrl Pts',(0.00570957765256976,-0.0352450361861252,
0.0793701284884993));
#104444=CARTESIAN_POINT('Ctrl Pts',(0.00551269728103495,-0.0349452761023764,
0.079279075272482));
#104445=CARTESIAN_POINT('Ctrl Pts',(0.00532323472649595,-0.0346444289983475,
0.0791734508942809));
#104446=CARTESIAN_POINT('Ctrl Pts',(0.0052467127159667,-0.0345231616327822,
0.0791283282321213));
#104447=CARTESIAN_POINT('Ctrl Pts',(0.00517809347021286,-0.0344132092796975,
0.079088671879969));
#104448=CARTESIAN_POINT('Ctrl Pts',(0.00511029802526044,-0.0343032738558974,
0.0790475982389298));
#104449=CARTESIAN_POINT('Ctrl Pts',(0.00504341188702641,-0.0341934961088741,
0.0790051621538775));
#104450=CARTESIAN_POINT('Ctrl Pts',(0.00527363581043336,-0.0345231616327822,
0.079238402221434));
#104451=CARTESIAN_POINT('Ctrl Pts',(0.00520349934970864,-0.0344132092796975,
0.0791991169662342));
#104452=CARTESIAN_POINT('Ctrl Pts',(0.0051341790922189,-0.0343032738558974,
0.0791583830206058));
#104453=CARTESIAN_POINT('Ctrl Pts',(0.00506576250848974,-0.0341934961088741,
0.079116254844272));
#104454=CARTESIAN_POINT('Ctrl Pts',(0.00530055890490002,-0.0345231616327822,
0.0793484762107467));
#104455=CARTESIAN_POINT('Ctrl Pts',(0.00522890522920441,-0.0344132092796975,
0.0793095620524994));
#104456=CARTESIAN_POINT('Ctrl Pts',(0.00515806015917737,-0.0343032738558974,
0.0792691678022817));
#104457=CARTESIAN_POINT('Ctrl Pts',(0.00508811312995308,-0.0341934961088741,
0.0792273475346664));
#104458=CARTESIAN_POINT('Ctrl Pts',(0.00532748199936668,-0.0345231616327822,
0.0794585502000594));
#104459=CARTESIAN_POINT('Ctrl Pts',(0.00525431110870019,-0.0344132092796975,
0.0794200071387646));
#104460=CARTESIAN_POINT('Ctrl Pts',(0.00518194122613583,-0.0343032738558974,
0.0793799525839576));
#104461=CARTESIAN_POINT('Ctrl Pts',(0.00511046375141642,-0.0341934961088741,
0.0793384402250608));
#104462=CARTESIAN_POINT('Origin',(0.0136037859726627,-0.0345625596230417,
0.0645528716695589));
#104463=CARTESIAN_POINT('Ctrl Pts',(0.00481196851860944,-0.0346945769586886,
0.0791531880022078));
#104464=CARTESIAN_POINT('Ctrl Pts',(0.00474302205908745,-0.0345846629176052,
0.0791075495358235));
#104465=CARTESIAN_POINT('Ctrl Pts',(0.00467500760808286,-0.0344746925050311,
0.0790604774898087));
#104466=CARTESIAN_POINT('Ctrl Pts',(0.00460801206445927,-0.0343648066253259,
0.0790120325382018));
#104467=CARTESIAN_POINT('Ctrl Pts',(0.00492143852377309,-0.0346945769586886,
0.0791239059334422));
#104468=CARTESIAN_POINT('Ctrl Pts',(0.00485289558595925,-0.0345846629176052,
0.0790797760190604));
#104469=CARTESIAN_POINT('Ctrl Pts',(0.00478525352934943,-0.0344746925050311,
0.0790342211273758));
#104470=CARTESIAN_POINT('Ctrl Pts',(0.00471859878368086,-0.0343648066253259,
0.0789872999865031));
#104471=CARTESIAN_POINT('Ctrl Pts',(0.00503090852893673,-0.0346945769586886,
0.0790946238646766));
#104472=CARTESIAN_POINT('Ctrl Pts',(0.00496276911283105,-0.0345846629176052,
0.0790520025022974));
#104473=CARTESIAN_POINT('Ctrl Pts',(0.004895499450616,-0.0344746925050311,
0.0790079647649429));
#104474=CARTESIAN_POINT('Ctrl Pts',(0.00482918550290245,-0.0343648066253259,
0.0789625674348044));
#104475=CARTESIAN_POINT('Ctrl Pts',(0.00514037853410038,-0.0346945769586886,
0.079065341795911));
#104476=CARTESIAN_POINT('Ctrl Pts',(0.00507264263970285,-0.0345846629176052,
0.0790242289855344));
#104477=CARTESIAN_POINT('Ctrl Pts',(0.00500574537188257,-0.0344746925050311,
0.0789817084025101));
#104478=CARTESIAN_POINT('Ctrl Pts',(0.00493977222212403,-0.0343648066253259,
0.0789378348831058));
#104479=CARTESIAN_POINT('Origin',(0.0140217424761463,-0.0345626446730268,
0.06479057851436));
#104480=CARTESIAN_POINT('Ctrl Pts',(0.00513841974862758,-0.0346945769586885,
0.0790658657503114));
#104481=CARTESIAN_POINT('Ctrl Pts',(0.0050354549722837,-0.034527515336289,
0.0790033361386388));
#104482=CARTESIAN_POINT('Ctrl Pts',(0.00493443006270726,-0.0343603235965159,
0.0789375522061625));
#104483=CARTESIAN_POINT('Ctrl Pts',(0.00483564091507221,-0.034193496108874,
0.0788687129533036));
#104484=CARTESIAN_POINT('Ctrl Pts',(0.00521100355815576,-0.0346945769586885,
0.0791078135622406));
#104485=CARTESIAN_POINT('Ctrl Pts',(0.00510716016809604,-0.034527515336289,
0.0790468042475196));
#104486=CARTESIAN_POINT('Ctrl Pts',(0.00500520860560947,-0.0343603235965159,
0.0789825133736288));
#104487=CARTESIAN_POINT('Ctrl Pts',(0.00490544757212831,-0.034193496108874,
0.0789151355659178));
#104488=CARTESIAN_POINT('Ctrl Pts',(0.00528358736768393,-0.0346945769586885,
0.0791497613741698));
#104489=CARTESIAN_POINT('Ctrl Pts',(0.00517886536390838,-0.034527515336289,
0.0790902723564003));
#104490=CARTESIAN_POINT('Ctrl Pts',(0.00507598714851168,-0.0343603235965159,
0.079027474541095));
#104491=CARTESIAN_POINT('Ctrl Pts',(0.00497525422918442,-0.034193496108874,
0.0789615581785319));
#104492=CARTESIAN_POINT('Ctrl Pts',(0.0053561711772121,-0.0346945769586885,
0.079191709186099));
#104493=CARTESIAN_POINT('Ctrl Pts',(0.00525057055972072,-0.034527515336289,
0.0791337404652811));
#104494=CARTESIAN_POINT('Ctrl Pts',(0.00514676569141389,-0.0343603235965159,
0.0790724357085613));
#104495=CARTESIAN_POINT('Ctrl Pts',(0.00504506088624052,-0.034193496108874,
0.0790079807911461));
#104496=CARTESIAN_POINT('Ctrl Pts',(0.00493979880522349,-0.0340223579322365,
0.0789378518926395));
#104497=CARTESIAN_POINT('Ctrl Pts',(0.00487376184038252,-0.0339125849573552,
0.0788939364575437));
#104498=CARTESIAN_POINT('Ctrl Pts',(0.00480868022641328,-0.0338030433565216,
0.078848685069592));
#104499=CARTESIAN_POINT('Ctrl Pts',(0.0047446320618954,-0.033693872113232,
0.0788021629755311));
#104500=CARTESIAN_POINT('Ctrl Pts',(0.00495975722197961,-0.0340223579322365,
0.0790493993777354));
#104501=CARTESIAN_POINT('Ctrl Pts',(0.00489218172639113,-0.0339125849573552,
0.0790057592212603));
#104502=CARTESIAN_POINT('Ctrl Pts',(0.00482555696515432,-0.0338030433565216,
0.0789607510744829));
#104503=CARTESIAN_POINT('Ctrl Pts',(0.00475996303784863,-0.033693872113232,
0.0789144400480211));
#104504=CARTESIAN_POINT('Ctrl Pts',(0.00497971563873574,-0.0340223579322365,
0.0791609468628312));
#104505=CARTESIAN_POINT('Ctrl Pts',(0.00491060161239974,-0.0339125849573552,
0.0791175819849769));
#104506=CARTESIAN_POINT('Ctrl Pts',(0.00484243370389537,-0.0338030433565216,
0.0790728170793739));
#104507=CARTESIAN_POINT('Ctrl Pts',(0.00477529401380186,-0.033693872113232,
0.0790267171205112));
#104508=CARTESIAN_POINT('Ctrl Pts',(0.00499967405549186,-0.0340223579322365,
0.0792724943479271));
#104509=CARTESIAN_POINT('Ctrl Pts',(0.00492902149840835,-0.0339125849573552,
0.0792294047486935));
#104510=CARTESIAN_POINT('Ctrl Pts',(0.00485931044263641,-0.0338030433565216,
0.0791848830842648));
#104511=CARTESIAN_POINT('Ctrl Pts',(0.00479062498975509,-0.033693872113232,
0.0791389941930013));
#104512=CARTESIAN_POINT('Origin',(0.0135419357555965,-0.0345589643414837,
0.0646559610905117));
#104513=CARTESIAN_POINT('Ctrl Pts',(0.00450435085242287,-0.034193496108874,
0.0789353648523489));
#104514=CARTESIAN_POINT('Ctrl Pts',(0.0044383635048895,-0.0340836138581106,
0.078885455037503));
#104515=CARTESIAN_POINT('Ctrl Pts',(0.00437344059821924,-0.0339738896643499,
0.0788342037006276));
#104516=CARTESIAN_POINT('Ctrl Pts',(0.00430966082853527,-0.0338644633294062,
0.0787816820072562));
#104517=CARTESIAN_POINT('Ctrl Pts',(0.00461544364277505,-0.034193496108874,
0.0789130142107752));
#104518=CARTESIAN_POINT('Ctrl Pts',(0.00454976449735345,-0.0340836138581106,
0.0788646362997217));
#104519=CARTESIAN_POINT('Ctrl Pts',(0.00448511794537918,-0.0339738896643499,
0.0788149225091984));
#104520=CARTESIAN_POINT('Ctrl Pts',(0.00442158246119149,-0.0338644633294062,
0.0787639420131593));
#104521=CARTESIAN_POINT('Ctrl Pts',(0.00472653643312723,-0.034193496108874,
0.0788906635692014));
#104522=CARTESIAN_POINT('Ctrl Pts',(0.00466116548981741,-0.0340836138581106,
0.0788438175619403));
#104523=CARTESIAN_POINT('Ctrl Pts',(0.00459679529253913,-0.0339738896643499,
0.0787956413177693));
#104524=CARTESIAN_POINT('Ctrl Pts',(0.0045335040938477,-0.0338644633294062,
0.0787462020190624));
#104525=CARTESIAN_POINT('Ctrl Pts',(0.0048376292234794,-0.034193496108874,
0.0788683129276277));
#104526=CARTESIAN_POINT('Ctrl Pts',(0.00477256648228136,-0.0340836138581106,
0.078822998824159));
#104527=CARTESIAN_POINT('Ctrl Pts',(0.00470847263969908,-0.0339738896643499,
0.0787763601263402));
#104528=CARTESIAN_POINT('Ctrl Pts',(0.00464542572650392,-0.0338644633294062,
0.0787284620249655));
#104529=CARTESIAN_POINT('Origin',(0.013980649207717,-0.0345610621862729,
0.064853649022503));
#104530=CARTESIAN_POINT('Ctrl Pts',(0.00486538773251886,-0.03424362768739,
0.0788893027482109));
#104531=CARTESIAN_POINT('Ctrl Pts',(0.00468664198271262,-0.033943005420186,
0.0787664103752259));
#104532=CARTESIAN_POINT('Ctrl Pts',(0.00451766078791165,-0.0336441434784162,
0.0786304032643261));
#104533=CARTESIAN_POINT('Ctrl Pts',(0.00507442535262118,-0.03424362768739,
0.0790264277764952));
#104534=CARTESIAN_POINT('Ctrl Pts',(0.00489050784711583,-0.033943005420186,
0.0789114193873213));
#104535=CARTESIAN_POINT('Ctrl Pts',(0.00471577573506724,-0.0336441434784162,
0.0787828843048311));
#104536=CARTESIAN_POINT('Ctrl Pts',(0.00464544788448532,-0.0335235895815127,
0.0787284786998444));
#104537=CARTESIAN_POINT('Ctrl Pts',(0.00458241611098779,-0.0334144449262719,
0.0786805925798768));
#104538=CARTESIAN_POINT('Ctrl Pts',(0.00452030121281923,-0.0333049234473133,
0.0786313492555552));
#104539=CARTESIAN_POINT('Ctrl Pts',(0.0044591883196958,-0.0331951640388588,
0.0785808044992326));
#104540=CARTESIAN_POINT('Ctrl Pts',(0.00465836273828975,-0.0335235895815127,
0.0788410592445124));
#104541=CARTESIAN_POINT('Ctrl Pts',(0.00459378107194419,-0.0334144449262719,
0.0787933509229345));
#104542=CARTESIAN_POINT('Ctrl Pts',(0.00453011082710756,-0.0333049234473133,
0.0787442535816515));
#104543=CARTESIAN_POINT('Ctrl Pts',(0.00446743910539777,-0.0331951640388588,
0.078693822626194));
#104544=CARTESIAN_POINT('Ctrl Pts',(0.00467127759209418,-0.0335235895815127,
0.0789536397891805));
#104545=CARTESIAN_POINT('Ctrl Pts',(0.00460514603290059,-0.0334144449262719,
0.0789061092659922));
#104546=CARTESIAN_POINT('Ctrl Pts',(0.00453992044139589,-0.0333049234473133,
0.0788571579077478));
#104547=CARTESIAN_POINT('Ctrl Pts',(0.00447568989109973,-0.0331951640388588,
0.0788068407531553));
#104548=CARTESIAN_POINT('Ctrl Pts',(0.0046841924458986,-0.0335235895815127,
0.0790662203338486));
#104549=CARTESIAN_POINT('Ctrl Pts',(0.00461651099385698,-0.0334144449262719,
0.0790188676090499));
#104550=CARTESIAN_POINT('Ctrl Pts',(0.00454973005568423,-0.0333049234473133,
0.0789700622338442));
#104551=CARTESIAN_POINT('Ctrl Pts',(0.0044839406768017,-0.0331951640388588,
0.0789198588801167));
#104552=CARTESIAN_POINT('Origin',(0.0156570923110334,-0.0326434571772002,
0.066235854630734));
#104553=CARTESIAN_POINT('Ctrl Pts',(0.00420900849951589,-0.0336938721132456,
0.0786989303646591));
#104554=CARTESIAN_POINT('Ctrl Pts',(0.0041823821005945,-0.0336474569764991,
0.0786760158951693));
#104555=CARTESIAN_POINT('Ctrl Pts',(0.00415602576892811,-0.033601104548885,
0.0786527913001756));
#104556=CARTESIAN_POINT('Ctrl Pts',(0.00408929759972816,-0.03348375086432,
0.0785939919678578));
#104557=CARTESIAN_POINT('Ctrl Pts',(0.00402434107867253,-0.0333660264760483,
0.0785332411619524));
#104558=CARTESIAN_POINT('Ctrl Pts',(0.00454583887293969,-0.0336938721132456,
0.0786529375520499));
#104559=CARTESIAN_POINT('Ctrl Pts',(0.00451948168521255,-0.0336474569764991,
0.078631994662508));
#104560=CARTESIAN_POINT('Ctrl Pts',(0.00449337146646129,-0.033601104548885,
0.0786107446638254));
#104561=CARTESIAN_POINT('Ctrl Pts',(0.00442726639855065,-0.03348375086432,
0.0785569445551631));
#104562=CARTESIAN_POINT('Ctrl Pts',(0.00436278456780856,-0.0333660264760482,
0.0785012092414052));
#104563=CARTESIAN_POINT('Ctrl Pts',(0.00454583887294235,-0.0336938721132427,
0.078652937552054));
#104564=CARTESIAN_POINT('Ctrl Pts',(0.00451948168521891,-0.0336474569765026,
0.0786319946625149));
#104565=CARTESIAN_POINT('Ctrl Pts',(0.00449337146647129,-0.0336011045488949,
0.0786107446638354));
#104566=CARTESIAN_POINT('Ctrl Pts',(0.00442781696373628,-0.0334847282606778,
0.0785573926367984));
#104567=CARTESIAN_POINT('Ctrl Pts',(0.00436385854011419,-0.0333679869945434,
0.0785021373052407));
#104568=CARTESIAN_POINT('Ctrl Pts',(0.00454583887293804,-0.0336938721132427,
0.0786529375520486));
#104569=CARTESIAN_POINT('Ctrl Pts',(0.004451573905417,-0.0335278710435084,
0.0785780365109017));
#104570=CARTESIAN_POINT('Ctrl Pts',(0.00435969097726898,-0.033362046922432,
0.0785002056948942));
#104571=CARTESIAN_POINT('Ctrl Pts',(0.00427015733847117,-0.0331951640388602,
0.0784193911134637));
#104572=CARTESIAN_POINT('Ctrl Pts',(0.00461259288962409,-0.0336938721132427,
0.0787036517618872));
#104573=CARTESIAN_POINT('Ctrl Pts',(0.00451726626550933,-0.0335278710435084,
0.0786301481563348));
#104574=CARTESIAN_POINT('Ctrl Pts',(0.00442427823103898,-0.033362046922432,
0.0785536809910323));
#104575=CARTESIAN_POINT('Ctrl Pts',(0.00433359525977046,-0.0331951640388602,
0.0784741967697822));
#104576=CARTESIAN_POINT('Ctrl Pts',(0.00467934690631015,-0.0336938721132427,
0.0787543659717258));
#104577=CARTESIAN_POINT('Ctrl Pts',(0.00458295862560166,-0.0335278710435084,
0.0786822598017678));
#104578=CARTESIAN_POINT('Ctrl Pts',(0.00448886548480899,-0.033362046922432,
0.0786071562871705));
#104579=CARTESIAN_POINT('Ctrl Pts',(0.00439703318106975,-0.0331951640388602,
0.0785290024261008));
#104580=CARTESIAN_POINT('Ctrl Pts',(0.0047461009229962,-0.0336938721132427,
0.0788050801815644));
#104581=CARTESIAN_POINT('Ctrl Pts',(0.00464865098569399,-0.0335278710435084,
0.0787343714472009));
#104582=CARTESIAN_POINT('Ctrl Pts',(0.004553452738579,-0.033362046922432,
0.0786606315833087));
#104583=CARTESIAN_POINT('Ctrl Pts',(0.00446047110236904,-0.0331951640388602,
0.0785838080824193));
#104584=CARTESIAN_POINT('Ctrl Pts',(0.0043648272482345,-0.0330240426238156,
0.0785010387842859));
#104585=CARTESIAN_POINT('Ctrl Pts',(0.00430488744996958,-0.0329142774063509,
0.0784492555177482));
#104586=CARTESIAN_POINT('Ctrl Pts',(0.00424598827429796,-0.0328043479726686,
0.0783962073122998));
#104587=CARTESIAN_POINT('Ctrl Pts',(0.00418820704702087,-0.0326943950436594,
0.0783419600486467));
#104588=CARTESIAN_POINT('Ctrl Pts',(0.0043706476364913,-0.0330240426238156,
0.0786142079455682));
#104589=CARTESIAN_POINT('Ctrl Pts',(0.00430914882277435,-0.0329142774063509,
0.0785625048605493));
#104590=CARTESIAN_POINT('Ctrl Pts',(0.00424868819684867,-0.0328043479726686,
0.0785095046473889));
#104591=CARTESIAN_POINT('Ctrl Pts',(0.00418934508315637,-0.0326943950436594,
0.0784552730702223));
#104592=CARTESIAN_POINT('Ctrl Pts',(0.0043764680247481,-0.0330240426238156,
0.0787273771068507));
#104593=CARTESIAN_POINT('Ctrl Pts',(0.00431341019557912,-0.0329142774063509,
0.0786757542033505));
#104594=CARTESIAN_POINT('Ctrl Pts',(0.00425138811939938,-0.0328043479726686,
0.0786228019824779));
#104595=CARTESIAN_POINT('Ctrl Pts',(0.00419048311929187,-0.0326943950436594,
0.0785685860917978));
#104596=CARTESIAN_POINT('Ctrl Pts',(0.0043822884130049,-0.0330240426238156,
0.078840546268133));
#104597=CARTESIAN_POINT('Ctrl Pts',(0.00431767156838389,-0.0329142774063509,
0.0787890035461516));
#104598=CARTESIAN_POINT('Ctrl Pts',(0.00425408804195009,-0.0328043479726686,
0.0787360993175669));
#104599=CARTESIAN_POINT('Ctrl Pts',(0.00419162115542737,-0.0326943950436594,
0.0786818991133733));
#104600=CARTESIAN_POINT('Origin',(0.0157403386267391,-0.0326396682855912,
0.0661443917975717));
#104601=CARTESIAN_POINT('Ctrl Pts',(0.00393312589888615,-0.0331951640388588,
0.0784439957875769));
#104602=CARTESIAN_POINT('Ctrl Pts',(0.00387398479359502,-0.0330855618255041,
0.0783862779747526));
#104603=CARTESIAN_POINT('Ctrl Pts',(0.00381599398283876,-0.0329757224427708,
0.0783272962084107));
#104604=CARTESIAN_POINT('Ctrl Pts',(0.00375923143222123,-0.0328657862078596,
0.0782671223756007));
#104605=CARTESIAN_POINT('Ctrl Pts',(0.00404614393586861,-0.0331951640388588,
0.0784357450084437));
#104606=CARTESIAN_POINT('Ctrl Pts',(0.00398711646836885,-0.0330855618255041,
0.0783795837904453));
#104607=CARTESIAN_POINT('Ctrl Pts',(0.00392920720516958,-0.0329757224427708,
0.0783221620897555));
#104608=CARTESIAN_POINT('Ctrl Pts',(0.00387249390945392,-0.0328657862078596,
0.0782635498007886));
#104609=CARTESIAN_POINT('Ctrl Pts',(0.00415916197285108,-0.0331951640388588,
0.0784274942293106));
#104610=CARTESIAN_POINT('Ctrl Pts',(0.00410024814314268,-0.0330855618255042,
0.0783728896061379));
#104611=CARTESIAN_POINT('Ctrl Pts',(0.0040424204275004,-0.0329757224427708,
0.0783170279711003));
#104612=CARTESIAN_POINT('Ctrl Pts',(0.00398575638668661,-0.0328657862078596,
0.0782599772259765));
#104613=CARTESIAN_POINT('Ctrl Pts',(0.00427218000983354,-0.0331951640388588,
0.0784192434501774));
#104614=CARTESIAN_POINT('Ctrl Pts',(0.00421337981791651,-0.0330855618255042,
0.0783661954218306));
#104615=CARTESIAN_POINT('Ctrl Pts',(0.00415563364983122,-0.0329757224427708,
0.0783118938524451));
#104616=CARTESIAN_POINT('Ctrl Pts',(0.0040990188639193,-0.0328657862078596,
0.0782564046511645));
#104617=CARTESIAN_POINT('Origin',(0.0160610598854413,-0.032640190883307,
0.0665027362489383));
#104618=CARTESIAN_POINT('Ctrl Pts',(0.00429703490787385,-0.0332451089994433,
0.0784434985984568));
#104619=CARTESIAN_POINT('Ctrl Pts',(0.00413510295888785,-0.0329451141710258,
0.0782991704632625));
#104620=CARTESIAN_POINT('Ctrl Pts',(0.00398450242663942,-0.0326442513127502,
0.0781430549726871));
#104621=CARTESIAN_POINT('Ctrl Pts',(0.00448723583637103,-0.0332451089994433,
0.0786057441124127));
#104622=CARTESIAN_POINT('Ctrl Pts',(0.004319184697711,-0.0329451141710258,
0.078468589522602));
#104623=CARTESIAN_POINT('Ctrl Pts',(0.00416194201899661,-0.0326442513127502,
0.0783191662757433));
#104624=CARTESIAN_POINT('Ctrl Pts',(0.00409904136003693,-0.0325229783203385,
0.0782564268255897));
#104625=CARTESIAN_POINT('Ctrl Pts',(0.00404243435707815,-0.032413025311208,
0.0782009458622309));
#104626=CARTESIAN_POINT('Ctrl Pts',(0.00398698363465686,-0.0323031222247695,
0.0781443023250954));
#104627=CARTESIAN_POINT('Ctrl Pts',(0.0039327576609294,-0.0321934096636184,
0.0780865712768841));
#104628=CARTESIAN_POINT('Ctrl Pts',(0.00409774433046492,-0.0325229783203385,
0.0783697381681987));
#104629=CARTESIAN_POINT('Ctrl Pts',(0.00403957533315467,-0.032413025311208,
0.078314239325316));
#104630=CARTESIAN_POINT('Ctrl Pts',(0.00398256322314985,-0.0323031222247695,
0.0782575455995092));
#104631=CARTESIAN_POINT('Ctrl Pts',(0.00392677846636474,-0.0321934096636184,
0.0781997321883418));
#104632=CARTESIAN_POINT('Ctrl Pts',(0.00409644730089292,-0.0325229783203385,
0.0784830495108077));
#104633=CARTESIAN_POINT('Ctrl Pts',(0.00403671630923118,-0.032413025311208,
0.078427532788401));
#104634=CARTESIAN_POINT('Ctrl Pts',(0.00397814281164285,-0.0323031222247695,
0.078370788873923));
#104635=CARTESIAN_POINT('Ctrl Pts',(0.00392079927180007,-0.0321934096636184,
0.0783128930997994));
#104636=CARTESIAN_POINT('Ctrl Pts',(0.00409515027132091,-0.0325229783203385,
0.0785963608534167));
#104637=CARTESIAN_POINT('Ctrl Pts',(0.0040338572853077,-0.032413025311208,
0.078540826251486));
#104638=CARTESIAN_POINT('Ctrl Pts',(0.00397372240013584,-0.0323031222247695,
0.0784840321483367));
#104639=CARTESIAN_POINT('Ctrl Pts',(0.0039148200772354,-0.0321934096636184,
0.0784260540112571));
#104640=CARTESIAN_POINT('Origin',(0.0157342914279694,-0.0326393375177525,
0.0661504019901444));
#104641=CARTESIAN_POINT('Ctrl Pts',(0.00367177297545991,-0.0326943950436594,
0.0781723890818772));
#104642=CARTESIAN_POINT('Ctrl Pts',(0.00361633691515119,-0.0325844576448127,
0.0781110320509036));
#104643=CARTESIAN_POINT('Ctrl Pts',(0.00356216589554312,-0.0324744968375319,
0.0780485241689818));
#104644=CARTESIAN_POINT('Ctrl Pts',(0.00350932821904061,-0.0323646534831894,
0.0779849464821874));
#104645=CARTESIAN_POINT('Ctrl Pts',(0.00378508595995979,-0.0326943950436594,
0.078171251046114));
#104646=CARTESIAN_POINT('Ctrl Pts',(0.0037296655839168,-0.0325844576448127,
0.078111455680438));
#104647=CARTESIAN_POINT('Ctrl Pts',(0.00367547795188571,-0.0324744968375319,
0.0780505098987116));
#104648=CARTESIAN_POINT('Ctrl Pts',(0.00362259141516232,-0.0323646534831894,
0.0779884927458501));
#104649=CARTESIAN_POINT('Ctrl Pts',(0.00389839894445967,-0.0326943950436594,
0.0781701130103508));
#104650=CARTESIAN_POINT('Ctrl Pts',(0.0038429942526824,-0.0325844576448127,
0.0781118793099724));
#104651=CARTESIAN_POINT('Ctrl Pts',(0.0037887900082283,-0.0324744968375319,
0.0780524956284414));
#104652=CARTESIAN_POINT('Ctrl Pts',(0.00373585461128402,-0.0323646534831894,
0.0779920390095128));
#104653=CARTESIAN_POINT('Ctrl Pts',(0.00401171192895955,-0.0326943950436594,
0.0781689749745877));
#104654=CARTESIAN_POINT('Ctrl Pts',(0.00395632292144801,-0.0325844576448127,
0.0781123029395069));
#104655=CARTESIAN_POINT('Ctrl Pts',(0.00390210206457089,-0.0324744968375319,
0.0780544813581712));
#104656=CARTESIAN_POINT('Ctrl Pts',(0.00384911780740573,-0.0323646534831894,
0.0779955852731756));
#104657=CARTESIAN_POINT('Origin',(0.0160879912199795,-0.032639557906681,
0.0664761530758608));
#104658=CARTESIAN_POINT('Ctrl Pts',(0.00403502269649379,-0.0327445246961875,
0.0781947707943522));
#104659=CARTESIAN_POINT('Ctrl Pts',(0.00388247167370257,-0.0324436878365474,
0.0780405607105505));
#104660=CARTESIAN_POINT('Ctrl Pts',(0.00374196976590213,-0.0321434074463187,
0.0778752979548999));
#104661=CARTESIAN_POINT('Ctrl Pts',(0.00421466201254181,-0.0327445246961875,
0.0783686377438561));
#104662=CARTESIAN_POINT('Ctrl Pts',(0.00405555349061777,-0.0324436878365474,
0.0782212028675482));
#104663=CARTESIAN_POINT('Ctrl Pts',(0.00390800237653284,-0.0321434074463187,
0.0780622021341126));
#104664=CARTESIAN_POINT('Ctrl Pts',(0.00378544379441447,-0.0322357242816073,
0.0779258369851489));
#104665=CARTESIAN_POINT('Ctrl Pts',(0.00366518828351864,-0.0319819883628706,
0.0777876665337693));
#104666=CARTESIAN_POINT('Ctrl Pts',(0.00355396866642955,-0.0317295851069886,
0.0776421238997756));
#104667=CARTESIAN_POINT('Ctrl Pts',(0.00395363164487792,-0.0322357242816073,
0.078110804136169));
#104668=CARTESIAN_POINT('Ctrl Pts',(0.0038274851701157,-0.0319819883628706,
0.077977990249695));
#104669=CARTESIAN_POINT('Ctrl Pts',(0.00371004567438076,-0.0317295851069886,
0.07783741846598));
#104670=CARTESIAN_POINT('Origin',(0.0160181918719063,-0.0326371942646663,
0.0665410410921116));
#104671=CARTESIAN_POINT('Origin',(0.015647607112183,-0.0326352985530941,
0.0662372906110294));
#104672=CARTESIAN_POINT('Ctrl Pts',(0.00342799009848551,-0.0321934096636183,
0.0778849078441259));
#104673=CARTESIAN_POINT('Ctrl Pts',(0.00337648280850493,-0.0320835708272304,
0.0778201492114634));
#104674=CARTESIAN_POINT('Ctrl Pts',(0.00332634557138288,-0.0319739230346346,
0.0777543622007505));
#104675=CARTESIAN_POINT('Ctrl Pts',(0.00327763607442989,-0.0318646057455576,
0.0776876359050153));
#104676=CARTESIAN_POINT('Ctrl Pts',(0.00354115110738701,-0.0321934096636183,
0.0778908870438393));
#104677=CARTESIAN_POINT('Ctrl Pts',(0.00348956135958248,-0.0320835708272304,
0.0778276889896818));
#104678=CARTESIAN_POINT('Ctrl Pts',(0.00343930941637432,-0.0319739230346346,
0.0777634599458147));
#104679=CARTESIAN_POINT('Ctrl Pts',(0.00339045326481254,-0.0318646057455576,
0.0776982870232187));
#104680=CARTESIAN_POINT('Ctrl Pts',(0.00365431211628852,-0.0321934096636183,
0.0778968662435527));
#104681=CARTESIAN_POINT('Ctrl Pts',(0.00360263991066004,-0.0320835708272304,
0.0778352287679003));
#104682=CARTESIAN_POINT('Ctrl Pts',(0.00355227326136576,-0.0319739230346346,
0.0777725576908789));
#104683=CARTESIAN_POINT('Ctrl Pts',(0.0035032704551952,-0.0318646057455576,
0.0777089381414222));
#104684=CARTESIAN_POINT('Ctrl Pts',(0.00376747312519003,-0.0321934096636183,
0.0779028454432661));
#104685=CARTESIAN_POINT('Ctrl Pts',(0.00371571846173759,-0.0320835708272304,
0.0778427685461188));
#104686=CARTESIAN_POINT('Ctrl Pts',(0.0036652371063572,-0.0319739230346346,
0.0777816554359431));
#104687=CARTESIAN_POINT('Ctrl Pts',(0.00361608764557785,-0.0318646057455576,
0.0777195892596256));
#104688=CARTESIAN_POINT('Ctrl Pts',(0.00384881685085818,-0.0320218834582387,
0.0779964878945564));
#104689=CARTESIAN_POINT('Ctrl Pts',(0.00380878421069954,-0.0319391099350659,
0.0779519958400047));
#104690=CARTESIAN_POINT('Ctrl Pts',(0.00376947057497083,-0.0318564869454916,
0.0779069056267691));
#104691=CARTESIAN_POINT('Ctrl Pts',(0.00373090151239011,-0.0317740741446485,
0.0778612527703433));
#104692=CARTESIAN_POINT('Ctrl Pts',(0.00384513550296807,-0.0320218834582387,
0.0780459173971374));
#104693=CARTESIAN_POINT('Ctrl Pts',(0.0038045884211826,-0.0319391099350659,
0.0780013870286538));
#104694=CARTESIAN_POINT('Ctrl Pts',(0.00376476125379159,-0.0318564869454916,
0.0779562504916215));
#104695=CARTESIAN_POINT('Ctrl Pts',(0.00372567994040288,-0.0317740741446485,
0.0779105433701943));
#104696=CARTESIAN_POINT('Ctrl Pts',(0.00384145415507796,-0.0320218834582387,
0.0780953468997184));
#104697=CARTESIAN_POINT('Ctrl Pts',(0.00380039263166567,-0.0319391099350659,
0.0780507782173028));
#104698=CARTESIAN_POINT('Ctrl Pts',(0.00376005193261236,-0.0318564869454916,
0.078005595356474));
#104699=CARTESIAN_POINT('Ctrl Pts',(0.00372045836841565,-0.0317740741446485,
0.0779598339700454));
#104700=CARTESIAN_POINT('Ctrl Pts',(0.00383777280718785,-0.0320218834582387,
0.0781447764022994));
#104701=CARTESIAN_POINT('Ctrl Pts',(0.00379619684214873,-0.0319391099350659,
0.0781001694059519));
#104702=CARTESIAN_POINT('Ctrl Pts',(0.00375534261143313,-0.0318564869454916,
0.0780549402213264));
#104703=CARTESIAN_POINT('Ctrl Pts',(0.00371523679642842,-0.0317740741446485,
0.0780091245698964));
#104704=CARTESIAN_POINT('Origin',(-0.00019750424675882,-0.0391228853390767,
0.0829042452738927));
#104705=CARTESIAN_POINT('Ctrl Pts',(0.00640200741755438,-0.0352722978779667,
0.0796381377683931));
#104706=CARTESIAN_POINT('Ctrl Pts',(0.00638408492046634,-0.0352466642097265,
0.0796321480458426));
#104707=CARTESIAN_POINT('Ctrl Pts',(0.00636615353960843,-0.0352210183808325,
0.079626238017773));
#104708=CARTESIAN_POINT('Ctrl Pts',(0.00634821247550811,-0.0351953608940152,
0.0796204079813843));
#104709=CARTESIAN_POINT('Origin',(0.00467811982047751,-0.0352456003065129,
0.0842248527964227));
#104710=CARTESIAN_POINT('Ctrl Pts',(0.00623051831428444,-0.035024121149334,
0.0795792570417599));
#104711=CARTESIAN_POINT('Ctrl Pts',(0.00615573252798837,-0.0349144232867421,
0.0795531781092734));
#104712=CARTESIAN_POINT('Ctrl Pts',(0.00608144104894163,-0.0348045283677512,
0.0795255376917175));
#104713=CARTESIAN_POINT('Ctrl Pts',(0.00600774035254011,-0.0346945769586886,
0.0794963676519038));
#104714=CARTESIAN_POINT('Ctrl Pts',(0.00627759032942455,-0.035024121149334,
0.0796823364635382));
#104715=CARTESIAN_POINT('Ctrl Pts',(0.00620138466642172,-0.0349144232867421,
0.0796569059287308));
#104716=CARTESIAN_POINT('Ctrl Pts',(0.00612565905796086,-0.0348045283677512,
0.0796298849470864));
#104717=CARTESIAN_POINT('Ctrl Pts',(0.0060505117868503,-0.0346945769586886,
0.0796013045196413));
#104718=CARTESIAN_POINT('Ctrl Pts',(0.00632466234456467,-0.035024121149334,
0.0797854158853166));
#104719=CARTESIAN_POINT('Ctrl Pts',(0.00624703680485506,-0.0349144232867421,
0.0797606337481882));
#104720=CARTESIAN_POINT('Ctrl Pts',(0.00616987706698009,-0.0348045283677512,
0.0797342322024552));
#104721=CARTESIAN_POINT('Ctrl Pts',(0.0060932832211605,-0.0346945769586886,
0.0797062413873788));
#104722=CARTESIAN_POINT('Ctrl Pts',(0.00637173435970478,-0.035024121149334,
0.0798884953070949));
#104723=CARTESIAN_POINT('Ctrl Pts',(0.00629268894328841,-0.0349144232867421,
0.0798643615676456));
#104724=CARTESIAN_POINT('Ctrl Pts',(0.00621409507599933,-0.0348045283677512,
0.0798385794578241));
#104725=CARTESIAN_POINT('Ctrl Pts',(0.00613605465547069,-0.0346945769586886,
0.0798111782551163));
#104726=CARTESIAN_POINT('Origin',(0.0123533304663821,-0.0345629067941944,
0.0639529949421231));
#104727=CARTESIAN_POINT('Ctrl Pts',(0.00589298787791728,-0.0351970973651596,
0.0796453688229808));
#104728=CARTESIAN_POINT('Ctrl Pts',(0.00581685699041973,-0.0350869349321778,
0.079614464191006));
#104729=CARTESIAN_POINT('Ctrl Pts',(0.00574130552715329,-0.0349764985129753,
0.0795819512390321));
#104730=CARTESIAN_POINT('Ctrl Pts',(0.00566643384677454,-0.0348659306849698,
0.0795478663268045));
#104731=CARTESIAN_POINT('Ctrl Pts',(0.00596702049102428,-0.0351970973651596,
0.0796095967270538));
#104732=CARTESIAN_POINT('Ctrl Pts',(0.00589138517743602,-0.0350869349321778,
0.0795797177166016));
#104733=CARTESIAN_POINT('Ctrl Pts',(0.00581630837650343,-0.0349764985129753,
0.0795482415384702));
#104734=CARTESIAN_POINT('Ctrl Pts',(0.00574188975287722,-0.0348659306849698,
0.0795152032454328));
#104735=CARTESIAN_POINT('Ctrl Pts',(0.00604105310413129,-0.0351970973651596,
0.0795738246311267));
#104736=CARTESIAN_POINT('Ctrl Pts',(0.0059659133644523,-0.0350869349321778,
0.0795449712421971));
#104737=CARTESIAN_POINT('Ctrl Pts',(0.00589131122585358,-0.0349764985129753,
0.0795145318379082));
#104738=CARTESIAN_POINT('Ctrl Pts',(0.0058173456589799,-0.0348659306849698,
0.0794825401640612));
#104739=CARTESIAN_POINT('Ctrl Pts',(0.00611508571723829,-0.0351970973651596,
0.0795380525351997));
#104740=CARTESIAN_POINT('Ctrl Pts',(0.00604044155146859,-0.0350869349321778,
0.0795102247677927));
#104741=CARTESIAN_POINT('Ctrl Pts',(0.00596631407520372,-0.0349764985129753,
0.0794808221373463));
#104742=CARTESIAN_POINT('Ctrl Pts',(0.00589280156508258,-0.0348659306849698,
0.0794498770826896));
#104743=CARTESIAN_POINT('Origin',(0.0127781825806878,-0.0345637187966566,
0.0641784412489904));
#104744=CARTESIAN_POINT('Ctrl Pts',(0.00614629913616949,-0.0352450361861252,
0.0795507115975138));
#104745=CARTESIAN_POINT('Ctrl Pts',(0.00594260796109335,-0.0349452761023764,
0.0794761296021067));
#104746=CARTESIAN_POINT('Ctrl Pts',(0.00574511327208869,-0.0346444289983475,
0.0793864166339374));
#104747=CARTESIAN_POINT('Ctrl Pts',(0.00638286995954464,-0.0352450361861252,
0.079631546277742));
#104748=CARTESIAN_POINT('Ctrl Pts',(0.00617613005455479,-0.0349452761023764,
0.079565886697119));
#104749=CARTESIAN_POINT('Ctrl Pts',(0.0059749232239849,-0.0346444289983475,
0.0794848411532883));
#104750=CARTESIAN_POINT('Ctrl Pts',(0.00589334924320917,-0.0345231616327822,
0.0794496650478157));
#104751=CARTESIAN_POINT('Ctrl Pts',(0.00582030082185705,-0.0344132092796975,
0.0794189216698));
#104752=CARTESIAN_POINT('Ctrl Pts',(0.0057478920719919,-0.0343032738558974,
0.0793866689290254));
#104753=CARTESIAN_POINT('Ctrl Pts',(0.00567621469917636,-0.0341934961088741,
0.0793529505211642));
#104754=CARTESIAN_POINT('Ctrl Pts',(0.00593385597004646,-0.0345231616327822,
0.0795554967123585));
#104755=CARTESIAN_POINT('Ctrl Pts',(0.0058593488081977,-0.0344132092796975,
0.0795253116625433));
#104756=CARTESIAN_POINT('Ctrl Pts',(0.00578546984452178,-0.0343032738558974,
0.0794935870482655));
#104757=CARTESIAN_POINT('Ctrl Pts',(0.00571231268542628,-0.0341934961088741,
0.0794603659368534));
#104758=CARTESIAN_POINT('Ctrl Pts',(0.00597436269688375,-0.0345231616327822,
0.0796613283769013));
#104759=CARTESIAN_POINT('Ctrl Pts',(0.00589839679453834,-0.0344132092796975,
0.0796317016552866));
#104760=CARTESIAN_POINT('Ctrl Pts',(0.00582304761705166,-0.0343032738558974,
0.0796005051675057));
#104761=CARTESIAN_POINT('Ctrl Pts',(0.0057484106716762,-0.0341934961088741,
0.0795677813525425));
#104762=CARTESIAN_POINT('Ctrl Pts',(0.00601486942372104,-0.0345231616327822,
0.0797671600414441));
#104763=CARTESIAN_POINT('Ctrl Pts',(0.00593744478087899,-0.0344132092796975,
0.07973809164803));
#104764=CARTESIAN_POINT('Ctrl Pts',(0.00586062538958153,-0.0343032738558974,
0.0797074232867459));
#104765=CARTESIAN_POINT('Ctrl Pts',(0.00578450865792613,-0.0341934961088741,
0.0796751967682317));
#104766=CARTESIAN_POINT('Origin',(0.0123577353792793,-0.0345625596231457,
0.0639417212994246));
#104767=CARTESIAN_POINT('Ctrl Pts',(0.00546514888907037,-0.0346945769586886,
0.079528816687218));
#104768=CARTESIAN_POINT('Ctrl Pts',(0.00539102607640815,-0.0345846629176052,
0.0794921793764874));
#104769=CARTESIAN_POINT('Ctrl Pts',(0.00531764824792714,-0.0344746925050311,
0.0794540029786887));
#104770=CARTESIAN_POINT('Ctrl Pts',(0.00524510922174087,-0.0343648066253259,
0.0794143367981118));
#104771=CARTESIAN_POINT('Ctrl Pts',(0.0055700856741824,-0.0346945769586886,
0.0794860452865853));
#104772=CARTESIAN_POINT('Ctrl Pts',(0.00549655227303962,-0.0345846629176052,
0.0794508540577936));
#104773=CARTESIAN_POINT('Ctrl Pts',(0.00542373405237037,-0.0344746925050311,
0.0794141361777164));
#104774=CARTESIAN_POINT('Ctrl Pts',(0.0053517241209721,-0.0343648066253259,
0.0793759390788612));
#104775=CARTESIAN_POINT('Ctrl Pts',(0.00567502245929443,-0.0346945769586886,
0.0794432738859526));
#104776=CARTESIAN_POINT('Ctrl Pts',(0.00560207846967109,-0.0345846629176052,
0.0794095287390998));
#104777=CARTESIAN_POINT('Ctrl Pts',(0.00552981985681359,-0.0344746925050311,
0.079374269376744));
#104778=CARTESIAN_POINT('Ctrl Pts',(0.00545833902020333,-0.0343648066253259,
0.0793375413596106));
#104779=CARTESIAN_POINT('Ctrl Pts',(0.00577995924440646,-0.0346945769586886,
0.0794005024853199));
#104780=CARTESIAN_POINT('Ctrl Pts',(0.00570760466630256,-0.0345846629176052,
0.0793682034204061));
#104781=CARTESIAN_POINT('Ctrl Pts',(0.00563590566125681,-0.0344746925050311,
0.0793344025757717));
#104782=CARTESIAN_POINT('Ctrl Pts',(0.00556495391943456,-0.0343648066253259,
0.07929914364036));
#104783=CARTESIAN_POINT('Origin',(0.0128021887384452,-0.0345626446730568,
0.0641251699148011));
#104784=CARTESIAN_POINT('Ctrl Pts',(0.00577808157344143,-0.0346945769586885,
0.0794012678091005));
#104785=CARTESIAN_POINT('Ctrl Pts',(0.00566809166668867,-0.0345275153362891,
0.0793521361704551));
#104786=CARTESIAN_POINT('Ctrl Pts',(0.00555961845572507,-0.0343603235965159,
0.0792995327425228));
#104787=CARTESIAN_POINT('Ctrl Pts',(0.00545298044386904,-0.034193496108874,
0.0792436178710481));
#104788=CARTESIAN_POINT('Ctrl Pts',(0.00585535049286178,-0.0346945769586885,
0.0794337876864509));
#104789=CARTESIAN_POINT('Ctrl Pts',(0.00574467944425767,-0.0345275153362891,
0.0793862744762595));
#104790=CARTESIAN_POINT('Ctrl Pts',(0.00563547401717934,-0.0343603235965159,
0.0793352684741054));
#104791=CARTESIAN_POINT('Ctrl Pts',(0.00552805495073345,-0.034193496108874,
0.0792809253334429));
#104792=CARTESIAN_POINT('Ctrl Pts',(0.00593261941228212,-0.0346945769586885,
0.0794663075638013));
#104793=CARTESIAN_POINT('Ctrl Pts',(0.00582126722182666,-0.0345275153362891,
0.0794204127820639));
#104794=CARTESIAN_POINT('Ctrl Pts',(0.00571132957863361,-0.0343603235965159,
0.079371004205688));
#104795=CARTESIAN_POINT('Ctrl Pts',(0.00560312945759786,-0.034193496108874,
0.0793182327958377));
#104796=CARTESIAN_POINT('Ctrl Pts',(0.00600988833170246,-0.0346945769586885,
0.0794988274411517));
#104797=CARTESIAN_POINT('Ctrl Pts',(0.00589785499939566,-0.0345275153362891,
0.0794545510878683));
#104798=CARTESIAN_POINT('Ctrl Pts',(0.00578718514008788,-0.0343603235965159,
0.0794067399372707));
#104799=CARTESIAN_POINT('Ctrl Pts',(0.00567820396446227,-0.034193496108874,
0.0793555402582325));
#104800=CARTESIAN_POINT('Ctrl Pts',(0.0055649824247782,-0.0340223579322365,
0.0792991571840227));
#104801=CARTESIAN_POINT('Ctrl Pts',(0.00549396211764549,-0.0339125849573554,
0.0792638646615878));
#104802=CARTESIAN_POINT('Ctrl Pts',(0.00542372218886624,-0.0338030433565221,
0.0792271269834706));
#104803=CARTESIAN_POINT('Ctrl Pts',(0.00535434829877516,-0.0336938721132328,
0.0791889990935798));
#104804=CARTESIAN_POINT('Ctrl Pts',(0.00559876407046006,-0.0340223579322365,
0.0794073236309725));
#104805=CARTESIAN_POINT('Ctrl Pts',(0.005526251865914,-0.0339125849573554,
0.0793724970455378));
#104806=CARTESIAN_POINT('Ctrl Pts',(0.00545451144424721,-0.0338030433565221,
0.0793361940982024));
#104807=CARTESIAN_POINT('Ctrl Pts',(0.00538363043395429,-0.0336938721132328,
0.0792984693470282));
#104808=CARTESIAN_POINT('Ctrl Pts',(0.00563254571614192,-0.0340223579322365,
0.0795154900779222));
#104809=CARTESIAN_POINT('Ctrl Pts',(0.0055585416141825,-0.0339125849573554,
0.0794811294294877));
#104810=CARTESIAN_POINT('Ctrl Pts',(0.00548530069962818,-0.0338030433565221,
0.0794452612129342));
#104811=CARTESIAN_POINT('Ctrl Pts',(0.00541291256913342,-0.0336938721132328,
0.0794079396004766));
#104812=CARTESIAN_POINT('Ctrl Pts',(0.00566632736182378,-0.0340223579322365,
0.079623656524872));
#104813=CARTESIAN_POINT('Ctrl Pts',(0.00559083136245101,-0.0339125849573554,
0.0795897618134376));
#104814=CARTESIAN_POINT('Ctrl Pts',(0.00551608995500914,-0.0338030433565221,
0.079554328327666));
#104815=CARTESIAN_POINT('Ctrl Pts',(0.00544219470431255,-0.0336938721132328,
0.079517409853925));
#104816=CARTESIAN_POINT('Origin',(0.0123092934001533,-0.0345589643415753,
0.0640517497171613));
#104817=CARTESIAN_POINT('Ctrl Pts',(0.00513265640034567,-0.034193496108874,
0.079351265854761));
#104818=CARTESIAN_POINT('Ctrl Pts',(0.00506093402518955,-0.0340836138595105,
0.0793100200018787));
#104819=CARTESIAN_POINT('Ctrl Pts',(0.0049900995601459,-0.0339738896671456,
0.0792673097954907));
#104820=CARTESIAN_POINT('Ctrl Pts',(0.00492024000019863,-0.0338644633335883,
0.0792231959767272));
#104821=CARTESIAN_POINT('Ctrl Pts',(0.00524007191268345,-0.034193496108874,
0.0793151678360314));
#104822=CARTESIAN_POINT('Ctrl Pts',(0.00516884730782287,-0.0340836138595105,
0.0792754031794364));
#104823=CARTESIAN_POINT('Ctrl Pts',(0.00509847972398642,-0.0339738896671456,
0.0792341837589416));
#104824=CARTESIAN_POINT('Ctrl Pts',(0.00502905568651178,-0.0338644633335883,
0.0791915683675986));
#104825=CARTESIAN_POINT('Ctrl Pts',(0.00534748742502123,-0.034193496108874,
0.0792790698173018));
#104826=CARTESIAN_POINT('Ctrl Pts',(0.00527676059045619,-0.0340836138595105,
0.0792407863569941));
#104827=CARTESIAN_POINT('Ctrl Pts',(0.00520685988782694,-0.0339738896671456,
0.0792010577223924));
#104828=CARTESIAN_POINT('Ctrl Pts',(0.00513787137282492,-0.0338644633335883,
0.07915994075847));
#104829=CARTESIAN_POINT('Ctrl Pts',(0.00545490293735901,-0.034193496108874,
0.0792429717985722));
#104830=CARTESIAN_POINT('Ctrl Pts',(0.00538467387308951,-0.0340836138595105,
0.0792061695345518));
#104831=CARTESIAN_POINT('Ctrl Pts',(0.00531524005166745,-0.0339738896671456,
0.0791679316858433));
#104832=CARTESIAN_POINT('Ctrl Pts',(0.00524668705913807,-0.0338644633335883,
0.0791283131493414));
#104833=CARTESIAN_POINT('Origin',(0.0127693243339131,-0.0345610621862859,
0.0641928934445164));
#104834=CARTESIAN_POINT('Ctrl Pts',(0.00548507328434942,-0.0342436276873901,
0.079260317044454));
#104835=CARTESIAN_POINT('Ctrl Pts',(0.00529233449968253,-0.0339430054201861,
0.0791607964973451));
#104836=CARTESIAN_POINT('Ctrl Pts',(0.00510763956107794,-0.0336441434784162,
0.079047040802694));
#104837=CARTESIAN_POINT('Ctrl Pts',(0.00570964890357818,-0.0342436276873901,
0.0793701614400689));
#104838=CARTESIAN_POINT('Ctrl Pts',(0.00551276726923501,-0.0339430054201861,
0.079279110902069));
#104839=CARTESIAN_POINT('Ctrl Pts',(0.0053233032545649,-0.0336441434784162,
0.0791734890977064));
#104840=CARTESIAN_POINT('Ctrl Pts',(0.00524671112969369,-0.0335235895815127,
0.0791283269140882));
#104841=CARTESIAN_POINT('Ctrl Pts',(0.00517817465829848,-0.0334144449262719,
0.0790887183664692));
#104842=CARTESIAN_POINT('Ctrl Pts',(0.00511037772958611,-0.0333049234473133,
0.0790476484015081));
#104843=CARTESIAN_POINT('Ctrl Pts',(0.00504341179212886,-0.0331951640388588,
0.0790051616821937));
#104844=CARTESIAN_POINT('Ctrl Pts',(0.00527363422971817,-0.0335235895815127,
0.0792384010671475));
#104845=CARTESIAN_POINT('Ctrl Pts',(0.00520358237089006,-0.0334144449262719,
0.079199163169007));
#104846=CARTESIAN_POINT('Ctrl Pts',(0.00513426065640893,-0.0333049234473133,
0.0791584329725919));
#104847=CARTESIAN_POINT('Ctrl Pts',(0.00506576244522471,-0.0331951640388588,
0.0791162545298161));
#104848=CARTESIAN_POINT('Ctrl Pts',(0.00530055732974265,-0.0335235895815127,
0.0793484752202068));
#104849=CARTESIAN_POINT('Ctrl Pts',(0.00522899008348163,-0.0334144449262719,
0.0793096079715449));
#104850=CARTESIAN_POINT('Ctrl Pts',(0.00515814358323175,-0.0333049234473133,
0.0792692175436757));
#104851=CARTESIAN_POINT('Ctrl Pts',(0.00508811309832056,-0.0331951640388588,
0.0792273473774384));
#104852=CARTESIAN_POINT('Ctrl Pts',(0.00532748042976713,-0.0335235895815127,
0.0794585493732661));
#104853=CARTESIAN_POINT('Ctrl Pts',(0.0052543977960732,-0.0334144449262719,
0.0794200527740827));
#104854=CARTESIAN_POINT('Ctrl Pts',(0.00518202651005457,-0.0333049234473133,
0.0793800021147596));
#104855=CARTESIAN_POINT('Ctrl Pts',(0.00511046375141641,-0.0331951640388588,
0.0793384402250607));
#104856=CARTESIAN_POINT('Origin',(0.0146057844810557,-0.0326434571769772,
0.0653540859141867));
#104857=CARTESIAN_POINT('Ctrl Pts',(0.00481000981123756,-0.0336938721132456,
0.0791537119357245));
#104858=CARTESIAN_POINT('Ctrl Pts',(0.004780721424868,-0.0336474569764991,
0.0791343153263458));
#104859=CARTESIAN_POINT('Ctrl Pts',(0.00475166210716029,-0.033601104548885,
0.0791145771884932));
#104860=CARTESIAN_POINT('Ctrl Pts',(0.00467809059905453,-0.0334837508643202,
0.0790646047636889));
#104861=CARTESIAN_POINT('Ctrl Pts',(0.00460603218462337,-0.0333660264760487,
0.0790124742068587));
#104862=CARTESIAN_POINT('Ctrl Pts',(0.00513841974863563,-0.0336938721132456,
0.0790658657503163));
#104863=CARTESIAN_POINT('Ctrl Pts',(0.00510964555513977,-0.0336474569764991,
0.0790483914332793));
#104864=CARTESIAN_POINT('Ctrl Pts',(0.00508107789221398,-0.033601104548885,
0.0790305814753285));
#104865=CARTESIAN_POINT('Ctrl Pts',(0.00500875114092382,-0.0334837508643202,
0.0789854907585086));
#104866=CARTESIAN_POINT('Ctrl Pts',(0.00493779228158005,-0.0333660264760487,
0.0789382766507001));
#104867=CARTESIAN_POINT('Ctrl Pts',(0.00513841974863763,-0.0336938721132427,
0.0790658657503215));
#104868=CARTESIAN_POINT('Ctrl Pts',(0.00510964555514579,-0.0336474569765026,
0.0790483914332867));
#104869=CARTESIAN_POINT('Ctrl Pts',(0.00508107789222398,-0.0336011045488949,
0.0790305814753385));
#104870=CARTESIAN_POINT('Ctrl Pts',(0.00500935352425746,-0.0334847282606778,
0.0789858663027726));
#104871=CARTESIAN_POINT('Ctrl Pts',(0.00493897410253327,-0.0333679869945434,
0.0789390627920544));
#104872=CARTESIAN_POINT('Ctrl Pts',(0.00513841974863386,-0.0336938721132428,
0.0790658657503152));
#104873=CARTESIAN_POINT('Ctrl Pts',(0.00503551049885303,-0.0335278710435084,
0.0790033698594408));
#104874=CARTESIAN_POINT('Ctrl Pts',(0.00493459730719635,-0.033362046922432,
0.0789376687471586));
#104875=CARTESIAN_POINT('Ctrl Pts',(0.00483564091507303,-0.0331951640388601,
0.0788687129533042));
#104876=CARTESIAN_POINT('Ctrl Pts',(0.0052110035658666,-0.0336938721132428,
0.079107813566697));
#104877=CARTESIAN_POINT('Ctrl Pts',(0.00510721617609314,-0.0335278710435084,
0.0790468371530738));
#104878=CARTESIAN_POINT('Ctrl Pts',(0.00500537750295989,-0.033362046922432,
0.0789826274452524));
#104879=CARTESIAN_POINT('Ctrl Pts',(0.00490544757953888,-0.0331951640388601,
0.078915135570846));
#104880=CARTESIAN_POINT('Ctrl Pts',(0.00528358738309935,-0.0336938721132428,
0.0791497613830787));
#104881=CARTESIAN_POINT('Ctrl Pts',(0.00517892185333324,-0.0335278710435084,
0.0790903044467068));
#104882=CARTESIAN_POINT('Ctrl Pts',(0.00507615769872343,-0.033362046922432,
0.0790275861433462));
#104883=CARTESIAN_POINT('Ctrl Pts',(0.00497525424400473,-0.0331951640388601,
0.0789615581883877));
#104884=CARTESIAN_POINT('Ctrl Pts',(0.0053561712003321,-0.0336938721132428,
0.0791917091994605));
#104885=CARTESIAN_POINT('Ctrl Pts',(0.00525062753057335,-0.0335278710435084,
0.0791337717403398));
#104886=CARTESIAN_POINT('Ctrl Pts',(0.00514693789448697,-0.033362046922432,
0.07907254484144));
#104887=CARTESIAN_POINT('Ctrl Pts',(0.00504506090847058,-0.0331951640388601,
0.0790079808059295));
#104888=CARTESIAN_POINT('Ctrl Pts',(0.00493979749091848,-0.0330240426238156,
0.0789378515219431));
#104889=CARTESIAN_POINT('Ctrl Pts',(0.00487384017162634,-0.0329142774063509,
0.0788939890306646));
#104890=CARTESIAN_POINT('Ctrl Pts',(0.00480875673042359,-0.0328043479726686,
0.0788487411503022));
#104891=CARTESIAN_POINT('Ctrl Pts',(0.00474463214041636,-0.0326943950436594,
0.0788021635505798));
#104892=CARTESIAN_POINT('Ctrl Pts',(0.00495975584059877,-0.0330240426238156,
0.0790493988225064));
#104893=CARTESIAN_POINT('Ctrl Pts',(0.00489226184856611,-0.0329142774063509,
0.0790058112769393));
#104894=CARTESIAN_POINT('Ctrl Pts',(0.00482563528463957,-0.0328043479726686,
0.0789608067120406));
#104895=CARTESIAN_POINT('Ctrl Pts',(0.00475996309019608,-0.0326943950436594,
0.0789144404313869));
#104896=CARTESIAN_POINT('Ctrl Pts',(0.00497971419027906,-0.0330240426238156,
0.0791609461230697));
#104897=CARTESIAN_POINT('Ctrl Pts',(0.00491068352550588,-0.0329142774063509,
0.079117633523214));
#104898=CARTESIAN_POINT('Ctrl Pts',(0.00484251383885554,-0.0328043479726686,
0.079072872273779));
#104899=CARTESIAN_POINT('Ctrl Pts',(0.0047752940399758,-0.0326943950436594,
0.0790267173121941));
#104900=CARTESIAN_POINT('Ctrl Pts',(0.00499967253995936,-0.0330240426238156,
0.079272493423633));
#104901=CARTESIAN_POINT('Ctrl Pts',(0.00492910520244565,-0.0329142774063509,
0.0792294557694886));
#104902=CARTESIAN_POINT('Ctrl Pts',(0.00485939239307151,-0.0328043479726686,
0.0791849378355174));
#104903=CARTESIAN_POINT('Ctrl Pts',(0.00479062498975551,-0.0326943950436594,
0.0791389941930012));
#104904=CARTESIAN_POINT('Origin',(0.014676911042144,-0.0326396682854563,
0.0652529107625777));
#104905=CARTESIAN_POINT('Ctrl Pts',(0.00450435085242291,-0.0331951640388587,
0.0789353648523489));
#104906=CARTESIAN_POINT('Ctrl Pts',(0.00443844213229608,-0.033085561825504,
0.0788855145076809));
#104907=CARTESIAN_POINT('Ctrl Pts',(0.00437351622090669,-0.0329757224427707,
0.0788342660060127));
#104908=CARTESIAN_POINT('Ctrl Pts',(0.00430965947891291,-0.0328657862078596,
0.0787816808958618));
#104909=CARTESIAN_POINT('Ctrl Pts',(0.00461544361159874,-0.0331951640388587,
0.0789130142170475));
#104910=CARTESIAN_POINT('Ctrl Pts',(0.00454984272625821,-0.033085561825504,
0.0788646939503983));
#104911=CARTESIAN_POINT('Ctrl Pts',(0.00448519324747173,-0.0329757224427707,
0.0788149829921797));
#104912=CARTESIAN_POINT('Ctrl Pts',(0.00442158108532942,-0.0328657862078596,
0.0787639409393561));
#104913=CARTESIAN_POINT('Ctrl Pts',(0.00472653637077457,-0.0331951640388587,
0.0788906635817461));
#104914=CARTESIAN_POINT('Ctrl Pts',(0.00466124332022035,-0.0330855618255041,
0.0788438733931158));
#104915=CARTESIAN_POINT('Ctrl Pts',(0.00459687027403676,-0.0329757224427707,
0.0787956999783466));
#104916=CARTESIAN_POINT('Ctrl Pts',(0.00453350269174592,-0.0328657862078596,
0.0787462009828505));
#104917=CARTESIAN_POINT('Ctrl Pts',(0.00483762912995039,-0.0331951640388587,
0.0788683129464448));
#104918=CARTESIAN_POINT('Ctrl Pts',(0.00477264391418249,-0.0330855618255041,
0.0788230528358333));
#104919=CARTESIAN_POINT('Ctrl Pts',(0.0047085473006018,-0.0329757224427707,
0.0787764169645136));
#104920=CARTESIAN_POINT('Ctrl Pts',(0.00464542429816242,-0.0328657862078596,
0.0787284610263448));
#104921=CARTESIAN_POINT('Origin',(0.0150400157860922,-0.0326401908834433,
0.0655682325287461));
#104922=CARTESIAN_POINT('Ctrl Pts',(0.0048653280158603,-0.0332451089994432,
0.0788892616908939));
#104923=CARTESIAN_POINT('Ctrl Pts',(0.00468658383678061,-0.0329451141710258,
0.0787663670809381));
#104924=CARTESIAN_POINT('Ctrl Pts',(0.00451760437546793,-0.0326442513127503,
0.0786303578593187));
#104925=CARTESIAN_POINT('Ctrl Pts',(0.00507436390812141,-0.0332451089994432,
0.0790263893531165));
#104926=CARTESIAN_POINT('Ctrl Pts',(0.00489044787464504,-0.0329451141710258,
0.0789113786608249));
#104927=CARTESIAN_POINT('Ctrl Pts',(0.00471571740271998,-0.0326442513127503,
0.0787828413942759));
#104928=CARTESIAN_POINT('Ctrl Pts',(0.00464544939608382,-0.0325229783203385,
0.0787284802064067));
#104929=CARTESIAN_POINT('Ctrl Pts',(0.00458233514771206,-0.0324130253112079,
0.0786805314657386));
#104930=CARTESIAN_POINT('Ctrl Pts',(0.00452022235312969,-0.0323031222247695,
0.0786312843981566));
#104931=CARTESIAN_POINT('Ctrl Pts',(0.00445918834845222,-0.0321934096636184,
0.0785808048931343));
#104932=CARTESIAN_POINT('Ctrl Pts',(0.00465836427094616,-0.0325229783203385,
0.0788410606161457));
#104933=CARTESIAN_POINT('Ctrl Pts',(0.00459369810411637,-0.0324130253112079,
0.0787932899067419));
#104934=CARTESIAN_POINT('Ctrl Pts',(0.00453002994364946,-0.0323031222247695,
0.0787441887399959));
#104935=CARTESIAN_POINT('Ctrl Pts',(0.00446743912456871,-0.0321934096636184,
0.078693822888795));
#104936=CARTESIAN_POINT('Ctrl Pts',(0.0046712791458085,-0.0325229783203385,
0.0789536410258846));
#104937=CARTESIAN_POINT('Ctrl Pts',(0.00460506106052067,-0.0324130253112079,
0.0789060483477451));
#104938=CARTESIAN_POINT('Ctrl Pts',(0.00453983753416924,-0.0323031222247695,
0.0788570930818352));
#104939=CARTESIAN_POINT('Ctrl Pts',(0.0044756899006852,-0.0321934096636184,
0.0788068408844558));
#104940=CARTESIAN_POINT('Ctrl Pts',(0.00468419402067084,-0.0325229783203385,
0.0790662214356236));
#104941=CARTESIAN_POINT('Ctrl Pts',(0.00461642401692498,-0.0324130253112079,
0.0790188067887484));
#104942=CARTESIAN_POINT('Ctrl Pts',(0.00454964512468902,-0.0323031222247695,
0.0789699974236745));
#104943=CARTESIAN_POINT('Ctrl Pts',(0.00448394067680168,-0.0321934096636184,
0.0789198588801165));
#104944=CARTESIAN_POINT('Origin',(0.0146716648041683,-0.0326393375176332,
0.065259631478032));
#104945=CARTESIAN_POINT('Ctrl Pts',(0.00421101742817708,-0.0326943950436594,
0.0786986560536431));
#104946=CARTESIAN_POINT('Ctrl Pts',(0.00414832842266803,-0.0325844576448127,
0.0786447308218798));
#104947=CARTESIAN_POINT('Ctrl Pts',(0.00408675024276515,-0.0324744968375318,
0.0785895052623301));
#104948=CARTESIAN_POINT('Ctrl Pts',(0.00402636081005524,-0.0323646534831894,
0.078533051221436));
#104949=CARTESIAN_POINT('Ctrl Pts',(0.00432329427224715,-0.0326943950436594,
0.0786833251088797));
#104950=CARTESIAN_POINT('Ctrl Pts',(0.0042608165558902,-0.0325844576448127,
0.0786309472624569));
#104951=CARTESIAN_POINT('Ctrl Pts',(0.00419941767762686,-0.0324744968375318,
0.0785772735675646));
#104952=CARTESIAN_POINT('Ctrl Pts',(0.0041391753567374,-0.0323646534831894,
0.0785223738791367));
#104953=CARTESIAN_POINT('Ctrl Pts',(0.00443557111631723,-0.0326943950436593,
0.0786679941641163));
#104954=CARTESIAN_POINT('Ctrl Pts',(0.00437330468911236,-0.0325844576448126,
0.078617163703034));
#104955=CARTESIAN_POINT('Ctrl Pts',(0.00431208511248856,-0.0324744968375318,
0.0785650418727991));
#104956=CARTESIAN_POINT('Ctrl Pts',(0.00425198990341955,-0.0323646534831894,
0.0785116965368374));
#104957=CARTESIAN_POINT('Ctrl Pts',(0.0045478479603873,-0.0326943950436593,
0.0786526632193529));
#104958=CARTESIAN_POINT('Ctrl Pts',(0.00448579282233453,-0.0325844576448126,
0.0786033801436111));
#104959=CARTESIAN_POINT('Ctrl Pts',(0.00442475254735027,-0.0324744968375318,
0.0785528101780337));
#104960=CARTESIAN_POINT('Ctrl Pts',(0.00436480445010171,-0.0323646534831894,
0.0785010191945382));
#104961=CARTESIAN_POINT('Origin',(0.0150634030036769,-0.0326395579067523,
0.0655384835811933));
#104962=CARTESIAN_POINT('Ctrl Pts',(0.00457420798906062,-0.0327445246961877,
0.0786753340175019));
#104963=CARTESIAN_POINT('Ctrl Pts',(0.00440353222819769,-0.0324436878365475,
0.0785414596392411));
#104964=CARTESIAN_POINT('Ctrl Pts',(0.00424342530435261,-0.0321434074463186,
0.0783951095882069));
#104965=CARTESIAN_POINT('Ctrl Pts',(0.00477422210243722,-0.0327445246961877,
0.0788253151978218));
#104966=CARTESIAN_POINT('Ctrl Pts',(0.00459788970894404,-0.0324436878365475,
0.0786989844750906));
#104967=CARTESIAN_POINT('Ctrl Pts',(0.00443157400340436,-0.0321434074463186,
0.0785597305681734));
#104968=CARTESIAN_POINT('Ctrl Pts',(0.0042928907472474,-0.0322357242816072,
0.0784398013625377));
#104969=CARTESIAN_POINT('Ctrl Pts',(0.00415626613751914,-0.0319819883628705,
0.0783177924384711));
#104970=CARTESIAN_POINT('Ctrl Pts',(0.00402768219139062,-0.0317295851069886,
0.0781873369658635));
#104971=CARTESIAN_POINT('Ctrl Pts',(0.00448293491741518,-0.0322357242816072,
0.0786022304651801));
#104972=CARTESIAN_POINT('Ctrl Pts',(0.00434113715143059,-0.0319819883628705,
0.0784862742014552));
#104973=CARTESIAN_POINT('Ctrl Pts',(0.00420700538499615,-0.0317295851069886,
0.0783615299399902));
#104974=CARTESIAN_POINT('Origin',(0.015002286670181,-0.032637194264492,
0.0656116081134578));
#104975=CARTESIAN_POINT('Origin',(0.0145965540519013,-0.0326352985529824,
0.0653566993818225));
#104976=CARTESIAN_POINT('Ctrl Pts',(0.00393312589888557,-0.0321934096636183,
0.0784439957875769));
#104977=CARTESIAN_POINT('Ctrl Pts',(0.00387390835043815,-0.0320835708272303,
0.0783862033712807));
#104978=CARTESIAN_POINT('Ctrl Pts',(0.00381592116162688,-0.0319739230346346,
0.0783272189728474));
#104979=CARTESIAN_POINT('Ctrl Pts',(0.00375923273119791,-0.0318646057455575,
0.0782671237526427));
#104980=CARTESIAN_POINT('Ctrl Pts',(0.0040461439918666,-0.0321934096636183,
0.0784357450043557));
#104981=CARTESIAN_POINT('Ctrl Pts',(0.00398704022815007,-0.0320835708272303,
0.0783795111956426));
#104982=CARTESIAN_POINT('Ctrl Pts',(0.00392913450276701,-0.0319739230346346,
0.0783220868555058));
#104983=CARTESIAN_POINT('Ctrl Pts',(0.00387249526342312,-0.0318646057455575,
0.0782635511403255));
#104984=CARTESIAN_POINT('Ctrl Pts',(0.00415916208484763,-0.0321934096636183,
0.0784274942211344));
#104985=CARTESIAN_POINT('Ctrl Pts',(0.00410017210586199,-0.0320835708272303,
0.0783728190200045));
#104986=CARTESIAN_POINT('Ctrl Pts',(0.00404234784390713,-0.0319739230346346,
0.0783169547381642));
#104987=CARTESIAN_POINT('Ctrl Pts',(0.00398575779564832,-0.0318646057455575,
0.0782599785280082));
#104988=CARTESIAN_POINT('Ctrl Pts',(0.00427218017782866,-0.0321934096636183,
0.0784192434379131));
#104989=CARTESIAN_POINT('Ctrl Pts',(0.00421330398357392,-0.0320835708272303,
0.0783661268443664));
#104990=CARTESIAN_POINT('Ctrl Pts',(0.00415556118504725,-0.0319739230346346,
0.0783118226208226));
#104991=CARTESIAN_POINT('Ctrl Pts',(0.00409902032787352,-0.0318646057455575,
0.078256405915691));
#104992=CARTESIAN_POINT('Ctrl Pts',(0.00436461899514258,-0.0320218834582382,
0.0785019524183383));
#104993=CARTESIAN_POINT('Ctrl Pts',(0.00431932569124386,-0.0319391099350654,
0.0784628286171652));
#104994=CARTESIAN_POINT('Ctrl Pts',(0.00427467075304835,-0.0318564869454911,
0.0784230212588178));
#104995=CARTESIAN_POINT('Ctrl Pts',(0.0042306839989288,-0.031774074144648,
0.0783825623741296));
#104996=CARTESIAN_POINT('Ctrl Pts',(0.0043671618351721,-0.0320218834582382,
0.0785514535497625));
#104997=CARTESIAN_POINT('Ctrl Pts',(0.00432135334416346,-0.0319391099350654,
0.0785123562134068));
#104998=CARTESIAN_POINT('Ctrl Pts',(0.00427618311774497,-0.0318564869454911,
0.0784725672591235));
#104999=CARTESIAN_POINT('Ctrl Pts',(0.00423168135085995,-0.031774074144648,
0.0784321187393798));
#105000=CARTESIAN_POINT('Ctrl Pts',(0.00436970467520161,-0.0320218834582382,
0.0786009546811868));
#105001=CARTESIAN_POINT('Ctrl Pts',(0.00432338099708305,-0.0319391099350654,
0.0785618838096484));
#105002=CARTESIAN_POINT('Ctrl Pts',(0.00427769548244158,-0.0318564869454911,
0.0785221132594293));
#105003=CARTESIAN_POINT('Ctrl Pts',(0.0042326787027911,-0.031774074144648,
0.0784816751046301));
#105004=CARTESIAN_POINT('Ctrl Pts',(0.00437224751523113,-0.0320218834582382,
0.078650455812611));
#105005=CARTESIAN_POINT('Ctrl Pts',(0.00432540865000264,-0.0319391099350654,
0.07861141140589));
#105006=CARTESIAN_POINT('Ctrl Pts',(0.0042792078471382,-0.0318564869454911,
0.078571659259735));
#105007=CARTESIAN_POINT('Ctrl Pts',(0.00423367605472224,-0.031774074144648,
0.0785312314698804));
#105008=CARTESIAN_POINT('Origin',(0.000965309449836182,-0.0391228853390901,
0.0838781491720797));
#105009=CARTESIAN_POINT('Ctrl Pts',(0.00710343017868775,-0.0352722978779664,
0.0798106577629517));
#105010=CARTESIAN_POINT('Ctrl Pts',(0.0070848982945471,-0.0352466642097263,
0.0798069615556662));
#105011=CARTESIAN_POINT('Ctrl Pts',(0.00706636758505475,-0.0352210183808324,
0.0798033455278783));
#105012=CARTESIAN_POINT('Ctrl Pts',(0.00704783729429126,-0.0351953608940152,
0.0797998100746452));
#105013=CARTESIAN_POINT('Origin',(0.00596800377611451,-0.0352456003065123,
0.0845772655798465));
#105014=CARTESIAN_POINT('Ctrl Pts',(0.00692591360635499,-0.0350241211493339,
0.0797737346122686));
#105015=CARTESIAN_POINT('Ctrl Pts',(0.00684844897138487,-0.0349144232867421,
0.0797572344643753));
#105016=CARTESIAN_POINT('Ctrl Pts',(0.00677127903993087,-0.0348045283677512,
0.0797391231910628));
#105017=CARTESIAN_POINT('Ctrl Pts',(0.00669450352012076,-0.0346945769586886,
0.0797194203123216));
#105018=CARTESIAN_POINT('Ctrl Pts',(0.00698553372184158,-0.0350241211493339,
0.0798701015341502));
#105019=CARTESIAN_POINT('Ctrl Pts',(0.00690674167209437,-0.0349144232867421,
0.0798544226288656));
#105020=CARTESIAN_POINT('Ctrl Pts',(0.0068282265556708,-0.0348045283677512,
0.0798371056511042));
#105021=CARTESIAN_POINT('Ctrl Pts',(0.00675008976585002,-0.0346945769586886,
0.0798181690393479));
#105022=CARTESIAN_POINT('Ctrl Pts',(0.00704515383732817,-0.0350241211493339,
0.0799664684560319));
#105023=CARTESIAN_POINT('Ctrl Pts',(0.00696503437280388,-0.0349144232867421,
0.0799516107933558));
#105024=CARTESIAN_POINT('Ctrl Pts',(0.00688517407141074,-0.0348045283677512,
0.0799350881111456));
#105025=CARTESIAN_POINT('Ctrl Pts',(0.00680567601157928,-0.0346945769586886,
0.0799169177663742));
#105026=CARTESIAN_POINT('Ctrl Pts',(0.00710477395281477,-0.0350241211493339,
0.0800628353779136));
#105027=CARTESIAN_POINT('Ctrl Pts',(0.00702332707351338,-0.0349144232867421,
0.0800487989578461));
#105028=CARTESIAN_POINT('Ctrl Pts',(0.00694212158715068,-0.0348045283677512,
0.0800330705711871));
#105029=CARTESIAN_POINT('Ctrl Pts',(0.00686126225730854,-0.0346945769586886,
0.0800156664934005));
#105030=CARTESIAN_POINT('Origin',(0.0110419555985394,-0.034562906794156,
0.0635032984105877));
#105031=CARTESIAN_POINT('Ctrl Pts',(0.00659933070161038,-0.0351970973651595,
0.0798816288633648));
#105032=CARTESIAN_POINT('Ctrl Pts',(0.00651992675144133,-0.0350869349321762,
0.0798605096539478));
#105033=CARTESIAN_POINT('Ctrl Pts',(0.00644089608062417,-0.0349764985129722,
0.0798377221855027));
#105034=CARTESIAN_POINT('Ctrl Pts',(0.00636234281354197,-0.0348659306849651,
0.0798132899527924));
#105035=CARTESIAN_POINT('Ctrl Pts',(0.00666829611299639,-0.0351970973651595,
0.079836860094309));
#105036=CARTESIAN_POINT('Ctrl Pts',(0.00658951237345017,-0.0350869349321762,
0.079816696307202));
#105037=CARTESIAN_POINT('Ctrl Pts',(0.00651108256433076,-0.0349764985129722,
0.0797948779463629));
#105038=CARTESIAN_POINT('Ctrl Pts',(0.00643310995768071,-0.0348659306849651,
0.0797714272968703));
#105039=CARTESIAN_POINT('Ctrl Pts',(0.00673726152438239,-0.0351970973651595,
0.0797920913252531));
#105040=CARTESIAN_POINT('Ctrl Pts',(0.00665909799545902,-0.0350869349321762,
0.0797728829604563));
#105041=CARTESIAN_POINT('Ctrl Pts',(0.00658126904803734,-0.0349764985129722,
0.0797520337072231));
#105042=CARTESIAN_POINT('Ctrl Pts',(0.00650387710181946,-0.0348659306849651,
0.0797295646409481));
#105043=CARTESIAN_POINT('Ctrl Pts',(0.00680622693576839,-0.0351970973651595,
0.0797473225561973));
#105044=CARTESIAN_POINT('Ctrl Pts',(0.00672868361746786,-0.0350869349321762,
0.0797290696137105));
#105045=CARTESIAN_POINT('Ctrl Pts',(0.00665145553174393,-0.0349764985129722,
0.0797091894680833));
#105046=CARTESIAN_POINT('Ctrl Pts',(0.0065746442459582,-0.0348659306849651,
0.0796877019850259));
#105047=CARTESIAN_POINT('Origin',(0.0114917135417066,-0.0345637187965474,
0.0636737189169973));
#105048=CARTESIAN_POINT('Ctrl Pts',(0.00683878082878371,-0.0352450361861253,
0.0797559697192978));
#105049=CARTESIAN_POINT('Ctrl Pts',(0.00662734821681258,-0.0349452761023765,
0.0797075050988219));
#105050=CARTESIAN_POINT('Ctrl Pts',(0.00642016681602617,-0.0346444289983475,
0.0796432521921873));
#105051=CARTESIAN_POINT('Ctrl Pts',(0.0070836174924134,-0.0352450361861253,
0.0798065168076678));
#105052=CARTESIAN_POINT('Ctrl Pts',(0.00687027846577064,-0.0349452761023765,
0.0797672863532487));
#105053=CARTESIAN_POINT('Ctrl Pts',(0.00666050051108305,-0.0346444289983475,
0.0797120977804287));
#105054=CARTESIAN_POINT('Ctrl Pts',(0.00657516103046764,-0.0345231616327822,
0.0796874229798397));
#105055=CARTESIAN_POINT('Ctrl Pts',(0.00649883545075899,-0.0344132092796975,
0.079666077417397));
#105056=CARTESIAN_POINT('Ctrl Pts',(0.00642295532522138,-0.0343032738558974,
0.0796431542218758));
#105057=CARTESIAN_POINT('Ctrl Pts',(0.00634761711281161,-0.034193496108874,
0.0796186852506402));
#105058=CARTESIAN_POINT('Ctrl Pts',(0.00662861257439584,-0.0345231616327822,
0.0797873432910419));
#105059=CARTESIAN_POINT('Ctrl Pts',(0.00655090973387383,-0.0344132092796975,
0.0797667344828785));
#105060=CARTESIAN_POINT('Ctrl Pts',(0.00647363717940205,-0.0343032738558974,
0.0797445195160698));
#105061=CARTESIAN_POINT('Ctrl Pts',(0.00639689317704112,-0.034193496108874,
0.0797207293863516));
#105062=CARTESIAN_POINT('Ctrl Pts',(0.00668206411832403,-0.0345231616327822,
0.079887263602244));
#105063=CARTESIAN_POINT('Ctrl Pts',(0.00660298401698866,-0.0344132092796975,
0.07986739154836));
#105064=CARTESIAN_POINT('Ctrl Pts',(0.00652431903358272,-0.0343032738558974,
0.0798458848102639));
#105065=CARTESIAN_POINT('Ctrl Pts',(0.00644616924127063,-0.034193496108874,
0.0798227735220631));
#105066=CARTESIAN_POINT('Ctrl Pts',(0.00673551566225223,-0.0345231616327822,
0.0799871839134462));
#105067=CARTESIAN_POINT('Ctrl Pts',(0.00665505830010349,-0.0344132092796975,
0.0799680486138414));
#105068=CARTESIAN_POINT('Ctrl Pts',(0.00657500088776339,-0.0343032738558974,
0.079947250104458));
#105069=CARTESIAN_POINT('Ctrl Pts',(0.00649544530550014,-0.034193496108874,
0.0799248176577745));
#105070=CARTESIAN_POINT('Origin',(0.0110449128153173,-0.0345625596230184,
0.0634915615823885));
#105071=CARTESIAN_POINT('Ctrl Pts',(0.00616025749492642,-0.0346945769586885,
0.0798196182199217));
#105072=CARTESIAN_POINT('Ctrl Pts',(0.00608212729015849,-0.0345846629176052,
0.079792559857121));
#105073=CARTESIAN_POINT('Ctrl Pts',(0.00600454329639,-0.0344746925050311,
0.0797638811721372));
#105074=CARTESIAN_POINT('Ctrl Pts',(0.00592760477141671,-0.0343648066253259,
0.0797336193219533));
#105075=CARTESIAN_POINT('Ctrl Pts',(0.00625900614419945,-0.0346945769586885,
0.0797640320179602));
#105076=CARTESIAN_POINT('Ctrl Pts',(0.00618164194539049,-0.0345846629176052,
0.0797383344614588));
#105077=CARTESIAN_POINT('Ctrl Pts',(0.00610479594750125,-0.0344746925050311,
0.0797110326558919));
#105078=CARTESIAN_POINT('Ctrl Pts',(0.00602856647000809,-0.0343648066253259,
0.079682161990121));
#105079=CARTESIAN_POINT('Ctrl Pts',(0.00635775479347248,-0.0346945769586885,
0.0797084458159986));
#105080=CARTESIAN_POINT('Ctrl Pts',(0.00628115660062249,-0.0345846629176052,
0.0796841090657966));
#105081=CARTESIAN_POINT('Ctrl Pts',(0.0062050485986125,-0.0344746925050311,
0.0796581841396467));
#105082=CARTESIAN_POINT('Ctrl Pts',(0.00612952816859947,-0.0343648066253259,
0.0796307046582887));
#105083=CARTESIAN_POINT('Ctrl Pts',(0.00645650344274552,-0.0346945769586885,
0.0796528596140371));
#105084=CARTESIAN_POINT('Ctrl Pts',(0.00638067125585449,-0.0345846629176052,
0.0796298836701343));
#105085=CARTESIAN_POINT('Ctrl Pts',(0.00630530124972375,-0.0344746925050311,
0.0796053356234015));
#105086=CARTESIAN_POINT('Ctrl Pts',(0.00623048986719085,-0.0343648066253259,
0.0795792473264565));
#105087=CARTESIAN_POINT('Origin',(0.0115088537350995,-0.0345626446730671,
0.0636178588735325));
#105088=CARTESIAN_POINT('Ctrl Pts',(0.00645473649828103,-0.0346945769586886,
0.0796538542375848));
#105089=CARTESIAN_POINT('Ctrl Pts',(0.00633945606765366,-0.0345275153362891,
0.0796188954072578));
#105090=CARTESIAN_POINT('Ctrl Pts',(0.00622524524263857,-0.0343603235965159,
0.0795803020713518));
#105091=CARTESIAN_POINT('Ctrl Pts',(0.00611244011171103,-0.034193496108874,
0.0795381933921864));
#105092=CARTESIAN_POINT('Ctrl Pts',(0.00653547195057605,-0.0346945769586886,
0.079676433322464));
#105093=CARTESIAN_POINT('Ctrl Pts',(0.00641971859197572,-0.0345275153362891,
0.07964316552851));
#105094=CARTESIAN_POINT('Ctrl Pts',(0.00630498153512684,-0.0343603235965159,
0.0796062487932162));
#105095=CARTESIAN_POINT('Ctrl Pts',(0.00619159849856314,-0.034193496108874,
0.0795657973433934));
#105096=CARTESIAN_POINT('Ctrl Pts',(0.00661620740287108,-0.0346945769586886,
0.0796990124073433));
#105097=CARTESIAN_POINT('Ctrl Pts',(0.00649998111629779,-0.0345275153362891,
0.0796674356497623));
#105098=CARTESIAN_POINT('Ctrl Pts',(0.00638471782761511,-0.0343603235965159,
0.0796321955150806));
#105099=CARTESIAN_POINT('Ctrl Pts',(0.00627075688541525,-0.034193496108874,
0.0795934012946004));
#105100=CARTESIAN_POINT('Ctrl Pts',(0.0066969428551661,-0.0346945769586886,
0.0797215914922225));
#105101=CARTESIAN_POINT('Ctrl Pts',(0.00658024364061985,-0.0345275153362891,
0.0796917057710145));
#105102=CARTESIAN_POINT('Ctrl Pts',(0.00646445412010338,-0.0343603235965159,
0.0796581422369451));
#105103=CARTESIAN_POINT('Ctrl Pts',(0.00634991527226737,-0.034193496108874,
0.0796210052458074));
#105104=CARTESIAN_POINT('Ctrl Pts',(0.00623051984523234,-0.0340223579322365,
0.0795792571906563));
#105105=CARTESIAN_POINT('Ctrl Pts',(0.00615563622847656,-0.0339125849573552,
0.0795531441650439));
#105106=CARTESIAN_POINT('Ctrl Pts',(0.00608134571052315,-0.0338030433565217,
0.0795254995718907));
#105107=CARTESIAN_POINT('Ctrl Pts',(0.00600774016254726,-0.0336938721132321,
0.0794963671857699));
#105108=CARTESIAN_POINT('Ctrl Pts',(0.00627759196310741,-0.0340223579322365,
0.079682336749976));
#105109=CARTESIAN_POINT('Ctrl Pts',(0.00620128661038585,-0.0339125849573552,
0.0796568729716383));
#105110=CARTESIAN_POINT('Ctrl Pts',(0.00612556191759411,-0.0338030433565217,
0.0796298477429105));
#105111=CARTESIAN_POINT('Ctrl Pts',(0.00605051166018825,-0.0336938721132321,
0.0796013042088853));
#105112=CARTESIAN_POINT('Ctrl Pts',(0.00632466408098248,-0.0340223579322365,
0.0797854163092957));
#105113=CARTESIAN_POINT('Ctrl Pts',(0.00624693699229514,-0.0339125849573552,
0.0797606017782327));
#105114=CARTESIAN_POINT('Ctrl Pts',(0.00616977812466508,-0.0338030433565217,
0.0797341959139303));
#105115=CARTESIAN_POINT('Ctrl Pts',(0.00609328315782925,-0.0336938721132321,
0.0797062412320008));
#105116=CARTESIAN_POINT('Ctrl Pts',(0.00637173619885756,-0.0340223579322365,
0.0798884958686154));
#105117=CARTESIAN_POINT('Ctrl Pts',(0.00629258737420443,-0.0339125849573552,
0.0798643305848271));
#105118=CARTESIAN_POINT('Ctrl Pts',(0.00621399433173604,-0.0338030433565217,
0.07983854408495));
#105119=CARTESIAN_POINT('Ctrl Pts',(0.00613605465547024,-0.0336938721132321,
0.0798111782551162));
#105120=CARTESIAN_POINT('Origin',(0.0110106430328453,-0.0345589643415453,
0.0636067937832463));
#105121=CARTESIAN_POINT('Ctrl Pts',(0.00580813378883228,-0.034193496108874,
0.0796851397875581));
#105122=CARTESIAN_POINT('Ctrl Pts',(0.00573180748894145,-0.0340836138581107,
0.0796532083673356));
#105123=CARTESIAN_POINT('Ctrl Pts',(0.0056561785655845,-0.0339738896643499,
0.079619712855787));
#105124=CARTESIAN_POINT('Ctrl Pts',(0.0055813409406497,-0.0338644633294062,
0.0795847026117196));
#105125=CARTESIAN_POINT('Ctrl Pts',(0.00591017801635925,-0.034193496108874,
0.0796358636789918));
#105126=CARTESIAN_POINT('Ctrl Pts',(0.0058345312048254,-0.0340836138581107,
0.0796053393882387));
#105127=CARTESIAN_POINT('Ctrl Pts',(0.00575955232620233,-0.0339738896643499,
0.0795732643915782));
#105128=CARTESIAN_POINT('Ctrl Pts',(0.00568533459227637,-0.0338644633294062,
0.0795396861739623));
#105129=CARTESIAN_POINT('Ctrl Pts',(0.00601222224388621,-0.034193496108874,
0.0795865875704255));
#105130=CARTESIAN_POINT('Ctrl Pts',(0.00593725492070934,-0.0340836138581107,
0.0795574704091419));
#105131=CARTESIAN_POINT('Ctrl Pts',(0.00586292608682015,-0.0339738896643499,
0.0795268159273693));
#105132=CARTESIAN_POINT('Ctrl Pts',(0.00578932824390305,-0.0338644633294062,
0.0794946697362049));
#105133=CARTESIAN_POINT('Ctrl Pts',(0.00611426647141318,-0.034193496108874,
0.0795373114618592));
#105134=CARTESIAN_POINT('Ctrl Pts',(0.00603997863659329,-0.0340836138581107,
0.079509601430045));
#105135=CARTESIAN_POINT('Ctrl Pts',(0.00596629984743797,-0.0339738896643499,
0.0794803674631605));
#105136=CARTESIAN_POINT('Ctrl Pts',(0.00589332189552972,-0.0338644633294062,
0.0794496532984475));
#105137=CARTESIAN_POINT('Origin',(0.011484736484883,-0.0345610621862571,
0.0636891673860762));
#105138=CARTESIAN_POINT('Ctrl Pts',(0.00614637285195932,-0.0342436276873901,
0.0795507385881505));
#105139=CARTESIAN_POINT('Ctrl Pts',(0.00594268063820261,-0.0339430054201861,
0.0794761593653965));
#105140=CARTESIAN_POINT('Ctrl Pts',(0.00574518470530769,-0.0336441434784164,
0.0793864490822531));
#105141=CARTESIAN_POINT('Ctrl Pts',(0.00638294477864433,-0.0342436276873901,
0.0796315700393595));
#105142=CARTESIAN_POINT('Ctrl Pts',(0.00617620395644838,-0.0339430054201861,
0.0795659132739087));
#105143=CARTESIAN_POINT('Ctrl Pts',(0.00597499599984848,-0.0336441434784164,
0.0794848704666239));
#105144=CARTESIAN_POINT('Ctrl Pts',(0.00589334750425107,-0.0335235895815127,
0.0794496639389884));
#105145=CARTESIAN_POINT('Ctrl Pts',(0.00582038719605378,-0.0334144449262719,
0.079418957614175));
#105146=CARTESIAN_POINT('Ctrl Pts',(0.00574797743486331,-0.0333049234473133,
0.0793867087064559));
#105147=CARTESIAN_POINT('Ctrl Pts',(0.00567621454590946,-0.0331951640388588,
0.0793529500650937));
#105148=CARTESIAN_POINT('Ctrl Pts',(0.00593385425712526,-0.0335235895815127,
0.0795554957652901));
#105149=CARTESIAN_POINT('Ctrl Pts',(0.00585943696547526,-0.0334144449262719,
0.0795253470956804));
#105150=CARTESIAN_POINT('Ctrl Pts',(0.00578555702619778,-0.0333049234473133,
0.0794936263836617));
#105151=CARTESIAN_POINT('Ctrl Pts',(0.00571231258324836,-0.0331951640388588,
0.0794603656328063));
#105152=CARTESIAN_POINT('Ctrl Pts',(0.00597436100999945,-0.0335235895815127,
0.0796613275915918));
#105153=CARTESIAN_POINT('Ctrl Pts',(0.00589848673489674,-0.0334144449262719,
0.0796317365771858));
#105154=CARTESIAN_POINT('Ctrl Pts',(0.00582313661753225,-0.0333049234473133,
0.0796005440608675));
#105155=CARTESIAN_POINT('Ctrl Pts',(0.00574841062058726,-0.0331951640388588,
0.079567781200519));
#105156=CARTESIAN_POINT('Ctrl Pts',(0.00601486776287364,-0.0335235895815127,
0.0797671594178934));
#105157=CARTESIAN_POINT('Ctrl Pts',(0.00593753650431821,-0.0334144449262719,
0.0797381260586913));
#105158=CARTESIAN_POINT('Ctrl Pts',(0.00586071620886671,-0.0333049234473133,
0.0797074617380733));
#105159=CARTESIAN_POINT('Ctrl Pts',(0.00578450865792616,-0.0331951640388588,
0.0796751967682316));
#105160=CARTESIAN_POINT('Origin',(0.0134522516024782,-0.0326434571769783,
0.0646110340170667));
#105161=CARTESIAN_POINT('Ctrl Pts',(0.00546327129297219,-0.0336938721132459,
0.0795295819804915));
#105162=CARTESIAN_POINT('Ctrl Pts',(0.00543178281450347,-0.0336474569764992,
0.0795140091273407));
#105163=CARTESIAN_POINT('Ctrl Pts',(0.0054004787935538,-0.033601104548885,
0.0794980687288541));
#105164=CARTESIAN_POINT('Ctrl Pts',(0.00532122421317455,-0.0334837508643204,
0.0794577113065546));
#105165=CARTESIAN_POINT('Ctrl Pts',(0.00524320030960904,-0.0333660264760491,
0.0794150231288218));
#105166=CARTESIAN_POINT('Ctrl Pts',(0.00577808157345017,-0.0336938721132459,
0.0794012678091044));
#105167=CARTESIAN_POINT('Ctrl Pts',(0.00574734416040578,-0.0336474569764992,
0.0793875376449905));
#105168=CARTESIAN_POINT('Ctrl Pts',(0.00571676958241522,-0.033601104548885,
0.0793734486014476));
#105169=CARTESIAN_POINT('Ctrl Pts',(0.00563936178381929,-0.0334837508643204,
0.0793377783840103));
#105170=CARTESIAN_POINT('Ctrl Pts',(0.00556304495947447,-0.0333660264760491,
0.0792998300768357));
#105171=CARTESIAN_POINT('Ctrl Pts',(0.00577808157345143,-0.0336938721132426,
0.0794012678091105));
#105172=CARTESIAN_POINT('Ctrl Pts',(0.00574734416041144,-0.0336474569765026,
0.0793875376449985));
#105173=CARTESIAN_POINT('Ctrl Pts',(0.00571676958242522,-0.0336011045488949,
0.0793734486014576));
#105174=CARTESIAN_POINT('Ctrl Pts',(0.00564000648535609,-0.0334847282606778,
0.0793380754683458));
#105175=CARTESIAN_POINT('Ctrl Pts',(0.00556431599105305,-0.0333679869945434,
0.0793004618977903));
#105176=CARTESIAN_POINT('Ctrl Pts',(0.00577808157344808,-0.0336938721132427,
0.0794012678091035));
#105177=CARTESIAN_POINT('Ctrl Pts',(0.00566815098175153,-0.0335278710435083,
0.0793521626660339));
#105178=CARTESIAN_POINT('Ctrl Pts',(0.0055597989879013,-0.033362046922432,
0.0792996274032657));
#105179=CARTESIAN_POINT('Ctrl Pts',(0.00545298044386996,-0.0331951640388602,
0.0792436178710486));
#105180=CARTESIAN_POINT('Ctrl Pts',(0.0058553505010703,-0.0336938721132427,
0.0794337876899056));
#105181=CARTESIAN_POINT('Ctrl Pts',(0.00574473913477446,-0.0335278710435083,
0.0793863001026801));
#105182=CARTESIAN_POINT('Ctrl Pts',(0.00563565587968916,-0.033362046922432,
0.0793353604777891));
#105183=CARTESIAN_POINT('Ctrl Pts',(0.00552805495870329,-0.0331951640388602,
0.0792809253374034));
#105184=CARTESIAN_POINT('Ctrl Pts',(0.00593261942869252,-0.0336938721132427,
0.0794663075707078));
#105185=CARTESIAN_POINT('Ctrl Pts',(0.0058213272877974,-0.0335278710435083,
0.0794204375393264));
#105186=CARTESIAN_POINT('Ctrl Pts',(0.00571151277147702,-0.033362046922432,
0.0793710935523126));
#105187=CARTESIAN_POINT('Ctrl Pts',(0.00560312947353661,-0.0331951640388602,
0.0793182328037582));
#105188=CARTESIAN_POINT('Ctrl Pts',(0.00600988835631474,-0.0336938721132427,
0.0794988274515099));
#105189=CARTESIAN_POINT('Ctrl Pts',(0.00589791544082033,-0.0335278710435083,
0.0794545749759726));
#105190=CARTESIAN_POINT('Ctrl Pts',(0.00578736966326488,-0.033362046922432,
0.079406826626836));
#105191=CARTESIAN_POINT('Ctrl Pts',(0.00567820398836994,-0.0331951640388602,
0.0793555402701131));
#105192=CARTESIAN_POINT('Ctrl Pts',(0.00556498107437625,-0.0330240426238155,
0.0792991569809753));
#105193=CARTESIAN_POINT('Ctrl Pts',(0.00549404642038312,-0.0329142774063509,
0.0792639070026458));
#105194=CARTESIAN_POINT('Ctrl Pts',(0.00542380511839599,-0.0328043479726686,
0.0792271730334723));
#105195=CARTESIAN_POINT('Ctrl Pts',(0.0053543484487492,-0.0326943950436594,
0.0791889996542524));
#105196=CARTESIAN_POINT('Ctrl Pts',(0.00559876263038315,-0.0330240426238155,
0.0794073232532546));
#105197=CARTESIAN_POINT('Ctrl Pts',(0.00552633788060809,-0.0329142774063509,
0.0793725386487708));
#105198=CARTESIAN_POINT('Ctrl Pts',(0.00545459611939459,-0.0328043479726686,
0.0793362394810067));
#105199=CARTESIAN_POINT('Ctrl Pts',(0.00538363053393696,-0.0326943950436594,
0.0792984697208099));
#105200=CARTESIAN_POINT('Ctrl Pts',(0.00563254418639006,-0.0330240426238155,
0.0795154895255338));
#105201=CARTESIAN_POINT('Ctrl Pts',(0.00555862934083307,-0.0329142774063509,
0.0794811702948958));
#105202=CARTESIAN_POINT('Ctrl Pts',(0.00548538712039319,-0.0328043479726686,
0.0794453059285411));
#105203=CARTESIAN_POINT('Ctrl Pts',(0.00541291261912473,-0.0326943950436594,
0.0794079397873673));
#105204=CARTESIAN_POINT('Ctrl Pts',(0.00566632574239696,-0.0330240426238155,
0.079623655797813));
#105205=CARTESIAN_POINT('Ctrl Pts',(0.00559092080105804,-0.0329142774063509,
0.0795898019410208));
#105206=CARTESIAN_POINT('Ctrl Pts',(0.00551617812139179,-0.0328043479726686,
0.0795543723760755));
#105207=CARTESIAN_POINT('Ctrl Pts',(0.0054421947043125,-0.0326943950436594,
0.0795174098539247));
#105208=CARTESIAN_POINT('Origin',(0.0135101367001887,-0.0326396682855018,
0.0645017421403));
#105209=CARTESIAN_POINT('Ctrl Pts',(0.00513265640034573,-0.0331951640388587,
0.0793512658547611));
#105210=CARTESIAN_POINT('Ctrl Pts',(0.00506101948527155,-0.0330855618255041,
0.079310069147964));
#105211=CARTESIAN_POINT('Ctrl Pts',(0.0049901823936565,-0.0329757224427708,
0.0792673621304551));
#105212=CARTESIAN_POINT('Ctrl Pts',(0.00492023851925387,-0.0328657862078596,
0.079223195041563));
#105213=CARTESIAN_POINT('Ctrl Pts',(0.00524007188253915,-0.0331951640388587,
0.0793151678461617));
#105214=CARTESIAN_POINT('Ctrl Pts',(0.00516893214450775,-0.0330855618255041,
0.0792754505703321));
#105215=CARTESIAN_POINT('Ctrl Pts',(0.00509856201103423,-0.0329757224427708,
0.0792342343260914));
#105216=CARTESIAN_POINT('Ctrl Pts',(0.0050290541842623,-0.0328657862078596,
0.0791915674730752));
#105217=CARTESIAN_POINT('Ctrl Pts',(0.00534748736473257,-0.0331951640388587,
0.0792790698375624));
#105218=CARTESIAN_POINT('Ctrl Pts',(0.00527684480374394,-0.0330855618255041,
0.0792408319927003));
#105219=CARTESIAN_POINT('Ctrl Pts',(0.00520694162841195,-0.0329757224427708,
0.0792011065217278));
#105220=CARTESIAN_POINT('Ctrl Pts',(0.00513786984927074,-0.0328657862078596,
0.0791599399045873));
#105221=CARTESIAN_POINT('Ctrl Pts',(0.00545490284692598,-0.0331951640388587,
0.0792429718289631));
#105222=CARTESIAN_POINT('Ctrl Pts',(0.00538475746298014,-0.0330855618255041,
0.0792062134150684));
#105223=CARTESIAN_POINT('Ctrl Pts',(0.00531532124578968,-0.0329757224427708,
0.0791679787173641));
#105224=CARTESIAN_POINT('Ctrl Pts',(0.00524668551427917,-0.0328657862078596,
0.0791283123360995));
#105225=CARTESIAN_POINT('Origin',(0.0139098985521678,-0.0326401908831938,
0.0647690684078328));
#105226=CARTESIAN_POINT('Ctrl Pts',(0.00548500889272825,-0.0332451089994433,
0.0792602837953681));
#105227=CARTESIAN_POINT('Ctrl Pts',(0.00529227138603548,-0.0329451141710259,
0.0791607608320634));
#105228=CARTESIAN_POINT('Ctrl Pts',(0.00510757790270678,-0.0326442513127503,
0.0790470028260727));
#105229=CARTESIAN_POINT('Ctrl Pts',(0.00570958312786032,-0.0332451089994433,
0.0793701310207078));
#105230=CARTESIAN_POINT('Ctrl Pts',(0.00551270266528155,-0.0329451141710259,
0.0792790780132568));
#105231=CARTESIAN_POINT('Ctrl Pts',(0.00532324000406695,-0.0326442513127503,
0.0791734538364954));
#105232=CARTESIAN_POINT('Ctrl Pts',(0.00524671281819513,-0.0325229783203385,
0.0791283282193173));
#105233=CARTESIAN_POINT('Ctrl Pts',(0.00517808667380982,-0.0324130253112079,
0.0790886678816234));
#105234=CARTESIAN_POINT('Ctrl Pts',(0.00511029136294131,-0.0323031222247694,
0.0790475939392694));
#105235=CARTESIAN_POINT('Ctrl Pts',(0.00504341187002752,-0.0321934096636184,
0.0790051620693853));
#105236=CARTESIAN_POINT('Ctrl Pts',(0.00527363592220037,-0.0325229783203385,
0.0792384022358722));
#105237=CARTESIAN_POINT('Ctrl Pts',(0.00520349240993164,-0.0324130253112079,
0.0791991130325715));
#105238=CARTESIAN_POINT('Ctrl Pts',(0.00513417228392672,-0.0323031222247694,
0.0791583787796175));
#105239=CARTESIAN_POINT('Ctrl Pts',(0.00506576249715715,-0.0321934096636184,
0.0791162547879437));
#105240=CARTESIAN_POINT('Ctrl Pts',(0.00530055902620562,-0.0325229783203385,
0.0793484762524271));
#105241=CARTESIAN_POINT('Ctrl Pts',(0.00522889814605345,-0.0324130253112079,
0.0793095581835195));
#105242=CARTESIAN_POINT('Ctrl Pts',(0.00515805320491213,-0.0323031222247694,
0.0792691636199657));
#105243=CARTESIAN_POINT('Ctrl Pts',(0.00508811312428678,-0.0321934096636184,
0.0792273475065022));
#105244=CARTESIAN_POINT('Ctrl Pts',(0.00532748213021086,-0.0325229783203385,
0.0794585502689819));
#105245=CARTESIAN_POINT('Ctrl Pts',(0.00525430388217526,-0.0324130253112079,
0.0794200033344676));
#105246=CARTESIAN_POINT('Ctrl Pts',(0.00518193412589754,-0.0323031222247694,
0.0793799484603138));
#105247=CARTESIAN_POINT('Ctrl Pts',(0.00511046375141641,-0.0321934096636184,
0.0793384402250607));
#105248=CARTESIAN_POINT('Origin',(0.0135057741594412,-0.0326393375177481,
0.0645090673885528));
#105249=CARTESIAN_POINT('Ctrl Pts',(0.00481196851860963,-0.0326943950436593,
0.0791531880022078));
#105250=CARTESIAN_POINT('Ctrl Pts',(0.00474301521096575,-0.0325844576448127,
0.0791075450027729));
#105251=CARTESIAN_POINT('Ctrl Pts',(0.00467500099545019,-0.0324744968375319,
0.0790604727056596));
#105252=CARTESIAN_POINT('Ctrl Pts',(0.00460801218396164,-0.0323646534831895,
0.0790120326246146));
#105253=CARTESIAN_POINT('Ctrl Pts',(0.00492143854934795,-0.0326943950436593,
0.0791239059266012));
#105254=CARTESIAN_POINT('Ctrl Pts',(0.00485288880358638,-0.0325844576448127,
0.0790797716293587));
#105255=CARTESIAN_POINT('Ctrl Pts',(0.00478524697607894,-0.0324744968375319,
0.0790342164875322));
#105256=CARTESIAN_POINT('Ctrl Pts',(0.00471859892841089,-0.0323646534831895,
0.0789873000644197));
#105257=CARTESIAN_POINT('Ctrl Pts',(0.00503090858008626,-0.0326943950436593,
0.0790946238509947));
#105258=CARTESIAN_POINT('Ctrl Pts',(0.00496276239620701,-0.0325844576448127,
0.0790519982559444));
#105259=CARTESIAN_POINT('Ctrl Pts',(0.0048954929567077,-0.0324744968375319,
0.0790079602694048));
#105260=CARTESIAN_POINT('Ctrl Pts',(0.00482918567286014,-0.0323646534831895,
0.0789625675042249));
#105261=CARTESIAN_POINT('Ctrl Pts',(0.00514037861082458,-0.0326943950436593,
0.0790653417753881));
#105262=CARTESIAN_POINT('Ctrl Pts',(0.00507263598882764,-0.0325844576448127,
0.0790242248825302));
#105263=CARTESIAN_POINT('Ctrl Pts',(0.00500573893733646,-0.0324744968375319,
0.0789817040512773));
#105264=CARTESIAN_POINT('Ctrl Pts',(0.00493977241730939,-0.0323646534831895,
0.0789378349440301));
#105265=CARTESIAN_POINT('Origin',(0.0139293728226059,-0.0326395579066818,
0.0647366228438751));
#105266=CARTESIAN_POINT('Ctrl Pts',(0.00516937218723801,-0.0327445246961877,
0.0790845300198918));
#105267=CARTESIAN_POINT('Ctrl Pts',(0.00498326334700908,-0.0324436878365475,
0.0789731026260901));
#105268=CARTESIAN_POINT('Ctrl Pts',(0.00480607638895177,-0.0321434074463188,
0.0788479733074025));
#105269=CARTESIAN_POINT('Ctrl Pts',(0.00538660675589261,-0.0327445246961877,
0.0792082601382198));
#105270=CARTESIAN_POINT('Ctrl Pts',(0.00519583135801167,-0.0324436878365475,
0.0791050258800291));
#105271=CARTESIAN_POINT('Ctrl Pts',(0.00501337395904593,-0.0321434074463188,
0.0789877149169289));
#105272=CARTESIAN_POINT('Ctrl Pts',(0.00486075314664532,-0.0322357242816073,
0.0788861130098361));
#105273=CARTESIAN_POINT('Ctrl Pts',(0.00470991408979555,-0.0319819883628706,
0.0787821897666999));
#105274=CARTESIAN_POINT('Ctrl Pts',(0.0045659936602703,-0.0317295851069886,
0.0786688788162117));
#105275=CARTESIAN_POINT('Ctrl Pts',(0.00506965652642701,-0.0322357242816073,
0.0790234424601218));
#105276=CARTESIAN_POINT('Ctrl Pts',(0.00491444370469541,-0.0319819883628706,
0.078926172518694));
#105277=CARTESIAN_POINT('Ctrl Pts',(0.00476573500564448,-0.0317295851069886,
0.0788192230710009));
#105278=CARTESIAN_POINT('Origin',(0.0138779033429583,-0.032637194264591,
0.0648168306758043));
#105279=CARTESIAN_POINT('Origin',(0.0134434215129649,-0.032635298552763,
0.0646147837559969));
#105280=CARTESIAN_POINT('Ctrl Pts',(0.00450435085242233,-0.0321934096636183,
0.0789353648523491));
#105281=CARTESIAN_POINT('Ctrl Pts',(0.00443835694162196,-0.0320835708272304,
0.0788854500733479));
#105282=CARTESIAN_POINT('Ctrl Pts',(0.00437343429372893,-0.0319739230346346,
0.078834198506393));
#105283=CARTESIAN_POINT('Ctrl Pts',(0.00430966094023589,-0.0318646057455576,
0.0787816820992405));
#105284=CARTESIAN_POINT('Ctrl Pts',(0.00461544366664279,-0.0321934096636183,
0.0789130142059733));
#105285=CARTESIAN_POINT('Ctrl Pts',(0.00454975798867498,-0.0320835708272304,
0.0788646314834606));
#105286=CARTESIAN_POINT('Ctrl Pts',(0.00448511168899753,-0.0319739230346346,
0.0788149174632018));
#105287=CARTESIAN_POINT('Ctrl Pts',(0.00442158259651064,-0.0318646057455576,
0.078763942098633));
#105288=CARTESIAN_POINT('Ctrl Pts',(0.00472653648086325,-0.0321934096636183,
0.0788906635595975));
#105289=CARTESIAN_POINT('Ctrl Pts',(0.004661159035728,-0.0320835708272304,
0.0788438128935734));
#105290=CARTESIAN_POINT('Ctrl Pts',(0.00459678908426614,-0.0319739230346346,
0.0787956364200106));
#105291=CARTESIAN_POINT('Ctrl Pts',(0.00453350425278539,-0.0318646057455576,
0.0787462020980255));
#105292=CARTESIAN_POINT('Ctrl Pts',(0.00483762929508372,-0.0321934096636183,
0.0788683129132217));
#105293=CARTESIAN_POINT('Ctrl Pts',(0.00477256008278102,-0.0320835708272304,
0.0788229943036862));
#105294=CARTESIAN_POINT('Ctrl Pts',(0.00470846647953474,-0.0319739230346346,
0.0787763553768194));
#105295=CARTESIAN_POINT('Ctrl Pts',(0.00464542590906015,-0.0318646057455576,
0.078728462097418));
#105296=CARTESIAN_POINT('Ctrl Pts',(0.0049397053886744,-0.0320218834582375,
0.0789387840527528));
#105297=CARTESIAN_POINT('Ctrl Pts',(0.00488986572349503,-0.0319391099350648,
0.0789056455106741));
#105298=CARTESIAN_POINT('Ctrl Pts',(0.00484057371788366,-0.0318564869454906,
0.0788717487930358));
#105299=CARTESIAN_POINT('Ctrl Pts',(0.00479186296961419,-0.0317740741446476,
0.0788371219408657));
#105300=CARTESIAN_POINT('Ctrl Pts',(0.00494843231451724,-0.0320218834582375,
0.0789875761506071));
#105301=CARTESIAN_POINT('Ctrl Pts',(0.00489808484155334,-0.0319391099350648,
0.0789545284347292));
#105302=CARTESIAN_POINT('Ctrl Pts',(0.00484828391756141,-0.0318564869454906,
0.0789207145587727));
#105303=CARTESIAN_POINT('Ctrl Pts',(0.00479906351662797,-0.0317740741446476,
0.0788861625380316));
#105304=CARTESIAN_POINT('Ctrl Pts',(0.00495715924036009,-0.0320218834582375,
0.0790363682484614));
#105305=CARTESIAN_POINT('Ctrl Pts',(0.00490630395961165,-0.0319391099350648,
0.0790034113587843));
#105306=CARTESIAN_POINT('Ctrl Pts',(0.00485599411723916,-0.0318564869454906,
0.0789696803245095));
#105307=CARTESIAN_POINT('Ctrl Pts',(0.00480626406364174,-0.0317740741446476,
0.0789352031351975));
#105308=CARTESIAN_POINT('Ctrl Pts',(0.00496588616620294,-0.0320218834582375,
0.0790851603463157));
#105309=CARTESIAN_POINT('Ctrl Pts',(0.00491452307766996,-0.0319391099350648,
0.0790522942828394));
#105310=CARTESIAN_POINT('Ctrl Pts',(0.00486370431691691,-0.0318564869454906,
0.0790186460902464));
#105311=CARTESIAN_POINT('Ctrl Pts',(0.00481346461065551,-0.0317740741446476,
0.0789842437323634));
#105312=CARTESIAN_POINT('Origin',(0.00224101653788164,-0.0391228853390896,
0.0846986343464964));
#105313=CARTESIAN_POINT('Ctrl Pts',(0.00782094450061722,-0.0352722978779661,
0.0798939058030755));
#105314=CARTESIAN_POINT('Ctrl Pts',(0.00780209548830728,-0.0352466642097262,
0.0798925614024518));
#105315=CARTESIAN_POINT('Ctrl Pts',(0.0077832576905389,-0.0352210183808323,
0.0798912964018642));
#105316=CARTESIAN_POINT('Ctrl Pts',(0.00776443040686705,-0.0351953608940152,
0.079890111287996));
#105317=CARTESIAN_POINT('Origin',(0.00729188564518976,-0.0352456003065119,
0.0847652341560871));
#105318=CARTESIAN_POINT('Ctrl Pts',(0.00764020000161069,-0.035024121149334,
0.0798795225284857));
#105319=CARTESIAN_POINT('Ctrl Pts',(0.00756127818153511,-0.0349144232867422,
0.0798728613823746));
#105320=CARTESIAN_POINT('Ctrl Pts',(0.00748244681359192,-0.0348045283677512,
0.0798645648789048));
#105321=CARTESIAN_POINT('Ctrl Pts',(0.00740380726618409,-0.0346945769586886,
0.0798546398874039));
#105322=CARTESIAN_POINT('Ctrl Pts',(0.00771142797260723,-0.035024121149334,
0.0799676571865457));
#105323=CARTESIAN_POINT('Ctrl Pts',(0.00763129213380823,-0.0349144232867422,
0.0799619771764862));
#105324=CARTESIAN_POINT('Ctrl Pts',(0.00755122573971058,-0.0348045283677512,
0.0799546373016919));
#105325=CARTESIAN_POINT('Ctrl Pts',(0.00747133169503169,-0.0346945769586886,
0.079945643147304));
#105326=CARTESIAN_POINT('Ctrl Pts',(0.00778265594360378,-0.035024121149334,
0.0800557918446057));
#105327=CARTESIAN_POINT('Ctrl Pts',(0.00770130608608136,-0.0349144232867422,
0.0800510929705979));
#105328=CARTESIAN_POINT('Ctrl Pts',(0.00762000466582925,-0.0348045283677512,
0.080044709724479));
#105329=CARTESIAN_POINT('Ctrl Pts',(0.00753885612387928,-0.0346945769586886,
0.0800366464072041));
#105330=CARTESIAN_POINT('Ctrl Pts',(0.00785388391460032,-0.035024121149334,
0.0801439265026657));
#105331=CARTESIAN_POINT('Ctrl Pts',(0.00777132003835448,-0.0349144232867422,
0.0801402087647095));
#105332=CARTESIAN_POINT('Ctrl Pts',(0.00768878359194791,-0.0348045283677512,
0.0801347821472661));
#105333=CARTESIAN_POINT('Ctrl Pts',(0.00760638055272687,-0.0346945769586886,
0.0801276496671042));
#105334=CARTESIAN_POINT('Origin',(0.00968455939246014,-0.0345629067942544,
0.0632215067238589));
#105335=CARTESIAN_POINT('Ctrl Pts',(0.0073297150359876,-0.0351970973651594,
0.0800274976926647));
#105336=CARTESIAN_POINT('Ctrl Pts',(0.00724829027087589,-0.0350869349321761,
0.0800164969683543));
#105337=CARTESIAN_POINT('Ctrl Pts',(0.00716702675339849,-0.0349764985129721,
0.0800037943554284));
#105338=CARTESIAN_POINT('Ctrl Pts',(0.00708603073156119,-0.0348659306849651,
0.0799894001131411));
#105339=CARTESIAN_POINT('Ctrl Pts',(0.0073925256199172,-0.0351970973651594,
0.0799744382807117));
#105340=CARTESIAN_POINT('Ctrl Pts',(0.00731183592104986,-0.0350869349321761,
0.0799643077119182));
#105341=CARTESIAN_POINT('Ctrl Pts',(0.00723128998868617,-0.0349764985129722,
0.0799524912569559));
#105342=CARTESIAN_POINT('Ctrl Pts',(0.00715099307359876,-0.0348659306849651,
0.0799389980817598));
#105343=CARTESIAN_POINT('Ctrl Pts',(0.00745533620384681,-0.0351970973651595,
0.0799213788687587));
#105344=CARTESIAN_POINT('Ctrl Pts',(0.00737538157122384,-0.0350869349321761,
0.0799121184554822));
#105345=CARTESIAN_POINT('Ctrl Pts',(0.00729555322397385,-0.0349764985129722,
0.0799011881584834));
#105346=CARTESIAN_POINT('Ctrl Pts',(0.00721595541563633,-0.0348659306849651,
0.0798885960503785));
#105347=CARTESIAN_POINT('Ctrl Pts',(0.00751814678777641,-0.0351970973651595,
0.0798683194568057));
#105348=CARTESIAN_POINT('Ctrl Pts',(0.00743892722139781,-0.0350869349321762,
0.0798599291990462));
#105349=CARTESIAN_POINT('Ctrl Pts',(0.00735981645926153,-0.0349764985129722,
0.0798498850600108));
#105350=CARTESIAN_POINT('Ctrl Pts',(0.0072809177576739,-0.0348659306849651,
0.0798381940189971));
#105351=CARTESIAN_POINT('Origin',(0.0101521302129177,-0.0345637187967259,
0.0633342137964626));
#105352=CARTESIAN_POINT('Ctrl Pts',(0.00755152776053585,-0.0352450361861252,
0.0798728183497645));
#105353=CARTESIAN_POINT('Ctrl Pts',(0.00733568813026428,-0.0349452761023764,
0.079851235420236));
#105354=CARTESIAN_POINT('Ctrl Pts',(0.00712208739215075,-0.0346444289983475,
0.0798134558818566));
#105355=CARTESIAN_POINT('Ctrl Pts',(0.00780076904397632,-0.0352450361861252,
0.0798922806884972));
#105356=CARTESIAN_POINT('Ctrl Pts',(0.0075841953795734,-0.0349452761023764,
0.0798800980479834));
#105357=CARTESIAN_POINT('Ctrl Pts',(0.00736915462442884,-0.0346444289983475,
0.0798516368029356));
#105358=CARTESIAN_POINT('Ctrl Pts',(0.00728139549856233,-0.0345231616327822,
0.0798378524435754));
#105359=CARTESIAN_POINT('Ctrl Pts',(0.00720299646048385,-0.0344132092796975,
0.0798262413289768));
#105360=CARTESIAN_POINT('Ctrl Pts',(0.00712484163418209,-0.0343032738558974,
0.0798130091911959));
#105361=CARTESIAN_POINT('Ctrl Pts',(0.00704703071079267,-0.0341934961088741,
0.0797981755468794));
#105362=CARTESIAN_POINT('Ctrl Pts',(0.00734694889680335,-0.0345231616327822,
0.0799302855984397));
#105363=CARTESIAN_POINT('Ctrl Pts',(0.00726727579782055,-0.0344132092796975,
0.079919578045144));
#105364=CARTESIAN_POINT('Ctrl Pts',(0.00718782828689733,-0.0343032738558974,
0.0799072230691017));
#105365=CARTESIAN_POINT('Ctrl Pts',(0.00710870774003284,-0.0341934961088741,
0.0798932391056347));
#105366=CARTESIAN_POINT('Ctrl Pts',(0.00741250229504438,-0.0345231616327822,
0.080022718753304));
#105367=CARTESIAN_POINT('Ctrl Pts',(0.00733155513515725,-0.0344132092796975,
0.0800129147613113));
#105368=CARTESIAN_POINT('Ctrl Pts',(0.00725081493961256,-0.0343032738558974,
0.0800014369470074));
#105369=CARTESIAN_POINT('Ctrl Pts',(0.00717038476927302,-0.0341934961088741,
0.07998830266439));
#105370=CARTESIAN_POINT('Ctrl Pts',(0.0074780556932854,-0.0345231616327822,
0.0801151519081683));
#105371=CARTESIAN_POINT('Ctrl Pts',(0.00739583447249395,-0.0344132092796975,
0.0801062514774786));
#105372=CARTESIAN_POINT('Ctrl Pts',(0.00731380159232779,-0.0343032738558974,
0.0800956508249132));
#105373=CARTESIAN_POINT('Ctrl Pts',(0.0072320617985132,-0.0341934961088741,
0.0800833662231453));
#105374=CARTESIAN_POINT('Origin',(0.00968602227619365,-0.0345625596230275,
0.0632094918065127));
#105375=CARTESIAN_POINT('Ctrl Pts',(0.00688633205822454,-0.0346945769586889,
0.0800210064864324));
#105376=CARTESIAN_POINT('Ctrl Pts',(0.00680542662135271,-0.0345846629176054,
0.080003953798107));
#105377=CARTESIAN_POINT('Ctrl Pts',(0.0067248600082248,-0.0344746925050312,
0.0799852251059319));
#105378=CARTESIAN_POINT('Ctrl Pts',(0.00664473535096407,-0.0343648066253259,
0.0799648448335961));
#105379=CARTESIAN_POINT('Ctrl Pts',(0.00697733524647039,-0.0346945769586889,
0.0799534821107523));
#105380=CARTESIAN_POINT('Ctrl Pts',(0.00689736032962549,-0.0345846629176054,
0.0799376834923582));
#105381=CARTESIAN_POINT('Ctrl Pts',(0.00681769846180846,-0.0344746925050312,
0.0799202283270848));
#105382=CARTESIAN_POINT('Ctrl Pts',(0.00673845162261766,-0.0343648066253259,
0.0799011394020439));
#105383=CARTESIAN_POINT('Ctrl Pts',(0.00706833843471624,-0.0346945769586889,
0.0798859577350721));
#105384=CARTESIAN_POINT('Ctrl Pts',(0.00698929403789827,-0.0345846629176054,
0.0798714131866095));
#105385=CARTESIAN_POINT('Ctrl Pts',(0.00691053691539213,-0.0344746925050312,
0.0798552315482378));
#105386=CARTESIAN_POINT('Ctrl Pts',(0.00683216789427126,-0.0343648066253259,
0.0798374339704917));
#105387=CARTESIAN_POINT('Ctrl Pts',(0.00715934162296208,-0.0346945769586889,
0.079818433359392));
#105388=CARTESIAN_POINT('Ctrl Pts',(0.00708122774617106,-0.0345846629176054,
0.0798051428808608));
#105389=CARTESIAN_POINT('Ctrl Pts',(0.0070033753689758,-0.0344746925050312,
0.0797902347693907));
#105390=CARTESIAN_POINT('Ctrl Pts',(0.00692588416592485,-0.0343648066253259,
0.0797737285389395));
#105391=CARTESIAN_POINT('Origin',(0.0101621341310956,-0.0345626446731115,
0.0632766459900518));
#105392=CARTESIAN_POINT('Ctrl Pts',(0.00715771327076763,-0.0346945769586885,
0.0798196415968991));
#105393=CARTESIAN_POINT('Ctrl Pts',(0.00703896035752182,-0.0345275153362891,
0.0797994068965281));
#105394=CARTESIAN_POINT('Ctrl Pts',(0.00692081309139195,-0.0343603235965159,
0.0797754322926102));
#105395=CARTESIAN_POINT('Ctrl Pts',(0.0068036198456941,-0.034193496108874,
0.0797477938847791));
#105396=CARTESIAN_POINT('Ctrl Pts',(0.00724064200962563,-0.0346945769586885,
0.0798319238036506));
#105397=CARTESIAN_POINT('Ctrl Pts',(0.00712163184064189,-0.0345275153362891,
0.0798134260789179));
#105398=CARTESIAN_POINT('Ctrl Pts',(0.00700317262594953,-0.0343603235965159,
0.0797911808094528));
#105399=CARTESIAN_POINT('Ctrl Pts',(0.00688561373748634,-0.034193496108874,
0.079765258993998));
#105400=CARTESIAN_POINT('Ctrl Pts',(0.00732357074848363,-0.0346945769586885,
0.0798442060104022));
#105401=CARTESIAN_POINT('Ctrl Pts',(0.00720430332376196,-0.0345275153362891,
0.0798274452613076));
#105402=CARTESIAN_POINT('Ctrl Pts',(0.00708553216050711,-0.0343603235965159,
0.0798069293262955));
#105403=CARTESIAN_POINT('Ctrl Pts',(0.00696760762927858,-0.034193496108874,
0.079782724103217));
#105404=CARTESIAN_POINT('Ctrl Pts',(0.00740649948734163,-0.0346945769586885,
0.0798564882171538));
#105405=CARTESIAN_POINT('Ctrl Pts',(0.00728697480688202,-0.0345275153362891,
0.0798414644436974));
#105406=CARTESIAN_POINT('Ctrl Pts',(0.00716789169506468,-0.0343603235965159,
0.0798226778431382));
#105407=CARTESIAN_POINT('Ctrl Pts',(0.00704960152107082,-0.034193496108874,
0.0798001892124359));
#105408=CARTESIAN_POINT('Ctrl Pts',(0.00692591514389262,-0.0340223579322365,
0.0797737345681123));
#105409=CARTESIAN_POINT('Ctrl Pts',(0.00684834917688344,-0.0339125849573552,
0.0797572128573353));
#105410=CARTESIAN_POINT('Ctrl Pts',(0.00677117967560313,-0.0338030433565217,
0.0797390973208946));
#105411=CARTESIAN_POINT('Ctrl Pts',(0.00669450327320398,-0.0336938721132321,
0.0797194198736759));
#105412=CARTESIAN_POINT('Ctrl Pts',(0.00698553537854258,-0.0340223579322365,
0.0798701016135747));
#105413=CARTESIAN_POINT('Ctrl Pts',(0.00690664025864068,-0.0339125849573552,
0.0798544022213296));
#105414=CARTESIAN_POINT('Ctrl Pts',(0.0068281255183652,-0.0338030433565217,
0.0798370809152107));
#105415=CARTESIAN_POINT('Ctrl Pts',(0.00675008960123868,-0.0336938721132321,
0.0798181687469174));
#105416=CARTESIAN_POINT('Ctrl Pts',(0.00704515561319254,-0.0340223579322365,
0.079966468659037));
#105417=CARTESIAN_POINT('Ctrl Pts',(0.00696493134039792,-0.0339125849573552,
0.0799515915853239));
#105418=CARTESIAN_POINT('Ctrl Pts',(0.00688507136112726,-0.0338030433565217,
0.0799350645095268));
#105419=CARTESIAN_POINT('Ctrl Pts',(0.00680567592927338,-0.0336938721132321,
0.079916917620159));
#105420=CARTESIAN_POINT('Ctrl Pts',(0.0071047758478425,-0.0340223579322365,
0.0800628357044994));
#105421=CARTESIAN_POINT('Ctrl Pts',(0.00702322242215516,-0.0339125849573552,
0.0800487809493182));
#105422=CARTESIAN_POINT('Ctrl Pts',(0.00694201720388932,-0.0338030433565217,
0.0800330481038429));
#105423=CARTESIAN_POINT('Ctrl Pts',(0.00686126225730807,-0.0336938721132321,
0.0800156664934005));
#105424=CARTESIAN_POINT('Origin',(0.00966646514550984,-0.0345589643415296,
0.0633281105098358));
#105425=CARTESIAN_POINT('Ctrl Pts',(0.0065201303359547,-0.034193496108874,
0.0799317212593736));
#105426=CARTESIAN_POINT('Ctrl Pts',(0.00644040382358729,-0.0340836138581107,
0.0799096078499084));
#105427=CARTESIAN_POINT('Ctrl Pts',(0.00636117315610799,-0.0339738896643499,
0.0798858552779883));
#105428=CARTESIAN_POINT('Ctrl Pts',(0.00628253770110186,-0.0338644633294062,
0.0798605007416777));
#105429=CARTESIAN_POINT('Ctrl Pts',(0.00661519398024474,-0.034193496108874,
0.0798700441746387));
#105430=CARTESIAN_POINT('Ctrl Pts',(0.00653631795835211,-0.0340836138581107,
0.0798492416365338));
#105431=CARTESIAN_POINT('Ctrl Pts',(0.00645791024753404,-0.0339738896643499,
0.079826816906109));
#105432=CARTESIAN_POINT('Ctrl Pts',(0.00638006927601672,-0.0338644633294062,
0.0798028054113491));
#105433=CARTESIAN_POINT('Ctrl Pts',(0.00671025762453478,-0.034193496108874,
0.0798083670899038));
#105434=CARTESIAN_POINT('Ctrl Pts',(0.00663223209311692,-0.0340836138581107,
0.0797888754231592));
#105435=CARTESIAN_POINT('Ctrl Pts',(0.00655464733896009,-0.0339738896643499,
0.0797677785342298));
#105436=CARTESIAN_POINT('Ctrl Pts',(0.00647760085093159,-0.0338644633294062,
0.0797451100810205));
#105437=CARTESIAN_POINT('Ctrl Pts',(0.00680532126882482,-0.034193496108874,
0.0797466900051689));
#105438=CARTESIAN_POINT('Ctrl Pts',(0.00672814622788174,-0.0340836138581107,
0.0797285092097846));
#105439=CARTESIAN_POINT('Ctrl Pts',(0.00665138443038615,-0.0339738896643499,
0.0797087401623506));
#105440=CARTESIAN_POINT('Ctrl Pts',(0.00657513242584646,-0.0338644633294062,
0.0796874147506919));
#105441=CARTESIAN_POINT('Origin',(0.0101471443791771,-0.0345610621862551,
0.0633504149063426));
#105442=CARTESIAN_POINT('Ctrl Pts',(0.00683885734612616,-0.03424362768739,
0.0797559872580669));
#105443=CARTESIAN_POINT('Ctrl Pts',(0.00662742405117035,-0.033943005420186,
0.079707525518562));
#105444=CARTESIAN_POINT('Ctrl Pts',(0.00642024175282514,-0.0336441434784162,
0.0796432754316819));
#105445=CARTESIAN_POINT('Ctrl Pts',(0.00708369469966236,-0.03424362768739,
0.079806531004598));
#105446=CARTESIAN_POINT('Ctrl Pts',(0.00687035511588059,-0.033943005420186,
0.0797673034581091));
#105447=CARTESIAN_POINT('Ctrl Pts',(0.00666057638702226,-0.0336441434784162,
0.0797121177413856));
#105448=CARTESIAN_POINT('Ctrl Pts',(0.00657515916624883,-0.0335235895815127,
0.0796874220977052));
#105449=CARTESIAN_POINT('Ctrl Pts',(0.00649892564889411,-0.0334144449262719,
0.0796661022527825));
#105450=CARTESIAN_POINT('Ctrl Pts',(0.00642304500041502,-0.0333049234473133,
0.0796431829868447));
#105451=CARTESIAN_POINT('Ctrl Pts',(0.00634761690359244,-0.0331951640388588,
0.0796186848173753));
#105452=CARTESIAN_POINT('Ctrl Pts',(0.00662861075628238,-0.0335235895815127,
0.0797873425661274));
#105453=CARTESIAN_POINT('Ctrl Pts',(0.00655100163695455,-0.0334144449262719,
0.079766758587578));
#105454=CARTESIAN_POINT('Ctrl Pts',(0.00647372860365686,-0.0333049234473133,
0.0797445476145333));
#105455=CARTESIAN_POINT('Ctrl Pts',(0.00639689303756167,-0.0331951640388588,
0.0797207290975084));
#105456=CARTESIAN_POINT('Ctrl Pts',(0.00668206234631593,-0.0335235895815127,
0.0798872630345496));
#105457=CARTESIAN_POINT('Ctrl Pts',(0.00660307762501498,-0.0334144449262719,
0.0798674149223736));
#105458=CARTESIAN_POINT('Ctrl Pts',(0.0065244122068987,-0.0333049234473133,
0.0798459122422219));
#105459=CARTESIAN_POINT('Ctrl Pts',(0.0064461691715309,-0.0331951640388588,
0.0798227733776415));
#105460=CARTESIAN_POINT('Ctrl Pts',(0.00673551393634947,-0.0335235895815127,
0.0799871835029718));
#105461=CARTESIAN_POINT('Ctrl Pts',(0.00665515361307542,-0.0334144449262719,
0.0799680712571691));
#105462=CARTESIAN_POINT('Ctrl Pts',(0.00657509581014055,-0.0333049234473133,
0.0799472768699105));
#105463=CARTESIAN_POINT('Ctrl Pts',(0.00649544530550012,-0.0331951640388588,
0.0799248176577745));
#105464=CARTESIAN_POINT('Origin',(0.0122146855780136,-0.0326434571770428,
0.0640184173121102));
#105465=CARTESIAN_POINT('Ctrl Pts',(0.00615849062091358,-0.0336938721132461,
0.0798206128038202));
#105466=CARTESIAN_POINT('Ctrl Pts',(0.00612529864246142,-0.0336474569764994,
0.0798091093000944));
#105467=CARTESIAN_POINT('Ctrl Pts',(0.00609224360138026,-0.033601104548885,
0.0797972180305801));
#105468=CARTESIAN_POINT('Ctrl Pts',(0.00600855584080445,-0.0334837508643205,
0.0797671120714434));
#105469=CARTESIAN_POINT('Ctrl Pts',(0.00592579693167301,-0.0333660264760493,
0.0797345394908715));
#105470=CARTESIAN_POINT('Ctrl Pts',(0.00645473649829036,-0.0336938721132461,
0.0796538542375875));
#105471=CARTESIAN_POINT('Ctrl Pts',(0.0064225206130628,-0.0336474569764994,
0.0796440847592869));
#105472=CARTESIAN_POINT('Ctrl Pts',(0.00639042129936673,-0.033601104548885,
0.0796339388227849));
#105473=CARTESIAN_POINT('Ctrl Pts',(0.00630915322069004,-0.0334837508643205,
0.0796082516453673));
#105474=CARTESIAN_POINT('Ctrl Pts',(0.00622868199325349,-0.0333660264760493,
0.0795801676063));
#105475=CARTESIAN_POINT('Ctrl Pts',(0.00645473649829103,-0.0336938721132426,
0.0796538542375947));
#105476=CARTESIAN_POINT('Ctrl Pts',(0.00642252061306816,-0.0336474569765026,
0.0796440847592955));
#105477=CARTESIAN_POINT('Ctrl Pts',(0.00639042129937673,-0.0336011045488949,
0.0796339388227949));
#105478=CARTESIAN_POINT('Ctrl Pts',(0.00630983007310182,-0.0334847282606778,
0.0796084655845773));
#105479=CARTESIAN_POINT('Ctrl Pts',(0.00623002219053035,-0.0333679869945434,
0.0795806351426612));
#105480=CARTESIAN_POINT('Ctrl Pts',(0.00645473649828801,-0.0336938721132428,
0.0796538542375868));
#105481=CARTESIAN_POINT('Ctrl Pts',(0.00633951823577612,-0.0335278710435084,
0.0796189142597623));
#105482=CARTESIAN_POINT('Ctrl Pts',(0.00622543621540167,-0.033362046922432,
0.0795803733589849));
#105483=CARTESIAN_POINT('Ctrl Pts',(0.00611244011171198,-0.0331951640388602,
0.0795381933921867));
#105484=CARTESIAN_POINT('Ctrl Pts',(0.00653547195915288,-0.0336938721132428,
0.0796764333248627));
#105485=CARTESIAN_POINT('Ctrl Pts',(0.00641978102365716,-0.0335278710435084,
0.0796431834716532));
#105486=CARTESIAN_POINT('Ctrl Pts',(0.00630517349471564,-0.033362046922432,
0.0796063172780069));
#105487=CARTESIAN_POINT('Ctrl Pts',(0.00619159850696651,-0.0331951640388602,
0.0795657973463238));
#105488=CARTESIAN_POINT('Ctrl Pts',(0.00661620742001775,-0.0336938721132428,
0.0796990124121386));
#105489=CARTESIAN_POINT('Ctrl Pts',(0.0065000438115382,-0.0335278710435084,
0.079667452683544));
#105490=CARTESIAN_POINT('Ctrl Pts',(0.00638491077402962,-0.033362046922432,
0.0796322611970289));
#105491=CARTESIAN_POINT('Ctrl Pts',(0.00627075690222105,-0.0331951640388602,
0.0795934013004609));
#105492=CARTESIAN_POINT('Ctrl Pts',(0.00669694288088262,-0.0336938721132428,
0.0797215914994144));
#105493=CARTESIAN_POINT('Ctrl Pts',(0.00658030659941925,-0.0335278710435084,
0.0796917218954349));
#105494=CARTESIAN_POINT('Ctrl Pts',(0.00646464805334359,-0.033362046922432,
0.0796582051160508));
#105495=CARTESIAN_POINT('Ctrl Pts',(0.00634991529747558,-0.0331951640388602,
0.079621005254598));
#105496=CARTESIAN_POINT('Ctrl Pts',(0.00623051848003017,-0.0330240426238156,
0.0795792571584604));
#105497=CARTESIAN_POINT('Ctrl Pts',(0.00615572517320382,-0.0329142774063509,
0.0795531756062954));
#105498=CARTESIAN_POINT('Ctrl Pts',(0.00608143375772474,-0.0328043479726686,
0.0795255348649484));
#105499=CARTESIAN_POINT('Ctrl Pts',(0.0060077403816101,-0.0326943950436594,
0.079496367723225));
#105500=CARTESIAN_POINT('Ctrl Pts',(0.00627759048704541,-0.0330240426238156,
0.0796823365557261));
#105501=CARTESIAN_POINT('Ctrl Pts',(0.00620137716109633,-0.0329142774063509,
0.0796569034663178));
#105502=CARTESIAN_POINT('Ctrl Pts',(0.00612565161302665,-0.0328043479726686,
0.079629882155248));
#105503=CARTESIAN_POINT('Ctrl Pts',(0.0060505118062303,-0.0326943950436594,
0.0796013045671887));
#105504=CARTESIAN_POINT('Ctrl Pts',(0.00632466249406064,-0.0330240426238156,
0.0797854159529919));
#105505=CARTESIAN_POINT('Ctrl Pts',(0.00624702914898885,-0.0329142774063509,
0.0797606313263402));
#105506=CARTESIAN_POINT('Ctrl Pts',(0.00616986946832855,-0.0328043479726686,
0.0797342294455475));
#105507=CARTESIAN_POINT('Ctrl Pts',(0.00609328323085051,-0.0326943950436594,
0.0797062414111525));
#105508=CARTESIAN_POINT('Ctrl Pts',(0.00637173450107587,-0.0330240426238156,
0.0798884953502576));
#105509=CARTESIAN_POINT('Ctrl Pts',(0.00629268113688136,-0.0329142774063509,
0.0798643591863626));
#105510=CARTESIAN_POINT('Ctrl Pts',(0.00621408732363045,-0.0328043479726686,
0.0798385767358471));
#105511=CARTESIAN_POINT('Ctrl Pts',(0.00613605465547072,-0.0326943950436594,
0.0798111782551163));
#105512=CARTESIAN_POINT('Origin',(0.0122584163300697,-0.03263966828561,
0.0639027323079114));
#105513=CARTESIAN_POINT('Ctrl Pts',(0.00580813378883238,-0.0331951640388587,
0.079685139787558));
#105514=CARTESIAN_POINT('Ctrl Pts',(0.0057318984357554,-0.0330855618255041,
0.0796532464153077));
#105515=CARTESIAN_POINT('Ctrl Pts',(0.00565626730716548,-0.0329757224427707,
0.0796197543971362));
#105516=CARTESIAN_POINT('Ctrl Pts',(0.00558133935703579,-0.0328657862078596,
0.0795847018708791));
#105517=CARTESIAN_POINT('Ctrl Pts',(0.00591017798772229,-0.0331951640388587,
0.0796358636928203));
#105518=CARTESIAN_POINT('Ctrl Pts',(0.00583462131316559,-0.0330855618255041,
0.0796053757729759));
#105519=CARTESIAN_POINT('Ctrl Pts',(0.005759640304047,-0.0329757224427707,
0.0795733042475063));
#105520=CARTESIAN_POINT('Ctrl Pts',(0.00568533299259563,-0.0328657862078596,
0.0795396854760575));
#105521=CARTESIAN_POINT('Ctrl Pts',(0.0060122221866122,-0.0331951640388587,
0.0795865875980825));
#105522=CARTESIAN_POINT('Ctrl Pts',(0.00593734419057578,-0.0330855618255041,
0.0795575051306441));
#105523=CARTESIAN_POINT('Ctrl Pts',(0.00586301330092851,-0.0329757224427707,
0.0795268540978765));
#105524=CARTESIAN_POINT('Ctrl Pts',(0.00578932662815546,-0.0328657862078596,
0.0794946690812359));
#105525=CARTESIAN_POINT('Ctrl Pts',(0.00611426638550211,-0.0331951640388587,
0.0795373115033448));
#105526=CARTESIAN_POINT('Ctrl Pts',(0.00604006706798597,-0.0330855618255041,
0.0795096344883123));
#105527=CARTESIAN_POINT('Ctrl Pts',(0.00596638629781003,-0.0329757224427707,
0.0794804039482466));
#105528=CARTESIAN_POINT('Ctrl Pts',(0.0058933202637153,-0.0328657862078596,
0.0794496526864143));
#105529=CARTESIAN_POINT('Origin',(0.0126885308057799,-0.0326401908832882,
0.0641178471829243));
#105530=CARTESIAN_POINT('Ctrl Pts',(0.00614630480086988,-0.0332451089994433,
0.0795507136716536));
#105531=CARTESIAN_POINT('Ctrl Pts',(0.0059426135521804,-0.0329451141710259,
0.0794761318915836));
#105532=CARTESIAN_POINT('Ctrl Pts',(0.00574511877339838,-0.0326442513127503,
0.0793864191329318));
#105533=CARTESIAN_POINT('Ctrl Pts',(0.00638287570903076,-0.0332451089994433,
0.0796315481037475));
#105534=CARTESIAN_POINT('Ctrl Pts',(0.00617613573985519,-0.0329451141710259,
0.0795658887414571));
#105535=CARTESIAN_POINT('Ctrl Pts',(0.00597492882869792,-0.0326442513127503,
0.0794848434108475));
#105536=CARTESIAN_POINT('Ctrl Pts',(0.00589334934302681,-0.0325229783203385,
0.0794496650223003));
#105537=CARTESIAN_POINT('Ctrl Pts',(0.00582029357792018,-0.032413025311208,
0.0794189185547979));
#105538=CARTESIAN_POINT('Ctrl Pts',(0.00574788492331688,-0.0323031222247695,
0.0793866654982792));
#105539=CARTESIAN_POINT('Ctrl Pts',(0.0056762146717219,-0.0321934096636184,
0.0793529504394689));
#105540=CARTESIAN_POINT('Ctrl Pts',(0.00593385608274179,-0.0325229783203385,
0.0795554967126749));
#105541=CARTESIAN_POINT('Ctrl Pts',(0.0058593414301243,-0.032413025311208,
0.0795253086296835));
#105542=CARTESIAN_POINT('Ctrl Pts',(0.0057854625583783,-0.0323031222247695,
0.0794935836940241));
#105543=CARTESIAN_POINT('Ctrl Pts',(0.0057123126671233,-0.0321934096636184,
0.0794603658823897));
#105544=CARTESIAN_POINT('Ctrl Pts',(0.00597436282245677,-0.0325229783203385,
0.0796613284030495));
#105545=CARTESIAN_POINT('Ctrl Pts',(0.00589838928232841,-0.032413025311208,
0.0796316987045691));
#105546=CARTESIAN_POINT('Ctrl Pts',(0.00582304019343971,-0.0323031222247695,
0.079600501889769));
#105547=CARTESIAN_POINT('Ctrl Pts',(0.00574841066252471,-0.0321934096636184,
0.0795677813253106));
#105548=CARTESIAN_POINT('Ctrl Pts',(0.00601486956217176,-0.0325229783203385,
0.0797671600934241));
#105549=CARTESIAN_POINT('Ctrl Pts',(0.00593743713453252,-0.032413025311208,
0.0797380887794547));
#105550=CARTESIAN_POINT('Ctrl Pts',(0.00586061782850113,-0.0323031222247695,
0.079707420085514));
#105551=CARTESIAN_POINT('Ctrl Pts',(0.00578450865792611,-0.0321934096636184,
0.0796751967682314));
#105552=CARTESIAN_POINT('Origin',(0.0122550062864071,-0.0326393375177815,
0.0639105465657135));
#105553=CARTESIAN_POINT('Ctrl Pts',(0.00546514888907057,-0.0326943950436593,
0.079528816687218));
#105554=CARTESIAN_POINT('Ctrl Pts',(0.00539101871414405,-0.0325844576448126,
0.0794921757374785));
#105555=CARTESIAN_POINT('Ctrl Pts',(0.00531764108782414,-0.0324744968375319,
0.0794539990610467));
#105556=CARTESIAN_POINT('Ctrl Pts',(0.00524510935113126,-0.0323646534831894,
0.0794143368688656));
#105557=CARTESIAN_POINT('Ctrl Pts',(0.00557008569869822,-0.0326943950436593,
0.0794860452765929));
#105558=CARTESIAN_POINT('Ctrl Pts',(0.00549654499397228,-0.0325844576448127,
0.0794508505527627));
#105559=CARTESIAN_POINT('Ctrl Pts',(0.00542372696924775,-0.0324744968375319,
0.0794141323958019));
#105560=CARTESIAN_POINT('Ctrl Pts',(0.00535172427432639,-0.0323646534831894,
0.079375939138024));
#105561=CARTESIAN_POINT('Ctrl Pts',(0.00567502250832588,-0.0326943950436593,
0.0794432738659678));
#105562=CARTESIAN_POINT('Ctrl Pts',(0.00560207127380052,-0.0325844576448127,
0.0794095253680468));
#105563=CARTESIAN_POINT('Ctrl Pts',(0.00552981285067137,-0.0324744968375319,
0.079374265730557));
#105564=CARTESIAN_POINT('Ctrl Pts',(0.00545833919752153,-0.0323646534831894,
0.0793375414071823));
#105565=CARTESIAN_POINT('Ctrl Pts',(0.00577995931795353,-0.0326943950436594,
0.0794005024553427));
#105566=CARTESIAN_POINT('Ctrl Pts',(0.00570759755362875,-0.0325844576448127,
0.0793682001833309));
#105567=CARTESIAN_POINT('Ctrl Pts',(0.00563589873209498,-0.0324744968375319,
0.0793343990653122));
#105568=CARTESIAN_POINT('Ctrl Pts',(0.00556495412071667,-0.0323646534831894,
0.0792991436763407));
#105569=CARTESIAN_POINT('Origin',(0.0127037850083422,-0.0326395579068186,
0.0640832166883785));
#105570=CARTESIAN_POINT('Ctrl Pts',(0.00581112919608697,-0.0327445246961877,
0.0794159055361228));
#105571=CARTESIAN_POINT('Ctrl Pts',(0.00561252232407842,-0.0324436878365475,
0.0793286824033436));
#105572=CARTESIAN_POINT('Ctrl Pts',(0.00542104967598372,-0.0321434074463186,
0.0792267471811069));
#105573=CARTESIAN_POINT('Ctrl Pts',(0.00604215830110225,-0.0327445246961877,
0.0795114332945799));
#105574=CARTESIAN_POINT('Ctrl Pts',(0.00583994854082175,-0.0324436878365475,
0.0794329235668505));
#105575=CARTESIAN_POINT('Ctrl Pts',(0.00564422691060632,-0.0321434074463186,
0.0793394056115336));
#105576=CARTESIAN_POINT('Ctrl Pts',(0.0054800754633449,-0.0322357242816072,
0.0792577333257527));
#105577=CARTESIAN_POINT('Ctrl Pts',(0.00531740078140711,-0.0319819883628705,
0.0791735346951717));
#105578=CARTESIAN_POINT('Ctrl Pts',(0.00516041357963271,-0.0317295851069886,
0.0790791552481808));
#105579=CARTESIAN_POINT('Ctrl Pts',(0.0057045435216485,-0.0322357242816072,
0.079367797356214));
#105580=CARTESIAN_POINT('Ctrl Pts',(0.00553836344308834,-0.0319819883628705,
0.0792907477421656));
#105581=CARTESIAN_POINT('Ctrl Pts',(0.0053774230364393,-0.0317295851069886,
0.079203279764923));
#105582=CARTESIAN_POINT('Origin',(0.0126627740881763,-0.0326371942646596,
0.0641692428934363));
#105583=CARTESIAN_POINT('Origin',(0.0122063950829564,-0.0326352985529098,
0.0640232441872437));
#105584=CARTESIAN_POINT('Ctrl Pts',(0.00513265640034522,-0.0321934096636183,
0.0793512658547612));
#105585=CARTESIAN_POINT('Ctrl Pts',(0.00506092689058805,-0.0320835708272303,
0.0793100158989374));
#105586=CARTESIAN_POINT('Ctrl Pts',(0.00499009265255341,-0.0319739230346346,
0.0792673054312881));
#105587=CARTESIAN_POINT('Ctrl Pts',(0.00492024011987723,-0.0318646057455575,
0.0792231960523004));
#105588=CARTESIAN_POINT('Ctrl Pts',(0.00524007193576123,-0.0321934096636183,
0.0793151678282759));
#105589=CARTESIAN_POINT('Ctrl Pts',(0.00516884024592239,-0.0320835708272303,
0.0792753992164001));
#105590=CARTESIAN_POINT('Ctrl Pts',(0.00509847288271428,-0.0319739230346346,
0.0792341795358164));
#105591=CARTESIAN_POINT('Ctrl Pts',(0.00502905582882334,-0.0318646057455575,
0.0791915684338096));
#105592=CARTESIAN_POINT('Ctrl Pts',(0.00534748747117725,-0.0321934096636183,
0.0792790698017906));
#105593=CARTESIAN_POINT('Ctrl Pts',(0.00527675360125673,-0.0320835708272303,
0.0792407825338627));
#105594=CARTESIAN_POINT('Ctrl Pts',(0.00520685311287515,-0.0319739230346346,
0.0792010536403447));
#105595=CARTESIAN_POINT('Ctrl Pts',(0.00513787153776944,-0.0318646057455575,
0.0791599408153188));
#105596=CARTESIAN_POINT('Ctrl Pts',(0.00545490300659327,-0.0321934096636183,
0.0792429717753053));
#105597=CARTESIAN_POINT('Ctrl Pts',(0.00538466695659108,-0.0320835708272303,
0.0792061658513254));
#105598=CARTESIAN_POINT('Ctrl Pts',(0.00531523334303603,-0.0319739230346346,
0.0791679277448729));
#105599=CARTESIAN_POINT('Ctrl Pts',(0.00524668724671554,-0.0318646057455575,
0.079128313196828));
#105600=CARTESIAN_POINT('Ctrl Pts',(0.00556500657548765,-0.032021883458237,
0.0793000937019742));
#105601=CARTESIAN_POINT('Ctrl Pts',(0.0055114065503203,-0.0319391099350643,
0.0792734630335944));
#105602=CARTESIAN_POINT('Ctrl Pts',(0.0054582548416672,-0.0318564869454901,
0.0792460115281513));
#105603=CARTESIAN_POINT('Ctrl Pts',(0.00540558829684642,-0.0317740741446471,
0.0792177627946431));
#105604=CARTESIAN_POINT('Ctrl Pts',(0.00557977995831009,-0.032021883458237,
0.0793474072857285));
#105605=CARTESIAN_POINT('Ctrl Pts',(0.0055256875131157,-0.0319391099350643,
0.0793209303725494));
#105606=CARTESIAN_POINT('Ctrl Pts',(0.00547204128187133,-0.0318564869454901,
0.079293624839943));
#105607=CARTESIAN_POINT('Ctrl Pts',(0.00541887848201503,-0.0317740741446471,
0.0792655142242119));
#105608=CARTESIAN_POINT('Ctrl Pts',(0.00559455334113253,-0.032021883458237,
0.0793947208694827));
#105609=CARTESIAN_POINT('Ctrl Pts',(0.0055399684759111,-0.0319391099350643,
0.0793683977115044));
#105610=CARTESIAN_POINT('Ctrl Pts',(0.00548582772207545,-0.0318564869454901,
0.0793412381517346));
#105611=CARTESIAN_POINT('Ctrl Pts',(0.00543216866718363,-0.0317740741446471,
0.0793132656537809));
#105612=CARTESIAN_POINT('Ctrl Pts',(0.00560932672395496,-0.032021883458237,
0.079442034453237));
#105613=CARTESIAN_POINT('Ctrl Pts',(0.00555424943870649,-0.0319391099350643,
0.0794158650504595));
#105614=CARTESIAN_POINT('Ctrl Pts',(0.00549961416227957,-0.0318564869454901,
0.0793888514635263));
#105615=CARTESIAN_POINT('Ctrl Pts',(0.00544545885235224,-0.0317740741446471,
0.0793610170833498));
#105616=CARTESIAN_POINT('Origin',(0.00360949835450093,-0.0391228853390903,
0.0853527612558224));
#105617=CARTESIAN_POINT('Ctrl Pts',(0.00854323475386372,-0.0352722978779658,
0.0798865690174418));
#105618=CARTESIAN_POINT('Ctrl Pts',(0.00852436587356845,-0.0352466642097259,
0.0798875976254809));
#105619=CARTESIAN_POINT('Ctrl Pts',(0.008505518070848,-0.0352210183808322,
0.0798887036019082));
#105620=CARTESIAN_POINT('Ctrl Pts',(0.00848669071177818,-0.0351953608940152,
0.0798898875173587));
#105621=CARTESIAN_POINT('Origin',(0.00862888701976859,-0.0352456003065125,
0.084785794148498));
#105622=CARTESIAN_POINT('Ctrl Pts',(0.00836211277690418,-0.0350241211493338,
0.0798949524517777));
#105623=CARTESIAN_POINT('Ctrl Pts',(0.00828297841597139,-0.034914423286742,
0.0798982353577021));
#105624=CARTESIAN_POINT('Ctrl Pts',(0.00820372882930312,-0.0348045283677512,
0.0798998844648908));
#105625=CARTESIAN_POINT('Ctrl Pts',(0.00812446544693723,-0.0346945769586886,
0.079899893883675));
#105626=CARTESIAN_POINT('Ctrl Pts',(0.00844382529575833,-0.0350241211493338,
0.0799734649098091));
#105627=CARTESIAN_POINT('Ctrl Pts',(0.00836360945795629,-0.034914423286742,
0.0799778733721265));
#105628=CARTESIAN_POINT('Ctrl Pts',(0.00828325448104889,-0.0348045283677512,
0.0799806263545093));
#105629=CARTESIAN_POINT('Ctrl Pts',(0.00820286315832291,-0.0346945769586886,
0.0799817165006773));
#105630=CARTESIAN_POINT('Ctrl Pts',(0.00852553781461249,-0.0350241211493338,
0.0800519773678404));
#105631=CARTESIAN_POINT('Ctrl Pts',(0.00844424049994119,-0.034914423286742,
0.0800575113865509));
#105632=CARTESIAN_POINT('Ctrl Pts',(0.00836278013279466,-0.0348045283677512,
0.0800613682441279));
#105633=CARTESIAN_POINT('Ctrl Pts',(0.00828126086970859,-0.0346945769586886,
0.0800635391176797));
#105634=CARTESIAN_POINT('Ctrl Pts',(0.00860725033346665,-0.0350241211493338,
0.0801304898258718));
#105635=CARTESIAN_POINT('Ctrl Pts',(0.0085248715419261,-0.034914423286742,
0.0801371494009753));
#105636=CARTESIAN_POINT('Ctrl Pts',(0.00844230578454043,-0.0348045283677512,
0.0801421101337464));
#105637=CARTESIAN_POINT('Ctrl Pts',(0.00835965858109427,-0.0346945769586886,
0.080145361734682));
#105638=CARTESIAN_POINT('Origin',(0.00830254879793467,-0.0345629067941517,
0.0631120639048819));
#105639=CARTESIAN_POINT('Ctrl Pts',(0.00807262228378706,-0.0351970973651502,
0.0800806748722953));
#105640=CARTESIAN_POINT('Ctrl Pts',(0.00799046082130408,-0.0350869349326827,
0.0800799661210889));
#105641=CARTESIAN_POINT('Ctrl Pts',(0.00790824603176679,-0.034976498513997,
0.0800775486914956));
#105642=CARTESIAN_POINT('Ctrl Pts',(0.00782608461120774,-0.0348659306865088,
0.0800734194454661));
#105643=CARTESIAN_POINT('Ctrl Pts',(0.00812828747982777,-0.0351970973651502,
0.080020161596071));
#105644=CARTESIAN_POINT('Ctrl Pts',(0.00804696434677294,-0.0350869349326827,
0.0800202240107124));
#105645=CARTESIAN_POINT('Ctrl Pts',(0.00796557254901559,-0.034976498513997,
0.0800185958141959));
#105646=CARTESIAN_POINT('Ctrl Pts',(0.00788421765618942,-0.0348659306865088,
0.0800152729087609));
#105647=CARTESIAN_POINT('Ctrl Pts',(0.00818395267586848,-0.0351970973651502,
0.0799596483198466));
#105648=CARTESIAN_POINT('Ctrl Pts',(0.0081034678722418,-0.0350869349326827,
0.0799604819003359));
#105649=CARTESIAN_POINT('Ctrl Pts',(0.00802289906626439,-0.034976498513997,
0.0799596429368962));
#105650=CARTESIAN_POINT('Ctrl Pts',(0.00794235070117111,-0.0348659306865088,
0.0799571263720558));
#105651=CARTESIAN_POINT('Ctrl Pts',(0.00823961787190918,-0.0351970973651502,
0.0798991350436223));
#105652=CARTESIAN_POINT('Ctrl Pts',(0.00815997139771065,-0.0350869349326827,
0.0799007397899595));
#105653=CARTESIAN_POINT('Ctrl Pts',(0.00808022558351319,-0.034976498513997,
0.0799006900595965));
#105654=CARTESIAN_POINT('Ctrl Pts',(0.00800048374615279,-0.0348659306865088,
0.0798989798353506));
#105655=CARTESIAN_POINT('Origin',(0.00878055862465359,-0.0345637187966198,
0.0631652800849412));
#105656=CARTESIAN_POINT('Ctrl Pts',(0.00827329948653789,-0.0352450361861252,
0.0798994147162095));
#105657=CARTESIAN_POINT('Ctrl Pts',(0.00805645675787159,-0.0349452761023764,
0.07990505385332));
#105658=CARTESIAN_POINT('Ctrl Pts',(0.00783980529366988,-0.0346444289983475,
0.0798943434890843));
#105659=CARTESIAN_POINT('Ctrl Pts',(0.00852301470585977,-0.0352450361861252,
0.0798874853725969));
#105660=CARTESIAN_POINT('Ctrl Pts',(0.00830662189975912,-0.0349452761023764,
0.0799025426735067));
#105661=CARTESIAN_POINT('Ctrl Pts',(0.00808970966532535,-0.0346444289983475,
0.0799012576070674));
#105662=CARTESIAN_POINT('Ctrl Pts',(0.00800091490804747,-0.0345231616327821,
0.0798985810765177));
#105663=CARTESIAN_POINT('Ctrl Pts',(0.00792167881126297,-0.0344132092796975,
0.0798968875239764));
#105664=CARTESIAN_POINT('Ctrl Pts',(0.00784248183249529,-0.0343032738558973,
0.0798935551226533));
#105665=CARTESIAN_POINT('Ctrl Pts',(0.00776342532287004,-0.034193496108874,
0.0798885907406878));
#105666=CARTESIAN_POINT('Ctrl Pts',(0.00807753634435134,-0.0345231616327821,
0.0799820693489749));
#105667=CARTESIAN_POINT('Ctrl Pts',(0.00799714947927311,-0.0344132092796975,
0.0799814319150588));
#105668=CARTESIAN_POINT('Ctrl Pts',(0.00791677994660534,-0.0343032738558973,
0.0799791317751354));
#105669=CARTESIAN_POINT('Ctrl Pts',(0.00783653063352568,-0.034193496108874,
0.079975174513377));
#105670=CARTESIAN_POINT('Ctrl Pts',(0.00815415778065521,-0.0345231616327821,
0.0800655576214321));
#105671=CARTESIAN_POINT('Ctrl Pts',(0.00807262014728325,-0.0344132092796975,
0.0800659763061411));
#105672=CARTESIAN_POINT('Ctrl Pts',(0.0079910780607154,-0.0343032738558973,
0.0800647084276175));
#105673=CARTESIAN_POINT('Ctrl Pts',(0.00790963594418132,-0.034193496108874,
0.0800617582860662));
#105674=CARTESIAN_POINT('Ctrl Pts',(0.00823077921695908,-0.0345231616327821,
0.0801490458938894));
#105675=CARTESIAN_POINT('Ctrl Pts',(0.00814809081529339,-0.0344132092796975,
0.0801505206972234));
#105676=CARTESIAN_POINT('Ctrl Pts',(0.00806537617482546,-0.0343032738558973,
0.0801502850800996));
#105677=CARTESIAN_POINT('Ctrl Pts',(0.00798274125483696,-0.034193496108874,
0.0801483420587555));
#105678=CARTESIAN_POINT('Origin',(0.00830249427756325,-0.034562559623222,
0.0630999603790713));
#105679=CARTESIAN_POINT('Ctrl Pts',(0.00763192194936664,-0.0346945769586885,
0.080129805473483));
#105680=CARTESIAN_POINT('Ctrl Pts',(0.00754951720746111,-0.0345846629176052,
0.0801230273907144));
#105681=CARTESIAN_POINT('Ctrl Pts',(0.00746723855859114,-0.0344746925050311,
0.0801145440540118));
#105682=CARTESIAN_POINT('Ctrl Pts',(0.00738519138275229,-0.0343648066253259,
0.0801043667685933));
#105683=CARTESIAN_POINT('Ctrl Pts',(0.00771374450194384,-0.0346945769586885,
0.0800514078238258));
#105684=CARTESIAN_POINT('Ctrl Pts',(0.00763242011927652,-0.0345846629176052,
0.0800457572971887));
#105685=CARTESIAN_POINT('Ctrl Pts',(0.00755119869677504,-0.0344746925050311,
0.0800384240505924));
#105686=CARTESIAN_POINT('Ctrl Pts',(0.00747018426588057,-0.0343648066253259,
0.0800294179100325));
#105687=CARTESIAN_POINT('Ctrl Pts',(0.00779556705452104,-0.0346945769586885,
0.0799730101741685));
#105688=CARTESIAN_POINT('Ctrl Pts',(0.00771532303109194,-0.0345846629176052,
0.0799684872036631));
#105689=CARTESIAN_POINT('Ctrl Pts',(0.00763515883495895,-0.0344746925050311,
0.079962304047173));
#105690=CARTESIAN_POINT('Ctrl Pts',(0.00755517714900886,-0.0343648066253259,
0.0799544690514716));
#105691=CARTESIAN_POINT('Ctrl Pts',(0.00787738960709824,-0.0346945769586885,
0.0798946125245113));
#105692=CARTESIAN_POINT('Ctrl Pts',(0.00779822594290735,-0.0345846629176052,
0.0798912171101374));
#105693=CARTESIAN_POINT('Ctrl Pts',(0.00771911897314285,-0.0344746925050311,
0.0798861840437536));
#105694=CARTESIAN_POINT('Ctrl Pts',(0.00764017003213714,-0.0343648066253259,
0.0798795201929108));
#105695=CARTESIAN_POINT('Origin',(0.0087832684994177,-0.0345626446731317,
0.0631069123950791));
#105696=CARTESIAN_POINT('Ctrl Pts',(0.00787592552726108,-0.0346945769586885,
0.0798960153213506));
#105697=CARTESIAN_POINT('Ctrl Pts',(0.00775557293577831,-0.034527515336289,
0.0798908238642481));
#105698=CARTESIAN_POINT('Ctrl Pts',(0.00763535248149831,-0.0343603235965159,
0.0798818460861438));
#105699=CARTESIAN_POINT('Ctrl Pts',(0.0075156193285227,-0.034193496108874,
0.0798691138238489));
#105700=CARTESIAN_POINT('Ctrl Pts',(0.00795973971693108,-0.0346945769586885,
0.0798978069522369));
#105701=CARTESIAN_POINT('Ctrl Pts',(0.00783934959902206,-0.034527515336289,
0.0798943710168944));
#105702=CARTESIAN_POINT('Ctrl Pts',(0.00771903639906606,-0.0343603235965159,
0.0798871480344464));
#105703=CARTESIAN_POINT('Ctrl Pts',(0.00759915563260076,-0.034193496108874,
0.0798761646558743));
#105704=CARTESIAN_POINT('Ctrl Pts',(0.00804355390660107,-0.0346945769586885,
0.0798995985831233));
#105705=CARTESIAN_POINT('Ctrl Pts',(0.00792312626226581,-0.034527515336289,
0.0798979181695408));
#105706=CARTESIAN_POINT('Ctrl Pts',(0.00780272031663381,-0.0343603235965159,
0.0798924499827489));
#105707=CARTESIAN_POINT('Ctrl Pts',(0.00768269193667881,-0.034193496108874,
0.0798832154878996));
#105708=CARTESIAN_POINT('Ctrl Pts',(0.00812736809627107,-0.0346945769586885,
0.0799013902140096));
#105709=CARTESIAN_POINT('Ctrl Pts',(0.00800690292550956,-0.034527515336289,
0.0799014653221871));
#105710=CARTESIAN_POINT('Ctrl Pts',(0.00788640423420156,-0.0343603235965159,
0.0798977519310515));
#105711=CARTESIAN_POINT('Ctrl Pts',(0.00776622824075686,-0.034193496108874,
0.0798902663199249));
#105712=CARTESIAN_POINT('Ctrl Pts',(0.00764020152149013,-0.0340223579322366,
0.0798795222919731));
#105713=CARTESIAN_POINT('Ctrl Pts',(0.00756117646586297,-0.0339125849573552,
0.0798728524532801));
#105714=CARTESIAN_POINT('Ctrl Pts',(0.0074823449903898,-0.0338030433565217,
0.0798645516663831));
#105715=CARTESIAN_POINT('Ctrl Pts',(0.00740380696623747,-0.0336938721132321,
0.0798546394831638));
#105716=CARTESIAN_POINT('Ctrl Pts',(0.00771142962619917,-0.0340223579322366,
0.0799676570577041));
#105717=CARTESIAN_POINT('Ctrl Pts',(0.00763118896228746,-0.0339125849573552,
0.0799619696403458));
#105718=CARTESIAN_POINT('Ctrl Pts',(0.00755112239888483,-0.0338030433565217,
0.0799546254241805));
#105719=CARTESIAN_POINT('Ctrl Pts',(0.00747133149506713,-0.0336938721132321,
0.0799456428778106));
#105720=CARTESIAN_POINT('Ctrl Pts',(0.0077826577309082,-0.0340223579322366,
0.0800557918234352));
#105721=CARTESIAN_POINT('Ctrl Pts',(0.00770120145871196,-0.0339125849573552,
0.0800510868274115));
#105722=CARTESIAN_POINT('Ctrl Pts',(0.00761989980737985,-0.0338030433565217,
0.0800446991819779));
#105723=CARTESIAN_POINT('Ctrl Pts',(0.00753885602389679,-0.0336938721132321,
0.0800366462724574));
#105724=CARTESIAN_POINT('Ctrl Pts',(0.00785388583561724,-0.0340223579322366,
0.0801439265891663));
#105725=CARTESIAN_POINT('Ctrl Pts',(0.00777121395513645,-0.0339125849573552,
0.0801402040144772));
#105726=CARTESIAN_POINT('Ctrl Pts',(0.00768867721587487,-0.0338030433565217,
0.0801347729397753));
#105727=CARTESIAN_POINT('Ctrl Pts',(0.00760638055272644,-0.0336938721132321,
0.0801276496671042));
#105728=CARTESIAN_POINT('Origin',(0.00829795822678823,-0.0345589643414324,
0.0632200948973638));
#105729=CARTESIAN_POINT('Ctrl Pts',(0.00725741743083934,-0.034193496108874,
0.0800871215330967));
#105730=CARTESIAN_POINT('Ctrl Pts',(0.00717554804072168,-0.0340836138581107,
0.0800751748760659));
#105731=CARTESIAN_POINT('Ctrl Pts',(0.00709396514407627,-0.03397388966435,
0.0800615398360225));
#105732=CARTESIAN_POINT('Ctrl Pts',(0.00701277198709879,-0.0338644633294062,
0.0800462408636525));
#105733=CARTESIAN_POINT('Ctrl Pts',(0.00734400128143384,-0.034193496108874,
0.0800140161566633));
#105734=CARTESIAN_POINT('Ctrl Pts',(0.00726313997116592,-0.0340836138581107,
0.0800032634396592));
#105735=CARTESIAN_POINT('Ctrl Pts',(0.00718253996459094,-0.03397388966435,
0.079990842626865));
#105736=CARTESIAN_POINT('Ctrl Pts',(0.00710230335410302,-0.0338644633294062,
0.0799767765305772));
#105737=CARTESIAN_POINT('Ctrl Pts',(0.00743058513202835,-0.034193496108874,
0.0799409107802299));
#105738=CARTESIAN_POINT('Ctrl Pts',(0.00735073190161015,-0.0340836138581107,
0.0799313520032526));
#105739=CARTESIAN_POINT('Ctrl Pts',(0.00727111478510562,-0.03397388966435,
0.0799201454177075));
#105740=CARTESIAN_POINT('Ctrl Pts',(0.00719183472110726,-0.0338644633294062,
0.0799073121975019));
#105741=CARTESIAN_POINT('Ctrl Pts',(0.00751716898262285,-0.034193496108874,
0.0798678054037965));
#105742=CARTESIAN_POINT('Ctrl Pts',(0.00743832383205439,-0.0340836138581107,
0.0798594405668459));
#105743=CARTESIAN_POINT('Ctrl Pts',(0.00735968960562029,-0.03397388966435,
0.07984944820855));
#105744=CARTESIAN_POINT('Ctrl Pts',(0.00728136608811149,-0.0338644633294062,
0.0798378478644266));
#105745=CARTESIAN_POINT('Origin',(0.00877764264291297,-0.0345610621863865,
0.0631819783347345));
#105746=CARTESIAN_POINT('Ctrl Pts',(0.00755160587270691,-0.03424362768739,
0.0798728261600692));
#105747=CARTESIAN_POINT('Ctrl Pts',(0.00733576592591758,-0.033943005420186,
0.0798512461743951));
#105748=CARTESIAN_POINT('Ctrl Pts',(0.00712216465073168,-0.0336441434784162,
0.0798134695460296));
#105749=CARTESIAN_POINT('Ctrl Pts',(0.00780084742177028,-0.03424362768739,
0.0798922850968461));
#105750=CARTESIAN_POINT('Ctrl Pts',(0.00758427356908182,-0.033943005420186,
0.0798801054111607));
#105751=CARTESIAN_POINT('Ctrl Pts',(0.00736923240383486,-0.0336441434784162,
0.0798516470967176));
#105752=CARTESIAN_POINT('Ctrl Pts',(0.00728139353848262,-0.0335235895815127,
0.0798378518020453));
#105753=CARTESIAN_POINT('Ctrl Pts',(0.00720308906007888,-0.0334144449262719,
0.0798262546637039));
#105754=CARTESIAN_POINT('Ctrl Pts',(0.00712493420746662,-0.0333049234473133,
0.0798130264900625));
#105755=CARTESIAN_POINT('Ctrl Pts',(0.0070470304489208,-0.0331951640388588,
0.0797981751432531));
#105756=CARTESIAN_POINT('Ctrl Pts',(0.00734694700217044,-0.0335235895815127,
0.0799302851071116));
#105757=CARTESIAN_POINT('Ctrl Pts',(0.00726736999733805,-0.0334144449262719,
0.0799195904412607));
#105758=CARTESIAN_POINT('Ctrl Pts',(0.00718792251191598,-0.0333049234473133,
0.0799072394875031));
#105759=CARTESIAN_POINT('Ctrl Pts',(0.00710870756545171,-0.0331951640388588,
0.0798932388365506));
#105760=CARTESIAN_POINT('Ctrl Pts',(0.00741250046585826,-0.0335235895815127,
0.0800227184121778));
#105761=CARTESIAN_POINT('Ctrl Pts',(0.00733165093459722,-0.0334144449262719,
0.0800129262188175));
#105762=CARTESIAN_POINT('Ctrl Pts',(0.00725091081636533,-0.0333049234473133,
0.0800014524849436));
#105763=CARTESIAN_POINT('Ctrl Pts',(0.00717038468198261,-0.0331951640388588,
0.0799883025298482));
#105764=CARTESIAN_POINT('Ctrl Pts',(0.00747805392954608,-0.0335235895815127,
0.0801151517172441));
#105765=CARTESIAN_POINT('Ctrl Pts',(0.00739593187185639,-0.0334144449262719,
0.0801062619963743));
#105766=CARTESIAN_POINT('Ctrl Pts',(0.00731389912081469,-0.0333049234473133,
0.0800956654823841));
#105767=CARTESIAN_POINT('Ctrl Pts',(0.00723206179851352,-0.0331951640388588,
0.0800833662231457));
#105768=CARTESIAN_POINT('Origin',(0.0109126035636551,-0.0326434571769533,
0.0635855817183451));
#105769=CARTESIAN_POINT('Ctrl Pts',(0.00688470377095714,-0.0336938721132463,
0.0800222146757731));
#105770=CARTESIAN_POINT('Ctrl Pts',(0.00685033174984972,-0.0336474569764994,
0.0800149619385979));
#105771=CARTESIAN_POINT('Ctrl Pts',(0.00681604698638109,-0.033601104548885,
0.0800073073304798));
#105772=CARTESIAN_POINT('Ctrl Pts',(0.0067292458553903,-0.0334837508694645,
0.0799879276243151));
#105773=CARTESIAN_POINT('Ctrl Pts',(0.00664305710187704,-0.0333660264863674,
0.0799659843310315));
#105774=CARTESIAN_POINT('Ctrl Pts',(0.00715771327077731,-0.0336938721132463,
0.0798196415969008));
#105775=CARTESIAN_POINT('Ctrl Pts',(0.00712452697712149,-0.0336474569764994,
0.0798139868749222));
#105776=CARTESIAN_POINT('Ctrl Pts',(0.00709140915307214,-0.033601104548885,
0.0798079440529407));
#105777=CARTESIAN_POINT('Ctrl Pts',(0.00700756244413778,-0.0334837508694645,
0.0797926450183462));
#105778=CARTESIAN_POINT('Ctrl Pts',(0.00692420589656798,-0.0333660264863674,
0.0797748681503462));
#105779=CARTESIAN_POINT('Ctrl Pts',(0.00715771327077761,-0.0336938721132426,
0.079819641596909));
#105780=CARTESIAN_POINT('Ctrl Pts',(0.00712452697712665,-0.0336474569765026,
0.0798139868749313));
#105781=CARTESIAN_POINT('Ctrl Pts',(0.00709140915308214,-0.0336011045488949,
0.0798079440529507));
#105782=CARTESIAN_POINT('Ctrl Pts',(0.0070082607730359,-0.033484728265791,
0.0797927724384774));
#105783=CARTESIAN_POINT('Ctrl Pts',(0.00692559412378843,-0.0333679870047995,
0.0797751640287754));
#105784=CARTESIAN_POINT('Ctrl Pts',(0.00715771327077482,-0.0336938721132428,
0.0798196415969002));
#105785=CARTESIAN_POINT('Ctrl Pts',(0.00703902439827544,-0.0335278710435084,
0.0797994178086434));
#105786=CARTESIAN_POINT('Ctrl Pts',(0.00692101149298736,-0.033362046922432,
0.0797754790828853));
#105787=CARTESIAN_POINT('Ctrl Pts',(0.00680361984569509,-0.0331951640388602,
0.0797477938847794));
#105788=CARTESIAN_POINT('Ctrl Pts',(0.00724064201843547,-0.0336938721132428,
0.0798319238049554));
#105789=CARTESIAN_POINT('Ctrl Pts',(0.00712169602890304,-0.0335278710435084,
0.0798134360558096));
#105790=CARTESIAN_POINT('Ctrl Pts',(0.00700337165529993,-0.033362046922432,
0.0797912246953047));
#105791=CARTESIAN_POINT('Ctrl Pts',(0.00688561374619074,-0.0331951640388602,
0.0797652589958522));
#105792=CARTESIAN_POINT('Ctrl Pts',(0.00732357076609612,-0.0336938721132428,
0.0798442060130106));
#105793=CARTESIAN_POINT('Ctrl Pts',(0.00720436765953065,-0.0335278710435084,
0.0798274543029757));
#105794=CARTESIAN_POINT('Ctrl Pts',(0.00708573181761249,-0.033362046922432,
0.079806970307724));
#105795=CARTESIAN_POINT('Ctrl Pts',(0.00696760764668638,-0.0331951640388602,
0.079782724106925));
#105796=CARTESIAN_POINT('Ctrl Pts',(0.00740649951375678,-0.0336938721132428,
0.0798564882210658));
#105797=CARTESIAN_POINT('Ctrl Pts',(0.00728703929015824,-0.0335278710435084,
0.0798414725501419));
#105798=CARTESIAN_POINT('Ctrl Pts',(0.00716809197992505,-0.033362046922432,
0.0798227159201434));
#105799=CARTESIAN_POINT('Ctrl Pts',(0.00704960154718203,-0.0331951640388602,
0.0798001892179978));
#105800=CARTESIAN_POINT('Ctrl Pts',(0.00692591378542022,-0.0330240426238155,
0.0797737347072755));
#105801=CARTESIAN_POINT('Ctrl Pts',(0.00684844136088866,-0.0329142774063509,
0.0797572329029329));
#105802=CARTESIAN_POINT('Ctrl Pts',(0.0067712714519193,-0.0328043479726686,
0.0797391213004156));
#105803=CARTESIAN_POINT('Ctrl Pts',(0.00669450355790043,-0.0326943950436594,
0.0797194203794371));
#105804=CARTESIAN_POINT('Ctrl Pts',(0.00698553388977376,-0.0330240426238155,
0.0798701016058561));
#105805=CARTESIAN_POINT('Ctrl Pts',(0.00690673391732854,-0.0329142774063509,
0.0798544211265362));
#105806=CARTESIAN_POINT('Ctrl Pts',(0.00682821881953199,-0.0328043479726686,
0.0798371038143781));
#105807=CARTESIAN_POINT('Ctrl Pts',(0.00675008979103648,-0.0326943950436594,
0.0798181690840916));
#105808=CARTESIAN_POINT('Ctrl Pts',(0.00704515399412731,-0.0330240426238155,
0.0799664685044368));
#105809=CARTESIAN_POINT('Ctrl Pts',(0.00696502647376842,-0.0329142774063509,
0.0799516093501394));
#105810=CARTESIAN_POINT('Ctrl Pts',(0.00688516618714469,-0.0328043479726686,
0.0799350863283406));
#105811=CARTESIAN_POINT('Ctrl Pts',(0.00680567602417252,-0.0326943950436594,
0.079916917788746));
#105812=CARTESIAN_POINT('Ctrl Pts',(0.00710477409848085,-0.0330240426238155,
0.0800628354030175));
#105813=CARTESIAN_POINT('Ctrl Pts',(0.00702331903020831,-0.0329142774063509,
0.0800487975737426));
#105814=CARTESIAN_POINT('Ctrl Pts',(0.00694211355475738,-0.0328043479726686,
0.0800330688423031));
#105815=CARTESIAN_POINT('Ctrl Pts',(0.00686126225730857,-0.0326943950436594,
0.0800156664934005));
#105816=CARTESIAN_POINT('Origin',(0.01094149030982,-0.0326396682856681,
0.0634653280083133));
#105817=CARTESIAN_POINT('Ctrl Pts',(0.00652013033595481,-0.0331951640388589,
0.0799317212593737));
#105818=CARTESIAN_POINT('Ctrl Pts',(0.00644049882193376,-0.0330855618255042,
0.0799096341992027));
#105819=CARTESIAN_POINT('Ctrl Pts',(0.00636126640444661,-0.0329757224427709,
0.0798858853695025));
#105820=CARTESIAN_POINT('Ctrl Pts',(0.00628253603712311,-0.0328657862078596,
0.0798605002051586));
#105821=CARTESIAN_POINT('Ctrl Pts',(0.00661519395356684,-0.0331951640388589,
0.0798700441919475));
#105822=CARTESIAN_POINT('Ctrl Pts',(0.0065364119163779,-0.0330855618255042,
0.0798492664407969));
#105823=CARTESIAN_POINT('Ctrl Pts',(0.00645800252691944,-0.0329757224427709,
0.0798268454212137));
#105824=CARTESIAN_POINT('Ctrl Pts',(0.00638006760147917,-0.0328657862078596,
0.0798028049194409));
#105825=CARTESIAN_POINT('Ctrl Pts',(0.00671025757117887,-0.0331951640388589,
0.0798083671245212));
#105826=CARTESIAN_POINT('Ctrl Pts',(0.00663232501082203,-0.0330855618255042,
0.0797888986823911));
#105827=CARTESIAN_POINT('Ctrl Pts',(0.00655473864939227,-0.0329757224427709,
0.079767805472925));
#105828=CARTESIAN_POINT('Ctrl Pts',(0.00647759916583523,-0.0328657862078596,
0.0797451096337231));
#105829=CARTESIAN_POINT('Ctrl Pts',(0.0068053211887909,-0.0331951640388589,
0.0797466900570949));
#105830=CARTESIAN_POINT('Ctrl Pts',(0.00672823810526616,-0.0330855618255042,
0.0797285309239853));
#105831=CARTESIAN_POINT('Ctrl Pts',(0.00665147477186511,-0.0329757224427709,
0.0797087655246363));
#105832=CARTESIAN_POINT('Ctrl Pts',(0.0065751307301913,-0.0328657862078596,
0.0796874143480053));
#105833=CARTESIAN_POINT('Origin',(0.0113951742473582,-0.0326401908833327,
0.0636248390000959));
#105834=CARTESIAN_POINT('Ctrl Pts',(0.00683878670877478,-0.0332451089994432,
0.0797559710671071));
#105835=CARTESIAN_POINT('Ctrl Pts',(0.00662735405075975,-0.0329451141710259,
0.0797075066694966));
#105836=CARTESIAN_POINT('Ctrl Pts',(0.00642017258716349,-0.0326442513127504,
0.0796432539819795));
#105837=CARTESIAN_POINT('Ctrl Pts',(0.00708362342542217,-0.0332451089994432,
0.0798065178986729));
#105838=CARTESIAN_POINT('Ctrl Pts',(0.00687028436246422,-0.0329451141710259,
0.0797672876689095));
#105839=CARTESIAN_POINT('Ctrl Pts',(0.00666050635454846,-0.0326442513127504,
0.0797120993177296));
#105840=CARTESIAN_POINT('Ctrl Pts',(0.00657516112630008,-0.0325229783203384,
0.0796874229420149));
#105841=CARTESIAN_POINT('Ctrl Pts',(0.0064988278735293,-0.0324130253112079,
0.0796660752348636));
#105842=CARTESIAN_POINT('Ctrl Pts',(0.00642294780292916,-0.0323031222247694,
0.0796431517141486));
#105843=CARTESIAN_POINT('Ctrl Pts',(0.00634761707533441,-0.0321934096636184,
0.0796186851730301));
#105844=CARTESIAN_POINT('Ctrl Pts',(0.00662861268624204,-0.0325229783203384,
0.0797873432772312));
#105845=CARTESIAN_POINT('Ctrl Pts',(0.00655090203386048,-0.0324130253112079,
0.0797667323986514));
#105846=CARTESIAN_POINT('Ctrl Pts',(0.00647362953031397,-0.0323031222247694,
0.0797445171014735));
#105847=CARTESIAN_POINT('Ctrl Pts',(0.0063968931520563,-0.0321934096636184,
0.0797207293346115));
#105848=CARTESIAN_POINT('Ctrl Pts',(0.00668206424618399,-0.0325229783203384,
0.0798872636124475));
#105849=CARTESIAN_POINT('Ctrl Pts',(0.00660297619419166,-0.0324130253112079,
0.0798673895624392));
#105850=CARTESIAN_POINT('Ctrl Pts',(0.00652431125769877,-0.0323031222247694,
0.0798458824887985));
#105851=CARTESIAN_POINT('Ctrl Pts',(0.00644616922877819,-0.0321934096636184,
0.079822773496193));
#105852=CARTESIAN_POINT('Ctrl Pts',(0.00673551580612595,-0.0325229783203384,
0.0799871839476638));
#105853=CARTESIAN_POINT('Ctrl Pts',(0.00665505035452285,-0.0324130253112079,
0.079968046726227));
#105854=CARTESIAN_POINT('Ctrl Pts',(0.00657499298508357,-0.0323031222247694,
0.0799472478761234));
#105855=CARTESIAN_POINT('Ctrl Pts',(0.00649544530550007,-0.0321934096636184,
0.0799248176577744));
#105856=CARTESIAN_POINT('Origin',(0.0109390865415934,-0.0326393375177802,
0.0634735080404004));
#105857=CARTESIAN_POINT('Ctrl Pts',(0.00616025749492643,-0.0326943950436593,
0.0798196182199216));
#105858=CARTESIAN_POINT('Ctrl Pts',(0.00608211952985911,-0.0325844576448127,
0.0797925571695433));
#105859=CARTESIAN_POINT('Ctrl Pts',(0.00600453570173563,-0.0324744968375319,
0.0797638781827858));
#105860=CARTESIAN_POINT('Ctrl Pts',(0.00592760490865445,-0.0323646534831894,
0.0797336193759323));
#105861=CARTESIAN_POINT('Ctrl Pts',(0.00625900616726944,-0.0326943950436593,
0.0797640320049739));
#105862=CARTESIAN_POINT('Ctrl Pts',(0.00618163428442377,-0.0325844576448127,
0.0797383318963751));
#105863=CARTESIAN_POINT('Ctrl Pts',(0.00610478844623147,-0.0324744968375319,
0.0797110297915496));
#105864=CARTESIAN_POINT('Ctrl Pts',(0.00602856662956808,-0.0323646534831894,
0.0796821620295969));
#105865=CARTESIAN_POINT('Ctrl Pts',(0.00635775483961245,-0.0326943950436593,
0.0797084457900262));
#105866=CARTESIAN_POINT('Ctrl Pts',(0.00628114903898843,-0.0325844576448127,
0.079684106623207));
#105867=CARTESIAN_POINT('Ctrl Pts',(0.00620504119072732,-0.0324744968375319,
0.0796581814003134));
#105868=CARTESIAN_POINT('Ctrl Pts',(0.00612952835048171,-0.0323646534831894,
0.0796307046832615));
#105869=CARTESIAN_POINT('Ctrl Pts',(0.00645650351195547,-0.0326943950436593,
0.0796528595750784));
#105870=CARTESIAN_POINT('Ctrl Pts',(0.00638066379355309,-0.0325844576448127,
0.0796298813500389));
#105871=CARTESIAN_POINT('Ctrl Pts',(0.00630529393522316,-0.0324744968375319,
0.0796053330090773));
#105872=CARTESIAN_POINT('Ctrl Pts',(0.00623049007139533,-0.0323646534831894,
0.0795792473369261));
#105873=CARTESIAN_POINT('Origin',(0.0114059678144438,-0.0326395579066531,
0.063588569718786));
#105874=CARTESIAN_POINT('Ctrl Pts',(0.00648935812421096,-0.0327445246961878,
0.0796642345763496));
#105875=CARTESIAN_POINT('Ctrl Pts',(0.00628138536943636,-0.0324436878365476,
0.0796025912655016));
#105876=CARTESIAN_POINT('Ctrl Pts',(0.00607864666934498,-0.0321434074463187,
0.0795254577190637));
#105877=CARTESIAN_POINT('Ctrl Pts',(0.00673053829859072,-0.0327445246961878,
0.0797300534451195));
#105878=CARTESIAN_POINT('Ctrl Pts',(0.00652008314462459,-0.0324436878365476,
0.0796775063931573));
#105879=CARTESIAN_POINT('Ctrl Pts',(0.00631418393018645,-0.0321434074463187,
0.0796092562796439));
#105880=CARTESIAN_POINT('Ctrl Pts',(0.00614109061444679,-0.0322357242816073,
0.07954880163591));
#105881=CARTESIAN_POINT('Ctrl Pts',(0.00596914578433222,-0.0319819883628706,
0.0794856554805864));
#105882=CARTESIAN_POINT('Ctrl Pts',(0.0058015675922602,-0.0317295851069886,
0.0794116959573514));
#105883=CARTESIAN_POINT('Ctrl Pts',(0.00637758335590217,-0.0322357242816073,
0.0796298644710376));
#105884=CARTESIAN_POINT('Ctrl Pts',(0.00620305677962344,-0.0319819883628706,
0.0795742503028096));
#105885=CARTESIAN_POINT('Ctrl Pts',(0.00603242279173021,-0.0317295851069886,
0.0795076432182694));
#105886=CARTESIAN_POINT('Origin',(0.0113760622196953,-0.0326371942645951,
0.0636790576134149));
#105887=CARTESIAN_POINT('Origin',(0.0109049834096659,-0.0326352985528477,
0.0635914096061122));
#105888=CARTESIAN_POINT('Ctrl Pts',(0.00580813378883181,-0.0321934096636183,
0.0796851397875583));
#105889=CARTESIAN_POINT('Ctrl Pts',(0.00573179989733588,-0.0320835708272303,
0.0796532051913567));
#105890=CARTESIAN_POINT('Ctrl Pts',(0.00565617116740778,-0.0319739230346346,
0.0796197093926018));
#105891=CARTESIAN_POINT('Ctrl Pts',(0.00558134107171666,-0.0318646057455575,
0.0795847026730352));
#105892=CARTESIAN_POINT('Ctrl Pts',(0.00591017803828295,-0.0321934096636183,
0.079635863668405));
#105893=CARTESIAN_POINT('Ctrl Pts',(0.00583452370287361,-0.0320835708272303,
0.0796053363419319));
#105894=CARTESIAN_POINT('Ctrl Pts',(0.00575954501148807,-0.0319739230346346,
0.0795732610600095));
#105895=CARTESIAN_POINT('Ctrl Pts',(0.00568533474460069,-0.0318646057455575,
0.0795396862230981));
#105896=CARTESIAN_POINT('Ctrl Pts',(0.00601222228773408,-0.0321934096636183,
0.0795865875492518));
#105897=CARTESIAN_POINT('Ctrl Pts',(0.00593724750841134,-0.0320835708272303,
0.079557467492507));
#105898=CARTESIAN_POINT('Ctrl Pts',(0.00586291885556837,-0.0319739230346346,
0.0795268127274173));
#105899=CARTESIAN_POINT('Ctrl Pts',(0.00578932841748471,-0.0318646057455575,
0.079494669773161));
#105900=CARTESIAN_POINT('Ctrl Pts',(0.00611426653718522,-0.0321934096636183,
0.0795373114300986));
#105901=CARTESIAN_POINT('Ctrl Pts',(0.00603997131394907,-0.0320835708272303,
0.0795095986430821));
#105902=CARTESIAN_POINT('Ctrl Pts',(0.00596629269964866,-0.0319739230346346,
0.0794803643948251));
#105903=CARTESIAN_POINT('Ctrl Pts',(0.00589332209036874,-0.0318646057455575,
0.0794496533232239));
#105904=CARTESIAN_POINT('Ctrl Pts',(0.00623066118232943,-0.0320218834582362,
0.0795801832969985));
#105905=CARTESIAN_POINT('Ctrl Pts',(0.00617414610159012,-0.0319391099350637,
0.0795604804838664));
#105906=CARTESIAN_POINT('Ctrl Pts',(0.00611797292409208,-0.0318564869454897,
0.0795399071172582));
#105907=CARTESIAN_POINT('Ctrl Pts',(0.00606218116559332,-0.0317740741446468,
0.0795184820018143));
#105908=CARTESIAN_POINT('Ctrl Pts',(0.00625124803705913,-0.0320218834582362,
0.0796252722031731));
#105909=CARTESIAN_POINT('Ctrl Pts',(0.00619426368980827,-0.0319391099350637,
0.0796057836494304));
#105910=CARTESIAN_POINT('Ctrl Pts',(0.00613761818442492,-0.0318564869454897,
0.0795854170847348));
#105911=CARTESIAN_POINT('Ctrl Pts',(0.00608135139475746,-0.0317740741446468,
0.0795641911952165));
#105912=CARTESIAN_POINT('Ctrl Pts',(0.00627183489178884,-0.0320218834582362,
0.0796703611093477));
#105913=CARTESIAN_POINT('Ctrl Pts',(0.00621438127802641,-0.0319391099350637,
0.0796510868149944));
#105914=CARTESIAN_POINT('Ctrl Pts',(0.00615726344475776,-0.0318564869454897,
0.0796309270522114));
#105915=CARTESIAN_POINT('Ctrl Pts',(0.00610052162392159,-0.0317740741446468,
0.0796099003886187));
#105916=CARTESIAN_POINT('Ctrl Pts',(0.00629242174651854,-0.0320218834582362,
0.0797154500155224));
#105917=CARTESIAN_POINT('Ctrl Pts',(0.00623449886624456,-0.0319391099350637,
0.0796963899805584));
#105918=CARTESIAN_POINT('Ctrl Pts',(0.00617690870509059,-0.0318564869454897,
0.079676437019688));
#105919=CARTESIAN_POINT('Ctrl Pts',(0.00611969185308573,-0.0317740741446468,
0.0796556095820209));
#105920=CARTESIAN_POINT('Origin',(0.00504917312395027,-0.0391228853391003,
0.0858302139279516));
#105921=CARTESIAN_POINT('Ctrl Pts',(0.00925890998965823,-0.0352722978779654,
0.0797887631115429));
#105922=CARTESIAN_POINT('Ctrl Pts',(0.00924031881489165,-0.0352466642097257,
0.0797921485064815));
#105923=CARTESIAN_POINT('Ctrl Pts',(0.00922175824832721,-0.0352210183808321,
0.0797956080180148));
#105924=CARTESIAN_POINT('Ctrl Pts',(0.00920322773255888,-0.0351953608940152,
0.0797991422917301));
#105925=CARTESIAN_POINT('Origin',(0.00995792258949127,-0.0352456003065099,
0.0846386213136292));
#105926=CARTESIAN_POINT('Ctrl Pts',(0.00908026693651953,-0.0350241211493339,
0.0798197810430369));
#105927=CARTESIAN_POINT('Ctrl Pts',(0.00900216803087394,-0.0349144232867421,
0.0798329562276092));
#105928=CARTESIAN_POINT('Ctrl Pts',(0.00892375003880367,-0.0348045283677512,
0.079844524938051));
#105929=CARTESIAN_POINT('Ctrl Pts',(0.00884511285236919,-0.0346945769586885,
0.0798544686185804));
#105930=CARTESIAN_POINT('Ctrl Pts',(0.00917117534799638,-0.0350241211493339,
0.0798874331126755));
#105931=CARTESIAN_POINT('Ctrl Pts',(0.00909214456287197,-0.0349144232867421,
0.0799018605232856));
#105932=CARTESIAN_POINT('Ctrl Pts',(0.00901276824914229,-0.0348045283677512,
0.0799146629466688));
#105933=CARTESIAN_POINT('Ctrl Pts',(0.00893314746755198,-0.0346945769586885,
0.0799258202011364));
#105934=CARTESIAN_POINT('Ctrl Pts',(0.00926208375947324,-0.0350241211493339,
0.0799550851823141));
#105935=CARTESIAN_POINT('Ctrl Pts',(0.00918212109487,-0.034914423286742,
0.079970764818962));
#105936=CARTESIAN_POINT('Ctrl Pts',(0.00910178645948091,-0.0348045283677512,
0.0799848009552867));
#105937=CARTESIAN_POINT('Ctrl Pts',(0.00902118208273476,-0.0346945769586885,
0.0799971717836925));
#105938=CARTESIAN_POINT('Ctrl Pts',(0.0093529921709501,-0.0350241211493339,
0.0800227372519528));
#105939=CARTESIAN_POINT('Ctrl Pts',(0.00927209762686803,-0.034914423286742,
0.0800396691146383));
#105940=CARTESIAN_POINT('Ctrl Pts',(0.00919080466981953,-0.0348045283677512,
0.0800549389639046));
#105941=CARTESIAN_POINT('Ctrl Pts',(0.00910921669791754,-0.0346945769586885,
0.0800685233662486));
#105942=CARTESIAN_POINT('Origin',(0.00691771894704748,-0.0345629067942052,
0.0631766959308064));
#105943=CARTESIAN_POINT('Ctrl Pts',(0.00881633635390863,-0.0351970973651503,
0.0800403217663952));
#105944=CARTESIAN_POINT('Ctrl Pts',(0.00873473392901711,-0.0350869349326827,
0.080049916165671));
#105945=CARTESIAN_POINT('Ctrl Pts',(0.00865286444338367,-0.034976498513997,
0.0800578220436516));
#105946=CARTESIAN_POINT('Ctrl Pts',(0.00857083335840892,-0.0348659306865088,
0.0800640229144731));
#105947=CARTESIAN_POINT('Ctrl Pts',(0.00886397828867158,-0.0351970973651503,
0.0799733089564085));
#105948=CARTESIAN_POINT('Ctrl Pts',(0.00878330423543964,-0.0350869349326827,
0.0799835633701211));
#105949=CARTESIAN_POINT('Ctrl Pts',(0.00870235016918374,-0.034976498513997,
0.079992149109619));
#105950=CARTESIAN_POINT('Ctrl Pts',(0.00862122031350391,-0.0348659306865088,
0.07999904887807));
#105951=CARTESIAN_POINT('Ctrl Pts',(0.00891162022343454,-0.0351970973651503,
0.0799062961464218));
#105952=CARTESIAN_POINT('Ctrl Pts',(0.00883187454186217,-0.0350869349326827,
0.0799172105745713));
#105953=CARTESIAN_POINT('Ctrl Pts',(0.00875183589498381,-0.034976498513997,
0.0799264761755864));
#105954=CARTESIAN_POINT('Ctrl Pts',(0.0086716072685989,-0.0348659306865088,
0.0799340748416668));
#105955=CARTESIAN_POINT('Ctrl Pts',(0.00895926215819749,-0.0351970973651503,
0.0798392833364352));
#105956=CARTESIAN_POINT('Ctrl Pts',(0.0088804448482847,-0.0350869349326827,
0.0798508577790214));
#105957=CARTESIAN_POINT('Ctrl Pts',(0.00880132162078388,-0.034976498513997,
0.0798608032415538));
#105958=CARTESIAN_POINT('Ctrl Pts',(0.00872199422369388,-0.0348659306865088,
0.0798691008052636));
#105959=CARTESIAN_POINT('Origin',(0.00739862927952232,-0.0345637187966112,
0.0631695819681397));
#105960=CARTESIAN_POINT('Ctrl Pts',(0.00899271323550525,-0.0352450361861251,
0.0798353393780459));
#105961=CARTESIAN_POINT('Ctrl Pts',(0.00877828714781084,-0.0349452761023764,
0.0798681116492347));
#105962=CARTESIAN_POINT('Ctrl Pts',(0.00856200168053271,-0.0346444289983474,
0.0798846393679849));
#105963=CARTESIAN_POINT('Ctrl Pts',(0.00923896423252717,-0.0352450361861251,
0.079792206484963));
#105964=CARTESIAN_POINT('Ctrl Pts',(0.0090261649285478,-0.0349452761023764,
0.0798342662646664));
#105965=CARTESIAN_POINT('Ctrl Pts',(0.00881080205033893,-0.0346444289983474,
0.0798601776431011));
#105966=CARTESIAN_POINT('Ctrl Pts',(0.00872237200801529,-0.0345231616327821,
0.0798686511518472));
#105967=CARTESIAN_POINT('Ctrl Pts',(0.00864354845310441,-0.0344132092796975,
0.0798769018696987));
#105968=CARTESIAN_POINT('Ctrl Pts',(0.00856455830553595,-0.0343032738558973,
0.0798835217587928));
#105969=CARTESIAN_POINT('Ctrl Pts',(0.00848550297805775,-0.034193496108874,
0.0798885049304476));
#105970=CARTESIAN_POINT('Ctrl Pts',(0.00880885311655982,-0.0345231616327821,
0.079941877881967));
#105971=CARTESIAN_POINT('Ctrl Pts',(0.00872902023426923,-0.0344132092796975,
0.079951320620144));
#105972=CARTESIAN_POINT('Ctrl Pts',(0.00864899615539753,-0.0343032738558973,
0.0799591115909203));
#105973=CARTESIAN_POINT('Ctrl Pts',(0.00856888365570858,-0.034193496108874,
0.0799652434392525));
#105974=CARTESIAN_POINT('Ctrl Pts',(0.00889533422510434,-0.0345231616327821,
0.0800151046120867));
#105975=CARTESIAN_POINT('Ctrl Pts',(0.00881449201543405,-0.0344132092796975,
0.0800257393705894));
#105976=CARTESIAN_POINT('Ctrl Pts',(0.00873343400525911,-0.0343032738558973,
0.0800347014230478));
#105977=CARTESIAN_POINT('Ctrl Pts',(0.00865226433335941,-0.034193496108874,
0.0800419819480574));
#105978=CARTESIAN_POINT('Ctrl Pts',(0.00898181533364887,-0.0345231616327821,
0.0800883313422065));
#105979=CARTESIAN_POINT('Ctrl Pts',(0.00889996379659887,-0.0344132092796975,
0.0801001581210348));
#105980=CARTESIAN_POINT('Ctrl Pts',(0.0088178718551207,-0.0343032738558973,
0.0801102912551753));
#105981=CARTESIAN_POINT('Ctrl Pts',(0.00873564501101023,-0.034193496108874,
0.0801187204568624));
#105982=CARTESIAN_POINT('Origin',(0.00691614788271578,-0.0345625596231992,
0.0631646946784457));
#105983=CARTESIAN_POINT('Ctrl Pts',(0.0083852687703767,-0.0346945769586885,
0.0801442993560538));
#105984=CARTESIAN_POINT('Ctrl Pts',(0.00830266429544345,-0.0345846629176052,
0.0801479027732564));
#105985=CARTESIAN_POINT('Ctrl Pts',(0.00821997119427492,-0.0344746925050311,
0.0801497985793136));
#105986=CARTESIAN_POINT('Ctrl Pts',(0.00813729543283345,-0.0343648066253259,
0.0801499847826831));
#105987=CARTESIAN_POINT('Ctrl Pts',(0.0084566202967524,-0.0346945769586885,
0.0800562648101871));
#105988=CARTESIAN_POINT('Ctrl Pts',(0.00837522898235808,-0.0345846629176052,
0.0800608514874877));
#105989=CARTESIAN_POINT('Ctrl Pts',(0.00829372891552425,-0.0344746925050311,
0.0800637558092479));
#105990=CARTESIAN_POINT('Ctrl Pts',(0.00821222453889692,-0.0343648066253259,
0.0800649744853856));
#105991=CARTESIAN_POINT('Ctrl Pts',(0.0085279718231281,-0.0346945769586885,
0.0799682302643205));
#105992=CARTESIAN_POINT('Ctrl Pts',(0.00844779366927271,-0.0345846629176052,
0.079973800201719));
#105993=CARTESIAN_POINT('Ctrl Pts',(0.00836748663677359,-0.0344746925050311,
0.0799777130391821));
#105994=CARTESIAN_POINT('Ctrl Pts',(0.00828715364496039,-0.0343648066253259,
0.0799799641880881));
#105995=CARTESIAN_POINT('Ctrl Pts',(0.00859932334950379,-0.0346945769586885,
0.0798801957184538));
#105996=CARTESIAN_POINT('Ctrl Pts',(0.00852035835618734,-0.0345846629176052,
0.0798867489159503));
#105997=CARTESIAN_POINT('Ctrl Pts',(0.00844124435802293,-0.0344746925050311,
0.0798916702691163));
#105998=CARTESIAN_POINT('Ctrl Pts',(0.00836208275102385,-0.0343648066253259,
0.0798949538907905));
#105999=CARTESIAN_POINT('Origin',(0.00739400237491167,-0.0345626446730793,
0.063111334887826));
#106000=CARTESIAN_POINT('Ctrl Pts',(0.00859804663143735,-0.0346945769586885,
0.0798817709516812));
#106001=CARTESIAN_POINT('Ctrl Pts',(0.00847799239398044,-0.034527515336289,
0.079891704610227));
#106002=CARTESIAN_POINT('Ctrl Pts',(0.00835759469993052,-0.0343603235965158,
0.0798978652428601));
#106003=CARTESIAN_POINT('Ctrl Pts',(0.00823720990302468,-0.0341934961088739,
0.0799002399214836));
#106004=CARTESIAN_POINT('Ctrl Pts',(0.00868142447208004,-0.0346945769586885,
0.079873043751613));
#106005=CARTESIAN_POINT('Ctrl Pts',(0.00856155302932274,-0.034527515336289,
0.0798847237924136));
#106006=CARTESIAN_POINT('Ctrl Pts',(0.00844128325513802,-0.0343603235965158,
0.0798926370077305));
#106007=CARTESIAN_POINT('Ctrl Pts',(0.00832097120197104,-0.0341934961088739,
0.0798967652804823));
#106008=CARTESIAN_POINT('Ctrl Pts',(0.00876480231272273,-0.0346945769586885,
0.0798643165515447));
#106009=CARTESIAN_POINT('Ctrl Pts',(0.00864511366466504,-0.034527515336289,
0.0798777429746003));
#106010=CARTESIAN_POINT('Ctrl Pts',(0.00852497181034551,-0.0343603235965158,
0.079887408772601));
#106011=CARTESIAN_POINT('Ctrl Pts',(0.0084047325009174,-0.0341934961088739,
0.079893290639481));
#106012=CARTESIAN_POINT('Ctrl Pts',(0.00884818015336542,-0.0346945769586885,
0.0798555893514764));
#106013=CARTESIAN_POINT('Ctrl Pts',(0.00872867430000733,-0.034527515336289,
0.0798707621567869));
#106014=CARTESIAN_POINT('Ctrl Pts',(0.00860866036555301,-0.0343603235965158,
0.0798821805374715));
#106015=CARTESIAN_POINT('Ctrl Pts',(0.00848849379986377,-0.0341934961088739,
0.0798898159984798));
#106016=CARTESIAN_POINT('Ctrl Pts',(0.00836211425515608,-0.0340223579322365,
0.0798949520266385));
#106017=CARTESIAN_POINT('Ctrl Pts',(0.00828287638324561,-0.0339125849573554,
0.0798982392473703));
#106018=CARTESIAN_POINT('Ctrl Pts',(0.0082036261530396,-0.0338030433565221,
0.0798998841183849));
#106019=CARTESIAN_POINT('Ctrl Pts',(0.0081244650986915,-0.0336938721132327,
0.0798998935202157));
#106020=CARTESIAN_POINT('Ctrl Pts',(0.00844382692016333,-0.0340223579322365,
0.0799734645747335));
#106021=CARTESIAN_POINT('Ctrl Pts',(0.00836350615544531,-0.0339125849573554,
0.0799778788262313));
#106022=CARTESIAN_POINT('Ctrl Pts',(0.00828315046645,-0.0338030433565221,
0.0799806275226956));
#106023=CARTESIAN_POINT('Ctrl Pts',(0.00820286292615929,-0.0336938721132327,
0.0799817162583713));
#106024=CARTESIAN_POINT('Ctrl Pts',(0.00852553958517058,-0.0340223579322365,
0.0800519771228286));
#106025=CARTESIAN_POINT('Ctrl Pts',(0.00844413592764502,-0.0339125849573554,
0.0800575184050923));
#106026=CARTESIAN_POINT('Ctrl Pts',(0.00836267477986041,-0.0338030433565221,
0.0800613709270064));
#106027=CARTESIAN_POINT('Ctrl Pts',(0.00828126075362708,-0.0336938721132327,
0.080063538996527));
#106028=CARTESIAN_POINT('Ctrl Pts',(0.00860725225017783,-0.0340223579322365,
0.0801304896709236));
#106029=CARTESIAN_POINT('Ctrl Pts',(0.00852476569984473,-0.0339125849573554,
0.0801371579839533));
#106030=CARTESIAN_POINT('Ctrl Pts',(0.00844219909327081,-0.0338030433565221,
0.0801421143313171));
#106031=CARTESIAN_POINT('Ctrl Pts',(0.00835965858109488,-0.0336938721132327,
0.0801453617346826));
#106032=CARTESIAN_POINT('Origin',(0.00692670444745188,-0.0345589643415875,
0.0632844504180948));
#106033=CARTESIAN_POINT('Ctrl Pts',(0.00800836761556648,-0.034193496108874,
0.0801488898535788));
#106034=CARTESIAN_POINT('Ctrl Pts',(0.00792564647794095,-0.0340836138595105,
0.0801472983549206));
#106035=CARTESIAN_POINT('Ctrl Pts',(0.00784299796419675,-0.0339738896671456,
0.0801439958795444));
#106036=CARTESIAN_POINT('Ctrl Pts',(0.00776052757088199,-0.0338644633335883,
0.0801389937451553));
#106037=CARTESIAN_POINT('Ctrl Pts',(0.00808510619341875,-0.034193496108874,
0.0800655091009042));
#106038=CARTESIAN_POINT('Ctrl Pts',(0.00800353482698184,-0.0340836138595105,
0.0800649757817782));
#106039=CARTESIAN_POINT('Ctrl Pts',(0.00792201363593965,-0.0339738896671456,
0.0800627547703019));
#106040=CARTESIAN_POINT('Ctrl Pts',(0.00784064676679219,-0.0338644633335883,
0.0800588559033197));
#106041=CARTESIAN_POINT('Ctrl Pts',(0.00816184477127103,-0.034193496108874,
0.0799821283482295));
#106042=CARTESIAN_POINT('Ctrl Pts',(0.00808142317602273,-0.0340836138595105,
0.0799826532086359));
#106043=CARTESIAN_POINT('Ctrl Pts',(0.00800102930768255,-0.0339738896671456,
0.0799815136610594));
#106044=CARTESIAN_POINT('Ctrl Pts',(0.00792076596270239,-0.0338644633335883,
0.079978718061484));
#106045=CARTESIAN_POINT('Ctrl Pts',(0.0082385833491233,-0.034193496108874,
0.0798987475955549));
#106046=CARTESIAN_POINT('Ctrl Pts',(0.00815931152506361,-0.0340836138595105,
0.0799003306354936));
#106047=CARTESIAN_POINT('Ctrl Pts',(0.00808004497942545,-0.0339738896671456,
0.0799002725518169));
#106048=CARTESIAN_POINT('Ctrl Pts',(0.00800088515861259,-0.0338644633335883,
0.0798985802196484));
#106049=CARTESIAN_POINT('Origin',(0.00739782913690974,-0.034561062186344,
0.0631865140171341));
#106050=CARTESIAN_POINT('Ctrl Pts',(0.0082733779616619,-0.03424362768739,
0.0798994126748766));
#106051=CARTESIAN_POINT('Ctrl Pts',(0.00805653528793645,-0.0339430054201859,
0.0799050547722985));
#106052=CARTESIAN_POINT('Ctrl Pts',(0.00783988365561877,-0.0336441434784161,
0.0798943473624435));
#106053=CARTESIAN_POINT('Ctrl Pts',(0.00852309301813404,-0.03424362768739,
0.0798874799228422));
#106054=CARTESIAN_POINT('Ctrl Pts',(0.00830670039557075,-0.0339430054201859,
0.0799025401788792));
#106055=CARTESIAN_POINT('Ctrl Pts',(0.00808978812157049,-0.0336441434784161,
0.0799012580713354));
#106056=CARTESIAN_POINT('Ctrl Pts',(0.00800091288301854,-0.0335235895815127,
0.0798985806857093));
#106057=CARTESIAN_POINT('Ctrl Pts',(0.007921772351967,-0.0334144449262719,
0.0798968891477485));
#106058=CARTESIAN_POINT('Ctrl Pts',(0.00784257584393467,-0.0333049234473133,
0.0798935606826039));
#106059=CARTESIAN_POINT('Ctrl Pts',(0.00776342501247529,-0.0331951640388588,
0.0798885903730654));
#106060=CARTESIAN_POINT('Ctrl Pts',(0.00807753440307829,-0.0335235895815127,
0.0799820690989813));
#106061=CARTESIAN_POINT('Ctrl Pts',(0.00799724448964452,-0.0334144449262719,
0.079981432407098));
#106062=CARTESIAN_POINT('Ctrl Pts',(0.00791687548640275,-0.0333049234473133,
0.0799791362545462));
#106063=CARTESIAN_POINT('Ctrl Pts',(0.00783653042659583,-0.0331951640388588,
0.0799751742682954));
#106064=CARTESIAN_POINT('Ctrl Pts',(0.00815415592313804,-0.0335235895815127,
0.0800655575122532));
#106065=CARTESIAN_POINT('Ctrl Pts',(0.00807271662732204,-0.0334144449262719,
0.0800659756664474));
#106066=CARTESIAN_POINT('Ctrl Pts',(0.00799117512887083,-0.0333049234473133,
0.0800647118264885));
#106067=CARTESIAN_POINT('Ctrl Pts',(0.00790963584071636,-0.0331951640388588,
0.0800617581635254));
#106068=CARTESIAN_POINT('Ctrl Pts',(0.00823077744319779,-0.0335235895815127,
0.0801490459255251));
#106069=CARTESIAN_POINT('Ctrl Pts',(0.00814818876499955,-0.0334144449262719,
0.0801505189257969));
#106070=CARTESIAN_POINT('Ctrl Pts',(0.00806547477133891,-0.0333049234473133,
0.0801502873984308));
#106071=CARTESIAN_POINT('Ctrl Pts',(0.0079827412548369,-0.0331951640388588,
0.0801483420587554));
#106072=CARTESIAN_POINT('Origin',(0.00956654017020789,-0.0326434571769428,
0.063319353312045));
#106073=CARTESIAN_POINT('Ctrl Pts',(0.00763045792790763,-0.0336938721132464,
0.0801312082143985));
#106074=CARTESIAN_POINT('Ctrl Pts',(0.00759544793145065,-0.0336474569764995,
0.0801283206237717));
#106075=CARTESIAN_POINT('Ctrl Pts',(0.00756047413679517,-0.033601104548885,
0.0801250233947924));
#106076=CARTESIAN_POINT('Ctrl Pts',(0.0074719285374094,-0.0334837508694645,
0.0801166755698235));
#106077=CARTESIAN_POINT('Ctrl Pts',(0.00738366918405866,-0.0333660264863676,
0.0801057076211362));
#106078=CARTESIAN_POINT('Ctrl Pts',(0.00787592552727102,-0.0336938721132464,
0.0798960153213509));
#106079=CARTESIAN_POINT('Ctrl Pts',(0.00784229219286244,-0.0336474569764995,
0.0798945645340381));
#106080=CARTESIAN_POINT('Ctrl Pts',(0.00780867814632869,-0.033601104548885,
0.0798927201254896));
#106081=CARTESIAN_POINT('Ctrl Pts',(0.007723575116262,-0.0334837508694645,
0.079888050507507));
#106082=CARTESIAN_POINT('Ctrl Pts',(0.00763864782761815,-0.0333660264863676,
0.0798808611610665));
#106083=CARTESIAN_POINT('Ctrl Pts',(0.00787592552727113,-0.0336938721132427,
0.0798960153213606));
#106084=CARTESIAN_POINT('Ctrl Pts',(0.00784229219286749,-0.0336474569765026,
0.0798945645340479));
#106085=CARTESIAN_POINT('Ctrl Pts',(0.00780867814633869,-0.0336011045488949,
0.0798927201254996));
#106086=CARTESIAN_POINT('Ctrl Pts',(0.00772428390860401,-0.033484728265791,
0.0798880893990749));
#106087=CARTESIAN_POINT('Ctrl Pts',(0.00764006219165131,-0.0333679870047996,
0.0798809807154008));
#106088=CARTESIAN_POINT('Ctrl Pts',(0.00787592552726848,-0.0336938721132429,
0.0798960153213509));
#106089=CARTESIAN_POINT('Ctrl Pts',(0.00775563783920221,-0.0335278710435085,
0.0798908266638833));
#106090=CARTESIAN_POINT('Ctrl Pts',(0.00763555518301437,-0.033362046922432,
0.07988186764115));
#106091=CARTESIAN_POINT('Ctrl Pts',(0.00751561932852367,-0.0331951640388601,
0.0798691138238489));
#106092=CARTESIAN_POINT('Ctrl Pts',(0.00795973972583508,-0.0336938721132429,
0.0798978069524273));
#106093=CARTESIAN_POINT('Ctrl Pts',(0.00783941453157574,-0.0335278710435085,
0.079894372870193));
#106094=CARTESIAN_POINT('Ctrl Pts',(0.00771923935936628,-0.033362046922432,
0.0798871666292529));
#106095=CARTESIAN_POINT('Ctrl Pts',(0.00759915564146883,-0.0331951640388601,
0.0798761646566227));
#106096=CARTESIAN_POINT('Ctrl Pts',(0.00804355392440168,-0.0336938721132429,
0.0798995985835036));
#106097=CARTESIAN_POINT('Ctrl Pts',(0.00792319122394927,-0.0335278710435085,
0.0798979190765027));
#106098=CARTESIAN_POINT('Ctrl Pts',(0.0078029235357182,-0.033362046922432,
0.0798924656173559));
#106099=CARTESIAN_POINT('Ctrl Pts',(0.007682691954414,-0.0331951640388601,
0.0798832154893964));
#106100=CARTESIAN_POINT('Ctrl Pts',(0.00812736812296829,-0.0336938721132429,
0.07990139021458));
#106101=CARTESIAN_POINT('Ctrl Pts',(0.0080069679163228,-0.0335278710435085,
0.0799014652828123));
#106102=CARTESIAN_POINT('Ctrl Pts',(0.00788660771207011,-0.033362046922432,
0.0798977646054588));
#106103=CARTESIAN_POINT('Ctrl Pts',(0.00776622826735916,-0.0331951640388601,
0.0798902663221702));
#106104=CARTESIAN_POINT('Ctrl Pts',(0.00764020019117138,-0.0330240426238155,
0.0798795226003004));
#106105=CARTESIAN_POINT('Ctrl Pts',(0.00756127043534926,-0.0329142774063509,
0.0798728607870927));
#106106=CARTESIAN_POINT('Ctrl Pts',(0.00748243904845313,-0.0328043479726686,
0.0798645639541958));
#106107=CARTESIAN_POINT('Ctrl Pts',(0.00740380731207764,-0.0326943950436594,
0.079854639949255));
#106108=CARTESIAN_POINT('Ctrl Pts',(0.00771142814820226,-0.0330240426238155,
0.0799676572366385));
#106109=CARTESIAN_POINT('Ctrl Pts',(0.00763128425189917,-0.0329142774063509,
0.0799619766579329));
#106110=CARTESIAN_POINT('Ctrl Pts',(0.00755121783437066,-0.0328043479726686,
0.0799546364490441));
#106111=CARTESIAN_POINT('Ctrl Pts',(0.00747133172562738,-0.0326943950436594,
0.0799456431885381));
#106112=CARTESIAN_POINT('Ctrl Pts',(0.00778265610523314,-0.0330240426238155,
0.0800557918729766));
#106113=CARTESIAN_POINT('Ctrl Pts',(0.00770129806844909,-0.0329142774063509,
0.0800510925287732));
#106114=CARTESIAN_POINT('Ctrl Pts',(0.0076199966202882,-0.0328043479726686,
0.0800447089438924));
#106115=CARTESIAN_POINT('Ctrl Pts',(0.00753885613917711,-0.0326943950436594,
0.0800366464278211));
#106116=CARTESIAN_POINT('Ctrl Pts',(0.00785388406226402,-0.0330240426238155,
0.0801439265093147));
#106117=CARTESIAN_POINT('Ctrl Pts',(0.007771311884999,-0.0329142774063509,
0.0801402083996134));
#106118=CARTESIAN_POINT('Ctrl Pts',(0.00768877540620573,-0.0328043479726686,
0.0801347814387407));
#106119=CARTESIAN_POINT('Ctrl Pts',(0.00760638055272684,-0.0326943950436594,
0.0801276496671042));
#106120=CARTESIAN_POINT('Origin',(0.00958012734946644,-0.0326396682856541,
0.0631964273685868));
#106121=CARTESIAN_POINT('Ctrl Pts',(0.00725741743083936,-0.0331951640388587,
0.0800871215330967));
#106122=CARTESIAN_POINT('Ctrl Pts',(0.00717564559242002,-0.0330855618255041,
0.0800751891111381));
#106123=CARTESIAN_POINT('Ctrl Pts',(0.00709406142859066,-0.0329757224427708,
0.0800615580031402));
#106124=CARTESIAN_POINT('Ctrl Pts',(0.00701277026899738,-0.0328657862078596,
0.0800462405399157));
#106125=CARTESIAN_POINT('Ctrl Pts',(0.00734400125713554,-0.0331951640388587,
0.0800140161771792));
#106126=CARTESIAN_POINT('Ctrl Pts',(0.00726323629710303,-0.0330855618255041,
0.0800032762722701));
#106127=CARTESIAN_POINT('Ctrl Pts',(0.00718263509021607,-0.0329757224427708,
0.0799908593514458));
#106128=CARTESIAN_POINT('Ctrl Pts',(0.00710230163111726,-0.0328657862078596,
0.0799767762524229));
#106129=CARTESIAN_POINT('Ctrl Pts',(0.00743058508343171,-0.0331951640388587,
0.0799409108212615));
#106130=CARTESIAN_POINT('Ctrl Pts',(0.00735082700178604,-0.0330855618255041,
0.079931363433402));
#106131=CARTESIAN_POINT('Ctrl Pts',(0.00727120875184148,-0.0329757224427708,
0.0799201606997513));
#106132=CARTESIAN_POINT('Ctrl Pts',(0.00719183299323715,-0.0328657862078596,
0.0799073119649301));
#106133=CARTESIAN_POINT('Ctrl Pts',(0.00751716890972788,-0.0331951640388587,
0.0798678054653439));
#106134=CARTESIAN_POINT('Ctrl Pts',(0.00743841770646904,-0.0330855618255041,
0.079859450594534));
#106135=CARTESIAN_POINT('Ctrl Pts',(0.0073597824134669,-0.0329757224427708,
0.0798494620480569));
#106136=CARTESIAN_POINT('Ctrl Pts',(0.00728136435535703,-0.0328657862078596,
0.0798378476774373));
#106137=CARTESIAN_POINT('Origin',(0.010050225882153,-0.0326401908832541,
0.0632978188934094));
#106138=CARTESIAN_POINT('Ctrl Pts',(0.00755153376308668,-0.0332451089994431,
0.0798728189499877));
#106139=CARTESIAN_POINT('Ctrl Pts',(0.00733569411506671,-0.0329451141710257,
0.0798512362473379));
#106140=CARTESIAN_POINT('Ctrl Pts',(0.00712209334210132,-0.0326442513127503,
0.0798134569342203));
#106141=CARTESIAN_POINT('Ctrl Pts',(0.00780077506694068,-0.0332451089994431,
0.0798922810272961));
#106142=CARTESIAN_POINT('Ctrl Pts',(0.00758420139466576,-0.0329451141710257,
0.079880098614218));
#106143=CARTESIAN_POINT('Ctrl Pts',(0.00736916061449163,-0.0326442513127503,
0.0798516375957339));
#106144=CARTESIAN_POINT('Ctrl Pts',(0.00728139558889851,-0.0325229783203384,
0.0798378523940379));
#106145=CARTESIAN_POINT('Ctrl Pts',(0.00720298866945899,-0.0324130253112079,
0.079826240113332));
#106146=CARTESIAN_POINT('Ctrl Pts',(0.00712483385690391,-0.0323031222247694,
0.0798130076460361));
#106147=CARTESIAN_POINT('Ctrl Pts',(0.00704703066388391,-0.0321934096636184,
0.0797981754745783));
#106148=CARTESIAN_POINT('Ctrl Pts',(0.00734694900603678,-0.0325229783203384,
0.0799302855707199));
#106149=CARTESIAN_POINT('Ctrl Pts',(0.00726726789730127,-0.0324130253112079,
0.0799195769424193));
#106150=CARTESIAN_POINT('Ctrl Pts',(0.00718782039549549,-0.0323031222247694,
0.0799072216322301));
#106151=CARTESIAN_POINT('Ctrl Pts',(0.00710870770876032,-0.0321934096636184,
0.0798932390574339));
#106152=CARTESIAN_POINT('Ctrl Pts',(0.00741250242317505,-0.0325229783203384,
0.080022718747402));
#106153=CARTESIAN_POINT('Ctrl Pts',(0.00733154712514356,-0.0324130253112079,
0.0800129137715066));
#106154=CARTESIAN_POINT('Ctrl Pts',(0.00725080693408707,-0.0323031222247694,
0.0800014356184241));
#106155=CARTESIAN_POINT('Ctrl Pts',(0.00717038475363674,-0.0321934096636184,
0.0799883026402895));
#106156=CARTESIAN_POINT('Ctrl Pts',(0.00747805584031332,-0.0325229783203384,
0.0801151519240841));
#106157=CARTESIAN_POINT('Ctrl Pts',(0.00739582635298584,-0.0324130253112079,
0.0801062506005939));
#106158=CARTESIAN_POINT('Ctrl Pts',(0.00731379347267864,-0.0323031222247694,
0.0800956496046182));
#106159=CARTESIAN_POINT('Ctrl Pts',(0.00723206179851315,-0.0321934096636184,
0.0800833662231452));
#106160=CARTESIAN_POINT('Origin',(0.00957876776548617,-0.0326393375177939,
0.0632048441708871));
#106161=CARTESIAN_POINT('Ctrl Pts',(0.0068863320582244,-0.0326943950436594,
0.0800210064864323));
#106162=CARTESIAN_POINT('Ctrl Pts',(0.00680541858540274,-0.0325844576448127,
0.0800039521043449));
#106163=CARTESIAN_POINT('Ctrl Pts',(0.00672485209879151,-0.0324744968375319,
0.079985223092015));
#106164=CARTESIAN_POINT('Ctrl Pts',(0.00664473549388511,-0.0323646534831895,
0.0799648448699489));
#106165=CARTESIAN_POINT('Ctrl Pts',(0.00697733526773067,-0.0326943950436594,
0.0799534820949769));
#106166=CARTESIAN_POINT('Ctrl Pts',(0.00689735240757747,-0.0325844576448127,
0.0799376819076747));
#106167=CARTESIAN_POINT('Ctrl Pts',(0.00681769066069115,-0.0324744968375319,
0.0799202264254871));
#106168=CARTESIAN_POINT('Ctrl Pts',(0.00673845178586718,-0.0323646534831895,
0.0799011394212102));
#106169=CARTESIAN_POINT('Ctrl Pts',(0.00706833847723695,-0.0326943950436594,
0.0798859577035216));
#106170=CARTESIAN_POINT('Ctrl Pts',(0.00698928622975219,-0.0325844576448127,
0.0798714117110046));
#106171=CARTESIAN_POINT('Ctrl Pts',(0.00691052922259079,-0.0324744968375319,
0.0798552297589591));
#106172=CARTESIAN_POINT('Ctrl Pts',(0.00683216807784924,-0.0323646534831895,
0.0798374339724716));
#106173=CARTESIAN_POINT('Ctrl Pts',(0.00715934168674322,-0.0326943950436594,
0.0798184333120662));
#106174=CARTESIAN_POINT('Ctrl Pts',(0.00708122005192691,-0.0325844576448127,
0.0798051415143344));
#106175=CARTESIAN_POINT('Ctrl Pts',(0.00700336778449043,-0.0324744968375319,
0.0797902330924312));
#106176=CARTESIAN_POINT('Ctrl Pts',(0.0069258843698313,-0.0323646534831895,
0.0797737285237329));
#106177=CARTESIAN_POINT('Origin',(0.0100563885920909,-0.032639557906725,
0.063260482814387));
#106178=CARTESIAN_POINT('Ctrl Pts',(0.0071933628962589,-0.0327445246961876,
0.0798256008432632));
#106179=CARTESIAN_POINT('Ctrl Pts',(0.006979304113298,-0.0324436878365474,
0.0797905095061824));
#106180=CARTESIAN_POINT('Ctrl Pts',(0.00676849667162067,-0.0321434074463187,
0.079739394077648));
#106181=CARTESIAN_POINT('Ctrl Pts',(0.00744089058457912,-0.0327445246961876,
0.0798606728194671));
#106182=CARTESIAN_POINT('Ctrl Pts',(0.00722550904042526,-0.0324436878365474,
0.0798349171416714));
#106183=CARTESIAN_POINT('Ctrl Pts',(0.00701267939537438,-0.0321434074463187,
0.0797930112150224));
#106184=CARTESIAN_POINT('Ctrl Pts',(0.00683337399614665,-0.0322357242816073,
0.0797547276191814));
#106185=CARTESIAN_POINT('Ctrl Pts',(0.00665487069054111,-0.0319819883628705,
0.0797136297917062));
#106186=CARTESIAN_POINT('Ctrl Pts',(0.00647934431636683,-0.0317295851069886,
0.0796612565780899));
#106187=CARTESIAN_POINT('Ctrl Pts',(0.00707816178894713,-0.0322357242816073,
0.0798055108496405));
#106188=CARTESIAN_POINT('Ctrl Pts',(0.00689804110331489,-0.0319819883628705,
0.079772209195888));
#106189=CARTESIAN_POINT('Ctrl Pts',(0.00672040453409841,-0.0317295851069886,
0.0797275134375627));
#106190=CARTESIAN_POINT('Origin',(0.0100380599527638,-0.0326371942645376,
0.0633540053487781));
#106191=CARTESIAN_POINT('Origin',(0.00955971053113989,-0.0326352985529813,
0.0633260903038244));
#106192=CARTESIAN_POINT('Ctrl Pts',(0.00652013033595464,-0.0321934096636183,
0.0799317212593738));
#106193=CARTESIAN_POINT('Ctrl Pts',(0.00644039589378846,-0.0320835708272304,
0.0799096056504534));
#106194=CARTESIAN_POINT('Ctrl Pts',(0.00636116538221627,-0.0319739230346346,
0.0798858527693486));
#106195=CARTESIAN_POINT('Ctrl Pts',(0.00628253783882057,-0.0318646057455576,
0.0798605007860826));
#106196=CARTESIAN_POINT('Ctrl Pts',(0.00661519400066897,-0.0321934096636183,
0.0798700441613876));
#106197=CARTESIAN_POINT('Ctrl Pts',(0.00653631013375223,-0.0320835708272304,
0.0798492395544918));
#106198=CARTESIAN_POINT('Ctrl Pts',(0.0064579025729425,-0.0319739230346346,
0.0798268145175876));
#106199=CARTESIAN_POINT('Ctrl Pts',(0.00638006943329853,-0.0318646057455576,
0.0798028054410061));
#106200=CARTESIAN_POINT('Ctrl Pts',(0.0067102576653833,-0.0321934096636183,
0.0798083670634014));
#106201=CARTESIAN_POINT('Ctrl Pts',(0.00663222437371599,-0.0320835708272304,
0.0797888734585301));
#106202=CARTESIAN_POINT('Ctrl Pts',(0.00655463976366873,-0.0319739230346346,
0.0797677762658266));
#106203=CARTESIAN_POINT('Ctrl Pts',(0.0064776010277765,-0.0318646057455576,
0.0797451100959295));
#106204=CARTESIAN_POINT('Ctrl Pts',(0.00680532133009763,-0.0321934096636183,
0.0797466899654153));
#106205=CARTESIAN_POINT('Ctrl Pts',(0.00672813861367976,-0.0320835708272304,
0.0797285073625685));
#106206=CARTESIAN_POINT('Ctrl Pts',(0.00665137695439496,-0.0319739230346346,
0.0797087380140656));
#106207=CARTESIAN_POINT('Ctrl Pts',(0.00657513262225446,-0.0318646057455576,
0.079687414750853));
#106208=CARTESIAN_POINT('Ctrl Pts',(0.00692617143840692,-0.0320218834582356,
0.0797746356575945));
#106209=CARTESIAN_POINT('Ctrl Pts',(0.00686763257867941,-0.0319391099350632,
0.0797621714248432));
#106210=CARTESIAN_POINT('Ctrl Pts',(0.00680932381690182,-0.0318564869454893,
0.0797488006513511));
#106211=CARTESIAN_POINT('Ctrl Pts',(0.00675128671408501,-0.0317740741446465,
0.0797345370408407));
#106212=CARTESIAN_POINT('Ctrl Pts',(0.00695224709804686,-0.0320218834582356,
0.0798167888072044));
#106213=CARTESIAN_POINT('Ctrl Pts',(0.00689326952593648,-0.0319391099350632,
0.0798045959590324));
#106214=CARTESIAN_POINT('Ctrl Pts',(0.00683451807987246,-0.0318564869454893,
0.0797914895551393));
#106215=CARTESIAN_POINT('Ctrl Pts',(0.00677603466127906,-0.0317740741446465,
0.079777483136791));
#106216=CARTESIAN_POINT('Ctrl Pts',(0.0069783227576868,-0.0320218834582356,
0.0798589419568143));
#106217=CARTESIAN_POINT('Ctrl Pts',(0.00691890647319356,-0.0319391099350632,
0.0798470204932217));
#106218=CARTESIAN_POINT('Ctrl Pts',(0.0068597123428431,-0.0318564869454893,
0.0798341784589275));
#106219=CARTESIAN_POINT('Ctrl Pts',(0.00680078260847311,-0.0317740741446465,
0.0798204292327412));
#106220=CARTESIAN_POINT('Ctrl Pts',(0.00700439841732674,-0.0320218834582356,
0.0799010951064242));
#106221=CARTESIAN_POINT('Ctrl Pts',(0.00694454342045063,-0.0319391099350632,
0.079889445027411));
#106222=CARTESIAN_POINT('Ctrl Pts',(0.00688490660581373,-0.0318564869454893,
0.0798768673627157));
#106223=CARTESIAN_POINT('Ctrl Pts',(0.00682553055566716,-0.0317740741446465,
0.0798633753286915));
#107893=UNCERTAINTY_MEASURE_WITH_UNIT(LENGTH_MEASURE(1.E-5),#107911,
'DISTANCE_ACCURACY_VALUE',
'Maximum model space distance between geometric entities at asserted c
onnectivities');
#107898=UNCERTAINTY_MEASURE_WITH_UNIT(LENGTH_MEASURE(1.E-5),#107911,
'DISTANCE_ACCURACY_VALUE',
'Maximum model space distance between geometric entities at asserted c
onnectivities');
#107905=(
GEOMETRIC_REPRESENTATION_CONTEXT(3)
GLOBAL_UNCERTAINTY_ASSIGNED_CONTEXT((#107893))
GLOBAL_UNIT_ASSIGNED_CONTEXT((#107911,#107912,#107913))
REPRESENTATION_CONTEXT('','3D')
);
#107910=(
GEOMETRIC_REPRESENTATION_CONTEXT(3)
GLOBAL_UNCERTAINTY_ASSIGNED_CONTEXT((#107898))
GLOBAL_UNIT_ASSIGNED_CONTEXT((#107911,#107912,#107913))
REPRESENTATION_CONTEXT('','3D')
);
#107911=(
LENGTH_UNIT()
NAMED_UNIT(*)
SI_UNIT($,.METRE.)
);
#107912=(
NAMED_UNIT(*)
PLANE_ANGLE_UNIT()
SI_UNIT($,.RADIAN.)
);
#107913=(
NAMED_UNIT(*)
SI_UNIT($,.STERADIAN.)
SOLID_ANGLE_UNIT()
);
#107920=SHAPE_DEFINITION_REPRESENTATION(#107931,#107952);
#107931=PRODUCT_DEFINITION_SHAPE('',$,#107964);
#107952=SHAPE_REPRESENTATION('',(#45717),#107905);
#107957=PRODUCT_DEFINITION_CONTEXT('part definition',#107992,'design');
#107964=PRODUCT_DEFINITION('Tensioner','Tensioner',#107975,#107957);
#107975=PRODUCT_DEFINITION_FORMATION('',$,#108000);
#107992=APPLICATION_CONTEXT('Managed model based 3d engineering');
#107993=PRODUCT_CONTEXT('part definition',#107992,'mechanical');
#108000=PRODUCT('Tensioner','Tensioner',
'LEGAL AND USAGE DISCLAIMER: this Data/Model is provided \X2\201C\X0\A
S IS\X2\201D\X0\ for informational and representational only. It is a 
geometric approximation and is NOT engineered, certified, or guarantee
d for dimensional accuracy, exact tolerances, or production-level prec
ision. Vendor disclaims all implied warranties including fitness for a
 particular purpose. DO NOT USE FOR DIRECT PHYSICAL MANUFACTURING, AUT
OMATED PRODUCTION, OR SAFETY-CRITICAL SYSTEMS without independent engi
neering verification and resolution of any design discrepancies.',(#107993));
#108010=PRESENTATION_STYLE_ASSIGNMENT((#108017));
#108017=SURFACE_STYLE_USAGE(.BOTH.,#108024);
#108024=SURFACE_SIDE_STYLE('',(#108031));
#108031=SURFACE_STYLE_FILL_AREA(#108038);
#108038=FILL_AREA_STYLE('Opaque(89,149,218)',(#108045));
#108045=FILL_AREA_STYLE_COLOUR('Opaque(89,149,218)',#108052);
#108052=COLOUR_RGB('Opaque(89,149,218)',0.349019607843137,0.584313725490196,
0.854901960784314);
ENDSEC;
END-ISO-10303-21;
